#275344=CARTESIAN_POINT('Ctrl Pts',(-8.81886000300005,15.2,-5.49451190900001));
#275345=CARTESIAN_POINT('Ctrl Pts',(-8.81886000300005,11.6,-5.49451190900001));
#275346=CARTESIAN_POINT('Ctrl Pts',(-8.81792317400006,15.2,-5.49405261600001));
#275347=CARTESIAN_POINT('Ctrl Pts',(-8.81792317400006,11.6,-5.49405261600001));
#275348=CARTESIAN_POINT('Ctrl Pts',(-8.81699508900006,15.2,-5.49359646700001));
#275349=CARTESIAN_POINT('Ctrl Pts',(-8.81699508900006,11.6,-5.49359646700001));
#275350=CARTESIAN_POINT('Ctrl Pts',(-8.81607576700006,15.2,-5.49314348900001));
#275351=CARTESIAN_POINT('Ctrl Pts',(-8.81607576700006,11.6,-5.49314348900001));
#275352=CARTESIAN_POINT('Ctrl Pts',(-8.81516521900006,15.2,-5.49269371000001));
#275353=CARTESIAN_POINT('Ctrl Pts',(-8.81516521900006,11.6,-5.49269371000001));
#275354=CARTESIAN_POINT('Ctrl Pts',(-8.81426346300006,15.2,-5.49224715500001));
#275355=CARTESIAN_POINT('Ctrl Pts',(-8.81426346300006,11.6,-5.49224715500001));
#275356=CARTESIAN_POINT('Ctrl Pts',(-8.81337051400006,15.2,-5.49180385500001));
#275357=CARTESIAN_POINT('Ctrl Pts',(-8.81337051400006,11.6,-5.49180385500001));
#275358=CARTESIAN_POINT('Ctrl Pts',(-8.81248638700006,15.2,-5.49136383300001));
#275359=CARTESIAN_POINT('Ctrl Pts',(-8.81248638700006,11.6,-5.49136383300001));
#275360=CARTESIAN_POINT('Ctrl Pts',(-8.81161109900006,15.2,-5.49092711900002));
#275361=CARTESIAN_POINT('Ctrl Pts',(-8.81161109900006,11.6,-5.49092711900002));
#275362=CARTESIAN_POINT('Ctrl Pts',(-8.81074466500005,15.2,-5.49049374100001));
#275363=CARTESIAN_POINT('Ctrl Pts',(-8.81074466500005,11.6,-5.49049374100001));
#275364=CARTESIAN_POINT('Ctrl Pts',(-8.80988709900006,15.2,-5.49006372600001));
#275365=CARTESIAN_POINT('Ctrl Pts',(-8.80988709900006,11.6,-5.49006372600001));
#275366=CARTESIAN_POINT('Ctrl Pts',(-8.80903841900006,15.2,-5.48963710300002));
#275367=CARTESIAN_POINT('Ctrl Pts',(-8.80903841900006,11.6,-5.48963710300002));
#275368=CARTESIAN_POINT('Ctrl Pts',(-8.80819864000006,15.2,-5.48921389900002));
#275369=CARTESIAN_POINT('Ctrl Pts',(-8.80819864000006,11.6,-5.48921389900002));
#275370=CARTESIAN_POINT('Ctrl Pts',(-8.80736777900006,15.2,-5.48879414400002));
#275371=CARTESIAN_POINT('Ctrl Pts',(-8.80736777900006,11.6,-5.48879414400002));
#275372=CARTESIAN_POINT('Ctrl Pts',(-8.80655058300006,15.2,-5.48838026300002));
#275373=CARTESIAN_POINT('Ctrl Pts',(-8.80655058300006,11.6,-5.48838026300002));
#275374=CARTESIAN_POINT('Ctrl Pts',(-8.80590483100006,15.2,-5.48805240200001));
#275375=CARTESIAN_POINT('Ctrl Pts',(-8.80590483100006,11.6,-5.48805240200001));
#275376=CARTESIAN_POINT('Ctrl Pts',(-8.80542564400006,15.2,-5.48780866000001));
#275377=CARTESIAN_POINT('Ctrl Pts',(-8.80542564400006,11.6,-5.48780866000001));
#275378=CARTESIAN_POINT('Ctrl Pts',(-8.80510947800006,15.2,-5.48764764400001));
#275379=CARTESIAN_POINT('Ctrl Pts',(-8.80510947800006,11.6,-5.48764764400001));
#275380=CARTESIAN_POINT('Ctrl Pts',(-8.80495412800006,15.2,-5.48756848000002));
#275381=CARTESIAN_POINT('Ctrl Pts',(-8.80495412800006,11.6,-5.48756848000002));
#275382=CARTESIAN_POINT('',(-8.80495412746579,12.2,-5.48756847941587));
#275383=CARTESIAN_POINT('',(-8.80495412746579,15.2,-5.48756847941587));
#275384=CARTESIAN_POINT('',(-8.80495412700006,12.2,-5.48756847900002));
#275385=CARTESIAN_POINT('Ctrl Pts',(-9.95917514600006,12.2,-5.75020264100001));
#275386=CARTESIAN_POINT('Ctrl Pts',(-9.95409037794778,12.2,-5.74984643423629));
#275387=CARTESIAN_POINT('Ctrl Pts',(-9.94901787496109,12.2,-5.74948339722987));
#275388=CARTESIAN_POINT('Ctrl Pts',(-9.94395764896434,12.2,-5.74911352693123));
#275389=CARTESIAN_POINT('Ctrl Pts',(-9.9401624798115,12.2,-5.74883612423245));
#275390=CARTESIAN_POINT('Ctrl Pts',(-9.93637421526921,12.2,-5.74855488063251));
#275391=CARTESIAN_POINT('Ctrl Pts',(-9.93259287576015,12.2,-5.74826981171152));
#275392=CARTESIAN_POINT('Ctrl Pts',(-9.92881153625109,12.2,-5.74798474279053));
#275393=CARTESIAN_POINT('Ctrl Pts',(-9.92503712276863,12.2,-5.7476958515911));
#275394=CARTESIAN_POINT('Ctrl Pts',(-9.92126966961447,12.2,-5.74740316876808));
#275395=CARTESIAN_POINT('Ctrl Pts',(-9.91750221646032,12.2,-5.74711048594505));
#275396=CARTESIAN_POINT('Ctrl Pts',(-9.91374172529696,12.2,-5.74681401298914));
#275397=CARTESIAN_POINT('Ctrl Pts',(-9.909988229975,12.2,-5.74651378250004));
#275398=CARTESIAN_POINT('Ctrl Pts',(-9.90623473465304,12.2,-5.74621355201095));
#275399=CARTESIAN_POINT('Ctrl Pts',(-9.90248823458913,12.2,-5.74590956273868));
#275400=CARTESIAN_POINT('Ctrl Pts',(-9.89874875768272,12.2,-5.74560183979185));
#275401=CARTESIAN_POINT('Ctrl Pts',(-9.89500928077632,12.2,-5.74529411684502));
#275402=CARTESIAN_POINT('Ctrl Pts',(-9.89127682625575,12.2,-5.74498266149818));
#275403=CARTESIAN_POINT('Ctrl Pts',(-9.88755142274585,12.2,-5.74466749807765));
#275404=CARTESIAN_POINT('Ctrl Pts',(-9.88382601923595,12.2,-5.74435233465712));
#275405=CARTESIAN_POINT('Ctrl Pts',(-9.88010766652519,12.2,-5.74403346444147));
#275406=CARTESIAN_POINT('Ctrl Pts',(-9.87639639528407,12.2,-5.74371091607869));
#275407=CARTESIAN_POINT('Ctrl Pts',(-9.87268512336873,12.2,-5.74338836765731));
#275408=CARTESIAN_POINT('Ctrl Pts',(-9.86898093399704,12.2,-5.7430621426099));
#275409=CARTESIAN_POINT('Ctrl Pts',(-9.86528385746071,12.2,-5.74273226768646));
#275410=CARTESIAN_POINT('Ctrl Pts',(-9.86158678159601,12.2,-5.74240239282295));
#275411=CARTESIAN_POINT('Ctrl Pts',(-9.85789681776428,12.2,-5.74206886966797));
#275412=CARTESIAN_POINT('Ctrl Pts',(-9.85421399685703,12.2,-5.7417317256799));
#275413=CARTESIAN_POINT('Ctrl Pts',(-9.85053117594978,12.2,-5.74139458169183));
#275414=CARTESIAN_POINT('Ctrl Pts',(-9.84685549666336,12.2,-5.74105381605546));
#275415=CARTESIAN_POINT('Ctrl Pts',(-9.84318698982168,12.2,-5.74070945948306));
#275416=CARTESIAN_POINT('Ctrl Pts',(-9.83829564758826,12.2,-5.74025031740737));
#275417=CARTESIAN_POINT('Ctrl Pts',(-9.83341705508244,12.2,-5.73978478939629));
#275418=CARTESIAN_POINT('Ctrl Pts',(-9.82855128681223,12.2,-5.73931294360218));
#275419=CARTESIAN_POINT('Ctrl Pts',(-9.82490195978086,12.2,-5.73895905917623));
#275420=CARTESIAN_POINT('Ctrl Pts',(-9.82125984466824,12.2,-5.73860162195762));
#275421=CARTESIAN_POINT('Ctrl Pts',(-9.81762497368261,12.2,-5.73824066144635));
#275422=CARTESIAN_POINT('Ctrl Pts',(-9.81399010335732,12.2,-5.73787970100065));
#275423=CARTESIAN_POINT('Ctrl Pts',(-9.81036247660667,12.2,-5.73751521608014));
#275424=CARTESIAN_POINT('Ctrl Pts',(-9.80674212286384,12.2,-5.73714723713487));
#275425=CARTESIAN_POINT('Ctrl Pts',(-9.80312176912101,12.2,-5.73677925818961));
#275426=CARTESIAN_POINT('Ctrl Pts',(-9.79950868946539,12.2,-5.73640778523779));
#275427=CARTESIAN_POINT('Ctrl Pts',(-9.79590291370507,12.2,-5.73603284729136));
#275428=CARTESIAN_POINT('Ctrl Pts',(-9.79229713794475,12.2,-5.73565790934494));
#275429=CARTESIAN_POINT('Ctrl Pts',(-9.7886986668058,12.2,-5.7352795069549));
#275430=CARTESIAN_POINT('Ctrl Pts',(-9.78510753050327,12.2,-5.73489767050872));
#275431=CARTESIAN_POINT('Ctrl Pts',(-9.78151639420074,12.2,-5.73451583406254));
#275432=CARTESIAN_POINT('Ctrl Pts',(-9.77793259291067,12.2,-5.7341305624446));
#275433=CARTESIAN_POINT('Ctrl Pts',(-9.77435615712329,12.2,-5.73374188700068));
#275434=CARTESIAN_POINT('Ctrl Pts',(-9.76958757564029,12.2,-5.73322365302838));
#275435=CARTESIAN_POINT('Ctrl Pts',(-9.76483208952837,12.2,-5.73269936735814));
#275436=CARTESIAN_POINT('Ctrl Pts',(-9.76008977010411,12.2,-5.73216910143996));
#275437=CARTESIAN_POINT('Ctrl Pts',(-9.75653303085899,12.2,-5.73177140203746));
#275438=CARTESIAN_POINT('Ctrl Pts',(-9.75298369860466,12.2,-5.73137033946868));
#275439=CARTESIAN_POINT('Ctrl Pts',(-9.74944180473333,12.2,-5.73096594406671));
#275440=CARTESIAN_POINT('Ctrl Pts',(-9.745899910862,12.2,-5.73056154866473));
#275441=CARTESIAN_POINT('Ctrl Pts',(-9.74236545397374,12.2,-5.73015382064624));
#275442=CARTESIAN_POINT('Ctrl Pts',(-9.73883846614291,12.2,-5.72974279078645));
#275443=CARTESIAN_POINT('Ctrl Pts',(-9.73531147831207,12.2,-5.72933176092667));
#275444=CARTESIAN_POINT('Ctrl Pts',(-9.73179195946162,12.2,-5.72891742980278));
#275445=CARTESIAN_POINT('Ctrl Pts',(-9.72827994045456,12.2,-5.72849982783914));
#275446=CARTESIAN_POINT('Ctrl Pts',(-9.72476792144751,12.2,-5.72808222587549));
#275447=CARTESIAN_POINT('Ctrl Pts',(-9.72126340215299,12.2,-5.72766135264331));
#275448=CARTESIAN_POINT('Ctrl Pts',(-9.71776641477902,12.2,-5.72723724211749));
#275449=CARTESIAN_POINT('Ctrl Pts',(-9.71426942676977,12.2,-5.72681313151463));
#275450=CARTESIAN_POINT('Ctrl Pts',(-9.71077996901264,12.2,-5.72638578120253));
#275451=CARTESIAN_POINT('Ctrl Pts',(-9.70729807450762,12.2,-5.72595522418117));
#275452=CARTESIAN_POINT('Ctrl Pts',(-9.70381618063515,12.2,-5.72552466723804));
#275453=CARTESIAN_POINT('Ctrl Pts',(-9.70034184847897,12.2,-5.72509090265343));
#275454=CARTESIAN_POINT('Ctrl Pts',(-9.69687511114725,12.2,-5.72465396371069));
#275455=CARTESIAN_POINT('Ctrl Pts',(-9.69340837381553,12.2,-5.72421702476795));
#275456=CARTESIAN_POINT('Ctrl Pts',(-9.68994923005378,12.2,-5.72377691043556));
#275457=CARTESIAN_POINT('Ctrl Pts',(-9.68649771220521,12.2,-5.72333365403297));
#275458=CARTESIAN_POINT('Ctrl Pts',(-9.68304619435663,12.2,-5.72289039763038));
#275459=CARTESIAN_POINT('Ctrl Pts',(-9.67960230117726,12.2,-5.72244399855281));
#275460=CARTESIAN_POINT('Ctrl Pts',(-9.67616606624479,12.2,-5.72199448873378));
#275461=CARTESIAN_POINT('Ctrl Pts',(-9.67272983131232,12.2,-5.72154497891475));
#275462=CARTESIAN_POINT('Ctrl Pts',(-9.66930125221604,12.2,-5.7210923596995));
#275463=CARTESIAN_POINT('Ctrl Pts',(-9.66588036288134,12.2,-5.72063666284132));
#275464=CARTESIAN_POINT('Ctrl Pts',(-9.66245947354664,12.2,-5.72018096598314));
#275465=CARTESIAN_POINT('Ctrl Pts',(-9.65904627296974,12.2,-5.71972219145018));
#275466=CARTESIAN_POINT('Ctrl Pts',(-9.6556407927174,12.2,-5.71926037305071));
#275467=CARTESIAN_POINT('Ctrl Pts',(-9.65223531184641,12.2,-5.71879855456734));
#275468=CARTESIAN_POINT('Ctrl Pts',(-9.64883755221928,12.2,-5.71833369164978));
#275469=CARTESIAN_POINT('Ctrl Pts',(-9.64544754526932,12.2,-5.71786581770637));
#275470=CARTESIAN_POINT('Ctrl Pts',(-9.64205753893523,12.2,-5.71739794384796));
#275471=CARTESIAN_POINT('Ctrl Pts',(-9.63867528399229,12.2,-5.71692705929846));
#275472=CARTESIAN_POINT('Ctrl Pts',(-9.63530081407221,12.2,-5.71645319787499));
#275473=CARTESIAN_POINT('Ctrl Pts',(-9.63192634415214,12.2,-5.71597933645153));
#275474=CARTESIAN_POINT('Ctrl Pts',(-9.62855965989462,12.2,-5.71550249684718));
#275475=CARTESIAN_POINT('Ctrl Pts',(-9.62520079160068,12.2,-5.71502271444769));
#275476=CARTESIAN_POINT('Ctrl Pts',(-9.62184192330675,12.2,-5.7145429320482));
#275477=CARTESIAN_POINT('Ctrl Pts',(-9.61849087136186,12.2,-5.71406020668239));
#275478=CARTESIAN_POINT('Ctrl Pts',(-9.615147669025,12.2,-5.71357457178337));
#275479=CARTESIAN_POINT('Ctrl Pts',(-9.61180446668813,12.2,-5.71308893688435));
#275480=CARTESIAN_POINT('Ctrl Pts',(-9.60846911280929,12.2,-5.71260039226878));
#275481=CARTESIAN_POINT('Ctrl Pts',(-9.60514164009616,12.2,-5.71210897337022));
#275482=CARTESIAN_POINT('Ctrl Pts',(-9.60181416738304,12.2,-5.71161755447166));
#275483=CARTESIAN_POINT('Ctrl Pts',(-9.59849457728684,12.2,-5.71112326023597));
#275484=CARTESIAN_POINT('Ctrl Pts',(-9.59518289940747,12.2,-5.71062612639619));
#275485=CARTESIAN_POINT('Ctrl Pts',(-9.5918712215281,12.2,-5.71012899255641));
#275486=CARTESIAN_POINT('Ctrl Pts',(-9.5885674572665,12.2,-5.70962901887432));
#275487=CARTESIAN_POINT('Ctrl Pts',(-9.58527164042683,12.2,-5.70912623960131));
#275488=CARTESIAN_POINT('Ctrl Pts',(-9.58087721757477,12.2,-5.70845586717639));
#275489=CARTESIAN_POINT('Ctrl Pts',(-9.57649691992405,12.2,-5.70778050829822));
#275490=CARTESIAN_POINT('Ctrl Pts',(-9.57213082774167,12.2,-5.70710024648337));
#275491=CARTESIAN_POINT('Ctrl Pts',(-9.56776473555929,12.2,-5.70641998466852));
#275492=CARTESIAN_POINT('Ctrl Pts',(-9.56341284680075,12.2,-5.70573481985865));
#275493=CARTESIAN_POINT('Ctrl Pts',(-9.55907524006581,12.2,-5.70504483615388));
#275494=CARTESIAN_POINT('Ctrl Pts',(-9.55256883055439,12.2,-5.70400986069076));
#275495=CARTESIAN_POINT('Ctrl Pts',(-9.54609455572192,12.2,-5.70296404560449));
#275496=CARTESIAN_POINT('Ctrl Pts',(-9.53965267920738,12.2,-5.70190767697575));
#275497=CARTESIAN_POINT('Ctrl Pts',(-9.5353580950594,12.2,-5.70120343125523));
#275498=CARTESIAN_POINT('Ctrl Pts',(-9.53107790966964,12.2,-5.70049449661066));
#275499=CARTESIAN_POINT('Ctrl Pts',(-9.52681220340578,12.2,-5.69978095839169));
#275500=CARTESIAN_POINT('Ctrl Pts',(-9.52254649656072,12.2,-5.6990674200755));
#275501=CARTESIAN_POINT('Ctrl Pts',(-9.51829526704999,12.2,-5.69834928007278));
#275502=CARTESIAN_POINT('Ctrl Pts',(-9.51405859552212,12.2,-5.69762662497454));
#275503=CARTESIAN_POINT('Ctrl Pts',(-9.5098219245715,12.2,-5.69690396997476));
#275504=CARTESIAN_POINT('Ctrl Pts',(-9.50559980981213,12.2,-5.69617680117049));
#275505=CARTESIAN_POINT('Ctrl Pts',(-9.50139233115459,12.2,-5.69544520611965));
#275506=CARTESIAN_POINT('Ctrl Pts',(-9.4971848519238,12.2,-5.69471361096912));
#275507=CARTESIAN_POINT('Ctrl Pts',(-9.49299201074995,12.2,-5.69397758987372));
#275508=CARTESIAN_POINT('Ctrl Pts',(-9.48881388596666,12.2,-5.69323723350003));
#275509=CARTESIAN_POINT('Ctrl Pts',(-9.48463576118336,12.2,-5.69249687712634));
#275510=CARTESIAN_POINT('Ctrl Pts',(-9.48047235300741,12.2,-5.69175218570216));
#275511=CARTESIAN_POINT('Ctrl Pts',(-9.47632374033838,12.2,-5.69100324866091));
#275512=CARTESIAN_POINT('Ctrl Pts',(-9.47217512823461,12.2,-5.6902543117217));
#275513=CARTESIAN_POINT('Ctrl Pts',(-9.46804131249317,12.2,-5.68950113035317));
#275514=CARTESIAN_POINT('Ctrl Pts',(-9.46392237497781,12.2,-5.68874379730055));
#275515=CARTESIAN_POINT('Ctrl Pts',(-9.45980343690124,12.2,-5.68798646414473));
#275516=CARTESIAN_POINT('Ctrl Pts',(-9.45569937597219,12.2,-5.68722497653366));
#275517=CARTESIAN_POINT('Ctrl Pts',(-9.45161027380643,12.2,-5.6864594301582));
#275518=CARTESIAN_POINT('Ctrl Pts',(-9.44752117219781,12.2,-5.68569388388704));
#275519=CARTESIAN_POINT('Ctrl Pts',(-9.44344702710667,12.2,-5.68492427853029));
#275520=CARTESIAN_POINT('Ctrl Pts',(-9.43938792354864,12.2,-5.68415070753823));
#275521=CARTESIAN_POINT('Ctrl Pts',(-9.43329926793507,12.2,-5.68299035099745));
#275522=CARTESIAN_POINT('Ctrl Pts',(-9.42724444977319,12.2,-5.68182107141003));
#275523=CARTESIAN_POINT('Ctrl Pts',(-9.42122374915626,12.2,-5.68064319187008));
#275524=CARTESIAN_POINT('Ctrl Pts',(-9.41720994838038,12.2,-5.67985793877212));
#275525=CARTESIAN_POINT('Ctrl Pts',(-9.41321130928653,12.2,-5.67906886372935));
#275526=CARTESIAN_POINT('Ctrl Pts',(-9.40922791645832,12.2,-5.6782760627417));
#275527=CARTESIAN_POINT('Ctrl Pts',(-9.40524452363011,12.2,-5.67748326175405));
#275528=CARTESIAN_POINT('Ctrl Pts',(-9.4012763745148,12.2,-5.67668673501318));
#275529=CARTESIAN_POINT('Ctrl Pts',(-9.39732355457872,12.2,-5.67588658130254));
#275530=CARTESIAN_POINT('Ctrl Pts',(-9.39337073518123,12.2,-5.67508642770091));
#275531=CARTESIAN_POINT('Ctrl Pts',(-9.38943324447615,12.2,-5.67428264574698));
#275532=CARTESIAN_POINT('Ctrl Pts',(-9.38551116429577,12.2,-5.67347533675766));
#275533=CARTESIAN_POINT('Ctrl Pts',(-9.38158908358101,12.2,-5.67266802765834));
#275534=CARTESIAN_POINT('Ctrl Pts',(-9.37768241456836,12.2,-5.67185718898666));
#275535=CARTESIAN_POINT('Ctrl Pts',(-9.37379124038544,12.2,-5.67104292262352));
#275536=CARTESIAN_POINT('Ctrl Pts',(-9.36892727292189,12.2,-5.67002508972507));
#275537=CARTESIAN_POINT('Ctrl Pts',(-9.36408751697371,12.2,-5.66900190092705));
#275538=CARTESIAN_POINT('Ctrl Pts',(-9.35927213787848,12.2,-5.66797355314885));
#275539=CARTESIAN_POINT('Ctrl Pts',(-9.35541983491722,12.2,-5.66715087499355));
#275540=CARTESIAN_POINT('Ctrl Pts',(-9.35158313178172,12.2,-5.66632489584701));
#275541=CARTESIAN_POINT('Ctrl Pts',(-9.34776211437084,12.2,-5.66549571885945));
#275542=CARTESIAN_POINT('Ctrl Pts',(-9.34394109643936,12.2,-5.66466654175891));
#275543=CARTESIAN_POINT('Ctrl Pts',(-9.34013576407524,12.2,-5.66383416589132));
#275544=CARTESIAN_POINT('Ctrl Pts',(-9.33634620195853,12.2,-5.66299869563711));
#275545=CARTESIAN_POINT('Ctrl Pts',(-9.33255664035815,12.2,-5.66216322549674));
#275546=CARTESIAN_POINT('Ctrl Pts',(-9.32878285161785,12.2,-5.66132466031647));
#275547=CARTESIAN_POINT('Ctrl Pts',(-9.32502491759068,12.2,-5.66048310805213));
#275548=CARTESIAN_POINT('Ctrl Pts',(-9.3212669830515,12.2,-5.65964155567312));
#275549=CARTESIAN_POINT('Ctrl Pts',(-9.31752490530313,12.2,-5.65879701334654));
#275550=CARTESIAN_POINT('Ctrl Pts',(-9.3137987712122,12.2,-5.65794958968906));
#275551=CARTESIAN_POINT('Ctrl Pts',(-9.31007263762896,12.2,-5.65710216614704));
#275552=CARTESIAN_POINT('Ctrl Pts',(-9.30636244611732,12.2,-5.65625185991588));
#275553=CARTESIAN_POINT('Ctrl Pts',(-9.30266828451113,12.2,-5.65539878033213));
#275554=CARTESIAN_POINT('Ctrl Pts',(-9.29897412240161,12.2,-5.65454570063215));
#275555=CARTESIAN_POINT('Ctrl Pts',(-9.2952959901743,12.2,-5.65368984571845));
#275556=CARTESIAN_POINT('Ctrl Pts',(-9.29163397547577,12.2,-5.65283132617148));
#275557=CARTESIAN_POINT('Ctrl Pts',(-9.2879719612762,12.2,-5.65197280674148));
#275558=CARTESIAN_POINT('Ctrl Pts',(-9.28432606282339,12.2,-5.65111162334815));
#275559=CARTESIAN_POINT('Ctrl Pts',(-9.28069637061846,12.2,-5.65024788464124));
#275560=CARTESIAN_POINT('Ctrl Pts',(-9.27706667791898,12.2,-5.64938414581665));
#275561=CARTESIAN_POINT('Ctrl Pts',(-9.273453189371,12.2,-5.64851785205074));
#275562=CARTESIAN_POINT('Ctrl Pts',(-9.26985599471421,12.2,-5.64764911699943));
#275563=CARTESIAN_POINT('Ctrl Pts',(-9.26625880054753,12.2,-5.64678038206649));
#275564=CARTESIAN_POINT('Ctrl Pts',(-9.26267789834029,12.2,-5.64590920418508));
#275565=CARTESIAN_POINT('Ctrl Pts',(-9.25911337957447,12.2,-5.64503569686784));
#275566=CARTESIAN_POINT('Ctrl Pts',(-9.25554886032297,12.2,-5.64416218943158));
#275567=CARTESIAN_POINT('Ctrl Pts',(-9.25200072389246,12.2,-5.64328635198677));
#275568=CARTESIAN_POINT('Ctrl Pts',(-9.24846905803332,12.2,-5.64240830105002));
#275569=CARTESIAN_POINT('Ctrl Pts',(-9.24493739217417,12.2,-5.64153025011328));
#275570=CARTESIAN_POINT('Ctrl Pts',(-9.24142219814474,12.2,-5.64064998448184));
#275571=CARTESIAN_POINT('Ctrl Pts',(-9.23792356617797,12.2,-5.63976762032242));
#275572=CARTESIAN_POINT('Ctrl Pts',(-9.23442493468789,12.2,-5.63888525628323));
#275573=CARTESIAN_POINT('Ctrl Pts',(-9.23094286375706,12.2,-5.6380007941294));
#275574=CARTESIAN_POINT('Ctrl Pts',(-9.22747744680235,12.2,-5.63711435080896));
#275575=CARTESIAN_POINT('Ctrl Pts',(-9.22401202937549,12.2,-5.63622790736773));
#275576=CARTESIAN_POINT('Ctrl Pts',(-9.22056326270751,12.2,-5.63533948328094));
#275577=CARTESIAN_POINT('Ctrl Pts',(-9.21713124018886,12.2,-5.63444919712112));
#275578=CARTESIAN_POINT('Ctrl Pts',(-9.21369921813782,12.2,-5.63355891108261));
#275579=CARTESIAN_POINT('Ctrl Pts',(-9.2102839409179,12.2,-5.63266676329989));
#275580=CARTESIAN_POINT('Ctrl Pts',(-9.20688549752797,12.2,-5.63177287403975));
#275581=CARTESIAN_POINT('Ctrl Pts',(-9.20348705367501,12.2,-5.63087898465782));
#275582=CARTESIAN_POINT('Ctrl Pts',(-9.20010544519518,12.2,-5.62998335421368));
#275583=CARTESIAN_POINT('Ctrl Pts',(-9.19674076451184,12.2,-5.62908610411981));
#275584=CARTESIAN_POINT('Ctrl Pts',(-9.19337608428694,12.2,-5.6281888541482));
#275585=CARTESIAN_POINT('Ctrl Pts',(-9.19002833246516,12.2,-5.62728998641658));
#275586=CARTESIAN_POINT('Ctrl Pts',(-9.1866976010141,12.2,-5.62638962182361));
#275587=CARTESIAN_POINT('Ctrl Pts',(-9.18336686910923,12.2,-5.62548925710797));
#275588=CARTESIAN_POINT('Ctrl Pts',(-9.18005315646755,12.2,-5.62458739670882));
#275589=CARTESIAN_POINT('Ctrl Pts',(-9.17675656045565,12.2,-5.6236841666595));
#275590=CARTESIAN_POINT('Ctrl Pts',(-9.17345996489292,12.2,-5.62278093673325));
#275591=CARTESIAN_POINT('Ctrl Pts',(-9.17018048252125,12.2,-5.62187633587755));
#275592=CARTESIAN_POINT('Ctrl Pts',(-9.16691820895679,12.2,-5.62097049240645));
#275593=CARTESIAN_POINT('Ctrl Pts',(-9.16365593494787,12.2,-5.62006464881194));
#275594=CARTESIAN_POINT('Ctrl Pts',(-9.16041086977495,12.2,-5.61915756073922));
#275595=CARTESIAN_POINT('Ctrl Pts',(-9.15718310854462,12.2,-5.6182493586341));
#275596=CARTESIAN_POINT('Ctrl Pts',(-9.15395534775407,12.2,-5.61734115665272));
#275597=CARTESIAN_POINT('Ctrl Pts',(-9.15074489128502,12.2,-5.61643183876044));
#275598=CARTESIAN_POINT('Ctrl Pts',(-9.14755183332206,12.2,-5.61552153689052));
#275599=CARTESIAN_POINT('Ctrl Pts',(-9.14356051054207,12.2,-5.61438365946009));
#275600=CARTESIAN_POINT('Ctrl Pts',(-9.13959637408344,12.2,-5.61324424281155));
#275601=CARTESIAN_POINT('Ctrl Pts',(-9.13565961339875,12.2,-5.61210354615743));
#275602=CARTESIAN_POINT('Ctrl Pts',(-9.13172285271406,12.2,-5.6109628495033));
#275603=CARTESIAN_POINT('Ctrl Pts',(-9.12781346627214,12.2,-5.6098208716136));
#275604=CARTESIAN_POINT('Ctrl Pts',(-9.12393164502069,12.2,-5.60867787584976));
#275605=CARTESIAN_POINT('Ctrl Pts',(-9.12004982376924,12.2,-5.60753488008593));
#275606=CARTESIAN_POINT('Ctrl Pts',(-9.11619556795187,12.2,-5.60639086647484));
#275607=CARTESIAN_POINT('Ctrl Pts',(-9.11236906774208,12.2,-5.60524610084988));
#275608=CARTESIAN_POINT('Ctrl Pts',(-9.1085425675323,12.2,-5.60410133522491));
#275609=CARTESIAN_POINT('Ctrl Pts',(-9.10474382473154,12.2,-5.60295581854716));
#275610=CARTESIAN_POINT('Ctrl Pts',(-9.10097303348009,12.2,-5.60180982132496));
#275611=CARTESIAN_POINT('Ctrl Pts',(-9.09720224222865,12.2,-5.60066382410277));
#275612=CARTESIAN_POINT('Ctrl Pts',(-9.09345939989119,12.2,-5.59951734792806));
#275613=CARTESIAN_POINT('Ctrl Pts',(-9.08974470452701,12.2,-5.59837066653397));
#275614=CARTESIAN_POINT('Ctrl Pts',(-9.08603000916283,12.2,-5.59722398513988));
#275615=CARTESIAN_POINT('Ctrl Pts',(-9.08234346030553,12.2,-5.59607709923335));
#275616=CARTESIAN_POINT('Ctrl Pts',(-9.07868525495831,12.2,-5.59493029173335));
#275617=CARTESIAN_POINT('Ctrl Pts',(-9.07502704961108,12.2,-5.59378348423334));
#275618=CARTESIAN_POINT('Ctrl Pts',(-9.07139718858651,12.2,-5.59263675178237));
#275619=CARTESIAN_POINT('Ctrl Pts',(-9.06779587072302,12.2,-5.59149038274939));
#275620=CARTESIAN_POINT('Ctrl Pts',(-9.06419455285953,12.2,-5.59034401371641));
#275621=CARTESIAN_POINT('Ctrl Pts',(-9.06062177702242,12.2,-5.58919800558618));
#275622=CARTESIAN_POINT('Ctrl Pts',(-9.05707774751005,12.2,-5.58805265239178));
#275623=CARTESIAN_POINT('Ctrl Pts',(-9.05353371799768,12.2,-5.58690729919738));
#275624=CARTESIAN_POINT('Ctrl Pts',(-9.05001843272618,12.2,-5.58576259785294));
#275625=CARTESIAN_POINT('Ctrl Pts',(-9.04653209654715,12.2,-5.58461884570022));
#275626=CARTESIAN_POINT('Ctrl Pts',(-9.04304576036813,12.2,-5.5834750935475));
#275627=CARTESIAN_POINT('Ctrl Pts',(-9.03958837427692,12.2,-5.58233229076888));
#275628=CARTESIAN_POINT('Ctrl Pts',(-9.03616014063545,12.2,-5.58119073710083));
#275629=CARTESIAN_POINT('Ctrl Pts',(-9.03273190699398,12.2,-5.58004918343277));
#275630=CARTESIAN_POINT('Ctrl Pts',(-9.02933282980129,12.2,-5.57890888160094));
#275631=CARTESIAN_POINT('Ctrl Pts',(-9.0259631145259,12.2,-5.57777013535106));
#275632=CARTESIAN_POINT('Ctrl Pts',(-9.02259339925052,12.2,-5.57663138910119));
#275633=CARTESIAN_POINT('Ctrl Pts',(-9.01925304713674,12.2,-5.57549420050135));
#275634=CARTESIAN_POINT('Ctrl Pts',(-9.0159422678336,12.2,-5.57435888008484));
#275635=CARTESIAN_POINT('Ctrl Pts',(-9.01263148889134,12.2,-5.57322355979209));
#275636=CARTESIAN_POINT('Ctrl Pts',(-9.00935028375105,12.2,-5.57209010840261));
#275637=CARTESIAN_POINT('Ctrl Pts',(-9.0060988646586,12.2,-5.57095884262298));
#275638=CARTESIAN_POINT('Ctrl Pts',(-9.00284744521174,12.2,-5.56982757672003));
#275639=CARTESIAN_POINT('Ctrl Pts',(-8.99962581084212,12.2,-5.5686984999809));
#275640=CARTESIAN_POINT('Ctrl Pts',(-8.99643417965913,12.2,-5.56757193289736));
#275641=CARTESIAN_POINT('Ctrl Pts',(-8.99324254847613,12.2,-5.56644536581384));
#275642=CARTESIAN_POINT('Ctrl Pts',(-8.99008091774436,12.2,-5.56532130925861));
#275643=CARTESIAN_POINT('Ctrl Pts',(-8.9869495066136,12.2,-5.56420009385517));
#275644=CARTESIAN_POINT('Ctrl Pts',(-8.98319181305189,12.2,-5.56285463529771));
#275645=CARTESIAN_POINT('Ctrl Pts',(-8.97947763719697,12.2,-5.56151326617684));
#275646=CARTESIAN_POINT('Ctrl Pts',(-8.97580735783326,12.2,-5.56017657160431));
#275647=CARTESIAN_POINT('Ctrl Pts',(-8.97213707880293,12.2,-5.55883987715319));
#275648=CARTESIAN_POINT('Ctrl Pts',(-8.9685106971594,12.2,-5.55750785349889));
#275649=CARTESIAN_POINT('Ctrl Pts',(-8.96492860102335,12.2,-5.55618109929107));
#275650=CARTESIAN_POINT('Ctrl Pts',(-8.96134650488731,12.2,-5.55485434508325));
#275651=CARTESIAN_POINT('Ctrl Pts',(-8.95780869174889,12.2,-5.55353285835752));
#275652=CARTESIAN_POINT('Ctrl Pts',(-8.95431555770721,12.2,-5.55221725107173));
#275653=CARTESIAN_POINT('Ctrl Pts',(-8.95082242334824,12.2,-5.55090164366644));
#275654=CARTESIAN_POINT('Ctrl Pts',(-8.94737396721143,12.2,-5.54959191300355));
#275655=CARTESIAN_POINT('Ctrl Pts',(-8.94397058786236,12.2,-5.54828868584962));
#275656=CARTESIAN_POINT('Ctrl Pts',(-8.94056720882241,12.2,-5.54698545881408));
#275657=CARTESIAN_POINT('Ctrl Pts',(-8.93720890657228,12.2,-5.54568873347425));
#275658=CARTESIAN_POINT('Ctrl Pts',(-8.93389608761129,12.2,-5.54439915043808));
#275659=CARTESIAN_POINT('Ctrl Pts',(-8.9305832686503,12.2,-5.54310956740191));
#275660=CARTESIAN_POINT('Ctrl Pts',(-8.92731593080235,12.2,-5.54182712500687));
#275661=CARTESIAN_POINT('Ctrl Pts',(-8.92409449066741,12.2,-5.54055248005283));
#275662=CARTESIAN_POINT('Ctrl Pts',(-8.92087305053247,12.2,-5.53927783509881));
#275663=CARTESIAN_POINT('Ctrl Pts',(-8.9176975042139,12.2,-5.5380109859087));
#275664=CARTESIAN_POINT('Ctrl Pts',(-8.91456827232441,12.2,-5.5367526051205));
#275665=CARTESIAN_POINT('Ctrl Pts',(-8.91143904015069,12.2,-5.53549422421799));
#275666=CARTESIAN_POINT('Ctrl Pts',(-8.90835612418982,12.2,-5.53424431125798));
#275667=CARTESIAN_POINT('Ctrl Pts',(-8.90531994710969,12.2,-5.53300355444075));
#275668=CARTESIAN_POINT('Ctrl Pts',(-8.90228377030535,12.2,-5.53176279773622));
#275669=CARTESIAN_POINT('Ctrl Pts',(-8.89929433564735,12.2,-5.53053119599766));
#275670=CARTESIAN_POINT('Ctrl Pts',(-8.89635207566886,12.2,-5.52930945629162));
#275671=CARTESIAN_POINT('Ctrl Pts',(-8.89340981569037,12.2,-5.52808771658559));
#275672=CARTESIAN_POINT('Ctrl Pts',(-8.89051473087686,12.2,-5.52687583798803));
#275673=CARTESIAN_POINT('Ctrl Pts',(-8.88766726131037,12.2,-5.52567454636428));
#275674=CARTESIAN_POINT('Ctrl Pts',(-8.88481979148523,12.2,-5.5244732546314));
#275675=CARTESIAN_POINT('Ctrl Pts',(-8.88201994158144,12.2,-5.52328254665789));
#275676=CARTESIAN_POINT('Ctrl Pts',(-8.87926815660021,12.2,-5.52210316717744));
#275677=CARTESIAN_POINT('Ctrl Pts',(-8.87651637186895,12.2,-5.52092378780412));
#275678=CARTESIAN_POINT('Ctrl Pts',(-8.87381265496687,12.2,-5.51975573906379));
#275679=CARTESIAN_POINT('Ctrl Pts',(-8.87115746421785,12.2,-5.51859977976719));
#275680=CARTESIAN_POINT('Ctrl Pts',(-8.86850227346883,12.2,-5.51744382047058));
#275681=CARTESIAN_POINT('Ctrl Pts',(-8.86589560838085,12.2,-5.51629995355806));
#275682=CARTESIAN_POINT('Ctrl Pts',(-8.86333793755377,12.2,-5.51516896118161));
#275683=CARTESIAN_POINT('Ctrl Pts',(-8.86078026649437,12.2,-5.51403796870243));
#275684=CARTESIAN_POINT('Ctrl Pts',(-8.8582715898829,12.2,-5.51291984943276));
#275685=CARTESIAN_POINT('Ctrl Pts',(-8.85581238379553,12.2,-5.51181541290152));
#275686=CARTESIAN_POINT('Ctrl Pts',(-8.85335317793155,12.2,-5.51071097647061));
#275687=CARTESIAN_POINT('Ctrl Pts',(-8.85094344409755,12.2,-5.50962021750255));
#275688=CARTESIAN_POINT('Ctrl Pts',(-8.84858366851663,12.2,-5.50854396829165));
#275689=CARTESIAN_POINT('Ctrl Pts',(-8.8462238929357,12.2,-5.50746771908076));
#275690=CARTESIAN_POINT('Ctrl Pts',(-8.84391407709403,12.2,-5.50640597620805));
#275691=CARTESIAN_POINT('Ctrl Pts',(-8.84165471647699,12.2,-5.50535959410958));
#275692=CARTESIAN_POINT('Ctrl Pts',(-8.83939535565472,12.2,-5.50431321191606));
#275693=CARTESIAN_POINT('Ctrl Pts',(-8.83718645120391,12.2,-5.50328218836858));
#275694=CARTESIAN_POINT('Ctrl Pts',(-8.83502851250643,12.2,-5.50226740039771));
#275695=CARTESIAN_POINT('Ctrl Pts',(-8.83287057400498,12.2,-5.50125261251901));
#275696=CARTESIAN_POINT('Ctrl Pts',(-8.83076360063357,12.2,-5.50025405960163));
#275697=CARTESIAN_POINT('Ctrl Pts',(-8.82870811303237,12.2,-5.49927264479954));
#275698=CARTESIAN_POINT('Ctrl Pts',(-8.82665262543117,12.2,-5.49829122999746));
#275699=CARTESIAN_POINT('Ctrl Pts',(-8.82464862187126,12.2,-5.49732695060138));
#275700=CARTESIAN_POINT('Ctrl Pts',(-8.82269663660656,12.2,-5.49638073980162));
#275701=CARTESIAN_POINT('Ctrl Pts',(-8.82074465116457,12.2,-5.49543452891593));
#275702=CARTESIAN_POINT('Ctrl Pts',(-8.81884468407904,12.2,-5.49450638212414));
#275703=CARTESIAN_POINT('Ctrl Pts',(-8.81699727948194,12.2,-5.49359725965922));
#275704=CARTESIAN_POINT('Ctrl Pts',(-8.81514987505265,12.2,-5.49268813727688));
#275705=CARTESIAN_POINT('Ctrl Pts',(-8.81335503191469,12.2,-5.4917980403285));
#275706=CARTESIAN_POINT('Ctrl Pts',(-8.81161331239693,12.2,-5.49092795294431));
#275707=CARTESIAN_POINT('Ctrl Pts',(-8.80929937863631,12.2,-5.48977201219011));
#275708=CARTESIAN_POINT('Ctrl Pts',(-8.80707920106142,12.2,-5.48865138494897));
#275709=CARTESIAN_POINT('Ctrl Pts',(-8.80495412800006,12.2,-5.48756848000002));
#275710=CARTESIAN_POINT('Ctrl Pts',(-8.80495412800006,15.2,-5.48756848000002));
#275711=CARTESIAN_POINT('Ctrl Pts',(-8.80654601357685,15.2,-5.48837968070677));
#275712=CARTESIAN_POINT('Ctrl Pts',(-8.80819126582659,15.2,-5.48921205180374));
#275713=CARTESIAN_POINT('Ctrl Pts',(-8.809889320289,15.2,-5.49006457388994));
#275714=CARTESIAN_POINT('Ctrl Pts',(-8.81159556362836,15.2,-5.49092120726858));
#275715=CARTESIAN_POINT('Ctrl Pts',(-8.81335511570803,15.2,-5.49179818670865));
#275716=CARTESIAN_POINT('Ctrl Pts',(-8.81516741715041,15.2,-5.49269451613673));
#275717=CARTESIAN_POINT('Ctrl Pts',(-8.81697971842817,15.2,-5.49359084548341));
#275718=CARTESIAN_POINT('Ctrl Pts',(-8.81884476611964,15.2,-5.49450652398393));
#275719=CARTESIAN_POINT('Ctrl Pts',(-8.82076201154996,15.2,-5.49544058544998));
#275720=CARTESIAN_POINT('Ctrl Pts',(-8.82267925698027,15.2,-5.49637464691604));
#275721=CARTESIAN_POINT('Ctrl Pts',(-8.824648700705,15.2,-5.49732708982732));
#275722=CARTESIAN_POINT('Ctrl Pts',(-8.82666980631291,15.2,-5.49829697667287));
#275723=CARTESIAN_POINT('Ctrl Pts',(-8.8286909121044,15.2,-5.49926686360652));
#275724=CARTESIAN_POINT('Ctrl Pts',(-8.8307636790539,15.2,-5.50025419422024));
#275725=CARTESIAN_POINT('Ctrl Pts',(-8.83288758275648,15.2,-5.50125805810941));
#275726=CARTESIAN_POINT('Ctrl Pts',(-8.83501148626615,15.2,-5.5022619219074));
#275727=CARTESIAN_POINT('Ctrl Pts',(-8.83718652676331,15.2,-5.5032823192667));
#275728=CARTESIAN_POINT('Ctrl Pts',(-8.83941219327598,15.2,-5.50431836423379));
#275729=CARTESIAN_POINT('Ctrl Pts',(-8.84163785978865,15.2,-5.50535440920089));
#275730=CARTESIAN_POINT('Ctrl Pts',(-8.84391415062677,15.2,-5.50640610420631));
#275731=CARTESIAN_POINT('Ctrl Pts',(-8.84624056437339,15.2,-5.50747258641693));
#275732=CARTESIAN_POINT('Ctrl Pts',(-8.84856697833133,15.2,-5.50853906872442));
#275733=CARTESIAN_POINT('Ctrl Pts',(-8.85094351562051,15.2,-5.50962034055873));
#275734=CARTESIAN_POINT('Ctrl Pts',(-8.85336968650611,15.2,-5.51071556661937));
#275735=CARTESIAN_POINT('Ctrl Pts',(-8.85579585717132,15.2,-5.51181079258052));
#275736=CARTESIAN_POINT('Ctrl Pts',(-8.85827166062738,15.2,-5.51291996937641));
#275737=CARTESIAN_POINT('Ctrl Pts',(-8.86079661537112,15.2,-5.51404228958621));
#275738=CARTESIAN_POINT('Ctrl Pts',(-8.86332157011486,15.2,-5.51516460979602));
#275739=CARTESIAN_POINT('Ctrl Pts',(-8.86589567860466,15.2,-5.51630007113808));
#275740=CARTESIAN_POINT('Ctrl Pts',(-8.86851846634056,15.2,-5.51744788067916));
#275741=CARTESIAN_POINT('Ctrl Pts',(-8.87114125407647,15.2,-5.51859569022025));
#275742=CARTESIAN_POINT('Ctrl Pts',(-8.87381272327231,15.2,-5.51975585284065));
#275743=CARTESIAN_POINT('Ctrl Pts',(-8.87653241117021,15.2,-5.52092759338061));
#275744=CARTESIAN_POINT('Ctrl Pts',(-8.87925209931515,15.2,-5.52209933402701));
#275745=CARTESIAN_POINT('Ctrl Pts',(-8.88202000817308,15.2,-5.52328265684124));
#275746=CARTESIAN_POINT('Ctrl Pts',(-8.88483568141196,15.2,-5.52447681032346));
#275747=CARTESIAN_POINT('Ctrl Pts',(-8.88765135439507,15.2,-5.5256709636972));
#275748=CARTESIAN_POINT('Ctrl Pts',(-8.89051479414961,15.2,-5.52687594635476));
#275749=CARTESIAN_POINT('Ctrl Pts',(-8.89342555597366,15.2,-5.52809103098278));
#275750=CARTESIAN_POINT('Ctrl Pts',(-8.8963363177977,15.2,-5.52930611561081));
#275751=CARTESIAN_POINT('Ctrl Pts',(-8.89929439944313,15.2,-5.53053130127758));
#275752=CARTESIAN_POINT('Ctrl Pts',(-8.90229936641411,15.2,-5.53176587589877));
#275753=CARTESIAN_POINT('Ctrl Pts',(-8.90530433365805,15.2,-5.53300045063209));
#275754=CARTESIAN_POINT('Ctrl Pts',(-8.90835618651481,15.2,-5.53424441469965));
#275755=CARTESIAN_POINT('Ctrl Pts',(-8.9114544946857,15.2,-5.53549707276831));
#275756=CARTESIAN_POINT('Ctrl Pts',(-8.91455280257515,15.2,-5.53674973072317));
#275757=CARTESIAN_POINT('Ctrl Pts',(-8.91769756619174,15.2,-5.53801108558147));
#275758=CARTESIAN_POINT('Ctrl Pts',(-8.92088836400686,15.2,-5.53928045845776));
#275759=CARTESIAN_POINT('Ctrl Pts',(-8.92407916182198,15.2,-5.54054983133406));
#275760=CARTESIAN_POINT('Ctrl Pts',(-8.92731599336455,15.2,-5.54182722173214));
#275761=CARTESIAN_POINT('Ctrl Pts',(-8.93059844440887,15.2,-5.54311197160163));
#275762=CARTESIAN_POINT('Ctrl Pts',(-8.93388089575133,15.2,-5.54439672158783));
#275763=CARTESIAN_POINT('Ctrl Pts',(-8.93720896609641,15.2,-5.54568882888127));
#275764=CARTESIAN_POINT('Ctrl Pts',(-8.94058224953474,15.2,-5.54698765010066));
#275765=CARTESIAN_POINT('Ctrl Pts',(-8.94395553266667,15.2,-5.54828647120208));
#275766=CARTESIAN_POINT('Ctrl Pts',(-8.94737402688413,15.2,-5.54959200568932));
#275767=CARTESIAN_POINT('Ctrl Pts',(-8.95083733100831,15.2,-5.550903625725));
#275768=CARTESIAN_POINT('Ctrl Pts',(-8.95430063513249,15.2,-5.55221524576068));
#275769=CARTESIAN_POINT('Ctrl Pts',(-8.95780874996059,15.2,-5.55353294947097));
#275770=CARTESIAN_POINT('Ctrl Pts',(-8.96136128017309,15.2,-5.55485612365535));
#275771=CARTESIAN_POINT('Ctrl Pts',(-8.96491381070828,15.2,-5.55617929795992));
#275772=CARTESIAN_POINT('Ctrl Pts',(-8.96851075529544,15.2,-5.55750794212235));
#275773=CARTESIAN_POINT('Ctrl Pts',(-8.97215172666352,15.2,-5.55884145636203));
#275774=CARTESIAN_POINT('Ctrl Pts',(-8.97579269770089,15.2,-5.56017497048057));
#275775=CARTESIAN_POINT('Ctrl Pts',(-8.9794776951951,15.2,-5.56151335337662));
#275776=CARTESIAN_POINT('Ctrl Pts',(-8.98320633349334,15.2,-5.56285602050061));
#275777=CARTESIAN_POINT('Ctrl Pts',(-8.98693497179157,15.2,-5.56419868762461));
#275778=CARTESIAN_POINT('Ctrl Pts',(-8.99070725611604,15.2,-5.56554563715898));
#275779=CARTESIAN_POINT('Ctrl Pts',(-8.99452280230889,15.2,-5.56689629644308));
#275780=CARTESIAN_POINT('Ctrl Pts',(-8.99770242425178,15.2,-5.5680218458874));
#275781=CARTESIAN_POINT('Ctrl Pts',(-9.00091209151763,15.2,-5.56914997208176));
#275782=CARTESIAN_POINT('Ctrl Pts',(-9.00415158832164,15.2,-5.5702803484011));
#275783=CARTESIAN_POINT('Ctrl Pts',(-9.00739108512563,15.2,-5.57141072472042));
#275784=CARTESIAN_POINT('Ctrl Pts',(-9.01066041008883,15.2,-5.57254335434425));
#275785=CARTESIAN_POINT('Ctrl Pts',(-9.01395935121486,15.2,-5.57367791476606));
#275786=CARTESIAN_POINT('Ctrl Pts',(-9.01725829234089,15.2,-5.57481247518789));
#275787=CARTESIAN_POINT('Ctrl Pts',(-9.02058684908886,15.2,-5.57594896675556));
#275788=CARTESIAN_POINT('Ctrl Pts',(-9.02394481103331,15.2,-5.57708707724167));
#275789=CARTESIAN_POINT('Ctrl Pts',(-9.02730277297776,15.2,-5.57822518772779));
#275790=CARTESIAN_POINT('Ctrl Pts',(-9.03069013840847,15.2,-5.57936491817877));
#275791=CARTESIAN_POINT('Ctrl Pts',(-9.03410670120185,15.2,-5.58050595797563));
#275792=CARTESIAN_POINT('Ctrl Pts',(-9.03752326399521,15.2,-5.58164699777248));
#275793=CARTESIAN_POINT('Ctrl Pts',(-9.0409690221759,15.2,-5.58278935031363));
#275794=CARTESIAN_POINT('Ctrl Pts',(-9.04444377071907,15.2,-5.58393271079979));
#275795=CARTESIAN_POINT('Ctrl Pts',(-9.04791851926226,15.2,-5.58507607128596));
#275796=CARTESIAN_POINT('Ctrl Pts',(-9.05142225763523,15.2,-5.58622044081932));
#275797=CARTESIAN_POINT('Ctrl Pts',(-9.05495478124785,15.2,-5.58736552137491));
#275798=CARTESIAN_POINT('Ctrl Pts',(-9.05848730486047,15.2,-5.5885106019305));
#275799=CARTESIAN_POINT('Ctrl Pts',(-9.06204861416326,15.2,-5.58965639411467));
#275800=CARTESIAN_POINT('Ctrl Pts',(-9.06563850719182,15.2,-5.59080260715807));
#275801=CARTESIAN_POINT('Ctrl Pts',(-9.06922840022036,15.2,-5.59194882020148));
#275802=CARTESIAN_POINT('Ctrl Pts',(-9.07284687567467,15.2,-5.5930954523889));
#275803=CARTESIAN_POINT('Ctrl Pts',(-9.07649373526034,15.2,-5.59424221870834));
#275804=CARTESIAN_POINT('Ctrl Pts',(-9.080140594846,15.2,-5.5953889850278));
#275805=CARTESIAN_POINT('Ctrl Pts',(-9.08381583734878,15.2,-5.59653588415004));
#275806=CARTESIAN_POINT('Ctrl Pts',(-9.08751926672607,15.2,-5.59768263560834));
#275807=CARTESIAN_POINT('Ctrl Pts',(-9.0912226956997,15.2,-5.59882938694166));
#275808=CARTESIAN_POINT('Ctrl Pts',(-9.09495431111479,15.2,-5.59997599026944));
#275809=CARTESIAN_POINT('Ctrl Pts',(-9.09871391375824,15.2,-5.60112216757509));
#275810=CARTESIAN_POINT('Ctrl Pts',(-9.10247351681149,15.2,-5.60226834500568));
#275811=CARTESIAN_POINT('Ctrl Pts',(-9.10626111065876,15.2,-5.60341409837796));
#275812=CARTESIAN_POINT('Ctrl Pts',(-9.11007649947594,15.2,-5.60455915330858));
#275813=CARTESIAN_POINT('Ctrl Pts',(-9.11389188829312,15.2,-5.60570420823918));
#275814=CARTESIAN_POINT('Ctrl Pts',(-9.11773507289039,15.2,-5.6068485657226));
#275815=CARTESIAN_POINT('Ctrl Pts',(-9.12160586073537,15.2,-5.6079919580838));
#275816=CARTESIAN_POINT('Ctrl Pts',(-9.12547664858033,15.2,-5.60913535044498));
#275817=CARTESIAN_POINT('Ctrl Pts',(-9.12937503967234,15.2,-5.61027777802153));
#275818=CARTESIAN_POINT('Ctrl Pts',(-9.13330084285269,15.2,-5.61141897634254));
#275819=CARTESIAN_POINT('Ctrl Pts',(-9.13722664603305,15.2,-5.61256017466353));
#275820=CARTESIAN_POINT('Ctrl Pts',(-9.14117986225791,15.2,-5.61370014517547));
#275821=CARTESIAN_POINT('Ctrl Pts',(-9.14516030267316,15.2,-5.61483862767555));
#275822=CARTESIAN_POINT('Ctrl Pts',(-9.14914074308841,15.2,-5.61597711017563));
#275823=CARTESIAN_POINT('Ctrl Pts',(-9.15314840722661,15.2,-5.61711410606457));
#275824=CARTESIAN_POINT('Ctrl Pts',(-9.15718310854461,15.2,-5.6182493586341));
#275825=CARTESIAN_POINT('Ctrl Pts',(-9.1612178098626,15.2,-5.61938461120361));
#275826=CARTESIAN_POINT('Ctrl Pts',(-9.16527954857928,15.2,-5.62051812167203));
#275827=CARTESIAN_POINT('Ctrl Pts',(-9.16936813901443,15.2,-5.62164963994107));
#275828=CARTESIAN_POINT('Ctrl Pts',(-9.17345672944959,15.2,-5.6227811582101));
#275829=CARTESIAN_POINT('Ctrl Pts',(-9.17757216966108,15.2,-5.62391068283891));
#275830=CARTESIAN_POINT('Ctrl Pts',(-9.18171428000832,15.2,-5.62503796874169));
#275831=CARTESIAN_POINT('Ctrl Pts',(-9.18502796846671,15.2,-5.62593979751306));
#275832=CARTESIAN_POINT('Ctrl Pts',(-9.18835872356594,15.2,-5.62684019365371));
#275833=CARTESIAN_POINT('Ctrl Pts',(-9.19170645280569,15.2,-5.62773903114698));
#275834=CARTESIAN_POINT('Ctrl Pts',(-9.1950541815893,15.2,-5.62863786851779));
#275835=CARTESIAN_POINT('Ctrl Pts',(-9.19841888494494,15.2,-5.62953514950466));
#275836=CARTESIAN_POINT('Ctrl Pts',(-9.20180046973936,15.2,-5.63043074949108));
#275837=CARTESIAN_POINT('Ctrl Pts',(-9.2051820549945,15.2,-5.63132634959952));
#275838=CARTESIAN_POINT('Ctrl Pts',(-9.20858052225944,15.2,-5.63222026905579));
#275839=CARTESIAN_POINT('Ctrl Pts',(-9.21199577755839,15.2,-5.63311238660422));
#275840=CARTESIAN_POINT('Ctrl Pts',(-9.21541103239202,15.2,-5.6340045040311));
#275841=CARTESIAN_POINT('Ctrl Pts',(-9.21884307743735,15.2,-5.63489482060821));
#275842=CARTESIAN_POINT('Ctrl Pts',(-9.22229182020988,15.2,-5.63578321470237));
#275843=CARTESIAN_POINT('Ctrl Pts',(-9.2257405634523,15.2,-5.63667160891759));
#275844=CARTESIAN_POINT('Ctrl Pts',(-9.22920600346796,15.2,-5.63755808168615));
#275845=CARTESIAN_POINT('Ctrl Pts',(-9.23268805205535,15.2,-5.63844251511168));
#275846=CARTESIAN_POINT('Ctrl Pts',(-9.23617010016832,15.2,-5.63932694841672));
#275847=CARTESIAN_POINT('Ctrl Pts',(-9.23966875394013,15.2,-5.64020934176098));
#275848=CARTESIAN_POINT('Ctrl Pts',(-9.24318392476279,15.2,-5.64108957791138));
#275849=CARTESIAN_POINT('Ctrl Pts',(-9.24669909606439,15.2,-5.64196981418171));
#275850=CARTESIAN_POINT('Ctrl Pts',(-9.25023078448187,15.2,-5.64284789414069));
#275851=CARTESIAN_POINT('Ctrl Pts',(-9.25377889906521,15.2,-5.64372370285493));
#275852=CARTESIAN_POINT('Ctrl Pts',(-9.2573270131651,15.2,-5.64459951144985));
#275853=CARTESIAN_POINT('Ctrl Pts',(-9.2608915536624,15.2,-5.64547304632609));
#275854=CARTESIAN_POINT('Ctrl Pts',(-9.26447243321381,15.2,-5.6463441957986));
#275855=CARTESIAN_POINT('Ctrl Pts',(-9.26805331325311,15.2,-5.64721534538981));
#275856=CARTESIAN_POINT('Ctrl Pts',(-9.2716505298031,15.2,-5.64808410911266));
#275857=CARTESIAN_POINT('Ctrl Pts',(-9.27526399577888,15.2,-5.64895037460415));
#275858=CARTESIAN_POINT('Ctrl Pts',(-9.27887746126233,15.2,-5.64981663997761));
#275859=CARTESIAN_POINT('Ctrl Pts',(-9.28250717538693,15.2,-5.65068040619046));
#275860=CARTESIAN_POINT('Ctrl Pts',(-9.28615305142057,15.2,-5.65154156234256));
#275861=CARTESIAN_POINT('Ctrl Pts',(-9.28979892795095,15.2,-5.65240271861198));
#275862=CARTESIAN_POINT('Ctrl Pts',(-9.29346096421862,15.2,-5.65326126572231));
#275863=CARTESIAN_POINT('Ctrl Pts',(-9.29713907476917,15.2,-5.65411709321728));
#275864=CARTESIAN_POINT('Ctrl Pts',(-9.30081718481857,15.2,-5.65497292059564));
#275865=CARTESIAN_POINT('Ctrl Pts',(-9.30451136788721,15.2,-5.65582602702467));
#275866=CARTESIAN_POINT('Ctrl Pts',(-9.30822153736005,15.2,-5.65667630584434));
#275867=CARTESIAN_POINT('Ctrl Pts',(-9.3119317073384,15.2,-5.65752658477986));
#275868=CARTESIAN_POINT('Ctrl Pts',(-9.31565786331827,15.2,-5.65837403525957));
#275869=CARTESIAN_POINT('Ctrl Pts',(-9.31939991929999,15.2,-5.65921855075003));
#275870=CARTESIAN_POINT('Ctrl Pts',(-9.3231419752817,15.2,-5.6600630662405));
#275871=CARTESIAN_POINT('Ctrl Pts',(-9.32689993141806,15.2,-5.66090464463618));
#275872=CARTESIAN_POINT('Ctrl Pts',(-9.33067370012535,15.2,-5.66174318290379));
#275873=CARTESIAN_POINT('Ctrl Pts',(-9.33444746831846,15.2,-5.66258172105715));
#275874=CARTESIAN_POINT('Ctrl Pts',(-9.33823705201902,15.2,-5.66341721691093));
#275875=CARTESIAN_POINT('Ctrl Pts',(-9.34204236228074,15.2,-5.66424956645779));
#275876=CARTESIAN_POINT('Ctrl Pts',(-9.34584767306092,15.2,-5.66508191611807));
#275877=CARTESIAN_POINT('Ctrl Pts',(-9.34966871181662,15.2,-5.66591111958483));
#275878=CARTESIAN_POINT('Ctrl Pts',(-9.35350539436063,15.2,-5.66673707318507));
#275879=CARTESIAN_POINT('Ctrl Pts',(-9.3573420763819,15.2,-5.66756302667276));
#275880=CARTESIAN_POINT('Ctrl Pts',(-9.36119440090951,15.2,-5.66838573019423));
#275881=CARTESIAN_POINT('Ctrl Pts',(-9.36506228375894,15.2,-5.66920508168302));
#275882=CARTESIAN_POINT('Ctrl Pts',(-9.36893016713539,15.2,-5.67002443328345));
#275883=CARTESIAN_POINT('Ctrl Pts',(-9.37281360963223,15.2,-5.6708404320139));
#275884=CARTESIAN_POINT('Ctrl Pts',(-9.37671252587417,15.2,-5.67165297837625));
#275885=CARTESIAN_POINT('Ctrl Pts',(-9.3806114415849,15.2,-5.67246552462789));
#275886=CARTESIAN_POINT('Ctrl Pts',(-9.38452583170395,15.2,-5.67327461622755));
#275887=CARTESIAN_POINT('Ctrl Pts',(-9.38845561243721,15.2,-5.67408015571747));
#275888=CARTESIAN_POINT('Ctrl Pts',(-9.3923853937059,15.2,-5.67488569531716));
#275889=CARTESIAN_POINT('Ctrl Pts',(-9.3963305643515,15.2,-5.67568768109977));
#275890=CARTESIAN_POINT('Ctrl Pts',(-9.40029104312391,15.2,-5.67648601536526));
#275891=CARTESIAN_POINT('Ctrl Pts',(-9.4042515213567,15.2,-5.67728434952198));
#275892=CARTESIAN_POINT('Ctrl Pts',(-9.4082273074975,15.2,-5.67807903148776));
#275893=CARTESIAN_POINT('Ctrl Pts',(-9.41221831761414,15.2,-5.67886996314571));
#275894=CARTESIAN_POINT('Ctrl Pts',(-9.41620932827454,15.2,-5.67966089491143));
#275895=CARTESIAN_POINT('Ctrl Pts',(-9.42021556338748,15.2,-5.68044807716821));
#275896=CARTESIAN_POINT('Ctrl Pts',(-9.42423694073607,15.2,-5.68123141349223));
#275897=CARTESIAN_POINT('Ctrl Pts',(-9.42825831753676,15.2,-5.68201474970952));
#275898=CARTESIAN_POINT('Ctrl Pts',(-9.43229483704532,15.2,-5.682794239489));
#275899=CARTESIAN_POINT('Ctrl Pts',(-9.43634641587924,15.2,-5.68356978714823));
#275900=CARTESIAN_POINT('Ctrl Pts',(-9.44039799526518,15.2,-5.68434533491312));
#275901=CARTESIAN_POINT('Ctrl Pts',(-9.4444646351331,15.2,-5.68511694119431));
#275902=CARTESIAN_POINT('Ctrl Pts',(-9.44854625379999,15.2,-5.68588451095837));
#275903=CARTESIAN_POINT('Ctrl Pts',(-9.45364827685554,15.2,-5.68684397311115));
#275904=CARTESIAN_POINT('Ctrl Pts',(-9.4587737026627,15.2,-5.68779713090737));
#275905=CARTESIAN_POINT('Ctrl Pts',(-9.46392237497781,15.2,-5.68874379730055));
#275906=CARTESIAN_POINT('Ctrl Pts',(-9.46804131249317,15.2,-5.68950113035317));
#275907=CARTESIAN_POINT('Ctrl Pts',(-9.47217512823459,15.2,-5.6902543117217));
#275908=CARTESIAN_POINT('Ctrl Pts',(-9.47632374033837,15.2,-5.69100324866091));
#275909=CARTESIAN_POINT('Ctrl Pts',(-9.48047235300741,15.2,-5.69175218570217));
#275910=CARTESIAN_POINT('Ctrl Pts',(-9.48463576118337,15.2,-5.69249687712635));
#275911=CARTESIAN_POINT('Ctrl Pts',(-9.48881388596666,15.2,-5.69323723350004));
#275912=CARTESIAN_POINT('Ctrl Pts',(-9.49299201074995,15.2,-5.69397758987372));
#275913=CARTESIAN_POINT('Ctrl Pts',(-9.49718485192381,15.2,-5.69471361096912));
#275914=CARTESIAN_POINT('Ctrl Pts',(-9.50139233115459,15.2,-5.69544520611965));
#275915=CARTESIAN_POINT('Ctrl Pts',(-9.50559980981211,15.2,-5.69617680117049));
#275916=CARTESIAN_POINT('Ctrl Pts',(-9.50982192457151,15.2,-5.69690396997477));
#275917=CARTESIAN_POINT('Ctrl Pts',(-9.51405859552212,15.2,-5.69762662497454));
#275918=CARTESIAN_POINT('Ctrl Pts',(-9.51829526704998,15.2,-5.69834928007278));
#275919=CARTESIAN_POINT('Ctrl Pts',(-9.52254649656072,15.2,-5.6990674200755));
#275920=CARTESIAN_POINT('Ctrl Pts',(-9.52681220340578,15.2,-5.69978095839169));
#275921=CARTESIAN_POINT('Ctrl Pts',(-9.53107790966964,15.2,-5.70049449661066));
#275922=CARTESIAN_POINT('Ctrl Pts',(-9.53535809505942,15.2,-5.70120343125524));
#275923=CARTESIAN_POINT('Ctrl Pts',(-9.53965267920739,15.2,-5.70190767697575));
#275924=CARTESIAN_POINT('Ctrl Pts',(-9.54394726394048,15.2,-5.70261192279221));
#275925=CARTESIAN_POINT('Ctrl Pts',(-9.5482562481357,15.2,-5.70331147900367));
#275926=CARTESIAN_POINT('Ctrl Pts',(-9.55257955314409,15.2,-5.70400625890916));
#275927=CARTESIAN_POINT('Ctrl Pts',(-9.55690285756343,15.2,-5.70470103871999));
#275928=CARTESIAN_POINT('Ctrl Pts',(-9.56124048313994,15.2,-5.70539104347189));
#275929=CARTESIAN_POINT('Ctrl Pts',(-9.56559235189437,15.2,-5.70607618719398));
#275930=CARTESIAN_POINT('Ctrl Pts',(-9.57103218828209,15.2,-5.7069326169166));
#275931=CARTESIAN_POINT('Ctrl Pts',(-9.57649427917041,15.2,-5.70778145088903));
#275932=CARTESIAN_POINT('Ctrl Pts',(-9.58197847243313,15.2,-5.70862252644498));
#275933=CARTESIAN_POINT('Ctrl Pts',(-9.58636582728242,15.2,-5.70929538692643));
#275934=CARTESIAN_POINT('Ctrl Pts',(-9.59076732850055,15.2,-5.70996328121627));
#275935=CARTESIAN_POINT('Ctrl Pts',(-9.59518289940747,15.2,-5.71062612639619));
#275936=CARTESIAN_POINT('Ctrl Pts',(-9.59849457728686,15.2,-5.71112326023597));
#275937=CARTESIAN_POINT('Ctrl Pts',(-9.60181416738305,15.2,-5.71161755447166));
#275938=CARTESIAN_POINT('Ctrl Pts',(-9.60514164009616,15.2,-5.71210897337022));
#275939=CARTESIAN_POINT('Ctrl Pts',(-9.60846911280928,15.2,-5.71260039226878));
#275940=CARTESIAN_POINT('Ctrl Pts',(-9.61180446668815,15.2,-5.71308893688435));
#275941=CARTESIAN_POINT('Ctrl Pts',(-9.615147669025,15.2,-5.71357457178337));
#275942=CARTESIAN_POINT('Ctrl Pts',(-9.61849087136186,15.2,-5.71406020668239));
#275943=CARTESIAN_POINT('Ctrl Pts',(-9.62184192330674,15.2,-5.7145429320482));
#275944=CARTESIAN_POINT('Ctrl Pts',(-9.62520079160068,15.2,-5.71502271444769));
#275945=CARTESIAN_POINT('Ctrl Pts',(-9.62855965989462,15.2,-5.71550249684718));
#275946=CARTESIAN_POINT('Ctrl Pts',(-9.63192634415213,15.2,-5.71597933645152));
#275947=CARTESIAN_POINT('Ctrl Pts',(-9.63530081407221,15.2,-5.71645319787499));
#275948=CARTESIAN_POINT('Ctrl Pts',(-9.63867528399228,15.2,-5.71692705929846));
#275949=CARTESIAN_POINT('Ctrl Pts',(-9.64205753893522,15.2,-5.71739794384796));
#275950=CARTESIAN_POINT('Ctrl Pts',(-9.64544754526932,15.2,-5.71786581770637));
#275951=CARTESIAN_POINT('Ctrl Pts',(-9.64883755221928,15.2,-5.71833369164978));
#275952=CARTESIAN_POINT('Ctrl Pts',(-9.65223531184643,15.2,-5.71879855456734));
#275953=CARTESIAN_POINT('Ctrl Pts',(-9.65564079271741,15.2,-5.71926037305071));
#275954=CARTESIAN_POINT('Ctrl Pts',(-9.65904627296972,15.2,-5.71972219145018));
#275955=CARTESIAN_POINT('Ctrl Pts',(-9.66245947354663,15.2,-5.72018096598314));
#275956=CARTESIAN_POINT('Ctrl Pts',(-9.66588036288134,15.2,-5.72063666284132));
#275957=CARTESIAN_POINT('Ctrl Pts',(-9.66930125221606,15.2,-5.7210923596995));
#275958=CARTESIAN_POINT('Ctrl Pts',(-9.67272983131233,15.2,-5.72154497891475));
#275959=CARTESIAN_POINT('Ctrl Pts',(-9.67616606624479,15.2,-5.72199448873378));
#275960=CARTESIAN_POINT('Ctrl Pts',(-9.67960230117725,15.2,-5.72244399855281));
#275961=CARTESIAN_POINT('Ctrl Pts',(-9.68304619435662,15.2,-5.72289039763038));
#275962=CARTESIAN_POINT('Ctrl Pts',(-9.68649771220521,15.2,-5.72333365403297));
#275963=CARTESIAN_POINT('Ctrl Pts',(-9.68994923005379,15.2,-5.72377691043556));
#275964=CARTESIAN_POINT('Ctrl Pts',(-9.69340837381555,15.2,-5.72421702476796));
#275965=CARTESIAN_POINT('Ctrl Pts',(-9.69687511114726,15.2,-5.72465396371069));
#275966=CARTESIAN_POINT('Ctrl Pts',(-9.70034184847896,15.2,-5.72509090265342));
#275967=CARTESIAN_POINT('Ctrl Pts',(-9.70381618063514,15.2,-5.72552466723804));
#275968=CARTESIAN_POINT('Ctrl Pts',(-9.70729807450762,15.2,-5.72595522418117));
#275969=CARTESIAN_POINT('Ctrl Pts',(-9.71077996901264,15.2,-5.72638578120253));
#275970=CARTESIAN_POINT('Ctrl Pts',(-9.71426942676977,15.2,-5.72681313151463));
#275971=CARTESIAN_POINT('Ctrl Pts',(-9.71776641477902,15.2,-5.72723724211749));
#275972=CARTESIAN_POINT('Ctrl Pts',(-9.72242906439922,15.2,-5.7278027227929));
#275973=CARTESIAN_POINT('Ctrl Pts',(-9.72710510388947,15.2,-5.72836244767296));
#275974=CARTESIAN_POINT('Ctrl Pts',(-9.73179445747181,15.2,-5.72891633824133));
#275975=CARTESIAN_POINT('Ctrl Pts',(-9.73531147281829,15.2,-5.72933175618647));
#275976=CARTESIAN_POINT('Ctrl Pts',(-9.73883597809413,15.2,-5.72974389375332));
#275977=CARTESIAN_POINT('Ctrl Pts',(-9.74236794184014,15.2,-5.73015271873875));
#275978=CARTESIAN_POINT('Ctrl Pts',(-9.74589990558615,15.2,-5.73056154372418));
#275979=CARTESIAN_POINT('Ctrl Pts',(-9.74943932694002,15.2,-5.73096705712652));
#275980=CARTESIAN_POINT('Ctrl Pts',(-9.7529861762268,15.2,-5.73136922711236));
#275981=CARTESIAN_POINT('Ctrl Pts',(-9.75653302615793,15.2,-5.73177139717127));
#275982=CARTESIAN_POINT('Ctrl Pts',(-9.76008730432449,15.2,-5.73217022509589));
#275983=CARTESIAN_POINT('Ctrl Pts',(-9.76364897830146,15.2,-5.73256567861124));
#275984=CARTESIAN_POINT('Ctrl Pts',(-9.76839787585902,15.2,-5.7330929498453));
#275985=CARTESIAN_POINT('Ctrl Pts',(-9.77315992287876,15.2,-5.73361422294126));
#275986=CARTESIAN_POINT('Ctrl Pts',(-9.77793504637643,15.2,-5.73412942673287));
#275987=CARTESIAN_POINT('Ctrl Pts',(-9.78151638916232,15.2,-5.73451582959412));
#275988=CARTESIAN_POINT('Ctrl Pts',(-9.78510508708951,15.2,-5.734898817421));
#275989=CARTESIAN_POINT('Ctrl Pts',(-9.78870111005434,15.2,-5.73527836092658));
#275990=CARTESIAN_POINT('Ctrl Pts',(-9.79229713301916,15.2,-5.73565790443214));
#275991=CARTESIAN_POINT('Ctrl Pts',(-9.7959004807284,15.2,-5.7360340042152));
#275992=CARTESIAN_POINT('Ctrl Pts',(-9.79951112251289,15.2,-5.73640662911881));
#275993=CARTESIAN_POINT('Ctrl Pts',(-9.80432531199617,15.2,-5.73690346236873));
#275994=CARTESIAN_POINT('Ctrl Pts',(-9.8091524688362,15.2,-5.73739411877364));
#275995=CARTESIAN_POINT('Ctrl Pts',(-9.81399251976667,15.2,-5.73787852746671));
#275996=CARTESIAN_POINT('Ctrl Pts',(-9.81762255763479,15.2,-5.73824183395351));
#275997=CARTESIAN_POINT('Ctrl Pts',(-9.82125984956925,15.2,-5.73860162582378));
#275998=CARTESIAN_POINT('Ctrl Pts',(-9.82490436435288,15.2,-5.73895787568615));
#275999=CARTESIAN_POINT('Ctrl Pts',(-9.8285488791365,15.2,-5.73931412554851));
#276000=CARTESIAN_POINT('Ctrl Pts',(-9.83220061632649,15.2,-5.73966683146062));
#276001=CARTESIAN_POINT('Ctrl Pts',(-9.83585954683383,15.2,-5.74001596488246));
#276002=CARTESIAN_POINT('Ctrl Pts',(-9.83951847734118,15.2,-5.7403650983043));
#276003=CARTESIAN_POINT('Ctrl Pts',(-9.84318460051701,15.2,-5.74071065853743));
#276004=CARTESIAN_POINT('Ctrl Pts',(-9.84685788538257,15.2,-5.74105261790049));
#276005=CARTESIAN_POINT('Ctrl Pts',(-9.85053117091544,15.2,-5.74139457732568));
#276006=CARTESIAN_POINT('Ctrl Pts',(-9.85421161878367,15.2,-5.74173293480819));
#276007=CARTESIAN_POINT('Ctrl Pts',(-9.8578991987789,15.2,-5.74206766185634));
#276008=CARTESIAN_POINT('Ctrl Pts',(-9.86281597098936,15.2,-5.74251396448586));
#276009=CARTESIAN_POINT('Ctrl Pts',(-9.86774542312871,15.2,-5.74295381429955));
#276010=CARTESIAN_POINT('Ctrl Pts',(-9.87268748461278,15.2,-5.74338714293122));
#276011=CARTESIAN_POINT('Ctrl Pts',(-9.87639403089416,15.2,-5.74371213941973));
#276012=CARTESIAN_POINT('Ctrl Pts',(-9.88010766974699,15.2,-5.74403346845046));
#276013=CARTESIAN_POINT('Ctrl Pts',(-9.88382836925522,15.2,-5.74435109991355));
#276014=CARTESIAN_POINT('Ctrl Pts',(-9.88754906876343,15.2,-5.74466873137664));
#276015=CARTESIAN_POINT('Ctrl Pts',(-9.89127682890582,15.2,-5.74498266487651));
#276016=CARTESIAN_POINT('Ctrl Pts',(-9.89501162118583,15.2,-5.74529287340741));
#276017=CARTESIAN_POINT('Ctrl Pts',(-9.89874641414433,15.2,-5.74560308199467));
#276018=CARTESIAN_POINT('Ctrl Pts',(-9.90248823858813,15.2,-5.74590956647255));
#276019=CARTESIAN_POINT('Ctrl Pts',(-9.90623706809226,15.2,-5.7462123000577));
#276020=CARTESIAN_POINT('Ctrl Pts',(-9.90998589691535,15.2,-5.74651503358786));
#276021=CARTESIAN_POINT('Ctrl Pts',(-9.91374173067972,15.2,-5.74681401720988));
#276022=CARTESIAN_POINT('Ctrl Pts',(-9.91750453887694,15.2,-5.74710922349049));
#276023=CARTESIAN_POINT('Ctrl Pts',(-9.92126734707416,15.2,-5.7474044297711));
#276024=CARTESIAN_POINT('Ctrl Pts',(-9.92503712877347,15.2,-5.74769585587613));
#276025=CARTESIAN_POINT('Ctrl Pts',(-9.92881384702844,15.2,-5.74798346974197));
#276026=CARTESIAN_POINT('Ctrl Pts',(-9.9325905652834,15.2,-5.74827108360781));
#276027=CARTESIAN_POINT('Ctrl Pts',(-9.93637421943378,15.2,-5.74855488345867));
#276028=CARTESIAN_POINT('Ctrl Pts',(-9.9401647829799,15.2,-5.74883484474145));
#276029=CARTESIAN_POINT('Ctrl Pts',(-9.94648238911965,15.2,-5.74930144689638));
#276030=CARTESIAN_POINT('Ctrl Pts',(-9.95281918628111,15.2,-5.74975738256963));
#276031=CARTESIAN_POINT('Ctrl Pts',(-9.95917514600006,15.2,-5.75020264100001));
#276032=CARTESIAN_POINT('Origin',(-5.66257110645729E-14,15.2,-1.77635683940025E-14));
#276033=CARTESIAN_POINT('',(-8.56667970938041,15.2,-5.85257411403214));
#276034=CARTESIAN_POINT('',(-8.56667970938041,12.2,-5.85257411403214));
#276035=CARTESIAN_POINT('',(-8.56667970900006,15.2,-5.85257411400002));
#276036=CARTESIAN_POINT('Origin',(-5.66257110645729E-14,12.2,-1.77635683940025E-14));
#276037=CARTESIAN_POINT('Origin',(-5.66257110645729E-14,15.2,-1.77635683940025E-14));
#276038=CARTESIAN_POINT('Origin',(-5.66257110645729E-14,15.2,-1.77635683940025E-14));
#276039=CARTESIAN_POINT('',(-9.27155330300005,15.2,-6.80355049700001));
#276040=CARTESIAN_POINT('',(-9.03946594400006,15.2,-7.10901226900001));
#276041=CARTESIAN_POINT('Origin',(-5.66257110645729E-14,15.2,-1.77635683940025E-14));
#276042=CARTESIAN_POINT('',(-9.03946594400006,12.2,-7.10901226900001));
#276043=CARTESIAN_POINT('',(-9.03946594400006,15.2,-7.10901226900001));
#276044=CARTESIAN_POINT('',(-9.27155330300005,12.2,-6.80355049700001));
#276045=CARTESIAN_POINT('Origin',(-5.66257110645729E-14,12.2,-1.77635683940025E-14));
#276046=CARTESIAN_POINT('',(-9.27155330200006,15.2,-6.80355049700001));
#276047=CARTESIAN_POINT('Ctrl Pts',(-9.03946594400006,15.2,-7.10901226900001));
#276048=CARTESIAN_POINT('Ctrl Pts',(-9.03946594400006,11.6,-7.10901226900001));
#276049=CARTESIAN_POINT('Ctrl Pts',(-9.03871859600006,15.2,-7.10885083600001));
#276050=CARTESIAN_POINT('Ctrl Pts',(-9.03871859600006,11.6,-7.10885083600001));
#276051=CARTESIAN_POINT('Ctrl Pts',(-9.03722439200006,15.2,-7.10852778400002));
#276052=CARTESIAN_POINT('Ctrl Pts',(-9.03722439200006,11.6,-7.10852778400002));
#276053=CARTESIAN_POINT('Ctrl Pts',(-9.03498456200006,15.2,-7.10804263900001));
#276054=CARTESIAN_POINT('Ctrl Pts',(-9.03498456200006,11.6,-7.10804263900001));
#276055=CARTESIAN_POINT('Ctrl Pts',(-9.03200107200006,15.2,-7.10739465100002));
#276056=CARTESIAN_POINT('Ctrl Pts',(-9.03200107200006,11.6,-7.10739465100002));
#276057=CARTESIAN_POINT('Ctrl Pts',(-9.02827662900006,15.2,-7.10658278400001));
#276058=CARTESIAN_POINT('Ctrl Pts',(-9.02827662900006,11.6,-7.10658278400001));
#276059=CARTESIAN_POINT('Ctrl Pts',(-9.02455710700006,15.2,-7.10576903500002));
#276060=CARTESIAN_POINT('Ctrl Pts',(-9.02455710700006,11.6,-7.10576903500002));
#276061=CARTESIAN_POINT('Ctrl Pts',(-9.02084250600005,15.2,-7.10495340800002));
#276062=CARTESIAN_POINT('Ctrl Pts',(-9.02084250600005,11.6,-7.10495340800002));
#276063=CARTESIAN_POINT('Ctrl Pts',(-9.01713282900005,15.2,-7.10413590400002));
#276064=CARTESIAN_POINT('Ctrl Pts',(-9.01713282900005,11.6,-7.10413590400002));
#276065=CARTESIAN_POINT('Ctrl Pts',(-9.01342808000006,15.2,-7.10331652800001));
#276066=CARTESIAN_POINT('Ctrl Pts',(-9.01342808000006,11.6,-7.10331652800001));
#276067=CARTESIAN_POINT('Ctrl Pts',(-9.00972826500006,15.2,-7.10249528800002));
#276068=CARTESIAN_POINT('Ctrl Pts',(-9.00972826500006,11.6,-7.10249528800002));
#276069=CARTESIAN_POINT('Ctrl Pts',(-9.00603338900006,15.2,-7.10167218900001));
#276070=CARTESIAN_POINT('Ctrl Pts',(-9.00603338900006,11.6,-7.10167218900001));
#276071=CARTESIAN_POINT('Ctrl Pts',(-9.00234345900006,15.2,-7.10084724000002));
#276072=CARTESIAN_POINT('Ctrl Pts',(-9.00234345900006,11.6,-7.10084724000002));
#276073=CARTESIAN_POINT('Ctrl Pts',(-8.99865848200006,15.2,-7.10002045100002));
#276074=CARTESIAN_POINT('Ctrl Pts',(-8.99865848200006,11.6,-7.10002045100002));
#276075=CARTESIAN_POINT('Ctrl Pts',(-8.99497846500006,15.2,-7.09919182900002));
#276076=CARTESIAN_POINT('Ctrl Pts',(-8.99497846500006,11.6,-7.09919182900002));
#276077=CARTESIAN_POINT('Ctrl Pts',(-8.99130341600006,15.2,-7.09836138400001));
#276078=CARTESIAN_POINT('Ctrl Pts',(-8.99130341600006,11.6,-7.09836138400001));
#276079=CARTESIAN_POINT('Ctrl Pts',(-8.98763333900006,15.2,-7.09752912300001));
#276080=CARTESIAN_POINT('Ctrl Pts',(-8.98763333900006,11.6,-7.09752912300001));
#276081=CARTESIAN_POINT('Ctrl Pts',(-8.98396824000006,15.2,-7.09669505000001));
#276082=CARTESIAN_POINT('Ctrl Pts',(-8.98396824000006,11.6,-7.09669505000001));
#276083=CARTESIAN_POINT('Ctrl Pts',(-8.98030812400006,15.2,-7.09585917500001));
#276084=CARTESIAN_POINT('Ctrl Pts',(-8.98030812400006,11.6,-7.09585917500001));
#276085=CARTESIAN_POINT('Ctrl Pts',(-8.97665299700006,15.2,-7.09502150300001));
#276086=CARTESIAN_POINT('Ctrl Pts',(-8.97665299700006,11.6,-7.09502150300001));
#276087=CARTESIAN_POINT('Ctrl Pts',(-8.97300286400006,15.2,-7.09418203900002));
#276088=CARTESIAN_POINT('Ctrl Pts',(-8.97300286400006,11.6,-7.09418203900002));
#276089=CARTESIAN_POINT('Ctrl Pts',(-8.96935772900006,15.2,-7.09334079100002));
#276090=CARTESIAN_POINT('Ctrl Pts',(-8.96935772900006,11.6,-7.09334079100002));
#276091=CARTESIAN_POINT('Ctrl Pts',(-8.96571759800005,15.2,-7.09249776700001));
#276092=CARTESIAN_POINT('Ctrl Pts',(-8.96571759800005,11.6,-7.09249776700001));
#276093=CARTESIAN_POINT('Ctrl Pts',(-8.96208247800006,15.2,-7.09165297200002));
#276094=CARTESIAN_POINT('Ctrl Pts',(-8.96208247800006,11.6,-7.09165297200002));
#276095=CARTESIAN_POINT('Ctrl Pts',(-8.95845237400006,15.2,-7.09080641500002));
#276096=CARTESIAN_POINT('Ctrl Pts',(-8.95845237400006,11.6,-7.09080641500002));
#276097=CARTESIAN_POINT('Ctrl Pts',(-8.95482729200006,15.2,-7.08995810200002));
#276098=CARTESIAN_POINT('Ctrl Pts',(-8.95482729200006,11.6,-7.08995810200002));
#276099=CARTESIAN_POINT('Ctrl Pts',(-8.95120723800006,15.2,-7.08910804300002));
#276100=CARTESIAN_POINT('Ctrl Pts',(-8.95120723800006,11.6,-7.08910804300002));
#276101=CARTESIAN_POINT('Ctrl Pts',(-8.94759221900006,15.2,-7.08825624300002));
#276102=CARTESIAN_POINT('Ctrl Pts',(-8.94759221900006,11.6,-7.08825624300002));
#276103=CARTESIAN_POINT('Ctrl Pts',(-8.94398223900006,15.2,-7.08740271100002));
#276104=CARTESIAN_POINT('Ctrl Pts',(-8.94398223900006,11.6,-7.08740271100002));
#276105=CARTESIAN_POINT('Ctrl Pts',(-8.94037730400006,15.2,-7.08654745200001));
#276106=CARTESIAN_POINT('Ctrl Pts',(-8.94037730400006,11.6,-7.08654745200001));
#276107=CARTESIAN_POINT('Ctrl Pts',(-8.93677742100006,15.2,-7.08569047400001));
#276108=CARTESIAN_POINT('Ctrl Pts',(-8.93677742100006,11.6,-7.08569047400001));
#276109=CARTESIAN_POINT('Ctrl Pts',(-8.93318259400005,15.2,-7.08483178600002));
#276110=CARTESIAN_POINT('Ctrl Pts',(-8.93318259400005,11.6,-7.08483178600002));
#276111=CARTESIAN_POINT('Ctrl Pts',(-8.92959282900006,15.2,-7.08397139300001));
#276112=CARTESIAN_POINT('Ctrl Pts',(-8.92959282900006,11.6,-7.08397139300001));
#276113=CARTESIAN_POINT('Ctrl Pts',(-8.92600813200006,15.2,-7.08310930200001));
#276114=CARTESIAN_POINT('Ctrl Pts',(-8.92600813200006,11.6,-7.08310930200001));
#276115=CARTESIAN_POINT('Ctrl Pts',(-8.92242850800006,15.2,-7.08224552100001));
#276116=CARTESIAN_POINT('Ctrl Pts',(-8.92242850800006,11.6,-7.08224552100001));
#276117=CARTESIAN_POINT('Ctrl Pts',(-8.91885396500006,15.2,-7.08138005800001));
#276118=CARTESIAN_POINT('Ctrl Pts',(-8.91885396500006,11.6,-7.08138005800001));
#276119=CARTESIAN_POINT('Ctrl Pts',(-8.91528450600006,15.2,-7.08051292100001));
#276120=CARTESIAN_POINT('Ctrl Pts',(-8.91528450600006,11.6,-7.08051292100001));
#276121=CARTESIAN_POINT('Ctrl Pts',(-8.91172013800006,15.2,-7.07964411500001));
#276122=CARTESIAN_POINT('Ctrl Pts',(-8.91172013800006,11.6,-7.07964411500001));
#276123=CARTESIAN_POINT('Ctrl Pts',(-8.90816086700006,15.2,-7.07877364900002));
#276124=CARTESIAN_POINT('Ctrl Pts',(-8.90816086700006,11.6,-7.07877364900002));
#276125=CARTESIAN_POINT('Ctrl Pts',(-8.90460669800006,15.2,-7.07790152900002));
#276126=CARTESIAN_POINT('Ctrl Pts',(-8.90460669800006,11.6,-7.07790152900002));
#276127=CARTESIAN_POINT('Ctrl Pts',(-8.90105763800005,15.2,-7.07702776600001));
#276128=CARTESIAN_POINT('Ctrl Pts',(-8.90105763800005,11.6,-7.07702776600001));
#276129=CARTESIAN_POINT('Ctrl Pts',(-8.89751369200006,15.2,-7.07615236300001));
#276130=CARTESIAN_POINT('Ctrl Pts',(-8.89751369200006,11.6,-7.07615236300001));
#276131=CARTESIAN_POINT('Ctrl Pts',(-8.89397486600006,15.2,-7.07527533000002));
#276132=CARTESIAN_POINT('Ctrl Pts',(-8.89397486600006,11.6,-7.07527533000002));
#276133=CARTESIAN_POINT('Ctrl Pts',(-8.89044116400006,15.2,-7.07439667400001));
#276134=CARTESIAN_POINT('Ctrl Pts',(-8.89044116400006,11.6,-7.07439667400001));
#276135=CARTESIAN_POINT('Ctrl Pts',(-8.88691259400006,15.2,-7.07351640200002));
#276136=CARTESIAN_POINT('Ctrl Pts',(-8.88691259400006,11.6,-7.07351640200002));
#276137=CARTESIAN_POINT('Ctrl Pts',(-8.88338916200006,15.2,-7.07263452100002));
#276138=CARTESIAN_POINT('Ctrl Pts',(-8.88338916200006,11.6,-7.07263452100002));
#276139=CARTESIAN_POINT('Ctrl Pts',(-8.87987087300005,15.2,-7.07175104100001));
#276140=CARTESIAN_POINT('Ctrl Pts',(-8.87987087300005,11.6,-7.07175104100001));
#276141=CARTESIAN_POINT('Ctrl Pts',(-8.87635773200006,15.2,-7.07086596600002));
#276142=CARTESIAN_POINT('Ctrl Pts',(-8.87635773200006,11.6,-7.07086596600002));
#276143=CARTESIAN_POINT('Ctrl Pts',(-8.87284974500006,15.2,-7.06997930700001));
#276144=CARTESIAN_POINT('Ctrl Pts',(-8.87284974500006,11.6,-7.06997930700001));
#276145=CARTESIAN_POINT('Ctrl Pts',(-8.86934691800005,15.2,-7.06909107000002));
#276146=CARTESIAN_POINT('Ctrl Pts',(-8.86934691800005,11.6,-7.06909107000002));
#276147=CARTESIAN_POINT('Ctrl Pts',(-8.86584925900006,15.2,-7.06820126200002));
#276148=CARTESIAN_POINT('Ctrl Pts',(-8.86584925900006,11.6,-7.06820126200002));
#276149=CARTESIAN_POINT('Ctrl Pts',(-8.86235677000006,15.2,-7.06730989100001));
#276150=CARTESIAN_POINT('Ctrl Pts',(-8.86235677000006,11.6,-7.06730989100001));
#276151=CARTESIAN_POINT('Ctrl Pts',(-8.85886945900005,15.2,-7.06641696400002));
#276152=CARTESIAN_POINT('Ctrl Pts',(-8.85886945900005,11.6,-7.06641696400002));
#276153=CARTESIAN_POINT('Ctrl Pts',(-8.85538733200006,15.2,-7.06552249100002));
#276154=CARTESIAN_POINT('Ctrl Pts',(-8.85538733200006,11.6,-7.06552249100002));
#276155=CARTESIAN_POINT('Ctrl Pts',(-8.85191039400006,15.2,-7.06462647700001));
#276156=CARTESIAN_POINT('Ctrl Pts',(-8.85191039400006,11.6,-7.06462647700001));
#276157=CARTESIAN_POINT('Ctrl Pts',(-8.84843865100006,15.2,-7.06372893100002));
#276158=CARTESIAN_POINT('Ctrl Pts',(-8.84843865100006,11.6,-7.06372893100002));
#276159=CARTESIAN_POINT('Ctrl Pts',(-8.84497210900006,15.2,-7.06282986200002));
#276160=CARTESIAN_POINT('Ctrl Pts',(-8.84497210900006,11.6,-7.06282986200002));
#276161=CARTESIAN_POINT('Ctrl Pts',(-8.84151077400006,15.2,-7.06192927400001));
#276162=CARTESIAN_POINT('Ctrl Pts',(-8.84151077400006,11.6,-7.06192927400001));
#276163=CARTESIAN_POINT('Ctrl Pts',(-8.83805465100006,15.2,-7.06102717900002));
#276164=CARTESIAN_POINT('Ctrl Pts',(-8.83805465100006,11.6,-7.06102717900002));
#276165=CARTESIAN_POINT('Ctrl Pts',(-8.83460374700006,15.2,-7.06012358200002));
#276166=CARTESIAN_POINT('Ctrl Pts',(-8.83460374700006,11.6,-7.06012358200002));
#276167=CARTESIAN_POINT('Ctrl Pts',(-8.83115806700006,15.2,-7.05921849000001));
#276168=CARTESIAN_POINT('Ctrl Pts',(-8.83115806700006,11.6,-7.05921849000001));
#276169=CARTESIAN_POINT('Ctrl Pts',(-8.82771761700005,15.2,-7.05831191300001));
#276170=CARTESIAN_POINT('Ctrl Pts',(-8.82771761700005,11.6,-7.05831191300001));
#276171=CARTESIAN_POINT('Ctrl Pts',(-8.82428240300005,15.2,-7.05740385900001));
#276172=CARTESIAN_POINT('Ctrl Pts',(-8.82428240300005,11.6,-7.05740385900001));
#276173=CARTESIAN_POINT('Ctrl Pts',(-8.82085243100006,15.2,-7.05649433500002));
#276174=CARTESIAN_POINT('Ctrl Pts',(-8.82085243100006,11.6,-7.05649433500002));
#276175=CARTESIAN_POINT('Ctrl Pts',(-8.81742770700006,15.2,-7.05558334800001));
#276176=CARTESIAN_POINT('Ctrl Pts',(-8.81742770700006,11.6,-7.05558334800001));
#276177=CARTESIAN_POINT('Ctrl Pts',(-8.81400823600006,15.2,-7.05467090600001));
#276178=CARTESIAN_POINT('Ctrl Pts',(-8.81400823600006,11.6,-7.05467090600001));
#276179=CARTESIAN_POINT('Ctrl Pts',(-8.81059402400006,15.2,-7.05375701900002));
#276180=CARTESIAN_POINT('Ctrl Pts',(-8.81059402400006,11.6,-7.05375701900002));
#276181=CARTESIAN_POINT('Ctrl Pts',(-8.80718507800006,15.2,-7.05284169300001));
#276182=CARTESIAN_POINT('Ctrl Pts',(-8.80718507800006,11.6,-7.05284169300001));
#276183=CARTESIAN_POINT('Ctrl Pts',(-8.80378140200006,15.2,-7.05192493600002));
#276184=CARTESIAN_POINT('Ctrl Pts',(-8.80378140200006,11.6,-7.05192493600002));
#276185=CARTESIAN_POINT('Ctrl Pts',(-8.80038300400006,15.2,-7.05100675600002));
#276186=CARTESIAN_POINT('Ctrl Pts',(-8.80038300400006,11.6,-7.05100675600002));
#276187=CARTESIAN_POINT('Ctrl Pts',(-8.79698988900006,15.2,-7.05008716200001));
#276188=CARTESIAN_POINT('Ctrl Pts',(-8.79698988900006,11.6,-7.05008716200001));
#276189=CARTESIAN_POINT('Ctrl Pts',(-8.79360206200005,15.2,-7.04916616100002));
#276190=CARTESIAN_POINT('Ctrl Pts',(-8.79360206200005,11.6,-7.04916616100002));
#276191=CARTESIAN_POINT('Ctrl Pts',(-8.79021953000005,15.2,-7.04824376100002));
#276192=CARTESIAN_POINT('Ctrl Pts',(-8.79021953000005,11.6,-7.04824376100002));
#276193=CARTESIAN_POINT('Ctrl Pts',(-8.78684229800006,15.2,-7.04731997100002));
#276194=CARTESIAN_POINT('Ctrl Pts',(-8.78684229800006,11.6,-7.04731997100002));
#276195=CARTESIAN_POINT('Ctrl Pts',(-8.78347037400006,15.2,-7.04639479800001));
#276196=CARTESIAN_POINT('Ctrl Pts',(-8.78347037400006,11.6,-7.04639479800001));
#276197=CARTESIAN_POINT('Ctrl Pts',(-8.78010376100006,15.2,-7.04546825000002));
#276198=CARTESIAN_POINT('Ctrl Pts',(-8.78010376100006,11.6,-7.04546825000002));
#276199=CARTESIAN_POINT('Ctrl Pts',(-8.77674246700006,15.2,-7.04454033500002));
#276200=CARTESIAN_POINT('Ctrl Pts',(-8.77674246700006,11.6,-7.04454033500002));
#276201=CARTESIAN_POINT('Ctrl Pts',(-8.77338649600006,15.2,-7.04361106300002));
#276202=CARTESIAN_POINT('Ctrl Pts',(-8.77338649600006,11.6,-7.04361106300002));
#276203=CARTESIAN_POINT('Ctrl Pts',(-8.77003585700006,15.2,-7.04268044000001));
#276204=CARTESIAN_POINT('Ctrl Pts',(-8.77003585700006,11.6,-7.04268044000001));
#276205=CARTESIAN_POINT('Ctrl Pts',(-8.76669055200006,15.2,-7.04174847400001));
#276206=CARTESIAN_POINT('Ctrl Pts',(-8.76669055200006,11.6,-7.04174847400001));
#276207=CARTESIAN_POINT('Ctrl Pts',(-8.76335059000006,15.2,-7.04081517500001));
#276208=CARTESIAN_POINT('Ctrl Pts',(-8.76335059000006,11.6,-7.04081517500001));
#276209=CARTESIAN_POINT('Ctrl Pts',(-8.76001597600006,15.2,-7.03988055000002));
#276210=CARTESIAN_POINT('Ctrl Pts',(-8.76001597600006,11.6,-7.03988055000002));
#276211=CARTESIAN_POINT('Ctrl Pts',(-8.75668671600006,15.2,-7.03894460800001));
#276212=CARTESIAN_POINT('Ctrl Pts',(-8.75668671600006,11.6,-7.03894460800001));
#276213=CARTESIAN_POINT('Ctrl Pts',(-8.75336281400006,15.2,-7.03800735500002));
#276214=CARTESIAN_POINT('Ctrl Pts',(-8.75336281400006,11.6,-7.03800735500002));
#276215=CARTESIAN_POINT('Ctrl Pts',(-8.75004427900006,15.2,-7.03706880200002));
#276216=CARTESIAN_POINT('Ctrl Pts',(-8.75004427900006,11.6,-7.03706880200002));
#276217=CARTESIAN_POINT('Ctrl Pts',(-8.74673111600006,15.2,-7.03612895700001));
#276218=CARTESIAN_POINT('Ctrl Pts',(-8.74673111600006,11.6,-7.03612895700001));
#276219=CARTESIAN_POINT('Ctrl Pts',(-8.74342333000006,15.2,-7.03518782500002));
#276220=CARTESIAN_POINT('Ctrl Pts',(-8.74342333000006,11.6,-7.03518782500002));
#276221=CARTESIAN_POINT('Ctrl Pts',(-8.74012092800006,15.2,-7.03424541800001));
#276222=CARTESIAN_POINT('Ctrl Pts',(-8.74012092800006,11.6,-7.03424541800001));
#276223=CARTESIAN_POINT('Ctrl Pts',(-8.73682391500006,15.2,-7.03330174300002));
#276224=CARTESIAN_POINT('Ctrl Pts',(-8.73682391500006,11.6,-7.03330174300002));
#276225=CARTESIAN_POINT('Ctrl Pts',(-8.73353229800006,15.2,-7.03235680900002));
#276226=CARTESIAN_POINT('Ctrl Pts',(-8.73353229800006,11.6,-7.03235680900002));
#276227=CARTESIAN_POINT('Ctrl Pts',(-8.73024608200006,15.2,-7.03141062300002));
#276228=CARTESIAN_POINT('Ctrl Pts',(-8.73024608200006,11.6,-7.03141062300002));
#276229=CARTESIAN_POINT('Ctrl Pts',(-8.72696527300005,15.2,-7.03046319400002));
#276230=CARTESIAN_POINT('Ctrl Pts',(-8.72696527300005,11.6,-7.03046319400002));
#276231=CARTESIAN_POINT('Ctrl Pts',(-8.72368987800006,15.2,-7.02951453100002));
#276232=CARTESIAN_POINT('Ctrl Pts',(-8.72368987800006,11.6,-7.02951453100002));
#276233=CARTESIAN_POINT('Ctrl Pts',(-8.72041990300006,15.2,-7.02856464100002));
#276234=CARTESIAN_POINT('Ctrl Pts',(-8.72041990300006,11.6,-7.02856464100002));
#276235=CARTESIAN_POINT('Ctrl Pts',(-8.71715535200006,15.2,-7.02761353400001));
#276236=CARTESIAN_POINT('Ctrl Pts',(-8.71715535200006,11.6,-7.02761353400001));
#276237=CARTESIAN_POINT('Ctrl Pts',(-8.71389623400006,15.2,-7.02666121800001));
#276238=CARTESIAN_POINT('Ctrl Pts',(-8.71389623400006,11.6,-7.02666121800001));
#276239=CARTESIAN_POINT('Ctrl Pts',(-8.71064255200006,15.2,-7.02570770100002));
#276240=CARTESIAN_POINT('Ctrl Pts',(-8.71064255200006,11.6,-7.02570770100002));
#276241=CARTESIAN_POINT('Ctrl Pts',(-8.70739431400006,15.2,-7.02475299200002));
#276242=CARTESIAN_POINT('Ctrl Pts',(-8.70739431400006,11.6,-7.02475299200002));
#276243=CARTESIAN_POINT('Ctrl Pts',(-8.70415152500006,15.2,-7.02379710000002));
#276244=CARTESIAN_POINT('Ctrl Pts',(-8.70415152500006,11.6,-7.02379710000002));
#276245=CARTESIAN_POINT('Ctrl Pts',(-8.70091419100006,15.2,-7.02284003200001));
#276246=CARTESIAN_POINT('Ctrl Pts',(-8.70091419100006,11.6,-7.02284003200001));
#276247=CARTESIAN_POINT('Ctrl Pts',(-8.69768231900006,15.2,-7.02188179800002));
#276248=CARTESIAN_POINT('Ctrl Pts',(-8.69768231900006,11.6,-7.02188179800002));
#276249=CARTESIAN_POINT('Ctrl Pts',(-8.69445591400006,15.2,-7.02092240600001));
#276250=CARTESIAN_POINT('Ctrl Pts',(-8.69445591400006,11.6,-7.02092240600001));
#276251=CARTESIAN_POINT('Ctrl Pts',(-8.69123498300005,15.2,-7.01996186500002));
#276252=CARTESIAN_POINT('Ctrl Pts',(-8.69123498300005,11.6,-7.01996186500002));
#276253=CARTESIAN_POINT('Ctrl Pts',(-8.68801953200006,15.2,-7.01900018400002));
#276254=CARTESIAN_POINT('Ctrl Pts',(-8.68801953200006,11.6,-7.01900018400002));
#276255=CARTESIAN_POINT('Ctrl Pts',(-8.68480956600006,15.2,-7.01803737000001));
#276256=CARTESIAN_POINT('Ctrl Pts',(-8.68480956600006,11.6,-7.01803737000001));
#276257=CARTESIAN_POINT('Ctrl Pts',(-8.68160509100005,15.2,-7.01707343300002));
#276258=CARTESIAN_POINT('Ctrl Pts',(-8.68160509100005,11.6,-7.01707343300002));
#276259=CARTESIAN_POINT('Ctrl Pts',(-8.67840611400006,15.2,-7.01610838100001));
#276260=CARTESIAN_POINT('Ctrl Pts',(-8.67840611400006,11.6,-7.01610838100001));
#276261=CARTESIAN_POINT('Ctrl Pts',(-8.67521264100005,15.2,-7.01514222400001));
#276262=CARTESIAN_POINT('Ctrl Pts',(-8.67521264100005,11.6,-7.01514222400001));
#276263=CARTESIAN_POINT('Ctrl Pts',(-8.67202467700006,15.2,-7.01417496900002));
#276264=CARTESIAN_POINT('Ctrl Pts',(-8.67202467700006,11.6,-7.01417496900002));
#276265=CARTESIAN_POINT('Ctrl Pts',(-8.66884222900006,15.2,-7.01320662700001));
#276266=CARTESIAN_POINT('Ctrl Pts',(-8.66884222900006,11.6,-7.01320662700001));
#276267=CARTESIAN_POINT('Ctrl Pts',(-8.66566530400006,15.2,-7.01223720400002));
#276268=CARTESIAN_POINT('Ctrl Pts',(-8.66566530400006,11.6,-7.01223720400002));
#276269=CARTESIAN_POINT('Ctrl Pts',(-8.66249390600006,15.2,-7.01126671100001));
#276270=CARTESIAN_POINT('Ctrl Pts',(-8.66249390600006,11.6,-7.01126671100001));
#276271=CARTESIAN_POINT('Ctrl Pts',(-8.65932804200006,15.2,-7.01029515700001));
#276272=CARTESIAN_POINT('Ctrl Pts',(-8.65932804200006,11.6,-7.01029515700001));
#276273=CARTESIAN_POINT('Ctrl Pts',(-8.65616771800006,15.2,-7.00932254900002));
#276274=CARTESIAN_POINT('Ctrl Pts',(-8.65616771800006,11.6,-7.00932254900002));
#276275=CARTESIAN_POINT('Ctrl Pts',(-8.65301294000006,15.2,-7.00834889700002));
#276276=CARTESIAN_POINT('Ctrl Pts',(-8.65301294000006,11.6,-7.00834889700002));
#276277=CARTESIAN_POINT('Ctrl Pts',(-8.64986371500006,15.2,-7.00737421000002));
#276278=CARTESIAN_POINT('Ctrl Pts',(-8.64986371500006,11.6,-7.00737421000002));
#276279=CARTESIAN_POINT('Ctrl Pts',(-8.64672004800006,15.2,-7.00639849700002));
#276280=CARTESIAN_POINT('Ctrl Pts',(-8.64672004800006,11.6,-7.00639849700002));
#276281=CARTESIAN_POINT('Ctrl Pts',(-8.64358194600005,15.2,-7.00542176600001));
#276282=CARTESIAN_POINT('Ctrl Pts',(-8.64358194600005,11.6,-7.00542176600001));
#276283=CARTESIAN_POINT('Ctrl Pts',(-8.64044941400006,15.2,-7.00444402600001));
#276284=CARTESIAN_POINT('Ctrl Pts',(-8.64044941400006,11.6,-7.00444402600001));
#276285=CARTESIAN_POINT('Ctrl Pts',(-8.63732245800006,15.2,-7.00346528800001));
#276286=CARTESIAN_POINT('Ctrl Pts',(-8.63732245800006,11.6,-7.00346528800001));
#276287=CARTESIAN_POINT('Ctrl Pts',(-8.63420108600006,15.2,-7.00248556000002));
#276288=CARTESIAN_POINT('Ctrl Pts',(-8.63420108600006,11.6,-7.00248556000002));
#276289=CARTESIAN_POINT('Ctrl Pts',(-8.63108530200006,15.2,-7.00150485000002));
#276290=CARTESIAN_POINT('Ctrl Pts',(-8.63108530200006,11.6,-7.00150485000002));
#276291=CARTESIAN_POINT('Ctrl Pts',(-8.62797511400006,15.2,-7.00052316700001));
#276292=CARTESIAN_POINT('Ctrl Pts',(-8.62797511400006,11.6,-7.00052316700001));
#276293=CARTESIAN_POINT('Ctrl Pts',(-8.62487052700006,15.2,-6.99954052200002));
#276294=CARTESIAN_POINT('Ctrl Pts',(-8.62487052700006,11.6,-6.99954052200002));
#276295=CARTESIAN_POINT('Ctrl Pts',(-8.62177154800005,15.2,-6.99855692200002));
#276296=CARTESIAN_POINT('Ctrl Pts',(-8.62177154800005,11.6,-6.99855692200002));
#276297=CARTESIAN_POINT('Ctrl Pts',(-8.61867818200006,15.2,-6.99757237900001));
#276298=CARTESIAN_POINT('Ctrl Pts',(-8.61867818200006,11.6,-6.99757237900001));
#276299=CARTESIAN_POINT('Ctrl Pts',(-8.61559043500005,15.2,-6.99658689800001));
#276300=CARTESIAN_POINT('Ctrl Pts',(-8.61559043500005,11.6,-6.99658689800001));
#276301=CARTESIAN_POINT('Ctrl Pts',(-8.61250831400006,15.2,-6.99560049200001));
#276302=CARTESIAN_POINT('Ctrl Pts',(-8.61250831400006,11.6,-6.99560049200001));
#276303=CARTESIAN_POINT('Ctrl Pts',(-8.60943182500005,15.2,-6.99461316800001));
#276304=CARTESIAN_POINT('Ctrl Pts',(-8.60943182500005,11.6,-6.99461316800001));
#276305=CARTESIAN_POINT('Ctrl Pts',(-8.60636097400005,15.2,-6.99362493600002));
#276306=CARTESIAN_POINT('Ctrl Pts',(-8.60636097400005,11.6,-6.99362493600002));
#276307=CARTESIAN_POINT('Ctrl Pts',(-8.60329576800006,15.2,-6.99263580600002));
#276308=CARTESIAN_POINT('Ctrl Pts',(-8.60329576800006,11.6,-6.99263580600002));
#276309=CARTESIAN_POINT('Ctrl Pts',(-8.60023621200006,15.2,-6.99164578600002));
#276310=CARTESIAN_POINT('Ctrl Pts',(-8.60023621200006,11.6,-6.99164578600002));
#276311=CARTESIAN_POINT('Ctrl Pts',(-8.59718231200005,15.2,-6.99065488500001));
#276312=CARTESIAN_POINT('Ctrl Pts',(-8.59718231200005,11.6,-6.99065488500001));
#276313=CARTESIAN_POINT('Ctrl Pts',(-8.59413407600006,15.2,-6.98966311400002));
#276314=CARTESIAN_POINT('Ctrl Pts',(-8.59413407600006,11.6,-6.98966311400002));
#276315=CARTESIAN_POINT('Ctrl Pts',(-8.59109150900006,15.2,-6.98867048200002));
#276316=CARTESIAN_POINT('Ctrl Pts',(-8.59109150900006,11.6,-6.98867048200002));
#276317=CARTESIAN_POINT('Ctrl Pts',(-8.58805461700006,15.2,-6.98767699600002));
#276318=CARTESIAN_POINT('Ctrl Pts',(-8.58805461700006,11.6,-6.98767699600002));
#276319=CARTESIAN_POINT('Ctrl Pts',(-8.58502340600005,15.2,-6.98668266800002));
#276320=CARTESIAN_POINT('Ctrl Pts',(-8.58502340600005,11.6,-6.98668266800002));
#276321=CARTESIAN_POINT('Ctrl Pts',(-8.58199788300006,15.2,-6.98568750700002));
#276322=CARTESIAN_POINT('Ctrl Pts',(-8.58199788300006,11.6,-6.98568750700002));
#276323=CARTESIAN_POINT('Ctrl Pts',(-8.57897805400006,15.2,-6.98469152300002));
#276324=CARTESIAN_POINT('Ctrl Pts',(-8.57897805400006,11.6,-6.98469152300002));
#276325=CARTESIAN_POINT('Ctrl Pts',(-8.57596392500006,15.2,-6.98369472200002));
#276326=CARTESIAN_POINT('Ctrl Pts',(-8.57596392500006,11.6,-6.98369472200002));
#276327=CARTESIAN_POINT('Ctrl Pts',(-8.57295550200006,15.2,-6.98269711800001));
#276328=CARTESIAN_POINT('Ctrl Pts',(-8.57295550200006,11.6,-6.98269711800001));
#276329=CARTESIAN_POINT('Ctrl Pts',(-8.56995279100006,15.2,-6.98169871900002));
#276330=CARTESIAN_POINT('Ctrl Pts',(-8.56995279100006,11.6,-6.98169871900002));
#276331=CARTESIAN_POINT('Ctrl Pts',(-8.56695580000006,15.2,-6.98069953300001));
#276332=CARTESIAN_POINT('Ctrl Pts',(-8.56695580000006,11.6,-6.98069953300001));
#276333=CARTESIAN_POINT('Ctrl Pts',(-8.56396453400006,15.2,-6.97969957100002));
#276334=CARTESIAN_POINT('Ctrl Pts',(-8.56396453400006,11.6,-6.97969957100002));
#276335=CARTESIAN_POINT('Ctrl Pts',(-8.56097900000006,15.2,-6.97869884300002));
#276336=CARTESIAN_POINT('Ctrl Pts',(-8.56097900000006,11.6,-6.97869884300002));
#276337=CARTESIAN_POINT('Ctrl Pts',(-8.55799920200005,15.2,-6.97769735700002));
#276338=CARTESIAN_POINT('Ctrl Pts',(-8.55799920200005,11.6,-6.97769735700002));
#276339=CARTESIAN_POINT('Ctrl Pts',(-8.55502514900006,15.2,-6.97669512400001));
#276340=CARTESIAN_POINT('Ctrl Pts',(-8.55502514900006,11.6,-6.97669512400001));
#276341=CARTESIAN_POINT('Ctrl Pts',(-8.55205684500006,15.2,-6.97569215300001));
#276342=CARTESIAN_POINT('Ctrl Pts',(-8.55205684500006,11.6,-6.97569215300001));
#276343=CARTESIAN_POINT('Ctrl Pts',(-8.54909429800006,15.2,-6.97468845400002));
#276344=CARTESIAN_POINT('Ctrl Pts',(-8.54909429800006,11.6,-6.97468845400002));
#276345=CARTESIAN_POINT('Ctrl Pts',(-8.54613751300005,15.2,-6.97368403700001));
#276346=CARTESIAN_POINT('Ctrl Pts',(-8.54613751300005,11.6,-6.97368403700001));
#276347=CARTESIAN_POINT('Ctrl Pts',(-8.54318649800006,15.2,-6.97267891200001));
#276348=CARTESIAN_POINT('Ctrl Pts',(-8.54318649800006,11.6,-6.97267891200001));
#276349=CARTESIAN_POINT('Ctrl Pts',(-8.54024125700005,15.2,-6.97167308800001));
#276350=CARTESIAN_POINT('Ctrl Pts',(-8.54024125700005,11.6,-6.97167308800001));
#276351=CARTESIAN_POINT('Ctrl Pts',(-8.53730179800005,15.2,-6.97066657500002));
#276352=CARTESIAN_POINT('Ctrl Pts',(-8.53730179800005,11.6,-6.97066657500002));
#276353=CARTESIAN_POINT('Ctrl Pts',(-8.53436812700006,15.2,-6.96965938200002));
#276354=CARTESIAN_POINT('Ctrl Pts',(-8.53436812700006,11.6,-6.96965938200002));
#276355=CARTESIAN_POINT('Ctrl Pts',(-8.53144025100006,15.2,-6.96865152100001));
#276356=CARTESIAN_POINT('Ctrl Pts',(-8.53144025100006,11.6,-6.96865152100001));
#276357=CARTESIAN_POINT('Ctrl Pts',(-8.52851817400006,15.2,-6.96764300000002));
#276358=CARTESIAN_POINT('Ctrl Pts',(-8.52851817400006,11.6,-6.96764300000002));
#276359=CARTESIAN_POINT('Ctrl Pts',(-8.52560190400006,15.2,-6.96663382900002));
#276360=CARTESIAN_POINT('Ctrl Pts',(-8.52560190400006,11.6,-6.96663382900002));
#276361=CARTESIAN_POINT('Ctrl Pts',(-8.52269144900006,15.2,-6.96562402000002));
#276362=CARTESIAN_POINT('Ctrl Pts',(-8.52269144900006,11.6,-6.96562402000002));
#276363=CARTESIAN_POINT('Ctrl Pts',(-8.51978681100006,15.2,-6.96461358000001));
#276364=CARTESIAN_POINT('Ctrl Pts',(-8.51978681100006,11.6,-6.96461358000001));
#276365=CARTESIAN_POINT('Ctrl Pts',(-8.51688800000005,15.2,-6.96360252200002));
#276366=CARTESIAN_POINT('Ctrl Pts',(-8.51688800000005,11.6,-6.96360252200002));
#276367=CARTESIAN_POINT('Ctrl Pts',(-8.51399502100006,15.2,-6.96259085300002));
#276368=CARTESIAN_POINT('Ctrl Pts',(-8.51399502100006,11.6,-6.96259085300002));
#276369=CARTESIAN_POINT('Ctrl Pts',(-8.51110788000006,15.2,-6.96157858500002));
#276370=CARTESIAN_POINT('Ctrl Pts',(-8.51110788000006,11.6,-6.96157858500002));
#276371=CARTESIAN_POINT('Ctrl Pts',(-8.50822658400006,15.2,-6.96056572800002));
#276372=CARTESIAN_POINT('Ctrl Pts',(-8.50822658400006,11.6,-6.96056572800002));
#276373=CARTESIAN_POINT('Ctrl Pts',(-8.50535113900006,15.2,-6.95955229100001));
#276374=CARTESIAN_POINT('Ctrl Pts',(-8.50535113900006,11.6,-6.95955229100001));
#276375=CARTESIAN_POINT('Ctrl Pts',(-8.50248155100006,15.2,-6.95853828600002));
#276376=CARTESIAN_POINT('Ctrl Pts',(-8.50248155100006,11.6,-6.95853828600002));
#276377=CARTESIAN_POINT('Ctrl Pts',(-8.49961782900006,15.2,-6.95752372000002));
#276378=CARTESIAN_POINT('Ctrl Pts',(-8.49961782900006,11.6,-6.95752372000002));
#276379=CARTESIAN_POINT('Ctrl Pts',(-8.49675997600006,15.2,-6.95650860700002));
#276380=CARTESIAN_POINT('Ctrl Pts',(-8.49675997600006,11.6,-6.95650860700002));
#276381=CARTESIAN_POINT('Ctrl Pts',(-8.49390800000006,15.2,-6.95549295400002));
#276382=CARTESIAN_POINT('Ctrl Pts',(-8.49390800000006,11.6,-6.95549295400002));
#276383=CARTESIAN_POINT('Ctrl Pts',(-8.49106190600006,15.2,-6.95447677400002));
#276384=CARTESIAN_POINT('Ctrl Pts',(-8.49106190600006,11.6,-6.95447677400002));
#276385=CARTESIAN_POINT('Ctrl Pts',(-8.48822170400006,15.2,-6.95346007500002));
#276386=CARTESIAN_POINT('Ctrl Pts',(-8.48822170400006,11.6,-6.95346007500002));
#276387=CARTESIAN_POINT('Ctrl Pts',(-8.48538739600006,15.2,-6.95244286800002));
#276388=CARTESIAN_POINT('Ctrl Pts',(-8.48538739600006,11.6,-6.95244286800002));
#276389=CARTESIAN_POINT('Ctrl Pts',(-8.48255899100005,15.2,-6.95142516400002));
#276390=CARTESIAN_POINT('Ctrl Pts',(-8.48255899100005,11.6,-6.95142516400002));
#276391=CARTESIAN_POINT('Ctrl Pts',(-8.47973649400006,15.2,-6.95040697300002));
#276392=CARTESIAN_POINT('Ctrl Pts',(-8.47973649400006,11.6,-6.95040697300002));
#276393=CARTESIAN_POINT('Ctrl Pts',(-8.47691991300006,15.2,-6.94938830400002));
#276394=CARTESIAN_POINT('Ctrl Pts',(-8.47691991300006,11.6,-6.94938830400002));
#276395=CARTESIAN_POINT('Ctrl Pts',(-8.47410925300006,15.2,-6.94836916900002));
#276396=CARTESIAN_POINT('Ctrl Pts',(-8.47410925300006,11.6,-6.94836916900002));
#276397=CARTESIAN_POINT('Ctrl Pts',(-8.47130452200006,15.2,-6.94734957900002));
#276398=CARTESIAN_POINT('Ctrl Pts',(-8.47130452200006,11.6,-6.94734957900002));
#276399=CARTESIAN_POINT('Ctrl Pts',(-8.46850572600006,15.2,-6.94632954200002));
#276400=CARTESIAN_POINT('Ctrl Pts',(-8.46850572600006,11.6,-6.94632954200002));
#276401=CARTESIAN_POINT('Ctrl Pts',(-8.46571286900006,15.2,-6.94530907100001));
#276402=CARTESIAN_POINT('Ctrl Pts',(-8.46571286900006,11.6,-6.94530907100001));
#276403=CARTESIAN_POINT('Ctrl Pts',(-8.46292596100006,15.2,-6.94428817600001));
#276404=CARTESIAN_POINT('Ctrl Pts',(-8.46292596100006,11.6,-6.94428817600001));
#276405=CARTESIAN_POINT('Ctrl Pts',(-8.46014500600005,15.2,-6.94326686700002));
#276406=CARTESIAN_POINT('Ctrl Pts',(-8.46014500600005,11.6,-6.94326686700002));
#276407=CARTESIAN_POINT('Ctrl Pts',(-8.45737001200006,15.2,-6.94224515400002));
#276408=CARTESIAN_POINT('Ctrl Pts',(-8.45737001200006,11.6,-6.94224515400002));
#276409=CARTESIAN_POINT('Ctrl Pts',(-8.45460098500006,15.2,-6.94122304900001));
#276410=CARTESIAN_POINT('Ctrl Pts',(-8.45460098500006,11.6,-6.94122304900001));
#276411=CARTESIAN_POINT('Ctrl Pts',(-8.45183793100006,15.2,-6.94020056100002));
#276412=CARTESIAN_POINT('Ctrl Pts',(-8.45183793100006,11.6,-6.94020056100002));
#276413=CARTESIAN_POINT('Ctrl Pts',(-8.44908085600006,15.2,-6.93917770200001));
#276414=CARTESIAN_POINT('Ctrl Pts',(-8.44908085600006,11.6,-6.93917770200001));
#276415=CARTESIAN_POINT('Ctrl Pts',(-8.44632976900006,15.2,-6.93815448200001));
#276416=CARTESIAN_POINT('Ctrl Pts',(-8.44632976900006,11.6,-6.93815448200001));
#276417=CARTESIAN_POINT('Ctrl Pts',(-8.44358467400006,15.2,-6.93713091300002));
#276418=CARTESIAN_POINT('Ctrl Pts',(-8.44358467400006,11.6,-6.93713091300002));
#276419=CARTESIAN_POINT('Ctrl Pts',(-8.44084557900005,15.2,-6.93610700400002));
#276420=CARTESIAN_POINT('Ctrl Pts',(-8.44084557900005,11.6,-6.93610700400002));
#276421=CARTESIAN_POINT('Ctrl Pts',(-8.43811248900005,15.2,-6.93508276600002));
#276422=CARTESIAN_POINT('Ctrl Pts',(-8.43811248900005,11.6,-6.93508276600002));
#276423=CARTESIAN_POINT('Ctrl Pts',(-8.43538541200006,15.2,-6.93405821000002));
#276424=CARTESIAN_POINT('Ctrl Pts',(-8.43538541200006,11.6,-6.93405821000002));
#276425=CARTESIAN_POINT('Ctrl Pts',(-8.43266435300006,15.2,-6.93303334900002));
#276426=CARTESIAN_POINT('Ctrl Pts',(-8.43266435300006,11.6,-6.93303334900002));
#276427=CARTESIAN_POINT('Ctrl Pts',(-8.42994932200006,15.2,-6.93200819000002));
#276428=CARTESIAN_POINT('Ctrl Pts',(-8.42994932200006,11.6,-6.93200819000002));
#276429=CARTESIAN_POINT('Ctrl Pts',(-8.42724032100006,15.2,-6.93098274800001));
#276430=CARTESIAN_POINT('Ctrl Pts',(-8.42724032100006,11.6,-6.93098274800001));
#276431=CARTESIAN_POINT('Ctrl Pts',(-8.42453736000006,15.2,-6.92995703000002));
#276432=CARTESIAN_POINT('Ctrl Pts',(-8.42453736000006,11.6,-6.92995703000002));
#276433=CARTESIAN_POINT('Ctrl Pts',(-8.42184044300006,15.2,-6.92893105000002));
#276434=CARTESIAN_POINT('Ctrl Pts',(-8.42184044300006,11.6,-6.92893105000002));
#276435=CARTESIAN_POINT('Ctrl Pts',(-8.41914957900006,15.2,-6.92790481800002));
#276436=CARTESIAN_POINT('Ctrl Pts',(-8.41914957900006,11.6,-6.92790481800002));
#276437=CARTESIAN_POINT('Ctrl Pts',(-8.41646477200005,15.2,-6.92687834500001));
#276438=CARTESIAN_POINT('Ctrl Pts',(-8.41646477200005,11.6,-6.92687834500001));
#276439=CARTESIAN_POINT('Ctrl Pts',(-8.41378603100006,15.2,-6.92585164200001));
#276440=CARTESIAN_POINT('Ctrl Pts',(-8.41378603100006,11.6,-6.92585164200001));
#276441=CARTESIAN_POINT('Ctrl Pts',(-8.41111336100006,15.2,-6.92482472000002));
#276442=CARTESIAN_POINT('Ctrl Pts',(-8.41111336100006,11.6,-6.92482472000002));
#276443=CARTESIAN_POINT('Ctrl Pts',(-8.40844676900005,15.2,-6.92379758900002));
#276444=CARTESIAN_POINT('Ctrl Pts',(-8.40844676900005,11.6,-6.92379758900002));
#276445=CARTESIAN_POINT('Ctrl Pts',(-8.40578626200006,15.2,-6.92277026300002));
#276446=CARTESIAN_POINT('Ctrl Pts',(-8.40578626200006,11.6,-6.92277026300002));
#276447=CARTESIAN_POINT('Ctrl Pts',(-8.40313184700006,15.2,-6.92174275100002));
#276448=CARTESIAN_POINT('Ctrl Pts',(-8.40313184700006,11.6,-6.92174275100002));
#276449=CARTESIAN_POINT('Ctrl Pts',(-8.40048352900006,15.2,-6.92071506500002));
#276450=CARTESIAN_POINT('Ctrl Pts',(-8.40048352900006,11.6,-6.92071506500002));
#276451=CARTESIAN_POINT('Ctrl Pts',(-8.39784131700006,15.2,-6.91968721500002));
#276452=CARTESIAN_POINT('Ctrl Pts',(-8.39784131700006,11.6,-6.91968721500002));
#276453=CARTESIAN_POINT('Ctrl Pts',(-8.39520521500006,15.2,-6.91865921400002));
#276454=CARTESIAN_POINT('Ctrl Pts',(-8.39520521500006,11.6,-6.91865921400002));
#276455=CARTESIAN_POINT('Ctrl Pts',(-8.39257523200006,15.2,-6.91763107400002));
#276456=CARTESIAN_POINT('Ctrl Pts',(-8.39257523200006,11.6,-6.91763107400002));
#276457=CARTESIAN_POINT('Ctrl Pts',(-8.38995137300006,15.2,-6.91660280300002));
#276458=CARTESIAN_POINT('Ctrl Pts',(-8.38995137300006,11.6,-6.91660280300002));
#276459=CARTESIAN_POINT('Ctrl Pts',(-8.38733364500006,15.2,-6.91557441500001));
#276460=CARTESIAN_POINT('Ctrl Pts',(-8.38733364500006,11.6,-6.91557441500001));
#276461=CARTESIAN_POINT('Ctrl Pts',(-8.38472205600005,15.2,-6.91454592100002));
#276462=CARTESIAN_POINT('Ctrl Pts',(-8.38472205600005,11.6,-6.91454592100002));
#276463=CARTESIAN_POINT('Ctrl Pts',(-8.38211661100006,15.2,-6.91351733200002));
#276464=CARTESIAN_POINT('Ctrl Pts',(-8.38211661100006,11.6,-6.91351733200002));
#276465=CARTESIAN_POINT('Ctrl Pts',(-8.37951731800005,15.2,-6.91248865900001));
#276466=CARTESIAN_POINT('Ctrl Pts',(-8.37951731800005,11.6,-6.91248865900001));
#276467=CARTESIAN_POINT('Ctrl Pts',(-8.37692418100006,15.2,-6.91145991600001));
#276468=CARTESIAN_POINT('Ctrl Pts',(-8.37692418100006,11.6,-6.91145991600001));
#276469=CARTESIAN_POINT('Ctrl Pts',(-8.37433721100006,15.2,-6.91043111100001));
#276470=CARTESIAN_POINT('Ctrl Pts',(-8.37433721100006,11.6,-6.91043111100001));
#276471=CARTESIAN_POINT('Ctrl Pts',(-8.37175641100006,15.2,-6.90940225800002));
#276472=CARTESIAN_POINT('Ctrl Pts',(-8.37175641100006,11.6,-6.90940225800002));
#276473=CARTESIAN_POINT('Ctrl Pts',(-8.36918179000006,15.2,-6.90837336800002));
#276474=CARTESIAN_POINT('Ctrl Pts',(-8.36918179000006,11.6,-6.90837336800002));
#276475=CARTESIAN_POINT('Ctrl Pts',(-8.36661335300006,15.2,-6.90734445300001));
#276476=CARTESIAN_POINT('Ctrl Pts',(-8.36661335300006,11.6,-6.90734445300001));
#276477=CARTESIAN_POINT('Ctrl Pts',(-8.36405110900006,15.2,-6.90631552400002));
#276478=CARTESIAN_POINT('Ctrl Pts',(-8.36405110900006,11.6,-6.90631552400002));
#276479=CARTESIAN_POINT('Ctrl Pts',(-8.36149506200006,15.2,-6.90528659300002));
#276480=CARTESIAN_POINT('Ctrl Pts',(-8.36149506200006,11.6,-6.90528659300002));
#276481=CARTESIAN_POINT('Ctrl Pts',(-8.35894522100006,15.2,-6.90425767200002));
#276482=CARTESIAN_POINT('Ctrl Pts',(-8.35894522100006,11.6,-6.90425767200002));
#276483=CARTESIAN_POINT('Ctrl Pts',(-8.35640159200006,15.2,-6.90322877200002));
#276484=CARTESIAN_POINT('Ctrl Pts',(-8.35640159200006,11.6,-6.90322877200002));
#276485=CARTESIAN_POINT('Ctrl Pts',(-8.35386418000006,15.2,-6.90219990600001));
#276486=CARTESIAN_POINT('Ctrl Pts',(-8.35386418000006,11.6,-6.90219990600001));
#276487=CARTESIAN_POINT('Ctrl Pts',(-8.35133299600006,15.2,-6.90117108400001));
#276488=CARTESIAN_POINT('Ctrl Pts',(-8.35133299600006,11.6,-6.90117108400001));
#276489=CARTESIAN_POINT('Ctrl Pts',(-8.34880804200005,15.2,-6.90014232000002));
#276490=CARTESIAN_POINT('Ctrl Pts',(-8.34880804200005,11.6,-6.90014232000002));
#276491=CARTESIAN_POINT('Ctrl Pts',(-8.34628932800005,15.2,-6.89911362500002));
#276492=CARTESIAN_POINT('Ctrl Pts',(-8.34628932800005,11.6,-6.89911362500002));
#276493=CARTESIAN_POINT('Ctrl Pts',(-8.34377685900006,15.2,-6.89808501100002));
#276494=CARTESIAN_POINT('Ctrl Pts',(-8.34377685900006,11.6,-6.89808501100002));
#276495=CARTESIAN_POINT('Ctrl Pts',(-8.34127064400005,15.2,-6.89705649000001));
#276496=CARTESIAN_POINT('Ctrl Pts',(-8.34127064400005,11.6,-6.89705649000001));
#276497=CARTESIAN_POINT('Ctrl Pts',(-8.33877068700006,15.2,-6.89602807400002));
#276498=CARTESIAN_POINT('Ctrl Pts',(-8.33877068700006,11.6,-6.89602807400002));
#276499=CARTESIAN_POINT('Ctrl Pts',(-8.33627699700006,15.2,-6.89499977500001));
#276500=CARTESIAN_POINT('Ctrl Pts',(-8.33627699700006,11.6,-6.89499977500001));
#276501=CARTESIAN_POINT('Ctrl Pts',(-8.33378957900005,15.2,-6.89397160500001));
#276502=CARTESIAN_POINT('Ctrl Pts',(-8.33378957900005,11.6,-6.89397160500001));
#276503=CARTESIAN_POINT('Ctrl Pts',(-8.33130844300005,15.2,-6.89294357600001));
#276504=CARTESIAN_POINT('Ctrl Pts',(-8.33130844300005,11.6,-6.89294357600001));
#276505=CARTESIAN_POINT('Ctrl Pts',(-8.32883359200006,15.2,-6.89191570100002));
#276506=CARTESIAN_POINT('Ctrl Pts',(-8.32883359200006,11.6,-6.89191570100002));
#276507=CARTESIAN_POINT('Ctrl Pts',(-8.32636503500006,15.2,-6.89088799200002));
#276508=CARTESIAN_POINT('Ctrl Pts',(-8.32636503500006,11.6,-6.89088799200002));
#276509=CARTESIAN_POINT('Ctrl Pts',(-8.32390277900006,15.2,-6.88986046100001));
#276510=CARTESIAN_POINT('Ctrl Pts',(-8.32390277900006,11.6,-6.88986046100001));
#276511=CARTESIAN_POINT('Ctrl Pts',(-8.32144683000006,15.2,-6.88883311900002));
#276512=CARTESIAN_POINT('Ctrl Pts',(-8.32144683000006,11.6,-6.88883311900002));
#276513=CARTESIAN_POINT('Ctrl Pts',(-8.31899719600005,15.2,-6.88780598100001));
#276514=CARTESIAN_POINT('Ctrl Pts',(-8.31899719600005,11.6,-6.88780598100001));
#276515=CARTESIAN_POINT('Ctrl Pts',(-8.31655388200006,15.2,-6.88677905700001));
#276516=CARTESIAN_POINT('Ctrl Pts',(-8.31655388200006,11.6,-6.88677905700001));
#276517=CARTESIAN_POINT('Ctrl Pts',(-8.31411689600005,15.2,-6.88575236100001));
#276518=CARTESIAN_POINT('Ctrl Pts',(-8.31411689600005,11.6,-6.88575236100001));
#276519=CARTESIAN_POINT('Ctrl Pts',(-8.31168624600006,15.2,-6.88472590400002));
#276520=CARTESIAN_POINT('Ctrl Pts',(-8.31168624600006,11.6,-6.88472590400002));
#276521=CARTESIAN_POINT('Ctrl Pts',(-8.30926193800006,15.2,-6.88369969900001));
#276522=CARTESIAN_POINT('Ctrl Pts',(-8.30926193800006,11.6,-6.88369969900001));
#276523=CARTESIAN_POINT('Ctrl Pts',(-8.30684397800006,15.2,-6.88267375900002));
#276524=CARTESIAN_POINT('Ctrl Pts',(-8.30684397800006,11.6,-6.88267375900002));
#276525=CARTESIAN_POINT('Ctrl Pts',(-8.30443237500005,15.2,-6.88164809600002));
#276526=CARTESIAN_POINT('Ctrl Pts',(-8.30443237500005,11.6,-6.88164809600002));
#276527=CARTESIAN_POINT('Ctrl Pts',(-8.30202713400006,15.2,-6.88062272300002));
#276528=CARTESIAN_POINT('Ctrl Pts',(-8.30202713400006,11.6,-6.88062272300002));
#276529=CARTESIAN_POINT('Ctrl Pts',(-8.29962826300006,15.2,-6.87959765300001));
#276530=CARTESIAN_POINT('Ctrl Pts',(-8.29962826300006,11.6,-6.87959765300001));
#276531=CARTESIAN_POINT('Ctrl Pts',(-8.29723576800006,15.2,-6.87857289700001));
#276532=CARTESIAN_POINT('Ctrl Pts',(-8.29723576800006,11.6,-6.87857289700001));
#276533=CARTESIAN_POINT('Ctrl Pts',(-8.29484965700006,15.2,-6.87754847000001));
#276534=CARTESIAN_POINT('Ctrl Pts',(-8.29484965700006,11.6,-6.87754847000001));
#276535=CARTESIAN_POINT('Ctrl Pts',(-8.29246993600006,15.2,-6.87652438300002));
#276536=CARTESIAN_POINT('Ctrl Pts',(-8.29246993600006,11.6,-6.87652438300002));
#276537=CARTESIAN_POINT('Ctrl Pts',(-8.29009661400006,15.2,-6.87550064900002));
#276538=CARTESIAN_POINT('Ctrl Pts',(-8.29009661400006,11.6,-6.87550064900002));
#276539=CARTESIAN_POINT('Ctrl Pts',(-8.28772969600006,15.2,-6.87447728100001));
#276540=CARTESIAN_POINT('Ctrl Pts',(-8.28772969600006,11.6,-6.87447728100001));
#276541=CARTESIAN_POINT('Ctrl Pts',(-8.28536918900006,15.2,-6.87345429300001));
#276542=CARTESIAN_POINT('Ctrl Pts',(-8.28536918900006,11.6,-6.87345429300001));
#276543=CARTESIAN_POINT('Ctrl Pts',(-8.28301510100006,15.2,-6.87243169500002));
#276544=CARTESIAN_POINT('Ctrl Pts',(-8.28301510100006,11.6,-6.87243169500002));
#276545=CARTESIAN_POINT('Ctrl Pts',(-8.28066743900006,15.2,-6.87140950400002));
#276546=CARTESIAN_POINT('Ctrl Pts',(-8.28066743900006,11.6,-6.87140950400002));
#276547=CARTESIAN_POINT('Ctrl Pts',(-8.27832621000006,15.2,-6.87038772900002));
#276548=CARTESIAN_POINT('Ctrl Pts',(-8.27832621000006,11.6,-6.87038772900002));
#276549=CARTESIAN_POINT('Ctrl Pts',(-8.27599142100006,15.2,-6.86936638500002));
#276550=CARTESIAN_POINT('Ctrl Pts',(-8.27599142100006,11.6,-6.86936638500002));
#276551=CARTESIAN_POINT('Ctrl Pts',(-8.27366307900006,15.2,-6.86834548500002));
#276552=CARTESIAN_POINT('Ctrl Pts',(-8.27366307900006,11.6,-6.86834548500002));
#276553=CARTESIAN_POINT('Ctrl Pts',(-8.27134119000006,15.2,-6.86732504200001));
#276554=CARTESIAN_POINT('Ctrl Pts',(-8.27134119000006,11.6,-6.86732504200001));
#276555=CARTESIAN_POINT('Ctrl Pts',(-8.26902576200006,15.2,-6.86630507000002));
#276556=CARTESIAN_POINT('Ctrl Pts',(-8.26902576200006,11.6,-6.86630507000002));
#276557=CARTESIAN_POINT('Ctrl Pts',(-8.26671680300005,15.2,-6.86528558000001));
#276558=CARTESIAN_POINT('Ctrl Pts',(-8.26671680300005,11.6,-6.86528558000001));
#276559=CARTESIAN_POINT('Ctrl Pts',(-8.26441431900006,15.2,-6.86426658600002));
#276560=CARTESIAN_POINT('Ctrl Pts',(-8.26441431900006,11.6,-6.86426658600002));
#276561=CARTESIAN_POINT('Ctrl Pts',(-8.26211831700006,15.2,-6.86324810400002));
#276562=CARTESIAN_POINT('Ctrl Pts',(-8.26211831700006,11.6,-6.86324810400002));
#276563=CARTESIAN_POINT('Ctrl Pts',(-8.25982880500005,15.2,-6.86223014300002));
#276564=CARTESIAN_POINT('Ctrl Pts',(-8.25982880500005,11.6,-6.86223014300002));
#276565=CARTESIAN_POINT('Ctrl Pts',(-8.25754578900005,15.2,-6.86121271800002));
#276566=CARTESIAN_POINT('Ctrl Pts',(-8.25754578900005,11.6,-6.86121271800002));
#276567=CARTESIAN_POINT('Ctrl Pts',(-8.25526927700006,15.2,-6.86019584300002));
#276568=CARTESIAN_POINT('Ctrl Pts',(-8.25526927700006,11.6,-6.86019584300002));
#276569=CARTESIAN_POINT('Ctrl Pts',(-8.25299927600006,15.2,-6.85917953200001));
#276570=CARTESIAN_POINT('Ctrl Pts',(-8.25299927600006,11.6,-6.85917953200001));
#276571=CARTESIAN_POINT('Ctrl Pts',(-8.25073579400006,15.2,-6.85816379700002));
#276572=CARTESIAN_POINT('Ctrl Pts',(-8.25073579400006,11.6,-6.85816379700002));
#276573=CARTESIAN_POINT('Ctrl Pts',(-8.24847883600006,15.2,-6.85714865200002));
#276574=CARTESIAN_POINT('Ctrl Pts',(-8.24847883600006,11.6,-6.85714865200002));
#276575=CARTESIAN_POINT('Ctrl Pts',(-8.24622841100006,15.2,-6.85613411000002));
#276576=CARTESIAN_POINT('Ctrl Pts',(-8.24622841100006,11.6,-6.85613411000002));
#276577=CARTESIAN_POINT('Ctrl Pts',(-8.24398452500006,15.2,-6.85512018700001));
#276578=CARTESIAN_POINT('Ctrl Pts',(-8.24398452500006,11.6,-6.85512018700001));
#276579=CARTESIAN_POINT('Ctrl Pts',(-8.24174718700006,15.2,-6.85410689300002));
#276580=CARTESIAN_POINT('Ctrl Pts',(-8.24174718700006,11.6,-6.85410689300002));
#276581=CARTESIAN_POINT('Ctrl Pts',(-8.23951640200006,15.2,-6.85309424500002));
#276582=CARTESIAN_POINT('Ctrl Pts',(-8.23951640200006,11.6,-6.85309424500002));
#276583=CARTESIAN_POINT('Ctrl Pts',(-8.23729218000006,15.2,-6.85208225400002));
#276584=CARTESIAN_POINT('Ctrl Pts',(-8.23729218000006,11.6,-6.85208225400002));
#276585=CARTESIAN_POINT('Ctrl Pts',(-8.23507452500005,15.2,-6.85107093700001));
#276586=CARTESIAN_POINT('Ctrl Pts',(-8.23507452500005,11.6,-6.85107093700001));
#276587=CARTESIAN_POINT('Ctrl Pts',(-8.23286344500006,15.2,-6.85006030300002));
#276588=CARTESIAN_POINT('Ctrl Pts',(-8.23286344500006,11.6,-6.85006030300002));
#276589=CARTESIAN_POINT('Ctrl Pts',(-8.23065894900006,15.2,-6.84905037100001));
#276590=CARTESIAN_POINT('Ctrl Pts',(-8.23065894900006,11.6,-6.84905037100001));
#276591=CARTESIAN_POINT('Ctrl Pts',(-8.22846104400006,15.2,-6.84804115200001));
#276592=CARTESIAN_POINT('Ctrl Pts',(-8.22846104400006,11.6,-6.84804115200001));
#276593=CARTESIAN_POINT('Ctrl Pts',(-8.22626973600006,15.2,-6.84703266000002));
#276594=CARTESIAN_POINT('Ctrl Pts',(-8.22626973600006,11.6,-6.84703266000002));
#276595=CARTESIAN_POINT('Ctrl Pts',(-8.22408503300006,15.2,-6.84602491000001));
#276596=CARTESIAN_POINT('Ctrl Pts',(-8.22408503300006,11.6,-6.84602491000001));
#276597=CARTESIAN_POINT('Ctrl Pts',(-8.22190694200006,15.2,-6.84501791600002));
#276598=CARTESIAN_POINT('Ctrl Pts',(-8.22190694200006,11.6,-6.84501791600002));
#276599=CARTESIAN_POINT('Ctrl Pts',(-8.21973547100006,15.2,-6.84401169100001));
#276600=CARTESIAN_POINT('Ctrl Pts',(-8.21973547100006,11.6,-6.84401169100001));
#276601=CARTESIAN_POINT('Ctrl Pts',(-8.21757062600006,15.2,-6.84300624900001));
#276602=CARTESIAN_POINT('Ctrl Pts',(-8.21757062600006,11.6,-6.84300624900001));
#276603=CARTESIAN_POINT('Ctrl Pts',(-8.21541241600006,15.2,-6.84200160600002));
#276604=CARTESIAN_POINT('Ctrl Pts',(-8.21541241600006,11.6,-6.84200160600002));
#276605=CARTESIAN_POINT('Ctrl Pts',(-8.21326084700006,15.2,-6.84099777500002));
#276606=CARTESIAN_POINT('Ctrl Pts',(-8.21326084700006,11.6,-6.84099777500002));
#276607=CARTESIAN_POINT('Ctrl Pts',(-8.21111592700005,15.2,-6.83999477000001));
#276608=CARTESIAN_POINT('Ctrl Pts',(-8.21111592700005,11.6,-6.83999477000001));
#276609=CARTESIAN_POINT('Ctrl Pts',(-8.20897766400006,15.2,-6.83899260600001));
#276610=CARTESIAN_POINT('Ctrl Pts',(-8.20897766400006,11.6,-6.83899260600001));
#276611=CARTESIAN_POINT('Ctrl Pts',(-8.20684606400006,15.2,-6.83799129700001));
#276612=CARTESIAN_POINT('Ctrl Pts',(-8.20684606400006,11.6,-6.83799129700001));
#276613=CARTESIAN_POINT('Ctrl Pts',(-8.20472113500006,15.2,-6.83699085700002));
#276614=CARTESIAN_POINT('Ctrl Pts',(-8.20472113500006,11.6,-6.83699085700002));
#276615=CARTESIAN_POINT('Ctrl Pts',(-8.20260288500006,15.2,-6.83599130200002));
#276616=CARTESIAN_POINT('Ctrl Pts',(-8.20260288500006,11.6,-6.83599130200002));
#276617=CARTESIAN_POINT('Ctrl Pts',(-8.20049132100005,15.2,-6.83499264500002));
#276618=CARTESIAN_POINT('Ctrl Pts',(-8.20049132100005,11.6,-6.83499264500002));
#276619=CARTESIAN_POINT('Ctrl Pts',(-8.19838644900006,15.2,-6.83399490000002));
#276620=CARTESIAN_POINT('Ctrl Pts',(-8.19838644900006,11.6,-6.83399490000002));
#276621=CARTESIAN_POINT('Ctrl Pts',(-8.19628827900006,15.2,-6.83299808400001));
#276622=CARTESIAN_POINT('Ctrl Pts',(-8.19628827900006,11.6,-6.83299808400001));
#276623=CARTESIAN_POINT('Ctrl Pts',(-8.19419681700005,15.2,-6.83200220900002));
#276624=CARTESIAN_POINT('Ctrl Pts',(-8.19419681700005,11.6,-6.83200220900002));
#276625=CARTESIAN_POINT('Ctrl Pts',(-8.19211207000006,15.2,-6.83100729200002));
#276626=CARTESIAN_POINT('Ctrl Pts',(-8.19211207000006,11.6,-6.83100729200002));
#276627=CARTESIAN_POINT('Ctrl Pts',(-8.19003404800006,15.2,-6.83001334600001));
#276628=CARTESIAN_POINT('Ctrl Pts',(-8.19003404800006,11.6,-6.83001334600001));
#276629=CARTESIAN_POINT('Ctrl Pts',(-8.18796275500006,15.2,-6.82902038700002));
#276630=CARTESIAN_POINT('Ctrl Pts',(-8.18796275500006,11.6,-6.82902038700002));
#276631=CARTESIAN_POINT('Ctrl Pts',(-8.18589820000006,15.2,-6.82802842800001));
#276632=CARTESIAN_POINT('Ctrl Pts',(-8.18589820000006,11.6,-6.82802842800001));
#276633=CARTESIAN_POINT('Ctrl Pts',(-8.18384039200006,15.2,-6.82703748600002));
#276634=CARTESIAN_POINT('Ctrl Pts',(-8.18384039200006,11.6,-6.82703748600002));
#276635=CARTESIAN_POINT('Ctrl Pts',(-8.18178933600005,15.2,-6.82604757600001));
#276636=CARTESIAN_POINT('Ctrl Pts',(-8.18178933600005,11.6,-6.82604757600001));
#276637=CARTESIAN_POINT('Ctrl Pts',(-8.17974504200006,15.2,-6.82505871000001));
#276638=CARTESIAN_POINT('Ctrl Pts',(-8.17974504200006,11.6,-6.82505871000001));
#276639=CARTESIAN_POINT('Ctrl Pts',(-8.17770751500005,15.2,-6.82407090600002));
#276640=CARTESIAN_POINT('Ctrl Pts',(-8.17770751500005,11.6,-6.82407090600002));
#276641=CARTESIAN_POINT('Ctrl Pts',(-8.17567676400006,15.2,-6.82308417800002));
#276642=CARTESIAN_POINT('Ctrl Pts',(-8.17567676400006,11.6,-6.82308417800002));
#276643=CARTESIAN_POINT('Ctrl Pts',(-8.17365279800006,15.2,-6.82209854300002));
#276644=CARTESIAN_POINT('Ctrl Pts',(-8.17365279800006,11.6,-6.82209854300002));
#276645=CARTESIAN_POINT('Ctrl Pts',(-8.17163562200006,15.2,-6.82111401300002));
#276646=CARTESIAN_POINT('Ctrl Pts',(-8.17163562200006,11.6,-6.82111401300002));
#276647=CARTESIAN_POINT('Ctrl Pts',(-8.16962524500006,15.2,-6.82013060400001));
#276648=CARTESIAN_POINT('Ctrl Pts',(-8.16962524500006,11.6,-6.82013060400001));
#276649=CARTESIAN_POINT('Ctrl Pts',(-8.16762167300006,15.2,-6.81914833300001));
#276650=CARTESIAN_POINT('Ctrl Pts',(-8.16762167300006,11.6,-6.81914833300001));
#276651=CARTESIAN_POINT('Ctrl Pts',(-8.16562491600006,15.2,-6.81816721500001));
#276652=CARTESIAN_POINT('Ctrl Pts',(-8.16562491600006,11.6,-6.81816721500001));
#276653=CARTESIAN_POINT('Ctrl Pts',(-8.16363498100005,15.2,-6.81718726300002));
#276654=CARTESIAN_POINT('Ctrl Pts',(-8.16363498100005,11.6,-6.81718726300002));
#276655=CARTESIAN_POINT('Ctrl Pts',(-8.16165187500006,15.2,-6.81620849600002));
#276656=CARTESIAN_POINT('Ctrl Pts',(-8.16165187500006,11.6,-6.81620849600002));
#276657=CARTESIAN_POINT('Ctrl Pts',(-8.15967560600006,15.2,-6.81523092700001));
#276658=CARTESIAN_POINT('Ctrl Pts',(-8.15967560600006,11.6,-6.81523092700001));
#276659=CARTESIAN_POINT('Ctrl Pts',(-8.15770618100006,15.2,-6.81425457200002));
#276660=CARTESIAN_POINT('Ctrl Pts',(-8.15770618100006,11.6,-6.81425457200002));
#276661=CARTESIAN_POINT('Ctrl Pts',(-8.15574360800005,15.2,-6.81327944800002));
#276662=CARTESIAN_POINT('Ctrl Pts',(-8.15574360800005,11.6,-6.81327944800002));
#276663=CARTESIAN_POINT('Ctrl Pts',(-8.15378789600006,15.2,-6.81230556900001));
#276664=CARTESIAN_POINT('Ctrl Pts',(-8.15378789600006,11.6,-6.81230556900001));
#276665=CARTESIAN_POINT('Ctrl Pts',(-8.15183905100006,15.2,-6.81133295000001));
#276666=CARTESIAN_POINT('Ctrl Pts',(-8.15183905100006,11.6,-6.81133295000001));
#276667=CARTESIAN_POINT('Ctrl Pts',(-8.14989708100006,15.2,-6.81036160900002));
#276668=CARTESIAN_POINT('Ctrl Pts',(-8.14989708100006,11.6,-6.81036160900002));
#276669=CARTESIAN_POINT('Ctrl Pts',(-8.14796199500006,15.2,-6.80939156100001));
#276670=CARTESIAN_POINT('Ctrl Pts',(-8.14796199500006,11.6,-6.80939156100001));
#276671=CARTESIAN_POINT('Ctrl Pts',(-8.14603380000005,15.2,-6.80842282100001));
#276672=CARTESIAN_POINT('Ctrl Pts',(-8.14603380000005,11.6,-6.80842282100001));
#276673=CARTESIAN_POINT('Ctrl Pts',(-8.14411250400006,15.2,-6.80745540700002));
#276674=CARTESIAN_POINT('Ctrl Pts',(-8.14411250400006,11.6,-6.80745540700002));
#276675=CARTESIAN_POINT('Ctrl Pts',(-8.14219811500006,15.2,-6.80648933300001));
#276676=CARTESIAN_POINT('Ctrl Pts',(-8.14219811500006,11.6,-6.80648933300001));
#276677=CARTESIAN_POINT('Ctrl Pts',(-8.14029063900006,15.2,-6.80552461600002));
#276678=CARTESIAN_POINT('Ctrl Pts',(-8.14029063900006,11.6,-6.80552461600002));
#276679=CARTESIAN_POINT('Ctrl Pts',(-8.13839008600005,15.2,-6.80456127100002));
#276680=CARTESIAN_POINT('Ctrl Pts',(-8.13839008600005,11.6,-6.80456127100002));
#276681=CARTESIAN_POINT('Ctrl Pts',(-8.13649646400006,15.2,-6.80359931600002));
#276682=CARTESIAN_POINT('Ctrl Pts',(-8.13649646400006,11.6,-6.80359931600002));
#276683=CARTESIAN_POINT('Ctrl Pts',(-8.13460977800006,15.2,-6.80263876500002));
#276684=CARTESIAN_POINT('Ctrl Pts',(-8.13460977800006,11.6,-6.80263876500002));
#276685=CARTESIAN_POINT('Ctrl Pts',(-8.13273003800006,15.2,-6.80167963700002));
#276686=CARTESIAN_POINT('Ctrl Pts',(-8.13273003800006,11.6,-6.80167963700002));
#276687=CARTESIAN_POINT('Ctrl Pts',(-8.13085725300006,15.2,-6.80072194600001));
#276688=CARTESIAN_POINT('Ctrl Pts',(-8.13085725300006,11.6,-6.80072194600001));
#276689=CARTESIAN_POINT('Ctrl Pts',(-8.12899142800006,15.2,-6.79976570900001));
#276690=CARTESIAN_POINT('Ctrl Pts',(-8.12899142800006,11.6,-6.79976570900001));
#276691=CARTESIAN_POINT('Ctrl Pts',(-8.12713257400006,15.2,-6.79881094300002));
#276692=CARTESIAN_POINT('Ctrl Pts',(-8.12713257400006,11.6,-6.79881094300002));
#276693=CARTESIAN_POINT('Ctrl Pts',(-8.12528069700006,15.2,-6.79785766400002));
#276694=CARTESIAN_POINT('Ctrl Pts',(-8.12528069700006,11.6,-6.79785766400002));
#276695=CARTESIAN_POINT('Ctrl Pts',(-8.12343580400006,15.2,-6.79690588900002));
#276696=CARTESIAN_POINT('Ctrl Pts',(-8.12343580400006,11.6,-6.79690588900002));
#276697=CARTESIAN_POINT('Ctrl Pts',(-8.12159790600005,15.2,-6.79595563300002));
#276698=CARTESIAN_POINT('Ctrl Pts',(-8.12159790600005,11.6,-6.79595563300002));
#276699=CARTESIAN_POINT('Ctrl Pts',(-8.11976700800006,15.2,-6.79500691500002));
#276700=CARTESIAN_POINT('Ctrl Pts',(-8.11976700800006,11.6,-6.79500691500002));
#276701=CARTESIAN_POINT('Ctrl Pts',(-8.11794312000006,15.2,-6.79405975100002));
#276702=CARTESIAN_POINT('Ctrl Pts',(-8.11794312000006,11.6,-6.79405975100002));
#276703=CARTESIAN_POINT('Ctrl Pts',(-8.11612624900006,15.2,-6.79311415700001));
#276704=CARTESIAN_POINT('Ctrl Pts',(-8.11612624900006,11.6,-6.79311415700001));
#276705=CARTESIAN_POINT('Ctrl Pts',(-8.11431640400006,15.2,-6.79217015000001));
#276706=CARTESIAN_POINT('Ctrl Pts',(-8.11431640400006,11.6,-6.79217015000001));
#276707=CARTESIAN_POINT('Ctrl Pts',(-8.11251359200006,15.2,-6.79122774800001));
#276708=CARTESIAN_POINT('Ctrl Pts',(-8.11251359200006,11.6,-6.79122774800001));
#276709=CARTESIAN_POINT('Ctrl Pts',(-8.11071782100005,15.2,-6.79028696700002));
#276710=CARTESIAN_POINT('Ctrl Pts',(-8.11071782100005,11.6,-6.79028696700002));
#276711=CARTESIAN_POINT('Ctrl Pts',(-8.10892909900006,15.2,-6.78934782500002));
#276712=CARTESIAN_POINT('Ctrl Pts',(-8.10892909900006,11.6,-6.78934782500002));
#276713=CARTESIAN_POINT('Ctrl Pts',(-8.10714743500006,15.2,-6.78841033800002));
#276714=CARTESIAN_POINT('Ctrl Pts',(-8.10714743500006,11.6,-6.78841033800002));
#276715=CARTESIAN_POINT('Ctrl Pts',(-8.10537283700006,15.2,-6.78747452400002));
#276716=CARTESIAN_POINT('Ctrl Pts',(-8.10537283700006,11.6,-6.78747452400002));
#276717=CARTESIAN_POINT('Ctrl Pts',(-8.10360531200006,15.2,-6.78654039900002));
#276718=CARTESIAN_POINT('Ctrl Pts',(-8.10360531200006,11.6,-6.78654039900002));
#276719=CARTESIAN_POINT('Ctrl Pts',(-8.10184486900006,15.2,-6.78560798200002));
#276720=CARTESIAN_POINT('Ctrl Pts',(-8.10184486900006,11.6,-6.78560798200002));
#276721=CARTESIAN_POINT('Ctrl Pts',(-8.10009151600006,15.2,-6.78467728800002));
#276722=CARTESIAN_POINT('Ctrl Pts',(-8.10009151600006,11.6,-6.78467728800002));
#276723=CARTESIAN_POINT('Ctrl Pts',(-8.09834526200006,15.2,-6.78374833700002));
#276724=CARTESIAN_POINT('Ctrl Pts',(-8.09834526200006,11.6,-6.78374833700002));
#276725=CARTESIAN_POINT('Ctrl Pts',(-8.09660611400006,15.2,-6.78282114600002));
#276726=CARTESIAN_POINT('Ctrl Pts',(-8.09660611400006,11.6,-6.78282114600002));
#276727=CARTESIAN_POINT('Ctrl Pts',(-8.09487408000006,15.2,-6.78189573100001));
#276728=CARTESIAN_POINT('Ctrl Pts',(-8.09487408000006,11.6,-6.78189573100001));
#276729=CARTESIAN_POINT('Ctrl Pts',(-8.09314916900006,15.2,-6.78097211100001));
#276730=CARTESIAN_POINT('Ctrl Pts',(-8.09314916900006,11.6,-6.78097211100001));
#276731=CARTESIAN_POINT('Ctrl Pts',(-8.09143138900006,15.2,-6.78005030300002));
#276732=CARTESIAN_POINT('Ctrl Pts',(-8.09143138900006,11.6,-6.78005030300002));
#276733=CARTESIAN_POINT('Ctrl Pts',(-8.08972074900005,15.2,-6.77913032500002));
#276734=CARTESIAN_POINT('Ctrl Pts',(-8.08972074900005,11.6,-6.77913032500002));
#276735=CARTESIAN_POINT('Ctrl Pts',(-8.08801725500006,15.2,-6.77821219500002));
#276736=CARTESIAN_POINT('Ctrl Pts',(-8.08801725500006,11.6,-6.77821219500002));
#276737=CARTESIAN_POINT('Ctrl Pts',(-8.08632091900006,15.2,-6.77729593100001));
#276738=CARTESIAN_POINT('Ctrl Pts',(-8.08632091900006,11.6,-6.77729593100001));
#276739=CARTESIAN_POINT('Ctrl Pts',(-8.08463174500006,15.2,-6.77638154900002));
#276740=CARTESIAN_POINT('Ctrl Pts',(-8.08463174500006,11.6,-6.77638154900002));
#276741=CARTESIAN_POINT('Ctrl Pts',(-8.08294974400006,15.2,-6.77546907100002));
#276742=CARTESIAN_POINT('Ctrl Pts',(-8.08294974400006,11.6,-6.77546907100002));
#276743=CARTESIAN_POINT('Ctrl Pts',(-8.08127492400006,15.2,-6.77455851200002));
#276744=CARTESIAN_POINT('Ctrl Pts',(-8.08127492400006,11.6,-6.77455851200002));
#276745=CARTESIAN_POINT('Ctrl Pts',(-8.07960729300006,15.2,-6.77364988900001));
#276746=CARTESIAN_POINT('Ctrl Pts',(-8.07960729300006,11.6,-6.77364988900001));
#276747=CARTESIAN_POINT('Ctrl Pts',(-8.07794685900006,15.2,-6.77274322400002));
#276748=CARTESIAN_POINT('Ctrl Pts',(-8.07794685900006,11.6,-6.77274322400002));
#276749=CARTESIAN_POINT('Ctrl Pts',(-8.07629363200006,15.2,-6.77183853400001));
#276750=CARTESIAN_POINT('Ctrl Pts',(-8.07629363200006,11.6,-6.77183853400001));
#276751=CARTESIAN_POINT('Ctrl Pts',(-8.07464761900006,15.2,-6.77093583600002));
#276752=CARTESIAN_POINT('Ctrl Pts',(-8.07464761900006,11.6,-6.77093583600002));
#276753=CARTESIAN_POINT('Ctrl Pts',(-8.07300882800006,15.2,-6.77003514800001));
#276754=CARTESIAN_POINT('Ctrl Pts',(-8.07300882800006,11.6,-6.77003514800001));
#276755=CARTESIAN_POINT('Ctrl Pts',(-8.07137726900006,15.2,-6.76913649000002));
#276756=CARTESIAN_POINT('Ctrl Pts',(-8.07137726900006,11.6,-6.76913649000002));
#276757=CARTESIAN_POINT('Ctrl Pts',(-8.06975294900005,15.2,-6.76823988100002));
#276758=CARTESIAN_POINT('Ctrl Pts',(-8.06975294900005,11.6,-6.76823988100002));
#276759=CARTESIAN_POINT('Ctrl Pts',(-8.06813587700006,15.2,-6.76734533800002));
#276760=CARTESIAN_POINT('Ctrl Pts',(-8.06813587700006,11.6,-6.76734533800002));
#276761=CARTESIAN_POINT('Ctrl Pts',(-8.06652606200006,15.2,-6.76645288100002));
#276762=CARTESIAN_POINT('Ctrl Pts',(-8.06652606200006,11.6,-6.76645288100002));
#276763=CARTESIAN_POINT('Ctrl Pts',(-8.06492351200006,15.2,-6.76556252900002));
#276764=CARTESIAN_POINT('Ctrl Pts',(-8.06492351200006,11.6,-6.76556252900002));
#276765=CARTESIAN_POINT('Ctrl Pts',(-8.06332823500006,15.2,-6.76467429900002));
#276766=CARTESIAN_POINT('Ctrl Pts',(-8.06332823500006,11.6,-6.76467429900002));
#276767=CARTESIAN_POINT('Ctrl Pts',(-8.06174024100006,15.2,-6.76378821200001));
#276768=CARTESIAN_POINT('Ctrl Pts',(-8.06174024100006,11.6,-6.76378821200001));
#276769=CARTESIAN_POINT('Ctrl Pts',(-8.06015953800006,15.2,-6.76290428500002));
#276770=CARTESIAN_POINT('Ctrl Pts',(-8.06015953800006,11.6,-6.76290428500002));
#276771=CARTESIAN_POINT('Ctrl Pts',(-8.05858613400006,15.2,-6.76202254000002));
#276772=CARTESIAN_POINT('Ctrl Pts',(-8.05858613400006,11.6,-6.76202254000002));
#276773=CARTESIAN_POINT('Ctrl Pts',(-8.05702003900005,15.2,-6.76114299200002));
#276774=CARTESIAN_POINT('Ctrl Pts',(-8.05702003900005,11.6,-6.76114299200002));
#276775=CARTESIAN_POINT('Ctrl Pts',(-8.05546126000005,15.2,-6.76026566400001));
#276776=CARTESIAN_POINT('Ctrl Pts',(-8.05546126000005,11.6,-6.76026566400001));
#276777=CARTESIAN_POINT('Ctrl Pts',(-8.05390980500006,15.2,-6.75939057400001));
#276778=CARTESIAN_POINT('Ctrl Pts',(-8.05390980500006,11.6,-6.75939057400001));
#276779=CARTESIAN_POINT('Ctrl Pts',(-8.05236568500005,15.2,-6.75851774000002));
#276780=CARTESIAN_POINT('Ctrl Pts',(-8.05236568500005,11.6,-6.75851774000002));
#276781=CARTESIAN_POINT('Ctrl Pts',(-8.05082890800006,15.2,-6.75764718400002));
#276782=CARTESIAN_POINT('Ctrl Pts',(-8.05082890800006,11.6,-6.75764718400002));
#276783=CARTESIAN_POINT('Ctrl Pts',(-8.04929948200006,15.2,-6.75677892300002));
#276784=CARTESIAN_POINT('Ctrl Pts',(-8.04929948200006,11.6,-6.75677892300002));
#276785=CARTESIAN_POINT('Ctrl Pts',(-8.04777741600006,15.2,-6.75591297900001));
#276786=CARTESIAN_POINT('Ctrl Pts',(-8.04777741600006,11.6,-6.75591297900001));
#276787=CARTESIAN_POINT('Ctrl Pts',(-8.04626271900006,15.2,-6.75504936900002));
#276788=CARTESIAN_POINT('Ctrl Pts',(-8.04626271900006,11.6,-6.75504936900002));
#276789=CARTESIAN_POINT('Ctrl Pts',(-8.04475540000006,15.2,-6.75418811400001));
#276790=CARTESIAN_POINT('Ctrl Pts',(-8.04475540000006,11.6,-6.75418811400001));
#276791=CARTESIAN_POINT('Ctrl Pts',(-8.04325546700005,15.2,-6.75332923500001));
#276792=CARTESIAN_POINT('Ctrl Pts',(-8.04325546700005,11.6,-6.75332923500001));
#276793=CARTESIAN_POINT('Ctrl Pts',(-8.04176292900006,15.2,-6.75247275100002));
#276794=CARTESIAN_POINT('Ctrl Pts',(-8.04176292900006,11.6,-6.75247275100002));
#276795=CARTESIAN_POINT('Ctrl Pts',(-8.04027779600006,15.2,-6.75161868200002));
#276796=CARTESIAN_POINT('Ctrl Pts',(-8.04027779600006,11.6,-6.75161868200002));
#276797=CARTESIAN_POINT('Ctrl Pts',(-8.03880007500006,15.2,-6.75076704800002));
#276798=CARTESIAN_POINT('Ctrl Pts',(-8.03880007500006,11.6,-6.75076704800002));
#276799=CARTESIAN_POINT('Ctrl Pts',(-8.03732977700006,15.2,-6.74991786800001));
#276800=CARTESIAN_POINT('Ctrl Pts',(-8.03732977700006,11.6,-6.74991786800001));
#276801=CARTESIAN_POINT('Ctrl Pts',(-8.03586690900006,15.2,-6.74907116500002));
#276802=CARTESIAN_POINT('Ctrl Pts',(-8.03586690900006,11.6,-6.74907116500002));
#276803=CARTESIAN_POINT('Ctrl Pts',(-8.03441148100006,15.2,-6.74822695700002));
#276804=CARTESIAN_POINT('Ctrl Pts',(-8.03441148100006,11.6,-6.74822695700002));
#276805=CARTESIAN_POINT('Ctrl Pts',(-8.03296350200006,15.2,-6.74738526600001));
#276806=CARTESIAN_POINT('Ctrl Pts',(-8.03296350200006,11.6,-6.74738526600001));
#276807=CARTESIAN_POINT('Ctrl Pts',(-8.03152298000006,15.2,-6.74654611000002));
#276808=CARTESIAN_POINT('Ctrl Pts',(-8.03152298000006,11.6,-6.74654611000002));
#276809=CARTESIAN_POINT('Ctrl Pts',(-8.03008992500006,15.2,-6.74570951200002));
#276810=CARTESIAN_POINT('Ctrl Pts',(-8.03008992500006,11.6,-6.74570951200002));
#276811=CARTESIAN_POINT('Ctrl Pts',(-8.02866434500006,15.2,-6.74487549200002));
#276812=CARTESIAN_POINT('Ctrl Pts',(-8.02866434500006,11.6,-6.74487549200002));
#276813=CARTESIAN_POINT('Ctrl Pts',(-8.02724625000005,15.2,-6.74404407000001));
#276814=CARTESIAN_POINT('Ctrl Pts',(-8.02724625000005,11.6,-6.74404407000001));
#276815=CARTESIAN_POINT('Ctrl Pts',(-8.02583565000005,15.2,-6.74321526700002));
#276816=CARTESIAN_POINT('Ctrl Pts',(-8.02583565000005,11.6,-6.74321526700002));
#276817=CARTESIAN_POINT('Ctrl Pts',(-8.02443255200006,15.2,-6.74238910500002));
#276818=CARTESIAN_POINT('Ctrl Pts',(-8.02443255200006,11.6,-6.74238910500002));
#276819=CARTESIAN_POINT('Ctrl Pts',(-8.02303696600006,15.2,-6.74156560400001));
#276820=CARTESIAN_POINT('Ctrl Pts',(-8.02303696600006,11.6,-6.74156560400001));
#276821=CARTESIAN_POINT('Ctrl Pts',(-8.02164890100006,15.2,-6.74074478500001));
#276822=CARTESIAN_POINT('Ctrl Pts',(-8.02164890100006,11.6,-6.74074478500001));
#276823=CARTESIAN_POINT('Ctrl Pts',(-8.02026836500006,15.2,-6.73992667000002));
#276824=CARTESIAN_POINT('Ctrl Pts',(-8.02026836500006,11.6,-6.73992667000002));
#276825=CARTESIAN_POINT('Ctrl Pts',(-8.01889537100006,15.2,-6.73911127900002));
#276826=CARTESIAN_POINT('Ctrl Pts',(-8.01889537100006,11.6,-6.73911127900002));
#276827=CARTESIAN_POINT('Ctrl Pts',(-8.01752992300005,15.2,-6.73829863500002));
#276828=CARTESIAN_POINT('Ctrl Pts',(-8.01752992300005,11.6,-6.73829863500002));
#276829=CARTESIAN_POINT('Ctrl Pts',(-8.01617203400006,15.2,-6.73748875800002));
#276830=CARTESIAN_POINT('Ctrl Pts',(-8.01617203400006,11.6,-6.73748875800002));
#276831=CARTESIAN_POINT('Ctrl Pts',(-8.01482171200006,15.2,-6.73668166900002));
#276832=CARTESIAN_POINT('Ctrl Pts',(-8.01482171200006,11.6,-6.73668166900002));
#276833=CARTESIAN_POINT('Ctrl Pts',(-8.01347896700005,15.2,-6.73587739300002));
#276834=CARTESIAN_POINT('Ctrl Pts',(-8.01347896700005,11.6,-6.73587739300002));
#276835=CARTESIAN_POINT('Ctrl Pts',(-8.01214380700005,15.2,-6.73507594700002));
#276836=CARTESIAN_POINT('Ctrl Pts',(-8.01214380700005,11.6,-6.73507594700002));
#276837=CARTESIAN_POINT('Ctrl Pts',(-8.01081624200006,15.2,-6.73427735600002));
#276838=CARTESIAN_POINT('Ctrl Pts',(-8.01081624200006,11.6,-6.73427735600002));
#276839=CARTESIAN_POINT('Ctrl Pts',(-8.00949628200006,15.2,-6.73348164200001));
#276840=CARTESIAN_POINT('Ctrl Pts',(-8.00949628200006,11.6,-6.73348164200001));
#276841=CARTESIAN_POINT('Ctrl Pts',(-8.00818393600006,15.2,-6.73268882500001));
#276842=CARTESIAN_POINT('Ctrl Pts',(-8.00818393600006,11.6,-6.73268882500001));
#276843=CARTESIAN_POINT('Ctrl Pts',(-8.00687921200005,15.2,-6.73189892800002));
#276844=CARTESIAN_POINT('Ctrl Pts',(-8.00687921200005,11.6,-6.73189892800002));
#276845=CARTESIAN_POINT('Ctrl Pts',(-8.00558212100006,15.2,-6.73111197200001));
#276846=CARTESIAN_POINT('Ctrl Pts',(-8.00558212100006,11.6,-6.73111197200001));
#276847=CARTESIAN_POINT('Ctrl Pts',(-8.00429267200006,15.2,-6.73032798200002));
#276848=CARTESIAN_POINT('Ctrl Pts',(-8.00429267200006,11.6,-6.73032798200002));
#276849=CARTESIAN_POINT('Ctrl Pts',(-8.00301087500005,15.2,-6.72954697800002));
#276850=CARTESIAN_POINT('Ctrl Pts',(-8.00301087500005,11.6,-6.72954697800002));
#276851=CARTESIAN_POINT('Ctrl Pts',(-8.00173673800006,15.2,-6.72876898400002));
#276852=CARTESIAN_POINT('Ctrl Pts',(-8.00173673800006,11.6,-6.72876898400002));
#276853=CARTESIAN_POINT('Ctrl Pts',(-8.00047027300005,15.2,-6.72799402200001));
#276854=CARTESIAN_POINT('Ctrl Pts',(-8.00047027300005,11.6,-6.72799402200001));
#276855=CARTESIAN_POINT('Ctrl Pts',(-7.99921148700006,15.2,-6.72722211400002));
#276856=CARTESIAN_POINT('Ctrl Pts',(-7.99921148700006,11.6,-6.72722211400002));
#276857=CARTESIAN_POINT('Ctrl Pts',(-7.99796039100006,15.2,-6.72645328300002));
#276858=CARTESIAN_POINT('Ctrl Pts',(-7.99796039100006,11.6,-6.72645328300002));
#276859=CARTESIAN_POINT('Ctrl Pts',(-7.99671699500006,15.2,-6.72568755200002));
#276860=CARTESIAN_POINT('Ctrl Pts',(-7.99671699500006,11.6,-6.72568755200002));
#276861=CARTESIAN_POINT('Ctrl Pts',(-7.99548130800006,15.2,-6.72492494400001));
#276862=CARTESIAN_POINT('Ctrl Pts',(-7.99548130800006,11.6,-6.72492494400001));
#276863=CARTESIAN_POINT('Ctrl Pts',(-7.99425333800006,15.2,-6.72416548300002));
#276864=CARTESIAN_POINT('Ctrl Pts',(-7.99425333800006,11.6,-6.72416548300002));
#276865=CARTESIAN_POINT('Ctrl Pts',(-7.99303309800005,15.2,-6.72340919000002));
#276866=CARTESIAN_POINT('Ctrl Pts',(-7.99303309800005,11.6,-6.72340919000002));
#276867=CARTESIAN_POINT('Ctrl Pts',(-7.99182059500006,15.2,-6.72265608900001));
#276868=CARTESIAN_POINT('Ctrl Pts',(-7.99182059500006,11.6,-6.72265608900001));
#276869=CARTESIAN_POINT('Ctrl Pts',(-7.99061584100006,15.2,-6.72190620500002));
#276870=CARTESIAN_POINT('Ctrl Pts',(-7.99061584100006,11.6,-6.72190620500002));
#276871=CARTESIAN_POINT('Ctrl Pts',(-7.98941884300006,15.2,-6.72115955900002));
#276872=CARTESIAN_POINT('Ctrl Pts',(-7.98941884300006,11.6,-6.72115955900002));
#276873=CARTESIAN_POINT('Ctrl Pts',(-7.98822961400005,15.2,-6.72041617700001));
#276874=CARTESIAN_POINT('Ctrl Pts',(-7.98822961400005,11.6,-6.72041617700001));
#276875=CARTESIAN_POINT('Ctrl Pts',(-7.98704816100006,15.2,-6.71967608000001));
#276876=CARTESIAN_POINT('Ctrl Pts',(-7.98704816100006,11.6,-6.71967608000001));
#276877=CARTESIAN_POINT('Ctrl Pts',(-7.98587449600006,15.2,-6.71893929400002));
#276878=CARTESIAN_POINT('Ctrl Pts',(-7.98587449600006,11.6,-6.71893929400002));
#276879=CARTESIAN_POINT('Ctrl Pts',(-7.98470862800006,15.2,-6.71820584100002));
#276880=CARTESIAN_POINT('Ctrl Pts',(-7.98470862800006,11.6,-6.71820584100002));
#276881=CARTESIAN_POINT('Ctrl Pts',(-7.98355056700006,15.2,-6.71747574700002));
#276882=CARTESIAN_POINT('Ctrl Pts',(-7.98355056700006,11.6,-6.71747574700002));
#276883=CARTESIAN_POINT('Ctrl Pts',(-7.98240032200006,15.2,-6.71674903500002));
#276884=CARTESIAN_POINT('Ctrl Pts',(-7.98240032200006,11.6,-6.71674903500002));
#276885=CARTESIAN_POINT('Ctrl Pts',(-7.98125790500006,15.2,-6.71602572900002));
#276886=CARTESIAN_POINT('Ctrl Pts',(-7.98125790500006,11.6,-6.71602572900002));
#276887=CARTESIAN_POINT('Ctrl Pts',(-7.98012332400006,15.2,-6.71530585300002));
#276888=CARTESIAN_POINT('Ctrl Pts',(-7.98012332400006,11.6,-6.71530585300002));
#276889=CARTESIAN_POINT('Ctrl Pts',(-7.97899659000005,15.2,-6.71458943300002));
#276890=CARTESIAN_POINT('Ctrl Pts',(-7.97899659000005,11.6,-6.71458943300002));
#276891=CARTESIAN_POINT('Ctrl Pts',(-7.97787771400006,15.2,-6.71387649200001));
#276892=CARTESIAN_POINT('Ctrl Pts',(-7.97787771400006,11.6,-6.71387649200001));
#276893=CARTESIAN_POINT('Ctrl Pts',(-7.97676670400006,15.2,-6.71316705500002));
#276894=CARTESIAN_POINT('Ctrl Pts',(-7.97676670400006,11.6,-6.71316705500002));
#276895=CARTESIAN_POINT('Ctrl Pts',(-7.97566357200005,15.2,-6.71246114600001));
#276896=CARTESIAN_POINT('Ctrl Pts',(-7.97566357200005,11.6,-6.71246114600001));
#276897=CARTESIAN_POINT('Ctrl Pts',(-7.97456832700006,15.2,-6.71175879200002));
#276898=CARTESIAN_POINT('Ctrl Pts',(-7.97456832700006,11.6,-6.71175879200002));
#276899=CARTESIAN_POINT('Ctrl Pts',(-7.97348098000005,15.2,-6.71106001600001));
#276900=CARTESIAN_POINT('Ctrl Pts',(-7.97348098000005,11.6,-6.71106001600001));
#276901=CARTESIAN_POINT('Ctrl Pts',(-7.97240154100006,15.2,-6.71036484500001));
#276902=CARTESIAN_POINT('Ctrl Pts',(-7.97240154100006,11.6,-6.71036484500001));
#276903=CARTESIAN_POINT('Ctrl Pts',(-7.97133002000006,15.2,-6.70967330200002));
#276904=CARTESIAN_POINT('Ctrl Pts',(-7.97133002000006,11.6,-6.70967330200002));
#276905=CARTESIAN_POINT('Ctrl Pts',(-7.97026642700006,15.2,-6.70898541300001));
#276906=CARTESIAN_POINT('Ctrl Pts',(-7.97026642700006,11.6,-6.70898541300001));
#276907=CARTESIAN_POINT('Ctrl Pts',(-7.96921077400006,15.2,-6.70830120300002));
#276908=CARTESIAN_POINT('Ctrl Pts',(-7.96921077400006,11.6,-6.70830120300002));
#276909=CARTESIAN_POINT('Ctrl Pts',(-7.96816307000006,15.2,-6.70762070000002));
#276910=CARTESIAN_POINT('Ctrl Pts',(-7.96816307000006,11.6,-6.70762070000002));
#276911=CARTESIAN_POINT('Ctrl Pts',(-7.96712332500006,15.2,-6.70694392700002));
#276912=CARTESIAN_POINT('Ctrl Pts',(-7.96712332500006,11.6,-6.70694392700002));
#276913=CARTESIAN_POINT('Ctrl Pts',(-7.96609155000005,15.2,-6.70627091100001));
#276914=CARTESIAN_POINT('Ctrl Pts',(-7.96609155000005,11.6,-6.70627091100001));
#276915=CARTESIAN_POINT('Ctrl Pts',(-7.96506775600006,15.2,-6.70560167700001));
#276916=CARTESIAN_POINT('Ctrl Pts',(-7.96506775600006,11.6,-6.70560167700001));
#276917=CARTESIAN_POINT('Ctrl Pts',(-7.96405195200006,15.2,-6.70493625300002));
#276918=CARTESIAN_POINT('Ctrl Pts',(-7.96405195200006,11.6,-6.70493625300002));
#276919=CARTESIAN_POINT('Ctrl Pts',(-7.96304415000006,15.2,-6.70427466300002));
#276920=CARTESIAN_POINT('Ctrl Pts',(-7.96304415000006,11.6,-6.70427466300002));
#276921=CARTESIAN_POINT('Ctrl Pts',(-7.96204436100006,15.2,-6.70361693500002));
#276922=CARTESIAN_POINT('Ctrl Pts',(-7.96204436100006,11.6,-6.70361693500002));
#276923=CARTESIAN_POINT('Ctrl Pts',(-7.96105259400005,15.2,-6.70296309300002));
#276924=CARTESIAN_POINT('Ctrl Pts',(-7.96105259400005,11.6,-6.70296309300002));
#276925=CARTESIAN_POINT('Ctrl Pts',(-7.96006886100006,15.2,-6.70231316600002));
#276926=CARTESIAN_POINT('Ctrl Pts',(-7.96006886100006,11.6,-6.70231316600002));
#276927=CARTESIAN_POINT('Ctrl Pts',(-7.95909317200006,15.2,-6.70166718000001));
#276928=CARTESIAN_POINT('Ctrl Pts',(-7.95909317200006,11.6,-6.70166718000001));
#276929=CARTESIAN_POINT('Ctrl Pts',(-7.95812553700006,15.2,-6.70102516100001));
#276930=CARTESIAN_POINT('Ctrl Pts',(-7.95812553700006,11.6,-6.70102516100001));
#276931=CARTESIAN_POINT('Ctrl Pts',(-7.95716596800006,15.2,-6.70038713600002));
#276932=CARTESIAN_POINT('Ctrl Pts',(-7.95716596800006,11.6,-6.70038713600002));
#276933=CARTESIAN_POINT('Ctrl Pts',(-7.95621447600006,15.2,-6.69975313400001));
#276934=CARTESIAN_POINT('Ctrl Pts',(-7.95621447600006,11.6,-6.69975313400001));
#276935=CARTESIAN_POINT('Ctrl Pts',(-7.95527107000006,15.2,-6.69912317900001));
#276936=CARTESIAN_POINT('Ctrl Pts',(-7.95527107000006,11.6,-6.69912317900001));
#276937=CARTESIAN_POINT('Ctrl Pts',(-7.95433576200006,15.2,-6.69849730100001));
#276938=CARTESIAN_POINT('Ctrl Pts',(-7.95433576200006,11.6,-6.69849730100001));
#276939=CARTESIAN_POINT('Ctrl Pts',(-7.95340856400006,15.2,-6.69787552700001));
#276940=CARTESIAN_POINT('Ctrl Pts',(-7.95340856400006,11.6,-6.69787552700001));
#276941=CARTESIAN_POINT('Ctrl Pts',(-7.95248948500006,15.2,-6.69725788300001));
#276942=CARTESIAN_POINT('Ctrl Pts',(-7.95248948500006,11.6,-6.69725788300001));
#276943=CARTESIAN_POINT('Ctrl Pts',(-7.95157853800006,15.2,-6.69664439800002));
#276944=CARTESIAN_POINT('Ctrl Pts',(-7.95157853800006,11.6,-6.69664439800002));
#276945=CARTESIAN_POINT('Ctrl Pts',(-7.95067573200006,15.2,-6.69603510000002));
#276946=CARTESIAN_POINT('Ctrl Pts',(-7.95067573200006,11.6,-6.69603510000002));
#276947=CARTESIAN_POINT('Ctrl Pts',(-7.94978107900006,15.2,-6.69543001700001));
#276948=CARTESIAN_POINT('Ctrl Pts',(-7.94978107900006,11.6,-6.69543001700001));
#276949=CARTESIAN_POINT('Ctrl Pts',(-7.94889459000006,15.2,-6.69482917500002));
#276950=CARTESIAN_POINT('Ctrl Pts',(-7.94889459000006,11.6,-6.69482917500002));
#276951=CARTESIAN_POINT('Ctrl Pts',(-7.94801627800006,15.2,-6.69423260500002));
#276952=CARTESIAN_POINT('Ctrl Pts',(-7.94801627800006,11.6,-6.69423260500002));
#276953=CARTESIAN_POINT('Ctrl Pts',(-7.94714615000006,15.2,-6.69364033500001));
#276954=CARTESIAN_POINT('Ctrl Pts',(-7.94714615000006,11.6,-6.69364033500001));
#276955=CARTESIAN_POINT('Ctrl Pts',(-7.94628422000006,15.2,-6.69305239200002));
#276956=CARTESIAN_POINT('Ctrl Pts',(-7.94628422000006,11.6,-6.69305239200002));
#276957=CARTESIAN_POINT('Ctrl Pts',(-7.94543050000006,15.2,-6.69246880700002));
#276958=CARTESIAN_POINT('Ctrl Pts',(-7.94543050000006,11.6,-6.69246880700002));
#276959=CARTESIAN_POINT('Ctrl Pts',(-7.94458499900006,15.2,-6.69188960600002));
#276960=CARTESIAN_POINT('Ctrl Pts',(-7.94458499900006,11.6,-6.69188960600002));
#276961=CARTESIAN_POINT('Ctrl Pts',(-7.94374773100006,15.2,-6.69131482000001));
#276962=CARTESIAN_POINT('Ctrl Pts',(-7.94374773100006,11.6,-6.69131482000001));
#276963=CARTESIAN_POINT('Ctrl Pts',(-7.94291870400006,15.2,-6.69074447800002));
#276964=CARTESIAN_POINT('Ctrl Pts',(-7.94291870400006,11.6,-6.69074447800002));
#276965=CARTESIAN_POINT('Ctrl Pts',(-7.94209793300006,15.2,-6.69017860900002));
#276966=CARTESIAN_POINT('Ctrl Pts',(-7.94209793300006,11.6,-6.69017860900002));
#276967=CARTESIAN_POINT('Ctrl Pts',(-7.94128542700006,15.2,-6.68961724100001));
#276968=CARTESIAN_POINT('Ctrl Pts',(-7.94128542700006,11.6,-6.68961724100001));
#276969=CARTESIAN_POINT('Ctrl Pts',(-7.94048119900006,15.2,-6.68906040700002));
#276970=CARTESIAN_POINT('Ctrl Pts',(-7.94048119900006,11.6,-6.68906040700002));
#276971=CARTESIAN_POINT('Ctrl Pts',(-7.93968525900006,15.2,-6.68850813300002));
#276972=CARTESIAN_POINT('Ctrl Pts',(-7.93968525900006,11.6,-6.68850813300002));
#276973=CARTESIAN_POINT('Ctrl Pts',(-7.93889762000005,15.2,-6.68796045200001));
#276974=CARTESIAN_POINT('Ctrl Pts',(-7.93889762000005,11.6,-6.68796045200001));
#276975=CARTESIAN_POINT('Ctrl Pts',(-7.93811829300005,15.2,-6.68741739000002));
#276976=CARTESIAN_POINT('Ctrl Pts',(-7.93811829300005,11.6,-6.68741739000002));
#276977=CARTESIAN_POINT('Ctrl Pts',(-7.93734729000006,15.2,-6.68687898200002));
#276978=CARTESIAN_POINT('Ctrl Pts',(-7.93734729000006,11.6,-6.68687898200002));
#276979=CARTESIAN_POINT('Ctrl Pts',(-7.93658462200005,15.2,-6.68634525500002));
#276980=CARTESIAN_POINT('Ctrl Pts',(-7.93658462200005,11.6,-6.68634525500002));
#276981=CARTESIAN_POINT('Ctrl Pts',(-7.93583464600006,15.2,-6.68581928800001));
#276982=CARTESIAN_POINT('Ctrl Pts',(-7.93583464600006,11.6,-6.68581928800001));
#276983=CARTESIAN_POINT('Ctrl Pts',(-7.93524212700006,15.2,-6.68540286400002));
#276984=CARTESIAN_POINT('Ctrl Pts',(-7.93524212700006,11.6,-6.68540286400002));
#276985=CARTESIAN_POINT('Ctrl Pts',(-7.93480250500006,15.2,-6.68509340800002));
#276986=CARTESIAN_POINT('Ctrl Pts',(-7.93480250500006,11.6,-6.68509340800002));
#276987=CARTESIAN_POINT('Ctrl Pts',(-7.93451247300006,15.2,-6.68488903500001));
#276988=CARTESIAN_POINT('Ctrl Pts',(-7.93451247300006,11.6,-6.68488903500001));
#276989=CARTESIAN_POINT('Ctrl Pts',(-7.93436997000006,15.2,-6.68478856700002));
#276990=CARTESIAN_POINT('Ctrl Pts',(-7.93436997000006,11.6,-6.68478856700002));
#276991=CARTESIAN_POINT('',(-7.93436997000006,12.2,-6.68478856700002));
#276992=CARTESIAN_POINT('',(-7.93436997000006,15.2,-6.68478856700002));
#276993=CARTESIAN_POINT('',(-7.93436997000006,12.2,-6.68478856700002));
#276994=CARTESIAN_POINT('Ctrl Pts',(-9.03946594400006,12.2,-7.10901226900001));
#276995=CARTESIAN_POINT('Ctrl Pts',(-9.03871859600006,12.2,-7.10885083600001));
#276996=CARTESIAN_POINT('Ctrl Pts',(-9.03722439200006,12.2,-7.10852778400002));
#276997=CARTESIAN_POINT('Ctrl Pts',(-9.03498456200006,12.2,-7.10804263900001));
#276998=CARTESIAN_POINT('Ctrl Pts',(-9.03200107200006,12.2,-7.10739465100002));
#276999=CARTESIAN_POINT('Ctrl Pts',(-9.02827662900006,12.2,-7.10658278400001));
#277000=CARTESIAN_POINT('Ctrl Pts',(-9.02455710700006,12.2,-7.10576903500002));
#277001=CARTESIAN_POINT('Ctrl Pts',(-9.02084250600005,12.2,-7.10495340800002));
#277002=CARTESIAN_POINT('Ctrl Pts',(-9.01713282900005,12.2,-7.10413590400002));
#277003=CARTESIAN_POINT('Ctrl Pts',(-9.01342808000006,12.2,-7.10331652800001));
#277004=CARTESIAN_POINT('Ctrl Pts',(-9.00972826500006,12.2,-7.10249528800002));
#277005=CARTESIAN_POINT('Ctrl Pts',(-9.00603338900006,12.2,-7.10167218900001));
#277006=CARTESIAN_POINT('Ctrl Pts',(-9.00234345900006,12.2,-7.10084724000002));
#277007=CARTESIAN_POINT('Ctrl Pts',(-8.99865848200006,12.2,-7.10002045100002));
#277008=CARTESIAN_POINT('Ctrl Pts',(-8.99497846500006,12.2,-7.09919182900002));
#277009=CARTESIAN_POINT('Ctrl Pts',(-8.99130341600006,12.2,-7.09836138400001));
#277010=CARTESIAN_POINT('Ctrl Pts',(-8.98763333900006,12.2,-7.09752912300001));
#277011=CARTESIAN_POINT('Ctrl Pts',(-8.98396824000006,12.2,-7.09669505000001));
#277012=CARTESIAN_POINT('Ctrl Pts',(-8.98030812400006,12.2,-7.09585917500001));
#277013=CARTESIAN_POINT('Ctrl Pts',(-8.97665299700006,12.2,-7.09502150300001));
#277014=CARTESIAN_POINT('Ctrl Pts',(-8.97300286400006,12.2,-7.09418203900002));
#277015=CARTESIAN_POINT('Ctrl Pts',(-8.96935772900006,12.2,-7.09334079100002));
#277016=CARTESIAN_POINT('Ctrl Pts',(-8.96571759800005,12.2,-7.09249776700001));
#277017=CARTESIAN_POINT('Ctrl Pts',(-8.96208247800006,12.2,-7.09165297200002));
#277018=CARTESIAN_POINT('Ctrl Pts',(-8.95845237400006,12.2,-7.09080641500002));
#277019=CARTESIAN_POINT('Ctrl Pts',(-8.95482729200006,12.2,-7.08995810200002));
#277020=CARTESIAN_POINT('Ctrl Pts',(-8.95120723800006,12.2,-7.08910804300002));
#277021=CARTESIAN_POINT('Ctrl Pts',(-8.94759221900006,12.2,-7.08825624300002));
#277022=CARTESIAN_POINT('Ctrl Pts',(-8.94398223900006,12.2,-7.08740271100002));
#277023=CARTESIAN_POINT('Ctrl Pts',(-8.94037730400006,12.2,-7.08654745200001));
#277024=CARTESIAN_POINT('Ctrl Pts',(-8.93677742100006,12.2,-7.08569047400001));
#277025=CARTESIAN_POINT('Ctrl Pts',(-8.93318259400005,12.2,-7.08483178600002));
#277026=CARTESIAN_POINT('Ctrl Pts',(-8.92959282900006,12.2,-7.08397139300001));
#277027=CARTESIAN_POINT('Ctrl Pts',(-8.92600813200006,12.2,-7.08310930200001));
#277028=CARTESIAN_POINT('Ctrl Pts',(-8.92242850800006,12.2,-7.08224552100001));
#277029=CARTESIAN_POINT('Ctrl Pts',(-8.91885396500006,12.2,-7.08138005800001));
#277030=CARTESIAN_POINT('Ctrl Pts',(-8.91528450600006,12.2,-7.08051292100001));
#277031=CARTESIAN_POINT('Ctrl Pts',(-8.91172013800006,12.2,-7.07964411500001));
#277032=CARTESIAN_POINT('Ctrl Pts',(-8.90816086700006,12.2,-7.07877364900002));
#277033=CARTESIAN_POINT('Ctrl Pts',(-8.90460669800006,12.2,-7.07790152900002));
#277034=CARTESIAN_POINT('Ctrl Pts',(-8.90105763800005,12.2,-7.07702776600001));
#277035=CARTESIAN_POINT('Ctrl Pts',(-8.89751369200006,12.2,-7.07615236300001));
#277036=CARTESIAN_POINT('Ctrl Pts',(-8.89397486600006,12.2,-7.07527533000002));
#277037=CARTESIAN_POINT('Ctrl Pts',(-8.89044116400006,12.2,-7.07439667400001));
#277038=CARTESIAN_POINT('Ctrl Pts',(-8.88691259400006,12.2,-7.07351640200002));
#277039=CARTESIAN_POINT('Ctrl Pts',(-8.88338916200006,12.2,-7.07263452100002));
#277040=CARTESIAN_POINT('Ctrl Pts',(-8.87987087300005,12.2,-7.07175104100001));
#277041=CARTESIAN_POINT('Ctrl Pts',(-8.87635773200006,12.2,-7.07086596600002));
#277042=CARTESIAN_POINT('Ctrl Pts',(-8.87284974500006,12.2,-7.06997930700001));
#277043=CARTESIAN_POINT('Ctrl Pts',(-8.86934691800005,12.2,-7.06909107000002));
#277044=CARTESIAN_POINT('Ctrl Pts',(-8.86584925900006,12.2,-7.06820126200002));
#277045=CARTESIAN_POINT('Ctrl Pts',(-8.86235677000006,12.2,-7.06730989100001));
#277046=CARTESIAN_POINT('Ctrl Pts',(-8.85886945900005,12.2,-7.06641696400002));
#277047=CARTESIAN_POINT('Ctrl Pts',(-8.85538733200006,12.2,-7.06552249100002));
#277048=CARTESIAN_POINT('Ctrl Pts',(-8.85191039400006,12.2,-7.06462647700001));
#277049=CARTESIAN_POINT('Ctrl Pts',(-8.84843865100006,12.2,-7.06372893100002));
#277050=CARTESIAN_POINT('Ctrl Pts',(-8.84497210900006,12.2,-7.06282986200002));
#277051=CARTESIAN_POINT('Ctrl Pts',(-8.84151077400006,12.2,-7.06192927400001));
#277052=CARTESIAN_POINT('Ctrl Pts',(-8.83805465100006,12.2,-7.06102717900002));
#277053=CARTESIAN_POINT('Ctrl Pts',(-8.83391356635052,12.2,-7.05994286263941));
#277054=CARTESIAN_POINT('Ctrl Pts',(-8.82978031732483,12.2,-7.05885630368031));
#277055=CARTESIAN_POINT('Ctrl Pts',(-8.82565491667528,12.2,-7.05776752231972));
#277056=CARTESIAN_POINT('Ctrl Pts',(-8.82153737602361,12.2,-7.05667653245971));
#277057=CARTESIAN_POINT('Ctrl Pts',(-8.81742770700006,12.2,-7.05558334800001));
#277058=CARTESIAN_POINT('Ctrl Pts',(-8.81400823600006,12.2,-7.05467090600001));
#277059=CARTESIAN_POINT('Ctrl Pts',(-8.81059402400006,12.2,-7.05375701900002));
#277060=CARTESIAN_POINT('Ctrl Pts',(-8.80718507800006,12.2,-7.05284169300001));
#277061=CARTESIAN_POINT('Ctrl Pts',(-8.80378140200006,12.2,-7.05192493600002));
#277062=CARTESIAN_POINT('Ctrl Pts',(-8.80038300400006,12.2,-7.05100675600002));
#277063=CARTESIAN_POINT('Ctrl Pts',(-8.79698988900006,12.2,-7.05008716200001));
#277064=CARTESIAN_POINT('Ctrl Pts',(-8.79360206200005,12.2,-7.04916616100002));
#277065=CARTESIAN_POINT('Ctrl Pts',(-8.79021953000005,12.2,-7.04824376100002));
#277066=CARTESIAN_POINT('Ctrl Pts',(-8.78684229800006,12.2,-7.04731997100002));
#277067=CARTESIAN_POINT('Ctrl Pts',(-8.78347037400006,12.2,-7.04639479800001));
#277068=CARTESIAN_POINT('Ctrl Pts',(-8.78010376100006,12.2,-7.04546825000002));
#277069=CARTESIAN_POINT('Ctrl Pts',(-8.77674246700006,12.2,-7.04454033500002));
#277070=CARTESIAN_POINT('Ctrl Pts',(-8.77338649600006,12.2,-7.04361106300002));
#277071=CARTESIAN_POINT('Ctrl Pts',(-8.77003585700006,12.2,-7.04268044000001));
#277072=CARTESIAN_POINT('Ctrl Pts',(-8.76669055200006,12.2,-7.04174847400001));
#277073=CARTESIAN_POINT('Ctrl Pts',(-8.76335059000006,12.2,-7.04081517500001));
#277074=CARTESIAN_POINT('Ctrl Pts',(-8.76001597600006,12.2,-7.03988055000002));
#277075=CARTESIAN_POINT('Ctrl Pts',(-8.75668671600006,12.2,-7.03894460800001));
#277076=CARTESIAN_POINT('Ctrl Pts',(-8.75336281400006,12.2,-7.03800735500002));
#277077=CARTESIAN_POINT('Ctrl Pts',(-8.75004427900006,12.2,-7.03706880200002));
#277078=CARTESIAN_POINT('Ctrl Pts',(-8.74673111600006,12.2,-7.03612895700001));
#277079=CARTESIAN_POINT('Ctrl Pts',(-8.74342333000006,12.2,-7.03518782500002));
#277080=CARTESIAN_POINT('Ctrl Pts',(-8.74012092800006,12.2,-7.03424541800001));
#277081=CARTESIAN_POINT('Ctrl Pts',(-8.73682391500006,12.2,-7.03330174300002));
#277082=CARTESIAN_POINT('Ctrl Pts',(-8.73353229800006,12.2,-7.03235680900002));
#277083=CARTESIAN_POINT('Ctrl Pts',(-8.73024608200006,12.2,-7.03141062300002));
#277084=CARTESIAN_POINT('Ctrl Pts',(-8.72696527300005,12.2,-7.03046319400002));
#277085=CARTESIAN_POINT('Ctrl Pts',(-8.72368987800006,12.2,-7.02951453100002));
#277086=CARTESIAN_POINT('Ctrl Pts',(-8.72041990300006,12.2,-7.02856464100002));
#277087=CARTESIAN_POINT('Ctrl Pts',(-8.71715535200006,12.2,-7.02761353400001));
#277088=CARTESIAN_POINT('Ctrl Pts',(-8.71389623400006,12.2,-7.02666121800001));
#277089=CARTESIAN_POINT('Ctrl Pts',(-8.71064255200006,12.2,-7.02570770100002));
#277090=CARTESIAN_POINT('Ctrl Pts',(-8.70739431400006,12.2,-7.02475299200002));
#277091=CARTESIAN_POINT('Ctrl Pts',(-8.70415152500006,12.2,-7.02379710000002));
#277092=CARTESIAN_POINT('Ctrl Pts',(-8.70091419100006,12.2,-7.02284003200001));
#277093=CARTESIAN_POINT('Ctrl Pts',(-8.69768231900006,12.2,-7.02188179800002));
#277094=CARTESIAN_POINT('Ctrl Pts',(-8.69445591400006,12.2,-7.02092240600001));
#277095=CARTESIAN_POINT('Ctrl Pts',(-8.69123498300005,12.2,-7.01996186500002));
#277096=CARTESIAN_POINT('Ctrl Pts',(-8.68801953200006,12.2,-7.01900018400002));
#277097=CARTESIAN_POINT('Ctrl Pts',(-8.68480956600006,12.2,-7.01803737000001));
#277098=CARTESIAN_POINT('Ctrl Pts',(-8.68160509100005,12.2,-7.01707343300002));
#277099=CARTESIAN_POINT('Ctrl Pts',(-8.67840611400006,12.2,-7.01610838100001));
#277100=CARTESIAN_POINT('Ctrl Pts',(-8.67521264100005,12.2,-7.01514222400001));
#277101=CARTESIAN_POINT('Ctrl Pts',(-8.67202467700006,12.2,-7.01417496900002));
#277102=CARTESIAN_POINT('Ctrl Pts',(-8.66884222900006,12.2,-7.01320662700001));
#277103=CARTESIAN_POINT('Ctrl Pts',(-8.66566530400006,12.2,-7.01223720400002));
#277104=CARTESIAN_POINT('Ctrl Pts',(-8.66249390600006,12.2,-7.01126671100001));
#277105=CARTESIAN_POINT('Ctrl Pts',(-8.65932804200006,12.2,-7.01029515700001));
#277106=CARTESIAN_POINT('Ctrl Pts',(-8.65616771800006,12.2,-7.00932254900002));
#277107=CARTESIAN_POINT('Ctrl Pts',(-8.65301294000006,12.2,-7.00834889700002));
#277108=CARTESIAN_POINT('Ctrl Pts',(-8.64986371500006,12.2,-7.00737421000002));
#277109=CARTESIAN_POINT('Ctrl Pts',(-8.64672004800006,12.2,-7.00639849700002));
#277110=CARTESIAN_POINT('Ctrl Pts',(-8.64358194600005,12.2,-7.00542176600001));
#277111=CARTESIAN_POINT('Ctrl Pts',(-8.64044941400006,12.2,-7.00444402600001));
#277112=CARTESIAN_POINT('Ctrl Pts',(-8.63732245800006,12.2,-7.00346528800001));
#277113=CARTESIAN_POINT('Ctrl Pts',(-8.63420108600006,12.2,-7.00248556000002));
#277114=CARTESIAN_POINT('Ctrl Pts',(-8.63108530200006,12.2,-7.00150485000002));
#277115=CARTESIAN_POINT('Ctrl Pts',(-8.62797511400006,12.2,-7.00052316700001));
#277116=CARTESIAN_POINT('Ctrl Pts',(-8.62487052700006,12.2,-6.99954052200002));
#277117=CARTESIAN_POINT('Ctrl Pts',(-8.62177154800005,12.2,-6.99855692200002));
#277118=CARTESIAN_POINT('Ctrl Pts',(-8.61867818200006,12.2,-6.99757237900001));
#277119=CARTESIAN_POINT('Ctrl Pts',(-8.61559043500005,12.2,-6.99658689800001));
#277120=CARTESIAN_POINT('Ctrl Pts',(-8.61250831400006,12.2,-6.99560049200001));
#277121=CARTESIAN_POINT('Ctrl Pts',(-8.60943182500005,12.2,-6.99461316800001));
#277122=CARTESIAN_POINT('Ctrl Pts',(-8.60636097400005,12.2,-6.99362493600002));
#277123=CARTESIAN_POINT('Ctrl Pts',(-8.60329576800006,12.2,-6.99263580600002));
#277124=CARTESIAN_POINT('Ctrl Pts',(-8.60023621200006,12.2,-6.99164578600002));
#277125=CARTESIAN_POINT('Ctrl Pts',(-8.59718231200005,12.2,-6.99065488500001));
#277126=CARTESIAN_POINT('Ctrl Pts',(-8.59413407600006,12.2,-6.98966311400002));
#277127=CARTESIAN_POINT('Ctrl Pts',(-8.59109150900006,12.2,-6.98867048200002));
#277128=CARTESIAN_POINT('Ctrl Pts',(-8.58805461700006,12.2,-6.98767699600002));
#277129=CARTESIAN_POINT('Ctrl Pts',(-8.58502340600005,12.2,-6.98668266800002));
#277130=CARTESIAN_POINT('Ctrl Pts',(-8.58199788300006,12.2,-6.98568750700002));
#277131=CARTESIAN_POINT('Ctrl Pts',(-8.57897805400006,12.2,-6.98469152300002));
#277132=CARTESIAN_POINT('Ctrl Pts',(-8.57596392500006,12.2,-6.98369472200002));
#277133=CARTESIAN_POINT('Ctrl Pts',(-8.57295550200006,12.2,-6.98269711800001));
#277134=CARTESIAN_POINT('Ctrl Pts',(-8.56995279100006,12.2,-6.98169871900002));
#277135=CARTESIAN_POINT('Ctrl Pts',(-8.56695580000006,12.2,-6.98069953300001));
#277136=CARTESIAN_POINT('Ctrl Pts',(-8.56396453400006,12.2,-6.97969957100002));
#277137=CARTESIAN_POINT('Ctrl Pts',(-8.56097900000006,12.2,-6.97869884300002));
#277138=CARTESIAN_POINT('Ctrl Pts',(-8.55799920200005,12.2,-6.97769735700002));
#277139=CARTESIAN_POINT('Ctrl Pts',(-8.55502514900006,12.2,-6.97669512400001));
#277140=CARTESIAN_POINT('Ctrl Pts',(-8.55205684500006,12.2,-6.97569215300001));
#277141=CARTESIAN_POINT('Ctrl Pts',(-8.54909429800006,12.2,-6.97468845400002));
#277142=CARTESIAN_POINT('Ctrl Pts',(-8.54613751300005,12.2,-6.97368403700001));
#277143=CARTESIAN_POINT('Ctrl Pts',(-8.54318649800006,12.2,-6.97267891200001));
#277144=CARTESIAN_POINT('Ctrl Pts',(-8.54024125700005,12.2,-6.97167308800001));
#277145=CARTESIAN_POINT('Ctrl Pts',(-8.53730179800005,12.2,-6.97066657500002));
#277146=CARTESIAN_POINT('Ctrl Pts',(-8.53436812700006,12.2,-6.96965938200002));
#277147=CARTESIAN_POINT('Ctrl Pts',(-8.53144025100006,12.2,-6.96865152100001));
#277148=CARTESIAN_POINT('Ctrl Pts',(-8.52851817400006,12.2,-6.96764300000002));
#277149=CARTESIAN_POINT('Ctrl Pts',(-8.52560190400006,12.2,-6.96663382900002));
#277150=CARTESIAN_POINT('Ctrl Pts',(-8.52269144900006,12.2,-6.96562402000002));
#277151=CARTESIAN_POINT('Ctrl Pts',(-8.51978681100006,12.2,-6.96461358000001));
#277152=CARTESIAN_POINT('Ctrl Pts',(-8.51688800000005,12.2,-6.96360252200002));
#277153=CARTESIAN_POINT('Ctrl Pts',(-8.51399502100006,12.2,-6.96259085300002));
#277154=CARTESIAN_POINT('Ctrl Pts',(-8.51110788000006,12.2,-6.96157858500002));
#277155=CARTESIAN_POINT('Ctrl Pts',(-8.50822658400006,12.2,-6.96056572800002));
#277156=CARTESIAN_POINT('Ctrl Pts',(-8.50535113900006,12.2,-6.95955229100001));
#277157=CARTESIAN_POINT('Ctrl Pts',(-8.50248155100006,12.2,-6.95853828600002));
#277158=CARTESIAN_POINT('Ctrl Pts',(-8.49961782900006,12.2,-6.95752372000002));
#277159=CARTESIAN_POINT('Ctrl Pts',(-8.49675997600006,12.2,-6.95650860700002));
#277160=CARTESIAN_POINT('Ctrl Pts',(-8.49390800000006,12.2,-6.95549295400002));
#277161=CARTESIAN_POINT('Ctrl Pts',(-8.49106190600006,12.2,-6.95447677400002));
#277162=CARTESIAN_POINT('Ctrl Pts',(-8.48822170400006,12.2,-6.95346007500002));
#277163=CARTESIAN_POINT('Ctrl Pts',(-8.48538739600006,12.2,-6.95244286800002));
#277164=CARTESIAN_POINT('Ctrl Pts',(-8.48255899100005,12.2,-6.95142516400002));
#277165=CARTESIAN_POINT('Ctrl Pts',(-8.47973649400006,12.2,-6.95040697300002));
#277166=CARTESIAN_POINT('Ctrl Pts',(-8.47691991300006,12.2,-6.94938830400002));
#277167=CARTESIAN_POINT('Ctrl Pts',(-8.47410925300006,12.2,-6.94836916900002));
#277168=CARTESIAN_POINT('Ctrl Pts',(-8.47130452200006,12.2,-6.94734957900002));
#277169=CARTESIAN_POINT('Ctrl Pts',(-8.46850572600006,12.2,-6.94632954200002));
#277170=CARTESIAN_POINT('Ctrl Pts',(-8.46571286900006,12.2,-6.94530907100001));
#277171=CARTESIAN_POINT('Ctrl Pts',(-8.46292596100006,12.2,-6.94428817600001));
#277172=CARTESIAN_POINT('Ctrl Pts',(-8.46014500600005,12.2,-6.94326686700002));
#277173=CARTESIAN_POINT('Ctrl Pts',(-8.45737001200006,12.2,-6.94224515400002));
#277174=CARTESIAN_POINT('Ctrl Pts',(-8.45460098500006,12.2,-6.94122304900001));
#277175=CARTESIAN_POINT('Ctrl Pts',(-8.45183793100006,12.2,-6.94020056100002));
#277176=CARTESIAN_POINT('Ctrl Pts',(-8.44908085600006,12.2,-6.93917770200001));
#277177=CARTESIAN_POINT('Ctrl Pts',(-8.44632976900006,12.2,-6.93815448200001));
#277178=CARTESIAN_POINT('Ctrl Pts',(-8.44358467400006,12.2,-6.93713091300002));
#277179=CARTESIAN_POINT('Ctrl Pts',(-8.44084557900005,12.2,-6.93610700400002));
#277180=CARTESIAN_POINT('Ctrl Pts',(-8.43811248900005,12.2,-6.93508276600002));
#277181=CARTESIAN_POINT('Ctrl Pts',(-8.43538541200006,12.2,-6.93405821000002));
#277182=CARTESIAN_POINT('Ctrl Pts',(-8.43266435300006,12.2,-6.93303334900002));
#277183=CARTESIAN_POINT('Ctrl Pts',(-8.42994932200006,12.2,-6.93200819000002));
#277184=CARTESIAN_POINT('Ctrl Pts',(-8.42724032100006,12.2,-6.93098274800001));
#277185=CARTESIAN_POINT('Ctrl Pts',(-8.42453736000006,12.2,-6.92995703000002));
#277186=CARTESIAN_POINT('Ctrl Pts',(-8.42184044300006,12.2,-6.92893105000002));
#277187=CARTESIAN_POINT('Ctrl Pts',(-8.41914957900006,12.2,-6.92790481800002));
#277188=CARTESIAN_POINT('Ctrl Pts',(-8.41646477200005,12.2,-6.92687834500001));
#277189=CARTESIAN_POINT('Ctrl Pts',(-8.41378603100006,12.2,-6.92585164200001));
#277190=CARTESIAN_POINT('Ctrl Pts',(-8.41111336100006,12.2,-6.92482472000002));
#277191=CARTESIAN_POINT('Ctrl Pts',(-8.40844676900005,12.2,-6.92379758900002));
#277192=CARTESIAN_POINT('Ctrl Pts',(-8.40578626200006,12.2,-6.92277026300002));
#277193=CARTESIAN_POINT('Ctrl Pts',(-8.40313184700006,12.2,-6.92174275100002));
#277194=CARTESIAN_POINT('Ctrl Pts',(-8.40048352900006,12.2,-6.92071506500002));
#277195=CARTESIAN_POINT('Ctrl Pts',(-8.39784131700006,12.2,-6.91968721500002));
#277196=CARTESIAN_POINT('Ctrl Pts',(-8.39520521500006,12.2,-6.91865921400002));
#277197=CARTESIAN_POINT('Ctrl Pts',(-8.39257523200006,12.2,-6.91763107400002));
#277198=CARTESIAN_POINT('Ctrl Pts',(-8.38995137300006,12.2,-6.91660280300002));
#277199=CARTESIAN_POINT('Ctrl Pts',(-8.38733364500006,12.2,-6.91557441500001));
#277200=CARTESIAN_POINT('Ctrl Pts',(-8.38472205600005,12.2,-6.91454592100002));
#277201=CARTESIAN_POINT('Ctrl Pts',(-8.38211661100006,12.2,-6.91351733200002));
#277202=CARTESIAN_POINT('Ctrl Pts',(-8.37951731800005,12.2,-6.91248865900001));
#277203=CARTESIAN_POINT('Ctrl Pts',(-8.37692418100006,12.2,-6.91145991600001));
#277204=CARTESIAN_POINT('Ctrl Pts',(-8.37433721100006,12.2,-6.91043111100001));
#277205=CARTESIAN_POINT('Ctrl Pts',(-8.37175641100006,12.2,-6.90940225800002));
#277206=CARTESIAN_POINT('Ctrl Pts',(-8.36918179000006,12.2,-6.90837336800002));
#277207=CARTESIAN_POINT('Ctrl Pts',(-8.36661335300006,12.2,-6.90734445300001));
#277208=CARTESIAN_POINT('Ctrl Pts',(-8.36405110900006,12.2,-6.90631552400002));
#277209=CARTESIAN_POINT('Ctrl Pts',(-8.36149506200006,12.2,-6.90528659300002));
#277210=CARTESIAN_POINT('Ctrl Pts',(-8.35894522100006,12.2,-6.90425767200002));
#277211=CARTESIAN_POINT('Ctrl Pts',(-8.35640159200006,12.2,-6.90322877200002));
#277212=CARTESIAN_POINT('Ctrl Pts',(-8.35386418000006,12.2,-6.90219990600001));
#277213=CARTESIAN_POINT('Ctrl Pts',(-8.35133299600006,12.2,-6.90117108400001));
#277214=CARTESIAN_POINT('Ctrl Pts',(-8.34880804200005,12.2,-6.90014232000002));
#277215=CARTESIAN_POINT('Ctrl Pts',(-8.34628932800005,12.2,-6.89911362500002));
#277216=CARTESIAN_POINT('Ctrl Pts',(-8.34377685900006,12.2,-6.89808501100002));
#277217=CARTESIAN_POINT('Ctrl Pts',(-8.34127064400005,12.2,-6.89705649000001));
#277218=CARTESIAN_POINT('Ctrl Pts',(-8.33877068700006,12.2,-6.89602807400002));
#277219=CARTESIAN_POINT('Ctrl Pts',(-8.33627699700006,12.2,-6.89499977500001));
#277220=CARTESIAN_POINT('Ctrl Pts',(-8.33378957900005,12.2,-6.89397160500001));
#277221=CARTESIAN_POINT('Ctrl Pts',(-8.33130844300005,12.2,-6.89294357600001));
#277222=CARTESIAN_POINT('Ctrl Pts',(-8.32883359200006,12.2,-6.89191570100002));
#277223=CARTESIAN_POINT('Ctrl Pts',(-8.32636503500006,12.2,-6.89088799200002));
#277224=CARTESIAN_POINT('Ctrl Pts',(-8.32390277900006,12.2,-6.88986046100001));
#277225=CARTESIAN_POINT('Ctrl Pts',(-8.32144683000006,12.2,-6.88883311900002));
#277226=CARTESIAN_POINT('Ctrl Pts',(-8.31899719600005,12.2,-6.88780598100001));
#277227=CARTESIAN_POINT('Ctrl Pts',(-8.31655388200006,12.2,-6.88677905700001));
#277228=CARTESIAN_POINT('Ctrl Pts',(-8.31411689600005,12.2,-6.88575236100001));
#277229=CARTESIAN_POINT('Ctrl Pts',(-8.31168624600006,12.2,-6.88472590400002));
#277230=CARTESIAN_POINT('Ctrl Pts',(-8.30926193800006,12.2,-6.88369969900001));
#277231=CARTESIAN_POINT('Ctrl Pts',(-8.30684397800006,12.2,-6.88267375900002));
#277232=CARTESIAN_POINT('Ctrl Pts',(-8.30443237500005,12.2,-6.88164809600002));
#277233=CARTESIAN_POINT('Ctrl Pts',(-8.30202713400006,12.2,-6.88062272300002));
#277234=CARTESIAN_POINT('Ctrl Pts',(-8.29962826300006,12.2,-6.87959765300001));
#277235=CARTESIAN_POINT('Ctrl Pts',(-8.29723576800006,12.2,-6.87857289700001));
#277236=CARTESIAN_POINT('Ctrl Pts',(-8.29484965700006,12.2,-6.87754847000001));
#277237=CARTESIAN_POINT('Ctrl Pts',(-8.29246993600006,12.2,-6.87652438300002));
#277238=CARTESIAN_POINT('Ctrl Pts',(-8.29009661400006,12.2,-6.87550064900002));
#277239=CARTESIAN_POINT('Ctrl Pts',(-8.28772969600006,12.2,-6.87447728100001));
#277240=CARTESIAN_POINT('Ctrl Pts',(-8.28536918900006,12.2,-6.87345429300001));
#277241=CARTESIAN_POINT('Ctrl Pts',(-8.28301510100006,12.2,-6.87243169500002));
#277242=CARTESIAN_POINT('Ctrl Pts',(-8.28066743900006,12.2,-6.87140950400002));
#277243=CARTESIAN_POINT('Ctrl Pts',(-8.27832621000006,12.2,-6.87038772900002));
#277244=CARTESIAN_POINT('Ctrl Pts',(-8.27599142100006,12.2,-6.86936638500002));
#277245=CARTESIAN_POINT('Ctrl Pts',(-8.27366307900006,12.2,-6.86834548500002));
#277246=CARTESIAN_POINT('Ctrl Pts',(-8.27134119000006,12.2,-6.86732504200001));
#277247=CARTESIAN_POINT('Ctrl Pts',(-8.26902576200006,12.2,-6.86630507000002));
#277248=CARTESIAN_POINT('Ctrl Pts',(-8.26671680300005,12.2,-6.86528558000001));
#277249=CARTESIAN_POINT('Ctrl Pts',(-8.26441431900006,12.2,-6.86426658600002));
#277250=CARTESIAN_POINT('Ctrl Pts',(-8.26211831700006,12.2,-6.86324810400002));
#277251=CARTESIAN_POINT('Ctrl Pts',(-8.25982880500005,12.2,-6.86223014300002));
#277252=CARTESIAN_POINT('Ctrl Pts',(-8.25754578900005,12.2,-6.86121271800002));
#277253=CARTESIAN_POINT('Ctrl Pts',(-8.25526927700006,12.2,-6.86019584300002));
#277254=CARTESIAN_POINT('Ctrl Pts',(-8.25299927600006,12.2,-6.85917953200001));
#277255=CARTESIAN_POINT('Ctrl Pts',(-8.25073579400006,12.2,-6.85816379700002));
#277256=CARTESIAN_POINT('Ctrl Pts',(-8.24847883600006,12.2,-6.85714865200002));
#277257=CARTESIAN_POINT('Ctrl Pts',(-8.24622841100006,12.2,-6.85613411000002));
#277258=CARTESIAN_POINT('Ctrl Pts',(-8.24398452500006,12.2,-6.85512018700001));
#277259=CARTESIAN_POINT('Ctrl Pts',(-8.24174718700006,12.2,-6.85410689300002));
#277260=CARTESIAN_POINT('Ctrl Pts',(-8.23951640200006,12.2,-6.85309424500002));
#277261=CARTESIAN_POINT('Ctrl Pts',(-8.23729218000006,12.2,-6.85208225400002));
#277262=CARTESIAN_POINT('Ctrl Pts',(-8.23507452500005,12.2,-6.85107093700001));
#277263=CARTESIAN_POINT('Ctrl Pts',(-8.23286344500006,12.2,-6.85006030300002));
#277264=CARTESIAN_POINT('Ctrl Pts',(-8.23065894900006,12.2,-6.84905037100001));
#277265=CARTESIAN_POINT('Ctrl Pts',(-8.22846104400006,12.2,-6.84804115200001));
#277266=CARTESIAN_POINT('Ctrl Pts',(-8.22626973600006,12.2,-6.84703266000002));
#277267=CARTESIAN_POINT('Ctrl Pts',(-8.22408503300006,12.2,-6.84602491000001));
#277268=CARTESIAN_POINT('Ctrl Pts',(-8.22190694200006,12.2,-6.84501791600002));
#277269=CARTESIAN_POINT('Ctrl Pts',(-8.21973547100006,12.2,-6.84401169100001));
#277270=CARTESIAN_POINT('Ctrl Pts',(-8.21757062600006,12.2,-6.84300624900001));
#277271=CARTESIAN_POINT('Ctrl Pts',(-8.21541241600006,12.2,-6.84200160600002));
#277272=CARTESIAN_POINT('Ctrl Pts',(-8.21326084700006,12.2,-6.84099777500002));
#277273=CARTESIAN_POINT('Ctrl Pts',(-8.21111592700005,12.2,-6.83999477000001));
#277274=CARTESIAN_POINT('Ctrl Pts',(-8.20897766400006,12.2,-6.83899260600001));
#277275=CARTESIAN_POINT('Ctrl Pts',(-8.20684606400006,12.2,-6.83799129700001));
#277276=CARTESIAN_POINT('Ctrl Pts',(-8.20472113500006,12.2,-6.83699085700002));
#277277=CARTESIAN_POINT('Ctrl Pts',(-8.20260288500006,12.2,-6.83599130200002));
#277278=CARTESIAN_POINT('Ctrl Pts',(-8.20049132100005,12.2,-6.83499264500002));
#277279=CARTESIAN_POINT('Ctrl Pts',(-8.19838644900006,12.2,-6.83399490000002));
#277280=CARTESIAN_POINT('Ctrl Pts',(-8.19628827900006,12.2,-6.83299808400001));
#277281=CARTESIAN_POINT('Ctrl Pts',(-8.19419681700005,12.2,-6.83200220900002));
#277282=CARTESIAN_POINT('Ctrl Pts',(-8.19211207000006,12.2,-6.83100729200002));
#277283=CARTESIAN_POINT('Ctrl Pts',(-8.19003404800006,12.2,-6.83001334600001));
#277284=CARTESIAN_POINT('Ctrl Pts',(-8.18796275500006,12.2,-6.82902038700002));
#277285=CARTESIAN_POINT('Ctrl Pts',(-8.18589820000006,12.2,-6.82802842800001));
#277286=CARTESIAN_POINT('Ctrl Pts',(-8.18384039200006,12.2,-6.82703748600002));
#277287=CARTESIAN_POINT('Ctrl Pts',(-8.18178933600005,12.2,-6.82604757600001));
#277288=CARTESIAN_POINT('Ctrl Pts',(-8.17974504200006,12.2,-6.82505871000001));
#277289=CARTESIAN_POINT('Ctrl Pts',(-8.17770751500005,12.2,-6.82407090600002));
#277290=CARTESIAN_POINT('Ctrl Pts',(-8.17567676400006,12.2,-6.82308417800002));
#277291=CARTESIAN_POINT('Ctrl Pts',(-8.17365279800006,12.2,-6.82209854300002));
#277292=CARTESIAN_POINT('Ctrl Pts',(-8.17163562200006,12.2,-6.82111401300002));
#277293=CARTESIAN_POINT('Ctrl Pts',(-8.16962524500006,12.2,-6.82013060400001));
#277294=CARTESIAN_POINT('Ctrl Pts',(-8.16762167300006,12.2,-6.81914833300001));
#277295=CARTESIAN_POINT('Ctrl Pts',(-8.16562491600006,12.2,-6.81816721500001));
#277296=CARTESIAN_POINT('Ctrl Pts',(-8.16363498100005,12.2,-6.81718726300002));
#277297=CARTESIAN_POINT('Ctrl Pts',(-8.16165187500006,12.2,-6.81620849600002));
#277298=CARTESIAN_POINT('Ctrl Pts',(-8.15967560600006,12.2,-6.81523092700001));
#277299=CARTESIAN_POINT('Ctrl Pts',(-8.15770618100006,12.2,-6.81425457200002));
#277300=CARTESIAN_POINT('Ctrl Pts',(-8.15574360800005,12.2,-6.81327944800002));
#277301=CARTESIAN_POINT('Ctrl Pts',(-8.15378789600006,12.2,-6.81230556900001));
#277302=CARTESIAN_POINT('Ctrl Pts',(-8.15183905100006,12.2,-6.81133295000001));
#277303=CARTESIAN_POINT('Ctrl Pts',(-8.14989708100006,12.2,-6.81036160900002));
#277304=CARTESIAN_POINT('Ctrl Pts',(-8.14796199500006,12.2,-6.80939156100001));
#277305=CARTESIAN_POINT('Ctrl Pts',(-8.14603380000005,12.2,-6.80842282100001));
#277306=CARTESIAN_POINT('Ctrl Pts',(-8.14411250400006,12.2,-6.80745540700002));
#277307=CARTESIAN_POINT('Ctrl Pts',(-8.14219811500006,12.2,-6.80648933300001));
#277308=CARTESIAN_POINT('Ctrl Pts',(-8.14029063900006,12.2,-6.80552461600002));
#277309=CARTESIAN_POINT('Ctrl Pts',(-8.13839008600005,12.2,-6.80456127100002));
#277310=CARTESIAN_POINT('Ctrl Pts',(-8.13649646400006,12.2,-6.80359931600002));
#277311=CARTESIAN_POINT('Ctrl Pts',(-8.13460977800006,12.2,-6.80263876500002));
#277312=CARTESIAN_POINT('Ctrl Pts',(-8.13273003800006,12.2,-6.80167963700002));
#277313=CARTESIAN_POINT('Ctrl Pts',(-8.13085725300006,12.2,-6.80072194600001));
#277314=CARTESIAN_POINT('Ctrl Pts',(-8.12899142800006,12.2,-6.79976570900001));
#277315=CARTESIAN_POINT('Ctrl Pts',(-8.12713257400006,12.2,-6.79881094300002));
#277316=CARTESIAN_POINT('Ctrl Pts',(-8.12528069700006,12.2,-6.79785766400002));
#277317=CARTESIAN_POINT('Ctrl Pts',(-8.12343580400006,12.2,-6.79690588900002));
#277318=CARTESIAN_POINT('Ctrl Pts',(-8.12159790600005,12.2,-6.79595563300002));
#277319=CARTESIAN_POINT('Ctrl Pts',(-8.11976700800006,12.2,-6.79500691500002));
#277320=CARTESIAN_POINT('Ctrl Pts',(-8.11794312000006,12.2,-6.79405975100002));
#277321=CARTESIAN_POINT('Ctrl Pts',(-8.11612624900006,12.2,-6.79311415700001));
#277322=CARTESIAN_POINT('Ctrl Pts',(-8.11431640400006,12.2,-6.79217015000001));
#277323=CARTESIAN_POINT('Ctrl Pts',(-8.11251359200006,12.2,-6.79122774800001));
#277324=CARTESIAN_POINT('Ctrl Pts',(-8.11071782100005,12.2,-6.79028696700002));
#277325=CARTESIAN_POINT('Ctrl Pts',(-8.10892909900006,12.2,-6.78934782500002));
#277326=CARTESIAN_POINT('Ctrl Pts',(-8.10714743500006,12.2,-6.78841033800002));
#277327=CARTESIAN_POINT('Ctrl Pts',(-8.10537283700006,12.2,-6.78747452400002));
#277328=CARTESIAN_POINT('Ctrl Pts',(-8.10360531200006,12.2,-6.78654039900002));
#277329=CARTESIAN_POINT('Ctrl Pts',(-8.10184486900006,12.2,-6.78560798200002));
#277330=CARTESIAN_POINT('Ctrl Pts',(-8.10009151600006,12.2,-6.78467728800002));
#277331=CARTESIAN_POINT('Ctrl Pts',(-8.09834526200006,12.2,-6.78374833700002));
#277332=CARTESIAN_POINT('Ctrl Pts',(-8.09660611400006,12.2,-6.78282114600002));
#277333=CARTESIAN_POINT('Ctrl Pts',(-8.09487408000006,12.2,-6.78189573100001));
#277334=CARTESIAN_POINT('Ctrl Pts',(-8.09314916900006,12.2,-6.78097211100001));
#277335=CARTESIAN_POINT('Ctrl Pts',(-8.09143138900006,12.2,-6.78005030300002));
#277336=CARTESIAN_POINT('Ctrl Pts',(-8.08972074900005,12.2,-6.77913032500002));
#277337=CARTESIAN_POINT('Ctrl Pts',(-8.08801725500006,12.2,-6.77821219500002));
#277338=CARTESIAN_POINT('Ctrl Pts',(-8.08632091900006,12.2,-6.77729593100001));
#277339=CARTESIAN_POINT('Ctrl Pts',(-8.08463174500006,12.2,-6.77638154900002));
#277340=CARTESIAN_POINT('Ctrl Pts',(-8.08294974400006,12.2,-6.77546907100002));
#277341=CARTESIAN_POINT('Ctrl Pts',(-8.08127492400006,12.2,-6.77455851200002));
#277342=CARTESIAN_POINT('Ctrl Pts',(-8.07960729300006,12.2,-6.77364988900001));
#277343=CARTESIAN_POINT('Ctrl Pts',(-8.07794685900006,12.2,-6.77274322400002));
#277344=CARTESIAN_POINT('Ctrl Pts',(-8.07629363200006,12.2,-6.77183853400001));
#277345=CARTESIAN_POINT('Ctrl Pts',(-8.07464761900006,12.2,-6.77093583600002));
#277346=CARTESIAN_POINT('Ctrl Pts',(-8.07300882800006,12.2,-6.77003514800001));
#277347=CARTESIAN_POINT('Ctrl Pts',(-8.07137726900006,12.2,-6.76913649000002));
#277348=CARTESIAN_POINT('Ctrl Pts',(-8.06975294900005,12.2,-6.76823988100002));
#277349=CARTESIAN_POINT('Ctrl Pts',(-8.06813587700006,12.2,-6.76734533800002));
#277350=CARTESIAN_POINT('Ctrl Pts',(-8.06652606200006,12.2,-6.76645288100002));
#277351=CARTESIAN_POINT('Ctrl Pts',(-8.06492351200006,12.2,-6.76556252900002));
#277352=CARTESIAN_POINT('Ctrl Pts',(-8.06332823500006,12.2,-6.76467429900002));
#277353=CARTESIAN_POINT('Ctrl Pts',(-8.06174024100006,12.2,-6.76378821200001));
#277354=CARTESIAN_POINT('Ctrl Pts',(-8.06015953800006,12.2,-6.76290428500002));
#277355=CARTESIAN_POINT('Ctrl Pts',(-8.05858613400006,12.2,-6.76202254000002));
#277356=CARTESIAN_POINT('Ctrl Pts',(-8.05702003900005,12.2,-6.76114299200002));
#277357=CARTESIAN_POINT('Ctrl Pts',(-8.05546126000005,12.2,-6.76026566400001));
#277358=CARTESIAN_POINT('Ctrl Pts',(-8.05390980500006,12.2,-6.75939057400001));
#277359=CARTESIAN_POINT('Ctrl Pts',(-8.05236568500005,12.2,-6.75851774000002));
#277360=CARTESIAN_POINT('Ctrl Pts',(-8.05082890800006,12.2,-6.75764718400002));
#277361=CARTESIAN_POINT('Ctrl Pts',(-8.04929948200006,12.2,-6.75677892300002));
#277362=CARTESIAN_POINT('Ctrl Pts',(-8.04777741600006,12.2,-6.75591297900001));
#277363=CARTESIAN_POINT('Ctrl Pts',(-8.04626271900006,12.2,-6.75504936900002));
#277364=CARTESIAN_POINT('Ctrl Pts',(-8.04475540000006,12.2,-6.75418811400001));
#277365=CARTESIAN_POINT('Ctrl Pts',(-8.04325546700005,12.2,-6.75332923500001));
#277366=CARTESIAN_POINT('Ctrl Pts',(-8.04176292900006,12.2,-6.75247275100002));
#277367=CARTESIAN_POINT('Ctrl Pts',(-8.04027779600006,12.2,-6.75161868200002));
#277368=CARTESIAN_POINT('Ctrl Pts',(-8.03880007500006,12.2,-6.75076704800002));
#277369=CARTESIAN_POINT('Ctrl Pts',(-8.03732977700006,12.2,-6.74991786800001));
#277370=CARTESIAN_POINT('Ctrl Pts',(-8.03586690900006,12.2,-6.74907116500002));
#277371=CARTESIAN_POINT('Ctrl Pts',(-8.03441148100006,12.2,-6.74822695700002));
#277372=CARTESIAN_POINT('Ctrl Pts',(-8.03296350200006,12.2,-6.74738526600001));
#277373=CARTESIAN_POINT('Ctrl Pts',(-8.03152298000006,12.2,-6.74654611000002));
#277374=CARTESIAN_POINT('Ctrl Pts',(-8.03008992500006,12.2,-6.74570951200002));
#277375=CARTESIAN_POINT('Ctrl Pts',(-8.02866434500006,12.2,-6.74487549200002));
#277376=CARTESIAN_POINT('Ctrl Pts',(-8.02724625000005,12.2,-6.74404407000001));
#277377=CARTESIAN_POINT('Ctrl Pts',(-8.02583565000005,12.2,-6.74321526700002));
#277378=CARTESIAN_POINT('Ctrl Pts',(-8.02443255200006,12.2,-6.74238910500002));
#277379=CARTESIAN_POINT('Ctrl Pts',(-8.02303696600006,12.2,-6.74156560400001));
#277380=CARTESIAN_POINT('Ctrl Pts',(-8.02164890100006,12.2,-6.74074478500001));
#277381=CARTESIAN_POINT('Ctrl Pts',(-8.02026836500006,12.2,-6.73992667000002));
#277382=CARTESIAN_POINT('Ctrl Pts',(-8.01889537100006,12.2,-6.73911127900002));
#277383=CARTESIAN_POINT('Ctrl Pts',(-8.01752992300005,12.2,-6.73829863500002));
#277384=CARTESIAN_POINT('Ctrl Pts',(-8.01617203400006,12.2,-6.73748875800002));
#277385=CARTESIAN_POINT('Ctrl Pts',(-8.01482171200006,12.2,-6.73668166900002));
#277386=CARTESIAN_POINT('Ctrl Pts',(-8.01347896700005,12.2,-6.73587739300002));
#277387=CARTESIAN_POINT('Ctrl Pts',(-8.01214380700005,12.2,-6.73507594700002));
#277388=CARTESIAN_POINT('Ctrl Pts',(-8.01081624200006,12.2,-6.73427735600002));
#277389=CARTESIAN_POINT('Ctrl Pts',(-8.00949628200006,12.2,-6.73348164200001));
#277390=CARTESIAN_POINT('Ctrl Pts',(-8.00818393600006,12.2,-6.73268882500001));
#277391=CARTESIAN_POINT('Ctrl Pts',(-8.00687921200005,12.2,-6.73189892800002));
#277392=CARTESIAN_POINT('Ctrl Pts',(-8.00558212100006,12.2,-6.73111197200001));
#277393=CARTESIAN_POINT('Ctrl Pts',(-8.00429267200006,12.2,-6.73032798200002));
#277394=CARTESIAN_POINT('Ctrl Pts',(-8.00301087500005,12.2,-6.72954697800002));
#277395=CARTESIAN_POINT('Ctrl Pts',(-8.00173673800006,12.2,-6.72876898400002));
#277396=CARTESIAN_POINT('Ctrl Pts',(-8.00047027300005,12.2,-6.72799402200001));
#277397=CARTESIAN_POINT('Ctrl Pts',(-7.99921148700006,12.2,-6.72722211400002));
#277398=CARTESIAN_POINT('Ctrl Pts',(-7.99796039100006,12.2,-6.72645328300002));
#277399=CARTESIAN_POINT('Ctrl Pts',(-7.99671699500006,12.2,-6.72568755200002));
#277400=CARTESIAN_POINT('Ctrl Pts',(-7.99548130800006,12.2,-6.72492494400001));
#277401=CARTESIAN_POINT('Ctrl Pts',(-7.99425333800006,12.2,-6.72416548300002));
#277402=CARTESIAN_POINT('Ctrl Pts',(-7.99303309800005,12.2,-6.72340919000002));
#277403=CARTESIAN_POINT('Ctrl Pts',(-7.99182059500006,12.2,-6.72265608900001));
#277404=CARTESIAN_POINT('Ctrl Pts',(-7.99061584100006,12.2,-6.72190620500002));
#277405=CARTESIAN_POINT('Ctrl Pts',(-7.98941884300006,12.2,-6.72115955900002));
#277406=CARTESIAN_POINT('Ctrl Pts',(-7.98822961400005,12.2,-6.72041617700001));
#277407=CARTESIAN_POINT('Ctrl Pts',(-7.98704816100006,12.2,-6.71967608000001));
#277408=CARTESIAN_POINT('Ctrl Pts',(-7.98587449600006,12.2,-6.71893929400002));
#277409=CARTESIAN_POINT('Ctrl Pts',(-7.98470862800006,12.2,-6.71820584100002));
#277410=CARTESIAN_POINT('Ctrl Pts',(-7.98355056700006,12.2,-6.71747574700002));
#277411=CARTESIAN_POINT('Ctrl Pts',(-7.98240032200006,12.2,-6.71674903500002));
#277412=CARTESIAN_POINT('Ctrl Pts',(-7.98125790500006,12.2,-6.71602572900002));
#277413=CARTESIAN_POINT('Ctrl Pts',(-7.98012332400006,12.2,-6.71530585300002));
#277414=CARTESIAN_POINT('Ctrl Pts',(-7.97899659000005,12.2,-6.71458943300002));
#277415=CARTESIAN_POINT('Ctrl Pts',(-7.97787771400006,12.2,-6.71387649200001));
#277416=CARTESIAN_POINT('Ctrl Pts',(-7.97676670400006,12.2,-6.71316705500002));
#277417=CARTESIAN_POINT('Ctrl Pts',(-7.97566357200005,12.2,-6.71246114600001));
#277418=CARTESIAN_POINT('Ctrl Pts',(-7.97456832700006,12.2,-6.71175879200002));
#277419=CARTESIAN_POINT('Ctrl Pts',(-7.97348098000005,12.2,-6.71106001600001));
#277420=CARTESIAN_POINT('Ctrl Pts',(-7.97240154100006,12.2,-6.71036484500001));
#277421=CARTESIAN_POINT('Ctrl Pts',(-7.97133002000006,12.2,-6.70967330200002));
#277422=CARTESIAN_POINT('Ctrl Pts',(-7.97026642700006,12.2,-6.70898541300001));
#277423=CARTESIAN_POINT('Ctrl Pts',(-7.96921077400006,12.2,-6.70830120300002));
#277424=CARTESIAN_POINT('Ctrl Pts',(-7.96816307000006,12.2,-6.70762070000002));
#277425=CARTESIAN_POINT('Ctrl Pts',(-7.96712332500006,12.2,-6.70694392700002));
#277426=CARTESIAN_POINT('Ctrl Pts',(-7.96609155000005,12.2,-6.70627091100001));
#277427=CARTESIAN_POINT('Ctrl Pts',(-7.96506775600006,12.2,-6.70560167700001));
#277428=CARTESIAN_POINT('Ctrl Pts',(-7.96405195200006,12.2,-6.70493625300002));
#277429=CARTESIAN_POINT('Ctrl Pts',(-7.96304415000006,12.2,-6.70427466300002));
#277430=CARTESIAN_POINT('Ctrl Pts',(-7.96204436100006,12.2,-6.70361693500002));
#277431=CARTESIAN_POINT('Ctrl Pts',(-7.96105259400005,12.2,-6.70296309300002));
#277432=CARTESIAN_POINT('Ctrl Pts',(-7.96006886100006,12.2,-6.70231316600002));
#277433=CARTESIAN_POINT('Ctrl Pts',(-7.95909317200006,12.2,-6.70166718000001));
#277434=CARTESIAN_POINT('Ctrl Pts',(-7.95812553700006,12.2,-6.70102516100001));
#277435=CARTESIAN_POINT('Ctrl Pts',(-7.95716596800006,12.2,-6.70038713600002));
#277436=CARTESIAN_POINT('Ctrl Pts',(-7.95621447600006,12.2,-6.69975313400001));
#277437=CARTESIAN_POINT('Ctrl Pts',(-7.95527107000006,12.2,-6.69912317900001));
#277438=CARTESIAN_POINT('Ctrl Pts',(-7.95433576200006,12.2,-6.69849730100001));
#277439=CARTESIAN_POINT('Ctrl Pts',(-7.95340856400006,12.2,-6.69787552700001));
#277440=CARTESIAN_POINT('Ctrl Pts',(-7.95248948500006,12.2,-6.69725788300001));
#277441=CARTESIAN_POINT('Ctrl Pts',(-7.95157853800006,12.2,-6.69664439800002));
#277442=CARTESIAN_POINT('Ctrl Pts',(-7.95067573200006,12.2,-6.69603510000002));
#277443=CARTESIAN_POINT('Ctrl Pts',(-7.94978107900006,12.2,-6.69543001700001));
#277444=CARTESIAN_POINT('Ctrl Pts',(-7.94889459000006,12.2,-6.69482917500002));
#277445=CARTESIAN_POINT('Ctrl Pts',(-7.94801627800006,12.2,-6.69423260500002));
#277446=CARTESIAN_POINT('Ctrl Pts',(-7.94714615000006,12.2,-6.69364033500001));
#277447=CARTESIAN_POINT('Ctrl Pts',(-7.94628422000006,12.2,-6.69305239200002));
#277448=CARTESIAN_POINT('Ctrl Pts',(-7.94543050000006,12.2,-6.69246880700002));
#277449=CARTESIAN_POINT('Ctrl Pts',(-7.94458499900006,12.2,-6.69188960600002));
#277450=CARTESIAN_POINT('Ctrl Pts',(-7.94374773100006,12.2,-6.69131482000001));
#277451=CARTESIAN_POINT('Ctrl Pts',(-7.94291870400006,12.2,-6.69074447800002));
#277452=CARTESIAN_POINT('Ctrl Pts',(-7.94209793300006,12.2,-6.69017860900002));
#277453=CARTESIAN_POINT('Ctrl Pts',(-7.94128542700006,12.2,-6.68961724100001));
#277454=CARTESIAN_POINT('Ctrl Pts',(-7.94048119900006,12.2,-6.68906040700002));
#277455=CARTESIAN_POINT('Ctrl Pts',(-7.93968525900006,12.2,-6.68850813300002));
#277456=CARTESIAN_POINT('Ctrl Pts',(-7.93889762000005,12.2,-6.68796045200001));
#277457=CARTESIAN_POINT('Ctrl Pts',(-7.93811829300005,12.2,-6.68741739000002));
#277458=CARTESIAN_POINT('Ctrl Pts',(-7.93734729000006,12.2,-6.68687898200002));
#277459=CARTESIAN_POINT('Ctrl Pts',(-7.93658462200005,12.2,-6.68634525500002));
#277460=CARTESIAN_POINT('Ctrl Pts',(-7.93583464600006,12.2,-6.68581928800001));
#277461=CARTESIAN_POINT('Ctrl Pts',(-7.93524212700006,12.2,-6.68540286400002));
#277462=CARTESIAN_POINT('Ctrl Pts',(-7.93480250600006,12.2,-6.68509340700002));
#277463=CARTESIAN_POINT('Ctrl Pts',(-7.93451247200006,12.2,-6.68488903400001));
#277464=CARTESIAN_POINT('Ctrl Pts',(-7.93436997000006,12.2,-6.68478856700002));
#277465=CARTESIAN_POINT('Ctrl Pts',(-7.93436997000006,15.2,-6.68478856700002));
#277466=CARTESIAN_POINT('Ctrl Pts',(-7.93451247200006,15.2,-6.68488903400001));
#277467=CARTESIAN_POINT('Ctrl Pts',(-7.93480250600006,15.2,-6.68509340700002));
#277468=CARTESIAN_POINT('Ctrl Pts',(-7.93524212700006,15.2,-6.68540286400002));
#277469=CARTESIAN_POINT('Ctrl Pts',(-7.93583464600006,15.2,-6.68581928800001));
#277470=CARTESIAN_POINT('Ctrl Pts',(-7.93658462200005,15.2,-6.68634525500002));
#277471=CARTESIAN_POINT('Ctrl Pts',(-7.93734729000006,15.2,-6.68687898200002));
#277472=CARTESIAN_POINT('Ctrl Pts',(-7.93811829300005,15.2,-6.68741739000002));
#277473=CARTESIAN_POINT('Ctrl Pts',(-7.93889762000005,15.2,-6.68796045200001));
#277474=CARTESIAN_POINT('Ctrl Pts',(-7.93968525900006,15.2,-6.68850813300002));
#277475=CARTESIAN_POINT('Ctrl Pts',(-7.94048119900006,15.2,-6.68906040700002));
#277476=CARTESIAN_POINT('Ctrl Pts',(-7.94128542700006,15.2,-6.68961724100001));
#277477=CARTESIAN_POINT('Ctrl Pts',(-7.94209793300006,15.2,-6.69017860900002));
#277478=CARTESIAN_POINT('Ctrl Pts',(-7.94291870400006,15.2,-6.69074447800002));
#277479=CARTESIAN_POINT('Ctrl Pts',(-7.94374773100006,15.2,-6.69131482000001));
#277480=CARTESIAN_POINT('Ctrl Pts',(-7.94458499900006,15.2,-6.69188960600002));
#277481=CARTESIAN_POINT('Ctrl Pts',(-7.94543050000006,15.2,-6.69246880700002));
#277482=CARTESIAN_POINT('Ctrl Pts',(-7.94628422000006,15.2,-6.69305239200002));
#277483=CARTESIAN_POINT('Ctrl Pts',(-7.94714615000006,15.2,-6.69364033500001));
#277484=CARTESIAN_POINT('Ctrl Pts',(-7.94801627800006,15.2,-6.69423260500002));
#277485=CARTESIAN_POINT('Ctrl Pts',(-7.94889459000006,15.2,-6.69482917500002));
#277486=CARTESIAN_POINT('Ctrl Pts',(-7.94978107900006,15.2,-6.69543001700001));
#277487=CARTESIAN_POINT('Ctrl Pts',(-7.95067573200006,15.2,-6.69603510000002));
#277488=CARTESIAN_POINT('Ctrl Pts',(-7.95157853800006,15.2,-6.69664439800002));
#277489=CARTESIAN_POINT('Ctrl Pts',(-7.95248948500006,15.2,-6.69725788300001));
#277490=CARTESIAN_POINT('Ctrl Pts',(-7.95340856400006,15.2,-6.69787552700001));
#277491=CARTESIAN_POINT('Ctrl Pts',(-7.95433576200006,15.2,-6.69849730100001));
#277492=CARTESIAN_POINT('Ctrl Pts',(-7.95527107000006,15.2,-6.69912317900001));
#277493=CARTESIAN_POINT('Ctrl Pts',(-7.95621447600006,15.2,-6.69975313400001));
#277494=CARTESIAN_POINT('Ctrl Pts',(-7.95716596800006,15.2,-6.70038713600002));
#277495=CARTESIAN_POINT('Ctrl Pts',(-7.95812553700006,15.2,-6.70102516100001));
#277496=CARTESIAN_POINT('Ctrl Pts',(-7.95909317200006,15.2,-6.70166718000001));
#277497=CARTESIAN_POINT('Ctrl Pts',(-7.96006886100006,15.2,-6.70231316600002));
#277498=CARTESIAN_POINT('Ctrl Pts',(-7.96105259400005,15.2,-6.70296309300002));
#277499=CARTESIAN_POINT('Ctrl Pts',(-7.96204436100006,15.2,-6.70361693500002));
#277500=CARTESIAN_POINT('Ctrl Pts',(-7.96304415000006,15.2,-6.70427466300002));
#277501=CARTESIAN_POINT('Ctrl Pts',(-7.96405195200006,15.2,-6.70493625300002));
#277502=CARTESIAN_POINT('Ctrl Pts',(-7.96506775600006,15.2,-6.70560167700001));
#277503=CARTESIAN_POINT('Ctrl Pts',(-7.96609155000005,15.2,-6.70627091100001));
#277504=CARTESIAN_POINT('Ctrl Pts',(-7.96712332500006,15.2,-6.70694392700002));
#277505=CARTESIAN_POINT('Ctrl Pts',(-7.96816307000006,15.2,-6.70762070000002));
#277506=CARTESIAN_POINT('Ctrl Pts',(-7.96921077400006,15.2,-6.70830120300002));
#277507=CARTESIAN_POINT('Ctrl Pts',(-7.97026642700006,15.2,-6.70898541300001));
#277508=CARTESIAN_POINT('Ctrl Pts',(-7.97133002000006,15.2,-6.70967330200002));
#277509=CARTESIAN_POINT('Ctrl Pts',(-7.97240154100006,15.2,-6.71036484500001));
#277510=CARTESIAN_POINT('Ctrl Pts',(-7.97348098000005,15.2,-6.71106001600001));
#277511=CARTESIAN_POINT('Ctrl Pts',(-7.97456832700006,15.2,-6.71175879200002));
#277512=CARTESIAN_POINT('Ctrl Pts',(-7.97566357200005,15.2,-6.71246114600001));
#277513=CARTESIAN_POINT('Ctrl Pts',(-7.97676670400006,15.2,-6.71316705500002));
#277514=CARTESIAN_POINT('Ctrl Pts',(-7.97787771400006,15.2,-6.71387649200001));
#277515=CARTESIAN_POINT('Ctrl Pts',(-7.97899659000005,15.2,-6.71458943300002));
#277516=CARTESIAN_POINT('Ctrl Pts',(-7.98012332400006,15.2,-6.71530585300002));
#277517=CARTESIAN_POINT('Ctrl Pts',(-7.98125790500006,15.2,-6.71602572900002));
#277518=CARTESIAN_POINT('Ctrl Pts',(-7.98240032200006,15.2,-6.71674903500002));
#277519=CARTESIAN_POINT('Ctrl Pts',(-7.98355056700006,15.2,-6.71747574700002));
#277520=CARTESIAN_POINT('Ctrl Pts',(-7.98470862800006,15.2,-6.71820584100002));
#277521=CARTESIAN_POINT('Ctrl Pts',(-7.98587449600006,15.2,-6.71893929400002));
#277522=CARTESIAN_POINT('Ctrl Pts',(-7.98704816100006,15.2,-6.71967608000001));
#277523=CARTESIAN_POINT('Ctrl Pts',(-7.98822961400005,15.2,-6.72041617700001));
#277524=CARTESIAN_POINT('Ctrl Pts',(-7.98941884300006,15.2,-6.72115955900002));
#277525=CARTESIAN_POINT('Ctrl Pts',(-7.99061584100006,15.2,-6.72190620500002));
#277526=CARTESIAN_POINT('Ctrl Pts',(-7.99182059500006,15.2,-6.72265608900001));
#277527=CARTESIAN_POINT('Ctrl Pts',(-7.99303309800005,15.2,-6.72340919000002));
#277528=CARTESIAN_POINT('Ctrl Pts',(-7.99425333800006,15.2,-6.72416548300002));
#277529=CARTESIAN_POINT('Ctrl Pts',(-7.99548130800006,15.2,-6.72492494400001));
#277530=CARTESIAN_POINT('Ctrl Pts',(-7.99671699500006,15.2,-6.72568755200002));
#277531=CARTESIAN_POINT('Ctrl Pts',(-7.99796039100006,15.2,-6.72645328300002));
#277532=CARTESIAN_POINT('Ctrl Pts',(-7.99921148700006,15.2,-6.72722211400002));
#277533=CARTESIAN_POINT('Ctrl Pts',(-8.00047027300005,15.2,-6.72799402200001));
#277534=CARTESIAN_POINT('Ctrl Pts',(-8.00173673800006,15.2,-6.72876898400002));
#277535=CARTESIAN_POINT('Ctrl Pts',(-8.00301087500005,15.2,-6.72954697800002));
#277536=CARTESIAN_POINT('Ctrl Pts',(-8.00429267200006,15.2,-6.73032798200002));
#277537=CARTESIAN_POINT('Ctrl Pts',(-8.00558212100006,15.2,-6.73111197200001));
#277538=CARTESIAN_POINT('Ctrl Pts',(-8.00687921200005,15.2,-6.73189892800002));
#277539=CARTESIAN_POINT('Ctrl Pts',(-8.00818393600006,15.2,-6.73268882500001));
#277540=CARTESIAN_POINT('Ctrl Pts',(-8.00949628200006,15.2,-6.73348164200001));
#277541=CARTESIAN_POINT('Ctrl Pts',(-8.01081624200006,15.2,-6.73427735600002));
#277542=CARTESIAN_POINT('Ctrl Pts',(-8.01214380700005,15.2,-6.73507594700002));
#277543=CARTESIAN_POINT('Ctrl Pts',(-8.01347896700005,15.2,-6.73587739300002));
#277544=CARTESIAN_POINT('Ctrl Pts',(-8.01482171200006,15.2,-6.73668166900002));
#277545=CARTESIAN_POINT('Ctrl Pts',(-8.01617203400006,15.2,-6.73748875800002));
#277546=CARTESIAN_POINT('Ctrl Pts',(-8.01752992300005,15.2,-6.73829863500002));
#277547=CARTESIAN_POINT('Ctrl Pts',(-8.01889537100006,15.2,-6.73911127900002));
#277548=CARTESIAN_POINT('Ctrl Pts',(-8.02026836500006,15.2,-6.73992667000002));
#277549=CARTESIAN_POINT('Ctrl Pts',(-8.02164890100006,15.2,-6.74074478500001));
#277550=CARTESIAN_POINT('Ctrl Pts',(-8.02303696600006,15.2,-6.74156560400001));
#277551=CARTESIAN_POINT('Ctrl Pts',(-8.02443255200006,15.2,-6.74238910500002));
#277552=CARTESIAN_POINT('Ctrl Pts',(-8.02583565000005,15.2,-6.74321526700002));
#277553=CARTESIAN_POINT('Ctrl Pts',(-8.02724625000005,15.2,-6.74404407000001));
#277554=CARTESIAN_POINT('Ctrl Pts',(-8.02866434500006,15.2,-6.74487549200002));
#277555=CARTESIAN_POINT('Ctrl Pts',(-8.03008992500006,15.2,-6.74570951200002));
#277556=CARTESIAN_POINT('Ctrl Pts',(-8.03152298000006,15.2,-6.74654611000002));
#277557=CARTESIAN_POINT('Ctrl Pts',(-8.03296350200006,15.2,-6.74738526600001));
#277558=CARTESIAN_POINT('Ctrl Pts',(-8.03441148100006,15.2,-6.74822695700002));
#277559=CARTESIAN_POINT('Ctrl Pts',(-8.03586690900006,15.2,-6.74907116500002));
#277560=CARTESIAN_POINT('Ctrl Pts',(-8.03732977700006,15.2,-6.74991786800001));
#277561=CARTESIAN_POINT('Ctrl Pts',(-8.03880007500006,15.2,-6.75076704800002));
#277562=CARTESIAN_POINT('Ctrl Pts',(-8.04027779600006,15.2,-6.75161868200002));
#277563=CARTESIAN_POINT('Ctrl Pts',(-8.04176292900006,15.2,-6.75247275100002));
#277564=CARTESIAN_POINT('Ctrl Pts',(-8.04325546700005,15.2,-6.75332923500001));
#277565=CARTESIAN_POINT('Ctrl Pts',(-8.04475540000006,15.2,-6.75418811400001));
#277566=CARTESIAN_POINT('Ctrl Pts',(-8.04626271900006,15.2,-6.75504936900002));
#277567=CARTESIAN_POINT('Ctrl Pts',(-8.04777741600006,15.2,-6.75591297900001));
#277568=CARTESIAN_POINT('Ctrl Pts',(-8.04929948200006,15.2,-6.75677892300002));
#277569=CARTESIAN_POINT('Ctrl Pts',(-8.05082890800006,15.2,-6.75764718400002));
#277570=CARTESIAN_POINT('Ctrl Pts',(-8.05236568500005,15.2,-6.75851774000002));
#277571=CARTESIAN_POINT('Ctrl Pts',(-8.05390980500006,15.2,-6.75939057400001));
#277572=CARTESIAN_POINT('Ctrl Pts',(-8.05546126000005,15.2,-6.76026566400001));
#277573=CARTESIAN_POINT('Ctrl Pts',(-8.05702003900005,15.2,-6.76114299200002));
#277574=CARTESIAN_POINT('Ctrl Pts',(-8.05858613400006,15.2,-6.76202254000002));
#277575=CARTESIAN_POINT('Ctrl Pts',(-8.06015953800006,15.2,-6.76290428500002));
#277576=CARTESIAN_POINT('Ctrl Pts',(-8.06174024100006,15.2,-6.76378821200001));
#277577=CARTESIAN_POINT('Ctrl Pts',(-8.06332823500006,15.2,-6.76467429900002));
#277578=CARTESIAN_POINT('Ctrl Pts',(-8.06492351200006,15.2,-6.76556252900002));
#277579=CARTESIAN_POINT('Ctrl Pts',(-8.06652606200006,15.2,-6.76645288100002));
#277580=CARTESIAN_POINT('Ctrl Pts',(-8.06813587700006,15.2,-6.76734533800002));
#277581=CARTESIAN_POINT('Ctrl Pts',(-8.06975294900005,15.2,-6.76823988100002));
#277582=CARTESIAN_POINT('Ctrl Pts',(-8.07137726900006,15.2,-6.76913649000002));
#277583=CARTESIAN_POINT('Ctrl Pts',(-8.07300882800006,15.2,-6.77003514800001));
#277584=CARTESIAN_POINT('Ctrl Pts',(-8.07464761900006,15.2,-6.77093583600002));
#277585=CARTESIAN_POINT('Ctrl Pts',(-8.07629363200006,15.2,-6.77183853400001));
#277586=CARTESIAN_POINT('Ctrl Pts',(-8.07794685900006,15.2,-6.77274322400002));
#277587=CARTESIAN_POINT('Ctrl Pts',(-8.07960729300006,15.2,-6.77364988900001));
#277588=CARTESIAN_POINT('Ctrl Pts',(-8.08127492400006,15.2,-6.77455851200002));
#277589=CARTESIAN_POINT('Ctrl Pts',(-8.08294974400006,15.2,-6.77546907100002));
#277590=CARTESIAN_POINT('Ctrl Pts',(-8.08463174500006,15.2,-6.77638154900002));
#277591=CARTESIAN_POINT('Ctrl Pts',(-8.08632091900006,15.2,-6.77729593100001));
#277592=CARTESIAN_POINT('Ctrl Pts',(-8.08801725500006,15.2,-6.77821219500002));
#277593=CARTESIAN_POINT('Ctrl Pts',(-8.08972074900005,15.2,-6.77913032500002));
#277594=CARTESIAN_POINT('Ctrl Pts',(-8.09143138900006,15.2,-6.78005030300002));
#277595=CARTESIAN_POINT('Ctrl Pts',(-8.09314916900006,15.2,-6.78097211100001));
#277596=CARTESIAN_POINT('Ctrl Pts',(-8.09487408000006,15.2,-6.78189573100001));
#277597=CARTESIAN_POINT('Ctrl Pts',(-8.09660611400006,15.2,-6.78282114600002));
#277598=CARTESIAN_POINT('Ctrl Pts',(-8.09834526200006,15.2,-6.78374833700002));
#277599=CARTESIAN_POINT('Ctrl Pts',(-8.10009151600006,15.2,-6.78467728800002));
#277600=CARTESIAN_POINT('Ctrl Pts',(-8.10184486900006,15.2,-6.78560798200002));
#277601=CARTESIAN_POINT('Ctrl Pts',(-8.10360531200006,15.2,-6.78654039900002));
#277602=CARTESIAN_POINT('Ctrl Pts',(-8.10537283700006,15.2,-6.78747452400002));
#277603=CARTESIAN_POINT('Ctrl Pts',(-8.10714743500006,15.2,-6.78841033800002));
#277604=CARTESIAN_POINT('Ctrl Pts',(-8.10892909900006,15.2,-6.78934782500002));
#277605=CARTESIAN_POINT('Ctrl Pts',(-8.11071782100005,15.2,-6.79028696700002));
#277606=CARTESIAN_POINT('Ctrl Pts',(-8.11251359200006,15.2,-6.79122774800001));
#277607=CARTESIAN_POINT('Ctrl Pts',(-8.11431640400006,15.2,-6.79217015000001));
#277608=CARTESIAN_POINT('Ctrl Pts',(-8.11612624900006,15.2,-6.79311415700001));
#277609=CARTESIAN_POINT('Ctrl Pts',(-8.11794312000006,15.2,-6.79405975100002));
#277610=CARTESIAN_POINT('Ctrl Pts',(-8.11976700800006,15.2,-6.79500691500002));
#277611=CARTESIAN_POINT('Ctrl Pts',(-8.12159790600005,15.2,-6.79595563300002));
#277612=CARTESIAN_POINT('Ctrl Pts',(-8.12343580400006,15.2,-6.79690588900002));
#277613=CARTESIAN_POINT('Ctrl Pts',(-8.12528069700006,15.2,-6.79785766400002));
#277614=CARTESIAN_POINT('Ctrl Pts',(-8.12713257400006,15.2,-6.79881094300002));
#277615=CARTESIAN_POINT('Ctrl Pts',(-8.12899142800006,15.2,-6.79976570900001));
#277616=CARTESIAN_POINT('Ctrl Pts',(-8.13085725300006,15.2,-6.80072194600001));
#277617=CARTESIAN_POINT('Ctrl Pts',(-8.13273003800006,15.2,-6.80167963700002));
#277618=CARTESIAN_POINT('Ctrl Pts',(-8.13460977800006,15.2,-6.80263876500002));
#277619=CARTESIAN_POINT('Ctrl Pts',(-8.13649646400006,15.2,-6.80359931600002));
#277620=CARTESIAN_POINT('Ctrl Pts',(-8.13839008600005,15.2,-6.80456127100002));
#277621=CARTESIAN_POINT('Ctrl Pts',(-8.14029063900006,15.2,-6.80552461600002));
#277622=CARTESIAN_POINT('Ctrl Pts',(-8.14219811500006,15.2,-6.80648933300001));
#277623=CARTESIAN_POINT('Ctrl Pts',(-8.14411250400006,15.2,-6.80745540700002));
#277624=CARTESIAN_POINT('Ctrl Pts',(-8.14603380000005,15.2,-6.80842282100001));
#277625=CARTESIAN_POINT('Ctrl Pts',(-8.14796199500006,15.2,-6.80939156100001));
#277626=CARTESIAN_POINT('Ctrl Pts',(-8.14989708100006,15.2,-6.81036160900002));
#277627=CARTESIAN_POINT('Ctrl Pts',(-8.15183905100006,15.2,-6.81133295000001));
#277628=CARTESIAN_POINT('Ctrl Pts',(-8.15378789600006,15.2,-6.81230556900001));
#277629=CARTESIAN_POINT('Ctrl Pts',(-8.15574360800005,15.2,-6.81327944800002));
#277630=CARTESIAN_POINT('Ctrl Pts',(-8.15770618100006,15.2,-6.81425457200002));
#277631=CARTESIAN_POINT('Ctrl Pts',(-8.15967560600006,15.2,-6.81523092700001));
#277632=CARTESIAN_POINT('Ctrl Pts',(-8.16165187500006,15.2,-6.81620849600002));
#277633=CARTESIAN_POINT('Ctrl Pts',(-8.16363498100005,15.2,-6.81718726300002));
#277634=CARTESIAN_POINT('Ctrl Pts',(-8.16562491600006,15.2,-6.81816721500001));
#277635=CARTESIAN_POINT('Ctrl Pts',(-8.16762167300006,15.2,-6.81914833300001));
#277636=CARTESIAN_POINT('Ctrl Pts',(-8.16962524500006,15.2,-6.82013060400001));
#277637=CARTESIAN_POINT('Ctrl Pts',(-8.17163562200006,15.2,-6.82111401300002));
#277638=CARTESIAN_POINT('Ctrl Pts',(-8.17365279800006,15.2,-6.82209854300002));
#277639=CARTESIAN_POINT('Ctrl Pts',(-8.17567676400006,15.2,-6.82308417800002));
#277640=CARTESIAN_POINT('Ctrl Pts',(-8.17770751500005,15.2,-6.82407090600002));
#277641=CARTESIAN_POINT('Ctrl Pts',(-8.17974504200006,15.2,-6.82505871000001));
#277642=CARTESIAN_POINT('Ctrl Pts',(-8.18178933600005,15.2,-6.82604757600001));
#277643=CARTESIAN_POINT('Ctrl Pts',(-8.18384039200006,15.2,-6.82703748600002));
#277644=CARTESIAN_POINT('Ctrl Pts',(-8.18589820000006,15.2,-6.82802842800001));
#277645=CARTESIAN_POINT('Ctrl Pts',(-8.18796275500006,15.2,-6.82902038700002));
#277646=CARTESIAN_POINT('Ctrl Pts',(-8.19003404800006,15.2,-6.83001334600001));
#277647=CARTESIAN_POINT('Ctrl Pts',(-8.19211207000006,15.2,-6.83100729200002));
#277648=CARTESIAN_POINT('Ctrl Pts',(-8.19419681700005,15.2,-6.83200220900002));
#277649=CARTESIAN_POINT('Ctrl Pts',(-8.19628827900006,15.2,-6.83299808400001));
#277650=CARTESIAN_POINT('Ctrl Pts',(-8.19838644900006,15.2,-6.83399490000002));
#277651=CARTESIAN_POINT('Ctrl Pts',(-8.20049132100005,15.2,-6.83499264500002));
#277652=CARTESIAN_POINT('Ctrl Pts',(-8.20260288500006,15.2,-6.83599130200002));
#277653=CARTESIAN_POINT('Ctrl Pts',(-8.20472113500006,15.2,-6.83699085700002));
#277654=CARTESIAN_POINT('Ctrl Pts',(-8.20684606400006,15.2,-6.83799129700001));
#277655=CARTESIAN_POINT('Ctrl Pts',(-8.20897766400006,15.2,-6.83899260600001));
#277656=CARTESIAN_POINT('Ctrl Pts',(-8.21111592700005,15.2,-6.83999477000001));
#277657=CARTESIAN_POINT('Ctrl Pts',(-8.21326084700006,15.2,-6.84099777500002));
#277658=CARTESIAN_POINT('Ctrl Pts',(-8.21541241600006,15.2,-6.84200160600002));
#277659=CARTESIAN_POINT('Ctrl Pts',(-8.21757062600006,15.2,-6.84300624900001));
#277660=CARTESIAN_POINT('Ctrl Pts',(-8.21973547100006,15.2,-6.84401169100001));
#277661=CARTESIAN_POINT('Ctrl Pts',(-8.22190694200006,15.2,-6.84501791600002));
#277662=CARTESIAN_POINT('Ctrl Pts',(-8.22408503300006,15.2,-6.84602491000001));
#277663=CARTESIAN_POINT('Ctrl Pts',(-8.22626973600006,15.2,-6.84703266000002));
#277664=CARTESIAN_POINT('Ctrl Pts',(-8.22846104400006,15.2,-6.84804115200001));
#277665=CARTESIAN_POINT('Ctrl Pts',(-8.23065894900006,15.2,-6.84905037100001));
#277666=CARTESIAN_POINT('Ctrl Pts',(-8.23286344500006,15.2,-6.85006030300002));
#277667=CARTESIAN_POINT('Ctrl Pts',(-8.23507452500005,15.2,-6.85107093700001));
#277668=CARTESIAN_POINT('Ctrl Pts',(-8.23729218000006,15.2,-6.85208225400002));
#277669=CARTESIAN_POINT('Ctrl Pts',(-8.23951640200006,15.2,-6.85309424500002));
#277670=CARTESIAN_POINT('Ctrl Pts',(-8.24174718700006,15.2,-6.85410689300002));
#277671=CARTESIAN_POINT('Ctrl Pts',(-8.24398452500006,15.2,-6.85512018700001));
#277672=CARTESIAN_POINT('Ctrl Pts',(-8.24622841100006,15.2,-6.85613411000002));
#277673=CARTESIAN_POINT('Ctrl Pts',(-8.24847883600006,15.2,-6.85714865200002));
#277674=CARTESIAN_POINT('Ctrl Pts',(-8.25073579400006,15.2,-6.85816379700002));
#277675=CARTESIAN_POINT('Ctrl Pts',(-8.25299927600006,15.2,-6.85917953200001));
#277676=CARTESIAN_POINT('Ctrl Pts',(-8.25526927700006,15.2,-6.86019584300002));
#277677=CARTESIAN_POINT('Ctrl Pts',(-8.25754578900005,15.2,-6.86121271800002));
#277678=CARTESIAN_POINT('Ctrl Pts',(-8.25982880500005,15.2,-6.86223014300002));
#277679=CARTESIAN_POINT('Ctrl Pts',(-8.26211831700006,15.2,-6.86324810400002));
#277680=CARTESIAN_POINT('Ctrl Pts',(-8.26441431900006,15.2,-6.86426658600002));
#277681=CARTESIAN_POINT('Ctrl Pts',(-8.26671680300005,15.2,-6.86528558000001));
#277682=CARTESIAN_POINT('Ctrl Pts',(-8.26902576200006,15.2,-6.86630507000002));
#277683=CARTESIAN_POINT('Ctrl Pts',(-8.27134119000006,15.2,-6.86732504200001));
#277684=CARTESIAN_POINT('Ctrl Pts',(-8.27366307900006,15.2,-6.86834548500002));
#277685=CARTESIAN_POINT('Ctrl Pts',(-8.27599142100006,15.2,-6.86936638500002));
#277686=CARTESIAN_POINT('Ctrl Pts',(-8.27832621000006,15.2,-6.87038772900002));
#277687=CARTESIAN_POINT('Ctrl Pts',(-8.28066743900006,15.2,-6.87140950400002));
#277688=CARTESIAN_POINT('Ctrl Pts',(-8.28301510100006,15.2,-6.87243169500002));
#277689=CARTESIAN_POINT('Ctrl Pts',(-8.28536918900006,15.2,-6.87345429300001));
#277690=CARTESIAN_POINT('Ctrl Pts',(-8.28772969600006,15.2,-6.87447728100001));
#277691=CARTESIAN_POINT('Ctrl Pts',(-8.29009661400006,15.2,-6.87550064900002));
#277692=CARTESIAN_POINT('Ctrl Pts',(-8.29246993600006,15.2,-6.87652438300002));
#277693=CARTESIAN_POINT('Ctrl Pts',(-8.29484965700006,15.2,-6.87754847000001));
#277694=CARTESIAN_POINT('Ctrl Pts',(-8.29723576800006,15.2,-6.87857289700001));
#277695=CARTESIAN_POINT('Ctrl Pts',(-8.29962826300006,15.2,-6.87959765300001));
#277696=CARTESIAN_POINT('Ctrl Pts',(-8.30202713400006,15.2,-6.88062272300002));
#277697=CARTESIAN_POINT('Ctrl Pts',(-8.30443237500005,15.2,-6.88164809600002));
#277698=CARTESIAN_POINT('Ctrl Pts',(-8.30684397800006,15.2,-6.88267375900002));
#277699=CARTESIAN_POINT('Ctrl Pts',(-8.30926193800006,15.2,-6.88369969900001));
#277700=CARTESIAN_POINT('Ctrl Pts',(-8.31168624600006,15.2,-6.88472590400002));
#277701=CARTESIAN_POINT('Ctrl Pts',(-8.31411689600005,15.2,-6.88575236100001));
#277702=CARTESIAN_POINT('Ctrl Pts',(-8.31655388200006,15.2,-6.88677905700001));
#277703=CARTESIAN_POINT('Ctrl Pts',(-8.31899719600005,15.2,-6.88780598100001));
#277704=CARTESIAN_POINT('Ctrl Pts',(-8.32144683000006,15.2,-6.88883311900002));
#277705=CARTESIAN_POINT('Ctrl Pts',(-8.32390277900006,15.2,-6.88986046100001));
#277706=CARTESIAN_POINT('Ctrl Pts',(-8.32636503500006,15.2,-6.89088799200002));
#277707=CARTESIAN_POINT('Ctrl Pts',(-8.32883359200006,15.2,-6.89191570100002));
#277708=CARTESIAN_POINT('Ctrl Pts',(-8.33130844300005,15.2,-6.89294357600001));
#277709=CARTESIAN_POINT('Ctrl Pts',(-8.33378957900005,15.2,-6.89397160500001));
#277710=CARTESIAN_POINT('Ctrl Pts',(-8.33627699700006,15.2,-6.89499977500001));
#277711=CARTESIAN_POINT('Ctrl Pts',(-8.33877068700006,15.2,-6.89602807400002));
#277712=CARTESIAN_POINT('Ctrl Pts',(-8.34127064400005,15.2,-6.89705649000001));
#277713=CARTESIAN_POINT('Ctrl Pts',(-8.34377685900006,15.2,-6.89808501100002));
#277714=CARTESIAN_POINT('Ctrl Pts',(-8.34628932800005,15.2,-6.89911362500002));
#277715=CARTESIAN_POINT('Ctrl Pts',(-8.34880804200005,15.2,-6.90014232000002));
#277716=CARTESIAN_POINT('Ctrl Pts',(-8.35133299600006,15.2,-6.90117108400001));
#277717=CARTESIAN_POINT('Ctrl Pts',(-8.35386418000006,15.2,-6.90219990600001));
#277718=CARTESIAN_POINT('Ctrl Pts',(-8.35640159200006,15.2,-6.90322877200002));
#277719=CARTESIAN_POINT('Ctrl Pts',(-8.35894522100006,15.2,-6.90425767200002));
#277720=CARTESIAN_POINT('Ctrl Pts',(-8.36149506200006,15.2,-6.90528659300002));
#277721=CARTESIAN_POINT('Ctrl Pts',(-8.36405110900006,15.2,-6.90631552400002));
#277722=CARTESIAN_POINT('Ctrl Pts',(-8.36661335300006,15.2,-6.90734445300001));
#277723=CARTESIAN_POINT('Ctrl Pts',(-8.36918179000006,15.2,-6.90837336800002));
#277724=CARTESIAN_POINT('Ctrl Pts',(-8.37175641100006,15.2,-6.90940225800002));
#277725=CARTESIAN_POINT('Ctrl Pts',(-8.37433721100006,15.2,-6.91043111100001));
#277726=CARTESIAN_POINT('Ctrl Pts',(-8.37692418100006,15.2,-6.91145991600001));
#277727=CARTESIAN_POINT('Ctrl Pts',(-8.37951731800005,15.2,-6.91248865900001));
#277728=CARTESIAN_POINT('Ctrl Pts',(-8.38211661100006,15.2,-6.91351733200002));
#277729=CARTESIAN_POINT('Ctrl Pts',(-8.38472205600005,15.2,-6.91454592100002));
#277730=CARTESIAN_POINT('Ctrl Pts',(-8.38733364500006,15.2,-6.91557441500001));
#277731=CARTESIAN_POINT('Ctrl Pts',(-8.38995137300006,15.2,-6.91660280300002));
#277732=CARTESIAN_POINT('Ctrl Pts',(-8.39257523200006,15.2,-6.91763107400002));
#277733=CARTESIAN_POINT('Ctrl Pts',(-8.39520521500006,15.2,-6.91865921400002));
#277734=CARTESIAN_POINT('Ctrl Pts',(-8.39784131700006,15.2,-6.91968721500002));
#277735=CARTESIAN_POINT('Ctrl Pts',(-8.40048352900006,15.2,-6.92071506500002));
#277736=CARTESIAN_POINT('Ctrl Pts',(-8.40313184700006,15.2,-6.92174275100002));
#277737=CARTESIAN_POINT('Ctrl Pts',(-8.40578626200006,15.2,-6.92277026300002));
#277738=CARTESIAN_POINT('Ctrl Pts',(-8.40844676900005,15.2,-6.92379758900002));
#277739=CARTESIAN_POINT('Ctrl Pts',(-8.41111336100006,15.2,-6.92482472000002));
#277740=CARTESIAN_POINT('Ctrl Pts',(-8.41378603100006,15.2,-6.92585164200001));
#277741=CARTESIAN_POINT('Ctrl Pts',(-8.41646477200005,15.2,-6.92687834500001));
#277742=CARTESIAN_POINT('Ctrl Pts',(-8.41914957900006,15.2,-6.92790481800002));
#277743=CARTESIAN_POINT('Ctrl Pts',(-8.42184044300006,15.2,-6.92893105000002));
#277744=CARTESIAN_POINT('Ctrl Pts',(-8.42453736000006,15.2,-6.92995703000002));
#277745=CARTESIAN_POINT('Ctrl Pts',(-8.42724032100006,15.2,-6.93098274800001));
#277746=CARTESIAN_POINT('Ctrl Pts',(-8.42994932200006,15.2,-6.93200819000002));
#277747=CARTESIAN_POINT('Ctrl Pts',(-8.43266435300006,15.2,-6.93303334900002));
#277748=CARTESIAN_POINT('Ctrl Pts',(-8.43538541200006,15.2,-6.93405821000002));
#277749=CARTESIAN_POINT('Ctrl Pts',(-8.43811248900005,15.2,-6.93508276600002));
#277750=CARTESIAN_POINT('Ctrl Pts',(-8.44084557900005,15.2,-6.93610700400002));
#277751=CARTESIAN_POINT('Ctrl Pts',(-8.44358467400006,15.2,-6.93713091300002));
#277752=CARTESIAN_POINT('Ctrl Pts',(-8.44632976900006,15.2,-6.93815448200001));
#277753=CARTESIAN_POINT('Ctrl Pts',(-8.44908085600006,15.2,-6.93917770200001));
#277754=CARTESIAN_POINT('Ctrl Pts',(-8.45183793100006,15.2,-6.94020056100002));
#277755=CARTESIAN_POINT('Ctrl Pts',(-8.45460098500006,15.2,-6.94122304900001));
#277756=CARTESIAN_POINT('Ctrl Pts',(-8.45737001200006,15.2,-6.94224515400002));
#277757=CARTESIAN_POINT('Ctrl Pts',(-8.46014500600005,15.2,-6.94326686700002));
#277758=CARTESIAN_POINT('Ctrl Pts',(-8.46292596100006,15.2,-6.94428817600001));
#277759=CARTESIAN_POINT('Ctrl Pts',(-8.46571286900006,15.2,-6.94530907100001));
#277760=CARTESIAN_POINT('Ctrl Pts',(-8.46850572600006,15.2,-6.94632954200002));
#277761=CARTESIAN_POINT('Ctrl Pts',(-8.47130452200006,15.2,-6.94734957900002));
#277762=CARTESIAN_POINT('Ctrl Pts',(-8.47410925300006,15.2,-6.94836916900002));
#277763=CARTESIAN_POINT('Ctrl Pts',(-8.47691991300006,15.2,-6.94938830400002));
#277764=CARTESIAN_POINT('Ctrl Pts',(-8.47973649400006,15.2,-6.95040697300002));
#277765=CARTESIAN_POINT('Ctrl Pts',(-8.48255899100005,15.2,-6.95142516400002));
#277766=CARTESIAN_POINT('Ctrl Pts',(-8.48538739600006,15.2,-6.95244286800002));
#277767=CARTESIAN_POINT('Ctrl Pts',(-8.48822170400006,15.2,-6.95346007500002));
#277768=CARTESIAN_POINT('Ctrl Pts',(-8.49106190600006,15.2,-6.95447677400002));
#277769=CARTESIAN_POINT('Ctrl Pts',(-8.49390800000006,15.2,-6.95549295400002));
#277770=CARTESIAN_POINT('Ctrl Pts',(-8.49675997600006,15.2,-6.95650860700002));
#277771=CARTESIAN_POINT('Ctrl Pts',(-8.49961782900006,15.2,-6.95752372000002));
#277772=CARTESIAN_POINT('Ctrl Pts',(-8.50248155100006,15.2,-6.95853828600002));
#277773=CARTESIAN_POINT('Ctrl Pts',(-8.50535113900006,15.2,-6.95955229100001));
#277774=CARTESIAN_POINT('Ctrl Pts',(-8.50822658400006,15.2,-6.96056572800002));
#277775=CARTESIAN_POINT('Ctrl Pts',(-8.51110788000006,15.2,-6.96157858500002));
#277776=CARTESIAN_POINT('Ctrl Pts',(-8.51399502100006,15.2,-6.96259085300002));
#277777=CARTESIAN_POINT('Ctrl Pts',(-8.51688800000005,15.2,-6.96360252200002));
#277778=CARTESIAN_POINT('Ctrl Pts',(-8.51978681100006,15.2,-6.96461358000001));
#277779=CARTESIAN_POINT('Ctrl Pts',(-8.52269144900006,15.2,-6.96562402000002));
#277780=CARTESIAN_POINT('Ctrl Pts',(-8.52560190400006,15.2,-6.96663382900002));
#277781=CARTESIAN_POINT('Ctrl Pts',(-8.52851817400006,15.2,-6.96764300000002));
#277782=CARTESIAN_POINT('Ctrl Pts',(-8.53144025100006,15.2,-6.96865152100001));
#277783=CARTESIAN_POINT('Ctrl Pts',(-8.53436812700006,15.2,-6.96965938200002));
#277784=CARTESIAN_POINT('Ctrl Pts',(-8.53730179800005,15.2,-6.97066657500002));
#277785=CARTESIAN_POINT('Ctrl Pts',(-8.54024125700005,15.2,-6.97167308800001));
#277786=CARTESIAN_POINT('Ctrl Pts',(-8.54318649800006,15.2,-6.97267891200001));
#277787=CARTESIAN_POINT('Ctrl Pts',(-8.54613751300005,15.2,-6.97368403700001));
#277788=CARTESIAN_POINT('Ctrl Pts',(-8.54909429800006,15.2,-6.97468845400002));
#277789=CARTESIAN_POINT('Ctrl Pts',(-8.55205684500006,15.2,-6.97569215300001));
#277790=CARTESIAN_POINT('Ctrl Pts',(-8.55502514900006,15.2,-6.97669512400001));
#277791=CARTESIAN_POINT('Ctrl Pts',(-8.55799920200005,15.2,-6.97769735700002));
#277792=CARTESIAN_POINT('Ctrl Pts',(-8.56097900000006,15.2,-6.97869884300002));
#277793=CARTESIAN_POINT('Ctrl Pts',(-8.56396453400006,15.2,-6.97969957100002));
#277794=CARTESIAN_POINT('Ctrl Pts',(-8.56695580000006,15.2,-6.98069953300001));
#277795=CARTESIAN_POINT('Ctrl Pts',(-8.56995279100006,15.2,-6.98169871900002));
#277796=CARTESIAN_POINT('Ctrl Pts',(-8.57295550200006,15.2,-6.98269711800001));
#277797=CARTESIAN_POINT('Ctrl Pts',(-8.57596392500006,15.2,-6.98369472200002));
#277798=CARTESIAN_POINT('Ctrl Pts',(-8.57897805400006,15.2,-6.98469152300002));
#277799=CARTESIAN_POINT('Ctrl Pts',(-8.58199788300006,15.2,-6.98568750700002));
#277800=CARTESIAN_POINT('Ctrl Pts',(-8.58502340600005,15.2,-6.98668266800002));
#277801=CARTESIAN_POINT('Ctrl Pts',(-8.58805461700006,15.2,-6.98767699600002));
#277802=CARTESIAN_POINT('Ctrl Pts',(-8.59109150900006,15.2,-6.98867048200002));
#277803=CARTESIAN_POINT('Ctrl Pts',(-8.59413407600006,15.2,-6.98966311400002));
#277804=CARTESIAN_POINT('Ctrl Pts',(-8.59718231200005,15.2,-6.99065488500001));
#277805=CARTESIAN_POINT('Ctrl Pts',(-8.60023621200006,15.2,-6.99164578600002));
#277806=CARTESIAN_POINT('Ctrl Pts',(-8.60329576800006,15.2,-6.99263580600002));
#277807=CARTESIAN_POINT('Ctrl Pts',(-8.60636097400005,15.2,-6.99362493600002));
#277808=CARTESIAN_POINT('Ctrl Pts',(-8.60943182500005,15.2,-6.99461316800001));
#277809=CARTESIAN_POINT('Ctrl Pts',(-8.61250831400006,15.2,-6.99560049200001));
#277810=CARTESIAN_POINT('Ctrl Pts',(-8.61559043500005,15.2,-6.99658689800001));
#277811=CARTESIAN_POINT('Ctrl Pts',(-8.61867818200006,15.2,-6.99757237900001));
#277812=CARTESIAN_POINT('Ctrl Pts',(-8.62177154800005,15.2,-6.99855692200002));
#277813=CARTESIAN_POINT('Ctrl Pts',(-8.62487052700006,15.2,-6.99954052200002));
#277814=CARTESIAN_POINT('Ctrl Pts',(-8.62797511400006,15.2,-7.00052316700001));
#277815=CARTESIAN_POINT('Ctrl Pts',(-8.63108530200006,15.2,-7.00150485000002));
#277816=CARTESIAN_POINT('Ctrl Pts',(-8.63420108600006,15.2,-7.00248556000002));
#277817=CARTESIAN_POINT('Ctrl Pts',(-8.63732245800006,15.2,-7.00346528800001));
#277818=CARTESIAN_POINT('Ctrl Pts',(-8.64044941400006,15.2,-7.00444402600001));
#277819=CARTESIAN_POINT('Ctrl Pts',(-8.64358194600005,15.2,-7.00542176600001));
#277820=CARTESIAN_POINT('Ctrl Pts',(-8.64672004800006,15.2,-7.00639849700002));
#277821=CARTESIAN_POINT('Ctrl Pts',(-8.64986371500006,15.2,-7.00737421000002));
#277822=CARTESIAN_POINT('Ctrl Pts',(-8.65301294000006,15.2,-7.00834889700002));
#277823=CARTESIAN_POINT('Ctrl Pts',(-8.65616771800006,15.2,-7.00932254900002));
#277824=CARTESIAN_POINT('Ctrl Pts',(-8.65932804200006,15.2,-7.01029515700001));
#277825=CARTESIAN_POINT('Ctrl Pts',(-8.66249390600006,15.2,-7.01126671100001));
#277826=CARTESIAN_POINT('Ctrl Pts',(-8.66566530400006,15.2,-7.01223720400002));
#277827=CARTESIAN_POINT('Ctrl Pts',(-8.66884222900006,15.2,-7.01320662700001));
#277828=CARTESIAN_POINT('Ctrl Pts',(-8.67202467700006,15.2,-7.01417496900002));
#277829=CARTESIAN_POINT('Ctrl Pts',(-8.67521264100005,15.2,-7.01514222400001));
#277830=CARTESIAN_POINT('Ctrl Pts',(-8.67840611400006,15.2,-7.01610838100001));
#277831=CARTESIAN_POINT('Ctrl Pts',(-8.68160509100005,15.2,-7.01707343300002));
#277832=CARTESIAN_POINT('Ctrl Pts',(-8.68480956600006,15.2,-7.01803737000001));
#277833=CARTESIAN_POINT('Ctrl Pts',(-8.68801953200006,15.2,-7.01900018400002));
#277834=CARTESIAN_POINT('Ctrl Pts',(-8.69123498300005,15.2,-7.01996186500002));
#277835=CARTESIAN_POINT('Ctrl Pts',(-8.69445591400006,15.2,-7.02092240600001));
#277836=CARTESIAN_POINT('Ctrl Pts',(-8.69768231900006,15.2,-7.02188179800002));
#277837=CARTESIAN_POINT('Ctrl Pts',(-8.70091419100006,15.2,-7.02284003200001));
#277838=CARTESIAN_POINT('Ctrl Pts',(-8.70415152500006,15.2,-7.02379710000002));
#277839=CARTESIAN_POINT('Ctrl Pts',(-8.70739431400006,15.2,-7.02475299200002));
#277840=CARTESIAN_POINT('Ctrl Pts',(-8.71064255200006,15.2,-7.02570770100002));
#277841=CARTESIAN_POINT('Ctrl Pts',(-8.71389623400006,15.2,-7.02666121800001));
#277842=CARTESIAN_POINT('Ctrl Pts',(-8.71715535200006,15.2,-7.02761353400001));
#277843=CARTESIAN_POINT('Ctrl Pts',(-8.72041990300006,15.2,-7.02856464100002));
#277844=CARTESIAN_POINT('Ctrl Pts',(-8.72368987800006,15.2,-7.02951453100002));
#277845=CARTESIAN_POINT('Ctrl Pts',(-8.72696527300005,15.2,-7.03046319400002));
#277846=CARTESIAN_POINT('Ctrl Pts',(-8.73024608200006,15.2,-7.03141062300002));
#277847=CARTESIAN_POINT('Ctrl Pts',(-8.73353229800006,15.2,-7.03235680900002));
#277848=CARTESIAN_POINT('Ctrl Pts',(-8.73682391500006,15.2,-7.03330174300002));
#277849=CARTESIAN_POINT('Ctrl Pts',(-8.74012092800006,15.2,-7.03424541800001));
#277850=CARTESIAN_POINT('Ctrl Pts',(-8.74342333000006,15.2,-7.03518782500002));
#277851=CARTESIAN_POINT('Ctrl Pts',(-8.74673111600006,15.2,-7.03612895700001));
#277852=CARTESIAN_POINT('Ctrl Pts',(-8.75004427900006,15.2,-7.03706880200002));
#277853=CARTESIAN_POINT('Ctrl Pts',(-8.75336281400006,15.2,-7.03800735500002));
#277854=CARTESIAN_POINT('Ctrl Pts',(-8.75668671600006,15.2,-7.03894460800001));
#277855=CARTESIAN_POINT('Ctrl Pts',(-8.76001597600006,15.2,-7.03988055000002));
#277856=CARTESIAN_POINT('Ctrl Pts',(-8.76335059000006,15.2,-7.04081517500001));
#277857=CARTESIAN_POINT('Ctrl Pts',(-8.76669055200006,15.2,-7.04174847400001));
#277858=CARTESIAN_POINT('Ctrl Pts',(-8.77003585700006,15.2,-7.04268044000001));
#277859=CARTESIAN_POINT('Ctrl Pts',(-8.77338649600006,15.2,-7.04361106300002));
#277860=CARTESIAN_POINT('Ctrl Pts',(-8.77674246700006,15.2,-7.04454033500002));
#277861=CARTESIAN_POINT('Ctrl Pts',(-8.78010376100006,15.2,-7.04546825000002));
#277862=CARTESIAN_POINT('Ctrl Pts',(-8.78347037400006,15.2,-7.04639479800001));
#277863=CARTESIAN_POINT('Ctrl Pts',(-8.78684229800006,15.2,-7.04731997100002));
#277864=CARTESIAN_POINT('Ctrl Pts',(-8.79021953000005,15.2,-7.04824376100002));
#277865=CARTESIAN_POINT('Ctrl Pts',(-8.79360206200005,15.2,-7.04916616100002));
#277866=CARTESIAN_POINT('Ctrl Pts',(-8.79698988900006,15.2,-7.05008716200001));
#277867=CARTESIAN_POINT('Ctrl Pts',(-8.80038300400006,15.2,-7.05100675600002));
#277868=CARTESIAN_POINT('Ctrl Pts',(-8.80378140200006,15.2,-7.05192493600002));
#277869=CARTESIAN_POINT('Ctrl Pts',(-8.80718507800006,15.2,-7.05284169300001));
#277870=CARTESIAN_POINT('Ctrl Pts',(-8.81059402400006,15.2,-7.05375701900002));
#277871=CARTESIAN_POINT('Ctrl Pts',(-8.81400823600006,15.2,-7.05467090600001));
#277872=CARTESIAN_POINT('Ctrl Pts',(-8.81742770700006,15.2,-7.05558334800001));
#277873=CARTESIAN_POINT('Ctrl Pts',(-8.82153737602403,15.2,-7.0566765324596));
#277874=CARTESIAN_POINT('Ctrl Pts',(-8.82565491667507,15.2,-7.05776752231977));
#277875=CARTESIAN_POINT('Ctrl Pts',(-8.82978031732504,15.2,-7.05885630368026));
#277876=CARTESIAN_POINT('Ctrl Pts',(-8.8339135663501,15.2,-7.05994286263952));
#277877=CARTESIAN_POINT('Ctrl Pts',(-8.83805465100006,15.2,-7.06102717900002));
#277878=CARTESIAN_POINT('Ctrl Pts',(-8.84151077400006,15.2,-7.06192927400001));
#277879=CARTESIAN_POINT('Ctrl Pts',(-8.84497210900006,15.2,-7.06282986200002));
#277880=CARTESIAN_POINT('Ctrl Pts',(-8.84843865100006,15.2,-7.06372893100002));
#277881=CARTESIAN_POINT('Ctrl Pts',(-8.85191039400006,15.2,-7.06462647700001));
#277882=CARTESIAN_POINT('Ctrl Pts',(-8.85538733200006,15.2,-7.06552249100002));
#277883=CARTESIAN_POINT('Ctrl Pts',(-8.85886945900005,15.2,-7.06641696400002));
#277884=CARTESIAN_POINT('Ctrl Pts',(-8.86235677000006,15.2,-7.06730989100001));
#277885=CARTESIAN_POINT('Ctrl Pts',(-8.86584925900006,15.2,-7.06820126200002));
#277886=CARTESIAN_POINT('Ctrl Pts',(-8.86934691800005,15.2,-7.06909107000002));
#277887=CARTESIAN_POINT('Ctrl Pts',(-8.87284974500006,15.2,-7.06997930700001));
#277888=CARTESIAN_POINT('Ctrl Pts',(-8.87635773200006,15.2,-7.07086596600002));
#277889=CARTESIAN_POINT('Ctrl Pts',(-8.87987087300005,15.2,-7.07175104100001));
#277890=CARTESIAN_POINT('Ctrl Pts',(-8.88338916200006,15.2,-7.07263452100002));
#277891=CARTESIAN_POINT('Ctrl Pts',(-8.88691259400006,15.2,-7.07351640200002));
#277892=CARTESIAN_POINT('Ctrl Pts',(-8.89044116400006,15.2,-7.07439667400001));
#277893=CARTESIAN_POINT('Ctrl Pts',(-8.89397486600006,15.2,-7.07527533000002));
#277894=CARTESIAN_POINT('Ctrl Pts',(-8.89751369200006,15.2,-7.07615236300001));
#277895=CARTESIAN_POINT('Ctrl Pts',(-8.90105763800005,15.2,-7.07702776600001));
#277896=CARTESIAN_POINT('Ctrl Pts',(-8.90460669800006,15.2,-7.07790152900002));
#277897=CARTESIAN_POINT('Ctrl Pts',(-8.90816086700006,15.2,-7.07877364900002));
#277898=CARTESIAN_POINT('Ctrl Pts',(-8.91172013800006,15.2,-7.07964411500001));
#277899=CARTESIAN_POINT('Ctrl Pts',(-8.91528450600006,15.2,-7.08051292100001));
#277900=CARTESIAN_POINT('Ctrl Pts',(-8.91885396500006,15.2,-7.08138005800001));
#277901=CARTESIAN_POINT('Ctrl Pts',(-8.92242850800006,15.2,-7.08224552100001));
#277902=CARTESIAN_POINT('Ctrl Pts',(-8.92600813200006,15.2,-7.08310930200001));
#277903=CARTESIAN_POINT('Ctrl Pts',(-8.92959282900006,15.2,-7.08397139300001));
#277904=CARTESIAN_POINT('Ctrl Pts',(-8.93318259400005,15.2,-7.08483178600002));
#277905=CARTESIAN_POINT('Ctrl Pts',(-8.93677742100006,15.2,-7.08569047400001));
#277906=CARTESIAN_POINT('Ctrl Pts',(-8.94037730400006,15.2,-7.08654745200001));
#277907=CARTESIAN_POINT('Ctrl Pts',(-8.94398223900006,15.2,-7.08740271100002));
#277908=CARTESIAN_POINT('Ctrl Pts',(-8.94759221900006,15.2,-7.08825624300002));
#277909=CARTESIAN_POINT('Ctrl Pts',(-8.95120723800006,15.2,-7.08910804300002));
#277910=CARTESIAN_POINT('Ctrl Pts',(-8.95482729200006,15.2,-7.08995810200002));
#277911=CARTESIAN_POINT('Ctrl Pts',(-8.95845237400006,15.2,-7.09080641500002));
#277912=CARTESIAN_POINT('Ctrl Pts',(-8.96208247800006,15.2,-7.09165297200002));
#277913=CARTESIAN_POINT('Ctrl Pts',(-8.96571759800005,15.2,-7.09249776700001));
#277914=CARTESIAN_POINT('Ctrl Pts',(-8.96935772900006,15.2,-7.09334079100002));
#277915=CARTESIAN_POINT('Ctrl Pts',(-8.97300286400006,15.2,-7.09418203900002));
#277916=CARTESIAN_POINT('Ctrl Pts',(-8.97665299700006,15.2,-7.09502150300001));
#277917=CARTESIAN_POINT('Ctrl Pts',(-8.98030812400006,15.2,-7.09585917500001));
#277918=CARTESIAN_POINT('Ctrl Pts',(-8.98396824000006,15.2,-7.09669505000001));
#277919=CARTESIAN_POINT('Ctrl Pts',(-8.98763333900006,15.2,-7.09752912300001));
#277920=CARTESIAN_POINT('Ctrl Pts',(-8.99130341600006,15.2,-7.09836138400001));
#277921=CARTESIAN_POINT('Ctrl Pts',(-8.99497846500006,15.2,-7.09919182900002));
#277922=CARTESIAN_POINT('Ctrl Pts',(-8.99865848200006,15.2,-7.10002045100002));
#277923=CARTESIAN_POINT('Ctrl Pts',(-9.00234345900006,15.2,-7.10084724000002));
#277924=CARTESIAN_POINT('Ctrl Pts',(-9.00603338900006,15.2,-7.10167218900001));
#277925=CARTESIAN_POINT('Ctrl Pts',(-9.00972826500006,15.2,-7.10249528800002));
#277926=CARTESIAN_POINT('Ctrl Pts',(-9.01342808000006,15.2,-7.10331652800001));
#277927=CARTESIAN_POINT('Ctrl Pts',(-9.01713282900005,15.2,-7.10413590400002));
#277928=CARTESIAN_POINT('Ctrl Pts',(-9.02084250600005,15.2,-7.10495340800002));
#277929=CARTESIAN_POINT('Ctrl Pts',(-9.02455710700006,15.2,-7.10576903500002));
#277930=CARTESIAN_POINT('Ctrl Pts',(-9.02827662900006,15.2,-7.10658278400001));
#277931=CARTESIAN_POINT('Ctrl Pts',(-9.03200107200006,15.2,-7.10739465100002));
#277932=CARTESIAN_POINT('Ctrl Pts',(-9.03498456200006,15.2,-7.10804263900001));
#277933=CARTESIAN_POINT('Ctrl Pts',(-9.03722439200006,15.2,-7.10852778400002));
#277934=CARTESIAN_POINT('Ctrl Pts',(-9.03871859600006,15.2,-7.10885083600001));
#277935=CARTESIAN_POINT('Ctrl Pts',(-9.03946594400006,15.2,-7.10901226900001));
#277936=CARTESIAN_POINT('Ctrl Pts',(-8.56667971000006,15.2,-5.85257411400002));
#277937=CARTESIAN_POINT('Ctrl Pts',(-8.56667971000006,11.6,-5.85257411400002));
#277938=CARTESIAN_POINT('Ctrl Pts',(-8.56681469200005,15.2,-5.85268447900001));
#277939=CARTESIAN_POINT('Ctrl Pts',(-8.56681469200005,11.6,-5.85268447900001));
#277940=CARTESIAN_POINT('Ctrl Pts',(-8.56708931800006,15.2,-5.85290912800002));
#277941=CARTESIAN_POINT('Ctrl Pts',(-8.56708931800006,11.6,-5.85290912800002));
#277942=CARTESIAN_POINT('Ctrl Pts',(-8.56750527400006,15.2,-5.85324973300001));
#277943=CARTESIAN_POINT('Ctrl Pts',(-8.56750527400006,11.6,-5.85324973300001));
#277944=CARTESIAN_POINT('Ctrl Pts',(-8.56806526200005,15.2,-5.85370897400002));
#277945=CARTESIAN_POINT('Ctrl Pts',(-8.56806526200005,11.6,-5.85370897400002));
#277946=CARTESIAN_POINT('Ctrl Pts',(-8.56877298400006,15.2,-5.85429055400001));
#277947=CARTESIAN_POINT('Ctrl Pts',(-8.56877298400006,11.6,-5.85429055400001));
#277948=CARTESIAN_POINT('Ctrl Pts',(-8.56949158200005,15.2,-5.85488228200001));
#277949=CARTESIAN_POINT('Ctrl Pts',(-8.56949158200005,11.6,-5.85488228200001));
#277950=CARTESIAN_POINT('Ctrl Pts',(-8.57021692700006,15.2,-5.85548078500001));
#277951=CARTESIAN_POINT('Ctrl Pts',(-8.57021692700006,11.6,-5.85548078500001));
#277952=CARTESIAN_POINT('Ctrl Pts',(-8.57094898300006,15.2,-5.85608606100001));
#277953=CARTESIAN_POINT('Ctrl Pts',(-8.57094898300006,11.6,-5.85608606100001));
#277954=CARTESIAN_POINT('Ctrl Pts',(-8.57168771900006,15.2,-5.85669810600002));
#277955=CARTESIAN_POINT('Ctrl Pts',(-8.57168771900006,11.6,-5.85669810600002));
#277956=CARTESIAN_POINT('Ctrl Pts',(-8.57243310300005,15.2,-5.85731691800002));
#277957=CARTESIAN_POINT('Ctrl Pts',(-8.57243310300005,11.6,-5.85731691800002));
#277958=CARTESIAN_POINT('Ctrl Pts',(-8.57318510400006,15.2,-5.85794249300001));
#277959=CARTESIAN_POINT('Ctrl Pts',(-8.57318510400006,11.6,-5.85794249300001));
#277960=CARTESIAN_POINT('Ctrl Pts',(-8.57394368900006,15.2,-5.85857482800002));
#277961=CARTESIAN_POINT('Ctrl Pts',(-8.57394368900006,11.6,-5.85857482800002));
#277962=CARTESIAN_POINT('Ctrl Pts',(-8.57470882600006,15.2,-5.85921392000002));
#277963=CARTESIAN_POINT('Ctrl Pts',(-8.57470882600006,11.6,-5.85921392000002));
#277964=CARTESIAN_POINT('Ctrl Pts',(-8.57548048600006,15.2,-5.85985976500002));
#277965=CARTESIAN_POINT('Ctrl Pts',(-8.57548048600006,11.6,-5.85985976500002));
#277966=CARTESIAN_POINT('Ctrl Pts',(-8.57625863500006,15.2,-5.86051236100002));
#277967=CARTESIAN_POINT('Ctrl Pts',(-8.57625863500006,11.6,-5.86051236100002));
#277968=CARTESIAN_POINT('Ctrl Pts',(-8.57704324400006,15.2,-5.86117170400002));
#277969=CARTESIAN_POINT('Ctrl Pts',(-8.57704324400006,11.6,-5.86117170400002));
#277970=CARTESIAN_POINT('Ctrl Pts',(-8.57783428100005,15.2,-5.86183779100002));
#277971=CARTESIAN_POINT('Ctrl Pts',(-8.57783428100005,11.6,-5.86183779100002));
#277972=CARTESIAN_POINT('Ctrl Pts',(-8.57863171500006,15.2,-5.86251061900001));
#277973=CARTESIAN_POINT('Ctrl Pts',(-8.57863171500006,11.6,-5.86251061900001));
#277974=CARTESIAN_POINT('Ctrl Pts',(-8.57943551500006,15.2,-5.86319018600002));
#277975=CARTESIAN_POINT('Ctrl Pts',(-8.57943551500006,11.6,-5.86319018600002));
#277976=CARTESIAN_POINT('Ctrl Pts',(-8.58024565200006,15.2,-5.86387648600001));
#277977=CARTESIAN_POINT('Ctrl Pts',(-8.58024565200006,11.6,-5.86387648600001));
#277978=CARTESIAN_POINT('Ctrl Pts',(-8.58106209400006,15.2,-5.86456951900002));
#277979=CARTESIAN_POINT('Ctrl Pts',(-8.58106209400006,11.6,-5.86456951900002));
#277980=CARTESIAN_POINT('Ctrl Pts',(-8.58188481200006,15.2,-5.86526928000002));
#277981=CARTESIAN_POINT('Ctrl Pts',(-8.58188481200006,11.6,-5.86526928000002));
#277982=CARTESIAN_POINT('Ctrl Pts',(-8.58271377600006,15.2,-5.86597576500001));
#277983=CARTESIAN_POINT('Ctrl Pts',(-8.58271377600006,11.6,-5.86597576500001));
#277984=CARTESIAN_POINT('Ctrl Pts',(-8.58354895500005,15.2,-5.86668897300001));
#277985=CARTESIAN_POINT('Ctrl Pts',(-8.58354895500005,11.6,-5.86668897300001));
#277986=CARTESIAN_POINT('Ctrl Pts',(-8.58439032000006,15.2,-5.86740890000002));
#277987=CARTESIAN_POINT('Ctrl Pts',(-8.58439032000006,11.6,-5.86740890000002));
#277988=CARTESIAN_POINT('Ctrl Pts',(-8.58523784000005,15.2,-5.86813554200001));
#277989=CARTESIAN_POINT('Ctrl Pts',(-8.58523784000005,11.6,-5.86813554200001));
#277990=CARTESIAN_POINT('Ctrl Pts',(-8.58609148800005,15.2,-5.86886889800001));
#277991=CARTESIAN_POINT('Ctrl Pts',(-8.58609148800005,11.6,-5.86886889800001));
#277992=CARTESIAN_POINT('Ctrl Pts',(-8.58695123200006,15.2,-5.86960896200001));
#277993=CARTESIAN_POINT('Ctrl Pts',(-8.58695123200006,11.6,-5.86960896200001));
#277994=CARTESIAN_POINT('Ctrl Pts',(-8.58781704400006,15.2,-5.87035573200002));
#277995=CARTESIAN_POINT('Ctrl Pts',(-8.58781704400006,11.6,-5.87035573200002));
#277996=CARTESIAN_POINT('Ctrl Pts',(-8.58868889600006,15.2,-5.87110920600002));
#277997=CARTESIAN_POINT('Ctrl Pts',(-8.58868889600006,11.6,-5.87110920600002));
#277998=CARTESIAN_POINT('Ctrl Pts',(-8.58956675800006,15.2,-5.87186938100002));
#277999=CARTESIAN_POINT('Ctrl Pts',(-8.58956675800006,11.6,-5.87186938100002));
#278000=CARTESIAN_POINT('Ctrl Pts',(-8.59045060000006,15.2,-5.87263625100002));
#278001=CARTESIAN_POINT('Ctrl Pts',(-8.59045060000006,11.6,-5.87263625100002));
#278002=CARTESIAN_POINT('Ctrl Pts',(-8.59134039400006,15.2,-5.87340981600001));
#278003=CARTESIAN_POINT('Ctrl Pts',(-8.59134039400006,11.6,-5.87340981600001));
#278004=CARTESIAN_POINT('Ctrl Pts',(-8.59223611300006,15.2,-5.87419007000002));
#278005=CARTESIAN_POINT('Ctrl Pts',(-8.59223611300006,11.6,-5.87419007000002));
#278006=CARTESIAN_POINT('Ctrl Pts',(-8.59313772800006,15.2,-5.87497701200002));
#278007=CARTESIAN_POINT('Ctrl Pts',(-8.59313772800006,11.6,-5.87497701200002));
#278008=CARTESIAN_POINT('Ctrl Pts',(-8.59404520800006,15.2,-5.87577063900002));
#278009=CARTESIAN_POINT('Ctrl Pts',(-8.59404520800006,11.6,-5.87577063900002));
#278010=CARTESIAN_POINT('Ctrl Pts',(-8.59495852900006,15.2,-5.87657094700001));
#278011=CARTESIAN_POINT('Ctrl Pts',(-8.59495852900006,11.6,-5.87657094700001));
#278012=CARTESIAN_POINT('Ctrl Pts',(-8.59587766000006,15.2,-5.87737793200001));
#278013=CARTESIAN_POINT('Ctrl Pts',(-8.59587766000006,11.6,-5.87737793200001));
#278014=CARTESIAN_POINT('Ctrl Pts',(-8.59680257500005,15.2,-5.87819159300001));
#278015=CARTESIAN_POINT('Ctrl Pts',(-8.59680257500005,11.6,-5.87819159300001));
#278016=CARTESIAN_POINT('Ctrl Pts',(-8.59773324400006,15.2,-5.87901192500001));
#278017=CARTESIAN_POINT('Ctrl Pts',(-8.59773324400006,11.6,-5.87901192500001));
#278018=CARTESIAN_POINT('Ctrl Pts',(-8.59866964200006,15.2,-5.87983892500001));
#278019=CARTESIAN_POINT('Ctrl Pts',(-8.59866964200006,11.6,-5.87983892500001));
#278020=CARTESIAN_POINT('Ctrl Pts',(-8.59961174000006,15.2,-5.88067259100002));
#278021=CARTESIAN_POINT('Ctrl Pts',(-8.59961174000006,11.6,-5.88067259100002));
#278022=CARTESIAN_POINT('Ctrl Pts',(-8.60055950900006,15.2,-5.88151292000001));
#278023=CARTESIAN_POINT('Ctrl Pts',(-8.60055950900006,11.6,-5.88151292000001));
#278024=CARTESIAN_POINT('Ctrl Pts',(-8.60151292500005,15.2,-5.88235990700002));
#278025=CARTESIAN_POINT('Ctrl Pts',(-8.60151292500005,11.6,-5.88235990700002));
#278026=CARTESIAN_POINT('Ctrl Pts',(-8.60247195900006,15.2,-5.88321355000001));
#278027=CARTESIAN_POINT('Ctrl Pts',(-8.60247195900006,11.6,-5.88321355000001));
#278028=CARTESIAN_POINT('Ctrl Pts',(-8.60343658500006,15.2,-5.88407384600002));
#278029=CARTESIAN_POINT('Ctrl Pts',(-8.60343658500006,11.6,-5.88407384600002));
#278030=CARTESIAN_POINT('Ctrl Pts',(-8.60440677400006,15.2,-5.88494079200002));
#278031=CARTESIAN_POINT('Ctrl Pts',(-8.60440677400006,11.6,-5.88494079200002));
#278032=CARTESIAN_POINT('Ctrl Pts',(-8.60538250200005,15.2,-5.88581438400002));
#278033=CARTESIAN_POINT('Ctrl Pts',(-8.60538250200005,11.6,-5.88581438400002));
#278034=CARTESIAN_POINT('Ctrl Pts',(-8.60636373900006,15.2,-5.88669461900002));
#278035=CARTESIAN_POINT('Ctrl Pts',(-8.60636373900006,11.6,-5.88669461900002));
#278036=CARTESIAN_POINT('Ctrl Pts',(-8.60735046200006,15.2,-5.88758149500002));
#278037=CARTESIAN_POINT('Ctrl Pts',(-8.60735046200006,11.6,-5.88758149500002));
#278038=CARTESIAN_POINT('Ctrl Pts',(-8.60834264200006,15.2,-5.88847500800001));
#278039=CARTESIAN_POINT('Ctrl Pts',(-8.60834264200006,11.6,-5.88847500800001));
#278040=CARTESIAN_POINT('Ctrl Pts',(-8.60934025400006,15.2,-5.88937515500002));
#278041=CARTESIAN_POINT('Ctrl Pts',(-8.60934025400006,11.6,-5.88937515500002));
#278042=CARTESIAN_POINT('Ctrl Pts',(-8.61034327100005,15.2,-5.89028193300001));
#278043=CARTESIAN_POINT('Ctrl Pts',(-8.61034327100005,11.6,-5.89028193300001));
#278044=CARTESIAN_POINT('Ctrl Pts',(-8.61135166800005,15.2,-5.89119533800002));
#278045=CARTESIAN_POINT('Ctrl Pts',(-8.61135166800005,11.6,-5.89119533800002));
#278046=CARTESIAN_POINT('Ctrl Pts',(-8.61236541700006,15.2,-5.89211536900001));
#278047=CARTESIAN_POINT('Ctrl Pts',(-8.61236541700006,11.6,-5.89211536900001));
#278048=CARTESIAN_POINT('Ctrl Pts',(-8.61338449500006,15.2,-5.89304202000001));
#278049=CARTESIAN_POINT('Ctrl Pts',(-8.61338449500006,11.6,-5.89304202000001));
#278050=CARTESIAN_POINT('Ctrl Pts',(-8.61440887300006,15.2,-5.89397529000002));
#278051=CARTESIAN_POINT('Ctrl Pts',(-8.61440887300006,11.6,-5.89397529000002));
#278052=CARTESIAN_POINT('Ctrl Pts',(-8.61543852900006,15.2,-5.89491517500001));
#278053=CARTESIAN_POINT('Ctrl Pts',(-8.61543852900006,11.6,-5.89491517500001));
#278054=CARTESIAN_POINT('Ctrl Pts',(-8.61647343400006,15.2,-5.89586167100002));
#278055=CARTESIAN_POINT('Ctrl Pts',(-8.61647343400006,11.6,-5.89586167100002));
#278056=CARTESIAN_POINT('Ctrl Pts',(-8.61751356400006,15.2,-5.89681477700001));
#278057=CARTESIAN_POINT('Ctrl Pts',(-8.61751356400006,11.6,-5.89681477700001));
#278058=CARTESIAN_POINT('Ctrl Pts',(-8.61855889400006,15.2,-5.89777448800002));
#278059=CARTESIAN_POINT('Ctrl Pts',(-8.61855889400006,11.6,-5.89777448800002));
#278060=CARTESIAN_POINT('Ctrl Pts',(-8.61960939900005,15.2,-5.89874080200002));
#278061=CARTESIAN_POINT('Ctrl Pts',(-8.61960939900005,11.6,-5.89874080200002));
#278062=CARTESIAN_POINT('Ctrl Pts',(-8.62066505300006,15.2,-5.89971371600001));
#278063=CARTESIAN_POINT('Ctrl Pts',(-8.62066505300006,11.6,-5.89971371600001));
#278064=CARTESIAN_POINT('Ctrl Pts',(-8.62172583200006,15.2,-5.90069322500002));
#278065=CARTESIAN_POINT('Ctrl Pts',(-8.62172583200006,11.6,-5.90069322500002));
#278066=CARTESIAN_POINT('Ctrl Pts',(-8.62279170900005,15.2,-5.90167932800002));
#278067=CARTESIAN_POINT('Ctrl Pts',(-8.62279170900005,11.6,-5.90167932800002));
#278068=CARTESIAN_POINT('Ctrl Pts',(-8.62386266200006,15.2,-5.90267202100001));
#278069=CARTESIAN_POINT('Ctrl Pts',(-8.62386266200006,11.6,-5.90267202100001));
#278070=CARTESIAN_POINT('Ctrl Pts',(-8.62493866400006,15.2,-5.90367130100002));
#278071=CARTESIAN_POINT('Ctrl Pts',(-8.62493866400006,11.6,-5.90367130100002));
#278072=CARTESIAN_POINT('Ctrl Pts',(-8.62601969300006,15.2,-5.90467716400001));
#278073=CARTESIAN_POINT('Ctrl Pts',(-8.62601969300006,11.6,-5.90467716400001));
#278074=CARTESIAN_POINT('Ctrl Pts',(-8.62710572200006,15.2,-5.90568960800002));
#278075=CARTESIAN_POINT('Ctrl Pts',(-8.62710572200006,11.6,-5.90568960800002));
#278076=CARTESIAN_POINT('Ctrl Pts',(-8.62819672800006,15.2,-5.90670862900001));
#278077=CARTESIAN_POINT('Ctrl Pts',(-8.62819672800006,11.6,-5.90670862900001));
#278078=CARTESIAN_POINT('Ctrl Pts',(-8.62929268600006,15.2,-5.90773422500002));
#278079=CARTESIAN_POINT('Ctrl Pts',(-8.62929268600006,11.6,-5.90773422500002));
#278080=CARTESIAN_POINT('Ctrl Pts',(-8.63039357300006,15.2,-5.90876639200002));
#278081=CARTESIAN_POINT('Ctrl Pts',(-8.63039357300006,11.6,-5.90876639200002));
#278082=CARTESIAN_POINT('Ctrl Pts',(-8.63149936300006,15.2,-5.90980512700002));
#278083=CARTESIAN_POINT('Ctrl Pts',(-8.63149936300006,11.6,-5.90980512700002));
#278084=CARTESIAN_POINT('Ctrl Pts',(-8.63261003400006,15.2,-5.91085042600002));
#278085=CARTESIAN_POINT('Ctrl Pts',(-8.63261003400006,11.6,-5.91085042600002));
#278086=CARTESIAN_POINT('Ctrl Pts',(-8.63372556100006,15.2,-5.91190228700002));
#278087=CARTESIAN_POINT('Ctrl Pts',(-8.63372556100006,11.6,-5.91190228700002));
#278088=CARTESIAN_POINT('Ctrl Pts',(-8.63484592000006,15.2,-5.91296070700002));
#278089=CARTESIAN_POINT('Ctrl Pts',(-8.63484592000006,11.6,-5.91296070700002));
#278090=CARTESIAN_POINT('Ctrl Pts',(-8.63597108800005,15.2,-5.91402568300002));
#278091=CARTESIAN_POINT('Ctrl Pts',(-8.63597108800005,11.6,-5.91402568300002));
#278092=CARTESIAN_POINT('Ctrl Pts',(-8.63710104100005,15.2,-5.91509721000002));
#278093=CARTESIAN_POINT('Ctrl Pts',(-8.63710104100005,11.6,-5.91509721000002));
#278094=CARTESIAN_POINT('Ctrl Pts',(-8.63823575600006,15.2,-5.91617528700001));
#278095=CARTESIAN_POINT('Ctrl Pts',(-8.63823575600006,11.6,-5.91617528700001));
#278096=CARTESIAN_POINT('Ctrl Pts',(-8.63937520800006,15.2,-5.91725991000001));
#278097=CARTESIAN_POINT('Ctrl Pts',(-8.63937520800006,11.6,-5.91725991000001));
#278098=CARTESIAN_POINT('Ctrl Pts',(-8.64051937700006,15.2,-5.91835107600001));
#278099=CARTESIAN_POINT('Ctrl Pts',(-8.64051937700006,11.6,-5.91835107600001));
#278100=CARTESIAN_POINT('Ctrl Pts',(-8.64166823700005,15.2,-5.91944878100002));
#278101=CARTESIAN_POINT('Ctrl Pts',(-8.64166823700005,11.6,-5.91944878100002));
#278102=CARTESIAN_POINT('Ctrl Pts',(-8.64282176500006,15.2,-5.92055302300002));
#278103=CARTESIAN_POINT('Ctrl Pts',(-8.64282176500006,11.6,-5.92055302300002));
#278104=CARTESIAN_POINT('Ctrl Pts',(-8.64397994000005,15.2,-5.92166379800001));
#278105=CARTESIAN_POINT('Ctrl Pts',(-8.64397994000005,11.6,-5.92166379800001));
#278106=CARTESIAN_POINT('Ctrl Pts',(-8.64514273700006,15.2,-5.92278110300001));
#278107=CARTESIAN_POINT('Ctrl Pts',(-8.64514273700006,11.6,-5.92278110300001));
#278108=CARTESIAN_POINT('Ctrl Pts',(-8.64631013400006,15.2,-5.92390493600002));
#278109=CARTESIAN_POINT('Ctrl Pts',(-8.64631013400006,11.6,-5.92390493600002));
#278110=CARTESIAN_POINT('Ctrl Pts',(-8.64748210800006,15.2,-5.92503529300001));
#278111=CARTESIAN_POINT('Ctrl Pts',(-8.64748210800006,11.6,-5.92503529300001));
#278112=CARTESIAN_POINT('Ctrl Pts',(-8.64865863600006,15.2,-5.92617216900001));
#278113=CARTESIAN_POINT('Ctrl Pts',(-8.64865863600006,11.6,-5.92617216900001));
#278114=CARTESIAN_POINT('Ctrl Pts',(-8.64983969600006,15.2,-5.92731556500001));
#278115=CARTESIAN_POINT('Ctrl Pts',(-8.64983969600006,11.6,-5.92731556500001));
#278116=CARTESIAN_POINT('Ctrl Pts',(-8.65102526500005,15.2,-5.92846547300002));
#278117=CARTESIAN_POINT('Ctrl Pts',(-8.65102526500005,11.6,-5.92846547300002));
#278118=CARTESIAN_POINT('Ctrl Pts',(-8.65221532200006,15.2,-5.92962189400002));
#278119=CARTESIAN_POINT('Ctrl Pts',(-8.65221532200006,11.6,-5.92962189400002));
#278120=CARTESIAN_POINT('Ctrl Pts',(-8.65340984400006,15.2,-5.93078482300001));
#278121=CARTESIAN_POINT('Ctrl Pts',(-8.65340984400006,11.6,-5.93078482300001));
#278122=CARTESIAN_POINT('Ctrl Pts',(-8.65460880700006,15.2,-5.93195425700002));
#278123=CARTESIAN_POINT('Ctrl Pts',(-8.65460880700006,11.6,-5.93195425700002));
#278124=CARTESIAN_POINT('Ctrl Pts',(-8.65581219200006,15.2,-5.93313019200002));
#278125=CARTESIAN_POINT('Ctrl Pts',(-8.65581219200006,11.6,-5.93313019200002));
#278126=CARTESIAN_POINT('Ctrl Pts',(-8.65701997300006,15.2,-5.93431262700002));
#278127=CARTESIAN_POINT('Ctrl Pts',(-8.65701997300006,11.6,-5.93431262700002));
#278128=CARTESIAN_POINT('Ctrl Pts',(-8.65823213200006,15.2,-5.93550155700001));
#278129=CARTESIAN_POINT('Ctrl Pts',(-8.65823213200006,11.6,-5.93550155700001));
#278130=CARTESIAN_POINT('Ctrl Pts',(-8.65944864600005,15.2,-5.93669697900002));
#278131=CARTESIAN_POINT('Ctrl Pts',(-8.65944864600005,11.6,-5.93669697900002));
#278132=CARTESIAN_POINT('Ctrl Pts',(-8.66066949100006,15.2,-5.93789889000002));
#278133=CARTESIAN_POINT('Ctrl Pts',(-8.66066949100006,11.6,-5.93789889000002));
#278134=CARTESIAN_POINT('Ctrl Pts',(-8.66189464700006,15.2,-5.93910728900001));
#278135=CARTESIAN_POINT('Ctrl Pts',(-8.66189464700006,11.6,-5.93910728900001));
#278136=CARTESIAN_POINT('Ctrl Pts',(-8.66312409300006,15.2,-5.94032216900001));
#278137=CARTESIAN_POINT('Ctrl Pts',(-8.66312409300006,11.6,-5.94032216900001));
#278138=CARTESIAN_POINT('Ctrl Pts',(-8.66435780700006,15.2,-5.94154352900001));
#278139=CARTESIAN_POINT('Ctrl Pts',(-8.66435780700006,11.6,-5.94154352900001));
#278140=CARTESIAN_POINT('Ctrl Pts',(-8.66559576700006,15.2,-5.94277136600001));
#278141=CARTESIAN_POINT('Ctrl Pts',(-8.66559576700006,11.6,-5.94277136600001));
#278142=CARTESIAN_POINT('Ctrl Pts',(-8.66683795200006,15.2,-5.94400567600001));
#278143=CARTESIAN_POINT('Ctrl Pts',(-8.66683795200006,11.6,-5.94400567600001));
#278144=CARTESIAN_POINT('Ctrl Pts',(-8.66808434000006,15.2,-5.94524645700002));
#278145=CARTESIAN_POINT('Ctrl Pts',(-8.66808434000006,11.6,-5.94524645700002));
#278146=CARTESIAN_POINT('Ctrl Pts',(-8.66933491100006,15.2,-5.94649370400001));
#278147=CARTESIAN_POINT('Ctrl Pts',(-8.66933491100006,11.6,-5.94649370400001));
#278148=CARTESIAN_POINT('Ctrl Pts',(-8.67058964300006,15.2,-5.94774741600002));
#278149=CARTESIAN_POINT('Ctrl Pts',(-8.67058964300006,11.6,-5.94774741600002));
#278150=CARTESIAN_POINT('Ctrl Pts',(-8.67184851500006,15.2,-5.94900758800001));
#278151=CARTESIAN_POINT('Ctrl Pts',(-8.67184851500006,11.6,-5.94900758800001));
#278152=CARTESIAN_POINT('Ctrl Pts',(-8.67311150600005,15.2,-5.95027421800002));
#278153=CARTESIAN_POINT('Ctrl Pts',(-8.67311150600005,11.6,-5.95027421800002));
#278154=CARTESIAN_POINT('Ctrl Pts',(-8.67437859500006,15.2,-5.95154730200001));
#278155=CARTESIAN_POINT('Ctrl Pts',(-8.67437859500006,11.6,-5.95154730200001));
#278156=CARTESIAN_POINT('Ctrl Pts',(-8.67564976200006,15.2,-5.95282683700002));
#278157=CARTESIAN_POINT('Ctrl Pts',(-8.67564976200006,11.6,-5.95282683700002));
#278158=CARTESIAN_POINT('Ctrl Pts',(-8.67692498600006,15.2,-5.95411282200002));
#278159=CARTESIAN_POINT('Ctrl Pts',(-8.67692498600006,11.6,-5.95411282200002));
#278160=CARTESIAN_POINT('Ctrl Pts',(-8.67820424500006,15.2,-5.95540525000001));
#278161=CARTESIAN_POINT('Ctrl Pts',(-8.67820424500006,11.6,-5.95540525000001));
#278162=CARTESIAN_POINT('Ctrl Pts',(-8.67948752100006,15.2,-5.95670412000001));
#278163=CARTESIAN_POINT('Ctrl Pts',(-8.67948752100006,11.6,-5.95670412000001));
#278164=CARTESIAN_POINT('Ctrl Pts',(-8.68077479100006,15.2,-5.95800942900001));
#278165=CARTESIAN_POINT('Ctrl Pts',(-8.68077479100006,11.6,-5.95800942900001));
#278166=CARTESIAN_POINT('Ctrl Pts',(-8.68206603400006,15.2,-5.95932117300002));
#278167=CARTESIAN_POINT('Ctrl Pts',(-8.68206603400006,11.6,-5.95932117300002));
#278168=CARTESIAN_POINT('Ctrl Pts',(-8.68336123200006,15.2,-5.96063934900001));
#278169=CARTESIAN_POINT('Ctrl Pts',(-8.68336123200006,11.6,-5.96063934900001));
#278170=CARTESIAN_POINT('Ctrl Pts',(-8.68466036500006,15.2,-5.96196395400002));
#278171=CARTESIAN_POINT('Ctrl Pts',(-8.68466036500006,11.6,-5.96196395400002));
#278172=CARTESIAN_POINT('Ctrl Pts',(-8.68596340900006,15.2,-5.96329498600002));
#278173=CARTESIAN_POINT('Ctrl Pts',(-8.68596340900006,11.6,-5.96329498600002));
#278174=CARTESIAN_POINT('Ctrl Pts',(-8.68727034800006,15.2,-5.96463244000002));
#278175=CARTESIAN_POINT('Ctrl Pts',(-8.68727034800006,11.6,-5.96463244000002));
#278176=CARTESIAN_POINT('Ctrl Pts',(-8.68858116100006,15.2,-5.96597631400002));
#278177=CARTESIAN_POINT('Ctrl Pts',(-8.68858116100006,11.6,-5.96597631400002));
#278178=CARTESIAN_POINT('Ctrl Pts',(-8.68989582600006,15.2,-5.96732660300002));
#278179=CARTESIAN_POINT('Ctrl Pts',(-8.68989582600006,11.6,-5.96732660300002));
#278180=CARTESIAN_POINT('Ctrl Pts',(-8.69121432400006,15.2,-5.96868330600002));
#278181=CARTESIAN_POINT('Ctrl Pts',(-8.69121432400006,11.6,-5.96868330600002));
#278182=CARTESIAN_POINT('Ctrl Pts',(-8.69253663700006,15.2,-5.97004641800002));
#278183=CARTESIAN_POINT('Ctrl Pts',(-8.69253663700006,11.6,-5.97004641800002));
#278184=CARTESIAN_POINT('Ctrl Pts',(-8.69386274300006,15.2,-5.97141593800002));
#278185=CARTESIAN_POINT('Ctrl Pts',(-8.69386274300006,11.6,-5.97141593800002));
#278186=CARTESIAN_POINT('Ctrl Pts',(-8.69519262200006,15.2,-5.97279186100002));
#278187=CARTESIAN_POINT('Ctrl Pts',(-8.69519262200006,11.6,-5.97279186100002));
#278188=CARTESIAN_POINT('Ctrl Pts',(-8.69652625700006,15.2,-5.97417418400001));
#278189=CARTESIAN_POINT('Ctrl Pts',(-8.69652625700006,11.6,-5.97417418400001));
#278190=CARTESIAN_POINT('Ctrl Pts',(-8.69786362600006,15.2,-5.97556290600001));
#278191=CARTESIAN_POINT('Ctrl Pts',(-8.69786362600006,11.6,-5.97556290600001));
#278192=CARTESIAN_POINT('Ctrl Pts',(-8.69920471000006,15.2,-5.97695802000001));
#278193=CARTESIAN_POINT('Ctrl Pts',(-8.69920471000006,11.6,-5.97695802000001));
#278194=CARTESIAN_POINT('Ctrl Pts',(-8.70054949000006,15.2,-5.97835952600001));
#278195=CARTESIAN_POINT('Ctrl Pts',(-8.70054949000006,11.6,-5.97835952600001));
#278196=CARTESIAN_POINT('Ctrl Pts',(-8.70189794500006,15.2,-5.97976741900001));
#278197=CARTESIAN_POINT('Ctrl Pts',(-8.70189794500006,11.6,-5.97976741900001));
#278198=CARTESIAN_POINT('Ctrl Pts',(-8.70325005900006,15.2,-5.98118169700002));
#278199=CARTESIAN_POINT('Ctrl Pts',(-8.70325005900006,11.6,-5.98118169700002));
#278200=CARTESIAN_POINT('Ctrl Pts',(-8.70460581000006,15.2,-5.98260235600002));
#278201=CARTESIAN_POINT('Ctrl Pts',(-8.70460581000006,11.6,-5.98260235600002));
#278202=CARTESIAN_POINT('Ctrl Pts',(-8.70596518000006,15.2,-5.98402939300002));
#278203=CARTESIAN_POINT('Ctrl Pts',(-8.70596518000006,11.6,-5.98402939300002));
#278204=CARTESIAN_POINT('Ctrl Pts',(-8.70732814900006,15.2,-5.98546280500001));
#278205=CARTESIAN_POINT('Ctrl Pts',(-8.70732814900006,11.6,-5.98546280500001));
#278206=CARTESIAN_POINT('Ctrl Pts',(-8.70869469900006,15.2,-5.98690258900002));
#278207=CARTESIAN_POINT('Ctrl Pts',(-8.70869469900006,11.6,-5.98690258900002));
#278208=CARTESIAN_POINT('Ctrl Pts',(-8.71006481000006,15.2,-5.98834874100002));
#278209=CARTESIAN_POINT('Ctrl Pts',(-8.71006481000006,11.6,-5.98834874100002));
#278210=CARTESIAN_POINT('Ctrl Pts',(-8.71143846400006,15.2,-5.98980125800002));
#278211=CARTESIAN_POINT('Ctrl Pts',(-8.71143846400006,11.6,-5.98980125800002));
#278212=CARTESIAN_POINT('Ctrl Pts',(-8.71281564200006,15.2,-5.99126013700002));
#278213=CARTESIAN_POINT('Ctrl Pts',(-8.71281564200006,11.6,-5.99126013700002));
#278214=CARTESIAN_POINT('Ctrl Pts',(-8.71419632600006,15.2,-5.99272537600001));
#278215=CARTESIAN_POINT('Ctrl Pts',(-8.71419632600006,11.6,-5.99272537600001));
#278216=CARTESIAN_POINT('Ctrl Pts',(-8.71558049500005,15.2,-5.99419696900001));
#278217=CARTESIAN_POINT('Ctrl Pts',(-8.71558049500005,11.6,-5.99419696900001));
#278218=CARTESIAN_POINT('Ctrl Pts',(-8.71696813200005,15.2,-5.99567491600002));
#278219=CARTESIAN_POINT('Ctrl Pts',(-8.71696813200005,11.6,-5.99567491600002));
#278220=CARTESIAN_POINT('Ctrl Pts',(-8.71835921700006,15.2,-5.99715921100002));
#278221=CARTESIAN_POINT('Ctrl Pts',(-8.71835921700006,11.6,-5.99715921100002));
#278222=CARTESIAN_POINT('Ctrl Pts',(-8.71975373500005,15.2,-5.99864985300002));
#278223=CARTESIAN_POINT('Ctrl Pts',(-8.71975373500005,11.6,-5.99864985300002));
#278224=CARTESIAN_POINT('Ctrl Pts',(-8.72115166300006,15.2,-6.00014683800002));
#278225=CARTESIAN_POINT('Ctrl Pts',(-8.72115166300006,11.6,-6.00014683800002));
#278226=CARTESIAN_POINT('Ctrl Pts',(-8.72255298500006,15.2,-6.00165016200001));
#278227=CARTESIAN_POINT('Ctrl Pts',(-8.72255298500006,11.6,-6.00165016200001));
#278228=CARTESIAN_POINT('Ctrl Pts',(-8.72395768300006,15.2,-6.00315982300001));
#278229=CARTESIAN_POINT('Ctrl Pts',(-8.72395768300006,11.6,-6.00315982300001));
#278230=CARTESIAN_POINT('Ctrl Pts',(-8.72536573800006,15.2,-6.00467581600002));
#278231=CARTESIAN_POINT('Ctrl Pts',(-8.72536573800006,11.6,-6.00467581600002));
#278232=CARTESIAN_POINT('Ctrl Pts',(-8.72677713200006,15.2,-6.00619814100002));
#278233=CARTESIAN_POINT('Ctrl Pts',(-8.72677713200006,11.6,-6.00619814100002));
#278234=CARTESIAN_POINT('Ctrl Pts',(-8.72819184600005,15.2,-6.00772679200002));
#278235=CARTESIAN_POINT('Ctrl Pts',(-8.72819184600005,11.6,-6.00772679200002));
#278236=CARTESIAN_POINT('Ctrl Pts',(-8.72960986400006,15.2,-6.00926176600002));
#278237=CARTESIAN_POINT('Ctrl Pts',(-8.72960986400006,11.6,-6.00926176600002));
#278238=CARTESIAN_POINT('Ctrl Pts',(-8.73103116600005,15.2,-6.01080306100001));
#278239=CARTESIAN_POINT('Ctrl Pts',(-8.73103116600005,11.6,-6.01080306100001));
#278240=CARTESIAN_POINT('Ctrl Pts',(-8.73245573500006,15.2,-6.01235067300002));
#278241=CARTESIAN_POINT('Ctrl Pts',(-8.73245573500006,11.6,-6.01235067300002));
#278242=CARTESIAN_POINT('Ctrl Pts',(-8.73388355200006,15.2,-6.01390459800001));
#278243=CARTESIAN_POINT('Ctrl Pts',(-8.73388355200006,11.6,-6.01390459800001));
#278244=CARTESIAN_POINT('Ctrl Pts',(-8.73531460000006,15.2,-6.01546483500002));
#278245=CARTESIAN_POINT('Ctrl Pts',(-8.73531460000006,11.6,-6.01546483500002));
#278246=CARTESIAN_POINT('Ctrl Pts',(-8.73674886200006,15.2,-6.01703137900002));
#278247=CARTESIAN_POINT('Ctrl Pts',(-8.73674886200006,11.6,-6.01703137900002));
#278248=CARTESIAN_POINT('Ctrl Pts',(-8.73818631900006,15.2,-6.01860422700002));
#278249=CARTESIAN_POINT('Ctrl Pts',(-8.73818631900006,11.6,-6.01860422700002));
#278250=CARTESIAN_POINT('Ctrl Pts',(-8.73962695400006,15.2,-6.02018337700001));
#278251=CARTESIAN_POINT('Ctrl Pts',(-8.73962695400006,11.6,-6.02018337700001));
#278252=CARTESIAN_POINT('Ctrl Pts',(-8.74107074900006,15.2,-6.02176882400002));
#278253=CARTESIAN_POINT('Ctrl Pts',(-8.74107074900006,11.6,-6.02176882400002));
#278254=CARTESIAN_POINT('Ctrl Pts',(-8.74251768700006,15.2,-6.02336056500001));
#278255=CARTESIAN_POINT('Ctrl Pts',(-8.74251768700006,11.6,-6.02336056500001));
#278256=CARTESIAN_POINT('Ctrl Pts',(-8.74396774900006,15.2,-6.02495859900002));
#278257=CARTESIAN_POINT('Ctrl Pts',(-8.74396774900006,11.6,-6.02495859900002));
#278258=CARTESIAN_POINT('Ctrl Pts',(-8.74542091900006,15.2,-6.02656292000002));
#278259=CARTESIAN_POINT('Ctrl Pts',(-8.74542091900006,11.6,-6.02656292000002));
#278260=CARTESIAN_POINT('Ctrl Pts',(-8.74687718000006,15.2,-6.02817352700002));
#278261=CARTESIAN_POINT('Ctrl Pts',(-8.74687718000006,11.6,-6.02817352700002));
#278262=CARTESIAN_POINT('Ctrl Pts',(-8.74833651400006,15.2,-6.02979041500002));
#278263=CARTESIAN_POINT('Ctrl Pts',(-8.74833651400006,11.6,-6.02979041500002));
#278264=CARTESIAN_POINT('Ctrl Pts',(-8.74979890300006,15.2,-6.03141358100002));
#278265=CARTESIAN_POINT('Ctrl Pts',(-8.74979890300006,11.6,-6.03141358100002));
#278266=CARTESIAN_POINT('Ctrl Pts',(-8.75126433000006,15.2,-6.03304302300002));
#278267=CARTESIAN_POINT('Ctrl Pts',(-8.75126433000006,11.6,-6.03304302300002));
#278268=CARTESIAN_POINT('Ctrl Pts',(-8.75273277900006,15.2,-6.03467873700002));
#278269=CARTESIAN_POINT('Ctrl Pts',(-8.75273277900006,11.6,-6.03467873700002));
#278270=CARTESIAN_POINT('Ctrl Pts',(-8.75420423300006,15.2,-6.03632072000002));
#278271=CARTESIAN_POINT('Ctrl Pts',(-8.75420423300006,11.6,-6.03632072000002));
#278272=CARTESIAN_POINT('Ctrl Pts',(-8.75567867300006,15.2,-6.03796896800001));
#278273=CARTESIAN_POINT('Ctrl Pts',(-8.75567867300006,11.6,-6.03796896800001));
#278274=CARTESIAN_POINT('Ctrl Pts',(-8.75715608400006,15.2,-6.03962347800002));
#278275=CARTESIAN_POINT('Ctrl Pts',(-8.75715608400006,11.6,-6.03962347800002));
#278276=CARTESIAN_POINT('Ctrl Pts',(-8.75863644800006,15.2,-6.04128424800002));
#278277=CARTESIAN_POINT('Ctrl Pts',(-8.75863644800006,11.6,-6.04128424800002));
#278278=CARTESIAN_POINT('Ctrl Pts',(-8.76011974800005,15.2,-6.04295127200002));
#278279=CARTESIAN_POINT('Ctrl Pts',(-8.76011974800005,11.6,-6.04295127200002));
#278280=CARTESIAN_POINT('Ctrl Pts',(-8.76160596900006,15.2,-6.04462455100002));
#278281=CARTESIAN_POINT('Ctrl Pts',(-8.76160596900006,11.6,-6.04462455100002));
#278282=CARTESIAN_POINT('Ctrl Pts',(-8.76309509200006,15.2,-6.04630407800002));
#278283=CARTESIAN_POINT('Ctrl Pts',(-8.76309509200006,11.6,-6.04630407800002));
#278284=CARTESIAN_POINT('Ctrl Pts',(-8.76458710000006,15.2,-6.04798985100001));
#278285=CARTESIAN_POINT('Ctrl Pts',(-8.76458710000006,11.6,-6.04798985100001));
#278286=CARTESIAN_POINT('Ctrl Pts',(-8.76608197800006,15.2,-6.04968186700001));
#278287=CARTESIAN_POINT('Ctrl Pts',(-8.76608197800006,11.6,-6.04968186700001));
#278288=CARTESIAN_POINT('Ctrl Pts',(-8.76757970900006,15.2,-6.05138012300002));
#278289=CARTESIAN_POINT('Ctrl Pts',(-8.76757970900006,11.6,-6.05138012300002));
#278290=CARTESIAN_POINT('Ctrl Pts',(-8.76908027600006,15.2,-6.05308461500002));
#278291=CARTESIAN_POINT('Ctrl Pts',(-8.76908027600006,11.6,-6.05308461500002));
#278292=CARTESIAN_POINT('Ctrl Pts',(-8.77058366300006,15.2,-6.05479534100001));
#278293=CARTESIAN_POINT('Ctrl Pts',(-8.77058366300006,11.6,-6.05479534100001));
#278294=CARTESIAN_POINT('Ctrl Pts',(-8.77208985300006,15.2,-6.05651229500002));
#278295=CARTESIAN_POINT('Ctrl Pts',(-8.77208985300006,11.6,-6.05651229500002));
#278296=CARTESIAN_POINT('Ctrl Pts',(-8.77359883000006,15.2,-6.05823547700002));
#278297=CARTESIAN_POINT('Ctrl Pts',(-8.77359883000006,11.6,-6.05823547700002));
#278298=CARTESIAN_POINT('Ctrl Pts',(-8.77511057700006,15.2,-6.05996488200002));
#278299=CARTESIAN_POINT('Ctrl Pts',(-8.77511057700006,11.6,-6.05996488200002));
#278300=CARTESIAN_POINT('Ctrl Pts',(-8.77662507900006,15.2,-6.06170050700002));
#278301=CARTESIAN_POINT('Ctrl Pts',(-8.77662507900006,11.6,-6.06170050700002));
#278302=CARTESIAN_POINT('Ctrl Pts',(-8.77814231800006,15.2,-6.06344234800002));
#278303=CARTESIAN_POINT('Ctrl Pts',(-8.77814231800006,11.6,-6.06344234800002));
#278304=CARTESIAN_POINT('Ctrl Pts',(-8.77966227900006,15.2,-6.06519040400002));
#278305=CARTESIAN_POINT('Ctrl Pts',(-8.77966227900006,11.6,-6.06519040400002));
#278306=CARTESIAN_POINT('Ctrl Pts',(-8.78118494600006,15.2,-6.06694467000001));
#278307=CARTESIAN_POINT('Ctrl Pts',(-8.78118494600006,11.6,-6.06694467000001));
#278308=CARTESIAN_POINT('Ctrl Pts',(-8.78271030200005,15.2,-6.06870514200001));
#278309=CARTESIAN_POINT('Ctrl Pts',(-8.78271030200005,11.6,-6.06870514200001));
#278310=CARTESIAN_POINT('Ctrl Pts',(-8.78423833200005,15.2,-6.07047181900001));
#278311=CARTESIAN_POINT('Ctrl Pts',(-8.78423833200005,11.6,-6.07047181900001));
#278312=CARTESIAN_POINT('Ctrl Pts',(-8.78576901900006,15.2,-6.07224469600002));
#278313=CARTESIAN_POINT('Ctrl Pts',(-8.78576901900006,11.6,-6.07224469600002));
#278314=CARTESIAN_POINT('Ctrl Pts',(-8.78730234600006,15.2,-6.07402377000002));
#278315=CARTESIAN_POINT('Ctrl Pts',(-8.78730234600006,11.6,-6.07402377000002));
#278316=CARTESIAN_POINT('Ctrl Pts',(-8.78883830100006,15.2,-6.07580903900002));
#278317=CARTESIAN_POINT('Ctrl Pts',(-8.78883830100006,11.6,-6.07580903900002));
#278318=CARTESIAN_POINT('Ctrl Pts',(-8.79037686400006,15.2,-6.07760049900002));
#278319=CARTESIAN_POINT('Ctrl Pts',(-8.79037686400006,11.6,-6.07760049900002));
#278320=CARTESIAN_POINT('Ctrl Pts',(-8.79191802100006,15.2,-6.07939814500002));
#278321=CARTESIAN_POINT('Ctrl Pts',(-8.79191802100006,11.6,-6.07939814500002));
#278322=CARTESIAN_POINT('Ctrl Pts',(-8.79346175700006,15.2,-6.08120197500002));
#278323=CARTESIAN_POINT('Ctrl Pts',(-8.79346175700006,11.6,-6.08120197500002));
#278324=CARTESIAN_POINT('Ctrl Pts',(-8.79500805500006,15.2,-6.08301198800002));
#278325=CARTESIAN_POINT('Ctrl Pts',(-8.79500805500006,11.6,-6.08301198800002));
#278326=CARTESIAN_POINT('Ctrl Pts',(-8.79655690000006,15.2,-6.08482817600001));
#278327=CARTESIAN_POINT('Ctrl Pts',(-8.79655690000006,11.6,-6.08482817600001));
#278328=CARTESIAN_POINT('Ctrl Pts',(-8.79810827500006,15.2,-6.08665054000002));
#278329=CARTESIAN_POINT('Ctrl Pts',(-8.79810827500006,11.6,-6.08665054000002));
#278330=CARTESIAN_POINT('Ctrl Pts',(-8.79966216600006,15.2,-6.08847907500002));
#278331=CARTESIAN_POINT('Ctrl Pts',(-8.79966216600006,11.6,-6.08847907500002));
#278332=CARTESIAN_POINT('Ctrl Pts',(-8.80121855800006,15.2,-6.09031377800001));
#278333=CARTESIAN_POINT('Ctrl Pts',(-8.80121855800006,11.6,-6.09031377800001));
#278334=CARTESIAN_POINT('Ctrl Pts',(-8.80277743400006,15.2,-6.09215464600001));
#278335=CARTESIAN_POINT('Ctrl Pts',(-8.80277743400006,11.6,-6.09215464600001));
#278336=CARTESIAN_POINT('Ctrl Pts',(-8.80433877800006,15.2,-6.09400167400001));
#278337=CARTESIAN_POINT('Ctrl Pts',(-8.80433877800006,11.6,-6.09400167400001));
#278338=CARTESIAN_POINT('Ctrl Pts',(-8.80590257700005,15.2,-6.09585486100002));
#278339=CARTESIAN_POINT('Ctrl Pts',(-8.80590257700005,11.6,-6.09585486100002));
#278340=CARTESIAN_POINT('Ctrl Pts',(-8.80746881400006,15.2,-6.09771420100002));
#278341=CARTESIAN_POINT('Ctrl Pts',(-8.80746881400006,11.6,-6.09771420100002));
#278342=CARTESIAN_POINT('Ctrl Pts',(-8.80903747400006,15.2,-6.09957969500002));
#278343=CARTESIAN_POINT('Ctrl Pts',(-8.80903747400006,11.6,-6.09957969500002));
#278344=CARTESIAN_POINT('Ctrl Pts',(-8.81060854200006,15.2,-6.10145133500002));
#278345=CARTESIAN_POINT('Ctrl Pts',(-8.81060854200006,11.6,-6.10145133500002));
#278346=CARTESIAN_POINT('Ctrl Pts',(-8.81218200200006,15.2,-6.10332912100001));
#278347=CARTESIAN_POINT('Ctrl Pts',(-8.81218200200006,11.6,-6.10332912100001));
#278348=CARTESIAN_POINT('Ctrl Pts',(-8.81375784100005,15.2,-6.10521304800002));
#278349=CARTESIAN_POINT('Ctrl Pts',(-8.81375784100005,11.6,-6.10521304800002));
#278350=CARTESIAN_POINT('Ctrl Pts',(-8.81533604000006,15.2,-6.10710311400001));
#278351=CARTESIAN_POINT('Ctrl Pts',(-8.81533604000006,11.6,-6.10710311400001));
#278352=CARTESIAN_POINT('Ctrl Pts',(-8.81691658800005,15.2,-6.10899931400001));
#278353=CARTESIAN_POINT('Ctrl Pts',(-8.81691658800005,11.6,-6.10899931400001));
#278354=CARTESIAN_POINT('Ctrl Pts',(-8.81849946900006,15.2,-6.11090164700002));
#278355=CARTESIAN_POINT('Ctrl Pts',(-8.81849946900006,11.6,-6.11090164700002));
#278356=CARTESIAN_POINT('Ctrl Pts',(-8.82008466600006,15.2,-6.11281010700001));
#278357=CARTESIAN_POINT('Ctrl Pts',(-8.82008466600006,11.6,-6.11281010700001));
#278358=CARTESIAN_POINT('Ctrl Pts',(-8.82167216500006,15.2,-6.11472469300002));
#278359=CARTESIAN_POINT('Ctrl Pts',(-8.82167216500006,11.6,-6.11472469300002));
#278360=CARTESIAN_POINT('Ctrl Pts',(-8.82326195200006,15.2,-6.11664540100002));
#278361=CARTESIAN_POINT('Ctrl Pts',(-8.82326195200006,11.6,-6.11664540100002));
#278362=CARTESIAN_POINT('Ctrl Pts',(-8.82485401100006,15.2,-6.11857222700002));
#278363=CARTESIAN_POINT('Ctrl Pts',(-8.82485401100006,11.6,-6.11857222700002));
#278364=CARTESIAN_POINT('Ctrl Pts',(-8.82644832900005,15.2,-6.12050516800001));
#278365=CARTESIAN_POINT('Ctrl Pts',(-8.82644832900005,11.6,-6.12050516800001));
#278366=CARTESIAN_POINT('Ctrl Pts',(-8.82804488900006,15.2,-6.12244422100002));
#278367=CARTESIAN_POINT('Ctrl Pts',(-8.82804488900006,11.6,-6.12244422100002));
#278368=CARTESIAN_POINT('Ctrl Pts',(-8.82964367800006,15.2,-6.12438938300001));
#278369=CARTESIAN_POINT('Ctrl Pts',(-8.82964367800006,11.6,-6.12438938300001));
#278370=CARTESIAN_POINT('Ctrl Pts',(-8.83124468100006,15.2,-6.12634065100002));
#278371=CARTESIAN_POINT('Ctrl Pts',(-8.83124468100006,11.6,-6.12634065100002));
#278372=CARTESIAN_POINT('Ctrl Pts',(-8.83284788200006,15.2,-6.12829802000002));
#278373=CARTESIAN_POINT('Ctrl Pts',(-8.83284788200006,11.6,-6.12829802000002));
#278374=CARTESIAN_POINT('Ctrl Pts',(-8.83445326800006,15.2,-6.13026148800002));
#278375=CARTESIAN_POINT('Ctrl Pts',(-8.83445326800006,11.6,-6.13026148800002));
#278376=CARTESIAN_POINT('Ctrl Pts',(-8.83606082300006,15.2,-6.13223105100002));
#278377=CARTESIAN_POINT('Ctrl Pts',(-8.83606082300006,11.6,-6.13223105100002));
#278378=CARTESIAN_POINT('Ctrl Pts',(-8.83767053400006,15.2,-6.13420670600001));
#278379=CARTESIAN_POINT('Ctrl Pts',(-8.83767053400006,11.6,-6.13420670600001));
#278380=CARTESIAN_POINT('Ctrl Pts',(-8.83928238600006,15.2,-6.13618845100002));
#278381=CARTESIAN_POINT('Ctrl Pts',(-8.83928238600006,11.6,-6.13618845100002));
#278382=CARTESIAN_POINT('Ctrl Pts',(-8.84089636400006,15.2,-6.13817628100002));
#278383=CARTESIAN_POINT('Ctrl Pts',(-8.84089636400006,11.6,-6.13817628100002));
#278384=CARTESIAN_POINT('Ctrl Pts',(-8.84251245500005,15.2,-6.14017019300002));
#278385=CARTESIAN_POINT('Ctrl Pts',(-8.84251245500005,11.6,-6.14017019300002));
#278386=CARTESIAN_POINT('Ctrl Pts',(-8.84413064300006,15.2,-6.14217018300002));
#278387=CARTESIAN_POINT('Ctrl Pts',(-8.84413064300006,11.6,-6.14217018300002));
#278388=CARTESIAN_POINT('Ctrl Pts',(-8.84575091500006,15.2,-6.14417625000002));
#278389=CARTESIAN_POINT('Ctrl Pts',(-8.84575091500006,11.6,-6.14417625000002));
#278390=CARTESIAN_POINT('Ctrl Pts',(-8.84737325600006,15.2,-6.14618838800002));
#278391=CARTESIAN_POINT('Ctrl Pts',(-8.84737325600006,11.6,-6.14618838800002));
#278392=CARTESIAN_POINT('Ctrl Pts',(-8.84899765200006,15.2,-6.14820659600002));
#278393=CARTESIAN_POINT('Ctrl Pts',(-8.84899765200006,11.6,-6.14820659600002));
#278394=CARTESIAN_POINT('Ctrl Pts',(-8.85062408800006,15.2,-6.15023087000001));
#278395=CARTESIAN_POINT('Ctrl Pts',(-8.85062408800006,11.6,-6.15023087000001));
#278396=CARTESIAN_POINT('Ctrl Pts',(-8.85225255100006,15.2,-6.15226120500001));
#278397=CARTESIAN_POINT('Ctrl Pts',(-8.85225255100006,11.6,-6.15226120500001));
#278398=CARTESIAN_POINT('Ctrl Pts',(-8.85388302600006,15.2,-6.15429759900002));
#278399=CARTESIAN_POINT('Ctrl Pts',(-8.85388302600006,11.6,-6.15429759900002));
#278400=CARTESIAN_POINT('Ctrl Pts',(-8.85551550100006,15.2,-6.15634004900001));
#278401=CARTESIAN_POINT('Ctrl Pts',(-8.85551550100006,11.6,-6.15634004900001));
#278402=CARTESIAN_POINT('Ctrl Pts',(-8.85714995900006,15.2,-6.15838855200002));
#278403=CARTESIAN_POINT('Ctrl Pts',(-8.85714995900006,11.6,-6.15838855200002));
#278404=CARTESIAN_POINT('Ctrl Pts',(-8.85878638800006,15.2,-6.16044310300002));
#278405=CARTESIAN_POINT('Ctrl Pts',(-8.85878638800006,11.6,-6.16044310300002));
#278406=CARTESIAN_POINT('Ctrl Pts',(-8.86042477400006,15.2,-6.16250370000002));
#278407=CARTESIAN_POINT('Ctrl Pts',(-8.86042477400006,11.6,-6.16250370000002));
#278408=CARTESIAN_POINT('Ctrl Pts',(-8.86206510200006,15.2,-6.16457033900002));
#278409=CARTESIAN_POINT('Ctrl Pts',(-8.86206510200006,11.6,-6.16457033900002));
#278410=CARTESIAN_POINT('Ctrl Pts',(-8.86370735900006,15.2,-6.16664301800002));
#278411=CARTESIAN_POINT('Ctrl Pts',(-8.86370735900006,11.6,-6.16664301800002));
#278412=CARTESIAN_POINT('Ctrl Pts',(-8.86535153100006,15.2,-6.16872173200001));
#278413=CARTESIAN_POINT('Ctrl Pts',(-8.86535153100006,11.6,-6.16872173200001));
#278414=CARTESIAN_POINT('Ctrl Pts',(-8.86699760400005,15.2,-6.17080647800002));
#278415=CARTESIAN_POINT('Ctrl Pts',(-8.86699760400005,11.6,-6.17080647800002));
#278416=CARTESIAN_POINT('Ctrl Pts',(-8.86864556400005,15.2,-6.17289725400001));
#278417=CARTESIAN_POINT('Ctrl Pts',(-8.86864556400005,11.6,-6.17289725400001));
#278418=CARTESIAN_POINT('Ctrl Pts',(-8.87029539800006,15.2,-6.17499405500002));
#278419=CARTESIAN_POINT('Ctrl Pts',(-8.87029539800006,11.6,-6.17499405500002));
#278420=CARTESIAN_POINT('Ctrl Pts',(-8.87194709200006,15.2,-6.17709687800001));
#278421=CARTESIAN_POINT('Ctrl Pts',(-8.87194709200006,11.6,-6.17709687800001));
#278422=CARTESIAN_POINT('Ctrl Pts',(-8.87360063200006,15.2,-6.17920572000001));
#278423=CARTESIAN_POINT('Ctrl Pts',(-8.87360063200006,11.6,-6.17920572000001));
#278424=CARTESIAN_POINT('Ctrl Pts',(-8.87525600500006,15.2,-6.18132057900001));
#278425=CARTESIAN_POINT('Ctrl Pts',(-8.87525600500006,11.6,-6.18132057900001));
#278426=CARTESIAN_POINT('Ctrl Pts',(-8.87691319700006,15.2,-6.18344144900002));
#278427=CARTESIAN_POINT('Ctrl Pts',(-8.87691319700006,11.6,-6.18344144900002));
#278428=CARTESIAN_POINT('Ctrl Pts',(-8.87857219500006,15.2,-6.18556832800002));
#278429=CARTESIAN_POINT('Ctrl Pts',(-8.87857219500006,11.6,-6.18556832800002));
#278430=CARTESIAN_POINT('Ctrl Pts',(-8.88023298500006,15.2,-6.18770121300001));
#278431=CARTESIAN_POINT('Ctrl Pts',(-8.88023298500006,11.6,-6.18770121300001));
#278432=CARTESIAN_POINT('Ctrl Pts',(-8.88189555400006,15.2,-6.18984010100001));
#278433=CARTESIAN_POINT('Ctrl Pts',(-8.88189555400006,11.6,-6.18984010100001));
#278434=CARTESIAN_POINT('Ctrl Pts',(-8.88355988700006,15.2,-6.19198498700002));
#278435=CARTESIAN_POINT('Ctrl Pts',(-8.88355988700006,11.6,-6.19198498700002));
#278436=CARTESIAN_POINT('Ctrl Pts',(-8.88522597300006,15.2,-6.19413586900002));
#278437=CARTESIAN_POINT('Ctrl Pts',(-8.88522597300006,11.6,-6.19413586900002));
#278438=CARTESIAN_POINT('Ctrl Pts',(-8.88689379800006,15.2,-6.19629274300002));
#278439=CARTESIAN_POINT('Ctrl Pts',(-8.88689379800006,11.6,-6.19629274300002));
#278440=CARTESIAN_POINT('Ctrl Pts',(-8.88856334800005,15.2,-6.19845560600002));
#278441=CARTESIAN_POINT('Ctrl Pts',(-8.88856334800005,11.6,-6.19845560600002));
#278442=CARTESIAN_POINT('Ctrl Pts',(-8.89023460900006,15.2,-6.20062445500002));
#278443=CARTESIAN_POINT('Ctrl Pts',(-8.89023460900006,11.6,-6.20062445500002));
#278444=CARTESIAN_POINT('Ctrl Pts',(-8.89190757000006,15.2,-6.20279928600001));
#278445=CARTESIAN_POINT('Ctrl Pts',(-8.89190757000006,11.6,-6.20279928600001));
#278446=CARTESIAN_POINT('Ctrl Pts',(-8.89358221600006,15.2,-6.20498009500002));
#278447=CARTESIAN_POINT('Ctrl Pts',(-8.89358221600006,11.6,-6.20498009500002));
#278448=CARTESIAN_POINT('Ctrl Pts',(-8.89525853400006,15.2,-6.20716688000002));
#278449=CARTESIAN_POINT('Ctrl Pts',(-8.89525853400006,11.6,-6.20716688000002));
#278450=CARTESIAN_POINT('Ctrl Pts',(-8.89693651200006,15.2,-6.20935963800001));
#278451=CARTESIAN_POINT('Ctrl Pts',(-8.89693651200006,11.6,-6.20935963800001));
#278452=CARTESIAN_POINT('Ctrl Pts',(-8.89861613600005,15.2,-6.21155836400002));
#278453=CARTESIAN_POINT('Ctrl Pts',(-8.89861613600005,11.6,-6.21155836400002));
#278454=CARTESIAN_POINT('Ctrl Pts',(-8.90029739200006,15.2,-6.21376305500001));
#278455=CARTESIAN_POINT('Ctrl Pts',(-8.90029739200006,11.6,-6.21376305500001));
#278456=CARTESIAN_POINT('Ctrl Pts',(-8.90198026900006,15.2,-6.21597370900002));
#278457=CARTESIAN_POINT('Ctrl Pts',(-8.90198026900006,11.6,-6.21597370900002));
#278458=CARTESIAN_POINT('Ctrl Pts',(-8.90366475400005,15.2,-6.21819032100002));
#278459=CARTESIAN_POINT('Ctrl Pts',(-8.90366475400005,11.6,-6.21819032100002));
#278460=CARTESIAN_POINT('Ctrl Pts',(-8.90535083200006,15.2,-6.22041288900002));
#278461=CARTESIAN_POINT('Ctrl Pts',(-8.90535083200006,11.6,-6.22041288900002));
#278462=CARTESIAN_POINT('Ctrl Pts',(-8.90703849000005,15.2,-6.22264140900001));
#278463=CARTESIAN_POINT('Ctrl Pts',(-8.90703849000005,11.6,-6.22264140900001));
#278464=CARTESIAN_POINT('Ctrl Pts',(-8.90872771800005,15.2,-6.22487587700002));
#278465=CARTESIAN_POINT('Ctrl Pts',(-8.90872771800005,11.6,-6.22487587700002));
#278466=CARTESIAN_POINT('Ctrl Pts',(-8.91041850200006,15.2,-6.22711629000002));
#278467=CARTESIAN_POINT('Ctrl Pts',(-8.91041850200006,11.6,-6.22711629000002));
#278468=CARTESIAN_POINT('Ctrl Pts',(-8.91211082800006,15.2,-6.22936264500002));
#278469=CARTESIAN_POINT('Ctrl Pts',(-8.91211082800006,11.6,-6.22936264500002));
#278470=CARTESIAN_POINT('Ctrl Pts',(-8.91380468400006,15.2,-6.23161493900002));
#278471=CARTESIAN_POINT('Ctrl Pts',(-8.91380468400006,11.6,-6.23161493900002));
#278472=CARTESIAN_POINT('Ctrl Pts',(-8.91550005600006,15.2,-6.23387316900001));
#278473=CARTESIAN_POINT('Ctrl Pts',(-8.91550005600006,11.6,-6.23387316900001));
#278474=CARTESIAN_POINT('Ctrl Pts',(-8.91719693400006,15.2,-6.23613733000001));
#278475=CARTESIAN_POINT('Ctrl Pts',(-8.91719693400006,11.6,-6.23613733000001));
#278476=CARTESIAN_POINT('Ctrl Pts',(-8.91889530300006,15.2,-6.23840741900001));
#278477=CARTESIAN_POINT('Ctrl Pts',(-8.91889530300006,11.6,-6.23840741900001));
#278478=CARTESIAN_POINT('Ctrl Pts',(-8.92059515000006,15.2,-6.24068343300002));
#278479=CARTESIAN_POINT('Ctrl Pts',(-8.92059515000006,11.6,-6.24068343300002));
#278480=CARTESIAN_POINT('Ctrl Pts',(-8.92229646500006,15.2,-6.24296536900002));
#278481=CARTESIAN_POINT('Ctrl Pts',(-8.92229646500006,11.6,-6.24296536900002));
#278482=CARTESIAN_POINT('Ctrl Pts',(-8.92399923400006,15.2,-6.24525322300002));
#278483=CARTESIAN_POINT('Ctrl Pts',(-8.92399923400006,11.6,-6.24525322300002));
#278484=CARTESIAN_POINT('Ctrl Pts',(-8.92570344300006,15.2,-6.24754699200002));
#278485=CARTESIAN_POINT('Ctrl Pts',(-8.92570344300006,11.6,-6.24754699200002));
#278486=CARTESIAN_POINT('Ctrl Pts',(-8.92740908100006,15.2,-6.24984667200001));
#278487=CARTESIAN_POINT('Ctrl Pts',(-8.92740908100006,11.6,-6.24984667200001));
#278488=CARTESIAN_POINT('Ctrl Pts',(-8.92911613500005,15.2,-6.25215226100002));
#278489=CARTESIAN_POINT('Ctrl Pts',(-8.92911613500005,11.6,-6.25215226100002));
#278490=CARTESIAN_POINT('Ctrl Pts',(-8.93082459500006,15.2,-6.25446375500001));
#278491=CARTESIAN_POINT('Ctrl Pts',(-8.93082459500006,11.6,-6.25446375500001));
#278492=CARTESIAN_POINT('Ctrl Pts',(-8.93253444400005,15.2,-6.25678115000002));
#278493=CARTESIAN_POINT('Ctrl Pts',(-8.93253444400005,11.6,-6.25678115000002));
#278494=CARTESIAN_POINT('Ctrl Pts',(-8.93424567300006,15.2,-6.25910444200001));
#278495=CARTESIAN_POINT('Ctrl Pts',(-8.93424567300006,11.6,-6.25910444200001));
#278496=CARTESIAN_POINT('Ctrl Pts',(-8.93595826900006,15.2,-6.26143363000002));
#278497=CARTESIAN_POINT('Ctrl Pts',(-8.93595826900006,11.6,-6.26143363000002));
#278498=CARTESIAN_POINT('Ctrl Pts',(-8.93767221800006,15.2,-6.26376870800001));
#278499=CARTESIAN_POINT('Ctrl Pts',(-8.93767221800006,11.6,-6.26376870800001));
#278500=CARTESIAN_POINT('Ctrl Pts',(-8.93938751100006,15.2,-6.26610967500002));
#278501=CARTESIAN_POINT('Ctrl Pts',(-8.93938751100006,11.6,-6.26610967500002));
#278502=CARTESIAN_POINT('Ctrl Pts',(-8.94110413200006,15.2,-6.26845652500001));
#278503=CARTESIAN_POINT('Ctrl Pts',(-8.94110413200006,11.6,-6.26845652500001));
#278504=CARTESIAN_POINT('Ctrl Pts',(-8.94282207100006,15.2,-6.27080925700002));
#278505=CARTESIAN_POINT('Ctrl Pts',(-8.94282207100006,11.6,-6.27080925700002));
#278506=CARTESIAN_POINT('Ctrl Pts',(-8.94454131600006,15.2,-6.27316786700002));
#278507=CARTESIAN_POINT('Ctrl Pts',(-8.94454131600006,11.6,-6.27316786700002));
#278508=CARTESIAN_POINT('Ctrl Pts',(-8.94626185300006,15.2,-6.27553235000001));
#278509=CARTESIAN_POINT('Ctrl Pts',(-8.94626185300006,11.6,-6.27553235000001));
#278510=CARTESIAN_POINT('Ctrl Pts',(-8.94798367300006,15.2,-6.27790270500002));
#278511=CARTESIAN_POINT('Ctrl Pts',(-8.94798367300006,11.6,-6.27790270500002));
#278512=CARTESIAN_POINT('Ctrl Pts',(-8.94970676000005,15.2,-6.28027892700001));
#278513=CARTESIAN_POINT('Ctrl Pts',(-8.94970676000005,11.6,-6.28027892700001));
#278514=CARTESIAN_POINT('Ctrl Pts',(-8.95143110500005,15.2,-6.28266101300002));
#278515=CARTESIAN_POINT('Ctrl Pts',(-8.95143110500005,11.6,-6.28266101300002));
#278516=CARTESIAN_POINT('Ctrl Pts',(-8.95315669400006,15.2,-6.28504896000001));
#278517=CARTESIAN_POINT('Ctrl Pts',(-8.95315669400006,11.6,-6.28504896000001));
#278518=CARTESIAN_POINT('Ctrl Pts',(-8.95488351600006,15.2,-6.28744276400001));
#278519=CARTESIAN_POINT('Ctrl Pts',(-8.95488351600006,11.6,-6.28744276400001));
#278520=CARTESIAN_POINT('Ctrl Pts',(-8.95661155800006,15.2,-6.28984242200002));
#278521=CARTESIAN_POINT('Ctrl Pts',(-8.95661155800006,11.6,-6.28984242200002));
#278522=CARTESIAN_POINT('Ctrl Pts',(-8.95834081000006,15.2,-6.29224793100001));
#278523=CARTESIAN_POINT('Ctrl Pts',(-8.95834081000006,11.6,-6.29224793100001));
#278524=CARTESIAN_POINT('Ctrl Pts',(-8.96007125900006,15.2,-6.29465928600002));
#278525=CARTESIAN_POINT('Ctrl Pts',(-8.96007125900006,11.6,-6.29465928600002));
#278526=CARTESIAN_POINT('Ctrl Pts',(-8.96180289200006,15.2,-6.29707648500001));
#278527=CARTESIAN_POINT('Ctrl Pts',(-8.96180289200006,11.6,-6.29707648500001));
#278528=CARTESIAN_POINT('Ctrl Pts',(-8.96353569900005,15.2,-6.29949952400001));
#278529=CARTESIAN_POINT('Ctrl Pts',(-8.96353569900005,11.6,-6.29949952400001));
#278530=CARTESIAN_POINT('Ctrl Pts',(-8.96526966700005,15.2,-6.30192840000002));
#278531=CARTESIAN_POINT('Ctrl Pts',(-8.96526966700005,11.6,-6.30192840000002));
#278532=CARTESIAN_POINT('Ctrl Pts',(-8.96700478400006,15.2,-6.30436311000001));
#278533=CARTESIAN_POINT('Ctrl Pts',(-8.96700478400006,11.6,-6.30436311000001));
#278534=CARTESIAN_POINT('Ctrl Pts',(-8.96874103900006,15.2,-6.30680364900002));
#278535=CARTESIAN_POINT('Ctrl Pts',(-8.96874103900006,11.6,-6.30680364900002));
#278536=CARTESIAN_POINT('Ctrl Pts',(-8.97047842000006,15.2,-6.30925001600002));
#278537=CARTESIAN_POINT('Ctrl Pts',(-8.97047842000006,11.6,-6.30925001600002));
#278538=CARTESIAN_POINT('Ctrl Pts',(-8.97221691500006,15.2,-6.31170220500002));
#278539=CARTESIAN_POINT('Ctrl Pts',(-8.97221691500006,11.6,-6.31170220500002));
#278540=CARTESIAN_POINT('Ctrl Pts',(-8.97395651200006,15.2,-6.31416021300002));
#278541=CARTESIAN_POINT('Ctrl Pts',(-8.97395651200006,11.6,-6.31416021300002));
#278542=CARTESIAN_POINT('Ctrl Pts',(-8.97569720200006,15.2,-6.31662403900001));
#278543=CARTESIAN_POINT('Ctrl Pts',(-8.97569720200006,11.6,-6.31662403900001));
#278544=CARTESIAN_POINT('Ctrl Pts',(-8.97743896900005,15.2,-6.31909367700001));
#278545=CARTESIAN_POINT('Ctrl Pts',(-8.97743896900005,11.6,-6.31909367700001));
#278546=CARTESIAN_POINT('Ctrl Pts',(-8.97918180500006,15.2,-6.32156912600002));
#278547=CARTESIAN_POINT('Ctrl Pts',(-8.97918180500006,11.6,-6.32156912600002));
#278548=CARTESIAN_POINT('Ctrl Pts',(-8.98092569500006,15.2,-6.32405038000002));
#278549=CARTESIAN_POINT('Ctrl Pts',(-8.98092569500006,11.6,-6.32405038000002));
#278550=CARTESIAN_POINT('Ctrl Pts',(-8.98267063200005,15.2,-6.32653743600001));
#278551=CARTESIAN_POINT('Ctrl Pts',(-8.98267063200005,11.6,-6.32653743600001));
#278552=CARTESIAN_POINT('Ctrl Pts',(-8.98441660000006,15.2,-6.32903029200002));
#278553=CARTESIAN_POINT('Ctrl Pts',(-8.98441660000006,11.6,-6.32903029200002));
#278554=CARTESIAN_POINT('Ctrl Pts',(-8.98616359200006,15.2,-6.33152894400002));
#278555=CARTESIAN_POINT('Ctrl Pts',(-8.98616359200006,11.6,-6.33152894400002));
#278556=CARTESIAN_POINT('Ctrl Pts',(-8.98791159200006,15.2,-6.33403338800001));
#278557=CARTESIAN_POINT('Ctrl Pts',(-8.98791159200006,11.6,-6.33403338800001));
#278558=CARTESIAN_POINT('Ctrl Pts',(-8.98966059100006,15.2,-6.33654362100001));
#278559=CARTESIAN_POINT('Ctrl Pts',(-8.98966059100006,11.6,-6.33654362100001));
#278560=CARTESIAN_POINT('Ctrl Pts',(-8.99141057700006,15.2,-6.33905964000002));
#278561=CARTESIAN_POINT('Ctrl Pts',(-8.99141057700006,11.6,-6.33905964000002));
#278562=CARTESIAN_POINT('Ctrl Pts',(-8.99316153900006,15.2,-6.34158144100001));
#278563=CARTESIAN_POINT('Ctrl Pts',(-8.99316153900006,11.6,-6.34158144100001));
#278564=CARTESIAN_POINT('Ctrl Pts',(-8.99491346500006,15.2,-6.34410902000001));
#278565=CARTESIAN_POINT('Ctrl Pts',(-8.99491346500006,11.6,-6.34410902000001));
#278566=CARTESIAN_POINT('Ctrl Pts',(-8.99666634400005,15.2,-6.34664237500001));
#278567=CARTESIAN_POINT('Ctrl Pts',(-8.99666634400005,11.6,-6.34664237500001));
#278568=CARTESIAN_POINT('Ctrl Pts',(-8.99842016600006,15.2,-6.34918150200001));
#278569=CARTESIAN_POINT('Ctrl Pts',(-8.99842016600006,11.6,-6.34918150200001));
#278570=CARTESIAN_POINT('Ctrl Pts',(-9.00017491800006,15.2,-6.35172639700002));
#278571=CARTESIAN_POINT('Ctrl Pts',(-9.00017491800006,11.6,-6.35172639700002));
#278572=CARTESIAN_POINT('Ctrl Pts',(-9.00193058900006,15.2,-6.35427705700002));
#278573=CARTESIAN_POINT('Ctrl Pts',(-9.00193058900006,11.6,-6.35427705700002));
#278574=CARTESIAN_POINT('Ctrl Pts',(-9.00368716800006,15.2,-6.35683347800001));
#278575=CARTESIAN_POINT('Ctrl Pts',(-9.00368716800006,11.6,-6.35683347800001));
#278576=CARTESIAN_POINT('Ctrl Pts',(-9.00544464500006,15.2,-6.35939565800002));
#278577=CARTESIAN_POINT('Ctrl Pts',(-9.00544464500006,11.6,-6.35939565800002));
#278578=CARTESIAN_POINT('Ctrl Pts',(-9.00720300700005,15.2,-6.36196359300002));
#278579=CARTESIAN_POINT('Ctrl Pts',(-9.00720300700005,11.6,-6.36196359300002));
#278580=CARTESIAN_POINT('Ctrl Pts',(-9.00896224300006,15.2,-6.36453727700002));
#278581=CARTESIAN_POINT('Ctrl Pts',(-9.00896224300006,11.6,-6.36453727700002));
#278582=CARTESIAN_POINT('Ctrl Pts',(-9.01072234200005,15.2,-6.36711671100001));
#278583=CARTESIAN_POINT('Ctrl Pts',(-9.01072234200005,11.6,-6.36711671100001));
#278584=CARTESIAN_POINT('Ctrl Pts',(-9.01248329500006,15.2,-6.36970188800002));
#278585=CARTESIAN_POINT('Ctrl Pts',(-9.01248329500006,11.6,-6.36970188800002));
#278586=CARTESIAN_POINT('Ctrl Pts',(-9.01424508900006,15.2,-6.37229280700002));
#278587=CARTESIAN_POINT('Ctrl Pts',(-9.01424508900006,11.6,-6.37229280700002));
#278588=CARTESIAN_POINT('Ctrl Pts',(-9.01600771300006,15.2,-6.37488946300002));
#278589=CARTESIAN_POINT('Ctrl Pts',(-9.01600771300006,11.6,-6.37488946300002));
#278590=CARTESIAN_POINT('Ctrl Pts',(-9.01777115600006,15.2,-6.37749185300001));
#278591=CARTESIAN_POINT('Ctrl Pts',(-9.01777115600006,11.6,-6.37749185300001));
#278592=CARTESIAN_POINT('Ctrl Pts',(-9.01953540800006,15.2,-6.38009997300002));
#278593=CARTESIAN_POINT('Ctrl Pts',(-9.01953540800006,11.6,-6.38009997300002));
#278594=CARTESIAN_POINT('Ctrl Pts',(-9.02130045700006,15.2,-6.38271382100001));
#278595=CARTESIAN_POINT('Ctrl Pts',(-9.02130045700006,11.6,-6.38271382100001));
#278596=CARTESIAN_POINT('Ctrl Pts',(-9.02306629300006,15.2,-6.38533339200002));
#278597=CARTESIAN_POINT('Ctrl Pts',(-9.02306629300006,11.6,-6.38533339200002));
#278598=CARTESIAN_POINT('Ctrl Pts',(-9.02483290400006,15.2,-6.38795868400001));
#278599=CARTESIAN_POINT('Ctrl Pts',(-9.02483290400006,11.6,-6.38795868400001));
#278600=CARTESIAN_POINT('Ctrl Pts',(-9.02660028000006,15.2,-6.39058969200001));
#278601=CARTESIAN_POINT('Ctrl Pts',(-9.02660028000006,11.6,-6.39058969200001));
#278602=CARTESIAN_POINT('Ctrl Pts',(-9.02836840900006,15.2,-6.39322641400002));
#278603=CARTESIAN_POINT('Ctrl Pts',(-9.02836840900006,11.6,-6.39322641400002));
#278604=CARTESIAN_POINT('Ctrl Pts',(-9.03013728200006,15.2,-6.39586884500002));
#278605=CARTESIAN_POINT('Ctrl Pts',(-9.03013728200006,11.6,-6.39586884500002));
#278606=CARTESIAN_POINT('Ctrl Pts',(-9.03190688600005,15.2,-6.39851698200002));
#278607=CARTESIAN_POINT('Ctrl Pts',(-9.03190688600005,11.6,-6.39851698200002));
#278608=CARTESIAN_POINT('Ctrl Pts',(-9.03367721300006,15.2,-6.40117082400002));
#278609=CARTESIAN_POINT('Ctrl Pts',(-9.03367721300006,11.6,-6.40117082400002));
#278610=CARTESIAN_POINT('Ctrl Pts',(-9.03544825000006,15.2,-6.40383036400002));
#278611=CARTESIAN_POINT('Ctrl Pts',(-9.03544825000006,11.6,-6.40383036400002));
#278612=CARTESIAN_POINT('Ctrl Pts',(-9.03721998600006,15.2,-6.40649560000002));
#278613=CARTESIAN_POINT('Ctrl Pts',(-9.03721998600006,11.6,-6.40649560000002));
#278614=CARTESIAN_POINT('Ctrl Pts',(-9.03899241400006,15.2,-6.40916652900002));
#278615=CARTESIAN_POINT('Ctrl Pts',(-9.03899241400006,11.6,-6.40916652900002));
#278616=CARTESIAN_POINT('Ctrl Pts',(-9.04076551800006,15.2,-6.41184314700002));
#278617=CARTESIAN_POINT('Ctrl Pts',(-9.04076551800006,11.6,-6.41184314700002));
#278618=CARTESIAN_POINT('Ctrl Pts',(-9.04253929100006,15.2,-6.41452545100002));
#278619=CARTESIAN_POINT('Ctrl Pts',(-9.04253929100006,11.6,-6.41452545100002));
#278620=CARTESIAN_POINT('Ctrl Pts',(-9.04431372100006,15.2,-6.41721343600001));
#278621=CARTESIAN_POINT('Ctrl Pts',(-9.04431372100006,11.6,-6.41721343600001));
#278622=CARTESIAN_POINT('Ctrl Pts',(-9.04608879800006,15.2,-6.41990710100002));
#278623=CARTESIAN_POINT('Ctrl Pts',(-9.04608879800006,11.6,-6.41990710100002));
#278624=CARTESIAN_POINT('Ctrl Pts',(-9.04786451100006,15.2,-6.42260644100002));
#278625=CARTESIAN_POINT('Ctrl Pts',(-9.04786451100006,11.6,-6.42260644100002));
#278626=CARTESIAN_POINT('Ctrl Pts',(-9.04964085000006,15.2,-6.42531145100002));
#278627=CARTESIAN_POINT('Ctrl Pts',(-9.04964085000006,11.6,-6.42531145100002));
#278628=CARTESIAN_POINT('Ctrl Pts',(-9.05141780400006,15.2,-6.42802213200002));
#278629=CARTESIAN_POINT('Ctrl Pts',(-9.05141780400006,11.6,-6.42802213200002));
#278630=CARTESIAN_POINT('Ctrl Pts',(-9.05319536300006,15.2,-6.43073847600002));
#278631=CARTESIAN_POINT('Ctrl Pts',(-9.05319536300006,11.6,-6.43073847600002));
#278632=CARTESIAN_POINT('Ctrl Pts',(-9.05497351500006,15.2,-6.43346048200002));
#278633=CARTESIAN_POINT('Ctrl Pts',(-9.05497351500006,11.6,-6.43346048200002));
#278634=CARTESIAN_POINT('Ctrl Pts',(-9.05675225100006,15.2,-6.43618814600002));
#278635=CARTESIAN_POINT('Ctrl Pts',(-9.05675225100006,11.6,-6.43618814600002));
#278636=CARTESIAN_POINT('Ctrl Pts',(-9.05853156100006,15.2,-6.43892146500002));
#278637=CARTESIAN_POINT('Ctrl Pts',(-9.05853156100006,11.6,-6.43892146500002));
#278638=CARTESIAN_POINT('Ctrl Pts',(-9.06031143300006,15.2,-6.44166043400002));
#278639=CARTESIAN_POINT('Ctrl Pts',(-9.06031143300006,11.6,-6.44166043400002));
#278640=CARTESIAN_POINT('Ctrl Pts',(-9.06209185800006,15.2,-6.44440505100001));
#278641=CARTESIAN_POINT('Ctrl Pts',(-9.06209185800006,11.6,-6.44440505100001));
#278642=CARTESIAN_POINT('Ctrl Pts',(-9.06387282500006,15.2,-6.44715531100001));
#278643=CARTESIAN_POINT('Ctrl Pts',(-9.06387282500006,11.6,-6.44715531100001));
#278644=CARTESIAN_POINT('Ctrl Pts',(-9.06565432400006,15.2,-6.44991121200002));
#278645=CARTESIAN_POINT('Ctrl Pts',(-9.06565432400006,11.6,-6.44991121200002));
#278646=CARTESIAN_POINT('Ctrl Pts',(-9.06743634400006,15.2,-6.45267275100001));
#278647=CARTESIAN_POINT('Ctrl Pts',(-9.06743634400006,11.6,-6.45267275100001));
#278648=CARTESIAN_POINT('Ctrl Pts',(-9.06921887500006,15.2,-6.45543992300002));
#278649=CARTESIAN_POINT('Ctrl Pts',(-9.06921887500006,11.6,-6.45543992300002));
#278650=CARTESIAN_POINT('Ctrl Pts',(-9.07100190700006,15.2,-6.45821272500001));
#278651=CARTESIAN_POINT('Ctrl Pts',(-9.07100190700006,11.6,-6.45821272500001));
#278652=CARTESIAN_POINT('Ctrl Pts',(-9.07278543000006,15.2,-6.46099115300002));
#278653=CARTESIAN_POINT('Ctrl Pts',(-9.07278543000006,11.6,-6.46099115300002));
#278654=CARTESIAN_POINT('Ctrl Pts',(-9.07456943400006,15.2,-6.46377520400002));
#278655=CARTESIAN_POINT('Ctrl Pts',(-9.07456943400006,11.6,-6.46377520400002));
#278656=CARTESIAN_POINT('Ctrl Pts',(-9.07635390800005,15.2,-6.46656487600002));
#278657=CARTESIAN_POINT('Ctrl Pts',(-9.07635390800005,11.6,-6.46656487600002));
#278658=CARTESIAN_POINT('Ctrl Pts',(-9.07813884200005,15.2,-6.46936016400002));
#278659=CARTESIAN_POINT('Ctrl Pts',(-9.07813884200005,11.6,-6.46936016400002));
#278660=CARTESIAN_POINT('Ctrl Pts',(-9.07992422600006,15.2,-6.47216106300001));
#278661=CARTESIAN_POINT('Ctrl Pts',(-9.07992422600006,11.6,-6.47216106300001));
#278662=CARTESIAN_POINT('Ctrl Pts',(-9.08171005000005,15.2,-6.47496757300001));
#278663=CARTESIAN_POINT('Ctrl Pts',(-9.08171005000005,11.6,-6.47496757300001));
#278664=CARTESIAN_POINT('Ctrl Pts',(-9.08349630400006,15.2,-6.47777968800002));
#278665=CARTESIAN_POINT('Ctrl Pts',(-9.08349630400006,11.6,-6.47777968800002));
#278666=CARTESIAN_POINT('Ctrl Pts',(-9.08528297600006,15.2,-6.48059740600001));
#278667=CARTESIAN_POINT('Ctrl Pts',(-9.08528297600006,11.6,-6.48059740600001));
#278668=CARTESIAN_POINT('Ctrl Pts',(-9.08707006000006,15.2,-6.48342072200002));
#278669=CARTESIAN_POINT('Ctrl Pts',(-9.08707006000006,11.6,-6.48342072200002));
#278670=CARTESIAN_POINT('Ctrl Pts',(-9.08885754100006,15.2,-6.48624963300002));
#278671=CARTESIAN_POINT('Ctrl Pts',(-9.08885754100006,11.6,-6.48624963300002));
#278672=CARTESIAN_POINT('Ctrl Pts',(-9.09064541400006,15.2,-6.48908413600001));
#278673=CARTESIAN_POINT('Ctrl Pts',(-9.09064541400006,11.6,-6.48908413600001));
#278674=CARTESIAN_POINT('Ctrl Pts',(-9.09243366600006,15.2,-6.49192422600001));
#278675=CARTESIAN_POINT('Ctrl Pts',(-9.09243366600006,11.6,-6.49192422600001));
#278676=CARTESIAN_POINT('Ctrl Pts',(-9.09422228600006,15.2,-6.49476990200001));
#278677=CARTESIAN_POINT('Ctrl Pts',(-9.09422228600006,11.6,-6.49476990200001));
#278678=CARTESIAN_POINT('Ctrl Pts',(-9.09601126800006,15.2,-6.49762115900002));
#278679=CARTESIAN_POINT('Ctrl Pts',(-9.09601126800006,11.6,-6.49762115900002));
#278680=CARTESIAN_POINT('Ctrl Pts',(-9.09780059900006,15.2,-6.50047799400002));
#278681=CARTESIAN_POINT('Ctrl Pts',(-9.09780059900006,11.6,-6.50047799400002));
#278682=CARTESIAN_POINT('Ctrl Pts',(-9.09959026900006,15.2,-6.50334040300002));
#278683=CARTESIAN_POINT('Ctrl Pts',(-9.09959026900006,11.6,-6.50334040300002));
#278684=CARTESIAN_POINT('Ctrl Pts',(-9.10138027000006,15.2,-6.50620838300001));
#278685=CARTESIAN_POINT('Ctrl Pts',(-9.10138027000006,11.6,-6.50620838300001));
#278686=CARTESIAN_POINT('Ctrl Pts',(-9.10317059000005,15.2,-6.50908193000002));
#278687=CARTESIAN_POINT('Ctrl Pts',(-9.10317059000005,11.6,-6.50908193000002));
#278688=CARTESIAN_POINT('Ctrl Pts',(-9.10496122200006,15.2,-6.51196104000002));
#278689=CARTESIAN_POINT('Ctrl Pts',(-9.10496122200006,11.6,-6.51196104000002));
#278690=CARTESIAN_POINT('Ctrl Pts',(-9.10675215200006,15.2,-6.51484571200001));
#278691=CARTESIAN_POINT('Ctrl Pts',(-9.10675215200006,11.6,-6.51484571200001));
#278692=CARTESIAN_POINT('Ctrl Pts',(-9.10854337500006,15.2,-6.51773593900002));
#278693=CARTESIAN_POINT('Ctrl Pts',(-9.10854337500006,11.6,-6.51773593900002));
#278694=CARTESIAN_POINT('Ctrl Pts',(-9.11033487900006,15.2,-6.52063172000001));
#278695=CARTESIAN_POINT('Ctrl Pts',(-9.11033487900006,11.6,-6.52063172000001));
#278696=CARTESIAN_POINT('Ctrl Pts',(-9.11212665300006,15.2,-6.52353305100001));
#278697=CARTESIAN_POINT('Ctrl Pts',(-9.11212665300006,11.6,-6.52353305100001));
#278698=CARTESIAN_POINT('Ctrl Pts',(-9.11391868900006,15.2,-6.52643992700002));
#278699=CARTESIAN_POINT('Ctrl Pts',(-9.11391868900006,11.6,-6.52643992700002));
#278700=CARTESIAN_POINT('Ctrl Pts',(-9.11571097600006,15.2,-6.52935234700001));
#278701=CARTESIAN_POINT('Ctrl Pts',(-9.11571097600006,11.6,-6.52935234700001));
#278702=CARTESIAN_POINT('Ctrl Pts',(-9.11750350600006,15.2,-6.53227030600001));
#278703=CARTESIAN_POINT('Ctrl Pts',(-9.11750350600006,11.6,-6.53227030600001));
#278704=CARTESIAN_POINT('Ctrl Pts',(-9.11929626800006,15.2,-6.53519380000001));
#278705=CARTESIAN_POINT('Ctrl Pts',(-9.11929626800006,11.6,-6.53519380000001));
#278706=CARTESIAN_POINT('Ctrl Pts',(-9.12108925300006,15.2,-6.53812282700001));
#278707=CARTESIAN_POINT('Ctrl Pts',(-9.12108925300006,11.6,-6.53812282700001));
#278708=CARTESIAN_POINT('Ctrl Pts',(-9.12288245100006,15.2,-6.54105738200002));
#278709=CARTESIAN_POINT('Ctrl Pts',(-9.12288245100006,11.6,-6.54105738200002));
#278710=CARTESIAN_POINT('Ctrl Pts',(-9.12467585400006,15.2,-6.54399746200002));
#278711=CARTESIAN_POINT('Ctrl Pts',(-9.12467585400006,11.6,-6.54399746200002));
#278712=CARTESIAN_POINT('Ctrl Pts',(-9.12646945000006,15.2,-6.54694306500001));
#278713=CARTESIAN_POINT('Ctrl Pts',(-9.12646945000006,11.6,-6.54694306500001));
#278714=CARTESIAN_POINT('Ctrl Pts',(-9.12826322900005,15.2,-6.54989418500002));
#278715=CARTESIAN_POINT('Ctrl Pts',(-9.12826322900005,11.6,-6.54989418500002));
#278716=CARTESIAN_POINT('Ctrl Pts',(-9.13005718400006,15.2,-6.55285082000002));
#278717=CARTESIAN_POINT('Ctrl Pts',(-9.13005718400006,11.6,-6.55285082000002));
#278718=CARTESIAN_POINT('Ctrl Pts',(-9.13185130600005,15.2,-6.55581296500002));
#278719=CARTESIAN_POINT('Ctrl Pts',(-9.13185130600005,11.6,-6.55581296500002));
#278720=CARTESIAN_POINT('Ctrl Pts',(-9.13364558200006,15.2,-6.55878061800002));
#278721=CARTESIAN_POINT('Ctrl Pts',(-9.13364558200006,11.6,-6.55878061800002));
#278722=CARTESIAN_POINT('Ctrl Pts',(-9.13544000500006,15.2,-6.56175377700002));
#278723=CARTESIAN_POINT('Ctrl Pts',(-9.13544000500006,11.6,-6.56175377700002));
#278724=CARTESIAN_POINT('Ctrl Pts',(-9.13723456500006,15.2,-6.56473243400002));
#278725=CARTESIAN_POINT('Ctrl Pts',(-9.13723456500006,11.6,-6.56473243400002));
#278726=CARTESIAN_POINT('Ctrl Pts',(-9.13902925300006,15.2,-6.56771658900002));
#278727=CARTESIAN_POINT('Ctrl Pts',(-9.13902925300006,11.6,-6.56771658900002));
#278728=CARTESIAN_POINT('Ctrl Pts',(-9.14082405800006,15.2,-6.57070623800001));
#278729=CARTESIAN_POINT('Ctrl Pts',(-9.14082405800006,11.6,-6.57070623800001));
#278730=CARTESIAN_POINT('Ctrl Pts',(-9.14261897300005,15.2,-6.57370137600001));
#278731=CARTESIAN_POINT('Ctrl Pts',(-9.14261897300005,11.6,-6.57370137600001));
#278732=CARTESIAN_POINT('Ctrl Pts',(-9.14441398600006,15.2,-6.57670200000001));
#278733=CARTESIAN_POINT('Ctrl Pts',(-9.14441398600006,11.6,-6.57670200000001));
#278734=CARTESIAN_POINT('Ctrl Pts',(-9.14620909000006,15.2,-6.57970810800002));
#278735=CARTESIAN_POINT('Ctrl Pts',(-9.14620909000006,11.6,-6.57970810800002));
#278736=CARTESIAN_POINT('Ctrl Pts',(-9.14800427400005,15.2,-6.58271969500002));
#278737=CARTESIAN_POINT('Ctrl Pts',(-9.14800427400005,11.6,-6.58271969500002));
#278738=CARTESIAN_POINT('Ctrl Pts',(-9.14979953000006,15.2,-6.58573675700002));
#278739=CARTESIAN_POINT('Ctrl Pts',(-9.14979953000006,11.6,-6.58573675700002));
#278740=CARTESIAN_POINT('Ctrl Pts',(-9.15159484800006,15.2,-6.58875929200001));
#278741=CARTESIAN_POINT('Ctrl Pts',(-9.15159484800006,11.6,-6.58875929200001));
#278742=CARTESIAN_POINT('Ctrl Pts',(-9.15339022000006,15.2,-6.59178729700002));
#278743=CARTESIAN_POINT('Ctrl Pts',(-9.15339022000006,11.6,-6.59178729700002));
#278744=CARTESIAN_POINT('Ctrl Pts',(-9.15518563400006,15.2,-6.59482076600002));
#278745=CARTESIAN_POINT('Ctrl Pts',(-9.15518563400006,11.6,-6.59482076600002));
#278746=CARTESIAN_POINT('Ctrl Pts',(-9.15698108400005,15.2,-6.59785969700001));
#278747=CARTESIAN_POINT('Ctrl Pts',(-9.15698108400005,11.6,-6.59785969700001));
#278748=CARTESIAN_POINT('Ctrl Pts',(-9.15877655800006,15.2,-6.60090408500002));
#278749=CARTESIAN_POINT('Ctrl Pts',(-9.15877655800006,11.6,-6.60090408500002));
#278750=CARTESIAN_POINT('Ctrl Pts',(-9.16057204800006,15.2,-6.60395392900002));
#278751=CARTESIAN_POINT('Ctrl Pts',(-9.16057204800006,11.6,-6.60395392900002));
#278752=CARTESIAN_POINT('Ctrl Pts',(-9.16236754400006,15.2,-6.60700922400002));
#278753=CARTESIAN_POINT('Ctrl Pts',(-9.16236754400006,11.6,-6.60700922400002));
#278754=CARTESIAN_POINT('Ctrl Pts',(-9.16416303800006,15.2,-6.61006996600002));
#278755=CARTESIAN_POINT('Ctrl Pts',(-9.16416303800006,11.6,-6.61006996600002));
#278756=CARTESIAN_POINT('Ctrl Pts',(-9.16595852200006,15.2,-6.61313615300001));
#278757=CARTESIAN_POINT('Ctrl Pts',(-9.16595852200006,11.6,-6.61313615300001));
#278758=CARTESIAN_POINT('Ctrl Pts',(-9.16775398400006,15.2,-6.61620778000002));
#278759=CARTESIAN_POINT('Ctrl Pts',(-9.16775398400006,11.6,-6.61620778000002));
#278760=CARTESIAN_POINT('Ctrl Pts',(-9.16954941700006,15.2,-6.61928484400002));
#278761=CARTESIAN_POINT('Ctrl Pts',(-9.16954941700006,11.6,-6.61928484400002));
#278762=CARTESIAN_POINT('Ctrl Pts',(-9.17134481000006,15.2,-6.62236734100001));
#278763=CARTESIAN_POINT('Ctrl Pts',(-9.17134481000006,11.6,-6.62236734100001));
#278764=CARTESIAN_POINT('Ctrl Pts',(-9.17314015700006,15.2,-6.62545526700002));
#278765=CARTESIAN_POINT('Ctrl Pts',(-9.17314015700006,11.6,-6.62545526700002));
#278766=CARTESIAN_POINT('Ctrl Pts',(-9.17493544600006,15.2,-6.62854862000002));
#278767=CARTESIAN_POINT('Ctrl Pts',(-9.17493544600006,11.6,-6.62854862000002));
#278768=CARTESIAN_POINT('Ctrl Pts',(-9.17673066900005,15.2,-6.63164739700001));
#278769=CARTESIAN_POINT('Ctrl Pts',(-9.17673066900005,11.6,-6.63164739700001));
#278770=CARTESIAN_POINT('Ctrl Pts',(-9.17852581900006,15.2,-6.63475159300001));
#278771=CARTESIAN_POINT('Ctrl Pts',(-9.17852581900006,11.6,-6.63475159300001));
#278772=CARTESIAN_POINT('Ctrl Pts',(-9.18032088300006,15.2,-6.63786120300002));
#278773=CARTESIAN_POINT('Ctrl Pts',(-9.18032088300006,11.6,-6.63786120300002));
#278774=CARTESIAN_POINT('Ctrl Pts',(-9.18211585500006,15.2,-6.64097622700002));
#278775=CARTESIAN_POINT('Ctrl Pts',(-9.18211585500006,11.6,-6.64097622700002));
#278776=CARTESIAN_POINT('Ctrl Pts',(-9.18391072400006,15.2,-6.64409665900001));
#278777=CARTESIAN_POINT('Ctrl Pts',(-9.18391072400006,11.6,-6.64409665900001));
#278778=CARTESIAN_POINT('Ctrl Pts',(-9.18570548500006,15.2,-6.64722249500001));
#278779=CARTESIAN_POINT('Ctrl Pts',(-9.18570548500006,11.6,-6.64722249500001));
#278780=CARTESIAN_POINT('Ctrl Pts',(-9.18750012400006,15.2,-6.65035373300002));
#278781=CARTESIAN_POINT('Ctrl Pts',(-9.18750012400006,11.6,-6.65035373300002));
#278782=CARTESIAN_POINT('Ctrl Pts',(-9.18929463600006,15.2,-6.65349037000002));
#278783=CARTESIAN_POINT('Ctrl Pts',(-9.18929463600006,11.6,-6.65349037000002));
#278784=CARTESIAN_POINT('Ctrl Pts',(-9.19108901000006,15.2,-6.65663240000002));
#278785=CARTESIAN_POINT('Ctrl Pts',(-9.19108901000006,11.6,-6.65663240000002));
#278786=CARTESIAN_POINT('Ctrl Pts',(-9.19288323700006,15.2,-6.65977982200002));
#278787=CARTESIAN_POINT('Ctrl Pts',(-9.19288323700006,11.6,-6.65977982200002));
#278788=CARTESIAN_POINT('Ctrl Pts',(-9.19467731000006,15.2,-6.66293263100001));
#278789=CARTESIAN_POINT('Ctrl Pts',(-9.19467731000006,11.6,-6.66293263100001));
#278790=CARTESIAN_POINT('Ctrl Pts',(-9.19647122000006,15.2,-6.66609082300001));
#278791=CARTESIAN_POINT('Ctrl Pts',(-9.19647122000006,11.6,-6.66609082300001));
#278792=CARTESIAN_POINT('Ctrl Pts',(-9.19826495500006,15.2,-6.66925439600002));
#278793=CARTESIAN_POINT('Ctrl Pts',(-9.19826495500006,11.6,-6.66925439600002));
#278794=CARTESIAN_POINT('Ctrl Pts',(-9.20005851100006,15.2,-6.67242334500001));
#278795=CARTESIAN_POINT('Ctrl Pts',(-9.20005851100006,11.6,-6.67242334500001));
#278796=CARTESIAN_POINT('Ctrl Pts',(-9.20185187600006,15.2,-6.67559766700002));
#278797=CARTESIAN_POINT('Ctrl Pts',(-9.20185187600006,11.6,-6.67559766700002));
#278798=CARTESIAN_POINT('Ctrl Pts',(-9.20364504200006,15.2,-6.67877735900002));
#278799=CARTESIAN_POINT('Ctrl Pts',(-9.20364504200006,11.6,-6.67877735900002));
#278800=CARTESIAN_POINT('Ctrl Pts',(-9.20543800000006,15.2,-6.68196241700001));
#278801=CARTESIAN_POINT('Ctrl Pts',(-9.20543800000006,11.6,-6.68196241700001));
#278802=CARTESIAN_POINT('Ctrl Pts',(-9.20723074300006,15.2,-6.68515283700001));
#278803=CARTESIAN_POINT('Ctrl Pts',(-9.20723074300006,11.6,-6.68515283700001));
#278804=CARTESIAN_POINT('Ctrl Pts',(-9.20902326000006,15.2,-6.68834861600001));
#278805=CARTESIAN_POINT('Ctrl Pts',(-9.20902326000006,11.6,-6.68834861600001));
#278806=CARTESIAN_POINT('Ctrl Pts',(-9.21081554300006,15.2,-6.69154975000002));
#278807=CARTESIAN_POINT('Ctrl Pts',(-9.21081554300006,11.6,-6.69154975000002));
#278808=CARTESIAN_POINT('Ctrl Pts',(-9.21260758500006,15.2,-6.69475623600002));
#278809=CARTESIAN_POINT('Ctrl Pts',(-9.21260758500006,11.6,-6.69475623600002));
#278810=CARTESIAN_POINT('Ctrl Pts',(-9.21439937500006,15.2,-6.69796807000001));
#278811=CARTESIAN_POINT('Ctrl Pts',(-9.21439937500006,11.6,-6.69796807000001));
#278812=CARTESIAN_POINT('Ctrl Pts',(-9.21619090600006,15.2,-6.70118524900002));
#278813=CARTESIAN_POINT('Ctrl Pts',(-9.21619090600006,11.6,-6.70118524900002));
#278814=CARTESIAN_POINT('Ctrl Pts',(-9.21798216800006,15.2,-6.70440776900002));
#278815=CARTESIAN_POINT('Ctrl Pts',(-9.21798216800006,11.6,-6.70440776900002));
#278816=CARTESIAN_POINT('Ctrl Pts',(-9.21977315400006,15.2,-6.70763562500002));
#278817=CARTESIAN_POINT('Ctrl Pts',(-9.21977315400006,11.6,-6.70763562500002));
#278818=CARTESIAN_POINT('Ctrl Pts',(-9.22156385400006,15.2,-6.71086881600001));
#278819=CARTESIAN_POINT('Ctrl Pts',(-9.22156385400006,11.6,-6.71086881600001));
#278820=CARTESIAN_POINT('Ctrl Pts',(-9.22335426000006,15.2,-6.71410733700001));
#278821=CARTESIAN_POINT('Ctrl Pts',(-9.22335426000006,11.6,-6.71410733700001));
#278822=CARTESIAN_POINT('Ctrl Pts',(-9.22514436500006,15.2,-6.71735118500001));
#278823=CARTESIAN_POINT('Ctrl Pts',(-9.22514436500006,11.6,-6.71735118500001));
#278824=CARTESIAN_POINT('Ctrl Pts',(-9.22693415700006,15.2,-6.72060035600002));
#278825=CARTESIAN_POINT('Ctrl Pts',(-9.22693415700006,11.6,-6.72060035600002));
#278826=CARTESIAN_POINT('Ctrl Pts',(-9.22872363300005,15.2,-6.72385484600002));
#278827=CARTESIAN_POINT('Ctrl Pts',(-9.22872363300005,11.6,-6.72385484600002));
#278828=CARTESIAN_POINT('Ctrl Pts',(-9.23051278000005,15.2,-6.72711465300001));
#278829=CARTESIAN_POINT('Ctrl Pts',(-9.23051278000005,11.6,-6.72711465300001));
#278830=CARTESIAN_POINT('Ctrl Pts',(-9.23230159100006,15.2,-6.73037977300002));
#278831=CARTESIAN_POINT('Ctrl Pts',(-9.23230159100006,11.6,-6.73037977300002));
#278832=CARTESIAN_POINT('Ctrl Pts',(-9.23409005700006,15.2,-6.73365020100002));
#278833=CARTESIAN_POINT('Ctrl Pts',(-9.23409005700006,11.6,-6.73365020100002));
#278834=CARTESIAN_POINT('Ctrl Pts',(-9.23587817000006,15.2,-6.73692593400002));
#278835=CARTESIAN_POINT('Ctrl Pts',(-9.23587817000006,11.6,-6.73692593400002));
#278836=CARTESIAN_POINT('Ctrl Pts',(-9.23766592000005,15.2,-6.74020696900002));
#278837=CARTESIAN_POINT('Ctrl Pts',(-9.23766592000005,11.6,-6.74020696900002));
#278838=CARTESIAN_POINT('Ctrl Pts',(-9.23945330000006,15.2,-6.74349330100001));
#278839=CARTESIAN_POINT('Ctrl Pts',(-9.23945330000006,11.6,-6.74349330100001));
#278840=CARTESIAN_POINT('Ctrl Pts',(-9.24124030000005,15.2,-6.74678492800002));
#278841=CARTESIAN_POINT('Ctrl Pts',(-9.24124030000005,11.6,-6.74678492800002));
#278842=CARTESIAN_POINT('Ctrl Pts',(-9.24302691300005,15.2,-6.75008184600002));
#278843=CARTESIAN_POINT('Ctrl Pts',(-9.24302691300005,11.6,-6.75008184600002));
#278844=CARTESIAN_POINT('Ctrl Pts',(-9.24481313200006,15.2,-6.75338405000002));
#278845=CARTESIAN_POINT('Ctrl Pts',(-9.24481313200006,11.6,-6.75338405000002));
#278846=CARTESIAN_POINT('Ctrl Pts',(-9.24659894900006,15.2,-6.75669153900002));
#278847=CARTESIAN_POINT('Ctrl Pts',(-9.24659894900006,11.6,-6.75669153900002));
#278848=CARTESIAN_POINT('Ctrl Pts',(-9.24838435600006,15.2,-6.76000431000002));
#278849=CARTESIAN_POINT('Ctrl Pts',(-9.24838435600006,11.6,-6.76000431000002));
#278850=CARTESIAN_POINT('Ctrl Pts',(-9.25016934500006,15.2,-6.76332235800002));
#278851=CARTESIAN_POINT('Ctrl Pts',(-9.25016934500006,11.6,-6.76332235800002));
#278852=CARTESIAN_POINT('Ctrl Pts',(-9.25195390900006,15.2,-6.76664567900002));
#278853=CARTESIAN_POINT('Ctrl Pts',(-9.25195390900006,11.6,-6.76664567900002));
#278854=CARTESIAN_POINT('Ctrl Pts',(-9.25373803600005,15.2,-6.76997427200002));
#278855=CARTESIAN_POINT('Ctrl Pts',(-9.25373803600005,11.6,-6.76997427200002));
#278856=CARTESIAN_POINT('Ctrl Pts',(-9.25552171800006,15.2,-6.77330812800002));
#278857=CARTESIAN_POINT('Ctrl Pts',(-9.25552171800006,11.6,-6.77330812800002));
#278858=CARTESIAN_POINT('Ctrl Pts',(-9.25730494300005,15.2,-6.77664724600002));
#278859=CARTESIAN_POINT('Ctrl Pts',(-9.25730494300005,11.6,-6.77664724600002));
#278860=CARTESIAN_POINT('Ctrl Pts',(-9.25908770300006,15.2,-6.77999162000001));
#278861=CARTESIAN_POINT('Ctrl Pts',(-9.25908770300006,11.6,-6.77999162000001));
#278862=CARTESIAN_POINT('Ctrl Pts',(-9.26086998700006,15.2,-6.78334124800001));
#278863=CARTESIAN_POINT('Ctrl Pts',(-9.26086998700006,11.6,-6.78334124800001));
#278864=CARTESIAN_POINT('Ctrl Pts',(-9.26265178900006,15.2,-6.78669612500002));
#278865=CARTESIAN_POINT('Ctrl Pts',(-9.26265178900006,11.6,-6.78669612500002));
#278866=CARTESIAN_POINT('Ctrl Pts',(-9.26443310200005,15.2,-6.79005624800002));
#278867=CARTESIAN_POINT('Ctrl Pts',(-9.26443310200005,11.6,-6.79005624800002));
#278868=CARTESIAN_POINT('Ctrl Pts',(-9.26621392500006,15.2,-6.79342161700002));
#278869=CARTESIAN_POINT('Ctrl Pts',(-9.26621392500006,11.6,-6.79342161700002));
#278870=CARTESIAN_POINT('Ctrl Pts',(-9.26799425300005,15.2,-6.79679223000001));
#278871=CARTESIAN_POINT('Ctrl Pts',(-9.26799425300005,11.6,-6.79679223000001));
#278872=CARTESIAN_POINT('Ctrl Pts',(-9.26941812100005,15.2,-6.79949291400002));
#278873=CARTESIAN_POINT('Ctrl Pts',(-9.26941812100005,11.6,-6.79949291400002));
#278874=CARTESIAN_POINT('Ctrl Pts',(-9.27048579800006,15.2,-6.80152078800001));
#278875=CARTESIAN_POINT('Ctrl Pts',(-9.27048579800006,11.6,-6.80152078800001));
#278876=CARTESIAN_POINT('Ctrl Pts',(-9.27119748500006,15.2,-6.80287375200002));
#278877=CARTESIAN_POINT('Ctrl Pts',(-9.27119748500006,11.6,-6.80287375200002));
#278878=CARTESIAN_POINT('Ctrl Pts',(-9.27155330300005,15.2,-6.80355049700001));
#278879=CARTESIAN_POINT('Ctrl Pts',(-9.27155330300005,11.6,-6.80355049700001));
#278880=CARTESIAN_POINT('Ctrl Pts',(-8.56667971000006,15.2,-5.85257411400002));
#278881=CARTESIAN_POINT('Ctrl Pts',(-8.56806288384934,15.2,-5.85370503502559));
#278882=CARTESIAN_POINT('Ctrl Pts',(-8.56948692484017,15.2,-5.85487627493062));
#278883=CARTESIAN_POINT('Ctrl Pts',(-8.57095065283135,15.2,-5.85608775313393));
#278884=CARTESIAN_POINT('Ctrl Pts',(-8.57242143965877,15.2,-5.85730507369751));
#278885=CARTESIAN_POINT('Ctrl Pts',(-8.57393230452754,15.2,-5.85856301222101));
#278886=CARTESIAN_POINT('Ctrl Pts',(-8.57548210844168,15.2,-5.85986145285899));
#278887=CARTESIAN_POINT('Ctrl Pts',(-8.57703191221504,15.2,-5.86115989337901));
#278888=CARTESIAN_POINT('Ctrl Pts',(-8.57862065441741,15.2,-5.86249883667505));
#278889=CARTESIAN_POINT('Ctrl Pts',(-8.58024722827499,15.2,-5.86387816920827));
#278890=CARTESIAN_POINT('Ctrl Pts',(-8.58187380213257,15.2,-5.8652575017415));
#278891=CARTESIAN_POINT('Ctrl Pts',(-8.58353820868947,15.1999999999999,
-5.86667722288291));
#278892=CARTESIAN_POINT('Ctrl Pts',(-8.58523937179385,15.2,-5.86813722031714));
#278893=CARTESIAN_POINT('Ctrl Pts',(-8.58694053505276,15.2,-5.86959721788399));
#278894=CARTESIAN_POINT('Ctrl Pts',(-8.58867845668591,15.2,-5.87109749028118));
#278895=CARTESIAN_POINT('Ctrl Pts',(-8.59045208820166,15.2,-5.87263792486786));
#278896=CARTESIAN_POINT('Ctrl Pts',(-8.59222571955631,15.2,-5.87417835931461));
#278897=CARTESIAN_POINT('Ctrl Pts',(-8.59403506469271,15.2,-5.87575895551878));
#278898=CARTESIAN_POINT('Ctrl Pts',(-8.5958791059675,15.2,-5.87737960096735));
#278899=CARTESIAN_POINT('Ctrl Pts',(-8.59772314724229,15.2,-5.87900024641592));
#278900=CARTESIAN_POINT('Ctrl Pts',(-8.59960188407517,15.2,-5.88066094137928));
#278901=CARTESIAN_POINT('Ctrl Pts',(-8.60151432942091,15.2,-5.8823615708991));
#278902=CARTESIAN_POINT('Ctrl Pts',(-8.60342677494035,15.2,-5.88406220057339));
#278903=CARTESIAN_POINT('Ctrl Pts',(-8.60537292788893,15.2,-5.88580276593591));
#278904=CARTESIAN_POINT('Ctrl Pts',(-8.60735182649905,15.2,-5.88758315445236));
#278905=CARTESIAN_POINT('Ctrl Pts',(-8.6093307249294,15.2,-5.88936354280707));
#278906=CARTESIAN_POINT('Ctrl Pts',(-8.61134236849269,15.2,-5.89118375430898));
#278907=CARTESIAN_POINT('Ctrl Pts',(-8.61338582016984,15.2,-5.89304367482648));
#278908=CARTESIAN_POINT('Ctrl Pts',(-8.615429271847,15.2,-5.89490359534398));
#278909=CARTESIAN_POINT('Ctrl Pts',(-8.61750453139654,15.2,-5.89680322461661));
#278910=CARTESIAN_POINT('Ctrl Pts',(-8.61961068615201,15.2,-5.89874245187776));
#278911=CARTESIAN_POINT('Ctrl Pts',(-8.62171684090748,15.2,-5.90068167913891));
#278912=CARTESIAN_POINT('Ctrl Pts',(-8.62385388904458,15.2,-5.90266050258931));
#278913=CARTESIAN_POINT('Ctrl Pts',(-8.62602094279714,15.2,-5.9046788090133));
#278914=CARTESIAN_POINT('Ctrl Pts',(-8.62818799674654,15.2,-5.90669711562061));
#278915=CARTESIAN_POINT('Ctrl Pts',(-8.63038505409052,15.2,-5.90875490690673));
#278916=CARTESIAN_POINT('Ctrl Pts',(-8.63261124812979,15.2,-5.91085206660608));
#278917=CARTESIAN_POINT('Ctrl Pts',(-8.63483744196683,15.2,-5.91294922611493));
#278918=CARTESIAN_POINT('Ctrl Pts',(-8.63709277010499,15.2,-5.91508575739324));
#278919=CARTESIAN_POINT('Ctrl Pts',(-8.63937638719897,15.2,-5.91726154574063));
#278920=CARTESIAN_POINT('Ctrl Pts',(-8.64166000429297,15.2,-5.91943733408802));
#278921=CARTESIAN_POINT('Ctrl Pts',(-8.64397191091524,15.2,-5.9216523775805));
#278922=CARTESIAN_POINT('Ctrl Pts',(-8.64631127799502,15.2,-5.92390656674592));
#278923=CARTESIAN_POINT('Ctrl Pts',(-8.6486506452873,15.2,-5.92616075611608));
#278924=CARTESIAN_POINT('Ctrl Pts',(-8.65101747287396,15.2,-5.92845408682341));
#278925=CARTESIAN_POINT('Ctrl Pts',(-8.65341095442223,15.2,-5.93078644936889));
#278926=CARTESIAN_POINT('Ctrl Pts',(-8.6558044357531,15.2,-5.93311881170251));
#278927=CARTESIAN_POINT('Ctrl Pts',(-8.65822457123507,15.2,-5.93549020269225));
#278928=CARTESIAN_POINT('Ctrl Pts',(-8.66067056874057,15.2,-5.93790051194886));
#278929=CARTESIAN_POINT('Ctrl Pts',(-8.66311656624608,15.2,-5.94031082120545));
#278930=CARTESIAN_POINT('Ctrl Pts',(-8.66558843005363,15.2,-5.94276004585515));
#278931=CARTESIAN_POINT('Ctrl Pts',(-8.66808538546118,15.2,-5.94524807326209));
#278932=CARTESIAN_POINT('Ctrl Pts',(-8.67058234109555,15.2,-5.94773610089503));
#278933=CARTESIAN_POINT('Ctrl Pts',(-8.67310438880402,15.2,-5.95026293009468));
#278934=CARTESIAN_POINT('Ctrl Pts',(-8.67565077648807,15.2,-5.95282844969823));
#278935=CARTESIAN_POINT('Ctrl Pts',(-8.67819716394084,15.2,-5.95539396906875));
#278936=CARTESIAN_POINT('Ctrl Pts',(-8.68076788847761,15.2,-5.95799817577096));
#278937=CARTESIAN_POINT('Ctrl Pts',(-8.68336221571668,15.2,-5.96064095625828));
#278938=CARTESIAN_POINT('Ctrl Pts',(-8.68595654295576,15.2,-5.96328373674558));
#278939=CARTESIAN_POINT('Ctrl Pts',(-8.68857446975996,15.2,-5.96596509348544));
#278940=CARTESIAN_POINT('Ctrl Pts',(-8.69121527746127,15.2,-5.96868490802027));
#278941=CARTESIAN_POINT('Ctrl Pts',(-8.69385608540248,15.2,-5.97140472280214));
#278942=CARTESIAN_POINT('Ctrl Pts',(-8.69651977346154,15.2,-5.97416299852474));
#278943=CARTESIAN_POINT('Ctrl Pts',(-8.69920563427612,15.2,-5.97695961826312));
#278944=CARTESIAN_POINT('Ctrl Pts',(-8.70189149484673,15.2,-5.97975623774748));
#278945=CARTESIAN_POINT('Ctrl Pts',(-8.70459952848798,15.2,-5.98259120266751));
#278946=CARTESIAN_POINT('Ctrl Pts',(-8.70732904423459,15.2,-5.98546439799293));
#278947=CARTESIAN_POINT('Ctrl Pts',(-8.71005855998121,15.2,-5.98833759331834));
#278948=CARTESIAN_POINT('Ctrl Pts',(-8.712809559009,15.2,-5.99124901789818));
#278949=CARTESIAN_POINT('Ctrl Pts',(-8.71558136182404,15.2,-5.99419855728936));
#278950=CARTESIAN_POINT('Ctrl Pts',(-8.71789119758718,15.2,-5.99665650687132));
#278951=CARTESIAN_POINT('Ctrl Pts',(-8.72021548140903,15.2,-5.99914092571506));
#278952=CARTESIAN_POINT('Ctrl Pts',(-8.72255382883885,15.2,-6.0016517460609));
#278953=CARTESIAN_POINT('Ctrl Pts',(-8.72489217626867,15.2,-6.00416256640674));
#278954=CARTESIAN_POINT('Ctrl Pts',(-8.72724458758246,15.2,-6.00669978913697));
#278955=CARTESIAN_POINT('Ctrl Pts',(-8.72961068502373,15.2,-6.00926334623189));
#278956=CARTESIAN_POINT('Ctrl Pts',(-8.731976782465,15.2,-6.0118269033268));
#278957=CARTESIAN_POINT('Ctrl Pts',(-8.73435656410001,15.2,-6.0144167953555));
#278958=CARTESIAN_POINT('Ctrl Pts',(-8.73674966076669,15.2,-6.01703295500828));
#278959=CARTESIAN_POINT('Ctrl Pts',(-8.73914275743336,15.2,-6.01964911466105));
#278960=CARTESIAN_POINT('Ctrl Pts',(-8.74154916827364,15.2,-6.02229154210031));
#278961=CARTESIAN_POINT('Ctrl Pts',(-8.74396852599302,15.2,-6.02496017079308));
#278962=CARTESIAN_POINT('Ctrl Pts',(-8.74638788371239,15.2,-6.02762879948585));
#278963=CARTESIAN_POINT('Ctrl Pts',(-8.74882019127601,15.2,-6.0303236283378));
#278964=CARTESIAN_POINT('Ctrl Pts',(-8.75126508565167,15.2,-6.0330445911864));
#278965=CARTESIAN_POINT('Ctrl Pts',(-8.75370998002734,15.2,-6.03576555403501));
#278966=CARTESIAN_POINT('Ctrl Pts',(-8.75616746439987,15.2,-6.038512650419));
#278967=CARTESIAN_POINT('Ctrl Pts',(-8.75863718217829,15.2,-6.04128581173981));
#278968=CARTESIAN_POINT('Ctrl Pts',(-8.7611068999567,15.2,-6.0440589730606));
#278969=CARTESIAN_POINT('Ctrl Pts',(-8.76358885294193,15.2,-6.04685820099616));
#278970=CARTESIAN_POINT('Ctrl Pts',(-8.76608269153957,15.2,-6.04968342731967));
#278971=CARTESIAN_POINT('Ctrl Pts',(-8.7685765301372,15.2,-6.05250865364318));
#278972=CARTESIAN_POINT('Ctrl Pts',(-8.77108225506726,15.2,-6.05535987786309));
#278973=CARTESIAN_POINT('Ctrl Pts',(-8.77359952284596,15.2,-6.05823703314296));
#278974=CARTESIAN_POINT('Ctrl Pts',(-8.77611679062466,15.2,-6.06111418842282));
#278975=CARTESIAN_POINT('Ctrl Pts',(-8.77864560165358,15.2,-6.06401727391984));
#278976=CARTESIAN_POINT('Ctrl Pts',(-8.78118561859893,15.2,-6.06694622190807));
#278977=CARTESIAN_POINT('Ctrl Pts',(-8.78372563526744,15.2,-6.06987516957704));
#278978=CARTESIAN_POINT('Ctrl Pts',(-8.78627685702285,15.2,-6.07282997980375));
#278979=CARTESIAN_POINT('Ctrl Pts',(-8.78883895271491,15.2,-6.07581058635177));
#278980=CARTESIAN_POINT('Ctrl Pts',(-8.79140104868625,15.2,-6.07879119322466));
#278981=CARTESIAN_POINT('Ctrl Pts',(-8.79397401767406,15.2,-6.08179759316655));
#278982=CARTESIAN_POINT('Ctrl Pts',(-8.79655753218712,15.2,-6.08482971955336));
#278983=CARTESIAN_POINT('Ctrl Pts',(-8.79914104670016,15.2,-6.08786184594017));
#278984=CARTESIAN_POINT('Ctrl Pts',(-8.80173510762689,15.2,-6.09091970129317));
#278985=CARTESIAN_POINT('Ctrl Pts',(-8.80433939137606,15.2,-6.09400321330497));
#278986=CARTESIAN_POINT('Ctrl Pts',(-8.80694367512524,15.2,-6.09708672531678));
#278987=CARTESIAN_POINT('Ctrl Pts',(-8.80955818265387,15.2,-6.1001958954091));
#278988=CARTESIAN_POINT('Ctrl Pts',(-8.81218259639541,15.2,-6.10333065591114));
#278989=CARTESIAN_POINT('Ctrl Pts',(-8.81480701013694,15.2,-6.10646541641319));
#278990=CARTESIAN_POINT('Ctrl Pts',(-8.81744132993878,15.2,-6.10962576694863));
#278991=CARTESIAN_POINT('Ctrl Pts',(-8.82008524132718,15.2,-6.11281163826675));
#278992=CARTESIAN_POINT('Ctrl Pts',(-8.82272915271557,15.2,-6.11599750958487));
#278993=CARTESIAN_POINT('Ctrl Pts',(-8.82538265717086,15.2,-6.11920890262307));
#278994=CARTESIAN_POINT('Ctrl Pts',(-8.82804544605928,15.2,-6.12244574803842));
#278995=CARTESIAN_POINT('Ctrl Pts',(-8.8301756772861,15.2,-6.12503522451181));
#278996=CARTESIAN_POINT('Ctrl Pts',(-8.83231185130607,15.2,-6.12764099158576));
#278997=CARTESIAN_POINT('Ctrl Pts',(-8.83445381058588,15.2,-6.13026301213885));
#278998=CARTESIAN_POINT('Ctrl Pts',(-8.83659576957385,15.2,-6.13288503233469));
#278999=CARTESIAN_POINT('Ctrl Pts',(-8.83874351450323,15.2,-6.13552330721506));
#279000=CARTESIAN_POINT('Ctrl Pts',(-8.84089689204905,15.2,-6.13817780127477));
#279001=CARTESIAN_POINT('Ctrl Pts',(-8.84305026988826,15.2,-6.14083229569616));
#279002=CARTESIAN_POINT('Ctrl Pts',(-8.84520928007816,15.2,-6.14350300849172));
#279003=CARTESIAN_POINT('Ctrl Pts',(-8.8473737699187,15.2,-6.14618990569476));
#279004=CARTESIAN_POINT('Ctrl Pts',(-8.84953825946433,15.2,-6.14887680253172));
#279005=CARTESIAN_POINT('Ctrl Pts',(-8.85170822732348,15.2,-6.15157988369332));
#279006=CARTESIAN_POINT('Ctrl Pts',(-8.85388352564275,15.2,-6.15429911260547));
#279007=CARTESIAN_POINT('Ctrl Pts',(-8.8560588242584,15.2,-6.15701834188811));
#279008=CARTESIAN_POINT('Ctrl Pts',(-8.85823945179819,15.2,-6.15975372025736));
#279009=CARTESIAN_POINT('Ctrl Pts',(-8.86042525969545,15.2,-6.16250521074171));
#279010=CARTESIAN_POINT('Ctrl Pts',(-8.86261106729488,15.2,-6.16525670085117));
#279011=CARTESIAN_POINT('Ctrl Pts',(-8.86480205507935,15.2,-6.16802430430459));
#279012=CARTESIAN_POINT('Ctrl Pts',(-8.86699807539933,15.2,-6.17080798501983));
#279013=CARTESIAN_POINT('Ctrl Pts',(-8.86919409601849,15.2,-6.17359166611435));
#279014=CARTESIAN_POINT('Ctrl Pts',(-8.87139514961294,15.2,-6.17639142383001));
#279015=CARTESIAN_POINT('Ctrl Pts',(-8.87360109024321,15.2,-6.17920722421854));
#279016=CARTESIAN_POINT('Ctrl Pts',(-8.87580703057293,15.2,-6.18202302422343));
#279017=CARTESIAN_POINT('Ctrl Pts',(-8.87801785844163,15.2,-6.1848548652799));
#279018=CARTESIAN_POINT('Ctrl Pts',(-8.88023342937113,15.2,-6.18770271326767));
#279019=CARTESIAN_POINT('Ctrl Pts',(-8.8824490006025,15.2,-6.19055056164345));
#279020=CARTESIAN_POINT('Ctrl Pts',(-8.88466931401767,15.2,-6.19341441575966));
#279021=CARTESIAN_POINT('Ctrl Pts',(-8.88689422925004,15.2,-6.19629424024995));
#279022=CARTESIAN_POINT('Ctrl Pts',(-8.88911914448241,15.2,-6.19917406474024));
#279023=CARTESIAN_POINT('Ctrl Pts',(-8.89134865964033,15.2,-6.20206986025183));
#279024=CARTESIAN_POINT('Ctrl Pts',(-8.89358263437363,15.2,-6.20498158946769));
#279025=CARTESIAN_POINT('Ctrl Pts',(-8.89581660880255,15.2,-6.20789331828683));
#279026=CARTESIAN_POINT('Ctrl Pts',(-8.898055043405,15.2,-6.21082098300581));
#279027=CARTESIAN_POINT('Ctrl Pts',(-8.90029779723184,15.2,-6.21376454572295));
#279028=CARTESIAN_POINT('Ctrl Pts',(-8.90254055136426,15.2,-6.21670810884115));
#279029=CARTESIAN_POINT('Ctrl Pts',(-8.90478762671167,15.2,-6.21966757138653));
#279030=CARTESIAN_POINT('Ctrl Pts',(-8.90703888283479,15.2,-6.22264289649476));
#279031=CARTESIAN_POINT('Ctrl Pts',(-8.90985295283532,15.2,-6.22636205267735));
#279032=CARTESIAN_POINT('Ctrl Pts',(-8.91267355956372,15.2,-6.23010599364642));
#279033=CARTESIAN_POINT('Ctrl Pts',(-8.91550043282813,15.2,-6.23387465225957));
#279034=CARTESIAN_POINT('Ctrl Pts',(-8.91776193125479,15.2,-6.23688957890362));
#279035=CARTESIAN_POINT('Ctrl Pts',(-8.92002744089597,15.2,-6.23992032246372));
#279036=CARTESIAN_POINT('Ctrl Pts',(-8.9222968284985,15.2,-6.24296684850622));
#279037=CARTESIAN_POINT('Ctrl Pts',(-8.92456621641023,15.2,-6.24601337496379));
#279038=CARTESIAN_POINT('Ctrl Pts',(-8.92683947885619,15.2,-6.24907568269497));
#279039=CARTESIAN_POINT('Ctrl Pts',(-8.929116486814,15.2,-6.25215373775323));
#279040=CARTESIAN_POINT('Ctrl Pts',(-8.93196274660615,15.2,-6.25600130636636));
#279041=CARTESIAN_POINT('Ctrl Pts',(-8.9348148543845,15.2,-6.25987347703545));
#279042=CARTESIAN_POINT('Ctrl Pts',(-8.93767255431549,15.2,-6.26377018071798));
#279043=CARTESIAN_POINT('Ctrl Pts',(-8.93995871407339,15.2,-6.26688754340916));
#279044=CARTESIAN_POINT('Ctrl Pts',(-8.94224845249498,15.2,-6.27002060719097));
#279045=CARTESIAN_POINT('Ctrl Pts',(-8.94454163904014,15.2,-6.27316933528114));
#279046=CARTESIAN_POINT('Ctrl Pts',(-8.94683482589775,15.2,-6.27631806380033));
#279047=CARTESIAN_POINT('Ctrl Pts',(-8.94913146166429,15.2,-6.27948245697554));
#279048=CARTESIAN_POINT('Ctrl Pts',(-8.95143141640109,15.2,-6.28266247876156));
#279049=CARTESIAN_POINT('Ctrl Pts',(-8.95373137082452,15.2,-6.28584250011431));
#279050=CARTESIAN_POINT('Ctrl Pts',(-8.9560346433614,15.2,-6.28903815024836));
#279051=CARTESIAN_POINT('Ctrl Pts',(-8.95834110906152,15.2,-6.29224939226258));
#279052=CARTESIAN_POINT('Ctrl Pts',(-8.96064757507589,15.2,-6.29546063471434));
#279053=CARTESIAN_POINT('Ctrl Pts',(-8.96295723229657,15.2,-6.29868746839159));
#279054=CARTESIAN_POINT('Ctrl Pts',(-8.96526995459398,15.2,-6.30192985895386));
#279055=CARTESIAN_POINT('Ctrl Pts',(-8.96758267657627,15.2,-6.30517224907435));
#279056=CARTESIAN_POINT('Ctrl Pts',(-8.96989846369191,15.2,-6.30843019532333));
#279057=CARTESIAN_POINT('Ctrl Pts',(-8.97221719033552,15.2,-6.31170365949917));
#279058=CARTESIAN_POINT('Ctrl Pts',(-8.97453591729504,15.2,-6.31497712412101));
#279059=CARTESIAN_POINT('Ctrl Pts',(-8.97685758585211,15.2,-6.31826610919745));
#279060=CARTESIAN_POINT('Ctrl Pts',(-8.97918206875676,15.2,-6.32157057754524));
#279061=CARTESIAN_POINT('Ctrl Pts',(-8.98208767222923,15.2,-6.32570116275486));
#279062=CARTESIAN_POINT('Ctrl Pts',(-8.98499767754044,15.2,-6.3298559384388));
#279063=CARTESIAN_POINT('Ctrl Pts',(-8.98791184191566,15.2,-6.3340348355234));
#279064=CARTESIAN_POINT('Ctrl Pts',(-8.99024317322525,15.2,-6.33737795291779));
#279065=CARTESIAN_POINT('Ctrl Pts',(-8.99257716749385,15.2,-6.34073650793572));
#279066=CARTESIAN_POINT('Ctrl Pts',(-8.99491370291935,15.2,-6.34411046349379));
#279067=CARTESIAN_POINT('Ctrl Pts',(-8.9972502386632,15.2,-6.34748441951156));
#279068=CARTESIAN_POINT('Ctrl Pts',(-8.99958931723872,15.2,-6.35087377702523));
#279069=CARTESIAN_POINT('Ctrl Pts',(-9.00193081619982,15.2,-6.3542784975451));
#279070=CARTESIAN_POINT('Ctrl Pts',(-9.00427231484188,15.2,-6.35768321760108));
#279071=CARTESIAN_POINT('Ctrl Pts',(-9.0066162363529,15.2,-6.36110330248731));
#279072=CARTESIAN_POINT('Ctrl Pts',(-9.00896245838311,15.2,-6.3645387138716));
#279073=CARTESIAN_POINT('Ctrl Pts',(-9.01130868073298,15.2,-6.36797412572396));
#279074=CARTESIAN_POINT('Ctrl Pts',(-9.01365720745451,15.2,-6.3714248660115));
#279075=CARTESIAN_POINT('Ctrl Pts',(-9.01600791775998,15.2,-6.37489089649399));
#279076=CARTESIAN_POINT('Ctrl Pts',(-9.01894630548169,15.2,-6.37922343436098));
#279077=CARTESIAN_POINT('Ctrl Pts',(-9.02188810778695,15.2,-6.38357986379644));
#279078=CARTESIAN_POINT('Ctrl Pts',(-9.024833095426,15.2,-6.38796011331156));
#279079=CARTESIAN_POINT('Ctrl Pts',(-9.02718908534464,15.2,-6.3914643126372));
#279080=CARTESIAN_POINT('Ctrl Pts',(-9.02954711368232,15.2,-6.39498375569034));
#279081=CARTESIAN_POINT('Ctrl Pts',(-9.03190706632253,15.2,-6.39851840762205));
#279082=CARTESIAN_POINT('Ctrl Pts',(-9.03426701928429,15.2,-6.40205306003535));
#279083=CARTESIAN_POINT('Ctrl Pts',(-9.03662889621487,15.2,-6.40560292010574));
#279084=CARTESIAN_POINT('Ctrl Pts',(-9.03899258307666,15.2,-6.40916795126072));
#279085=CARTESIAN_POINT('Ctrl Pts',(-9.0413562696164,15.2,-6.41273298192997));
#279086=CARTESIAN_POINT('Ctrl Pts',(-9.04372176464837,15.2,-6.41631318334646));
#279087=CARTESIAN_POINT('Ctrl Pts',(-9.04608895662135,15.2,-6.41990851916213));
#279088=CARTESIAN_POINT('Ctrl Pts',(-9.04845614891687,15.2,-6.42350385546766));
#279089=CARTESIAN_POINT('Ctrl Pts',(-9.05082503831251,15.2,-6.42711432488845));
#279090=CARTESIAN_POINT('Ctrl Pts',(-9.05319551127505,15.2,-6.43073989147495));
#279091=CARTESIAN_POINT('Ctrl Pts',(-9.05556598423759,15.2,-6.43436545806145));
#279092=CARTESIAN_POINT('Ctrl Pts',(-9.05793804126972,15.2,-6.43800612276077));
#279093=CARTESIAN_POINT('Ctrl Pts',(-9.06031157162145,15.2,-6.44166184657267));
#279094=CARTESIAN_POINT('Ctrl Pts',(-9.0626851016498,15.2,-6.44531756988648));
#279095=CARTESIAN_POINT('Ctrl Pts',(-9.06506010570969,15.2,-6.44898835265985));
#279096=CARTESIAN_POINT('Ctrl Pts',(-9.06743647174844,15.2,-6.45267415926412));
#279097=CARTESIAN_POINT('Ctrl Pts',(-9.06981283811096,15.2,-6.45635996637058));
#279098=CARTESIAN_POINT('Ctrl Pts',(-9.0721905676009,15.2,-6.46006079468401));
#279099=CARTESIAN_POINT('Ctrl Pts',(-9.07456955189735,15.2,-6.4637766098325));
#279100=CARTESIAN_POINT('Ctrl Pts',(-9.07694853586966,15.2,-6.46749242447471));
#279101=CARTESIAN_POINT('Ctrl Pts',(-9.07932877337237,15.2,-6.47122322472885));
#279102=CARTESIAN_POINT('Ctrl Pts',(-9.08171015728871,15.2,-6.47496897397721));
#279103=CARTESIAN_POINT('Ctrl Pts',(-9.0834961953071,15.2,-6.47777828604108));
#279104=CARTESIAN_POINT('Ctrl Pts',(-9.08528287729666,15.2,-6.48059600691573));
#279105=CARTESIAN_POINT('Ctrl Pts',(-9.0870701589876,15.2,-6.48342212020326));
#279106=CARTESIAN_POINT('Ctrl Pts',(-9.08885744067855,15.2,-6.4862482334908));
#279107=CARTESIAN_POINT('Ctrl Pts',(-9.09064532242522,15.2,-6.4890827392013));
#279108=CARTESIAN_POINT('Ctrl Pts',(-9.09243375765184,15.2,-6.49192562184689));
#279109=CARTESIAN_POINT('Ctrl Pts',(-9.09422219320335,15.2,-6.49476850500892));
#279110=CARTESIAN_POINT('Ctrl Pts',(-9.09601118414669,15.2,-6.49761976600662));
#279111=CARTESIAN_POINT('Ctrl Pts',(-9.09780068415683,15.2,-6.50047938813169));
#279112=CARTESIAN_POINT('Ctrl Pts',(-9.09959018384188,15.2,-6.50333900973727));
#279113=CARTESIAN_POINT('Ctrl Pts',(-9.1013801930769,15.2,-6.50620699290073));
#279114=CARTESIAN_POINT('Ctrl Pts',(-9.10317066813689,15.2,-6.50908332108862));
#279115=CARTESIAN_POINT('Ctrl Pts',(-9.10496114319688,15.2,-6.51195964927651));
#279116=CARTESIAN_POINT('Ctrl Pts',(-9.1067520827753,15.2,-6.51484432377786));
#279117=CARTESIAN_POINT('Ctrl Pts',(-9.10854344526001,15.2,-6.51773732747758));
#279118=CARTESIAN_POINT('Ctrl Pts',(-9.11093192846448,15.2,-6.52159466556869));
#279119=CARTESIAN_POINT('Ctrl Pts',(-9.11332115958528,15.2,-6.5254668126087));
#279120=CARTESIAN_POINT('Ctrl Pts',(-9.11571103633431,15.2,-6.52935373112279));
#279121=CARTESIAN_POINT('Ctrl Pts',(-9.11750344430311,15.2,-6.53226892067035));
#279122=CARTESIAN_POINT('Ctrl Pts',(-9.11929621564698,15.2,-6.53519241856187));
#279123=CARTESIAN_POINT('Ctrl Pts',(-9.12108930665761,15.2,-6.53812420965575));
#279124=CARTESIAN_POINT('Ctrl Pts',(-9.12288239734251,15.2,-6.54105600021703));
#279125=CARTESIAN_POINT('Ctrl Pts',(-9.12467580924405,15.2,-6.54399608354453));
#279126=CARTESIAN_POINT('Ctrl Pts',(-9.12646949597057,15.2,-6.5469444446048));
#279127=CARTESIAN_POINT('Ctrl Pts',(-9.12826318269709,15.2,-6.54989280566507));
#279128=CARTESIAN_POINT('Ctrl Pts',(-9.13005714644206,15.2,-6.55284944326355));
#279129=CARTESIAN_POINT('Ctrl Pts',(-9.13185134455168,15.2,-6.55581434200265));
#279130=CARTESIAN_POINT('Ctrl Pts',(-9.13364554266131,15.2,-6.55877924074175));
#279131=CARTESIAN_POINT('Ctrl Pts',(-9.13543997387214,15.2,-6.5617524027254));
#279132=CARTESIAN_POINT('Ctrl Pts',(-9.13723459698176,15.2,-6.56473380846392));
#279133=CARTESIAN_POINT('Ctrl Pts',(-9.13902922009137,15.2,-6.56771521420243));
#279134=CARTESIAN_POINT('Ctrl Pts',(-9.14082403420296,15.2,-6.57070486649963));
#279135=CARTESIAN_POINT('Ctrl Pts',(-9.14261899734608,15.2,-6.57370274718166));
#279136=CARTESIAN_POINT('Ctrl Pts',(-9.14441396048919,15.2,-6.5767006278637));
#279137=CARTESIAN_POINT('Ctrl Pts',(-9.14620907240727,15.2,-6.57970673897014));
#279138=CARTESIAN_POINT('Ctrl Pts',(-9.14800429159204,15.2,-6.58272106310952));
#279139=CARTESIAN_POINT('Ctrl Pts',(-9.14979951110294,15.2,-6.5857353877965));
#279140=CARTESIAN_POINT('Ctrl Pts',(-9.15159483843051,15.2,-6.58875792658575));
#279141=CARTESIAN_POINT('Ctrl Pts',(-9.15339023094145,15.2,-6.591788663694));
#279142=CARTESIAN_POINT('Ctrl Pts',(-9.15518562312623,15.2,-6.59481940025167));
#279143=CARTESIAN_POINT('Ctrl Pts',(-9.1569810810563,15.2,-6.59785833376379));
#279144=CARTESIAN_POINT('Ctrl Pts',(-9.15877656233077,15.2,-6.60090544955625));
#279145=CARTESIAN_POINT('Ctrl Pts',(-9.16057204360524,15.2,-6.60395256534871));
#279146=CARTESIAN_POINT('Ctrl Pts',(-9.16236754756099,15.2,-6.60700786346127));
#279147=CARTESIAN_POINT('Ctrl Pts',(-9.16416303566243,15.2,-6.61007132755902));
#279148=CARTESIAN_POINT('Ctrl Pts',(-9.16595852376386,15.2,-6.61313479165675));
#279149=CARTESIAN_POINT('Ctrl Pts',(-9.16775399481528,15.2,-6.61620642219517));
#279150=CARTESIAN_POINT('Ctrl Pts',(-9.16954940704173,15.2,-6.61928620224996));
#279151=CARTESIAN_POINT('Ctrl Pts',(-9.17194329022776,15.2,-6.62339257602934));
#279152=CARTESIAN_POINT('Ctrl Pts',(-9.1743370700721,15.2,-6.62751343742149));
#279153=CARTESIAN_POINT('Ctrl Pts',(-9.1767306510914,15.2,-6.63164875242608));
#279154=CARTESIAN_POINT('Ctrl Pts',(-9.17852583669283,15.2,-6.63475023839782));
#279155=CARTESIAN_POINT('Ctrl Pts',(-9.18032090972761,15.2,-6.63785985188584));
#279156=CARTESIAN_POINT('Ctrl Pts',(-9.1821158294957,15.2,-6.64097757935659));
#279157=CARTESIAN_POINT('Ctrl Pts',(-9.1839107492638,15.2,-6.64409530682733));
#279158=CARTESIAN_POINT('Ctrl Pts',(-9.18570551742541,15.2,-6.6472211457024));
#279159=CARTESIAN_POINT('Ctrl Pts',(-9.18750009220169,15.2,-6.65035508272781));
#279160=CARTESIAN_POINT('Ctrl Pts',(-9.18929466697797,15.2,-6.65348901975321));
#279161=CARTESIAN_POINT('Ctrl Pts',(-9.19108904920546,15.2,-6.65663105373061));
#279162=CARTESIAN_POINT('Ctrl Pts',(-9.19288319848176,15.2,-6.65978116875544));
#279163=CARTESIAN_POINT('Ctrl Pts',(-9.19587344738425,15.2,-6.66503136065424));
#279164=CARTESIAN_POINT('Ctrl Pts',(-9.19886305158896,15.2,-6.67030399831107));
#279165=CARTESIAN_POINT('Ctrl Pts',(-9.20185182624172,15.2,-6.67559900949162));
#279166=CARTESIAN_POINT('Ctrl Pts',(-9.20424284609425,15.2,-6.67983501866692));
#279167=CARTESIAN_POINT('Ctrl Pts',(-9.20663333593562,15.2,-6.6840853469439));
#279168=CARTESIAN_POINT('Ctrl Pts',(-9.20902320189913,15.2,-6.68834995545556));
#279169=CARTESIAN_POINT('Ctrl Pts',(-9.21081560120895,15.2,-6.69154841154878));
#279170=CARTESIAN_POINT('Ctrl Pts',(-9.21260765075567,15.2,-6.69475490061058));
#279171=CARTESIAN_POINT('Ctrl Pts',(-9.2143993105717,15.2,-6.69796940686363));
#279172=CARTESIAN_POINT('Ctrl Pts',(-9.21619097038772,15.2,-6.70118391311667));
#279173=CARTESIAN_POINT('Ctrl Pts',(-9.21798224052702,15.2,-6.70440643593556));
#279174=CARTESIAN_POINT('Ctrl Pts',(-9.21977308271192,15.2,-6.70763695906889));
#279175=CARTESIAN_POINT('Ctrl Pts',(-9.22156392489683,15.2,-6.71086748220223));
#279176=CARTESIAN_POINT('Ctrl Pts',(-9.22335433901509,15.2,-6.71410600670124));
#279177=CARTESIAN_POINT('Ctrl Pts',(-9.22514428682506,15.2,-6.71735251574996));
#279178=CARTESIAN_POINT('Ctrl Pts',(-9.22753088412179,15.2,-6.72168119487477));
#279179=CARTESIAN_POINT('Ctrl Pts',(-9.22991665462957,15.2,-6.72602406893459));
#279180=CARTESIAN_POINT('Ctrl Pts',(-9.23230150514831,15.2,-6.730381100729));
#279181=CARTESIAN_POINT('Ctrl Pts',(-9.23468635534212,15.2,-6.73473813192977));
#279182=CARTESIAN_POINT('Ctrl Pts',(-9.23707028615185,15.2,-6.73910931940226));
#279183=CARTESIAN_POINT('Ctrl Pts',(-9.23945320502344,15.2,-6.74349462473031));
#279184=CARTESIAN_POINT('Ctrl Pts',(-9.24124039425829,15.2,-6.74678360387572));
#279185=CARTESIAN_POINT('Ctrl Pts',(-9.24302701403688,15.2,-6.75008052466064));
#279186=CARTESIAN_POINT('Ctrl Pts',(-9.24481303130537,15.2,-6.7533853708732));
#279187=CARTESIAN_POINT('Ctrl Pts',(-9.24659904857387,15.2,-6.75669021708576));
#279188=CARTESIAN_POINT('Ctrl Pts',(-9.24838446267574,15.2,-6.76000299138112));
#279189=CARTESIAN_POINT('Ctrl Pts',(-9.25016923831931,15.2,-6.76332367555106));
#279190=CARTESIAN_POINT('Ctrl Pts',(-9.25195401428712,15.2,-6.76664436032426));
#279191=CARTESIAN_POINT('Ctrl Pts',(-9.25373815124641,15.2,-6.76997295699134));
#279192=CARTESIAN_POINT('Ctrl Pts',(-9.25552160417219,15.2,-6.77330944418565));
#279193=CARTESIAN_POINT('Ctrl Pts',(-9.25730505677395,15.2,-6.77664593077383));
#279194=CARTESIAN_POINT('Ctrl Pts',(-9.25908782435398,15.2,-6.77999030870202));
#279195=CARTESIAN_POINT('Ctrl Pts',(-9.2608698668365,15.2,-6.78334256091528));
#279196=CARTESIAN_POINT('Ctrl Pts',(-9.26265190931903,15.2,-6.78669481312853));
#279197=CARTESIAN_POINT('Ctrl Pts',(-9.26443322619546,15.2,-6.7900549376617));
#279198=CARTESIAN_POINT('Ctrl Pts',(-9.26621380150165,15.2,-6.79342292836566));
#279199=CARTESIAN_POINT('Ctrl Pts',(-9.26799437680784,15.2,-6.79679091906962));
#279200=CARTESIAN_POINT('Ctrl Pts',(-9.26977421267685,15.2,-6.80016677138531));
#279201=CARTESIAN_POINT('Ctrl Pts',(-9.27155330300005,15.2,-6.80355049700001));
#279202=CARTESIAN_POINT('Ctrl Pts',(-8.56667971000006,12.2,-5.85257411400002));
#279203=CARTESIAN_POINT('Ctrl Pts',(-8.56806288384934,12.2,-5.85370503502559));
#279204=CARTESIAN_POINT('Ctrl Pts',(-8.56948692484017,12.2,-5.85487627493062));
#279205=CARTESIAN_POINT('Ctrl Pts',(-8.57095065283135,12.2,-5.85608775313393));
#279206=CARTESIAN_POINT('Ctrl Pts',(-8.57242143965877,12.2,-5.85730507369751));
#279207=CARTESIAN_POINT('Ctrl Pts',(-8.57393230452754,12.2,-5.85856301222101));
#279208=CARTESIAN_POINT('Ctrl Pts',(-8.57548210844168,12.2,-5.85986145285899));
#279209=CARTESIAN_POINT('Ctrl Pts',(-8.57703191221504,12.2,-5.86115989337901));
#279210=CARTESIAN_POINT('Ctrl Pts',(-8.57862065441741,12.2,-5.86249883667505));
#279211=CARTESIAN_POINT('Ctrl Pts',(-8.58024722827499,12.2,-5.86387816920827));
#279212=CARTESIAN_POINT('Ctrl Pts',(-8.58187380213257,12.2,-5.8652575017415));
#279213=CARTESIAN_POINT('Ctrl Pts',(-8.58353820868947,12.2,-5.86667722288291));
#279214=CARTESIAN_POINT('Ctrl Pts',(-8.58523937179385,12.2,-5.86813722031714));
#279215=CARTESIAN_POINT('Ctrl Pts',(-8.58694053505276,12.2,-5.86959721788399));
#279216=CARTESIAN_POINT('Ctrl Pts',(-8.58867845668591,12.2,-5.87109749028118));
#279217=CARTESIAN_POINT('Ctrl Pts',(-8.59045208820166,12.2,-5.87263792486786));
#279218=CARTESIAN_POINT('Ctrl Pts',(-8.59222571955631,12.2,-5.87417835931461));
#279219=CARTESIAN_POINT('Ctrl Pts',(-8.59403506469271,12.2,-5.87575895551878));
#279220=CARTESIAN_POINT('Ctrl Pts',(-8.5958791059675,12.2,-5.87737960096735));
#279221=CARTESIAN_POINT('Ctrl Pts',(-8.59772314724229,12.2,-5.87900024641592));
#279222=CARTESIAN_POINT('Ctrl Pts',(-8.59960188407517,12.2,-5.88066094137928));
#279223=CARTESIAN_POINT('Ctrl Pts',(-8.60151432942091,12.2,-5.8823615708991));
#279224=CARTESIAN_POINT('Ctrl Pts',(-8.60342677494035,12.2,-5.88406220057339));
#279225=CARTESIAN_POINT('Ctrl Pts',(-8.60537292788893,12.2,-5.88580276593591));
#279226=CARTESIAN_POINT('Ctrl Pts',(-8.60735182649905,12.2,-5.88758315445236));
#279227=CARTESIAN_POINT('Ctrl Pts',(-8.6093307249294,12.2,-5.88936354280707));
#279228=CARTESIAN_POINT('Ctrl Pts',(-8.61134236849269,12.2,-5.89118375430898));
#279229=CARTESIAN_POINT('Ctrl Pts',(-8.61338582016984,12.2,-5.89304367482648));
#279230=CARTESIAN_POINT('Ctrl Pts',(-8.615429271847,12.2,-5.89490359534398));
#279231=CARTESIAN_POINT('Ctrl Pts',(-8.61750453139654,12.2,-5.89680322461661));
#279232=CARTESIAN_POINT('Ctrl Pts',(-8.61961068615201,12.2,-5.89874245187776));
#279233=CARTESIAN_POINT('Ctrl Pts',(-8.62171684090748,12.2,-5.90068167913891));
#279234=CARTESIAN_POINT('Ctrl Pts',(-8.62385388904457,12.2,-5.90266050258931));
#279235=CARTESIAN_POINT('Ctrl Pts',(-8.62602094279714,12.2,-5.9046788090133));
#279236=CARTESIAN_POINT('Ctrl Pts',(-8.62818799674654,12.2,-5.90669711562061));
#279237=CARTESIAN_POINT('Ctrl Pts',(-8.63038505409052,12.2,-5.90875490690673));
#279238=CARTESIAN_POINT('Ctrl Pts',(-8.63261124812979,12.2,-5.91085206660607));
#279239=CARTESIAN_POINT('Ctrl Pts',(-8.63483744196683,12.2,-5.91294922611493));
#279240=CARTESIAN_POINT('Ctrl Pts',(-8.63709277010497,12.2,-5.91508575739323));
#279241=CARTESIAN_POINT('Ctrl Pts',(-8.63937638719896,12.2,-5.91726154574061));
#279242=CARTESIAN_POINT('Ctrl Pts',(-8.64166000429295,12.2,-5.919437334088));
#279243=CARTESIAN_POINT('Ctrl Pts',(-8.64397191091524,12.2,-5.9216523775805));
#279244=CARTESIAN_POINT('Ctrl Pts',(-8.64631127799502,12.2,-5.92390656674592));
#279245=CARTESIAN_POINT('Ctrl Pts',(-8.6486506452873,12.2,-5.92616075611608));
#279246=CARTESIAN_POINT('Ctrl Pts',(-8.65101747287396,12.2,-5.92845408682341));
#279247=CARTESIAN_POINT('Ctrl Pts',(-8.65341095442223,12.2,-5.93078644936889));
#279248=CARTESIAN_POINT('Ctrl Pts',(-8.6558044357531,12.2,-5.93311881170251));
#279249=CARTESIAN_POINT('Ctrl Pts',(-8.65822457123506,12.2,-5.93549020269223));
#279250=CARTESIAN_POINT('Ctrl Pts',(-8.66067056874055,12.2,-5.93790051194884));
#279251=CARTESIAN_POINT('Ctrl Pts',(-8.66311656624606,12.2,-5.94031082120544));
#279252=CARTESIAN_POINT('Ctrl Pts',(-8.66558843005363,12.2,-5.94276004585516));
#279253=CARTESIAN_POINT('Ctrl Pts',(-8.66808538546118,12.2,-5.94524807326209));
#279254=CARTESIAN_POINT('Ctrl Pts',(-8.67058234109555,12.2,-5.94773610089504));
#279255=CARTESIAN_POINT('Ctrl Pts',(-8.67310438880401,12.2,-5.95026293009466));
#279256=CARTESIAN_POINT('Ctrl Pts',(-8.67565077648806,12.2,-5.95282844969821));
#279257=CARTESIAN_POINT('Ctrl Pts',(-8.67819716394083,12.2,-5.95539396906874));
#279258=CARTESIAN_POINT('Ctrl Pts',(-8.68076788847761,12.2,-5.95799817577096));
#279259=CARTESIAN_POINT('Ctrl Pts',(-8.68336221571668,12.2,-5.96064095625827));
#279260=CARTESIAN_POINT('Ctrl Pts',(-8.68595654295576,12.2,-5.96328373674558));
#279261=CARTESIAN_POINT('Ctrl Pts',(-8.68857446975996,12.2,-5.96596509348544));
#279262=CARTESIAN_POINT('Ctrl Pts',(-8.69121527746127,12.2,-5.96868490802027));
#279263=CARTESIAN_POINT('Ctrl Pts',(-8.69385608540248,12.2,-5.97140472280214));
#279264=CARTESIAN_POINT('Ctrl Pts',(-8.69651977346155,12.2,-5.97416299852475));
#279265=CARTESIAN_POINT('Ctrl Pts',(-8.69920563427613,12.2,-5.97695961826314));
#279266=CARTESIAN_POINT('Ctrl Pts',(-8.70189149484674,12.2,-5.9797562377475));
#279267=CARTESIAN_POINT('Ctrl Pts',(-8.70459952848798,12.2,-5.98259120266751));
#279268=CARTESIAN_POINT('Ctrl Pts',(-8.70732904423459,12.2,-5.98546439799293));
#279269=CARTESIAN_POINT('Ctrl Pts',(-8.71005855998121,12.2,-5.98833759331834));
#279270=CARTESIAN_POINT('Ctrl Pts',(-8.712809559009,12.2,-5.99124901789818));
#279271=CARTESIAN_POINT('Ctrl Pts',(-8.71558136182404,12.2,-5.99419855728936));
#279272=CARTESIAN_POINT('Ctrl Pts',(-8.71789119758718,12.2,-5.99665650687131));
#279273=CARTESIAN_POINT('Ctrl Pts',(-8.72021548140903,12.2,-5.99914092571506));
#279274=CARTESIAN_POINT('Ctrl Pts',(-8.72255382883885,12.2,-6.0016517460609));
#279275=CARTESIAN_POINT('Ctrl Pts',(-8.72489217626867,12.2,-6.00416256640674));
#279276=CARTESIAN_POINT('Ctrl Pts',(-8.72724458758245,12.2,-6.00669978913697));
#279277=CARTESIAN_POINT('Ctrl Pts',(-8.72961068502373,12.2,-6.00926334623188));
#279278=CARTESIAN_POINT('Ctrl Pts',(-8.731976782465,12.2,-6.0118269033268));
#279279=CARTESIAN_POINT('Ctrl Pts',(-8.73435656410001,12.2,-6.0144167953555));
#279280=CARTESIAN_POINT('Ctrl Pts',(-8.73674966076669,12.2,-6.01703295500828));
#279281=CARTESIAN_POINT('Ctrl Pts',(-8.73914275743336,12.2,-6.01964911466105));
#279282=CARTESIAN_POINT('Ctrl Pts',(-8.74154916827364,12.2,-6.02229154210031));
#279283=CARTESIAN_POINT('Ctrl Pts',(-8.74396852599302,12.2,-6.02496017079308));
#279284=CARTESIAN_POINT('Ctrl Pts',(-8.74638788371239,12.2,-6.02762879948585));
#279285=CARTESIAN_POINT('Ctrl Pts',(-8.74882019127601,12.2,-6.0303236283378));
#279286=CARTESIAN_POINT('Ctrl Pts',(-8.75126508565167,12.2,-6.0330445911864));
#279287=CARTESIAN_POINT('Ctrl Pts',(-8.75370998002734,12.2,-6.03576555403501));
#279288=CARTESIAN_POINT('Ctrl Pts',(-8.75616746439987,12.2,-6.038512650419));
#279289=CARTESIAN_POINT('Ctrl Pts',(-8.75863718217829,12.2,-6.04128581173981));
#279290=CARTESIAN_POINT('Ctrl Pts',(-8.7611068999567,12.2,-6.0440589730606));
#279291=CARTESIAN_POINT('Ctrl Pts',(-8.76358885294193,12.2,-6.04685820099616));
#279292=CARTESIAN_POINT('Ctrl Pts',(-8.76608269153956,12.2,-6.04968342731967));
#279293=CARTESIAN_POINT('Ctrl Pts',(-8.76857653013719,12.2,-6.05250865364318));
#279294=CARTESIAN_POINT('Ctrl Pts',(-8.77108225506726,12.2,-6.05535987786309));
#279295=CARTESIAN_POINT('Ctrl Pts',(-8.77359952284596,12.2,-6.05823703314296));
#279296=CARTESIAN_POINT('Ctrl Pts',(-8.77611679062466,12.2,-6.06111418842282));
#279297=CARTESIAN_POINT('Ctrl Pts',(-8.77864560165358,12.2,-6.06401727391984));
#279298=CARTESIAN_POINT('Ctrl Pts',(-8.78118561859893,12.2,-6.06694622190807));
#279299=CARTESIAN_POINT('Ctrl Pts',(-8.78372563526744,12.2,-6.06987516957704));
#279300=CARTESIAN_POINT('Ctrl Pts',(-8.78627685702285,12.2,-6.07282997980376));
#279301=CARTESIAN_POINT('Ctrl Pts',(-8.78883895271491,12.2,-6.07581058635177));
#279302=CARTESIAN_POINT('Ctrl Pts',(-8.79140104868625,12.2,-6.07879119322467));
#279303=CARTESIAN_POINT('Ctrl Pts',(-8.79397401767406,12.2,-6.08179759316655));
#279304=CARTESIAN_POINT('Ctrl Pts',(-8.79655753218712,12.2,-6.08482971955336));
#279305=CARTESIAN_POINT('Ctrl Pts',(-8.79914104670016,12.2,-6.08786184594017));
#279306=CARTESIAN_POINT('Ctrl Pts',(-8.80173510762689,12.2,-6.09091970129317));
#279307=CARTESIAN_POINT('Ctrl Pts',(-8.80433939137607,12.2,-6.09400321330498));
#279308=CARTESIAN_POINT('Ctrl Pts',(-8.80694367512525,12.2,-6.09708672531679));
#279309=CARTESIAN_POINT('Ctrl Pts',(-8.80955818265387,12.2,-6.1001958954091));
#279310=CARTESIAN_POINT('Ctrl Pts',(-8.81218259639541,12.2,-6.10333065591114));
#279311=CARTESIAN_POINT('Ctrl Pts',(-8.81480701013694,12.2,-6.10646541641319));
#279312=CARTESIAN_POINT('Ctrl Pts',(-8.81744132993878,12.2,-6.10962576694863));
#279313=CARTESIAN_POINT('Ctrl Pts',(-8.82008524132718,12.2,-6.11281163826675));
#279314=CARTESIAN_POINT('Ctrl Pts',(-8.82272915271557,12.2,-6.11599750958487));
#279315=CARTESIAN_POINT('Ctrl Pts',(-8.82538265717086,12.2,-6.11920890262307));
#279316=CARTESIAN_POINT('Ctrl Pts',(-8.82804544605928,12.2,-6.12244574803842));
#279317=CARTESIAN_POINT('Ctrl Pts',(-8.8301756772861,12.2,-6.12503522451181));
#279318=CARTESIAN_POINT('Ctrl Pts',(-8.83231185130607,12.2,-6.12764099158576));
#279319=CARTESIAN_POINT('Ctrl Pts',(-8.83445381058588,12.2,-6.13026301213885));
#279320=CARTESIAN_POINT('Ctrl Pts',(-8.83659576957385,12.2,-6.13288503233469));
#279321=CARTESIAN_POINT('Ctrl Pts',(-8.83874351450323,12.2,-6.13552330721506));
#279322=CARTESIAN_POINT('Ctrl Pts',(-8.84089689204905,12.2,-6.13817780127477));
#279323=CARTESIAN_POINT('Ctrl Pts',(-8.84305026988826,12.2,-6.14083229569616));
#279324=CARTESIAN_POINT('Ctrl Pts',(-8.84520928007816,12.2,-6.14350300849172));
#279325=CARTESIAN_POINT('Ctrl Pts',(-8.8473737699187,12.2,-6.14618990569475));
#279326=CARTESIAN_POINT('Ctrl Pts',(-8.84953825946433,12.2,-6.14887680253171));
#279327=CARTESIAN_POINT('Ctrl Pts',(-8.85170822732348,12.2,-6.15157988369332));
#279328=CARTESIAN_POINT('Ctrl Pts',(-8.85388352564275,12.2,-6.15429911260547));
#279329=CARTESIAN_POINT('Ctrl Pts',(-8.8560588242584,12.2,-6.15701834188811));
#279330=CARTESIAN_POINT('Ctrl Pts',(-8.85823945179819,12.2,-6.15975372025736));
#279331=CARTESIAN_POINT('Ctrl Pts',(-8.86042525969545,12.2,-6.16250521074171));
#279332=CARTESIAN_POINT('Ctrl Pts',(-8.8631575194181,12.2,-6.1659445736597));
#279333=CARTESIAN_POINT('Ctrl Pts',(-8.8658978728794,12.2,-6.16940911354923));
#279334=CARTESIAN_POINT('Ctrl Pts',(-8.86864603267148,12.2,-6.172898760495));
#279335=CARTESIAN_POINT('Ctrl Pts',(-8.87084456032542,12.2,-6.17569047782338));
#279336=CARTESIAN_POINT('Ctrl Pts',(-8.87304808434192,12.2,-6.17849826257591));
#279337=CARTESIAN_POINT('Ctrl Pts',(-8.87525645943795,12.2,-6.18132208137362));
#279338=CARTESIAN_POINT('Ctrl Pts',(-8.87746483483486,12.2,-6.18414590055607));
#279339=CARTESIAN_POINT('Ctrl Pts',(-8.87967806187132,12.2,-6.18698575165742));
#279340=CARTESIAN_POINT('Ctrl Pts',(-8.88189599521473,12.2,-6.18984160075857));
#279341=CARTESIAN_POINT('Ctrl Pts',(-8.88411392825596,12.2,-6.19269744947061));
#279342=CARTESIAN_POINT('Ctrl Pts',(-8.88633656964897,12.2,-6.19556929464607));
#279343=CARTESIAN_POINT('Ctrl Pts',(-8.8885637754109,12.2,-6.19845710201947));
#279344=CARTESIAN_POINT('Ctrl Pts',(-8.89079098147626,12.2,-6.20134490978636));
#279345=CARTESIAN_POINT('Ctrl Pts',(-8.89302275296397,12.2,-6.20424867817396));
#279346=CARTESIAN_POINT('Ctrl Pts',(-8.8952589489849,12.2,-6.20716837323528));
#279347=CARTESIAN_POINT('Ctrl Pts',(-8.89749514470114,12.2,-6.21008806789879));
#279348=CARTESIAN_POINT('Ctrl Pts',(-8.89973576435583,12.2,-6.21302368800751));
#279349=CARTESIAN_POINT('Ctrl Pts',(-8.90198067061634,12.2,-6.2159751980424));
#279350=CARTESIAN_POINT('Ctrl Pts',(-8.9042255771827,12.2,-6.21892670847943));
#279351=CARTESIAN_POINT('Ctrl Pts',(-8.90647476709946,12.2,-6.22189410942071));
#279352=CARTESIAN_POINT('Ctrl Pts',(-8.90872810700003,12.2,-6.22487736324994));
#279353=CARTESIAN_POINT('Ctrl Pts',(-8.91098144690061,12.2,-6.22786061707918));
#279354=CARTESIAN_POINT('Ctrl Pts',(-8.91323893409335,12.2,-6.23085972520474));
#279355=CARTESIAN_POINT('Ctrl Pts',(-8.91550043282813,12.2,-6.23387465225957));
#279356=CARTESIAN_POINT('Ctrl Pts',(-8.91776193125479,12.2,-6.23688957890362));
#279357=CARTESIAN_POINT('Ctrl Pts',(-8.92002744089597,12.2,-6.23992032246372));
#279358=CARTESIAN_POINT('Ctrl Pts',(-8.9222968284985,12.2,-6.24296684850622));
#279359=CARTESIAN_POINT('Ctrl Pts',(-8.92456621641023,12.2,-6.2460133749638));
#279360=CARTESIAN_POINT('Ctrl Pts',(-8.92683947885618,12.2,-6.24907568269497));
#279361=CARTESIAN_POINT('Ctrl Pts',(-8.929116486814,12.2,-6.25215373775322));
#279362=CARTESIAN_POINT('Ctrl Pts',(-8.93139349446158,12.2,-6.2552317923921));
#279363=CARTESIAN_POINT('Ctrl Pts',(-8.93367424523641,12.2,-6.258325592265));
#279364=CARTESIAN_POINT('Ctrl Pts',(-8.935958607105,12.2,-6.26143510228757));
#279365=CARTESIAN_POINT('Ctrl Pts',(-8.93938515006349,12.2,-6.26609936753325));
#279366=CARTESIAN_POINT('Ctrl Pts',(-8.9428198185254,12.2,-6.27079898012494));
#279367=CARTESIAN_POINT('Ctrl Pts',(-8.94626217331649,12.2,-6.27553381745053));
#279368=CARTESIAN_POINT('Ctrl Pts',(-8.94855707671901,12.2,-6.27869037595431));
#279369=CARTESIAN_POINT('Ctrl Pts',(-8.95085539610796,12.2,-6.28186259047346));
#279370=CARTESIAN_POINT('Ctrl Pts',(-8.95315700223339,12.2,-6.28505042425829));
#279371=CARTESIAN_POINT('Ctrl Pts',(-8.95545860835881,12.2,-6.28823825804313));
#279372=CARTESIAN_POINT('Ctrl Pts',(-8.95776350188742,12.2,-6.29144171166591));
#279373=CARTESIAN_POINT('Ctrl Pts',(-8.96007155540241,12.2,-6.2946607475096));
#279374=CARTESIAN_POINT('Ctrl Pts',(-8.96237960860292,12.2,-6.2978797829147));
#279375=CARTESIAN_POINT('Ctrl Pts',(-8.9646908219466,12.2,-6.3011144018654));
#279376=CARTESIAN_POINT('Ctrl Pts',(-8.96700506849013,12.2,-6.30436456728108));
#279377=CARTESIAN_POINT('Ctrl Pts',(-8.96931931534898,12.2,-6.30761473313958));
#279378=CARTESIAN_POINT('Ctrl Pts',(-8.97163659549987,12.2,-6.31088044553658));
#279379=CARTESIAN_POINT('Ctrl Pts',(-8.97395678557107,12.2,-6.31416166799478));
#279380=CARTESIAN_POINT('Ctrl Pts',(-8.97627697532613,12.2,-6.3174428900059));
#279381=CARTESIAN_POINT('Ctrl Pts',(-8.97860007328637,12.2,-6.32073962412056));
#279382=CARTESIAN_POINT('Ctrl Pts',(-8.98092595648493,12.2,-6.32405183023766));
#279383=CARTESIAN_POINT('Ctrl Pts',(-8.98325184000039,12.2,-6.32736403680605));
#279384=CARTESIAN_POINT('Ctrl Pts',(-8.98558051028843,12.2,-6.33069171767352));
#279385=CARTESIAN_POINT('Ctrl Pts',(-8.98791184191566,12.2,-6.3340348355234));
#279386=CARTESIAN_POINT('Ctrl Pts',(-8.99024317322525,12.2,-6.33737795291779));
#279387=CARTESIAN_POINT('Ctrl Pts',(-8.99257716749385,12.2,-6.34073650793572));
#279388=CARTESIAN_POINT('Ctrl Pts',(-8.99491370291935,12.2,-6.34411046349379));
#279389=CARTESIAN_POINT('Ctrl Pts',(-8.9972502386632,12.2,-6.34748441951156));
#279390=CARTESIAN_POINT('Ctrl Pts',(-8.99958931723872,12.2,-6.35087377702523));
#279391=CARTESIAN_POINT('Ctrl Pts',(-9.00193081619982,12.2,-6.3542784975451));
#279392=CARTESIAN_POINT('Ctrl Pts',(-9.00427231484188,12.2,-6.35768321760108));
#279393=CARTESIAN_POINT('Ctrl Pts',(-9.0066162363529,12.2,-6.36110330248731));
#279394=CARTESIAN_POINT('Ctrl Pts',(-9.00896245838311,12.2,-6.3645387138716));
#279395=CARTESIAN_POINT('Ctrl Pts',(-9.01130868073298,12.2,-6.36797412572396));
#279396=CARTESIAN_POINT('Ctrl Pts',(-9.01365720745451,12.2,-6.3714248660115));
#279397=CARTESIAN_POINT('Ctrl Pts',(-9.01600791775998,12.2,-6.37489089649399));
#279398=CARTESIAN_POINT('Ctrl Pts',(-9.01835862774518,12.2,-6.37835692650424));
#279399=CARTESIAN_POINT('Ctrl Pts',(-9.02071152312996,12.2,-6.38183824699623));
#279400=CARTESIAN_POINT('Ctrl Pts',(-9.02306648638168,12.2,-6.38533482165327));
#279401=CARTESIAN_POINT('Ctrl Pts',(-9.02542144995427,12.2,-6.38883139678672));
#279402=CARTESIAN_POINT('Ctrl Pts',(-9.02777848116317,12.2,-6.3923432262133));
#279403=CARTESIAN_POINT('Ctrl Pts',(-9.03013746479171,12.2,-6.39587027151661));
#279404=CARTESIAN_POINT('Ctrl Pts',(-9.03249644842025,12.2,-6.39939731681992));
#279405=CARTESIAN_POINT('Ctrl Pts',(-9.03485738446018,12.2,-6.40293958068339));
#279406=CARTESIAN_POINT('Ctrl Pts',(-9.03722015931136,12.2,-6.40649702382327));
#279407=CARTESIAN_POINT('Ctrl Pts',(-9.03958293384062,12.2,-6.41005446647846));
#279408=CARTESIAN_POINT('Ctrl Pts',(-9.04194754608948,12.2,-6.41362708990791));
#279409=CARTESIAN_POINT('Ctrl Pts',(-9.0443138827401,12.2,-6.41721485596418));
#279410=CARTESIAN_POINT('Ctrl Pts',(-9.04668021971314,12.2,-6.42080262250928));
#279411=CARTESIAN_POINT('Ctrl Pts',(-9.0490482813804,12.2,-6.42440553203445));
#279412=CARTESIAN_POINT('Ctrl Pts',(-9.05141795562083,12.2,-6.42802354839985));
#279413=CARTESIAN_POINT('Ctrl Pts',(-9.05378762953839,12.2,-6.43164156427229));
#279414=CARTESIAN_POINT('Ctrl Pts',(-9.05615891469182,12.2,-6.43527468591496));
#279415=CARTESIAN_POINT('Ctrl Pts',(-9.05853170133109,12.2,-6.43892287722686));
#279416=CARTESIAN_POINT('Ctrl Pts',(-9.06090448829365,12.2,-6.44257106903582));
#279417=CARTESIAN_POINT('Ctrl Pts',(-9.06327877618818,12.2,-6.4462343287427));
#279418=CARTESIAN_POINT('Ctrl Pts',(-9.06565445460312,12.2,-6.44991262201711));
#279419=CARTESIAN_POINT('Ctrl Pts',(-9.06803013269437,12.2,-6.45359091479036));
#279420=CARTESIAN_POINT('Ctrl Pts',(-9.07040720007513,12.2,-6.45728423970382));
#279421=CARTESIAN_POINT('Ctrl Pts',(-9.07278555004731,12.2,-6.46099255845528));
#279422=CARTESIAN_POINT('Ctrl Pts',(-9.07516390034354,12.2,-6.46470087771199));
#279423=CARTESIAN_POINT('Ctrl Pts',(-9.07754353184263,12.2,-6.46842419346764));
#279424=CARTESIAN_POINT('Ctrl Pts',(-9.07992433619469,12.2,-6.4721624660057));
#279425=CARTESIAN_POINT('Ctrl Pts',(-9.08230514022236,12.2,-6.47590073803442));
#279426=CARTESIAN_POINT('Ctrl Pts',(-9.08468711684124,12.2,-6.47965396932436));
#279427=CARTESIAN_POINT('Ctrl Pts',(-9.0870701589876,12.2,-6.48342212020326));
#279428=CARTESIAN_POINT('Ctrl Pts',(-9.08885744067855,12.2,-6.48624823349079));
#279429=CARTESIAN_POINT('Ctrl Pts',(-9.09064532242522,12.2,-6.4890827392013));
#279430=CARTESIAN_POINT('Ctrl Pts',(-9.09243375765184,12.2,-6.49192562184688));
#279431=CARTESIAN_POINT('Ctrl Pts',(-9.09422219320335,12.2,-6.49476850500892));
#279432=CARTESIAN_POINT('Ctrl Pts',(-9.09601118414669,12.2,-6.49761976600661));
#279433=CARTESIAN_POINT('Ctrl Pts',(-9.09780068415682,12.2,-6.50047938813169));
#279434=CARTESIAN_POINT('Ctrl Pts',(-9.09959018384188,12.2,-6.50333900973726));
#279435=CARTESIAN_POINT('Ctrl Pts',(-9.1013801930769,12.2,-6.50620699290073));
#279436=CARTESIAN_POINT('Ctrl Pts',(-9.10317066813689,12.2,-6.50908332108862));
#279437=CARTESIAN_POINT('Ctrl Pts',(-9.10496114319688,12.2,-6.51195964927651));
#279438=CARTESIAN_POINT('Ctrl Pts',(-9.1067520827753,12.2,-6.51484432377786));
#279439=CARTESIAN_POINT('Ctrl Pts',(-9.10854344526001,12.2,-6.51773732747758));
#279440=CARTESIAN_POINT('Ctrl Pts',(-9.11033480774472,12.2,-6.5206303311773));
#279441=CARTESIAN_POINT('Ctrl Pts',(-9.11212659112207,12.2,-6.52353166530653));
#279442=CARTESIAN_POINT('Ctrl Pts',(-9.11391875177342,12.2,-6.52644131296398));
#279443=CARTESIAN_POINT('Ctrl Pts',(-9.11571091242477,12.2,-6.52935096062143));
#279444=CARTESIAN_POINT('Ctrl Pts',(-9.11750345090314,12.2,-6.53226892280484));
#279445=CARTESIAN_POINT('Ctrl Pts',(-9.1192963235463,12.2,-6.53519518290613));
#279446=CARTESIAN_POINT('Ctrl Pts',(-9.12108919618947,12.2,-6.53812144300742));
#279447=CARTESIAN_POINT('Ctrl Pts',(-9.12288240335759,12.2,-6.54105600101645));
#279448=CARTESIAN_POINT('Ctrl Pts',(-9.12467590187574,12.2,-6.54399884207509));
#279449=CARTESIAN_POINT('Ctrl Pts',(-9.1264694007197,12.2,-6.54694168366835));
#279450=CARTESIAN_POINT('Ctrl Pts',(-9.12826318826373,12.2,-6.54989280803055));
#279451=CARTESIAN_POINT('Ctrl Pts',(-9.13005722610782,12.2,-6.55285219817011));
#279452=CARTESIAN_POINT('Ctrl Pts',(-9.131851263626,12.2,-6.55581158777205));
#279453=CARTESIAN_POINT('Ctrl Pts',(-9.13364554887279,12.2,-6.55877924443433));
#279454=CARTESIAN_POINT('Ctrl Pts',(-9.13544003960558,12.2,-6.56175515214246));
#279455=CARTESIAN_POINT('Ctrl Pts',(-9.13723453033836,12.2,-6.5647310598506));
#279456=CARTESIAN_POINT('Ctrl Pts',(-9.13902922651089,12.2,-6.56771521753427));
#279457=CARTESIAN_POINT('Ctrl Pts',(-9.14082408565403,12.2,-6.57070761059293));
#279458=CARTESIAN_POINT('Ctrl Pts',(-9.14261894479717,12.2,-6.5737000036516));
#279459=CARTESIAN_POINT('Ctrl Pts',(-9.14441396688194,12.2,-6.5767006307426));
#279460=CARTESIAN_POINT('Ctrl Pts',(-9.14620911002505,12.2,-6.57970947775828));
#279461=CARTESIAN_POINT('Ctrl Pts',(-9.14800425316816,12.2,-6.58271832477397));
#279462=CARTESIAN_POINT('Ctrl Pts',(-9.14979951716959,12.2,-6.58573538963095));
#279463=CARTESIAN_POINT('Ctrl Pts',(-9.15159486127103,12.2,-6.58876065914535));
#279464=CARTESIAN_POINT('Ctrl Pts',(-9.15339020537247,12.2,-6.59178592865973));
#279465=CARTESIAN_POINT('Ctrl Pts',(-9.15518562849488,12.2,-6.5948194014044));
#279466=CARTESIAN_POINT('Ctrl Pts',(-9.15698108968601,12.2,-6.59786106069489));
#279467=CARTESIAN_POINT('Ctrl Pts',(-9.15937503815829,12.2,-6.60191660678392));
#279468=CARTESIAN_POINT('Ctrl Pts',(-9.16176905130973,12.2,-6.605986708391));
#279469=CARTESIAN_POINT('Ctrl Pts',(-9.16416303566243,12.2,-6.61007132755901));
#279470=CARTESIAN_POINT('Ctrl Pts',(-9.16595852376386,12.2,-6.61313479165675));
#279471=CARTESIAN_POINT('Ctrl Pts',(-9.16775399481528,12.2,-6.61620642219517));
#279472=CARTESIAN_POINT('Ctrl Pts',(-9.16954940704172,12.2,-6.61928620224996));
#279473=CARTESIAN_POINT('Ctrl Pts',(-9.17194329022776,12.2,-6.62339257602934));
#279474=CARTESIAN_POINT('Ctrl Pts',(-9.1743370700721,12.2,-6.62751343742149));
#279475=CARTESIAN_POINT('Ctrl Pts',(-9.1767306510914,12.2,-6.63164875242609));
#279476=CARTESIAN_POINT('Ctrl Pts',(-9.17852583669283,12.2,-6.63475023839782));
#279477=CARTESIAN_POINT('Ctrl Pts',(-9.18032090972761,12.2,-6.63785985188584));
#279478=CARTESIAN_POINT('Ctrl Pts',(-9.1821158294957,12.2,-6.64097757935659));
#279479=CARTESIAN_POINT('Ctrl Pts',(-9.1839107492638,12.2,-6.64409530682733));
#279480=CARTESIAN_POINT('Ctrl Pts',(-9.18570551742541,12.2,-6.6472211457024));
#279481=CARTESIAN_POINT('Ctrl Pts',(-9.18750009220169,12.2,-6.65035508272781));
#279482=CARTESIAN_POINT('Ctrl Pts',(-9.18929466697797,12.2,-6.65348901975322));
#279483=CARTESIAN_POINT('Ctrl Pts',(-9.19108904920546,12.2,-6.65663105373061));
#279484=CARTESIAN_POINT('Ctrl Pts',(-9.19288319848176,12.2,-6.65978116875544));
#279485=CARTESIAN_POINT('Ctrl Pts',(-9.19467734775807,12.2,-6.66293128378026));
#279486=CARTESIAN_POINT('Ctrl Pts',(-9.19647126521969,12.2,-6.66608947912071));
#279487=CARTESIAN_POINT('Ctrl Pts',(-9.19826490998788,12.2,-6.66925573967164));
#279488=CARTESIAN_POINT('Ctrl Pts',(-9.20005855475607,12.2,-6.67242200022257));
#279489=CARTESIAN_POINT('Ctrl Pts',(-9.2018519283576,12.2,-6.67559632525625));
#279490=CARTESIAN_POINT('Ctrl Pts',(-9.20364498962584,12.2,-6.67877869980621));
#279491=CARTESIAN_POINT('Ctrl Pts',(-9.20543805121982,12.2,-6.6819610749343));
#279492=CARTESIAN_POINT('Ctrl Pts',(-9.20723080226369,12.2,-6.68515149878128));
#279493=CARTESIAN_POINT('Ctrl Pts',(-9.20902320189913,12.2,-6.68834995545555));
#279494=CARTESIAN_POINT('Ctrl Pts',(-9.21081560120895,12.2,-6.69154841154877));
#279495=CARTESIAN_POINT('Ctrl Pts',(-9.21260765075567,12.2,-6.69475490061058));
#279496=CARTESIAN_POINT('Ctrl Pts',(-9.21439931057169,12.2,-6.69796940686362));
#279497=CARTESIAN_POINT('Ctrl Pts',(-9.21619097038772,12.2,-6.70118391311667));
#279498=CARTESIAN_POINT('Ctrl Pts',(-9.21798224052702,12.2,-6.70440643593556));
#279499=CARTESIAN_POINT('Ctrl Pts',(-9.21977308271192,12.2,-6.70763695906889));
#279500=CARTESIAN_POINT('Ctrl Pts',(-9.22156392489683,12.2,-6.71086748220222));
#279501=CARTESIAN_POINT('Ctrl Pts',(-9.22335433901509,12.2,-6.71410600670123));
#279502=CARTESIAN_POINT('Ctrl Pts',(-9.22514428682506,12.2,-6.71735251574995));
#279503=CARTESIAN_POINT('Ctrl Pts',(-9.22693423463502,12.2,-6.72059902479868));
#279504=CARTESIAN_POINT('Ctrl Pts',(-9.22872371752001,12.2,-6.72385351788039));
#279505=CARTESIAN_POINT('Ctrl Pts',(-9.23051269578838,12.2,-6.72711598088615));
#279506=CARTESIAN_POINT('Ctrl Pts',(-9.233494326344,12.2,-6.73255341942663));
#279507=CARTESIAN_POINT('Ctrl Pts',(-9.23647455619045,12.2,-6.73801299262213));
#279508=CARTESIAN_POINT('Ctrl Pts',(-9.23945320502344,12.2,-6.74349462473031));
#279509=CARTESIAN_POINT('Ctrl Pts',(-9.2412403942583,12.2,-6.74678360387573));
#279510=CARTESIAN_POINT('Ctrl Pts',(-9.24302701403688,12.2,-6.75008052466064));
#279511=CARTESIAN_POINT('Ctrl Pts',(-9.24481303130537,12.2,-6.7533853708732));
#279512=CARTESIAN_POINT('Ctrl Pts',(-9.24659904857387,12.2,-6.75669021708576));
#279513=CARTESIAN_POINT('Ctrl Pts',(-9.24838446267574,12.2,-6.76000299138112));
#279514=CARTESIAN_POINT('Ctrl Pts',(-9.25016923831931,12.2,-6.76332367555106));
#279515=CARTESIAN_POINT('Ctrl Pts',(-9.25195401428712,12.2,-6.76664436032426));
#279516=CARTESIAN_POINT('Ctrl Pts',(-9.25373815124641,12.2,-6.76997295699134));
#279517=CARTESIAN_POINT('Ctrl Pts',(-9.25552160417219,12.2,-6.77330944418565));
#279518=CARTESIAN_POINT('Ctrl Pts',(-9.25730505677395,12.2,-6.77664593077383));
#279519=CARTESIAN_POINT('Ctrl Pts',(-9.25908782435398,12.2,-6.77999030870202));
#279520=CARTESIAN_POINT('Ctrl Pts',(-9.2608698668365,12.2,-6.78334256091528));
#279521=CARTESIAN_POINT('Ctrl Pts',(-9.26265190931903,12.2,-6.78669481312853));
#279522=CARTESIAN_POINT('Ctrl Pts',(-9.26443322619546,12.2,-6.7900549376617));
#279523=CARTESIAN_POINT('Ctrl Pts',(-9.26621380150165,12.2,-6.79342292836566));
#279524=CARTESIAN_POINT('Ctrl Pts',(-9.26799437680784,12.2,-6.79679091906963));
#279525=CARTESIAN_POINT('Ctrl Pts',(-9.26977421267685,12.2,-6.80016677138531));
#279526=CARTESIAN_POINT('Ctrl Pts',(-9.27155330300005,12.2,-6.80355049700001));
#279527=CARTESIAN_POINT('Origin',(-5.66257110645729E-14,15.2,-1.77635683940025E-14));
#279528=CARTESIAN_POINT('',(-7.64657512344065,15.2,-7.01216898588537));
#279529=CARTESIAN_POINT('',(-7.64657512344065,12.2,-7.01216898588537));
#279530=CARTESIAN_POINT('',(-7.64657512300006,15.2,-7.01216898500002));
#279531=CARTESIAN_POINT('Origin',(-5.66257110645729E-14,12.2,-1.77635683940025E-14));
#279532=CARTESIAN_POINT('Origin',(-5.66257110645729E-14,15.2,-1.77635683940025E-14));
#279533=CARTESIAN_POINT('Origin',(-5.66257110645729E-14,15.2,-1.77635683940025E-14));
#279534=CARTESIAN_POINT('',(-8.20893607000006,15.2,-8.05377977100001));
#279535=CARTESIAN_POINT('',(-7.93573928331785,15.2,-8.32310290898372));
#279536=CARTESIAN_POINT('Origin',(-5.66257110645729E-14,15.2,-1.77635683940025E-14));
#279537=CARTESIAN_POINT('',(-7.93573928331785,12.2,-8.32310290898372));
#279538=CARTESIAN_POINT('',(-7.93573928300006,15.2,-8.32310290900002));
#279539=CARTESIAN_POINT('',(-8.20893607000006,12.2,-8.05377977100001));
#279540=CARTESIAN_POINT('Origin',(-5.66257110645729E-14,12.2,-1.77635683940025E-14));
#279541=CARTESIAN_POINT('',(-8.20893607000006,15.2,-8.05377977100001));
#279542=CARTESIAN_POINT('Ctrl Pts',(-7.64657512400006,15.2,-7.01216898700002));
#279543=CARTESIAN_POINT('Ctrl Pts',(-7.64657512400006,11.6,-7.01216898700002));
#279544=CARTESIAN_POINT('Ctrl Pts',(-7.64669302700005,15.2,-7.01229743700001));
#279545=CARTESIAN_POINT('Ctrl Pts',(-7.64669302700005,11.6,-7.01229743700001));
#279546=CARTESIAN_POINT('Ctrl Pts',(-7.64693288600006,15.2,-7.01255888400001));
#279547=CARTESIAN_POINT('Ctrl Pts',(-7.64693288600006,11.6,-7.01255888400001));
#279548=CARTESIAN_POINT('Ctrl Pts',(-7.64729613400006,15.2,-7.01295521700001));
#279549=CARTESIAN_POINT('Ctrl Pts',(-7.64729613400006,11.6,-7.01295521700001));
#279550=CARTESIAN_POINT('Ctrl Pts',(-7.64778506600006,15.2,-7.01348948000001));
#279551=CARTESIAN_POINT('Ctrl Pts',(-7.64778506600006,11.6,-7.01348948000001));
#279552=CARTESIAN_POINT('Ctrl Pts',(-7.64840281700006,15.2,-7.01416585800001));
#279553=CARTESIAN_POINT('Ctrl Pts',(-7.64840281700006,11.6,-7.01416585800001));
#279554=CARTESIAN_POINT('Ctrl Pts',(-7.64902989000006,15.2,-7.01485383100002));
#279555=CARTESIAN_POINT('Ctrl Pts',(-7.64902989000006,11.6,-7.01485383100002));
#279556=CARTESIAN_POINT('Ctrl Pts',(-7.64966267500006,15.2,-7.01554946900002));
#279557=CARTESIAN_POINT('Ctrl Pts',(-7.64966267500006,11.6,-7.01554946900002));
#279558=CARTESIAN_POINT('Ctrl Pts',(-7.65030113900006,15.2,-7.01625276700002));
#279559=CARTESIAN_POINT('Ctrl Pts',(-7.65030113900006,11.6,-7.01625276700002));
#279560=CARTESIAN_POINT('Ctrl Pts',(-7.65094525300006,15.2,-7.01696371500002));
#279561=CARTESIAN_POINT('Ctrl Pts',(-7.65094525300006,11.6,-7.01696371500002));
#279562=CARTESIAN_POINT('Ctrl Pts',(-7.65159498500006,15.2,-7.01768230800001));
#279563=CARTESIAN_POINT('Ctrl Pts',(-7.65159498500006,11.6,-7.01768230800001));
#279564=CARTESIAN_POINT('Ctrl Pts',(-7.65225030200006,15.2,-7.01840853700002));
#279565=CARTESIAN_POINT('Ctrl Pts',(-7.65225030200006,11.6,-7.01840853700002));
#279566=CARTESIAN_POINT('Ctrl Pts',(-7.65291117500006,15.2,-7.01914239300002));
#279567=CARTESIAN_POINT('Ctrl Pts',(-7.65291117500006,11.6,-7.01914239300002));
#279568=CARTESIAN_POINT('Ctrl Pts',(-7.65357757300006,15.2,-7.01988387000001));
#279569=CARTESIAN_POINT('Ctrl Pts',(-7.65357757300006,11.6,-7.01988387000001));
#279570=CARTESIAN_POINT('Ctrl Pts',(-7.65424946500006,15.2,-7.02063296100001));
#279571=CARTESIAN_POINT('Ctrl Pts',(-7.65424946500006,11.6,-7.02063296100001));
#279572=CARTESIAN_POINT('Ctrl Pts',(-7.65492682000006,15.2,-7.02138965600002));
#279573=CARTESIAN_POINT('Ctrl Pts',(-7.65492682000006,11.6,-7.02138965600002));
#279574=CARTESIAN_POINT('Ctrl Pts',(-7.65560960800006,15.2,-7.02215394900002));
#279575=CARTESIAN_POINT('Ctrl Pts',(-7.65560960800006,11.6,-7.02215394900002));
#279576=CARTESIAN_POINT('Ctrl Pts',(-7.65629779900006,15.2,-7.02292583300002));
#279577=CARTESIAN_POINT('Ctrl Pts',(-7.65629779900006,11.6,-7.02292583300002));
#279578=CARTESIAN_POINT('Ctrl Pts',(-7.65699136200006,15.2,-7.02370530000002));
#279579=CARTESIAN_POINT('Ctrl Pts',(-7.65699136200006,11.6,-7.02370530000002));
#279580=CARTESIAN_POINT('Ctrl Pts',(-7.65769027000006,15.2,-7.02449234200002));
#279581=CARTESIAN_POINT('Ctrl Pts',(-7.65769027000006,11.6,-7.02449234200002));
#279582=CARTESIAN_POINT('Ctrl Pts',(-7.65839449000006,15.2,-7.02528695200002));
#279583=CARTESIAN_POINT('Ctrl Pts',(-7.65839449000006,11.6,-7.02528695200002));
#279584=CARTESIAN_POINT('Ctrl Pts',(-7.65910399300005,15.2,-7.02608912100001));
#279585=CARTESIAN_POINT('Ctrl Pts',(-7.65910399300005,11.6,-7.02608912100001));
#279586=CARTESIAN_POINT('Ctrl Pts',(-7.65981875000006,15.2,-7.02689884500002));
#279587=CARTESIAN_POINT('Ctrl Pts',(-7.65981875000006,11.6,-7.02689884500002));
#279588=CARTESIAN_POINT('Ctrl Pts',(-7.66053873200006,15.2,-7.02771611300002));
#279589=CARTESIAN_POINT('Ctrl Pts',(-7.66053873200006,11.6,-7.02771611300002));
#279590=CARTESIAN_POINT('Ctrl Pts',(-7.66126391000006,15.2,-7.02854092000001));
#279591=CARTESIAN_POINT('Ctrl Pts',(-7.66126391000006,11.6,-7.02854092000001));
#279592=CARTESIAN_POINT('Ctrl Pts',(-7.66199425500006,15.2,-7.02937325800002));
#279593=CARTESIAN_POINT('Ctrl Pts',(-7.66199425500006,11.6,-7.02937325800002));
#279594=CARTESIAN_POINT('Ctrl Pts',(-7.66272973800006,15.2,-7.03021311800001));
#279595=CARTESIAN_POINT('Ctrl Pts',(-7.66272973800006,11.6,-7.03021311800001));
#279596=CARTESIAN_POINT('Ctrl Pts',(-7.66347032900006,15.2,-7.03106049500001));
#279597=CARTESIAN_POINT('Ctrl Pts',(-7.66347032900006,11.6,-7.03106049500001));
#279598=CARTESIAN_POINT('Ctrl Pts',(-7.66421600000006,15.2,-7.03191538200001));
#279599=CARTESIAN_POINT('Ctrl Pts',(-7.66421600000006,11.6,-7.03191538200001));
#279600=CARTESIAN_POINT('Ctrl Pts',(-7.66496672300006,15.2,-7.03277777000002));
#279601=CARTESIAN_POINT('Ctrl Pts',(-7.66496672300006,11.6,-7.03277777000002));
#279602=CARTESIAN_POINT('Ctrl Pts',(-7.66572246900005,15.2,-7.03364765100002));
#279603=CARTESIAN_POINT('Ctrl Pts',(-7.66572246900005,11.6,-7.03364765100002));
#279604=CARTESIAN_POINT('Ctrl Pts',(-7.66648321200006,15.2,-7.03452502000002));
#279605=CARTESIAN_POINT('Ctrl Pts',(-7.66648321200006,11.6,-7.03452502000002));
#279606=CARTESIAN_POINT('Ctrl Pts',(-7.66724892000005,15.2,-7.03540986900002));
#279607=CARTESIAN_POINT('Ctrl Pts',(-7.66724892000005,11.6,-7.03540986900002));
#279608=CARTESIAN_POINT('Ctrl Pts',(-7.66801956900006,15.2,-7.03630219100001));
#279609=CARTESIAN_POINT('Ctrl Pts',(-7.66801956900006,11.6,-7.03630219100001));
#279610=CARTESIAN_POINT('Ctrl Pts',(-7.66879512900006,15.2,-7.03720197800001));
#279611=CARTESIAN_POINT('Ctrl Pts',(-7.66879512900006,11.6,-7.03720197800001));
#279612=CARTESIAN_POINT('Ctrl Pts',(-7.66957557200006,15.2,-7.03810922400002));
#279613=CARTESIAN_POINT('Ctrl Pts',(-7.66957557200006,11.6,-7.03810922400002));
#279614=CARTESIAN_POINT('Ctrl Pts',(-7.67036087200006,15.2,-7.03902392000002));
#279615=CARTESIAN_POINT('Ctrl Pts',(-7.67036087200006,11.6,-7.03902392000002));
#279616=CARTESIAN_POINT('Ctrl Pts',(-7.67115100100006,15.2,-7.03994606100002));
#279617=CARTESIAN_POINT('Ctrl Pts',(-7.67115100100006,11.6,-7.03994606100002));
#279618=CARTESIAN_POINT('Ctrl Pts',(-7.67194593100006,15.2,-7.04087563800002));
#279619=CARTESIAN_POINT('Ctrl Pts',(-7.67194593100006,11.6,-7.04087563800002));
#279620=CARTESIAN_POINT('Ctrl Pts',(-7.67274563400005,15.2,-7.04181264600001));
#279621=CARTESIAN_POINT('Ctrl Pts',(-7.67274563400005,11.6,-7.04181264600001));
#279622=CARTESIAN_POINT('Ctrl Pts',(-7.67355008500005,15.2,-7.04275707600001));
#279623=CARTESIAN_POINT('Ctrl Pts',(-7.67355008500005,11.6,-7.04275707600001));
#279624=CARTESIAN_POINT('Ctrl Pts',(-7.67435925800006,15.2,-7.04370892300001));
#279625=CARTESIAN_POINT('Ctrl Pts',(-7.67435925800006,11.6,-7.04370892300001));
#279626=CARTESIAN_POINT('Ctrl Pts',(-7.67517312200006,15.2,-7.04466817700002));
#279627=CARTESIAN_POINT('Ctrl Pts',(-7.67517312200006,11.6,-7.04466817700002));
#279628=CARTESIAN_POINT('Ctrl Pts',(-7.67599165500006,15.2,-7.04563483400002));
#279629=CARTESIAN_POINT('Ctrl Pts',(-7.67599165500006,11.6,-7.04563483400002));
#279630=CARTESIAN_POINT('Ctrl Pts',(-7.67681482700005,15.2,-7.04660888500002));
#279631=CARTESIAN_POINT('Ctrl Pts',(-7.67681482700005,11.6,-7.04660888500002));
#279632=CARTESIAN_POINT('Ctrl Pts',(-7.67764261400006,15.2,-7.04759032400001));
#279633=CARTESIAN_POINT('Ctrl Pts',(-7.67764261400006,11.6,-7.04759032400001));
#279634=CARTESIAN_POINT('Ctrl Pts',(-7.67847498800006,15.2,-7.04857914500002));
#279635=CARTESIAN_POINT('Ctrl Pts',(-7.67847498800006,11.6,-7.04857914500002));
#279636=CARTESIAN_POINT('Ctrl Pts',(-7.67931192300006,15.2,-7.04957533800001));
#279637=CARTESIAN_POINT('Ctrl Pts',(-7.67931192300006,11.6,-7.04957533800001));
#279638=CARTESIAN_POINT('Ctrl Pts',(-7.68015339400005,15.2,-7.05057889900001));
#279639=CARTESIAN_POINT('Ctrl Pts',(-7.68015339400005,11.6,-7.05057889900001));
#279640=CARTESIAN_POINT('Ctrl Pts',(-7.68099937300006,15.2,-7.05158981900002));
#279641=CARTESIAN_POINT('Ctrl Pts',(-7.68099937300006,11.6,-7.05158981900002));
#279642=CARTESIAN_POINT('Ctrl Pts',(-7.68184983600006,15.2,-7.05260809300002));
#279643=CARTESIAN_POINT('Ctrl Pts',(-7.68184983600006,11.6,-7.05260809300002));
#279644=CARTESIAN_POINT('Ctrl Pts',(-7.68270475700006,15.2,-7.05363371400002));
#279645=CARTESIAN_POINT('Ctrl Pts',(-7.68270475700006,11.6,-7.05363371400002));
#279646=CARTESIAN_POINT('Ctrl Pts',(-7.68356411100005,15.2,-7.05466667300002));
#279647=CARTESIAN_POINT('Ctrl Pts',(-7.68356411100005,11.6,-7.05466667300002));
#279648=CARTESIAN_POINT('Ctrl Pts',(-7.68442787100006,15.2,-7.05570696600001));
#279649=CARTESIAN_POINT('Ctrl Pts',(-7.68442787100006,11.6,-7.05570696600001));
#279650=CARTESIAN_POINT('Ctrl Pts',(-7.68529601300005,15.2,-7.05675458400002));
#279651=CARTESIAN_POINT('Ctrl Pts',(-7.68529601300005,11.6,-7.05675458400002));
#279652=CARTESIAN_POINT('Ctrl Pts',(-7.68616851000005,15.2,-7.05780952100002));
#279653=CARTESIAN_POINT('Ctrl Pts',(-7.68616851000005,11.6,-7.05780952100002));
#279654=CARTESIAN_POINT('Ctrl Pts',(-7.68704533800006,15.2,-7.05887177000001));
#279655=CARTESIAN_POINT('Ctrl Pts',(-7.68704533800006,11.6,-7.05887177000001));
#279656=CARTESIAN_POINT('Ctrl Pts',(-7.68792647200006,15.2,-7.05994132500001));
#279657=CARTESIAN_POINT('Ctrl Pts',(-7.68792647200006,11.6,-7.05994132500001));
#279658=CARTESIAN_POINT('Ctrl Pts',(-7.68881188700006,15.2,-7.06101817800001));
#279659=CARTESIAN_POINT('Ctrl Pts',(-7.68881188700006,11.6,-7.06101817800001));
#279660=CARTESIAN_POINT('Ctrl Pts',(-7.68970155800006,15.2,-7.06210232300001));
#279661=CARTESIAN_POINT('Ctrl Pts',(-7.68970155800006,11.6,-7.06210232300001));
#279662=CARTESIAN_POINT('Ctrl Pts',(-7.69059546000006,15.2,-7.06319375400002));
#279663=CARTESIAN_POINT('Ctrl Pts',(-7.69059546000006,11.6,-7.06319375400002));
#279664=CARTESIAN_POINT('Ctrl Pts',(-7.69149356900006,15.2,-7.06429246300001));
#279665=CARTESIAN_POINT('Ctrl Pts',(-7.69149356900006,11.6,-7.06429246300001));
#279666=CARTESIAN_POINT('Ctrl Pts',(-7.69239586000006,15.2,-7.06539844300002));
#279667=CARTESIAN_POINT('Ctrl Pts',(-7.69239586000006,11.6,-7.06539844300002));
#279668=CARTESIAN_POINT('Ctrl Pts',(-7.69330230900006,15.2,-7.06651168900001));
#279669=CARTESIAN_POINT('Ctrl Pts',(-7.69330230900006,11.6,-7.06651168900001));
#279670=CARTESIAN_POINT('Ctrl Pts',(-7.69421289200006,15.2,-7.06763219300001));
#279671=CARTESIAN_POINT('Ctrl Pts',(-7.69421289200006,11.6,-7.06763219300001));
#279672=CARTESIAN_POINT('Ctrl Pts',(-7.69512758300006,15.2,-7.06875994900001));
#279673=CARTESIAN_POINT('Ctrl Pts',(-7.69512758300006,11.6,-7.06875994900001));
#279674=CARTESIAN_POINT('Ctrl Pts',(-7.69604636100006,15.2,-7.06989495100002));
#279675=CARTESIAN_POINT('Ctrl Pts',(-7.69604636100006,11.6,-7.06989495100002));
#279676=CARTESIAN_POINT('Ctrl Pts',(-7.69696919900006,15.2,-7.07103719000001));
#279677=CARTESIAN_POINT('Ctrl Pts',(-7.69696919900006,11.6,-7.07103719000001));
#279678=CARTESIAN_POINT('Ctrl Pts',(-7.69789607400006,15.2,-7.07218666200002));
#279679=CARTESIAN_POINT('Ctrl Pts',(-7.69789607400006,11.6,-7.07218666200002));
#279680=CARTESIAN_POINT('Ctrl Pts',(-7.69882696400006,15.2,-7.07334335800001));
#279681=CARTESIAN_POINT('Ctrl Pts',(-7.69882696400006,11.6,-7.07334335800001));
#279682=CARTESIAN_POINT('Ctrl Pts',(-7.69976184300005,15.2,-7.07450727300002));
#279683=CARTESIAN_POINT('Ctrl Pts',(-7.69976184300005,11.6,-7.07450727300002));
#279684=CARTESIAN_POINT('Ctrl Pts',(-7.70070068900005,15.2,-7.07567840100002));
#279685=CARTESIAN_POINT('Ctrl Pts',(-7.70070068900005,11.6,-7.07567840100002));
#279686=CARTESIAN_POINT('Ctrl Pts',(-7.70164347700005,15.2,-7.07685673500002));
#279687=CARTESIAN_POINT('Ctrl Pts',(-7.70164347700005,11.6,-7.07685673500002));
#279688=CARTESIAN_POINT('Ctrl Pts',(-7.70259018400005,15.2,-7.07804226800001));
#279689=CARTESIAN_POINT('Ctrl Pts',(-7.70259018400005,11.6,-7.07804226800001));
#279690=CARTESIAN_POINT('Ctrl Pts',(-7.70354078800005,15.2,-7.07923499200002));
#279691=CARTESIAN_POINT('Ctrl Pts',(-7.70354078800005,11.6,-7.07923499200002));
#279692=CARTESIAN_POINT('Ctrl Pts',(-7.70449526500006,15.2,-7.08043490300001));
#279693=CARTESIAN_POINT('Ctrl Pts',(-7.70449526500006,11.6,-7.08043490300001));
#279694=CARTESIAN_POINT('Ctrl Pts',(-7.70545359200005,15.2,-7.08164199400001));
#279695=CARTESIAN_POINT('Ctrl Pts',(-7.70545359200005,11.6,-7.08164199400001));
#279696=CARTESIAN_POINT('Ctrl Pts',(-7.70641574500005,15.2,-7.08285625800002));
#279697=CARTESIAN_POINT('Ctrl Pts',(-7.70641574500005,11.6,-7.08285625800002));
#279698=CARTESIAN_POINT('Ctrl Pts',(-7.70738170300006,15.2,-7.08407768800001));
#279699=CARTESIAN_POINT('Ctrl Pts',(-7.70738170300006,11.6,-7.08407768800001));
#279700=CARTESIAN_POINT('Ctrl Pts',(-7.70835144200006,15.2,-7.08530627800001));
#279701=CARTESIAN_POINT('Ctrl Pts',(-7.70835144200006,11.6,-7.08530627800001));
#279702=CARTESIAN_POINT('Ctrl Pts',(-7.70932493900006,15.2,-7.08654202100002));
#279703=CARTESIAN_POINT('Ctrl Pts',(-7.70932493900006,11.6,-7.08654202100002));
#279704=CARTESIAN_POINT('Ctrl Pts',(-7.71030217200006,15.2,-7.08778491300002));
#279705=CARTESIAN_POINT('Ctrl Pts',(-7.71030217200006,11.6,-7.08778491300002));
#279706=CARTESIAN_POINT('Ctrl Pts',(-7.71128311900006,15.2,-7.08903494500002));
#279707=CARTESIAN_POINT('Ctrl Pts',(-7.71128311900006,11.6,-7.08903494500002));
#279708=CARTESIAN_POINT('Ctrl Pts',(-7.71226775600006,15.2,-7.09029211100002));
#279709=CARTESIAN_POINT('Ctrl Pts',(-7.71226775600006,11.6,-7.09029211100002));
#279710=CARTESIAN_POINT('Ctrl Pts',(-7.71325606200006,15.2,-7.09155640600001));
#279711=CARTESIAN_POINT('Ctrl Pts',(-7.71325606200006,11.6,-7.09155640600001));
#279712=CARTESIAN_POINT('Ctrl Pts',(-7.71424801400006,15.2,-7.09282782200002));
#279713=CARTESIAN_POINT('Ctrl Pts',(-7.71424801400006,11.6,-7.09282782200002));
#279714=CARTESIAN_POINT('Ctrl Pts',(-7.71524359000006,15.2,-7.09410635300002));
#279715=CARTESIAN_POINT('Ctrl Pts',(-7.71524359000006,11.6,-7.09410635300002));
#279716=CARTESIAN_POINT('Ctrl Pts',(-7.71624276900006,15.2,-7.09539199400002));
#279717=CARTESIAN_POINT('Ctrl Pts',(-7.71624276900006,11.6,-7.09539199400002));
#279718=CARTESIAN_POINT('Ctrl Pts',(-7.71724552800006,15.2,-7.09668473700001));
#279719=CARTESIAN_POINT('Ctrl Pts',(-7.71724552800006,11.6,-7.09668473700001));
#279720=CARTESIAN_POINT('Ctrl Pts',(-7.71825184400006,15.2,-7.09798457600002));
#279721=CARTESIAN_POINT('Ctrl Pts',(-7.71825184400006,11.6,-7.09798457600002));
#279722=CARTESIAN_POINT('Ctrl Pts',(-7.71926169800006,15.2,-7.09929150500002));
#279723=CARTESIAN_POINT('Ctrl Pts',(-7.71926169800006,11.6,-7.09929150500002));
#279724=CARTESIAN_POINT('Ctrl Pts',(-7.72027506500006,15.2,-7.10060551700002));
#279725=CARTESIAN_POINT('Ctrl Pts',(-7.72027506500006,11.6,-7.10060551700002));
#279726=CARTESIAN_POINT('Ctrl Pts',(-7.72129192600006,15.2,-7.10192660800002));
#279727=CARTESIAN_POINT('Ctrl Pts',(-7.72129192600006,11.6,-7.10192660800002));
#279728=CARTESIAN_POINT('Ctrl Pts',(-7.72231225800006,15.2,-7.10325476900002));
#279729=CARTESIAN_POINT('Ctrl Pts',(-7.72231225800006,11.6,-7.10325476900002));
#279730=CARTESIAN_POINT('Ctrl Pts',(-7.72333604000006,15.2,-7.10458999400001));
#279731=CARTESIAN_POINT('Ctrl Pts',(-7.72333604000006,11.6,-7.10458999400001));
#279732=CARTESIAN_POINT('Ctrl Pts',(-7.72436325100006,15.2,-7.10593227900001));
#279733=CARTESIAN_POINT('Ctrl Pts',(-7.72436325100006,11.6,-7.10593227900001));
#279734=CARTESIAN_POINT('Ctrl Pts',(-7.72539386900006,15.2,-7.10728161400001));
#279735=CARTESIAN_POINT('Ctrl Pts',(-7.72539386900006,11.6,-7.10728161400001));
#279736=CARTESIAN_POINT('Ctrl Pts',(-7.72642787400006,15.2,-7.10863799800002));
#279737=CARTESIAN_POINT('Ctrl Pts',(-7.72642787400006,11.6,-7.10863799800002));
#279738=CARTESIAN_POINT('Ctrl Pts',(-7.72746524300005,15.2,-7.11000141900002));
#279739=CARTESIAN_POINT('Ctrl Pts',(-7.72746524300005,11.6,-7.11000141900002));
#279740=CARTESIAN_POINT('Ctrl Pts',(-7.72850595600006,15.2,-7.11137187600002));
#279741=CARTESIAN_POINT('Ctrl Pts',(-7.72850595600006,11.6,-7.11137187600002));
#279742=CARTESIAN_POINT('Ctrl Pts',(-7.72954999300006,15.2,-7.11274935900001));
#279743=CARTESIAN_POINT('Ctrl Pts',(-7.72954999300006,11.6,-7.11274935900001));
#279744=CARTESIAN_POINT('Ctrl Pts',(-7.73059733100006,15.2,-7.11413386300002));
#279745=CARTESIAN_POINT('Ctrl Pts',(-7.73059733100006,11.6,-7.11413386300002));
#279746=CARTESIAN_POINT('Ctrl Pts',(-7.73164795100006,15.2,-7.11552538200002));
#279747=CARTESIAN_POINT('Ctrl Pts',(-7.73164795100006,11.6,-7.11552538200002));
#279748=CARTESIAN_POINT('Ctrl Pts',(-7.73270183200006,15.2,-7.11692391000001));
#279749=CARTESIAN_POINT('Ctrl Pts',(-7.73270183200006,11.6,-7.11692391000001));
#279750=CARTESIAN_POINT('Ctrl Pts',(-7.73375895200005,15.2,-7.11832944100002));
#279751=CARTESIAN_POINT('Ctrl Pts',(-7.73375895200005,11.6,-7.11832944100002));
#279752=CARTESIAN_POINT('Ctrl Pts',(-7.73481929200006,15.2,-7.11974196800002));
#279753=CARTESIAN_POINT('Ctrl Pts',(-7.73481929200006,11.6,-7.11974196800002));
#279754=CARTESIAN_POINT('Ctrl Pts',(-7.73588283000005,15.2,-7.12116148600002));
#279755=CARTESIAN_POINT('Ctrl Pts',(-7.73588283000005,11.6,-7.12116148600002));
#279756=CARTESIAN_POINT('Ctrl Pts',(-7.73694954800006,15.2,-7.12258798800002));
#279757=CARTESIAN_POINT('Ctrl Pts',(-7.73694954800006,11.6,-7.12258798800002));
#279758=CARTESIAN_POINT('Ctrl Pts',(-7.73801942400006,15.2,-7.12402146700001));
#279759=CARTESIAN_POINT('Ctrl Pts',(-7.73801942400006,11.6,-7.12402146700001));
#279760=CARTESIAN_POINT('Ctrl Pts',(-7.73909243700006,15.2,-7.12546191900002));
#279761=CARTESIAN_POINT('Ctrl Pts',(-7.73909243700006,11.6,-7.12546191900002));
#279762=CARTESIAN_POINT('Ctrl Pts',(-7.74016856800006,15.2,-7.12690933700002));
#279763=CARTESIAN_POINT('Ctrl Pts',(-7.74016856800006,11.6,-7.12690933700002));
#279764=CARTESIAN_POINT('Ctrl Pts',(-7.74124779800006,15.2,-7.12836371300002));
#279765=CARTESIAN_POINT('Ctrl Pts',(-7.74124779800006,11.6,-7.12836371300002));
#279766=CARTESIAN_POINT('Ctrl Pts',(-7.74233010400006,15.2,-7.12982504500002));
#279767=CARTESIAN_POINT('Ctrl Pts',(-7.74233010400006,11.6,-7.12982504500002));
#279768=CARTESIAN_POINT('Ctrl Pts',(-7.74341546800006,15.2,-7.13129332400002));
#279769=CARTESIAN_POINT('Ctrl Pts',(-7.74341546800006,11.6,-7.13129332400002));
#279770=CARTESIAN_POINT('Ctrl Pts',(-7.74450387100006,15.2,-7.13276854400001));
#279771=CARTESIAN_POINT('Ctrl Pts',(-7.74450387100006,11.6,-7.13276854400001));
#279772=CARTESIAN_POINT('Ctrl Pts',(-7.74559529200006,15.2,-7.13425070000002));
#279773=CARTESIAN_POINT('Ctrl Pts',(-7.74559529200006,11.6,-7.13425070000002));
#279774=CARTESIAN_POINT('Ctrl Pts',(-7.74668971000006,15.2,-7.13573978500002));
#279775=CARTESIAN_POINT('Ctrl Pts',(-7.74668971000006,11.6,-7.13573978500002));
#279776=CARTESIAN_POINT('Ctrl Pts',(-7.74778710800006,15.2,-7.13723579300002));
#279777=CARTESIAN_POINT('Ctrl Pts',(-7.74778710800006,11.6,-7.13723579300002));
#279778=CARTESIAN_POINT('Ctrl Pts',(-7.74888746500006,15.2,-7.13873871900002));
#279779=CARTESIAN_POINT('Ctrl Pts',(-7.74888746500006,11.6,-7.13873871900002));
#279780=CARTESIAN_POINT('Ctrl Pts',(-7.74999076100006,15.2,-7.14024855600002));
#279781=CARTESIAN_POINT('Ctrl Pts',(-7.74999076100006,11.6,-7.14024855600002));
#279782=CARTESIAN_POINT('Ctrl Pts',(-7.75109697900006,15.2,-7.14176529900002));
#279783=CARTESIAN_POINT('Ctrl Pts',(-7.75109697900006,11.6,-7.14176529900002));
#279784=CARTESIAN_POINT('Ctrl Pts',(-7.75220609600006,15.2,-7.14328894200002));
#279785=CARTESIAN_POINT('Ctrl Pts',(-7.75220609600006,11.6,-7.14328894200002));
#279786=CARTESIAN_POINT('Ctrl Pts',(-7.75331809500006,15.2,-7.14481947600002));
#279787=CARTESIAN_POINT('Ctrl Pts',(-7.75331809500006,11.6,-7.14481947600002));
#279788=CARTESIAN_POINT('Ctrl Pts',(-7.75443295700006,15.2,-7.14635689900001));
#279789=CARTESIAN_POINT('Ctrl Pts',(-7.75443295700006,11.6,-7.14635689900001));
#279790=CARTESIAN_POINT('Ctrl Pts',(-7.75555066300005,15.2,-7.14790120400002));
#279791=CARTESIAN_POINT('Ctrl Pts',(-7.75555066300005,11.6,-7.14790120400002));
#279792=CARTESIAN_POINT('Ctrl Pts',(-7.75667119100006,15.2,-7.14945238400002));
#279793=CARTESIAN_POINT('Ctrl Pts',(-7.75667119100006,11.6,-7.14945238400002));
#279794=CARTESIAN_POINT('Ctrl Pts',(-7.75779452600006,15.2,-7.15101043300002));
#279795=CARTESIAN_POINT('Ctrl Pts',(-7.75779452600006,11.6,-7.15101043300002));
#279796=CARTESIAN_POINT('Ctrl Pts',(-7.75892064700006,15.2,-7.15257534600001));
#279797=CARTESIAN_POINT('Ctrl Pts',(-7.75892064700006,11.6,-7.15257534600001));
#279798=CARTESIAN_POINT('Ctrl Pts',(-7.76004953500006,15.2,-7.15414711700002));
#279799=CARTESIAN_POINT('Ctrl Pts',(-7.76004953500006,11.6,-7.15414711700002));
#279800=CARTESIAN_POINT('Ctrl Pts',(-7.76118117200006,15.2,-7.15572573900002));
#279801=CARTESIAN_POINT('Ctrl Pts',(-7.76118117200006,11.6,-7.15572573900002));
#279802=CARTESIAN_POINT('Ctrl Pts',(-7.76231553900006,15.2,-7.15731120800001));
#279803=CARTESIAN_POINT('Ctrl Pts',(-7.76231553900006,11.6,-7.15731120800001));
#279804=CARTESIAN_POINT('Ctrl Pts',(-7.76345261600006,15.2,-7.15890351600001));
#279805=CARTESIAN_POINT('Ctrl Pts',(-7.76345261600006,11.6,-7.15890351600001));
#279806=CARTESIAN_POINT('Ctrl Pts',(-7.76459238700006,15.2,-7.16050265800002));
#279807=CARTESIAN_POINT('Ctrl Pts',(-7.76459238700006,11.6,-7.16050265800002));
#279808=CARTESIAN_POINT('Ctrl Pts',(-7.76573483200006,15.2,-7.16210862900001));
#279809=CARTESIAN_POINT('Ctrl Pts',(-7.76573483200006,11.6,-7.16210862900001));
#279810=CARTESIAN_POINT('Ctrl Pts',(-7.76687993200006,15.2,-7.16372142100001));
#279811=CARTESIAN_POINT('Ctrl Pts',(-7.76687993200006,11.6,-7.16372142100001));
#279812=CARTESIAN_POINT('Ctrl Pts',(-7.76802767000006,15.2,-7.16534103000001));
#279813=CARTESIAN_POINT('Ctrl Pts',(-7.76802767000006,11.6,-7.16534103000001));
#279814=CARTESIAN_POINT('Ctrl Pts',(-7.76917802700006,15.2,-7.16696745000001));
#279815=CARTESIAN_POINT('Ctrl Pts',(-7.76917802700006,11.6,-7.16696745000001));
#279816=CARTESIAN_POINT('Ctrl Pts',(-7.77033098400005,15.2,-7.16860067400001));
#279817=CARTESIAN_POINT('Ctrl Pts',(-7.77033098400005,11.6,-7.16860067400001));
#279818=CARTESIAN_POINT('Ctrl Pts',(-7.77148652400006,15.2,-7.17024069600001));
#279819=CARTESIAN_POINT('Ctrl Pts',(-7.77148652400006,11.6,-7.17024069600001));
#279820=CARTESIAN_POINT('Ctrl Pts',(-7.77264462900006,15.2,-7.17188751300001));
#279821=CARTESIAN_POINT('Ctrl Pts',(-7.77264462900006,11.6,-7.17188751300001));
#279822=CARTESIAN_POINT('Ctrl Pts',(-7.77380527900006,15.2,-7.17354111600002));
#279823=CARTESIAN_POINT('Ctrl Pts',(-7.77380527900006,11.6,-7.17354111600002));
#279824=CARTESIAN_POINT('Ctrl Pts',(-7.77496845900006,15.2,-7.17520150000002));
#279825=CARTESIAN_POINT('Ctrl Pts',(-7.77496845900006,11.6,-7.17520150000002));
#279826=CARTESIAN_POINT('Ctrl Pts',(-7.77613414800006,15.2,-7.17686866000002));
#279827=CARTESIAN_POINT('Ctrl Pts',(-7.77613414800006,11.6,-7.17686866000002));
#279828=CARTESIAN_POINT('Ctrl Pts',(-7.77730233100005,15.2,-7.17854259000001));
#279829=CARTESIAN_POINT('Ctrl Pts',(-7.77730233100005,11.6,-7.17854259000001));
#279830=CARTESIAN_POINT('Ctrl Pts',(-7.77847298700006,15.2,-7.18022328300002));
#279831=CARTESIAN_POINT('Ctrl Pts',(-7.77847298700006,11.6,-7.18022328300002));
#279832=CARTESIAN_POINT('Ctrl Pts',(-7.77964610100006,15.2,-7.18191073400002));
#279833=CARTESIAN_POINT('Ctrl Pts',(-7.77964610100006,11.6,-7.18191073400002));
#279834=CARTESIAN_POINT('Ctrl Pts',(-7.78082165300006,15.2,-7.18360493900001));
#279835=CARTESIAN_POINT('Ctrl Pts',(-7.78082165300006,11.6,-7.18360493900001));
#279836=CARTESIAN_POINT('Ctrl Pts',(-7.78199962800005,15.2,-7.18530588900002));
#279837=CARTESIAN_POINT('Ctrl Pts',(-7.78199962800005,11.6,-7.18530588900002));
#279838=CARTESIAN_POINT('Ctrl Pts',(-7.78318000600006,15.2,-7.18701358000001));
#279839=CARTESIAN_POINT('Ctrl Pts',(-7.78318000600006,11.6,-7.18701358000001));
#279840=CARTESIAN_POINT('Ctrl Pts',(-7.78436277200005,15.2,-7.18872800600002));
#279841=CARTESIAN_POINT('Ctrl Pts',(-7.78436277200005,11.6,-7.18872800600002));
#279842=CARTESIAN_POINT('Ctrl Pts',(-7.78554790600006,15.2,-7.19044916200002));
#279843=CARTESIAN_POINT('Ctrl Pts',(-7.78554790600006,11.6,-7.19044916200002));
#279844=CARTESIAN_POINT('Ctrl Pts',(-7.78673539200006,15.2,-7.19217704100001));
#279845=CARTESIAN_POINT('Ctrl Pts',(-7.78673539200006,11.6,-7.19217704100001));
#279846=CARTESIAN_POINT('Ctrl Pts',(-7.78792521300005,15.2,-7.19391163700001));
#279847=CARTESIAN_POINT('Ctrl Pts',(-7.78792521300005,11.6,-7.19391163700001));
#279848=CARTESIAN_POINT('Ctrl Pts',(-7.78911735000006,15.2,-7.19565294600002));
#279849=CARTESIAN_POINT('Ctrl Pts',(-7.78911735000006,11.6,-7.19565294600002));
#279850=CARTESIAN_POINT('Ctrl Pts',(-7.79031178800006,15.2,-7.19740096100002));
#279851=CARTESIAN_POINT('Ctrl Pts',(-7.79031178800006,11.6,-7.19740096100002));
#279852=CARTESIAN_POINT('Ctrl Pts',(-7.79150850800006,15.2,-7.19915567700002));
#279853=CARTESIAN_POINT('Ctrl Pts',(-7.79150850800006,11.6,-7.19915567700002));
#279854=CARTESIAN_POINT('Ctrl Pts',(-7.79270749500006,15.2,-7.20091708700001));
#279855=CARTESIAN_POINT('Ctrl Pts',(-7.79270749500006,11.6,-7.20091708700001));
#279856=CARTESIAN_POINT('Ctrl Pts',(-7.79390872900006,15.2,-7.20268518700002));
#279857=CARTESIAN_POINT('Ctrl Pts',(-7.79390872900006,11.6,-7.20268518700002));
#279858=CARTESIAN_POINT('Ctrl Pts',(-7.79511219600005,15.2,-7.20445996900001));
#279859=CARTESIAN_POINT('Ctrl Pts',(-7.79511219600005,11.6,-7.20445996900001));
#279860=CARTESIAN_POINT('Ctrl Pts',(-7.79631787700006,15.2,-7.20624143100002));
#279861=CARTESIAN_POINT('Ctrl Pts',(-7.79631787700006,11.6,-7.20624143100002));
#279862=CARTESIAN_POINT('Ctrl Pts',(-7.79752575600006,15.2,-7.20802956400002));
#279863=CARTESIAN_POINT('Ctrl Pts',(-7.79752575600006,11.6,-7.20802956400002));
#279864=CARTESIAN_POINT('Ctrl Pts',(-7.79873581700006,15.2,-7.20982436300002));
#279865=CARTESIAN_POINT('Ctrl Pts',(-7.79873581700006,11.6,-7.20982436300002));
#279866=CARTESIAN_POINT('Ctrl Pts',(-7.79994804200006,15.2,-7.21162582400002));
#279867=CARTESIAN_POINT('Ctrl Pts',(-7.79994804200006,11.6,-7.21162582400002));
#279868=CARTESIAN_POINT('Ctrl Pts',(-7.80116241500006,15.2,-7.21343393900002));
#279869=CARTESIAN_POINT('Ctrl Pts',(-7.80116241500006,11.6,-7.21343393900002));
#279870=CARTESIAN_POINT('Ctrl Pts',(-7.80237891700006,15.2,-7.21524870400001));
#279871=CARTESIAN_POINT('Ctrl Pts',(-7.80237891700006,11.6,-7.21524870400001));
#279872=CARTESIAN_POINT('Ctrl Pts',(-7.80359753600005,15.2,-7.21707011200002));
#279873=CARTESIAN_POINT('Ctrl Pts',(-7.80359753600005,11.6,-7.21707011200002));
#279874=CARTESIAN_POINT('Ctrl Pts',(-7.80481825200006,15.2,-7.21889815900001));
#279875=CARTESIAN_POINT('Ctrl Pts',(-7.80481825200006,11.6,-7.21889815900001));
#279876=CARTESIAN_POINT('Ctrl Pts',(-7.80604105000006,15.2,-7.22073283800002));
#279877=CARTESIAN_POINT('Ctrl Pts',(-7.80604105000006,11.6,-7.22073283800002));
#279878=CARTESIAN_POINT('Ctrl Pts',(-7.80726591200006,15.2,-7.22257414400002));
#279879=CARTESIAN_POINT('Ctrl Pts',(-7.80726591200006,11.6,-7.22257414400002));
#279880=CARTESIAN_POINT('Ctrl Pts',(-7.80849282300006,15.2,-7.22442207200002));
#279881=CARTESIAN_POINT('Ctrl Pts',(-7.80849282300006,11.6,-7.22442207200002));
#279882=CARTESIAN_POINT('Ctrl Pts',(-7.80972176800006,15.2,-7.22627661400002));
#279883=CARTESIAN_POINT('Ctrl Pts',(-7.80972176800006,11.6,-7.22627661400002));
#279884=CARTESIAN_POINT('Ctrl Pts',(-7.81095272700006,15.2,-7.22813776700002));
#279885=CARTESIAN_POINT('Ctrl Pts',(-7.81095272700006,11.6,-7.22813776700002));
#279886=CARTESIAN_POINT('Ctrl Pts',(-7.81218568800006,15.2,-7.23000552500002));
#279887=CARTESIAN_POINT('Ctrl Pts',(-7.81218568800006,11.6,-7.23000552500002));
#279888=CARTESIAN_POINT('Ctrl Pts',(-7.81342063200006,15.2,-7.23187988100002));
#279889=CARTESIAN_POINT('Ctrl Pts',(-7.81342063200006,11.6,-7.23187988100002));
#279890=CARTESIAN_POINT('Ctrl Pts',(-7.81465754300006,15.2,-7.23376083000002));
#279891=CARTESIAN_POINT('Ctrl Pts',(-7.81465754300006,11.6,-7.23376083000002));
#279892=CARTESIAN_POINT('Ctrl Pts',(-7.81589640700006,15.2,-7.23564836800002));
#279893=CARTESIAN_POINT('Ctrl Pts',(-7.81589640700006,11.6,-7.23564836800002));
#279894=CARTESIAN_POINT('Ctrl Pts',(-7.81713720600005,15.2,-7.23754248800001));
#279895=CARTESIAN_POINT('Ctrl Pts',(-7.81713720600005,11.6,-7.23754248800001));
#279896=CARTESIAN_POINT('Ctrl Pts',(-7.81837992500006,15.2,-7.23944318200001));
#279897=CARTESIAN_POINT('Ctrl Pts',(-7.81837992500006,11.6,-7.23944318200001));
#279898=CARTESIAN_POINT('Ctrl Pts',(-7.81962454700006,15.2,-7.24135045000001));
#279899=CARTESIAN_POINT('Ctrl Pts',(-7.81962454700006,11.6,-7.24135045000001));
#279900=CARTESIAN_POINT('Ctrl Pts',(-7.82087105900005,15.2,-7.24326428200002));
#279901=CARTESIAN_POINT('Ctrl Pts',(-7.82087105900005,11.6,-7.24326428200002));
#279902=CARTESIAN_POINT('Ctrl Pts',(-7.82211944200006,15.2,-7.24518467400002));
#279903=CARTESIAN_POINT('Ctrl Pts',(-7.82211944200006,11.6,-7.24518467400002));
#279904=CARTESIAN_POINT('Ctrl Pts',(-7.82336968300006,15.2,-7.24711161900002));
#279905=CARTESIAN_POINT('Ctrl Pts',(-7.82336968300006,11.6,-7.24711161900002));
#279906=CARTESIAN_POINT('Ctrl Pts',(-7.82462176300006,15.2,-7.24904511400001));
#279907=CARTESIAN_POINT('Ctrl Pts',(-7.82462176300006,11.6,-7.24904511400001));
#279908=CARTESIAN_POINT('Ctrl Pts',(-7.82587566900006,15.2,-7.25098515300001));
#279909=CARTESIAN_POINT('Ctrl Pts',(-7.82587566900006,11.6,-7.25098515300001));
#279910=CARTESIAN_POINT('Ctrl Pts',(-7.82713138500006,15.2,-7.25293172800002));
#279911=CARTESIAN_POINT('Ctrl Pts',(-7.82713138500006,11.6,-7.25293172800002));
#279912=CARTESIAN_POINT('Ctrl Pts',(-7.82838889500006,15.2,-7.25488483600002));
#279913=CARTESIAN_POINT('Ctrl Pts',(-7.82838889500006,11.6,-7.25488483600002));
#279914=CARTESIAN_POINT('Ctrl Pts',(-7.82964818300006,15.2,-7.25684447100001));
#279915=CARTESIAN_POINT('Ctrl Pts',(-7.82964818300006,11.6,-7.25684447100001));
#279916=CARTESIAN_POINT('Ctrl Pts',(-7.83090923600006,15.2,-7.25881062600001));
#279917=CARTESIAN_POINT('Ctrl Pts',(-7.83090923600006,11.6,-7.25881062600001));
#279918=CARTESIAN_POINT('Ctrl Pts',(-7.83217203600006,15.2,-7.26078329800002));
#279919=CARTESIAN_POINT('Ctrl Pts',(-7.83217203600006,11.6,-7.26078329800002));
#279920=CARTESIAN_POINT('Ctrl Pts',(-7.83343656900006,15.2,-7.26276247900002));
#279921=CARTESIAN_POINT('Ctrl Pts',(-7.83343656900006,11.6,-7.26276247900002));
#279922=CARTESIAN_POINT('Ctrl Pts',(-7.83470281800006,15.2,-7.26474816500001));
#279923=CARTESIAN_POINT('Ctrl Pts',(-7.83470281800006,11.6,-7.26474816500001));
#279924=CARTESIAN_POINT('Ctrl Pts',(-7.83597077100006,15.2,-7.26674035100002));
#279925=CARTESIAN_POINT('Ctrl Pts',(-7.83597077100006,11.6,-7.26674035100002));
#279926=CARTESIAN_POINT('Ctrl Pts',(-7.83724040900006,15.2,-7.26873902900002));
#279927=CARTESIAN_POINT('Ctrl Pts',(-7.83724040900006,11.6,-7.26873902900002));
#279928=CARTESIAN_POINT('Ctrl Pts',(-7.83851172000006,15.2,-7.27074419600001));
#279929=CARTESIAN_POINT('Ctrl Pts',(-7.83851172000006,11.6,-7.27074419600001));
#279930=CARTESIAN_POINT('Ctrl Pts',(-7.83978468700005,15.2,-7.27275584500001));
#279931=CARTESIAN_POINT('Ctrl Pts',(-7.83978468700005,11.6,-7.27275584500001));
#279932=CARTESIAN_POINT('Ctrl Pts',(-7.84105929600006,15.2,-7.27477397100002));
#279933=CARTESIAN_POINT('Ctrl Pts',(-7.84105929600006,11.6,-7.27477397100002));
#279934=CARTESIAN_POINT('Ctrl Pts',(-7.84233553200006,15.2,-7.27679857100001));
#279935=CARTESIAN_POINT('Ctrl Pts',(-7.84233553200006,11.6,-7.27679857100001));
#279936=CARTESIAN_POINT('Ctrl Pts',(-7.84361337800006,15.2,-7.27882963500001));
#279937=CARTESIAN_POINT('Ctrl Pts',(-7.84361337800006,11.6,-7.27882963500001));
#279938=CARTESIAN_POINT('Ctrl Pts',(-7.84489282200005,15.2,-7.28086716100002));
#279939=CARTESIAN_POINT('Ctrl Pts',(-7.84489282200005,11.6,-7.28086716100002));
#279940=CARTESIAN_POINT('Ctrl Pts',(-7.84617384900006,15.2,-7.28291114200001));
#279941=CARTESIAN_POINT('Ctrl Pts',(-7.84617384900006,11.6,-7.28291114200001));
#279942=CARTESIAN_POINT('Ctrl Pts',(-7.84745644200005,15.2,-7.28496157300001));
#279943=CARTESIAN_POINT('Ctrl Pts',(-7.84745644200005,11.6,-7.28496157300001));
#279944=CARTESIAN_POINT('Ctrl Pts',(-7.84874058700006,15.2,-7.28701844800002));
#279945=CARTESIAN_POINT('Ctrl Pts',(-7.84874058700006,11.6,-7.28701844800002));
#279946=CARTESIAN_POINT('Ctrl Pts',(-7.85002627100006,15.2,-7.28908176300001));
#279947=CARTESIAN_POINT('Ctrl Pts',(-7.85002627100006,11.6,-7.28908176300001));
#279948=CARTESIAN_POINT('Ctrl Pts',(-7.85131347600006,15.2,-7.29115151100002));
#279949=CARTESIAN_POINT('Ctrl Pts',(-7.85131347600006,11.6,-7.29115151100002));
#279950=CARTESIAN_POINT('Ctrl Pts',(-7.85260219100006,15.2,-7.29322768800002));
#279951=CARTESIAN_POINT('Ctrl Pts',(-7.85260219100006,11.6,-7.29322768800002));
#279952=CARTESIAN_POINT('Ctrl Pts',(-7.85389239900006,15.2,-7.29531028800002));
#279953=CARTESIAN_POINT('Ctrl Pts',(-7.85389239900006,11.6,-7.29531028800002));
#279954=CARTESIAN_POINT('Ctrl Pts',(-7.85518408700005,15.2,-7.29739930400001));
#279955=CARTESIAN_POINT('Ctrl Pts',(-7.85518408700005,11.6,-7.29739930400001));
#279956=CARTESIAN_POINT('Ctrl Pts',(-7.85647723900006,15.2,-7.29949473300002));
#279957=CARTESIAN_POINT('Ctrl Pts',(-7.85647723900006,11.6,-7.29949473300002));
#279958=CARTESIAN_POINT('Ctrl Pts',(-7.85777184100005,15.2,-7.30159656800001));
#279959=CARTESIAN_POINT('Ctrl Pts',(-7.85777184100005,11.6,-7.30159656800001));
#279960=CARTESIAN_POINT('Ctrl Pts',(-7.85906787900006,15.2,-7.30370480400002));
#279961=CARTESIAN_POINT('Ctrl Pts',(-7.85906787900006,11.6,-7.30370480400002));
#279962=CARTESIAN_POINT('Ctrl Pts',(-7.86036533900005,15.2,-7.30581943700002));
#279963=CARTESIAN_POINT('Ctrl Pts',(-7.86036533900005,11.6,-7.30581943700002));
#279964=CARTESIAN_POINT('Ctrl Pts',(-7.86166420600006,15.2,-7.30794046000002));
#279965=CARTESIAN_POINT('Ctrl Pts',(-7.86166420600006,11.6,-7.30794046000002));
#279966=CARTESIAN_POINT('Ctrl Pts',(-7.86296446600005,15.2,-7.31006786700001));
#279967=CARTESIAN_POINT('Ctrl Pts',(-7.86296446600005,11.6,-7.31006786700001));
#279968=CARTESIAN_POINT('Ctrl Pts',(-7.86426610500006,15.2,-7.31220165500002));
#279969=CARTESIAN_POINT('Ctrl Pts',(-7.86426610500006,11.6,-7.31220165500002));
#279970=CARTESIAN_POINT('Ctrl Pts',(-7.86556910800006,15.2,-7.31434181700001));
#279971=CARTESIAN_POINT('Ctrl Pts',(-7.86556910800006,11.6,-7.31434181700001));
#279972=CARTESIAN_POINT('Ctrl Pts',(-7.86687346200006,15.2,-7.31648834800002));
#279973=CARTESIAN_POINT('Ctrl Pts',(-7.86687346200006,11.6,-7.31648834800002));
#279974=CARTESIAN_POINT('Ctrl Pts',(-7.86817915300006,15.2,-7.31864124200002));
#279975=CARTESIAN_POINT('Ctrl Pts',(-7.86817915300006,11.6,-7.31864124200002));
#279976=CARTESIAN_POINT('Ctrl Pts',(-7.86948616400006,15.2,-7.32080049500002));
#279977=CARTESIAN_POINT('Ctrl Pts',(-7.86948616400006,11.6,-7.32080049500002));
#279978=CARTESIAN_POINT('Ctrl Pts',(-7.87079448500006,15.2,-7.32296610000001));
#279979=CARTESIAN_POINT('Ctrl Pts',(-7.87079448500006,11.6,-7.32296610000001));
#279980=CARTESIAN_POINT('Ctrl Pts',(-7.87210409900006,15.2,-7.32513805300002));
#279981=CARTESIAN_POINT('Ctrl Pts',(-7.87210409900006,11.6,-7.32513805300002));
#279982=CARTESIAN_POINT('Ctrl Pts',(-7.87341499400006,15.2,-7.32731634800002));
#279983=CARTESIAN_POINT('Ctrl Pts',(-7.87341499400006,11.6,-7.32731634800002));
#279984=CARTESIAN_POINT('Ctrl Pts',(-7.87472715600006,15.2,-7.32950098000002));
#279985=CARTESIAN_POINT('Ctrl Pts',(-7.87472715600006,11.6,-7.32950098000002));
#279986=CARTESIAN_POINT('Ctrl Pts',(-7.87604057000006,15.2,-7.33169194300002));
#279987=CARTESIAN_POINT('Ctrl Pts',(-7.87604057000006,11.6,-7.33169194300002));
#279988=CARTESIAN_POINT('Ctrl Pts',(-7.87735522200006,15.2,-7.33388923300001));
#279989=CARTESIAN_POINT('Ctrl Pts',(-7.87735522200006,11.6,-7.33388923300001));
#279990=CARTESIAN_POINT('Ctrl Pts',(-7.87867110000006,15.2,-7.33609284300002));
#279991=CARTESIAN_POINT('Ctrl Pts',(-7.87867110000006,11.6,-7.33609284300002));
#279992=CARTESIAN_POINT('Ctrl Pts',(-7.87998818900006,15.2,-7.33830276900001));
#279993=CARTESIAN_POINT('Ctrl Pts',(-7.87998818900006,11.6,-7.33830276900001));
#279994=CARTESIAN_POINT('Ctrl Pts',(-7.88130647600005,15.2,-7.34051900600001));
#279995=CARTESIAN_POINT('Ctrl Pts',(-7.88130647600005,11.6,-7.34051900600001));
#279996=CARTESIAN_POINT('Ctrl Pts',(-7.88262594600005,15.2,-7.34274154700002));
#279997=CARTESIAN_POINT('Ctrl Pts',(-7.88262594600005,11.6,-7.34274154700002));
#279998=CARTESIAN_POINT('Ctrl Pts',(-7.88394658700006,15.2,-7.34497038800002));
#279999=CARTESIAN_POINT('Ctrl Pts',(-7.88394658700006,11.6,-7.34497038800002));
#280000=CARTESIAN_POINT('Ctrl Pts',(-7.88526838500006,15.2,-7.34720552200002));
#280001=CARTESIAN_POINT('Ctrl Pts',(-7.88526838500006,11.6,-7.34720552200002));
#280002=CARTESIAN_POINT('Ctrl Pts',(-7.88659132600006,15.2,-7.34944694700002));
#280003=CARTESIAN_POINT('Ctrl Pts',(-7.88659132600006,11.6,-7.34944694700002));
#280004=CARTESIAN_POINT('Ctrl Pts',(-7.88791539700006,15.2,-7.35169465400002));
#280005=CARTESIAN_POINT('Ctrl Pts',(-7.88791539700006,11.6,-7.35169465400002));
#280006=CARTESIAN_POINT('Ctrl Pts',(-7.88924058300006,15.2,-7.35394864100002));
#280007=CARTESIAN_POINT('Ctrl Pts',(-7.88924058300006,11.6,-7.35394864100002));
#280008=CARTESIAN_POINT('Ctrl Pts',(-7.89056687300006,15.2,-7.35620890000002));
#280009=CARTESIAN_POINT('Ctrl Pts',(-7.89056687300006,11.6,-7.35620890000002));
#280010=CARTESIAN_POINT('Ctrl Pts',(-7.89189425200006,15.2,-7.35847542700002));
#280011=CARTESIAN_POINT('Ctrl Pts',(-7.89189425200006,11.6,-7.35847542700002));
#280012=CARTESIAN_POINT('Ctrl Pts',(-7.89322270800006,15.2,-7.36074821600001));
#280013=CARTESIAN_POINT('Ctrl Pts',(-7.89322270800006,11.6,-7.36074821600001));
#280014=CARTESIAN_POINT('Ctrl Pts',(-7.89455222700005,15.2,-7.36302726400002));
#280015=CARTESIAN_POINT('Ctrl Pts',(-7.89455222700005,11.6,-7.36302726400002));
#280016=CARTESIAN_POINT('Ctrl Pts',(-7.89588279500006,15.2,-7.36531256200001));
#280017=CARTESIAN_POINT('Ctrl Pts',(-7.89588279500006,11.6,-7.36531256200001));
#280018=CARTESIAN_POINT('Ctrl Pts',(-7.89721440000006,15.2,-7.36760410800001));
#280019=CARTESIAN_POINT('Ctrl Pts',(-7.89721440000006,11.6,-7.36760410800001));
#280020=CARTESIAN_POINT('Ctrl Pts',(-7.89854702700006,15.2,-7.36990189500002));
#280021=CARTESIAN_POINT('Ctrl Pts',(-7.89854702700006,11.6,-7.36990189500002));
#280022=CARTESIAN_POINT('Ctrl Pts',(-7.89988066500006,15.2,-7.37220591900002));
#280023=CARTESIAN_POINT('Ctrl Pts',(-7.89988066500006,11.6,-7.37220591900002));
#280024=CARTESIAN_POINT('Ctrl Pts',(-7.90121530100006,15.2,-7.37451617400002));
#280025=CARTESIAN_POINT('Ctrl Pts',(-7.90121530100006,11.6,-7.37451617400002));
#280026=CARTESIAN_POINT('Ctrl Pts',(-7.90255092000006,15.2,-7.37683265400002));
#280027=CARTESIAN_POINT('Ctrl Pts',(-7.90255092000006,11.6,-7.37683265400002));
#280028=CARTESIAN_POINT('Ctrl Pts',(-7.90388750900006,15.2,-7.37915535500001));
#280029=CARTESIAN_POINT('Ctrl Pts',(-7.90388750900006,11.6,-7.37915535500001));
#280030=CARTESIAN_POINT('Ctrl Pts',(-7.90522505700006,15.2,-7.38148427100001));
#280031=CARTESIAN_POINT('Ctrl Pts',(-7.90522505700006,11.6,-7.38148427100001));
#280032=CARTESIAN_POINT('Ctrl Pts',(-7.90656355000006,15.2,-7.38381939700002));
#280033=CARTESIAN_POINT('Ctrl Pts',(-7.90656355000006,11.6,-7.38381939700002));
#280034=CARTESIAN_POINT('Ctrl Pts',(-7.90790297600005,15.2,-7.38616072800002));
#280035=CARTESIAN_POINT('Ctrl Pts',(-7.90790297600005,11.6,-7.38616072800002));
#280036=CARTESIAN_POINT('Ctrl Pts',(-7.90924332000006,15.2,-7.38850825800001));
#280037=CARTESIAN_POINT('Ctrl Pts',(-7.90924332000006,11.6,-7.38850825800001));
#280038=CARTESIAN_POINT('Ctrl Pts',(-7.91058457100006,15.2,-7.39086198300001));
#280039=CARTESIAN_POINT('Ctrl Pts',(-7.91058457100006,11.6,-7.39086198300001));
#280040=CARTESIAN_POINT('Ctrl Pts',(-7.91192671500006,15.2,-7.39322189600002));
#280041=CARTESIAN_POINT('Ctrl Pts',(-7.91192671500006,11.6,-7.39322189600002));
#280042=CARTESIAN_POINT('Ctrl Pts',(-7.91326974000006,15.2,-7.39558799400001));
#280043=CARTESIAN_POINT('Ctrl Pts',(-7.91326974000006,11.6,-7.39558799400001));
#280044=CARTESIAN_POINT('Ctrl Pts',(-7.91461363300006,15.2,-7.39796027100001));
#280045=CARTESIAN_POINT('Ctrl Pts',(-7.91461363300006,11.6,-7.39796027100001));
#280046=CARTESIAN_POINT('Ctrl Pts',(-7.91595838200006,15.2,-7.40033872100001));
#280047=CARTESIAN_POINT('Ctrl Pts',(-7.91595838200006,11.6,-7.40033872100001));
#280048=CARTESIAN_POINT('Ctrl Pts',(-7.91730397300006,15.2,-7.40272333900001));
#280049=CARTESIAN_POINT('Ctrl Pts',(-7.91730397300006,11.6,-7.40272333900001));
#280050=CARTESIAN_POINT('Ctrl Pts',(-7.91865039500006,15.2,-7.40511412000001));
#280051=CARTESIAN_POINT('Ctrl Pts',(-7.91865039500006,11.6,-7.40511412000001));
#280052=CARTESIAN_POINT('Ctrl Pts',(-7.91999763300005,15.2,-7.40751106000002));
#280053=CARTESIAN_POINT('Ctrl Pts',(-7.91999763300005,11.6,-7.40751106000002));
#280054=CARTESIAN_POINT('Ctrl Pts',(-7.92134567800005,15.2,-7.40991415100002));
#280055=CARTESIAN_POINT('Ctrl Pts',(-7.92134567800005,11.6,-7.40991415100002));
#280056=CARTESIAN_POINT('Ctrl Pts',(-7.92269451400006,15.2,-7.41232339000002));
#280057=CARTESIAN_POINT('Ctrl Pts',(-7.92269451400006,11.6,-7.41232339000002));
#280058=CARTESIAN_POINT('Ctrl Pts',(-7.92404413000006,15.2,-7.41473877200002));
#280059=CARTESIAN_POINT('Ctrl Pts',(-7.92404413000006,11.6,-7.41473877200002));
#280060=CARTESIAN_POINT('Ctrl Pts',(-7.92539451300006,15.2,-7.41716029100001));
#280061=CARTESIAN_POINT('Ctrl Pts',(-7.92539451300006,11.6,-7.41716029100001));
#280062=CARTESIAN_POINT('Ctrl Pts',(-7.92674565300005,15.2,-7.41958794100002));
#280063=CARTESIAN_POINT('Ctrl Pts',(-7.92674565300005,11.6,-7.41958794100002));
#280064=CARTESIAN_POINT('Ctrl Pts',(-7.92809753400006,15.2,-7.42202171900002));
#280065=CARTESIAN_POINT('Ctrl Pts',(-7.92809753400006,11.6,-7.42202171900002));
#280066=CARTESIAN_POINT('Ctrl Pts',(-7.92945014600006,15.2,-7.42446161800002));
#280067=CARTESIAN_POINT('Ctrl Pts',(-7.92945014600006,11.6,-7.42446161800002));
#280068=CARTESIAN_POINT('Ctrl Pts',(-7.93080347700006,15.2,-7.42690763300001));
#280069=CARTESIAN_POINT('Ctrl Pts',(-7.93080347700006,11.6,-7.42690763300001));
#280070=CARTESIAN_POINT('Ctrl Pts',(-7.93215751200006,15.2,-7.42935976000001));
#280071=CARTESIAN_POINT('Ctrl Pts',(-7.93215751200006,11.6,-7.42935976000001));
#280072=CARTESIAN_POINT('Ctrl Pts',(-7.93351224100006,15.2,-7.43181799300002));
#280073=CARTESIAN_POINT('Ctrl Pts',(-7.93351224100006,11.6,-7.43181799300002));
#280074=CARTESIAN_POINT('Ctrl Pts',(-7.93486765300005,15.2,-7.43428232700002));
#280075=CARTESIAN_POINT('Ctrl Pts',(-7.93486765300005,11.6,-7.43428232700002));
#280076=CARTESIAN_POINT('Ctrl Pts',(-7.93622373300006,15.2,-7.43675275700002));
#280077=CARTESIAN_POINT('Ctrl Pts',(-7.93622373300006,11.6,-7.43675275700002));
#280078=CARTESIAN_POINT('Ctrl Pts',(-7.93758046900006,15.2,-7.43922927700002));
#280079=CARTESIAN_POINT('Ctrl Pts',(-7.93758046900006,11.6,-7.43922927700002));
#280080=CARTESIAN_POINT('Ctrl Pts',(-7.93893785100006,15.2,-7.44171188300002));
#280081=CARTESIAN_POINT('Ctrl Pts',(-7.93893785100006,11.6,-7.44171188300002));
#280082=CARTESIAN_POINT('Ctrl Pts',(-7.94029586500006,15.2,-7.44420056900001));
#280083=CARTESIAN_POINT('Ctrl Pts',(-7.94029586500006,11.6,-7.44420056900001));
#280084=CARTESIAN_POINT('Ctrl Pts',(-7.94165450000006,15.2,-7.44669533000001));
#280085=CARTESIAN_POINT('Ctrl Pts',(-7.94165450000006,11.6,-7.44669533000001));
#280086=CARTESIAN_POINT('Ctrl Pts',(-7.94301374500006,15.2,-7.44919616200002));
#280087=CARTESIAN_POINT('Ctrl Pts',(-7.94301374500006,11.6,-7.44919616200002));
#280088=CARTESIAN_POINT('Ctrl Pts',(-7.94437358600005,15.2,-7.45170305800002));
#280089=CARTESIAN_POINT('Ctrl Pts',(-7.94437358600005,11.6,-7.45170305800002));
#280090=CARTESIAN_POINT('Ctrl Pts',(-7.94573401200006,15.2,-7.45421601400002));
#280091=CARTESIAN_POINT('Ctrl Pts',(-7.94573401200006,11.6,-7.45421601400002));
#280092=CARTESIAN_POINT('Ctrl Pts',(-7.94709501100006,15.2,-7.45673502500001));
#280093=CARTESIAN_POINT('Ctrl Pts',(-7.94709501100006,11.6,-7.45673502500001));
#280094=CARTESIAN_POINT('Ctrl Pts',(-7.94845657000005,15.2,-7.45926008500001));
#280095=CARTESIAN_POINT('Ctrl Pts',(-7.94845657000005,11.6,-7.45926008500001));
#280096=CARTESIAN_POINT('Ctrl Pts',(-7.94981868000006,15.2,-7.46179119000002));
#280097=CARTESIAN_POINT('Ctrl Pts',(-7.94981868000006,11.6,-7.46179119000002));
#280098=CARTESIAN_POINT('Ctrl Pts',(-7.95118132600006,15.2,-7.46432833400001));
#280099=CARTESIAN_POINT('Ctrl Pts',(-7.95118132600006,11.6,-7.46432833400001));
#280100=CARTESIAN_POINT('Ctrl Pts',(-7.95254449800006,15.2,-7.46687151200002));
#280101=CARTESIAN_POINT('Ctrl Pts',(-7.95254449800006,11.6,-7.46687151200002));
#280102=CARTESIAN_POINT('Ctrl Pts',(-7.95390818400006,15.2,-7.46942072000002));
#280103=CARTESIAN_POINT('Ctrl Pts',(-7.95390818400006,11.6,-7.46942072000002));
#280104=CARTESIAN_POINT('Ctrl Pts',(-7.95527237200006,15.2,-7.47197595100002));
#280105=CARTESIAN_POINT('Ctrl Pts',(-7.95527237200006,11.6,-7.47197595100002));
#280106=CARTESIAN_POINT('Ctrl Pts',(-7.95663705000005,15.2,-7.47453720100002));
#280107=CARTESIAN_POINT('Ctrl Pts',(-7.95663705000005,11.6,-7.47453720100002));
#280108=CARTESIAN_POINT('Ctrl Pts',(-7.95800220700006,15.2,-7.47710446400002));
#280109=CARTESIAN_POINT('Ctrl Pts',(-7.95800220700006,11.6,-7.47710446400002));
#280110=CARTESIAN_POINT('Ctrl Pts',(-7.95936783200006,15.2,-7.47967773800001));
#280111=CARTESIAN_POINT('Ctrl Pts',(-7.95936783200006,11.6,-7.47967773800001));
#280112=CARTESIAN_POINT('Ctrl Pts',(-7.96073391200006,15.2,-7.48225701400001));
#280113=CARTESIAN_POINT('Ctrl Pts',(-7.96073391200006,11.6,-7.48225701400001));
#280114=CARTESIAN_POINT('Ctrl Pts',(-7.96210043600006,15.2,-7.48484228900002));
#280115=CARTESIAN_POINT('Ctrl Pts',(-7.96210043600006,11.6,-7.48484228900002));
#280116=CARTESIAN_POINT('Ctrl Pts',(-7.96346739300006,15.2,-7.48743355600002));
#280117=CARTESIAN_POINT('Ctrl Pts',(-7.96346739300006,11.6,-7.48743355600002));
#280118=CARTESIAN_POINT('Ctrl Pts',(-7.96483477000006,15.2,-7.49003081400001));
#280119=CARTESIAN_POINT('Ctrl Pts',(-7.96483477000006,11.6,-7.49003081400001));
#280120=CARTESIAN_POINT('Ctrl Pts',(-7.96620255700006,15.2,-7.49263405300002));
#280121=CARTESIAN_POINT('Ctrl Pts',(-7.96620255700006,11.6,-7.49263405300002));
#280122=CARTESIAN_POINT('Ctrl Pts',(-7.96757074100006,15.2,-7.49524327100002));
#280123=CARTESIAN_POINT('Ctrl Pts',(-7.96757074100006,11.6,-7.49524327100002));
#280124=CARTESIAN_POINT('Ctrl Pts',(-7.96893931300006,15.2,-7.49785846200002));
#280125=CARTESIAN_POINT('Ctrl Pts',(-7.96893931300006,11.6,-7.49785846200002));
#280126=CARTESIAN_POINT('Ctrl Pts',(-7.97030826000006,15.2,-7.50047962100002));
#280127=CARTESIAN_POINT('Ctrl Pts',(-7.97030826000006,11.6,-7.50047962100002));
#280128=CARTESIAN_POINT('Ctrl Pts',(-7.97167757100006,15.2,-7.50310674200002));
#280129=CARTESIAN_POINT('Ctrl Pts',(-7.97167757100006,11.6,-7.50310674200002));
#280130=CARTESIAN_POINT('Ctrl Pts',(-7.97304723400006,15.2,-7.50573982200001));
#280131=CARTESIAN_POINT('Ctrl Pts',(-7.97304723400006,11.6,-7.50573982200001));
#280132=CARTESIAN_POINT('Ctrl Pts',(-7.97441723900005,15.2,-7.50837885600002));
#280133=CARTESIAN_POINT('Ctrl Pts',(-7.97441723900005,11.6,-7.50837885600002));
#280134=CARTESIAN_POINT('Ctrl Pts',(-7.97578757400006,15.2,-7.51102383600001));
#280135=CARTESIAN_POINT('Ctrl Pts',(-7.97578757400006,11.6,-7.51102383600001));
#280136=CARTESIAN_POINT('Ctrl Pts',(-7.97715822700006,15.2,-7.51367475900001));
#280137=CARTESIAN_POINT('Ctrl Pts',(-7.97715822700006,11.6,-7.51367475900001));
#280138=CARTESIAN_POINT('Ctrl Pts',(-7.97852918800006,15.2,-7.51633161900001));
#280139=CARTESIAN_POINT('Ctrl Pts',(-7.97852918800006,11.6,-7.51633161900001));
#280140=CARTESIAN_POINT('Ctrl Pts',(-7.97990044600006,15.2,-7.51899441200001));
#280141=CARTESIAN_POINT('Ctrl Pts',(-7.97990044600006,11.6,-7.51899441200001));
#280142=CARTESIAN_POINT('Ctrl Pts',(-7.98127198900006,15.2,-7.52166313300001));
#280143=CARTESIAN_POINT('Ctrl Pts',(-7.98127198900006,11.6,-7.52166313300001));
#280144=CARTESIAN_POINT('Ctrl Pts',(-7.98264380500005,15.2,-7.52433777700002));
#280145=CARTESIAN_POINT('Ctrl Pts',(-7.98264380500005,11.6,-7.52433777700002));
#280146=CARTESIAN_POINT('Ctrl Pts',(-7.98401588500005,15.2,-7.52701833700002));
#280147=CARTESIAN_POINT('Ctrl Pts',(-7.98401588500005,11.6,-7.52701833700002));
#280148=CARTESIAN_POINT('Ctrl Pts',(-7.98538821700006,15.2,-7.52970480900002));
#280149=CARTESIAN_POINT('Ctrl Pts',(-7.98538821700006,11.6,-7.52970480900002));
#280150=CARTESIAN_POINT('Ctrl Pts',(-7.98676079000006,15.2,-7.53239719000002));
#280151=CARTESIAN_POINT('Ctrl Pts',(-7.98676079000006,11.6,-7.53239719000002));
#280152=CARTESIAN_POINT('Ctrl Pts',(-7.98813359300006,15.2,-7.53509547300002));
#280153=CARTESIAN_POINT('Ctrl Pts',(-7.98813359300006,11.6,-7.53509547300002));
#280154=CARTESIAN_POINT('Ctrl Pts',(-7.98950661400006,15.2,-7.53779965300001));
#280155=CARTESIAN_POINT('Ctrl Pts',(-7.98950661400006,11.6,-7.53779965300001));
#280156=CARTESIAN_POINT('Ctrl Pts',(-7.99087984500006,15.2,-7.54050972600002));
#280157=CARTESIAN_POINT('Ctrl Pts',(-7.99087984500006,11.6,-7.54050972600002));
#280158=CARTESIAN_POINT('Ctrl Pts',(-7.99225327200006,15.2,-7.54322568500001));
#280159=CARTESIAN_POINT('Ctrl Pts',(-7.99225327200006,11.6,-7.54322568500001));
#280160=CARTESIAN_POINT('Ctrl Pts',(-7.99362688500005,15.2,-7.54594752700001));
#280161=CARTESIAN_POINT('Ctrl Pts',(-7.99362688500005,11.6,-7.54594752700001));
#280162=CARTESIAN_POINT('Ctrl Pts',(-7.99500067400006,15.2,-7.54867524600002));
#280163=CARTESIAN_POINT('Ctrl Pts',(-7.99500067400006,11.6,-7.54867524600002));
#280164=CARTESIAN_POINT('Ctrl Pts',(-7.99637462700005,15.2,-7.55140883700002));
#280165=CARTESIAN_POINT('Ctrl Pts',(-7.99637462700005,11.6,-7.55140883700002));
#280166=CARTESIAN_POINT('Ctrl Pts',(-7.99774873400006,15.2,-7.55414829500002));
#280167=CARTESIAN_POINT('Ctrl Pts',(-7.99774873400006,11.6,-7.55414829500002));
#280168=CARTESIAN_POINT('Ctrl Pts',(-7.99912298400006,15.2,-7.55689361500002));
#280169=CARTESIAN_POINT('Ctrl Pts',(-7.99912298400006,11.6,-7.55689361500002));
#280170=CARTESIAN_POINT('Ctrl Pts',(-8.00049736600006,15.2,-7.55964479300002));
#280171=CARTESIAN_POINT('Ctrl Pts',(-8.00049736600006,11.6,-7.55964479300002));
#280172=CARTESIAN_POINT('Ctrl Pts',(-8.00187187000006,15.2,-7.56240182300001));
#280173=CARTESIAN_POINT('Ctrl Pts',(-8.00187187000006,11.6,-7.56240182300001));
#280174=CARTESIAN_POINT('Ctrl Pts',(-8.00324648500006,15.2,-7.56516470000002));
#280175=CARTESIAN_POINT('Ctrl Pts',(-8.00324648500006,11.6,-7.56516470000002));
#280176=CARTESIAN_POINT('Ctrl Pts',(-8.00462120000006,15.2,-7.56793341800002));
#280177=CARTESIAN_POINT('Ctrl Pts',(-8.00462120000006,11.6,-7.56793341800002));
#280178=CARTESIAN_POINT('Ctrl Pts',(-8.00599600400006,15.2,-7.57070797400001));
#280179=CARTESIAN_POINT('Ctrl Pts',(-8.00599600400006,11.6,-7.57070797400001));
#280180=CARTESIAN_POINT('Ctrl Pts',(-8.00737088600006,15.2,-7.57348836200002));
#280181=CARTESIAN_POINT('Ctrl Pts',(-8.00737088600006,11.6,-7.57348836200002));
#280182=CARTESIAN_POINT('Ctrl Pts',(-8.00874583800006,15.2,-7.57627457800002));
#280183=CARTESIAN_POINT('Ctrl Pts',(-8.00874583800006,11.6,-7.57627457800002));
#280184=CARTESIAN_POINT('Ctrl Pts',(-8.01012084800006,15.2,-7.57906661500002));
#280185=CARTESIAN_POINT('Ctrl Pts',(-8.01012084800006,11.6,-7.57906661500002));
#280186=CARTESIAN_POINT('Ctrl Pts',(-8.01149590400006,15.2,-7.58186447000002));
#280187=CARTESIAN_POINT('Ctrl Pts',(-8.01149590400006,11.6,-7.58186447000002));
#280188=CARTESIAN_POINT('Ctrl Pts',(-8.01287099700006,15.2,-7.58466813700001));
#280189=CARTESIAN_POINT('Ctrl Pts',(-8.01287099700006,11.6,-7.58466813700001));
#280190=CARTESIAN_POINT('Ctrl Pts',(-8.01424611600006,15.2,-7.58747761000001));
#280191=CARTESIAN_POINT('Ctrl Pts',(-8.01424611600006,11.6,-7.58747761000001));
#280192=CARTESIAN_POINT('Ctrl Pts',(-8.01562125100006,15.2,-7.59029288600002));
#280193=CARTESIAN_POINT('Ctrl Pts',(-8.01562125100006,11.6,-7.59029288600002));
#280194=CARTESIAN_POINT('Ctrl Pts',(-8.01699639200006,15.2,-7.59311396000002));
#280195=CARTESIAN_POINT('Ctrl Pts',(-8.01699639200006,11.6,-7.59311396000002));
#280196=CARTESIAN_POINT('Ctrl Pts',(-8.01837152700006,15.2,-7.59594082500002));
#280197=CARTESIAN_POINT('Ctrl Pts',(-8.01837152700006,11.6,-7.59594082500002));
#280198=CARTESIAN_POINT('Ctrl Pts',(-8.01974664600005,15.2,-7.59877347800002));
#280199=CARTESIAN_POINT('Ctrl Pts',(-8.01974664600005,11.6,-7.59877347800002));
#280200=CARTESIAN_POINT('Ctrl Pts',(-8.02112174100006,15.2,-7.60161191300002));
#280201=CARTESIAN_POINT('Ctrl Pts',(-8.02112174100006,11.6,-7.60161191300002));
#280202=CARTESIAN_POINT('Ctrl Pts',(-8.02249679900006,15.2,-7.60445612600002));
#280203=CARTESIAN_POINT('Ctrl Pts',(-8.02249679900006,11.6,-7.60445612600002));
#280204=CARTESIAN_POINT('Ctrl Pts',(-8.02387181100006,15.2,-7.60730611100002));
#280205=CARTESIAN_POINT('Ctrl Pts',(-8.02387181100006,11.6,-7.60730611100002));
#280206=CARTESIAN_POINT('Ctrl Pts',(-8.02524676500006,15.2,-7.61016186300001));
#280207=CARTESIAN_POINT('Ctrl Pts',(-8.02524676500006,11.6,-7.61016186300001));
#280208=CARTESIAN_POINT('Ctrl Pts',(-8.02662165400006,15.2,-7.61302337700001));
#280209=CARTESIAN_POINT('Ctrl Pts',(-8.02662165400006,11.6,-7.61302337700001));
#280210=CARTESIAN_POINT('Ctrl Pts',(-8.02799646500005,15.2,-7.61589064900001));
#280211=CARTESIAN_POINT('Ctrl Pts',(-8.02799646500005,11.6,-7.61589064900001));
#280212=CARTESIAN_POINT('Ctrl Pts',(-8.02937118700006,15.2,-7.61876367400002));
#280213=CARTESIAN_POINT('Ctrl Pts',(-8.02937118700006,11.6,-7.61876367400002));
#280214=CARTESIAN_POINT('Ctrl Pts',(-8.03074581300006,15.2,-7.62164244600001));
#280215=CARTESIAN_POINT('Ctrl Pts',(-8.03074581300006,11.6,-7.62164244600001));
#280216=CARTESIAN_POINT('Ctrl Pts',(-8.03212033200005,15.2,-7.62452696000001));
#280217=CARTESIAN_POINT('Ctrl Pts',(-8.03212033200005,11.6,-7.62452696000001));
#280218=CARTESIAN_POINT('Ctrl Pts',(-8.03349473300005,15.2,-7.62741721300002));
#280219=CARTESIAN_POINT('Ctrl Pts',(-8.03349473300005,11.6,-7.62741721300002));
#280220=CARTESIAN_POINT('Ctrl Pts',(-8.03486900600006,15.2,-7.63031319800002));
#280221=CARTESIAN_POINT('Ctrl Pts',(-8.03486900600006,11.6,-7.63031319800002));
#280222=CARTESIAN_POINT('Ctrl Pts',(-8.03624314100006,15.2,-7.63321491200001));
#280223=CARTESIAN_POINT('Ctrl Pts',(-8.03624314100006,11.6,-7.63321491200001));
#280224=CARTESIAN_POINT('Ctrl Pts',(-8.03761712700006,15.2,-7.63612234800001));
#280225=CARTESIAN_POINT('Ctrl Pts',(-8.03761712700006,11.6,-7.63612234800001));
#280226=CARTESIAN_POINT('Ctrl Pts',(-8.03899095600006,15.2,-7.63903550000002));
#280227=CARTESIAN_POINT('Ctrl Pts',(-8.03899095600006,11.6,-7.63903550000002));
#280228=CARTESIAN_POINT('Ctrl Pts',(-8.04036461700005,15.2,-7.64195436700002));
#280229=CARTESIAN_POINT('Ctrl Pts',(-8.04036461700005,11.6,-7.64195436700002));
#280230=CARTESIAN_POINT('Ctrl Pts',(-8.04173810000006,15.2,-7.64487894200002));
#280231=CARTESIAN_POINT('Ctrl Pts',(-8.04173810000006,11.6,-7.64487894200002));
#280232=CARTESIAN_POINT('Ctrl Pts',(-8.04311139500006,15.2,-7.64780921900002));
#280233=CARTESIAN_POINT('Ctrl Pts',(-8.04311139500006,11.6,-7.64780921900002));
#280234=CARTESIAN_POINT('Ctrl Pts',(-8.04448449200006,15.2,-7.65074519500001));
#280235=CARTESIAN_POINT('Ctrl Pts',(-8.04448449200006,11.6,-7.65074519500001));
#280236=CARTESIAN_POINT('Ctrl Pts',(-8.04585738100006,15.2,-7.65368686400001));
#280237=CARTESIAN_POINT('Ctrl Pts',(-8.04585738100006,11.6,-7.65368686400001));
#280238=CARTESIAN_POINT('Ctrl Pts',(-8.04723005200006,15.2,-7.65663422200002));
#280239=CARTESIAN_POINT('Ctrl Pts',(-8.04723005200006,11.6,-7.65663422200002));
#280240=CARTESIAN_POINT('Ctrl Pts',(-8.04860249700006,15.2,-7.65958726300001));
#280241=CARTESIAN_POINT('Ctrl Pts',(-8.04860249700006,11.6,-7.65958726300001));
#280242=CARTESIAN_POINT('Ctrl Pts',(-8.04997470400006,15.2,-7.66254598200002));
#280243=CARTESIAN_POINT('Ctrl Pts',(-8.04997470400006,11.6,-7.66254598200002));
#280244=CARTESIAN_POINT('Ctrl Pts',(-8.05134666400006,15.2,-7.66551037400002));
#280245=CARTESIAN_POINT('Ctrl Pts',(-8.05134666400006,11.6,-7.66551037400002));
#280246=CARTESIAN_POINT('Ctrl Pts',(-8.05271836600006,15.2,-7.66848043600002));
#280247=CARTESIAN_POINT('Ctrl Pts',(-8.05271836600006,11.6,-7.66848043600002));
#280248=CARTESIAN_POINT('Ctrl Pts',(-8.05408980300006,15.2,-7.67145616100001));
#280249=CARTESIAN_POINT('Ctrl Pts',(-8.05408980300006,11.6,-7.67145616100001));
#280250=CARTESIAN_POINT('Ctrl Pts',(-8.05546096300005,15.2,-7.67443754500002));
#280251=CARTESIAN_POINT('Ctrl Pts',(-8.05546096300005,11.6,-7.67443754500002));
#280252=CARTESIAN_POINT('Ctrl Pts',(-8.05683183700006,15.2,-7.67742458300001));
#280253=CARTESIAN_POINT('Ctrl Pts',(-8.05683183700006,11.6,-7.67742458300001));
#280254=CARTESIAN_POINT('Ctrl Pts',(-8.05820241600006,15.2,-7.68041726900002));
#280255=CARTESIAN_POINT('Ctrl Pts',(-8.05820241600006,11.6,-7.68041726900002));
#280256=CARTESIAN_POINT('Ctrl Pts',(-8.05957268800006,15.2,-7.68341560100002));
#280257=CARTESIAN_POINT('Ctrl Pts',(-8.05957268800006,11.6,-7.68341560100002));
#280258=CARTESIAN_POINT('Ctrl Pts',(-8.06094264600006,15.2,-7.68641957000002));
#280259=CARTESIAN_POINT('Ctrl Pts',(-8.06094264600006,11.6,-7.68641957000002));
#280260=CARTESIAN_POINT('Ctrl Pts',(-8.06231227900006,15.2,-7.68942917500001));
#280261=CARTESIAN_POINT('Ctrl Pts',(-8.06231227900006,11.6,-7.68942917500001));
#280262=CARTESIAN_POINT('Ctrl Pts',(-8.06368157800006,15.2,-7.69244440900002));
#280263=CARTESIAN_POINT('Ctrl Pts',(-8.06368157800006,11.6,-7.69244440900002));
#280264=CARTESIAN_POINT('Ctrl Pts',(-8.06505053200006,15.2,-7.69546526700001));
#280265=CARTESIAN_POINT('Ctrl Pts',(-8.06505053200006,11.6,-7.69546526700001));
#280266=CARTESIAN_POINT('Ctrl Pts',(-8.06641913400006,15.2,-7.69849174400001));
#280267=CARTESIAN_POINT('Ctrl Pts',(-8.06641913400006,11.6,-7.69849174400001));
#280268=CARTESIAN_POINT('Ctrl Pts',(-8.06778737300006,15.2,-7.70152383700001));
#280269=CARTESIAN_POINT('Ctrl Pts',(-8.06778737300006,11.6,-7.70152383700001));
#280270=CARTESIAN_POINT('Ctrl Pts',(-8.06915523900006,15.2,-7.70456153800002));
#280271=CARTESIAN_POINT('Ctrl Pts',(-8.06915523900006,11.6,-7.70456153800002));
#280272=CARTESIAN_POINT('Ctrl Pts',(-8.07052272400006,15.2,-7.70760484600002));
#280273=CARTESIAN_POINT('Ctrl Pts',(-8.07052272400006,11.6,-7.70760484600002));
#280274=CARTESIAN_POINT('Ctrl Pts',(-8.07188981800006,15.2,-7.71065375300001));
#280275=CARTESIAN_POINT('Ctrl Pts',(-8.07188981800006,11.6,-7.71065375300001));
#280276=CARTESIAN_POINT('Ctrl Pts',(-8.07325651000006,15.2,-7.71370825500002));
#280277=CARTESIAN_POINT('Ctrl Pts',(-8.07325651000006,11.6,-7.71370825500002));
#280278=CARTESIAN_POINT('Ctrl Pts',(-8.07462279200006,15.2,-7.71676834700001));
#280279=CARTESIAN_POINT('Ctrl Pts',(-8.07462279200006,11.6,-7.71676834700001));
#280280=CARTESIAN_POINT('Ctrl Pts',(-8.07598865500006,15.2,-7.71983402500001));
#280281=CARTESIAN_POINT('Ctrl Pts',(-8.07598865500006,11.6,-7.71983402500001));
#280282=CARTESIAN_POINT('Ctrl Pts',(-8.07735408800006,15.2,-7.72290528300001));
#280283=CARTESIAN_POINT('Ctrl Pts',(-8.07735408800006,11.6,-7.72290528300001));
#280284=CARTESIAN_POINT('Ctrl Pts',(-8.07871908400006,15.2,-7.72598211700001));
#280285=CARTESIAN_POINT('Ctrl Pts',(-8.07871908400006,11.6,-7.72598211700001));
#280286=CARTESIAN_POINT('Ctrl Pts',(-8.08008363200006,15.2,-7.72906452200001));
#280287=CARTESIAN_POINT('Ctrl Pts',(-8.08008363200006,11.6,-7.72906452200001));
#280288=CARTESIAN_POINT('Ctrl Pts',(-8.08144772300006,15.2,-7.73215249200002));
#280289=CARTESIAN_POINT('Ctrl Pts',(-8.08144772300006,11.6,-7.73215249200002));
#280290=CARTESIAN_POINT('Ctrl Pts',(-8.08281134800006,15.2,-7.73524602300002));
#280291=CARTESIAN_POINT('Ctrl Pts',(-8.08281134800006,11.6,-7.73524602300002));
#280292=CARTESIAN_POINT('Ctrl Pts',(-8.08417449700006,15.2,-7.73834511200001));
#280293=CARTESIAN_POINT('Ctrl Pts',(-8.08417449700006,11.6,-7.73834511200001));
#280294=CARTESIAN_POINT('Ctrl Pts',(-8.08553716200005,15.2,-7.74144975000001));
#280295=CARTESIAN_POINT('Ctrl Pts',(-8.08553716200005,11.6,-7.74144975000001));
#280296=CARTESIAN_POINT('Ctrl Pts',(-8.08689933300006,15.2,-7.74455993500001));
#280297=CARTESIAN_POINT('Ctrl Pts',(-8.08689933300006,11.6,-7.74455993500001));
#280298=CARTESIAN_POINT('Ctrl Pts',(-8.08826100100006,15.2,-7.74767566300002));
#280299=CARTESIAN_POINT('Ctrl Pts',(-8.08826100100006,11.6,-7.74767566300002));
#280300=CARTESIAN_POINT('Ctrl Pts',(-8.08962215600006,15.2,-7.75079692600002));
#280301=CARTESIAN_POINT('Ctrl Pts',(-8.08962215600006,11.6,-7.75079692600002));
#280302=CARTESIAN_POINT('Ctrl Pts',(-8.09098279100006,15.2,-7.75392372200002));
#280303=CARTESIAN_POINT('Ctrl Pts',(-8.09098279100006,11.6,-7.75392372200002));
#280304=CARTESIAN_POINT('Ctrl Pts',(-8.09234289500005,15.2,-7.75705604400001));
#280305=CARTESIAN_POINT('Ctrl Pts',(-8.09234289500005,11.6,-7.75705604400001));
#280306=CARTESIAN_POINT('Ctrl Pts',(-8.09370246000006,15.2,-7.76019388800002));
#280307=CARTESIAN_POINT('Ctrl Pts',(-8.09370246000006,11.6,-7.76019388800002));
#280308=CARTESIAN_POINT('Ctrl Pts',(-8.09506147400005,15.2,-7.76333725000002));
#280309=CARTESIAN_POINT('Ctrl Pts',(-8.09506147400005,11.6,-7.76333725000002));
#280310=CARTESIAN_POINT('Ctrl Pts',(-8.09641993300006,15.2,-7.76648612400002));
#280311=CARTESIAN_POINT('Ctrl Pts',(-8.09641993300006,11.6,-7.76648612400002));
#280312=CARTESIAN_POINT('Ctrl Pts',(-8.09777782400005,15.2,-7.76964050600002));
#280313=CARTESIAN_POINT('Ctrl Pts',(-8.09777782400005,11.6,-7.76964050600002));
#280314=CARTESIAN_POINT('Ctrl Pts',(-8.09913513900005,15.2,-7.77280039000001));
#280315=CARTESIAN_POINT('Ctrl Pts',(-8.09913513900005,11.6,-7.77280039000001));
#280316=CARTESIAN_POINT('Ctrl Pts',(-8.10049186900006,15.2,-7.77596577200002));
#280317=CARTESIAN_POINT('Ctrl Pts',(-8.10049186900006,11.6,-7.77596577200002));
#280318=CARTESIAN_POINT('Ctrl Pts',(-8.10184800600006,15.2,-7.77913664800002));
#280319=CARTESIAN_POINT('Ctrl Pts',(-8.10184800600006,11.6,-7.77913664800002));
#280320=CARTESIAN_POINT('Ctrl Pts',(-8.10320354000006,15.2,-7.78231301200002));
#280321=CARTESIAN_POINT('Ctrl Pts',(-8.10320354000006,11.6,-7.78231301200002));
#280322=CARTESIAN_POINT('Ctrl Pts',(-8.10455846200006,15.2,-7.78549485800001));
#280323=CARTESIAN_POINT('Ctrl Pts',(-8.10455846200006,11.6,-7.78549485800001));
#280324=CARTESIAN_POINT('Ctrl Pts',(-8.10591276400006,15.2,-7.78868218400002));
#280325=CARTESIAN_POINT('Ctrl Pts',(-8.10591276400006,11.6,-7.78868218400002));
#280326=CARTESIAN_POINT('Ctrl Pts',(-8.10726643600006,15.2,-7.79187498200002));
#280327=CARTESIAN_POINT('Ctrl Pts',(-8.10726643600006,11.6,-7.79187498200002));
#280328=CARTESIAN_POINT('Ctrl Pts',(-8.10861947000006,15.2,-7.79507325000001));
#280329=CARTESIAN_POINT('Ctrl Pts',(-8.10861947000006,11.6,-7.79507325000001));
#280330=CARTESIAN_POINT('Ctrl Pts',(-8.10997185700005,15.2,-7.79827698300001));
#280331=CARTESIAN_POINT('Ctrl Pts',(-8.10997185700005,11.6,-7.79827698300001));
#280332=CARTESIAN_POINT('Ctrl Pts',(-8.11132358700006,15.2,-7.80148617400001));
#280333=CARTESIAN_POINT('Ctrl Pts',(-8.11132358700006,11.6,-7.80148617400001));
#280334=CARTESIAN_POINT('Ctrl Pts',(-8.11267465400006,15.2,-7.80470081900001));
#280335=CARTESIAN_POINT('Ctrl Pts',(-8.11267465400006,11.6,-7.80470081900001));
#280336=CARTESIAN_POINT('Ctrl Pts',(-8.11402504600006,15.2,-7.80792091400001));
#280337=CARTESIAN_POINT('Ctrl Pts',(-8.11402504600006,11.6,-7.80792091400001));
#280338=CARTESIAN_POINT('Ctrl Pts',(-8.11537475500005,15.2,-7.81114645400002));
#280339=CARTESIAN_POINT('Ctrl Pts',(-8.11537475500005,11.6,-7.81114645400002));
#280340=CARTESIAN_POINT('Ctrl Pts',(-8.11672377400006,15.2,-7.81437743400001));
#280341=CARTESIAN_POINT('Ctrl Pts',(-8.11672377400006,11.6,-7.81437743400001));
#280342=CARTESIAN_POINT('Ctrl Pts',(-8.11807209300006,15.2,-7.81761384900002));
#280343=CARTESIAN_POINT('Ctrl Pts',(-8.11807209300006,11.6,-7.81761384900002));
#280344=CARTESIAN_POINT('Ctrl Pts',(-8.11941970300006,15.2,-7.82085569400002));
#280345=CARTESIAN_POINT('Ctrl Pts',(-8.11941970300006,11.6,-7.82085569400002));
#280346=CARTESIAN_POINT('Ctrl Pts',(-8.12076659600006,15.2,-7.82410296400001));
#280347=CARTESIAN_POINT('Ctrl Pts',(-8.12076659600006,11.6,-7.82410296400001));
#280348=CARTESIAN_POINT('Ctrl Pts',(-8.12211276200006,15.2,-7.82735565500002));
#280349=CARTESIAN_POINT('Ctrl Pts',(-8.12211276200006,11.6,-7.82735565500002));
#280350=CARTESIAN_POINT('Ctrl Pts',(-8.12345819500005,15.2,-7.83061376200001));
#280351=CARTESIAN_POINT('Ctrl Pts',(-8.12345819500005,11.6,-7.83061376200001));
#280352=CARTESIAN_POINT('Ctrl Pts',(-8.12480288300006,15.2,-7.83387728000001));
#280353=CARTESIAN_POINT('Ctrl Pts',(-8.12480288300006,11.6,-7.83387728000001));
#280354=CARTESIAN_POINT('Ctrl Pts',(-8.12614682100006,15.2,-7.83714620400002));
#280355=CARTESIAN_POINT('Ctrl Pts',(-8.12614682100006,11.6,-7.83714620400002));
#280356=CARTESIAN_POINT('Ctrl Pts',(-8.12748999700006,15.2,-7.84042052900002));
#280357=CARTESIAN_POINT('Ctrl Pts',(-8.12748999700006,11.6,-7.84042052900002));
#280358=CARTESIAN_POINT('Ctrl Pts',(-8.12883240400006,15.2,-7.84370025200002));
#280359=CARTESIAN_POINT('Ctrl Pts',(-8.12883240400006,11.6,-7.84370025200002));
#280360=CARTESIAN_POINT('Ctrl Pts',(-8.13017403400006,15.2,-7.84698536500001));
#280361=CARTESIAN_POINT('Ctrl Pts',(-8.13017403400006,11.6,-7.84698536500001));
#280362=CARTESIAN_POINT('Ctrl Pts',(-8.13151487800006,15.2,-7.85027586600001));
#280363=CARTESIAN_POINT('Ctrl Pts',(-8.13151487800006,11.6,-7.85027586600001));
#280364=CARTESIAN_POINT('Ctrl Pts',(-8.13285492800006,15.2,-7.85357174900001));
#280365=CARTESIAN_POINT('Ctrl Pts',(-8.13285492800006,11.6,-7.85357174900001));
#280366=CARTESIAN_POINT('Ctrl Pts',(-8.13419417400005,15.2,-7.85687301000002));
#280367=CARTESIAN_POINT('Ctrl Pts',(-8.13419417400005,11.6,-7.85687301000002));
#280368=CARTESIAN_POINT('Ctrl Pts',(-8.13553260800006,15.2,-7.86017964300001));
#280369=CARTESIAN_POINT('Ctrl Pts',(-8.13553260800006,11.6,-7.86017964300001));
#280370=CARTESIAN_POINT('Ctrl Pts',(-8.13687022200006,15.2,-7.86349164400002));
#280371=CARTESIAN_POINT('Ctrl Pts',(-8.13687022200006,11.6,-7.86349164400002));
#280372=CARTESIAN_POINT('Ctrl Pts',(-8.13820700800006,15.2,-7.86680900800001));
#280373=CARTESIAN_POINT('Ctrl Pts',(-8.13820700800006,11.6,-7.86680900800001));
#280374=CARTESIAN_POINT('Ctrl Pts',(-8.13954295700006,15.2,-7.87013173000001));
#280375=CARTESIAN_POINT('Ctrl Pts',(-8.13954295700006,11.6,-7.87013173000001));
#280376=CARTESIAN_POINT('Ctrl Pts',(-8.14087806000006,15.2,-7.87345980500002));
#280377=CARTESIAN_POINT('Ctrl Pts',(-8.14087806000006,11.6,-7.87345980500002));
#280378=CARTESIAN_POINT('Ctrl Pts',(-8.14221230900005,15.2,-7.87679322900001));
#280379=CARTESIAN_POINT('Ctrl Pts',(-8.14221230900005,11.6,-7.87679322900001));
#280380=CARTESIAN_POINT('Ctrl Pts',(-8.14354569800006,15.2,-7.88013199700002));
#280381=CARTESIAN_POINT('Ctrl Pts',(-8.14354569800006,11.6,-7.88013199700002));
#280382=CARTESIAN_POINT('Ctrl Pts',(-8.14487821400006,15.2,-7.88347610400002));
#280383=CARTESIAN_POINT('Ctrl Pts',(-8.14487821400006,11.6,-7.88347610400002));
#280384=CARTESIAN_POINT('Ctrl Pts',(-8.14620985300006,15.2,-7.88682554500002));
#280385=CARTESIAN_POINT('Ctrl Pts',(-8.14620985300006,11.6,-7.88682554500002));
#280386=CARTESIAN_POINT('Ctrl Pts',(-8.14754060400006,15.2,-7.89018031600002));
#280387=CARTESIAN_POINT('Ctrl Pts',(-8.14754060400006,11.6,-7.89018031600002));
#280388=CARTESIAN_POINT('Ctrl Pts',(-8.14887046000005,15.2,-7.89354041100002));
#280389=CARTESIAN_POINT('Ctrl Pts',(-8.14887046000005,11.6,-7.89354041100002));
#280390=CARTESIAN_POINT('Ctrl Pts',(-8.15019941300006,15.2,-7.89690582600001));
#280391=CARTESIAN_POINT('Ctrl Pts',(-8.15019941300006,11.6,-7.89690582600001));
#280392=CARTESIAN_POINT('Ctrl Pts',(-8.15152745300006,15.2,-7.90027655700002));
#280393=CARTESIAN_POINT('Ctrl Pts',(-8.15152745300006,11.6,-7.90027655700002));
#280394=CARTESIAN_POINT('Ctrl Pts',(-8.15285457300006,15.2,-7.90365259800001));
#280395=CARTESIAN_POINT('Ctrl Pts',(-8.15285457300006,11.6,-7.90365259800001));
#280396=CARTESIAN_POINT('Ctrl Pts',(-8.15418076600006,15.2,-7.90703394400002));
#280397=CARTESIAN_POINT('Ctrl Pts',(-8.15418076600006,11.6,-7.90703394400002));
#280398=CARTESIAN_POINT('Ctrl Pts',(-8.15550602100006,15.2,-7.91042059200001));
#280399=CARTESIAN_POINT('Ctrl Pts',(-8.15550602100006,11.6,-7.91042059200001));
#280400=CARTESIAN_POINT('Ctrl Pts',(-8.15683033200006,15.2,-7.91381253500001));
#280401=CARTESIAN_POINT('Ctrl Pts',(-8.15683033200006,11.6,-7.91381253500001));
#280402=CARTESIAN_POINT('Ctrl Pts',(-8.15815368900006,15.2,-7.91720976900002));
#280403=CARTESIAN_POINT('Ctrl Pts',(-8.15815368900006,11.6,-7.91720976900002));
#280404=CARTESIAN_POINT('Ctrl Pts',(-8.15947608700006,15.2,-7.92061229100002));
#280405=CARTESIAN_POINT('Ctrl Pts',(-8.15947608700006,11.6,-7.92061229100002));
#280406=CARTESIAN_POINT('Ctrl Pts',(-8.16079751400006,15.2,-7.92402009500002));
#280407=CARTESIAN_POINT('Ctrl Pts',(-8.16079751400006,11.6,-7.92402009500002));
#280408=CARTESIAN_POINT('Ctrl Pts',(-8.16211796400006,15.2,-7.92743317400002));
#280409=CARTESIAN_POINT('Ctrl Pts',(-8.16211796400006,11.6,-7.92743317400002));
#280410=CARTESIAN_POINT('Ctrl Pts',(-8.16343743000006,15.2,-7.93085152700002));
#280411=CARTESIAN_POINT('Ctrl Pts',(-8.16343743000006,11.6,-7.93085152700002));
#280412=CARTESIAN_POINT('Ctrl Pts',(-8.16475590200006,15.2,-7.93427514600002));
#280413=CARTESIAN_POINT('Ctrl Pts',(-8.16475590200006,11.6,-7.93427514600002));
#280414=CARTESIAN_POINT('Ctrl Pts',(-8.16607337200006,15.2,-7.93770403000002));
#280415=CARTESIAN_POINT('Ctrl Pts',(-8.16607337200006,11.6,-7.93770403000002));
#280416=CARTESIAN_POINT('Ctrl Pts',(-8.16738983300005,15.2,-7.94113817000002));
#280417=CARTESIAN_POINT('Ctrl Pts',(-8.16738983300005,11.6,-7.94113817000002));
#280418=CARTESIAN_POINT('Ctrl Pts',(-8.16870527600006,15.2,-7.94457756400002));
#280419=CARTESIAN_POINT('Ctrl Pts',(-8.16870527600006,11.6,-7.94457756400002));
#280420=CARTESIAN_POINT('Ctrl Pts',(-8.17001969400006,15.2,-7.94802220500002));
#280421=CARTESIAN_POINT('Ctrl Pts',(-8.17001969400006,11.6,-7.94802220500002));
#280422=CARTESIAN_POINT('Ctrl Pts',(-8.17133307700006,15.2,-7.95147209200002));
#280423=CARTESIAN_POINT('Ctrl Pts',(-8.17133307700006,11.6,-7.95147209200002));
#280424=CARTESIAN_POINT('Ctrl Pts',(-8.17264542000006,15.2,-7.95492721600001));
#280425=CARTESIAN_POINT('Ctrl Pts',(-8.17264542000006,11.6,-7.95492721600001));
#280426=CARTESIAN_POINT('Ctrl Pts',(-8.17395671300006,15.2,-7.95838757500002));
#280427=CARTESIAN_POINT('Ctrl Pts',(-8.17395671300006,11.6,-7.95838757500002));
#280428=CARTESIAN_POINT('Ctrl Pts',(-8.17526694900006,15.2,-7.96185316300001));
#280429=CARTESIAN_POINT('Ctrl Pts',(-8.17526694900006,11.6,-7.96185316300001));
#280430=CARTESIAN_POINT('Ctrl Pts',(-8.17657612000006,15.2,-7.96532397700001));
#280431=CARTESIAN_POINT('Ctrl Pts',(-8.17657612000006,11.6,-7.96532397700001));
#280432=CARTESIAN_POINT('Ctrl Pts',(-8.17788421700006,15.2,-7.96880001000002));
#280433=CARTESIAN_POINT('Ctrl Pts',(-8.17788421700006,11.6,-7.96880001000002));
#280434=CARTESIAN_POINT('Ctrl Pts',(-8.17919123500005,15.2,-7.97228125900002));
#280435=CARTESIAN_POINT('Ctrl Pts',(-8.17919123500005,11.6,-7.97228125900002));
#280436=CARTESIAN_POINT('Ctrl Pts',(-8.18049716300006,15.2,-7.97576771900002));
#280437=CARTESIAN_POINT('Ctrl Pts',(-8.18049716300006,11.6,-7.97576771900002));
#280438=CARTESIAN_POINT('Ctrl Pts',(-8.18180199500006,15.2,-7.97925938400001));
#280439=CARTESIAN_POINT('Ctrl Pts',(-8.18180199500006,11.6,-7.97925938400001));
#280440=CARTESIAN_POINT('Ctrl Pts',(-8.18310572200006,15.2,-7.98275625000001));
#280441=CARTESIAN_POINT('Ctrl Pts',(-8.18310572200006,11.6,-7.98275625000001));
#280442=CARTESIAN_POINT('Ctrl Pts',(-8.18440833700006,15.2,-7.98625831200001));
#280443=CARTESIAN_POINT('Ctrl Pts',(-8.18440833700006,11.6,-7.98625831200001));
#280444=CARTESIAN_POINT('Ctrl Pts',(-8.18570982900006,15.2,-7.98976556500002));
#280445=CARTESIAN_POINT('Ctrl Pts',(-8.18570982900006,11.6,-7.98976556500002));
#280446=CARTESIAN_POINT('Ctrl Pts',(-8.18701019300006,15.2,-7.99327800400001));
#280447=CARTESIAN_POINT('Ctrl Pts',(-8.18701019300006,11.6,-7.99327800400001));
#280448=CARTESIAN_POINT('Ctrl Pts',(-8.18830942000006,15.2,-7.99679562500001));
#280449=CARTESIAN_POINT('Ctrl Pts',(-8.18830942000006,11.6,-7.99679562500001));
#280450=CARTESIAN_POINT('Ctrl Pts',(-8.18960750500005,15.2,-8.00031842400001));
#280451=CARTESIAN_POINT('Ctrl Pts',(-8.18960750500005,11.6,-8.00031842400001));
#280452=CARTESIAN_POINT('Ctrl Pts',(-8.19090444000006,15.2,-8.00384639600002));
#280453=CARTESIAN_POINT('Ctrl Pts',(-8.19090444000006,11.6,-8.00384639600002));
#280454=CARTESIAN_POINT('Ctrl Pts',(-8.19220021800006,15.2,-8.00737953800001));
#280455=CARTESIAN_POINT('Ctrl Pts',(-8.19220021800006,11.6,-8.00737953800001));
#280456=CARTESIAN_POINT('Ctrl Pts',(-8.19349483100006,15.2,-8.01091784200001));
#280457=CARTESIAN_POINT('Ctrl Pts',(-8.19349483100006,11.6,-8.01091784200001));
#280458=CARTESIAN_POINT('Ctrl Pts',(-8.19478827300006,15.2,-8.01446130700001));
#280459=CARTESIAN_POINT('Ctrl Pts',(-8.19478827300006,11.6,-8.01446130700001));
#280460=CARTESIAN_POINT('Ctrl Pts',(-8.19608053200006,15.2,-8.01800992700001));
#280461=CARTESIAN_POINT('Ctrl Pts',(-8.19608053200006,11.6,-8.01800992700001));
#280462=CARTESIAN_POINT('Ctrl Pts',(-8.19737160100006,15.2,-8.02156369400001));
#280463=CARTESIAN_POINT('Ctrl Pts',(-8.19737160100006,11.6,-8.02156369400001));
#280464=CARTESIAN_POINT('Ctrl Pts',(-8.19866147000005,15.2,-8.02512260400002));
#280465=CARTESIAN_POINT('Ctrl Pts',(-8.19866147000005,11.6,-8.02512260400002));
#280466=CARTESIAN_POINT('Ctrl Pts',(-8.19995012900005,15.2,-8.02868665000002));
#280467=CARTESIAN_POINT('Ctrl Pts',(-8.19995012900005,11.6,-8.02868665000002));
#280468=CARTESIAN_POINT('Ctrl Pts',(-8.20123757100006,15.2,-8.03225582900001));
#280469=CARTESIAN_POINT('Ctrl Pts',(-8.20123757100006,11.6,-8.03225582900001));
#280470=CARTESIAN_POINT('Ctrl Pts',(-8.20252378800006,15.2,-8.03583013400001));
#280471=CARTESIAN_POINT('Ctrl Pts',(-8.20252378800006,11.6,-8.03583013400001));
#280472=CARTESIAN_POINT('Ctrl Pts',(-8.20380877600006,15.2,-8.03940956400002));
#280473=CARTESIAN_POINT('Ctrl Pts',(-8.20380877600006,11.6,-8.03940956400002));
#280474=CARTESIAN_POINT('Ctrl Pts',(-8.20509253000006,15.2,-8.04299411600002));
#280475=CARTESIAN_POINT('Ctrl Pts',(-8.20509253000006,11.6,-8.04299411600002));
#280476=CARTESIAN_POINT('Ctrl Pts',(-8.20637504900006,15.2,-8.04658378800001));
#280477=CARTESIAN_POINT('Ctrl Pts',(-8.20637504900006,11.6,-8.04658378800001));
#280478=CARTESIAN_POINT('Ctrl Pts',(-8.20740007500006,15.2,-8.04945962200001));
#280479=CARTESIAN_POINT('Ctrl Pts',(-8.20740007500006,11.6,-8.04945962200001));
#280480=CARTESIAN_POINT('Ctrl Pts',(-8.20816828900006,15.2,-8.05161880000002));
#280481=CARTESIAN_POINT('Ctrl Pts',(-8.20816828900006,11.6,-8.05161880000002));
#280482=CARTESIAN_POINT('Ctrl Pts',(-8.20868018400006,15.2,-8.05305927700001));
#280483=CARTESIAN_POINT('Ctrl Pts',(-8.20868018400006,11.6,-8.05305927700001));
#280484=CARTESIAN_POINT('Ctrl Pts',(-8.20893607000006,15.2,-8.05377977100001));
#280485=CARTESIAN_POINT('Ctrl Pts',(-8.20893607000006,11.6,-8.05377977100001));
#280486=CARTESIAN_POINT('Ctrl Pts',(-7.64657512400006,15.2,-7.01216898700002));
#280487=CARTESIAN_POINT('Ctrl Pts',(-7.64778328679899,15.2,-7.01348522587027));
#280488=CARTESIAN_POINT('Ctrl Pts',(-7.64902613388113,15.2,-7.01484722203433));
#280489=CARTESIAN_POINT('Ctrl Pts',(-7.65030255133521,15.2,-7.01625467938746));
#280490=CARTESIAN_POINT('Ctrl Pts',(-7.65158512431943,15.2,-7.01766892421138));
#280491=CARTESIAN_POINT('Ctrl Pts',(-7.65290158882944,15.2,-7.01912907735244));
#280492=CARTESIAN_POINT('Ctrl Pts',(-7.65425083088893,15.2,-7.02063486217904));
#280493=CARTESIAN_POINT('Ctrl Pts',(-7.65560007282589,15.2,-7.02214064686888));
#280494=CARTESIAN_POINT('Ctrl Pts',(-7.6569820926347,15.2,-7.02369206393294));
#280495=CARTESIAN_POINT('Ctrl Pts',(-7.65839581074999,15.2,-7.02528884179159));
#280496=CARTESIAN_POINT('Ctrl Pts',(-7.65980952886529,15.2,-7.02688561965024));
#280497=CARTESIAN_POINT('Ctrl Pts',(-7.66125494568895,15.1999999999999,
-7.02852776104979));
#280498=CARTESIAN_POINT('Ctrl Pts',(-7.66273101487395,15.2,-7.03021499707016));
#280499=CARTESIAN_POINT('Ctrl Pts',(-7.66420708419303,15.2,-7.03190223324379));
#280500=CARTESIAN_POINT('Ctrl Pts',(-7.66571380278172,15.2,-7.03363456758543));
#280501=CARTESIAN_POINT('Ctrl Pts',(-7.66725015536747,15.2,-7.03541173743532));
#280502=CARTESIAN_POINT('Ctrl Pts',(-7.66878650781365,15.2,-7.03718890712378));
#280503=CARTESIAN_POINT('Ctrl Pts',(-7.67035249574304,15.2,-7.03901091194339));
#280504=CARTESIAN_POINT('Ctrl Pts',(-7.67194712427573,15.2,-7.04087749571745));
#280505=CARTESIAN_POINT('Ctrl Pts',(-7.67354175280843,15.2,-7.04274407949153));
#280506=CARTESIAN_POINT('Ctrl Pts',(-7.67516502602135,15.2,-7.04465524296655));
#280507=CARTESIAN_POINT('Ctrl Pts',(-7.67681598062681,15.2,-7.04661073189355));
#280508=CARTESIAN_POINT('Ctrl Pts',(-7.67846693538224,15.2,-7.04856622099817));
#280509=CARTESIAN_POINT('Ctrl Pts',(-7.68014557084944,15.2,-7.05056603617498));
#280510=CARTESIAN_POINT('Ctrl Pts',(-7.68185095069424,15.2,-7.05260992995607));
#280511=CARTESIAN_POINT('Ctrl Pts',(-7.68355633038413,15.2,-7.05465382355151));
#280512=CARTESIAN_POINT('Ctrl Pts',(-7.68528845682534,15.2,-7.05674179384187));
#280513=CARTESIAN_POINT('Ctrl Pts',(-7.68704641459593,15.2,-7.05887359659964));
#280514=CARTESIAN_POINT('Ctrl Pts',(-7.68880437236652,15.2,-7.06100539935743));
#280515=CARTESIAN_POINT('Ctrl Pts',(-7.69058816346834,15.2,-7.06318103452004));
#280516=CARTESIAN_POINT('Ctrl Pts',(-7.69239689940154,15.2,-7.06540025935418));
#280517=CARTESIAN_POINT('Ctrl Pts',(-7.69420563533474,15.2,-7.06761948418832));
#280518=CARTESIAN_POINT('Ctrl Pts',(-7.69603931658333,15.2,-7.06988230103532));
#280519=CARTESIAN_POINT('Ctrl Pts',(-7.69789707751419,15.2,-7.07218846778191));
#280520=CARTESIAN_POINT('Ctrl Pts',(-7.6997548386138,15.2,-7.07449463473798));
#280521=CARTESIAN_POINT('Ctrl Pts',(-7.7016366791741,15.2,-7.07684415463993));
#280522=CARTESIAN_POINT('Ctrl Pts',(-7.70354175636227,15.2,-7.07923678885552));
#280523=CARTESIAN_POINT('Ctrl Pts',(-7.70544683337737,15.2,-7.08162942285377));
#280524=CARTESIAN_POINT('Ctrl Pts',(-7.70737514672789,15.2,-7.08406517436941));
#280525=CARTESIAN_POINT('Ctrl Pts',(-7.70932587299913,15.2,-7.08654380820715));
#280526=CARTESIAN_POINT('Ctrl Pts',(-7.71127659927036,15.2,-7.08902244204489));
#280527=CARTESIAN_POINT('Ctrl Pts',(-7.71324973925656,15.2,-7.09154395937487));
#280528=CARTESIAN_POINT('Ctrl Pts',(-7.71524449051593,15.2,-7.09410813019545));
#280529=CARTESIAN_POINT('Ctrl Pts',(-7.71723924195649,15.2,-7.09667230124895));
#280530=CARTESIAN_POINT('Ctrl Pts',(-7.71925560443252,15.2,-7.09927912477326));
#280531=CARTESIAN_POINT('Ctrl Pts',(-7.7212927938778,15.2,-7.10192837566951));
#280532=CARTESIAN_POINT('Ctrl Pts',(-7.72332998313804,15.2,-7.10457762632511));
#280533=CARTESIAN_POINT('Ctrl Pts',(-7.72538800039852,15.2,-7.10726930092739));
#280534=CARTESIAN_POINT('Ctrl Pts',(-7.72746607899908,15.2,-7.1100031779237));
#280535=CARTESIAN_POINT('Ctrl Pts',(-7.72954415759964,15.2,-7.11273705492003));
#280536=CARTESIAN_POINT('Ctrl Pts',(-7.73164230023916,15.2,-7.11551313281472));
#280537=CARTESIAN_POINT('Ctrl Pts',(-7.73375975674422,15.2,-7.11833118970945));
#280538=CARTESIAN_POINT('Ctrl Pts',(-7.73587721344161,15.2,-7.12114924686015));
#280539=CARTESIAN_POINT('Ctrl Pts',(-7.73801398519903,15.2,-7.12400928335858));
#280540=CARTESIAN_POINT('Ctrl Pts',(-7.74016934292524,15.2,-7.12691107683075));
#280541=CARTESIAN_POINT('Ctrl Pts',(-7.74232470045566,15.2,-7.12981287003936));
#280542=CARTESIAN_POINT('Ctrl Pts',(-7.74449864221298,15.2,-7.13275642378339));
#280543=CARTESIAN_POINT('Ctrl Pts',(-7.74669045496669,15.2,-7.13574151575828));
#280544=CARTESIAN_POINT('Ctrl Pts',(-7.74888226772041,15.2,-7.13872660773317));
#280545=CARTESIAN_POINT('Ctrl Pts',(-7.751091952672,15.2,-7.14175324162221));
#280546=CARTESIAN_POINT('Ctrl Pts',(-7.75331881053465,15.2,-7.14482119791159));
#280547=CARTESIAN_POINT('Ctrl Pts',(-7.75554566859958,15.2,-7.14788915447964));
#280548=CARTESIAN_POINT('Ctrl Pts',(-7.75778970044714,15.2,-7.15099843786054));
#280549=CARTESIAN_POINT('Ctrl Pts',(-7.76005022248809,15.2,-7.15414883011834));
#280550=CARTESIAN_POINT('Ctrl Pts',(-7.76231074432373,15.2,-7.15729922208999));
#280551=CARTESIAN_POINT('Ctrl Pts',(-7.76458775655725,15.2,-7.16049072517074));
#280552=CARTESIAN_POINT('Ctrl Pts',(-7.76688059148441,15.2,-7.16372312523475));
#280553=CARTESIAN_POINT('Ctrl Pts',(-7.76917342641157,15.2,-7.16695552529877));
#280554=CARTESIAN_POINT('Ctrl Pts',(-7.77148208440855,15.2,-7.17022882502503));
#280555=CARTESIAN_POINT('Ctrl Pts',(-7.77380591132344,15.2,-7.1735428110695));
#280556=CARTESIAN_POINT('Ctrl Pts',(-7.77574243382289,15.2,-7.1763044662069));
#280557=CARTESIAN_POINT('Ctrl Pts',(-7.77768949117817,15.2,-7.17909437651173));
#280558=CARTESIAN_POINT('Ctrl Pts',(-7.77964671041376,15.2,-7.18191242227416));
#280559=CARTESIAN_POINT('Ctrl Pts',(-7.78160392964934,15.2,-7.18473046803657));
#280560=CARTESIAN_POINT('Ctrl Pts',(-7.78357131294,15.2,-7.18757664781318));
#280561=CARTESIAN_POINT('Ctrl Pts',(-7.78554849399062,15.2,-7.19045084275672));
#280562=CARTESIAN_POINT('Ctrl Pts',(-7.78752567504124,15.2,-7.19332503770024));
#280563=CARTESIAN_POINT('Ctrl Pts',(-7.78951265463893,15.2,-7.19622724628885));
#280564=CARTESIAN_POINT('Ctrl Pts',(-7.79150907470837,15.2,-7.19915735052494));
#280565=CARTESIAN_POINT('Ctrl Pts',(-7.79350549477779,15.2,-7.20208745476103));
#280566=CARTESIAN_POINT('Ctrl Pts',(-7.79551135383639,15.2,-7.2050454544546));
#280567=CARTESIAN_POINT('Ctrl Pts',(-7.79752630148447,15.2,-7.20803123050991));
#280568=CARTESIAN_POINT('Ctrl Pts',(-7.79954124913253,15.2,-7.21101700656521));
#280569=CARTESIAN_POINT('Ctrl Pts',(-7.80156528368813,15.2,-7.21403056018646));
#280570=CARTESIAN_POINT('Ctrl Pts',(-7.80359806042469,15.2,-7.21707177192401));
#280571=CARTESIAN_POINT('Ctrl Pts',(-7.80563083716125,15.2,-7.22011298366154));
#280572=CARTESIAN_POINT('Ctrl Pts',(-7.80767235392262,15.2,-7.2231818550512));
#280573=CARTESIAN_POINT('Ctrl Pts',(-7.80972227170081,15.2,-7.22627826692762));
#280574=CARTESIAN_POINT('Ctrl Pts',(-7.81177218947903,15.2,-7.22937467880403));
#280575=CARTESIAN_POINT('Ctrl Pts',(-7.81383050736948,15.2,-7.23249863307319));
#280576=CARTESIAN_POINT('Ctrl Pts',(-7.81589689101494,15.2,-7.23565001385754));
#280577=CARTESIAN_POINT('Ctrl Pts',(-7.81796327466039,15.2,-7.23880139464188));
#280578=CARTESIAN_POINT('Ctrl Pts',(-7.8200377222773,15.2,-7.24198019922819));
#280579=CARTESIAN_POINT('Ctrl Pts',(-7.82211990672239,15.2,-7.24518631270265));
#280580=CARTESIAN_POINT('Ctrl Pts',(-7.82420209116748,15.2,-7.24839242617711));
#280581=CARTESIAN_POINT('Ctrl Pts',(-7.826292010146,15.2,-7.251625849902));
#280582=CARTESIAN_POINT('Ctrl Pts',(-7.82838933979937,15.2,-7.25488646816811));
#280583=CARTESIAN_POINT('Ctrl Pts',(-7.83048666922415,15.2,-7.25814708607882));
#280584=CARTESIAN_POINT('Ctrl Pts',(-7.83259141104903,15.2,-7.26143489747436));
#280585=CARTESIAN_POINT('Ctrl Pts',(-7.83470324366548,15.2,-7.26474978954136));
#280586=CARTESIAN_POINT('Ctrl Pts',(-7.8368150765121,15.2,-7.26806468196968));
#280587=CARTESIAN_POINT('Ctrl Pts',(-7.83893400051145,15.2,-7.27140665157262));
#280588=CARTESIAN_POINT('Ctrl Pts',(-7.84105970245533,15.2,-7.27477558900096));
#280589=CARTESIAN_POINT('Ctrl Pts',(-7.84318540439921,15.2,-7.2781445264293));
#280590=CARTESIAN_POINT('Ctrl Pts',(-7.84531788327079,15.2,-7.28154042926555));
#280591=CARTESIAN_POINT('Ctrl Pts',(-7.8474568297286,15.2,-7.28496318356893));
#280592=CARTESIAN_POINT('Ctrl Pts',(-7.84959577618641,15.2,-7.2883859378723));
#280593=CARTESIAN_POINT('Ctrl Pts',(-7.85174119063211,15.2,-7.29183554548579));
#280594=CARTESIAN_POINT('Ctrl Pts',(-7.8538927687253,15.2,-7.29531189162982));
#280595=CARTESIAN_POINT('Ctrl Pts',(-7.85647466257781,15.2,-7.29948350723001));
#280596=CARTESIAN_POINT('Ctrl Pts',(-7.85906542972445,15.2,-7.30369362700386));
#280597=CARTESIAN_POINT('Ctrl Pts',(-7.86166455453335,15.2,-7.30794205648804));
#280598=CARTESIAN_POINT('Ctrl Pts',(-7.86339730416987,15.2,-7.31077434242493));
#280599=CARTESIAN_POINT('Ctrl Pts',(-7.86513376794754,15.2,-7.31362365599012));
#280600=CARTESIAN_POINT('Ctrl Pts',(-7.86687379608283,15.2,-7.31648993853246));
#280601=CARTESIAN_POINT('Ctrl Pts',(-7.8686138244552,15.2,-7.31935622146532));
#280602=CARTESIAN_POINT('Ctrl Pts',(-7.87035741474857,15.2,-7.32223947390259));
#280603=CARTESIAN_POINT('Ctrl Pts',(-7.8721044194869,15.2,-7.32513963892921));
#280604=CARTESIAN_POINT('Ctrl Pts',(-7.8742881752908,15.2,-7.32876484501491));
#280605=CARTESIAN_POINT('Ctrl Pts',(-7.87647726583108,15.2,-7.33241647642887));
#280606=CARTESIAN_POINT('Ctrl Pts',(-7.8786714030537,15.2,-7.3360944224727));
#280607=CARTESIAN_POINT('Ctrl Pts',(-7.88042671268832,15.2,-7.33903677906723));
#280608=CARTESIAN_POINT('Ctrl Pts',(-7.88218525180583,15.2,-7.34199597845954));
#280609=CARTESIAN_POINT('Ctrl Pts',(-7.88394687610606,15.2,-7.34497196104849));
#280610=CARTESIAN_POINT('Ctrl Pts',(-7.88570850064631,15.2,-7.34794794404292));
#280611=CARTESIAN_POINT('Ctrl Pts',(-7.88747320981608,15.2,-7.35094071248756));
#280612=CARTESIAN_POINT('Ctrl Pts',(-7.88924085922323,15.2,-7.35395020947007));
#280613=CARTESIAN_POINT('Ctrl Pts',(-7.89100850838952,15.2,-7.35695970604254));
#280614=CARTESIAN_POINT('Ctrl Pts',(-7.89277909937803,15.2,-7.3599859298373));
#280615=CARTESIAN_POINT('Ctrl Pts',(-7.89455248912176,15.2,-7.36302882630968));
#280616=CARTESIAN_POINT('Ctrl Pts',(-7.89632587910712,15.2,-7.36607172319666));
#280617=CARTESIAN_POINT('Ctrl Pts',(-7.89810206675392,15.2,-7.36913129149951));
#280618=CARTESIAN_POINT('Ctrl Pts',(-7.89988091462883,15.2,-7.37220747700159));
#280619=CARTESIAN_POINT('Ctrl Pts',(-7.90165976226136,15.2,-7.37528366208454));
#280620=CARTESIAN_POINT('Ctrl Pts',(-7.9034412671759,15.2,-7.37837646237136));
#280621=CARTESIAN_POINT('Ctrl Pts',(-7.90522529300786,15.2,-7.38148582304886));
#280622=CARTESIAN_POINT('Ctrl Pts',(-7.90700931908289,15.2,-7.38459518415));
#280623=CARTESIAN_POINT('Ctrl Pts',(-7.90879586575977,15.2,-7.38772110534022));
#280624=CARTESIAN_POINT('Ctrl Pts',(-7.91058479441298,15.2,-7.39086353029033));
#280625=CARTESIAN_POINT('Ctrl Pts',(-7.91237372282244,15.2,-7.39400595481229));
#280626=CARTESIAN_POINT('Ctrl Pts',(-7.91416503376754,15.2,-7.39716488463093));
#280627=CARTESIAN_POINT('Ctrl Pts',(-7.9159585922318,15.2,-7.40034026248078));
#280628=CARTESIAN_POINT('Ctrl Pts',(-7.91820054049541,15.2,-7.40430948511758));
#280629=CARTESIAN_POINT('Ctrl Pts',(-7.92044600027689,15.2,-7.40830440833977));
#280630=CARTESIAN_POINT('Ctrl Pts',(-7.92269470872235,15.2,-7.41232492527499));
#280631=CARTESIAN_POINT('Ctrl Pts',(-7.92449367557676,15.2,-7.41554133899845));
#280632=CARTESIAN_POINT('Ctrl Pts',(-7.92629472267131,15.2,-7.41877413202094));
#280633=CARTESIAN_POINT('Ctrl Pts',(-7.92809771688079,15.2,-7.42202324953238));
#280634=CARTESIAN_POINT('Ctrl Pts',(-7.92990071084462,15.2,-7.42527236660113));
#280635=CARTESIAN_POINT('Ctrl Pts',(-7.93170565234697,15.2,-7.42853780720556));
#280636=CARTESIAN_POINT('Ctrl Pts',(-7.93351241142132,15.2,-7.43181951771341));
#280637=CARTESIAN_POINT('Ctrl Pts',(-7.93531917074182,15.2,-7.43510122866839));
#280638=CARTESIAN_POINT('Ctrl Pts',(-7.93712774630829,15.2,-7.43839920875926));
#280639=CARTESIAN_POINT('Ctrl Pts',(-7.93893800902628,15.2,-7.44171340301054));
#280640=CARTESIAN_POINT('Ctrl Pts',(-7.94074827149763,15.2,-7.44502759681028));
#280641=CARTESIAN_POINT('Ctrl Pts',(-7.94256022203805,15.2,-7.44835800521968));
#280642=CARTESIAN_POINT('Ctrl Pts',(-7.94437373194521,15.2,-7.45170457244446));
#280643=CARTESIAN_POINT('Ctrl Pts',(-7.94618724209945,15.2,-7.45505114012521));
#280644=CARTESIAN_POINT('Ctrl Pts',(-7.9480023113316,15.2,-7.45841386751856));
#280645=CARTESIAN_POINT('Ctrl Pts',(-7.94981881404171,15.2,-7.46179269975828));
#280646=CARTESIAN_POINT('Ctrl Pts',(-7.95163531675183,15.2,-7.46517153199799));
#280647=CARTESIAN_POINT('Ctrl Pts',(-7.95345325198433,15.2,-7.46856646932567));
#280648=CARTESIAN_POINT('Ctrl Pts',(-7.95527249480583,15.2,-7.47197745629099));
#280649=CARTESIAN_POINT('Ctrl Pts',(-7.95709173737946,15.2,-7.47538844279156));
#280650=CARTESIAN_POINT('Ctrl Pts',(-7.95891228836167,15.2,-7.4788154805357));
#280651=CARTESIAN_POINT('Ctrl Pts',(-7.96073402299881,15.2,-7.48225851371428));
#280652=CARTESIAN_POINT('Ctrl Pts',(-7.96301119148139,15.2,-7.48656230553934));
#280653=CARTESIAN_POINT('Ctrl Pts',(-7.96529020949449,15.2,-7.49089109085549));
#280654=CARTESIAN_POINT('Ctrl Pts',(-7.96757083796672,15.2,-7.49524476425828));
#280655=CARTESIAN_POINT('Ctrl Pts',(-7.96939534084394,15.2,-7.49872770317033));
#280656=CARTESIAN_POINT('Ctrl Pts',(-7.97122087557127,15.2,-7.50222656891201));
#280657=CARTESIAN_POINT('Ctrl Pts',(-7.97304731978201,15.2,-7.50574131104962));
#280658=CARTESIAN_POINT('Ctrl Pts',(-7.97487376374389,15.2,-7.50925605270834));
#280659=CARTESIAN_POINT('Ctrl Pts',(-7.97670111765941,15.2,-7.51278666767974));
#280660=CARTESIAN_POINT('Ctrl Pts',(-7.97852926224048,15.2,-7.51633310223921));
#280661=CARTESIAN_POINT('Ctrl Pts',(-7.98035740707063,15.2,-7.51987953728188));
#280662=CARTESIAN_POINT('Ctrl Pts',(-7.98218634148551,15.2,-7.52344179445225));
#280663=CARTESIAN_POINT('Ctrl Pts',(-7.98401594830752,15.2,-7.5270198155933));
#280664=CARTESIAN_POINT('Ctrl Pts',(-7.98584555488024,15.2,-7.53059783624684));
#280665=CARTESIAN_POINT('Ctrl Pts',(-7.98767583300565,15.2,-7.53419162483724));
#280666=CARTESIAN_POINT('Ctrl Pts',(-7.98950666630039,15.2,-7.53780112593003));
#280667=CARTESIAN_POINT('Ctrl Pts',(-7.99133749984458,15.2,-7.54141062751461));
#280668=CARTESIAN_POINT('Ctrl Pts',(-7.99316888828883,15.2,-7.54503584132052));
#280669=CARTESIAN_POINT('Ctrl Pts',(-7.99500071516648,15.2,-7.54867671429774));
#280670=CARTESIAN_POINT('Ctrl Pts',(-7.99683254179453,15.2,-7.5523175867789));
#280671=CARTESIAN_POINT('Ctrl Pts',(-7.99866480678408,15.2,-7.55597411753806));
#280672=CARTESIAN_POINT('Ctrl Pts',(-8.00049739622581,15.2,-7.55964625547553));
#280673=CARTESIAN_POINT('Ctrl Pts',(-8.00232998591722,15.2,-7.56331839391334));
#280674=CARTESIAN_POINT('Ctrl Pts',(-8.00416290063055,15.2,-7.56700613667224));
#280675=CARTESIAN_POINT('Ctrl Pts',(-8.00599602367491,15.2,-7.57070943231951));
#280676=CARTESIAN_POINT('Ctrl Pts',(-8.00782914646951,15.2,-7.57441272746221));
#280677=CARTESIAN_POINT('Ctrl Pts',(-8.00966248152796,15.2,-7.57813157536295));
#280678=CARTESIAN_POINT('Ctrl Pts',(-8.01149591293363,15.2,-7.5818659223894));
#280679=CARTESIAN_POINT('Ctrl Pts',(-8.01332934458909,15.2,-7.58560026992465));
#280680=CARTESIAN_POINT('Ctrl Pts',(-8.01516287429861,15.2,-7.58935011545238));
#280681=CARTESIAN_POINT('Ctrl Pts',(-8.01699639051797,15.2,-7.59311540778586));
#280682=CARTESIAN_POINT('Ctrl Pts',(-8.01882990648751,15.2,-7.59688069960631));
#280683=CARTESIAN_POINT('Ctrl Pts',(-8.02066340849183,15.2,-7.60066143731065));
#280684=CARTESIAN_POINT('Ctrl Pts',(-8.0224967871753,15.2,-7.60445756838763));
#280685=CARTESIAN_POINT('Ctrl Pts',(-8.02433016610857,15.2,-7.60825369998183));
#280686=CARTESIAN_POINT('Ctrl Pts',(-8.02616342168349,15.2,-7.6120652229775));
#280687=CARTESIAN_POINT('Ctrl Pts',(-8.02799644278339,15.2,-7.61589208724161));
#280688=CARTESIAN_POINT('Ctrl Pts',(-8.02982946388329,15.2,-7.61971895150572));
#280689=CARTESIAN_POINT('Ctrl Pts',(-8.0316622529776,15.2,-7.62356115500774));
#280690=CARTESIAN_POINT('Ctrl Pts',(-8.03349470129966,15.2,-7.627418646664));
#280691=CARTESIAN_POINT('Ctrl Pts',(-8.03532714937206,15.2,-7.63127613779468));
#280692=CARTESIAN_POINT('Ctrl Pts',(-8.03715925531522,15.2,-7.63514891677531));
#280693=CARTESIAN_POINT('Ctrl Pts',(-8.03899091400714,15.2,-7.6390369286973));
#280694=CARTESIAN_POINT('Ctrl Pts',(-8.04082257294861,15.2,-7.64292494114903));
#280695=CARTESIAN_POINT('Ctrl Pts',(-8.04265378397744,15.2,-7.64682818924774));
#280696=CARTESIAN_POINT('Ctrl Pts',(-8.04448444029937,15.2,-7.65074661890729));
#280697=CARTESIAN_POINT('Ctrl Pts',(-8.04631509637188,15.2,-7.65466504803296));
#280698=CARTESIAN_POINT('Ctrl Pts',(-8.04814519867778,15.2,-7.65859866004553));
#280699=CARTESIAN_POINT('Ctrl Pts',(-8.04997464208383,15.2,-7.66254739994396));
#280700=CARTESIAN_POINT('Ctrl Pts',(-8.05180408573913,15.2,-7.6664961403804));
#280701=CARTESIAN_POINT('Ctrl Pts',(-8.05363286990777,15.2,-7.67046001126325));
#280702=CARTESIAN_POINT('Ctrl Pts',(-8.05546089176531,15.2,-7.67443895906907));
#280703=CARTESIAN_POINT('Ctrl Pts',(-8.0577459189627,15.2,-7.67941264355528));
#280704=CARTESIAN_POINT('Ctrl Pts',(-8.06002975383759,15.2,-7.68440988458806));
#280705=CARTESIAN_POINT('Ctrl Pts',(-8.06231219578194,15.2,-7.68943058292334));
#280706=CARTESIAN_POINT('Ctrl Pts',(-8.06459463772628,15.2,-7.69445128125862));
#280707=CARTESIAN_POINT('Ctrl Pts',(-8.06687568611503,15.2,-7.69949543347758));
#280708=CARTESIAN_POINT('Ctrl Pts',(-8.06915514403155,15.2,-7.70456294035446));
#280709=CARTESIAN_POINT('Ctrl Pts',(-8.07052281873177,15.2,-7.70760344437012));
#280710=CARTESIAN_POINT('Ctrl Pts',(-8.07188992144589,15.2,-7.71065235643226));
#280711=CARTESIAN_POINT('Ctrl Pts',(-8.0732564077561,15.2,-7.71370965309988));
#280712=CARTESIAN_POINT('Ctrl Pts',(-8.07462289406632,15.2,-7.71676694976752));
#280713=CARTESIAN_POINT('Ctrl Pts',(-8.07598876516518,15.2,-7.71983263181279));
#280714=CARTESIAN_POINT('Ctrl Pts',(-8.07735397886553,15.2,-7.72290667732684));
#280715=CARTESIAN_POINT('Ctrl Pts',(-8.07871919256587,15.2,-7.72598072284089));
#280716=CARTESIAN_POINT('Ctrl Pts',(-8.08008374933296,15.2,-7.72906313216229));
#280717=CARTESIAN_POINT('Ctrl Pts',(-8.08144760649173,15.2,-7.73215388225828));
#280718=CARTESIAN_POINT('Ctrl Pts',(-8.08281146365049,15.2,-7.73524463235428));
#280719=CARTESIAN_POINT('Ctrl Pts',(-8.08417462120098,15.2,-7.73834372525835));
#280720=CARTESIAN_POINT('Ctrl Pts',(-8.08553703835988,15.2,-7.74145113639472));
#280721=CARTESIAN_POINT('Ctrl Pts',(-8.08689945551878,15.2,-7.7445585475311));
#280722=CARTESIAN_POINT('Ctrl Pts',(-8.08826113143478,15.2,-7.74767427943733));
#280723=CARTESIAN_POINT('Ctrl Pts',(-8.08962202570342,15.2,-7.75079830860395));
#280724=CARTESIAN_POINT('Ctrl Pts',(-8.09098291997206,15.2,-7.75392233777057));
#280725=CARTESIAN_POINT('Ctrl Pts',(-8.09234303323634,15.2,-7.75705466433054));
#280726=CARTESIAN_POINT('Ctrl Pts',(-8.09370232202041,15.2,-7.76019526679865));
#280727=CARTESIAN_POINT('Ctrl Pts',(-8.09506161105141,15.2,-7.76333586983731));
#280728=CARTESIAN_POINT('Ctrl Pts',(-8.09642007779883,15.2,-7.7664847491616));
#280729=CARTESIAN_POINT('Ctrl Pts',(-8.09777768028768,15.2,-7.76964188220488));
#280730=CARTESIAN_POINT('Ctrl Pts',(-8.09913528252989,15.2,-7.77279901467461));
#280731=CARTESIAN_POINT('Ctrl Pts',(-8.10049202074717,15.2,-7.77596440096061));
#280732=CARTESIAN_POINT('Ctrl Pts',(-8.10184785540617,15.2,-7.77913802034602));
#280733=CARTESIAN_POINT('Ctrl Pts',(-8.10320369006516,15.2,-7.78231163973143));
#280734=CARTESIAN_POINT('Ctrl Pts',(-8.10455862031101,15.2,-7.7854934905709));
#280735=CARTESIAN_POINT('Ctrl Pts',(-8.10591260651796,15.2,-7.78868355205287));
#280736=CARTESIAN_POINT('Ctrl Pts',(-8.10726659272491,15.2,-7.79187361353483));
#280737=CARTESIAN_POINT('Ctrl Pts',(-8.10861963499181,15.2,-7.79507188608236));
#280738=CARTESIAN_POINT('Ctrl Pts',(-8.10997169278217,15.2,-7.79827834752205));
#280739=CARTESIAN_POINT('Ctrl Pts',(-8.11132375057252,15.2,-7.80148480896174));
#280740=CARTESIAN_POINT('Ctrl Pts',(-8.11267482528518,15.2,-7.80469945793326));
#280741=CARTESIAN_POINT('Ctrl Pts',(-8.11402487511122,15.2,-7.80792227489881));
#280742=CARTESIAN_POINT('Ctrl Pts',(-8.11537492493727,15.2,-7.81114509186436));
#280743=CARTESIAN_POINT('Ctrl Pts',(-8.1167239517217,15.2,-7.81437607632928));
#280744=CARTESIAN_POINT('Ctrl Pts',(-8.11807191546454,15.2,-7.81761520579384));
#280745=CARTESIAN_POINT('Ctrl Pts',(-8.11941987945226,15.2,-7.82085433584683));
#280746=CARTESIAN_POINT('Ctrl Pts',(-8.12076678004801,15.2,-7.82410161065208));
#280747=CARTESIAN_POINT('Ctrl Pts',(-8.12211257899344,15.2,-7.82735700970964));
#280748=CARTESIAN_POINT('Ctrl Pts',(-8.12345837769439,15.2,-7.8306124081758));
#280749=CARTESIAN_POINT('Ctrl Pts',(-8.12480307457515,15.2,-7.8338759306875));
#280750=CARTESIAN_POINT('Ctrl Pts',(-8.12614663080166,15.2,-7.83714755489968));
#280751=CARTESIAN_POINT('Ctrl Pts',(-8.12749018702817,15.2,-7.84041917911187));
#280752=CARTESIAN_POINT('Ctrl Pts',(-8.12883260141174,15.2,-7.84369890577722));
#280753=CARTESIAN_POINT('Ctrl Pts',(-8.13017383765457,15.2,-7.84698671232513));
#280754=CARTESIAN_POINT('Ctrl Pts',(-8.1315150738974,15.2,-7.85027451887304));
#280755=CARTESIAN_POINT('Ctrl Pts',(-8.13285513171538,15.2,-7.85357040655335));
#280756=CARTESIAN_POINT('Ctrl Pts',(-8.13419397100006,15.2,-7.85687435301662));
#280757=CARTESIAN_POINT('Ctrl Pts',(-8.13597909020845,15.2,-7.8612796153678));
#280758=CARTESIAN_POINT('Ctrl Pts',(-8.13776204531384,15.2,-7.86569920457347));
#280759=CARTESIAN_POINT('Ctrl Pts',(-8.13954274579954,15.2,-7.87013306898324));
#280760=CARTESIAN_POINT('Ctrl Pts',(-8.1408782710425,15.2,-7.8734584669885));
#280761=CARTESIAN_POINT('Ctrl Pts',(-8.14221252822721,15.2,-7.87679189515169));
#280762=CARTESIAN_POINT('Ctrl Pts',(-8.14354547997034,15.2,-7.88013333211432));
#280763=CARTESIAN_POINT('Ctrl Pts',(-8.14487843171346,15.2,-7.88347476907694));
#280764=CARTESIAN_POINT('Ctrl Pts',(-8.14621007741024,15.2,-7.88682421454305));
#280765=CARTESIAN_POINT('Ctrl Pts',(-8.14754038024294,15.2,-7.89018164701968));
#280766=CARTESIAN_POINT('Ctrl Pts',(-8.14887068307564,15.2,-7.8935390794963));
#280767=CARTESIAN_POINT('Ctrl Pts',(-8.15019964362439,15.2,-7.89690449907083));
#280768=CARTESIAN_POINT('Ctrl Pts',(-8.15152722299886,15.2,-7.90027788450523));
#280769=CARTESIAN_POINT('Ctrl Pts',(-8.15285480237333,15.2,-7.90365126993963));
#280770=CARTESIAN_POINT('Ctrl Pts',(-8.15418100253699,15.2,-7.90703262048783));
#280771=CARTESIAN_POINT('Ctrl Pts',(-8.15550578482231,15.2,-7.91042191540566));
#280772=CARTESIAN_POINT('Ctrl Pts',(-8.15683056710763,15.2,-7.91381121032349));
#280773=CARTESIAN_POINT('Ctrl Pts',(-8.15815393230972,15.2,-7.91720844841578));
#280774=CARTESIAN_POINT('Ctrl Pts',(-8.15947584401189,15.2,-7.92061361074931));
#280775=CARTESIAN_POINT('Ctrl Pts',(-8.1607977559542,15.2,-7.92401877370144));
#280776=CARTESIAN_POINT('Ctrl Pts',(-8.16211821336277,15.2,-7.9274318581808));
#280777=CARTESIAN_POINT('Ctrl Pts',(-8.16343718180427,15.2,-7.93085284430408));
#280778=CARTESIAN_POINT('Ctrl Pts',(-8.16475615000615,15.2,-7.93427382980588));
#280779=CARTESIAN_POINT('Ctrl Pts',(-8.16607362742023,15.2,-7.93770271745056));
#280780=CARTESIAN_POINT('Ctrl Pts',(-8.16738957877132,15.2,-7.9411394841233));
#280781=CARTESIAN_POINT('Ctrl Pts',(-8.1687055301224,15.2,-7.94457625079604));
#280782=CARTESIAN_POINT('Ctrl Pts',(-8.17001995477432,15.2,-7.94802089676783));
#280783=CARTESIAN_POINT('Ctrl Pts',(-8.17133281710148,15.2,-7.95147340168475));
#280784=CARTESIAN_POINT('Ctrl Pts',(-8.17264567942864,15.2,-7.95492590660167));
#280785=CARTESIAN_POINT('Ctrl Pts',(-8.17395697999766,15.2,-7.95838626900931));
#280786=CARTESIAN_POINT('Ctrl Pts',(-8.17526668274173,15.2,-7.96185446946661));
#280787=CARTESIAN_POINT('Ctrl Pts',(-8.17701295322578,15.2,-7.96647873716306));
#280788=CARTESIAN_POINT('Ctrl Pts',(-8.17875638333175,15.2,-7.97111693799453));
#280789=CARTESIAN_POINT('Ctrl Pts',(-8.18049688925963,15.2,-7.97576902102724));
#280790=CARTESIAN_POINT('Ctrl Pts',(-8.18180226858697,15.2,-7.97925808298485));
#280791=CARTESIAN_POINT('Ctrl Pts',(-8.18310600370109,15.2,-7.98275495329611));
#280792=CARTESIAN_POINT('Ctrl Pts',(-8.18440805655197,15.2,-7.9862596104281));
#280793=CARTESIAN_POINT('Ctrl Pts',(-8.18571010940285,15.2,-7.98976426756009));
#280794=CARTESIAN_POINT('Ctrl Pts',(-8.1870104792056,15.2,-7.9932767103777));
#280795=CARTESIAN_POINT('Ctrl Pts',(-8.18830913461659,15.2,-7.99679691987545));
#280796=CARTESIAN_POINT('Ctrl Pts',(-8.18960779002758,15.2,-8.00031712937321));
#280797=CARTESIAN_POINT('Ctrl Pts',(-8.19090473189713,15.2,-8.00384510606176));
#280798=CARTESIAN_POINT('Ctrl Pts',(-8.19219992676674,15.2,-8.00738082855829));
#280799=CARTESIAN_POINT('Ctrl Pts',(-8.19349512163635,15.2,-8.01091655105482));
#280800=CARTESIAN_POINT('Ctrl Pts',(-8.19478857108935,15.2,-8.01446002052605));
#280801=CARTESIAN_POINT('Ctrl Pts',(-8.19608023433425,15.2,-8.01801121339634));
#280802=CARTESIAN_POINT('Ctrl Pts',(-8.19737189757914,15.2,-8.02156240626663));
#280803=CARTESIAN_POINT('Ctrl Pts',(-8.19866177459974,15.2,-8.02512132039559));
#280804=CARTESIAN_POINT('Ctrl Pts',(-8.19994982449251,15.2,-8.02868793252666));
#280805=CARTESIAN_POINT('Ctrl Pts',(-8.20123787438529,15.2,-8.03225454465772));
#280806=CARTESIAN_POINT('Ctrl Pts',(-8.20252409654982,15.2,-8.03582885306697));
#280807=CARTESIAN_POINT('Ctrl Pts',(-8.20380846725341,15.2,-8.03941084372744));
#280808=CARTESIAN_POINT('Ctrl Pts',(-8.2055209616804,15.2,-8.04418683170854));
#280809=CARTESIAN_POINT('Ctrl Pts',(-8.20723016286852,15.2,-8.04897647635779));
#280810=CARTESIAN_POINT('Ctrl Pts',(-8.20893607000006,15.2,-8.05377977100001));
#280811=CARTESIAN_POINT('Ctrl Pts',(-7.64657512400006,12.2,-7.01216898700002));
#280812=CARTESIAN_POINT('Ctrl Pts',(-7.64778328679899,12.2,-7.01348522587027));
#280813=CARTESIAN_POINT('Ctrl Pts',(-7.64902613388113,12.2,-7.01484722203433));
#280814=CARTESIAN_POINT('Ctrl Pts',(-7.65030255133521,12.2,-7.01625467938746));
#280815=CARTESIAN_POINT('Ctrl Pts',(-7.65158512431943,12.2,-7.01766892421138));
#280816=CARTESIAN_POINT('Ctrl Pts',(-7.65290158882944,12.2,-7.01912907735244));
#280817=CARTESIAN_POINT('Ctrl Pts',(-7.65425083088893,12.2,-7.02063486217904));
#280818=CARTESIAN_POINT('Ctrl Pts',(-7.65560007282589,12.2,-7.02214064686888));
#280819=CARTESIAN_POINT('Ctrl Pts',(-7.6569820926347,12.2,-7.02369206393294));
#280820=CARTESIAN_POINT('Ctrl Pts',(-7.65839581074999,12.2,-7.02528884179159));
#280821=CARTESIAN_POINT('Ctrl Pts',(-7.65980952886529,12.2,-7.02688561965024));
#280822=CARTESIAN_POINT('Ctrl Pts',(-7.66125494568895,12.2,-7.02852776104979));
#280823=CARTESIAN_POINT('Ctrl Pts',(-7.66273101487395,12.2,-7.03021499707016));
#280824=CARTESIAN_POINT('Ctrl Pts',(-7.66420708419303,12.2,-7.03190223324379));
#280825=CARTESIAN_POINT('Ctrl Pts',(-7.66571380278172,12.2,-7.03363456758543));
#280826=CARTESIAN_POINT('Ctrl Pts',(-7.66725015536747,12.2,-7.03541173743532));
#280827=CARTESIAN_POINT('Ctrl Pts',(-7.66878650781365,12.2,-7.03718890712378));
#280828=CARTESIAN_POINT('Ctrl Pts',(-7.67035249574304,12.2,-7.03901091194339));
#280829=CARTESIAN_POINT('Ctrl Pts',(-7.67194712427573,12.2,-7.04087749571745));
#280830=CARTESIAN_POINT('Ctrl Pts',(-7.67354175280843,12.2,-7.04274407949153));
#280831=CARTESIAN_POINT('Ctrl Pts',(-7.67516502602135,12.2,-7.04465524296655));
#280832=CARTESIAN_POINT('Ctrl Pts',(-7.67681598062681,12.2,-7.04661073189355));
#280833=CARTESIAN_POINT('Ctrl Pts',(-7.67846693538224,12.2,-7.04856622099817));
#280834=CARTESIAN_POINT('Ctrl Pts',(-7.68014557084944,12.2,-7.05056603617498));
#280835=CARTESIAN_POINT('Ctrl Pts',(-7.68185095069424,12.2,-7.05260992995607));
#280836=CARTESIAN_POINT('Ctrl Pts',(-7.68355633038413,12.2,-7.05465382355151));
#280837=CARTESIAN_POINT('Ctrl Pts',(-7.68528845682534,12.2,-7.05674179384187));
#280838=CARTESIAN_POINT('Ctrl Pts',(-7.68704641459593,12.2,-7.05887359659964));
#280839=CARTESIAN_POINT('Ctrl Pts',(-7.68880437236652,12.2,-7.06100539935743));
#280840=CARTESIAN_POINT('Ctrl Pts',(-7.69058816346834,12.2,-7.06318103452004));
#280841=CARTESIAN_POINT('Ctrl Pts',(-7.69239689940154,12.2,-7.06540025935418));
#280842=CARTESIAN_POINT('Ctrl Pts',(-7.69420563533474,12.2,-7.06761948418832));
#280843=CARTESIAN_POINT('Ctrl Pts',(-7.69603931658333,12.2,-7.06988230103532));
#280844=CARTESIAN_POINT('Ctrl Pts',(-7.69789707751419,12.2,-7.07218846778191));
#280845=CARTESIAN_POINT('Ctrl Pts',(-7.6997548386138,12.2,-7.07449463473798));
#280846=CARTESIAN_POINT('Ctrl Pts',(-7.7016366791741,12.2,-7.07684415463993));
#280847=CARTESIAN_POINT('Ctrl Pts',(-7.70354175636227,12.2,-7.07923678885552));
#280848=CARTESIAN_POINT('Ctrl Pts',(-7.70544683337737,12.2,-7.08162942285377));
#280849=CARTESIAN_POINT('Ctrl Pts',(-7.70737514672789,12.2,-7.08406517436941));
#280850=CARTESIAN_POINT('Ctrl Pts',(-7.70932587299913,12.2,-7.08654380820715));
#280851=CARTESIAN_POINT('Ctrl Pts',(-7.71127659927036,12.2,-7.08902244204489));
#280852=CARTESIAN_POINT('Ctrl Pts',(-7.71324973925656,12.2,-7.09154395937487));
#280853=CARTESIAN_POINT('Ctrl Pts',(-7.71524449051593,12.2,-7.09410813019545));
#280854=CARTESIAN_POINT('Ctrl Pts',(-7.71723924195649,12.2,-7.09667230124895));
#280855=CARTESIAN_POINT('Ctrl Pts',(-7.71925560443252,12.2,-7.09927912477326));
#280856=CARTESIAN_POINT('Ctrl Pts',(-7.7212927938778,12.2,-7.10192837566951));
#280857=CARTESIAN_POINT('Ctrl Pts',(-7.72332998313804,12.2,-7.10457762632511));
#280858=CARTESIAN_POINT('Ctrl Pts',(-7.72538800039851,12.2,-7.10726930092738));
#280859=CARTESIAN_POINT('Ctrl Pts',(-7.72746607899907,12.2,-7.11000317792369));
#280860=CARTESIAN_POINT('Ctrl Pts',(-7.72954415759963,12.2,-7.11273705492002));
#280861=CARTESIAN_POINT('Ctrl Pts',(-7.73164230023916,12.2,-7.11551313281472));
#280862=CARTESIAN_POINT('Ctrl Pts',(-7.73375975674422,12.2,-7.11833118970945));
#280863=CARTESIAN_POINT('Ctrl Pts',(-7.73587721344161,12.2,-7.12114924686015));
#280864=CARTESIAN_POINT('Ctrl Pts',(-7.73801398519903,12.2,-7.12400928335858));
#280865=CARTESIAN_POINT('Ctrl Pts',(-7.74016934292524,12.2,-7.12691107683076));
#280866=CARTESIAN_POINT('Ctrl Pts',(-7.74232470045566,12.2,-7.12981287003937));
#280867=CARTESIAN_POINT('Ctrl Pts',(-7.74449864221298,12.2,-7.13275642378339));
#280868=CARTESIAN_POINT('Ctrl Pts',(-7.74669045496669,12.2,-7.13574151575828));
#280869=CARTESIAN_POINT('Ctrl Pts',(-7.74888226772041,12.2,-7.13872660773317));
#280870=CARTESIAN_POINT('Ctrl Pts',(-7.751091952672,12.2,-7.14175324162222));
#280871=CARTESIAN_POINT('Ctrl Pts',(-7.75331881053465,12.2,-7.14482119791159));
#280872=CARTESIAN_POINT('Ctrl Pts',(-7.75554566859958,12.2,-7.14788915447965));
#280873=CARTESIAN_POINT('Ctrl Pts',(-7.75778970044715,12.2,-7.15099843786056));
#280874=CARTESIAN_POINT('Ctrl Pts',(-7.7600502224881,12.2,-7.15414883011836));
#280875=CARTESIAN_POINT('Ctrl Pts',(-7.76231074432374,12.2,-7.15729922209));
#280876=CARTESIAN_POINT('Ctrl Pts',(-7.76458775655725,12.2,-7.16049072517075));
#280877=CARTESIAN_POINT('Ctrl Pts',(-7.76688059148441,12.2,-7.16372312523475));
#280878=CARTESIAN_POINT('Ctrl Pts',(-7.76917342641157,12.2,-7.16695552529877));
#280879=CARTESIAN_POINT('Ctrl Pts',(-7.77148208440854,12.2,-7.17022882502502));
#280880=CARTESIAN_POINT('Ctrl Pts',(-7.77380591132343,12.2,-7.17354281106948));
#280881=CARTESIAN_POINT('Ctrl Pts',(-7.77574243382287,12.2,-7.17630446620688));
#280882=CARTESIAN_POINT('Ctrl Pts',(-7.77768949117817,12.2,-7.17909437651173));
#280883=CARTESIAN_POINT('Ctrl Pts',(-7.77964671041376,12.2,-7.18191242227415));
#280884=CARTESIAN_POINT('Ctrl Pts',(-7.78160392964934,12.2,-7.18473046803657));
#280885=CARTESIAN_POINT('Ctrl Pts',(-7.78357131294001,12.2,-7.18757664781319));
#280886=CARTESIAN_POINT('Ctrl Pts',(-7.78554849399063,12.2,-7.19045084275673));
#280887=CARTESIAN_POINT('Ctrl Pts',(-7.78752567504125,12.2,-7.19332503770025));
#280888=CARTESIAN_POINT('Ctrl Pts',(-7.78951265463893,12.2,-7.19622724628885));
#280889=CARTESIAN_POINT('Ctrl Pts',(-7.79150907470837,12.2,-7.19915735052494));
#280890=CARTESIAN_POINT('Ctrl Pts',(-7.79350549477779,12.2,-7.20208745476104));
#280891=CARTESIAN_POINT('Ctrl Pts',(-7.79551135383639,12.2,-7.2050454544546));
#280892=CARTESIAN_POINT('Ctrl Pts',(-7.79752630148447,12.2,-7.20803123050992));
#280893=CARTESIAN_POINT('Ctrl Pts',(-7.79954124913254,12.2,-7.21101700656522));
#280894=CARTESIAN_POINT('Ctrl Pts',(-7.80156528368812,12.2,-7.21403056018645));
#280895=CARTESIAN_POINT('Ctrl Pts',(-7.80359806042469,12.2,-7.217071771924));
#280896=CARTESIAN_POINT('Ctrl Pts',(-7.80563083716125,12.2,-7.22011298366153));
#280897=CARTESIAN_POINT('Ctrl Pts',(-7.80767235392262,12.2,-7.2231818550512));
#280898=CARTESIAN_POINT('Ctrl Pts',(-7.80972227170081,12.2,-7.22627826692761));
#280899=CARTESIAN_POINT('Ctrl Pts',(-7.81177218947903,12.2,-7.22937467880403));
#280900=CARTESIAN_POINT('Ctrl Pts',(-7.81383050736948,12.2,-7.2324986330732));
#280901=CARTESIAN_POINT('Ctrl Pts',(-7.81589689101494,12.2,-7.23565001385754));
#280902=CARTESIAN_POINT('Ctrl Pts',(-7.81796327466039,12.2,-7.23880139464188));
#280903=CARTESIAN_POINT('Ctrl Pts',(-7.82003772227731,12.2,-7.24198019922819));
#280904=CARTESIAN_POINT('Ctrl Pts',(-7.8221199067224,12.2,-7.24518631270266));
#280905=CARTESIAN_POINT('Ctrl Pts',(-7.82420209116748,12.2,-7.24839242617712));
#280906=CARTESIAN_POINT('Ctrl Pts',(-7.826292010146,12.2,-7.251625849902));
#280907=CARTESIAN_POINT('Ctrl Pts',(-7.82838933979937,12.2,-7.25488646816811));
#280908=CARTESIAN_POINT('Ctrl Pts',(-7.83048666922415,12.2,-7.25814708607882));
#280909=CARTESIAN_POINT('Ctrl Pts',(-7.83259141104903,12.2,-7.26143489747436));
#280910=CARTESIAN_POINT('Ctrl Pts',(-7.83470324366548,12.2,-7.26474978954136));
#280911=CARTESIAN_POINT('Ctrl Pts',(-7.8368150765121,12.2,-7.26806468196968));
#280912=CARTESIAN_POINT('Ctrl Pts',(-7.83893400051145,12.2,-7.27140665157263));
#280913=CARTESIAN_POINT('Ctrl Pts',(-7.84105970245533,12.2,-7.27477558900097));
#280914=CARTESIAN_POINT('Ctrl Pts',(-7.84318540439921,12.2,-7.2781445264293));
#280915=CARTESIAN_POINT('Ctrl Pts',(-7.8453178832708,12.2,-7.28154042926556));
#280916=CARTESIAN_POINT('Ctrl Pts',(-7.84745682972861,12.2,-7.28496318356893));
#280917=CARTESIAN_POINT('Ctrl Pts',(-7.84959577618641,12.2,-7.2883859378723));
#280918=CARTESIAN_POINT('Ctrl Pts',(-7.85174119063212,12.2,-7.2918355454858));
#280919=CARTESIAN_POINT('Ctrl Pts',(-7.8538927687253,12.2,-7.29531189162983));
#280920=CARTESIAN_POINT('Ctrl Pts',(-7.85604434681847,12.2,-7.29878823777386));
#280921=CARTESIAN_POINT('Ctrl Pts',(-7.85820208679777,12.2,-7.30229132184845));
#280922=CARTESIAN_POINT('Ctrl Pts',(-7.86036569061691,12.2,-7.3058210342776));
#280923=CARTESIAN_POINT('Ctrl Pts',(-7.86252929443604,12.2,-7.30935074670676));
#280924=CARTESIAN_POINT('Ctrl Pts',(-7.86469876073591,12.2,-7.31290708506164));
#280925=CARTESIAN_POINT('Ctrl Pts',(-7.86687379608283,12.2,-7.31648993853245));
#280926=CARTESIAN_POINT('Ctrl Pts',(-7.86904883142975,12.2,-7.32007279200327));
#280927=CARTESIAN_POINT('Ctrl Pts',(-7.87122943191116,12.2,-7.32368216048709));
#280928=CARTESIAN_POINT('Ctrl Pts',(-7.87341531074052,12.2,-7.32731793223964));
#280929=CARTESIAN_POINT('Ctrl Pts',(-7.87516401389931,12.2,-7.3302265498002));
#280930=CARTESIAN_POINT('Ctrl Pts',(-7.87691609317994,12.2,-7.33315206547728));
#280931=CARTESIAN_POINT('Ctrl Pts',(-7.8786714030537,12.2,-7.3360944224727));
#280932=CARTESIAN_POINT('Ctrl Pts',(-7.88042671268832,12.2,-7.33903677906723));
#280933=CARTESIAN_POINT('Ctrl Pts',(-7.88218525180583,12.2,-7.34199597845954));
#280934=CARTESIAN_POINT('Ctrl Pts',(-7.88394687610606,12.2,-7.34497196104849));
#280935=CARTESIAN_POINT('Ctrl Pts',(-7.88570850064631,12.2,-7.34794794404292));
#280936=CARTESIAN_POINT('Ctrl Pts',(-7.88747320981609,12.2,-7.35094071248757));
#280937=CARTESIAN_POINT('Ctrl Pts',(-7.88924085922323,12.2,-7.35395020947008));
#280938=CARTESIAN_POINT('Ctrl Pts',(-7.89100850838953,12.2,-7.35695970604255));
#280939=CARTESIAN_POINT('Ctrl Pts',(-7.89277909937803,12.2,-7.3599859298373));
#280940=CARTESIAN_POINT('Ctrl Pts',(-7.89455248912176,12.2,-7.36302882630968));
#280941=CARTESIAN_POINT('Ctrl Pts',(-7.89632587910712,12.2,-7.36607172319666));
#280942=CARTESIAN_POINT('Ctrl Pts',(-7.89810206675392,12.2,-7.36913129149951));
#280943=CARTESIAN_POINT('Ctrl Pts',(-7.89988091462883,12.2,-7.37220747700159));
#280944=CARTESIAN_POINT('Ctrl Pts',(-7.90165976226136,12.2,-7.37528366208455));
#280945=CARTESIAN_POINT('Ctrl Pts',(-7.9034412671759,12.2,-7.37837646237136));
#280946=CARTESIAN_POINT('Ctrl Pts',(-7.90522529300786,12.2,-7.38148582304886));
#280947=CARTESIAN_POINT('Ctrl Pts',(-7.90700931908289,12.2,-7.38459518415));
#280948=CARTESIAN_POINT('Ctrl Pts',(-7.90879586575977,12.2,-7.38772110534021));
#280949=CARTESIAN_POINT('Ctrl Pts',(-7.91058479441298,12.2,-7.39086353029033));
#280950=CARTESIAN_POINT('Ctrl Pts',(-7.91237372282244,12.2,-7.39400595481229));
#280951=CARTESIAN_POINT('Ctrl Pts',(-7.91416503376754,12.2,-7.39716488463093));
#280952=CARTESIAN_POINT('Ctrl Pts',(-7.9159585922318,12.2,-7.40034026248078));
#280953=CARTESIAN_POINT('Ctrl Pts',(-7.91775215094043,12.2,-7.40351564076328));
#280954=CARTESIAN_POINT('Ctrl Pts',(-7.91954795652011,12.2,-7.40670746824044));
#280955=CARTESIAN_POINT('Ctrl Pts',(-7.92134587579294,12.2,-7.40991568798548));
#280956=CARTESIAN_POINT('Ctrl Pts',(-7.9231437948208,12.2,-7.41312390729339));
#280957=CARTESIAN_POINT('Ctrl Pts',(-7.92494382559738,12.2,-7.41634852125891));
#280958=CARTESIAN_POINT('Ctrl Pts',(-7.92674583800542,12.2,-7.41958947243673));
#280959=CARTESIAN_POINT('Ctrl Pts',(-7.92854785065898,12.2,-7.42283042405612));
#280960=CARTESIAN_POINT('Ctrl Pts',(-7.93035184389329,12.2,-7.42608771360763));
#280961=CARTESIAN_POINT('Ctrl Pts',(-7.93215768549172,12.2,-7.42936128650828));
#280962=CARTESIAN_POINT('Ctrl Pts',(-7.93396352709014,12.2,-7.43263485940892));
#280963=CARTESIAN_POINT('Ctrl Pts',(-7.9357712199971,12.2,-7.43592471539755));
#280964=CARTESIAN_POINT('Ctrl Pts',(-7.93758063076256,12.2,-7.43923079902384));
#280965=CARTESIAN_POINT('Ctrl Pts',(-7.93939004128148,12.2,-7.44253688219967));
#280966=CARTESIAN_POINT('Ctrl Pts',(-7.94120117155267,12.2,-7.44585919355828));
#280967=CARTESIAN_POINT('Ctrl Pts',(-7.94301389402381,12.2,-7.44919767802268));
#280968=CARTESIAN_POINT('Ctrl Pts',(-7.94482661674193,12.2,-7.45253616294194));
#280969=CARTESIAN_POINT('Ctrl Pts',(-7.94664092989783,12.2,-7.45589082048797));
#280970=CARTESIAN_POINT('Ctrl Pts',(-7.94845670799693,12.2,-7.45926159678441));
#280971=CARTESIAN_POINT('Ctrl Pts',(-7.95027248584863,12.2,-7.46263237262158));
#280972=CARTESIAN_POINT('Ctrl Pts',(-7.95208972816681,12.2,-7.46601926705391));
#280973=CARTESIAN_POINT('Ctrl Pts',(-7.9539083093514,12.2,-7.46942222549692));
#280974=CARTESIAN_POINT('Ctrl Pts',(-7.95572689078377,12.2,-7.47282518440357));
#280975=CARTESIAN_POINT('Ctrl Pts',(-7.95754681050731,12.2,-7.47624420602161));
#280976=CARTESIAN_POINT('Ctrl Pts',(-7.95936794603098,12.2,-7.47967923904849));
#280977=CARTESIAN_POINT('Ctrl Pts',(-7.96118908130653,12.2,-7.48311427160735));
#280978=CARTESIAN_POINT('Ctrl Pts',(-7.96301143108625,12.2,-7.48656531198448));
#280979=CARTESIAN_POINT('Ctrl Pts',(-7.964834872326,12.2,-7.49003230903334));
#280980=CARTESIAN_POINT('Ctrl Pts',(-7.96711417406201,12.2,-7.4943660556987));
#280981=CARTESIAN_POINT('Ctrl Pts',(-7.96939518206196,12.2,-7.49872473117026));
#280982=CARTESIAN_POINT('Ctrl Pts',(-7.97167765886746,12.2,-7.50310823144676));
#280983=CARTESIAN_POINT('Ctrl Pts',(-7.97350364041137,12.2,-7.50661503185908));
#280984=CARTESIAN_POINT('Ctrl Pts',(-7.97533056256594,12.2,-7.51013772196472));
#280985=CARTESIAN_POINT('Ctrl Pts',(-7.97715830425694,12.2,-7.51367624378017));
#280986=CARTESIAN_POINT('Ctrl Pts',(-7.9789860456989,12.2,-7.51721476511349));
#280987=CARTESIAN_POINT('Ctrl Pts',(-7.98081460814177,12.2,-7.52076912063723));
#280988=CARTESIAN_POINT('Ctrl Pts',(-7.98264387082552,12.2,-7.52433925573324));
#280989=CARTESIAN_POINT('Ctrl Pts',(-7.9844731337585,12.2,-7.52790939131568));
#280990=CARTESIAN_POINT('Ctrl Pts',(-7.98630309936101,12.2,-7.53149530585554));
#280991=CARTESIAN_POINT('Ctrl Pts',(-7.98813364768304,12.2,-7.53509694755286));
#280992=CARTESIAN_POINT('Ctrl Pts',(-7.98996419575566,12.2,-7.53869858875946));
#280993=CARTESIAN_POINT('Ctrl Pts',(-7.9917953287226,12.2,-7.54231595590735));
#280994=CARTESIAN_POINT('Ctrl Pts',(-7.99362692868392,12.2,-7.5459489956643));
#280995=CARTESIAN_POINT('Ctrl Pts',(-7.9954585288948,12.2,-7.54958203591625));
#280996=CARTESIAN_POINT('Ctrl Pts',(-7.99729059673478,12.2,-7.55323074782494));
#280997=CARTESIAN_POINT('Ctrl Pts',(-7.99912301700964,12.2,-7.55689507948579));
#280998=CARTESIAN_POINT('Ctrl Pts',(-8.00095543703482,12.2,-7.56055941064737));
#280999=CARTESIAN_POINT('Ctrl Pts',(-8.00278821065578,12.2,-7.56423936167444));
#281000=CARTESIAN_POINT('Ctrl Pts',(-8.00462122195036,12.2,-7.56793487687075));
#281001=CARTESIAN_POINT('Ctrl Pts',(-8.00645423349468,12.2,-7.57163039257056));
#281002=CARTESIAN_POINT('Ctrl Pts',(-8.00828748325846,12.2,-7.57534147510517));
#281003=CARTESIAN_POINT('Ctrl Pts',(-8.01012085952506,12.2,-7.57906806947495));
#281004=CARTESIAN_POINT('Ctrl Pts',(-8.01195423579165,12.2,-7.58279466384472));
#281005=CARTESIAN_POINT('Ctrl Pts',(-8.01378773657214,12.2,-7.58653676989129));
#281006=CARTESIAN_POINT('Ctrl Pts',(-8.01562125278317,12.2,-7.59029433609766));
#281007=CARTESIAN_POINT('Ctrl Pts',(-8.01745476874439,12.2,-7.59405190179206));
#281008=CARTESIAN_POINT('Ctrl Pts',(-8.01928829781258,12.2,-7.59782492632881));
#281009=CARTESIAN_POINT('Ctrl Pts',(-8.02112173178214,12.2,-7.6016133574807));
#281010=CARTESIAN_POINT('Ctrl Pts',(-8.0229551660015,12.2,-7.60540178914877));
#281011=CARTESIAN_POINT('Ctrl Pts',(-8.02478850271655,12.2,-7.60920562673968));
#281012=CARTESIAN_POINT('Ctrl Pts',(-8.02662163481644,12.2,-7.61302481711606));
#281013=CARTESIAN_POINT('Ctrl Pts',(-8.02845476666656,12.2,-7.61684400697208));
#281014=CARTESIAN_POINT('Ctrl Pts',(-8.0302876903417,12.2,-7.62067855060665));
#281015=CARTESIAN_POINT('Ctrl Pts',(-8.03212030235857,12.2,-7.62452839440204));
#281016=CARTESIAN_POINT('Ctrl Pts',(-8.03395291462513,12.2,-7.62837823872196));
#281017=CARTESIAN_POINT('Ctrl Pts',(-8.03578521218844,12.2,-7.632243385587));
#281018=CARTESIAN_POINT('Ctrl Pts',(-8.03761708799087,12.2,-7.63612377760477));
#281019=CARTESIAN_POINT('Ctrl Pts',(-8.03944896354372,12.2,-7.64000416909386));
#281020=CARTESIAN_POINT('Ctrl Pts',(-8.04128041861114,12.2,-7.64389980889278));
#281021=CARTESIAN_POINT('Ctrl Pts',(-8.04311134535038,12.2,-7.64781064340539));
#281022=CARTESIAN_POINT('Ctrl Pts',(-8.04494227233908,12.2,-7.65172147845086));
#281023=CARTESIAN_POINT('Ctrl Pts',(-8.04677267074162,12.2,-7.65564750982872));
#281024=CARTESIAN_POINT('Ctrl Pts',(-8.04860243767464,12.2,-7.65958868282229));
#281025=CARTESIAN_POINT('Ctrl Pts',(-8.05043220435835,12.2,-7.66352985527887));
#281026=CARTESIAN_POINT('Ctrl Pts',(-8.05226133673446,12.2,-7.66748616979299));
#281027=CARTESIAN_POINT('Ctrl Pts',(-8.05408973350974,12.2,-7.67145757516543));
#281028=CARTESIAN_POINT('Ctrl Pts',(-8.05591813053414,12.2,-7.67542898107897));
#281029=CARTESIAN_POINT('Ctrl Pts',(-8.05774579051655,12.2,-7.67941547698038));
#281030=CARTESIAN_POINT('Ctrl Pts',(-8.05957260961606,12.2,-7.68341701064389));
#281031=CARTESIAN_POINT('Ctrl Pts',(-8.061856133366,12.2,-7.68841892745067));
#281032=CARTESIAN_POINT('Ctrl Pts',(-8.06413834403262,12.2,-7.69344434071793));
#281033=CARTESIAN_POINT('Ctrl Pts',(-8.06641904340754,12.2,-7.69849314828861));
#281034=CARTESIAN_POINT('Ctrl Pts',(-8.06824360275832,12.2,-7.70253219401496));
#281035=CARTESIAN_POINT('Ctrl Pts',(-8.070067194374,12.2,-7.70658621244861));
#281036=CARTESIAN_POINT('Ctrl Pts',(-8.0718897172606,12.2,-7.71065515115128));
#281037=CARTESIAN_POINT('Ctrl Pts',(-8.0737122403955,12.2,-7.71472409040834));
#281038=CARTESIAN_POINT('Ctrl Pts',(-8.07553369376639,12.2,-7.71880794960248));
#281039=CARTESIAN_POINT('Ctrl Pts',(-8.07735397886553,12.2,-7.72290667732684));
#281040=CARTESIAN_POINT('Ctrl Pts',(-8.07871919256587,12.2,-7.72598072284089));
#281041=CARTESIAN_POINT('Ctrl Pts',(-8.08008374933296,12.2,-7.72906313216229));
#281042=CARTESIAN_POINT('Ctrl Pts',(-8.08144760649173,12.2,-7.73215388225828));
#281043=CARTESIAN_POINT('Ctrl Pts',(-8.08281146365049,12.2,-7.73524463235428));
#281044=CARTESIAN_POINT('Ctrl Pts',(-8.08417462120097,12.2,-7.73834372525835));
#281045=CARTESIAN_POINT('Ctrl Pts',(-8.08553703835988,12.2,-7.74145113639472));
#281046=CARTESIAN_POINT('Ctrl Pts',(-8.08689945551878,12.2,-7.7445585475311));
#281047=CARTESIAN_POINT('Ctrl Pts',(-8.08826113143478,12.2,-7.74767427943733));
#281048=CARTESIAN_POINT('Ctrl Pts',(-8.08962202570342,12.2,-7.75079830860395));
#281049=CARTESIAN_POINT('Ctrl Pts',(-8.09098291997206,12.2,-7.75392233777057));
#281050=CARTESIAN_POINT('Ctrl Pts',(-8.09234303323634,12.2,-7.75705466433054));
#281051=CARTESIAN_POINT('Ctrl Pts',(-8.09370232202041,12.2,-7.76019526679865));
#281052=CARTESIAN_POINT('Ctrl Pts',(-8.09506161105141,12.2,-7.76333586983731));
#281053=CARTESIAN_POINT('Ctrl Pts',(-8.09642007779883,12.2,-7.7664847491616));
#281054=CARTESIAN_POINT('Ctrl Pts',(-8.09777768028768,12.2,-7.76964188220488));
#281055=CARTESIAN_POINT('Ctrl Pts',(-8.09913528252989,12.2,-7.77279901467461));
#281056=CARTESIAN_POINT('Ctrl Pts',(-8.10049202074717,12.2,-7.77596440096061));
#281057=CARTESIAN_POINT('Ctrl Pts',(-8.10184785540617,12.2,-7.77913802034602));
#281058=CARTESIAN_POINT('Ctrl Pts',(-8.10320369006516,12.2,-7.78231163973142));
#281059=CARTESIAN_POINT('Ctrl Pts',(-8.10455862031101,12.2,-7.7854934905709));
#281060=CARTESIAN_POINT('Ctrl Pts',(-8.10591260651796,12.2,-7.78868355205286));
#281061=CARTESIAN_POINT('Ctrl Pts',(-8.10726659272491,12.2,-7.79187361353483));
#281062=CARTESIAN_POINT('Ctrl Pts',(-8.10861963499181,12.2,-7.79507188608236));
#281063=CARTESIAN_POINT('Ctrl Pts',(-8.10997169278217,12.2,-7.79827834752205));
#281064=CARTESIAN_POINT('Ctrl Pts',(-8.11132375057252,12.2,-7.80148480896174));
#281065=CARTESIAN_POINT('Ctrl Pts',(-8.11267482528518,12.2,-7.80469945793325));
#281066=CARTESIAN_POINT('Ctrl Pts',(-8.11402487511122,12.2,-7.80792227489881));
#281067=CARTESIAN_POINT('Ctrl Pts',(-8.11537492493727,12.2,-7.81114509186436));
#281068=CARTESIAN_POINT('Ctrl Pts',(-8.1167239517217,12.2,-7.81437607632928));
#281069=CARTESIAN_POINT('Ctrl Pts',(-8.11807191546454,12.2,-7.81761520579384));
#281070=CARTESIAN_POINT('Ctrl Pts',(-8.11941987945226,12.2,-7.82085433584683));
#281071=CARTESIAN_POINT('Ctrl Pts',(-8.12076678004801,12.2,-7.82410161065208));
#281072=CARTESIAN_POINT('Ctrl Pts',(-8.12211257899344,12.2,-7.82735700970964));
#281073=CARTESIAN_POINT('Ctrl Pts',(-8.12390697717988,12.2,-7.83169754080072));
#281074=CARTESIAN_POINT('Ctrl Pts',(-8.12569941704539,12.2,-7.83605251407049));
#281075=CARTESIAN_POINT('Ctrl Pts',(-8.12748980474051,12.2,-7.84042187845532));
#281076=CARTESIAN_POINT('Ctrl Pts',(-8.12883259557284,12.2,-7.84369890189279));
#281077=CARTESIAN_POINT('Ctrl Pts',(-8.13017423313587,12.2,-7.84698401969482));
#281078=CARTESIAN_POINT('Ctrl Pts',(-8.13151467933727,12.2,-7.85027721115781));
#281079=CARTESIAN_POINT('Ctrl Pts',(-8.13330194110149,12.2,-7.85466813350729));
#281080=CARTESIAN_POINT('Ctrl Pts',(-8.13508708265155,12.2,-7.8590734087585));
#281081=CARTESIAN_POINT('Ctrl Pts',(-8.13687001513746,12.2,-7.86349298511139));
#281082=CARTESIAN_POINT('Ctrl Pts',(-8.13820721438043,12.2,-7.86680766707499));
#281083=CARTESIAN_POINT('Ctrl Pts',(-8.13954317114856,12.2,-7.87013039323764));
#281084=CARTESIAN_POINT('Ctrl Pts',(-8.14087784651673,12.2,-7.87346114224161));
#281085=CARTESIAN_POINT('Ctrl Pts',(-8.1422125218849,12.2,-7.87679189124559));
#281086=CARTESIAN_POINT('Ctrl Pts',(-8.14354591771979,12.2,-7.88013066364091));
#281087=CARTESIAN_POINT('Ctrl Pts',(-8.14487799454652,12.2,-7.88347743714363));
#281088=CARTESIAN_POINT('Ctrl Pts',(-8.14621007137323,12.2,-7.88682421064635));
#281089=CARTESIAN_POINT('Ctrl Pts',(-8.1475408302079,12.2,-7.89017898563784));
#281090=CARTESIAN_POINT('Ctrl Pts',(-8.14887023397618,12.2,-7.89354174034943));
#281091=CARTESIAN_POINT('Ctrl Pts',(-8.15019963774445,12.2,-7.89690449506101));
#281092=CARTESIAN_POINT('Ctrl Pts',(-8.15152768522553,12.2,-7.90027523048724));
#281093=CARTESIAN_POINT('Ctrl Pts',(-8.15285434092753,12.2,-7.9036539235301));
#281094=CARTESIAN_POINT('Ctrl Pts',(-8.15418099687053,12.2,-7.90703261718674));
#281095=CARTESIAN_POINT('Ctrl Pts',(-8.15550626026313,12.2,-7.91041926979558));
#281096=CARTESIAN_POINT('Ctrl Pts',(-8.15683009383033,12.2,-7.91381385849832));
#281097=CARTESIAN_POINT('Ctrl Pts',(-8.15815392715703,12.2,-7.91720844658438));
#281098=CARTESIAN_POINT('Ctrl Pts',(-8.15947633197548,12.2,-7.92061097312839));
#281099=CARTESIAN_POINT('Ctrl Pts',(-8.16079726988569,12.2,-7.92402141417183));
#281100=CARTESIAN_POINT('Ctrl Pts',(-8.16211820779591,12.2,-7.92743185521529));
#281101=CARTESIAN_POINT('Ctrl Pts',(-8.1634376811765,12.2,-7.93085021121197));
#281102=CARTESIAN_POINT('Ctrl Pts',(-8.1647556515096,12.2,-7.93427646218641));
#281103=CARTESIAN_POINT('Ctrl Pts',(-8.1660736218427,12.2,-7.93770271316086));
#281104=CARTESIAN_POINT('Ctrl Pts',(-8.16739008997401,12.2,-7.94113685873964));
#281105=CARTESIAN_POINT('Ctrl Pts',(-8.16870501972387,12.2,-7.94457887579683));
#281106=CARTESIAN_POINT('Ctrl Pts',(-8.17001994947374,12.2,-7.94802089285403));
#281107=CARTESIAN_POINT('Ctrl Pts',(-8.1713333401379,12.2,-7.95147078329948));
#281108=CARTESIAN_POINT('Ctrl Pts',(-8.17264515738206,12.2,-7.95492852433987));
#281109=CARTESIAN_POINT('Ctrl Pts',(-8.17395697462621,12.2,-7.95838626538026));
#281110=CARTESIAN_POINT('Ctrl Pts',(-8.17526721787878,12.2,-7.96185185807003));
#281111=CARTESIAN_POINT('Ctrl Pts',(-8.17657585124812,12.2,-7.9653252810261));
#281112=CARTESIAN_POINT('Ctrl Pts',(-8.17788448485519,12.2,-7.96879870461317));
#281113=CARTESIAN_POINT('Ctrl Pts',(-8.17919150969515,12.2,-7.97227995843579));
#281114=CARTESIAN_POINT('Ctrl Pts',(-8.18049688925964,12.2,-7.97576902102725));
#281115=CARTESIAN_POINT('Ctrl Pts',(-8.18180226858697,12.2,-7.97925808298485));
#281116=CARTESIAN_POINT('Ctrl Pts',(-8.18310600370109,12.2,-7.98275495329611));
#281117=CARTESIAN_POINT('Ctrl Pts',(-8.18440805655197,12.2,-7.9862596104281));
#281118=CARTESIAN_POINT('Ctrl Pts',(-8.18614412694096,12.2,-7.99093248639187));
#281119=CARTESIAN_POINT('Ctrl Pts',(-8.18787720500818,12.2,-7.99561920371212));
#281120=CARTESIAN_POINT('Ctrl Pts',(-8.18960721736694,12.2,-8.00031971688249));
#281121=CARTESIAN_POINT('Ctrl Pts',(-8.19133722996142,12.2,-8.0050202306933));
#281122=CARTESIAN_POINT('Ctrl Pts',(-8.19306417772778,12.2,-8.00973453997248));
#281123=CARTESIAN_POINT('Ctrl Pts',(-8.19478797743263,12.2,-8.01446259611994));
#281124=CARTESIAN_POINT('Ctrl Pts',(-8.19608082709383,12.2,-8.01800863790843));
#281125=CARTESIAN_POINT('Ctrl Pts',(-8.19737190427557,12.2,-8.0215624105664));
#281126=CARTESIAN_POINT('Ctrl Pts',(-8.19866116752624,12.2,-8.02512388803653));
#281127=CARTESIAN_POINT('Ctrl Pts',(-8.19995043077691,12.2,-8.02868536550668));
#281128=CARTESIAN_POINT('Ctrl Pts',(-8.20123787865643,12.2,-8.03225454801044));
#281129=CARTESIAN_POINT('Ctrl Pts',(-8.20252348074057,12.2,-8.03583141523005));
#281130=CARTESIAN_POINT('Ctrl Pts',(-8.20466615095866,12.2,-8.04179286081266));
#281131=CARTESIAN_POINT('Ctrl Pts',(-8.20680368620185,12.2,-8.04777565302446));
#281132=CARTESIAN_POINT('Ctrl Pts',(-8.20893607000006,12.2,-8.05377977100001));
#281133=CARTESIAN_POINT('Ctrl Pts',(-7.93573928400006,15.2,-8.32310290900002));
#281134=CARTESIAN_POINT('Ctrl Pts',(-7.93573928400006,11.6,-8.32310290900002));
#281135=CARTESIAN_POINT('Ctrl Pts',(-7.93502251600006,15.2,-8.32283676100002));
#281136=CARTESIAN_POINT('Ctrl Pts',(-7.93502251600006,11.6,-8.32283676100002));
#281137=CARTESIAN_POINT('Ctrl Pts',(-7.93358949600006,15.2,-8.32230434800002));
#281138=CARTESIAN_POINT('Ctrl Pts',(-7.93358949600006,11.6,-8.32230434800002));
#281139=CARTESIAN_POINT('Ctrl Pts',(-7.93144150800006,15.2,-8.32150538100001));
#281140=CARTESIAN_POINT('Ctrl Pts',(-7.93144150800006,11.6,-8.32150538100001));
#281141=CARTESIAN_POINT('Ctrl Pts',(-7.92858060400006,15.2,-8.32043939400002));
#281142=CARTESIAN_POINT('Ctrl Pts',(-7.92858060400006,11.6,-8.32043939400002));
#281143=CARTESIAN_POINT('Ctrl Pts',(-7.92500961100006,15.2,-8.31910574700002));
#281144=CARTESIAN_POINT('Ctrl Pts',(-7.92500961100006,11.6,-8.31910574700002));
#281145=CARTESIAN_POINT('Ctrl Pts',(-7.92144375600006,15.2,-8.31777093800002));
#281146=CARTESIAN_POINT('Ctrl Pts',(-7.92144375600006,11.6,-8.31777093800002));
#281147=CARTESIAN_POINT('Ctrl Pts',(-7.91788304100006,15.2,-8.31643496900002));
#281148=CARTESIAN_POINT('Ctrl Pts',(-7.91788304100006,11.6,-8.31643496900002));
#281149=CARTESIAN_POINT('Ctrl Pts',(-7.91432746600006,15.2,-8.31509784400002));
#281150=CARTESIAN_POINT('Ctrl Pts',(-7.91432746600006,11.6,-8.31509784400002));
#281151=CARTESIAN_POINT('Ctrl Pts',(-7.91077703600005,15.2,-8.31375956800001));
#281152=CARTESIAN_POINT('Ctrl Pts',(-7.91077703600005,11.6,-8.31375956800001));
#281153=CARTESIAN_POINT('Ctrl Pts',(-7.90723175400006,15.2,-8.31242014700001));
#281154=CARTESIAN_POINT('Ctrl Pts',(-7.90723175400006,11.6,-8.31242014700001));
#281155=CARTESIAN_POINT('Ctrl Pts',(-7.90369162500006,15.2,-8.31107959100001));
#281156=CARTESIAN_POINT('Ctrl Pts',(-7.90369162500006,11.6,-8.31107959100001));
#281157=CARTESIAN_POINT('Ctrl Pts',(-7.90015665700006,15.2,-8.30973790700002));
#281158=CARTESIAN_POINT('Ctrl Pts',(-7.90015665700006,11.6,-8.30973790700002));
#281159=CARTESIAN_POINT('Ctrl Pts',(-7.89662685200006,15.2,-8.30839510700002));
#281160=CARTESIAN_POINT('Ctrl Pts',(-7.89662685200006,11.6,-8.30839510700002));
#281161=CARTESIAN_POINT('Ctrl Pts',(-7.89310221700006,15.2,-8.30705119800001));
#281162=CARTESIAN_POINT('Ctrl Pts',(-7.89310221700006,11.6,-8.30705119800001));
#281163=CARTESIAN_POINT('Ctrl Pts',(-7.88958275900006,15.2,-8.30570619200002));
#281164=CARTESIAN_POINT('Ctrl Pts',(-7.88958275900006,11.6,-8.30570619200002));
#281165=CARTESIAN_POINT('Ctrl Pts',(-7.88606848200006,15.2,-8.30436009400002));
#281166=CARTESIAN_POINT('Ctrl Pts',(-7.88606848200006,11.6,-8.30436009400002));
#281167=CARTESIAN_POINT('Ctrl Pts',(-7.88255938900006,15.2,-8.30301291500002));
#281168=CARTESIAN_POINT('Ctrl Pts',(-7.88255938900006,11.6,-8.30301291500002));
#281169=CARTESIAN_POINT('Ctrl Pts',(-7.87905548600006,15.2,-8.30166465900002));
#281170=CARTESIAN_POINT('Ctrl Pts',(-7.87905548600006,11.6,-8.30166465900002));
#281171=CARTESIAN_POINT('Ctrl Pts',(-7.87555677500006,15.2,-8.30031533300001));
#281172=CARTESIAN_POINT('Ctrl Pts',(-7.87555677500006,11.6,-8.30031533300001));
#281173=CARTESIAN_POINT('Ctrl Pts',(-7.87206326300005,15.2,-8.29896494600002));
#281174=CARTESIAN_POINT('Ctrl Pts',(-7.87206326300005,11.6,-8.29896494600002));
#281175=CARTESIAN_POINT('Ctrl Pts',(-7.86857495100006,15.2,-8.29761350400002));
#281176=CARTESIAN_POINT('Ctrl Pts',(-7.86857495100006,11.6,-8.29761350400002));
#281177=CARTESIAN_POINT('Ctrl Pts',(-7.86509184800006,15.2,-8.29626101600001));
#281178=CARTESIAN_POINT('Ctrl Pts',(-7.86509184800006,11.6,-8.29626101600001));
#281179=CARTESIAN_POINT('Ctrl Pts',(-7.86161395500006,15.2,-8.29490748900002));
#281180=CARTESIAN_POINT('Ctrl Pts',(-7.86161395500006,11.6,-8.29490748900002));
#281181=CARTESIAN_POINT('Ctrl Pts',(-7.85814127800006,15.2,-8.29355293000001));
#281182=CARTESIAN_POINT('Ctrl Pts',(-7.85814127800006,11.6,-8.29355293000001));
#281183=CARTESIAN_POINT('Ctrl Pts',(-7.85467382200006,15.2,-8.29219735000001));
#281184=CARTESIAN_POINT('Ctrl Pts',(-7.85467382200006,11.6,-8.29219735000001));
#281185=CARTESIAN_POINT('Ctrl Pts',(-7.85121159100005,15.2,-8.29084075600001));
#281186=CARTESIAN_POINT('Ctrl Pts',(-7.85121159100005,11.6,-8.29084075600001));
#281187=CARTESIAN_POINT('Ctrl Pts',(-7.84775459100005,15.2,-8.28948315400002));
#281188=CARTESIAN_POINT('Ctrl Pts',(-7.84775459100005,11.6,-8.28948315400002));
#281189=CARTESIAN_POINT('Ctrl Pts',(-7.84430282600006,15.2,-8.28812455600002));
#281190=CARTESIAN_POINT('Ctrl Pts',(-7.84430282600006,11.6,-8.28812455600002));
#281191=CARTESIAN_POINT('Ctrl Pts',(-7.84085629900006,15.2,-8.28676496700002));
#281192=CARTESIAN_POINT('Ctrl Pts',(-7.84085629900006,11.6,-8.28676496700002));
#281193=CARTESIAN_POINT('Ctrl Pts',(-7.83741501900005,15.2,-8.28540439500001));
#281194=CARTESIAN_POINT('Ctrl Pts',(-7.83741501900005,11.6,-8.28540439500001));
#281195=CARTESIAN_POINT('Ctrl Pts',(-7.83397898600006,15.2,-8.28404285000002));
#281196=CARTESIAN_POINT('Ctrl Pts',(-7.83397898600006,11.6,-8.28404285000002));
#281197=CARTESIAN_POINT('Ctrl Pts',(-7.83054820600006,15.2,-8.28268033700001));
#281198=CARTESIAN_POINT('Ctrl Pts',(-7.83054820600006,11.6,-8.28268033700001));
#281199=CARTESIAN_POINT('Ctrl Pts',(-7.82712268500006,15.2,-8.28131686600001));
#281200=CARTESIAN_POINT('Ctrl Pts',(-7.82712268500006,11.6,-8.28131686600001));
#281201=CARTESIAN_POINT('Ctrl Pts',(-7.82370242500006,15.2,-8.27995244400002));
#281202=CARTESIAN_POINT('Ctrl Pts',(-7.82370242500006,11.6,-8.27995244400002));
#281203=CARTESIAN_POINT('Ctrl Pts',(-7.82028743300006,15.2,-8.27858708000001));
#281204=CARTESIAN_POINT('Ctrl Pts',(-7.82028743300006,11.6,-8.27858708000001));
#281205=CARTESIAN_POINT('Ctrl Pts',(-7.81687771300006,15.2,-8.27722078100001));
#281206=CARTESIAN_POINT('Ctrl Pts',(-7.81687771300006,11.6,-8.27722078100001));
#281207=CARTESIAN_POINT('Ctrl Pts',(-7.81347326900006,15.2,-8.27585355600002));
#281208=CARTESIAN_POINT('Ctrl Pts',(-7.81347326900006,11.6,-8.27585355600002));
#281209=CARTESIAN_POINT('Ctrl Pts',(-7.81007410700005,15.2,-8.27448541300001));
#281210=CARTESIAN_POINT('Ctrl Pts',(-7.81007410700005,11.6,-8.27448541300001));
#281211=CARTESIAN_POINT('Ctrl Pts',(-7.80668023000005,15.2,-8.27311636000001));
#281212=CARTESIAN_POINT('Ctrl Pts',(-7.80668023000005,11.6,-8.27311636000001));
#281213=CARTESIAN_POINT('Ctrl Pts',(-7.80329164300006,15.2,-8.27174640500001));
#281214=CARTESIAN_POINT('Ctrl Pts',(-7.80329164300006,11.6,-8.27174640500001));
#281215=CARTESIAN_POINT('Ctrl Pts',(-7.79990835200006,15.2,-8.27037555700001));
#281216=CARTESIAN_POINT('Ctrl Pts',(-7.79990835200006,11.6,-8.27037555700001));
#281217=CARTESIAN_POINT('Ctrl Pts',(-7.79653036100005,15.2,-8.26900382300002));
#281218=CARTESIAN_POINT('Ctrl Pts',(-7.79653036100005,11.6,-8.26900382300002));
#281219=CARTESIAN_POINT('Ctrl Pts',(-7.79315767400006,15.2,-8.26763121300001));
#281220=CARTESIAN_POINT('Ctrl Pts',(-7.79315767400006,11.6,-8.26763121300001));
#281221=CARTESIAN_POINT('Ctrl Pts',(-7.78979029600006,15.2,-8.26625773300002));
#281222=CARTESIAN_POINT('Ctrl Pts',(-7.78979029600006,11.6,-8.26625773300002));
#281223=CARTESIAN_POINT('Ctrl Pts',(-7.78642823100006,15.2,-8.26488339200001));
#281224=CARTESIAN_POINT('Ctrl Pts',(-7.78642823100006,11.6,-8.26488339200001));
#281225=CARTESIAN_POINT('Ctrl Pts',(-7.78307148500006,15.2,-8.26350819900001));
#281226=CARTESIAN_POINT('Ctrl Pts',(-7.78307148500006,11.6,-8.26350819900001));
#281227=CARTESIAN_POINT('Ctrl Pts',(-7.77972006200006,15.2,-8.26213216200001));
#281228=CARTESIAN_POINT('Ctrl Pts',(-7.77972006200006,11.6,-8.26213216200001));
#281229=CARTESIAN_POINT('Ctrl Pts',(-7.77637396600006,15.2,-8.26075528800001));
#281230=CARTESIAN_POINT('Ctrl Pts',(-7.77637396600006,11.6,-8.26075528800001));
#281231=CARTESIAN_POINT('Ctrl Pts',(-7.77303320300006,15.2,-8.25937758700002));
#281232=CARTESIAN_POINT('Ctrl Pts',(-7.77303320300006,11.6,-8.25937758700002));
#281233=CARTESIAN_POINT('Ctrl Pts',(-7.76969777700005,15.2,-8.25799906700002));
#281234=CARTESIAN_POINT('Ctrl Pts',(-7.76969777700005,11.6,-8.25799906700002));
#281235=CARTESIAN_POINT('Ctrl Pts',(-7.76636769300006,15.2,-8.25661973600001));
#281236=CARTESIAN_POINT('Ctrl Pts',(-7.76636769300006,11.6,-8.25661973600001));
#281237=CARTESIAN_POINT('Ctrl Pts',(-7.76304295400006,15.2,-8.25523960300002));
#281238=CARTESIAN_POINT('Ctrl Pts',(-7.76304295400006,11.6,-8.25523960300002));
#281239=CARTESIAN_POINT('Ctrl Pts',(-7.75972356700006,15.2,-8.25385867500002));
#281240=CARTESIAN_POINT('Ctrl Pts',(-7.75972356700006,11.6,-8.25385867500002));
#281241=CARTESIAN_POINT('Ctrl Pts',(-7.75640953500006,15.2,-8.25247696200002));
#281242=CARTESIAN_POINT('Ctrl Pts',(-7.75640953500006,11.6,-8.25247696200002));
#281243=CARTESIAN_POINT('Ctrl Pts',(-7.75310086300006,15.2,-8.25109447100001));
#281244=CARTESIAN_POINT('Ctrl Pts',(-7.75310086300006,11.6,-8.25109447100001));
#281245=CARTESIAN_POINT('Ctrl Pts',(-7.74979755700006,15.2,-8.24971121200001));
#281246=CARTESIAN_POINT('Ctrl Pts',(-7.74979755700006,11.6,-8.24971121200001));
#281247=CARTESIAN_POINT('Ctrl Pts',(-7.74649962000005,15.2,-8.24832719300002));
#281248=CARTESIAN_POINT('Ctrl Pts',(-7.74649962000005,11.6,-8.24832719300002));
#281249=CARTESIAN_POINT('Ctrl Pts',(-7.74320705800006,15.2,-8.24694242100002));
#281250=CARTESIAN_POINT('Ctrl Pts',(-7.74320705800006,11.6,-8.24694242100002));
#281251=CARTESIAN_POINT('Ctrl Pts',(-7.73991987400005,15.2,-8.24555690600001));
#281252=CARTESIAN_POINT('Ctrl Pts',(-7.73991987400005,11.6,-8.24555690600001));
#281253=CARTESIAN_POINT('Ctrl Pts',(-7.73663807400006,15.2,-8.24417065600001));
#281254=CARTESIAN_POINT('Ctrl Pts',(-7.73663807400006,11.6,-8.24417065600001));
#281255=CARTESIAN_POINT('Ctrl Pts',(-7.73336166200006,15.2,-8.24278368100002));
#281256=CARTESIAN_POINT('Ctrl Pts',(-7.73336166200006,11.6,-8.24278368100002));
#281257=CARTESIAN_POINT('Ctrl Pts',(-7.73009064300006,15.2,-8.24139598700001));
#281258=CARTESIAN_POINT('Ctrl Pts',(-7.73009064300006,11.6,-8.24139598700001));
#281259=CARTESIAN_POINT('Ctrl Pts',(-7.72682502200006,15.2,-8.24000758400001));
#281260=CARTESIAN_POINT('Ctrl Pts',(-7.72682502200006,11.6,-8.24000758400001));
#281261=CARTESIAN_POINT('Ctrl Pts',(-7.72356480300005,15.2,-8.23861848000002));
#281262=CARTESIAN_POINT('Ctrl Pts',(-7.72356480300005,11.6,-8.23861848000002));
#281263=CARTESIAN_POINT('Ctrl Pts',(-7.72030999100006,15.2,-8.23722868500001));
#281264=CARTESIAN_POINT('Ctrl Pts',(-7.72030999100006,11.6,-8.23722868500001));
#281265=CARTESIAN_POINT('Ctrl Pts',(-7.71706059200006,15.2,-8.23583820700001));
#281266=CARTESIAN_POINT('Ctrl Pts',(-7.71706059200006,11.6,-8.23583820700001));
#281267=CARTESIAN_POINT('Ctrl Pts',(-7.71381660800006,15.2,-8.23444705300002));
#281268=CARTESIAN_POINT('Ctrl Pts',(-7.71381660800006,11.6,-8.23444705300002));
#281269=CARTESIAN_POINT('Ctrl Pts',(-7.71057804500006,15.2,-8.23305523500002));
#281270=CARTESIAN_POINT('Ctrl Pts',(-7.71057804500006,11.6,-8.23305523500002));
#281271=CARTESIAN_POINT('Ctrl Pts',(-7.70734490800006,15.2,-8.23166275800002));
#281272=CARTESIAN_POINT('Ctrl Pts',(-7.70734490800006,11.6,-8.23166275800002));
#281273=CARTESIAN_POINT('Ctrl Pts',(-7.70411720100006,15.2,-8.23026963400002));
#281274=CARTESIAN_POINT('Ctrl Pts',(-7.70411720100006,11.6,-8.23026963400002));
#281275=CARTESIAN_POINT('Ctrl Pts',(-7.70089493000006,15.2,-8.22887586900002));
#281276=CARTESIAN_POINT('Ctrl Pts',(-7.70089493000006,11.6,-8.22887586900002));
#281277=CARTESIAN_POINT('Ctrl Pts',(-7.69767809900006,15.2,-8.22748147300001));
#281278=CARTESIAN_POINT('Ctrl Pts',(-7.69767809900006,11.6,-8.22748147300001));
#281279=CARTESIAN_POINT('Ctrl Pts',(-7.69446671100006,15.2,-8.22608645500001));
#281280=CARTESIAN_POINT('Ctrl Pts',(-7.69446671100006,11.6,-8.22608645500001));
#281281=CARTESIAN_POINT('Ctrl Pts',(-7.69126077400006,15.2,-8.22469082400002));
#281282=CARTESIAN_POINT('Ctrl Pts',(-7.69126077400006,11.6,-8.22469082400002));
#281283=CARTESIAN_POINT('Ctrl Pts',(-7.68806028900006,15.2,-8.22329458900001));
#281284=CARTESIAN_POINT('Ctrl Pts',(-7.68806028900006,11.6,-8.22329458900001));
#281285=CARTESIAN_POINT('Ctrl Pts',(-7.68486526500006,15.2,-8.22189775700001));
#281286=CARTESIAN_POINT('Ctrl Pts',(-7.68486526500006,11.6,-8.22189775700001));
#281287=CARTESIAN_POINT('Ctrl Pts',(-7.68167570300006,15.2,-8.22050033900002));
#281288=CARTESIAN_POINT('Ctrl Pts',(-7.68167570300006,11.6,-8.22050033900002));
#281289=CARTESIAN_POINT('Ctrl Pts',(-7.67849160900005,15.2,-8.21910234200002));
#281290=CARTESIAN_POINT('Ctrl Pts',(-7.67849160900005,11.6,-8.21910234200002));
#281291=CARTESIAN_POINT('Ctrl Pts',(-7.67531298800006,15.2,-8.21770377700001));
#281292=CARTESIAN_POINT('Ctrl Pts',(-7.67531298800006,11.6,-8.21770377700001));
#281293=CARTESIAN_POINT('Ctrl Pts',(-7.67213984400006,15.2,-8.21630465100002));
#281294=CARTESIAN_POINT('Ctrl Pts',(-7.67213984400006,11.6,-8.21630465100002));
#281295=CARTESIAN_POINT('Ctrl Pts',(-7.66897218200006,15.2,-8.21490497400001));
#281296=CARTESIAN_POINT('Ctrl Pts',(-7.66897218200006,11.6,-8.21490497400001));
#281297=CARTESIAN_POINT('Ctrl Pts',(-7.66581000700005,15.2,-8.21350475500001));
#281298=CARTESIAN_POINT('Ctrl Pts',(-7.66581000700005,11.6,-8.21350475500001));
#281299=CARTESIAN_POINT('Ctrl Pts',(-7.66265332400006,15.2,-8.21210400200002));
#281300=CARTESIAN_POINT('Ctrl Pts',(-7.66265332400006,11.6,-8.21210400200002));
#281301=CARTESIAN_POINT('Ctrl Pts',(-7.65950213700006,15.2,-8.21070272500002));
#281302=CARTESIAN_POINT('Ctrl Pts',(-7.65950213700006,11.6,-8.21070272500002));
#281303=CARTESIAN_POINT('Ctrl Pts',(-7.65635645000006,15.2,-8.20930093200002));
#281304=CARTESIAN_POINT('Ctrl Pts',(-7.65635645000006,11.6,-8.20930093200002));
#281305=CARTESIAN_POINT('Ctrl Pts',(-7.65321627000005,15.2,-8.20789863500002));
#281306=CARTESIAN_POINT('Ctrl Pts',(-7.65321627000005,11.6,-8.20789863500002));
#281307=CARTESIAN_POINT('Ctrl Pts',(-7.65008160000006,15.2,-8.20649583800002));
#281308=CARTESIAN_POINT('Ctrl Pts',(-7.65008160000006,11.6,-8.20649583800002));
#281309=CARTESIAN_POINT('Ctrl Pts',(-7.64695244500006,15.2,-8.20509255500001));
#281310=CARTESIAN_POINT('Ctrl Pts',(-7.64695244500006,11.6,-8.20509255500001));
#281311=CARTESIAN_POINT('Ctrl Pts',(-7.64382881000006,15.2,-8.20368879300002));
#281312=CARTESIAN_POINT('Ctrl Pts',(-7.64382881000006,11.6,-8.20368879300002));
#281313=CARTESIAN_POINT('Ctrl Pts',(-7.64071069900006,15.2,-8.20228456000001));
#281314=CARTESIAN_POINT('Ctrl Pts',(-7.64071069900006,11.6,-8.20228456000001));
#281315=CARTESIAN_POINT('Ctrl Pts',(-7.63759811700006,15.2,-8.20087986700001));
#281316=CARTESIAN_POINT('Ctrl Pts',(-7.63759811700006,11.6,-8.20087986700001));
#281317=CARTESIAN_POINT('Ctrl Pts',(-7.63449107100006,15.2,-8.19947472200001));
#281318=CARTESIAN_POINT('Ctrl Pts',(-7.63449107100006,11.6,-8.19947472200001));
#281319=CARTESIAN_POINT('Ctrl Pts',(-7.63138956200006,15.2,-8.19806913500001));
#281320=CARTESIAN_POINT('Ctrl Pts',(-7.63138956200006,11.6,-8.19806913500001));
#281321=CARTESIAN_POINT('Ctrl Pts',(-7.62829359600006,15.2,-8.19666311500002));
#281322=CARTESIAN_POINT('Ctrl Pts',(-7.62829359600006,11.6,-8.19666311500002));
#281323=CARTESIAN_POINT('Ctrl Pts',(-7.62520317900006,15.2,-8.19525667200002));
#281324=CARTESIAN_POINT('Ctrl Pts',(-7.62520317900006,11.6,-8.19525667200002));
#281325=CARTESIAN_POINT('Ctrl Pts',(-7.62211831500006,15.2,-8.19384981300002));
#281326=CARTESIAN_POINT('Ctrl Pts',(-7.62211831500006,11.6,-8.19384981300002));
#281327=CARTESIAN_POINT('Ctrl Pts',(-7.61903900800006,15.2,-8.19244254900001));
#281328=CARTESIAN_POINT('Ctrl Pts',(-7.61903900800006,11.6,-8.19244254900001));
#281329=CARTESIAN_POINT('Ctrl Pts',(-7.61596526500006,15.2,-8.19103488900002));
#281330=CARTESIAN_POINT('Ctrl Pts',(-7.61596526500006,11.6,-8.19103488900002));
#281331=CARTESIAN_POINT('Ctrl Pts',(-7.61289708700006,15.2,-8.18962684300002));
#281332=CARTESIAN_POINT('Ctrl Pts',(-7.61289708700006,11.6,-8.18962684300002));
#281333=CARTESIAN_POINT('Ctrl Pts',(-7.60983448200006,15.2,-8.18821841900002));
#281334=CARTESIAN_POINT('Ctrl Pts',(-7.60983448200006,11.6,-8.18821841900002));
#281335=CARTESIAN_POINT('Ctrl Pts',(-7.60677745300006,15.2,-8.18680962700002));
#281336=CARTESIAN_POINT('Ctrl Pts',(-7.60677745300006,11.6,-8.18680962700002));
#281337=CARTESIAN_POINT('Ctrl Pts',(-7.60372600600006,15.2,-8.18540047600001));
#281338=CARTESIAN_POINT('Ctrl Pts',(-7.60372600600006,11.6,-8.18540047600001));
#281339=CARTESIAN_POINT('Ctrl Pts',(-7.60068014400006,15.2,-8.18399097600001));
#281340=CARTESIAN_POINT('Ctrl Pts',(-7.60068014400006,11.6,-8.18399097600001));
#281341=CARTESIAN_POINT('Ctrl Pts',(-7.59763987400006,15.2,-8.18258113800002));
#281342=CARTESIAN_POINT('Ctrl Pts',(-7.59763987400006,11.6,-8.18258113800002));
#281343=CARTESIAN_POINT('Ctrl Pts',(-7.59460519800006,15.2,-8.18117096700002));
#281344=CARTESIAN_POINT('Ctrl Pts',(-7.59460519800006,11.6,-8.18117096700002));
#281345=CARTESIAN_POINT('Ctrl Pts',(-7.59157612400006,15.2,-8.17976047600002));
#281346=CARTESIAN_POINT('Ctrl Pts',(-7.59157612400006,11.6,-8.17976047600002));
#281347=CARTESIAN_POINT('Ctrl Pts',(-7.58855265400006,15.2,-8.17834967500002));
#281348=CARTESIAN_POINT('Ctrl Pts',(-7.58855265400006,11.6,-8.17834967500002));
#281349=CARTESIAN_POINT('Ctrl Pts',(-7.58553479300006,15.2,-8.17693857100002));
#281350=CARTESIAN_POINT('Ctrl Pts',(-7.58553479300006,11.6,-8.17693857100002));
#281351=CARTESIAN_POINT('Ctrl Pts',(-7.58252254900006,15.2,-8.17552717500002));
#281352=CARTESIAN_POINT('Ctrl Pts',(-7.58252254900006,11.6,-8.17552717500002));
#281353=CARTESIAN_POINT('Ctrl Pts',(-7.57951592200006,15.2,-8.17411549700001));
#281354=CARTESIAN_POINT('Ctrl Pts',(-7.57951592200006,11.6,-8.17411549700001));
#281355=CARTESIAN_POINT('Ctrl Pts',(-7.57651492000005,15.2,-8.17270354500002));
#281356=CARTESIAN_POINT('Ctrl Pts',(-7.57651492000005,11.6,-8.17270354500002));
#281357=CARTESIAN_POINT('Ctrl Pts',(-7.57351954700006,15.2,-8.17129132900002));
#281358=CARTESIAN_POINT('Ctrl Pts',(-7.57351954700006,11.6,-8.17129132900002));
#281359=CARTESIAN_POINT('Ctrl Pts',(-7.57052980700006,15.2,-8.16987886100002));
#281360=CARTESIAN_POINT('Ctrl Pts',(-7.57052980700006,11.6,-8.16987886100002));
#281361=CARTESIAN_POINT('Ctrl Pts',(-7.56754570500006,15.2,-8.16846614700001));
#281362=CARTESIAN_POINT('Ctrl Pts',(-7.56754570500006,11.6,-8.16846614700001));
#281363=CARTESIAN_POINT('Ctrl Pts',(-7.56456724700006,15.2,-8.16705320000001));
#281364=CARTESIAN_POINT('Ctrl Pts',(-7.56456724700006,11.6,-8.16705320000001));
#281365=CARTESIAN_POINT('Ctrl Pts',(-7.56159443700006,15.2,-8.16564002700002));
#281366=CARTESIAN_POINT('Ctrl Pts',(-7.56159443700006,11.6,-8.16564002700002));
#281367=CARTESIAN_POINT('Ctrl Pts',(-7.55862727900006,15.2,-8.16422664000001));
#281368=CARTESIAN_POINT('Ctrl Pts',(-7.55862727900006,11.6,-8.16422664000001));
#281369=CARTESIAN_POINT('Ctrl Pts',(-7.55566577800005,15.2,-8.16281304700002));
#281370=CARTESIAN_POINT('Ctrl Pts',(-7.55566577800005,11.6,-8.16281304700002));
#281371=CARTESIAN_POINT('Ctrl Pts',(-7.55270994000006,15.2,-8.16139925900002));
#281372=CARTESIAN_POINT('Ctrl Pts',(-7.55270994000006,11.6,-8.16139925900002));
#281373=CARTESIAN_POINT('Ctrl Pts',(-7.54975976900005,15.2,-8.15998528500002));
#281374=CARTESIAN_POINT('Ctrl Pts',(-7.54975976900005,11.6,-8.15998528500002));
#281375=CARTESIAN_POINT('Ctrl Pts',(-7.54681526900006,15.2,-8.15857113500002));
#281376=CARTESIAN_POINT('Ctrl Pts',(-7.54681526900006,11.6,-8.15857113500002));
#281377=CARTESIAN_POINT('Ctrl Pts',(-7.54387644600006,15.2,-8.15715681800001));
#281378=CARTESIAN_POINT('Ctrl Pts',(-7.54387644600006,11.6,-8.15715681800001));
#281379=CARTESIAN_POINT('Ctrl Pts',(-7.54094330500005,15.2,-8.15574234600002));
#281380=CARTESIAN_POINT('Ctrl Pts',(-7.54094330500005,11.6,-8.15574234600002));
#281381=CARTESIAN_POINT('Ctrl Pts',(-7.53801584800006,15.2,-8.15432772800002));
#281382=CARTESIAN_POINT('Ctrl Pts',(-7.53801584800006,11.6,-8.15432772800002));
#281383=CARTESIAN_POINT('Ctrl Pts',(-7.53509408300006,15.2,-8.15291297300002));
#281384=CARTESIAN_POINT('Ctrl Pts',(-7.53509408300006,11.6,-8.15291297300002));
#281385=CARTESIAN_POINT('Ctrl Pts',(-7.53217801300006,15.2,-8.15149809200001));
#281386=CARTESIAN_POINT('Ctrl Pts',(-7.53217801300006,11.6,-8.15149809200001));
#281387=CARTESIAN_POINT('Ctrl Pts',(-7.52926764400006,15.2,-8.15008309300002));
#281388=CARTESIAN_POINT('Ctrl Pts',(-7.52926764400006,11.6,-8.15008309300002));
#281389=CARTESIAN_POINT('Ctrl Pts',(-7.52636298100006,15.2,-8.14866798900002));
#281390=CARTESIAN_POINT('Ctrl Pts',(-7.52636298100006,11.6,-8.14866798900002));
#281391=CARTESIAN_POINT('Ctrl Pts',(-7.52346402700006,15.2,-8.14725278900001));
#281392=CARTESIAN_POINT('Ctrl Pts',(-7.52346402700006,11.6,-8.14725278900001));
#281393=CARTESIAN_POINT('Ctrl Pts',(-7.52057078800006,15.2,-8.14583750100002));
#281394=CARTESIAN_POINT('Ctrl Pts',(-7.52057078800006,11.6,-8.14583750100002));
#281395=CARTESIAN_POINT('Ctrl Pts',(-7.51768326900006,15.2,-8.14442213800002));
#281396=CARTESIAN_POINT('Ctrl Pts',(-7.51768326900006,11.6,-8.14442213800002));
#281397=CARTESIAN_POINT('Ctrl Pts',(-7.51480147300006,15.2,-8.14300670900002));
#281398=CARTESIAN_POINT('Ctrl Pts',(-7.51480147300006,11.6,-8.14300670900002));
#281399=CARTESIAN_POINT('Ctrl Pts',(-7.51192540700006,15.2,-8.14159122300002));
#281400=CARTESIAN_POINT('Ctrl Pts',(-7.51192540700006,11.6,-8.14159122300002));
#281401=CARTESIAN_POINT('Ctrl Pts',(-7.50905507600006,15.2,-8.14017569100002));
#281402=CARTESIAN_POINT('Ctrl Pts',(-7.50905507600006,11.6,-8.14017569100002));
#281403=CARTESIAN_POINT('Ctrl Pts',(-7.50619048200006,15.2,-8.13876012300002));
#281404=CARTESIAN_POINT('Ctrl Pts',(-7.50619048200006,11.6,-8.13876012300002));
#281405=CARTESIAN_POINT('Ctrl Pts',(-7.50333163300006,15.2,-8.13734453000002));
#281406=CARTESIAN_POINT('Ctrl Pts',(-7.50333163300006,11.6,-8.13734453000002));
#281407=CARTESIAN_POINT('Ctrl Pts',(-7.50047853100006,15.2,-8.13592892200001));
#281408=CARTESIAN_POINT('Ctrl Pts',(-7.50047853100006,11.6,-8.13592892200001));
#281409=CARTESIAN_POINT('Ctrl Pts',(-7.49763118300006,15.2,-8.13451330800002));
#281410=CARTESIAN_POINT('Ctrl Pts',(-7.49763118300006,11.6,-8.13451330800002));
#281411=CARTESIAN_POINT('Ctrl Pts',(-7.49478959200006,15.2,-8.13309769900001));
#281412=CARTESIAN_POINT('Ctrl Pts',(-7.49478959200006,11.6,-8.13309769900001));
#281413=CARTESIAN_POINT('Ctrl Pts',(-7.49195376600006,15.2,-8.13168210600002));
#281414=CARTESIAN_POINT('Ctrl Pts',(-7.49195376600006,11.6,-8.13168210600002));
#281415=CARTESIAN_POINT('Ctrl Pts',(-7.48912370600006,15.2,-8.13026653800001));
#281416=CARTESIAN_POINT('Ctrl Pts',(-7.48912370600006,11.6,-8.13026653800001));
#281417=CARTESIAN_POINT('Ctrl Pts',(-7.48629941800006,15.2,-8.12885100600001));
#281418=CARTESIAN_POINT('Ctrl Pts',(-7.48629941800006,11.6,-8.12885100600001));
#281419=CARTESIAN_POINT('Ctrl Pts',(-7.48348090800006,15.2,-8.12743552100001));
#281420=CARTESIAN_POINT('Ctrl Pts',(-7.48348090800006,11.6,-8.12743552100001));
#281421=CARTESIAN_POINT('Ctrl Pts',(-7.48066818000006,15.2,-8.12602009200001));
#281422=CARTESIAN_POINT('Ctrl Pts',(-7.48066818000006,11.6,-8.12602009200001));
#281423=CARTESIAN_POINT('Ctrl Pts',(-7.47786123900006,15.2,-8.12460473100002));
#281424=CARTESIAN_POINT('Ctrl Pts',(-7.47786123900006,11.6,-8.12460473100002));
#281425=CARTESIAN_POINT('Ctrl Pts',(-7.47506009000006,15.2,-8.12318944700002));
#281426=CARTESIAN_POINT('Ctrl Pts',(-7.47506009000006,11.6,-8.12318944700002));
#281427=CARTESIAN_POINT('Ctrl Pts',(-7.47226473700006,15.2,-8.12177425100002));
#281428=CARTESIAN_POINT('Ctrl Pts',(-7.47226473700006,11.6,-8.12177425100002));
#281429=CARTESIAN_POINT('Ctrl Pts',(-7.46947518600006,15.2,-8.12035915500001));
#281430=CARTESIAN_POINT('Ctrl Pts',(-7.46947518600006,11.6,-8.12035915500001));
#281431=CARTESIAN_POINT('Ctrl Pts',(-7.46669144100006,15.2,-8.11894416700002));
#281432=CARTESIAN_POINT('Ctrl Pts',(-7.46669144100006,11.6,-8.11894416700002));
#281433=CARTESIAN_POINT('Ctrl Pts',(-7.46391350600006,15.2,-8.11752929900001));
#281434=CARTESIAN_POINT('Ctrl Pts',(-7.46391350600006,11.6,-8.11752929900001));
#281435=CARTESIAN_POINT('Ctrl Pts',(-7.46114138800006,15.2,-8.11611456100002));
#281436=CARTESIAN_POINT('Ctrl Pts',(-7.46114138800006,11.6,-8.11611456100002));
#281437=CARTESIAN_POINT('Ctrl Pts',(-7.45837509000006,15.2,-8.11469996500002));
#281438=CARTESIAN_POINT('Ctrl Pts',(-7.45837509000006,11.6,-8.11469996500002));
#281439=CARTESIAN_POINT('Ctrl Pts',(-7.45561461800006,15.2,-8.11328551900001));
#281440=CARTESIAN_POINT('Ctrl Pts',(-7.45561461800006,11.6,-8.11328551900001));
#281441=CARTESIAN_POINT('Ctrl Pts',(-7.45285997600006,15.2,-8.11187123600002));
#281442=CARTESIAN_POINT('Ctrl Pts',(-7.45285997600006,11.6,-8.11187123600002));
#281443=CARTESIAN_POINT('Ctrl Pts',(-7.45011117000006,15.2,-8.11045712500002));
#281444=CARTESIAN_POINT('Ctrl Pts',(-7.45011117000006,11.6,-8.11045712500002));
#281445=CARTESIAN_POINT('Ctrl Pts',(-7.44736820400006,15.2,-8.10904319800001));
#281446=CARTESIAN_POINT('Ctrl Pts',(-7.44736820400006,11.6,-8.10904319800001));
#281447=CARTESIAN_POINT('Ctrl Pts',(-7.44463108200006,15.2,-8.10762946600001));
#281448=CARTESIAN_POINT('Ctrl Pts',(-7.44463108200006,11.6,-8.10762946600001));
#281449=CARTESIAN_POINT('Ctrl Pts',(-7.44189981100006,15.2,-8.10621593800001));
#281450=CARTESIAN_POINT('Ctrl Pts',(-7.44189981100006,11.6,-8.10621593800001));
#281451=CARTESIAN_POINT('Ctrl Pts',(-7.43917439300006,15.2,-8.10480262600001));
#281452=CARTESIAN_POINT('Ctrl Pts',(-7.43917439300006,11.6,-8.10480262600001));
#281453=CARTESIAN_POINT('Ctrl Pts',(-7.43645483600006,15.2,-8.10338954200001));
#281454=CARTESIAN_POINT('Ctrl Pts',(-7.43645483600006,11.6,-8.10338954200001));
#281455=CARTESIAN_POINT('Ctrl Pts',(-7.43374114300006,15.2,-8.10197669500001));
#281456=CARTESIAN_POINT('Ctrl Pts',(-7.43374114300006,11.6,-8.10197669500001));
#281457=CARTESIAN_POINT('Ctrl Pts',(-7.43103332000006,15.2,-8.10056409500002));
#281458=CARTESIAN_POINT('Ctrl Pts',(-7.43103332000006,11.6,-8.10056409500002));
#281459=CARTESIAN_POINT('Ctrl Pts',(-7.42833137000006,15.2,-8.09915175500001));
#281460=CARTESIAN_POINT('Ctrl Pts',(-7.42833137000006,11.6,-8.09915175500001));
#281461=CARTESIAN_POINT('Ctrl Pts',(-7.42563529900006,15.2,-8.09773968600001));
#281462=CARTESIAN_POINT('Ctrl Pts',(-7.42563529900006,11.6,-8.09773968600001));
#281463=CARTESIAN_POINT('Ctrl Pts',(-7.42294511200006,15.2,-8.09632789700002));
#281464=CARTESIAN_POINT('Ctrl Pts',(-7.42294511200006,11.6,-8.09632789700002));
#281465=CARTESIAN_POINT('Ctrl Pts',(-7.42026081300006,15.2,-8.09491640100001));
#281466=CARTESIAN_POINT('Ctrl Pts',(-7.42026081300006,11.6,-8.09491640100001));
#281467=CARTESIAN_POINT('Ctrl Pts',(-7.41758240900006,15.2,-8.09350520800002));
#281468=CARTESIAN_POINT('Ctrl Pts',(-7.41758240900006,11.6,-8.09350520800002));
#281469=CARTESIAN_POINT('Ctrl Pts',(-7.41490990300006,15.2,-8.09209433000002));
#281470=CARTESIAN_POINT('Ctrl Pts',(-7.41490990300006,11.6,-8.09209433000002));
#281471=CARTESIAN_POINT('Ctrl Pts',(-7.41224330000006,15.2,-8.09068377600001));
#281472=CARTESIAN_POINT('Ctrl Pts',(-7.41224330000006,11.6,-8.09068377600001));
#281473=CARTESIAN_POINT('Ctrl Pts',(-7.40958260500006,15.2,-8.08927355900002));
#281474=CARTESIAN_POINT('Ctrl Pts',(-7.40958260500006,11.6,-8.08927355900002));
#281475=CARTESIAN_POINT('Ctrl Pts',(-7.40692782300005,15.2,-8.08786369000002));
#281476=CARTESIAN_POINT('Ctrl Pts',(-7.40692782300005,11.6,-8.08786369000002));
#281477=CARTESIAN_POINT('Ctrl Pts',(-7.40427895900006,15.2,-8.08645417900001));
#281478=CARTESIAN_POINT('Ctrl Pts',(-7.40427895900006,11.6,-8.08645417900001));
#281479=CARTESIAN_POINT('Ctrl Pts',(-7.40163601900006,15.2,-8.08504503800001));
#281480=CARTESIAN_POINT('Ctrl Pts',(-7.40163601900006,11.6,-8.08504503800001));
#281481=CARTESIAN_POINT('Ctrl Pts',(-7.39899900500006,15.2,-8.08363627800002));
#281482=CARTESIAN_POINT('Ctrl Pts',(-7.39899900500006,11.6,-8.08363627800002));
#281483=CARTESIAN_POINT('Ctrl Pts',(-7.39636792500006,15.2,-8.08222791100001));
#281484=CARTESIAN_POINT('Ctrl Pts',(-7.39636792500006,11.6,-8.08222791100001));
#281485=CARTESIAN_POINT('Ctrl Pts',(-7.39374278200006,15.2,-8.08081994600002));
#281486=CARTESIAN_POINT('Ctrl Pts',(-7.39374278200006,11.6,-8.08081994600002));
#281487=CARTESIAN_POINT('Ctrl Pts',(-7.39112358200006,15.2,-8.07941239800002));
#281488=CARTESIAN_POINT('Ctrl Pts',(-7.39112358200006,11.6,-8.07941239800002));
#281489=CARTESIAN_POINT('Ctrl Pts',(-7.38851032900006,15.2,-8.07800527400002));
#281490=CARTESIAN_POINT('Ctrl Pts',(-7.38851032900006,11.6,-8.07800527400002));
#281491=CARTESIAN_POINT('Ctrl Pts',(-7.38590302800006,15.2,-8.07659859000001));
#281492=CARTESIAN_POINT('Ctrl Pts',(-7.38590302800006,11.6,-8.07659859000001));
#281493=CARTESIAN_POINT('Ctrl Pts',(-7.38330168300006,15.2,-8.07519235400001));
#281494=CARTESIAN_POINT('Ctrl Pts',(-7.38330168300006,11.6,-8.07519235400001));
#281495=CARTESIAN_POINT('Ctrl Pts',(-7.38070630100006,15.2,-8.07378657700001));
#281496=CARTESIAN_POINT('Ctrl Pts',(-7.38070630100006,11.6,-8.07378657700001));
#281497=CARTESIAN_POINT('Ctrl Pts',(-7.37811688700006,15.2,-8.07238127400002));
#281498=CARTESIAN_POINT('Ctrl Pts',(-7.37811688700006,11.6,-8.07238127400002));
#281499=CARTESIAN_POINT('Ctrl Pts',(-7.37553344400006,15.2,-8.07097645400002));
#281500=CARTESIAN_POINT('Ctrl Pts',(-7.37553344400006,11.6,-8.07097645400002));
#281501=CARTESIAN_POINT('Ctrl Pts',(-7.37295597700006,15.2,-8.06957212800001));
#281502=CARTESIAN_POINT('Ctrl Pts',(-7.37295597700006,11.6,-8.06957212800001));
#281503=CARTESIAN_POINT('Ctrl Pts',(-7.37038449300006,15.2,-8.06816830900001));
#281504=CARTESIAN_POINT('Ctrl Pts',(-7.37038449300006,11.6,-8.06816830900001));
#281505=CARTESIAN_POINT('Ctrl Pts',(-7.36781899500006,15.2,-8.06676500900002));
#281506=CARTESIAN_POINT('Ctrl Pts',(-7.36781899500006,11.6,-8.06676500900002));
#281507=CARTESIAN_POINT('Ctrl Pts',(-7.36525948900006,15.2,-8.06536223600002));
#281508=CARTESIAN_POINT('Ctrl Pts',(-7.36525948900006,11.6,-8.06536223600002));
#281509=CARTESIAN_POINT('Ctrl Pts',(-7.36270597800006,15.2,-8.06396000700002));
#281510=CARTESIAN_POINT('Ctrl Pts',(-7.36270597800006,11.6,-8.06396000700002));
#281511=CARTESIAN_POINT('Ctrl Pts',(-7.36015847000006,15.2,-8.06255832900002));
#281512=CARTESIAN_POINT('Ctrl Pts',(-7.36015847000006,11.6,-8.06255832900002));
#281513=CARTESIAN_POINT('Ctrl Pts',(-7.35761696800005,15.2,-8.06115721700002));
#281514=CARTESIAN_POINT('Ctrl Pts',(-7.35761696800005,11.6,-8.06115721700002));
#281515=CARTESIAN_POINT('Ctrl Pts',(-7.35508147700005,15.2,-8.05975668000002));
#281516=CARTESIAN_POINT('Ctrl Pts',(-7.35508147700005,11.6,-8.05975668000002));
#281517=CARTESIAN_POINT('Ctrl Pts',(-7.35255200200006,15.2,-8.05835673200002));
#281518=CARTESIAN_POINT('Ctrl Pts',(-7.35255200200006,11.6,-8.05835673200002));
#281519=CARTESIAN_POINT('Ctrl Pts',(-7.35002854900006,15.2,-8.05695738400001));
#281520=CARTESIAN_POINT('Ctrl Pts',(-7.35002854900006,11.6,-8.05695738400001));
#281521=CARTESIAN_POINT('Ctrl Pts',(-7.34751112100006,15.2,-8.05555864700001));
#281522=CARTESIAN_POINT('Ctrl Pts',(-7.34751112100006,11.6,-8.05555864700001));
#281523=CARTESIAN_POINT('Ctrl Pts',(-7.34499972500006,15.2,-8.05416053400002));
#281524=CARTESIAN_POINT('Ctrl Pts',(-7.34499972500006,11.6,-8.05416053400002));
#281525=CARTESIAN_POINT('Ctrl Pts',(-7.34249436400006,15.2,-8.05276305700002));
#281526=CARTESIAN_POINT('Ctrl Pts',(-7.34249436400006,11.6,-8.05276305700002));
#281527=CARTESIAN_POINT('Ctrl Pts',(-7.33999504500006,15.2,-8.05136622600001));
#281528=CARTESIAN_POINT('Ctrl Pts',(-7.33999504500006,11.6,-8.05136622600001));
#281529=CARTESIAN_POINT('Ctrl Pts',(-7.33750177100006,15.2,-8.04997005600002));
#281530=CARTESIAN_POINT('Ctrl Pts',(-7.33750177100006,11.6,-8.04997005600002));
#281531=CARTESIAN_POINT('Ctrl Pts',(-7.33501454800006,15.2,-8.04857455600001));
#281532=CARTESIAN_POINT('Ctrl Pts',(-7.33501454800006,11.6,-8.04857455600001));
#281533=CARTESIAN_POINT('Ctrl Pts',(-7.33253338100006,15.2,-8.04717974000001));
#281534=CARTESIAN_POINT('Ctrl Pts',(-7.33253338100006,11.6,-8.04717974000001));
#281535=CARTESIAN_POINT('Ctrl Pts',(-7.33005827500006,15.2,-8.04578561900002));
#281536=CARTESIAN_POINT('Ctrl Pts',(-7.33005827500006,11.6,-8.04578561900002));
#281537=CARTESIAN_POINT('Ctrl Pts',(-7.32758923400006,15.2,-8.04439220600001));
#281538=CARTESIAN_POINT('Ctrl Pts',(-7.32758923400006,11.6,-8.04439220600001));
#281539=CARTESIAN_POINT('Ctrl Pts',(-7.32512626500006,15.2,-8.04299951200001));
#281540=CARTESIAN_POINT('Ctrl Pts',(-7.32512626500006,11.6,-8.04299951200001));
#281541=CARTESIAN_POINT('Ctrl Pts',(-7.32266937000006,15.2,-8.04160755000002));
#281542=CARTESIAN_POINT('Ctrl Pts',(-7.32266937000006,11.6,-8.04160755000002));
#281543=CARTESIAN_POINT('Ctrl Pts',(-7.32021855600006,15.2,-8.04021633200002));
#281544=CARTESIAN_POINT('Ctrl Pts',(-7.32021855600006,11.6,-8.04021633200002));
#281545=CARTESIAN_POINT('Ctrl Pts',(-7.31777382800006,15.2,-8.03882587000002));
#281546=CARTESIAN_POINT('Ctrl Pts',(-7.31777382800006,11.6,-8.03882587000002));
#281547=CARTESIAN_POINT('Ctrl Pts',(-7.31533519000005,15.2,-8.03743617600002));
#281548=CARTESIAN_POINT('Ctrl Pts',(-7.31533519000005,11.6,-8.03743617600002));
#281549=CARTESIAN_POINT('Ctrl Pts',(-7.31290264900006,15.2,-8.03604726400001));
#281550=CARTESIAN_POINT('Ctrl Pts',(-7.31290264900006,11.6,-8.03604726400001));
#281551=CARTESIAN_POINT('Ctrl Pts',(-7.31047620800005,15.2,-8.03465914400002));
#281552=CARTESIAN_POINT('Ctrl Pts',(-7.31047620800005,11.6,-8.03465914400002));
#281553=CARTESIAN_POINT('Ctrl Pts',(-7.30805587300006,15.2,-8.03327182900002));
#281554=CARTESIAN_POINT('Ctrl Pts',(-7.30805587300006,11.6,-8.03327182900002));
#281555=CARTESIAN_POINT('Ctrl Pts',(-7.30564164700006,15.2,-8.03188533200002));
#281556=CARTESIAN_POINT('Ctrl Pts',(-7.30564164700006,11.6,-8.03188533200002));
#281557=CARTESIAN_POINT('Ctrl Pts',(-7.30323353700006,15.2,-8.03049966500001));
#281558=CARTESIAN_POINT('Ctrl Pts',(-7.30323353700006,11.6,-8.03049966500001));
#281559=CARTESIAN_POINT('Ctrl Pts',(-7.30083154800006,15.2,-8.02911484100001));
#281560=CARTESIAN_POINT('Ctrl Pts',(-7.30083154800006,11.6,-8.02911484100001));
#281561=CARTESIAN_POINT('Ctrl Pts',(-7.29843568500006,15.2,-8.02773087300002));
#281562=CARTESIAN_POINT('Ctrl Pts',(-7.29843568500006,11.6,-8.02773087300002));
#281563=CARTESIAN_POINT('Ctrl Pts',(-7.29604595200006,15.2,-8.02634777100002));
#281564=CARTESIAN_POINT('Ctrl Pts',(-7.29604595200006,11.6,-8.02634777100002));
#281565=CARTESIAN_POINT('Ctrl Pts',(-7.29366235400006,15.2,-8.02496555000002));
#281566=CARTESIAN_POINT('Ctrl Pts',(-7.29366235400006,11.6,-8.02496555000002));
#281567=CARTESIAN_POINT('Ctrl Pts',(-7.29128489700006,15.2,-8.02358422100001));
#281568=CARTESIAN_POINT('Ctrl Pts',(-7.29128489700006,11.6,-8.02358422100001));
#281569=CARTESIAN_POINT('Ctrl Pts',(-7.28891358600006,15.2,-8.02220379800002));
#281570=CARTESIAN_POINT('Ctrl Pts',(-7.28891358600006,11.6,-8.02220379800002));
#281571=CARTESIAN_POINT('Ctrl Pts',(-7.28654842500006,15.2,-8.02082429200001));
#281572=CARTESIAN_POINT('Ctrl Pts',(-7.28654842500006,11.6,-8.02082429200001));
#281573=CARTESIAN_POINT('Ctrl Pts',(-7.28418942000006,15.2,-8.01944571800002));
#281574=CARTESIAN_POINT('Ctrl Pts',(-7.28418942000006,11.6,-8.01944571800002));
#281575=CARTESIAN_POINT('Ctrl Pts',(-7.28183657600006,15.2,-8.01806808600002));
#281576=CARTESIAN_POINT('Ctrl Pts',(-7.28183657600006,11.6,-8.01806808600002));
#281577=CARTESIAN_POINT('Ctrl Pts',(-7.27948989700006,15.2,-8.01669141200002));
#281578=CARTESIAN_POINT('Ctrl Pts',(-7.27948989700006,11.6,-8.01669141200002));
#281579=CARTESIAN_POINT('Ctrl Pts',(-7.27714938800006,15.2,-8.01531570600002));
#281580=CARTESIAN_POINT('Ctrl Pts',(-7.27714938800006,11.6,-8.01531570600002));
#281581=CARTESIAN_POINT('Ctrl Pts',(-7.27481505600006,15.2,-8.01394098200002));
#281582=CARTESIAN_POINT('Ctrl Pts',(-7.27481505600006,11.6,-8.01394098200002));
#281583=CARTESIAN_POINT('Ctrl Pts',(-7.27248690400006,15.2,-8.01256725300002));
#281584=CARTESIAN_POINT('Ctrl Pts',(-7.27248690400006,11.6,-8.01256725300002));
#281585=CARTESIAN_POINT('Ctrl Pts',(-7.27016493900006,15.2,-8.01119453200002));
#281586=CARTESIAN_POINT('Ctrl Pts',(-7.27016493900006,11.6,-8.01119453200002));
#281587=CARTESIAN_POINT('Ctrl Pts',(-7.26784916400006,15.2,-8.00982283100002));
#281588=CARTESIAN_POINT('Ctrl Pts',(-7.26784916400006,11.6,-8.00982283100002));
#281589=CARTESIAN_POINT('Ctrl Pts',(-7.26553958500006,15.2,-8.00845216300001));
#281590=CARTESIAN_POINT('Ctrl Pts',(-7.26553958500006,11.6,-8.00845216300001));
#281591=CARTESIAN_POINT('Ctrl Pts',(-7.26323620700006,15.2,-8.00708254200002));
#281592=CARTESIAN_POINT('Ctrl Pts',(-7.26323620700006,11.6,-8.00708254200002));
#281593=CARTESIAN_POINT('Ctrl Pts',(-7.26093903400006,15.2,-8.00571398200002));
#281594=CARTESIAN_POINT('Ctrl Pts',(-7.26093903400006,11.6,-8.00571398200002));
#281595=CARTESIAN_POINT('Ctrl Pts',(-7.25864807300006,15.2,-8.00434649300002));
#281596=CARTESIAN_POINT('Ctrl Pts',(-7.25864807300006,11.6,-8.00434649300002));
#281597=CARTESIAN_POINT('Ctrl Pts',(-7.25636332800006,15.2,-8.00298009100001));
#281598=CARTESIAN_POINT('Ctrl Pts',(-7.25636332800006,11.6,-8.00298009100001));
#281599=CARTESIAN_POINT('Ctrl Pts',(-7.25408480500006,15.2,-8.00161478700002));
#281600=CARTESIAN_POINT('Ctrl Pts',(-7.25408480500006,11.6,-8.00161478700002));
#281601=CARTESIAN_POINT('Ctrl Pts',(-7.25181250700006,15.2,-8.00025059700002));
#281602=CARTESIAN_POINT('Ctrl Pts',(-7.25181250700006,11.6,-8.00025059700002));
#281603=CARTESIAN_POINT('Ctrl Pts',(-7.24954644200006,15.2,-7.99888753100002));
#281604=CARTESIAN_POINT('Ctrl Pts',(-7.24954644200006,11.6,-7.99888753100002));
#281605=CARTESIAN_POINT('Ctrl Pts',(-7.24728661100006,15.2,-7.99752560500002));
#281606=CARTESIAN_POINT('Ctrl Pts',(-7.24728661100006,11.6,-7.99752560500002));
#281607=CARTESIAN_POINT('Ctrl Pts',(-7.24503302300006,15.2,-7.99616483000002));
#281608=CARTESIAN_POINT('Ctrl Pts',(-7.24503302300006,11.6,-7.99616483000002));
#281609=CARTESIAN_POINT('Ctrl Pts',(-7.24278568100006,15.2,-7.99480522100002));
#281610=CARTESIAN_POINT('Ctrl Pts',(-7.24278568100006,11.6,-7.99480522100002));
#281611=CARTESIAN_POINT('Ctrl Pts',(-7.24054459100006,15.2,-7.99344679100002));
#281612=CARTESIAN_POINT('Ctrl Pts',(-7.24054459100006,11.6,-7.99344679100002));
#281613=CARTESIAN_POINT('Ctrl Pts',(-7.23830975800006,15.2,-7.99208955400001));
#281614=CARTESIAN_POINT('Ctrl Pts',(-7.23830975800006,11.6,-7.99208955400001));
#281615=CARTESIAN_POINT('Ctrl Pts',(-7.23608118600006,15.2,-7.99073352300002));
#281616=CARTESIAN_POINT('Ctrl Pts',(-7.23608118600006,11.6,-7.99073352300002));
#281617=CARTESIAN_POINT('Ctrl Pts',(-7.23385888100006,15.2,-7.98937871000001));
#281618=CARTESIAN_POINT('Ctrl Pts',(-7.23385888100006,11.6,-7.98937871000001));
#281619=CARTESIAN_POINT('Ctrl Pts',(-7.23164285000006,15.2,-7.98802513000001));
#281620=CARTESIAN_POINT('Ctrl Pts',(-7.23164285000006,11.6,-7.98802513000001));
#281621=CARTESIAN_POINT('Ctrl Pts',(-7.22943309400006,15.2,-7.98667279800001));
#281622=CARTESIAN_POINT('Ctrl Pts',(-7.22943309400006,11.6,-7.98667279800001));
#281623=CARTESIAN_POINT('Ctrl Pts',(-7.22722962100006,15.2,-7.98532172500002));
#281624=CARTESIAN_POINT('Ctrl Pts',(-7.22722962100006,11.6,-7.98532172500002));
#281625=CARTESIAN_POINT('Ctrl Pts',(-7.22503243500006,15.2,-7.98397192600002));
#281626=CARTESIAN_POINT('Ctrl Pts',(-7.22503243500006,11.6,-7.98397192600002));
#281627=CARTESIAN_POINT('Ctrl Pts',(-7.22284154100006,15.2,-7.98262341500001));
#281628=CARTESIAN_POINT('Ctrl Pts',(-7.22284154100006,11.6,-7.98262341500001));
#281629=CARTESIAN_POINT('Ctrl Pts',(-7.22065694500006,15.2,-7.98127620500001));
#281630=CARTESIAN_POINT('Ctrl Pts',(-7.22065694500006,11.6,-7.98127620500001));
#281631=CARTESIAN_POINT('Ctrl Pts',(-7.21847865200006,15.2,-7.97993031000002));
#281632=CARTESIAN_POINT('Ctrl Pts',(-7.21847865200006,11.6,-7.97993031000002));
#281633=CARTESIAN_POINT('Ctrl Pts',(-7.21630666700006,15.2,-7.97858574400002));
#281634=CARTESIAN_POINT('Ctrl Pts',(-7.21630666700006,11.6,-7.97858574400002));
#281635=CARTESIAN_POINT('Ctrl Pts',(-7.21414099500006,15.2,-7.97724252200001));
#281636=CARTESIAN_POINT('Ctrl Pts',(-7.21414099500006,11.6,-7.97724252200001));
#281637=CARTESIAN_POINT('Ctrl Pts',(-7.21198164100006,15.2,-7.97590065400002));
#281638=CARTESIAN_POINT('Ctrl Pts',(-7.21198164100006,11.6,-7.97590065400002));
#281639=CARTESIAN_POINT('Ctrl Pts',(-7.20982861000006,15.2,-7.97456016000002));
#281640=CARTESIAN_POINT('Ctrl Pts',(-7.20982861000006,11.6,-7.97456016000002));
#281641=CARTESIAN_POINT('Ctrl Pts',(-7.20768190700006,15.2,-7.97322104900001));
#281642=CARTESIAN_POINT('Ctrl Pts',(-7.20768190700006,11.6,-7.97322104900001));
#281643=CARTESIAN_POINT('Ctrl Pts',(-7.20554153900006,15.2,-7.97188333700002));
#281644=CARTESIAN_POINT('Ctrl Pts',(-7.20554153900006,11.6,-7.97188333700002));
#281645=CARTESIAN_POINT('Ctrl Pts',(-7.20340750800006,15.2,-7.97054703800002));
#281646=CARTESIAN_POINT('Ctrl Pts',(-7.20340750800006,11.6,-7.97054703800002));
#281647=CARTESIAN_POINT('Ctrl Pts',(-7.20127982200006,15.2,-7.96921216600002));
#281648=CARTESIAN_POINT('Ctrl Pts',(-7.20127982200006,11.6,-7.96921216600002));
#281649=CARTESIAN_POINT('Ctrl Pts',(-7.19915848500006,15.2,-7.96787873500002));
#281650=CARTESIAN_POINT('Ctrl Pts',(-7.19915848500006,11.6,-7.96787873500002));
#281651=CARTESIAN_POINT('Ctrl Pts',(-7.19704350100006,15.2,-7.96654675900001));
#281652=CARTESIAN_POINT('Ctrl Pts',(-7.19704350100006,11.6,-7.96654675900001));
#281653=CARTESIAN_POINT('Ctrl Pts',(-7.19493487700006,15.2,-7.96521625400001));
#281654=CARTESIAN_POINT('Ctrl Pts',(-7.19493487700006,11.6,-7.96521625400001));
#281655=CARTESIAN_POINT('Ctrl Pts',(-7.19283261800006,15.2,-7.96388723200002));
#281656=CARTESIAN_POINT('Ctrl Pts',(-7.19283261800006,11.6,-7.96388723200002));
#281657=CARTESIAN_POINT('Ctrl Pts',(-7.19073672800006,15.2,-7.96255970800001));
#281658=CARTESIAN_POINT('Ctrl Pts',(-7.19073672800006,11.6,-7.96255970800001));
#281659=CARTESIAN_POINT('Ctrl Pts',(-7.18864721300006,15.2,-7.96123369700001));
#281660=CARTESIAN_POINT('Ctrl Pts',(-7.18864721300006,11.6,-7.96123369700001));
#281661=CARTESIAN_POINT('Ctrl Pts',(-7.18656407900006,15.2,-7.95990921400002));
#281662=CARTESIAN_POINT('Ctrl Pts',(-7.18656407900006,11.6,-7.95990921400002));
#281663=CARTESIAN_POINT('Ctrl Pts',(-7.18448732900006,15.2,-7.95858627200002));
#281664=CARTESIAN_POINT('Ctrl Pts',(-7.18448732900006,11.6,-7.95858627200002));
#281665=CARTESIAN_POINT('Ctrl Pts',(-7.18241697000006,15.2,-7.95726488600002));
#281666=CARTESIAN_POINT('Ctrl Pts',(-7.18241697000006,11.6,-7.95726488600002));
#281667=CARTESIAN_POINT('Ctrl Pts',(-7.18035300600006,15.2,-7.95594507100001));
#281668=CARTESIAN_POINT('Ctrl Pts',(-7.18035300600006,11.6,-7.95594507100001));
#281669=CARTESIAN_POINT('Ctrl Pts',(-7.17829544400006,15.2,-7.95462684200002));
#281670=CARTESIAN_POINT('Ctrl Pts',(-7.17829544400006,11.6,-7.95462684200002));
#281671=CARTESIAN_POINT('Ctrl Pts',(-7.17624428700006,15.2,-7.95331021100001));
#281672=CARTESIAN_POINT('Ctrl Pts',(-7.17624428700006,11.6,-7.95331021100001));
#281673=CARTESIAN_POINT('Ctrl Pts',(-7.17419954100006,15.2,-7.95199519700001));
#281674=CARTESIAN_POINT('Ctrl Pts',(-7.17419954100006,11.6,-7.95199519700001));
#281675=CARTESIAN_POINT('Ctrl Pts',(-7.17216121300006,15.2,-7.95068181000002));
#281676=CARTESIAN_POINT('Ctrl Pts',(-7.17216121300006,11.6,-7.95068181000002));
#281677=CARTESIAN_POINT('Ctrl Pts',(-7.17012930600006,15.2,-7.94937007000001));
#281678=CARTESIAN_POINT('Ctrl Pts',(-7.17012930600006,11.6,-7.94937007000001));
#281679=CARTESIAN_POINT('Ctrl Pts',(-7.16810382600006,15.2,-7.94805998700002));
#281680=CARTESIAN_POINT('Ctrl Pts',(-7.16810382600006,11.6,-7.94805998700002));
#281681=CARTESIAN_POINT('Ctrl Pts',(-7.16608477700006,15.2,-7.94675157900001));
#281682=CARTESIAN_POINT('Ctrl Pts',(-7.16608477700006,11.6,-7.94675157900001));
#281683=CARTESIAN_POINT('Ctrl Pts',(-7.16407216700006,15.2,-7.94544485900002));
#281684=CARTESIAN_POINT('Ctrl Pts',(-7.16407216700006,11.6,-7.94544485900002));
#281685=CARTESIAN_POINT('Ctrl Pts',(-7.16206599800006,15.2,-7.94413984400002));
#281686=CARTESIAN_POINT('Ctrl Pts',(-7.16206599800006,11.6,-7.94413984400002));
#281687=CARTESIAN_POINT('Ctrl Pts',(-7.16006627800006,15.2,-7.94283654700001));
#281688=CARTESIAN_POINT('Ctrl Pts',(-7.16006627800006,11.6,-7.94283654700001));
#281689=CARTESIAN_POINT('Ctrl Pts',(-7.15807301100006,15.2,-7.94153498400001));
#281690=CARTESIAN_POINT('Ctrl Pts',(-7.15807301100006,11.6,-7.94153498400001));
#281691=CARTESIAN_POINT('Ctrl Pts',(-7.15608620200006,15.2,-7.94023517100002));
#281692=CARTESIAN_POINT('Ctrl Pts',(-7.15608620200006,11.6,-7.94023517100002));
#281693=CARTESIAN_POINT('Ctrl Pts',(-7.15410585700006,15.2,-7.93893712100001));
#281694=CARTESIAN_POINT('Ctrl Pts',(-7.15410585700006,11.6,-7.93893712100001));
#281695=CARTESIAN_POINT('Ctrl Pts',(-7.15213198100006,15.2,-7.93764085100002));
#281696=CARTESIAN_POINT('Ctrl Pts',(-7.15213198100006,11.6,-7.93764085100002));
#281697=CARTESIAN_POINT('Ctrl Pts',(-7.15016457900005,15.2,-7.93634637500002));
#281698=CARTESIAN_POINT('Ctrl Pts',(-7.15016457900005,11.6,-7.93634637500002));
#281699=CARTESIAN_POINT('Ctrl Pts',(-7.14820365700006,15.2,-7.93505371000002));
#281700=CARTESIAN_POINT('Ctrl Pts',(-7.14820365700006,11.6,-7.93505371000002));
#281701=CARTESIAN_POINT('Ctrl Pts',(-7.14624921900006,15.2,-7.93376287100001));
#281702=CARTESIAN_POINT('Ctrl Pts',(-7.14624921900006,11.6,-7.93376287100001));
#281703=CARTESIAN_POINT('Ctrl Pts',(-7.14430127000006,15.2,-7.93247387100001));
#281704=CARTESIAN_POINT('Ctrl Pts',(-7.14430127000006,11.6,-7.93247387100001));
#281705=CARTESIAN_POINT('Ctrl Pts',(-7.14235981800006,15.2,-7.93118672800002));
#281706=CARTESIAN_POINT('Ctrl Pts',(-7.14235981800006,11.6,-7.93118672800002));
#281707=CARTESIAN_POINT('Ctrl Pts',(-7.14042486500006,15.2,-7.92990145700001));
#281708=CARTESIAN_POINT('Ctrl Pts',(-7.14042486500006,11.6,-7.92990145700001));
#281709=CARTESIAN_POINT('Ctrl Pts',(-7.13849641900006,15.2,-7.92861807300002));
#281710=CARTESIAN_POINT('Ctrl Pts',(-7.13849641900006,11.6,-7.92861807300002));
#281711=CARTESIAN_POINT('Ctrl Pts',(-7.13657448400006,15.2,-7.92733659100002));
#281712=CARTESIAN_POINT('Ctrl Pts',(-7.13657448400006,11.6,-7.92733659100002));
#281713=CARTESIAN_POINT('Ctrl Pts',(-7.13465906500006,15.2,-7.92605702900002));
#281714=CARTESIAN_POINT('Ctrl Pts',(-7.13465906500006,11.6,-7.92605702900002));
#281715=CARTESIAN_POINT('Ctrl Pts',(-7.13275016800006,15.2,-7.92477940100002));
#281716=CARTESIAN_POINT('Ctrl Pts',(-7.13275016800006,11.6,-7.92477940100002));
#281717=CARTESIAN_POINT('Ctrl Pts',(-7.13084779900006,15.2,-7.92350372200002));
#281718=CARTESIAN_POINT('Ctrl Pts',(-7.13084779900006,11.6,-7.92350372200002));
#281719=CARTESIAN_POINT('Ctrl Pts',(-7.12895196100006,15.2,-7.92223001000002));
#281720=CARTESIAN_POINT('Ctrl Pts',(-7.12895196100006,11.6,-7.92223001000002));
#281721=CARTESIAN_POINT('Ctrl Pts',(-7.12706266200006,15.2,-7.92095827900001));
#281722=CARTESIAN_POINT('Ctrl Pts',(-7.12706266200006,11.6,-7.92095827900001));
#281723=CARTESIAN_POINT('Ctrl Pts',(-7.12517990500006,15.2,-7.91968854600002));
#281724=CARTESIAN_POINT('Ctrl Pts',(-7.12517990500006,11.6,-7.91968854600002));
#281725=CARTESIAN_POINT('Ctrl Pts',(-7.12330369600005,15.2,-7.91842082600001));
#281726=CARTESIAN_POINT('Ctrl Pts',(-7.12330369600005,11.6,-7.91842082600001));
#281727=CARTESIAN_POINT('Ctrl Pts',(-7.12143404200006,15.2,-7.91715513600002));
#281728=CARTESIAN_POINT('Ctrl Pts',(-7.12143404200006,11.6,-7.91715513600002));
#281729=CARTESIAN_POINT('Ctrl Pts',(-7.11957094800006,15.2,-7.91589149100002));
#281730=CARTESIAN_POINT('Ctrl Pts',(-7.11957094800006,11.6,-7.91589149100002));
#281731=CARTESIAN_POINT('Ctrl Pts',(-7.11771441600006,15.2,-7.91462990800002));
#281732=CARTESIAN_POINT('Ctrl Pts',(-7.11771441600006,11.6,-7.91462990800002));
#281733=CARTESIAN_POINT('Ctrl Pts',(-7.11586445500005,15.2,-7.91337040400002));
#281734=CARTESIAN_POINT('Ctrl Pts',(-7.11586445500005,11.6,-7.91337040400002));
#281735=CARTESIAN_POINT('Ctrl Pts',(-7.11402107000006,15.2,-7.91211299300001));
#281736=CARTESIAN_POINT('Ctrl Pts',(-7.11402107000006,11.6,-7.91211299300001));
#281737=CARTESIAN_POINT('Ctrl Pts',(-7.11218426500006,15.2,-7.91085769300001));
#281738=CARTESIAN_POINT('Ctrl Pts',(-7.11218426500006,11.6,-7.91085769300001));
#281739=CARTESIAN_POINT('Ctrl Pts',(-7.11035404400006,15.2,-7.90960451900002));
#281740=CARTESIAN_POINT('Ctrl Pts',(-7.11035404400006,11.6,-7.90960451900002));
#281741=CARTESIAN_POINT('Ctrl Pts',(-7.10853041700005,15.2,-7.90835348800002));
#281742=CARTESIAN_POINT('Ctrl Pts',(-7.10853041700005,11.6,-7.90835348800002));
#281743=CARTESIAN_POINT('Ctrl Pts',(-7.10671338600006,15.2,-7.90710461700002));
#281744=CARTESIAN_POINT('Ctrl Pts',(-7.10671338600006,11.6,-7.90710461700002));
#281745=CARTESIAN_POINT('Ctrl Pts',(-7.10490295600006,15.2,-7.90585792200002));
#281746=CARTESIAN_POINT('Ctrl Pts',(-7.10490295600006,11.6,-7.90585792200002));
#281747=CARTESIAN_POINT('Ctrl Pts',(-7.10309913500006,15.2,-7.90461341900001));
#281748=CARTESIAN_POINT('Ctrl Pts',(-7.10309913500006,11.6,-7.90461341900001));
#281749=CARTESIAN_POINT('Ctrl Pts',(-7.10130192600006,15.2,-7.90337112600002));
#281750=CARTESIAN_POINT('Ctrl Pts',(-7.10130192600006,11.6,-7.90337112600002));
#281751=CARTESIAN_POINT('Ctrl Pts',(-7.09951133700006,15.2,-7.90213105800002));
#281752=CARTESIAN_POINT('Ctrl Pts',(-7.09951133700006,11.6,-7.90213105800002));
#281753=CARTESIAN_POINT('Ctrl Pts',(-7.09772736900006,15.2,-7.90089323300001));
#281754=CARTESIAN_POINT('Ctrl Pts',(-7.09772736900006,11.6,-7.90089323300001));
#281755=CARTESIAN_POINT('Ctrl Pts',(-7.09595003200006,15.2,-7.89965766700002));
#281756=CARTESIAN_POINT('Ctrl Pts',(-7.09595003200006,11.6,-7.89965766700002));
#281757=CARTESIAN_POINT('Ctrl Pts',(-7.09417932900006,15.2,-7.89842437800001));
#281758=CARTESIAN_POINT('Ctrl Pts',(-7.09417932900006,11.6,-7.89842437800001));
#281759=CARTESIAN_POINT('Ctrl Pts',(-7.09241526600006,15.2,-7.89719338000002));
#281760=CARTESIAN_POINT('Ctrl Pts',(-7.09241526600006,11.6,-7.89719338000002));
#281761=CARTESIAN_POINT('Ctrl Pts',(-7.09065785000006,15.2,-7.89596469400001));
#281762=CARTESIAN_POINT('Ctrl Pts',(-7.09065785000006,11.6,-7.89596469400001));
#281763=CARTESIAN_POINT('Ctrl Pts',(-7.08890708300006,15.2,-7.89473833400002));
#281764=CARTESIAN_POINT('Ctrl Pts',(-7.08890708300006,11.6,-7.89473833400002));
#281765=CARTESIAN_POINT('Ctrl Pts',(-7.08716297200006,15.2,-7.89351431800001));
#281766=CARTESIAN_POINT('Ctrl Pts',(-7.08716297200006,11.6,-7.89351431800001));
#281767=CARTESIAN_POINT('Ctrl Pts',(-7.08542552400006,15.2,-7.89229266300002));
#281768=CARTESIAN_POINT('Ctrl Pts',(-7.08542552400006,11.6,-7.89229266300002));
#281769=CARTESIAN_POINT('Ctrl Pts',(-7.08369474300006,15.2,-7.89107338700001));
#281770=CARTESIAN_POINT('Ctrl Pts',(-7.08369474300006,11.6,-7.89107338700001));
#281771=CARTESIAN_POINT('Ctrl Pts',(-7.08197063600006,15.2,-7.88985650600001));
#281772=CARTESIAN_POINT('Ctrl Pts',(-7.08197063600006,11.6,-7.88985650600001));
#281773=CARTESIAN_POINT('Ctrl Pts',(-7.08025320600006,15.2,-7.88864203800002));
#281774=CARTESIAN_POINT('Ctrl Pts',(-7.08025320600006,11.6,-7.88864203800002));
#281775=CARTESIAN_POINT('Ctrl Pts',(-7.07854246000006,15.2,-7.88742999900002));
#281776=CARTESIAN_POINT('Ctrl Pts',(-7.07854246000006,11.6,-7.88742999900002));
#281777=CARTESIAN_POINT('Ctrl Pts',(-7.07683840300006,15.2,-7.88622040800002));
#281778=CARTESIAN_POINT('Ctrl Pts',(-7.07683840300006,11.6,-7.88622040800002));
#281779=CARTESIAN_POINT('Ctrl Pts',(-7.07514104100006,15.2,-7.88501328300002));
#281780=CARTESIAN_POINT('Ctrl Pts',(-7.07514104100006,11.6,-7.88501328300002));
#281781=CARTESIAN_POINT('Ctrl Pts',(-7.07345037900006,15.2,-7.88380863900001));
#281782=CARTESIAN_POINT('Ctrl Pts',(-7.07345037900006,11.6,-7.88380863900001));
#281783=CARTESIAN_POINT('Ctrl Pts',(-7.07176642300006,15.2,-7.88260649600002));
#281784=CARTESIAN_POINT('Ctrl Pts',(-7.07176642300006,11.6,-7.88260649600002));
#281785=CARTESIAN_POINT('Ctrl Pts',(-7.07008917700006,15.2,-7.88140687100002));
#281786=CARTESIAN_POINT('Ctrl Pts',(-7.07008917700006,11.6,-7.88140687100002));
#281787=CARTESIAN_POINT('Ctrl Pts',(-7.06841864900006,15.2,-7.88020978100001));
#281788=CARTESIAN_POINT('Ctrl Pts',(-7.06841864900006,11.6,-7.88020978100001));
#281789=CARTESIAN_POINT('Ctrl Pts',(-7.06675484400006,15.2,-7.87901524400001));
#281790=CARTESIAN_POINT('Ctrl Pts',(-7.06675484400006,11.6,-7.87901524400001));
#281791=CARTESIAN_POINT('Ctrl Pts',(-7.06509776700006,15.2,-7.87782327800001));
#281792=CARTESIAN_POINT('Ctrl Pts',(-7.06509776700006,11.6,-7.87782327800001));
#281793=CARTESIAN_POINT('Ctrl Pts',(-7.06344742100006,15.2,-7.87663390200001));
#281794=CARTESIAN_POINT('Ctrl Pts',(-7.06344742100006,11.6,-7.87663390200001));
#281795=CARTESIAN_POINT('Ctrl Pts',(-7.06180381600006,15.2,-7.87544713100001));
#281796=CARTESIAN_POINT('Ctrl Pts',(-7.06180381600006,11.6,-7.87544713100001));
#281797=CARTESIAN_POINT('Ctrl Pts',(-7.06016695600006,15.2,-7.87426298700002));
#281798=CARTESIAN_POINT('Ctrl Pts',(-7.06016695600006,11.6,-7.87426298700002));
#281799=CARTESIAN_POINT('Ctrl Pts',(-7.05853684500005,15.2,-7.87308148400002));
#281800=CARTESIAN_POINT('Ctrl Pts',(-7.05853684500005,11.6,-7.87308148400002));
#281801=CARTESIAN_POINT('Ctrl Pts',(-7.05691349000006,15.2,-7.87190264400002));
#281802=CARTESIAN_POINT('Ctrl Pts',(-7.05691349000006,11.6,-7.87190264400002));
#281803=CARTESIAN_POINT('Ctrl Pts',(-7.05529689500006,15.2,-7.87072648200001));
#281804=CARTESIAN_POINT('Ctrl Pts',(-7.05529689500006,11.6,-7.87072648200001));
#281805=CARTESIAN_POINT('Ctrl Pts',(-7.05368706800006,15.2,-7.86955301900001));
#281806=CARTESIAN_POINT('Ctrl Pts',(-7.05368706800006,11.6,-7.86955301900001));
#281807=CARTESIAN_POINT('Ctrl Pts',(-7.05208401300006,15.2,-7.86838227100001));
#281808=CARTESIAN_POINT('Ctrl Pts',(-7.05208401300006,11.6,-7.86838227100001));
#281809=CARTESIAN_POINT('Ctrl Pts',(-7.05048773700006,15.2,-7.86721425700001));
#281810=CARTESIAN_POINT('Ctrl Pts',(-7.05048773700006,11.6,-7.86721425700001));
#281811=CARTESIAN_POINT('Ctrl Pts',(-7.04889824400006,15.2,-7.86604899600002));
#281812=CARTESIAN_POINT('Ctrl Pts',(-7.04889824400006,11.6,-7.86604899600002));
#281813=CARTESIAN_POINT('Ctrl Pts',(-7.04731554000006,15.2,-7.86488650600001));
#281814=CARTESIAN_POINT('Ctrl Pts',(-7.04731554000006,11.6,-7.86488650600001));
#281815=CARTESIAN_POINT('Ctrl Pts',(-7.04573963100006,15.2,-7.86372680800002));
#281816=CARTESIAN_POINT('Ctrl Pts',(-7.04573963100006,11.6,-7.86372680800002));
#281817=CARTESIAN_POINT('Ctrl Pts',(-7.04417052200006,15.2,-7.86256991700002));
#281818=CARTESIAN_POINT('Ctrl Pts',(-7.04417052200006,11.6,-7.86256991700002));
#281819=CARTESIAN_POINT('Ctrl Pts',(-7.04260822000006,15.2,-7.86141585300002));
#281820=CARTESIAN_POINT('Ctrl Pts',(-7.04260822000006,11.6,-7.86141585300002));
#281821=CARTESIAN_POINT('Ctrl Pts',(-7.04105273000006,15.2,-7.86026463600002));
#281822=CARTESIAN_POINT('Ctrl Pts',(-7.04105273000006,11.6,-7.86026463600002));
#281823=CARTESIAN_POINT('Ctrl Pts',(-7.03950405700006,15.2,-7.85911628400001));
#281824=CARTESIAN_POINT('Ctrl Pts',(-7.03950405700006,11.6,-7.85911628400001));
#281825=CARTESIAN_POINT('Ctrl Pts',(-7.03796220600006,15.2,-7.85797081600002));
#281826=CARTESIAN_POINT('Ctrl Pts',(-7.03796220600006,11.6,-7.85797081600002));
#281827=CARTESIAN_POINT('Ctrl Pts',(-7.03642718500006,15.2,-7.85682825100002));
#281828=CARTESIAN_POINT('Ctrl Pts',(-7.03642718500006,11.6,-7.85682825100002));
#281829=CARTESIAN_POINT('Ctrl Pts',(-7.03489899900006,15.2,-7.85568860800002));
#281830=CARTESIAN_POINT('Ctrl Pts',(-7.03489899900006,11.6,-7.85568860800002));
#281831=CARTESIAN_POINT('Ctrl Pts',(-7.03337765200006,15.2,-7.85455190700001));
#281832=CARTESIAN_POINT('Ctrl Pts',(-7.03337765200006,11.6,-7.85455190700001));
#281833=CARTESIAN_POINT('Ctrl Pts',(-7.03186315100006,15.2,-7.85341816500001));
#281834=CARTESIAN_POINT('Ctrl Pts',(-7.03186315100006,11.6,-7.85341816500001));
#281835=CARTESIAN_POINT('Ctrl Pts',(-7.03035550200005,15.2,-7.85228740300001));
#281836=CARTESIAN_POINT('Ctrl Pts',(-7.03035550200005,11.6,-7.85228740300001));
#281837=CARTESIAN_POINT('Ctrl Pts',(-7.02885471100006,15.2,-7.85115964100001));
#281838=CARTESIAN_POINT('Ctrl Pts',(-7.02885471100006,11.6,-7.85115964100001));
#281839=CARTESIAN_POINT('Ctrl Pts',(-7.02736078200005,15.2,-7.85003489800002));
#281840=CARTESIAN_POINT('Ctrl Pts',(-7.02736078200005,11.6,-7.85003489800002));
#281841=CARTESIAN_POINT('Ctrl Pts',(-7.02587372100006,15.2,-7.84891319200002));
#281842=CARTESIAN_POINT('Ctrl Pts',(-7.02587372100006,11.6,-7.84891319200002));
#281843=CARTESIAN_POINT('Ctrl Pts',(-7.02439353500006,15.2,-7.84779454400002));
#281844=CARTESIAN_POINT('Ctrl Pts',(-7.02439353500006,11.6,-7.84779454400002));
#281845=CARTESIAN_POINT('Ctrl Pts',(-7.02292023000005,15.2,-7.84667897200002));
#281846=CARTESIAN_POINT('Ctrl Pts',(-7.02292023000005,11.6,-7.84667897200002));
#281847=CARTESIAN_POINT('Ctrl Pts',(-7.02145381000006,15.2,-7.84556649900002));
#281848=CARTESIAN_POINT('Ctrl Pts',(-7.02145381000006,11.6,-7.84556649900002));
#281849=CARTESIAN_POINT('Ctrl Pts',(-7.01999428200006,15.2,-7.84445714300002));
#281850=CARTESIAN_POINT('Ctrl Pts',(-7.01999428200006,11.6,-7.84445714300002));
#281851=CARTESIAN_POINT('Ctrl Pts',(-7.01854165200006,15.2,-7.84335092300001));
#281852=CARTESIAN_POINT('Ctrl Pts',(-7.01854165200006,11.6,-7.84335092300001));
#281853=CARTESIAN_POINT('Ctrl Pts',(-7.01709592400006,15.2,-7.84224785900002));
#281854=CARTESIAN_POINT('Ctrl Pts',(-7.01709592400006,11.6,-7.84224785900002));
#281855=CARTESIAN_POINT('Ctrl Pts',(-7.01565710600006,15.2,-7.84114797200001));
#281856=CARTESIAN_POINT('Ctrl Pts',(-7.01565710600006,11.6,-7.84114797200001));
#281857=CARTESIAN_POINT('Ctrl Pts',(-7.01422520300006,15.2,-7.84005128300001));
#281858=CARTESIAN_POINT('Ctrl Pts',(-7.01422520300006,11.6,-7.84005128300001));
#281859=CARTESIAN_POINT('Ctrl Pts',(-7.01280022000006,15.2,-7.83895780900002));
#281860=CARTESIAN_POINT('Ctrl Pts',(-7.01280022000006,11.6,-7.83895780900002));
#281861=CARTESIAN_POINT('Ctrl Pts',(-7.01138216400006,15.2,-7.83786757300001));
#281862=CARTESIAN_POINT('Ctrl Pts',(-7.01138216400006,11.6,-7.83786757300001));
#281863=CARTESIAN_POINT('Ctrl Pts',(-7.00997103900006,15.2,-7.83678059500001));
#281864=CARTESIAN_POINT('Ctrl Pts',(-7.00997103900006,11.6,-7.83678059500001));
#281865=CARTESIAN_POINT('Ctrl Pts',(-7.00856685400006,15.2,-7.83569689500001));
#281866=CARTESIAN_POINT('Ctrl Pts',(-7.00856685400006,11.6,-7.83569689500001));
#281867=CARTESIAN_POINT('Ctrl Pts',(-7.00716961100006,15.2,-7.83461649300002));
#281868=CARTESIAN_POINT('Ctrl Pts',(-7.00716961100006,11.6,-7.83461649300002));
#281869=CARTESIAN_POINT('Ctrl Pts',(-7.00577931900006,15.2,-7.83353941000002));
#281870=CARTESIAN_POINT('Ctrl Pts',(-7.00577931900006,11.6,-7.83353941000002));
#281871=CARTESIAN_POINT('Ctrl Pts',(-7.00439598300005,15.2,-7.83246566700001));
#281872=CARTESIAN_POINT('Ctrl Pts',(-7.00439598300005,11.6,-7.83246566700001));
#281873=CARTESIAN_POINT('Ctrl Pts',(-7.00301960800005,15.2,-7.83139528400002));
#281874=CARTESIAN_POINT('Ctrl Pts',(-7.00301960800005,11.6,-7.83139528400002));
#281875=CARTESIAN_POINT('Ctrl Pts',(-7.00165020000005,15.2,-7.83032828300002));
#281876=CARTESIAN_POINT('Ctrl Pts',(-7.00165020000005,11.6,-7.83032828300002));
#281877=CARTESIAN_POINT('Ctrl Pts',(-7.00028776600006,15.2,-7.82926468300002));
#281878=CARTESIAN_POINT('Ctrl Pts',(-7.00028776600006,11.6,-7.82926468300002));
#281879=CARTESIAN_POINT('Ctrl Pts',(-6.99893231000006,15.2,-7.82820450600001));
#281880=CARTESIAN_POINT('Ctrl Pts',(-6.99893231000006,11.6,-7.82820450600001));
#281881=CARTESIAN_POINT('Ctrl Pts',(-6.99758384000006,15.2,-7.82714777300002));
#281882=CARTESIAN_POINT('Ctrl Pts',(-6.99758384000006,11.6,-7.82714777300002));
#281883=CARTESIAN_POINT('Ctrl Pts',(-6.99624236100005,15.2,-7.82609450600001));
#281884=CARTESIAN_POINT('Ctrl Pts',(-6.99624236100005,11.6,-7.82609450600001));
#281885=CARTESIAN_POINT('Ctrl Pts',(-6.99490787900006,15.2,-7.82504472400002));
#281886=CARTESIAN_POINT('Ctrl Pts',(-6.99490787900006,11.6,-7.82504472400002));
#281887=CARTESIAN_POINT('Ctrl Pts',(-6.99358039900006,15.2,-7.82399845200001));
#281888=CARTESIAN_POINT('Ctrl Pts',(-6.99358039900006,11.6,-7.82399845200001));
#281889=CARTESIAN_POINT('Ctrl Pts',(-6.99225992900006,15.2,-7.82295570700001));
#281890=CARTESIAN_POINT('Ctrl Pts',(-6.99225992900006,11.6,-7.82295570700001));
#281891=CARTESIAN_POINT('Ctrl Pts',(-6.99094647300006,15.2,-7.82191651400002));
#281892=CARTESIAN_POINT('Ctrl Pts',(-6.99094647300006,11.6,-7.82191651400002));
#281893=CARTESIAN_POINT('Ctrl Pts',(-6.98964003800006,15.2,-7.82088089200002));
#281894=CARTESIAN_POINT('Ctrl Pts',(-6.98964003800006,11.6,-7.82088089200002));
#281895=CARTESIAN_POINT('Ctrl Pts',(-6.98834063000006,15.2,-7.81984886400001));
#281896=CARTESIAN_POINT('Ctrl Pts',(-6.98834063000006,11.6,-7.81984886400001));
#281897=CARTESIAN_POINT('Ctrl Pts',(-6.98704825400006,15.2,-7.81882045200001));
#281898=CARTESIAN_POINT('Ctrl Pts',(-6.98704825400006,11.6,-7.81882045200001));
#281899=CARTESIAN_POINT('Ctrl Pts',(-6.98576291700006,15.2,-7.81779567700001));
#281900=CARTESIAN_POINT('Ctrl Pts',(-6.98576291700006,11.6,-7.81779567700001));
#281901=CARTESIAN_POINT('Ctrl Pts',(-6.98448462500005,15.2,-7.81677456100001));
#281902=CARTESIAN_POINT('Ctrl Pts',(-6.98448462500005,11.6,-7.81677456100001));
#281903=CARTESIAN_POINT('Ctrl Pts',(-6.98321338300006,15.2,-7.81575712600001));
#281904=CARTESIAN_POINT('Ctrl Pts',(-6.98321338300006,11.6,-7.81575712600001));
#281905=CARTESIAN_POINT('Ctrl Pts',(-6.98194919900006,15.2,-7.81474339500001));
#281906=CARTESIAN_POINT('Ctrl Pts',(-6.98194919900006,11.6,-7.81474339500001));
#281907=CARTESIAN_POINT('Ctrl Pts',(-6.98069207700006,15.2,-7.81373338900002));
#281908=CARTESIAN_POINT('Ctrl Pts',(-6.98069207700006,11.6,-7.81373338900002));
#281909=CARTESIAN_POINT('Ctrl Pts',(-6.97944202300006,15.2,-7.81272712900002));
#281910=CARTESIAN_POINT('Ctrl Pts',(-6.97944202300006,11.6,-7.81272712900002));
#281911=CARTESIAN_POINT('Ctrl Pts',(-6.97819904600006,15.2,-7.81172464200001));
#281912=CARTESIAN_POINT('Ctrl Pts',(-6.97819904600006,11.6,-7.81172464200001));
#281913=CARTESIAN_POINT('Ctrl Pts',(-6.97696314800006,15.2,-7.81072594500002));
#281914=CARTESIAN_POINT('Ctrl Pts',(-6.97696314800006,11.6,-7.81072594500002));
#281915=CARTESIAN_POINT('Ctrl Pts',(-6.97573433800006,15.2,-7.80973106400002));
#281916=CARTESIAN_POINT('Ctrl Pts',(-6.97573433800006,11.6,-7.80973106400002));
#281917=CARTESIAN_POINT('Ctrl Pts',(-6.97451262200006,15.2,-7.80874002000001));
#281918=CARTESIAN_POINT('Ctrl Pts',(-6.97451262200006,11.6,-7.80874002000001));
#281919=CARTESIAN_POINT('Ctrl Pts',(-6.97329800400006,15.2,-7.80775283600001));
#281920=CARTESIAN_POINT('Ctrl Pts',(-6.97329800400006,11.6,-7.80775283600001));
#281921=CARTESIAN_POINT('Ctrl Pts',(-6.97209049200006,15.2,-7.80676953600001));
#281922=CARTESIAN_POINT('Ctrl Pts',(-6.97209049200006,11.6,-7.80676953600001));
#281923=CARTESIAN_POINT('Ctrl Pts',(-6.97089009100006,15.2,-7.80579014100002));
#281924=CARTESIAN_POINT('Ctrl Pts',(-6.97089009100006,11.6,-7.80579014100002));
#281925=CARTESIAN_POINT('Ctrl Pts',(-6.96969680800006,15.2,-7.80481467500002));
#281926=CARTESIAN_POINT('Ctrl Pts',(-6.96969680800006,11.6,-7.80481467500002));
#281927=CARTESIAN_POINT('Ctrl Pts',(-6.96851064900006,15.2,-7.80384316100001));
#281928=CARTESIAN_POINT('Ctrl Pts',(-6.96851064900006,11.6,-7.80384316100001));
#281929=CARTESIAN_POINT('Ctrl Pts',(-6.96733161900006,15.2,-7.80287562300002));
#281930=CARTESIAN_POINT('Ctrl Pts',(-6.96733161900006,11.6,-7.80287562300002));
#281931=CARTESIAN_POINT('Ctrl Pts',(-6.96615972600005,15.2,-7.80191208300002));
#281932=CARTESIAN_POINT('Ctrl Pts',(-6.96615972600005,11.6,-7.80191208300002));
#281933=CARTESIAN_POINT('Ctrl Pts',(-6.96499497600006,15.2,-7.80095256500001));
#281934=CARTESIAN_POINT('Ctrl Pts',(-6.96499497600006,11.6,-7.80095256500001));
#281935=CARTESIAN_POINT('Ctrl Pts',(-6.96383737400006,15.2,-7.79999709300002));
#281936=CARTESIAN_POINT('Ctrl Pts',(-6.96383737400006,11.6,-7.79999709300002));
#281937=CARTESIAN_POINT('Ctrl Pts',(-6.96268692700006,15.2,-7.79904568800001));
#281938=CARTESIAN_POINT('Ctrl Pts',(-6.96268692700006,11.6,-7.79904568800001));
#281939=CARTESIAN_POINT('Ctrl Pts',(-6.96154364000006,15.2,-7.79809837700002));
#281940=CARTESIAN_POINT('Ctrl Pts',(-6.96154364000006,11.6,-7.79809837700002));
#281941=CARTESIAN_POINT('Ctrl Pts',(-6.96040752100005,15.2,-7.79715518200002));
#281942=CARTESIAN_POINT('Ctrl Pts',(-6.96040752100005,11.6,-7.79715518200002));
#281943=CARTESIAN_POINT('Ctrl Pts',(-6.95927857600006,15.2,-7.79621612700002));
#281944=CARTESIAN_POINT('Ctrl Pts',(-6.95927857600006,11.6,-7.79621612700002));
#281945=CARTESIAN_POINT('Ctrl Pts',(-6.95815681000005,15.2,-7.79528123600001));
#281946=CARTESIAN_POINT('Ctrl Pts',(-6.95815681000005,11.6,-7.79528123600001));
#281947=CARTESIAN_POINT('Ctrl Pts',(-6.95704223000006,15.2,-7.79435053500002));
#281948=CARTESIAN_POINT('Ctrl Pts',(-6.95704223000006,11.6,-7.79435053500002));
#281949=CARTESIAN_POINT('Ctrl Pts',(-6.95593484300006,15.2,-7.79342404500002));
#281950=CARTESIAN_POINT('Ctrl Pts',(-6.95593484300006,11.6,-7.79342404500002));
#281951=CARTESIAN_POINT('Ctrl Pts',(-6.95483465400006,15.2,-7.79250179100002));
#281952=CARTESIAN_POINT('Ctrl Pts',(-6.95483465400006,11.6,-7.79250179100002));
#281953=CARTESIAN_POINT('Ctrl Pts',(-6.95374167100006,15.2,-7.79158379900001));
#281954=CARTESIAN_POINT('Ctrl Pts',(-6.95374167100006,11.6,-7.79158379900001));
#281955=CARTESIAN_POINT('Ctrl Pts',(-6.95265589800006,15.2,-7.79067009300002));
#281956=CARTESIAN_POINT('Ctrl Pts',(-6.95265589800006,11.6,-7.79067009300002));
#281957=CARTESIAN_POINT('Ctrl Pts',(-6.95157734400006,15.2,-7.78976069600001));
#281958=CARTESIAN_POINT('Ctrl Pts',(-6.95157734400006,11.6,-7.78976069600001));
#281959=CARTESIAN_POINT('Ctrl Pts',(-6.95050601300006,15.2,-7.78885563600002));
#281960=CARTESIAN_POINT('Ctrl Pts',(-6.95050601300006,11.6,-7.78885563600002));
#281961=CARTESIAN_POINT('Ctrl Pts',(-6.94944191300006,15.2,-7.78795493400001));
#281962=CARTESIAN_POINT('Ctrl Pts',(-6.94944191300006,11.6,-7.78795493400001));
#281963=CARTESIAN_POINT('Ctrl Pts',(-6.94838505000006,15.2,-7.78705861700002));
#281964=CARTESIAN_POINT('Ctrl Pts',(-6.94838505000006,11.6,-7.78705861700002));
#281965=CARTESIAN_POINT('Ctrl Pts',(-6.94733542900006,15.2,-7.78616671000002));
#281966=CARTESIAN_POINT('Ctrl Pts',(-6.94733542900006,11.6,-7.78616671000002));
#281967=CARTESIAN_POINT('Ctrl Pts',(-6.94629305800006,15.2,-7.78527923700001));
#281968=CARTESIAN_POINT('Ctrl Pts',(-6.94629305800006,11.6,-7.78527923700001));
#281969=CARTESIAN_POINT('Ctrl Pts',(-6.94525794400006,15.2,-7.78439622500001));
#281970=CARTESIAN_POINT('Ctrl Pts',(-6.94525794400006,11.6,-7.78439622500001));
#281971=CARTESIAN_POINT('Ctrl Pts',(-6.94423009200006,15.2,-7.78351769800001));
#281972=CARTESIAN_POINT('Ctrl Pts',(-6.94423009200006,11.6,-7.78351769800001));
#281973=CARTESIAN_POINT('Ctrl Pts',(-6.94320950800006,15.2,-7.78264368200002));
#281974=CARTESIAN_POINT('Ctrl Pts',(-6.94320950800006,11.6,-7.78264368200002));
#281975=CARTESIAN_POINT('Ctrl Pts',(-6.94219620100006,15.2,-7.78177420300001));
#281976=CARTESIAN_POINT('Ctrl Pts',(-6.94219620100006,11.6,-7.78177420300001));
#281977=CARTESIAN_POINT('Ctrl Pts',(-6.94119017500006,15.2,-7.78090928600002));
#281978=CARTESIAN_POINT('Ctrl Pts',(-6.94119017500006,11.6,-7.78090928600002));
#281979=CARTESIAN_POINT('Ctrl Pts',(-6.94019143600006,15.2,-7.78004895700001));
#281980=CARTESIAN_POINT('Ctrl Pts',(-6.94019143600006,11.6,-7.78004895700001));
#281981=CARTESIAN_POINT('Ctrl Pts',(-6.93919999400006,15.2,-7.77919324200001));
#281982=CARTESIAN_POINT('Ctrl Pts',(-6.93919999400006,11.6,-7.77919324200001));
#281983=CARTESIAN_POINT('Ctrl Pts',(-6.93821585300006,15.2,-7.77834216700001));
#281984=CARTESIAN_POINT('Ctrl Pts',(-6.93821585300006,11.6,-7.77834216700001));
#281985=CARTESIAN_POINT('Ctrl Pts',(-6.93723901900006,15.2,-7.77749575800001));
#281986=CARTESIAN_POINT('Ctrl Pts',(-6.93723901900006,11.6,-7.77749575800001));
#281987=CARTESIAN_POINT('Ctrl Pts',(-6.93626950100006,15.2,-7.77665404200001));
#281988=CARTESIAN_POINT('Ctrl Pts',(-6.93626950100006,11.6,-7.77665404200001));
#281989=CARTESIAN_POINT('Ctrl Pts',(-6.93530730300006,15.2,-7.77581704500002));
#281990=CARTESIAN_POINT('Ctrl Pts',(-6.93530730300006,11.6,-7.77581704500002));
#281991=CARTESIAN_POINT('Ctrl Pts',(-6.93435243400006,15.2,-7.77498479200001));
#281992=CARTESIAN_POINT('Ctrl Pts',(-6.93435243400006,11.6,-7.77498479200001));
#281993=CARTESIAN_POINT('Ctrl Pts',(-6.93340489800006,15.2,-7.77415731300002));
#281994=CARTESIAN_POINT('Ctrl Pts',(-6.93340489800006,11.6,-7.77415731300002));
#281995=CARTESIAN_POINT('Ctrl Pts',(-6.93246470300006,15.2,-7.77333463100002));
#281996=CARTESIAN_POINT('Ctrl Pts',(-6.93246470300006,11.6,-7.77333463100002));
#281997=CARTESIAN_POINT('Ctrl Pts',(-6.93153185600006,15.2,-7.77251677600002));
#281998=CARTESIAN_POINT('Ctrl Pts',(-6.93153185600006,11.6,-7.77251677600002));
#281999=CARTESIAN_POINT('Ctrl Pts',(-6.93060636400006,15.2,-7.77170377300001));
#282000=CARTESIAN_POINT('Ctrl Pts',(-6.93060636400006,11.6,-7.77170377300001));
#282001=CARTESIAN_POINT('Ctrl Pts',(-6.92968823200006,15.2,-7.77089565100002));
#282002=CARTESIAN_POINT('Ctrl Pts',(-6.92968823200006,11.6,-7.77089565100002));
#282003=CARTESIAN_POINT('Ctrl Pts',(-6.92877746800006,15.2,-7.77009243500002));
#282004=CARTESIAN_POINT('Ctrl Pts',(-6.92877746800006,11.6,-7.77009243500002));
#282005=CARTESIAN_POINT('Ctrl Pts',(-6.92787407800005,15.2,-7.76929415300001));
#282006=CARTESIAN_POINT('Ctrl Pts',(-6.92787407800005,11.6,-7.76929415300001));
#282007=CARTESIAN_POINT('Ctrl Pts',(-6.92697807000005,15.2,-7.76850083500002));
#282008=CARTESIAN_POINT('Ctrl Pts',(-6.92697807000005,11.6,-7.76850083500002));
#282009=CARTESIAN_POINT('Ctrl Pts',(-6.92608944900006,15.2,-7.76771250600002));
#282010=CARTESIAN_POINT('Ctrl Pts',(-6.92608944900006,11.6,-7.76771250600002));
#282011=CARTESIAN_POINT('Ctrl Pts',(-6.92520822300006,15.2,-7.76692919400002));
#282012=CARTESIAN_POINT('Ctrl Pts',(-6.92520822300006,11.6,-7.76692919400002));
#282013=CARTESIAN_POINT('Ctrl Pts',(-6.92433439800006,15.2,-7.76615092800002));
#282014=CARTESIAN_POINT('Ctrl Pts',(-6.92433439800006,11.6,-7.76615092800002));
#282015=CARTESIAN_POINT('Ctrl Pts',(-6.92346798200006,15.2,-7.76537773600002));
#282016=CARTESIAN_POINT('Ctrl Pts',(-6.92346798200006,11.6,-7.76537773600002));
#282017=CARTESIAN_POINT('Ctrl Pts',(-6.92260898000006,15.2,-7.76460964400002));
#282018=CARTESIAN_POINT('Ctrl Pts',(-6.92260898000006,11.6,-7.76460964400002));
#282019=CARTESIAN_POINT('Ctrl Pts',(-6.92175740000006,15.2,-7.76384668300001));
#282020=CARTESIAN_POINT('Ctrl Pts',(-6.92175740000006,11.6,-7.76384668300001));
#282021=CARTESIAN_POINT('Ctrl Pts',(-6.92091324900006,15.2,-7.76308888100001));
#282022=CARTESIAN_POINT('Ctrl Pts',(-6.92091324900006,11.6,-7.76308888100001));
#282023=CARTESIAN_POINT('Ctrl Pts',(-6.92007653400006,15.2,-7.76233626500002));
#282024=CARTESIAN_POINT('Ctrl Pts',(-6.92007653400006,11.6,-7.76233626500002));
#282025=CARTESIAN_POINT('Ctrl Pts',(-6.91924726000006,15.2,-7.76158886500002));
#282026=CARTESIAN_POINT('Ctrl Pts',(-6.91924726000006,11.6,-7.76158886500002));
#282027=CARTESIAN_POINT('Ctrl Pts',(-6.91842543700006,15.2,-7.76084670900002));
#282028=CARTESIAN_POINT('Ctrl Pts',(-6.91842543700006,11.6,-7.76084670900002));
#282029=CARTESIAN_POINT('Ctrl Pts',(-6.91761106900006,15.2,-7.76010982800001));
#282030=CARTESIAN_POINT('Ctrl Pts',(-6.91761106900006,11.6,-7.76010982800001));
#282031=CARTESIAN_POINT('Ctrl Pts',(-6.91680416500006,15.2,-7.75937824900002));
#282032=CARTESIAN_POINT('Ctrl Pts',(-6.91680416500006,11.6,-7.75937824900002));
#282033=CARTESIAN_POINT('Ctrl Pts',(-6.91600473100006,15.2,-7.75865200100001));
#282034=CARTESIAN_POINT('Ctrl Pts',(-6.91600473100006,11.6,-7.75865200100001));
#282035=CARTESIAN_POINT('Ctrl Pts',(-6.91521277400006,15.2,-7.75793111500001));
#282036=CARTESIAN_POINT('Ctrl Pts',(-6.91521277400006,11.6,-7.75793111500001));
#282037=CARTESIAN_POINT('Ctrl Pts',(-6.91442830100006,15.2,-7.75721562100002));
#282038=CARTESIAN_POINT('Ctrl Pts',(-6.91442830100006,11.6,-7.75721562100002));
#282039=CARTESIAN_POINT('Ctrl Pts',(-6.91365131900006,15.2,-7.75650554700002));
#282040=CARTESIAN_POINT('Ctrl Pts',(-6.91365131900006,11.6,-7.75650554700002));
#282041=CARTESIAN_POINT('Ctrl Pts',(-6.91288183600006,15.2,-7.75580092300002));
#282042=CARTESIAN_POINT('Ctrl Pts',(-6.91288183600006,11.6,-7.75580092300002));
#282043=CARTESIAN_POINT('Ctrl Pts',(-6.91211985800006,15.2,-7.75510178100002));
#282044=CARTESIAN_POINT('Ctrl Pts',(-6.91211985800006,11.6,-7.75510178100002));
#282045=CARTESIAN_POINT('Ctrl Pts',(-6.91136539200006,15.2,-7.75440814800002));
#282046=CARTESIAN_POINT('Ctrl Pts',(-6.91136539200006,11.6,-7.75440814800002));
#282047=CARTESIAN_POINT('Ctrl Pts',(-6.91061844600006,15.2,-7.75372005700002));
#282048=CARTESIAN_POINT('Ctrl Pts',(-6.91061844600006,11.6,-7.75372005700002));
#282049=CARTESIAN_POINT('Ctrl Pts',(-6.90987902600006,15.2,-7.75303753700002));
#282050=CARTESIAN_POINT('Ctrl Pts',(-6.90987902600006,11.6,-7.75303753700002));
#282051=CARTESIAN_POINT('Ctrl Pts',(-6.90914714100006,15.2,-7.75236061900002));
#282052=CARTESIAN_POINT('Ctrl Pts',(-6.90914714100006,11.6,-7.75236061900002));
#282053=CARTESIAN_POINT('Ctrl Pts',(-6.90842279600006,15.2,-7.75168933500002));
#282054=CARTESIAN_POINT('Ctrl Pts',(-6.90842279600006,11.6,-7.75168933500002));
#282055=CARTESIAN_POINT('Ctrl Pts',(-6.90770600000006,15.2,-7.75102371400001));
#282056=CARTESIAN_POINT('Ctrl Pts',(-6.90770600000006,11.6,-7.75102371400001));
#282057=CARTESIAN_POINT('Ctrl Pts',(-6.90699675800006,15.2,-7.75036378800002));
#282058=CARTESIAN_POINT('Ctrl Pts',(-6.90699675800006,11.6,-7.75036378800002));
#282059=CARTESIAN_POINT('Ctrl Pts',(-6.90629508000006,15.2,-7.74970958700001));
#282060=CARTESIAN_POINT('Ctrl Pts',(-6.90629508000006,11.6,-7.74970958700001));
#282061=CARTESIAN_POINT('Ctrl Pts',(-6.90560097000006,15.2,-7.74906114500002));
#282062=CARTESIAN_POINT('Ctrl Pts',(-6.90560097000006,11.6,-7.74906114500002));
#282063=CARTESIAN_POINT('Ctrl Pts',(-6.90491443800005,15.2,-7.74841849200002));
#282064=CARTESIAN_POINT('Ctrl Pts',(-6.90491443800005,11.6,-7.74841849200002));
#282065=CARTESIAN_POINT('Ctrl Pts',(-6.90423549100006,15.2,-7.74778165800001));
#282066=CARTESIAN_POINT('Ctrl Pts',(-6.90423549100006,11.6,-7.74778165800001));
#282067=CARTESIAN_POINT('Ctrl Pts',(-6.90356800200006,15.2,-7.74715431200002));
#282068=CARTESIAN_POINT('Ctrl Pts',(-6.90356800200006,11.6,-7.74715431200002));
#282069=CARTESIAN_POINT('Ctrl Pts',(-6.90304077600006,15.2,-7.74665780200002));
#282070=CARTESIAN_POINT('Ctrl Pts',(-6.90304077600006,11.6,-7.74665780200002));
#282071=CARTESIAN_POINT('Ctrl Pts',(-6.90264967000005,15.2,-7.74628893100001));
#282072=CARTESIAN_POINT('Ctrl Pts',(-6.90264967000005,11.6,-7.74628893100001));
#282073=CARTESIAN_POINT('Ctrl Pts',(-6.90239167400006,15.2,-7.74604536200002));
#282074=CARTESIAN_POINT('Ctrl Pts',(-6.90239167400006,11.6,-7.74604536200002));
#282075=CARTESIAN_POINT('Ctrl Pts',(-6.90226492000006,15.2,-7.74592563800002));
#282076=CARTESIAN_POINT('Ctrl Pts',(-6.90226492000006,11.6,-7.74592563800002));
#282077=CARTESIAN_POINT('',(-6.90226492000223,12.2,-7.74592563733579));
#282078=CARTESIAN_POINT('',(-6.90226492000223,15.2,-7.74592563733579));
#282079=CARTESIAN_POINT('',(-6.90226492000006,12.2,-7.74592563700002));
#282080=CARTESIAN_POINT('Ctrl Pts',(-7.93573928312123,12.2,-8.32310290867369));
#282081=CARTESIAN_POINT('Ctrl Pts',(-7.93215544686481,12.2,-8.32177217006299));
#282082=CARTESIAN_POINT('Ctrl Pts',(-7.9285793196337,12.2,-8.320439684464));
#282083=CARTESIAN_POINT('Ctrl Pts',(-7.9250108958958,12.2,-8.31910545665107));
#282084=CARTESIAN_POINT('Ctrl Pts',(-7.92144247215791,12.2,-8.31777122883814));
#282085=CARTESIAN_POINT('Ctrl Pts',(-7.9178817551368,12.2,-8.31643525657686));
#282086=CARTESIAN_POINT('Ctrl Pts',(-7.91432875292083,12.2,-8.31509755651716));
#282087=CARTESIAN_POINT('Ctrl Pts',(-7.91077575070486,12.2,-8.31375985645747));
#282088=CARTESIAN_POINT('Ctrl Pts',(-7.90723046392704,12.2,-8.31242042849342));
#282089=CARTESIAN_POINT('Ctrl Pts',(-7.9036929159712,12.2,-8.31107930933406));
#282090=CARTESIAN_POINT('Ctrl Pts',(-7.9001553673727,12.2,-8.30973818993105));
#282091=CARTESIAN_POINT('Ctrl Pts',(-7.89662555700969,12.2,-8.30839538038589));
#282092=CARTESIAN_POINT('Ctrl Pts',(-7.89310351045721,12.2,-8.3070509233986));
#282093=CARTESIAN_POINT('Ctrl Pts',(-7.88958146454457,12.2,-8.30570646665556));
#282094=CARTESIAN_POINT('Ctrl Pts',(-7.88606718362318,12.2,-8.30436036262094));
#282095=CARTESIAN_POINT('Ctrl Pts',(-7.88256068608459,12.2,-8.3030126456281));
#282096=CARTESIAN_POINT('Ctrl Pts',(-7.87905418854601,12.2,-8.30166492863525));
#282097=CARTESIAN_POINT('Ctrl Pts',(-7.87555547453582,12.2,-8.30031559610586));
#282098=CARTESIAN_POINT('Ctrl Pts',(-7.8720645630635,12.2,-8.2989646822738));
#282099=CARTESIAN_POINT('Ctrl Pts',(-7.86741001464514,12.2,-8.29716346391286));
#282100=CARTESIAN_POINT('Ctrl Pts',(-7.86276933845468,12.2,-8.29535943319745));
#282101=CARTESIAN_POINT('Ctrl Pts',(-7.85814258399815,12.2,-8.29355267501209));
#282102=CARTESIAN_POINT('Ctrl Pts',(-7.85467251736775,12.2,-8.29219760606535));
#282103=CARTESIAN_POINT('Ctrl Pts',(-7.85121028169792,12.2,-8.29084100413487));
#282104=CARTESIAN_POINT('Ctrl Pts',(-7.84775589898862,12.2,-8.28948290464563));
#282105=CARTESIAN_POINT('Ctrl Pts',(-7.84430151690686,12.2,-8.28812480540311));
#282106=CARTESIAN_POINT('Ctrl Pts',(-7.8408549865497,12.2,-8.28676520938565));
#282107=CARTESIAN_POINT('Ctrl Pts',(-7.83741633042532,12.2,-8.28540415155998));
#282108=CARTESIAN_POINT('Ctrl Pts',(-7.83397767430094,12.2,-8.28404309373431));
#282109=CARTESIAN_POINT('Ctrl Pts',(-7.83054689030472,12.2,-8.28268057405543));
#282110=CARTESIAN_POINT('Ctrl Pts',(-7.82712400028857,12.2,-8.28131662826545));
#282111=CARTESIAN_POINT('Ctrl Pts',(-7.82370111027241,12.2,-8.27995268247547));
#282112=CARTESIAN_POINT('Ctrl Pts',(-7.82028611349482,12.2,-8.27858731074114));
#282113=CARTESIAN_POINT('Ctrl Pts',(-7.81687903201977,12.2,-8.27722054949293));
#282114=CARTESIAN_POINT('Ctrl Pts',(-7.81347195054471,12.2,-8.27585378824472));
#282115=CARTESIAN_POINT('Ctrl Pts',(-7.81007278429725,12.2,-8.27448563789939));
#282116=CARTESIAN_POINT('Ctrl Pts',(-7.80668155287811,12.2,-8.27311613465761));
#282117=CARTESIAN_POINT('Ctrl Pts',(-7.80329032145898,12.2,-8.27174663141583));
#282118=CARTESIAN_POINT('Ctrl Pts',(-7.79990702624761,12.2,-8.27037577554912));
#282119=CARTESIAN_POINT('Ctrl Pts',(-7.79653168774416,12.2,-8.26900360426582));
#282120=CARTESIAN_POINT('Ctrl Pts',(-7.79315634862753,12.2,-8.26763143273325));
#282121=CARTESIAN_POINT('Ctrl Pts',(-7.78978896557149,12.2,-8.26625794518364));
#282122=CARTESIAN_POINT('Ctrl Pts',(-7.78642956000099,12.2,-8.26488317869199));
#282123=CARTESIAN_POINT('Ctrl Pts',(-7.78307015504078,12.2,-8.26350841245009));
#282124=CARTESIAN_POINT('Ctrl Pts',(-7.77971872771451,12.2,-8.26213236773578));
#282125=CARTESIAN_POINT('Ctrl Pts',(-7.77637529858655,12.2,-8.26075508096688));
#282126=CARTESIAN_POINT('Ctrl Pts',(-7.77303186945859,12.2,-8.25937779419796));
#282127=CARTESIAN_POINT('Ctrl Pts',(-7.76969643988251,12.2,-8.25799926661625));
#282128=CARTESIAN_POINT('Ctrl Pts',(-7.76636902892078,12.2,-8.25661953533294));
#282129=CARTESIAN_POINT('Ctrl Pts',(-7.76304161795905,12.2,-8.25523980404964));
#282130=CARTESIAN_POINT('Ctrl Pts',(-7.75972222642969,12.2,-8.25385886876648));
#282131=CARTESIAN_POINT('Ctrl Pts',(-7.75641087500833,12.2,-8.25247676752503));
#282132=CARTESIAN_POINT('Ctrl Pts',(-7.75309952358697,12.2,-8.25109466628356));
#282133=CARTESIAN_POINT('Ctrl Pts',(-7.7497962130903,12.2,-8.24971139966717));
#282134=CARTESIAN_POINT('Ctrl Pts',(-7.74650096408431,12.2,-8.2483270049259));
#282135=CARTESIAN_POINT('Ctrl Pts',(-7.74320571507833,12.2,-8.24694261018463));
#282136=CARTESIAN_POINT('Ctrl Pts',(-7.73991852723015,12.2,-8.24555708680177));
#282137=CARTESIAN_POINT('Ctrl Pts',(-7.73663942172319,12.2,-8.24417047501897));
#282138=CARTESIAN_POINT('Ctrl Pts',(-7.73336031562052,12.2,-8.24278386298426));
#282139=CARTESIAN_POINT('Ctrl Pts',(-7.73008929189515,12.2,-8.24139616141592));
#282140=CARTESIAN_POINT('Ctrl Pts',(-7.72682637179704,12.2,-8.24000740846395));
#282141=CARTESIAN_POINT('Ctrl Pts',(-7.7235634522917,12.2,-8.23861865576426));
#282142=CARTESIAN_POINT('Ctrl Pts',(-7.72030863636521,12.2,-8.23722885299999));
#282143=CARTESIAN_POINT('Ctrl Pts',(-7.71706194515526,12.2,-8.23583803777259));
#282144=CARTESIAN_POINT('Ctrl Pts',(-7.7138152539453,12.2,-8.23444722254519));
#282145=CARTESIAN_POINT('Ctrl Pts',(-7.71057668662994,12.2,-8.23305539574767));
#282146=CARTESIAN_POINT('Ctrl Pts',(-7.70734626516469,12.2,-8.23166259604819));
#282147=CARTESIAN_POINT('Ctrl Pts',(-7.70411584369943,12.2,-8.23026979634871));
#282148=CARTESIAN_POINT('Ctrl Pts',(-7.70089356871654,12.2,-8.22887602369935));
#282149=CARTESIAN_POINT('Ctrl Pts',(-7.69767945979166,12.2,-8.22748131750002));
#282150=CARTESIAN_POINT('Ctrl Pts',(-7.69446535086678,12.2,-8.2260866113007));
#282151=CARTESIAN_POINT('Ctrl Pts',(-7.69125940849989,12.2,-8.22469097263474));
#282152=CARTESIAN_POINT('Ctrl Pts',(-7.68806165453202,12.2,-8.22329443993556));
#282153=CARTESIAN_POINT('Ctrl Pts',(-7.68486390056416,12.2,-8.22189790723637));
#282154=CARTESIAN_POINT('Ctrl Pts',(-7.68167433502656,12.2,-8.22050048050616));
#282155=CARTESIAN_POINT('Ctrl Pts',(-7.67849297785725,12.2,-8.21910220023721));
#282156=CARTESIAN_POINT('Ctrl Pts',(-7.67531162068794,12.2,-8.21770391996824));
#282157=CARTESIAN_POINT('Ctrl Pts',(-7.67213847240943,12.2,-8.21630478603757));
#282158=CARTESIAN_POINT('Ctrl Pts',(-7.66897355443996,12.2,-8.21490483879688));
#282159=CARTESIAN_POINT('Ctrl Pts',(-7.66580863589553,12.2,-8.21350489130186));
#282160=CARTESIAN_POINT('Ctrl Pts',(-7.66265194833678,12.2,-8.21210413009828));
#282161=CARTESIAN_POINT('Ctrl Pts',(-7.65950351133866,12.2,-8.21070259572783));
#282162=CARTESIAN_POINT('Ctrl Pts',(-7.65635507491252,12.2,-8.20930106161198));
#282163=CARTESIAN_POINT('Ctrl Pts',(-7.65321489037758,12.2,-8.20789875536284));
#282164=CARTESIAN_POINT('Ctrl Pts',(-7.65008297840876,12.2,-8.20649571628874));
#282165=CARTESIAN_POINT('Ctrl Pts',(-7.64695106643993,12.2,-8.20509267721465));
#282166=CARTESIAN_POINT('Ctrl Pts',(-7.64382742716476,12.2,-8.20368890713743));
#282167=CARTESIAN_POINT('Ctrl Pts',(-7.64071208126384,12.2,-8.20228444497374));
#282168=CARTESIAN_POINT('Ctrl Pts',(-7.63759673536292,12.2,-8.20087998281006));
#282169=CARTESIAN_POINT('Ctrl Pts',(-7.63448968465434,12.2,-8.19947482942327));
#282170=CARTESIAN_POINT('Ctrl Pts',(-7.63139094775282,12.2,-8.19806902675963));
#282171=CARTESIAN_POINT('Ctrl Pts',(-7.62829221085129,12.2,-8.19666322409599));
#282172=CARTESIAN_POINT('Ctrl Pts',(-7.6252017895415,12.2,-8.1952567725022));
#282173=CARTESIAN_POINT('Ctrl Pts',(-7.62211970461109,12.2,-8.19384971188671));
#282174=CARTESIAN_POINT('Ctrl Pts',(-7.61903761968067,12.2,-8.19244265127122));
#282175=CARTESIAN_POINT('Ctrl Pts',(-7.61596387180803,12.2,-8.19103498302244));
#282176=CARTESIAN_POINT('Ctrl Pts',(-7.6128984808766,12.2,-8.18962674882368));
#282177=CARTESIAN_POINT('Ctrl Pts',(-7.60983308938827,12.2,-8.18821851436909));
#282178=CARTESIAN_POINT('Ctrl Pts',(-7.60677605614401,12.2,-8.18680971328102));
#282179=CARTESIAN_POINT('Ctrl Pts',(-7.60372740161874,12.2,-8.18540038845112));
#282180=CARTESIAN_POINT('Ctrl Pts',(-7.60067874764731,12.2,-8.18399106387725));
#282181=CARTESIAN_POINT('Ctrl Pts',(-7.59763847248716,12.2,-8.18258121676309));
#282182=CARTESIAN_POINT('Ctrl Pts',(-7.59460659786349,12.2,-8.18117088670215));
#282183=CARTESIAN_POINT('Ctrl Pts',(-7.59157472323982,12.2,-8.17976055664121));
#282184=CARTESIAN_POINT('Ctrl Pts',(-7.58855124891122,12.2,-8.17834974691161));
#282185=CARTESIAN_POINT('Ctrl Pts',(-7.58553619685484,12.2,-8.17693849783785));
#282186=CARTESIAN_POINT('Ctrl Pts',(-7.58151612762892,12.2,-8.17505683249163));
#282187=CARTESIAN_POINT('Ctrl Pts',(-7.57751103041939,12.2,-8.17317438777057));
#282188=CARTESIAN_POINT('Ctrl Pts',(-7.57352095591071,12.2,-8.17129126625791));
#282189=CARTESIAN_POINT('Ctrl Pts',(-7.56953088085838,12.2,-8.16940814448868));
#282190=CARTESIAN_POINT('Ctrl Pts',(-7.56555582840605,12.2,-8.16752434579888));
#282191=CARTESIAN_POINT('Ctrl Pts',(-7.56159585000564,12.2,-8.1656399734654));
#282192=CARTESIAN_POINT('Ctrl Pts',(-7.55763587214477,12.2,-8.16375560138867));
#282193=CARTESIAN_POINT('Ctrl Pts',(-7.55369096720059,12.2,-8.16187065609021));
#282194=CARTESIAN_POINT('Ctrl Pts',(-7.54976118740919,12.2,-8.15998524129995));
#282195=CARTESIAN_POINT('Ctrl Pts',(-7.54583140708236,12.2,-8.1580998262528));
#282196=CARTESIAN_POINT('Ctrl Pts',(-7.54191675189306,12.2,-8.15621394142504));
#282197=CARTESIAN_POINT('Ctrl Pts',(-7.53801727095833,12.2,-8.15432769376669));
#282198=CARTESIAN_POINT('Ctrl Pts',(-7.53411779002358,12.2,-8.15244144610833));
#282199=CARTESIAN_POINT('Ctrl Pts',(-7.53023348535174,12.2,-8.15055483317495));
#282200=CARTESIAN_POINT('Ctrl Pts',(-7.5263644076424,12.2,-8.14866796468318));
#282201=CARTESIAN_POINT('Ctrl Pts',(-7.52249533046023,12.2,-8.1467810964485));
#282202=CARTESIAN_POINT('Ctrl Pts',(-7.51864147918963,12.2,-8.14489397017781));
#282203=CARTESIAN_POINT('Ctrl Pts',(-7.51480290548595,12.2,-8.14300669476797));
#282204=CARTESIAN_POINT('Ctrl Pts',(-7.51096433125928,12.2,-8.141119419101));
#282205=CARTESIAN_POINT('Ctrl Pts',(-7.50714103620837,12.2,-8.13923199231373));
#282206=CARTESIAN_POINT('Ctrl Pts',(-7.50333306916907,12.2,-8.13734452593308));
#282207=CARTESIAN_POINT('Ctrl Pts',(-7.4995251026486,12.2,-8.1354570598096));
#282208=CARTESIAN_POINT('Ctrl Pts',(-7.49573246448723,12.2,-8.13356955182223));
#282209=CARTESIAN_POINT('Ctrl Pts',(-7.4919552078506,12.2,-8.13168211242098));
#282210=CARTESIAN_POINT('Ctrl Pts',(-7.48817795069932,12.2,-8.12979467276257));
#282211=CARTESIAN_POINT('Ctrl Pts',(-7.48441607204093,12.2,-8.12790730106497));
#282212=CARTESIAN_POINT('Ctrl Pts',(-7.48066962620645,12.2,-8.12602010870117));
#282213=CARTESIAN_POINT('Ctrl Pts',(-7.47692318088242,12.2,-8.1241329165945));
#282214=CARTESIAN_POINT('Ctrl Pts',(-7.4731921677234,12.2,-8.12224590358893));
#282215=CARTESIAN_POINT('Ctrl Pts',(-7.46947663780388,12.2,-8.12035918218759));
#282216=CARTESIAN_POINT('Ctrl Pts',(-7.46576110737813,12.2,-8.11847246052918));
#282217=CARTESIAN_POINT('Ctrl Pts',(-7.46206105915984,12.2,-8.1165860293236));
#282218=CARTESIAN_POINT('Ctrl Pts',(-7.45837654618227,12.2,-8.1147000023875));
#282219=CARTESIAN_POINT('Ctrl Pts',(-7.45469203370671,12.2,-8.11281397570838));
#282220=CARTESIAN_POINT('Ctrl Pts',(-7.4510230568293,12.2,-8.11092835183589));
#282221=CARTESIAN_POINT('Ctrl Pts',(-7.4473696655552,12.2,-8.10904324700689));
#282222=CARTESIAN_POINT('Ctrl Pts',(-7.44371627378333,12.2,-8.10715814192103));
#282223=CARTESIAN_POINT('Ctrl Pts',(-7.44007846809209,12.2,-8.10527355415142));
#282224=CARTESIAN_POINT('Ctrl Pts',(-7.43645630172902,12.2,-8.10338960110433));
#282225=CARTESIAN_POINT('Ctrl Pts',(-7.43283413585948,12.2,-8.10150564831394));
#282226=CARTESIAN_POINT('Ctrl Pts',(-7.42922760845351,12.2,-8.0996223269651));
#282227=CARTESIAN_POINT('Ctrl Pts',(-7.42563677057877,12.2,-8.09773975634114));
#282228=CARTESIAN_POINT('Ctrl Pts',(-7.42204593221477,12.2,-8.09585718546067));
#282229=CARTESIAN_POINT('Ctrl Pts',(-7.41847078438843,12.2,-8.0939753645803));
#282230=CARTESIAN_POINT('Ctrl Pts',(-7.41491137874999,12.2,-8.09209441103335));
#282231=CARTESIAN_POINT('Ctrl Pts',(-7.41135197311155,12.2,-8.09021345748639));
#282232=CARTESIAN_POINT('Ctrl Pts',(-7.4078083084694,12.2,-8.08833337134231));
#282233=CARTESIAN_POINT('Ctrl Pts',(-7.40428043938986,12.2,-8.08645427118445));
#282234=CARTESIAN_POINT('Ctrl Pts',(-7.40075257079099,12.2,-8.08457517128261));
#282235=CARTESIAN_POINT('Ctrl Pts',(-7.39724049557693,12.2,-8.08269705748415));
#282236=CARTESIAN_POINT('Ctrl Pts',(-7.39374426773571,12.2,-8.08082005018462));
#282237=CARTESIAN_POINT('Ctrl Pts',(-7.39024803941813,12.2,-8.07894304262935));
#282238=CARTESIAN_POINT('Ctrl Pts',(-7.38676765735409,12.2,-8.07706714246778));
#282239=CARTESIAN_POINT('Ctrl Pts',(-7.38330317316689,12.2,-8.07519246847683));
#282240=CARTESIAN_POINT('Ctrl Pts',(-7.37983868945174,12.2,-8.07331779474132));
#282241=CARTESIAN_POINT('Ctrl Pts',(-7.3763901061623,12.2,-8.07144435001955));
#282242=CARTESIAN_POINT('Ctrl Pts',(-7.37295747299743,12.2,-8.06957225489473));
#282243=CARTESIAN_POINT('Ctrl Pts',(-7.36952483936486,12.2,-8.06770015951484));
#282244=CARTESIAN_POINT('Ctrl Pts',(-7.36610815729102,12.2,-8.06582941485169));
#282245=CARTESIAN_POINT('Ctrl Pts',(-7.36270747821495,12.2,-8.06396014454544));
#282246=CARTESIAN_POINT('Ctrl Pts',(-7.35930679960223,12.2,-8.06209087449389));
#282247=CARTESIAN_POINT('Ctrl Pts',(-7.35592212564285,12.2,-8.06022307811124));
#282248=CARTESIAN_POINT('Ctrl Pts',(-7.35255350775053,12.2,-8.05835688215259));
#282249=CARTESIAN_POINT('Ctrl Pts',(-7.34918488939922,12.2,-8.05649068593966));
#282250=CARTESIAN_POINT('Ctrl Pts',(-7.34583232715261,12.2,-8.05462608910192));
#282251=CARTESIAN_POINT('Ctrl Pts',(-7.34249587419406,12.2,-8.0527632183894));
#282252=CARTESIAN_POINT('Ctrl Pts',(-7.33915942169009,12.2,-8.0509003479307));
#282253=CARTESIAN_POINT('Ctrl Pts',(-7.33583907811755,12.2,-8.04903920397751));
#282254=CARTESIAN_POINT('Ctrl Pts',(-7.33253489672121,12.2,-8.04717991403648));
#282255=CARTESIAN_POINT('Ctrl Pts',(-7.32923071487467,12.2,-8.04532062384212));
#282256=CARTESIAN_POINT('Ctrl Pts',(-7.32594269547659,12.2,-8.04346318794932));
#282257=CARTESIAN_POINT('Ctrl Pts',(-7.32267088996601,12.2,-8.04160773584834));
#282258=CARTESIAN_POINT('Ctrl Pts',(-7.31939908490122,12.2,-8.03975228400016));
#282259=CARTESIAN_POINT('Ctrl Pts',(-7.3161434951248,12.2,-8.03789881556546));
#282260=CARTESIAN_POINT('Ctrl Pts',(-7.31290417455464,12.2,-8.03604746232771));
#282261=CARTESIAN_POINT('Ctrl Pts',(-7.3096648535431,12.2,-8.03419610883771));
#282262=CARTESIAN_POINT('Ctrl Pts',(-7.3064417995482,12.2,-8.03234686841334));
#282263=CARTESIAN_POINT('Ctrl Pts',(-7.30323506724781,12.2,-8.03049987574875));
#282264=CARTESIAN_POINT('Ctrl Pts',(-7.30002833538435,12.2,-8.02865288333581));
#282265=CARTESIAN_POINT('Ctrl Pts',(-7.29683792555837,12.2,-8.02680813845364));
#282266=CARTESIAN_POINT('Ctrl Pts',(-7.29366388976062,12.2,-8.02496577332624));
#282267=CARTESIAN_POINT('Ctrl Pts',(-7.29048985353041,12.2,-8.0231234079478));
#282268=CARTESIAN_POINT('Ctrl Pts',(-7.28733219257952,12.2,-8.02128342287237));
#282269=CARTESIAN_POINT('Ctrl Pts',(-7.28419096024165,12.2,-8.01944595355));
#282270=CARTESIAN_POINT('Ctrl Pts',(-7.28104972790377,12.2,-8.01760848422763));
#282271=CARTESIAN_POINT('Ctrl Pts',(-7.27792492280393,12.2,-8.01577353110556));
#282272=CARTESIAN_POINT('Ctrl Pts',(-7.27481660052511,12.2,-8.01394123045042));
#282273=CARTESIAN_POINT('Ctrl Pts',(-7.2717082786698,12.2,-8.01210893004493));
#282274=CARTESIAN_POINT('Ctrl Pts',(-7.26861643917305,12.2,-8.01027928238799));
#282275=CARTESIAN_POINT('Ctrl Pts',(-7.26554113524376,12.2,-8.00845242475125));
#282276=CARTESIAN_POINT('Ctrl Pts',(-7.26246583089545,12.2,-8.00662556686559));
#282277=CARTESIAN_POINT('Ctrl Pts',(-7.2594070613084,12.2,-8.00480150117622));
#282278=CARTESIAN_POINT('Ctrl Pts',(-7.25636488297762,12.2,-8.00298036524392));
#282279=CARTESIAN_POINT('Ctrl Pts',(-7.25332270506134,12.2,-8.00115922955977));
#282280=CARTESIAN_POINT('Ctrl Pts',(-7.25029711703457,12.2,-7.99934102533912));
#282281=CARTESIAN_POINT('Ctrl Pts',(-7.24728817194613,12.2,-7.99752589293175));
#282282=CARTESIAN_POINT('Ctrl Pts',(-7.24277475410848,12.2,-7.99480319419703));
#282283=CARTESIAN_POINT('Ctrl Pts',(-7.23829878510839,12.2,-7.99208740894731));
#282284=CARTESIAN_POINT('Ctrl Pts',(-7.23386044993378,12.2,-7.98937901854522));
#282285=CARTESIAN_POINT('Ctrl Pts',(-7.23090155954861,12.2,-7.98757342477982));
#282286=CARTESIAN_POINT('Ctrl Pts',(-7.22795939422332,12.2,-7.98577111992305));
#282287=CARTESIAN_POINT('Ctrl Pts',(-7.22503400800832,12.2,-7.98397224799167));
#282288=CARTESIAN_POINT('Ctrl Pts',(-7.22210862179332,12.2,-7.98217337606029));
#282289=CARTESIAN_POINT('Ctrl Pts',(-7.21920001571086,12.2,-7.98037793704044));
#282290=CARTESIAN_POINT('Ctrl Pts',(-7.21630824477718,12.2,-7.97858607966536));
#282291=CARTESIAN_POINT('Ctrl Pts',(-7.21341647423752,12.2,-7.97679422253443));
#282292=CARTESIAN_POINT('Ctrl Pts',(-7.210541537323,12.2,-7.97500594559678));
#282293=CARTESIAN_POINT('Ctrl Pts',(-7.20768349071027,12.2,-7.97322139873455));
#282294=CARTESIAN_POINT('Ctrl Pts',(-7.20482544370815,12.2,-7.97143685162918));
#282295=CARTESIAN_POINT('Ctrl Pts',(-7.20198428635432,12.2,-7.96965603490592));
#282296=CARTESIAN_POINT('Ctrl Pts',(-7.19916007281324,12.2,-7.96787909847614));
#282297=CARTESIAN_POINT('Ctrl Pts',(-7.19562980607929,12.2,-7.96565792805996));
#282298=CARTESIAN_POINT('Ctrl Pts',(-7.192126014643,12.2,-7.96344282174945));
#282299=CARTESIAN_POINT('Ctrl Pts',(-7.18864880777018,12.2,-7.96123407869443));
#282300=CARTESIAN_POINT('Ctrl Pts',(-7.18517160127638,12.2,-7.95902533588016));
#282301=CARTESIAN_POINT('Ctrl Pts',(-7.1817209772268,12.2,-7.95682295612061));
#282302=CARTESIAN_POINT('Ctrl Pts',(-7.17829704572285,12.2,-7.95462724184554));
#282303=CARTESIAN_POINT('Ctrl Pts',(-7.1748731138457,12.2,-7.95243152733112));
#282304=CARTESIAN_POINT('Ctrl Pts',(-7.17147587422639,12.2,-7.95024247967488));
#282305=CARTESIAN_POINT('Ctrl Pts',(-7.16810543422419,12.2,-7.94806040599375));
#282306=CARTESIAN_POINT('Ctrl Pts',(-7.16473499422198,12.2,-7.94587833231261));
#282307=CARTESIAN_POINT('Ctrl Pts',(-7.16139135518046,12.2,-7.94370323307859));
#282308=CARTESIAN_POINT('Ctrl Pts',(-7.15807462594216,12.2,-7.94153542175855));
#282309=CARTESIAN_POINT('Ctrl Pts',(-7.15475789670386,12.2,-7.93936761043851));
#282310=CARTESIAN_POINT('Ctrl Pts',(-7.15146807792705,12.2,-7.93720708489693));
#282311=CARTESIAN_POINT('Ctrl Pts',(-7.14820527838718,12.2,-7.93505416673328));
#282312=CARTESIAN_POINT('Ctrl Pts',(-7.1449424788473,12.2,-7.93290124856964));
#282313=CARTESIAN_POINT('Ctrl Pts',(-7.14170669717808,12.2,-7.93075593470691));
#282314=CARTESIAN_POINT('Ctrl Pts',(-7.13849804696834,12.2,-7.92861854866483));
#282315=CARTESIAN_POINT('Ctrl Pts',(-7.1352893967586,12.2,-7.92648116262276));
#282316=CARTESIAN_POINT('Ctrl Pts',(-7.13210787598566,12.2,-7.92435170576144));
#282317=CARTESIAN_POINT('Ctrl Pts',(-7.12895359591477,12.2,-7.92223050541377));
#282318=CARTESIAN_POINT('Ctrl Pts',(-7.12579931584389,12.2,-7.9201093050661));
#282319=CARTESIAN_POINT('Ctrl Pts',(-7.12267227614361,12.2,-7.91799636081627));
#282320=CARTESIAN_POINT('Ctrl Pts',(-7.11957258856001,12.2,-7.91589200650114));
#282321=CARTESIAN_POINT('Ctrl Pts',(-7.11647290097642,12.2,-7.91378765218601));
#282322=CARTESIAN_POINT('Ctrl Pts',(-7.11340056493333,12.2,-7.91169188988889));
#282323=CARTESIAN_POINT('Ctrl Pts',(-7.11035569243332,12.2,-7.90960505474999));
#282324=CARTESIAN_POINT('Ctrl Pts',(-7.1073108199333,12.2,-7.9075182196111));
#282325=CARTESIAN_POINT('Ctrl Pts',(-7.1042934119952,12.2,-7.90544031415824));
#282326=CARTESIAN_POINT('Ctrl Pts',(-7.10130358094003,12.2,-7.90337168227387));
#282327=CARTESIAN_POINT('Ctrl Pts',(-7.09831374988486,12.2,-7.9013030503895));
#282328=CARTESIAN_POINT('Ctrl Pts',(-7.09535149272347,12.2,-7.89924369204327));
#282329=CARTESIAN_POINT('Ctrl Pts',(-7.09241692751658,12.2,-7.89719395780768));
#282330=CARTESIAN_POINT('Ctrl Pts',(-7.08948236230969,12.2,-7.89514422357207));
#282331=CARTESIAN_POINT('Ctrl Pts',(-7.08657548391596,12.2,-7.89310411410564));
#282332=CARTESIAN_POINT('Ctrl Pts',(-7.08369641127853,12.2,-7.89107398563395));
#282333=CARTESIAN_POINT('Ctrl Pts',(-7.08081733864111,12.2,-7.88904385716226));
#282334=CARTESIAN_POINT('Ctrl Pts',(-7.07796606838923,12.2,-7.88702370822752));
#282335=CARTESIAN_POINT('Ctrl Pts',(-7.07514271568067,12.2,-7.88501390305838));
#282336=CARTESIAN_POINT('Ctrl Pts',(-7.07231936297211,12.2,-7.88300409788925));
#282337=CARTESIAN_POINT('Ctrl Pts',(-7.06952392673015,12.2,-7.88100463642787));
#282338=CARTESIAN_POINT('Ctrl Pts',(-7.06675652562136,12.2,-7.8790158864982));
#282339=CARTESIAN_POINT('Ctrl Pts',(-7.06398912451256,12.2,-7.87702713656852));
#282340=CARTESIAN_POINT('Ctrl Pts',(-7.06124975452084,12.2,-7.87504909936403));
#282341=CARTESIAN_POINT('Ctrl Pts',(-7.05853853362037,12.2,-7.87308214943438));
#282342=CARTESIAN_POINT('Ctrl Pts',(-7.05528506865801,12.2,-7.87072180960457));
#282343=CARTESIAN_POINT('Ctrl Pts',(-7.05207213696025,12.2,-7.8683774363129));
#282344=CARTESIAN_POINT('Ctrl Pts',(-7.04889994107727,12.2,-7.86604968864819));
#282345=CARTESIAN_POINT('Ctrl Pts',(-7.0457277451943,12.2,-7.86372194098349));
#282346=CARTESIAN_POINT('Ctrl Pts',(-7.04259628549976,12.2,-7.86141082187582));
#282347=CARTESIAN_POINT('Ctrl Pts',(-7.03950576269359,12.2,-7.85911700512507));
#282348=CARTESIAN_POINT('Ctrl Pts',(-7.03641523988741,12.2,-7.85682318837432));
#282349=CARTESIAN_POINT('Ctrl Pts',(-7.03336565587143,12.2,-7.854546673907));
#282350=CARTESIAN_POINT('Ctrl Pts',(-7.03035721681124,12.2,-7.85228815323783));
#282351=CARTESIAN_POINT('Ctrl Pts',(-7.02734877747779,12.2,-7.8500296323635));
#282352=CARTESIAN_POINT('Ctrl Pts',(-7.02438147990668,12.2,-7.84778910417424));
#282353=CARTESIAN_POINT('Ctrl Pts',(-7.02145553283236,12.2,-7.84556727813731));
#282354=CARTESIAN_POINT('Ctrl Pts',(-7.01852958602383,12.2,-7.84334545230219));
#282355=CARTESIAN_POINT('Ctrl Pts',(-7.0156449897193,12.2,-7.84114232482326));
#282356=CARTESIAN_POINT('Ctrl Pts',(-7.01280195172628,12.2,-7.83895861847598));
#282357=CARTESIAN_POINT('Ctrl Pts',(-7.00995891373326,12.2,-7.83677491212871));
#282358=CARTESIAN_POINT('Ctrl Pts',(-7.00715743354507,12.2,-7.83461062967385));
#282359=CARTESIAN_POINT('Ctrl Pts',(-7.00439772355913,12.2,-7.83246650725036));
#282360=CARTESIAN_POINT('Ctrl Pts',(-7.00163801332253,12.2,-7.83032238463211));
#282361=CARTESIAN_POINT('Ctrl Pts',(-6.99892007034333,12.2,-7.82819842264841));
#282362=CARTESIAN_POINT('Ctrl Pts',(-6.99624410998289,12.2,-7.82609537709659));
#282363=CARTESIAN_POINT('Ctrl Pts',(-6.99356814986552,12.2,-7.82399233173581));
#282364=CARTESIAN_POINT('Ctrl Pts',(-6.99093417092248,12.2,-7.82191020433345));
#282365=CARTESIAN_POINT('Ctrl Pts',(-6.98834238801665,12.2,-7.81984976799165));
#282366=CARTESIAN_POINT('Ctrl Pts',(-6.98575060511082,12.2,-7.81778933164984));
#282367=CARTESIAN_POINT('Ctrl Pts',(-6.98320101896006,12.2,-7.81575058769804));
#282368=CARTESIAN_POINT('Ctrl Pts',(-6.98069384429828,12.2,-7.81373432576976));
#282369=CARTESIAN_POINT('Ctrl Pts',(-6.97818666940873,12.2,-7.81171806365833));
#282370=CARTESIAN_POINT('Ctrl Pts',(-6.97572190940799,12.2,-7.80972428723889));
#282371=CARTESIAN_POINT('Ctrl Pts',(-6.97329978024078,12.2,-7.80775380678441));
#282372=CARTESIAN_POINT('Ctrl Pts',(-6.97087765129358,12.2,-7.80578332650892));
#282373=CARTESIAN_POINT('Ctrl Pts',(-6.96849815374008,12.2,-7.80383614243011));
#282374=CARTESIAN_POINT('Ctrl Pts',(-6.96616151174164,12.2,-7.80191308849997));
#282375=CARTESIAN_POINT('Ctrl Pts',(-6.96382486974319,12.2,-7.79999003456982));
#282376=CARTESIAN_POINT('Ctrl Pts',(-6.96153108101764,12.2,-7.79809111005829));
#282377=CARTESIAN_POINT('Ctrl Pts',(-6.95928037098448,12.2,-7.79621716819798));
#282378=CARTESIAN_POINT('Ctrl Pts',(-6.95702966074689,12.2,-7.79434322616746));
#282379=CARTESIAN_POINT('Ctrl Pts',(-6.95482202850409,12.2,-7.79249426894052));
#282380=CARTESIAN_POINT('Ctrl Pts',(-6.95265770247241,12.2,-7.79067117009293));
#282381=CARTESIAN_POINT('Ctrl Pts',(-6.95049337663734,12.2,-7.78884807141093));
#282382=CARTESIAN_POINT('Ctrl Pts',(-6.94837235616622,12.2,-7.78705083291782));
#282383=CARTESIAN_POINT('Ctrl Pts',(-6.94629487223237,12.2,-7.78528035222416));
#282384=CARTESIAN_POINT('Ctrl Pts',(-6.94421738829851,12.2,-7.7835098715305));
#282385=CARTESIAN_POINT('Ctrl Pts',(-6.94218344007158,12.2,-7.78176615019914));
#282386=CARTESIAN_POINT('Ctrl Pts',(-6.94019326030863,12.2,-7.7800501105936));
#282387=CARTESIAN_POINT('Ctrl Pts',(-6.93820308036491,12.2,-7.7783340708322));
#282388=CARTESIAN_POINT('Ctrl Pts',(-6.93625667117666,12.2,-7.77664571293258));
#282389=CARTESIAN_POINT('Ctrl Pts',(-6.93435426707596,12.2,-7.77498598526073));
#282390=CARTESIAN_POINT('Ctrl Pts',(-6.93245186314808,12.2,-7.77332625773965));
#282391=CARTESIAN_POINT('Ctrl Pts',(-6.93059346418344,12.2,-7.77169516153665));
#282392=CARTESIAN_POINT('Ctrl Pts',(-6.92877931141796,12.2,-7.77009366842948));
#282393=CARTESIAN_POINT('Ctrl Pts',(-6.92696515865248,12.2,-7.7684921753223));
#282394=CARTESIAN_POINT('Ctrl Pts',(-6.92519525247513,12.2,-7.76692029032111));
#282395=CARTESIAN_POINT('Ctrl Pts',(-6.9234698356192,12.2,-7.76537901112575));
#282396=CARTESIAN_POINT('Ctrl Pts',(-6.92174441876326,12.2,-7.76383773193041));
#282397=CARTESIAN_POINT('Ctrl Pts',(-6.92006349083027,12.2,-7.76232705999294));
#282398=CARTESIAN_POINT('Ctrl Pts',(-6.91842730097,12.2,-7.76084802787785));
#282399=CARTESIAN_POINT('Ctrl Pts',(-6.91679111096111,12.2,-7.7593689956284));
#282400=CARTESIAN_POINT('Ctrl Pts',(-6.91519965756486,12.2,-7.75792160234866));
#282401=CARTESIAN_POINT('Ctrl Pts',(-6.91365319364922,12.2,-7.75650690943966));
#282402=CARTESIAN_POINT('Ctrl Pts',(-6.91210672987404,12.2,-7.75509221665915));
#282403=CARTESIAN_POINT('Ctrl Pts',(-6.91060525482109,12.2,-7.75371022434943));
#282404=CARTESIAN_POINT('Ctrl Pts',(-6.90914902603396,12.2,-7.75236202747556));
#282405=CARTESIAN_POINT('Ctrl Pts',(-6.90672896680257,12.2,-7.75012150296511));
#282406=CARTESIAN_POINT('Ctrl Pts',(-6.90443386327613,12.2,-7.74797428786345));
#282407=CARTESIAN_POINT('Ctrl Pts',(-6.90226492000006,12.2,-7.74592563800002));
#282408=CARTESIAN_POINT('Ctrl Pts',(-6.90226492000006,15.2,-7.74592563800002));
#282409=CARTESIAN_POINT('Ctrl Pts',(-6.90356378046103,15.2,-7.7471524613731));
#282410=CARTESIAN_POINT('Ctrl Pts',(-6.90490788387611,15.2,-7.74841464066746));
#282411=CARTESIAN_POINT('Ctrl Pts',(-6.90629697189785,15.2,-7.74971102657464));
#282412=CARTESIAN_POINT('Ctrl Pts',(-6.90769275880418,15.2,-7.75101366430997));
#282413=CARTESIAN_POINT('Ctrl Pts',(-6.90913396276099,15.2,-7.75235084375419));
#282414=CARTESIAN_POINT('Ctrl Pts',(-6.91062032766887,15.2,-7.75372144989929));
#282415=CARTESIAN_POINT('Ctrl Pts',(-6.91210669244173,15.2,-7.7550920559199));
#282416=CARTESIAN_POINT('Ctrl Pts',(-6.9136382162239,15.2,-7.75649608786879));
#282417=CARTESIAN_POINT('Ctrl Pts',(-6.91521464499997,15.2,-7.75793246298329));
#282418=CARTESIAN_POINT('Ctrl Pts',(-6.91679107377605,15.2,-7.75936883809779));
#282419=CARTESIAN_POINT('Ctrl Pts',(-6.91841240636048,15.2,-7.76083755765297));
#282420=CARTESIAN_POINT('Ctrl Pts',(-6.9200783941306,15.2,-7.76233756883827));
#282421=CARTESIAN_POINT('Ctrl Pts',(-6.92174438205206,15.2,-7.76383758015982));
#282422=CARTESIAN_POINT('Ctrl Pts',(-6.92345502352597,15.2,-7.76536888232471));
#282423=CARTESIAN_POINT('Ctrl Pts',(-6.92521007345795,15.2,-7.76693045566184));
#282424=CARTESIAN_POINT('Ctrl Pts',(-6.92696512323052,15.2,-7.76849202885716));
#282425=CARTESIAN_POINT('Ctrl Pts',(-6.92876458116769,15.2,-7.77008387276886));
#282426=CARTESIAN_POINT('Ctrl Pts',(-6.93060820402582,15.2,-7.77170499321737));
#282427=CARTESIAN_POINT('Ctrl Pts',(-6.93245182688396,15.2,-7.77332611366589));
#282428=CARTESIAN_POINT('Ctrl Pts',(-6.93433961609195,15.2,-7.77497651296247));
#282429=CARTESIAN_POINT('Ctrl Pts',(-6.93627133093655,15.2,-7.77665522165026));
#282430=CARTESIAN_POINT('Ctrl Pts',(-6.9382030459566,15.2,-7.77833393049054));
#282431=CARTESIAN_POINT('Ctrl Pts',(-6.94017868920707,15.2,-7.78004095185096));
#282432=CARTESIAN_POINT('Ctrl Pts',(-6.94219802148676,15.2,-7.78177534369736));
#282433=CARTESIAN_POINT('Ctrl Pts',(-6.94421735358306,15.2,-7.78350973538623));
#282434=CARTESIAN_POINT('Ctrl Pts',(-6.94628037779796,15.2,-7.78527149973637));
#282435=CARTESIAN_POINT('Ctrl Pts',(-6.94838686063996,15.2,-7.7870597195892));
#282436=CARTESIAN_POINT('Ctrl Pts',(-6.95049334348198,15.2,-7.78884793944203));
#282437=CARTESIAN_POINT('Ctrl Pts',(-6.95264328442885,15.2,-7.79066261461775));
#282438=CARTESIAN_POINT('Ctrl Pts',(-6.9548364553473,15.2,-7.79250285638312));
#282439=CARTESIAN_POINT('Ctrl Pts',(-6.95702962626574,15.2,-7.79434309814849));
#282440=CARTESIAN_POINT('Ctrl Pts',(-6.9592660269873,15.2,-7.79620890371429));
#282441=CARTESIAN_POINT('Ctrl Pts',(-6.96154543173487,15.2,-7.79809940581058));
#282442=CARTESIAN_POINT('Ctrl Pts',(-6.96382483668951,15.2,-7.7999899080786));
#282443=CARTESIAN_POINT('Ctrl Pts',(-6.96614724335662,15.2,-7.80190510681569));
#282444=CARTESIAN_POINT('Ctrl Pts',(-6.96851243140407,15.2,-7.80384415508909));
#282445=CARTESIAN_POINT('Ctrl Pts',(-6.97087761923667,15.2,-7.80578320318635));
#282446=CARTESIAN_POINT('Ctrl Pts',(-6.97328558639354,15.2,-7.8077461019956));
#282447=CARTESIAN_POINT('Ctrl Pts',(-6.97573611148221,15.2,-7.80973202326574));
#282448=CARTESIAN_POINT('Ctrl Pts',(-6.97818663657087,15.2,-7.81171794453589));
#282449=CARTESIAN_POINT('Ctrl Pts',(-6.98067972228528,15.2,-7.81372688950389));
#282450=CARTESIAN_POINT('Ctrl Pts',(-6.9832151471903,15.2,-7.81575805176192));
#282451=CARTESIAN_POINT('Ctrl Pts',(-6.98575057232562,15.2,-7.81778921420446));
#282452=CARTESIAN_POINT('Ctrl Pts',(-6.98832833832333,15.2,-7.81984259528247));
#282453=CARTESIAN_POINT('Ctrl Pts',(-6.99094822838461,15.2,-7.82191740689648));
#282454=CARTESIAN_POINT('Ctrl Pts',(-6.99356811820792,15.2,-7.82399221832202));
#282455=CARTESIAN_POINT('Ctrl Pts',(-6.99623013164313,15.2,-7.82608846065803));
#282456=CARTESIAN_POINT('Ctrl Pts',(-6.99893405647376,15.2,-7.82820536700736));
#282457=CARTESIAN_POINT('Ctrl Pts',(-7.00163798130439,15.2,-7.83032227335668));
#282458=CARTESIAN_POINT('Ctrl Pts',(-7.00438381468365,15.2,-7.83245984109461));
#282459=CARTESIAN_POINT('Ctrl Pts',(-7.00717134841282,15.2,-7.83461732251482));
#282460=CARTESIAN_POINT('Ctrl Pts',(-7.00995888239519,15.2,-7.83677480413101));
#282461=CARTESIAN_POINT('Ctrl Pts',(-7.01278811455884,15.2,-7.83895219861528));
#282462=CARTESIAN_POINT('Ctrl Pts',(-7.01565883502779,15.2,-7.84114877167919));
#282463=CARTESIAN_POINT('Ctrl Pts',(-7.018529555236,15.2,-7.84334534454358));
#282464=CARTESIAN_POINT('Ctrl Pts',(-7.02144176517394,15.2,-7.84556109653948));
#282465=CARTESIAN_POINT('Ctrl Pts',(-7.02439525523331,15.2,-7.84779531304165));
#282466=CARTESIAN_POINT('Ctrl Pts',(-7.0273487452927,15.2,-7.85002952954382));
#282467=CARTESIAN_POINT('Ctrl Pts',(-7.03034351624243,15.2,-7.85228220670049));
#282468=CARTESIAN_POINT('Ctrl Pts',(-7.03337936319807,15.2,-7.85455264656372));
#282469=CARTESIAN_POINT('Ctrl Pts',(-7.03641521042948,15.2,-7.85682308663319));
#282470=CARTESIAN_POINT('Ctrl Pts',(-7.03949213200048,15.2,-7.85911128702447));
#282471=CARTESIAN_POINT('Ctrl Pts',(-7.04260992333984,15.2,-7.8614165649846));
#282472=CARTESIAN_POINT('Ctrl Pts',(-7.045727714396,15.2,-7.86372184273533));
#282473=CARTESIAN_POINT('Ctrl Pts',(-7.04888637774473,15.2,-7.86604419574202));
#282474=CARTESIAN_POINT('Ctrl Pts',(-7.05208570772644,15.2,-7.86838295450105));
#282475=CARTESIAN_POINT('Ctrl Pts',(-7.05528503770815,15.2,-7.87072171326007));
#282476=CARTESIAN_POINT('Ctrl Pts',(-7.05852503785898,15.2,-7.87307687564098));
#282477=CARTESIAN_POINT('Ctrl Pts',(-7.06180550207137,15.2,-7.87544778755417));
#282478=CARTESIAN_POINT('Ctrl Pts',(-7.06453922234769,15.2,-7.8774235475536));
#282479=CARTESIAN_POINT('Ctrl Pts',(-7.06730104553029,15.2,-7.87941024455887));
#282480=CARTESIAN_POINT('Ctrl Pts',(-7.0700908562927,15.2,-7.88140750462777));
#282481=CARTESIAN_POINT('Ctrl Pts',(-7.07288066705511,15.2,-7.88340476469665));
#282482=CARTESIAN_POINT('Ctrl Pts',(-7.07569846384115,15.2,-7.88541258855086));
#282483=CARTESIAN_POINT('Ctrl Pts',(-7.07854413225677,15.2,-7.88743061099056));
#282484=CARTESIAN_POINT('Ctrl Pts',(-7.0813898006724,15.2,-7.88944863343025));
#282485=CARTESIAN_POINT('Ctrl Pts',(-7.08426333932221,15.2,-7.89147685152221));
#282486=CARTESIAN_POINT('Ctrl Pts',(-7.08716463772498,15.2,-7.89351490825832));
#282487=CARTESIAN_POINT('Ctrl Pts',(-7.09006593612776,15.2,-7.89555296499443));
#282488=CARTESIAN_POINT('Ctrl Pts',(-7.0929949911381,15.2,-7.89760085926397));
#282489=CARTESIAN_POINT('Ctrl Pts',(-7.0959516905266,15.2,-7.89965823621778));
#282490=CARTESIAN_POINT('Ctrl Pts',(-7.0989083899151,15.2,-7.9017156131716));
#282491=CARTESIAN_POINT('Ctrl Pts',(-7.10189273333459,15.2,-7.90378247417979));
#282492=CARTESIAN_POINT('Ctrl Pts',(-7.10490460840547,15.2,-7.90585847015249));
#282493=CARTESIAN_POINT('Ctrl Pts',(-7.10791648347634,15.2,-7.90793446612519));
#282494=CARTESIAN_POINT('Ctrl Pts',(-7.11095589075484,15.2,-7.91001959731986));
#282495=CARTESIAN_POINT('Ctrl Pts',(-7.11402271520072,15.2,-7.91211352086199));
#282496=CARTESIAN_POINT('Ctrl Pts',(-7.1170895396466,15.2,-7.91420744440412));
#282497=CARTESIAN_POINT('Ctrl Pts',(-7.12018378327127,15.2,-7.9163101608446));
#282498=CARTESIAN_POINT('Ctrl Pts',(-7.12330533509578,15.2,-7.91842133372843));
#282499=CARTESIAN_POINT('Ctrl Pts',(-7.1264268869203,15.2,-7.92053250661227));
#282500=CARTESIAN_POINT('Ctrl Pts',(-7.12957574601321,15.2,-7.92265213501098));
#282501=CARTESIAN_POINT('Ctrl Pts',(-7.13275180039043,15.2,-7.92477988855331));
#282502=CARTESIAN_POINT('Ctrl Pts',(-7.13592785476766,15.2,-7.92690764209564));
#282503=CARTESIAN_POINT('Ctrl Pts',(-7.13913110641476,15.2,-7.92904352002977));
#282504=CARTESIAN_POINT('Ctrl Pts',(-7.14236144322252,15.2,-7.93118719628039));
#282505=CARTESIAN_POINT('Ctrl Pts',(-7.14559177967818,15.2,-7.93333087229737));
#282506=CARTESIAN_POINT('Ctrl Pts',(-7.14884920186948,15.2,-7.93548234663131));
#282507=CARTESIAN_POINT('Ctrl Pts',(-7.15213359907873,15.2,-7.93764129924261));
#282508=CARTESIAN_POINT('Ctrl Pts',(-7.15541799664599,15.2,-7.93980025208922));
#282509=CARTESIAN_POINT('Ctrl Pts',(-7.15872936978221,15.2,-7.94196668192182));
#282510=CARTESIAN_POINT('Ctrl Pts',(-7.16206760978002,15.2,-7.94414027324069));
#282511=CARTESIAN_POINT('Ctrl Pts',(-7.16540584977783,15.2,-7.94631386455955));
#282512=CARTESIAN_POINT('Ctrl Pts',(-7.1687709559585,15.2,-7.94849461763107));
#282513=CARTESIAN_POINT('Ctrl Pts',(-7.17216281783134,15.2,-7.95068222138053));
#282514=CARTESIAN_POINT('Ctrl Pts',(-7.17555467970418,15.2,-7.95286982512998));
#282515=CARTESIAN_POINT('Ctrl Pts',(-7.1789732998021,15.2,-7.95506427963502));
#282516=CARTESIAN_POINT('Ctrl Pts',(-7.18241856837514,15.2,-7.95726527849452));
#282517=CARTESIAN_POINT('Ctrl Pts',(-7.18586383694817,15.2,-7.95946627735403));
#282518=CARTESIAN_POINT('Ctrl Pts',(-7.18933575323386,15.2,-7.96167382010558));
#282519=CARTESIAN_POINT('Ctrl Pts',(-7.19283421003802,15.2,-7.96388760635526));
#282520=CARTESIAN_POINT('Ctrl Pts',(-7.19633266684219,15.2,-7.96610139260493));
#282521=CARTESIAN_POINT('Ctrl Pts',(-7.19985766398591,15.2,-7.96832142071588));
#282522=CARTESIAN_POINT('Ctrl Pts',(-7.20340909398455,15.2,-7.97054739460446));
#282523=CARTESIAN_POINT('Ctrl Pts',(-7.20625023813829,15.2,-7.97232817381238));
#282524=CARTESIAN_POINT('Ctrl Pts',(-7.20910829908769,15.2,-7.9741127577585));
#282525=CARTESIAN_POINT('Ctrl Pts',(-7.21198322216725,15.2,-7.97590099766784));
#282526=CARTESIAN_POINT('Ctrl Pts',(-7.2148581448551,15.2,-7.97768923733353));
#282527=CARTESIAN_POINT('Ctrl Pts',(-7.21774992864015,15.2,-7.97948113197249));
#282528=CARTESIAN_POINT('Ctrl Pts',(-7.22065852051237,15.2,-7.98127653360326));
#282529=CARTESIAN_POINT('Ctrl Pts',(-7.22356711278089,15.2,-7.98307193547865));
#282530=CARTESIAN_POINT('Ctrl Pts',(-7.22649251279589,15.2,-7.9848708442767));
#282531=CARTESIAN_POINT('Ctrl Pts',(-7.22943466495734,15.2,-7.9866731129307));
#282532=CARTESIAN_POINT('Ctrl Pts',(-7.23237681671792,15.2,-7.98847538133914));
#282533=CARTESIAN_POINT('Ctrl Pts',(-7.23533572015325,15.2,-7.99028101134255));
#282534=CARTESIAN_POINT('Ctrl Pts',(-7.23831132283497,15.2,-7.99208985522921));
#282535=CARTESIAN_POINT('Ctrl Pts',(-7.24203082649119,15.2,-7.99435091027237));
#282536=CARTESIAN_POINT('Ctrl Pts',(-7.24577642101596,15.2,-7.99661699101844));
#282537=CARTESIAN_POINT('Ctrl Pts',(-7.24954800032015,15.2,-7.99888781580985));
#282538=CARTESIAN_POINT('Ctrl Pts',(-7.25256526392795,15.2,-8.000704475742));
#282539=CARTESIAN_POINT('Ctrl Pts',(-7.25559915698775,15.2,-8.00252417225784));
#282540=CARTESIAN_POINT('Ctrl Pts',(-7.25864962726619,15.2,-8.00434676485736));
#282541=CARTESIAN_POINT('Ctrl Pts',(-7.26170009712902,15.2,-8.00616935720856));
#282542=CARTESIAN_POINT('Ctrl Pts',(-7.26476714392154,15.2,-8.00799484455141));
#282543=CARTESIAN_POINT('Ctrl Pts',(-7.26785071254431,15.2,-8.00982308899306));
#282544=CARTESIAN_POINT('Ctrl Pts',(-7.27093428158721,15.2,-8.01165133368381));
#282545=CARTESIAN_POINT('Ctrl Pts',(-7.27403437218955,15.2,-8.01348233304148));
#282546=CARTESIAN_POINT('Ctrl Pts',(-7.27715093247159,15.2,-8.0153159516416));
#282547=CARTESIAN_POINT('Ctrl Pts',(-7.28026749232901,15.2,-8.01714956999188));
#282548=CARTESIAN_POINT('Ctrl Pts',(-7.283400520347,15.2,-8.01898580619718));
#282549=CARTESIAN_POINT('Ctrl Pts',(-7.28654996347673,15.2,-8.02082452465771));
#282550=CARTESIAN_POINT('Ctrl Pts',(-7.28969940703557,15.2,-8.02266324336877));
#282551=CARTESIAN_POINT('Ctrl Pts',(-7.292865265517,15.2,-8.02450444388685));
#282552=CARTESIAN_POINT('Ctrl Pts',(-7.29604748576049,15.2,-8.02634799121793));
#282553=CARTESIAN_POINT('Ctrl Pts',(-7.29922970557041,15.2,-8.02819153829781));
#282554=CARTESIAN_POINT('Ctrl Pts',(-7.30242828572217,15.2,-8.03003743141303));
#282555=CARTESIAN_POINT('Ctrl Pts',(-7.3056431754577,15.2,-8.03188553920617));
#282556=CARTESIAN_POINT('Ctrl Pts',(-7.30885806563126,15.2,-8.03373364725113));
#282557=CARTESIAN_POINT('Ctrl Pts',(-7.31208926192854,15.2,-8.03558396869904));
#282558=CARTESIAN_POINT('Ctrl Pts',(-7.31533671421666,15.2,-8.03743637146668));
#282559=CARTESIAN_POINT('Ctrl Pts',(-7.31858416650477,15.2,-8.03928877423431));
#282560=CARTESIAN_POINT('Ctrl Pts',(-7.3218478750642,15.2,-8.04114325924939));
#282561=CARTESIAN_POINT('Ctrl Pts',(-7.32512778407793,15.2,-8.0429996952952));
#282562=CARTESIAN_POINT('Ctrl Pts',(-7.32840769264477,15.2,-8.04485613108806));
#282563=CARTESIAN_POINT('Ctrl Pts',(-7.33170380280908,15.2,-8.04671451783959));
#282564=CARTESIAN_POINT('Ctrl Pts',(-7.33501606199774,15.2,-8.04857472697374));
#282565=CARTESIAN_POINT('Ctrl Pts',(-7.3383283216377,15.2,-8.05043493636135));
#282566=CARTESIAN_POINT('Ctrl Pts',(-7.34165673003512,15.2,-8.05229696774187));
#282567=CARTESIAN_POINT('Ctrl Pts',(-7.34500123433016,15.2,-8.05416069328806));
#282568=CARTESIAN_POINT('Ctrl Pts',(-7.34834573816952,15.2,-8.05602441858032));
#282569=CARTESIAN_POINT('Ctrl Pts',(-7.35170633762062,15.2,-8.05788983861401));
#282570=CARTESIAN_POINT('Ctrl Pts',(-7.35508298073244,15.2,-8.0597568270724));
#282571=CARTESIAN_POINT('Ctrl Pts',(-7.35845962430432,15.2,-8.06162381578516));
#282572=CARTESIAN_POINT('Ctrl Pts',(-7.36185231054002,15.2,-8.06349237199257));
#282573=CARTESIAN_POINT('Ctrl Pts',(-7.36526098828637,15.2,-8.06536237218803));
#282574=CARTESIAN_POINT('Ctrl Pts',(-7.36866966556828,15.2,-8.06723237212871));
#282575=CARTESIAN_POINT('Ctrl Pts',(-7.37209433201785,15.2,-8.06910381485011));
#282576=CARTESIAN_POINT('Ctrl Pts',(-7.37553493773554,15.2,-8.07097657736359));
#282577=CARTESIAN_POINT('Ctrl Pts',(-7.37897554392202,15.2,-8.07284934013224));
#282578=CARTESIAN_POINT('Ctrl Pts',(-7.38243208706319,15.2,-8.07472342313161));
#282579=CARTESIAN_POINT('Ctrl Pts',(-7.38590451730901,15.2,-8.07659870217832));
#282580=CARTESIAN_POINT('Ctrl Pts',(-7.38937694708172,15.2,-8.07847398096954));
#282581=CARTESIAN_POINT('Ctrl Pts',(-7.39286526071272,15.2,-8.08035045800401));
#282582=CARTESIAN_POINT('Ctrl Pts',(-7.39636940876661,15.2,-8.08222801127757));
#282583=CARTESIAN_POINT('Ctrl Pts',(-7.39987355729795,15.2,-8.08410556480694));
#282584=CARTESIAN_POINT('Ctrl Pts',(-7.4033935392149,15.2,-8.0859841941234));
#282585=CARTESIAN_POINT('Ctrl Pts',(-7.40692930279752,15.2,-8.08786377967034));
#282586=CARTESIAN_POINT('Ctrl Pts',(-7.41046506589838,15.2,-8.08974336496119));
#282587=CARTESIAN_POINT('Ctrl Pts',(-7.41401661033778,15.2,-8.0916239070713));
#282588=CARTESIAN_POINT('Ctrl Pts',(-7.41758388293342,15.2,-8.09350528641741));
#282589=CARTESIAN_POINT('Ctrl Pts',(-7.42115115601511,15.2,-8.09538666601985));
#282590=CARTESIAN_POINT('Ctrl Pts',(-7.42473415948997,15.2,-8.09726888440849));
#282591=CARTESIAN_POINT('Ctrl Pts',(-7.42833283974166,15.2,-8.09915182273335));
#282592=CARTESIAN_POINT('Ctrl Pts',(-7.43193151999336,15.2,-8.1010347610582));
#282593=CARTESIAN_POINT('Ctrl Pts',(-7.4355458758802,15.2,-8.10291842034701));
#282594=CARTESIAN_POINT('Ctrl Pts',(-7.43917585880184,15.2,-8.10480268328309));
#282595=CARTESIAN_POINT('Ctrl Pts',(-7.4428058412289,15.2,-8.10668694596244));
#282596=CARTESIAN_POINT('Ctrl Pts',(-7.44645144939133,15.2,-8.10857181374707));
#282597=CARTESIAN_POINT('Ctrl Pts',(-7.45011262999751,15.2,-8.1104571709904));
#282598=CARTESIAN_POINT('Ctrl Pts',(-7.45377381110251,15.2,-8.1123425284906));
#282599=CARTESIAN_POINT('Ctrl Pts',(-7.45745056659253,15.2,-8.11422837511668));
#282600=CARTESIAN_POINT('Ctrl Pts',(-7.46114284362869,15.2,-8.11611459677508));
#282601=CARTESIAN_POINT('Ctrl Pts',(-7.46483512016178,15.2,-8.11800081817648));
#282602=CARTESIAN_POINT('Ctrl Pts',(-7.46854291870671,15.2,-8.11988741574448));
#282603=CARTESIAN_POINT('Ctrl Pts',(-7.4722661871791,15.2,-8.12177427581243));
#282604=CARTESIAN_POINT('Ctrl Pts',(-7.4759894561588,15.2,-8.12366113613748));
#282605=CARTESIAN_POINT('Ctrl Pts',(-7.47972819549303,15.2,-8.1255482602684));
#282606=CARTESIAN_POINT('Ctrl Pts',(-7.48348235405317,15.2,-8.12743553529887));
#282607=CARTESIAN_POINT('Ctrl Pts',(-7.48723651210181,15.2,-8.12932281007221));
#282608=CARTESIAN_POINT('Ctrl Pts',(-7.49100608902614,15.2,-8.13121023609446));
#282609=CARTESIAN_POINT('Ctrl Pts',(-7.49479103288239,15.2,-8.13309770282905));
#282610=CARTESIAN_POINT('Ctrl Pts',(-7.49857597725434,15.2,-8.1349851698208));
#282611=CARTESIAN_POINT('Ctrl Pts',(-7.50237629019201,15.2,-8.13687267729312));
#282612=CARTESIAN_POINT('Ctrl Pts',(-7.50619191851206,15.2,-8.13876011689598));
#282613=CARTESIAN_POINT('Ctrl Pts',(-7.51000754631224,15.2,-8.14064755624167));
#282614=CARTESIAN_POINT('Ctrl Pts',(-7.51383848990446,15.2,-8.14253492761949));
#282615=CARTESIAN_POINT('Ctrl Pts',(-7.5176846992253,15.2,-8.14442212122617));
#282616=CARTESIAN_POINT('Ctrl Pts',(-7.52153090907019,15.2,-8.14630931508999));
#282617=CARTESIAN_POINT('Ctrl Pts',(-7.52539238303256,15.2,-8.148196332657));
#282618=CARTESIAN_POINT('Ctrl Pts',(-7.5292690708004,15.2,-8.15008306687093));
#282619=CARTESIAN_POINT('Ctrl Pts',(-7.53314575804004,15.2,-8.15196980082778));
#282620=CARTESIAN_POINT('Ctrl Pts',(-7.53703766095438,15.2,-8.15385625034579));
#282621=CARTESIAN_POINT('Ctrl Pts',(-7.5409447254112,15.2,-8.15574230919165));
#282622=CARTESIAN_POINT('Ctrl Pts',(-7.54485179040036,15.2,-8.15762836829447));
#282623=CARTESIAN_POINT('Ctrl Pts',(-7.54877401763127,15.2,-8.15951403878722));
#282624=CARTESIAN_POINT('Ctrl Pts',(-7.55271135675268,15.2,-8.16139921250964));
#282625=CARTESIAN_POINT('Ctrl Pts',(-7.55664869533762,15.2,-8.16328438597519));
#282626=CARTESIAN_POINT('Ctrl Pts',(-7.56060114712165,15.2,-8.16516906444316));
#282627=CARTESIAN_POINT('Ctrl Pts',(-7.56456865835132,15.2,-8.16705314323364));
#282628=CARTESIAN_POINT('Ctrl Pts',(-7.56853617012155,15.2,-8.16893722228082));
#282629=CARTESIAN_POINT('Ctrl Pts',(-7.57251874414324,15.2,-8.17082070146963));
#282630=CARTESIAN_POINT('Ctrl Pts',(-7.57651632724999,15.2,-8.17270347901669));
#282631=CARTESIAN_POINT('Ctrl Pts',(-7.5815133058611,15.2,-8.17505695082224));
#282632=CARTESIAN_POINT('Ctrl Pts',(-7.58653373882422,15.2,-8.17740932297951));
#282633=CARTESIAN_POINT('Ctrl Pts',(-7.59157752502775,15.2,-8.1797603984763));
#282634=CARTESIAN_POINT('Ctrl Pts',(-7.59460379663991,15.2,-8.18117104372312));
#282635=CARTESIAN_POINT('Ctrl Pts',(-7.59763847642735,15.2,-8.18258122316021));
#282636=CARTESIAN_POINT('Ctrl Pts',(-7.60068154195557,15.2,-8.18399089144874));
#282637=CARTESIAN_POINT('Ctrl Pts',(-7.60372460748379,15.2,-8.18540055973726));
#282638=CARTESIAN_POINT('Ctrl Pts',(-7.60677605917854,15.2,-8.18680971968094));
#282639=CARTESIAN_POINT('Ctrl Pts',(-7.60983587569162,15.2,-8.18821832683814));
#282640=CARTESIAN_POINT('Ctrl Pts',(-7.6128956922047,15.2,-8.18962693399533));
#282641=CARTESIAN_POINT('Ctrl Pts',(-7.61596387372557,15.2,-8.19103498854425));
#282642=CARTESIAN_POINT('Ctrl Pts',(-7.61904039827933,15.2,-8.19244244970152));
#282643=CARTESIAN_POINT('Ctrl Pts',(-7.62211692339197,15.2,-8.19384991111449));
#282644=CARTESIAN_POINT('Ctrl Pts',(-7.62520179237365,15.2,-8.19525677853563));
#282645=CARTESIAN_POINT('Ctrl Pts',(-7.62829498390766,15.2,-8.19666300953158));
#282646=CARTESIAN_POINT('Ctrl Pts',(-7.63138817487973,15.2,-8.19806924027206));
#282647=CARTESIAN_POINT('Ctrl Pts',(-7.63448968784177,15.2,-8.19947483601944));
#282648=CARTESIAN_POINT('Ctrl Pts',(-7.63759950155175,15.2,-8.2008797542885));
#282649=CARTESIAN_POINT('Ctrl Pts',(-7.64070931526173,15.2,-8.20228467255755));
#282650=CARTESIAN_POINT('Ctrl Pts',(-7.64382743082045,15.2,-8.20368891358738));
#282651=CARTESIAN_POINT('Ctrl Pts',(-7.64695382533258,15.2,-8.20509243541132));
#282652=CARTESIAN_POINT('Ctrl Pts',(-7.65008021984471,15.2,-8.20649595723526));
#282653=CARTESIAN_POINT('Ctrl Pts',(-7.65321489374752,15.2,-8.20789876165096));
#282654=CARTESIAN_POINT('Ctrl Pts',(-7.65635782671666,15.2,-8.20930080593335));
#282655=CARTESIAN_POINT('Ctrl Pts',(-7.6595007596858,15.2,-8.21070285021575));
#282656=CARTESIAN_POINT('Ctrl Pts',(-7.66265195113792,15.2,-8.21210413616483));
#282657=CARTESIAN_POINT('Ctrl Pts',(-7.66581137964743,15.2,-8.21350462136402));
#282658=CARTESIAN_POINT('Ctrl Pts',(-7.66897080815692,15.2,-8.21490510656321));
#282659=CARTESIAN_POINT('Ctrl Pts',(-7.67213847447665,15.2,-8.21630479169355));
#282660=CARTESIAN_POINT('Ctrl Pts',(-7.67531435664396,15.2,-8.21770363650437));
#282661=CARTESIAN_POINT('Ctrl Pts',(-7.67849023881125,15.2,-8.21910248131519));
#282662=CARTESIAN_POINT('Ctrl Pts',(-7.68167433725452,15.2,-8.22050048596276));
#282663=CARTESIAN_POINT('Ctrl Pts',(-7.68486662984576,15.2,-8.22189761016211));
#282664=CARTESIAN_POINT('Ctrl Pts',(-7.68805892301693,15.2,-8.22329473461529));
#282665=CARTESIAN_POINT('Ctrl Pts',(-7.69125941179872,15.2,-8.22469097810154));
#282666=CARTESIAN_POINT('Ctrl Pts',(-7.69446807439117,15.2,-8.2260863020542));
#282667=CARTESIAN_POINT('Ctrl Pts',(-7.69767673640071,15.2,-8.22748162575338));
#282668=CARTESIAN_POINT('Ctrl Pts',(-7.70089357186813,15.2,-8.2288760301526));
#282669=CARTESIAN_POINT('Ctrl Pts',(-7.70411856033499,15.2,-8.23026947393523));
#282670=CARTESIAN_POINT('Ctrl Pts',(-7.70734354880185,15.2,-8.23166291771784));
#282671=CARTESIAN_POINT('Ctrl Pts',(-7.71057669030596,15.2,-8.23305540169553));
#282672=CARTESIAN_POINT('Ctrl Pts',(-7.71381796324461,15.2,-8.23444688694295));
#282673=CARTESIAN_POINT('Ctrl Pts',(-7.71705923618327,15.2,-8.23583837219038));
#282674=CARTESIAN_POINT('Ctrl Pts',(-7.7203086398173,15.2,-8.23722885852626));
#282675=CARTESIAN_POINT('Ctrl Pts',(-7.72356615475538,15.2,-8.23861830723209));
#282676=CARTESIAN_POINT('Ctrl Pts',(-7.72682366969345,15.2,-8.24000775593793));
#282677=CARTESIAN_POINT('Ctrl Pts',(-7.73008929492962,15.2,-8.2413961673491));
#282678=CARTESIAN_POINT('Ctrl Pts',(-7.7333630098933,15.2,-8.24278350113212));
#282679=CARTESIAN_POINT('Ctrl Pts',(-7.73663672485699,15.2,-8.24417083491514));
#282680=CARTESIAN_POINT('Ctrl Pts',(-7.73991852930344,15.2,-8.24555709223157));
#282681=CARTESIAN_POINT('Ctrl Pts',(-7.74320840180781,15.2,-8.2469422349314));
#282682=CARTESIAN_POINT('Ctrl Pts',(-7.74649827490985,15.2,-8.24832737788286));
#282683=CARTESIAN_POINT('Ctrl Pts',(-7.74979621608915,15.2,-8.249711404834));
#282684=CARTESIAN_POINT('Ctrl Pts',(-7.75310220519572,15.2,-8.25109427928482));
#282685=CARTESIAN_POINT('Ctrl Pts',(-7.7564081937017,15.2,-8.25247715348442));
#282686=CARTESIAN_POINT('Ctrl Pts',(-7.75972222986558,15.2,-8.25385887468408));
#282687=CARTESIAN_POINT('Ctrl Pts',(-7.76304429232891,15.2,-8.25523940442548));
#282688=CARTESIAN_POINT('Ctrl Pts',(-7.76636635479223,15.2,-8.25661993416688));
#282689=CARTESIAN_POINT('Ctrl Pts',(-7.76969644324246,15.2,-8.25799927246176));
#282690=CARTESIAN_POINT('Ctrl Pts',(-7.77303453726137,15.2,-8.25937738225128));
#282691=CARTESIAN_POINT('Ctrl Pts',(-7.77637263128028,15.2,-8.26075549204079));
#282692=CARTESIAN_POINT('Ctrl Pts',(-7.77971873168696,15.2,-8.26213237365917));
#282693=CARTESIAN_POINT('Ctrl Pts',(-7.78307281574696,15.2,-8.26350798799044));
#282694=CARTESIAN_POINT('Ctrl Pts',(-7.78642689980696,15.2,-8.26488360232171));
#282695=CARTESIAN_POINT('Ctrl Pts',(-7.7897889688726,15.2,-8.26625795105011));
#282696=CARTESIAN_POINT('Ctrl Pts',(-7.79315900087447,15.2,-8.26763099537534));
#282697=CARTESIAN_POINT('Ctrl Pts',(-7.79652903287633,15.2,-8.26900403970057));
#282698=CARTESIAN_POINT('Ctrl Pts',(-7.79990702778598,15.2,-8.27037578065088));
#282699=CARTESIAN_POINT('Ctrl Pts',(-7.80329296624521,15.2,-8.27174618143461));
#282700=CARTESIAN_POINT('Ctrl Pts',(-7.80667890531956,15.2,-8.2731165824673));
#282701=CARTESIAN_POINT('Ctrl Pts',(-7.81007278709614,15.2,-8.27448564326627));
#282702=CARTESIAN_POINT('Ctrl Pts',(-7.8134745902166,15.2,-8.27585332679818));
#282703=CARTESIAN_POINT('Ctrl Pts',(-7.81687639271907,15.2,-8.27722101008163));
#282704=CARTESIAN_POINT('Ctrl Pts',(-7.82028611704716,15.2,-8.27858731639565));
#282705=CARTESIAN_POINT('Ctrl Pts',(-7.82370374263631,15.2,-8.27995220874742));
#282706=CARTESIAN_POINT('Ctrl Pts',(-7.82712136822545,15.2,-8.28131710109918));
#282707=CARTESIAN_POINT('Ctrl Pts',(-7.83054689374844,15.2,-8.28268057986474));
#282708=CARTESIAN_POINT('Ctrl Pts',(-7.83398029962438,15.2,-8.28404260819013));
#282709=CARTESIAN_POINT('Ctrl Pts',(-7.83741370550031,15.2,-8.28540463651551));
#282710=CARTESIAN_POINT('Ctrl Pts',(-7.8408549901753,15.2,-8.28676521536607));
#282711=CARTESIAN_POINT('Ctrl Pts',(-7.84430413555,15.2,-8.28812430827503));
#282712=CARTESIAN_POINT('Ctrl Pts',(-7.8477532809247,15.2,-8.28948340118399));
#282713=CARTESIAN_POINT('Ctrl Pts',(-7.85121028493238,15.2,-8.29084100993467));
#282714=CARTESIAN_POINT('Ctrl Pts',(-7.85467512788913,15.2,-8.29219709634385));
#282715=CARTESIAN_POINT('Ctrl Pts',(-7.85813997084589,15.2,-8.29355318275304));
#282716=CARTESIAN_POINT('Ctrl Pts',(-7.8616126521135,15.2,-8.29490774905296));
#282717=CARTESIAN_POINT('Ctrl Pts',(-7.86509314986836,15.2,-8.29626075598824));
#282718=CARTESIAN_POINT('Ctrl Pts',(-7.86857364762321,15.2,-8.29761376292352));
#282719=CARTESIAN_POINT('Ctrl Pts',(-7.87206196289928,15.2,-8.29896521160459));
#282720=CARTESIAN_POINT('Ctrl Pts',(-7.87555807393786,15.2,-8.30031506743076));
#282721=CARTESIAN_POINT('Ctrl Pts',(-7.87905418561156,15.2,-8.30166492350216));
#282722=CARTESIAN_POINT('Ctrl Pts',(-7.88255809365415,15.2,-8.30301318591478));
#282723=CARTESIAN_POINT('Ctrl Pts',(-7.88606977879056,15.2,-8.30435982398526));
#282724=CARTESIAN_POINT('Ctrl Pts',(-7.88958146328901,15.2,-8.30570646181111));
#282725=CARTESIAN_POINT('Ctrl Pts',(-7.89310092559542,15.2,-8.30705147627872));
#282726=CARTESIAN_POINT('Ctrl Pts',(-7.8966281448846,15.2,-8.30839482993809));
#282727=CARTESIAN_POINT('Ctrl Pts',(-7.90015536417378,15.2,-8.30973818359747));
#282728=CARTESIAN_POINT('Ctrl Pts',(-7.90369033743249,15.2,-8.31107987547719));
#282729=CARTESIAN_POINT('Ctrl Pts',(-7.90723304227822,15.2,-8.31241986322624));
#282730=CARTESIAN_POINT('Ctrl Pts',(-7.91077574712395,15.2,-8.31375985097529));
#282731=CARTESIAN_POINT('Ctrl Pts',(-7.91432618135994,15.2,-8.31509813342464));
#282732=CARTESIAN_POINT('Ctrl Pts',(-7.91788432603843,15.2,-8.31643468000715));
#282733=CARTESIAN_POINT('Ctrl Pts',(-7.92381456738474,15.2,-8.31866225772561));
#282734=CARTESIAN_POINT('Ctrl Pts',(-7.92976622247684,15.2,-8.32088501090861));
#282735=CARTESIAN_POINT('Ctrl Pts',(-7.93573928312123,15.2,-8.32310290867369));
#282736=CARTESIAN_POINT('Origin',(-5.66257110645729E-14,15.2,-1.77635683940025E-14));
#282737=CARTESIAN_POINT('',(-6.57080831900006,15.2,-8.02901631800001));
#282738=CARTESIAN_POINT('',(-6.57080831900006,12.2,-8.02901631800001));
#282739=CARTESIAN_POINT('',(-6.57080831900006,15.2,-8.02901631800001));
#282740=CARTESIAN_POINT('Origin',(-5.66257110645729E-14,12.2,-1.77635683940025E-14));
#282741=CARTESIAN_POINT('Origin',(-5.66257110645729E-14,15.2,-1.77635683940025E-14));
#282742=CARTESIAN_POINT('Origin',(-5.66257110645729E-14,15.2,-1.77635683940025E-14));
#282743=CARTESIAN_POINT('',(-6.97920857100006,15.2,-9.14005731500002));
#282744=CARTESIAN_POINT('',(-6.67046385600006,15.2,-9.36775917400002));
#282745=CARTESIAN_POINT('Origin',(-5.66257110645729E-14,15.2,-1.77635683940025E-14));
#282746=CARTESIAN_POINT('',(-6.67046385600006,12.2,-9.36775917400002));
#282747=CARTESIAN_POINT('',(-6.67046385600006,15.2,-9.36775917400002));
#282748=CARTESIAN_POINT('',(-6.97920857100006,12.2,-9.14005731500002));
#282749=CARTESIAN_POINT('Origin',(-5.66257110645729E-14,12.2,-1.77635683940025E-14));
#282750=CARTESIAN_POINT('',(-6.97920857100006,15.2,-9.14005731500002));
#282751=CARTESIAN_POINT('Ctrl Pts',(-6.67046385600006,15.2,-9.36775917400002));
#282752=CARTESIAN_POINT('Ctrl Pts',(-6.67046385600006,11.6,-9.36775917400002));
#282753=CARTESIAN_POINT('Ctrl Pts',(-6.66979226100006,15.2,-9.36739373000002));
#282754=CARTESIAN_POINT('Ctrl Pts',(-6.66979226100006,11.6,-9.36739373000002));
#282755=CARTESIAN_POINT('Ctrl Pts',(-6.66844959800006,15.2,-9.36666279600002));
#282756=CARTESIAN_POINT('Ctrl Pts',(-6.66844959800006,11.6,-9.36666279600002));
#282757=CARTESIAN_POINT('Ctrl Pts',(-6.66643717700006,15.2,-9.36556627000002));
#282758=CARTESIAN_POINT('Ctrl Pts',(-6.66643717700006,11.6,-9.36556627000002));
#282759=CARTESIAN_POINT('Ctrl Pts',(-6.66375709900006,15.2,-9.36410398400002));
#282760=CARTESIAN_POINT('Ctrl Pts',(-6.66375709900006,11.6,-9.36410398400002));
#282761=CARTESIAN_POINT('Ctrl Pts',(-6.66041225200006,15.2,-9.36227570600002));
#282762=CARTESIAN_POINT('Ctrl Pts',(-6.66041225200006,11.6,-9.36227570600002));
#282763=CARTESIAN_POINT('Ctrl Pts',(-6.65707265500005,15.2,-9.36044701000002));
#282764=CARTESIAN_POINT('Ctrl Pts',(-6.65707265500005,11.6,-9.36044701000002));
#282765=CARTESIAN_POINT('Ctrl Pts',(-6.65373831000006,15.2,-9.35861789600001));
#282766=CARTESIAN_POINT('Ctrl Pts',(-6.65373831000006,11.6,-9.35861789600001));
#282767=CARTESIAN_POINT('Ctrl Pts',(-6.65040921900006,15.2,-9.35678837000001));
#282768=CARTESIAN_POINT('Ctrl Pts',(-6.65040921900006,11.6,-9.35678837000001));
#282769=CARTESIAN_POINT('Ctrl Pts',(-6.64708538300006,15.2,-9.35495843700001));
#282770=CARTESIAN_POINT('Ctrl Pts',(-6.64708538300006,11.6,-9.35495843700001));
#282771=CARTESIAN_POINT('Ctrl Pts',(-6.64376680700006,15.2,-9.35312810300001));
#282772=CARTESIAN_POINT('Ctrl Pts',(-6.64376680700006,11.6,-9.35312810300001));
#282773=CARTESIAN_POINT('Ctrl Pts',(-6.64045349300006,15.2,-9.35129737900001));
#282774=CARTESIAN_POINT('Ctrl Pts',(-6.64045349300006,11.6,-9.35129737900001));
#282775=CARTESIAN_POINT('Ctrl Pts',(-6.63714544700006,15.2,-9.34946627300001));
#282776=CARTESIAN_POINT('Ctrl Pts',(-6.63714544700006,11.6,-9.34946627300001));
#282777=CARTESIAN_POINT('Ctrl Pts',(-6.63384267100006,15.2,-9.34763479700001));
#282778=CARTESIAN_POINT('Ctrl Pts',(-6.63384267100006,11.6,-9.34763479700001));
#282779=CARTESIAN_POINT('Ctrl Pts',(-6.63054517000006,15.2,-9.34580296000001));
#282780=CARTESIAN_POINT('Ctrl Pts',(-6.63054517000006,11.6,-9.34580296000001));
#282781=CARTESIAN_POINT('Ctrl Pts',(-6.62725294900006,15.2,-9.34397077300002));
#282782=CARTESIAN_POINT('Ctrl Pts',(-6.62725294900006,11.6,-9.34397077300002));
#282783=CARTESIAN_POINT('Ctrl Pts',(-6.62396601100006,15.2,-9.34213824300001));
#282784=CARTESIAN_POINT('Ctrl Pts',(-6.62396601100006,11.6,-9.34213824300001));
#282785=CARTESIAN_POINT('Ctrl Pts',(-6.62068436000006,15.2,-9.34030538000002));
#282786=CARTESIAN_POINT('Ctrl Pts',(-6.62068436000006,11.6,-9.34030538000002));
#282787=CARTESIAN_POINT('Ctrl Pts',(-6.61740799800006,15.2,-9.33847218900001));
#282788=CARTESIAN_POINT('Ctrl Pts',(-6.61740799800006,11.6,-9.33847218900001));
#282789=CARTESIAN_POINT('Ctrl Pts',(-6.61413692800005,15.2,-9.33663868000002));
#282790=CARTESIAN_POINT('Ctrl Pts',(-6.61413692800005,11.6,-9.33663868000002));
#282791=CARTESIAN_POINT('Ctrl Pts',(-6.61087115500006,15.2,-9.33480485900001));
#282792=CARTESIAN_POINT('Ctrl Pts',(-6.61087115500006,11.6,-9.33480485900001));
#282793=CARTESIAN_POINT('Ctrl Pts',(-6.60761068100006,15.2,-9.33297073500002));
#282794=CARTESIAN_POINT('Ctrl Pts',(-6.60761068100006,11.6,-9.33297073500002));
#282795=CARTESIAN_POINT('Ctrl Pts',(-6.60435550800006,15.2,-9.33113631500002));
#282796=CARTESIAN_POINT('Ctrl Pts',(-6.60435550800006,11.6,-9.33113631500002));
#282797=CARTESIAN_POINT('Ctrl Pts',(-6.60110564300005,15.2,-9.32930161000002));
#282798=CARTESIAN_POINT('Ctrl Pts',(-6.60110564300005,11.6,-9.32930161000002));
#282799=CARTESIAN_POINT('Ctrl Pts',(-6.59786108600006,15.2,-9.32746662500002));
#282800=CARTESIAN_POINT('Ctrl Pts',(-6.59786108600006,11.6,-9.32746662500002));
#282801=CARTESIAN_POINT('Ctrl Pts',(-6.59462184300006,15.2,-9.32563137200002));
#282802=CARTESIAN_POINT('Ctrl Pts',(-6.59462184300006,11.6,-9.32563137200002));
#282803=CARTESIAN_POINT('Ctrl Pts',(-6.59138791700006,15.2,-9.32379585900001));
#282804=CARTESIAN_POINT('Ctrl Pts',(-6.59138791700006,11.6,-9.32379585900001));
#282805=CARTESIAN_POINT('Ctrl Pts',(-6.58815931000006,15.2,-9.32196009500002));
#282806=CARTESIAN_POINT('Ctrl Pts',(-6.58815931000006,11.6,-9.32196009500002));
#282807=CARTESIAN_POINT('Ctrl Pts',(-6.58493602700006,15.2,-9.32012408600002));
#282808=CARTESIAN_POINT('Ctrl Pts',(-6.58493602700006,11.6,-9.32012408600002));
#282809=CARTESIAN_POINT('Ctrl Pts',(-6.58171807300006,15.2,-9.31828784500001));
#282810=CARTESIAN_POINT('Ctrl Pts',(-6.58171807300006,11.6,-9.31828784500001));
#282811=CARTESIAN_POINT('Ctrl Pts',(-6.57850544800006,15.2,-9.31645137700002));
#282812=CARTESIAN_POINT('Ctrl Pts',(-6.57850544800006,11.6,-9.31645137700002));
#282813=CARTESIAN_POINT('Ctrl Pts',(-6.57529815700006,15.2,-9.31461469100002));
#282814=CARTESIAN_POINT('Ctrl Pts',(-6.57529815700006,11.6,-9.31461469100002));
#282815=CARTESIAN_POINT('Ctrl Pts',(-6.57209620400006,15.2,-9.31277779500002));
#282816=CARTESIAN_POINT('Ctrl Pts',(-6.57209620400006,11.6,-9.31277779500002));
#282817=CARTESIAN_POINT('Ctrl Pts',(-6.56889959100006,15.2,-9.31094070000002));
#282818=CARTESIAN_POINT('Ctrl Pts',(-6.56889959100006,11.6,-9.31094070000002));
#282819=CARTESIAN_POINT('Ctrl Pts',(-6.56570832300006,15.2,-9.30910341200001));
#282820=CARTESIAN_POINT('Ctrl Pts',(-6.56570832300006,11.6,-9.30910341200001));
#282821=CARTESIAN_POINT('Ctrl Pts',(-6.56252240200006,15.2,-9.30726594200002));
#282822=CARTESIAN_POINT('Ctrl Pts',(-6.56252240200006,11.6,-9.30726594200002));
#282823=CARTESIAN_POINT('Ctrl Pts',(-6.55934183200006,15.2,-9.30542829500002));
#282824=CARTESIAN_POINT('Ctrl Pts',(-6.55934183200006,11.6,-9.30542829500002));
#282825=CARTESIAN_POINT('Ctrl Pts',(-6.55616661700006,15.2,-9.30359048400001));
#282826=CARTESIAN_POINT('Ctrl Pts',(-6.55616661700006,11.6,-9.30359048400001));
#282827=CARTESIAN_POINT('Ctrl Pts',(-6.55299676000006,15.2,-9.30175251500001));
#282828=CARTESIAN_POINT('Ctrl Pts',(-6.55299676000006,11.6,-9.30175251500001));
#282829=CARTESIAN_POINT('Ctrl Pts',(-6.54983226500006,15.2,-9.29991439900002));
#282830=CARTESIAN_POINT('Ctrl Pts',(-6.54983226500006,11.6,-9.29991439900002));
#282831=CARTESIAN_POINT('Ctrl Pts',(-6.54667313400005,15.2,-9.29807614200002));
#282832=CARTESIAN_POINT('Ctrl Pts',(-6.54667313400005,11.6,-9.29807614200002));
#282833=CARTESIAN_POINT('Ctrl Pts',(-6.54351937200006,15.2,-9.29623775500002));
#282834=CARTESIAN_POINT('Ctrl Pts',(-6.54351937200006,11.6,-9.29623775500002));
#282835=CARTESIAN_POINT('Ctrl Pts',(-6.54037098100006,15.2,-9.29439924500001));
#282836=CARTESIAN_POINT('Ctrl Pts',(-6.54037098100006,11.6,-9.29439924500001));
#282837=CARTESIAN_POINT('Ctrl Pts',(-6.53722796600006,15.2,-9.29256062200002));
#282838=CARTESIAN_POINT('Ctrl Pts',(-6.53722796600006,11.6,-9.29256062200002));
#282839=CARTESIAN_POINT('Ctrl Pts',(-6.53409033000006,15.2,-9.29072189400001));
#282840=CARTESIAN_POINT('Ctrl Pts',(-6.53409033000006,11.6,-9.29072189400001));
#282841=CARTESIAN_POINT('Ctrl Pts',(-6.53095807500006,15.2,-9.28888307000001));
#282842=CARTESIAN_POINT('Ctrl Pts',(-6.53095807500006,11.6,-9.28888307000001));
#282843=CARTESIAN_POINT('Ctrl Pts',(-6.52783120600006,15.2,-9.28704416000001));
#282844=CARTESIAN_POINT('Ctrl Pts',(-6.52783120600006,11.6,-9.28704416000001));
#282845=CARTESIAN_POINT('Ctrl Pts',(-6.52470972700006,15.2,-9.28520517200001));
#282846=CARTESIAN_POINT('Ctrl Pts',(-6.52470972700006,11.6,-9.28520517200001));
#282847=CARTESIAN_POINT('Ctrl Pts',(-6.52159363900005,15.2,-9.28336611300002));
#282848=CARTESIAN_POINT('Ctrl Pts',(-6.52159363900005,11.6,-9.28336611300002));
#282849=CARTESIAN_POINT('Ctrl Pts',(-6.51848294800006,15.2,-9.28152699600002));
#282850=CARTESIAN_POINT('Ctrl Pts',(-6.51848294800006,11.6,-9.28152699600002));
#282851=CARTESIAN_POINT('Ctrl Pts',(-6.51537765500006,15.2,-9.27968782700002));
#282852=CARTESIAN_POINT('Ctrl Pts',(-6.51537765500006,11.6,-9.27968782700002));
#282853=CARTESIAN_POINT('Ctrl Pts',(-6.51227776500006,15.2,-9.27784861500001));
#282854=CARTESIAN_POINT('Ctrl Pts',(-6.51227776500006,11.6,-9.27784861500001));
#282855=CARTESIAN_POINT('Ctrl Pts',(-6.50918328200006,15.2,-9.27600936900001));
#282856=CARTESIAN_POINT('Ctrl Pts',(-6.50918328200006,11.6,-9.27600936900001));
#282857=CARTESIAN_POINT('Ctrl Pts',(-6.50609420700006,15.2,-9.27417010000001));
#282858=CARTESIAN_POINT('Ctrl Pts',(-6.50609420700006,11.6,-9.27417010000001));
#282859=CARTESIAN_POINT('Ctrl Pts',(-6.50301054600006,15.2,-9.27233081400002));
#282860=CARTESIAN_POINT('Ctrl Pts',(-6.50301054600006,11.6,-9.27233081400002));
#282861=CARTESIAN_POINT('Ctrl Pts',(-6.49993230100006,15.2,-9.27049152200001));
#282862=CARTESIAN_POINT('Ctrl Pts',(-6.49993230100006,11.6,-9.27049152200001));
#282863=CARTESIAN_POINT('Ctrl Pts',(-6.49685947500006,15.2,-9.26865223300002));
#282864=CARTESIAN_POINT('Ctrl Pts',(-6.49685947500006,11.6,-9.26865223300002));
#282865=CARTESIAN_POINT('Ctrl Pts',(-6.49379207300006,15.2,-9.26681295500002));
#282866=CARTESIAN_POINT('Ctrl Pts',(-6.49379207300006,11.6,-9.26681295500002));
#282867=CARTESIAN_POINT('Ctrl Pts',(-6.49073009700006,15.2,-9.26497369800002));
#282868=CARTESIAN_POINT('Ctrl Pts',(-6.49073009700006,11.6,-9.26497369800002));
#282869=CARTESIAN_POINT('Ctrl Pts',(-6.48767355200006,15.2,-9.26313447100001));
#282870=CARTESIAN_POINT('Ctrl Pts',(-6.48767355200006,11.6,-9.26313447100001));
#282871=CARTESIAN_POINT('Ctrl Pts',(-6.48462244000005,15.2,-9.26129528200001));
#282872=CARTESIAN_POINT('Ctrl Pts',(-6.48462244000005,11.6,-9.26129528200001));
#282873=CARTESIAN_POINT('Ctrl Pts',(-6.48157676400006,15.2,-9.25945614200002));
#282874=CARTESIAN_POINT('Ctrl Pts',(-6.48157676400006,11.6,-9.25945614200002));
#282875=CARTESIAN_POINT('Ctrl Pts',(-6.47853652900006,15.2,-9.25761705800002));
#282876=CARTESIAN_POINT('Ctrl Pts',(-6.47853652900006,11.6,-9.25761705800002));
#282877=CARTESIAN_POINT('Ctrl Pts',(-6.47550173800005,15.2,-9.25577804100002));
#282878=CARTESIAN_POINT('Ctrl Pts',(-6.47550173800005,11.6,-9.25577804100002));
#282879=CARTESIAN_POINT('Ctrl Pts',(-6.47247239300006,15.2,-9.25393910000002));
#282880=CARTESIAN_POINT('Ctrl Pts',(-6.47247239300006,11.6,-9.25393910000002));
#282881=CARTESIAN_POINT('Ctrl Pts',(-6.46944849900006,15.2,-9.25210024200002));
#282882=CARTESIAN_POINT('Ctrl Pts',(-6.46944849900006,11.6,-9.25210024200002));
#282883=CARTESIAN_POINT('Ctrl Pts',(-6.46643005900006,15.2,-9.25026147900001));
#282884=CARTESIAN_POINT('Ctrl Pts',(-6.46643005900006,11.6,-9.25026147900001));
#282885=CARTESIAN_POINT('Ctrl Pts',(-6.46341707600006,15.2,-9.24842281800002));
#282886=CARTESIAN_POINT('Ctrl Pts',(-6.46341707600006,11.6,-9.24842281800002));
#282887=CARTESIAN_POINT('Ctrl Pts',(-6.46040955400006,15.2,-9.24658427100002));
#282888=CARTESIAN_POINT('Ctrl Pts',(-6.46040955400006,11.6,-9.24658427100002));
#282889=CARTESIAN_POINT('Ctrl Pts',(-6.45740749600006,15.2,-9.24474584400001));
#282890=CARTESIAN_POINT('Ctrl Pts',(-6.45740749600006,11.6,-9.24474584400001));
#282891=CARTESIAN_POINT('Ctrl Pts',(-6.45441090500006,15.2,-9.24290754900002));
#282892=CARTESIAN_POINT('Ctrl Pts',(-6.45441090500006,11.6,-9.24290754900002));
#282893=CARTESIAN_POINT('Ctrl Pts',(-6.45141978500006,15.2,-9.24106939400002));
#282894=CARTESIAN_POINT('Ctrl Pts',(-6.45141978500006,11.6,-9.24106939400002));
#282895=CARTESIAN_POINT('Ctrl Pts',(-6.44843413900006,15.2,-9.23923138800001));
#282896=CARTESIAN_POINT('Ctrl Pts',(-6.44843413900006,11.6,-9.23923138800001));
#282897=CARTESIAN_POINT('Ctrl Pts',(-6.44545397200006,15.2,-9.23739354200002));
#282898=CARTESIAN_POINT('Ctrl Pts',(-6.44545397200006,11.6,-9.23739354200002));
#282899=CARTESIAN_POINT('Ctrl Pts',(-6.44247928500006,15.2,-9.23555586400001));
#282900=CARTESIAN_POINT('Ctrl Pts',(-6.44247928500006,11.6,-9.23555586400001));
#282901=CARTESIAN_POINT('Ctrl Pts',(-6.43951008200006,15.2,-9.23371836400002));
#282902=CARTESIAN_POINT('Ctrl Pts',(-6.43951008200006,11.6,-9.23371836400002));
#282903=CARTESIAN_POINT('Ctrl Pts',(-6.43654636800005,15.2,-9.23188105000002));
#282904=CARTESIAN_POINT('Ctrl Pts',(-6.43654636800005,11.6,-9.23188105000002));
#282905=CARTESIAN_POINT('Ctrl Pts',(-6.43358814400006,15.2,-9.23004393300002));
#282906=CARTESIAN_POINT('Ctrl Pts',(-6.43358814400006,11.6,-9.23004393300002));
#282907=CARTESIAN_POINT('Ctrl Pts',(-6.43063541500006,15.2,-9.22820702200001));
#282908=CARTESIAN_POINT('Ctrl Pts',(-6.43063541500006,11.6,-9.22820702200001));
#282909=CARTESIAN_POINT('Ctrl Pts',(-6.42768818400006,15.2,-9.22637032800001));
#282910=CARTESIAN_POINT('Ctrl Pts',(-6.42768818400006,11.6,-9.22637032800001));
#282911=CARTESIAN_POINT('Ctrl Pts',(-6.42474645500006,15.2,-9.22453385700001));
#282912=CARTESIAN_POINT('Ctrl Pts',(-6.42474645500006,11.6,-9.22453385700001));
#282913=CARTESIAN_POINT('Ctrl Pts',(-6.42181023000005,15.2,-9.22269762200001));
#282914=CARTESIAN_POINT('Ctrl Pts',(-6.42181023000005,11.6,-9.22269762200001));
#282915=CARTESIAN_POINT('Ctrl Pts',(-6.41887951300006,15.2,-9.22086163100002));
#282916=CARTESIAN_POINT('Ctrl Pts',(-6.41887951300006,11.6,-9.22086163100002));
#282917=CARTESIAN_POINT('Ctrl Pts',(-6.41595430900006,15.2,-9.21902589200002));
#282918=CARTESIAN_POINT('Ctrl Pts',(-6.41595430900006,11.6,-9.21902589200002));
#282919=CARTESIAN_POINT('Ctrl Pts',(-6.41303461900006,15.2,-9.21719041800002));
#282920=CARTESIAN_POINT('Ctrl Pts',(-6.41303461900006,11.6,-9.21719041800002));
#282921=CARTESIAN_POINT('Ctrl Pts',(-6.41012044700005,15.2,-9.21535521600001));
#282922=CARTESIAN_POINT('Ctrl Pts',(-6.41012044700005,11.6,-9.21535521600001));
#282923=CARTESIAN_POINT('Ctrl Pts',(-6.40721179700006,15.2,-9.21352029700002));
#282924=CARTESIAN_POINT('Ctrl Pts',(-6.40721179700006,11.6,-9.21352029700002));
#282925=CARTESIAN_POINT('Ctrl Pts',(-6.40430867200006,15.2,-9.21168566900001));
#282926=CARTESIAN_POINT('Ctrl Pts',(-6.40430867200006,11.6,-9.21168566900001));
#282927=CARTESIAN_POINT('Ctrl Pts',(-6.40141107500006,15.2,-9.20985134500001));
#282928=CARTESIAN_POINT('Ctrl Pts',(-6.40141107500006,11.6,-9.20985134500001));
#282929=CARTESIAN_POINT('Ctrl Pts',(-6.39851901000006,15.2,-9.20801733000001));
#282930=CARTESIAN_POINT('Ctrl Pts',(-6.39851901000006,11.6,-9.20801733000001));
#282931=CARTESIAN_POINT('Ctrl Pts',(-6.39563248000006,15.2,-9.20618363800001));
#282932=CARTESIAN_POINT('Ctrl Pts',(-6.39563248000006,11.6,-9.20618363800001));
#282933=CARTESIAN_POINT('Ctrl Pts',(-6.39275149000006,15.2,-9.20435027600002));
#282934=CARTESIAN_POINT('Ctrl Pts',(-6.39275149000006,11.6,-9.20435027600002));
#282935=CARTESIAN_POINT('Ctrl Pts',(-6.38987604000006,15.2,-9.20251725400002));
#282936=CARTESIAN_POINT('Ctrl Pts',(-6.38987604000006,11.6,-9.20251725400002));
#282937=CARTESIAN_POINT('Ctrl Pts',(-6.38700613600006,15.2,-9.20068458400002));
#282938=CARTESIAN_POINT('Ctrl Pts',(-6.38700613600006,11.6,-9.20068458400002));
#282939=CARTESIAN_POINT('Ctrl Pts',(-6.38414178100006,15.2,-9.19885227300002));
#282940=CARTESIAN_POINT('Ctrl Pts',(-6.38414178100006,11.6,-9.19885227300002));
#282941=CARTESIAN_POINT('Ctrl Pts',(-6.38128297700006,15.2,-9.19702033200002));
#282942=CARTESIAN_POINT('Ctrl Pts',(-6.38128297700006,11.6,-9.19702033200002));
#282943=CARTESIAN_POINT('Ctrl Pts',(-6.37842973000006,15.2,-9.19518877200002));
#282944=CARTESIAN_POINT('Ctrl Pts',(-6.37842973000006,11.6,-9.19518877200002));
#282945=CARTESIAN_POINT('Ctrl Pts',(-6.37558204100006,15.2,-9.19335760100001));
#282946=CARTESIAN_POINT('Ctrl Pts',(-6.37558204100006,11.6,-9.19335760100001));
#282947=CARTESIAN_POINT('Ctrl Pts',(-6.37273991300006,15.2,-9.19152682900001));
#282948=CARTESIAN_POINT('Ctrl Pts',(-6.37273991300006,11.6,-9.19152682900001));
#282949=CARTESIAN_POINT('Ctrl Pts',(-6.36990335200006,15.2,-9.18969646800001));
#282950=CARTESIAN_POINT('Ctrl Pts',(-6.36990335200006,11.6,-9.18969646800001));
#282951=CARTESIAN_POINT('Ctrl Pts',(-6.36707236000006,15.2,-9.18786652500001));
#282952=CARTESIAN_POINT('Ctrl Pts',(-6.36707236000006,11.6,-9.18786652500001));
#282953=CARTESIAN_POINT('Ctrl Pts',(-6.36424693800006,15.2,-9.18603701200002));
#282954=CARTESIAN_POINT('Ctrl Pts',(-6.36424693800006,11.6,-9.18603701200002));
#282955=CARTESIAN_POINT('Ctrl Pts',(-6.36142709400006,15.2,-9.18420793900001));
#282956=CARTESIAN_POINT('Ctrl Pts',(-6.36142709400006,11.6,-9.18420793900001));
#282957=CARTESIAN_POINT('Ctrl Pts',(-6.35861282700006,15.2,-9.18237931400002));
#282958=CARTESIAN_POINT('Ctrl Pts',(-6.35861282700006,11.6,-9.18237931400002));
#282959=CARTESIAN_POINT('Ctrl Pts',(-6.35580414300006,15.2,-9.18055114900002));
#282960=CARTESIAN_POINT('Ctrl Pts',(-6.35580414300006,11.6,-9.18055114900002));
#282961=CARTESIAN_POINT('Ctrl Pts',(-6.35300104500006,15.2,-9.17872345400001));
#282962=CARTESIAN_POINT('Ctrl Pts',(-6.35300104500006,11.6,-9.17872345400001));
#282963=CARTESIAN_POINT('Ctrl Pts',(-6.35020353500006,15.2,-9.17689623700002));
#282964=CARTESIAN_POINT('Ctrl Pts',(-6.35020353500006,11.6,-9.17689623700002));
#282965=CARTESIAN_POINT('Ctrl Pts',(-6.34741161800005,15.2,-9.17506951100002));
#282966=CARTESIAN_POINT('Ctrl Pts',(-6.34741161800005,11.6,-9.17506951100002));
#282967=CARTESIAN_POINT('Ctrl Pts',(-6.34462529700006,15.2,-9.17324328400002));
#282968=CARTESIAN_POINT('Ctrl Pts',(-6.34462529700006,11.6,-9.17324328400002));
#282969=CARTESIAN_POINT('Ctrl Pts',(-6.34184457400006,15.2,-9.17141756700002));
#282970=CARTESIAN_POINT('Ctrl Pts',(-6.34184457400006,11.6,-9.17141756700002));
#282971=CARTESIAN_POINT('Ctrl Pts',(-6.33906945400006,15.2,-9.16959237000002));
#282972=CARTESIAN_POINT('Ctrl Pts',(-6.33906945400006,11.6,-9.16959237000002));
#282973=CARTESIAN_POINT('Ctrl Pts',(-6.33629993900006,15.2,-9.16776770200002));
#282974=CARTESIAN_POINT('Ctrl Pts',(-6.33629993900006,11.6,-9.16776770200002));
#282975=CARTESIAN_POINT('Ctrl Pts',(-6.33353603400006,15.2,-9.16594357600001));
#282976=CARTESIAN_POINT('Ctrl Pts',(-6.33353603400006,11.6,-9.16594357600001));
#282977=CARTESIAN_POINT('Ctrl Pts',(-6.33077774100006,15.2,-9.16411999900001));
#282978=CARTESIAN_POINT('Ctrl Pts',(-6.33077774100006,11.6,-9.16411999900001));
#282979=CARTESIAN_POINT('Ctrl Pts',(-6.32802506300005,15.2,-9.16229698300001));
#282980=CARTESIAN_POINT('Ctrl Pts',(-6.32802506300005,11.6,-9.16229698300001));
#282981=CARTESIAN_POINT('Ctrl Pts',(-6.32527800500006,15.2,-9.16047453800001));
#282982=CARTESIAN_POINT('Ctrl Pts',(-6.32527800500006,11.6,-9.16047453800001));
#282983=CARTESIAN_POINT('Ctrl Pts',(-6.32253656800006,15.2,-9.15865267500001));
#282984=CARTESIAN_POINT('Ctrl Pts',(-6.32253656800006,11.6,-9.15865267500001));
#282985=CARTESIAN_POINT('Ctrl Pts',(-6.31980075800006,15.2,-9.15683140300001));
#282986=CARTESIAN_POINT('Ctrl Pts',(-6.31980075800006,11.6,-9.15683140300001));
#282987=CARTESIAN_POINT('Ctrl Pts',(-6.31707057700006,15.2,-9.15501073400002));
#282988=CARTESIAN_POINT('Ctrl Pts',(-6.31707057700006,11.6,-9.15501073400002));
#282989=CARTESIAN_POINT('Ctrl Pts',(-6.31434602800006,15.2,-9.15319067500001));
#282990=CARTESIAN_POINT('Ctrl Pts',(-6.31434602800006,11.6,-9.15319067500001));
#282991=CARTESIAN_POINT('Ctrl Pts',(-6.31162711400005,15.2,-9.15137124000001));
#282992=CARTESIAN_POINT('Ctrl Pts',(-6.31162711400005,11.6,-9.15137124000001));
#282993=CARTESIAN_POINT('Ctrl Pts',(-6.30891384000006,15.2,-9.14955243900001));
#282994=CARTESIAN_POINT('Ctrl Pts',(-6.30891384000006,11.6,-9.14955243900001));
#282995=CARTESIAN_POINT('Ctrl Pts',(-6.30620620800006,15.2,-9.14773428000002));
#282996=CARTESIAN_POINT('Ctrl Pts',(-6.30620620800006,11.6,-9.14773428000002));
#282997=CARTESIAN_POINT('Ctrl Pts',(-6.30350422100006,15.2,-9.14591677500002));
#282998=CARTESIAN_POINT('Ctrl Pts',(-6.30350422100006,11.6,-9.14591677500002));
#282999=CARTESIAN_POINT('Ctrl Pts',(-6.30080788400006,15.2,-9.14409993500002));
#283000=CARTESIAN_POINT('Ctrl Pts',(-6.30080788400006,11.6,-9.14409993500002));
#283001=CARTESIAN_POINT('Ctrl Pts',(-6.29811719900006,15.2,-9.14228377000001));
#283002=CARTESIAN_POINT('Ctrl Pts',(-6.29811719900006,11.6,-9.14228377000001));
#283003=CARTESIAN_POINT('Ctrl Pts',(-6.29543217000006,15.2,-9.14046829000002));
#283004=CARTESIAN_POINT('Ctrl Pts',(-6.29543217000006,11.6,-9.14046829000002));
#283005=CARTESIAN_POINT('Ctrl Pts',(-6.29275279900006,15.2,-9.13865350600001));
#283006=CARTESIAN_POINT('Ctrl Pts',(-6.29275279900006,11.6,-9.13865350600001));
#283007=CARTESIAN_POINT('Ctrl Pts',(-6.29007909100006,15.2,-9.13683942900001));
#283008=CARTESIAN_POINT('Ctrl Pts',(-6.29007909100006,11.6,-9.13683942900001));
#283009=CARTESIAN_POINT('Ctrl Pts',(-6.28741104800006,15.2,-9.13502606900002));
#283010=CARTESIAN_POINT('Ctrl Pts',(-6.28741104800006,11.6,-9.13502606900002));
#283011=CARTESIAN_POINT('Ctrl Pts',(-6.28474867400006,15.2,-9.13321343700002));
#283012=CARTESIAN_POINT('Ctrl Pts',(-6.28474867400006,11.6,-9.13321343700002));
#283013=CARTESIAN_POINT('Ctrl Pts',(-6.28209197200006,15.2,-9.13140154300002));
#283014=CARTESIAN_POINT('Ctrl Pts',(-6.28209197200006,11.6,-9.13140154300002));
#283015=CARTESIAN_POINT('Ctrl Pts',(-6.27944094700006,15.2,-9.12959039800001));
#283016=CARTESIAN_POINT('Ctrl Pts',(-6.27944094700006,11.6,-9.12959039800001));
#283017=CARTESIAN_POINT('Ctrl Pts',(-6.27679559900006,15.2,-9.12778001300002));
#283018=CARTESIAN_POINT('Ctrl Pts',(-6.27679559900006,11.6,-9.12778001300002));
#283019=CARTESIAN_POINT('Ctrl Pts',(-6.27415593500006,15.2,-9.12597039800002));
#283020=CARTESIAN_POINT('Ctrl Pts',(-6.27415593500006,11.6,-9.12597039800002));
#283021=CARTESIAN_POINT('Ctrl Pts',(-6.27152195600006,15.2,-9.12416156500001));
#283022=CARTESIAN_POINT('Ctrl Pts',(-6.27152195600006,11.6,-9.12416156500001));
#283023=CARTESIAN_POINT('Ctrl Pts',(-6.26889366400006,15.2,-9.12235352300002));
#283024=CARTESIAN_POINT('Ctrl Pts',(-6.26889366400006,11.6,-9.12235352300002));
#283025=CARTESIAN_POINT('Ctrl Pts',(-6.26627106600006,15.2,-9.12054628500002));
#283026=CARTESIAN_POINT('Ctrl Pts',(-6.26627106600006,11.6,-9.12054628500002));
#283027=CARTESIAN_POINT('Ctrl Pts',(-6.26365416200006,15.2,-9.11873986000002));
#283028=CARTESIAN_POINT('Ctrl Pts',(-6.26365416200006,11.6,-9.11873986000002));
#283029=CARTESIAN_POINT('Ctrl Pts',(-6.26104295800006,15.2,-9.11693426000001));
#283030=CARTESIAN_POINT('Ctrl Pts',(-6.26104295800006,11.6,-9.11693426000001));
#283031=CARTESIAN_POINT('Ctrl Pts',(-6.25843745500006,15.2,-9.11512949500001));
#283032=CARTESIAN_POINT('Ctrl Pts',(-6.25843745500006,11.6,-9.11512949500001));
#283033=CARTESIAN_POINT('Ctrl Pts',(-6.25583765700005,15.2,-9.11332557600002));
#283034=CARTESIAN_POINT('Ctrl Pts',(-6.25583765700005,11.6,-9.11332557600002));
#283035=CARTESIAN_POINT('Ctrl Pts',(-6.25324356800006,15.2,-9.11152251400001));
#283036=CARTESIAN_POINT('Ctrl Pts',(-6.25324356800006,11.6,-9.11152251400001));
#283037=CARTESIAN_POINT('Ctrl Pts',(-6.25065519100006,15.2,-9.10972032100002));
#283038=CARTESIAN_POINT('Ctrl Pts',(-6.25065519100006,11.6,-9.10972032100002));
#283039=CARTESIAN_POINT('Ctrl Pts',(-6.24807252900006,15.2,-9.10791900700002));
#283040=CARTESIAN_POINT('Ctrl Pts',(-6.24807252900006,11.6,-9.10791900700002));
#283041=CARTESIAN_POINT('Ctrl Pts',(-6.24549558500005,15.2,-9.10611858200001));
#283042=CARTESIAN_POINT('Ctrl Pts',(-6.24549558500005,11.6,-9.10611858200001));
#283043=CARTESIAN_POINT('Ctrl Pts',(-6.24292436400006,15.2,-9.10431905900002));
#283044=CARTESIAN_POINT('Ctrl Pts',(-6.24292436400006,11.6,-9.10431905900002));
#283045=CARTESIAN_POINT('Ctrl Pts',(-6.24035886600006,15.2,-9.10252044800002));
#283046=CARTESIAN_POINT('Ctrl Pts',(-6.24035886600006,11.6,-9.10252044800002));
#283047=CARTESIAN_POINT('Ctrl Pts',(-6.23779909800006,15.2,-9.10072276100001));
#283048=CARTESIAN_POINT('Ctrl Pts',(-6.23779909800006,11.6,-9.10072276100001));
#283049=CARTESIAN_POINT('Ctrl Pts',(-6.23524506100006,15.2,-9.09892600700001));
#283050=CARTESIAN_POINT('Ctrl Pts',(-6.23524506100006,11.6,-9.09892600700001));
#283051=CARTESIAN_POINT('Ctrl Pts',(-6.23269675900006,15.2,-9.09713019900002));
#283052=CARTESIAN_POINT('Ctrl Pts',(-6.23269675900006,11.6,-9.09713019900002));
#283053=CARTESIAN_POINT('Ctrl Pts',(-6.23015419600006,15.2,-9.09533534700002));
#283054=CARTESIAN_POINT('Ctrl Pts',(-6.23015419600006,11.6,-9.09533534700002));
#283055=CARTESIAN_POINT('Ctrl Pts',(-6.22761737300006,15.2,-9.09354146400002));
#283056=CARTESIAN_POINT('Ctrl Pts',(-6.22761737300006,11.6,-9.09354146400002));
#283057=CARTESIAN_POINT('Ctrl Pts',(-6.22508629500006,15.2,-9.09174855900002));
#283058=CARTESIAN_POINT('Ctrl Pts',(-6.22508629500006,11.6,-9.09174855900002));
#283059=CARTESIAN_POINT('Ctrl Pts',(-6.22256096500006,15.2,-9.08995664500001));
#283060=CARTESIAN_POINT('Ctrl Pts',(-6.22256096500006,11.6,-9.08995664500001));
#283061=CARTESIAN_POINT('Ctrl Pts',(-6.22004138600006,15.2,-9.08816573200001));
#283062=CARTESIAN_POINT('Ctrl Pts',(-6.22004138600006,11.6,-9.08816573200001));
#283063=CARTESIAN_POINT('Ctrl Pts',(-6.21752756200006,15.2,-9.08637583200001));
#283064=CARTESIAN_POINT('Ctrl Pts',(-6.21752756200006,11.6,-9.08637583200001));
#283065=CARTESIAN_POINT('Ctrl Pts',(-6.21501949600006,15.2,-9.08458695700002));
#283066=CARTESIAN_POINT('Ctrl Pts',(-6.21501949600006,11.6,-9.08458695700002));
#283067=CARTESIAN_POINT('Ctrl Pts',(-6.21251719100006,15.2,-9.08279911600001));
#283068=CARTESIAN_POINT('Ctrl Pts',(-6.21251719100006,11.6,-9.08279911600001));
#283069=CARTESIAN_POINT('Ctrl Pts',(-6.21002065000006,15.2,-9.08101232300002));
#283070=CARTESIAN_POINT('Ctrl Pts',(-6.21002065000006,11.6,-9.08101232300002));
#283071=CARTESIAN_POINT('Ctrl Pts',(-6.20752987700006,15.2,-9.07922658700001));
#283072=CARTESIAN_POINT('Ctrl Pts',(-6.20752987700006,11.6,-9.07922658700001));
#283073=CARTESIAN_POINT('Ctrl Pts',(-6.20504487400006,15.2,-9.07744192200001));
#283074=CARTESIAN_POINT('Ctrl Pts',(-6.20504487400006,11.6,-9.07744192200001));
#283075=CARTESIAN_POINT('Ctrl Pts',(-6.20256564600006,15.2,-9.07565833800002));
#283076=CARTESIAN_POINT('Ctrl Pts',(-6.20256564600006,11.6,-9.07565833800002));
#283077=CARTESIAN_POINT('Ctrl Pts',(-6.20009219500006,15.2,-9.07387584600002));
#283078=CARTESIAN_POINT('Ctrl Pts',(-6.20009219500006,11.6,-9.07387584600002));
#283079=CARTESIAN_POINT('Ctrl Pts',(-6.19762452500006,15.2,-9.07209445800002));
#283080=CARTESIAN_POINT('Ctrl Pts',(-6.19762452500006,11.6,-9.07209445800002));
#283081=CARTESIAN_POINT('Ctrl Pts',(-6.19516263900006,15.2,-9.07031418600001));
#283082=CARTESIAN_POINT('Ctrl Pts',(-6.19516263900006,11.6,-9.07031418600001));
#283083=CARTESIAN_POINT('Ctrl Pts',(-6.19270653900006,15.2,-9.06853504200001));
#283084=CARTESIAN_POINT('Ctrl Pts',(-6.19270653900006,11.6,-9.06853504200001));
#283085=CARTESIAN_POINT('Ctrl Pts',(-6.19025623000006,15.2,-9.06675703600002));
#283086=CARTESIAN_POINT('Ctrl Pts',(-6.19025623000006,11.6,-9.06675703600002));
#283087=CARTESIAN_POINT('Ctrl Pts',(-6.18781171500006,15.2,-9.06498018100002));
#283088=CARTESIAN_POINT('Ctrl Pts',(-6.18781171500006,11.6,-9.06498018100002));
#283089=CARTESIAN_POINT('Ctrl Pts',(-6.18537299700006,15.2,-9.06320448700002));
#283090=CARTESIAN_POINT('Ctrl Pts',(-6.18537299700006,11.6,-9.06320448700002));
#283091=CARTESIAN_POINT('Ctrl Pts',(-6.18294008000006,15.2,-9.06142996800002));
#283092=CARTESIAN_POINT('Ctrl Pts',(-6.18294008000006,11.6,-9.06142996800002));
#283093=CARTESIAN_POINT('Ctrl Pts',(-6.18051296500005,15.2,-9.05965663400002));
#283094=CARTESIAN_POINT('Ctrl Pts',(-6.18051296500005,11.6,-9.05965663400002));
#283095=CARTESIAN_POINT('Ctrl Pts',(-6.17809165700006,15.2,-9.05788449800001));
#283096=CARTESIAN_POINT('Ctrl Pts',(-6.17809165700006,11.6,-9.05788449800001));
#283097=CARTESIAN_POINT('Ctrl Pts',(-6.17567615900006,15.2,-9.05611357000002));
#283098=CARTESIAN_POINT('Ctrl Pts',(-6.17567615900006,11.6,-9.05611357000002));
#283099=CARTESIAN_POINT('Ctrl Pts',(-6.17326647500006,15.2,-9.05434386300002));
#283100=CARTESIAN_POINT('Ctrl Pts',(-6.17326647500006,11.6,-9.05434386300002));
#283101=CARTESIAN_POINT('Ctrl Pts',(-6.17086260700006,15.2,-9.05257538800001));
#283102=CARTESIAN_POINT('Ctrl Pts',(-6.17086260700006,11.6,-9.05257538800001));
#283103=CARTESIAN_POINT('Ctrl Pts',(-6.16846455700006,15.2,-9.05080815900002));
#283104=CARTESIAN_POINT('Ctrl Pts',(-6.16846455700006,11.6,-9.05080815900002));
#283105=CARTESIAN_POINT('Ctrl Pts',(-6.16607233200006,15.2,-9.04904218600001));
#283106=CARTESIAN_POINT('Ctrl Pts',(-6.16607233200006,11.6,-9.04904218600001));
#283107=CARTESIAN_POINT('Ctrl Pts',(-6.16368593200006,15.2,-9.04727748100001));
#283108=CARTESIAN_POINT('Ctrl Pts',(-6.16368593200006,11.6,-9.04727748100001));
#283109=CARTESIAN_POINT('Ctrl Pts',(-6.16130536200005,15.2,-9.04551405600002));
#283110=CARTESIAN_POINT('Ctrl Pts',(-6.16130536200005,11.6,-9.04551405600002));
#283111=CARTESIAN_POINT('Ctrl Pts',(-6.15893062400006,15.2,-9.04375192400002));
#283112=CARTESIAN_POINT('Ctrl Pts',(-6.15893062400006,11.6,-9.04375192400002));
#283113=CARTESIAN_POINT('Ctrl Pts',(-6.15656172200006,15.2,-9.04199109600002));
#283114=CARTESIAN_POINT('Ctrl Pts',(-6.15656172200006,11.6,-9.04199109600002));
#283115=CARTESIAN_POINT('Ctrl Pts',(-6.15419866000006,15.2,-9.04023158300001));
#283116=CARTESIAN_POINT('Ctrl Pts',(-6.15419866000006,11.6,-9.04023158300001));
#283117=CARTESIAN_POINT('Ctrl Pts',(-6.15184143900006,15.2,-9.03847340000001));
#283118=CARTESIAN_POINT('Ctrl Pts',(-6.15184143900006,11.6,-9.03847340000001));
#283119=CARTESIAN_POINT('Ctrl Pts',(-6.14949006400006,15.2,-9.03671655700002));
#283120=CARTESIAN_POINT('Ctrl Pts',(-6.14949006400006,11.6,-9.03671655700002));
#283121=CARTESIAN_POINT('Ctrl Pts',(-6.14714453800006,15.2,-9.03496106700001));
#283122=CARTESIAN_POINT('Ctrl Pts',(-6.14714453800006,11.6,-9.03496106700001));
#283123=CARTESIAN_POINT('Ctrl Pts',(-6.14480486400006,15.2,-9.03320694000002));
#283124=CARTESIAN_POINT('Ctrl Pts',(-6.14480486400006,11.6,-9.03320694000002));
#283125=CARTESIAN_POINT('Ctrl Pts',(-6.14247104500006,15.2,-9.03145419100002));
#283126=CARTESIAN_POINT('Ctrl Pts',(-6.14247104500006,11.6,-9.03145419100002));
#283127=CARTESIAN_POINT('Ctrl Pts',(-6.14014308400006,15.2,-9.02970283200002));
#283128=CARTESIAN_POINT('Ctrl Pts',(-6.14014308400006,11.6,-9.02970283200002));
#283129=CARTESIAN_POINT('Ctrl Pts',(-6.13782098400006,15.2,-9.02795287300002));
#283130=CARTESIAN_POINT('Ctrl Pts',(-6.13782098400006,11.6,-9.02795287300002));
#283131=CARTESIAN_POINT('Ctrl Pts',(-6.13550475100006,15.2,-9.02620432800001));
#283132=CARTESIAN_POINT('Ctrl Pts',(-6.13550475100006,11.6,-9.02620432800001));
#283133=CARTESIAN_POINT('Ctrl Pts',(-6.13319438500006,15.2,-9.02445720900002));
#283134=CARTESIAN_POINT('Ctrl Pts',(-6.13319438500006,11.6,-9.02445720900002));
#283135=CARTESIAN_POINT('Ctrl Pts',(-6.13088988900006,15.2,-9.02271152900001));
#283136=CARTESIAN_POINT('Ctrl Pts',(-6.13088988900006,11.6,-9.02271152900001));
#283137=CARTESIAN_POINT('Ctrl Pts',(-6.12859126900006,15.2,-9.02096729900002));
#283138=CARTESIAN_POINT('Ctrl Pts',(-6.12859126900006,11.6,-9.02096729900002));
#283139=CARTESIAN_POINT('Ctrl Pts',(-6.12629852600006,15.2,-9.01922453300001));
#283140=CARTESIAN_POINT('Ctrl Pts',(-6.12629852600006,11.6,-9.01922453300001));
#283141=CARTESIAN_POINT('Ctrl Pts',(-6.12401166400006,15.2,-9.01748324100001));
#283142=CARTESIAN_POINT('Ctrl Pts',(-6.12401166400006,11.6,-9.01748324100001));
#283143=CARTESIAN_POINT('Ctrl Pts',(-6.12173068600006,15.2,-9.01574343800002));
#283144=CARTESIAN_POINT('Ctrl Pts',(-6.12173068600006,11.6,-9.01574343800002));
#283145=CARTESIAN_POINT('Ctrl Pts',(-6.11945559600006,15.2,-9.01400513500001));
#283146=CARTESIAN_POINT('Ctrl Pts',(-6.11945559600006,11.6,-9.01400513500001));
#283147=CARTESIAN_POINT('Ctrl Pts',(-6.11718639600006,15.2,-9.01226834500001));
#283148=CARTESIAN_POINT('Ctrl Pts',(-6.11718639600006,11.6,-9.01226834500001));
#283149=CARTESIAN_POINT('Ctrl Pts',(-6.11492309000006,15.2,-9.01053308200002));
#283150=CARTESIAN_POINT('Ctrl Pts',(-6.11492309000006,11.6,-9.01053308200002));
#283151=CARTESIAN_POINT('Ctrl Pts',(-6.11266568000006,15.2,-9.00879935600001));
#283152=CARTESIAN_POINT('Ctrl Pts',(-6.11266568000006,11.6,-9.00879935600001));
#283153=CARTESIAN_POINT('Ctrl Pts',(-6.11041417200005,15.2,-9.00706718000002));
#283154=CARTESIAN_POINT('Ctrl Pts',(-6.11041417200005,11.6,-9.00706718000002));
#283155=CARTESIAN_POINT('Ctrl Pts',(-6.10816856500006,15.2,-9.00533656900001));
#283156=CARTESIAN_POINT('Ctrl Pts',(-6.10816856500006,11.6,-9.00533656900001));
#283157=CARTESIAN_POINT('Ctrl Pts',(-6.10592886600006,15.2,-9.00360753300001));
#283158=CARTESIAN_POINT('Ctrl Pts',(-6.10592886600006,11.6,-9.00360753300001));
#283159=CARTESIAN_POINT('Ctrl Pts',(-6.10369507600006,15.2,-9.00188008700002));
#283160=CARTESIAN_POINT('Ctrl Pts',(-6.10369507600006,11.6,-9.00188008700002));
#283161=CARTESIAN_POINT('Ctrl Pts',(-6.10146719900006,15.2,-9.00015424200001));
#283162=CARTESIAN_POINT('Ctrl Pts',(-6.10146719900006,11.6,-9.00015424200001));
#283163=CARTESIAN_POINT('Ctrl Pts',(-6.09924523800006,15.2,-8.99843001200002));
#283164=CARTESIAN_POINT('Ctrl Pts',(-6.09924523800006,11.6,-8.99843001200002));
#283165=CARTESIAN_POINT('Ctrl Pts',(-6.09702919700006,15.2,-8.99670741000002));
#283166=CARTESIAN_POINT('Ctrl Pts',(-6.09702919700006,11.6,-8.99670741000002));
#283167=CARTESIAN_POINT('Ctrl Pts',(-6.09481907700006,15.2,-8.99498644800002));
#283168=CARTESIAN_POINT('Ctrl Pts',(-6.09481907700006,11.6,-8.99498644800002));
#283169=CARTESIAN_POINT('Ctrl Pts',(-6.09261488400006,15.2,-8.99326713800002));
#283170=CARTESIAN_POINT('Ctrl Pts',(-6.09261488400006,11.6,-8.99326713800002));
#283171=CARTESIAN_POINT('Ctrl Pts',(-6.09041662000006,15.2,-8.99154949500002));
#283172=CARTESIAN_POINT('Ctrl Pts',(-6.09041662000006,11.6,-8.99154949500002));
#283173=CARTESIAN_POINT('Ctrl Pts',(-6.08822428600006,15.2,-8.98983353000002));
#283174=CARTESIAN_POINT('Ctrl Pts',(-6.08822428600006,11.6,-8.98983353000002));
#283175=CARTESIAN_POINT('Ctrl Pts',(-6.08603788900006,15.2,-8.98811925800001));
#283176=CARTESIAN_POINT('Ctrl Pts',(-6.08603788900006,11.6,-8.98811925800001));
#283177=CARTESIAN_POINT('Ctrl Pts',(-6.08385743000006,15.2,-8.98640669100002));
#283178=CARTESIAN_POINT('Ctrl Pts',(-6.08385743000006,11.6,-8.98640669100002));
#283179=CARTESIAN_POINT('Ctrl Pts',(-6.08168291200006,15.2,-8.98469584100001));
#283180=CARTESIAN_POINT('Ctrl Pts',(-6.08168291200006,11.6,-8.98469584100001));
#283181=CARTESIAN_POINT('Ctrl Pts',(-6.07951433900006,15.2,-8.98298672300001));
#283182=CARTESIAN_POINT('Ctrl Pts',(-6.07951433900006,11.6,-8.98298672300001));
#283183=CARTESIAN_POINT('Ctrl Pts',(-6.07735171400006,15.2,-8.98127934900002));
#283184=CARTESIAN_POINT('Ctrl Pts',(-6.07735171400006,11.6,-8.98127934900002));
#283185=CARTESIAN_POINT('Ctrl Pts',(-6.07519504000006,15.2,-8.97957373400001));
#283186=CARTESIAN_POINT('Ctrl Pts',(-6.07519504000006,11.6,-8.97957373400001));
#283187=CARTESIAN_POINT('Ctrl Pts',(-6.07304431900006,15.2,-8.97786988800001));
#283188=CARTESIAN_POINT('Ctrl Pts',(-6.07304431900006,11.6,-8.97786988800001));
#283189=CARTESIAN_POINT('Ctrl Pts',(-6.07089955600006,15.2,-8.97616782700002));
#283190=CARTESIAN_POINT('Ctrl Pts',(-6.07089955600006,11.6,-8.97616782700002));
#283191=CARTESIAN_POINT('Ctrl Pts',(-6.06876075400006,15.2,-8.97446756300001));
#283192=CARTESIAN_POINT('Ctrl Pts',(-6.06876075400006,11.6,-8.97446756300001));
#283193=CARTESIAN_POINT('Ctrl Pts',(-6.06662791600006,15.2,-8.97276910900001));
#283194=CARTESIAN_POINT('Ctrl Pts',(-6.06662791600006,11.6,-8.97276910900001));
#283195=CARTESIAN_POINT('Ctrl Pts',(-6.06450104400006,15.2,-8.97107248000001));
#283196=CARTESIAN_POINT('Ctrl Pts',(-6.06450104400006,11.6,-8.97107248000001));
#283197=CARTESIAN_POINT('Ctrl Pts',(-6.06238014200006,15.2,-8.96937768800001));
#283198=CARTESIAN_POINT('Ctrl Pts',(-6.06238014200006,11.6,-8.96937768800001));
#283199=CARTESIAN_POINT('Ctrl Pts',(-6.06026521300006,15.2,-8.96768474600002));
#283200=CARTESIAN_POINT('Ctrl Pts',(-6.06026521300006,11.6,-8.96768474600002));
#283201=CARTESIAN_POINT('Ctrl Pts',(-6.05815626100005,15.2,-8.96599367000002));
#283202=CARTESIAN_POINT('Ctrl Pts',(-6.05815626100005,11.6,-8.96599367000002));
#283203=CARTESIAN_POINT('Ctrl Pts',(-6.05605328900006,15.2,-8.96430447000002));
#283204=CARTESIAN_POINT('Ctrl Pts',(-6.05605328900006,11.6,-8.96430447000002));
#283205=CARTESIAN_POINT('Ctrl Pts',(-6.05395629800006,15.2,-8.96261716200002));
#283206=CARTESIAN_POINT('Ctrl Pts',(-6.05395629800006,11.6,-8.96261716200002));
#283207=CARTESIAN_POINT('Ctrl Pts',(-6.05186529400005,15.2,-8.96093175800001));
#283208=CARTESIAN_POINT('Ctrl Pts',(-6.05186529400005,11.6,-8.96093175800001));
#283209=CARTESIAN_POINT('Ctrl Pts',(-6.04978027800006,15.2,-8.95924827300002));
#283210=CARTESIAN_POINT('Ctrl Pts',(-6.04978027800006,11.6,-8.95924827300002));
#283211=CARTESIAN_POINT('Ctrl Pts',(-6.04770125400006,15.2,-8.95756672100001));
#283212=CARTESIAN_POINT('Ctrl Pts',(-6.04770125400006,11.6,-8.95756672100001));
#283213=CARTESIAN_POINT('Ctrl Pts',(-6.04562822600006,15.2,-8.95588711400002));
#283214=CARTESIAN_POINT('Ctrl Pts',(-6.04562822600006,11.6,-8.95588711400002));
#283215=CARTESIAN_POINT('Ctrl Pts',(-6.04356119600006,15.2,-8.95420946700002));
#283216=CARTESIAN_POINT('Ctrl Pts',(-6.04356119600006,11.6,-8.95420946700002));
#283217=CARTESIAN_POINT('Ctrl Pts',(-6.04150016700006,15.2,-8.95253379300001));
#283218=CARTESIAN_POINT('Ctrl Pts',(-6.04150016700006,11.6,-8.95253379300001));
#283219=CARTESIAN_POINT('Ctrl Pts',(-6.03944514200006,15.2,-8.95086010500002));
#283220=CARTESIAN_POINT('Ctrl Pts',(-6.03944514200006,11.6,-8.95086010500002));
#283221=CARTESIAN_POINT('Ctrl Pts',(-6.03739612600006,15.2,-8.94918841900001));
#283222=CARTESIAN_POINT('Ctrl Pts',(-6.03739612600006,11.6,-8.94918841900001));
#283223=CARTESIAN_POINT('Ctrl Pts',(-6.03535312000006,15.2,-8.94751874800002));
#283224=CARTESIAN_POINT('Ctrl Pts',(-6.03535312000006,11.6,-8.94751874800002));
#283225=CARTESIAN_POINT('Ctrl Pts',(-6.03331612900006,15.2,-8.94585110500002));
#283226=CARTESIAN_POINT('Ctrl Pts',(-6.03331612900006,11.6,-8.94585110500002));
#283227=CARTESIAN_POINT('Ctrl Pts',(-6.03128515400006,15.2,-8.94418550400001));
#283228=CARTESIAN_POINT('Ctrl Pts',(-6.03128515400006,11.6,-8.94418550400001));
#283229=CARTESIAN_POINT('Ctrl Pts',(-6.02926019900006,15.2,-8.94252196100001));
#283230=CARTESIAN_POINT('Ctrl Pts',(-6.02926019900006,11.6,-8.94252196100001));
#283231=CARTESIAN_POINT('Ctrl Pts',(-6.02724126900006,15.2,-8.94086048800002));
#283232=CARTESIAN_POINT('Ctrl Pts',(-6.02724126900006,11.6,-8.94086048800002));
#283233=CARTESIAN_POINT('Ctrl Pts',(-6.02522836400006,15.2,-8.93920110000002));
#283234=CARTESIAN_POINT('Ctrl Pts',(-6.02522836400006,11.6,-8.93920110000002));
#283235=CARTESIAN_POINT('Ctrl Pts',(-6.02322148900006,15.2,-8.93754381100001));
#283236=CARTESIAN_POINT('Ctrl Pts',(-6.02322148900006,11.6,-8.93754381100001));
#283237=CARTESIAN_POINT('Ctrl Pts',(-6.02122064700006,15.2,-8.93588863500002));
#283238=CARTESIAN_POINT('Ctrl Pts',(-6.02122064700006,11.6,-8.93588863500002));
#283239=CARTESIAN_POINT('Ctrl Pts',(-6.01922584100006,15.2,-8.93423558600002));
#283240=CARTESIAN_POINT('Ctrl Pts',(-6.01922584100006,11.6,-8.93423558600002));
#283241=CARTESIAN_POINT('Ctrl Pts',(-6.01723707400006,15.2,-8.93258467900001));
#283242=CARTESIAN_POINT('Ctrl Pts',(-6.01723707400006,11.6,-8.93258467900001));
#283243=CARTESIAN_POINT('Ctrl Pts',(-6.01525434800006,15.2,-8.93093592700002));
#283244=CARTESIAN_POINT('Ctrl Pts',(-6.01525434800006,11.6,-8.93093592700002));
#283245=CARTESIAN_POINT('Ctrl Pts',(-6.01327766800006,15.2,-8.92928934400001));
#283246=CARTESIAN_POINT('Ctrl Pts',(-6.01327766800006,11.6,-8.92928934400001));
#283247=CARTESIAN_POINT('Ctrl Pts',(-6.01130703700006,15.2,-8.92764494600002));
#283248=CARTESIAN_POINT('Ctrl Pts',(-6.01130703700006,11.6,-8.92764494600002));
#283249=CARTESIAN_POINT('Ctrl Pts',(-6.00934245600006,15.2,-8.92600274700002));
#283250=CARTESIAN_POINT('Ctrl Pts',(-6.00934245600006,11.6,-8.92600274700002));
#283251=CARTESIAN_POINT('Ctrl Pts',(-6.00738393100006,15.2,-8.92436276200002));
#283252=CARTESIAN_POINT('Ctrl Pts',(-6.00738393100006,11.6,-8.92436276200002));
#283253=CARTESIAN_POINT('Ctrl Pts',(-6.00543146200006,15.2,-8.92272500300002));
#283254=CARTESIAN_POINT('Ctrl Pts',(-6.00543146200006,11.6,-8.92272500300002));
#283255=CARTESIAN_POINT('Ctrl Pts',(-6.00348505500006,15.2,-8.92108948700002));
#283256=CARTESIAN_POINT('Ctrl Pts',(-6.00348505500006,11.6,-8.92108948700002));
#283257=CARTESIAN_POINT('Ctrl Pts',(-6.00154471100006,15.2,-8.91945622800002));
#283258=CARTESIAN_POINT('Ctrl Pts',(-6.00154471100006,11.6,-8.91945622800002));
#283259=CARTESIAN_POINT('Ctrl Pts',(-5.99961043400006,15.2,-8.91782524000002));
#283260=CARTESIAN_POINT('Ctrl Pts',(-5.99961043400006,11.6,-8.91782524000002));
#283261=CARTESIAN_POINT('Ctrl Pts',(-5.99768222800006,15.2,-8.91619653700002));
#283262=CARTESIAN_POINT('Ctrl Pts',(-5.99768222800006,11.6,-8.91619653700002));
#283263=CARTESIAN_POINT('Ctrl Pts',(-5.99576009400006,15.2,-8.91457013600002));
#283264=CARTESIAN_POINT('Ctrl Pts',(-5.99576009400006,11.6,-8.91457013600002));
#283265=CARTESIAN_POINT('Ctrl Pts',(-5.99384403600006,15.2,-8.91294604900001));
#283266=CARTESIAN_POINT('Ctrl Pts',(-5.99384403600006,11.6,-8.91294604900001));
#283267=CARTESIAN_POINT('Ctrl Pts',(-5.99193405800006,15.2,-8.91132429300002));
#283268=CARTESIAN_POINT('Ctrl Pts',(-5.99193405800006,11.6,-8.91132429300002));
#283269=CARTESIAN_POINT('Ctrl Pts',(-5.99003016200006,15.2,-8.90970488200002));
#283270=CARTESIAN_POINT('Ctrl Pts',(-5.99003016200006,11.6,-8.90970488200002));
#283271=CARTESIAN_POINT('Ctrl Pts',(-5.98813235200006,15.2,-8.90808783100002));
#283272=CARTESIAN_POINT('Ctrl Pts',(-5.98813235200006,11.6,-8.90808783100002));
#283273=CARTESIAN_POINT('Ctrl Pts',(-5.98624062900006,15.2,-8.90647315300001));
#283274=CARTESIAN_POINT('Ctrl Pts',(-5.98624062900006,11.6,-8.90647315300001));
#283275=CARTESIAN_POINT('Ctrl Pts',(-5.98435500000006,15.2,-8.90486086600001));
#283276=CARTESIAN_POINT('Ctrl Pts',(-5.98435500000006,11.6,-8.90486086600001));
#283277=CARTESIAN_POINT('Ctrl Pts',(-5.98247546400006,15.2,-8.90325098400002));
#283278=CARTESIAN_POINT('Ctrl Pts',(-5.98247546400006,11.6,-8.90325098400002));
#283279=CARTESIAN_POINT('Ctrl Pts',(-5.98060202600006,15.2,-8.90164352000001));
#283280=CARTESIAN_POINT('Ctrl Pts',(-5.98060202600006,11.6,-8.90164352000001));
#283281=CARTESIAN_POINT('Ctrl Pts',(-5.97873468900006,15.2,-8.90003849100001));
#283282=CARTESIAN_POINT('Ctrl Pts',(-5.97873468900006,11.6,-8.90003849100001));
#283283=CARTESIAN_POINT('Ctrl Pts',(-5.97687345600006,15.2,-8.89843591300002));
#283284=CARTESIAN_POINT('Ctrl Pts',(-5.97687345600006,11.6,-8.89843591300002));
#283285=CARTESIAN_POINT('Ctrl Pts',(-5.97501833000006,15.2,-8.89683579900002));
#283286=CARTESIAN_POINT('Ctrl Pts',(-5.97501833000006,11.6,-8.89683579900002));
#283287=CARTESIAN_POINT('Ctrl Pts',(-5.97316931400006,15.2,-8.89523816500001));
#283288=CARTESIAN_POINT('Ctrl Pts',(-5.97316931400006,11.6,-8.89523816500001));
#283289=CARTESIAN_POINT('Ctrl Pts',(-5.97132641200006,15.2,-8.89364302600002));
#283290=CARTESIAN_POINT('Ctrl Pts',(-5.97132641200006,11.6,-8.89364302600002));
#283291=CARTESIAN_POINT('Ctrl Pts',(-5.96948962500006,15.2,-8.89205039900002));
#283292=CARTESIAN_POINT('Ctrl Pts',(-5.96948962500006,11.6,-8.89205039900002));
#283293=CARTESIAN_POINT('Ctrl Pts',(-5.96765895700006,15.2,-8.89046029700001));
#283294=CARTESIAN_POINT('Ctrl Pts',(-5.96765895700006,11.6,-8.89046029700001));
#283295=CARTESIAN_POINT('Ctrl Pts',(-5.96583441200006,15.2,-8.88887273700002));
#283296=CARTESIAN_POINT('Ctrl Pts',(-5.96583441200006,11.6,-8.88887273700002));
#283297=CARTESIAN_POINT('Ctrl Pts',(-5.96401599300005,15.2,-8.88728773400001));
#283298=CARTESIAN_POINT('Ctrl Pts',(-5.96401599300005,11.6,-8.88728773400001));
#283299=CARTESIAN_POINT('Ctrl Pts',(-5.96220370200006,15.2,-8.88570530200001));
#283300=CARTESIAN_POINT('Ctrl Pts',(-5.96220370200006,11.6,-8.88570530200001));
#283301=CARTESIAN_POINT('Ctrl Pts',(-5.96039754200006,15.2,-8.88412545900002));
#283302=CARTESIAN_POINT('Ctrl Pts',(-5.96039754200006,11.6,-8.88412545900002));
#283303=CARTESIAN_POINT('Ctrl Pts',(-5.95859751600006,15.2,-8.88254821900002));
#283304=CARTESIAN_POINT('Ctrl Pts',(-5.95859751600006,11.6,-8.88254821900002));
#283305=CARTESIAN_POINT('Ctrl Pts',(-5.95680362900006,15.2,-8.88097359800001));
#283306=CARTESIAN_POINT('Ctrl Pts',(-5.95680362900006,11.6,-8.88097359800001));
#283307=CARTESIAN_POINT('Ctrl Pts',(-5.95501588200006,15.2,-8.87940161100002));
#283308=CARTESIAN_POINT('Ctrl Pts',(-5.95501588200006,11.6,-8.87940161100002));
#283309=CARTESIAN_POINT('Ctrl Pts',(-5.95323427900006,15.2,-8.87783227600002));
#283310=CARTESIAN_POINT('Ctrl Pts',(-5.95323427900006,11.6,-8.87783227600002));
#283311=CARTESIAN_POINT('Ctrl Pts',(-5.95145882200006,15.2,-8.87626560600001));
#283312=CARTESIAN_POINT('Ctrl Pts',(-5.95145882200006,11.6,-8.87626560600001));
#283313=CARTESIAN_POINT('Ctrl Pts',(-5.94968951600006,15.2,-8.87470161900002));
#283314=CARTESIAN_POINT('Ctrl Pts',(-5.94968951600006,11.6,-8.87470161900002));
#283315=CARTESIAN_POINT('Ctrl Pts',(-5.94792636200006,15.2,-8.87314032800001));
#283316=CARTESIAN_POINT('Ctrl Pts',(-5.94792636200006,11.6,-8.87314032800001));
#283317=CARTESIAN_POINT('Ctrl Pts',(-5.94616936500006,15.2,-8.87158175200002));
#283318=CARTESIAN_POINT('Ctrl Pts',(-5.94616936500006,11.6,-8.87158175200002));
#283319=CARTESIAN_POINT('Ctrl Pts',(-5.94441852600006,15.2,-8.87002590600002));
#283320=CARTESIAN_POINT('Ctrl Pts',(-5.94441852600006,11.6,-8.87002590600002));
#283321=CARTESIAN_POINT('Ctrl Pts',(-5.94267384900006,15.2,-8.86847280400002));
#283322=CARTESIAN_POINT('Ctrl Pts',(-5.94267384900006,11.6,-8.86847280400002));
#283323=CARTESIAN_POINT('Ctrl Pts',(-5.94093533700006,15.2,-8.86692246600001));
#283324=CARTESIAN_POINT('Ctrl Pts',(-5.94093533700006,11.6,-8.86692246600001));
#283325=CARTESIAN_POINT('Ctrl Pts',(-5.93920299300006,15.2,-8.86537490400002));
#283326=CARTESIAN_POINT('Ctrl Pts',(-5.93920299300006,11.6,-8.86537490400002));
#283327=CARTESIAN_POINT('Ctrl Pts',(-5.93747681900005,15.2,-8.86383013700001));
#283328=CARTESIAN_POINT('Ctrl Pts',(-5.93747681900005,11.6,-8.86383013700001));
#283329=CARTESIAN_POINT('Ctrl Pts',(-5.93575682000006,15.2,-8.86228817900001));
#283330=CARTESIAN_POINT('Ctrl Pts',(-5.93575682000006,11.6,-8.86228817900001));
#283331=CARTESIAN_POINT('Ctrl Pts',(-5.93404299900006,15.2,-8.86074904800001));
#283332=CARTESIAN_POINT('Ctrl Pts',(-5.93404299900006,11.6,-8.86074904800001));
#283333=CARTESIAN_POINT('Ctrl Pts',(-5.93233535700006,15.2,-8.85921276000002));
#283334=CARTESIAN_POINT('Ctrl Pts',(-5.93233535700006,11.6,-8.85921276000002));
#283335=CARTESIAN_POINT('Ctrl Pts',(-5.93063389800006,15.2,-8.85767933100002));
#283336=CARTESIAN_POINT('Ctrl Pts',(-5.93063389800006,11.6,-8.85767933100002));
#283337=CARTESIAN_POINT('Ctrl Pts',(-5.92893862600006,15.2,-8.85614877700002));
#283338=CARTESIAN_POINT('Ctrl Pts',(-5.92893862600006,11.6,-8.85614877700002));
#283339=CARTESIAN_POINT('Ctrl Pts',(-5.92724954300006,15.2,-8.85462111500001));
#283340=CARTESIAN_POINT('Ctrl Pts',(-5.92724954300006,11.6,-8.85462111500001));
#283341=CARTESIAN_POINT('Ctrl Pts',(-5.92556665300005,15.2,-8.85309636200001));
#283342=CARTESIAN_POINT('Ctrl Pts',(-5.92556665300005,11.6,-8.85309636200001));
#283343=CARTESIAN_POINT('Ctrl Pts',(-5.92388995600006,15.2,-8.85157453400002));
#283344=CARTESIAN_POINT('Ctrl Pts',(-5.92388995600006,11.6,-8.85157453400002));
#283345=CARTESIAN_POINT('Ctrl Pts',(-5.92221945900006,15.2,-8.85005564700002));
#283346=CARTESIAN_POINT('Ctrl Pts',(-5.92221945900006,11.6,-8.85005564700002));
#283347=CARTESIAN_POINT('Ctrl Pts',(-5.92055516300006,15.2,-8.84853971800002));
#283348=CARTESIAN_POINT('Ctrl Pts',(-5.92055516300006,11.6,-8.84853971800002));
#283349=CARTESIAN_POINT('Ctrl Pts',(-5.91889707100006,15.2,-8.84702676400002));
#283350=CARTESIAN_POINT('Ctrl Pts',(-5.91889707100006,11.6,-8.84702676400002));
#283351=CARTESIAN_POINT('Ctrl Pts',(-5.91724518600006,15.2,-8.84551680200002));
#283352=CARTESIAN_POINT('Ctrl Pts',(-5.91724518600006,11.6,-8.84551680200002));
#283353=CARTESIAN_POINT('Ctrl Pts',(-5.91559951200006,15.2,-8.84400984900001));
#283354=CARTESIAN_POINT('Ctrl Pts',(-5.91559951200006,11.6,-8.84400984900001));
#283355=CARTESIAN_POINT('Ctrl Pts',(-5.91396005000006,15.2,-8.84250592100001));
#283356=CARTESIAN_POINT('Ctrl Pts',(-5.91396005000006,11.6,-8.84250592100001));
#283357=CARTESIAN_POINT('Ctrl Pts',(-5.91232680500006,15.2,-8.84100503500001));
#283358=CARTESIAN_POINT('Ctrl Pts',(-5.91232680500006,11.6,-8.84100503500001));
#283359=CARTESIAN_POINT('Ctrl Pts',(-5.91069977900006,15.2,-8.83950721000001));
#283360=CARTESIAN_POINT('Ctrl Pts',(-5.91069977900006,11.6,-8.83950721000001));
#283361=CARTESIAN_POINT('Ctrl Pts',(-5.90907897600006,15.2,-8.83801246000001));
#283362=CARTESIAN_POINT('Ctrl Pts',(-5.90907897600006,11.6,-8.83801246000001));
#283363=CARTESIAN_POINT('Ctrl Pts',(-5.90746439700006,15.2,-8.83652080200001));
#283364=CARTESIAN_POINT('Ctrl Pts',(-5.90746439700006,11.6,-8.83652080200001));
#283365=CARTESIAN_POINT('Ctrl Pts',(-5.90585604700006,15.2,-8.83503225700002));
#283366=CARTESIAN_POINT('Ctrl Pts',(-5.90585604700006,11.6,-8.83503225700002));
#283367=CARTESIAN_POINT('Ctrl Pts',(-5.90425392900006,15.2,-8.83354683900002));
#283368=CARTESIAN_POINT('Ctrl Pts',(-5.90425392900006,11.6,-8.83354683900002));
#283369=CARTESIAN_POINT('Ctrl Pts',(-5.90265804300006,15.2,-8.83206456600002));
#283370=CARTESIAN_POINT('Ctrl Pts',(-5.90265804300006,11.6,-8.83206456600002));
#283371=CARTESIAN_POINT('Ctrl Pts',(-5.90106839700006,15.2,-8.83058545500001));
#283372=CARTESIAN_POINT('Ctrl Pts',(-5.90106839700006,11.6,-8.83058545500001));
#283373=CARTESIAN_POINT('Ctrl Pts',(-5.89948498900006,15.2,-8.82910952300002));
#283374=CARTESIAN_POINT('Ctrl Pts',(-5.89948498900006,11.6,-8.82910952300002));
#283375=CARTESIAN_POINT('Ctrl Pts',(-5.89790782500006,15.2,-8.82763679000002));
#283376=CARTESIAN_POINT('Ctrl Pts',(-5.89790782500006,11.6,-8.82763679000002));
#283377=CARTESIAN_POINT('Ctrl Pts',(-5.89633690700006,15.2,-8.82616727000002));
#283378=CARTESIAN_POINT('Ctrl Pts',(-5.89633690700006,11.6,-8.82616727000002));
#283379=CARTESIAN_POINT('Ctrl Pts',(-5.89477223700006,15.2,-8.82470098400002));
#283380=CARTESIAN_POINT('Ctrl Pts',(-5.89477223700006,11.6,-8.82470098400002));
#283381=CARTESIAN_POINT('Ctrl Pts',(-5.89321382100006,15.2,-8.82323794600002));
#283382=CARTESIAN_POINT('Ctrl Pts',(-5.89321382100006,11.6,-8.82323794600002));
#283383=CARTESIAN_POINT('Ctrl Pts',(-5.89166165900005,15.2,-8.82177817600001));
#283384=CARTESIAN_POINT('Ctrl Pts',(-5.89166165900005,11.6,-8.82177817600001));
#283385=CARTESIAN_POINT('Ctrl Pts',(-5.89011575500006,15.2,-8.82032169100002));
#283386=CARTESIAN_POINT('Ctrl Pts',(-5.89011575500006,11.6,-8.82032169100002));
#283387=CARTESIAN_POINT('Ctrl Pts',(-5.88857611200006,15.2,-8.81886851000001));
#283388=CARTESIAN_POINT('Ctrl Pts',(-5.88857611200006,11.6,-8.81886851000001));
#283389=CARTESIAN_POINT('Ctrl Pts',(-5.88704273400006,15.2,-8.81741864800002));
#283390=CARTESIAN_POINT('Ctrl Pts',(-5.88704273400006,11.6,-8.81741864800002));
#283391=CARTESIAN_POINT('Ctrl Pts',(-5.88551562100006,15.2,-8.81597212600001));
#283392=CARTESIAN_POINT('Ctrl Pts',(-5.88551562100006,11.6,-8.81597212600001));
#283393=CARTESIAN_POINT('Ctrl Pts',(-5.88399477900006,15.2,-8.81452896000001));
#283394=CARTESIAN_POINT('Ctrl Pts',(-5.88399477900006,11.6,-8.81452896000001));
#283395=CARTESIAN_POINT('Ctrl Pts',(-5.88248021000005,15.2,-8.81308916900002));
#283396=CARTESIAN_POINT('Ctrl Pts',(-5.88248021000005,11.6,-8.81308916900002));
#283397=CARTESIAN_POINT('Ctrl Pts',(-5.88097191600006,15.2,-8.81165276900001));
#283398=CARTESIAN_POINT('Ctrl Pts',(-5.88097191600006,11.6,-8.81165276900001));
#283399=CARTESIAN_POINT('Ctrl Pts',(-5.87946990200006,15.2,-8.81021978100001));
#283400=CARTESIAN_POINT('Ctrl Pts',(-5.87946990200006,11.6,-8.81021978100001));
#283401=CARTESIAN_POINT('Ctrl Pts',(-5.87797416900006,15.2,-8.80879022300002));
#283402=CARTESIAN_POINT('Ctrl Pts',(-5.87797416900006,11.6,-8.80879022300002));
#283403=CARTESIAN_POINT('Ctrl Pts',(-5.87648472000006,15.2,-8.80736411100001));
#283404=CARTESIAN_POINT('Ctrl Pts',(-5.87648472000006,11.6,-8.80736411100001));
#283405=CARTESIAN_POINT('Ctrl Pts',(-5.87500155900006,15.2,-8.80594146500002));
#283406=CARTESIAN_POINT('Ctrl Pts',(-5.87500155900006,11.6,-8.80594146500002));
#283407=CARTESIAN_POINT('Ctrl Pts',(-5.87352468900006,15.2,-8.80452230300002));
#283408=CARTESIAN_POINT('Ctrl Pts',(-5.87352468900006,11.6,-8.80452230300002));
#283409=CARTESIAN_POINT('Ctrl Pts',(-5.87205411200006,15.2,-8.80310664200002));
#283410=CARTESIAN_POINT('Ctrl Pts',(-5.87205411200006,11.6,-8.80310664200002));
#283411=CARTESIAN_POINT('Ctrl Pts',(-5.87058983200006,15.2,-8.80169450300002));
#283412=CARTESIAN_POINT('Ctrl Pts',(-5.87058983200006,11.6,-8.80169450300002));
#283413=CARTESIAN_POINT('Ctrl Pts',(-5.86913185000006,15.2,-8.80028590300002));
#283414=CARTESIAN_POINT('Ctrl Pts',(-5.86913185000006,11.6,-8.80028590300002));
#283415=CARTESIAN_POINT('Ctrl Pts',(-5.86768017200006,15.2,-8.79888086200001));
#283416=CARTESIAN_POINT('Ctrl Pts',(-5.86768017200006,11.6,-8.79888086200001));
#283417=CARTESIAN_POINT('Ctrl Pts',(-5.86623479900005,15.2,-8.79747939600002));
#283418=CARTESIAN_POINT('Ctrl Pts',(-5.86623479900005,11.6,-8.79747939600002));
#283419=CARTESIAN_POINT('Ctrl Pts',(-5.86479573400006,15.2,-8.79608152700002));
#283420=CARTESIAN_POINT('Ctrl Pts',(-5.86479573400006,11.6,-8.79608152700002));
#283421=CARTESIAN_POINT('Ctrl Pts',(-5.86336298000006,15.2,-8.79468727200001));
#283422=CARTESIAN_POINT('Ctrl Pts',(-5.86336298000006,11.6,-8.79468727200001));
#283423=CARTESIAN_POINT('Ctrl Pts',(-5.86193653900006,15.2,-8.79329665000002));
#283424=CARTESIAN_POINT('Ctrl Pts',(-5.86193653900006,11.6,-8.79329665000002));
#283425=CARTESIAN_POINT('Ctrl Pts',(-5.86051641600006,15.2,-8.79190968000002));
#283426=CARTESIAN_POINT('Ctrl Pts',(-5.86051641600006,11.6,-8.79190968000002));
#283427=CARTESIAN_POINT('Ctrl Pts',(-5.85910261300006,15.2,-8.79052638100001));
#283428=CARTESIAN_POINT('Ctrl Pts',(-5.85910261300006,11.6,-8.79052638100001));
#283429=CARTESIAN_POINT('Ctrl Pts',(-5.85769513200006,15.2,-8.78914677200001));
#283430=CARTESIAN_POINT('Ctrl Pts',(-5.85769513200006,11.6,-8.78914677200001));
#283431=CARTESIAN_POINT('Ctrl Pts',(-5.85629397700006,15.2,-8.78777087300002));
#283432=CARTESIAN_POINT('Ctrl Pts',(-5.85629397700006,11.6,-8.78777087300002));
#283433=CARTESIAN_POINT('Ctrl Pts',(-5.85489915200006,15.2,-8.78639870300002));
#283434=CARTESIAN_POINT('Ctrl Pts',(-5.85489915200006,11.6,-8.78639870300002));
#283435=CARTESIAN_POINT('Ctrl Pts',(-5.85351065700006,15.2,-8.78503028000001));
#283436=CARTESIAN_POINT('Ctrl Pts',(-5.85351065700006,11.6,-8.78503028000001));
#283437=CARTESIAN_POINT('Ctrl Pts',(-5.85212849700006,15.2,-8.78366562400002));
#283438=CARTESIAN_POINT('Ctrl Pts',(-5.85212849700006,11.6,-8.78366562400002));
#283439=CARTESIAN_POINT('Ctrl Pts',(-5.85075267500006,15.2,-8.78230475600001));
#283440=CARTESIAN_POINT('Ctrl Pts',(-5.85075267500006,11.6,-8.78230475600001));
#283441=CARTESIAN_POINT('Ctrl Pts',(-5.84938319300006,15.2,-8.78094769400001));
#283442=CARTESIAN_POINT('Ctrl Pts',(-5.84938319300006,11.6,-8.78094769400001));
#283443=CARTESIAN_POINT('Ctrl Pts',(-5.84802005400006,15.2,-8.77959445700002));
#283444=CARTESIAN_POINT('Ctrl Pts',(-5.84802005400006,11.6,-8.77959445700002));
#283445=CARTESIAN_POINT('Ctrl Pts',(-5.84666326000006,15.2,-8.77824506500002));
#283446=CARTESIAN_POINT('Ctrl Pts',(-5.84666326000006,11.6,-8.77824506500002));
#283447=CARTESIAN_POINT('Ctrl Pts',(-5.84531281700006,15.2,-8.77689953800001));
#283448=CARTESIAN_POINT('Ctrl Pts',(-5.84531281700006,11.6,-8.77689953800001));
#283449=CARTESIAN_POINT('Ctrl Pts',(-5.84396872500006,15.2,-8.77555789600001));
#283450=CARTESIAN_POINT('Ctrl Pts',(-5.84396872500006,11.6,-8.77555789600001));
#283451=CARTESIAN_POINT('Ctrl Pts',(-5.84263098700006,15.2,-8.77422015900001));
#283452=CARTESIAN_POINT('Ctrl Pts',(-5.84263098700006,11.6,-8.77422015900001));
#283453=CARTESIAN_POINT('Ctrl Pts',(-5.84129960800006,15.2,-8.77288634600001));
#283454=CARTESIAN_POINT('Ctrl Pts',(-5.84129960800006,11.6,-8.77288634600001));
#283455=CARTESIAN_POINT('Ctrl Pts',(-5.83997459000006,15.2,-8.77155647700001));
#283456=CARTESIAN_POINT('Ctrl Pts',(-5.83997459000006,11.6,-8.77155647700001));
#283457=CARTESIAN_POINT('Ctrl Pts',(-5.83865593500006,15.2,-8.77023057400002));
#283458=CARTESIAN_POINT('Ctrl Pts',(-5.83865593500006,11.6,-8.77023057400002));
#283459=CARTESIAN_POINT('Ctrl Pts',(-5.83734364600006,15.2,-8.76890865500001));
#283460=CARTESIAN_POINT('Ctrl Pts',(-5.83734364600006,11.6,-8.76890865500001));
#283461=CARTESIAN_POINT('Ctrl Pts',(-5.83603772700005,15.2,-8.76759074100002));
#283462=CARTESIAN_POINT('Ctrl Pts',(-5.83603772700005,11.6,-8.76759074100002));
#283463=CARTESIAN_POINT('Ctrl Pts',(-5.83473817900006,15.2,-8.76627685200001));
#283464=CARTESIAN_POINT('Ctrl Pts',(-5.83473817900006,11.6,-8.76627685200001));
#283465=CARTESIAN_POINT('Ctrl Pts',(-5.83344500700006,15.2,-8.76496700800002));
#283466=CARTESIAN_POINT('Ctrl Pts',(-5.83344500700006,11.6,-8.76496700800002));
#283467=CARTESIAN_POINT('Ctrl Pts',(-5.83215821300006,15.2,-8.76366123100001));
#283468=CARTESIAN_POINT('Ctrl Pts',(-5.83215821300006,11.6,-8.76366123100001));
#283469=CARTESIAN_POINT('Ctrl Pts',(-5.83087780000006,15.2,-8.76235953900002));
#283470=CARTESIAN_POINT('Ctrl Pts',(-5.83087780000006,11.6,-8.76235953900002));
#283471=CARTESIAN_POINT('Ctrl Pts',(-5.82960377000005,15.2,-8.76106195500002));
#283472=CARTESIAN_POINT('Ctrl Pts',(-5.82960377000005,11.6,-8.76106195500002));
#283473=CARTESIAN_POINT('Ctrl Pts',(-5.82833612700006,15.2,-8.75976849900002));
#283474=CARTESIAN_POINT('Ctrl Pts',(-5.82833612700006,11.6,-8.75976849900002));
#283475=CARTESIAN_POINT('Ctrl Pts',(-5.82707487300006,15.2,-8.75847919000002));
#283476=CARTESIAN_POINT('Ctrl Pts',(-5.82707487300006,11.6,-8.75847919000002));
#283477=CARTESIAN_POINT('Ctrl Pts',(-5.82582001200006,15.2,-8.75719405100002));
#283478=CARTESIAN_POINT('Ctrl Pts',(-5.82582001200006,11.6,-8.75719405100002));
#283479=CARTESIAN_POINT('Ctrl Pts',(-5.82457154700006,15.2,-8.75591310200001));
#283480=CARTESIAN_POINT('Ctrl Pts',(-5.82457154700006,11.6,-8.75591310200001));
#283481=CARTESIAN_POINT('Ctrl Pts',(-5.82332948000006,15.2,-8.75463636300001));
#283482=CARTESIAN_POINT('Ctrl Pts',(-5.82332948000006,11.6,-8.75463636300001));
#283483=CARTESIAN_POINT('Ctrl Pts',(-5.82209381200006,15.2,-8.75336385700002));
#283484=CARTESIAN_POINT('Ctrl Pts',(-5.82209381200006,11.6,-8.75336385700002));
#283485=CARTESIAN_POINT('Ctrl Pts',(-5.82086454900006,15.2,-8.75209560300001));
#283486=CARTESIAN_POINT('Ctrl Pts',(-5.82086454900006,11.6,-8.75209560300001));
#283487=CARTESIAN_POINT('Ctrl Pts',(-5.81964169300006,15.2,-8.75083162500001));
#283488=CARTESIAN_POINT('Ctrl Pts',(-5.81964169300006,11.6,-8.75083162500001));
#283489=CARTESIAN_POINT('Ctrl Pts',(-5.81842524600006,15.2,-8.74957194100002));
#283490=CARTESIAN_POINT('Ctrl Pts',(-5.81842524600006,11.6,-8.74957194100002));
#283491=CARTESIAN_POINT('Ctrl Pts',(-5.81721521200006,15.2,-8.74831657400001));
#283492=CARTESIAN_POINT('Ctrl Pts',(-5.81721521200006,11.6,-8.74831657400001));
#283493=CARTESIAN_POINT('Ctrl Pts',(-5.81601159400006,15.2,-8.74706554600002));
#283494=CARTESIAN_POINT('Ctrl Pts',(-5.81601159400006,11.6,-8.74706554600002));
#283495=CARTESIAN_POINT('Ctrl Pts',(-5.81481439300005,15.2,-8.74581887800002));
#283496=CARTESIAN_POINT('Ctrl Pts',(-5.81481439300005,11.6,-8.74581887800002));
#283497=CARTESIAN_POINT('Ctrl Pts',(-5.81362361300005,15.2,-8.74457659100001));
#283498=CARTESIAN_POINT('Ctrl Pts',(-5.81362361300005,11.6,-8.74457659100001));
#283499=CARTESIAN_POINT('Ctrl Pts',(-5.81243925700006,15.2,-8.74333870700001));
#283500=CARTESIAN_POINT('Ctrl Pts',(-5.81243925700006,11.6,-8.74333870700001));
#283501=CARTESIAN_POINT('Ctrl Pts',(-5.81126132800006,15.2,-8.74210524800001));
#283502=CARTESIAN_POINT('Ctrl Pts',(-5.81126132800006,11.6,-8.74210524800001));
#283503=CARTESIAN_POINT('Ctrl Pts',(-5.81008982800006,15.2,-8.74087623600002));
#283504=CARTESIAN_POINT('Ctrl Pts',(-5.81008982800006,11.6,-8.74087623600002));
#283505=CARTESIAN_POINT('Ctrl Pts',(-5.80892476100006,15.2,-8.73965169300002));
#283506=CARTESIAN_POINT('Ctrl Pts',(-5.80892476100006,11.6,-8.73965169300002));
#283507=CARTESIAN_POINT('Ctrl Pts',(-5.80776612900006,15.2,-8.73843163900002));
#283508=CARTESIAN_POINT('Ctrl Pts',(-5.80776612900006,11.6,-8.73843163900002));
#283509=CARTESIAN_POINT('Ctrl Pts',(-5.80661393400006,15.2,-8.73721609800001));
#283510=CARTESIAN_POINT('Ctrl Pts',(-5.80661393400006,11.6,-8.73721609800001));
#283511=CARTESIAN_POINT('Ctrl Pts',(-5.80546818100006,15.2,-8.73600509300001));
#283512=CARTESIAN_POINT('Ctrl Pts',(-5.80546818100006,11.6,-8.73600509300001));
#283513=CARTESIAN_POINT('Ctrl Pts',(-5.80432887200006,15.2,-8.73479864500002));
#283514=CARTESIAN_POINT('Ctrl Pts',(-5.80432887200006,11.6,-8.73479864500002));
#283515=CARTESIAN_POINT('Ctrl Pts',(-5.80319600900006,15.2,-8.73359677600002));
#283516=CARTESIAN_POINT('Ctrl Pts',(-5.80319600900006,11.6,-8.73359677600002));
#283517=CARTESIAN_POINT('Ctrl Pts',(-5.80206959600006,15.2,-8.73239950900001));
#283518=CARTESIAN_POINT('Ctrl Pts',(-5.80206959600006,11.6,-8.73239950900001));
#283519=CARTESIAN_POINT('Ctrl Pts',(-5.80094963500006,15.2,-8.73120686600002));
#283520=CARTESIAN_POINT('Ctrl Pts',(-5.80094963500006,11.6,-8.73120686600002));
#283521=CARTESIAN_POINT('Ctrl Pts',(-5.79983612800006,15.2,-8.73001887100001));
#283522=CARTESIAN_POINT('Ctrl Pts',(-5.79983612800006,11.6,-8.73001887100001));
#283523=CARTESIAN_POINT('Ctrl Pts',(-5.79872908000006,15.2,-8.72883554600002));
#283524=CARTESIAN_POINT('Ctrl Pts',(-5.79872908000006,11.6,-8.72883554600002));
#283525=CARTESIAN_POINT('Ctrl Pts',(-5.79762849300006,15.2,-8.72765691300001));
#283526=CARTESIAN_POINT('Ctrl Pts',(-5.79762849300006,11.6,-8.72765691300001));
#283527=CARTESIAN_POINT('Ctrl Pts',(-5.79653437000006,15.2,-8.72648299600002));
#283528=CARTESIAN_POINT('Ctrl Pts',(-5.79653437000006,11.6,-8.72648299600002));
#283529=CARTESIAN_POINT('Ctrl Pts',(-5.79544671200006,15.2,-8.72531381700002));
#283530=CARTESIAN_POINT('Ctrl Pts',(-5.79544671200006,11.6,-8.72531381700002));
#283531=CARTESIAN_POINT('Ctrl Pts',(-5.79436552400006,15.2,-8.72414939900001));
#283532=CARTESIAN_POINT('Ctrl Pts',(-5.79436552400006,11.6,-8.72414939900001));
#283533=CARTESIAN_POINT('Ctrl Pts',(-5.79329080800006,15.2,-8.72298976600002));
#283534=CARTESIAN_POINT('Ctrl Pts',(-5.79329080800006,11.6,-8.72298976600002));
#283535=CARTESIAN_POINT('Ctrl Pts',(-5.79222256600006,15.2,-8.72183494100002));
#283536=CARTESIAN_POINT('Ctrl Pts',(-5.79222256600006,11.6,-8.72183494100002));
#283537=CARTESIAN_POINT('Ctrl Pts',(-5.79116080300006,15.2,-8.72068494800001));
#283538=CARTESIAN_POINT('Ctrl Pts',(-5.79116080300006,11.6,-8.72068494800001));
#283539=CARTESIAN_POINT('Ctrl Pts',(-5.79010551900006,15.2,-8.71953980900001));
#283540=CARTESIAN_POINT('Ctrl Pts',(-5.79010551900006,11.6,-8.71953980900001));
#283541=CARTESIAN_POINT('Ctrl Pts',(-5.78905671900006,15.2,-8.71839954800001));
#283542=CARTESIAN_POINT('Ctrl Pts',(-5.78905671900006,11.6,-8.71839954800001));
#283543=CARTESIAN_POINT('Ctrl Pts',(-5.78801440500006,15.2,-8.71726418900002));
#283544=CARTESIAN_POINT('Ctrl Pts',(-5.78801440500006,11.6,-8.71726418900002));
#283545=CARTESIAN_POINT('Ctrl Pts',(-5.78697858000006,15.2,-8.71613375700001));
#283546=CARTESIAN_POINT('Ctrl Pts',(-5.78697858000006,11.6,-8.71613375700001));
#283547=CARTESIAN_POINT('Ctrl Pts',(-5.78594924700006,15.2,-8.71500827300002));
#283548=CARTESIAN_POINT('Ctrl Pts',(-5.78594924700006,11.6,-8.71500827300002));
#283549=CARTESIAN_POINT('Ctrl Pts',(-5.78492640800006,15.2,-8.71388776300002));
#283550=CARTESIAN_POINT('Ctrl Pts',(-5.78492640800006,11.6,-8.71388776300002));
#283551=CARTESIAN_POINT('Ctrl Pts',(-5.78391006700006,15.2,-8.71277225000001));
#283552=CARTESIAN_POINT('Ctrl Pts',(-5.78391006700006,11.6,-8.71277225000001));
#283553=CARTESIAN_POINT('Ctrl Pts',(-5.78290022600005,15.2,-8.71166175800001));
#283554=CARTESIAN_POINT('Ctrl Pts',(-5.78290022600005,11.6,-8.71166175800001));
#283555=CARTESIAN_POINT('Ctrl Pts',(-5.78189688700006,15.2,-8.71055631200001));
#283556=CARTESIAN_POINT('Ctrl Pts',(-5.78189688700006,11.6,-8.71055631200001));
#283557=CARTESIAN_POINT('Ctrl Pts',(-5.78090005400006,15.2,-8.70945593700002));
#283558=CARTESIAN_POINT('Ctrl Pts',(-5.78090005400006,11.6,-8.70945593700002));
#283559=CARTESIAN_POINT('Ctrl Pts',(-5.77990973100006,15.2,-8.70836065500002));
#283560=CARTESIAN_POINT('Ctrl Pts',(-5.77990973100006,11.6,-8.70836065500002));
#283561=CARTESIAN_POINT('Ctrl Pts',(-5.77892591700006,15.2,-8.70727049300001));
#283562=CARTESIAN_POINT('Ctrl Pts',(-5.77892591700006,11.6,-8.70727049300001));
#283563=CARTESIAN_POINT('Ctrl Pts',(-5.77794861800006,15.2,-8.70618547500002));
#283564=CARTESIAN_POINT('Ctrl Pts',(-5.77794861800006,11.6,-8.70618547500002));
#283565=CARTESIAN_POINT('Ctrl Pts',(-5.77697783600006,15.2,-8.70510562400002));
#283566=CARTESIAN_POINT('Ctrl Pts',(-5.77697783600006,11.6,-8.70510562400002));
#283567=CARTESIAN_POINT('Ctrl Pts',(-5.77601357300006,15.2,-8.70403096700001));
#283568=CARTESIAN_POINT('Ctrl Pts',(-5.77601357300006,11.6,-8.70403096700001));
#283569=CARTESIAN_POINT('Ctrl Pts',(-5.77505583400006,15.2,-8.70296152800002));
#283570=CARTESIAN_POINT('Ctrl Pts',(-5.77505583400006,11.6,-8.70296152800002));
#283571=CARTESIAN_POINT('Ctrl Pts',(-5.77410461900006,15.2,-8.70189733200002));
#283572=CARTESIAN_POINT('Ctrl Pts',(-5.77410461900006,11.6,-8.70189733200002));
#283573=CARTESIAN_POINT('Ctrl Pts',(-5.77315993200005,15.2,-8.70083840400002));
#283574=CARTESIAN_POINT('Ctrl Pts',(-5.77315993200005,11.6,-8.70083840400002));
#283575=CARTESIAN_POINT('Ctrl Pts',(-5.77222177600006,15.2,-8.69978477000002));
#283576=CARTESIAN_POINT('Ctrl Pts',(-5.77222177600006,11.6,-8.69978477000002));
#283577=CARTESIAN_POINT('Ctrl Pts',(-5.77129015400006,15.2,-8.69873645500002));
#283578=CARTESIAN_POINT('Ctrl Pts',(-5.77129015400006,11.6,-8.69873645500002));
#283579=CARTESIAN_POINT('Ctrl Pts',(-5.77036506700006,15.2,-8.69769348400002));
#283580=CARTESIAN_POINT('Ctrl Pts',(-5.77036506700006,11.6,-8.69769348400002));
#283581=CARTESIAN_POINT('Ctrl Pts',(-5.76944652100006,15.2,-8.69665588300002));
#283582=CARTESIAN_POINT('Ctrl Pts',(-5.76944652100006,11.6,-8.69665588300002));
#283583=CARTESIAN_POINT('Ctrl Pts',(-5.76853451500006,15.2,-8.69562367700001));
#283584=CARTESIAN_POINT('Ctrl Pts',(-5.76853451500006,11.6,-8.69562367700001));
#283585=CARTESIAN_POINT('Ctrl Pts',(-5.76762905500006,15.2,-8.69459689400001));
#283586=CARTESIAN_POINT('Ctrl Pts',(-5.76762905500006,11.6,-8.69459689400001));
#283587=CARTESIAN_POINT('Ctrl Pts',(-5.76673014200006,15.2,-8.69357555700002));
#283588=CARTESIAN_POINT('Ctrl Pts',(-5.76673014200006,11.6,-8.69357555700002));
#283589=CARTESIAN_POINT('Ctrl Pts',(-5.76583777900006,15.2,-8.69255969400001));
#283590=CARTESIAN_POINT('Ctrl Pts',(-5.76583777900006,11.6,-8.69255969400001));
#283591=CARTESIAN_POINT('Ctrl Pts',(-5.76495197000006,15.2,-8.69154933000001));
#283592=CARTESIAN_POINT('Ctrl Pts',(-5.76495197000006,11.6,-8.69154933000001));
#283593=CARTESIAN_POINT('Ctrl Pts',(-5.76407271500006,15.2,-8.69054449200001));
#283594=CARTESIAN_POINT('Ctrl Pts',(-5.76407271500006,11.6,-8.69054449200001));
#283595=CARTESIAN_POINT('Ctrl Pts',(-5.76320002000006,15.2,-8.68954520600001));
#283596=CARTESIAN_POINT('Ctrl Pts',(-5.76320002000006,11.6,-8.68954520600001));
#283597=CARTESIAN_POINT('Ctrl Pts',(-5.76233388600006,15.2,-8.68855149800002));
#283598=CARTESIAN_POINT('Ctrl Pts',(-5.76233388600006,11.6,-8.68855149800002));
#283599=CARTESIAN_POINT('Ctrl Pts',(-5.76147431600006,15.2,-8.68756339600001));
#283600=CARTESIAN_POINT('Ctrl Pts',(-5.76147431600006,11.6,-8.68756339600001));
#283601=CARTESIAN_POINT('Ctrl Pts',(-5.76062131200006,15.2,-8.68658092600001));
#283602=CARTESIAN_POINT('Ctrl Pts',(-5.76062131200006,11.6,-8.68658092600001));
#283603=CARTESIAN_POINT('Ctrl Pts',(-5.75977487800006,15.2,-8.68560411500002));
#283604=CARTESIAN_POINT('Ctrl Pts',(-5.75977487800006,11.6,-8.68560411500002));
#283605=CARTESIAN_POINT('Ctrl Pts',(-5.75893501600006,15.2,-8.68463298900001));
#283606=CARTESIAN_POINT('Ctrl Pts',(-5.75893501600006,11.6,-8.68463298900001));
#283607=CARTESIAN_POINT('Ctrl Pts',(-5.75810173000006,15.2,-8.68366757600001));
#283608=CARTESIAN_POINT('Ctrl Pts',(-5.75810173000006,11.6,-8.68366757600001));
#283609=CARTESIAN_POINT('Ctrl Pts',(-5.75727502100006,15.2,-8.68270790200001));
#283610=CARTESIAN_POINT('Ctrl Pts',(-5.75727502100006,11.6,-8.68270790200001));
#283611=CARTESIAN_POINT('Ctrl Pts',(-5.75645489300006,15.2,-8.68175399800002));
#283612=CARTESIAN_POINT('Ctrl Pts',(-5.75645489300006,11.6,-8.68175399800002));
#283613=CARTESIAN_POINT('Ctrl Pts',(-5.75564134700006,15.2,-8.68080588500002));
#283614=CARTESIAN_POINT('Ctrl Pts',(-5.75564134700006,11.6,-8.68080588500002));
#283615=CARTESIAN_POINT('Ctrl Pts',(-5.75483438800005,15.2,-8.67986359700001));
#283616=CARTESIAN_POINT('Ctrl Pts',(-5.75483438800005,11.6,-8.67986359700001));
#283617=CARTESIAN_POINT('Ctrl Pts',(-5.75403401900005,15.2,-8.67892715900001));
#283618=CARTESIAN_POINT('Ctrl Pts',(-5.75403401900005,11.6,-8.67892715900001));
#283619=CARTESIAN_POINT('Ctrl Pts',(-5.75324024000006,15.2,-8.67799659800001));
#283620=CARTESIAN_POINT('Ctrl Pts',(-5.75324024000006,11.6,-8.67799659800001));
#283621=CARTESIAN_POINT('Ctrl Pts',(-5.75245305600006,15.2,-8.67707194200002));
#283622=CARTESIAN_POINT('Ctrl Pts',(-5.75245305600006,11.6,-8.67707194200002));
#283623=CARTESIAN_POINT('Ctrl Pts',(-5.75167246900006,15.2,-8.67615322100002));
#283624=CARTESIAN_POINT('Ctrl Pts',(-5.75167246900006,11.6,-8.67615322100002));
#283625=CARTESIAN_POINT('Ctrl Pts',(-5.75089848100006,15.2,-8.67524046100002));
#283626=CARTESIAN_POINT('Ctrl Pts',(-5.75089848100006,11.6,-8.67524046100002));
#283627=CARTESIAN_POINT('Ctrl Pts',(-5.75013109600006,15.2,-8.67433369300001));
#283628=CARTESIAN_POINT('Ctrl Pts',(-5.75013109600006,11.6,-8.67433369300001));
#283629=CARTESIAN_POINT('Ctrl Pts',(-5.74937031600006,15.2,-8.67343294300002));
#283630=CARTESIAN_POINT('Ctrl Pts',(-5.74937031600006,11.6,-8.67343294300002));
#283631=CARTESIAN_POINT('Ctrl Pts',(-5.74861614500006,15.2,-8.67253824000001));
#283632=CARTESIAN_POINT('Ctrl Pts',(-5.74861614500006,11.6,-8.67253824000001));
#283633=CARTESIAN_POINT('Ctrl Pts',(-5.74786858400006,15.2,-8.67164961300002));
#283634=CARTESIAN_POINT('Ctrl Pts',(-5.74786858400006,11.6,-8.67164961300002));
#283635=CARTESIAN_POINT('Ctrl Pts',(-5.74712763600006,15.2,-8.67076709200001));
#283636=CARTESIAN_POINT('Ctrl Pts',(-5.74712763600006,11.6,-8.67076709200001));
#283637=CARTESIAN_POINT('Ctrl Pts',(-5.74639330500006,15.2,-8.66989070400002));
#283638=CARTESIAN_POINT('Ctrl Pts',(-5.74639330500006,11.6,-8.66989070400002));
#283639=CARTESIAN_POINT('Ctrl Pts',(-5.74566559300006,15.2,-8.66902047900002));
#283640=CARTESIAN_POINT('Ctrl Pts',(-5.74566559300006,11.6,-8.66902047900002));
#283641=CARTESIAN_POINT('Ctrl Pts',(-5.74494450300006,15.2,-8.66815644700001));
#283642=CARTESIAN_POINT('Ctrl Pts',(-5.74494450300006,11.6,-8.66815644700001));
#283643=CARTESIAN_POINT('Ctrl Pts',(-5.74423003600006,15.2,-8.66729863600002));
#283644=CARTESIAN_POINT('Ctrl Pts',(-5.74423003600006,11.6,-8.66729863600002));
#283645=CARTESIAN_POINT('Ctrl Pts',(-5.74352219700006,15.2,-8.66644707700001));
#283646=CARTESIAN_POINT('Ctrl Pts',(-5.74352219700006,11.6,-8.66644707700001));
#283647=CARTESIAN_POINT('Ctrl Pts',(-5.74282098800006,15.2,-8.66560180000001));
#283648=CARTESIAN_POINT('Ctrl Pts',(-5.74282098800006,11.6,-8.66560180000001));
#283649=CARTESIAN_POINT('Ctrl Pts',(-5.74212641100006,15.2,-8.66476283200001));
#283650=CARTESIAN_POINT('Ctrl Pts',(-5.74212641100006,11.6,-8.66476283200001));
#283651=CARTESIAN_POINT('Ctrl Pts',(-5.74143847000006,15.2,-8.66393020500002));
#283652=CARTESIAN_POINT('Ctrl Pts',(-5.74143847000006,11.6,-8.66393020500002));
#283653=CARTESIAN_POINT('Ctrl Pts',(-5.74075716700006,15.2,-8.66310395100001));
#283654=CARTESIAN_POINT('Ctrl Pts',(-5.74075716700006,11.6,-8.66310395100001));
#283655=CARTESIAN_POINT('Ctrl Pts',(-5.74008250400006,15.2,-8.66228409600001));
#283656=CARTESIAN_POINT('Ctrl Pts',(-5.74008250400006,11.6,-8.66228409600001));
#283657=CARTESIAN_POINT('Ctrl Pts',(-5.73941448500006,15.2,-8.66147067400002));
#283658=CARTESIAN_POINT('Ctrl Pts',(-5.73941448500006,11.6,-8.66147067400002));
#283659=CARTESIAN_POINT('Ctrl Pts',(-5.73875311300006,15.2,-8.66066371300001));
#283660=CARTESIAN_POINT('Ctrl Pts',(-5.73875311300006,11.6,-8.66066371300001));
#283661=CARTESIAN_POINT('Ctrl Pts',(-5.73809838900006,15.2,-8.65986324600001));
#283662=CARTESIAN_POINT('Ctrl Pts',(-5.73809838900006,11.6,-8.65986324600001));
#283663=CARTESIAN_POINT('Ctrl Pts',(-5.73745031600006,15.2,-8.65906930200002));
#283664=CARTESIAN_POINT('Ctrl Pts',(-5.73745031600006,11.6,-8.65906930200002));
#283665=CARTESIAN_POINT('Ctrl Pts',(-5.73680889900006,15.2,-8.65828191300002));
#283666=CARTESIAN_POINT('Ctrl Pts',(-5.73680889900006,11.6,-8.65828191300002));
#283667=CARTESIAN_POINT('Ctrl Pts',(-5.73617413900006,15.2,-8.65750111000001));
#283668=CARTESIAN_POINT('Ctrl Pts',(-5.73617413900006,11.6,-8.65750111000001));
#283669=CARTESIAN_POINT('Ctrl Pts',(-5.73554603700006,15.2,-8.65672692500001));
#283670=CARTESIAN_POINT('Ctrl Pts',(-5.73554603700006,11.6,-8.65672692500001));
#283671=CARTESIAN_POINT('Ctrl Pts',(-5.73492459900006,15.2,-8.65595938700002));
#283672=CARTESIAN_POINT('Ctrl Pts',(-5.73492459900006,11.6,-8.65595938700002));
#283673=CARTESIAN_POINT('Ctrl Pts',(-5.73430982600006,15.2,-8.65519853100002));
#283674=CARTESIAN_POINT('Ctrl Pts',(-5.73430982600006,11.6,-8.65519853100002));
#283675=CARTESIAN_POINT('Ctrl Pts',(-5.73370172100006,15.2,-8.65444438600001));
#283676=CARTESIAN_POINT('Ctrl Pts',(-5.73370172100006,11.6,-8.65444438600001));
#283677=CARTESIAN_POINT('Ctrl Pts',(-5.73310028700006,15.2,-8.65369698500002));
#283678=CARTESIAN_POINT('Ctrl Pts',(-5.73310028700006,11.6,-8.65369698500002));
#283679=CARTESIAN_POINT('Ctrl Pts',(-5.73250552600006,15.2,-8.65295636100001));
#283680=CARTESIAN_POINT('Ctrl Pts',(-5.73250552600006,11.6,-8.65295636100001));
#283681=CARTESIAN_POINT('Ctrl Pts',(-5.73191744100006,15.2,-8.65222254500001));
#283682=CARTESIAN_POINT('Ctrl Pts',(-5.73191744100006,11.6,-8.65222254500001));
#283683=CARTESIAN_POINT('Ctrl Pts',(-5.73133603500006,15.2,-8.65149557000001));
#283684=CARTESIAN_POINT('Ctrl Pts',(-5.73133603500006,11.6,-8.65149557000001));
#283685=CARTESIAN_POINT('Ctrl Pts',(-5.73076462000006,15.2,-8.65077961500001));
#283686=CARTESIAN_POINT('Ctrl Pts',(-5.73076462000006,11.6,-8.65077961500001));
#283687=CARTESIAN_POINT('Ctrl Pts',(-5.73031342200006,15.2,-8.65021312700001));
#283688=CARTESIAN_POINT('Ctrl Pts',(-5.73031342200006,11.6,-8.65021312700001));
#283689=CARTESIAN_POINT('Ctrl Pts',(-5.72997879300006,15.2,-8.64979235000002));
#283690=CARTESIAN_POINT('Ctrl Pts',(-5.72997879300006,11.6,-8.64979235000002));
#283691=CARTESIAN_POINT('Ctrl Pts',(-5.72975808700006,15.2,-8.64951454400002));
#283692=CARTESIAN_POINT('Ctrl Pts',(-5.72975808700006,11.6,-8.64951454400002));
#283693=CARTESIAN_POINT('Ctrl Pts',(-5.72964966100006,15.2,-8.64937799900002));
#283694=CARTESIAN_POINT('Ctrl Pts',(-5.72964966100006,11.6,-8.64937799900002));
#283695=CARTESIAN_POINT('',(-5.72964966108803,12.2,-8.64937799846615));
#283696=CARTESIAN_POINT('',(-5.72964966108803,15.2,-8.64937799846615));
#283697=CARTESIAN_POINT('',(-5.72964966100006,12.2,-8.64937799800002));
#283698=CARTESIAN_POINT('Ctrl Pts',(-6.67046385600006,12.2,-9.36775917400002));
#283699=CARTESIAN_POINT('Ctrl Pts',(-6.66979226100006,12.2,-9.36739373000002));
#283700=CARTESIAN_POINT('Ctrl Pts',(-6.66844959800006,12.2,-9.36666279600002));
#283701=CARTESIAN_POINT('Ctrl Pts',(-6.66643717700006,12.2,-9.36556627000002));
#283702=CARTESIAN_POINT('Ctrl Pts',(-6.66375709900006,12.2,-9.36410398400002));
#283703=CARTESIAN_POINT('Ctrl Pts',(-6.66041225200006,12.2,-9.36227570600002));
#283704=CARTESIAN_POINT('Ctrl Pts',(-6.65707265500005,12.2,-9.36044701000002));
#283705=CARTESIAN_POINT('Ctrl Pts',(-6.65373831000006,12.2,-9.35861789600001));
#283706=CARTESIAN_POINT('Ctrl Pts',(-6.65040921900006,12.2,-9.35678837000001));
#283707=CARTESIAN_POINT('Ctrl Pts',(-6.64708538300006,12.2,-9.35495843700001));
#283708=CARTESIAN_POINT('Ctrl Pts',(-6.64376680700006,12.2,-9.35312810300001));
#283709=CARTESIAN_POINT('Ctrl Pts',(-6.64045349300006,12.2,-9.35129737900001));
#283710=CARTESIAN_POINT('Ctrl Pts',(-6.63714544700006,12.2,-9.34946627300001));
#283711=CARTESIAN_POINT('Ctrl Pts',(-6.63384267100006,12.2,-9.34763479700001));
#283712=CARTESIAN_POINT('Ctrl Pts',(-6.63054517000006,12.2,-9.34580296000001));
#283713=CARTESIAN_POINT('Ctrl Pts',(-6.62725294900006,12.2,-9.34397077300002));
#283714=CARTESIAN_POINT('Ctrl Pts',(-6.62396601100006,12.2,-9.34213824300001));
#283715=CARTESIAN_POINT('Ctrl Pts',(-6.62068436000006,12.2,-9.34030538000002));
#283716=CARTESIAN_POINT('Ctrl Pts',(-6.61740799800006,12.2,-9.33847218900001));
#283717=CARTESIAN_POINT('Ctrl Pts',(-6.61413692800005,12.2,-9.33663868000002));
#283718=CARTESIAN_POINT('Ctrl Pts',(-6.61087115500006,12.2,-9.33480485900001));
#283719=CARTESIAN_POINT('Ctrl Pts',(-6.60761068100006,12.2,-9.33297073500002));
#283720=CARTESIAN_POINT('Ctrl Pts',(-6.60435550800006,12.2,-9.33113631500002));
#283721=CARTESIAN_POINT('Ctrl Pts',(-6.60110564300005,12.2,-9.32930161000002));
#283722=CARTESIAN_POINT('Ctrl Pts',(-6.59786108600006,12.2,-9.32746662500002));
#283723=CARTESIAN_POINT('Ctrl Pts',(-6.59462184300006,12.2,-9.32563137200002));
#283724=CARTESIAN_POINT('Ctrl Pts',(-6.59138791700006,12.2,-9.32379585900001));
#283725=CARTESIAN_POINT('Ctrl Pts',(-6.58815931000006,12.2,-9.32196009500002));
#283726=CARTESIAN_POINT('Ctrl Pts',(-6.58493602700006,12.2,-9.32012408600002));
#283727=CARTESIAN_POINT('Ctrl Pts',(-6.58171807300006,12.2,-9.31828784500001));
#283728=CARTESIAN_POINT('Ctrl Pts',(-6.57850544800006,12.2,-9.31645137700002));
#283729=CARTESIAN_POINT('Ctrl Pts',(-6.57529815700006,12.2,-9.31461469100002));
#283730=CARTESIAN_POINT('Ctrl Pts',(-6.57209620400006,12.2,-9.31277779500002));
#283731=CARTESIAN_POINT('Ctrl Pts',(-6.56889959100006,12.2,-9.31094070000002));
#283732=CARTESIAN_POINT('Ctrl Pts',(-6.56570832300006,12.2,-9.30910341200001));
#283733=CARTESIAN_POINT('Ctrl Pts',(-6.56252240200006,12.2,-9.30726594200002));
#283734=CARTESIAN_POINT('Ctrl Pts',(-6.55934183200006,12.2,-9.30542829500002));
#283735=CARTESIAN_POINT('Ctrl Pts',(-6.55616661700006,12.2,-9.30359048400001));
#283736=CARTESIAN_POINT('Ctrl Pts',(-6.55299676000006,12.2,-9.30175251500001));
#283737=CARTESIAN_POINT('Ctrl Pts',(-6.54983226500006,12.2,-9.29991439900002));
#283738=CARTESIAN_POINT('Ctrl Pts',(-6.54667313400005,12.2,-9.29807614200002));
#283739=CARTESIAN_POINT('Ctrl Pts',(-6.54351937200006,12.2,-9.29623775500002));
#283740=CARTESIAN_POINT('Ctrl Pts',(-6.54037098100006,12.2,-9.29439924500001));
#283741=CARTESIAN_POINT('Ctrl Pts',(-6.53722796600006,12.2,-9.29256062200002));
#283742=CARTESIAN_POINT('Ctrl Pts',(-6.53409033000006,12.2,-9.29072189400001));
#283743=CARTESIAN_POINT('Ctrl Pts',(-6.53095807500006,12.2,-9.28888307000001));
#283744=CARTESIAN_POINT('Ctrl Pts',(-6.52783120600006,12.2,-9.28704416000001));
#283745=CARTESIAN_POINT('Ctrl Pts',(-6.52470972700006,12.2,-9.28520517200001));
#283746=CARTESIAN_POINT('Ctrl Pts',(-6.52159363900005,12.2,-9.28336611300002));
#283747=CARTESIAN_POINT('Ctrl Pts',(-6.51848294800006,12.2,-9.28152699600002));
#283748=CARTESIAN_POINT('Ctrl Pts',(-6.51537765500006,12.2,-9.27968782700002));
#283749=CARTESIAN_POINT('Ctrl Pts',(-6.51227776500006,12.2,-9.27784861500001));
#283750=CARTESIAN_POINT('Ctrl Pts',(-6.50918328200006,12.2,-9.27600936900001));
#283751=CARTESIAN_POINT('Ctrl Pts',(-6.50609420700006,12.2,-9.27417010000001));
#283752=CARTESIAN_POINT('Ctrl Pts',(-6.50301054600006,12.2,-9.27233081400002));
#283753=CARTESIAN_POINT('Ctrl Pts',(-6.49993230100006,12.2,-9.27049152200001));
#283754=CARTESIAN_POINT('Ctrl Pts',(-6.49685947500006,12.2,-9.26865223300002));
#283755=CARTESIAN_POINT('Ctrl Pts',(-6.49379207300006,12.2,-9.26681295500002));
#283756=CARTESIAN_POINT('Ctrl Pts',(-6.49073009700006,12.2,-9.26497369800002));
#283757=CARTESIAN_POINT('Ctrl Pts',(-6.48767355200006,12.2,-9.26313447100001));
#283758=CARTESIAN_POINT('Ctrl Pts',(-6.48462244000005,12.2,-9.26129528200001));
#283759=CARTESIAN_POINT('Ctrl Pts',(-6.48157676400006,12.2,-9.25945614200002));
#283760=CARTESIAN_POINT('Ctrl Pts',(-6.47853652900006,12.2,-9.25761705800002));
#283761=CARTESIAN_POINT('Ctrl Pts',(-6.47550173800005,12.2,-9.25577804100002));
#283762=CARTESIAN_POINT('Ctrl Pts',(-6.47247239300006,12.2,-9.25393910000002));
#283763=CARTESIAN_POINT('Ctrl Pts',(-6.46944849900006,12.2,-9.25210024200002));
#283764=CARTESIAN_POINT('Ctrl Pts',(-6.46643005900006,12.2,-9.25026147900001));
#283765=CARTESIAN_POINT('Ctrl Pts',(-6.46341707600006,12.2,-9.24842281800002));
#283766=CARTESIAN_POINT('Ctrl Pts',(-6.46040955400006,12.2,-9.24658427100002));
#283767=CARTESIAN_POINT('Ctrl Pts',(-6.45740749600006,12.2,-9.24474584400001));
#283768=CARTESIAN_POINT('Ctrl Pts',(-6.45441090500006,12.2,-9.24290754900002));
#283769=CARTESIAN_POINT('Ctrl Pts',(-6.45141978500006,12.2,-9.24106939400002));
#283770=CARTESIAN_POINT('Ctrl Pts',(-6.44843413900006,12.2,-9.23923138800001));
#283771=CARTESIAN_POINT('Ctrl Pts',(-6.44545397200006,12.2,-9.23739354200002));
#283772=CARTESIAN_POINT('Ctrl Pts',(-6.44247928500006,12.2,-9.23555586400001));
#283773=CARTESIAN_POINT('Ctrl Pts',(-6.43951008200006,12.2,-9.23371836400002));
#283774=CARTESIAN_POINT('Ctrl Pts',(-6.43654636800005,12.2,-9.23188105000002));
#283775=CARTESIAN_POINT('Ctrl Pts',(-6.43358814400006,12.2,-9.23004393300002));
#283776=CARTESIAN_POINT('Ctrl Pts',(-6.43063541500006,12.2,-9.22820702200001));
#283777=CARTESIAN_POINT('Ctrl Pts',(-6.42768818400006,12.2,-9.22637032800001));
#283778=CARTESIAN_POINT('Ctrl Pts',(-6.42474645500006,12.2,-9.22453385700001));
#283779=CARTESIAN_POINT('Ctrl Pts',(-6.42181023000005,12.2,-9.22269762200001));
#283780=CARTESIAN_POINT('Ctrl Pts',(-6.41887951300006,12.2,-9.22086163100002));
#283781=CARTESIAN_POINT('Ctrl Pts',(-6.41595430900006,12.2,-9.21902589200002));
#283782=CARTESIAN_POINT('Ctrl Pts',(-6.41303461900006,12.2,-9.21719041800002));
#283783=CARTESIAN_POINT('Ctrl Pts',(-6.41012044700005,12.2,-9.21535521600001));
#283784=CARTESIAN_POINT('Ctrl Pts',(-6.40721179700006,12.2,-9.21352029700002));
#283785=CARTESIAN_POINT('Ctrl Pts',(-6.40430867200006,12.2,-9.21168566900001));
#283786=CARTESIAN_POINT('Ctrl Pts',(-6.40141107500006,12.2,-9.20985134500001));
#283787=CARTESIAN_POINT('Ctrl Pts',(-6.39851901000006,12.2,-9.20801733000001));
#283788=CARTESIAN_POINT('Ctrl Pts',(-6.39563248000006,12.2,-9.20618363800001));
#283789=CARTESIAN_POINT('Ctrl Pts',(-6.39275149000006,12.2,-9.20435027600002));
#283790=CARTESIAN_POINT('Ctrl Pts',(-6.38987604000006,12.2,-9.20251725400002));
#283791=CARTESIAN_POINT('Ctrl Pts',(-6.38700613600006,12.2,-9.20068458400002));
#283792=CARTESIAN_POINT('Ctrl Pts',(-6.38414178100006,12.2,-9.19885227300002));
#283793=CARTESIAN_POINT('Ctrl Pts',(-6.38128297700006,12.2,-9.19702033200002));
#283794=CARTESIAN_POINT('Ctrl Pts',(-6.37842973000006,12.2,-9.19518877200002));
#283795=CARTESIAN_POINT('Ctrl Pts',(-6.37558204100006,12.2,-9.19335760100001));
#283796=CARTESIAN_POINT('Ctrl Pts',(-6.37273991300006,12.2,-9.19152682900001));
#283797=CARTESIAN_POINT('Ctrl Pts',(-6.36990335200006,12.2,-9.18969646800001));
#283798=CARTESIAN_POINT('Ctrl Pts',(-6.36707236000006,12.2,-9.18786652500001));
#283799=CARTESIAN_POINT('Ctrl Pts',(-6.36424693800006,12.2,-9.18603701200002));
#283800=CARTESIAN_POINT('Ctrl Pts',(-6.36142709400006,12.2,-9.18420793900001));
#283801=CARTESIAN_POINT('Ctrl Pts',(-6.35861282700006,12.2,-9.18237931400002));
#283802=CARTESIAN_POINT('Ctrl Pts',(-6.35580414300006,12.2,-9.18055114900002));
#283803=CARTESIAN_POINT('Ctrl Pts',(-6.35300104500006,12.2,-9.17872345400001));
#283804=CARTESIAN_POINT('Ctrl Pts',(-6.35020353500006,12.2,-9.17689623700002));
#283805=CARTESIAN_POINT('Ctrl Pts',(-6.34741161800005,12.2,-9.17506951100002));
#283806=CARTESIAN_POINT('Ctrl Pts',(-6.34462529700006,12.2,-9.17324328400002));
#283807=CARTESIAN_POINT('Ctrl Pts',(-6.34184457400006,12.2,-9.17141756700002));
#283808=CARTESIAN_POINT('Ctrl Pts',(-6.33906945400006,12.2,-9.16959237000002));
#283809=CARTESIAN_POINT('Ctrl Pts',(-6.33629993900006,12.2,-9.16776770200002));
#283810=CARTESIAN_POINT('Ctrl Pts',(-6.33353603400006,12.2,-9.16594357600001));
#283811=CARTESIAN_POINT('Ctrl Pts',(-6.33077774100006,12.2,-9.16411999900001));
#283812=CARTESIAN_POINT('Ctrl Pts',(-6.32802506300005,12.2,-9.16229698300001));
#283813=CARTESIAN_POINT('Ctrl Pts',(-6.32527800500006,12.2,-9.16047453800001));
#283814=CARTESIAN_POINT('Ctrl Pts',(-6.32253656800006,12.2,-9.15865267500001));
#283815=CARTESIAN_POINT('Ctrl Pts',(-6.31980075800006,12.2,-9.15683140300001));
#283816=CARTESIAN_POINT('Ctrl Pts',(-6.31707057700006,12.2,-9.15501073400002));
#283817=CARTESIAN_POINT('Ctrl Pts',(-6.31434602800006,12.2,-9.15319067500001));
#283818=CARTESIAN_POINT('Ctrl Pts',(-6.31162711400005,12.2,-9.15137124000001));
#283819=CARTESIAN_POINT('Ctrl Pts',(-6.30891384000006,12.2,-9.14955243900001));
#283820=CARTESIAN_POINT('Ctrl Pts',(-6.30620620800006,12.2,-9.14773428000002));
#283821=CARTESIAN_POINT('Ctrl Pts',(-6.30350422100006,12.2,-9.14591677500002));
#283822=CARTESIAN_POINT('Ctrl Pts',(-6.30080788400006,12.2,-9.14409993500002));
#283823=CARTESIAN_POINT('Ctrl Pts',(-6.29811719900006,12.2,-9.14228377000001));
#283824=CARTESIAN_POINT('Ctrl Pts',(-6.29543217000006,12.2,-9.14046829000002));
#283825=CARTESIAN_POINT('Ctrl Pts',(-6.29275279900006,12.2,-9.13865350600001));
#283826=CARTESIAN_POINT('Ctrl Pts',(-6.29007909100006,12.2,-9.13683942900001));
#283827=CARTESIAN_POINT('Ctrl Pts',(-6.28741104800006,12.2,-9.13502606900002));
#283828=CARTESIAN_POINT('Ctrl Pts',(-6.28474867400006,12.2,-9.13321343700002));
#283829=CARTESIAN_POINT('Ctrl Pts',(-6.28209197200006,12.2,-9.13140154300002));
#283830=CARTESIAN_POINT('Ctrl Pts',(-6.27944094700006,12.2,-9.12959039800001));
#283831=CARTESIAN_POINT('Ctrl Pts',(-6.27679559900006,12.2,-9.12778001300002));
#283832=CARTESIAN_POINT('Ctrl Pts',(-6.27415593500006,12.2,-9.12597039800002));
#283833=CARTESIAN_POINT('Ctrl Pts',(-6.27152195600006,12.2,-9.12416156500001));
#283834=CARTESIAN_POINT('Ctrl Pts',(-6.26889366400006,12.2,-9.12235352300002));
#283835=CARTESIAN_POINT('Ctrl Pts',(-6.26627106600006,12.2,-9.12054628500002));
#283836=CARTESIAN_POINT('Ctrl Pts',(-6.26365416200006,12.2,-9.11873986000002));
#283837=CARTESIAN_POINT('Ctrl Pts',(-6.26104295800006,12.2,-9.11693426000001));
#283838=CARTESIAN_POINT('Ctrl Pts',(-6.25843745500006,12.2,-9.11512949500001));
#283839=CARTESIAN_POINT('Ctrl Pts',(-6.25583765700005,12.2,-9.11332557600002));
#283840=CARTESIAN_POINT('Ctrl Pts',(-6.25324356800006,12.2,-9.11152251400001));
#283841=CARTESIAN_POINT('Ctrl Pts',(-6.25065519100006,12.2,-9.10972032100002));
#283842=CARTESIAN_POINT('Ctrl Pts',(-6.24807252900006,12.2,-9.10791900700002));
#283843=CARTESIAN_POINT('Ctrl Pts',(-6.24549558500005,12.2,-9.10611858200001));
#283844=CARTESIAN_POINT('Ctrl Pts',(-6.24292436400006,12.2,-9.10431905900002));
#283845=CARTESIAN_POINT('Ctrl Pts',(-6.24035886600006,12.2,-9.10252044800002));
#283846=CARTESIAN_POINT('Ctrl Pts',(-6.23779909800006,12.2,-9.10072276100001));
#283847=CARTESIAN_POINT('Ctrl Pts',(-6.23524506100006,12.2,-9.09892600700001));
#283848=CARTESIAN_POINT('Ctrl Pts',(-6.23269675900006,12.2,-9.09713019900002));
#283849=CARTESIAN_POINT('Ctrl Pts',(-6.23015419600006,12.2,-9.09533534700002));
#283850=CARTESIAN_POINT('Ctrl Pts',(-6.22761737300006,12.2,-9.09354146400002));
#283851=CARTESIAN_POINT('Ctrl Pts',(-6.22508629500006,12.2,-9.09174855900002));
#283852=CARTESIAN_POINT('Ctrl Pts',(-6.22256096500006,12.2,-9.08995664500001));
#283853=CARTESIAN_POINT('Ctrl Pts',(-6.22004138600006,12.2,-9.08816573200001));
#283854=CARTESIAN_POINT('Ctrl Pts',(-6.21752756200006,12.2,-9.08637583200001));
#283855=CARTESIAN_POINT('Ctrl Pts',(-6.21501949600006,12.2,-9.08458695700002));
#283856=CARTESIAN_POINT('Ctrl Pts',(-6.21251719100006,12.2,-9.08279911600001));
#283857=CARTESIAN_POINT('Ctrl Pts',(-6.21002065000006,12.2,-9.08101232300002));
#283858=CARTESIAN_POINT('Ctrl Pts',(-6.20752987700006,12.2,-9.07922658700001));
#283859=CARTESIAN_POINT('Ctrl Pts',(-6.20504487400006,12.2,-9.07744192200001));
#283860=CARTESIAN_POINT('Ctrl Pts',(-6.20256564600006,12.2,-9.07565833800002));
#283861=CARTESIAN_POINT('Ctrl Pts',(-6.20009219500006,12.2,-9.07387584600002));
#283862=CARTESIAN_POINT('Ctrl Pts',(-6.19762452500006,12.2,-9.07209445800002));
#283863=CARTESIAN_POINT('Ctrl Pts',(-6.19516263900006,12.2,-9.07031418600001));
#283864=CARTESIAN_POINT('Ctrl Pts',(-6.19270653900006,12.2,-9.06853504200001));
#283865=CARTESIAN_POINT('Ctrl Pts',(-6.19025623000006,12.2,-9.06675703600002));
#283866=CARTESIAN_POINT('Ctrl Pts',(-6.18781171500006,12.2,-9.06498018100002));
#283867=CARTESIAN_POINT('Ctrl Pts',(-6.18537299700006,12.2,-9.06320448700002));
#283868=CARTESIAN_POINT('Ctrl Pts',(-6.18294008000006,12.2,-9.06142996800002));
#283869=CARTESIAN_POINT('Ctrl Pts',(-6.18051296500005,12.2,-9.05965663400002));
#283870=CARTESIAN_POINT('Ctrl Pts',(-6.17809165700006,12.2,-9.05788449800001));
#283871=CARTESIAN_POINT('Ctrl Pts',(-6.17567615900006,12.2,-9.05611357000002));
#283872=CARTESIAN_POINT('Ctrl Pts',(-6.17326647500006,12.2,-9.05434386300002));
#283873=CARTESIAN_POINT('Ctrl Pts',(-6.17086260700006,12.2,-9.05257538800001));
#283874=CARTESIAN_POINT('Ctrl Pts',(-6.16846455700006,12.2,-9.05080815900002));
#283875=CARTESIAN_POINT('Ctrl Pts',(-6.16607233200006,12.2,-9.04904218600001));
#283876=CARTESIAN_POINT('Ctrl Pts',(-6.16368593200006,12.2,-9.04727748100001));
#283877=CARTESIAN_POINT('Ctrl Pts',(-6.16130536200005,12.2,-9.04551405600002));
#283878=CARTESIAN_POINT('Ctrl Pts',(-6.15893062400006,12.2,-9.04375192400002));
#283879=CARTESIAN_POINT('Ctrl Pts',(-6.15656172200006,12.2,-9.04199109600002));
#283880=CARTESIAN_POINT('Ctrl Pts',(-6.15419866000006,12.2,-9.04023158300001));
#283881=CARTESIAN_POINT('Ctrl Pts',(-6.15184143900006,12.2,-9.03847340000001));
#283882=CARTESIAN_POINT('Ctrl Pts',(-6.14949006400006,12.2,-9.03671655700002));
#283883=CARTESIAN_POINT('Ctrl Pts',(-6.14714453800006,12.2,-9.03496106700001));
#283884=CARTESIAN_POINT('Ctrl Pts',(-6.14480486400006,12.2,-9.03320694000002));
#283885=CARTESIAN_POINT('Ctrl Pts',(-6.14247104500006,12.2,-9.03145419100002));
#283886=CARTESIAN_POINT('Ctrl Pts',(-6.14014308400006,12.2,-9.02970283200002));
#283887=CARTESIAN_POINT('Ctrl Pts',(-6.13782098400006,12.2,-9.02795287300002));
#283888=CARTESIAN_POINT('Ctrl Pts',(-6.13550475100006,12.2,-9.02620432800001));
#283889=CARTESIAN_POINT('Ctrl Pts',(-6.13319438500006,12.2,-9.02445720900002));
#283890=CARTESIAN_POINT('Ctrl Pts',(-6.13088988900006,12.2,-9.02271152900001));
#283891=CARTESIAN_POINT('Ctrl Pts',(-6.12859126900006,12.2,-9.02096729900002));
#283892=CARTESIAN_POINT('Ctrl Pts',(-6.12629852600006,12.2,-9.01922453300001));
#283893=CARTESIAN_POINT('Ctrl Pts',(-6.12401166400006,12.2,-9.01748324100001));
#283894=CARTESIAN_POINT('Ctrl Pts',(-6.12173068600006,12.2,-9.01574343800002));
#283895=CARTESIAN_POINT('Ctrl Pts',(-6.11945559600006,12.2,-9.01400513500001));
#283896=CARTESIAN_POINT('Ctrl Pts',(-6.11718639600006,12.2,-9.01226834500001));
#283897=CARTESIAN_POINT('Ctrl Pts',(-6.11492309000006,12.2,-9.01053308200002));
#283898=CARTESIAN_POINT('Ctrl Pts',(-6.11266568000006,12.2,-9.00879935600001));
#283899=CARTESIAN_POINT('Ctrl Pts',(-6.11041417200005,12.2,-9.00706718000002));
#283900=CARTESIAN_POINT('Ctrl Pts',(-6.10816856500006,12.2,-9.00533656900001));
#283901=CARTESIAN_POINT('Ctrl Pts',(-6.10592886600006,12.2,-9.00360753300001));
#283902=CARTESIAN_POINT('Ctrl Pts',(-6.10369507600006,12.2,-9.00188008700002));
#283903=CARTESIAN_POINT('Ctrl Pts',(-6.10146719900006,12.2,-9.00015424200001));
#283904=CARTESIAN_POINT('Ctrl Pts',(-6.09924523800006,12.2,-8.99843001200002));
#283905=CARTESIAN_POINT('Ctrl Pts',(-6.09702919700006,12.2,-8.99670741000002));
#283906=CARTESIAN_POINT('Ctrl Pts',(-6.09481907700006,12.2,-8.99498644800002));
#283907=CARTESIAN_POINT('Ctrl Pts',(-6.09261488400006,12.2,-8.99326713800002));
#283908=CARTESIAN_POINT('Ctrl Pts',(-6.09041662000006,12.2,-8.99154949500002));
#283909=CARTESIAN_POINT('Ctrl Pts',(-6.08822428600006,12.2,-8.98983353000002));
#283910=CARTESIAN_POINT('Ctrl Pts',(-6.08603788900006,12.2,-8.98811925800001));
#283911=CARTESIAN_POINT('Ctrl Pts',(-6.08385743000006,12.2,-8.98640669100002));
#283912=CARTESIAN_POINT('Ctrl Pts',(-6.08168291200006,12.2,-8.98469584100001));
#283913=CARTESIAN_POINT('Ctrl Pts',(-6.07951433900006,12.2,-8.98298672300001));
#283914=CARTESIAN_POINT('Ctrl Pts',(-6.07735171400006,12.2,-8.98127934900002));
#283915=CARTESIAN_POINT('Ctrl Pts',(-6.07519504000006,12.2,-8.97957373400001));
#283916=CARTESIAN_POINT('Ctrl Pts',(-6.07304431900006,12.2,-8.97786988800001));
#283917=CARTESIAN_POINT('Ctrl Pts',(-6.07089955600006,12.2,-8.97616782700002));
#283918=CARTESIAN_POINT('Ctrl Pts',(-6.06876075400006,12.2,-8.97446756300001));
#283919=CARTESIAN_POINT('Ctrl Pts',(-6.06662791600006,12.2,-8.97276910900001));
#283920=CARTESIAN_POINT('Ctrl Pts',(-6.06450104400006,12.2,-8.97107248000001));
#283921=CARTESIAN_POINT('Ctrl Pts',(-6.06238014200006,12.2,-8.96937768800001));
#283922=CARTESIAN_POINT('Ctrl Pts',(-6.06026521300006,12.2,-8.96768474600002));
#283923=CARTESIAN_POINT('Ctrl Pts',(-6.05815626100005,12.2,-8.96599367000002));
#283924=CARTESIAN_POINT('Ctrl Pts',(-6.05605328900006,12.2,-8.96430447000002));
#283925=CARTESIAN_POINT('Ctrl Pts',(-6.05395629800006,12.2,-8.96261716200002));
#283926=CARTESIAN_POINT('Ctrl Pts',(-6.05186529400005,12.2,-8.96093175800001));
#283927=CARTESIAN_POINT('Ctrl Pts',(-6.04978027800006,12.2,-8.95924827300002));
#283928=CARTESIAN_POINT('Ctrl Pts',(-6.04770125400006,12.2,-8.95756672100001));
#283929=CARTESIAN_POINT('Ctrl Pts',(-6.04562822600006,12.2,-8.95588711400002));
#283930=CARTESIAN_POINT('Ctrl Pts',(-6.04356119600006,12.2,-8.95420946700002));
#283931=CARTESIAN_POINT('Ctrl Pts',(-6.04150016700006,12.2,-8.95253379300001));
#283932=CARTESIAN_POINT('Ctrl Pts',(-6.03944514200006,12.2,-8.95086010500002));
#283933=CARTESIAN_POINT('Ctrl Pts',(-6.03739612600006,12.2,-8.94918841900001));
#283934=CARTESIAN_POINT('Ctrl Pts',(-6.03535312000006,12.2,-8.94751874800002));
#283935=CARTESIAN_POINT('Ctrl Pts',(-6.03331612900006,12.2,-8.94585110500002));
#283936=CARTESIAN_POINT('Ctrl Pts',(-6.03128515400006,12.2,-8.94418550400001));
#283937=CARTESIAN_POINT('Ctrl Pts',(-6.02926019900006,12.2,-8.94252196100001));
#283938=CARTESIAN_POINT('Ctrl Pts',(-6.02724126900006,12.2,-8.94086048800002));
#283939=CARTESIAN_POINT('Ctrl Pts',(-6.02522836400006,12.2,-8.93920110000002));
#283940=CARTESIAN_POINT('Ctrl Pts',(-6.02322148900006,12.2,-8.93754381100001));
#283941=CARTESIAN_POINT('Ctrl Pts',(-6.02122064700006,12.2,-8.93588863500002));
#283942=CARTESIAN_POINT('Ctrl Pts',(-6.01922584100006,12.2,-8.93423558600002));
#283943=CARTESIAN_POINT('Ctrl Pts',(-6.01723707400006,12.2,-8.93258467900001));
#283944=CARTESIAN_POINT('Ctrl Pts',(-6.01525434800006,12.2,-8.93093592700002));
#283945=CARTESIAN_POINT('Ctrl Pts',(-6.01327766800006,12.2,-8.92928934400001));
#283946=CARTESIAN_POINT('Ctrl Pts',(-6.01130703700006,12.2,-8.92764494600002));
#283947=CARTESIAN_POINT('Ctrl Pts',(-6.00934245600006,12.2,-8.92600274700002));
#283948=CARTESIAN_POINT('Ctrl Pts',(-6.00738393100006,12.2,-8.92436276200002));
#283949=CARTESIAN_POINT('Ctrl Pts',(-6.00543146200006,12.2,-8.92272500300002));
#283950=CARTESIAN_POINT('Ctrl Pts',(-6.00348505500006,12.2,-8.92108948700002));
#283951=CARTESIAN_POINT('Ctrl Pts',(-6.00154471100006,12.2,-8.91945622800002));
#283952=CARTESIAN_POINT('Ctrl Pts',(-5.99961043400006,12.2,-8.91782524000002));
#283953=CARTESIAN_POINT('Ctrl Pts',(-5.99768222800006,12.2,-8.91619653700002));
#283954=CARTESIAN_POINT('Ctrl Pts',(-5.99576009400006,12.2,-8.91457013600002));
#283955=CARTESIAN_POINT('Ctrl Pts',(-5.99384403600006,12.2,-8.91294604900001));
#283956=CARTESIAN_POINT('Ctrl Pts',(-5.99193405800006,12.2,-8.91132429300002));
#283957=CARTESIAN_POINT('Ctrl Pts',(-5.99003016200006,12.2,-8.90970488200002));
#283958=CARTESIAN_POINT('Ctrl Pts',(-5.98813235200006,12.2,-8.90808783100002));
#283959=CARTESIAN_POINT('Ctrl Pts',(-5.98624062900006,12.2,-8.90647315300001));
#283960=CARTESIAN_POINT('Ctrl Pts',(-5.98435500000006,12.2,-8.90486086600001));
#283961=CARTESIAN_POINT('Ctrl Pts',(-5.98247546400006,12.2,-8.90325098400002));
#283962=CARTESIAN_POINT('Ctrl Pts',(-5.98060202600006,12.2,-8.90164352000001));
#283963=CARTESIAN_POINT('Ctrl Pts',(-5.97873468900006,12.2,-8.90003849100001));
#283964=CARTESIAN_POINT('Ctrl Pts',(-5.97687345600006,12.2,-8.89843591300002));
#283965=CARTESIAN_POINT('Ctrl Pts',(-5.97501833000006,12.2,-8.89683579900002));
#283966=CARTESIAN_POINT('Ctrl Pts',(-5.97316931400006,12.2,-8.89523816500001));
#283967=CARTESIAN_POINT('Ctrl Pts',(-5.97132641200006,12.2,-8.89364302600002));
#283968=CARTESIAN_POINT('Ctrl Pts',(-5.96948962500006,12.2,-8.89205039900002));
#283969=CARTESIAN_POINT('Ctrl Pts',(-5.96765895700006,12.2,-8.89046029700001));
#283970=CARTESIAN_POINT('Ctrl Pts',(-5.96583441200006,12.2,-8.88887273700002));
#283971=CARTESIAN_POINT('Ctrl Pts',(-5.96401599300005,12.2,-8.88728773400001));
#283972=CARTESIAN_POINT('Ctrl Pts',(-5.96220370200006,12.2,-8.88570530200001));
#283973=CARTESIAN_POINT('Ctrl Pts',(-5.96039754200006,12.2,-8.88412545900002));
#283974=CARTESIAN_POINT('Ctrl Pts',(-5.95859751600006,12.2,-8.88254821900002));
#283975=CARTESIAN_POINT('Ctrl Pts',(-5.95680362900006,12.2,-8.88097359800001));
#283976=CARTESIAN_POINT('Ctrl Pts',(-5.95501588200006,12.2,-8.87940161100002));
#283977=CARTESIAN_POINT('Ctrl Pts',(-5.95323427900006,12.2,-8.87783227600002));
#283978=CARTESIAN_POINT('Ctrl Pts',(-5.95145882200006,12.2,-8.87626560600001));
#283979=CARTESIAN_POINT('Ctrl Pts',(-5.94968951600006,12.2,-8.87470161900002));
#283980=CARTESIAN_POINT('Ctrl Pts',(-5.94792636200006,12.2,-8.87314032800001));
#283981=CARTESIAN_POINT('Ctrl Pts',(-5.94616936500006,12.2,-8.87158175200002));
#283982=CARTESIAN_POINT('Ctrl Pts',(-5.94441852600006,12.2,-8.87002590600002));
#283983=CARTESIAN_POINT('Ctrl Pts',(-5.94267384900006,12.2,-8.86847280400002));
#283984=CARTESIAN_POINT('Ctrl Pts',(-5.94093533700006,12.2,-8.86692246600001));
#283985=CARTESIAN_POINT('Ctrl Pts',(-5.93920299300006,12.2,-8.86537490400002));
#283986=CARTESIAN_POINT('Ctrl Pts',(-5.93747681900005,12.2,-8.86383013700001));
#283987=CARTESIAN_POINT('Ctrl Pts',(-5.93575682000006,12.2,-8.86228817900001));
#283988=CARTESIAN_POINT('Ctrl Pts',(-5.93404299900006,12.2,-8.86074904800001));
#283989=CARTESIAN_POINT('Ctrl Pts',(-5.93233535700006,12.2,-8.85921276000002));
#283990=CARTESIAN_POINT('Ctrl Pts',(-5.93063389800006,12.2,-8.85767933100002));
#283991=CARTESIAN_POINT('Ctrl Pts',(-5.92893862600006,12.2,-8.85614877700002));
#283992=CARTESIAN_POINT('Ctrl Pts',(-5.92724954300006,12.2,-8.85462111500001));
#283993=CARTESIAN_POINT('Ctrl Pts',(-5.92556665300005,12.2,-8.85309636200001));
#283994=CARTESIAN_POINT('Ctrl Pts',(-5.92388995600006,12.2,-8.85157453400002));
#283995=CARTESIAN_POINT('Ctrl Pts',(-5.92221945900006,12.2,-8.85005564700002));
#283996=CARTESIAN_POINT('Ctrl Pts',(-5.92055516300006,12.2,-8.84853971800002));
#283997=CARTESIAN_POINT('Ctrl Pts',(-5.91889707100006,12.2,-8.84702676400002));
#283998=CARTESIAN_POINT('Ctrl Pts',(-5.91724518600006,12.2,-8.84551680200002));
#283999=CARTESIAN_POINT('Ctrl Pts',(-5.91559951200006,12.2,-8.84400984900001));
#284000=CARTESIAN_POINT('Ctrl Pts',(-5.91396005000006,12.2,-8.84250592100001));
#284001=CARTESIAN_POINT('Ctrl Pts',(-5.91232680500006,12.2,-8.84100503500001));
#284002=CARTESIAN_POINT('Ctrl Pts',(-5.91069977900006,12.2,-8.83950721000001));
#284003=CARTESIAN_POINT('Ctrl Pts',(-5.90907897600006,12.2,-8.83801246000001));
#284004=CARTESIAN_POINT('Ctrl Pts',(-5.90746439700006,12.2,-8.83652080200001));
#284005=CARTESIAN_POINT('Ctrl Pts',(-5.90585604700006,12.2,-8.83503225700002));
#284006=CARTESIAN_POINT('Ctrl Pts',(-5.90425392900006,12.2,-8.83354683900002));
#284007=CARTESIAN_POINT('Ctrl Pts',(-5.90265804300006,12.2,-8.83206456600002));
#284008=CARTESIAN_POINT('Ctrl Pts',(-5.90106839700006,12.2,-8.83058545500001));
#284009=CARTESIAN_POINT('Ctrl Pts',(-5.89948498900006,12.2,-8.82910952300002));
#284010=CARTESIAN_POINT('Ctrl Pts',(-5.89790782500006,12.2,-8.82763679000002));
#284011=CARTESIAN_POINT('Ctrl Pts',(-5.89633690700006,12.2,-8.82616727000002));
#284012=CARTESIAN_POINT('Ctrl Pts',(-5.89477223700006,12.2,-8.82470098400002));
#284013=CARTESIAN_POINT('Ctrl Pts',(-5.89321382100006,12.2,-8.82323794600002));
#284014=CARTESIAN_POINT('Ctrl Pts',(-5.89166165900005,12.2,-8.82177817600001));
#284015=CARTESIAN_POINT('Ctrl Pts',(-5.89011575500006,12.2,-8.82032169100002));
#284016=CARTESIAN_POINT('Ctrl Pts',(-5.88857611200006,12.2,-8.81886851000001));
#284017=CARTESIAN_POINT('Ctrl Pts',(-5.88704273400006,12.2,-8.81741864800002));
#284018=CARTESIAN_POINT('Ctrl Pts',(-5.88551562100006,12.2,-8.81597212600001));
#284019=CARTESIAN_POINT('Ctrl Pts',(-5.88399477900006,12.2,-8.81452896000001));
#284020=CARTESIAN_POINT('Ctrl Pts',(-5.88248021000005,12.2,-8.81308916900002));
#284021=CARTESIAN_POINT('Ctrl Pts',(-5.88097191600006,12.2,-8.81165276900001));
#284022=CARTESIAN_POINT('Ctrl Pts',(-5.87946990200006,12.2,-8.81021978100001));
#284023=CARTESIAN_POINT('Ctrl Pts',(-5.87797416900006,12.2,-8.80879022300002));
#284024=CARTESIAN_POINT('Ctrl Pts',(-5.87648472000006,12.2,-8.80736411100001));
#284025=CARTESIAN_POINT('Ctrl Pts',(-5.87500155900006,12.2,-8.80594146500002));
#284026=CARTESIAN_POINT('Ctrl Pts',(-5.87352468900006,12.2,-8.80452230300002));
#284027=CARTESIAN_POINT('Ctrl Pts',(-5.87205411200006,12.2,-8.80310664200002));
#284028=CARTESIAN_POINT('Ctrl Pts',(-5.87058983200006,12.2,-8.80169450300002));
#284029=CARTESIAN_POINT('Ctrl Pts',(-5.86913185000006,12.2,-8.80028590300002));
#284030=CARTESIAN_POINT('Ctrl Pts',(-5.86768017200006,12.2,-8.79888086200001));
#284031=CARTESIAN_POINT('Ctrl Pts',(-5.86623479900005,12.2,-8.79747939600002));
#284032=CARTESIAN_POINT('Ctrl Pts',(-5.86479573400006,12.2,-8.79608152700002));
#284033=CARTESIAN_POINT('Ctrl Pts',(-5.86336298000006,12.2,-8.79468727200001));
#284034=CARTESIAN_POINT('Ctrl Pts',(-5.86193653900006,12.2,-8.79329665000002));
#284035=CARTESIAN_POINT('Ctrl Pts',(-5.86051641600006,12.2,-8.79190968000002));
#284036=CARTESIAN_POINT('Ctrl Pts',(-5.85910261300006,12.2,-8.79052638100001));
#284037=CARTESIAN_POINT('Ctrl Pts',(-5.85769513200006,12.2,-8.78914677200001));
#284038=CARTESIAN_POINT('Ctrl Pts',(-5.85629397700006,12.2,-8.78777087300002));
#284039=CARTESIAN_POINT('Ctrl Pts',(-5.85489915200006,12.2,-8.78639870300002));
#284040=CARTESIAN_POINT('Ctrl Pts',(-5.85351065700006,12.2,-8.78503028000001));
#284041=CARTESIAN_POINT('Ctrl Pts',(-5.85212849700006,12.2,-8.78366562400002));
#284042=CARTESIAN_POINT('Ctrl Pts',(-5.85075267500006,12.2,-8.78230475600001));
#284043=CARTESIAN_POINT('Ctrl Pts',(-5.84938319300006,12.2,-8.78094769400001));
#284044=CARTESIAN_POINT('Ctrl Pts',(-5.84802005400006,12.2,-8.77959445700002));
#284045=CARTESIAN_POINT('Ctrl Pts',(-5.84666326000006,12.2,-8.77824506500002));
#284046=CARTESIAN_POINT('Ctrl Pts',(-5.84531281700006,12.2,-8.77689953800001));
#284047=CARTESIAN_POINT('Ctrl Pts',(-5.84396872500006,12.2,-8.77555789600001));
#284048=CARTESIAN_POINT('Ctrl Pts',(-5.84263098700006,12.2,-8.77422015900001));
#284049=CARTESIAN_POINT('Ctrl Pts',(-5.84129960800006,12.2,-8.77288634600001));
#284050=CARTESIAN_POINT('Ctrl Pts',(-5.83997459000006,12.2,-8.77155647700001));
#284051=CARTESIAN_POINT('Ctrl Pts',(-5.83865593500006,12.2,-8.77023057400002));
#284052=CARTESIAN_POINT('Ctrl Pts',(-5.83734364600006,12.2,-8.76890865500001));
#284053=CARTESIAN_POINT('Ctrl Pts',(-5.83603772700005,12.2,-8.76759074100002));
#284054=CARTESIAN_POINT('Ctrl Pts',(-5.83473817900006,12.2,-8.76627685200001));
#284055=CARTESIAN_POINT('Ctrl Pts',(-5.83344500700006,12.2,-8.76496700800002));
#284056=CARTESIAN_POINT('Ctrl Pts',(-5.83215821300006,12.2,-8.76366123100001));
#284057=CARTESIAN_POINT('Ctrl Pts',(-5.83087780000006,12.2,-8.76235953900002));
#284058=CARTESIAN_POINT('Ctrl Pts',(-5.82960377000005,12.2,-8.76106195500002));
#284059=CARTESIAN_POINT('Ctrl Pts',(-5.82833612700006,12.2,-8.75976849900002));
#284060=CARTESIAN_POINT('Ctrl Pts',(-5.82707487300006,12.2,-8.75847919000002));
#284061=CARTESIAN_POINT('Ctrl Pts',(-5.82582001200006,12.2,-8.75719405100002));
#284062=CARTESIAN_POINT('Ctrl Pts',(-5.82457154700006,12.2,-8.75591310200001));
#284063=CARTESIAN_POINT('Ctrl Pts',(-5.82332948000006,12.2,-8.75463636300001));
#284064=CARTESIAN_POINT('Ctrl Pts',(-5.82209381200006,12.2,-8.75336385700002));
#284065=CARTESIAN_POINT('Ctrl Pts',(-5.82086454900006,12.2,-8.75209560300001));
#284066=CARTESIAN_POINT('Ctrl Pts',(-5.81964169300006,12.2,-8.75083162500001));
#284067=CARTESIAN_POINT('Ctrl Pts',(-5.81842524600006,12.2,-8.74957194100002));
#284068=CARTESIAN_POINT('Ctrl Pts',(-5.81721521200006,12.2,-8.74831657400001));
#284069=CARTESIAN_POINT('Ctrl Pts',(-5.81601159400006,12.2,-8.74706554600002));
#284070=CARTESIAN_POINT('Ctrl Pts',(-5.81481439300005,12.2,-8.74581887800002));
#284071=CARTESIAN_POINT('Ctrl Pts',(-5.81362361300005,12.2,-8.74457659100001));
#284072=CARTESIAN_POINT('Ctrl Pts',(-5.81243925700006,12.2,-8.74333870700001));
#284073=CARTESIAN_POINT('Ctrl Pts',(-5.81126132800006,12.2,-8.74210524800001));
#284074=CARTESIAN_POINT('Ctrl Pts',(-5.81008982800006,12.2,-8.74087623600002));
#284075=CARTESIAN_POINT('Ctrl Pts',(-5.80892476100006,12.2,-8.73965169300002));
#284076=CARTESIAN_POINT('Ctrl Pts',(-5.80776612900006,12.2,-8.73843163900002));
#284077=CARTESIAN_POINT('Ctrl Pts',(-5.80661393400006,12.2,-8.73721609800001));
#284078=CARTESIAN_POINT('Ctrl Pts',(-5.80546818100006,12.2,-8.73600509300001));
#284079=CARTESIAN_POINT('Ctrl Pts',(-5.80432887200006,12.2,-8.73479864500002));
#284080=CARTESIAN_POINT('Ctrl Pts',(-5.80319600900006,12.2,-8.73359677600002));
#284081=CARTESIAN_POINT('Ctrl Pts',(-5.80206959600006,12.2,-8.73239950900001));
#284082=CARTESIAN_POINT('Ctrl Pts',(-5.80094963500006,12.2,-8.73120686600002));
#284083=CARTESIAN_POINT('Ctrl Pts',(-5.79983612800006,12.2,-8.73001887100001));
#284084=CARTESIAN_POINT('Ctrl Pts',(-5.79872908000006,12.2,-8.72883554600002));
#284085=CARTESIAN_POINT('Ctrl Pts',(-5.79762849300006,12.2,-8.72765691300001));
#284086=CARTESIAN_POINT('Ctrl Pts',(-5.79653437000006,12.2,-8.72648299600002));
#284087=CARTESIAN_POINT('Ctrl Pts',(-5.79544671200006,12.2,-8.72531381700002));
#284088=CARTESIAN_POINT('Ctrl Pts',(-5.79436552400006,12.2,-8.72414939900001));
#284089=CARTESIAN_POINT('Ctrl Pts',(-5.79329080800006,12.2,-8.72298976600002));
#284090=CARTESIAN_POINT('Ctrl Pts',(-5.79222256600006,12.2,-8.72183494100002));
#284091=CARTESIAN_POINT('Ctrl Pts',(-5.79116080300006,12.2,-8.72068494800001));
#284092=CARTESIAN_POINT('Ctrl Pts',(-5.79010551900006,12.2,-8.71953980900001));
#284093=CARTESIAN_POINT('Ctrl Pts',(-5.78905671900006,12.2,-8.71839954800001));
#284094=CARTESIAN_POINT('Ctrl Pts',(-5.78801440500006,12.2,-8.71726418900002));
#284095=CARTESIAN_POINT('Ctrl Pts',(-5.78697858000006,12.2,-8.71613375700001));
#284096=CARTESIAN_POINT('Ctrl Pts',(-5.78594924700006,12.2,-8.71500827300002));
#284097=CARTESIAN_POINT('Ctrl Pts',(-5.78492640800006,12.2,-8.71388776300002));
#284098=CARTESIAN_POINT('Ctrl Pts',(-5.78391006700006,12.2,-8.71277225000001));
#284099=CARTESIAN_POINT('Ctrl Pts',(-5.78290022600005,12.2,-8.71166175800001));
#284100=CARTESIAN_POINT('Ctrl Pts',(-5.78189688700006,12.2,-8.71055631200001));
#284101=CARTESIAN_POINT('Ctrl Pts',(-5.78090005400006,12.2,-8.70945593700002));
#284102=CARTESIAN_POINT('Ctrl Pts',(-5.77990973100006,12.2,-8.70836065500002));
#284103=CARTESIAN_POINT('Ctrl Pts',(-5.77892591700006,12.2,-8.70727049300001));
#284104=CARTESIAN_POINT('Ctrl Pts',(-5.77794861800006,12.2,-8.70618547500002));
#284105=CARTESIAN_POINT('Ctrl Pts',(-5.77697783600006,12.2,-8.70510562400002));
#284106=CARTESIAN_POINT('Ctrl Pts',(-5.77601357300006,12.2,-8.70403096700001));
#284107=CARTESIAN_POINT('Ctrl Pts',(-5.77505583400006,12.2,-8.70296152800002));
#284108=CARTESIAN_POINT('Ctrl Pts',(-5.77410461900006,12.2,-8.70189733200002));
#284109=CARTESIAN_POINT('Ctrl Pts',(-5.77315993200005,12.2,-8.70083840400002));
#284110=CARTESIAN_POINT('Ctrl Pts',(-5.77222177600006,12.2,-8.69978477000002));
#284111=CARTESIAN_POINT('Ctrl Pts',(-5.77129015400006,12.2,-8.69873645500002));
#284112=CARTESIAN_POINT('Ctrl Pts',(-5.77036506700006,12.2,-8.69769348400002));
#284113=CARTESIAN_POINT('Ctrl Pts',(-5.76944652100006,12.2,-8.69665588300002));
#284114=CARTESIAN_POINT('Ctrl Pts',(-5.76853451500006,12.2,-8.69562367700001));
#284115=CARTESIAN_POINT('Ctrl Pts',(-5.76762905500006,12.2,-8.69459689400001));
#284116=CARTESIAN_POINT('Ctrl Pts',(-5.76673014200006,12.2,-8.69357555700002));
#284117=CARTESIAN_POINT('Ctrl Pts',(-5.76583777900006,12.2,-8.69255969400001));
#284118=CARTESIAN_POINT('Ctrl Pts',(-5.76495197000006,12.2,-8.69154933000001));
#284119=CARTESIAN_POINT('Ctrl Pts',(-5.76407271500006,12.2,-8.69054449200001));
#284120=CARTESIAN_POINT('Ctrl Pts',(-5.76320002000006,12.2,-8.68954520600001));
#284121=CARTESIAN_POINT('Ctrl Pts',(-5.76233388600006,12.2,-8.68855149800002));
#284122=CARTESIAN_POINT('Ctrl Pts',(-5.76147431600006,12.2,-8.68756339600001));
#284123=CARTESIAN_POINT('Ctrl Pts',(-5.76062131200006,12.2,-8.68658092600001));
#284124=CARTESIAN_POINT('Ctrl Pts',(-5.75977487800006,12.2,-8.68560411500002));
#284125=CARTESIAN_POINT('Ctrl Pts',(-5.75893501600006,12.2,-8.68463298900001));
#284126=CARTESIAN_POINT('Ctrl Pts',(-5.75810173000006,12.2,-8.68366757600001));
#284127=CARTESIAN_POINT('Ctrl Pts',(-5.75727502100006,12.2,-8.68270790200001));
#284128=CARTESIAN_POINT('Ctrl Pts',(-5.75645489300006,12.2,-8.68175399800002));
#284129=CARTESIAN_POINT('Ctrl Pts',(-5.75564134700006,12.2,-8.68080588500002));
#284130=CARTESIAN_POINT('Ctrl Pts',(-5.75483438800005,12.2,-8.67986359700001));
#284131=CARTESIAN_POINT('Ctrl Pts',(-5.75403401900005,12.2,-8.67892715900001));
#284132=CARTESIAN_POINT('Ctrl Pts',(-5.75324024000006,12.2,-8.67799659800001));
#284133=CARTESIAN_POINT('Ctrl Pts',(-5.75245305600006,12.2,-8.67707194200002));
#284134=CARTESIAN_POINT('Ctrl Pts',(-5.75167246900006,12.2,-8.67615322100002));
#284135=CARTESIAN_POINT('Ctrl Pts',(-5.75089848100006,12.2,-8.67524046100002));
#284136=CARTESIAN_POINT('Ctrl Pts',(-5.75013109600006,12.2,-8.67433369300001));
#284137=CARTESIAN_POINT('Ctrl Pts',(-5.74937031600006,12.2,-8.67343294300002));
#284138=CARTESIAN_POINT('Ctrl Pts',(-5.74861614500006,12.2,-8.67253824000001));
#284139=CARTESIAN_POINT('Ctrl Pts',(-5.74786858400006,12.2,-8.67164961300002));
#284140=CARTESIAN_POINT('Ctrl Pts',(-5.74712763600006,12.2,-8.67076709200001));
#284141=CARTESIAN_POINT('Ctrl Pts',(-5.74639330500006,12.2,-8.66989070400002));
#284142=CARTESIAN_POINT('Ctrl Pts',(-5.74566559300006,12.2,-8.66902047900002));
#284143=CARTESIAN_POINT('Ctrl Pts',(-5.74494450300006,12.2,-8.66815644700001));
#284144=CARTESIAN_POINT('Ctrl Pts',(-5.74423003600006,12.2,-8.66729863600002));
#284145=CARTESIAN_POINT('Ctrl Pts',(-5.74352219700006,12.2,-8.66644707700001));
#284146=CARTESIAN_POINT('Ctrl Pts',(-5.74282098800006,12.2,-8.66560180000001));
#284147=CARTESIAN_POINT('Ctrl Pts',(-5.74212641100006,12.2,-8.66476283200001));
#284148=CARTESIAN_POINT('Ctrl Pts',(-5.74143847000006,12.2,-8.66393020500002));
#284149=CARTESIAN_POINT('Ctrl Pts',(-5.74075716700006,12.2,-8.66310395100001));
#284150=CARTESIAN_POINT('Ctrl Pts',(-5.74008250400006,12.2,-8.66228409600001));
#284151=CARTESIAN_POINT('Ctrl Pts',(-5.73941448500006,12.2,-8.66147067400002));
#284152=CARTESIAN_POINT('Ctrl Pts',(-5.73875311300006,12.2,-8.66066371300001));
#284153=CARTESIAN_POINT('Ctrl Pts',(-5.73809838900006,12.2,-8.65986324600001));
#284154=CARTESIAN_POINT('Ctrl Pts',(-5.73745031600006,12.2,-8.65906930200002));
#284155=CARTESIAN_POINT('Ctrl Pts',(-5.73680889900006,12.2,-8.65828191300002));
#284156=CARTESIAN_POINT('Ctrl Pts',(-5.73617413900006,12.2,-8.65750111000001));
#284157=CARTESIAN_POINT('Ctrl Pts',(-5.73554603700006,12.2,-8.65672692500001));
#284158=CARTESIAN_POINT('Ctrl Pts',(-5.73492459900006,12.2,-8.65595938700002));
#284159=CARTESIAN_POINT('Ctrl Pts',(-5.73430982600006,12.2,-8.65519853100002));
#284160=CARTESIAN_POINT('Ctrl Pts',(-5.73370172100006,12.2,-8.65444438600001));
#284161=CARTESIAN_POINT('Ctrl Pts',(-5.73310028700006,12.2,-8.65369698500002));
#284162=CARTESIAN_POINT('Ctrl Pts',(-5.73250552600006,12.2,-8.65295636100001));
#284163=CARTESIAN_POINT('Ctrl Pts',(-5.73191744100006,12.2,-8.65222254500001));
#284164=CARTESIAN_POINT('Ctrl Pts',(-5.73133603500006,12.2,-8.65149557000001));
#284165=CARTESIAN_POINT('Ctrl Pts',(-5.73076462000006,12.2,-8.65077961500001));
#284166=CARTESIAN_POINT('Ctrl Pts',(-5.73031342200006,12.2,-8.65021312700001));
#284167=CARTESIAN_POINT('Ctrl Pts',(-5.72997879300006,12.2,-8.64979235000002));
#284168=CARTESIAN_POINT('Ctrl Pts',(-5.72975808700006,12.2,-8.64951454400002));
#284169=CARTESIAN_POINT('Ctrl Pts',(-5.72964966100006,12.2,-8.64937799900002));
#284170=CARTESIAN_POINT('Ctrl Pts',(-5.72964966100006,15.2,-8.64937799900002));
#284171=CARTESIAN_POINT('Ctrl Pts',(-5.72975808700006,15.2,-8.64951454400002));
#284172=CARTESIAN_POINT('Ctrl Pts',(-5.72997879300006,15.2,-8.64979235000002));
#284173=CARTESIAN_POINT('Ctrl Pts',(-5.73031342200006,15.2,-8.65021312700001));
#284174=CARTESIAN_POINT('Ctrl Pts',(-5.73076462000006,15.2,-8.65077961500001));
#284175=CARTESIAN_POINT('Ctrl Pts',(-5.73133603500006,15.2,-8.65149557000001));
#284176=CARTESIAN_POINT('Ctrl Pts',(-5.73191744100006,15.2,-8.65222254500001));
#284177=CARTESIAN_POINT('Ctrl Pts',(-5.73250552600006,15.2,-8.65295636100001));
#284178=CARTESIAN_POINT('Ctrl Pts',(-5.73310028700006,15.2,-8.65369698500002));
#284179=CARTESIAN_POINT('Ctrl Pts',(-5.73370172100006,15.2,-8.65444438600001));
#284180=CARTESIAN_POINT('Ctrl Pts',(-5.73430982600006,15.2,-8.65519853100002));
#284181=CARTESIAN_POINT('Ctrl Pts',(-5.73492459900006,15.2,-8.65595938700002));
#284182=CARTESIAN_POINT('Ctrl Pts',(-5.73554603700006,15.2,-8.65672692500001));
#284183=CARTESIAN_POINT('Ctrl Pts',(-5.73617413900006,15.2,-8.65750111000001));
#284184=CARTESIAN_POINT('Ctrl Pts',(-5.73680889900006,15.2,-8.65828191300002));
#284185=CARTESIAN_POINT('Ctrl Pts',(-5.73745031600006,15.2,-8.65906930200002));
#284186=CARTESIAN_POINT('Ctrl Pts',(-5.73809838900006,15.2,-8.65986324600001));
#284187=CARTESIAN_POINT('Ctrl Pts',(-5.73875311300006,15.2,-8.66066371300001));
#284188=CARTESIAN_POINT('Ctrl Pts',(-5.73941448500006,15.2,-8.66147067400002));
#284189=CARTESIAN_POINT('Ctrl Pts',(-5.74008250400006,15.2,-8.66228409600001));
#284190=CARTESIAN_POINT('Ctrl Pts',(-5.74075716700006,15.2,-8.66310395100001));
#284191=CARTESIAN_POINT('Ctrl Pts',(-5.74143847000006,15.2,-8.66393020500002));
#284192=CARTESIAN_POINT('Ctrl Pts',(-5.74212641100006,15.2,-8.66476283200001));
#284193=CARTESIAN_POINT('Ctrl Pts',(-5.74282098800006,15.2,-8.66560180000001));
#284194=CARTESIAN_POINT('Ctrl Pts',(-5.74352219700006,15.2,-8.66644707700001));
#284195=CARTESIAN_POINT('Ctrl Pts',(-5.74423003600006,15.2,-8.66729863600002));
#284196=CARTESIAN_POINT('Ctrl Pts',(-5.74494450300006,15.2,-8.66815644700001));
#284197=CARTESIAN_POINT('Ctrl Pts',(-5.74566559300006,15.2,-8.66902047900002));
#284198=CARTESIAN_POINT('Ctrl Pts',(-5.74639330500006,15.2,-8.66989070400002));
#284199=CARTESIAN_POINT('Ctrl Pts',(-5.74712763600006,15.2,-8.67076709200001));
#284200=CARTESIAN_POINT('Ctrl Pts',(-5.74786858400006,15.2,-8.67164961300002));
#284201=CARTESIAN_POINT('Ctrl Pts',(-5.74861614500006,15.2,-8.67253824000001));
#284202=CARTESIAN_POINT('Ctrl Pts',(-5.74937031600006,15.2,-8.67343294300002));
#284203=CARTESIAN_POINT('Ctrl Pts',(-5.75013109600006,15.2,-8.67433369300001));
#284204=CARTESIAN_POINT('Ctrl Pts',(-5.75089848100006,15.2,-8.67524046100002));
#284205=CARTESIAN_POINT('Ctrl Pts',(-5.75167246900006,15.2,-8.67615322100002));
#284206=CARTESIAN_POINT('Ctrl Pts',(-5.75245305600006,15.2,-8.67707194200002));
#284207=CARTESIAN_POINT('Ctrl Pts',(-5.75324024000006,15.2,-8.67799659800001));
#284208=CARTESIAN_POINT('Ctrl Pts',(-5.75403401900005,15.2,-8.67892715900001));
#284209=CARTESIAN_POINT('Ctrl Pts',(-5.75483438800005,15.2,-8.67986359700001));
#284210=CARTESIAN_POINT('Ctrl Pts',(-5.75564134700006,15.2,-8.68080588500002));
#284211=CARTESIAN_POINT('Ctrl Pts',(-5.75645489300006,15.2,-8.68175399800002));
#284212=CARTESIAN_POINT('Ctrl Pts',(-5.75727502100006,15.2,-8.68270790200001));
#284213=CARTESIAN_POINT('Ctrl Pts',(-5.75810173000006,15.2,-8.68366757600001));
#284214=CARTESIAN_POINT('Ctrl Pts',(-5.75893501600006,15.2,-8.68463298900001));
#284215=CARTESIAN_POINT('Ctrl Pts',(-5.75977487800006,15.2,-8.68560411500002));
#284216=CARTESIAN_POINT('Ctrl Pts',(-5.76062131200006,15.2,-8.68658092600001));
#284217=CARTESIAN_POINT('Ctrl Pts',(-5.76147431600006,15.2,-8.68756339600001));
#284218=CARTESIAN_POINT('Ctrl Pts',(-5.76233388600006,15.2,-8.68855149800002));
#284219=CARTESIAN_POINT('Ctrl Pts',(-5.76320002000006,15.2,-8.68954520600001));
#284220=CARTESIAN_POINT('Ctrl Pts',(-5.76407271500006,15.2,-8.69054449200001));
#284221=CARTESIAN_POINT('Ctrl Pts',(-5.76495197000006,15.2,-8.69154933000001));
#284222=CARTESIAN_POINT('Ctrl Pts',(-5.76583777900006,15.2,-8.69255969400001));
#284223=CARTESIAN_POINT('Ctrl Pts',(-5.76673014200006,15.2,-8.69357555700002));
#284224=CARTESIAN_POINT('Ctrl Pts',(-5.76762905500006,15.2,-8.69459689400001));
#284225=CARTESIAN_POINT('Ctrl Pts',(-5.76853451500006,15.2,-8.69562367700001));
#284226=CARTESIAN_POINT('Ctrl Pts',(-5.76944652100006,15.2,-8.69665588300002));
#284227=CARTESIAN_POINT('Ctrl Pts',(-5.77036506700006,15.2,-8.69769348400002));
#284228=CARTESIAN_POINT('Ctrl Pts',(-5.77129015400006,15.2,-8.69873645500002));
#284229=CARTESIAN_POINT('Ctrl Pts',(-5.77222177600006,15.2,-8.69978477000002));
#284230=CARTESIAN_POINT('Ctrl Pts',(-5.77315993200005,15.2,-8.70083840400002));
#284231=CARTESIAN_POINT('Ctrl Pts',(-5.77410461900006,15.2,-8.70189733200002));
#284232=CARTESIAN_POINT('Ctrl Pts',(-5.77505583400006,15.2,-8.70296152800002));
#284233=CARTESIAN_POINT('Ctrl Pts',(-5.77601357300006,15.2,-8.70403096700001));
#284234=CARTESIAN_POINT('Ctrl Pts',(-5.77697783600006,15.2,-8.70510562400002));
#284235=CARTESIAN_POINT('Ctrl Pts',(-5.77794861800006,15.2,-8.70618547500002));
#284236=CARTESIAN_POINT('Ctrl Pts',(-5.77892591700006,15.2,-8.70727049300001));
#284237=CARTESIAN_POINT('Ctrl Pts',(-5.77990973100006,15.2,-8.70836065500002));
#284238=CARTESIAN_POINT('Ctrl Pts',(-5.78090005400006,15.2,-8.70945593700002));
#284239=CARTESIAN_POINT('Ctrl Pts',(-5.78189688700006,15.2,-8.71055631200001));
#284240=CARTESIAN_POINT('Ctrl Pts',(-5.78290022600005,15.2,-8.71166175800001));
#284241=CARTESIAN_POINT('Ctrl Pts',(-5.78391006700006,15.2,-8.71277225000001));
#284242=CARTESIAN_POINT('Ctrl Pts',(-5.78492640800006,15.2,-8.71388776300002));
#284243=CARTESIAN_POINT('Ctrl Pts',(-5.78594924700006,15.2,-8.71500827300002));
#284244=CARTESIAN_POINT('Ctrl Pts',(-5.78697858000006,15.2,-8.71613375700001));
#284245=CARTESIAN_POINT('Ctrl Pts',(-5.78801440500006,15.2,-8.71726418900002));
#284246=CARTESIAN_POINT('Ctrl Pts',(-5.78905671900006,15.2,-8.71839954800001));
#284247=CARTESIAN_POINT('Ctrl Pts',(-5.79010551900006,15.2,-8.71953980900001));
#284248=CARTESIAN_POINT('Ctrl Pts',(-5.79116080300006,15.2,-8.72068494800001));
#284249=CARTESIAN_POINT('Ctrl Pts',(-5.79222256600006,15.2,-8.72183494100002));
#284250=CARTESIAN_POINT('Ctrl Pts',(-5.79329080800006,15.2,-8.72298976600002));
#284251=CARTESIAN_POINT('Ctrl Pts',(-5.79436552400006,15.2,-8.72414939900001));
#284252=CARTESIAN_POINT('Ctrl Pts',(-5.79544671200006,15.2,-8.72531381700002));
#284253=CARTESIAN_POINT('Ctrl Pts',(-5.79653437000006,15.2,-8.72648299600002));
#284254=CARTESIAN_POINT('Ctrl Pts',(-5.79762849300006,15.2,-8.72765691300001));
#284255=CARTESIAN_POINT('Ctrl Pts',(-5.79872908000006,15.2,-8.72883554600002));
#284256=CARTESIAN_POINT('Ctrl Pts',(-5.79983612800006,15.2,-8.73001887100001));
#284257=CARTESIAN_POINT('Ctrl Pts',(-5.80094963500006,15.2,-8.73120686600002));
#284258=CARTESIAN_POINT('Ctrl Pts',(-5.80206959600006,15.2,-8.73239950900001));
#284259=CARTESIAN_POINT('Ctrl Pts',(-5.80319600900006,15.2,-8.73359677600002));
#284260=CARTESIAN_POINT('Ctrl Pts',(-5.80432887200006,15.2,-8.73479864500002));
#284261=CARTESIAN_POINT('Ctrl Pts',(-5.80546818100006,15.2,-8.73600509300001));
#284262=CARTESIAN_POINT('Ctrl Pts',(-5.80661393400006,15.2,-8.73721609800001));
#284263=CARTESIAN_POINT('Ctrl Pts',(-5.80776612900006,15.2,-8.73843163900002));
#284264=CARTESIAN_POINT('Ctrl Pts',(-5.80892476100006,15.2,-8.73965169300002));
#284265=CARTESIAN_POINT('Ctrl Pts',(-5.81008982800006,15.2,-8.74087623600002));
#284266=CARTESIAN_POINT('Ctrl Pts',(-5.81126132800006,15.2,-8.74210524800001));
#284267=CARTESIAN_POINT('Ctrl Pts',(-5.81243925700006,15.2,-8.74333870700001));
#284268=CARTESIAN_POINT('Ctrl Pts',(-5.81362361300005,15.2,-8.74457659100001));
#284269=CARTESIAN_POINT('Ctrl Pts',(-5.81481439300005,15.2,-8.74581887800002));
#284270=CARTESIAN_POINT('Ctrl Pts',(-5.81601159400006,15.2,-8.74706554600002));
#284271=CARTESIAN_POINT('Ctrl Pts',(-5.81721521200006,15.2,-8.74831657400001));
#284272=CARTESIAN_POINT('Ctrl Pts',(-5.81842524600006,15.2,-8.74957194100002));
#284273=CARTESIAN_POINT('Ctrl Pts',(-5.81964169300006,15.2,-8.75083162500001));
#284274=CARTESIAN_POINT('Ctrl Pts',(-5.82086454900006,15.2,-8.75209560300001));
#284275=CARTESIAN_POINT('Ctrl Pts',(-5.82209381200006,15.2,-8.75336385700002));
#284276=CARTESIAN_POINT('Ctrl Pts',(-5.82332948000006,15.2,-8.75463636300001));
#284277=CARTESIAN_POINT('Ctrl Pts',(-5.82457154700006,15.2,-8.75591310200001));
#284278=CARTESIAN_POINT('Ctrl Pts',(-5.82582001200006,15.2,-8.75719405100002));
#284279=CARTESIAN_POINT('Ctrl Pts',(-5.82707487300006,15.2,-8.75847919000002));
#284280=CARTESIAN_POINT('Ctrl Pts',(-5.82833612700006,15.2,-8.75976849900002));
#284281=CARTESIAN_POINT('Ctrl Pts',(-5.82960377000005,15.2,-8.76106195500002));
#284282=CARTESIAN_POINT('Ctrl Pts',(-5.83087780000006,15.2,-8.76235953900002));
#284283=CARTESIAN_POINT('Ctrl Pts',(-5.83215821300006,15.2,-8.76366123100001));
#284284=CARTESIAN_POINT('Ctrl Pts',(-5.83344500700006,15.2,-8.76496700800002));
#284285=CARTESIAN_POINT('Ctrl Pts',(-5.83473817900006,15.2,-8.76627685200001));
#284286=CARTESIAN_POINT('Ctrl Pts',(-5.83603772700005,15.2,-8.76759074100002));
#284287=CARTESIAN_POINT('Ctrl Pts',(-5.83734364600006,15.2,-8.76890865500001));
#284288=CARTESIAN_POINT('Ctrl Pts',(-5.83865593500006,15.2,-8.77023057400002));
#284289=CARTESIAN_POINT('Ctrl Pts',(-5.83997459000006,15.2,-8.77155647700001));
#284290=CARTESIAN_POINT('Ctrl Pts',(-5.84129960800006,15.2,-8.77288634600001));
#284291=CARTESIAN_POINT('Ctrl Pts',(-5.84263098700006,15.2,-8.77422015900001));
#284292=CARTESIAN_POINT('Ctrl Pts',(-5.84396872500006,15.2,-8.77555789600001));
#284293=CARTESIAN_POINT('Ctrl Pts',(-5.84531281700006,15.2,-8.77689953800001));
#284294=CARTESIAN_POINT('Ctrl Pts',(-5.84666326000006,15.2,-8.77824506500002));
#284295=CARTESIAN_POINT('Ctrl Pts',(-5.84802005400006,15.2,-8.77959445700002));
#284296=CARTESIAN_POINT('Ctrl Pts',(-5.84938319300006,15.2,-8.78094769400001));
#284297=CARTESIAN_POINT('Ctrl Pts',(-5.85075267500006,15.2,-8.78230475600001));
#284298=CARTESIAN_POINT('Ctrl Pts',(-5.85212849700006,15.2,-8.78366562400002));
#284299=CARTESIAN_POINT('Ctrl Pts',(-5.85351065700006,15.2,-8.78503028000001));
#284300=CARTESIAN_POINT('Ctrl Pts',(-5.85489915200006,15.2,-8.78639870300002));
#284301=CARTESIAN_POINT('Ctrl Pts',(-5.85629397700006,15.2,-8.78777087300002));
#284302=CARTESIAN_POINT('Ctrl Pts',(-5.85769513200006,15.2,-8.78914677200001));
#284303=CARTESIAN_POINT('Ctrl Pts',(-5.85910261300006,15.2,-8.79052638100001));
#284304=CARTESIAN_POINT('Ctrl Pts',(-5.86051641600006,15.2,-8.79190968000002));
#284305=CARTESIAN_POINT('Ctrl Pts',(-5.86193653900006,15.2,-8.79329665000002));
#284306=CARTESIAN_POINT('Ctrl Pts',(-5.86336298000006,15.2,-8.79468727200001));
#284307=CARTESIAN_POINT('Ctrl Pts',(-5.86479573400006,15.2,-8.79608152700002));
#284308=CARTESIAN_POINT('Ctrl Pts',(-5.86623479900005,15.2,-8.79747939600002));
#284309=CARTESIAN_POINT('Ctrl Pts',(-5.86768017200006,15.2,-8.79888086200001));
#284310=CARTESIAN_POINT('Ctrl Pts',(-5.86913185000006,15.2,-8.80028590300002));
#284311=CARTESIAN_POINT('Ctrl Pts',(-5.87058983200006,15.2,-8.80169450300002));
#284312=CARTESIAN_POINT('Ctrl Pts',(-5.87205411200006,15.2,-8.80310664200002));
#284313=CARTESIAN_POINT('Ctrl Pts',(-5.87352468900006,15.2,-8.80452230300002));
#284314=CARTESIAN_POINT('Ctrl Pts',(-5.87500155900006,15.2,-8.80594146500002));
#284315=CARTESIAN_POINT('Ctrl Pts',(-5.87648472000006,15.2,-8.80736411100001));
#284316=CARTESIAN_POINT('Ctrl Pts',(-5.87797416900006,15.2,-8.80879022300002));
#284317=CARTESIAN_POINT('Ctrl Pts',(-5.87946990200006,15.2,-8.81021978100001));
#284318=CARTESIAN_POINT('Ctrl Pts',(-5.88097191600006,15.2,-8.81165276900001));
#284319=CARTESIAN_POINT('Ctrl Pts',(-5.88248021000005,15.2,-8.81308916900002));
#284320=CARTESIAN_POINT('Ctrl Pts',(-5.88399477900006,15.2,-8.81452896000001));
#284321=CARTESIAN_POINT('Ctrl Pts',(-5.88551562100006,15.2,-8.81597212600001));
#284322=CARTESIAN_POINT('Ctrl Pts',(-5.88704273400006,15.2,-8.81741864800002));
#284323=CARTESIAN_POINT('Ctrl Pts',(-5.88857611200006,15.2,-8.81886851000001));
#284324=CARTESIAN_POINT('Ctrl Pts',(-5.89011575500006,15.2,-8.82032169100002));
#284325=CARTESIAN_POINT('Ctrl Pts',(-5.89166165900005,15.2,-8.82177817600001));
#284326=CARTESIAN_POINT('Ctrl Pts',(-5.89321382100006,15.2,-8.82323794600002));
#284327=CARTESIAN_POINT('Ctrl Pts',(-5.89477223700006,15.2,-8.82470098400002));
#284328=CARTESIAN_POINT('Ctrl Pts',(-5.89633690700006,15.2,-8.82616727000002));
#284329=CARTESIAN_POINT('Ctrl Pts',(-5.89790782500006,15.2,-8.82763679000002));
#284330=CARTESIAN_POINT('Ctrl Pts',(-5.89948498900006,15.2,-8.82910952300002));
#284331=CARTESIAN_POINT('Ctrl Pts',(-5.90106839700006,15.2,-8.83058545500001));
#284332=CARTESIAN_POINT('Ctrl Pts',(-5.90265804300006,15.2,-8.83206456600002));
#284333=CARTESIAN_POINT('Ctrl Pts',(-5.90425392900006,15.2,-8.83354683900002));
#284334=CARTESIAN_POINT('Ctrl Pts',(-5.90585604700006,15.2,-8.83503225700002));
#284335=CARTESIAN_POINT('Ctrl Pts',(-5.90746439700006,15.2,-8.83652080200001));
#284336=CARTESIAN_POINT('Ctrl Pts',(-5.90907897600006,15.2,-8.83801246000001));
#284337=CARTESIAN_POINT('Ctrl Pts',(-5.91069977900006,15.2,-8.83950721000001));
#284338=CARTESIAN_POINT('Ctrl Pts',(-5.91232680500006,15.2,-8.84100503500001));
#284339=CARTESIAN_POINT('Ctrl Pts',(-5.91396005000006,15.2,-8.84250592100001));
#284340=CARTESIAN_POINT('Ctrl Pts',(-5.91559951200006,15.2,-8.84400984900001));
#284341=CARTESIAN_POINT('Ctrl Pts',(-5.91724518600006,15.2,-8.84551680200002));
#284342=CARTESIAN_POINT('Ctrl Pts',(-5.91889707100006,15.2,-8.84702676400002));
#284343=CARTESIAN_POINT('Ctrl Pts',(-5.92055516300006,15.2,-8.84853971800002));
#284344=CARTESIAN_POINT('Ctrl Pts',(-5.92221945900006,15.2,-8.85005564700002));
#284345=CARTESIAN_POINT('Ctrl Pts',(-5.92388995600006,15.2,-8.85157453400002));
#284346=CARTESIAN_POINT('Ctrl Pts',(-5.92556665300005,15.2,-8.85309636200001));
#284347=CARTESIAN_POINT('Ctrl Pts',(-5.92724954300006,15.2,-8.85462111500001));
#284348=CARTESIAN_POINT('Ctrl Pts',(-5.92893862600006,15.2,-8.85614877700002));
#284349=CARTESIAN_POINT('Ctrl Pts',(-5.93063389800006,15.2,-8.85767933100002));
#284350=CARTESIAN_POINT('Ctrl Pts',(-5.93233535700006,15.2,-8.85921276000002));
#284351=CARTESIAN_POINT('Ctrl Pts',(-5.93404299900006,15.2,-8.86074904800001));
#284352=CARTESIAN_POINT('Ctrl Pts',(-5.93575682000006,15.2,-8.86228817900001));
#284353=CARTESIAN_POINT('Ctrl Pts',(-5.93747681900005,15.2,-8.86383013700001));
#284354=CARTESIAN_POINT('Ctrl Pts',(-5.93920299300006,15.2,-8.86537490400002));
#284355=CARTESIAN_POINT('Ctrl Pts',(-5.94093533700006,15.2,-8.86692246600001));
#284356=CARTESIAN_POINT('Ctrl Pts',(-5.94267384900006,15.2,-8.86847280400002));
#284357=CARTESIAN_POINT('Ctrl Pts',(-5.94441852600006,15.2,-8.87002590600002));
#284358=CARTESIAN_POINT('Ctrl Pts',(-5.94616936500006,15.2,-8.87158175200002));
#284359=CARTESIAN_POINT('Ctrl Pts',(-5.94792636200006,15.2,-8.87314032800001));
#284360=CARTESIAN_POINT('Ctrl Pts',(-5.94968951600006,15.2,-8.87470161900002));
#284361=CARTESIAN_POINT('Ctrl Pts',(-5.95145882200006,15.2,-8.87626560600001));
#284362=CARTESIAN_POINT('Ctrl Pts',(-5.95323427900006,15.2,-8.87783227600002));
#284363=CARTESIAN_POINT('Ctrl Pts',(-5.95501588200006,15.2,-8.87940161100002));
#284364=CARTESIAN_POINT('Ctrl Pts',(-5.95680362900006,15.2,-8.88097359800001));
#284365=CARTESIAN_POINT('Ctrl Pts',(-5.95859751600006,15.2,-8.88254821900002));
#284366=CARTESIAN_POINT('Ctrl Pts',(-5.96039754200006,15.2,-8.88412545900002));
#284367=CARTESIAN_POINT('Ctrl Pts',(-5.96220370200006,15.2,-8.88570530200001));
#284368=CARTESIAN_POINT('Ctrl Pts',(-5.96401599300005,15.2,-8.88728773400001));
#284369=CARTESIAN_POINT('Ctrl Pts',(-5.96583441200006,15.2,-8.88887273700002));
#284370=CARTESIAN_POINT('Ctrl Pts',(-5.96765895700006,15.2,-8.89046029700001));
#284371=CARTESIAN_POINT('Ctrl Pts',(-5.96948962500006,15.2,-8.89205039900002));
#284372=CARTESIAN_POINT('Ctrl Pts',(-5.97132641200006,15.2,-8.89364302600002));
#284373=CARTESIAN_POINT('Ctrl Pts',(-5.97316931400006,15.2,-8.89523816500001));
#284374=CARTESIAN_POINT('Ctrl Pts',(-5.97501833000006,15.2,-8.89683579900002));
#284375=CARTESIAN_POINT('Ctrl Pts',(-5.97687345600006,15.2,-8.89843591300002));
#284376=CARTESIAN_POINT('Ctrl Pts',(-5.97873468900006,15.2,-8.90003849100001));
#284377=CARTESIAN_POINT('Ctrl Pts',(-5.98060202600006,15.2,-8.90164352000001));
#284378=CARTESIAN_POINT('Ctrl Pts',(-5.98247546400006,15.2,-8.90325098400002));
#284379=CARTESIAN_POINT('Ctrl Pts',(-5.98435500000006,15.2,-8.90486086600001));
#284380=CARTESIAN_POINT('Ctrl Pts',(-5.98624062900006,15.2,-8.90647315300001));
#284381=CARTESIAN_POINT('Ctrl Pts',(-5.98813235200006,15.2,-8.90808783100002));
#284382=CARTESIAN_POINT('Ctrl Pts',(-5.99003016200006,15.2,-8.90970488200002));
#284383=CARTESIAN_POINT('Ctrl Pts',(-5.99193405800006,15.2,-8.91132429300002));
#284384=CARTESIAN_POINT('Ctrl Pts',(-5.99384403600006,15.2,-8.91294604900001));
#284385=CARTESIAN_POINT('Ctrl Pts',(-5.99576009400006,15.2,-8.91457013600002));
#284386=CARTESIAN_POINT('Ctrl Pts',(-5.99768222800006,15.2,-8.91619653700002));
#284387=CARTESIAN_POINT('Ctrl Pts',(-5.99961043400006,15.2,-8.91782524000002));
#284388=CARTESIAN_POINT('Ctrl Pts',(-6.00154471100006,15.2,-8.91945622800002));
#284389=CARTESIAN_POINT('Ctrl Pts',(-6.00348505500006,15.2,-8.92108948700002));
#284390=CARTESIAN_POINT('Ctrl Pts',(-6.00543146200006,15.2,-8.92272500300002));
#284391=CARTESIAN_POINT('Ctrl Pts',(-6.00738393100006,15.2,-8.92436276200002));
#284392=CARTESIAN_POINT('Ctrl Pts',(-6.00934245600006,15.2,-8.92600274700002));
#284393=CARTESIAN_POINT('Ctrl Pts',(-6.01130703700006,15.2,-8.92764494600002));
#284394=CARTESIAN_POINT('Ctrl Pts',(-6.01327766800006,15.2,-8.92928934400001));
#284395=CARTESIAN_POINT('Ctrl Pts',(-6.01525434800006,15.2,-8.93093592700002));
#284396=CARTESIAN_POINT('Ctrl Pts',(-6.01723707400006,15.2,-8.93258467900001));
#284397=CARTESIAN_POINT('Ctrl Pts',(-6.01922584100006,15.2,-8.93423558600002));
#284398=CARTESIAN_POINT('Ctrl Pts',(-6.02122064700006,15.2,-8.93588863500002));
#284399=CARTESIAN_POINT('Ctrl Pts',(-6.02322148900006,15.2,-8.93754381100001));
#284400=CARTESIAN_POINT('Ctrl Pts',(-6.02522836400006,15.2,-8.93920110000002));
#284401=CARTESIAN_POINT('Ctrl Pts',(-6.02724126900006,15.2,-8.94086048800002));
#284402=CARTESIAN_POINT('Ctrl Pts',(-6.02926019900006,15.2,-8.94252196100001));
#284403=CARTESIAN_POINT('Ctrl Pts',(-6.03128515400006,15.2,-8.94418550400001));
#284404=CARTESIAN_POINT('Ctrl Pts',(-6.03331612900006,15.2,-8.94585110500002));
#284405=CARTESIAN_POINT('Ctrl Pts',(-6.03535312000006,15.2,-8.94751874800002));
#284406=CARTESIAN_POINT('Ctrl Pts',(-6.03739612600006,15.2,-8.94918841900001));
#284407=CARTESIAN_POINT('Ctrl Pts',(-6.03944514200006,15.2,-8.95086010500002));
#284408=CARTESIAN_POINT('Ctrl Pts',(-6.04150016700006,15.2,-8.95253379300001));
#284409=CARTESIAN_POINT('Ctrl Pts',(-6.04356119600006,15.2,-8.95420946700002));
#284410=CARTESIAN_POINT('Ctrl Pts',(-6.04562822600006,15.2,-8.95588711400002));
#284411=CARTESIAN_POINT('Ctrl Pts',(-6.04770125400006,15.2,-8.95756672100001));
#284412=CARTESIAN_POINT('Ctrl Pts',(-6.04978027800006,15.2,-8.95924827300002));
#284413=CARTESIAN_POINT('Ctrl Pts',(-6.05186529400005,15.2,-8.96093175800001));
#284414=CARTESIAN_POINT('Ctrl Pts',(-6.05395629800006,15.2,-8.96261716200002));
#284415=CARTESIAN_POINT('Ctrl Pts',(-6.05605328900006,15.2,-8.96430447000002));
#284416=CARTESIAN_POINT('Ctrl Pts',(-6.05815626100005,15.2,-8.96599367000002));
#284417=CARTESIAN_POINT('Ctrl Pts',(-6.06026521300006,15.2,-8.96768474600002));
#284418=CARTESIAN_POINT('Ctrl Pts',(-6.06238014200006,15.2,-8.96937768800001));
#284419=CARTESIAN_POINT('Ctrl Pts',(-6.06450104400006,15.2,-8.97107248000001));
#284420=CARTESIAN_POINT('Ctrl Pts',(-6.06662791600006,15.2,-8.97276910900001));
#284421=CARTESIAN_POINT('Ctrl Pts',(-6.06876075400006,15.2,-8.97446756300001));
#284422=CARTESIAN_POINT('Ctrl Pts',(-6.07089955600006,15.2,-8.97616782700002));
#284423=CARTESIAN_POINT('Ctrl Pts',(-6.07304431900006,15.2,-8.97786988800001));
#284424=CARTESIAN_POINT('Ctrl Pts',(-6.07519504000006,15.2,-8.97957373400001));
#284425=CARTESIAN_POINT('Ctrl Pts',(-6.07735171400006,15.2,-8.98127934900002));
#284426=CARTESIAN_POINT('Ctrl Pts',(-6.07951433900006,15.2,-8.98298672300001));
#284427=CARTESIAN_POINT('Ctrl Pts',(-6.08168291200006,15.2,-8.98469584100001));
#284428=CARTESIAN_POINT('Ctrl Pts',(-6.08385743000006,15.2,-8.98640669100002));
#284429=CARTESIAN_POINT('Ctrl Pts',(-6.08603788900006,15.2,-8.98811925800001));
#284430=CARTESIAN_POINT('Ctrl Pts',(-6.08822428600006,15.2,-8.98983353000002));
#284431=CARTESIAN_POINT('Ctrl Pts',(-6.09041662000006,15.2,-8.99154949500002));
#284432=CARTESIAN_POINT('Ctrl Pts',(-6.09261488400006,15.2,-8.99326713800002));
#284433=CARTESIAN_POINT('Ctrl Pts',(-6.09481907700006,15.2,-8.99498644800002));
#284434=CARTESIAN_POINT('Ctrl Pts',(-6.09702919700006,15.2,-8.99670741000002));
#284435=CARTESIAN_POINT('Ctrl Pts',(-6.09924523800006,15.2,-8.99843001200002));
#284436=CARTESIAN_POINT('Ctrl Pts',(-6.10146719900006,15.2,-9.00015424200001));
#284437=CARTESIAN_POINT('Ctrl Pts',(-6.10369507600006,15.2,-9.00188008700002));
#284438=CARTESIAN_POINT('Ctrl Pts',(-6.10592886600006,15.2,-9.00360753300001));
#284439=CARTESIAN_POINT('Ctrl Pts',(-6.10816856500006,15.2,-9.00533656900001));
#284440=CARTESIAN_POINT('Ctrl Pts',(-6.11041417200005,15.2,-9.00706718000002));
#284441=CARTESIAN_POINT('Ctrl Pts',(-6.11266568000006,15.2,-9.00879935600001));
#284442=CARTESIAN_POINT('Ctrl Pts',(-6.11492309000006,15.2,-9.01053308200002));
#284443=CARTESIAN_POINT('Ctrl Pts',(-6.11718639600006,15.2,-9.01226834500001));
#284444=CARTESIAN_POINT('Ctrl Pts',(-6.11945559600006,15.2,-9.01400513500001));
#284445=CARTESIAN_POINT('Ctrl Pts',(-6.12173068600006,15.2,-9.01574343800002));
#284446=CARTESIAN_POINT('Ctrl Pts',(-6.12401166400006,15.2,-9.01748324100001));
#284447=CARTESIAN_POINT('Ctrl Pts',(-6.12629852600006,15.2,-9.01922453300001));
#284448=CARTESIAN_POINT('Ctrl Pts',(-6.12859126900006,15.2,-9.02096729900002));
#284449=CARTESIAN_POINT('Ctrl Pts',(-6.13088988900006,15.2,-9.02271152900001));
#284450=CARTESIAN_POINT('Ctrl Pts',(-6.13319438500006,15.2,-9.02445720900002));
#284451=CARTESIAN_POINT('Ctrl Pts',(-6.13550475100006,15.2,-9.02620432800001));
#284452=CARTESIAN_POINT('Ctrl Pts',(-6.13782098400006,15.2,-9.02795287300002));
#284453=CARTESIAN_POINT('Ctrl Pts',(-6.14014308400006,15.2,-9.02970283200002));
#284454=CARTESIAN_POINT('Ctrl Pts',(-6.14247104500006,15.2,-9.03145419100002));
#284455=CARTESIAN_POINT('Ctrl Pts',(-6.14480486400006,15.2,-9.03320694000002));
#284456=CARTESIAN_POINT('Ctrl Pts',(-6.14714453800006,15.2,-9.03496106700001));
#284457=CARTESIAN_POINT('Ctrl Pts',(-6.14949006400006,15.2,-9.03671655700002));
#284458=CARTESIAN_POINT('Ctrl Pts',(-6.15184143900006,15.2,-9.03847340000001));
#284459=CARTESIAN_POINT('Ctrl Pts',(-6.15419866000006,15.2,-9.04023158300001));
#284460=CARTESIAN_POINT('Ctrl Pts',(-6.15656172200006,15.2,-9.04199109600002));
#284461=CARTESIAN_POINT('Ctrl Pts',(-6.15893062400006,15.2,-9.04375192400002));
#284462=CARTESIAN_POINT('Ctrl Pts',(-6.16130536200005,15.2,-9.04551405600002));
#284463=CARTESIAN_POINT('Ctrl Pts',(-6.16368593200006,15.2,-9.04727748100001));
#284464=CARTESIAN_POINT('Ctrl Pts',(-6.16607233200006,15.2,-9.04904218600001));
#284465=CARTESIAN_POINT('Ctrl Pts',(-6.16846455700006,15.2,-9.05080815900002));
#284466=CARTESIAN_POINT('Ctrl Pts',(-6.17086260700006,15.2,-9.05257538800001));
#284467=CARTESIAN_POINT('Ctrl Pts',(-6.17326647500006,15.2,-9.05434386300002));
#284468=CARTESIAN_POINT('Ctrl Pts',(-6.17567615900006,15.2,-9.05611357000002));
#284469=CARTESIAN_POINT('Ctrl Pts',(-6.17809165700006,15.2,-9.05788449800001));
#284470=CARTESIAN_POINT('Ctrl Pts',(-6.18051296500005,15.2,-9.05965663400002));
#284471=CARTESIAN_POINT('Ctrl Pts',(-6.18294008000006,15.2,-9.06142996800002));
#284472=CARTESIAN_POINT('Ctrl Pts',(-6.18537299700006,15.2,-9.06320448700002));
#284473=CARTESIAN_POINT('Ctrl Pts',(-6.18781171500006,15.2,-9.06498018100002));
#284474=CARTESIAN_POINT('Ctrl Pts',(-6.19025623000006,15.2,-9.06675703600002));
#284475=CARTESIAN_POINT('Ctrl Pts',(-6.19270653900006,15.2,-9.06853504200001));
#284476=CARTESIAN_POINT('Ctrl Pts',(-6.19516263900006,15.2,-9.07031418600001));
#284477=CARTESIAN_POINT('Ctrl Pts',(-6.19762452500006,15.2,-9.07209445800002));
#284478=CARTESIAN_POINT('Ctrl Pts',(-6.20009219500006,15.2,-9.07387584600002));
#284479=CARTESIAN_POINT('Ctrl Pts',(-6.20256564600006,15.2,-9.07565833800002));
#284480=CARTESIAN_POINT('Ctrl Pts',(-6.20504487400006,15.2,-9.07744192200001));
#284481=CARTESIAN_POINT('Ctrl Pts',(-6.20752987700006,15.2,-9.07922658700001));
#284482=CARTESIAN_POINT('Ctrl Pts',(-6.21002065000006,15.2,-9.08101232300002));
#284483=CARTESIAN_POINT('Ctrl Pts',(-6.21251719100006,15.2,-9.08279911600001));
#284484=CARTESIAN_POINT('Ctrl Pts',(-6.21501949600006,15.2,-9.08458695700002));
#284485=CARTESIAN_POINT('Ctrl Pts',(-6.21752756200006,15.2,-9.08637583200001));
#284486=CARTESIAN_POINT('Ctrl Pts',(-6.22004138600006,15.2,-9.08816573200001));
#284487=CARTESIAN_POINT('Ctrl Pts',(-6.22256096500006,15.2,-9.08995664500001));
#284488=CARTESIAN_POINT('Ctrl Pts',(-6.22508629500006,15.2,-9.09174855900002));
#284489=CARTESIAN_POINT('Ctrl Pts',(-6.22761737300006,15.2,-9.09354146400002));
#284490=CARTESIAN_POINT('Ctrl Pts',(-6.23015419600006,15.2,-9.09533534700002));
#284491=CARTESIAN_POINT('Ctrl Pts',(-6.23269675900006,15.2,-9.09713019900002));
#284492=CARTESIAN_POINT('Ctrl Pts',(-6.23524506100006,15.2,-9.09892600700001));
#284493=CARTESIAN_POINT('Ctrl Pts',(-6.23779909800006,15.2,-9.10072276100001));
#284494=CARTESIAN_POINT('Ctrl Pts',(-6.24035886600006,15.2,-9.10252044800002));
#284495=CARTESIAN_POINT('Ctrl Pts',(-6.24292436400006,15.2,-9.10431905900002));
#284496=CARTESIAN_POINT('Ctrl Pts',(-6.24549558500005,15.2,-9.10611858200001));
#284497=CARTESIAN_POINT('Ctrl Pts',(-6.24807252900006,15.2,-9.10791900700002));
#284498=CARTESIAN_POINT('Ctrl Pts',(-6.25065519100006,15.2,-9.10972032100002));
#284499=CARTESIAN_POINT('Ctrl Pts',(-6.25324356800006,15.2,-9.11152251400001));
#284500=CARTESIAN_POINT('Ctrl Pts',(-6.25583765700005,15.2,-9.11332557600002));
#284501=CARTESIAN_POINT('Ctrl Pts',(-6.25843745500006,15.2,-9.11512949500001));
#284502=CARTESIAN_POINT('Ctrl Pts',(-6.26104295800006,15.2,-9.11693426000001));
#284503=CARTESIAN_POINT('Ctrl Pts',(-6.26365416200006,15.2,-9.11873986000002));
#284504=CARTESIAN_POINT('Ctrl Pts',(-6.26627106600006,15.2,-9.12054628500002));
#284505=CARTESIAN_POINT('Ctrl Pts',(-6.26889366400006,15.2,-9.12235352300002));
#284506=CARTESIAN_POINT('Ctrl Pts',(-6.27152195600006,15.2,-9.12416156500001));
#284507=CARTESIAN_POINT('Ctrl Pts',(-6.27415593500006,15.2,-9.12597039800002));
#284508=CARTESIAN_POINT('Ctrl Pts',(-6.27679559900006,15.2,-9.12778001300002));
#284509=CARTESIAN_POINT('Ctrl Pts',(-6.27944094700006,15.2,-9.12959039800001));
#284510=CARTESIAN_POINT('Ctrl Pts',(-6.28209197200006,15.2,-9.13140154300002));
#284511=CARTESIAN_POINT('Ctrl Pts',(-6.28474867400006,15.2,-9.13321343700002));
#284512=CARTESIAN_POINT('Ctrl Pts',(-6.28741104800006,15.2,-9.13502606900002));
#284513=CARTESIAN_POINT('Ctrl Pts',(-6.29007909100006,15.2,-9.13683942900001));
#284514=CARTESIAN_POINT('Ctrl Pts',(-6.29275279900006,15.2,-9.13865350600001));
#284515=CARTESIAN_POINT('Ctrl Pts',(-6.29543217000006,15.2,-9.14046829000002));
#284516=CARTESIAN_POINT('Ctrl Pts',(-6.29811719900006,15.2,-9.14228377000001));
#284517=CARTESIAN_POINT('Ctrl Pts',(-6.30080788400006,15.2,-9.14409993500002));
#284518=CARTESIAN_POINT('Ctrl Pts',(-6.30350422100006,15.2,-9.14591677500002));
#284519=CARTESIAN_POINT('Ctrl Pts',(-6.30620620800006,15.2,-9.14773428000002));
#284520=CARTESIAN_POINT('Ctrl Pts',(-6.30891384000006,15.2,-9.14955243900001));
#284521=CARTESIAN_POINT('Ctrl Pts',(-6.31162711400005,15.2,-9.15137124000001));
#284522=CARTESIAN_POINT('Ctrl Pts',(-6.31434602800006,15.2,-9.15319067500001));
#284523=CARTESIAN_POINT('Ctrl Pts',(-6.31707057700006,15.2,-9.15501073400002));
#284524=CARTESIAN_POINT('Ctrl Pts',(-6.31980075800006,15.2,-9.15683140300001));
#284525=CARTESIAN_POINT('Ctrl Pts',(-6.32253656800006,15.2,-9.15865267500001));
#284526=CARTESIAN_POINT('Ctrl Pts',(-6.32527800500006,15.2,-9.16047453800001));
#284527=CARTESIAN_POINT('Ctrl Pts',(-6.32802506300005,15.2,-9.16229698300001));
#284528=CARTESIAN_POINT('Ctrl Pts',(-6.33077774100006,15.2,-9.16411999900001));
#284529=CARTESIAN_POINT('Ctrl Pts',(-6.33353603400006,15.2,-9.16594357600001));
#284530=CARTESIAN_POINT('Ctrl Pts',(-6.33629993900006,15.2,-9.16776770200002));
#284531=CARTESIAN_POINT('Ctrl Pts',(-6.33906945400006,15.2,-9.16959237000002));
#284532=CARTESIAN_POINT('Ctrl Pts',(-6.34184457400006,15.2,-9.17141756700002));
#284533=CARTESIAN_POINT('Ctrl Pts',(-6.34462529700006,15.2,-9.17324328400002));
#284534=CARTESIAN_POINT('Ctrl Pts',(-6.34741161800005,15.2,-9.17506951100002));
#284535=CARTESIAN_POINT('Ctrl Pts',(-6.35020353500006,15.2,-9.17689623700002));
#284536=CARTESIAN_POINT('Ctrl Pts',(-6.35300104500006,15.2,-9.17872345400001));
#284537=CARTESIAN_POINT('Ctrl Pts',(-6.35580414300006,15.2,-9.18055114900002));
#284538=CARTESIAN_POINT('Ctrl Pts',(-6.35861282700006,15.2,-9.18237931400002));
#284539=CARTESIAN_POINT('Ctrl Pts',(-6.36142709400006,15.2,-9.18420793900001));
#284540=CARTESIAN_POINT('Ctrl Pts',(-6.36424693800006,15.2,-9.18603701200002));
#284541=CARTESIAN_POINT('Ctrl Pts',(-6.36707236000006,15.2,-9.18786652500001));
#284542=CARTESIAN_POINT('Ctrl Pts',(-6.36990335200006,15.2,-9.18969646800001));
#284543=CARTESIAN_POINT('Ctrl Pts',(-6.37273991300006,15.2,-9.19152682900001));
#284544=CARTESIAN_POINT('Ctrl Pts',(-6.37558204100006,15.2,-9.19335760100001));
#284545=CARTESIAN_POINT('Ctrl Pts',(-6.37842973000006,15.2,-9.19518877200002));
#284546=CARTESIAN_POINT('Ctrl Pts',(-6.38128297700006,15.2,-9.19702033200002));
#284547=CARTESIAN_POINT('Ctrl Pts',(-6.38414178100006,15.2,-9.19885227300002));
#284548=CARTESIAN_POINT('Ctrl Pts',(-6.38700613600006,15.2,-9.20068458400002));
#284549=CARTESIAN_POINT('Ctrl Pts',(-6.38987604000006,15.2,-9.20251725400002));
#284550=CARTESIAN_POINT('Ctrl Pts',(-6.39275149000006,15.2,-9.20435027600002));
#284551=CARTESIAN_POINT('Ctrl Pts',(-6.39563248000006,15.2,-9.20618363800001));
#284552=CARTESIAN_POINT('Ctrl Pts',(-6.39851901000006,15.2,-9.20801733000001));
#284553=CARTESIAN_POINT('Ctrl Pts',(-6.40141107500006,15.2,-9.20985134500001));
#284554=CARTESIAN_POINT('Ctrl Pts',(-6.40430867200006,15.2,-9.21168566900001));
#284555=CARTESIAN_POINT('Ctrl Pts',(-6.40721179700006,15.2,-9.21352029700002));
#284556=CARTESIAN_POINT('Ctrl Pts',(-6.41012044700005,15.2,-9.21535521600001));
#284557=CARTESIAN_POINT('Ctrl Pts',(-6.41303461900006,15.2,-9.21719041800002));
#284558=CARTESIAN_POINT('Ctrl Pts',(-6.41595430900006,15.2,-9.21902589200002));
#284559=CARTESIAN_POINT('Ctrl Pts',(-6.41887951300006,15.2,-9.22086163100002));
#284560=CARTESIAN_POINT('Ctrl Pts',(-6.42181023000005,15.2,-9.22269762200001));
#284561=CARTESIAN_POINT('Ctrl Pts',(-6.42474645500006,15.2,-9.22453385700001));
#284562=CARTESIAN_POINT('Ctrl Pts',(-6.42768818400006,15.2,-9.22637032800001));
#284563=CARTESIAN_POINT('Ctrl Pts',(-6.43063541500006,15.2,-9.22820702200001));
#284564=CARTESIAN_POINT('Ctrl Pts',(-6.43358814400006,15.2,-9.23004393300002));
#284565=CARTESIAN_POINT('Ctrl Pts',(-6.43654636800005,15.2,-9.23188105000002));
#284566=CARTESIAN_POINT('Ctrl Pts',(-6.43951008200006,15.2,-9.23371836400002));
#284567=CARTESIAN_POINT('Ctrl Pts',(-6.44247928500006,15.2,-9.23555586400001));
#284568=CARTESIAN_POINT('Ctrl Pts',(-6.44545397200006,15.2,-9.23739354200002));
#284569=CARTESIAN_POINT('Ctrl Pts',(-6.44843413900006,15.2,-9.23923138800001));
#284570=CARTESIAN_POINT('Ctrl Pts',(-6.45141978500006,15.2,-9.24106939400002));
#284571=CARTESIAN_POINT('Ctrl Pts',(-6.45441090500006,15.2,-9.24290754900002));
#284572=CARTESIAN_POINT('Ctrl Pts',(-6.45740749600006,15.2,-9.24474584400001));
#284573=CARTESIAN_POINT('Ctrl Pts',(-6.46040955400006,15.2,-9.24658427100002));
#284574=CARTESIAN_POINT('Ctrl Pts',(-6.46341707600006,15.2,-9.24842281800002));
#284575=CARTESIAN_POINT('Ctrl Pts',(-6.46643005900006,15.2,-9.25026147900001));
#284576=CARTESIAN_POINT('Ctrl Pts',(-6.46944849900006,15.2,-9.25210024200002));
#284577=CARTESIAN_POINT('Ctrl Pts',(-6.47247239300006,15.2,-9.25393910000002));
#284578=CARTESIAN_POINT('Ctrl Pts',(-6.47550173800005,15.2,-9.25577804100002));
#284579=CARTESIAN_POINT('Ctrl Pts',(-6.47853652900006,15.2,-9.25761705800002));
#284580=CARTESIAN_POINT('Ctrl Pts',(-6.48157676400006,15.2,-9.25945614200002));
#284581=CARTESIAN_POINT('Ctrl Pts',(-6.48462244000005,15.2,-9.26129528200001));
#284582=CARTESIAN_POINT('Ctrl Pts',(-6.48767355200006,15.2,-9.26313447100001));
#284583=CARTESIAN_POINT('Ctrl Pts',(-6.49073009700006,15.2,-9.26497369800002));
#284584=CARTESIAN_POINT('Ctrl Pts',(-6.49379207300006,15.2,-9.26681295500002));
#284585=CARTESIAN_POINT('Ctrl Pts',(-6.49685947500006,15.2,-9.26865223300002));
#284586=CARTESIAN_POINT('Ctrl Pts',(-6.49993230100006,15.2,-9.27049152200001));
#284587=CARTESIAN_POINT('Ctrl Pts',(-6.50301054600006,15.2,-9.27233081400002));
#284588=CARTESIAN_POINT('Ctrl Pts',(-6.50609420700006,15.2,-9.27417010000001));
#284589=CARTESIAN_POINT('Ctrl Pts',(-6.50918328200006,15.2,-9.27600936900001));
#284590=CARTESIAN_POINT('Ctrl Pts',(-6.51227776500006,15.2,-9.27784861500001));
#284591=CARTESIAN_POINT('Ctrl Pts',(-6.51537765500006,15.2,-9.27968782700002));
#284592=CARTESIAN_POINT('Ctrl Pts',(-6.51848294800006,15.2,-9.28152699600002));
#284593=CARTESIAN_POINT('Ctrl Pts',(-6.52159363900005,15.2,-9.28336611300002));
#284594=CARTESIAN_POINT('Ctrl Pts',(-6.52470972700006,15.2,-9.28520517200001));
#284595=CARTESIAN_POINT('Ctrl Pts',(-6.52783120600006,15.2,-9.28704416000001));
#284596=CARTESIAN_POINT('Ctrl Pts',(-6.53095807500006,15.2,-9.28888307000001));
#284597=CARTESIAN_POINT('Ctrl Pts',(-6.53409033000006,15.2,-9.29072189400001));
#284598=CARTESIAN_POINT('Ctrl Pts',(-6.53722796600006,15.2,-9.29256062200002));
#284599=CARTESIAN_POINT('Ctrl Pts',(-6.54037098100006,15.2,-9.29439924500001));
#284600=CARTESIAN_POINT('Ctrl Pts',(-6.54351937200006,15.2,-9.29623775500002));
#284601=CARTESIAN_POINT('Ctrl Pts',(-6.54667313400005,15.2,-9.29807614200002));
#284602=CARTESIAN_POINT('Ctrl Pts',(-6.54983226500006,15.2,-9.29991439900002));
#284603=CARTESIAN_POINT('Ctrl Pts',(-6.55299676000006,15.2,-9.30175251500001));
#284604=CARTESIAN_POINT('Ctrl Pts',(-6.55616661700006,15.2,-9.30359048400001));
#284605=CARTESIAN_POINT('Ctrl Pts',(-6.55934183200006,15.2,-9.30542829500002));
#284606=CARTESIAN_POINT('Ctrl Pts',(-6.56252240200006,15.2,-9.30726594200002));
#284607=CARTESIAN_POINT('Ctrl Pts',(-6.56570832300006,15.2,-9.30910341200001));
#284608=CARTESIAN_POINT('Ctrl Pts',(-6.56889959100006,15.2,-9.31094070000002));
#284609=CARTESIAN_POINT('Ctrl Pts',(-6.57209620400006,15.2,-9.31277779500002));
#284610=CARTESIAN_POINT('Ctrl Pts',(-6.57529815700006,15.2,-9.31461469100002));
#284611=CARTESIAN_POINT('Ctrl Pts',(-6.57850544800006,15.2,-9.31645137700002));
#284612=CARTESIAN_POINT('Ctrl Pts',(-6.58171807300006,15.2,-9.31828784500001));
#284613=CARTESIAN_POINT('Ctrl Pts',(-6.58493602700006,15.2,-9.32012408600002));
#284614=CARTESIAN_POINT('Ctrl Pts',(-6.58815931000006,15.2,-9.32196009500002));
#284615=CARTESIAN_POINT('Ctrl Pts',(-6.59138791700006,15.2,-9.32379585900001));
#284616=CARTESIAN_POINT('Ctrl Pts',(-6.59462184300006,15.2,-9.32563137200002));
#284617=CARTESIAN_POINT('Ctrl Pts',(-6.59786108600006,15.2,-9.32746662500002));
#284618=CARTESIAN_POINT('Ctrl Pts',(-6.60110564300005,15.2,-9.32930161000002));
#284619=CARTESIAN_POINT('Ctrl Pts',(-6.60435550800006,15.2,-9.33113631500002));
#284620=CARTESIAN_POINT('Ctrl Pts',(-6.60761068100006,15.2,-9.33297073500002));
#284621=CARTESIAN_POINT('Ctrl Pts',(-6.61087115500006,15.2,-9.33480485900001));
#284622=CARTESIAN_POINT('Ctrl Pts',(-6.61413692800005,15.2,-9.33663868000002));
#284623=CARTESIAN_POINT('Ctrl Pts',(-6.61740799800006,15.2,-9.33847218900001));
#284624=CARTESIAN_POINT('Ctrl Pts',(-6.62068436000006,15.2,-9.34030538000002));
#284625=CARTESIAN_POINT('Ctrl Pts',(-6.62396601100006,15.2,-9.34213824300001));
#284626=CARTESIAN_POINT('Ctrl Pts',(-6.62725294900006,15.2,-9.34397077300002));
#284627=CARTESIAN_POINT('Ctrl Pts',(-6.63054517000006,15.2,-9.34580296000001));
#284628=CARTESIAN_POINT('Ctrl Pts',(-6.63384267100006,15.2,-9.34763479700001));
#284629=CARTESIAN_POINT('Ctrl Pts',(-6.63714544700006,15.2,-9.34946627300001));
#284630=CARTESIAN_POINT('Ctrl Pts',(-6.64045349300006,15.2,-9.35129737900001));
#284631=CARTESIAN_POINT('Ctrl Pts',(-6.64376680700006,15.2,-9.35312810300001));
#284632=CARTESIAN_POINT('Ctrl Pts',(-6.64708538300006,15.2,-9.35495843700001));
#284633=CARTESIAN_POINT('Ctrl Pts',(-6.65040921900006,15.2,-9.35678837000001));
#284634=CARTESIAN_POINT('Ctrl Pts',(-6.65373831000006,15.2,-9.35861789600001));
#284635=CARTESIAN_POINT('Ctrl Pts',(-6.65707265500005,15.2,-9.36044701000002));
#284636=CARTESIAN_POINT('Ctrl Pts',(-6.66041225200006,15.2,-9.36227570600002));
#284637=CARTESIAN_POINT('Ctrl Pts',(-6.66375709900006,15.2,-9.36410398400002));
#284638=CARTESIAN_POINT('Ctrl Pts',(-6.66643717700006,15.2,-9.36556627000002));
#284639=CARTESIAN_POINT('Ctrl Pts',(-6.66844959800006,15.2,-9.36666279600002));
#284640=CARTESIAN_POINT('Ctrl Pts',(-6.66979226100006,15.2,-9.36739373000002));
#284641=CARTESIAN_POINT('Ctrl Pts',(-6.67046385600006,15.2,-9.36775917400002));
#284642=CARTESIAN_POINT('Ctrl Pts',(-6.57080831900006,15.2,-8.02901631800001));
#284643=CARTESIAN_POINT('Ctrl Pts',(-6.57080831900006,11.6,-8.02901631800001));
#284644=CARTESIAN_POINT('Ctrl Pts',(-6.57090674100006,15.2,-8.02916024100002));
#284645=CARTESIAN_POINT('Ctrl Pts',(-6.57090674100006,11.6,-8.02916024100002));
#284646=CARTESIAN_POINT('Ctrl Pts',(-6.57110695100006,15.2,-8.02945316300002));
#284647=CARTESIAN_POINT('Ctrl Pts',(-6.57110695100006,11.6,-8.02945316300002));
#284648=CARTESIAN_POINT('Ctrl Pts',(-6.57141009900006,15.2,-8.02989715700001));
#284649=CARTESIAN_POINT('Ctrl Pts',(-6.57141009900006,11.6,-8.02989715700001));
#284650=CARTESIAN_POINT('Ctrl Pts',(-6.57181802000006,15.2,-8.03049556400002));
#284651=CARTESIAN_POINT('Ctrl Pts',(-6.57181802000006,11.6,-8.03049556400002));
#284652=CARTESIAN_POINT('Ctrl Pts',(-6.57233322400006,15.2,-8.03125297300002));
#284653=CARTESIAN_POINT('Ctrl Pts',(-6.57233322400006,11.6,-8.03125297300002));
#284654=CARTESIAN_POINT('Ctrl Pts',(-6.57285600600006,15.2,-8.03202318500002));
#284655=CARTESIAN_POINT('Ctrl Pts',(-6.57285600600006,11.6,-8.03202318500002));
#284656=CARTESIAN_POINT('Ctrl Pts',(-6.57338335000006,15.2,-8.03280179700002));
#284657=CARTESIAN_POINT('Ctrl Pts',(-6.57338335000006,11.6,-8.03280179700002));
#284658=CARTESIAN_POINT('Ctrl Pts',(-6.57391522700006,15.2,-8.03358880000001));
#284659=CARTESIAN_POINT('Ctrl Pts',(-6.57391522700006,11.6,-8.03358880000001));
#284660=CARTESIAN_POINT('Ctrl Pts',(-6.57445160600005,15.2,-8.03438417800002));
#284661=CARTESIAN_POINT('Ctrl Pts',(-6.57445160600005,11.6,-8.03438417800002));
#284662=CARTESIAN_POINT('Ctrl Pts',(-6.57499245700006,15.2,-8.03518792300002));
#284663=CARTESIAN_POINT('Ctrl Pts',(-6.57499245700006,11.6,-8.03518792300002));
#284664=CARTESIAN_POINT('Ctrl Pts',(-6.57553775200006,15.2,-8.03600002100002));
#284665=CARTESIAN_POINT('Ctrl Pts',(-6.57553775200006,11.6,-8.03600002100002));
#284666=CARTESIAN_POINT('Ctrl Pts',(-6.57608746000006,15.2,-8.03682046000001));
#284667=CARTESIAN_POINT('Ctrl Pts',(-6.57608746000006,11.6,-8.03682046000001));
#284668=CARTESIAN_POINT('Ctrl Pts',(-6.57664155100006,15.2,-8.03764922800001));
#284669=CARTESIAN_POINT('Ctrl Pts',(-6.57664155100006,11.6,-8.03764922800001));
#284670=CARTESIAN_POINT('Ctrl Pts',(-6.57719999700006,15.2,-8.03848631500001));
#284671=CARTESIAN_POINT('Ctrl Pts',(-6.57719999700006,11.6,-8.03848631500001));
#284672=CARTESIAN_POINT('Ctrl Pts',(-6.57776276900006,15.2,-8.03933170500001));
#284673=CARTESIAN_POINT('Ctrl Pts',(-6.57776276900006,11.6,-8.03933170500001));
#284674=CARTESIAN_POINT('Ctrl Pts',(-6.57832983700006,15.2,-8.04018539000002));
#284675=CARTESIAN_POINT('Ctrl Pts',(-6.57832983700006,11.6,-8.04018539000002));
#284676=CARTESIAN_POINT('Ctrl Pts',(-6.57890117200005,15.2,-8.04104735800001));
#284677=CARTESIAN_POINT('Ctrl Pts',(-6.57890117200005,11.6,-8.04104735800001));
#284678=CARTESIAN_POINT('Ctrl Pts',(-6.57947674700006,15.2,-8.04191759500002));
#284679=CARTESIAN_POINT('Ctrl Pts',(-6.57947674700006,11.6,-8.04191759500002));
#284680=CARTESIAN_POINT('Ctrl Pts',(-6.58005653200005,15.2,-8.04279609000002));
#284681=CARTESIAN_POINT('Ctrl Pts',(-6.58005653200005,11.6,-8.04279609000002));
#284682=CARTESIAN_POINT('Ctrl Pts',(-6.58064050000006,15.2,-8.04368283300001));
#284683=CARTESIAN_POINT('Ctrl Pts',(-6.58064050000006,11.6,-8.04368283300001));
#284684=CARTESIAN_POINT('Ctrl Pts',(-6.58122862000006,15.2,-8.04457781100002));
#284685=CARTESIAN_POINT('Ctrl Pts',(-6.58122862000006,11.6,-8.04457781100002));
#284686=CARTESIAN_POINT('Ctrl Pts',(-6.58182086700006,15.2,-8.04548101200002));
#284687=CARTESIAN_POINT('Ctrl Pts',(-6.58182086700006,11.6,-8.04548101200002));
#284688=CARTESIAN_POINT('Ctrl Pts',(-6.58241721200006,15.2,-8.04639242700001));
#284689=CARTESIAN_POINT('Ctrl Pts',(-6.58241721200006,11.6,-8.04639242700001));
#284690=CARTESIAN_POINT('Ctrl Pts',(-6.58301762700006,15.2,-8.04731204200002));
#284691=CARTESIAN_POINT('Ctrl Pts',(-6.58301762700006,11.6,-8.04731204200002));
#284692=CARTESIAN_POINT('Ctrl Pts',(-6.58362208300006,15.2,-8.04823984600001));
#284693=CARTESIAN_POINT('Ctrl Pts',(-6.58362208300006,11.6,-8.04823984600001));
#284694=CARTESIAN_POINT('Ctrl Pts',(-6.58423055400006,15.2,-8.04917582900002));
#284695=CARTESIAN_POINT('Ctrl Pts',(-6.58423055400006,11.6,-8.04917582900002));
#284696=CARTESIAN_POINT('Ctrl Pts',(-6.58484301300006,15.2,-8.05011997800002));
#284697=CARTESIAN_POINT('Ctrl Pts',(-6.58484301300006,11.6,-8.05011997800002));
#284698=CARTESIAN_POINT('Ctrl Pts',(-6.58545943100005,15.2,-8.05107228200002));
#284699=CARTESIAN_POINT('Ctrl Pts',(-6.58545943100005,11.6,-8.05107228200002));
#284700=CARTESIAN_POINT('Ctrl Pts',(-6.58607978300005,15.2,-8.05203273100001));
#284701=CARTESIAN_POINT('Ctrl Pts',(-6.58607978300005,11.6,-8.05203273100001));
#284702=CARTESIAN_POINT('Ctrl Pts',(-6.58670404000006,15.2,-8.05300131300001));
#284703=CARTESIAN_POINT('Ctrl Pts',(-6.58670404000006,11.6,-8.05300131300001));
#284704=CARTESIAN_POINT('Ctrl Pts',(-6.58733217600005,15.2,-8.05397801700002));
#284705=CARTESIAN_POINT('Ctrl Pts',(-6.58733217600005,11.6,-8.05397801700002));
#284706=CARTESIAN_POINT('Ctrl Pts',(-6.58796416400006,15.2,-8.05496283100002));
#284707=CARTESIAN_POINT('Ctrl Pts',(-6.58796416400006,11.6,-8.05496283100002));
#284708=CARTESIAN_POINT('Ctrl Pts',(-6.58859997800006,15.2,-8.05595574500002));
#284709=CARTESIAN_POINT('Ctrl Pts',(-6.58859997800006,11.6,-8.05595574500002));
#284710=CARTESIAN_POINT('Ctrl Pts',(-6.58923959000006,15.2,-8.05695674700001));
#284711=CARTESIAN_POINT('Ctrl Pts',(-6.58923959000006,11.6,-8.05695674700001));
#284712=CARTESIAN_POINT('Ctrl Pts',(-6.58988297600006,15.2,-8.05796582700001));
#284713=CARTESIAN_POINT('Ctrl Pts',(-6.58988297600006,11.6,-8.05796582700001));
#284714=CARTESIAN_POINT('Ctrl Pts',(-6.59053010700006,15.2,-8.05898297300002));
#284715=CARTESIAN_POINT('Ctrl Pts',(-6.59053010700006,11.6,-8.05898297300002));
#284716=CARTESIAN_POINT('Ctrl Pts',(-6.59118095900006,15.2,-8.06000817400001));
#284717=CARTESIAN_POINT('Ctrl Pts',(-6.59118095900006,11.6,-8.06000817400001));
#284718=CARTESIAN_POINT('Ctrl Pts',(-6.59183550500006,15.2,-8.06104142000001));
#284719=CARTESIAN_POINT('Ctrl Pts',(-6.59183550500006,11.6,-8.06104142000001));
#284720=CARTESIAN_POINT('Ctrl Pts',(-6.59249371900006,15.2,-8.06208270100001));
#284721=CARTESIAN_POINT('Ctrl Pts',(-6.59249371900006,11.6,-8.06208270100001));
#284722=CARTESIAN_POINT('Ctrl Pts',(-6.59315557600006,15.2,-8.06313200300002));
#284723=CARTESIAN_POINT('Ctrl Pts',(-6.59315557600006,11.6,-8.06313200300002));
#284724=CARTESIAN_POINT('Ctrl Pts',(-6.59382104900006,15.2,-8.06418931800001));
#284725=CARTESIAN_POINT('Ctrl Pts',(-6.59382104900006,11.6,-8.06418931800001));
#284726=CARTESIAN_POINT('Ctrl Pts',(-6.59449011500006,15.2,-8.06525463500002));
#284727=CARTESIAN_POINT('Ctrl Pts',(-6.59449011500006,11.6,-8.06525463500002));
#284728=CARTESIAN_POINT('Ctrl Pts',(-6.59516274600006,15.2,-8.06632794100001));
#284729=CARTESIAN_POINT('Ctrl Pts',(-6.59516274600006,11.6,-8.06632794100001));
#284730=CARTESIAN_POINT('Ctrl Pts',(-6.59583891700006,15.2,-8.06740922800002));
#284731=CARTESIAN_POINT('Ctrl Pts',(-6.59583891700006,11.6,-8.06740922800002));
#284732=CARTESIAN_POINT('Ctrl Pts',(-6.59651860500006,15.2,-8.06849848300002));
#284733=CARTESIAN_POINT('Ctrl Pts',(-6.59651860500006,11.6,-8.06849848300002));
#284734=CARTESIAN_POINT('Ctrl Pts',(-6.59720178300006,15.2,-8.06959569800001));
#284735=CARTESIAN_POINT('Ctrl Pts',(-6.59720178300006,11.6,-8.06959569800001));
#284736=CARTESIAN_POINT('Ctrl Pts',(-6.59788842600006,15.2,-8.07070086000002));
#284737=CARTESIAN_POINT('Ctrl Pts',(-6.59788842600006,11.6,-8.07070086000002));
#284738=CARTESIAN_POINT('Ctrl Pts',(-6.59857851000006,15.2,-8.07181396000002));
#284739=CARTESIAN_POINT('Ctrl Pts',(-6.59857851000006,11.6,-8.07181396000002));
#284740=CARTESIAN_POINT('Ctrl Pts',(-6.59927200900006,15.2,-8.07293498700002));
#284741=CARTESIAN_POINT('Ctrl Pts',(-6.59927200900006,11.6,-8.07293498700002));
#284742=CARTESIAN_POINT('Ctrl Pts',(-6.59996890100006,15.2,-8.07406392900001));
#284743=CARTESIAN_POINT('Ctrl Pts',(-6.59996890100006,11.6,-8.07406392900001));
#284744=CARTESIAN_POINT('Ctrl Pts',(-6.60066916000006,15.2,-8.07520077800002));
#284745=CARTESIAN_POINT('Ctrl Pts',(-6.60066916000006,11.6,-8.07520077800002));
#284746=CARTESIAN_POINT('Ctrl Pts',(-6.60137276000006,15.2,-8.07634552200001));
#284747=CARTESIAN_POINT('Ctrl Pts',(-6.60137276000006,11.6,-8.07634552200001));
#284748=CARTESIAN_POINT('Ctrl Pts',(-6.60207968000006,15.2,-8.07749815200001));
#284749=CARTESIAN_POINT('Ctrl Pts',(-6.60207968000006,11.6,-8.07749815200001));
#284750=CARTESIAN_POINT('Ctrl Pts',(-6.60278989300005,15.2,-8.07865865600002));
#284751=CARTESIAN_POINT('Ctrl Pts',(-6.60278989300005,11.6,-8.07865865600002));
#284752=CARTESIAN_POINT('Ctrl Pts',(-6.60350337600006,15.2,-8.07982702500002));
#284753=CARTESIAN_POINT('Ctrl Pts',(-6.60350337600006,11.6,-8.07982702500002));
#284754=CARTESIAN_POINT('Ctrl Pts',(-6.60422010600006,15.2,-8.08100324800002));
#284755=CARTESIAN_POINT('Ctrl Pts',(-6.60422010600006,11.6,-8.08100324800002));
#284756=CARTESIAN_POINT('Ctrl Pts',(-6.60494005800006,15.2,-8.08218731500002));
#284757=CARTESIAN_POINT('Ctrl Pts',(-6.60494005800006,11.6,-8.08218731500002));
#284758=CARTESIAN_POINT('Ctrl Pts',(-6.60566320900006,15.2,-8.08337921500001));
#284759=CARTESIAN_POINT('Ctrl Pts',(-6.60566320900006,11.6,-8.08337921500001));
#284760=CARTESIAN_POINT('Ctrl Pts',(-6.60638953400006,15.2,-8.08457893900002));
#284761=CARTESIAN_POINT('Ctrl Pts',(-6.60638953400006,11.6,-8.08457893900002));
#284762=CARTESIAN_POINT('Ctrl Pts',(-6.60711901100006,15.2,-8.08578647500001));
#284763=CARTESIAN_POINT('Ctrl Pts',(-6.60711901100006,11.6,-8.08578647500001));
#284764=CARTESIAN_POINT('Ctrl Pts',(-6.60785161500006,15.2,-8.08700181500001));
#284765=CARTESIAN_POINT('Ctrl Pts',(-6.60785161500006,11.6,-8.08700181500001));
#284766=CARTESIAN_POINT('Ctrl Pts',(-6.60858732500006,15.2,-8.08822494800001));
#284767=CARTESIAN_POINT('Ctrl Pts',(-6.60858732500006,11.6,-8.08822494800001));
#284768=CARTESIAN_POINT('Ctrl Pts',(-6.60932611700006,15.2,-8.08945586400002));
#284769=CARTESIAN_POINT('Ctrl Pts',(-6.60932611700006,11.6,-8.08945586400002));
#284770=CARTESIAN_POINT('Ctrl Pts',(-6.61006796600006,15.2,-8.09069455200002));
#284771=CARTESIAN_POINT('Ctrl Pts',(-6.61006796600006,11.6,-8.09069455200002));
#284772=CARTESIAN_POINT('Ctrl Pts',(-6.61081285100006,15.2,-8.09194100300001));
#284773=CARTESIAN_POINT('Ctrl Pts',(-6.61081285100006,11.6,-8.09194100300001));
#284774=CARTESIAN_POINT('Ctrl Pts',(-6.61156074900005,15.2,-8.09319520700001));
#284775=CARTESIAN_POINT('Ctrl Pts',(-6.61156074900005,11.6,-8.09319520700001));
#284776=CARTESIAN_POINT('Ctrl Pts',(-6.61231163600006,15.2,-8.09445715400001));
#284777=CARTESIAN_POINT('Ctrl Pts',(-6.61231163600006,11.6,-8.09445715400001));
#284778=CARTESIAN_POINT('Ctrl Pts',(-6.61306549000006,15.2,-8.09572683400001));
#284779=CARTESIAN_POINT('Ctrl Pts',(-6.61306549000006,11.6,-8.09572683400001));
#284780=CARTESIAN_POINT('Ctrl Pts',(-6.61382229000006,15.2,-8.09700423600002));
#284781=CARTESIAN_POINT('Ctrl Pts',(-6.61382229000006,11.6,-8.09700423600002));
#284782=CARTESIAN_POINT('Ctrl Pts',(-6.61458201100006,15.2,-8.09828935200001));
#284783=CARTESIAN_POINT('Ctrl Pts',(-6.61458201100006,11.6,-8.09828935200001));
#284784=CARTESIAN_POINT('Ctrl Pts',(-6.61534463100006,15.2,-8.09958217100002));
#284785=CARTESIAN_POINT('Ctrl Pts',(-6.61534463100006,11.6,-8.09958217100002));
#284786=CARTESIAN_POINT('Ctrl Pts',(-6.61611012900006,15.2,-8.10088268300002));
#284787=CARTESIAN_POINT('Ctrl Pts',(-6.61611012900006,11.6,-8.10088268300002));
#284788=CARTESIAN_POINT('Ctrl Pts',(-6.61687848200006,15.2,-8.10219087900002));
#284789=CARTESIAN_POINT('Ctrl Pts',(-6.61687848200006,11.6,-8.10219087900002));
#284790=CARTESIAN_POINT('Ctrl Pts',(-6.61764966700006,15.2,-8.10350674900001));
#284791=CARTESIAN_POINT('Ctrl Pts',(-6.61764966700006,11.6,-8.10350674900001));
#284792=CARTESIAN_POINT('Ctrl Pts',(-6.61842366400006,15.2,-8.10483028300002));
#284793=CARTESIAN_POINT('Ctrl Pts',(-6.61842366400006,11.6,-8.10483028300002));
#284794=CARTESIAN_POINT('Ctrl Pts',(-6.61920045000006,15.2,-8.10616147100001));
#284795=CARTESIAN_POINT('Ctrl Pts',(-6.61920045000006,11.6,-8.10616147100001));
#284796=CARTESIAN_POINT('Ctrl Pts',(-6.61998000200006,15.2,-8.10750030400002));
#284797=CARTESIAN_POINT('Ctrl Pts',(-6.61998000200006,11.6,-8.10750030400002));
#284798=CARTESIAN_POINT('Ctrl Pts',(-6.62076230000006,15.2,-8.10884677100002));
#284799=CARTESIAN_POINT('Ctrl Pts',(-6.62076230000006,11.6,-8.10884677100002));
#284800=CARTESIAN_POINT('Ctrl Pts',(-6.62154732100006,15.2,-8.11020086400001));
#284801=CARTESIAN_POINT('Ctrl Pts',(-6.62154732100006,11.6,-8.11020086400001));
#284802=CARTESIAN_POINT('Ctrl Pts',(-6.62233504600006,15.2,-8.11156257400001));
#284803=CARTESIAN_POINT('Ctrl Pts',(-6.62233504600006,11.6,-8.11156257400001));
#284804=CARTESIAN_POINT('Ctrl Pts',(-6.62312545000006,15.2,-8.11293188900001));
#284805=CARTESIAN_POINT('Ctrl Pts',(-6.62312545000006,11.6,-8.11293188900001));
#284806=CARTESIAN_POINT('Ctrl Pts',(-6.62391851400006,15.2,-8.11430880100002));
#284807=CARTESIAN_POINT('Ctrl Pts',(-6.62391851400006,11.6,-8.11430880100002));
#284808=CARTESIAN_POINT('Ctrl Pts',(-6.62471421500006,15.2,-8.11569329900001));
#284809=CARTESIAN_POINT('Ctrl Pts',(-6.62471421500006,11.6,-8.11569329900001));
#284810=CARTESIAN_POINT('Ctrl Pts',(-6.62551253400006,15.2,-8.11708537600002));
#284811=CARTESIAN_POINT('Ctrl Pts',(-6.62551253400006,11.6,-8.11708537600002));
#284812=CARTESIAN_POINT('Ctrl Pts',(-6.62631344800006,15.2,-8.11848502000002));
#284813=CARTESIAN_POINT('Ctrl Pts',(-6.62631344800006,11.6,-8.11848502000002));
#284814=CARTESIAN_POINT('Ctrl Pts',(-6.62711693700006,15.2,-8.11989222400002));
#284815=CARTESIAN_POINT('Ctrl Pts',(-6.62711693700006,11.6,-8.11989222400002));
#284816=CARTESIAN_POINT('Ctrl Pts',(-6.62792298000006,15.2,-8.12130697600002));
#284817=CARTESIAN_POINT('Ctrl Pts',(-6.62792298000006,11.6,-8.12130697600002));
#284818=CARTESIAN_POINT('Ctrl Pts',(-6.62873155500006,15.2,-8.12272926700001));
#284819=CARTESIAN_POINT('Ctrl Pts',(-6.62873155500006,11.6,-8.12272926700001));
#284820=CARTESIAN_POINT('Ctrl Pts',(-6.62954264200006,15.2,-8.12415909000002));
#284821=CARTESIAN_POINT('Ctrl Pts',(-6.62954264200006,11.6,-8.12415909000002));
#284822=CARTESIAN_POINT('Ctrl Pts',(-6.63035622100006,15.2,-8.12559643400002));
#284823=CARTESIAN_POINT('Ctrl Pts',(-6.63035622100006,11.6,-8.12559643400002));
#284824=CARTESIAN_POINT('Ctrl Pts',(-6.63117227000006,15.2,-8.12704128900002));
#284825=CARTESIAN_POINT('Ctrl Pts',(-6.63117227000006,11.6,-8.12704128900002));
#284826=CARTESIAN_POINT('Ctrl Pts',(-6.63199077100006,15.2,-8.12849364600002));
#284827=CARTESIAN_POINT('Ctrl Pts',(-6.63199077100006,11.6,-8.12849364600002));
#284828=CARTESIAN_POINT('Ctrl Pts',(-6.63281170000006,15.2,-8.12995349700002));
#284829=CARTESIAN_POINT('Ctrl Pts',(-6.63281170000006,11.6,-8.12995349700002));
#284830=CARTESIAN_POINT('Ctrl Pts',(-6.63363504000006,15.2,-8.13142083100002));
#284831=CARTESIAN_POINT('Ctrl Pts',(-6.63363504000006,11.6,-8.13142083100002));
#284832=CARTESIAN_POINT('Ctrl Pts',(-6.63446076800006,15.2,-8.13289564100002));
#284833=CARTESIAN_POINT('Ctrl Pts',(-6.63446076800006,11.6,-8.13289564100002));
#284834=CARTESIAN_POINT('Ctrl Pts',(-6.63528886600006,15.2,-8.13437791500002));
#284835=CARTESIAN_POINT('Ctrl Pts',(-6.63528886600006,11.6,-8.13437791500002));
#284836=CARTESIAN_POINT('Ctrl Pts',(-6.63611931200006,15.2,-8.13586764600002));
#284837=CARTESIAN_POINT('Ctrl Pts',(-6.63611931200006,11.6,-8.13586764600002));
#284838=CARTESIAN_POINT('Ctrl Pts',(-6.63695208700006,15.2,-8.13736482400002));
#284839=CARTESIAN_POINT('Ctrl Pts',(-6.63695208700006,11.6,-8.13736482400002));
#284840=CARTESIAN_POINT('Ctrl Pts',(-6.63778717100006,15.2,-8.13886943900001));
#284841=CARTESIAN_POINT('Ctrl Pts',(-6.63778717100006,11.6,-8.13886943900001));
#284842=CARTESIAN_POINT('Ctrl Pts',(-6.63862454400006,15.2,-8.14038148300002));
#284843=CARTESIAN_POINT('Ctrl Pts',(-6.63862454400006,11.6,-8.14038148300002));
#284844=CARTESIAN_POINT('Ctrl Pts',(-6.63946418700006,15.2,-8.14190094700002));
#284845=CARTESIAN_POINT('Ctrl Pts',(-6.63946418700006,11.6,-8.14190094700002));
#284846=CARTESIAN_POINT('Ctrl Pts',(-6.64030607900005,15.2,-8.14342782100002));
#284847=CARTESIAN_POINT('Ctrl Pts',(-6.64030607900005,11.6,-8.14342782100002));
#284848=CARTESIAN_POINT('Ctrl Pts',(-6.64115020100006,15.2,-8.14496209700001));
#284849=CARTESIAN_POINT('Ctrl Pts',(-6.64115020100006,11.6,-8.14496209700001));
#284850=CARTESIAN_POINT('Ctrl Pts',(-6.64199653400006,15.2,-8.14650376600002));
#284851=CARTESIAN_POINT('Ctrl Pts',(-6.64199653400006,11.6,-8.14650376600002));
#284852=CARTESIAN_POINT('Ctrl Pts',(-6.64284505800006,15.2,-8.14805281700002));
#284853=CARTESIAN_POINT('Ctrl Pts',(-6.64284505800006,11.6,-8.14805281700002));
#284854=CARTESIAN_POINT('Ctrl Pts',(-6.64369575300006,15.2,-8.14960924300001));
#284855=CARTESIAN_POINT('Ctrl Pts',(-6.64369575300006,11.6,-8.14960924300001));
#284856=CARTESIAN_POINT('Ctrl Pts',(-6.64454859900006,15.2,-8.15117303500001));
#284857=CARTESIAN_POINT('Ctrl Pts',(-6.64454859900006,11.6,-8.15117303500001));
#284858=CARTESIAN_POINT('Ctrl Pts',(-6.64540358000006,15.2,-8.15274418300002));
#284859=CARTESIAN_POINT('Ctrl Pts',(-6.64540358000006,11.6,-8.15274418300002));
#284860=CARTESIAN_POINT('Ctrl Pts',(-6.64626067400006,15.2,-8.15432267900002));
#284861=CARTESIAN_POINT('Ctrl Pts',(-6.64626067400006,11.6,-8.15432267900002));
#284862=CARTESIAN_POINT('Ctrl Pts',(-6.64711986400006,15.2,-8.15590851400002));
#284863=CARTESIAN_POINT('Ctrl Pts',(-6.64711986400006,11.6,-8.15590851400002));
#284864=CARTESIAN_POINT('Ctrl Pts',(-6.64798112800006,15.2,-8.15750167800001));
#284865=CARTESIAN_POINT('Ctrl Pts',(-6.64798112800006,11.6,-8.15750167800001));
#284866=CARTESIAN_POINT('Ctrl Pts',(-6.64884444900006,15.2,-8.15910216300002));
#284867=CARTESIAN_POINT('Ctrl Pts',(-6.64884444900006,11.6,-8.15910216300002));
#284868=CARTESIAN_POINT('Ctrl Pts',(-6.64970980800006,15.2,-8.16070996000001));
#284869=CARTESIAN_POINT('Ctrl Pts',(-6.64970980800006,11.6,-8.16070996000001));
#284870=CARTESIAN_POINT('Ctrl Pts',(-6.65057718600006,15.2,-8.16232506100001));
#284871=CARTESIAN_POINT('Ctrl Pts',(-6.65057718600006,11.6,-8.16232506100001));
#284872=CARTESIAN_POINT('Ctrl Pts',(-6.65144656600006,15.2,-8.16394745500002));
#284873=CARTESIAN_POINT('Ctrl Pts',(-6.65144656600006,11.6,-8.16394745500002));
#284874=CARTESIAN_POINT('Ctrl Pts',(-6.65231792600006,15.2,-8.16557713600002));
#284875=CARTESIAN_POINT('Ctrl Pts',(-6.65231792600006,11.6,-8.16557713600002));
#284876=CARTESIAN_POINT('Ctrl Pts',(-6.65319124900006,15.2,-8.16721409300002));
#284877=CARTESIAN_POINT('Ctrl Pts',(-6.65319124900006,11.6,-8.16721409300002));
#284878=CARTESIAN_POINT('Ctrl Pts',(-6.65406651700006,15.2,-8.16885831900001));
#284879=CARTESIAN_POINT('Ctrl Pts',(-6.65406651700006,11.6,-8.16885831900001));
#284880=CARTESIAN_POINT('Ctrl Pts',(-6.65494371100006,15.2,-8.17050980400002));
#284881=CARTESIAN_POINT('Ctrl Pts',(-6.65494371100006,11.6,-8.17050980400002));
#284882=CARTESIAN_POINT('Ctrl Pts',(-6.65582281300006,15.2,-8.17216853900002));
#284883=CARTESIAN_POINT('Ctrl Pts',(-6.65582281300006,11.6,-8.17216853900002));
#284884=CARTESIAN_POINT('Ctrl Pts',(-6.65670380500006,15.2,-8.17383451600002));
#284885=CARTESIAN_POINT('Ctrl Pts',(-6.65670380500006,11.6,-8.17383451600002));
#284886=CARTESIAN_POINT('Ctrl Pts',(-6.65758666800006,15.2,-8.17550772700002));
#284887=CARTESIAN_POINT('Ctrl Pts',(-6.65758666800006,11.6,-8.17550772700002));
#284888=CARTESIAN_POINT('Ctrl Pts',(-6.65847138400006,15.2,-8.17718816300001));
#284889=CARTESIAN_POINT('Ctrl Pts',(-6.65847138400006,11.6,-8.17718816300001));
#284890=CARTESIAN_POINT('Ctrl Pts',(-6.65935793500006,15.2,-8.17887581400001));
#284891=CARTESIAN_POINT('Ctrl Pts',(-6.65935793500006,11.6,-8.17887581400001));
#284892=CARTESIAN_POINT('Ctrl Pts',(-6.66024630300006,15.2,-8.18057067400002));
#284893=CARTESIAN_POINT('Ctrl Pts',(-6.66024630300006,11.6,-8.18057067400002));
#284894=CARTESIAN_POINT('Ctrl Pts',(-6.66113647000006,15.2,-8.18227273100002));
#284895=CARTESIAN_POINT('Ctrl Pts',(-6.66113647000006,11.6,-8.18227273100002));
#284896=CARTESIAN_POINT('Ctrl Pts',(-6.66202841900006,15.2,-8.18398198000001));
#284897=CARTESIAN_POINT('Ctrl Pts',(-6.66202841900006,11.6,-8.18398198000001));
#284898=CARTESIAN_POINT('Ctrl Pts',(-6.66292212900006,15.2,-8.18569840900001));
#284899=CARTESIAN_POINT('Ctrl Pts',(-6.66292212900006,11.6,-8.18569840900001));
#284900=CARTESIAN_POINT('Ctrl Pts',(-6.66381758700005,15.2,-8.18742201300001));
#284901=CARTESIAN_POINT('Ctrl Pts',(-6.66381758700005,11.6,-8.18742201300001));
#284902=CARTESIAN_POINT('Ctrl Pts',(-6.66471477200006,15.2,-8.18915278000001));
#284903=CARTESIAN_POINT('Ctrl Pts',(-6.66471477200006,11.6,-8.18915278000001));
#284904=CARTESIAN_POINT('Ctrl Pts',(-6.66561366700006,15.2,-8.19089070400001));
#284905=CARTESIAN_POINT('Ctrl Pts',(-6.66561366700006,11.6,-8.19089070400001));
#284906=CARTESIAN_POINT('Ctrl Pts',(-6.66651425400006,15.2,-8.19263577600001));
#284907=CARTESIAN_POINT('Ctrl Pts',(-6.66651425400006,11.6,-8.19263577600001));
#284908=CARTESIAN_POINT('Ctrl Pts',(-6.66741651800006,15.2,-8.19438798600002));
#284909=CARTESIAN_POINT('Ctrl Pts',(-6.66741651800006,11.6,-8.19438798600002));
#284910=CARTESIAN_POINT('Ctrl Pts',(-6.66832043800006,15.2,-8.19614732700002));
#284911=CARTESIAN_POINT('Ctrl Pts',(-6.66832043800006,11.6,-8.19614732700002));
#284912=CARTESIAN_POINT('Ctrl Pts',(-6.66922600000006,15.2,-8.19791379200002));
#284913=CARTESIAN_POINT('Ctrl Pts',(-6.66922600000006,11.6,-8.19791379200002));
#284914=CARTESIAN_POINT('Ctrl Pts',(-6.67013318300006,15.2,-8.19968736900002));
#284915=CARTESIAN_POINT('Ctrl Pts',(-6.67013318300006,11.6,-8.19968736900002));
#284916=CARTESIAN_POINT('Ctrl Pts',(-6.67104197300006,15.2,-8.20146805200002));
#284917=CARTESIAN_POINT('Ctrl Pts',(-6.67104197300006,11.6,-8.20146805200002));
#284918=CARTESIAN_POINT('Ctrl Pts',(-6.67195235200006,15.2,-8.20325583300002));
#284919=CARTESIAN_POINT('Ctrl Pts',(-6.67195235200006,11.6,-8.20325583300002));
#284920=CARTESIAN_POINT('Ctrl Pts',(-6.67286430200006,15.2,-8.20505070200002));
#284921=CARTESIAN_POINT('Ctrl Pts',(-6.67286430200006,11.6,-8.20505070200002));
#284922=CARTESIAN_POINT('Ctrl Pts',(-6.67377780700006,15.2,-8.20685265200002));
#284923=CARTESIAN_POINT('Ctrl Pts',(-6.67377780700006,11.6,-8.20685265200002));
#284924=CARTESIAN_POINT('Ctrl Pts',(-6.67469285000006,15.2,-8.20866167300002));
#284925=CARTESIAN_POINT('Ctrl Pts',(-6.67469285000006,11.6,-8.20866167300002));
#284926=CARTESIAN_POINT('Ctrl Pts',(-6.67560941300006,15.2,-8.21047775800002));
#284927=CARTESIAN_POINT('Ctrl Pts',(-6.67560941300006,11.6,-8.21047775800002));
#284928=CARTESIAN_POINT('Ctrl Pts',(-6.67652747900005,15.2,-8.21230089900002));
#284929=CARTESIAN_POINT('Ctrl Pts',(-6.67652747900005,11.6,-8.21230089900002));
#284930=CARTESIAN_POINT('Ctrl Pts',(-6.67744703200006,15.2,-8.21413108800002));
#284931=CARTESIAN_POINT('Ctrl Pts',(-6.67744703200006,11.6,-8.21413108800002));
#284932=CARTESIAN_POINT('Ctrl Pts',(-6.67836805600006,15.2,-8.21596831500001));
#284933=CARTESIAN_POINT('Ctrl Pts',(-6.67836805600006,11.6,-8.21596831500001));
#284934=CARTESIAN_POINT('Ctrl Pts',(-6.67929053300006,15.2,-8.21781257300002));
#284935=CARTESIAN_POINT('Ctrl Pts',(-6.67929053300006,11.6,-8.21781257300002));
#284936=CARTESIAN_POINT('Ctrl Pts',(-6.68021444700006,15.2,-8.21966385300002));
#284937=CARTESIAN_POINT('Ctrl Pts',(-6.68021444700006,11.6,-8.21966385300002));
#284938=CARTESIAN_POINT('Ctrl Pts',(-6.68113978100005,15.2,-8.22152214800001));
#284939=CARTESIAN_POINT('Ctrl Pts',(-6.68113978100005,11.6,-8.22152214800001));
#284940=CARTESIAN_POINT('Ctrl Pts',(-6.68206651900006,15.2,-8.22338745000001));
#284941=CARTESIAN_POINT('Ctrl Pts',(-6.68206651900006,11.6,-8.22338745000001));
#284942=CARTESIAN_POINT('Ctrl Pts',(-6.68299464500006,15.2,-8.22525974700002));
#284943=CARTESIAN_POINT('Ctrl Pts',(-6.68299464500006,11.6,-8.22525974700002));
#284944=CARTESIAN_POINT('Ctrl Pts',(-6.68392414200006,15.2,-8.22713903600001));
#284945=CARTESIAN_POINT('Ctrl Pts',(-6.68392414200006,11.6,-8.22713903600001));
#284946=CARTESIAN_POINT('Ctrl Pts',(-6.68485499200006,15.2,-8.22902530700001));
#284947=CARTESIAN_POINT('Ctrl Pts',(-6.68485499200006,11.6,-8.22902530700001));
#284948=CARTESIAN_POINT('Ctrl Pts',(-6.68578718200005,15.2,-8.23091855000002));
#284949=CARTESIAN_POINT('Ctrl Pts',(-6.68578718200005,11.6,-8.23091855000002));
#284950=CARTESIAN_POINT('Ctrl Pts',(-6.68672069300006,15.2,-8.23281875900001));
#284951=CARTESIAN_POINT('Ctrl Pts',(-6.68672069300006,11.6,-8.23281875900001));
#284952=CARTESIAN_POINT('Ctrl Pts',(-6.68765551100006,15.2,-8.23472592600002));
#284953=CARTESIAN_POINT('Ctrl Pts',(-6.68765551100006,11.6,-8.23472592600002));
#284954=CARTESIAN_POINT('Ctrl Pts',(-6.68859161800006,15.2,-8.23664004100002));
#284955=CARTESIAN_POINT('Ctrl Pts',(-6.68859161800006,11.6,-8.23664004100002));
#284956=CARTESIAN_POINT('Ctrl Pts',(-6.68952899900006,15.2,-8.23856109700002));
#284957=CARTESIAN_POINT('Ctrl Pts',(-6.68952899900006,11.6,-8.23856109700002));
#284958=CARTESIAN_POINT('Ctrl Pts',(-6.69046763700006,15.2,-8.24048908700002));
#284959=CARTESIAN_POINT('Ctrl Pts',(-6.69046763700006,11.6,-8.24048908700002));
#284960=CARTESIAN_POINT('Ctrl Pts',(-6.69140751900006,15.2,-8.24242400100001));
#284961=CARTESIAN_POINT('Ctrl Pts',(-6.69140751900006,11.6,-8.24242400100001));
#284962=CARTESIAN_POINT('Ctrl Pts',(-6.69234862600006,15.2,-8.24436583300002));
#284963=CARTESIAN_POINT('Ctrl Pts',(-6.69234862600006,11.6,-8.24436583300002));
#284964=CARTESIAN_POINT('Ctrl Pts',(-6.69329094300006,15.2,-8.24631457300002));
#284965=CARTESIAN_POINT('Ctrl Pts',(-6.69329094300006,11.6,-8.24631457300002));
#284966=CARTESIAN_POINT('Ctrl Pts',(-6.69423445500006,15.2,-8.24827021500001));
#284967=CARTESIAN_POINT('Ctrl Pts',(-6.69423445500006,11.6,-8.24827021500001));
#284968=CARTESIAN_POINT('Ctrl Pts',(-6.69517914500006,15.2,-8.25023274900002));
#284969=CARTESIAN_POINT('Ctrl Pts',(-6.69517914500006,11.6,-8.25023274900002));
#284970=CARTESIAN_POINT('Ctrl Pts',(-6.69612499800006,15.2,-8.25220216900002));
#284971=CARTESIAN_POINT('Ctrl Pts',(-6.69612499800006,11.6,-8.25220216900002));
#284972=CARTESIAN_POINT('Ctrl Pts',(-6.69707199900006,15.2,-8.25417846500001));
#284973=CARTESIAN_POINT('Ctrl Pts',(-6.69707199900006,11.6,-8.25417846500001));
#284974=CARTESIAN_POINT('Ctrl Pts',(-6.69802013200006,15.2,-8.25616163100002));
#284975=CARTESIAN_POINT('Ctrl Pts',(-6.69802013200006,11.6,-8.25616163100002));
#284976=CARTESIAN_POINT('Ctrl Pts',(-6.69896938100006,15.2,-8.25815165900002));
#284977=CARTESIAN_POINT('Ctrl Pts',(-6.69896938100006,11.6,-8.25815165900002));
#284978=CARTESIAN_POINT('Ctrl Pts',(-6.69991973100006,15.2,-8.26014853800002));
#284979=CARTESIAN_POINT('Ctrl Pts',(-6.69991973100006,11.6,-8.26014853800002));
#284980=CARTESIAN_POINT('Ctrl Pts',(-6.70087116700006,15.2,-8.26215226500001));
#284981=CARTESIAN_POINT('Ctrl Pts',(-6.70087116700006,11.6,-8.26215226500001));
#284982=CARTESIAN_POINT('Ctrl Pts',(-6.70182367300006,15.2,-8.26416282800002));
#284983=CARTESIAN_POINT('Ctrl Pts',(-6.70182367300006,11.6,-8.26416282800002));
#284984=CARTESIAN_POINT('Ctrl Pts',(-6.70277723400006,15.2,-8.26618022100002));
#284985=CARTESIAN_POINT('Ctrl Pts',(-6.70277723400006,11.6,-8.26618022100002));
#284986=CARTESIAN_POINT('Ctrl Pts',(-6.70373183500006,15.2,-8.26820443600001));
#284987=CARTESIAN_POINT('Ctrl Pts',(-6.70373183500006,11.6,-8.26820443600001));
#284988=CARTESIAN_POINT('Ctrl Pts',(-6.70468746000005,15.2,-8.27023546500002));
#284989=CARTESIAN_POINT('Ctrl Pts',(-6.70468746000005,11.6,-8.27023546500002));
#284990=CARTESIAN_POINT('Ctrl Pts',(-6.70564409500006,15.2,-8.27227330000002));
#284991=CARTESIAN_POINT('Ctrl Pts',(-6.70564409500006,11.6,-8.27227330000002));
#284992=CARTESIAN_POINT('Ctrl Pts',(-6.70660172400006,15.2,-8.27431793400002));
#284993=CARTESIAN_POINT('Ctrl Pts',(-6.70660172400006,11.6,-8.27431793400002));
#284994=CARTESIAN_POINT('Ctrl Pts',(-6.70756033200006,15.2,-8.27636935700001));
#284995=CARTESIAN_POINT('Ctrl Pts',(-6.70756033200006,11.6,-8.27636935700001));
#284996=CARTESIAN_POINT('Ctrl Pts',(-6.70851990500006,15.2,-8.27842756400001));
#284997=CARTESIAN_POINT('Ctrl Pts',(-6.70851990500006,11.6,-8.27842756400001));
#284998=CARTESIAN_POINT('Ctrl Pts',(-6.70948042600005,15.2,-8.28049254600002));
#284999=CARTESIAN_POINT('Ctrl Pts',(-6.70948042600005,11.6,-8.28049254600002));
#285000=CARTESIAN_POINT('Ctrl Pts',(-6.71044188300006,15.2,-8.28256429500002));
#285001=CARTESIAN_POINT('Ctrl Pts',(-6.71044188300006,11.6,-8.28256429500002));
#285002=CARTESIAN_POINT('Ctrl Pts',(-6.71140426000005,15.2,-8.28464280400001));
#285003=CARTESIAN_POINT('Ctrl Pts',(-6.71140426000005,11.6,-8.28464280400001));
#285004=CARTESIAN_POINT('Ctrl Pts',(-6.71236754100006,15.2,-8.28672806400002));
#285005=CARTESIAN_POINT('Ctrl Pts',(-6.71236754100006,11.6,-8.28672806400002));
#285006=CARTESIAN_POINT('Ctrl Pts',(-6.71333171300006,15.2,-8.28882006800002));
#285007=CARTESIAN_POINT('Ctrl Pts',(-6.71333171300006,11.6,-8.28882006800002));
#285008=CARTESIAN_POINT('Ctrl Pts',(-6.71429675900006,15.2,-8.29091880900001));
#285009=CARTESIAN_POINT('Ctrl Pts',(-6.71429675900006,11.6,-8.29091880900001));
#285010=CARTESIAN_POINT('Ctrl Pts',(-6.71526266700006,15.2,-8.29302427800001));
#285011=CARTESIAN_POINT('Ctrl Pts',(-6.71526266700006,11.6,-8.29302427800001));
#285012=CARTESIAN_POINT('Ctrl Pts',(-6.71622942200006,15.2,-8.29513646900002));
#285013=CARTESIAN_POINT('Ctrl Pts',(-6.71622942200006,11.6,-8.29513646900002));
#285014=CARTESIAN_POINT('Ctrl Pts',(-6.71719700800006,15.2,-8.29725537200002));
#285015=CARTESIAN_POINT('Ctrl Pts',(-6.71719700800006,11.6,-8.29725537200002));
#285016=CARTESIAN_POINT('Ctrl Pts',(-6.71816541100006,15.2,-8.29938098200002));
#285017=CARTESIAN_POINT('Ctrl Pts',(-6.71816541100006,11.6,-8.29938098200002));
#285018=CARTESIAN_POINT('Ctrl Pts',(-6.71913461600006,15.2,-8.30151328900002));
#285019=CARTESIAN_POINT('Ctrl Pts',(-6.71913461600006,11.6,-8.30151328900002));
#285020=CARTESIAN_POINT('Ctrl Pts',(-6.72010461200006,15.2,-8.30365228700002));
#285021=CARTESIAN_POINT('Ctrl Pts',(-6.72010461200006,11.6,-8.30365228700002));
#285022=CARTESIAN_POINT('Ctrl Pts',(-6.72107538000006,15.2,-8.30579796800002));
#285023=CARTESIAN_POINT('Ctrl Pts',(-6.72107538000006,11.6,-8.30579796800002));
#285024=CARTESIAN_POINT('Ctrl Pts',(-6.72204690900006,15.2,-8.30795032300001));
#285025=CARTESIAN_POINT('Ctrl Pts',(-6.72204690900006,11.6,-8.30795032300001));
#285026=CARTESIAN_POINT('Ctrl Pts',(-6.72301918300006,15.2,-8.31010934800002));
#285027=CARTESIAN_POINT('Ctrl Pts',(-6.72301918300006,11.6,-8.31010934800002));
#285028=CARTESIAN_POINT('Ctrl Pts',(-6.72399218800006,15.2,-8.31227503100001));
#285029=CARTESIAN_POINT('Ctrl Pts',(-6.72399218800006,11.6,-8.31227503100001));
#285030=CARTESIAN_POINT('Ctrl Pts',(-6.72496591100006,15.2,-8.31444736700002));
#285031=CARTESIAN_POINT('Ctrl Pts',(-6.72496591100006,11.6,-8.31444736700002));
#285032=CARTESIAN_POINT('Ctrl Pts',(-6.72594033700006,15.2,-8.31662634800002));
#285033=CARTESIAN_POINT('Ctrl Pts',(-6.72594033700006,11.6,-8.31662634800002));
#285034=CARTESIAN_POINT('Ctrl Pts',(-6.72691545200006,15.2,-8.31881196600002));
#285035=CARTESIAN_POINT('Ctrl Pts',(-6.72691545200006,11.6,-8.31881196600002));
#285036=CARTESIAN_POINT('Ctrl Pts',(-6.72789124200006,15.2,-8.32100421400002));
#285037=CARTESIAN_POINT('Ctrl Pts',(-6.72789124200006,11.6,-8.32100421400002));
#285038=CARTESIAN_POINT('Ctrl Pts',(-6.72886769300006,15.2,-8.32320308500002));
#285039=CARTESIAN_POINT('Ctrl Pts',(-6.72886769300006,11.6,-8.32320308500002));
#285040=CARTESIAN_POINT('Ctrl Pts',(-6.72984479100006,15.2,-8.32540857000001));
#285041=CARTESIAN_POINT('Ctrl Pts',(-6.72984479100006,11.6,-8.32540857000001));
#285042=CARTESIAN_POINT('Ctrl Pts',(-6.73082252300006,15.2,-8.32762066300001));
#285043=CARTESIAN_POINT('Ctrl Pts',(-6.73082252300006,11.6,-8.32762066300001));
#285044=CARTESIAN_POINT('Ctrl Pts',(-6.73180087300006,15.2,-8.32983935500001));
#285045=CARTESIAN_POINT('Ctrl Pts',(-6.73180087300006,11.6,-8.32983935500001));
#285046=CARTESIAN_POINT('Ctrl Pts',(-6.73277982900006,15.2,-8.33206464000002));
#285047=CARTESIAN_POINT('Ctrl Pts',(-6.73277982900006,11.6,-8.33206464000002));
#285048=CARTESIAN_POINT('Ctrl Pts',(-6.73375937800006,15.2,-8.33429650900002));
#285049=CARTESIAN_POINT('Ctrl Pts',(-6.73375937800006,11.6,-8.33429650900002));
#285050=CARTESIAN_POINT('Ctrl Pts',(-6.73473950400005,15.2,-8.33653495700002));
#285051=CARTESIAN_POINT('Ctrl Pts',(-6.73473950400005,11.6,-8.33653495700002));
#285052=CARTESIAN_POINT('Ctrl Pts',(-6.73572019500006,15.2,-8.33877997400002));
#285053=CARTESIAN_POINT('Ctrl Pts',(-6.73572019500006,11.6,-8.33877997400002));
#285054=CARTESIAN_POINT('Ctrl Pts',(-6.73670143700006,15.2,-8.34103155300001));
#285055=CARTESIAN_POINT('Ctrl Pts',(-6.73670143700006,11.6,-8.34103155300001));
#285056=CARTESIAN_POINT('Ctrl Pts',(-6.73768321600006,15.2,-8.34328968900002));
#285057=CARTESIAN_POINT('Ctrl Pts',(-6.73768321600006,11.6,-8.34328968900002));
#285058=CARTESIAN_POINT('Ctrl Pts',(-6.73866551900006,15.2,-8.34555437100001));
#285059=CARTESIAN_POINT('Ctrl Pts',(-6.73866551900006,11.6,-8.34555437100001));
#285060=CARTESIAN_POINT('Ctrl Pts',(-6.73964833200006,15.2,-8.34782559500002));
#285061=CARTESIAN_POINT('Ctrl Pts',(-6.73964833200006,11.6,-8.34782559500002));
#285062=CARTESIAN_POINT('Ctrl Pts',(-6.74063164200006,15.2,-8.35010335100002));
#285063=CARTESIAN_POINT('Ctrl Pts',(-6.74063164200006,11.6,-8.35010335100002));
#285064=CARTESIAN_POINT('Ctrl Pts',(-6.74161543500006,15.2,-8.35238763300002));
#285065=CARTESIAN_POINT('Ctrl Pts',(-6.74161543500006,11.6,-8.35238763300002));
#285066=CARTESIAN_POINT('Ctrl Pts',(-6.74259969900006,15.2,-8.35467843300002));
#285067=CARTESIAN_POINT('Ctrl Pts',(-6.74259969900006,11.6,-8.35467843300002));
#285068=CARTESIAN_POINT('Ctrl Pts',(-6.74358442000006,15.2,-8.35697574500001));
#285069=CARTESIAN_POINT('Ctrl Pts',(-6.74358442000006,11.6,-8.35697574500001));
#285070=CARTESIAN_POINT('Ctrl Pts',(-6.74456958400006,15.2,-8.35927956000001));
#285071=CARTESIAN_POINT('Ctrl Pts',(-6.74456958400006,11.6,-8.35927956000001));
#285072=CARTESIAN_POINT('Ctrl Pts',(-6.74555517700006,15.2,-8.36158987000001));
#285073=CARTESIAN_POINT('Ctrl Pts',(-6.74555517700006,11.6,-8.36158987000001));
#285074=CARTESIAN_POINT('Ctrl Pts',(-6.74654118900006,15.2,-8.36390667000002));
#285075=CARTESIAN_POINT('Ctrl Pts',(-6.74654118900006,11.6,-8.36390667000002));
#285076=CARTESIAN_POINT('Ctrl Pts',(-6.74752760400006,15.2,-8.36622995200001));
#285077=CARTESIAN_POINT('Ctrl Pts',(-6.74752760400006,11.6,-8.36622995200001));
#285078=CARTESIAN_POINT('Ctrl Pts',(-6.74851441000006,15.2,-8.36855970800002));
#285079=CARTESIAN_POINT('Ctrl Pts',(-6.74851441000006,11.6,-8.36855970800002));
#285080=CARTESIAN_POINT('Ctrl Pts',(-6.74950159300006,15.2,-8.37089593100002));
#285081=CARTESIAN_POINT('Ctrl Pts',(-6.74950159300006,11.6,-8.37089593100002));
#285082=CARTESIAN_POINT('Ctrl Pts',(-6.75048914200006,15.2,-8.37323861500002));
#285083=CARTESIAN_POINT('Ctrl Pts',(-6.75048914200006,11.6,-8.37323861500002));
#285084=CARTESIAN_POINT('Ctrl Pts',(-6.75147704200006,15.2,-8.37558775000002));
#285085=CARTESIAN_POINT('Ctrl Pts',(-6.75147704200006,11.6,-8.37558775000002));
#285086=CARTESIAN_POINT('Ctrl Pts',(-6.75246528000006,15.2,-8.37794333100002));
#285087=CARTESIAN_POINT('Ctrl Pts',(-6.75246528000006,11.6,-8.37794333100002));
#285088=CARTESIAN_POINT('Ctrl Pts',(-6.75345384400006,15.2,-8.38030535000001));
#285089=CARTESIAN_POINT('Ctrl Pts',(-6.75345384400006,11.6,-8.38030535000001));
#285090=CARTESIAN_POINT('Ctrl Pts',(-6.75444272200005,15.2,-8.38267380000002));
#285091=CARTESIAN_POINT('Ctrl Pts',(-6.75444272200005,11.6,-8.38267380000002));
#285092=CARTESIAN_POINT('Ctrl Pts',(-6.75543189900006,15.2,-8.38504867300001));
#285093=CARTESIAN_POINT('Ctrl Pts',(-6.75543189900006,11.6,-8.38504867300001));
#285094=CARTESIAN_POINT('Ctrl Pts',(-6.75642136400006,15.2,-8.38742996300001));
#285095=CARTESIAN_POINT('Ctrl Pts',(-6.75642136400006,11.6,-8.38742996300001));
#285096=CARTESIAN_POINT('Ctrl Pts',(-6.75741110400006,15.2,-8.38981766200002));
#285097=CARTESIAN_POINT('Ctrl Pts',(-6.75741110400006,11.6,-8.38981766200002));
#285098=CARTESIAN_POINT('Ctrl Pts',(-6.75840110500006,15.2,-8.39221176300001));
#285099=CARTESIAN_POINT('Ctrl Pts',(-6.75840110500006,11.6,-8.39221176300001));
#285100=CARTESIAN_POINT('Ctrl Pts',(-6.75939135700006,15.2,-8.39461225900001));
#285101=CARTESIAN_POINT('Ctrl Pts',(-6.75939135700006,11.6,-8.39461225900001));
#285102=CARTESIAN_POINT('Ctrl Pts',(-6.76038184400006,15.2,-8.39701914200001));
#285103=CARTESIAN_POINT('Ctrl Pts',(-6.76038184400006,11.6,-8.39701914200001));
#285104=CARTESIAN_POINT('Ctrl Pts',(-6.76137255500006,15.2,-8.39943240700002));
#285105=CARTESIAN_POINT('Ctrl Pts',(-6.76137255500006,11.6,-8.39943240700002));
#285106=CARTESIAN_POINT('Ctrl Pts',(-6.76236347800006,15.2,-8.40185204500001));
#285107=CARTESIAN_POINT('Ctrl Pts',(-6.76236347800006,11.6,-8.40185204500001));
#285108=CARTESIAN_POINT('Ctrl Pts',(-6.76335460000006,15.2,-8.40427804800001));
#285109=CARTESIAN_POINT('Ctrl Pts',(-6.76335460000006,11.6,-8.40427804800001));
#285110=CARTESIAN_POINT('Ctrl Pts',(-6.76434590800006,15.2,-8.40671041100002));
#285111=CARTESIAN_POINT('Ctrl Pts',(-6.76434590800006,11.6,-8.40671041100002));
#285112=CARTESIAN_POINT('Ctrl Pts',(-6.76533739000006,15.2,-8.40914912700002));
#285113=CARTESIAN_POINT('Ctrl Pts',(-6.76533739000006,11.6,-8.40914912700002));
#285114=CARTESIAN_POINT('Ctrl Pts',(-6.76632903400006,15.2,-8.41159418600002));
#285115=CARTESIAN_POINT('Ctrl Pts',(-6.76632903400006,11.6,-8.41159418600002));
#285116=CARTESIAN_POINT('Ctrl Pts',(-6.76732082700005,15.2,-8.41404558300002));
#285117=CARTESIAN_POINT('Ctrl Pts',(-6.76732082700005,11.6,-8.41404558300002));
#285118=CARTESIAN_POINT('Ctrl Pts',(-6.76831275600006,15.2,-8.41650331100002));
#285119=CARTESIAN_POINT('Ctrl Pts',(-6.76831275600006,11.6,-8.41650331100002));
#285120=CARTESIAN_POINT('Ctrl Pts',(-6.76930481100006,15.2,-8.41896736400002));
#285121=CARTESIAN_POINT('Ctrl Pts',(-6.76930481100006,11.6,-8.41896736400002));
#285122=CARTESIAN_POINT('Ctrl Pts',(-6.77029697800006,15.2,-8.42143773200002));
#285123=CARTESIAN_POINT('Ctrl Pts',(-6.77029697800006,11.6,-8.42143773200002));
#285124=CARTESIAN_POINT('Ctrl Pts',(-6.77128924400006,15.2,-8.42391441000002));
#285125=CARTESIAN_POINT('Ctrl Pts',(-6.77128924400006,11.6,-8.42391441000002));
#285126=CARTESIAN_POINT('Ctrl Pts',(-6.77228160000006,15.2,-8.42639739000001));
#285127=CARTESIAN_POINT('Ctrl Pts',(-6.77228160000006,11.6,-8.42639739000001));
#285128=CARTESIAN_POINT('Ctrl Pts',(-6.77327403000006,15.2,-8.42888666600001));
#285129=CARTESIAN_POINT('Ctrl Pts',(-6.77327403000006,11.6,-8.42888666600001));
#285130=CARTESIAN_POINT('Ctrl Pts',(-6.77426652500006,15.2,-8.43138223000001));
#285131=CARTESIAN_POINT('Ctrl Pts',(-6.77426652500006,11.6,-8.43138223000001));
#285132=CARTESIAN_POINT('Ctrl Pts',(-6.77525907000006,15.2,-8.43388407500001));
#285133=CARTESIAN_POINT('Ctrl Pts',(-6.77525907000006,11.6,-8.43388407500001));
#285134=CARTESIAN_POINT('Ctrl Pts',(-6.77625165600006,15.2,-8.43639219400002));
#285135=CARTESIAN_POINT('Ctrl Pts',(-6.77625165600006,11.6,-8.43639219400002));
#285136=CARTESIAN_POINT('Ctrl Pts',(-6.77724426900006,15.2,-8.43890658100002));
#285137=CARTESIAN_POINT('Ctrl Pts',(-6.77724426900006,11.6,-8.43890658100002));
#285138=CARTESIAN_POINT('Ctrl Pts',(-6.77823689800006,15.2,-8.44142722800001));
#285139=CARTESIAN_POINT('Ctrl Pts',(-6.77823689800006,11.6,-8.44142722800001));
#285140=CARTESIAN_POINT('Ctrl Pts',(-6.77922953100006,15.2,-8.44395412900001));
#285141=CARTESIAN_POINT('Ctrl Pts',(-6.77922953100006,11.6,-8.44395412900001));
#285142=CARTESIAN_POINT('Ctrl Pts',(-6.78022215500006,15.2,-8.44648727600001));
#285143=CARTESIAN_POINT('Ctrl Pts',(-6.78022215500006,11.6,-8.44648727600001));
#285144=CARTESIAN_POINT('Ctrl Pts',(-6.78121475800006,15.2,-8.44902666100002));
#285145=CARTESIAN_POINT('Ctrl Pts',(-6.78121475800006,11.6,-8.44902666100002));
#285146=CARTESIAN_POINT('Ctrl Pts',(-6.78220733100006,15.2,-8.45157227900001));
#285147=CARTESIAN_POINT('Ctrl Pts',(-6.78220733100006,11.6,-8.45157227900001));
#285148=CARTESIAN_POINT('Ctrl Pts',(-6.78319986000006,15.2,-8.45412412300002));
#285149=CARTESIAN_POINT('Ctrl Pts',(-6.78319986000006,11.6,-8.45412412300002));
#285150=CARTESIAN_POINT('Ctrl Pts',(-6.78419233200006,15.2,-8.45668218600002));
#285151=CARTESIAN_POINT('Ctrl Pts',(-6.78419233200006,11.6,-8.45668218600002));
#285152=CARTESIAN_POINT('Ctrl Pts',(-6.78518473900006,15.2,-8.45924645900002));
#285153=CARTESIAN_POINT('Ctrl Pts',(-6.78518473900006,11.6,-8.45924645900002));
#285154=CARTESIAN_POINT('Ctrl Pts',(-6.78617706600006,15.2,-8.46181693800002));
#285155=CARTESIAN_POINT('Ctrl Pts',(-6.78617706600006,11.6,-8.46181693800002));
#285156=CARTESIAN_POINT('Ctrl Pts',(-6.78716930300006,15.2,-8.46439361500002));
#285157=CARTESIAN_POINT('Ctrl Pts',(-6.78716930300006,11.6,-8.46439361500002));
#285158=CARTESIAN_POINT('Ctrl Pts',(-6.78816143700006,15.2,-8.46697648200001));
#285159=CARTESIAN_POINT('Ctrl Pts',(-6.78816143700006,11.6,-8.46697648200001));
#285160=CARTESIAN_POINT('Ctrl Pts',(-6.78915345800006,15.2,-8.46956553300002));
#285161=CARTESIAN_POINT('Ctrl Pts',(-6.78915345800006,11.6,-8.46956553300002));
#285162=CARTESIAN_POINT('Ctrl Pts',(-6.79014535300006,15.2,-8.47216076000001));
#285163=CARTESIAN_POINT('Ctrl Pts',(-6.79014535300006,11.6,-8.47216076000001));
#285164=CARTESIAN_POINT('Ctrl Pts',(-6.79113711200006,15.2,-8.47476215800001));
#285165=CARTESIAN_POINT('Ctrl Pts',(-6.79113711200006,11.6,-8.47476215800001));
#285166=CARTESIAN_POINT('Ctrl Pts',(-6.79212872200006,15.2,-8.47736971900002));
#285167=CARTESIAN_POINT('Ctrl Pts',(-6.79212872200006,11.6,-8.47736971900002));
#285168=CARTESIAN_POINT('Ctrl Pts',(-6.79312017300005,15.2,-8.47998343700001));
#285169=CARTESIAN_POINT('Ctrl Pts',(-6.79312017300005,11.6,-8.47998343700001));
#285170=CARTESIAN_POINT('Ctrl Pts',(-6.79411145300006,15.2,-8.48260330400001));
#285171=CARTESIAN_POINT('Ctrl Pts',(-6.79411145300006,11.6,-8.48260330400001));
#285172=CARTESIAN_POINT('Ctrl Pts',(-6.79510255000006,15.2,-8.48522931400002));
#285173=CARTESIAN_POINT('Ctrl Pts',(-6.79510255000006,11.6,-8.48522931400002));
#285174=CARTESIAN_POINT('Ctrl Pts',(-6.79609345300006,15.2,-8.48786145900002));
#285175=CARTESIAN_POINT('Ctrl Pts',(-6.79609345300006,11.6,-8.48786145900002));
#285176=CARTESIAN_POINT('Ctrl Pts',(-6.79708415200006,15.2,-8.49049973300002));
#285177=CARTESIAN_POINT('Ctrl Pts',(-6.79708415200006,11.6,-8.49049973300002));
#285178=CARTESIAN_POINT('Ctrl Pts',(-6.79807463300006,15.2,-8.49314413000002));
#285179=CARTESIAN_POINT('Ctrl Pts',(-6.79807463300006,11.6,-8.49314413000002));
#285180=CARTESIAN_POINT('Ctrl Pts',(-6.79906488700006,15.2,-8.49579464200002));
#285181=CARTESIAN_POINT('Ctrl Pts',(-6.79906488700006,11.6,-8.49579464200002));
#285182=CARTESIAN_POINT('Ctrl Pts',(-6.80005490300006,15.2,-8.49845126300002));
#285183=CARTESIAN_POINT('Ctrl Pts',(-6.80005490300006,11.6,-8.49845126300002));
#285184=CARTESIAN_POINT('Ctrl Pts',(-6.80104466800006,15.2,-8.50111398400001));
#285185=CARTESIAN_POINT('Ctrl Pts',(-6.80104466800006,11.6,-8.50111398400001));
#285186=CARTESIAN_POINT('Ctrl Pts',(-6.80203417100006,15.2,-8.50378280200001));
#285187=CARTESIAN_POINT('Ctrl Pts',(-6.80203417100006,11.6,-8.50378280200001));
#285188=CARTESIAN_POINT('Ctrl Pts',(-6.80302340200006,15.2,-8.50645770700002));
#285189=CARTESIAN_POINT('Ctrl Pts',(-6.80302340200006,11.6,-8.50645770700002));
#285190=CARTESIAN_POINT('Ctrl Pts',(-6.80401234900006,15.2,-8.50913869300001));
#285191=CARTESIAN_POINT('Ctrl Pts',(-6.80401234900006,11.6,-8.50913869300001));
#285192=CARTESIAN_POINT('Ctrl Pts',(-6.80500100400006,15.2,-8.51182575500001));
#285193=CARTESIAN_POINT('Ctrl Pts',(-6.80500100400006,11.6,-8.51182575500001));
#285194=CARTESIAN_POINT('Ctrl Pts',(-6.80598935100006,15.2,-8.51451888400002));
#285195=CARTESIAN_POINT('Ctrl Pts',(-6.80598935100006,11.6,-8.51451888400002));
#285196=CARTESIAN_POINT('Ctrl Pts',(-6.80697738200006,15.2,-8.51721807500001));
#285197=CARTESIAN_POINT('Ctrl Pts',(-6.80697738200006,11.6,-8.51721807500001));
#285198=CARTESIAN_POINT('Ctrl Pts',(-6.80796508500006,15.2,-8.51992331800002));
#285199=CARTESIAN_POINT('Ctrl Pts',(-6.80796508500006,11.6,-8.51992331800002));
#285200=CARTESIAN_POINT('Ctrl Pts',(-6.80895244900006,15.2,-8.52263461100002));
#285201=CARTESIAN_POINT('Ctrl Pts',(-6.80895244900006,11.6,-8.52263461100002));
#285202=CARTESIAN_POINT('Ctrl Pts',(-6.80993946500006,15.2,-8.52535194300001));
#285203=CARTESIAN_POINT('Ctrl Pts',(-6.80993946500006,11.6,-8.52535194300001));
#285204=CARTESIAN_POINT('Ctrl Pts',(-6.81092612100006,15.2,-8.52807531000002));
#285205=CARTESIAN_POINT('Ctrl Pts',(-6.81092612100006,11.6,-8.52807531000002));
#285206=CARTESIAN_POINT('Ctrl Pts',(-6.81191240500006,15.2,-8.53080470500002));
#285207=CARTESIAN_POINT('Ctrl Pts',(-6.81191240500006,11.6,-8.53080470500002));
#285208=CARTESIAN_POINT('Ctrl Pts',(-6.81289830700006,15.2,-8.53354012000001));
#285209=CARTESIAN_POINT('Ctrl Pts',(-6.81289830700006,11.6,-8.53354012000001));
#285210=CARTESIAN_POINT('Ctrl Pts',(-6.81388381700006,15.2,-8.53628154900001));
#285211=CARTESIAN_POINT('Ctrl Pts',(-6.81388381700006,11.6,-8.53628154900001));
#285212=CARTESIAN_POINT('Ctrl Pts',(-6.81486892200006,15.2,-8.53902898500002));
#285213=CARTESIAN_POINT('Ctrl Pts',(-6.81486892200006,11.6,-8.53902898500002));
#285214=CARTESIAN_POINT('Ctrl Pts',(-6.81585361400006,15.2,-8.54178242200001));
#285215=CARTESIAN_POINT('Ctrl Pts',(-6.81585361400006,11.6,-8.54178242200001));
#285216=CARTESIAN_POINT('Ctrl Pts',(-6.81683788100006,15.2,-8.54454185300002));
#285217=CARTESIAN_POINT('Ctrl Pts',(-6.81683788100006,11.6,-8.54454185300002));
#285218=CARTESIAN_POINT('Ctrl Pts',(-6.81782171200005,15.2,-8.54730727200002));
#285219=CARTESIAN_POINT('Ctrl Pts',(-6.81782171200005,11.6,-8.54730727200002));
#285220=CARTESIAN_POINT('Ctrl Pts',(-6.81880509800005,15.2,-8.55007867000002));
#285221=CARTESIAN_POINT('Ctrl Pts',(-6.81880509800005,11.6,-8.55007867000002));
#285222=CARTESIAN_POINT('Ctrl Pts',(-6.81978802600006,15.2,-8.55285604300001));
#285223=CARTESIAN_POINT('Ctrl Pts',(-6.81978802600006,11.6,-8.55285604300001));
#285224=CARTESIAN_POINT('Ctrl Pts',(-6.82077048700005,15.2,-8.55563938300002));
#285225=CARTESIAN_POINT('Ctrl Pts',(-6.82077048700005,11.6,-8.55563938300002));
#285226=CARTESIAN_POINT('Ctrl Pts',(-6.82175247000006,15.2,-8.55842868400002));
#285227=CARTESIAN_POINT('Ctrl Pts',(-6.82175247000006,11.6,-8.55842868400002));
#285228=CARTESIAN_POINT('Ctrl Pts',(-6.82273396500006,15.2,-8.56122393900002));
#285229=CARTESIAN_POINT('Ctrl Pts',(-6.82273396500006,11.6,-8.56122393900002));
#285230=CARTESIAN_POINT('Ctrl Pts',(-6.82371496100005,15.2,-8.56402514100001));
#285231=CARTESIAN_POINT('Ctrl Pts',(-6.82371496100005,11.6,-8.56402514100001));
#285232=CARTESIAN_POINT('Ctrl Pts',(-6.82469544700006,15.2,-8.56683228400002));
#285233=CARTESIAN_POINT('Ctrl Pts',(-6.82469544700006,11.6,-8.56683228400002));
#285234=CARTESIAN_POINT('Ctrl Pts',(-6.82567541400006,15.2,-8.56964536100002));
#285235=CARTESIAN_POINT('Ctrl Pts',(-6.82567541400006,11.6,-8.56964536100002));
#285236=CARTESIAN_POINT('Ctrl Pts',(-6.82665485100006,15.2,-8.57246436600001));
#285237=CARTESIAN_POINT('Ctrl Pts',(-6.82665485100006,11.6,-8.57246436600001));
#285238=CARTESIAN_POINT('Ctrl Pts',(-6.82763374600006,15.2,-8.57528929200001));
#285239=CARTESIAN_POINT('Ctrl Pts',(-6.82763374600006,11.6,-8.57528929200001));
#285240=CARTESIAN_POINT('Ctrl Pts',(-6.82861209100006,15.2,-8.57812013100002));
#285241=CARTESIAN_POINT('Ctrl Pts',(-6.82861209100006,11.6,-8.57812013100002));
#285242=CARTESIAN_POINT('Ctrl Pts',(-6.82958987600006,15.2,-8.58095688000001));
#285243=CARTESIAN_POINT('Ctrl Pts',(-6.82958987600006,11.6,-8.58095688000001));
#285244=CARTESIAN_POINT('Ctrl Pts',(-6.83056708700006,15.2,-8.58379952900002));
#285245=CARTESIAN_POINT('Ctrl Pts',(-6.83056708700006,11.6,-8.58379952900002));
#285246=CARTESIAN_POINT('Ctrl Pts',(-6.83154371800006,15.2,-8.58664807300002));
#285247=CARTESIAN_POINT('Ctrl Pts',(-6.83154371800006,11.6,-8.58664807300002));
#285248=CARTESIAN_POINT('Ctrl Pts',(-6.83251975600006,15.2,-8.58950250500002));
#285249=CARTESIAN_POINT('Ctrl Pts',(-6.83251975600006,11.6,-8.58950250500002));
#285250=CARTESIAN_POINT('Ctrl Pts',(-6.83349519400006,15.2,-8.59236281800002));
#285251=CARTESIAN_POINT('Ctrl Pts',(-6.83349519400006,11.6,-8.59236281800002));
#285252=CARTESIAN_POINT('Ctrl Pts',(-6.83447001700006,15.2,-8.59522900700001));
#285253=CARTESIAN_POINT('Ctrl Pts',(-6.83447001700006,11.6,-8.59522900700001));
#285254=CARTESIAN_POINT('Ctrl Pts',(-6.83544421900006,15.2,-8.59810106300002));
#285255=CARTESIAN_POINT('Ctrl Pts',(-6.83544421900006,11.6,-8.59810106300002));
#285256=CARTESIAN_POINT('Ctrl Pts',(-6.83641778800006,15.2,-8.60097898100002));
#285257=CARTESIAN_POINT('Ctrl Pts',(-6.83641778800006,11.6,-8.60097898100002));
#285258=CARTESIAN_POINT('Ctrl Pts',(-6.83739071400006,15.2,-8.60386275500002));
#285259=CARTESIAN_POINT('Ctrl Pts',(-6.83739071400006,11.6,-8.60386275500002));
#285260=CARTESIAN_POINT('Ctrl Pts',(-6.83836298800006,15.2,-8.60675237800002));
#285261=CARTESIAN_POINT('Ctrl Pts',(-6.83836298800006,11.6,-8.60675237800002));
#285262=CARTESIAN_POINT('Ctrl Pts',(-6.83933459800006,15.2,-8.60964784300002));
#285263=CARTESIAN_POINT('Ctrl Pts',(-6.83933459800006,11.6,-8.60964784300002));
#285264=CARTESIAN_POINT('Ctrl Pts',(-6.84030553600006,15.2,-8.61254914500002));
#285265=CARTESIAN_POINT('Ctrl Pts',(-6.84030553600006,11.6,-8.61254914500002));
#285266=CARTESIAN_POINT('Ctrl Pts',(-6.84127579200006,15.2,-8.61545627500002));
#285267=CARTESIAN_POINT('Ctrl Pts',(-6.84127579200006,11.6,-8.61545627500002));
#285268=CARTESIAN_POINT('Ctrl Pts',(-6.84224535400006,15.2,-8.61836922800002));
#285269=CARTESIAN_POINT('Ctrl Pts',(-6.84224535400006,11.6,-8.61836922800002));
#285270=CARTESIAN_POINT('Ctrl Pts',(-6.84321421300006,15.2,-8.62128799800002));
#285271=CARTESIAN_POINT('Ctrl Pts',(-6.84321421300006,11.6,-8.62128799800002));
#285272=CARTESIAN_POINT('Ctrl Pts',(-6.84418236000006,15.2,-8.62421257800002));
#285273=CARTESIAN_POINT('Ctrl Pts',(-6.84418236000006,11.6,-8.62421257800002));
#285274=CARTESIAN_POINT('Ctrl Pts',(-6.84514978400006,15.2,-8.62714296000001));
#285275=CARTESIAN_POINT('Ctrl Pts',(-6.84514978400006,11.6,-8.62714296000001));
#285276=CARTESIAN_POINT('Ctrl Pts',(-6.84611647700006,15.2,-8.63007914000002));
#285277=CARTESIAN_POINT('Ctrl Pts',(-6.84611647700006,11.6,-8.63007914000002));
#285278=CARTESIAN_POINT('Ctrl Pts',(-6.84708242700006,15.2,-8.63302111000002));
#285279=CARTESIAN_POINT('Ctrl Pts',(-6.84708242700006,11.6,-8.63302111000002));
#285280=CARTESIAN_POINT('Ctrl Pts',(-6.84804762500006,15.2,-8.63596886400002));
#285281=CARTESIAN_POINT('Ctrl Pts',(-6.84804762500006,11.6,-8.63596886400002));
#285282=CARTESIAN_POINT('Ctrl Pts',(-6.84901206200006,15.2,-8.63892239500002));
#285283=CARTESIAN_POINT('Ctrl Pts',(-6.84901206200006,11.6,-8.63892239500002));
#285284=CARTESIAN_POINT('Ctrl Pts',(-6.84997572700006,15.2,-8.64188169800002));
#285285=CARTESIAN_POINT('Ctrl Pts',(-6.84997572700006,11.6,-8.64188169800002));
#285286=CARTESIAN_POINT('Ctrl Pts',(-6.85093861100006,15.2,-8.64484676500001));
#285287=CARTESIAN_POINT('Ctrl Pts',(-6.85093861100006,11.6,-8.64484676500001));
#285288=CARTESIAN_POINT('Ctrl Pts',(-6.85190070400005,15.2,-8.64781759100002));
#285289=CARTESIAN_POINT('Ctrl Pts',(-6.85190070400005,11.6,-8.64781759100002));
#285290=CARTESIAN_POINT('Ctrl Pts',(-6.85286199700006,15.2,-8.65079416800001));
#285291=CARTESIAN_POINT('Ctrl Pts',(-6.85286199700006,11.6,-8.65079416800001));
#285292=CARTESIAN_POINT('Ctrl Pts',(-6.85382248000006,15.2,-8.65377649100001));
#285293=CARTESIAN_POINT('Ctrl Pts',(-6.85382248000006,11.6,-8.65377649100001));
#285294=CARTESIAN_POINT('Ctrl Pts',(-6.85478214300006,15.2,-8.65676455300001));
#285295=CARTESIAN_POINT('Ctrl Pts',(-6.85478214300006,11.6,-8.65676455300001));
#285296=CARTESIAN_POINT('Ctrl Pts',(-6.85574097600006,15.2,-8.65975834700001));
#285297=CARTESIAN_POINT('Ctrl Pts',(-6.85574097600006,11.6,-8.65975834700001));
#285298=CARTESIAN_POINT('Ctrl Pts',(-6.85669897100006,15.2,-8.66275786700001));
#285299=CARTESIAN_POINT('Ctrl Pts',(-6.85669897100006,11.6,-8.66275786700001));
#285300=CARTESIAN_POINT('Ctrl Pts',(-6.85765611700006,15.2,-8.66576310700001));
#285301=CARTESIAN_POINT('Ctrl Pts',(-6.85765611700006,11.6,-8.66576310700001));
#285302=CARTESIAN_POINT('Ctrl Pts',(-6.85861240500006,15.2,-8.66877406100001));
#285303=CARTESIAN_POINT('Ctrl Pts',(-6.85861240500006,11.6,-8.66877406100001));
#285304=CARTESIAN_POINT('Ctrl Pts',(-6.85956782600006,15.2,-8.67179072200001));
#285305=CARTESIAN_POINT('Ctrl Pts',(-6.85956782600006,11.6,-8.67179072200001));
#285306=CARTESIAN_POINT('Ctrl Pts',(-6.86052237000006,15.2,-8.67481308300002));
#285307=CARTESIAN_POINT('Ctrl Pts',(-6.86052237000006,11.6,-8.67481308300002));
#285308=CARTESIAN_POINT('Ctrl Pts',(-6.86147602800006,15.2,-8.67784113800001));
#285309=CARTESIAN_POINT('Ctrl Pts',(-6.86147602800006,11.6,-8.67784113800001));
#285310=CARTESIAN_POINT('Ctrl Pts',(-6.86242879000006,15.2,-8.68087488200001));
#285311=CARTESIAN_POINT('Ctrl Pts',(-6.86242879000006,11.6,-8.68087488200001));
#285312=CARTESIAN_POINT('Ctrl Pts',(-6.86338064600006,15.2,-8.68391430700001));
#285313=CARTESIAN_POINT('Ctrl Pts',(-6.86338064600006,11.6,-8.68391430700001));
#285314=CARTESIAN_POINT('Ctrl Pts',(-6.86433158900006,15.2,-8.68695940700002));
#285315=CARTESIAN_POINT('Ctrl Pts',(-6.86433158900006,11.6,-8.68695940700002));
#285316=CARTESIAN_POINT('Ctrl Pts',(-6.86528160700006,15.2,-8.69001017600001));
#285317=CARTESIAN_POINT('Ctrl Pts',(-6.86528160700006,11.6,-8.69001017600001));
#285318=CARTESIAN_POINT('Ctrl Pts',(-6.86623069200006,15.2,-8.69306660700002));
#285319=CARTESIAN_POINT('Ctrl Pts',(-6.86623069200006,11.6,-8.69306660700002));
#285320=CARTESIAN_POINT('Ctrl Pts',(-6.86717883600005,15.2,-8.69612869500001));
#285321=CARTESIAN_POINT('Ctrl Pts',(-6.86717883600005,11.6,-8.69612869500001));
#285322=CARTESIAN_POINT('Ctrl Pts',(-6.86812602700006,15.2,-8.69919643300002));
#285323=CARTESIAN_POINT('Ctrl Pts',(-6.86812602700006,11.6,-8.69919643300002));
#285324=CARTESIAN_POINT('Ctrl Pts',(-6.86907225800006,15.2,-8.70226981300002));
#285325=CARTESIAN_POINT('Ctrl Pts',(-6.86907225800006,11.6,-8.70226981300002));
#285326=CARTESIAN_POINT('Ctrl Pts',(-6.87001751800006,15.2,-8.70534883200002));
#285327=CARTESIAN_POINT('Ctrl Pts',(-6.87001751800006,11.6,-8.70534883200002));
#285328=CARTESIAN_POINT('Ctrl Pts',(-6.87096179900006,15.2,-8.70843348100001));
#285329=CARTESIAN_POINT('Ctrl Pts',(-6.87096179900006,11.6,-8.70843348100001));
#285330=CARTESIAN_POINT('Ctrl Pts',(-6.87190509000006,15.2,-8.71152375400002));
#285331=CARTESIAN_POINT('Ctrl Pts',(-6.87190509000006,11.6,-8.71152375400002));
#285332=CARTESIAN_POINT('Ctrl Pts',(-6.87284738500006,15.2,-8.71461964600002));
#285333=CARTESIAN_POINT('Ctrl Pts',(-6.87284738500006,11.6,-8.71461964600002));
#285334=CARTESIAN_POINT('Ctrl Pts',(-6.87378867400006,15.2,-8.71772115000002));
#285335=CARTESIAN_POINT('Ctrl Pts',(-6.87378867400006,11.6,-8.71772115000002));
#285336=CARTESIAN_POINT('Ctrl Pts',(-6.87472894500006,15.2,-8.72082826000002));
#285337=CARTESIAN_POINT('Ctrl Pts',(-6.87472894500006,11.6,-8.72082826000002));
#285338=CARTESIAN_POINT('Ctrl Pts',(-6.87566819300006,15.2,-8.72394096800001));
#285339=CARTESIAN_POINT('Ctrl Pts',(-6.87566819300006,11.6,-8.72394096800001));
#285340=CARTESIAN_POINT('Ctrl Pts',(-6.87660640700006,15.2,-8.72705927100002));
#285341=CARTESIAN_POINT('Ctrl Pts',(-6.87660640700006,11.6,-8.72705927100002));
#285342=CARTESIAN_POINT('Ctrl Pts',(-6.87754357700006,15.2,-8.73018316100002));
#285343=CARTESIAN_POINT('Ctrl Pts',(-6.87754357700006,11.6,-8.73018316100002));
#285344=CARTESIAN_POINT('Ctrl Pts',(-6.87847969500006,15.2,-8.73331263000001));
#285345=CARTESIAN_POINT('Ctrl Pts',(-6.87847969500006,11.6,-8.73331263000001));
#285346=CARTESIAN_POINT('Ctrl Pts',(-6.87941475200006,15.2,-8.73644767400001));
#285347=CARTESIAN_POINT('Ctrl Pts',(-6.87941475200006,11.6,-8.73644767400001));
#285348=CARTESIAN_POINT('Ctrl Pts',(-6.88034873900006,15.2,-8.73958828600001));
#285349=CARTESIAN_POINT('Ctrl Pts',(-6.88034873900006,11.6,-8.73958828600001));
#285350=CARTESIAN_POINT('Ctrl Pts',(-6.88128164800006,15.2,-8.74273446000002));
#285351=CARTESIAN_POINT('Ctrl Pts',(-6.88128164800006,11.6,-8.74273446000002));
#285352=CARTESIAN_POINT('Ctrl Pts',(-6.88221346800006,15.2,-8.74588619000002));
#285353=CARTESIAN_POINT('Ctrl Pts',(-6.88221346800006,11.6,-8.74588619000002));
#285354=CARTESIAN_POINT('Ctrl Pts',(-6.88314419200006,15.2,-8.74904347000001));
#285355=CARTESIAN_POINT('Ctrl Pts',(-6.88314419200006,11.6,-8.74904347000001));
#285356=CARTESIAN_POINT('Ctrl Pts',(-6.88407381100006,15.2,-8.75220629200001));
#285357=CARTESIAN_POINT('Ctrl Pts',(-6.88407381100006,11.6,-8.75220629200001));
#285358=CARTESIAN_POINT('Ctrl Pts',(-6.88500231400006,15.2,-8.75537465100001));
#285359=CARTESIAN_POINT('Ctrl Pts',(-6.88500231400006,11.6,-8.75537465100001));
#285360=CARTESIAN_POINT('Ctrl Pts',(-6.88592969500006,15.2,-8.75854854100002));
#285361=CARTESIAN_POINT('Ctrl Pts',(-6.88592969500006,11.6,-8.75854854100002));
#285362=CARTESIAN_POINT('Ctrl Pts',(-6.88685594400006,15.2,-8.76172795500001));
#285363=CARTESIAN_POINT('Ctrl Pts',(-6.88685594400006,11.6,-8.76172795500001));
#285364=CARTESIAN_POINT('Ctrl Pts',(-6.88778105300006,15.2,-8.76491288800001));
#285365=CARTESIAN_POINT('Ctrl Pts',(-6.88778105300006,11.6,-8.76491288800001));
#285366=CARTESIAN_POINT('Ctrl Pts',(-6.88870501100006,15.2,-8.76810333200002));
#285367=CARTESIAN_POINT('Ctrl Pts',(-6.88870501100006,11.6,-8.76810333200002));
#285368=CARTESIAN_POINT('Ctrl Pts',(-6.88962781100006,15.2,-8.77129928300001));
#285369=CARTESIAN_POINT('Ctrl Pts',(-6.88962781100006,11.6,-8.77129928300001));
#285370=CARTESIAN_POINT('Ctrl Pts',(-6.89054944500006,15.2,-8.77450073400002));
#285371=CARTESIAN_POINT('Ctrl Pts',(-6.89054944500006,11.6,-8.77450073400002));
#285372=CARTESIAN_POINT('Ctrl Pts',(-6.89146990300006,15.2,-8.77770767800002));
#285373=CARTESIAN_POINT('Ctrl Pts',(-6.89146990300006,11.6,-8.77770767800002));
#285374=CARTESIAN_POINT('Ctrl Pts',(-6.89238917600006,15.2,-8.78092010900002));
#285375=CARTESIAN_POINT('Ctrl Pts',(-6.89238917600006,11.6,-8.78092010900002));
#285376=CARTESIAN_POINT('Ctrl Pts',(-6.89330725700006,15.2,-8.78413802100001));
#285377=CARTESIAN_POINT('Ctrl Pts',(-6.89330725700006,11.6,-8.78413802100001));
#285378=CARTESIAN_POINT('Ctrl Pts',(-6.89422413500006,15.2,-8.78736140900001));
#285379=CARTESIAN_POINT('Ctrl Pts',(-6.89422413500006,11.6,-8.78736140900001));
#285380=CARTESIAN_POINT('Ctrl Pts',(-6.89513980400006,15.2,-8.79059026500002));
#285381=CARTESIAN_POINT('Ctrl Pts',(-6.89513980400006,11.6,-8.79059026500002));
#285382=CARTESIAN_POINT('Ctrl Pts',(-6.89605425400006,15.2,-8.79382458400002));
#285383=CARTESIAN_POINT('Ctrl Pts',(-6.89605425400006,11.6,-8.79382458400002));
#285384=CARTESIAN_POINT('Ctrl Pts',(-6.89696747600006,15.2,-8.79706435900001));
#285385=CARTESIAN_POINT('Ctrl Pts',(-6.89696747600006,11.6,-8.79706435900001));
#285386=CARTESIAN_POINT('Ctrl Pts',(-6.89787946300005,15.2,-8.80030958500001));
#285387=CARTESIAN_POINT('Ctrl Pts',(-6.89787946300005,11.6,-8.80030958500001));
#285388=CARTESIAN_POINT('Ctrl Pts',(-6.89879020600006,15.2,-8.80356025400001));
#285389=CARTESIAN_POINT('Ctrl Pts',(-6.89879020600006,11.6,-8.80356025400001));
#285390=CARTESIAN_POINT('Ctrl Pts',(-6.89969969600006,15.2,-8.80681636200002));
#285391=CARTESIAN_POINT('Ctrl Pts',(-6.89969969600006,11.6,-8.80681636200002));
#285392=CARTESIAN_POINT('Ctrl Pts',(-6.90060792400006,15.2,-8.81007790200002));
#285393=CARTESIAN_POINT('Ctrl Pts',(-6.90060792400006,11.6,-8.81007790200002));
#285394=CARTESIAN_POINT('Ctrl Pts',(-6.90151488200006,15.2,-8.81334486800002));
#285395=CARTESIAN_POINT('Ctrl Pts',(-6.90151488200006,11.6,-8.81334486800002));
#285396=CARTESIAN_POINT('Ctrl Pts',(-6.90242056300006,15.2,-8.81661725300001));
#285397=CARTESIAN_POINT('Ctrl Pts',(-6.90242056300006,11.6,-8.81661725300001));
#285398=CARTESIAN_POINT('Ctrl Pts',(-6.90332495800006,15.2,-8.81989505100002));
#285399=CARTESIAN_POINT('Ctrl Pts',(-6.90332495800006,11.6,-8.81989505100002));
#285400=CARTESIAN_POINT('Ctrl Pts',(-6.90422805600006,15.2,-8.82317825800002));
#285401=CARTESIAN_POINT('Ctrl Pts',(-6.90422805600006,11.6,-8.82317825800002));
#285402=CARTESIAN_POINT('Ctrl Pts',(-6.90512985200006,15.2,-8.82646686600001));
#285403=CARTESIAN_POINT('Ctrl Pts',(-6.90512985200006,11.6,-8.82646686600001));
#285404=CARTESIAN_POINT('Ctrl Pts',(-6.90603033600006,15.2,-8.82976086800002));
#285405=CARTESIAN_POINT('Ctrl Pts',(-6.90603033600006,11.6,-8.82976086800002));
#285406=CARTESIAN_POINT('Ctrl Pts',(-6.90692950100006,15.2,-8.83306026000002));
#285407=CARTESIAN_POINT('Ctrl Pts',(-6.90692950100006,11.6,-8.83306026000002));
#285408=CARTESIAN_POINT('Ctrl Pts',(-6.90782733600006,15.2,-8.83636503500002));
#285409=CARTESIAN_POINT('Ctrl Pts',(-6.90782733600006,11.6,-8.83636503500002));
#285410=CARTESIAN_POINT('Ctrl Pts',(-6.90872383500006,15.2,-8.83967518700001));
#285411=CARTESIAN_POINT('Ctrl Pts',(-6.90872383500006,11.6,-8.83967518700001));
#285412=CARTESIAN_POINT('Ctrl Pts',(-6.90961899000006,15.2,-8.84299071000001));
#285413=CARTESIAN_POINT('Ctrl Pts',(-6.90961899000006,11.6,-8.84299071000001));
#285414=CARTESIAN_POINT('Ctrl Pts',(-6.91051279100006,15.2,-8.84631159700002));
#285415=CARTESIAN_POINT('Ctrl Pts',(-6.91051279100006,11.6,-8.84631159700002));
#285416=CARTESIAN_POINT('Ctrl Pts',(-6.91140523100006,15.2,-8.84963784300002));
#285417=CARTESIAN_POINT('Ctrl Pts',(-6.91140523100006,11.6,-8.84963784300002));
#285418=CARTESIAN_POINT('Ctrl Pts',(-6.91229630100006,15.2,-8.85296944200002));
#285419=CARTESIAN_POINT('Ctrl Pts',(-6.91229630100006,11.6,-8.85296944200002));
#285420=CARTESIAN_POINT('Ctrl Pts',(-6.91318599400006,15.2,-8.85630638800002));
#285421=CARTESIAN_POINT('Ctrl Pts',(-6.91318599400006,11.6,-8.85630638800002));
#285422=CARTESIAN_POINT('Ctrl Pts',(-6.91407430200006,15.2,-8.85964867300002));
#285423=CARTESIAN_POINT('Ctrl Pts',(-6.91407430200006,11.6,-8.85964867300002));
#285424=CARTESIAN_POINT('Ctrl Pts',(-6.91496121500006,15.2,-8.86299629400002));
#285425=CARTESIAN_POINT('Ctrl Pts',(-6.91496121500006,11.6,-8.86299629400002));
#285426=CARTESIAN_POINT('Ctrl Pts',(-6.91584672600006,15.2,-8.86634924200001));
#285427=CARTESIAN_POINT('Ctrl Pts',(-6.91584672600006,11.6,-8.86634924200001));
#285428=CARTESIAN_POINT('Ctrl Pts',(-6.91673082700006,15.2,-8.86970751300002));
#285429=CARTESIAN_POINT('Ctrl Pts',(-6.91673082700006,11.6,-8.86970751300002));
#285430=CARTESIAN_POINT('Ctrl Pts',(-6.91761351000006,15.2,-8.87307110000001));
#285431=CARTESIAN_POINT('Ctrl Pts',(-6.91761351000006,11.6,-8.87307110000001));
#285432=CARTESIAN_POINT('Ctrl Pts',(-6.91849476600006,15.2,-8.87643999800002));
#285433=CARTESIAN_POINT('Ctrl Pts',(-6.91849476600006,11.6,-8.87643999800002));
#285434=CARTESIAN_POINT('Ctrl Pts',(-6.91937458800005,15.2,-8.87981420000001));
#285435=CARTESIAN_POINT('Ctrl Pts',(-6.91937458800005,11.6,-8.87981420000001));
#285436=CARTESIAN_POINT('Ctrl Pts',(-6.92025296800006,15.2,-8.88319369900002));
#285437=CARTESIAN_POINT('Ctrl Pts',(-6.92025296800006,11.6,-8.88319369900002));
#285438=CARTESIAN_POINT('Ctrl Pts',(-6.92112989800005,15.2,-8.88657849200002));
#285439=CARTESIAN_POINT('Ctrl Pts',(-6.92112989800005,11.6,-8.88657849200002));
#285440=CARTESIAN_POINT('Ctrl Pts',(-6.92200536800006,15.2,-8.88996857000001));
#285441=CARTESIAN_POINT('Ctrl Pts',(-6.92200536800006,11.6,-8.88996857000001));
#285442=CARTESIAN_POINT('Ctrl Pts',(-6.92287937300006,15.2,-8.89336392900002));
#285443=CARTESIAN_POINT('Ctrl Pts',(-6.92287937300006,11.6,-8.89336392900002));
#285444=CARTESIAN_POINT('Ctrl Pts',(-6.92375190400006,15.2,-8.89676456100002));
#285445=CARTESIAN_POINT('Ctrl Pts',(-6.92375190400006,11.6,-8.89676456100002));
#285446=CARTESIAN_POINT('Ctrl Pts',(-6.92462295300006,15.2,-8.90017046300001));
#285447=CARTESIAN_POINT('Ctrl Pts',(-6.92462295300006,11.6,-8.90017046300001));
#285448=CARTESIAN_POINT('Ctrl Pts',(-6.92549251200006,15.2,-8.90358162500002));
#285449=CARTESIAN_POINT('Ctrl Pts',(-6.92549251200006,11.6,-8.90358162500002));
#285450=CARTESIAN_POINT('Ctrl Pts',(-6.92636057200006,15.2,-8.90699804400001));
#285451=CARTESIAN_POINT('Ctrl Pts',(-6.92636057200006,11.6,-8.90699804400001));
#285452=CARTESIAN_POINT('Ctrl Pts',(-6.92722712700006,15.2,-8.91041971300002));
#285453=CARTESIAN_POINT('Ctrl Pts',(-6.92722712700006,11.6,-8.91041971300002));
#285454=CARTESIAN_POINT('Ctrl Pts',(-6.92809216800006,15.2,-8.91384662700002));
#285455=CARTESIAN_POINT('Ctrl Pts',(-6.92809216800006,11.6,-8.91384662700002));
#285456=CARTESIAN_POINT('Ctrl Pts',(-6.92895568900005,15.2,-8.91727877800001));
#285457=CARTESIAN_POINT('Ctrl Pts',(-6.92895568900005,11.6,-8.91727877800001));
#285458=CARTESIAN_POINT('Ctrl Pts',(-6.92981767900006,15.2,-8.92071616200001));
#285459=CARTESIAN_POINT('Ctrl Pts',(-6.92981767900006,11.6,-8.92071616200001));
#285460=CARTESIAN_POINT('Ctrl Pts',(-6.93067813200006,15.2,-8.92415877200002));
#285461=CARTESIAN_POINT('Ctrl Pts',(-6.93067813200006,11.6,-8.92415877200002));
#285462=CARTESIAN_POINT('Ctrl Pts',(-6.93153704100006,15.2,-8.92760660300001));
#285463=CARTESIAN_POINT('Ctrl Pts',(-6.93153704100006,11.6,-8.92760660300001));
#285464=CARTESIAN_POINT('Ctrl Pts',(-6.93239439700006,15.2,-8.93105964700002));
#285465=CARTESIAN_POINT('Ctrl Pts',(-6.93239439700006,11.6,-8.93105964700002));
#285466=CARTESIAN_POINT('Ctrl Pts',(-6.93325019300006,15.2,-8.93451789900002));
#285467=CARTESIAN_POINT('Ctrl Pts',(-6.93325019300006,11.6,-8.93451789900002));
#285468=CARTESIAN_POINT('Ctrl Pts',(-6.93410442200006,15.2,-8.93798135500001));
#285469=CARTESIAN_POINT('Ctrl Pts',(-6.93410442200006,11.6,-8.93798135500001));
#285470=CARTESIAN_POINT('Ctrl Pts',(-6.93495707400006,15.2,-8.94145000600002));
#285471=CARTESIAN_POINT('Ctrl Pts',(-6.93495707400006,11.6,-8.94145000600002));
#285472=CARTESIAN_POINT('Ctrl Pts',(-6.93580814300006,15.2,-8.94492384900002));
#285473=CARTESIAN_POINT('Ctrl Pts',(-6.93580814300006,11.6,-8.94492384900002));
#285474=CARTESIAN_POINT('Ctrl Pts',(-6.93665762200006,15.2,-8.94840287600001));
#285475=CARTESIAN_POINT('Ctrl Pts',(-6.93665762200006,11.6,-8.94840287600001));
#285476=CARTESIAN_POINT('Ctrl Pts',(-6.93750550100006,15.2,-8.95188708100001));
#285477=CARTESIAN_POINT('Ctrl Pts',(-6.93750550100006,11.6,-8.95188708100001));
#285478=CARTESIAN_POINT('Ctrl Pts',(-6.93835177400006,15.2,-8.95537645900001));
#285479=CARTESIAN_POINT('Ctrl Pts',(-6.93835177400006,11.6,-8.95537645900001));
#285480=CARTESIAN_POINT('Ctrl Pts',(-6.93919643300006,15.2,-8.95887100400002));
#285481=CARTESIAN_POINT('Ctrl Pts',(-6.93919643300006,11.6,-8.95887100400002));
#285482=CARTESIAN_POINT('Ctrl Pts',(-6.94003947100006,15.2,-8.96237071000002));
#285483=CARTESIAN_POINT('Ctrl Pts',(-6.94003947100006,11.6,-8.96237071000002));
#285484=CARTESIAN_POINT('Ctrl Pts',(-6.94088088100006,15.2,-8.96587557000002));
#285485=CARTESIAN_POINT('Ctrl Pts',(-6.94088088100006,11.6,-8.96587557000002));
#285486=CARTESIAN_POINT('Ctrl Pts',(-6.94172065300006,15.2,-8.96938558000001));
#285487=CARTESIAN_POINT('Ctrl Pts',(-6.94172065300006,11.6,-8.96938558000001));
#285488=CARTESIAN_POINT('Ctrl Pts',(-6.94255878100006,15.2,-8.97290073300002));
#285489=CARTESIAN_POINT('Ctrl Pts',(-6.94255878100006,11.6,-8.97290073300002));
#285490=CARTESIAN_POINT('Ctrl Pts',(-6.94339525800006,15.2,-8.97642102300001));
#285491=CARTESIAN_POINT('Ctrl Pts',(-6.94339525800006,11.6,-8.97642102300001));
#285492=CARTESIAN_POINT('Ctrl Pts',(-6.94423007700006,15.2,-8.97994644400002));
#285493=CARTESIAN_POINT('Ctrl Pts',(-6.94423007700006,11.6,-8.97994644400002));
#285494=CARTESIAN_POINT('Ctrl Pts',(-6.94506322800006,15.2,-8.98347699100002));
#285495=CARTESIAN_POINT('Ctrl Pts',(-6.94506322800006,11.6,-8.98347699100002));
#285496=CARTESIAN_POINT('Ctrl Pts',(-6.94589470500006,15.2,-8.98701265600002));
#285497=CARTESIAN_POINT('Ctrl Pts',(-6.94589470500006,11.6,-8.98701265600002));
#285498=CARTESIAN_POINT('Ctrl Pts',(-6.94672450200006,15.2,-8.99055343700002));
#285499=CARTESIAN_POINT('Ctrl Pts',(-6.94672450200006,11.6,-8.99055343700002));
#285500=CARTESIAN_POINT('Ctrl Pts',(-6.94755260900005,15.2,-8.99409932400001));
#285501=CARTESIAN_POINT('Ctrl Pts',(-6.94755260900005,11.6,-8.99409932400001));
#285502=CARTESIAN_POINT('Ctrl Pts',(-6.94837902000006,15.2,-8.99765031300002));
#285503=CARTESIAN_POINT('Ctrl Pts',(-6.94837902000006,11.6,-8.99765031300002));
#285504=CARTESIAN_POINT('Ctrl Pts',(-6.94920372700006,15.2,-9.00120639800001));
#285505=CARTESIAN_POINT('Ctrl Pts',(-6.94920372700006,11.6,-9.00120639800001));
#285506=CARTESIAN_POINT('Ctrl Pts',(-6.95002672400006,15.2,-9.00476757400002));
#285507=CARTESIAN_POINT('Ctrl Pts',(-6.95002672400006,11.6,-9.00476757400002));
#285508=CARTESIAN_POINT('Ctrl Pts',(-6.95084800200005,15.2,-9.00833383300002));
#285509=CARTESIAN_POINT('Ctrl Pts',(-6.95084800200005,11.6,-9.00833383300002));
#285510=CARTESIAN_POINT('Ctrl Pts',(-6.95166755500006,15.2,-9.01190517100002));
#285511=CARTESIAN_POINT('Ctrl Pts',(-6.95166755500006,11.6,-9.01190517100002));
#285512=CARTESIAN_POINT('Ctrl Pts',(-6.95248537400006,15.2,-9.01548158100002));
#285513=CARTESIAN_POINT('Ctrl Pts',(-6.95248537400006,11.6,-9.01548158100002));
#285514=CARTESIAN_POINT('Ctrl Pts',(-6.95330145500006,15.2,-9.01906305900001));
#285515=CARTESIAN_POINT('Ctrl Pts',(-6.95330145500006,11.6,-9.01906305900001));
#285516=CARTESIAN_POINT('Ctrl Pts',(-6.95411578700006,15.2,-9.02264959600002));
#285517=CARTESIAN_POINT('Ctrl Pts',(-6.95411578700006,11.6,-9.02264959600002));
#285518=CARTESIAN_POINT('Ctrl Pts',(-6.95492836400006,15.2,-9.02624119000001));
#285519=CARTESIAN_POINT('Ctrl Pts',(-6.95492836400006,11.6,-9.02624119000001));
#285520=CARTESIAN_POINT('Ctrl Pts',(-6.95573917800006,15.2,-9.02983783100002));
#285521=CARTESIAN_POINT('Ctrl Pts',(-6.95573917800006,11.6,-9.02983783100002));
#285522=CARTESIAN_POINT('Ctrl Pts',(-6.95654822400006,15.2,-9.03343951600002));
#285523=CARTESIAN_POINT('Ctrl Pts',(-6.95654822400006,11.6,-9.03343951600002));
#285524=CARTESIAN_POINT('Ctrl Pts',(-6.95735549400006,15.2,-9.03704623800002));
#285525=CARTESIAN_POINT('Ctrl Pts',(-6.95735549400006,11.6,-9.03704623800002));
#285526=CARTESIAN_POINT('Ctrl Pts',(-6.95816097900006,15.2,-9.04065799200002));
#285527=CARTESIAN_POINT('Ctrl Pts',(-6.95816097900006,11.6,-9.04065799200002));
#285528=CARTESIAN_POINT('Ctrl Pts',(-6.95896467400006,15.2,-9.04427477200001));
#285529=CARTESIAN_POINT('Ctrl Pts',(-6.95896467400006,11.6,-9.04427477200001));
#285530=CARTESIAN_POINT('Ctrl Pts',(-6.95976657100006,15.2,-9.04789657100002));
#285531=CARTESIAN_POINT('Ctrl Pts',(-6.95976657100006,11.6,-9.04789657100002));
#285532=CARTESIAN_POINT('Ctrl Pts',(-6.96056666300006,15.2,-9.05152338500002));
#285533=CARTESIAN_POINT('Ctrl Pts',(-6.96056666300006,11.6,-9.05152338500002));
#285534=CARTESIAN_POINT('Ctrl Pts',(-6.96136494300006,15.2,-9.05515520900002));
#285535=CARTESIAN_POINT('Ctrl Pts',(-6.96136494300006,11.6,-9.05515520900002));
#285536=CARTESIAN_POINT('Ctrl Pts',(-6.96216140500006,15.2,-9.05879203500002));
#285537=CARTESIAN_POINT('Ctrl Pts',(-6.96216140500006,11.6,-9.05879203500002));
#285538=CARTESIAN_POINT('Ctrl Pts',(-6.96295604000006,15.2,-9.06243385600002));
#285539=CARTESIAN_POINT('Ctrl Pts',(-6.96295604000006,11.6,-9.06243385600002));
#285540=CARTESIAN_POINT('Ctrl Pts',(-6.96374884000006,15.2,-9.06608066900001));
#285541=CARTESIAN_POINT('Ctrl Pts',(-6.96374884000006,11.6,-9.06608066900001));
#285542=CARTESIAN_POINT('Ctrl Pts',(-6.96453980000006,15.2,-9.06973246600002));
#285543=CARTESIAN_POINT('Ctrl Pts',(-6.96453980000006,11.6,-9.06973246600002));
#285544=CARTESIAN_POINT('Ctrl Pts',(-6.96532891100006,15.2,-9.07338924200002));
#285545=CARTESIAN_POINT('Ctrl Pts',(-6.96532891100006,11.6,-9.07338924200002));
#285546=CARTESIAN_POINT('Ctrl Pts',(-6.96611616800006,15.2,-9.07705099100001));
#285547=CARTESIAN_POINT('Ctrl Pts',(-6.96611616800006,11.6,-9.07705099100001));
#285548=CARTESIAN_POINT('Ctrl Pts',(-6.96690156100006,15.2,-9.08071770700002));
#285549=CARTESIAN_POINT('Ctrl Pts',(-6.96690156100006,11.6,-9.08071770700002));
#285550=CARTESIAN_POINT('Ctrl Pts',(-6.96768508700006,15.2,-9.08438938500002));
#285551=CARTESIAN_POINT('Ctrl Pts',(-6.96768508700006,11.6,-9.08438938500002));
#285552=CARTESIAN_POINT('Ctrl Pts',(-6.96846673800006,15.2,-9.08806602100002));
#285553=CARTESIAN_POINT('Ctrl Pts',(-6.96846673800006,11.6,-9.08806602100002));
#285554=CARTESIAN_POINT('Ctrl Pts',(-6.96924650800006,15.2,-9.09174760800001));
#285555=CARTESIAN_POINT('Ctrl Pts',(-6.96924650800006,11.6,-9.09174760800001));
#285556=CARTESIAN_POINT('Ctrl Pts',(-6.97002439000006,15.2,-9.09543414100002));
#285557=CARTESIAN_POINT('Ctrl Pts',(-6.97002439000006,11.6,-9.09543414100002));
#285558=CARTESIAN_POINT('Ctrl Pts',(-6.97080037900006,15.2,-9.09912561500001));
#285559=CARTESIAN_POINT('Ctrl Pts',(-6.97080037900006,11.6,-9.09912561500001));
#285560=CARTESIAN_POINT('Ctrl Pts',(-6.97157446400006,15.2,-9.10282202200002));
#285561=CARTESIAN_POINT('Ctrl Pts',(-6.97157446400006,11.6,-9.10282202200002));
#285562=CARTESIAN_POINT('Ctrl Pts',(-6.97234663900006,15.2,-9.10652335600002));
#285563=CARTESIAN_POINT('Ctrl Pts',(-6.97234663900006,11.6,-9.10652335600002));
#285564=CARTESIAN_POINT('Ctrl Pts',(-6.97311689200006,15.2,-9.11022960800001));
#285565=CARTESIAN_POINT('Ctrl Pts',(-6.97311689200006,11.6,-9.11022960800001));
#285566=CARTESIAN_POINT('Ctrl Pts',(-6.97388521800006,15.2,-9.11394077400002));
#285567=CARTESIAN_POINT('Ctrl Pts',(-6.97388521800006,11.6,-9.11394077400002));
#285568=CARTESIAN_POINT('Ctrl Pts',(-6.97465160800006,15.2,-9.11765684500002));
#285569=CARTESIAN_POINT('Ctrl Pts',(-6.97465160800006,11.6,-9.11765684500002));
#285570=CARTESIAN_POINT('Ctrl Pts',(-6.97541605700006,15.2,-9.12137781700002));
#285571=CARTESIAN_POINT('Ctrl Pts',(-6.97541605700006,11.6,-9.12137781700002));
#285572=CARTESIAN_POINT('Ctrl Pts',(-6.97617855900006,15.2,-9.12510368500002));
#285573=CARTESIAN_POINT('Ctrl Pts',(-6.97617855900006,11.6,-9.12510368500002));
#285574=CARTESIAN_POINT('Ctrl Pts',(-6.97693911100006,15.2,-9.12883444900002));
#285575=CARTESIAN_POINT('Ctrl Pts',(-6.97693911100006,11.6,-9.12883444900002));
#285576=CARTESIAN_POINT('Ctrl Pts',(-6.97769771300006,15.2,-9.13257010500002));
#285577=CARTESIAN_POINT('Ctrl Pts',(-6.97769771300006,11.6,-9.13257010500002));
#285578=CARTESIAN_POINT('Ctrl Pts',(-6.97830303200006,15.2,-9.13556254300002));
#285579=CARTESIAN_POINT('Ctrl Pts',(-6.97830303200006,11.6,-9.13556254300002));
#285580=CARTESIAN_POINT('Ctrl Pts',(-6.97875614300006,15.2,-9.13780907300002));
#285581=CARTESIAN_POINT('Ctrl Pts',(-6.97875614300006,11.6,-9.13780907300002));
#285582=CARTESIAN_POINT('Ctrl Pts',(-6.97905782800006,15.2,-9.13930773800002));
#285583=CARTESIAN_POINT('Ctrl Pts',(-6.97905782800006,11.6,-9.13930773800002));
#285584=CARTESIAN_POINT('Ctrl Pts',(-6.97920857100006,15.2,-9.14005731500002));
#285585=CARTESIAN_POINT('Ctrl Pts',(-6.97920857100006,11.6,-9.14005731500002));
#285586=CARTESIAN_POINT('Ctrl Pts',(-6.57080831900006,15.2,-8.02901631800001));
#285587=CARTESIAN_POINT('Ctrl Pts',(-6.57090674100006,15.2,-8.02916024100002));
#285588=CARTESIAN_POINT('Ctrl Pts',(-6.57110695100006,15.2,-8.02945316300002));
#285589=CARTESIAN_POINT('Ctrl Pts',(-6.57141009900006,15.2,-8.02989715700001));
#285590=CARTESIAN_POINT('Ctrl Pts',(-6.57181802000006,15.2,-8.03049556400002));
#285591=CARTESIAN_POINT('Ctrl Pts',(-6.57233322400006,15.2,-8.03125297300002));
#285592=CARTESIAN_POINT('Ctrl Pts',(-6.57285600600006,15.2,-8.03202318500002));
#285593=CARTESIAN_POINT('Ctrl Pts',(-6.57338335000006,15.2,-8.03280179700002));
#285594=CARTESIAN_POINT('Ctrl Pts',(-6.57391522700006,15.2,-8.03358880000001));
#285595=CARTESIAN_POINT('Ctrl Pts',(-6.57445160600005,15.2,-8.03438417800002));
#285596=CARTESIAN_POINT('Ctrl Pts',(-6.57499245700006,15.2,-8.03518792300002));
#285597=CARTESIAN_POINT('Ctrl Pts',(-6.57553775200006,15.2,-8.03600002100002));
#285598=CARTESIAN_POINT('Ctrl Pts',(-6.57608746000006,15.2,-8.03682046000001));
#285599=CARTESIAN_POINT('Ctrl Pts',(-6.57664155100006,15.2,-8.03764922800001));
#285600=CARTESIAN_POINT('Ctrl Pts',(-6.57719999700006,15.2,-8.03848631500001));
#285601=CARTESIAN_POINT('Ctrl Pts',(-6.57776276900006,15.2,-8.03933170500001));
#285602=CARTESIAN_POINT('Ctrl Pts',(-6.57832983700006,15.2,-8.04018539000002));
#285603=CARTESIAN_POINT('Ctrl Pts',(-6.57890117200005,15.2,-8.04104735800001));
#285604=CARTESIAN_POINT('Ctrl Pts',(-6.57947674700006,15.2,-8.04191759500002));
#285605=CARTESIAN_POINT('Ctrl Pts',(-6.58005653200005,15.2,-8.04279609000002));
#285606=CARTESIAN_POINT('Ctrl Pts',(-6.58064050000006,15.2,-8.04368283300001));
#285607=CARTESIAN_POINT('Ctrl Pts',(-6.58122862000006,15.2,-8.04457781100002));
#285608=CARTESIAN_POINT('Ctrl Pts',(-6.58182086700006,15.2,-8.04548101200002));
#285609=CARTESIAN_POINT('Ctrl Pts',(-6.58241721200006,15.2,-8.04639242700001));
#285610=CARTESIAN_POINT('Ctrl Pts',(-6.58301762700006,15.2,-8.04731204200002));
#285611=CARTESIAN_POINT('Ctrl Pts',(-6.58362208300006,15.2,-8.04823984600001));
#285612=CARTESIAN_POINT('Ctrl Pts',(-6.58423055400006,15.2,-8.04917582900002));
#285613=CARTESIAN_POINT('Ctrl Pts',(-6.58484301300006,15.2,-8.05011997800002));
#285614=CARTESIAN_POINT('Ctrl Pts',(-6.58545943100005,15.2,-8.05107228200002));
#285615=CARTESIAN_POINT('Ctrl Pts',(-6.58607978300005,15.2,-8.05203273100001));
#285616=CARTESIAN_POINT('Ctrl Pts',(-6.58670404000006,15.2,-8.05300131300001));
#285617=CARTESIAN_POINT('Ctrl Pts',(-6.58733217600005,15.2,-8.05397801700002));
#285618=CARTESIAN_POINT('Ctrl Pts',(-6.58796416400006,15.2,-8.05496283100002));
#285619=CARTESIAN_POINT('Ctrl Pts',(-6.58859997800006,15.2,-8.05595574500002));
#285620=CARTESIAN_POINT('Ctrl Pts',(-6.58923959000006,15.2,-8.05695674700001));
#285621=CARTESIAN_POINT('Ctrl Pts',(-6.58988297600006,15.2,-8.05796582700001));
#285622=CARTESIAN_POINT('Ctrl Pts',(-6.59053010700006,15.2,-8.05898297300002));
#285623=CARTESIAN_POINT('Ctrl Pts',(-6.59118095900006,15.2,-8.06000817400001));
#285624=CARTESIAN_POINT('Ctrl Pts',(-6.59183550500006,15.2,-8.06104142000001));
#285625=CARTESIAN_POINT('Ctrl Pts',(-6.59249371900006,15.2,-8.06208270100001));
#285626=CARTESIAN_POINT('Ctrl Pts',(-6.59315557600006,15.2,-8.06313200300002));
#285627=CARTESIAN_POINT('Ctrl Pts',(-6.59382104900006,15.2,-8.06418931800001));
#285628=CARTESIAN_POINT('Ctrl Pts',(-6.59449011500006,15.2,-8.06525463500002));
#285629=CARTESIAN_POINT('Ctrl Pts',(-6.59516274600006,15.2,-8.06632794100001));
#285630=CARTESIAN_POINT('Ctrl Pts',(-6.59583891700006,15.2,-8.06740922800002));
#285631=CARTESIAN_POINT('Ctrl Pts',(-6.59651860500006,15.2,-8.06849848300002));
#285632=CARTESIAN_POINT('Ctrl Pts',(-6.59720178300006,15.2,-8.06959569800001));
#285633=CARTESIAN_POINT('Ctrl Pts',(-6.59788842600006,15.2,-8.07070086000002));
#285634=CARTESIAN_POINT('Ctrl Pts',(-6.59857851000006,15.2,-8.07181396000002));
#285635=CARTESIAN_POINT('Ctrl Pts',(-6.59927200900006,15.2,-8.07293498700002));
#285636=CARTESIAN_POINT('Ctrl Pts',(-6.59996890100006,15.2,-8.07406392900001));
#285637=CARTESIAN_POINT('Ctrl Pts',(-6.60066916000006,15.2,-8.07520077800002));
#285638=CARTESIAN_POINT('Ctrl Pts',(-6.60137276000006,15.2,-8.07634552200001));
#285639=CARTESIAN_POINT('Ctrl Pts',(-6.60207968000006,15.2,-8.07749815200001));
#285640=CARTESIAN_POINT('Ctrl Pts',(-6.60278989300005,15.2,-8.07865865600002));
#285641=CARTESIAN_POINT('Ctrl Pts',(-6.60350337600006,15.2,-8.07982702500002));
#285642=CARTESIAN_POINT('Ctrl Pts',(-6.60422010600006,15.2,-8.08100324800002));
#285643=CARTESIAN_POINT('Ctrl Pts',(-6.60494005800006,15.2,-8.08218731500002));
#285644=CARTESIAN_POINT('Ctrl Pts',(-6.60566320900006,15.2,-8.08337921500001));
#285645=CARTESIAN_POINT('Ctrl Pts',(-6.60638953400006,15.2,-8.08457893900002));
#285646=CARTESIAN_POINT('Ctrl Pts',(-6.60711901100006,15.2,-8.08578647500001));
#285647=CARTESIAN_POINT('Ctrl Pts',(-6.60785161500006,15.2,-8.08700181500001));
#285648=CARTESIAN_POINT('Ctrl Pts',(-6.60858732500006,15.2,-8.08822494800001));
#285649=CARTESIAN_POINT('Ctrl Pts',(-6.60932611700006,15.2,-8.08945586400002));
#285650=CARTESIAN_POINT('Ctrl Pts',(-6.61006796600006,15.2,-8.09069455200002));
#285651=CARTESIAN_POINT('Ctrl Pts',(-6.61081285100006,15.2,-8.09194100300001));
#285652=CARTESIAN_POINT('Ctrl Pts',(-6.61156074900005,15.2,-8.09319520700001));
#285653=CARTESIAN_POINT('Ctrl Pts',(-6.61231163600006,15.2,-8.09445715400001));
#285654=CARTESIAN_POINT('Ctrl Pts',(-6.61306549000006,15.2,-8.09572683400001));
#285655=CARTESIAN_POINT('Ctrl Pts',(-6.61382229000006,15.2,-8.09700423600002));
#285656=CARTESIAN_POINT('Ctrl Pts',(-6.61458201100006,15.2,-8.09828935200001));
#285657=CARTESIAN_POINT('Ctrl Pts',(-6.61534463100006,15.2,-8.09958217100002));
#285658=CARTESIAN_POINT('Ctrl Pts',(-6.61611012900006,15.2,-8.10088268300002));
#285659=CARTESIAN_POINT('Ctrl Pts',(-6.61687848200006,15.2,-8.10219087900002));
#285660=CARTESIAN_POINT('Ctrl Pts',(-6.61764966700006,15.2,-8.10350674900001));
#285661=CARTESIAN_POINT('Ctrl Pts',(-6.61842366400006,15.2,-8.10483028300002));
#285662=CARTESIAN_POINT('Ctrl Pts',(-6.61920045000006,15.2,-8.10616147100001));
#285663=CARTESIAN_POINT('Ctrl Pts',(-6.61998000200006,15.2,-8.10750030400002));
#285664=CARTESIAN_POINT('Ctrl Pts',(-6.62076230000006,15.2,-8.10884677100002));
#285665=CARTESIAN_POINT('Ctrl Pts',(-6.62154732100006,15.2,-8.11020086400001));
#285666=CARTESIAN_POINT('Ctrl Pts',(-6.62233504600006,15.2,-8.11156257400001));
#285667=CARTESIAN_POINT('Ctrl Pts',(-6.62312545000006,15.2,-8.11293188900001));
#285668=CARTESIAN_POINT('Ctrl Pts',(-6.62391851400006,15.2,-8.11430880100002));
#285669=CARTESIAN_POINT('Ctrl Pts',(-6.62471421500006,15.2,-8.11569329900001));
#285670=CARTESIAN_POINT('Ctrl Pts',(-6.62551253400006,15.2,-8.11708537600002));
#285671=CARTESIAN_POINT('Ctrl Pts',(-6.62631344800006,15.2,-8.11848502000002));
#285672=CARTESIAN_POINT('Ctrl Pts',(-6.62711693700006,15.2,-8.11989222400002));
#285673=CARTESIAN_POINT('Ctrl Pts',(-6.62792298000006,15.2,-8.12130697600002));
#285674=CARTESIAN_POINT('Ctrl Pts',(-6.62873155500006,15.2,-8.12272926700001));
#285675=CARTESIAN_POINT('Ctrl Pts',(-6.62954264200006,15.2,-8.12415909000002));
#285676=CARTESIAN_POINT('Ctrl Pts',(-6.63035622100006,15.2,-8.12559643400002));
#285677=CARTESIAN_POINT('Ctrl Pts',(-6.63117227000006,15.2,-8.12704128900002));
#285678=CARTESIAN_POINT('Ctrl Pts',(-6.63199077100006,15.2,-8.12849364600002));
#285679=CARTESIAN_POINT('Ctrl Pts',(-6.63281170000006,15.2,-8.12995349700002));
#285680=CARTESIAN_POINT('Ctrl Pts',(-6.63363504000006,15.2,-8.13142083100002));
#285681=CARTESIAN_POINT('Ctrl Pts',(-6.63446076800006,15.2,-8.13289564100002));
#285682=CARTESIAN_POINT('Ctrl Pts',(-6.63528886600006,15.2,-8.13437791500002));
#285683=CARTESIAN_POINT('Ctrl Pts',(-6.63611931200006,15.2,-8.13586764600002));
#285684=CARTESIAN_POINT('Ctrl Pts',(-6.63695208700006,15.2,-8.13736482400002));
#285685=CARTESIAN_POINT('Ctrl Pts',(-6.63778717100006,15.2,-8.13886943900001));
#285686=CARTESIAN_POINT('Ctrl Pts',(-6.63862454400006,15.2,-8.14038148300002));
#285687=CARTESIAN_POINT('Ctrl Pts',(-6.63946418700006,15.2,-8.14190094700002));
#285688=CARTESIAN_POINT('Ctrl Pts',(-6.64030607900005,15.2,-8.14342782100002));
#285689=CARTESIAN_POINT('Ctrl Pts',(-6.64115020100006,15.2,-8.14496209700001));
#285690=CARTESIAN_POINT('Ctrl Pts',(-6.64199653400006,15.2,-8.14650376600002));
#285691=CARTESIAN_POINT('Ctrl Pts',(-6.64284505800006,15.2,-8.14805281700002));
#285692=CARTESIAN_POINT('Ctrl Pts',(-6.64369575300006,15.2,-8.14960924300001));
#285693=CARTESIAN_POINT('Ctrl Pts',(-6.64454859900006,15.2,-8.15117303500001));
#285694=CARTESIAN_POINT('Ctrl Pts',(-6.64540358000006,15.2,-8.15274418300002));
#285695=CARTESIAN_POINT('Ctrl Pts',(-6.64626067400006,15.2,-8.15432267900002));
#285696=CARTESIAN_POINT('Ctrl Pts',(-6.64711986400006,15.2,-8.15590851400002));
#285697=CARTESIAN_POINT('Ctrl Pts',(-6.64798112800006,15.2,-8.15750167800001));
#285698=CARTESIAN_POINT('Ctrl Pts',(-6.64884444900006,15.2,-8.15910216300002));
#285699=CARTESIAN_POINT('Ctrl Pts',(-6.64970980800006,15.2,-8.16070996000001));
#285700=CARTESIAN_POINT('Ctrl Pts',(-6.65057718600006,15.2,-8.16232506100001));
#285701=CARTESIAN_POINT('Ctrl Pts',(-6.65144656600006,15.2,-8.16394745500002));
#285702=CARTESIAN_POINT('Ctrl Pts',(-6.65231792600006,15.2,-8.16557713600002));
#285703=CARTESIAN_POINT('Ctrl Pts',(-6.65319124900006,15.2,-8.16721409300002));
#285704=CARTESIAN_POINT('Ctrl Pts',(-6.65406651700006,15.2,-8.16885831900001));
#285705=CARTESIAN_POINT('Ctrl Pts',(-6.65494371100006,15.2,-8.17050980400002));
#285706=CARTESIAN_POINT('Ctrl Pts',(-6.65582281300006,15.2,-8.17216853900002));
#285707=CARTESIAN_POINT('Ctrl Pts',(-6.65670380500006,15.2,-8.17383451600002));
#285708=CARTESIAN_POINT('Ctrl Pts',(-6.65758666800006,15.2,-8.17550772700002));
#285709=CARTESIAN_POINT('Ctrl Pts',(-6.65847138400006,15.2,-8.17718816300001));
#285710=CARTESIAN_POINT('Ctrl Pts',(-6.65935793500006,15.2,-8.17887581400001));
#285711=CARTESIAN_POINT('Ctrl Pts',(-6.66024630300006,15.2,-8.18057067400002));
#285712=CARTESIAN_POINT('Ctrl Pts',(-6.66113647000006,15.2,-8.18227273100002));
#285713=CARTESIAN_POINT('Ctrl Pts',(-6.66202841900006,15.2,-8.18398198000001));
#285714=CARTESIAN_POINT('Ctrl Pts',(-6.66292212900006,15.2,-8.18569840900001));
#285715=CARTESIAN_POINT('Ctrl Pts',(-6.66381758700005,15.2,-8.18742201300001));
#285716=CARTESIAN_POINT('Ctrl Pts',(-6.66471477200006,15.2,-8.18915278000001));
#285717=CARTESIAN_POINT('Ctrl Pts',(-6.66561366700006,15.2,-8.19089070400001));
#285718=CARTESIAN_POINT('Ctrl Pts',(-6.66651425400006,15.2,-8.19263577600001));
#285719=CARTESIAN_POINT('Ctrl Pts',(-6.66741651800006,15.2,-8.19438798600002));
#285720=CARTESIAN_POINT('Ctrl Pts',(-6.66832043800006,15.2,-8.19614732700002));
#285721=CARTESIAN_POINT('Ctrl Pts',(-6.66922600000006,15.2,-8.19791379200002));
#285722=CARTESIAN_POINT('Ctrl Pts',(-6.67013318300006,15.2,-8.19968736900002));
#285723=CARTESIAN_POINT('Ctrl Pts',(-6.67104197300006,15.2,-8.20146805200002));
#285724=CARTESIAN_POINT('Ctrl Pts',(-6.67195235200006,15.2,-8.20325583300002));
#285725=CARTESIAN_POINT('Ctrl Pts',(-6.67286430200006,15.2,-8.20505070200002));
#285726=CARTESIAN_POINT('Ctrl Pts',(-6.67377780700006,15.2,-8.20685265200002));
#285727=CARTESIAN_POINT('Ctrl Pts',(-6.67469285000006,15.2,-8.20866167300002));
#285728=CARTESIAN_POINT('Ctrl Pts',(-6.67560941300006,15.2,-8.21047775800002));
#285729=CARTESIAN_POINT('Ctrl Pts',(-6.67652747900005,15.2,-8.21230089900002));
#285730=CARTESIAN_POINT('Ctrl Pts',(-6.67744703200006,15.2,-8.21413108800002));
#285731=CARTESIAN_POINT('Ctrl Pts',(-6.67836805600006,15.2,-8.21596831500001));
#285732=CARTESIAN_POINT('Ctrl Pts',(-6.67929053300006,15.2,-8.21781257300002));
#285733=CARTESIAN_POINT('Ctrl Pts',(-6.68021444700006,15.2,-8.21966385300002));
#285734=CARTESIAN_POINT('Ctrl Pts',(-6.68113978100005,15.2,-8.22152214800001));
#285735=CARTESIAN_POINT('Ctrl Pts',(-6.68206651900006,15.2,-8.22338745000001));
#285736=CARTESIAN_POINT('Ctrl Pts',(-6.68299464500006,15.2,-8.22525974700002));
#285737=CARTESIAN_POINT('Ctrl Pts',(-6.68392414200006,15.2,-8.22713903600001));
#285738=CARTESIAN_POINT('Ctrl Pts',(-6.68485499200006,15.2,-8.22902530700001));
#285739=CARTESIAN_POINT('Ctrl Pts',(-6.68578718200005,15.2,-8.23091855000002));
#285740=CARTESIAN_POINT('Ctrl Pts',(-6.68672069300006,15.2,-8.23281875900001));
#285741=CARTESIAN_POINT('Ctrl Pts',(-6.68765551100006,15.2,-8.23472592600002));
#285742=CARTESIAN_POINT('Ctrl Pts',(-6.68859161800006,15.2,-8.23664004100002));
#285743=CARTESIAN_POINT('Ctrl Pts',(-6.68952899900006,15.2,-8.23856109700002));
#285744=CARTESIAN_POINT('Ctrl Pts',(-6.69046763700006,15.2,-8.24048908700002));
#285745=CARTESIAN_POINT('Ctrl Pts',(-6.69140751900006,15.2,-8.24242400100001));
#285746=CARTESIAN_POINT('Ctrl Pts',(-6.69234862600006,15.2,-8.24436583300002));
#285747=CARTESIAN_POINT('Ctrl Pts',(-6.69329094300006,15.2,-8.24631457300002));
#285748=CARTESIAN_POINT('Ctrl Pts',(-6.69423445500006,15.2,-8.24827021500001));
#285749=CARTESIAN_POINT('Ctrl Pts',(-6.69517914500006,15.2,-8.25023274900002));
#285750=CARTESIAN_POINT('Ctrl Pts',(-6.69612499800006,15.2,-8.25220216900002));
#285751=CARTESIAN_POINT('Ctrl Pts',(-6.69707199900006,15.2,-8.25417846500001));
#285752=CARTESIAN_POINT('Ctrl Pts',(-6.69802013200006,15.2,-8.25616163100002));
#285753=CARTESIAN_POINT('Ctrl Pts',(-6.69896938100006,15.2,-8.25815165900002));
#285754=CARTESIAN_POINT('Ctrl Pts',(-6.69991973100006,15.2,-8.26014853800002));
#285755=CARTESIAN_POINT('Ctrl Pts',(-6.70087116700006,15.2,-8.26215226500001));
#285756=CARTESIAN_POINT('Ctrl Pts',(-6.70182367300006,15.2,-8.26416282800002));
#285757=CARTESIAN_POINT('Ctrl Pts',(-6.70277723400006,15.2,-8.26618022100002));
#285758=CARTESIAN_POINT('Ctrl Pts',(-6.70373183500006,15.2,-8.26820443600001));
#285759=CARTESIAN_POINT('Ctrl Pts',(-6.70468746000005,15.2,-8.27023546500002));
#285760=CARTESIAN_POINT('Ctrl Pts',(-6.70564409500006,15.2,-8.27227330000002));
#285761=CARTESIAN_POINT('Ctrl Pts',(-6.70660172400006,15.2,-8.27431793400002));
#285762=CARTESIAN_POINT('Ctrl Pts',(-6.70756033200006,15.2,-8.27636935700001));
#285763=CARTESIAN_POINT('Ctrl Pts',(-6.70851990500006,15.2,-8.27842756400001));
#285764=CARTESIAN_POINT('Ctrl Pts',(-6.70948042600005,15.2,-8.28049254600002));
#285765=CARTESIAN_POINT('Ctrl Pts',(-6.71044188300006,15.2,-8.28256429500002));
#285766=CARTESIAN_POINT('Ctrl Pts',(-6.71140426000005,15.2,-8.28464280400001));
#285767=CARTESIAN_POINT('Ctrl Pts',(-6.71236754100006,15.2,-8.28672806400002));
#285768=CARTESIAN_POINT('Ctrl Pts',(-6.71333171300006,15.2,-8.28882006800002));
#285769=CARTESIAN_POINT('Ctrl Pts',(-6.71429675900006,15.2,-8.29091880900001));
#285770=CARTESIAN_POINT('Ctrl Pts',(-6.71526266700006,15.2,-8.29302427800001));
#285771=CARTESIAN_POINT('Ctrl Pts',(-6.71622942200006,15.2,-8.29513646900002));
#285772=CARTESIAN_POINT('Ctrl Pts',(-6.71719700800006,15.2,-8.29725537200002));
#285773=CARTESIAN_POINT('Ctrl Pts',(-6.71816541100006,15.2,-8.29938098200002));
#285774=CARTESIAN_POINT('Ctrl Pts',(-6.71913461600006,15.2,-8.30151328900002));
#285775=CARTESIAN_POINT('Ctrl Pts',(-6.72010461200006,15.2,-8.30365228700002));
#285776=CARTESIAN_POINT('Ctrl Pts',(-6.72107538000006,15.2,-8.30579796800002));
#285777=CARTESIAN_POINT('Ctrl Pts',(-6.72204690900006,15.2,-8.30795032300001));
#285778=CARTESIAN_POINT('Ctrl Pts',(-6.72301918300006,15.2,-8.31010934800002));
#285779=CARTESIAN_POINT('Ctrl Pts',(-6.72399218800006,15.2,-8.31227503100001));
#285780=CARTESIAN_POINT('Ctrl Pts',(-6.72496591100006,15.2,-8.31444736700002));
#285781=CARTESIAN_POINT('Ctrl Pts',(-6.72594033700006,15.2,-8.31662634800002));
#285782=CARTESIAN_POINT('Ctrl Pts',(-6.72691545200006,15.2,-8.31881196600002));
#285783=CARTESIAN_POINT('Ctrl Pts',(-6.72789124200006,15.2,-8.32100421400002));
#285784=CARTESIAN_POINT('Ctrl Pts',(-6.72886769300006,15.2,-8.32320308500002));
#285785=CARTESIAN_POINT('Ctrl Pts',(-6.72984479100006,15.2,-8.32540857000001));
#285786=CARTESIAN_POINT('Ctrl Pts',(-6.73082252300006,15.2,-8.32762066300001));
#285787=CARTESIAN_POINT('Ctrl Pts',(-6.73180087300006,15.2,-8.32983935500001));
#285788=CARTESIAN_POINT('Ctrl Pts',(-6.73277982900006,15.2,-8.33206464000002));
#285789=CARTESIAN_POINT('Ctrl Pts',(-6.73375937800006,15.2,-8.33429650900002));
#285790=CARTESIAN_POINT('Ctrl Pts',(-6.73473950400005,15.2,-8.33653495700002));
#285791=CARTESIAN_POINT('Ctrl Pts',(-6.73572019500006,15.2,-8.33877997400002));
#285792=CARTESIAN_POINT('Ctrl Pts',(-6.73670143700006,15.2,-8.34103155300001));
#285793=CARTESIAN_POINT('Ctrl Pts',(-6.73768321600006,15.2,-8.34328968900002));
#285794=CARTESIAN_POINT('Ctrl Pts',(-6.73866551900006,15.2,-8.34555437100001));
#285795=CARTESIAN_POINT('Ctrl Pts',(-6.73964833200006,15.2,-8.34782559500002));
#285796=CARTESIAN_POINT('Ctrl Pts',(-6.74063164200006,15.2,-8.35010335100002));
#285797=CARTESIAN_POINT('Ctrl Pts',(-6.74161543500006,15.2,-8.35238763300002));
#285798=CARTESIAN_POINT('Ctrl Pts',(-6.74259969900006,15.2,-8.35467843300002));
#285799=CARTESIAN_POINT('Ctrl Pts',(-6.74358442000006,15.2,-8.35697574500001));
#285800=CARTESIAN_POINT('Ctrl Pts',(-6.74456958400006,15.2,-8.35927956000001));
#285801=CARTESIAN_POINT('Ctrl Pts',(-6.74555517700006,15.2,-8.36158987000001));
#285802=CARTESIAN_POINT('Ctrl Pts',(-6.74654118900006,15.2,-8.36390667000002));
#285803=CARTESIAN_POINT('Ctrl Pts',(-6.74752760400006,15.2,-8.36622995200001));
#285804=CARTESIAN_POINT('Ctrl Pts',(-6.74851441000006,15.2,-8.36855970800002));
#285805=CARTESIAN_POINT('Ctrl Pts',(-6.74950159300006,15.2,-8.37089593100002));
#285806=CARTESIAN_POINT('Ctrl Pts',(-6.75048914200006,15.2,-8.37323861500002));
#285807=CARTESIAN_POINT('Ctrl Pts',(-6.75147704200006,15.2,-8.37558775000002));
#285808=CARTESIAN_POINT('Ctrl Pts',(-6.75246528000006,15.2,-8.37794333100002));
#285809=CARTESIAN_POINT('Ctrl Pts',(-6.75345384400006,15.2,-8.38030535000001));
#285810=CARTESIAN_POINT('Ctrl Pts',(-6.75444272200005,15.2,-8.38267380000002));
#285811=CARTESIAN_POINT('Ctrl Pts',(-6.75543189900006,15.2,-8.38504867300001));
#285812=CARTESIAN_POINT('Ctrl Pts',(-6.75642136400006,15.2,-8.38742996300001));
#285813=CARTESIAN_POINT('Ctrl Pts',(-6.75741110400006,15.2,-8.38981766200002));
#285814=CARTESIAN_POINT('Ctrl Pts',(-6.75840110500006,15.2,-8.39221176300001));
#285815=CARTESIAN_POINT('Ctrl Pts',(-6.75939135700006,15.2,-8.39461225900001));
#285816=CARTESIAN_POINT('Ctrl Pts',(-6.76038184400006,15.2,-8.39701914200001));
#285817=CARTESIAN_POINT('Ctrl Pts',(-6.76137255500006,15.2,-8.39943240700002));
#285818=CARTESIAN_POINT('Ctrl Pts',(-6.76236347800006,15.2,-8.40185204500001));
#285819=CARTESIAN_POINT('Ctrl Pts',(-6.76335460000006,15.2,-8.40427804800001));
#285820=CARTESIAN_POINT('Ctrl Pts',(-6.76434590800006,15.2,-8.40671041100002));
#285821=CARTESIAN_POINT('Ctrl Pts',(-6.76533739000006,15.2,-8.40914912700002));
#285822=CARTESIAN_POINT('Ctrl Pts',(-6.76632903400006,15.2,-8.41159418600002));
#285823=CARTESIAN_POINT('Ctrl Pts',(-6.76732082700005,15.2,-8.41404558300002));
#285824=CARTESIAN_POINT('Ctrl Pts',(-6.76831275600006,15.2,-8.41650331100002));
#285825=CARTESIAN_POINT('Ctrl Pts',(-6.76930481100006,15.2,-8.41896736400002));
#285826=CARTESIAN_POINT('Ctrl Pts',(-6.77029697800006,15.2,-8.42143773200002));
#285827=CARTESIAN_POINT('Ctrl Pts',(-6.77128924400006,15.2,-8.42391441000002));
#285828=CARTESIAN_POINT('Ctrl Pts',(-6.77228160000006,15.2,-8.42639739000001));
#285829=CARTESIAN_POINT('Ctrl Pts',(-6.77327403000006,15.2,-8.42888666600001));
#285830=CARTESIAN_POINT('Ctrl Pts',(-6.77426652500006,15.2,-8.43138223000001));
#285831=CARTESIAN_POINT('Ctrl Pts',(-6.77525907000006,15.2,-8.43388407500001));
#285832=CARTESIAN_POINT('Ctrl Pts',(-6.77625165600006,15.2,-8.43639219400002));
#285833=CARTESIAN_POINT('Ctrl Pts',(-6.77724426900006,15.2,-8.43890658100002));
#285834=CARTESIAN_POINT('Ctrl Pts',(-6.77823689800006,15.2,-8.44142722800001));
#285835=CARTESIAN_POINT('Ctrl Pts',(-6.77922953100006,15.2,-8.44395412900001));
#285836=CARTESIAN_POINT('Ctrl Pts',(-6.78022215500006,15.2,-8.44648727600001));
#285837=CARTESIAN_POINT('Ctrl Pts',(-6.78121475800006,15.2,-8.44902666100002));
#285838=CARTESIAN_POINT('Ctrl Pts',(-6.78220733100006,15.2,-8.45157227900001));
#285839=CARTESIAN_POINT('Ctrl Pts',(-6.78319986000006,15.2,-8.45412412300002));
#285840=CARTESIAN_POINT('Ctrl Pts',(-6.78419233200006,15.2,-8.45668218600002));
#285841=CARTESIAN_POINT('Ctrl Pts',(-6.78518473900006,15.2,-8.45924645900002));
#285842=CARTESIAN_POINT('Ctrl Pts',(-6.78617706600006,15.2,-8.46181693800002));
#285843=CARTESIAN_POINT('Ctrl Pts',(-6.78716930300006,15.2,-8.46439361500002));
#285844=CARTESIAN_POINT('Ctrl Pts',(-6.78816143700006,15.2,-8.46697648200001));
#285845=CARTESIAN_POINT('Ctrl Pts',(-6.78915345800006,15.2,-8.46956553300002));
#285846=CARTESIAN_POINT('Ctrl Pts',(-6.79014535300006,15.2,-8.47216076000001));
#285847=CARTESIAN_POINT('Ctrl Pts',(-6.79113711200006,15.2,-8.47476215800001));
#285848=CARTESIAN_POINT('Ctrl Pts',(-6.79212872200006,15.2,-8.47736971900002));
#285849=CARTESIAN_POINT('Ctrl Pts',(-6.79312017300005,15.2,-8.47998343700001));
#285850=CARTESIAN_POINT('Ctrl Pts',(-6.79411145300006,15.2,-8.48260330400001));
#285851=CARTESIAN_POINT('Ctrl Pts',(-6.79510255000006,15.2,-8.48522931400002));
#285852=CARTESIAN_POINT('Ctrl Pts',(-6.79609345300006,15.2,-8.48786145900002));
#285853=CARTESIAN_POINT('Ctrl Pts',(-6.79708415200006,15.2,-8.49049973300002));
#285854=CARTESIAN_POINT('Ctrl Pts',(-6.79807463300006,15.2,-8.49314413000002));
#285855=CARTESIAN_POINT('Ctrl Pts',(-6.79906488700006,15.2,-8.49579464200002));
#285856=CARTESIAN_POINT('Ctrl Pts',(-6.80005490300006,15.2,-8.49845126300002));
#285857=CARTESIAN_POINT('Ctrl Pts',(-6.80104466800006,15.2,-8.50111398400001));
#285858=CARTESIAN_POINT('Ctrl Pts',(-6.80203417100006,15.2,-8.50378280200001));
#285859=CARTESIAN_POINT('Ctrl Pts',(-6.80302340200006,15.2,-8.50645770700002));
#285860=CARTESIAN_POINT('Ctrl Pts',(-6.80401234900006,15.2,-8.50913869300001));
#285861=CARTESIAN_POINT('Ctrl Pts',(-6.80500100400006,15.2,-8.51182575500001));
#285862=CARTESIAN_POINT('Ctrl Pts',(-6.80598935100006,15.2,-8.51451888400002));
#285863=CARTESIAN_POINT('Ctrl Pts',(-6.80697738200006,15.2,-8.51721807500001));
#285864=CARTESIAN_POINT('Ctrl Pts',(-6.80796508500006,15.2,-8.51992331800002));
#285865=CARTESIAN_POINT('Ctrl Pts',(-6.80895244900006,15.2,-8.52263461100002));
#285866=CARTESIAN_POINT('Ctrl Pts',(-6.80993946500006,15.2,-8.52535194300001));
#285867=CARTESIAN_POINT('Ctrl Pts',(-6.81092612100006,15.2,-8.52807531000002));
#285868=CARTESIAN_POINT('Ctrl Pts',(-6.81191240500006,15.2,-8.53080470500002));
#285869=CARTESIAN_POINT('Ctrl Pts',(-6.81289830700006,15.2,-8.53354012000001));
#285870=CARTESIAN_POINT('Ctrl Pts',(-6.81388381700006,15.2,-8.53628154900001));
#285871=CARTESIAN_POINT('Ctrl Pts',(-6.81486892200006,15.2,-8.53902898500002));
#285872=CARTESIAN_POINT('Ctrl Pts',(-6.81585361400006,15.2,-8.54178242200001));
#285873=CARTESIAN_POINT('Ctrl Pts',(-6.81683788100006,15.2,-8.54454185300002));
#285874=CARTESIAN_POINT('Ctrl Pts',(-6.81782171200005,15.2,-8.54730727200002));
#285875=CARTESIAN_POINT('Ctrl Pts',(-6.81880509800005,15.2,-8.55007867000002));
#285876=CARTESIAN_POINT('Ctrl Pts',(-6.81978802600006,15.2,-8.55285604300001));
#285877=CARTESIAN_POINT('Ctrl Pts',(-6.82077048700005,15.2,-8.55563938300002));
#285878=CARTESIAN_POINT('Ctrl Pts',(-6.82175247000006,15.2,-8.55842868400002));
#285879=CARTESIAN_POINT('Ctrl Pts',(-6.82273396500006,15.2,-8.56122393900002));
#285880=CARTESIAN_POINT('Ctrl Pts',(-6.82371496100005,15.2,-8.56402514100001));
#285881=CARTESIAN_POINT('Ctrl Pts',(-6.82469544700006,15.2,-8.56683228400002));
#285882=CARTESIAN_POINT('Ctrl Pts',(-6.82567541400006,15.2,-8.56964536100002));
#285883=CARTESIAN_POINT('Ctrl Pts',(-6.82665485100006,15.2,-8.57246436600001));
#285884=CARTESIAN_POINT('Ctrl Pts',(-6.82763374600006,15.2,-8.57528929200001));
#285885=CARTESIAN_POINT('Ctrl Pts',(-6.82861209100006,15.2,-8.57812013100002));
#285886=CARTESIAN_POINT('Ctrl Pts',(-6.82958987600006,15.2,-8.58095688000001));
#285887=CARTESIAN_POINT('Ctrl Pts',(-6.83056708700006,15.2,-8.58379952900002));
#285888=CARTESIAN_POINT('Ctrl Pts',(-6.83154371800006,15.2,-8.58664807300002));
#285889=CARTESIAN_POINT('Ctrl Pts',(-6.83251975600006,15.2,-8.58950250500002));
#285890=CARTESIAN_POINT('Ctrl Pts',(-6.83349519400006,15.2,-8.59236281800002));
#285891=CARTESIAN_POINT('Ctrl Pts',(-6.83447001700006,15.2,-8.59522900700001));
#285892=CARTESIAN_POINT('Ctrl Pts',(-6.83544421900006,15.2,-8.59810106300002));
#285893=CARTESIAN_POINT('Ctrl Pts',(-6.83641778800006,15.2,-8.60097898100002));
#285894=CARTESIAN_POINT('Ctrl Pts',(-6.83739071400006,15.2,-8.60386275500002));
#285895=CARTESIAN_POINT('Ctrl Pts',(-6.83836298800006,15.2,-8.60675237800002));
#285896=CARTESIAN_POINT('Ctrl Pts',(-6.83933459800006,15.2,-8.60964784300002));
#285897=CARTESIAN_POINT('Ctrl Pts',(-6.84030553600006,15.2,-8.61254914500002));
#285898=CARTESIAN_POINT('Ctrl Pts',(-6.84127579200006,15.2,-8.61545627500002));
#285899=CARTESIAN_POINT('Ctrl Pts',(-6.84224535400006,15.2,-8.61836922800002));
#285900=CARTESIAN_POINT('Ctrl Pts',(-6.84321421300006,15.2,-8.62128799800002));
#285901=CARTESIAN_POINT('Ctrl Pts',(-6.84418236000006,15.2,-8.62421257800002));
#285902=CARTESIAN_POINT('Ctrl Pts',(-6.84514978400006,15.2,-8.62714296000001));
#285903=CARTESIAN_POINT('Ctrl Pts',(-6.84611647700006,15.2,-8.63007914000002));
#285904=CARTESIAN_POINT('Ctrl Pts',(-6.84708242700006,15.2,-8.63302111000002));
#285905=CARTESIAN_POINT('Ctrl Pts',(-6.84804762500006,15.2,-8.63596886400002));
#285906=CARTESIAN_POINT('Ctrl Pts',(-6.84901206200006,15.2,-8.63892239500002));
#285907=CARTESIAN_POINT('Ctrl Pts',(-6.84997572700006,15.2,-8.64188169800002));
#285908=CARTESIAN_POINT('Ctrl Pts',(-6.85093861100006,15.2,-8.64484676500001));
#285909=CARTESIAN_POINT('Ctrl Pts',(-6.85190070400005,15.2,-8.64781759100002));
#285910=CARTESIAN_POINT('Ctrl Pts',(-6.85286199700006,15.2,-8.65079416800001));
#285911=CARTESIAN_POINT('Ctrl Pts',(-6.85382248000006,15.2,-8.65377649100001));
#285912=CARTESIAN_POINT('Ctrl Pts',(-6.85478214300006,15.2,-8.65676455300001));
#285913=CARTESIAN_POINT('Ctrl Pts',(-6.85574097600006,15.2,-8.65975834700001));
#285914=CARTESIAN_POINT('Ctrl Pts',(-6.85669897100006,15.2,-8.66275786700001));
#285915=CARTESIAN_POINT('Ctrl Pts',(-6.85765611700006,15.2,-8.66576310700001));
#285916=CARTESIAN_POINT('Ctrl Pts',(-6.85861240500006,15.2,-8.66877406100001));
#285917=CARTESIAN_POINT('Ctrl Pts',(-6.85956782600006,15.2,-8.67179072200001));
#285918=CARTESIAN_POINT('Ctrl Pts',(-6.86052237000006,15.2,-8.67481308300002));
#285919=CARTESIAN_POINT('Ctrl Pts',(-6.86147602800006,15.2,-8.67784113800001));
#285920=CARTESIAN_POINT('Ctrl Pts',(-6.86242879000006,15.2,-8.68087488200001));
#285921=CARTESIAN_POINT('Ctrl Pts',(-6.86338064600006,15.2,-8.68391430700001));
#285922=CARTESIAN_POINT('Ctrl Pts',(-6.86433158900006,15.2,-8.68695940700002));
#285923=CARTESIAN_POINT('Ctrl Pts',(-6.86528160700006,15.2,-8.69001017600001));
#285924=CARTESIAN_POINT('Ctrl Pts',(-6.86623069200006,15.2,-8.69306660700002));
#285925=CARTESIAN_POINT('Ctrl Pts',(-6.86717883600005,15.2,-8.69612869500001));
#285926=CARTESIAN_POINT('Ctrl Pts',(-6.86812602700006,15.2,-8.69919643300002));
#285927=CARTESIAN_POINT('Ctrl Pts',(-6.86907225800006,15.2,-8.70226981300002));
#285928=CARTESIAN_POINT('Ctrl Pts',(-6.87001751800006,15.2,-8.70534883200002));
#285929=CARTESIAN_POINT('Ctrl Pts',(-6.87096179900006,15.2,-8.70843348100001));
#285930=CARTESIAN_POINT('Ctrl Pts',(-6.87190509000006,15.2,-8.71152375400002));
#285931=CARTESIAN_POINT('Ctrl Pts',(-6.87284738500006,15.2,-8.71461964600002));
#285932=CARTESIAN_POINT('Ctrl Pts',(-6.87378867400006,15.2,-8.71772115000002));
#285933=CARTESIAN_POINT('Ctrl Pts',(-6.87472894500006,15.2,-8.72082826000002));
#285934=CARTESIAN_POINT('Ctrl Pts',(-6.87566819300006,15.2,-8.72394096800001));
#285935=CARTESIAN_POINT('Ctrl Pts',(-6.87660640700006,15.2,-8.72705927100002));
#285936=CARTESIAN_POINT('Ctrl Pts',(-6.87754357700006,15.2,-8.73018316100002));
#285937=CARTESIAN_POINT('Ctrl Pts',(-6.87847969500006,15.2,-8.73331263000001));
#285938=CARTESIAN_POINT('Ctrl Pts',(-6.87941475200006,15.2,-8.73644767400001));
#285939=CARTESIAN_POINT('Ctrl Pts',(-6.88034873900006,15.2,-8.73958828600001));
#285940=CARTESIAN_POINT('Ctrl Pts',(-6.88128164800006,15.2,-8.74273446000002));
#285941=CARTESIAN_POINT('Ctrl Pts',(-6.88221346800006,15.2,-8.74588619000002));
#285942=CARTESIAN_POINT('Ctrl Pts',(-6.88314419200006,15.2,-8.74904347000001));
#285943=CARTESIAN_POINT('Ctrl Pts',(-6.88407381100006,15.2,-8.75220629200001));
#285944=CARTESIAN_POINT('Ctrl Pts',(-6.88500231400006,15.2,-8.75537465100001));
#285945=CARTESIAN_POINT('Ctrl Pts',(-6.88592969500006,15.2,-8.75854854100002));
#285946=CARTESIAN_POINT('Ctrl Pts',(-6.88685594400006,15.2,-8.76172795500001));
#285947=CARTESIAN_POINT('Ctrl Pts',(-6.88778105300006,15.2,-8.76491288800001));
#285948=CARTESIAN_POINT('Ctrl Pts',(-6.88870501100006,15.2,-8.76810333200002));
#285949=CARTESIAN_POINT('Ctrl Pts',(-6.88962781100006,15.2,-8.77129928300001));
#285950=CARTESIAN_POINT('Ctrl Pts',(-6.89054944500006,15.2,-8.77450073400002));
#285951=CARTESIAN_POINT('Ctrl Pts',(-6.89146990300006,15.2,-8.77770767800002));
#285952=CARTESIAN_POINT('Ctrl Pts',(-6.89238917600006,15.2,-8.78092010900002));
#285953=CARTESIAN_POINT('Ctrl Pts',(-6.89330725700006,15.2,-8.78413802100001));
#285954=CARTESIAN_POINT('Ctrl Pts',(-6.89422413500006,15.2,-8.78736140900001));
#285955=CARTESIAN_POINT('Ctrl Pts',(-6.89513980400006,15.2,-8.79059026500002));
#285956=CARTESIAN_POINT('Ctrl Pts',(-6.89605425400006,15.2,-8.79382458400002));
#285957=CARTESIAN_POINT('Ctrl Pts',(-6.89696747600006,15.2,-8.79706435900001));
#285958=CARTESIAN_POINT('Ctrl Pts',(-6.89787946300005,15.2,-8.80030958500001));
#285959=CARTESIAN_POINT('Ctrl Pts',(-6.89879020600006,15.2,-8.80356025400001));
#285960=CARTESIAN_POINT('Ctrl Pts',(-6.89969969600006,15.2,-8.80681636200002));
#285961=CARTESIAN_POINT('Ctrl Pts',(-6.90060792400006,15.2,-8.81007790200002));
#285962=CARTESIAN_POINT('Ctrl Pts',(-6.90151488200006,15.2,-8.81334486800002));
#285963=CARTESIAN_POINT('Ctrl Pts',(-6.90242056300006,15.2,-8.81661725300001));
#285964=CARTESIAN_POINT('Ctrl Pts',(-6.90332495800006,15.2,-8.81989505100002));
#285965=CARTESIAN_POINT('Ctrl Pts',(-6.90422805600006,15.2,-8.82317825800002));
#285966=CARTESIAN_POINT('Ctrl Pts',(-6.90512985200006,15.2,-8.82646686600001));
#285967=CARTESIAN_POINT('Ctrl Pts',(-6.90603033600006,15.2,-8.82976086800002));
#285968=CARTESIAN_POINT('Ctrl Pts',(-6.90692950100006,15.2,-8.83306026000002));
#285969=CARTESIAN_POINT('Ctrl Pts',(-6.90782733600006,15.2,-8.83636503500002));
#285970=CARTESIAN_POINT('Ctrl Pts',(-6.90872383500006,15.2,-8.83967518700001));
#285971=CARTESIAN_POINT('Ctrl Pts',(-6.90961899000006,15.2,-8.84299071000001));
#285972=CARTESIAN_POINT('Ctrl Pts',(-6.91051279100006,15.2,-8.84631159700002));
#285973=CARTESIAN_POINT('Ctrl Pts',(-6.91140523100006,15.2,-8.84963784300002));
#285974=CARTESIAN_POINT('Ctrl Pts',(-6.91229630100006,15.2,-8.85296944200002));
#285975=CARTESIAN_POINT('Ctrl Pts',(-6.91318599400006,15.2,-8.85630638800002));
#285976=CARTESIAN_POINT('Ctrl Pts',(-6.91407430200006,15.2,-8.85964867300002));
#285977=CARTESIAN_POINT('Ctrl Pts',(-6.91496121500006,15.2,-8.86299629400002));
#285978=CARTESIAN_POINT('Ctrl Pts',(-6.91584672600006,15.2,-8.86634924200001));
#285979=CARTESIAN_POINT('Ctrl Pts',(-6.91673082700006,15.2,-8.86970751300002));
#285980=CARTESIAN_POINT('Ctrl Pts',(-6.91761351000006,15.2,-8.87307110000001));
#285981=CARTESIAN_POINT('Ctrl Pts',(-6.91849476600006,15.2,-8.87643999800002));
#285982=CARTESIAN_POINT('Ctrl Pts',(-6.91937458800005,15.2,-8.87981420000001));
#285983=CARTESIAN_POINT('Ctrl Pts',(-6.92025296800006,15.2,-8.88319369900002));
#285984=CARTESIAN_POINT('Ctrl Pts',(-6.92112989800005,15.2,-8.88657849200002));
#285985=CARTESIAN_POINT('Ctrl Pts',(-6.92200536800006,15.2,-8.88996857000001));
#285986=CARTESIAN_POINT('Ctrl Pts',(-6.92287937300006,15.2,-8.89336392900002));
#285987=CARTESIAN_POINT('Ctrl Pts',(-6.92375190400006,15.2,-8.89676456100002));
#285988=CARTESIAN_POINT('Ctrl Pts',(-6.92462295300006,15.2,-8.90017046300001));
#285989=CARTESIAN_POINT('Ctrl Pts',(-6.92549251200006,15.2,-8.90358162500002));
#285990=CARTESIAN_POINT('Ctrl Pts',(-6.92636057200006,15.2,-8.90699804400001));
#285991=CARTESIAN_POINT('Ctrl Pts',(-6.92722712700006,15.2,-8.91041971300002));
#285992=CARTESIAN_POINT('Ctrl Pts',(-6.92809216800006,15.2,-8.91384662700002));
#285993=CARTESIAN_POINT('Ctrl Pts',(-6.92895568900005,15.2,-8.91727877800001));
#285994=CARTESIAN_POINT('Ctrl Pts',(-6.92981767900006,15.2,-8.92071616200001));
#285995=CARTESIAN_POINT('Ctrl Pts',(-6.93067813200006,15.2,-8.92415877200002));
#285996=CARTESIAN_POINT('Ctrl Pts',(-6.93153704100006,15.2,-8.92760660300001));
#285997=CARTESIAN_POINT('Ctrl Pts',(-6.93239439700006,15.2,-8.93105964700002));
#285998=CARTESIAN_POINT('Ctrl Pts',(-6.93325019300006,15.2,-8.93451789900002));
#285999=CARTESIAN_POINT('Ctrl Pts',(-6.93410442200006,15.2,-8.93798135500001));
#286000=CARTESIAN_POINT('Ctrl Pts',(-6.93495707400006,15.2,-8.94145000600002));
#286001=CARTESIAN_POINT('Ctrl Pts',(-6.93580814300006,15.2,-8.94492384900002));
#286002=CARTESIAN_POINT('Ctrl Pts',(-6.93665762200006,15.2,-8.94840287600001));
#286003=CARTESIAN_POINT('Ctrl Pts',(-6.93750550100006,15.2,-8.95188708100001));
#286004=CARTESIAN_POINT('Ctrl Pts',(-6.93835177400006,15.2,-8.95537645900001));
#286005=CARTESIAN_POINT('Ctrl Pts',(-6.93919643300006,15.2,-8.95887100400002));
#286006=CARTESIAN_POINT('Ctrl Pts',(-6.94003947100006,15.2,-8.96237071000002));
#286007=CARTESIAN_POINT('Ctrl Pts',(-6.94088088100006,15.2,-8.96587557000002));
#286008=CARTESIAN_POINT('Ctrl Pts',(-6.94172065300006,15.2,-8.96938558000001));
#286009=CARTESIAN_POINT('Ctrl Pts',(-6.94255878100006,15.2,-8.97290073300002));
#286010=CARTESIAN_POINT('Ctrl Pts',(-6.94339525800006,15.2,-8.97642102300001));
#286011=CARTESIAN_POINT('Ctrl Pts',(-6.94423007700006,15.2,-8.97994644400002));
#286012=CARTESIAN_POINT('Ctrl Pts',(-6.94506322800006,15.2,-8.98347699100002));
#286013=CARTESIAN_POINT('Ctrl Pts',(-6.94589470500006,15.2,-8.98701265600002));
#286014=CARTESIAN_POINT('Ctrl Pts',(-6.94672450200006,15.2,-8.99055343700002));
#286015=CARTESIAN_POINT('Ctrl Pts',(-6.94755260900005,15.2,-8.99409932400001));
#286016=CARTESIAN_POINT('Ctrl Pts',(-6.94837902000006,15.2,-8.99765031300002));
#286017=CARTESIAN_POINT('Ctrl Pts',(-6.94920372700006,15.2,-9.00120639800001));
#286018=CARTESIAN_POINT('Ctrl Pts',(-6.95002672400006,15.2,-9.00476757400002));
#286019=CARTESIAN_POINT('Ctrl Pts',(-6.95084800200005,15.2,-9.00833383300002));
#286020=CARTESIAN_POINT('Ctrl Pts',(-6.95166755500006,15.2,-9.01190517100002));
#286021=CARTESIAN_POINT('Ctrl Pts',(-6.95248537400006,15.2,-9.01548158100002));
#286022=CARTESIAN_POINT('Ctrl Pts',(-6.95330145500006,15.2,-9.01906305900001));
#286023=CARTESIAN_POINT('Ctrl Pts',(-6.95411578700006,15.2,-9.02264959600002));
#286024=CARTESIAN_POINT('Ctrl Pts',(-6.95492836400006,15.2,-9.02624119000001));
#286025=CARTESIAN_POINT('Ctrl Pts',(-6.95573917800006,15.2,-9.02983783100002));
#286026=CARTESIAN_POINT('Ctrl Pts',(-6.95654822400006,15.2,-9.03343951600002));
#286027=CARTESIAN_POINT('Ctrl Pts',(-6.95735549400006,15.2,-9.03704623800002));
#286028=CARTESIAN_POINT('Ctrl Pts',(-6.95816097900006,15.2,-9.04065799200002));
#286029=CARTESIAN_POINT('Ctrl Pts',(-6.95896467400006,15.2,-9.04427477200001));
#286030=CARTESIAN_POINT('Ctrl Pts',(-6.95976657100006,15.2,-9.04789657100002));
#286031=CARTESIAN_POINT('Ctrl Pts',(-6.96056666300006,15.2,-9.05152338500002));
#286032=CARTESIAN_POINT('Ctrl Pts',(-6.96136494300006,15.2,-9.05515520900002));
#286033=CARTESIAN_POINT('Ctrl Pts',(-6.96216140500006,15.2,-9.05879203500002));
#286034=CARTESIAN_POINT('Ctrl Pts',(-6.96295604000006,15.2,-9.06243385600002));
#286035=CARTESIAN_POINT('Ctrl Pts',(-6.96374884000006,15.2,-9.06608066900001));
#286036=CARTESIAN_POINT('Ctrl Pts',(-6.96453980000006,15.2,-9.06973246600002));
#286037=CARTESIAN_POINT('Ctrl Pts',(-6.96532891100006,15.2,-9.07338924200002));
#286038=CARTESIAN_POINT('Ctrl Pts',(-6.96611616800006,15.2,-9.07705099100001));
#286039=CARTESIAN_POINT('Ctrl Pts',(-6.96690156100006,15.2,-9.08071770700002));
#286040=CARTESIAN_POINT('Ctrl Pts',(-6.96768508700006,15.2,-9.08438938500002));
#286041=CARTESIAN_POINT('Ctrl Pts',(-6.96846673800006,15.2,-9.08806602100002));
#286042=CARTESIAN_POINT('Ctrl Pts',(-6.96924650800006,15.2,-9.09174760800001));
#286043=CARTESIAN_POINT('Ctrl Pts',(-6.97002439000006,15.2,-9.09543414100002));
#286044=CARTESIAN_POINT('Ctrl Pts',(-6.97080037900006,15.2,-9.09912561500001));
#286045=CARTESIAN_POINT('Ctrl Pts',(-6.97157446400006,15.2,-9.10282202200002));
#286046=CARTESIAN_POINT('Ctrl Pts',(-6.97234663900006,15.2,-9.10652335600002));
#286047=CARTESIAN_POINT('Ctrl Pts',(-6.97311689200006,15.2,-9.11022960800001));
#286048=CARTESIAN_POINT('Ctrl Pts',(-6.97388521800006,15.2,-9.11394077400002));
#286049=CARTESIAN_POINT('Ctrl Pts',(-6.97465160800006,15.2,-9.11765684500002));
#286050=CARTESIAN_POINT('Ctrl Pts',(-6.97541605700006,15.2,-9.12137781700002));
#286051=CARTESIAN_POINT('Ctrl Pts',(-6.97617855900006,15.2,-9.12510368500002));
#286052=CARTESIAN_POINT('Ctrl Pts',(-6.97693911100006,15.2,-9.12883444900002));
#286053=CARTESIAN_POINT('Ctrl Pts',(-6.97769771300006,15.2,-9.13257010500002));
#286054=CARTESIAN_POINT('Ctrl Pts',(-6.97830303200006,15.2,-9.13556254300002));
#286055=CARTESIAN_POINT('Ctrl Pts',(-6.97875614300006,15.2,-9.13780907300002));
#286056=CARTESIAN_POINT('Ctrl Pts',(-6.97905782800006,15.2,-9.13930773800002));
#286057=CARTESIAN_POINT('Ctrl Pts',(-6.97920857100006,15.2,-9.14005731500002));
#286058=CARTESIAN_POINT('Ctrl Pts',(-6.57080831900006,12.2,-8.02901631800001));
#286059=CARTESIAN_POINT('Ctrl Pts',(-6.57090674100006,12.2,-8.02916024100002));
#286060=CARTESIAN_POINT('Ctrl Pts',(-6.57110695100006,12.2,-8.02945316300002));
#286061=CARTESIAN_POINT('Ctrl Pts',(-6.57141009900006,12.2,-8.02989715700001));
#286062=CARTESIAN_POINT('Ctrl Pts',(-6.57181802000006,12.2,-8.03049556400002));
#286063=CARTESIAN_POINT('Ctrl Pts',(-6.57233322400006,12.2,-8.03125297300002));
#286064=CARTESIAN_POINT('Ctrl Pts',(-6.57285600600006,12.2,-8.03202318500002));
#286065=CARTESIAN_POINT('Ctrl Pts',(-6.57338335000006,12.2,-8.03280179700002));
#286066=CARTESIAN_POINT('Ctrl Pts',(-6.57391522700006,12.2,-8.03358880000001));
#286067=CARTESIAN_POINT('Ctrl Pts',(-6.57445160600005,12.2,-8.03438417800002));
#286068=CARTESIAN_POINT('Ctrl Pts',(-6.57499245700006,12.2,-8.03518792300002));
#286069=CARTESIAN_POINT('Ctrl Pts',(-6.57553775200006,12.2,-8.03600002100002));
#286070=CARTESIAN_POINT('Ctrl Pts',(-6.57608746000006,12.2,-8.03682046000001));
#286071=CARTESIAN_POINT('Ctrl Pts',(-6.57664155100006,12.2,-8.03764922800001));
#286072=CARTESIAN_POINT('Ctrl Pts',(-6.57719999700006,12.2,-8.03848631500001));
#286073=CARTESIAN_POINT('Ctrl Pts',(-6.57776276900006,12.2,-8.03933170500001));
#286074=CARTESIAN_POINT('Ctrl Pts',(-6.57832983700006,12.2,-8.04018539000002));
#286075=CARTESIAN_POINT('Ctrl Pts',(-6.57890117200005,12.2,-8.04104735800001));
#286076=CARTESIAN_POINT('Ctrl Pts',(-6.57947674700006,12.2,-8.04191759500002));
#286077=CARTESIAN_POINT('Ctrl Pts',(-6.58005653200005,12.2,-8.04279609000002));
#286078=CARTESIAN_POINT('Ctrl Pts',(-6.58064050000006,12.2,-8.04368283300001));
#286079=CARTESIAN_POINT('Ctrl Pts',(-6.58122862000006,12.2,-8.04457781100002));
#286080=CARTESIAN_POINT('Ctrl Pts',(-6.58182086700006,12.2,-8.04548101200002));
#286081=CARTESIAN_POINT('Ctrl Pts',(-6.58241721200006,12.2,-8.04639242700001));
#286082=CARTESIAN_POINT('Ctrl Pts',(-6.58301762700006,12.2,-8.04731204200002));
#286083=CARTESIAN_POINT('Ctrl Pts',(-6.58362208300006,12.2,-8.04823984600001));
#286084=CARTESIAN_POINT('Ctrl Pts',(-6.58423055400006,12.2,-8.04917582900002));
#286085=CARTESIAN_POINT('Ctrl Pts',(-6.58484301300006,12.2,-8.05011997800002));
#286086=CARTESIAN_POINT('Ctrl Pts',(-6.58545943100005,12.2,-8.05107228200002));
#286087=CARTESIAN_POINT('Ctrl Pts',(-6.58607978300005,12.2,-8.05203273100001));
#286088=CARTESIAN_POINT('Ctrl Pts',(-6.58670404000006,12.2,-8.05300131300001));
#286089=CARTESIAN_POINT('Ctrl Pts',(-6.58733217600005,12.2,-8.05397801700002));
#286090=CARTESIAN_POINT('Ctrl Pts',(-6.58796416400006,12.2,-8.05496283100002));
#286091=CARTESIAN_POINT('Ctrl Pts',(-6.58859997800006,12.2,-8.05595574500002));
#286092=CARTESIAN_POINT('Ctrl Pts',(-6.58923959000006,12.2,-8.05695674700001));
#286093=CARTESIAN_POINT('Ctrl Pts',(-6.58988297600006,12.2,-8.05796582700001));
#286094=CARTESIAN_POINT('Ctrl Pts',(-6.59053010700006,12.2,-8.05898297300002));
#286095=CARTESIAN_POINT('Ctrl Pts',(-6.59118095900006,12.2,-8.06000817400001));
#286096=CARTESIAN_POINT('Ctrl Pts',(-6.59183550500006,12.2,-8.06104142000001));
#286097=CARTESIAN_POINT('Ctrl Pts',(-6.59249371900006,12.2,-8.06208270100001));
#286098=CARTESIAN_POINT('Ctrl Pts',(-6.59315557600006,12.2,-8.06313200300002));
#286099=CARTESIAN_POINT('Ctrl Pts',(-6.59382104900006,12.2,-8.06418931800001));
#286100=CARTESIAN_POINT('Ctrl Pts',(-6.59449011500006,12.2,-8.06525463500002));
#286101=CARTESIAN_POINT('Ctrl Pts',(-6.59516274600006,12.2,-8.06632794100001));
#286102=CARTESIAN_POINT('Ctrl Pts',(-6.59583891700006,12.2,-8.06740922800002));
#286103=CARTESIAN_POINT('Ctrl Pts',(-6.59651860500006,12.2,-8.06849848300002));
#286104=CARTESIAN_POINT('Ctrl Pts',(-6.59720178300006,12.2,-8.06959569800001));
#286105=CARTESIAN_POINT('Ctrl Pts',(-6.59788842600006,12.2,-8.07070086000002));
#286106=CARTESIAN_POINT('Ctrl Pts',(-6.59857851000006,12.2,-8.07181396000002));
#286107=CARTESIAN_POINT('Ctrl Pts',(-6.59927200900006,12.2,-8.07293498700002));
#286108=CARTESIAN_POINT('Ctrl Pts',(-6.59996890100006,12.2,-8.07406392900001));
#286109=CARTESIAN_POINT('Ctrl Pts',(-6.60066916000006,12.2,-8.07520077800002));
#286110=CARTESIAN_POINT('Ctrl Pts',(-6.60137276000006,12.2,-8.07634552200001));
#286111=CARTESIAN_POINT('Ctrl Pts',(-6.60207968000006,12.2,-8.07749815200001));
#286112=CARTESIAN_POINT('Ctrl Pts',(-6.60278989300005,12.2,-8.07865865600002));
#286113=CARTESIAN_POINT('Ctrl Pts',(-6.60350337600006,12.2,-8.07982702500002));
#286114=CARTESIAN_POINT('Ctrl Pts',(-6.60422010600006,12.2,-8.08100324800002));
#286115=CARTESIAN_POINT('Ctrl Pts',(-6.60494005800006,12.2,-8.08218731500002));
#286116=CARTESIAN_POINT('Ctrl Pts',(-6.60566320900006,12.2,-8.08337921500001));
#286117=CARTESIAN_POINT('Ctrl Pts',(-6.60638953400006,12.2,-8.08457893900002));
#286118=CARTESIAN_POINT('Ctrl Pts',(-6.60711901100006,12.2,-8.08578647500001));
#286119=CARTESIAN_POINT('Ctrl Pts',(-6.60785161500006,12.2,-8.08700181500001));
#286120=CARTESIAN_POINT('Ctrl Pts',(-6.60858732500006,12.2,-8.08822494800001));
#286121=CARTESIAN_POINT('Ctrl Pts',(-6.60932611700006,12.2,-8.08945586400002));
#286122=CARTESIAN_POINT('Ctrl Pts',(-6.61006796600006,12.2,-8.09069455200002));
#286123=CARTESIAN_POINT('Ctrl Pts',(-6.61081285100006,12.2,-8.09194100300001));
#286124=CARTESIAN_POINT('Ctrl Pts',(-6.61156074900005,12.2,-8.09319520700001));
#286125=CARTESIAN_POINT('Ctrl Pts',(-6.61231163600006,12.2,-8.09445715400001));
#286126=CARTESIAN_POINT('Ctrl Pts',(-6.61306549000006,12.2,-8.09572683400001));
#286127=CARTESIAN_POINT('Ctrl Pts',(-6.61382229000006,12.2,-8.09700423600002));
#286128=CARTESIAN_POINT('Ctrl Pts',(-6.61458201100006,12.2,-8.09828935200001));
#286129=CARTESIAN_POINT('Ctrl Pts',(-6.61534463100006,12.2,-8.09958217100002));
#286130=CARTESIAN_POINT('Ctrl Pts',(-6.61611012900006,12.2,-8.10088268300002));
#286131=CARTESIAN_POINT('Ctrl Pts',(-6.61687848200006,12.2,-8.10219087900002));
#286132=CARTESIAN_POINT('Ctrl Pts',(-6.61764966700006,12.2,-8.10350674900001));
#286133=CARTESIAN_POINT('Ctrl Pts',(-6.61842366400006,12.2,-8.10483028300002));
#286134=CARTESIAN_POINT('Ctrl Pts',(-6.61920045000006,12.2,-8.10616147100001));
#286135=CARTESIAN_POINT('Ctrl Pts',(-6.61998000200006,12.2,-8.10750030400002));
#286136=CARTESIAN_POINT('Ctrl Pts',(-6.62076230000006,12.2,-8.10884677100002));
#286137=CARTESIAN_POINT('Ctrl Pts',(-6.62154732100006,12.2,-8.11020086400001));
#286138=CARTESIAN_POINT('Ctrl Pts',(-6.62233504600006,12.2,-8.11156257400001));
#286139=CARTESIAN_POINT('Ctrl Pts',(-6.62312545000006,12.2,-8.11293188900001));
#286140=CARTESIAN_POINT('Ctrl Pts',(-6.62391851400006,12.2,-8.11430880100002));
#286141=CARTESIAN_POINT('Ctrl Pts',(-6.62471421500006,12.2,-8.11569329900001));
#286142=CARTESIAN_POINT('Ctrl Pts',(-6.62551253400006,12.2,-8.11708537600002));
#286143=CARTESIAN_POINT('Ctrl Pts',(-6.62631344800006,12.2,-8.11848502000002));
#286144=CARTESIAN_POINT('Ctrl Pts',(-6.62711693700006,12.2,-8.11989222400002));
#286145=CARTESIAN_POINT('Ctrl Pts',(-6.62792298000006,12.2,-8.12130697600002));
#286146=CARTESIAN_POINT('Ctrl Pts',(-6.62873155500006,12.2,-8.12272926700001));
#286147=CARTESIAN_POINT('Ctrl Pts',(-6.62954264200006,12.2,-8.12415909000002));
#286148=CARTESIAN_POINT('Ctrl Pts',(-6.63035622100006,12.2,-8.12559643400002));
#286149=CARTESIAN_POINT('Ctrl Pts',(-6.63117227000006,12.2,-8.12704128900002));
#286150=CARTESIAN_POINT('Ctrl Pts',(-6.63199077100006,12.2,-8.12849364600002));
#286151=CARTESIAN_POINT('Ctrl Pts',(-6.63281170000006,12.2,-8.12995349700002));
#286152=CARTESIAN_POINT('Ctrl Pts',(-6.63363504000006,12.2,-8.13142083100002));
#286153=CARTESIAN_POINT('Ctrl Pts',(-6.63446076800006,12.2,-8.13289564100002));
#286154=CARTESIAN_POINT('Ctrl Pts',(-6.63528886600006,12.2,-8.13437791500002));
#286155=CARTESIAN_POINT('Ctrl Pts',(-6.63611931200006,12.2,-8.13586764600002));
#286156=CARTESIAN_POINT('Ctrl Pts',(-6.63695208700006,12.2,-8.13736482400002));
#286157=CARTESIAN_POINT('Ctrl Pts',(-6.63778717100006,12.2,-8.13886943900001));
#286158=CARTESIAN_POINT('Ctrl Pts',(-6.63862454400006,12.2,-8.14038148300002));
#286159=CARTESIAN_POINT('Ctrl Pts',(-6.63946418700006,12.2,-8.14190094700002));
#286160=CARTESIAN_POINT('Ctrl Pts',(-6.64030607900005,12.2,-8.14342782100002));
#286161=CARTESIAN_POINT('Ctrl Pts',(-6.64115020100006,12.2,-8.14496209700001));
#286162=CARTESIAN_POINT('Ctrl Pts',(-6.64199653400006,12.2,-8.14650376600002));
#286163=CARTESIAN_POINT('Ctrl Pts',(-6.64284505800006,12.2,-8.14805281700002));
#286164=CARTESIAN_POINT('Ctrl Pts',(-6.64369575300006,12.2,-8.14960924300001));
#286165=CARTESIAN_POINT('Ctrl Pts',(-6.64454859900006,12.2,-8.15117303500001));
#286166=CARTESIAN_POINT('Ctrl Pts',(-6.64540358000006,12.2,-8.15274418300002));
#286167=CARTESIAN_POINT('Ctrl Pts',(-6.64626067400006,12.2,-8.15432267900002));
#286168=CARTESIAN_POINT('Ctrl Pts',(-6.64711986400006,12.2,-8.15590851400002));
#286169=CARTESIAN_POINT('Ctrl Pts',(-6.64798112800006,12.2,-8.15750167800001));
#286170=CARTESIAN_POINT('Ctrl Pts',(-6.64884444900006,12.2,-8.15910216300002));
#286171=CARTESIAN_POINT('Ctrl Pts',(-6.64970980800006,12.2,-8.16070996000001));
#286172=CARTESIAN_POINT('Ctrl Pts',(-6.65057718600006,12.2,-8.16232506100001));
#286173=CARTESIAN_POINT('Ctrl Pts',(-6.65144656600006,12.2,-8.16394745500002));
#286174=CARTESIAN_POINT('Ctrl Pts',(-6.65231792600006,12.2,-8.16557713600002));
#286175=CARTESIAN_POINT('Ctrl Pts',(-6.65319124900006,12.2,-8.16721409300002));
#286176=CARTESIAN_POINT('Ctrl Pts',(-6.65406651700006,12.2,-8.16885831900001));
#286177=CARTESIAN_POINT('Ctrl Pts',(-6.65494371100006,12.2,-8.17050980400002));
#286178=CARTESIAN_POINT('Ctrl Pts',(-6.65582281300006,12.2,-8.17216853900002));
#286179=CARTESIAN_POINT('Ctrl Pts',(-6.65670380500006,12.2,-8.17383451600002));
#286180=CARTESIAN_POINT('Ctrl Pts',(-6.65758666800006,12.2,-8.17550772700002));
#286181=CARTESIAN_POINT('Ctrl Pts',(-6.65847138400006,12.2,-8.17718816300001));
#286182=CARTESIAN_POINT('Ctrl Pts',(-6.65935793500006,12.2,-8.17887581400001));
#286183=CARTESIAN_POINT('Ctrl Pts',(-6.66024630300006,12.2,-8.18057067400002));
#286184=CARTESIAN_POINT('Ctrl Pts',(-6.66113647000006,12.2,-8.18227273100002));
#286185=CARTESIAN_POINT('Ctrl Pts',(-6.66202841900006,12.2,-8.18398198000001));
#286186=CARTESIAN_POINT('Ctrl Pts',(-6.66292212900006,12.2,-8.18569840900001));
#286187=CARTESIAN_POINT('Ctrl Pts',(-6.66381758700005,12.2,-8.18742201300001));
#286188=CARTESIAN_POINT('Ctrl Pts',(-6.66471477200006,12.2,-8.18915278000001));
#286189=CARTESIAN_POINT('Ctrl Pts',(-6.66561366700006,12.2,-8.19089070400001));
#286190=CARTESIAN_POINT('Ctrl Pts',(-6.66651425400006,12.2,-8.19263577600001));
#286191=CARTESIAN_POINT('Ctrl Pts',(-6.66741651800006,12.2,-8.19438798600002));
#286192=CARTESIAN_POINT('Ctrl Pts',(-6.66832043800006,12.2,-8.19614732700002));
#286193=CARTESIAN_POINT('Ctrl Pts',(-6.66922600000006,12.2,-8.19791379200002));
#286194=CARTESIAN_POINT('Ctrl Pts',(-6.67013318300006,12.2,-8.19968736900002));
#286195=CARTESIAN_POINT('Ctrl Pts',(-6.67104197300006,12.2,-8.20146805200002));
#286196=CARTESIAN_POINT('Ctrl Pts',(-6.67195235200006,12.2,-8.20325583300002));
#286197=CARTESIAN_POINT('Ctrl Pts',(-6.67286430200006,12.2,-8.20505070200002));
#286198=CARTESIAN_POINT('Ctrl Pts',(-6.67377780700006,12.2,-8.20685265200002));
#286199=CARTESIAN_POINT('Ctrl Pts',(-6.67469285000006,12.2,-8.20866167300002));
#286200=CARTESIAN_POINT('Ctrl Pts',(-6.67560941300006,12.2,-8.21047775800002));
#286201=CARTESIAN_POINT('Ctrl Pts',(-6.67652747900005,12.2,-8.21230089900002));
#286202=CARTESIAN_POINT('Ctrl Pts',(-6.67744703200006,12.2,-8.21413108800002));
#286203=CARTESIAN_POINT('Ctrl Pts',(-6.67836805600006,12.2,-8.21596831500001));
#286204=CARTESIAN_POINT('Ctrl Pts',(-6.67929053300006,12.2,-8.21781257300002));
#286205=CARTESIAN_POINT('Ctrl Pts',(-6.68021444700006,12.2,-8.21966385300002));
#286206=CARTESIAN_POINT('Ctrl Pts',(-6.68113978100005,12.2,-8.22152214800001));
#286207=CARTESIAN_POINT('Ctrl Pts',(-6.68206651900006,12.2,-8.22338745000001));
#286208=CARTESIAN_POINT('Ctrl Pts',(-6.68299464500006,12.2,-8.22525974700002));
#286209=CARTESIAN_POINT('Ctrl Pts',(-6.68392414200006,12.2,-8.22713903600001));
#286210=CARTESIAN_POINT('Ctrl Pts',(-6.68485499200006,12.2,-8.22902530700001));
#286211=CARTESIAN_POINT('Ctrl Pts',(-6.68578718200005,12.2,-8.23091855000002));
#286212=CARTESIAN_POINT('Ctrl Pts',(-6.68672069300006,12.2,-8.23281875900001));
#286213=CARTESIAN_POINT('Ctrl Pts',(-6.68765551100006,12.2,-8.23472592600002));
#286214=CARTESIAN_POINT('Ctrl Pts',(-6.68859161800006,12.2,-8.23664004100002));
#286215=CARTESIAN_POINT('Ctrl Pts',(-6.68952899900006,12.2,-8.23856109700002));
#286216=CARTESIAN_POINT('Ctrl Pts',(-6.69046763700006,12.2,-8.24048908700002));
#286217=CARTESIAN_POINT('Ctrl Pts',(-6.69140751900006,12.2,-8.24242400100001));
#286218=CARTESIAN_POINT('Ctrl Pts',(-6.69234862600006,12.2,-8.24436583300002));
#286219=CARTESIAN_POINT('Ctrl Pts',(-6.69329094300006,12.2,-8.24631457300002));
#286220=CARTESIAN_POINT('Ctrl Pts',(-6.69423445500006,12.2,-8.24827021500001));
#286221=CARTESIAN_POINT('Ctrl Pts',(-6.69517914500006,12.2,-8.25023274900002));
#286222=CARTESIAN_POINT('Ctrl Pts',(-6.69612499800006,12.2,-8.25220216900002));
#286223=CARTESIAN_POINT('Ctrl Pts',(-6.69707199900006,12.2,-8.25417846500001));
#286224=CARTESIAN_POINT('Ctrl Pts',(-6.69802013200006,12.2,-8.25616163100002));
#286225=CARTESIAN_POINT('Ctrl Pts',(-6.69896938100006,12.2,-8.25815165900002));
#286226=CARTESIAN_POINT('Ctrl Pts',(-6.69991973100006,12.2,-8.26014853800002));
#286227=CARTESIAN_POINT('Ctrl Pts',(-6.70087116700006,12.2,-8.26215226500001));
#286228=CARTESIAN_POINT('Ctrl Pts',(-6.70182367300006,12.2,-8.26416282800002));
#286229=CARTESIAN_POINT('Ctrl Pts',(-6.70277723400006,12.2,-8.26618022100002));
#286230=CARTESIAN_POINT('Ctrl Pts',(-6.70373183500006,12.2,-8.26820443600001));
#286231=CARTESIAN_POINT('Ctrl Pts',(-6.70468746000005,12.2,-8.27023546500002));
#286232=CARTESIAN_POINT('Ctrl Pts',(-6.70564409500006,12.2,-8.27227330000002));
#286233=CARTESIAN_POINT('Ctrl Pts',(-6.70660172400006,12.2,-8.27431793400002));
#286234=CARTESIAN_POINT('Ctrl Pts',(-6.70756033200006,12.2,-8.27636935700001));
#286235=CARTESIAN_POINT('Ctrl Pts',(-6.70851990500006,12.2,-8.27842756400001));
#286236=CARTESIAN_POINT('Ctrl Pts',(-6.70948042600005,12.2,-8.28049254600002));
#286237=CARTESIAN_POINT('Ctrl Pts',(-6.71044188300006,12.2,-8.28256429500002));
#286238=CARTESIAN_POINT('Ctrl Pts',(-6.71140426000005,12.2,-8.28464280400001));
#286239=CARTESIAN_POINT('Ctrl Pts',(-6.71236754100006,12.2,-8.28672806400002));
#286240=CARTESIAN_POINT('Ctrl Pts',(-6.71333171300006,12.2,-8.28882006800002));
#286241=CARTESIAN_POINT('Ctrl Pts',(-6.71429675900006,12.2,-8.29091880900001));
#286242=CARTESIAN_POINT('Ctrl Pts',(-6.71526266700006,12.2,-8.29302427800001));
#286243=CARTESIAN_POINT('Ctrl Pts',(-6.71622942200006,12.2,-8.29513646900002));
#286244=CARTESIAN_POINT('Ctrl Pts',(-6.71719700800006,12.2,-8.29725537200002));
#286245=CARTESIAN_POINT('Ctrl Pts',(-6.71816541100006,12.2,-8.29938098200002));
#286246=CARTESIAN_POINT('Ctrl Pts',(-6.71913461600006,12.2,-8.30151328900002));
#286247=CARTESIAN_POINT('Ctrl Pts',(-6.72010461200006,12.2,-8.30365228700002));
#286248=CARTESIAN_POINT('Ctrl Pts',(-6.72107538000006,12.2,-8.30579796800002));
#286249=CARTESIAN_POINT('Ctrl Pts',(-6.72204690900006,12.2,-8.30795032300001));
#286250=CARTESIAN_POINT('Ctrl Pts',(-6.72301918300006,12.2,-8.31010934800002));
#286251=CARTESIAN_POINT('Ctrl Pts',(-6.72399218800006,12.2,-8.31227503100001));
#286252=CARTESIAN_POINT('Ctrl Pts',(-6.72496591100006,12.2,-8.31444736700002));
#286253=CARTESIAN_POINT('Ctrl Pts',(-6.72594033700006,12.2,-8.31662634800002));
#286254=CARTESIAN_POINT('Ctrl Pts',(-6.72691545200006,12.2,-8.31881196600002));
#286255=CARTESIAN_POINT('Ctrl Pts',(-6.72789124200006,12.2,-8.32100421400002));
#286256=CARTESIAN_POINT('Ctrl Pts',(-6.72886769300006,12.2,-8.32320308500002));
#286257=CARTESIAN_POINT('Ctrl Pts',(-6.72984479100006,12.2,-8.32540857000001));
#286258=CARTESIAN_POINT('Ctrl Pts',(-6.73082252300006,12.2,-8.32762066300001));
#286259=CARTESIAN_POINT('Ctrl Pts',(-6.73180087300006,12.2,-8.32983935500001));
#286260=CARTESIAN_POINT('Ctrl Pts',(-6.73277982900006,12.2,-8.33206464000002));
#286261=CARTESIAN_POINT('Ctrl Pts',(-6.73375937800006,12.2,-8.33429650900002));
#286262=CARTESIAN_POINT('Ctrl Pts',(-6.73473950400005,12.2,-8.33653495700002));
#286263=CARTESIAN_POINT('Ctrl Pts',(-6.73572019500006,12.2,-8.33877997400002));
#286264=CARTESIAN_POINT('Ctrl Pts',(-6.73670143700006,12.2,-8.34103155300001));
#286265=CARTESIAN_POINT('Ctrl Pts',(-6.73768321600006,12.2,-8.34328968900002));
#286266=CARTESIAN_POINT('Ctrl Pts',(-6.73866551900006,12.2,-8.34555437100001));
#286267=CARTESIAN_POINT('Ctrl Pts',(-6.73964833200006,12.2,-8.34782559500002));
#286268=CARTESIAN_POINT('Ctrl Pts',(-6.74063164200006,12.2,-8.35010335100002));
#286269=CARTESIAN_POINT('Ctrl Pts',(-6.74161543500006,12.2,-8.35238763300002));
#286270=CARTESIAN_POINT('Ctrl Pts',(-6.74259969900006,12.2,-8.35467843300002));
#286271=CARTESIAN_POINT('Ctrl Pts',(-6.74358442000006,12.2,-8.35697574500001));
#286272=CARTESIAN_POINT('Ctrl Pts',(-6.74456958400006,12.2,-8.35927956000001));
#286273=CARTESIAN_POINT('Ctrl Pts',(-6.74555517700006,12.2,-8.36158987000001));
#286274=CARTESIAN_POINT('Ctrl Pts',(-6.74654118900006,12.2,-8.36390667000002));
#286275=CARTESIAN_POINT('Ctrl Pts',(-6.74752760400006,12.2,-8.36622995200001));
#286276=CARTESIAN_POINT('Ctrl Pts',(-6.74851441000006,12.2,-8.36855970800002));
#286277=CARTESIAN_POINT('Ctrl Pts',(-6.74950159300006,12.2,-8.37089593100002));
#286278=CARTESIAN_POINT('Ctrl Pts',(-6.75048914200006,12.2,-8.37323861500002));
#286279=CARTESIAN_POINT('Ctrl Pts',(-6.75147704200006,12.2,-8.37558775000002));
#286280=CARTESIAN_POINT('Ctrl Pts',(-6.75246528000006,12.2,-8.37794333100002));
#286281=CARTESIAN_POINT('Ctrl Pts',(-6.75345384400006,12.2,-8.38030535000001));
#286282=CARTESIAN_POINT('Ctrl Pts',(-6.75444272200005,12.2,-8.38267380000002));
#286283=CARTESIAN_POINT('Ctrl Pts',(-6.75543189900006,12.2,-8.38504867300001));
#286284=CARTESIAN_POINT('Ctrl Pts',(-6.75642136400006,12.2,-8.38742996300001));
#286285=CARTESIAN_POINT('Ctrl Pts',(-6.75741110400006,12.2,-8.38981766200002));
#286286=CARTESIAN_POINT('Ctrl Pts',(-6.75840110500006,12.2,-8.39221176300001));
#286287=CARTESIAN_POINT('Ctrl Pts',(-6.75939135700006,12.2,-8.39461225900001));
#286288=CARTESIAN_POINT('Ctrl Pts',(-6.76038184400006,12.2,-8.39701914200001));
#286289=CARTESIAN_POINT('Ctrl Pts',(-6.76137255500006,12.2,-8.39943240700002));
#286290=CARTESIAN_POINT('Ctrl Pts',(-6.76236347800006,12.2,-8.40185204500001));
#286291=CARTESIAN_POINT('Ctrl Pts',(-6.76335460000006,12.2,-8.40427804800001));
#286292=CARTESIAN_POINT('Ctrl Pts',(-6.76434590800006,12.2,-8.40671041100002));
#286293=CARTESIAN_POINT('Ctrl Pts',(-6.76533739000006,12.2,-8.40914912700002));
#286294=CARTESIAN_POINT('Ctrl Pts',(-6.76632903400006,12.2,-8.41159418600002));
#286295=CARTESIAN_POINT('Ctrl Pts',(-6.76732082700005,12.2,-8.41404558300002));
#286296=CARTESIAN_POINT('Ctrl Pts',(-6.76831275600006,12.2,-8.41650331100002));
#286297=CARTESIAN_POINT('Ctrl Pts',(-6.76930481100006,12.2,-8.41896736400002));
#286298=CARTESIAN_POINT('Ctrl Pts',(-6.77029697800006,12.2,-8.42143773200002));
#286299=CARTESIAN_POINT('Ctrl Pts',(-6.77128924400006,12.2,-8.42391441000002));
#286300=CARTESIAN_POINT('Ctrl Pts',(-6.77228160000006,12.2,-8.42639739000001));
#286301=CARTESIAN_POINT('Ctrl Pts',(-6.77327403000006,12.2,-8.42888666600001));
#286302=CARTESIAN_POINT('Ctrl Pts',(-6.77426652500006,12.2,-8.43138223000001));
#286303=CARTESIAN_POINT('Ctrl Pts',(-6.77525907000006,12.2,-8.43388407500001));
#286304=CARTESIAN_POINT('Ctrl Pts',(-6.77625165600006,12.2,-8.43639219400002));
#286305=CARTESIAN_POINT('Ctrl Pts',(-6.77724426900006,12.2,-8.43890658100002));
#286306=CARTESIAN_POINT('Ctrl Pts',(-6.77823689800006,12.2,-8.44142722800001));
#286307=CARTESIAN_POINT('Ctrl Pts',(-6.77922953100006,12.2,-8.44395412900001));
#286308=CARTESIAN_POINT('Ctrl Pts',(-6.78022215500006,12.2,-8.44648727600001));
#286309=CARTESIAN_POINT('Ctrl Pts',(-6.78121475800006,12.2,-8.44902666100002));
#286310=CARTESIAN_POINT('Ctrl Pts',(-6.78220733100006,12.2,-8.45157227900001));
#286311=CARTESIAN_POINT('Ctrl Pts',(-6.78319986000006,12.2,-8.45412412300002));
#286312=CARTESIAN_POINT('Ctrl Pts',(-6.78419233200006,12.2,-8.45668218600002));
#286313=CARTESIAN_POINT('Ctrl Pts',(-6.78518473900006,12.2,-8.45924645900002));
#286314=CARTESIAN_POINT('Ctrl Pts',(-6.78617706600006,12.2,-8.46181693800002));
#286315=CARTESIAN_POINT('Ctrl Pts',(-6.78716930300006,12.2,-8.46439361500002));
#286316=CARTESIAN_POINT('Ctrl Pts',(-6.78816143700006,12.2,-8.46697648200001));
#286317=CARTESIAN_POINT('Ctrl Pts',(-6.78915345800006,12.2,-8.46956553300002));
#286318=CARTESIAN_POINT('Ctrl Pts',(-6.79014535300006,12.2,-8.47216076000001));
#286319=CARTESIAN_POINT('Ctrl Pts',(-6.79113711200006,12.2,-8.47476215800001));
#286320=CARTESIAN_POINT('Ctrl Pts',(-6.79212872200006,12.2,-8.47736971900002));
#286321=CARTESIAN_POINT('Ctrl Pts',(-6.79312017300005,12.2,-8.47998343700001));
#286322=CARTESIAN_POINT('Ctrl Pts',(-6.79411145300006,12.2,-8.48260330400001));
#286323=CARTESIAN_POINT('Ctrl Pts',(-6.79510255000006,12.2,-8.48522931400002));
#286324=CARTESIAN_POINT('Ctrl Pts',(-6.79609345300006,12.2,-8.48786145900002));
#286325=CARTESIAN_POINT('Ctrl Pts',(-6.79708415200006,12.2,-8.49049973300002));
#286326=CARTESIAN_POINT('Ctrl Pts',(-6.79807463300006,12.2,-8.49314413000002));
#286327=CARTESIAN_POINT('Ctrl Pts',(-6.79906488700006,12.2,-8.49579464200002));
#286328=CARTESIAN_POINT('Ctrl Pts',(-6.80005490300006,12.2,-8.49845126300002));
#286329=CARTESIAN_POINT('Ctrl Pts',(-6.80104466800006,12.2,-8.50111398400001));
#286330=CARTESIAN_POINT('Ctrl Pts',(-6.80203417100006,12.2,-8.50378280200001));
#286331=CARTESIAN_POINT('Ctrl Pts',(-6.80302340200006,12.2,-8.50645770700002));
#286332=CARTESIAN_POINT('Ctrl Pts',(-6.80401234900006,12.2,-8.50913869300001));
#286333=CARTESIAN_POINT('Ctrl Pts',(-6.80500100400006,12.2,-8.51182575500001));
#286334=CARTESIAN_POINT('Ctrl Pts',(-6.80598935100006,12.2,-8.51451888400002));
#286335=CARTESIAN_POINT('Ctrl Pts',(-6.80697738200006,12.2,-8.51721807500001));
#286336=CARTESIAN_POINT('Ctrl Pts',(-6.80796508500006,12.2,-8.51992331800002));
#286337=CARTESIAN_POINT('Ctrl Pts',(-6.80895244900006,12.2,-8.52263461100002));
#286338=CARTESIAN_POINT('Ctrl Pts',(-6.80993946500006,12.2,-8.52535194300001));
#286339=CARTESIAN_POINT('Ctrl Pts',(-6.81092612100006,12.2,-8.52807531000002));
#286340=CARTESIAN_POINT('Ctrl Pts',(-6.81191240500006,12.2,-8.53080470500002));
#286341=CARTESIAN_POINT('Ctrl Pts',(-6.81289830700006,12.2,-8.53354012000001));
#286342=CARTESIAN_POINT('Ctrl Pts',(-6.81388381700006,12.2,-8.53628154900001));
#286343=CARTESIAN_POINT('Ctrl Pts',(-6.81486892200006,12.2,-8.53902898500002));
#286344=CARTESIAN_POINT('Ctrl Pts',(-6.81585361400006,12.2,-8.54178242200001));
#286345=CARTESIAN_POINT('Ctrl Pts',(-6.81683788100006,12.2,-8.54454185300002));
#286346=CARTESIAN_POINT('Ctrl Pts',(-6.81782171200005,12.2,-8.54730727200002));
#286347=CARTESIAN_POINT('Ctrl Pts',(-6.81880509800005,12.2,-8.55007867000002));
#286348=CARTESIAN_POINT('Ctrl Pts',(-6.81978802600006,12.2,-8.55285604300001));
#286349=CARTESIAN_POINT('Ctrl Pts',(-6.82077048700005,12.2,-8.55563938300002));
#286350=CARTESIAN_POINT('Ctrl Pts',(-6.82175247000006,12.2,-8.55842868400002));
#286351=CARTESIAN_POINT('Ctrl Pts',(-6.82273396500006,12.2,-8.56122393900002));
#286352=CARTESIAN_POINT('Ctrl Pts',(-6.82371496100005,12.2,-8.56402514100001));
#286353=CARTESIAN_POINT('Ctrl Pts',(-6.82469544700006,12.2,-8.56683228400002));
#286354=CARTESIAN_POINT('Ctrl Pts',(-6.82567541400006,12.2,-8.56964536100002));
#286355=CARTESIAN_POINT('Ctrl Pts',(-6.82665485100006,12.2,-8.57246436600001));
#286356=CARTESIAN_POINT('Ctrl Pts',(-6.82763374600006,12.2,-8.57528929200001));
#286357=CARTESIAN_POINT('Ctrl Pts',(-6.82861209100006,12.2,-8.57812013100002));
#286358=CARTESIAN_POINT('Ctrl Pts',(-6.82958987600006,12.2,-8.58095688000001));
#286359=CARTESIAN_POINT('Ctrl Pts',(-6.83056708700006,12.2,-8.58379952900002));
#286360=CARTESIAN_POINT('Ctrl Pts',(-6.83154371800006,12.2,-8.58664807300002));
#286361=CARTESIAN_POINT('Ctrl Pts',(-6.83251975600006,12.2,-8.58950250500002));
#286362=CARTESIAN_POINT('Ctrl Pts',(-6.83349519400006,12.2,-8.59236281800002));
#286363=CARTESIAN_POINT('Ctrl Pts',(-6.83447001700006,12.2,-8.59522900700001));
#286364=CARTESIAN_POINT('Ctrl Pts',(-6.83544421900006,12.2,-8.59810106300002));
#286365=CARTESIAN_POINT('Ctrl Pts',(-6.83641778800006,12.2,-8.60097898100002));
#286366=CARTESIAN_POINT('Ctrl Pts',(-6.83739071400006,12.2,-8.60386275500002));
#286367=CARTESIAN_POINT('Ctrl Pts',(-6.83836298800006,12.2,-8.60675237800002));
#286368=CARTESIAN_POINT('Ctrl Pts',(-6.83933459800006,12.2,-8.60964784300002));
#286369=CARTESIAN_POINT('Ctrl Pts',(-6.84030553600006,12.2,-8.61254914500002));
#286370=CARTESIAN_POINT('Ctrl Pts',(-6.84127579200006,12.2,-8.61545627500002));
#286371=CARTESIAN_POINT('Ctrl Pts',(-6.84224535400006,12.2,-8.61836922800002));
#286372=CARTESIAN_POINT('Ctrl Pts',(-6.84321421300006,12.2,-8.62128799800002));
#286373=CARTESIAN_POINT('Ctrl Pts',(-6.84418236000006,12.2,-8.62421257800002));
#286374=CARTESIAN_POINT('Ctrl Pts',(-6.84514978400006,12.2,-8.62714296000001));
#286375=CARTESIAN_POINT('Ctrl Pts',(-6.84611647700006,12.2,-8.63007914000002));
#286376=CARTESIAN_POINT('Ctrl Pts',(-6.84708242700006,12.2,-8.63302111000002));
#286377=CARTESIAN_POINT('Ctrl Pts',(-6.84804762500006,12.2,-8.63596886400002));
#286378=CARTESIAN_POINT('Ctrl Pts',(-6.84901206200006,12.2,-8.63892239500002));
#286379=CARTESIAN_POINT('Ctrl Pts',(-6.84997572700006,12.2,-8.64188169800002));
#286380=CARTESIAN_POINT('Ctrl Pts',(-6.85093861100006,12.2,-8.64484676500001));
#286381=CARTESIAN_POINT('Ctrl Pts',(-6.85190070400005,12.2,-8.64781759100002));
#286382=CARTESIAN_POINT('Ctrl Pts',(-6.85286199700006,12.2,-8.65079416800001));
#286383=CARTESIAN_POINT('Ctrl Pts',(-6.85382248000006,12.2,-8.65377649100001));
#286384=CARTESIAN_POINT('Ctrl Pts',(-6.85478214300006,12.2,-8.65676455300001));
#286385=CARTESIAN_POINT('Ctrl Pts',(-6.85574097600006,12.2,-8.65975834700001));
#286386=CARTESIAN_POINT('Ctrl Pts',(-6.85669897100006,12.2,-8.66275786700001));
#286387=CARTESIAN_POINT('Ctrl Pts',(-6.85765611700006,12.2,-8.66576310700001));
#286388=CARTESIAN_POINT('Ctrl Pts',(-6.85861240500006,12.2,-8.66877406100001));
#286389=CARTESIAN_POINT('Ctrl Pts',(-6.85956782600006,12.2,-8.67179072200001));
#286390=CARTESIAN_POINT('Ctrl Pts',(-6.86052237000006,12.2,-8.67481308300002));
#286391=CARTESIAN_POINT('Ctrl Pts',(-6.86147602800006,12.2,-8.67784113800001));
#286392=CARTESIAN_POINT('Ctrl Pts',(-6.86242879000006,12.2,-8.68087488200001));
#286393=CARTESIAN_POINT('Ctrl Pts',(-6.86338064600006,12.2,-8.68391430700001));
#286394=CARTESIAN_POINT('Ctrl Pts',(-6.86433158900006,12.2,-8.68695940700002));
#286395=CARTESIAN_POINT('Ctrl Pts',(-6.86528160700006,12.2,-8.69001017600001));
#286396=CARTESIAN_POINT('Ctrl Pts',(-6.86623069200006,12.2,-8.69306660700002));
#286397=CARTESIAN_POINT('Ctrl Pts',(-6.86717883600005,12.2,-8.69612869500001));
#286398=CARTESIAN_POINT('Ctrl Pts',(-6.86812602700006,12.2,-8.69919643300002));
#286399=CARTESIAN_POINT('Ctrl Pts',(-6.86907225800006,12.2,-8.70226981300002));
#286400=CARTESIAN_POINT('Ctrl Pts',(-6.87001751800006,12.2,-8.70534883200002));
#286401=CARTESIAN_POINT('Ctrl Pts',(-6.87096179900006,12.2,-8.70843348100001));
#286402=CARTESIAN_POINT('Ctrl Pts',(-6.87190509000006,12.2,-8.71152375400002));
#286403=CARTESIAN_POINT('Ctrl Pts',(-6.87284738500006,12.2,-8.71461964600002));
#286404=CARTESIAN_POINT('Ctrl Pts',(-6.87378867400006,12.2,-8.71772115000002));
#286405=CARTESIAN_POINT('Ctrl Pts',(-6.87472894500006,12.2,-8.72082826000002));
#286406=CARTESIAN_POINT('Ctrl Pts',(-6.87566819300006,12.2,-8.72394096800001));
#286407=CARTESIAN_POINT('Ctrl Pts',(-6.87660640700006,12.2,-8.72705927100002));
#286408=CARTESIAN_POINT('Ctrl Pts',(-6.87754357700006,12.2,-8.73018316100002));
#286409=CARTESIAN_POINT('Ctrl Pts',(-6.87847969500006,12.2,-8.73331263000001));
#286410=CARTESIAN_POINT('Ctrl Pts',(-6.87941475200006,12.2,-8.73644767400001));
#286411=CARTESIAN_POINT('Ctrl Pts',(-6.88034873900006,12.2,-8.73958828600001));
#286412=CARTESIAN_POINT('Ctrl Pts',(-6.88128164800006,12.2,-8.74273446000002));
#286413=CARTESIAN_POINT('Ctrl Pts',(-6.88221346800006,12.2,-8.74588619000002));
#286414=CARTESIAN_POINT('Ctrl Pts',(-6.88314419200006,12.2,-8.74904347000001));
#286415=CARTESIAN_POINT('Ctrl Pts',(-6.88407381100006,12.2,-8.75220629200001));
#286416=CARTESIAN_POINT('Ctrl Pts',(-6.88500231400006,12.2,-8.75537465100001));
#286417=CARTESIAN_POINT('Ctrl Pts',(-6.88592969500006,12.2,-8.75854854100002));
#286418=CARTESIAN_POINT('Ctrl Pts',(-6.88685594400006,12.2,-8.76172795500001));
#286419=CARTESIAN_POINT('Ctrl Pts',(-6.88778105300006,12.2,-8.76491288800001));
#286420=CARTESIAN_POINT('Ctrl Pts',(-6.88870501100006,12.2,-8.76810333200002));
#286421=CARTESIAN_POINT('Ctrl Pts',(-6.88962781100006,12.2,-8.77129928300001));
#286422=CARTESIAN_POINT('Ctrl Pts',(-6.89054944500006,12.2,-8.77450073400002));
#286423=CARTESIAN_POINT('Ctrl Pts',(-6.89146990300006,12.2,-8.77770767800002));
#286424=CARTESIAN_POINT('Ctrl Pts',(-6.89238917600006,12.2,-8.78092010900002));
#286425=CARTESIAN_POINT('Ctrl Pts',(-6.89330725700006,12.2,-8.78413802100001));
#286426=CARTESIAN_POINT('Ctrl Pts',(-6.89422413500006,12.2,-8.78736140900001));
#286427=CARTESIAN_POINT('Ctrl Pts',(-6.89513980400006,12.2,-8.79059026500002));
#286428=CARTESIAN_POINT('Ctrl Pts',(-6.89605425400006,12.2,-8.79382458400002));
#286429=CARTESIAN_POINT('Ctrl Pts',(-6.89696747600006,12.2,-8.79706435900001));
#286430=CARTESIAN_POINT('Ctrl Pts',(-6.89787946300005,12.2,-8.80030958500001));
#286431=CARTESIAN_POINT('Ctrl Pts',(-6.89879020600006,12.2,-8.80356025400001));
#286432=CARTESIAN_POINT('Ctrl Pts',(-6.89969969600006,12.2,-8.80681636200002));
#286433=CARTESIAN_POINT('Ctrl Pts',(-6.90060792400006,12.2,-8.81007790200002));
#286434=CARTESIAN_POINT('Ctrl Pts',(-6.90151488200006,12.2,-8.81334486800002));
#286435=CARTESIAN_POINT('Ctrl Pts',(-6.90242056300006,12.2,-8.81661725300001));
#286436=CARTESIAN_POINT('Ctrl Pts',(-6.90332495800006,12.2,-8.81989505100002));
#286437=CARTESIAN_POINT('Ctrl Pts',(-6.90422805600006,12.2,-8.82317825800002));
#286438=CARTESIAN_POINT('Ctrl Pts',(-6.90512985200006,12.2,-8.82646686600001));
#286439=CARTESIAN_POINT('Ctrl Pts',(-6.90603033600006,12.2,-8.82976086800002));
#286440=CARTESIAN_POINT('Ctrl Pts',(-6.90692950100006,12.2,-8.83306026000002));
#286441=CARTESIAN_POINT('Ctrl Pts',(-6.90782733600006,12.2,-8.83636503500002));
#286442=CARTESIAN_POINT('Ctrl Pts',(-6.90872383500006,12.2,-8.83967518700001));
#286443=CARTESIAN_POINT('Ctrl Pts',(-6.90961899000006,12.2,-8.84299071000001));
#286444=CARTESIAN_POINT('Ctrl Pts',(-6.91051279100006,12.2,-8.84631159700002));
#286445=CARTESIAN_POINT('Ctrl Pts',(-6.91140523100006,12.2,-8.84963784300002));
#286446=CARTESIAN_POINT('Ctrl Pts',(-6.91229630100006,12.2,-8.85296944200002));
#286447=CARTESIAN_POINT('Ctrl Pts',(-6.91318599400006,12.2,-8.85630638800002));
#286448=CARTESIAN_POINT('Ctrl Pts',(-6.91407430200006,12.2,-8.85964867300002));
#286449=CARTESIAN_POINT('Ctrl Pts',(-6.91496121500006,12.2,-8.86299629400002));
#286450=CARTESIAN_POINT('Ctrl Pts',(-6.91584672600006,12.2,-8.86634924200001));
#286451=CARTESIAN_POINT('Ctrl Pts',(-6.91673082700006,12.2,-8.86970751300002));
#286452=CARTESIAN_POINT('Ctrl Pts',(-6.91761351000006,12.2,-8.87307110000001));
#286453=CARTESIAN_POINT('Ctrl Pts',(-6.91849476600006,12.2,-8.87643999800002));
#286454=CARTESIAN_POINT('Ctrl Pts',(-6.91937458800005,12.2,-8.87981420000001));
#286455=CARTESIAN_POINT('Ctrl Pts',(-6.92025296800006,12.2,-8.88319369900002));
#286456=CARTESIAN_POINT('Ctrl Pts',(-6.92112989800005,12.2,-8.88657849200002));
#286457=CARTESIAN_POINT('Ctrl Pts',(-6.92200536800006,12.2,-8.88996857000001));
#286458=CARTESIAN_POINT('Ctrl Pts',(-6.92287937300006,12.2,-8.89336392900002));
#286459=CARTESIAN_POINT('Ctrl Pts',(-6.92375190400006,12.2,-8.89676456100002));
#286460=CARTESIAN_POINT('Ctrl Pts',(-6.92462295300006,12.2,-8.90017046300001));
#286461=CARTESIAN_POINT('Ctrl Pts',(-6.92549251200006,12.2,-8.90358162500002));
#286462=CARTESIAN_POINT('Ctrl Pts',(-6.92636057200006,12.2,-8.90699804400001));
#286463=CARTESIAN_POINT('Ctrl Pts',(-6.92722712700006,12.2,-8.91041971300002));
#286464=CARTESIAN_POINT('Ctrl Pts',(-6.92809216800006,12.2,-8.91384662700002));
#286465=CARTESIAN_POINT('Ctrl Pts',(-6.92895568900005,12.2,-8.91727877800001));
#286466=CARTESIAN_POINT('Ctrl Pts',(-6.92981767900006,12.2,-8.92071616200001));
#286467=CARTESIAN_POINT('Ctrl Pts',(-6.93067813200006,12.2,-8.92415877200002));
#286468=CARTESIAN_POINT('Ctrl Pts',(-6.93153704100006,12.2,-8.92760660300001));
#286469=CARTESIAN_POINT('Ctrl Pts',(-6.93239439700006,12.2,-8.93105964700002));
#286470=CARTESIAN_POINT('Ctrl Pts',(-6.93325019300006,12.2,-8.93451789900002));
#286471=CARTESIAN_POINT('Ctrl Pts',(-6.93410442200006,12.2,-8.93798135500001));
#286472=CARTESIAN_POINT('Ctrl Pts',(-6.93495707400006,12.2,-8.94145000600002));
#286473=CARTESIAN_POINT('Ctrl Pts',(-6.93580814300006,12.2,-8.94492384900002));
#286474=CARTESIAN_POINT('Ctrl Pts',(-6.93665762200006,12.2,-8.94840287600001));
#286475=CARTESIAN_POINT('Ctrl Pts',(-6.93750550100006,12.2,-8.95188708100001));
#286476=CARTESIAN_POINT('Ctrl Pts',(-6.93835177400006,12.2,-8.95537645900001));
#286477=CARTESIAN_POINT('Ctrl Pts',(-6.93919643300006,12.2,-8.95887100400002));
#286478=CARTESIAN_POINT('Ctrl Pts',(-6.94003947100006,12.2,-8.96237071000002));
#286479=CARTESIAN_POINT('Ctrl Pts',(-6.94088088100006,12.2,-8.96587557000002));
#286480=CARTESIAN_POINT('Ctrl Pts',(-6.94172065300006,12.2,-8.96938558000001));
#286481=CARTESIAN_POINT('Ctrl Pts',(-6.94255878100006,12.2,-8.97290073300002));
#286482=CARTESIAN_POINT('Ctrl Pts',(-6.94339525800006,12.2,-8.97642102300001));
#286483=CARTESIAN_POINT('Ctrl Pts',(-6.94423007700006,12.2,-8.97994644400002));
#286484=CARTESIAN_POINT('Ctrl Pts',(-6.94506322800006,12.2,-8.98347699100002));
#286485=CARTESIAN_POINT('Ctrl Pts',(-6.94589470500006,12.2,-8.98701265600002));
#286486=CARTESIAN_POINT('Ctrl Pts',(-6.94672450200006,12.2,-8.99055343700002));
#286487=CARTESIAN_POINT('Ctrl Pts',(-6.94755260900005,12.2,-8.99409932400001));
#286488=CARTESIAN_POINT('Ctrl Pts',(-6.94837902000006,12.2,-8.99765031300002));
#286489=CARTESIAN_POINT('Ctrl Pts',(-6.94920372700006,12.2,-9.00120639800001));
#286490=CARTESIAN_POINT('Ctrl Pts',(-6.95002672400006,12.2,-9.00476757400002));
#286491=CARTESIAN_POINT('Ctrl Pts',(-6.95084800200005,12.2,-9.00833383300002));
#286492=CARTESIAN_POINT('Ctrl Pts',(-6.95166755500006,12.2,-9.01190517100002));
#286493=CARTESIAN_POINT('Ctrl Pts',(-6.95248537400006,12.2,-9.01548158100002));
#286494=CARTESIAN_POINT('Ctrl Pts',(-6.95330145500006,12.2,-9.01906305900001));
#286495=CARTESIAN_POINT('Ctrl Pts',(-6.95411578700006,12.2,-9.02264959600002));
#286496=CARTESIAN_POINT('Ctrl Pts',(-6.95492836400006,12.2,-9.02624119000001));
#286497=CARTESIAN_POINT('Ctrl Pts',(-6.95573917800006,12.2,-9.02983783100002));
#286498=CARTESIAN_POINT('Ctrl Pts',(-6.95654822400006,12.2,-9.03343951600002));
#286499=CARTESIAN_POINT('Ctrl Pts',(-6.95735549400006,12.2,-9.03704623800002));
#286500=CARTESIAN_POINT('Ctrl Pts',(-6.95816097900006,12.2,-9.04065799200002));
#286501=CARTESIAN_POINT('Ctrl Pts',(-6.95896467400006,12.2,-9.04427477200001));
#286502=CARTESIAN_POINT('Ctrl Pts',(-6.95976657100006,12.2,-9.04789657100002));
#286503=CARTESIAN_POINT('Ctrl Pts',(-6.96056666300006,12.2,-9.05152338500002));
#286504=CARTESIAN_POINT('Ctrl Pts',(-6.96136494300006,12.2,-9.05515520900002));
#286505=CARTESIAN_POINT('Ctrl Pts',(-6.96216140500006,12.2,-9.05879203500002));
#286506=CARTESIAN_POINT('Ctrl Pts',(-6.96295604000006,12.2,-9.06243385600002));
#286507=CARTESIAN_POINT('Ctrl Pts',(-6.96374884000006,12.2,-9.06608066900001));
#286508=CARTESIAN_POINT('Ctrl Pts',(-6.96453980000006,12.2,-9.06973246600002));
#286509=CARTESIAN_POINT('Ctrl Pts',(-6.96532891100006,12.2,-9.07338924200002));
#286510=CARTESIAN_POINT('Ctrl Pts',(-6.96611616800006,12.2,-9.07705099100001));
#286511=CARTESIAN_POINT('Ctrl Pts',(-6.96690156100006,12.2,-9.08071770700002));
#286512=CARTESIAN_POINT('Ctrl Pts',(-6.96768508700006,12.2,-9.08438938500002));
#286513=CARTESIAN_POINT('Ctrl Pts',(-6.96846673800006,12.2,-9.08806602100002));
#286514=CARTESIAN_POINT('Ctrl Pts',(-6.96924650800006,12.2,-9.09174760800001));
#286515=CARTESIAN_POINT('Ctrl Pts',(-6.97002439000006,12.2,-9.09543414100002));
#286516=CARTESIAN_POINT('Ctrl Pts',(-6.97080037900006,12.2,-9.09912561500001));
#286517=CARTESIAN_POINT('Ctrl Pts',(-6.97157446400006,12.2,-9.10282202200002));
#286518=CARTESIAN_POINT('Ctrl Pts',(-6.97234663900006,12.2,-9.10652335600002));
#286519=CARTESIAN_POINT('Ctrl Pts',(-6.97311689200006,12.2,-9.11022960800001));
#286520=CARTESIAN_POINT('Ctrl Pts',(-6.97388521800006,12.2,-9.11394077400002));
#286521=CARTESIAN_POINT('Ctrl Pts',(-6.97465160800006,12.2,-9.11765684500002));
#286522=CARTESIAN_POINT('Ctrl Pts',(-6.97541605700006,12.2,-9.12137781700002));
#286523=CARTESIAN_POINT('Ctrl Pts',(-6.97617855900006,12.2,-9.12510368500002));
#286524=CARTESIAN_POINT('Ctrl Pts',(-6.97693911100006,12.2,-9.12883444900002));
#286525=CARTESIAN_POINT('Ctrl Pts',(-6.97769771300006,12.2,-9.13257010500002));
#286526=CARTESIAN_POINT('Ctrl Pts',(-6.97830303200006,12.2,-9.13556254300002));
#286527=CARTESIAN_POINT('Ctrl Pts',(-6.97875614300006,12.2,-9.13780907300002));
#286528=CARTESIAN_POINT('Ctrl Pts',(-6.97905782800006,12.2,-9.13930773800002));
#286529=CARTESIAN_POINT('Ctrl Pts',(-6.97920857100006,12.2,-9.14005731500002));
#286530=CARTESIAN_POINT('Origin',(-5.66257110645729E-14,15.2,-1.77635683940025E-14));
#286531=CARTESIAN_POINT('',(-5.36127880600006,15.2,-8.88241603200001));
#286532=CARTESIAN_POINT('',(-5.36127880600006,12.2,-8.88241603200001));
#286533=CARTESIAN_POINT('',(-5.36127880600006,15.2,-8.88241603200001));
#286534=CARTESIAN_POINT('Origin',(-5.66257110645729E-14,12.2,-1.77635683940025E-14));
#286535=CARTESIAN_POINT('Origin',(-5.66257110645729E-14,15.2,-1.77635683940025E-14));
#286536=CARTESIAN_POINT('Origin',(-5.66257110645729E-14,15.2,-1.77635683940025E-14));
#286537=CARTESIAN_POINT('',(-5.60740451300005,15.2,-10.040269649));
#286538=CARTESIAN_POINT('',(-5.26939701900006,15.2,-10.221714878));
#286539=CARTESIAN_POINT('Origin',(-5.66257110645729E-14,15.2,-1.77635683940025E-14));
#286540=CARTESIAN_POINT('',(-5.26939701900006,12.2,-10.221714878));
#286541=CARTESIAN_POINT('',(-5.26939701900006,15.2,-10.221714878));
#286542=CARTESIAN_POINT('',(-5.60740451300005,12.2,-10.040269649));
#286543=CARTESIAN_POINT('Origin',(-5.66257110645729E-14,12.2,-1.77635683940025E-14));
#286544=CARTESIAN_POINT('',(-5.60740451300005,15.2,-10.040269649));
#286545=CARTESIAN_POINT('Ctrl Pts',(-5.36127880600006,15.2,-8.88241603200001));
#286546=CARTESIAN_POINT('Ctrl Pts',(-5.36127880600006,11.6,-8.88241603200001));
#286547=CARTESIAN_POINT('Ctrl Pts',(-5.36135574300006,15.2,-8.88257249700001));
#286548=CARTESIAN_POINT('Ctrl Pts',(-5.36135574300006,11.6,-8.88257249700001));
#286549=CARTESIAN_POINT('Ctrl Pts',(-5.36151222900005,15.2,-8.88289093000001));
#286550=CARTESIAN_POINT('Ctrl Pts',(-5.36151222900005,11.6,-8.88289093000001));
#286551=CARTESIAN_POINT('Ctrl Pts',(-5.36174910500006,15.2,-8.88337354800001));
#286552=CARTESIAN_POINT('Ctrl Pts',(-5.36174910500006,11.6,-8.88337354800001));
#286553=CARTESIAN_POINT('Ctrl Pts',(-5.36206771100006,15.2,-8.88402391700001));
#286554=CARTESIAN_POINT('Ctrl Pts',(-5.36206771100006,11.6,-8.88402391700001));
#286555=CARTESIAN_POINT('Ctrl Pts',(-5.36246988000006,15.2,-8.88484693800002));
#286556=CARTESIAN_POINT('Ctrl Pts',(-5.36246988000006,11.6,-8.88484693800002));
#286557=CARTESIAN_POINT('Ctrl Pts',(-5.36287772900006,15.2,-8.88568371000002));
#286558=CARTESIAN_POINT('Ctrl Pts',(-5.36287772900006,11.6,-8.88568371000002));
#286559=CARTESIAN_POINT('Ctrl Pts',(-5.36328889700005,15.2,-8.88652944600001));
#286560=CARTESIAN_POINT('Ctrl Pts',(-5.36328889700005,11.6,-8.88652944600001));
#286561=CARTESIAN_POINT('Ctrl Pts',(-5.36370335800005,15.2,-8.88738413200001));
#286562=CARTESIAN_POINT('Ctrl Pts',(-5.36370335800005,11.6,-8.88738413200001));
#286563=CARTESIAN_POINT('Ctrl Pts',(-5.36412108300006,15.2,-8.88824775000002));
#286564=CARTESIAN_POINT('Ctrl Pts',(-5.36412108300006,11.6,-8.88824775000002));
#286565=CARTESIAN_POINT('Ctrl Pts',(-5.36454204500005,15.2,-8.88912028400001));
#286566=CARTESIAN_POINT('Ctrl Pts',(-5.36454204500005,11.6,-8.88912028400001));
#286567=CARTESIAN_POINT('Ctrl Pts',(-5.36496621600006,15.2,-8.89000172000001));
#286568=CARTESIAN_POINT('Ctrl Pts',(-5.36496621600006,11.6,-8.89000172000001));
#286569=CARTESIAN_POINT('Ctrl Pts',(-5.36539356700006,15.2,-8.89089203900001));
#286570=CARTESIAN_POINT('Ctrl Pts',(-5.36539356700006,11.6,-8.89089203900001));
#286571=CARTESIAN_POINT('Ctrl Pts',(-5.36582407300005,15.2,-8.89179122800002));
#286572=CARTESIAN_POINT('Ctrl Pts',(-5.36582407300005,11.6,-8.89179122800002));
#286573=CARTESIAN_POINT('Ctrl Pts',(-5.36625770500006,15.2,-8.89269926800001));
#286574=CARTESIAN_POINT('Ctrl Pts',(-5.36625770500006,11.6,-8.89269926800001));
#286575=CARTESIAN_POINT('Ctrl Pts',(-5.36669443700006,15.2,-8.89361614500002));
#286576=CARTESIAN_POINT('Ctrl Pts',(-5.36669443700006,11.6,-8.89361614500002));
#286577=CARTESIAN_POINT('Ctrl Pts',(-5.36713424100006,15.2,-8.89454184300002));
#286578=CARTESIAN_POINT('Ctrl Pts',(-5.36713424100006,11.6,-8.89454184300002));
#286579=CARTESIAN_POINT('Ctrl Pts',(-5.36757709000006,15.2,-8.89547634600002));
#286580=CARTESIAN_POINT('Ctrl Pts',(-5.36757709000006,11.6,-8.89547634600002));
#286581=CARTESIAN_POINT('Ctrl Pts',(-5.36802295900006,15.2,-8.89641963800001));
#286582=CARTESIAN_POINT('Ctrl Pts',(-5.36802295900006,11.6,-8.89641963800001));
#286583=CARTESIAN_POINT('Ctrl Pts',(-5.36847181900006,15.2,-8.89737170400002));
#286584=CARTESIAN_POINT('Ctrl Pts',(-5.36847181900006,11.6,-8.89737170400002));
#286585=CARTESIAN_POINT('Ctrl Pts',(-5.36892364700006,15.2,-8.89833252800001));
#286586=CARTESIAN_POINT('Ctrl Pts',(-5.36892364700006,11.6,-8.89833252800001));
#286587=CARTESIAN_POINT('Ctrl Pts',(-5.36937841200006,15.2,-8.89930209500001));
#286588=CARTESIAN_POINT('Ctrl Pts',(-5.36937841200006,11.6,-8.89930209500001));
#286589=CARTESIAN_POINT('Ctrl Pts',(-5.36983609200006,15.2,-8.90028038900001));
#286590=CARTESIAN_POINT('Ctrl Pts',(-5.36983609200006,11.6,-8.90028038900001));
#286591=CARTESIAN_POINT('Ctrl Pts',(-5.37029665900006,15.2,-8.90126739500002));
#286592=CARTESIAN_POINT('Ctrl Pts',(-5.37029665900006,11.6,-8.90126739500002));
#286593=CARTESIAN_POINT('Ctrl Pts',(-5.37076008700006,15.2,-8.90226309800001));
#286594=CARTESIAN_POINT('Ctrl Pts',(-5.37076008700006,11.6,-8.90226309800001));
#286595=CARTESIAN_POINT('Ctrl Pts',(-5.37122635100006,15.2,-8.90326748100001));
#286596=CARTESIAN_POINT('Ctrl Pts',(-5.37122635100006,11.6,-8.90326748100001));
#286597=CARTESIAN_POINT('Ctrl Pts',(-5.37169542500005,15.2,-8.90428053100001));
#286598=CARTESIAN_POINT('Ctrl Pts',(-5.37169542500005,11.6,-8.90428053100001));
#286599=CARTESIAN_POINT('Ctrl Pts',(-5.37216728300006,15.2,-8.90530223200001));
#286600=CARTESIAN_POINT('Ctrl Pts',(-5.37216728300006,11.6,-8.90530223200001));
#286601=CARTESIAN_POINT('Ctrl Pts',(-5.37264189900006,15.2,-8.90633257000001));
#286602=CARTESIAN_POINT('Ctrl Pts',(-5.37264189900006,11.6,-8.90633257000001));
#286603=CARTESIAN_POINT('Ctrl Pts',(-5.37311925100005,15.2,-8.90737152700002));
#286604=CARTESIAN_POINT('Ctrl Pts',(-5.37311925100005,11.6,-8.90737152700002));
#286605=CARTESIAN_POINT('Ctrl Pts',(-5.37359931100006,15.2,-8.90841909100001));
#286606=CARTESIAN_POINT('Ctrl Pts',(-5.37359931100006,11.6,-8.90841909100001));
#286607=CARTESIAN_POINT('Ctrl Pts',(-5.37408205300006,15.2,-8.90947524700002));
#286608=CARTESIAN_POINT('Ctrl Pts',(-5.37408205300006,11.6,-8.90947524700002));
#286609=CARTESIAN_POINT('Ctrl Pts',(-5.37456745500006,15.2,-8.91053997800002));
#286610=CARTESIAN_POINT('Ctrl Pts',(-5.37456745500006,11.6,-8.91053997800002));
#286611=CARTESIAN_POINT('Ctrl Pts',(-5.37505549100006,15.2,-8.91161327200001));
#286612=CARTESIAN_POINT('Ctrl Pts',(-5.37505549100006,11.6,-8.91161327200001));
#286613=CARTESIAN_POINT('Ctrl Pts',(-5.37554613600006,15.2,-8.91269511100001));
#286614=CARTESIAN_POINT('Ctrl Pts',(-5.37554613600006,11.6,-8.91269511100001));
#286615=CARTESIAN_POINT('Ctrl Pts',(-5.37603936500005,15.2,-8.91378548300001));
#286616=CARTESIAN_POINT('Ctrl Pts',(-5.37603936500005,11.6,-8.91378548300001));
#286617=CARTESIAN_POINT('Ctrl Pts',(-5.37653515500006,15.2,-8.91488437200002));
#286618=CARTESIAN_POINT('Ctrl Pts',(-5.37653515500006,11.6,-8.91488437200002));
#286619=CARTESIAN_POINT('Ctrl Pts',(-5.37703348100006,15.2,-8.91599176500002));
#286620=CARTESIAN_POINT('Ctrl Pts',(-5.37703348100006,11.6,-8.91599176500002));
#286621=CARTESIAN_POINT('Ctrl Pts',(-5.37753431800006,15.2,-8.91710764600001));
#286622=CARTESIAN_POINT('Ctrl Pts',(-5.37753431800006,11.6,-8.91710764600001));
#286623=CARTESIAN_POINT('Ctrl Pts',(-5.37803764200006,15.2,-8.91823200100001));
#286624=CARTESIAN_POINT('Ctrl Pts',(-5.37803764200006,11.6,-8.91823200100001));
#286625=CARTESIAN_POINT('Ctrl Pts',(-5.37854343200006,15.2,-8.91936481500002));
#286626=CARTESIAN_POINT('Ctrl Pts',(-5.37854343200006,11.6,-8.91936481500002));
#286627=CARTESIAN_POINT('Ctrl Pts',(-5.37905166000006,15.2,-8.92050607500002));
#286628=CARTESIAN_POINT('Ctrl Pts',(-5.37905166000006,11.6,-8.92050607500002));
#286629=CARTESIAN_POINT('Ctrl Pts',(-5.37956230500006,15.2,-8.92165576600001));
#286630=CARTESIAN_POINT('Ctrl Pts',(-5.37956230500006,11.6,-8.92165576600001));
#286631=CARTESIAN_POINT('Ctrl Pts',(-5.38007534200006,15.2,-8.92281387300002));
#286632=CARTESIAN_POINT('Ctrl Pts',(-5.38007534200006,11.6,-8.92281387300002));
#286633=CARTESIAN_POINT('Ctrl Pts',(-5.38059074800006,15.2,-8.92398038200002));
#286634=CARTESIAN_POINT('Ctrl Pts',(-5.38059074800006,11.6,-8.92398038200002));
#286635=CARTESIAN_POINT('Ctrl Pts',(-5.38110850100006,15.2,-8.92515528100001));
#286636=CARTESIAN_POINT('Ctrl Pts',(-5.38110850100006,11.6,-8.92515528100001));
#286637=CARTESIAN_POINT('Ctrl Pts',(-5.38162857400006,15.2,-8.92633855400002));
#286638=CARTESIAN_POINT('Ctrl Pts',(-5.38162857400006,11.6,-8.92633855400002));
#286639=CARTESIAN_POINT('Ctrl Pts',(-5.38215094700006,15.2,-8.92753018600001));
#286640=CARTESIAN_POINT('Ctrl Pts',(-5.38215094700006,11.6,-8.92753018600001));
#286641=CARTESIAN_POINT('Ctrl Pts',(-5.38267559700006,15.2,-8.92873016600002));
#286642=CARTESIAN_POINT('Ctrl Pts',(-5.38267559700006,11.6,-8.92873016600002));
#286643=CARTESIAN_POINT('Ctrl Pts',(-5.38320250000006,15.2,-8.92993847700001));
#286644=CARTESIAN_POINT('Ctrl Pts',(-5.38320250000006,11.6,-8.92993847700001));
#286645=CARTESIAN_POINT('Ctrl Pts',(-5.38373163200006,15.2,-8.93115510700002));
#286646=CARTESIAN_POINT('Ctrl Pts',(-5.38373163200006,11.6,-8.93115510700002));
#286647=CARTESIAN_POINT('Ctrl Pts',(-5.38426297200005,15.2,-8.93238004100001));
#286648=CARTESIAN_POINT('Ctrl Pts',(-5.38426297200005,11.6,-8.93238004100001));
#286649=CARTESIAN_POINT('Ctrl Pts',(-5.38479649700006,15.2,-8.93361326700001));
#286650=CARTESIAN_POINT('Ctrl Pts',(-5.38479649700006,11.6,-8.93361326700001));
#286651=CARTESIAN_POINT('Ctrl Pts',(-5.38533218400006,15.2,-8.93485477000001));
#286652=CARTESIAN_POINT('Ctrl Pts',(-5.38533218400006,11.6,-8.93485477000001));
#286653=CARTESIAN_POINT('Ctrl Pts',(-5.38587001200006,15.2,-8.93610453600001));
#286654=CARTESIAN_POINT('Ctrl Pts',(-5.38587001200006,11.6,-8.93610453600001));
#286655=CARTESIAN_POINT('Ctrl Pts',(-5.38640995700006,15.2,-8.93736255200002));
#286656=CARTESIAN_POINT('Ctrl Pts',(-5.38640995700006,11.6,-8.93736255200002));
#286657=CARTESIAN_POINT('Ctrl Pts',(-5.38695199800006,15.2,-8.93862880300002));
#286658=CARTESIAN_POINT('Ctrl Pts',(-5.38695199800006,11.6,-8.93862880300002));
#286659=CARTESIAN_POINT('Ctrl Pts',(-5.38749611100005,15.2,-8.93990327800001));
#286660=CARTESIAN_POINT('Ctrl Pts',(-5.38749611100005,11.6,-8.93990327800001));
#286661=CARTESIAN_POINT('Ctrl Pts',(-5.38804227600005,15.2,-8.94118596000002));
#286662=CARTESIAN_POINT('Ctrl Pts',(-5.38804227600005,11.6,-8.94118596000002));
#286663=CARTESIAN_POINT('Ctrl Pts',(-5.38859046900006,15.2,-8.94247684000002));
#286664=CARTESIAN_POINT('Ctrl Pts',(-5.38859046900006,11.6,-8.94247684000002));
#286665=CARTESIAN_POINT('Ctrl Pts',(-5.38914067100006,15.2,-8.94377590100002));
#286666=CARTESIAN_POINT('Ctrl Pts',(-5.38914067100006,11.6,-8.94377590100002));
#286667=CARTESIAN_POINT('Ctrl Pts',(-5.38969285900006,15.2,-8.94508313100001));
#286668=CARTESIAN_POINT('Ctrl Pts',(-5.38969285900006,11.6,-8.94508313100001));
#286669=CARTESIAN_POINT('Ctrl Pts',(-5.39024701000006,15.2,-8.94639851600001));
#286670=CARTESIAN_POINT('Ctrl Pts',(-5.39024701000006,11.6,-8.94639851600001));
#286671=CARTESIAN_POINT('Ctrl Pts',(-5.39080310300006,15.2,-8.94772204400001));
#286672=CARTESIAN_POINT('Ctrl Pts',(-5.39080310300006,11.6,-8.94772204400001));
#286673=CARTESIAN_POINT('Ctrl Pts',(-5.39136111800006,15.2,-8.94905370100001));
#286674=CARTESIAN_POINT('Ctrl Pts',(-5.39136111800006,11.6,-8.94905370100001));
#286675=CARTESIAN_POINT('Ctrl Pts',(-5.39192103300006,15.2,-8.95039347300001));
#286676=CARTESIAN_POINT('Ctrl Pts',(-5.39192103300006,11.6,-8.95039347300001));
#286677=CARTESIAN_POINT('Ctrl Pts',(-5.39248282700005,15.2,-8.95174134800002));
#286678=CARTESIAN_POINT('Ctrl Pts',(-5.39248282700005,11.6,-8.95174134800002));
#286679=CARTESIAN_POINT('Ctrl Pts',(-5.39304647700006,15.2,-8.95309731200001));
#286680=CARTESIAN_POINT('Ctrl Pts',(-5.39304647700006,11.6,-8.95309731200001));
#286681=CARTESIAN_POINT('Ctrl Pts',(-5.39361196500006,15.2,-8.95446135300002));
#286682=CARTESIAN_POINT('Ctrl Pts',(-5.39361196500006,11.6,-8.95446135300002));
#286683=CARTESIAN_POINT('Ctrl Pts',(-5.39417926700006,15.2,-8.95583345700001));
#286684=CARTESIAN_POINT('Ctrl Pts',(-5.39417926700006,11.6,-8.95583345700001));
#286685=CARTESIAN_POINT('Ctrl Pts',(-5.39474836400006,15.2,-8.95721361200001));
#286686=CARTESIAN_POINT('Ctrl Pts',(-5.39474836400006,11.6,-8.95721361200001));
#286687=CARTESIAN_POINT('Ctrl Pts',(-5.39531923500006,15.2,-8.95860180500001));
#286688=CARTESIAN_POINT('Ctrl Pts',(-5.39531923500006,11.6,-8.95860180500001));
#286689=CARTESIAN_POINT('Ctrl Pts',(-5.39589185800006,15.2,-8.95999802100001));
#286690=CARTESIAN_POINT('Ctrl Pts',(-5.39589185800006,11.6,-8.95999802100001));
#286691=CARTESIAN_POINT('Ctrl Pts',(-5.39646621500006,15.2,-8.96140225000002));
#286692=CARTESIAN_POINT('Ctrl Pts',(-5.39646621500006,11.6,-8.96140225000002));
#286693=CARTESIAN_POINT('Ctrl Pts',(-5.39704228400006,15.2,-8.96281447600002));
#286694=CARTESIAN_POINT('Ctrl Pts',(-5.39704228400006,11.6,-8.96281447600002));
#286695=CARTESIAN_POINT('Ctrl Pts',(-5.39762004300006,15.2,-8.96423469000002));
#286696=CARTESIAN_POINT('Ctrl Pts',(-5.39762004300006,11.6,-8.96423469000002));
#286697=CARTESIAN_POINT('Ctrl Pts',(-5.39819947500006,15.2,-8.96566287700002));
#286698=CARTESIAN_POINT('Ctrl Pts',(-5.39819947500006,11.6,-8.96566287700002));
#286699=CARTESIAN_POINT('Ctrl Pts',(-5.39878055600005,15.2,-8.96709902300002));
#286700=CARTESIAN_POINT('Ctrl Pts',(-5.39878055600005,11.6,-8.96709902300002));
#286701=CARTESIAN_POINT('Ctrl Pts',(-5.39936326900006,15.2,-8.96854312000002));
#286702=CARTESIAN_POINT('Ctrl Pts',(-5.39936326900006,11.6,-8.96854312000002));
#286703=CARTESIAN_POINT('Ctrl Pts',(-5.39994759300006,15.2,-8.96999515000001));
#286704=CARTESIAN_POINT('Ctrl Pts',(-5.39994759300006,11.6,-8.96999515000001));
#286705=CARTESIAN_POINT('Ctrl Pts',(-5.40053350800005,15.2,-8.97145510400001));
#286706=CARTESIAN_POINT('Ctrl Pts',(-5.40053350800005,11.6,-8.97145510400001));
#286707=CARTESIAN_POINT('Ctrl Pts',(-5.40112099300006,15.2,-8.97292296800002));
#286708=CARTESIAN_POINT('Ctrl Pts',(-5.40112099300006,11.6,-8.97292296800002));
#286709=CARTESIAN_POINT('Ctrl Pts',(-5.40171003000006,15.2,-8.97439872800001));
#286710=CARTESIAN_POINT('Ctrl Pts',(-5.40171003000006,11.6,-8.97439872800001));
#286711=CARTESIAN_POINT('Ctrl Pts',(-5.40230059700006,15.2,-8.97588237500001));
#286712=CARTESIAN_POINT('Ctrl Pts',(-5.40230059700006,11.6,-8.97588237500001));
#286713=CARTESIAN_POINT('Ctrl Pts',(-5.40289267700006,15.2,-8.97737389500002));
#286714=CARTESIAN_POINT('Ctrl Pts',(-5.40289267700006,11.6,-8.97737389500002));
#286715=CARTESIAN_POINT('Ctrl Pts',(-5.40348624900005,15.2,-8.97887327500002));
#286716=CARTESIAN_POINT('Ctrl Pts',(-5.40348624900005,11.6,-8.97887327500002));
#286717=CARTESIAN_POINT('Ctrl Pts',(-5.40408129300006,15.2,-8.98038050300002));
#286718=CARTESIAN_POINT('Ctrl Pts',(-5.40408129300006,11.6,-8.98038050300002));
#286719=CARTESIAN_POINT('Ctrl Pts',(-5.40467779100006,15.2,-8.98189556700002));
#286720=CARTESIAN_POINT('Ctrl Pts',(-5.40467779100006,11.6,-8.98189556700002));
#286721=CARTESIAN_POINT('Ctrl Pts',(-5.40527572300006,15.2,-8.98341845500001));
#286722=CARTESIAN_POINT('Ctrl Pts',(-5.40527572300006,11.6,-8.98341845500001));
#286723=CARTESIAN_POINT('Ctrl Pts',(-5.40587507000006,15.2,-8.98494915300001));
#286724=CARTESIAN_POINT('Ctrl Pts',(-5.40587507000006,11.6,-8.98494915300001));
#286725=CARTESIAN_POINT('Ctrl Pts',(-5.40647581300005,15.2,-8.98648765100001));
#286726=CARTESIAN_POINT('Ctrl Pts',(-5.40647581300005,11.6,-8.98648765100001));
#286727=CARTESIAN_POINT('Ctrl Pts',(-5.40707793100006,15.2,-8.98803393600001));
#286728=CARTESIAN_POINT('Ctrl Pts',(-5.40707793100006,11.6,-8.98803393600001));
#286729=CARTESIAN_POINT('Ctrl Pts',(-5.40768140800005,15.2,-8.98958799500001));
#286730=CARTESIAN_POINT('Ctrl Pts',(-5.40768140800005,11.6,-8.98958799500001));
#286731=CARTESIAN_POINT('Ctrl Pts',(-5.40828622400006,15.2,-8.99114981800002));
#286732=CARTESIAN_POINT('Ctrl Pts',(-5.40828622400006,11.6,-8.99114981800002));
#286733=CARTESIAN_POINT('Ctrl Pts',(-5.40889235900006,15.2,-8.99271939000002));
#286734=CARTESIAN_POINT('Ctrl Pts',(-5.40889235900006,11.6,-8.99271939000002));
#286735=CARTESIAN_POINT('Ctrl Pts',(-5.40949979600006,15.2,-8.99429670100002));
#286736=CARTESIAN_POINT('Ctrl Pts',(-5.40949979600006,11.6,-8.99429670100002));
#286737=CARTESIAN_POINT('Ctrl Pts',(-5.41010851400006,15.2,-8.99588173800002));
#286738=CARTESIAN_POINT('Ctrl Pts',(-5.41010851400006,11.6,-8.99588173800002));
#286739=CARTESIAN_POINT('Ctrl Pts',(-5.41071849700006,15.2,-8.99747449100002));
#286740=CARTESIAN_POINT('Ctrl Pts',(-5.41071849700006,11.6,-8.99747449100002));
#286741=CARTESIAN_POINT('Ctrl Pts',(-5.41132972500006,15.2,-8.99907494500002));
#286742=CARTESIAN_POINT('Ctrl Pts',(-5.41132972500006,11.6,-8.99907494500002));
#286743=CARTESIAN_POINT('Ctrl Pts',(-5.41194218100006,15.2,-9.00068309100002));
#286744=CARTESIAN_POINT('Ctrl Pts',(-5.41194218100006,11.6,-9.00068309100002));
#286745=CARTESIAN_POINT('Ctrl Pts',(-5.41255584400006,15.2,-9.00229891600001));
#286746=CARTESIAN_POINT('Ctrl Pts',(-5.41255584400006,11.6,-9.00229891600001));
#286747=CARTESIAN_POINT('Ctrl Pts',(-5.41317069800006,15.2,-9.00392240700001));
#286748=CARTESIAN_POINT('Ctrl Pts',(-5.41317069800006,11.6,-9.00392240700001));
#286749=CARTESIAN_POINT('Ctrl Pts',(-5.41378672400006,15.2,-9.00555355400002));
#286750=CARTESIAN_POINT('Ctrl Pts',(-5.41378672400006,11.6,-9.00555355400002));
#286751=CARTESIAN_POINT('Ctrl Pts',(-5.41440390400005,15.2,-9.00719234400002));
#286752=CARTESIAN_POINT('Ctrl Pts',(-5.41440390400005,11.6,-9.00719234400002));
#286753=CARTESIAN_POINT('Ctrl Pts',(-5.41502222100006,15.2,-9.00883876600002));
#286754=CARTESIAN_POINT('Ctrl Pts',(-5.41502222100006,11.6,-9.00883876600002));
#286755=CARTESIAN_POINT('Ctrl Pts',(-5.41564165400006,15.2,-9.01049280800001));
#286756=CARTESIAN_POINT('Ctrl Pts',(-5.41564165400006,11.6,-9.01049280800001));
#286757=CARTESIAN_POINT('Ctrl Pts',(-5.41626218800006,15.2,-9.01215445900002));
#286758=CARTESIAN_POINT('Ctrl Pts',(-5.41626218800006,11.6,-9.01215445900002));
#286759=CARTESIAN_POINT('Ctrl Pts',(-5.41688380400006,15.2,-9.01382370600002));
#286760=CARTESIAN_POINT('Ctrl Pts',(-5.41688380400006,11.6,-9.01382370600002));
#286761=CARTESIAN_POINT('Ctrl Pts',(-5.41750648400006,15.2,-9.01550053800002));
#286762=CARTESIAN_POINT('Ctrl Pts',(-5.41750648400006,11.6,-9.01550053800002));
#286763=CARTESIAN_POINT('Ctrl Pts',(-5.41813021000006,15.2,-9.01718494400002));
#286764=CARTESIAN_POINT('Ctrl Pts',(-5.41813021000006,11.6,-9.01718494400002));
#286765=CARTESIAN_POINT('Ctrl Pts',(-5.41875496600006,15.2,-9.01887691300002));
#286766=CARTESIAN_POINT('Ctrl Pts',(-5.41875496600006,11.6,-9.01887691300002));
#286767=CARTESIAN_POINT('Ctrl Pts',(-5.41938073300006,15.2,-9.02057643200001));
#286768=CARTESIAN_POINT('Ctrl Pts',(-5.41938073300006,11.6,-9.02057643200001));
#286769=CARTESIAN_POINT('Ctrl Pts',(-5.42000749500006,15.2,-9.02228349000002));
#286770=CARTESIAN_POINT('Ctrl Pts',(-5.42000749500006,11.6,-9.02228349000002));
#286771=CARTESIAN_POINT('Ctrl Pts',(-5.42063523200006,15.2,-9.02399807600002));
#286772=CARTESIAN_POINT('Ctrl Pts',(-5.42063523200006,11.6,-9.02399807600002));
#286773=CARTESIAN_POINT('Ctrl Pts',(-5.42126392900006,15.2,-9.02572017700002));
#286774=CARTESIAN_POINT('Ctrl Pts',(-5.42126392900006,11.6,-9.02572017700002));
#286775=CARTESIAN_POINT('Ctrl Pts',(-5.42189356700006,15.2,-9.02744978400002));
#286776=CARTESIAN_POINT('Ctrl Pts',(-5.42189356700006,11.6,-9.02744978400002));
#286777=CARTESIAN_POINT('Ctrl Pts',(-5.42252413200006,15.2,-9.02918688400002));
#286778=CARTESIAN_POINT('Ctrl Pts',(-5.42252413200006,11.6,-9.02918688400002));
#286779=CARTESIAN_POINT('Ctrl Pts',(-5.42315560300006,15.2,-9.03093146700002));
#286780=CARTESIAN_POINT('Ctrl Pts',(-5.42315560300006,11.6,-9.03093146700002));
#286781=CARTESIAN_POINT('Ctrl Pts',(-5.42378796400006,15.2,-9.03268352000002));
#286782=CARTESIAN_POINT('Ctrl Pts',(-5.42378796400006,11.6,-9.03268352000002));
#286783=CARTESIAN_POINT('Ctrl Pts',(-5.42442119900006,15.2,-9.03444303200001));
#286784=CARTESIAN_POINT('Ctrl Pts',(-5.42442119900006,11.6,-9.03444303200001));
#286785=CARTESIAN_POINT('Ctrl Pts',(-5.42505529100006,15.2,-9.03620999300001));
#286786=CARTESIAN_POINT('Ctrl Pts',(-5.42505529100006,11.6,-9.03620999300001));
#286787=CARTESIAN_POINT('Ctrl Pts',(-5.42569022200006,15.2,-9.03798439200001));
#286788=CARTESIAN_POINT('Ctrl Pts',(-5.42569022200006,11.6,-9.03798439200001));
#286789=CARTESIAN_POINT('Ctrl Pts',(-5.42632597500006,15.2,-9.03976621700001));
#286790=CARTESIAN_POINT('Ctrl Pts',(-5.42632597500006,11.6,-9.03976621700001));
#286791=CARTESIAN_POINT('Ctrl Pts',(-5.42696253600006,15.2,-9.04155545600002));
#286792=CARTESIAN_POINT('Ctrl Pts',(-5.42696253600006,11.6,-9.04155545600002));
#286793=CARTESIAN_POINT('Ctrl Pts',(-5.42759988400006,15.2,-9.04335209900001));
#286794=CARTESIAN_POINT('Ctrl Pts',(-5.42759988400006,11.6,-9.04335209900001));
#286795=CARTESIAN_POINT('Ctrl Pts',(-5.42823800600006,15.2,-9.04515613500001));
#286796=CARTESIAN_POINT('Ctrl Pts',(-5.42823800600006,11.6,-9.04515613500001));
#286797=CARTESIAN_POINT('Ctrl Pts',(-5.42887688500006,15.2,-9.04696755200002));
#286798=CARTESIAN_POINT('Ctrl Pts',(-5.42887688500006,11.6,-9.04696755200002));
#286799=CARTESIAN_POINT('Ctrl Pts',(-5.42951650300005,15.2,-9.04878634000001));
#286800=CARTESIAN_POINT('Ctrl Pts',(-5.42951650300005,11.6,-9.04878634000001));
#286801=CARTESIAN_POINT('Ctrl Pts',(-5.43015684400006,15.2,-9.05061248700001));
#286802=CARTESIAN_POINT('Ctrl Pts',(-5.43015684400006,11.6,-9.05061248700001));
#286803=CARTESIAN_POINT('Ctrl Pts',(-5.43079789200006,15.2,-9.05244598400002));
#286804=CARTESIAN_POINT('Ctrl Pts',(-5.43079789200006,11.6,-9.05244598400002));
#286805=CARTESIAN_POINT('Ctrl Pts',(-5.43143963200006,15.2,-9.05428681700002));
#286806=CARTESIAN_POINT('Ctrl Pts',(-5.43143963200006,11.6,-9.05428681700002));
#286807=CARTESIAN_POINT('Ctrl Pts',(-5.43208204500006,15.2,-9.05613497700001));
#286808=CARTESIAN_POINT('Ctrl Pts',(-5.43208204500006,11.6,-9.05613497700001));
#286809=CARTESIAN_POINT('Ctrl Pts',(-5.43272511700006,15.2,-9.05799045400002));
#286810=CARTESIAN_POINT('Ctrl Pts',(-5.43272511700006,11.6,-9.05799045400002));
#286811=CARTESIAN_POINT('Ctrl Pts',(-5.43336883000006,15.2,-9.05985323500002));
#286812=CARTESIAN_POINT('Ctrl Pts',(-5.43336883000006,11.6,-9.05985323500002));
#286813=CARTESIAN_POINT('Ctrl Pts',(-5.43401316900006,15.2,-9.06172331100001));
#286814=CARTESIAN_POINT('Ctrl Pts',(-5.43401316900006,11.6,-9.06172331100001));
#286815=CARTESIAN_POINT('Ctrl Pts',(-5.43465811900006,15.2,-9.06360066900002));
#286816=CARTESIAN_POINT('Ctrl Pts',(-5.43465811900006,11.6,-9.06360066900002));
#286817=CARTESIAN_POINT('Ctrl Pts',(-5.43530366400006,15.2,-9.06548530000002));
#286818=CARTESIAN_POINT('Ctrl Pts',(-5.43530366400006,11.6,-9.06548530000002));
#286819=CARTESIAN_POINT('Ctrl Pts',(-5.43594978500006,15.2,-9.06737719300001));
#286820=CARTESIAN_POINT('Ctrl Pts',(-5.43594978500006,11.6,-9.06737719300001));
#286821=CARTESIAN_POINT('Ctrl Pts',(-5.43659647000006,15.2,-9.06927633700001));
#286822=CARTESIAN_POINT('Ctrl Pts',(-5.43659647000006,11.6,-9.06927633700001));
#286823=CARTESIAN_POINT('Ctrl Pts',(-5.43724370200006,15.2,-9.07118272100002));
#286824=CARTESIAN_POINT('Ctrl Pts',(-5.43724370200006,11.6,-9.07118272100002));
#286825=CARTESIAN_POINT('Ctrl Pts',(-5.43789146400006,15.2,-9.07309633400001));
#286826=CARTESIAN_POINT('Ctrl Pts',(-5.43789146400006,11.6,-9.07309633400001));
#286827=CARTESIAN_POINT('Ctrl Pts',(-5.43853974200006,15.2,-9.07501716600001));
#286828=CARTESIAN_POINT('Ctrl Pts',(-5.43853974200006,11.6,-9.07501716600001));
#286829=CARTESIAN_POINT('Ctrl Pts',(-5.43918852000006,15.2,-9.07694520700002));
#286830=CARTESIAN_POINT('Ctrl Pts',(-5.43918852000006,11.6,-9.07694520700002));
#286831=CARTESIAN_POINT('Ctrl Pts',(-5.43983778200006,15.2,-9.07888044600002));
#286832=CARTESIAN_POINT('Ctrl Pts',(-5.43983778200006,11.6,-9.07888044600002));
#286833=CARTESIAN_POINT('Ctrl Pts',(-5.44048751200005,15.2,-9.08082287200001));
#286834=CARTESIAN_POINT('Ctrl Pts',(-5.44048751200005,11.6,-9.08082287200001));
#286835=CARTESIAN_POINT('Ctrl Pts',(-5.44113769600005,15.2,-9.08277247400001));
#286836=CARTESIAN_POINT('Ctrl Pts',(-5.44113769600005,11.6,-9.08277247400001));
#286837=CARTESIAN_POINT('Ctrl Pts',(-5.44178831900005,15.2,-9.08472924200002));
#286838=CARTESIAN_POINT('Ctrl Pts',(-5.44178831900005,11.6,-9.08472924200002));
#286839=CARTESIAN_POINT('Ctrl Pts',(-5.44243936400005,15.2,-9.08669316600001));
#286840=CARTESIAN_POINT('Ctrl Pts',(-5.44243936400005,11.6,-9.08669316600001));
#286841=CARTESIAN_POINT('Ctrl Pts',(-5.44309081700006,15.2,-9.08866423400001));
#286842=CARTESIAN_POINT('Ctrl Pts',(-5.44309081700006,11.6,-9.08866423400001));
#286843=CARTESIAN_POINT('Ctrl Pts',(-5.44374266300006,15.2,-9.09064243800002));
#286844=CARTESIAN_POINT('Ctrl Pts',(-5.44374266300006,11.6,-9.09064243800002));
#286845=CARTESIAN_POINT('Ctrl Pts',(-5.44439488400006,15.2,-9.09262776600002));
#286846=CARTESIAN_POINT('Ctrl Pts',(-5.44439488400006,11.6,-9.09262776600002));
#286847=CARTESIAN_POINT('Ctrl Pts',(-5.44504746900006,15.2,-9.09462020700002));
#286848=CARTESIAN_POINT('Ctrl Pts',(-5.44504746900006,11.6,-9.09462020700002));
#286849=CARTESIAN_POINT('Ctrl Pts',(-5.44570040100006,15.2,-9.09661975100001));
#286850=CARTESIAN_POINT('Ctrl Pts',(-5.44570040100006,11.6,-9.09661975100001));
#286851=CARTESIAN_POINT('Ctrl Pts',(-5.44635366500006,15.2,-9.09862638900002));
#286852=CARTESIAN_POINT('Ctrl Pts',(-5.44635366500006,11.6,-9.09862638900002));
#286853=CARTESIAN_POINT('Ctrl Pts',(-5.44700724700006,15.2,-9.10064010900001));
#286854=CARTESIAN_POINT('Ctrl Pts',(-5.44700724700006,11.6,-9.10064010900001));
#286855=CARTESIAN_POINT('Ctrl Pts',(-5.44766113200006,15.2,-9.10266090100002));
#286856=CARTESIAN_POINT('Ctrl Pts',(-5.44766113200006,11.6,-9.10266090100002));
#286857=CARTESIAN_POINT('Ctrl Pts',(-5.44831530400006,15.2,-9.10468875600002));
#286858=CARTESIAN_POINT('Ctrl Pts',(-5.44831530400006,11.6,-9.10468875600002));
#286859=CARTESIAN_POINT('Ctrl Pts',(-5.44896974900006,15.2,-9.10672366200002));
#286860=CARTESIAN_POINT('Ctrl Pts',(-5.44896974900006,11.6,-9.10672366200002));
#286861=CARTESIAN_POINT('Ctrl Pts',(-5.44962445200006,15.2,-9.10876561000002));
#286862=CARTESIAN_POINT('Ctrl Pts',(-5.44962445200006,11.6,-9.10876561000002));
#286863=CARTESIAN_POINT('Ctrl Pts',(-5.45027939900006,15.2,-9.11081458800002));
#286864=CARTESIAN_POINT('Ctrl Pts',(-5.45027939900006,11.6,-9.11081458800002));
#286865=CARTESIAN_POINT('Ctrl Pts',(-5.45093457600006,15.2,-9.11287058900001));
#286866=CARTESIAN_POINT('Ctrl Pts',(-5.45093457600006,11.6,-9.11287058900001));
#286867=CARTESIAN_POINT('Ctrl Pts',(-5.45158996700006,15.2,-9.11493360000001));
#286868=CARTESIAN_POINT('Ctrl Pts',(-5.45158996700006,11.6,-9.11493360000001));
#286869=CARTESIAN_POINT('Ctrl Pts',(-5.45224555800006,15.2,-9.11700361100002));
#286870=CARTESIAN_POINT('Ctrl Pts',(-5.45224555800006,11.6,-9.11700361100002));
#286871=CARTESIAN_POINT('Ctrl Pts',(-5.45290133500006,15.2,-9.11908061300002));
#286872=CARTESIAN_POINT('Ctrl Pts',(-5.45290133500006,11.6,-9.11908061300002));
#286873=CARTESIAN_POINT('Ctrl Pts',(-5.45355728400006,15.2,-9.12116459600002));
#286874=CARTESIAN_POINT('Ctrl Pts',(-5.45355728400006,11.6,-9.12116459600002));
#286875=CARTESIAN_POINT('Ctrl Pts',(-5.45421338900006,15.2,-9.12325554900002));
#286876=CARTESIAN_POINT('Ctrl Pts',(-5.45421338900006,11.6,-9.12325554900002));
#286877=CARTESIAN_POINT('Ctrl Pts',(-5.45486963700006,15.2,-9.12535346200002));
#286878=CARTESIAN_POINT('Ctrl Pts',(-5.45486963700006,11.6,-9.12535346200002));
#286879=CARTESIAN_POINT('Ctrl Pts',(-5.45552601400006,15.2,-9.12745832600002));
#286880=CARTESIAN_POINT('Ctrl Pts',(-5.45552601400006,11.6,-9.12745832600002));
#286881=CARTESIAN_POINT('Ctrl Pts',(-5.45618250500006,15.2,-9.12957013000002));
#286882=CARTESIAN_POINT('Ctrl Pts',(-5.45618250500006,11.6,-9.12957013000002));
#286883=CARTESIAN_POINT('Ctrl Pts',(-5.45683909700006,15.2,-9.13168886400002));
#286884=CARTESIAN_POINT('Ctrl Pts',(-5.45683909700006,11.6,-9.13168886400002));
#286885=CARTESIAN_POINT('Ctrl Pts',(-5.45749577500006,15.2,-9.13381451800002));
#286886=CARTESIAN_POINT('Ctrl Pts',(-5.45749577500006,11.6,-9.13381451800002));
#286887=CARTESIAN_POINT('Ctrl Pts',(-5.45815252500006,15.2,-9.13594708400002));
#286888=CARTESIAN_POINT('Ctrl Pts',(-5.45815252500006,11.6,-9.13594708400002));
#286889=CARTESIAN_POINT('Ctrl Pts',(-5.45880933300006,15.2,-9.13808654900001));
#286890=CARTESIAN_POINT('Ctrl Pts',(-5.45880933300006,11.6,-9.13808654900001));
#286891=CARTESIAN_POINT('Ctrl Pts',(-5.45946618600006,15.2,-9.14023290400002));
#286892=CARTESIAN_POINT('Ctrl Pts',(-5.45946618600006,11.6,-9.14023290400002));
#286893=CARTESIAN_POINT('Ctrl Pts',(-5.46012307000006,15.2,-9.14238614000002));
#286894=CARTESIAN_POINT('Ctrl Pts',(-5.46012307000006,11.6,-9.14238614000002));
#286895=CARTESIAN_POINT('Ctrl Pts',(-5.46077997000006,15.2,-9.14454624700002));
#286896=CARTESIAN_POINT('Ctrl Pts',(-5.46077997000006,11.6,-9.14454624700002));
#286897=CARTESIAN_POINT('Ctrl Pts',(-5.46143687300006,15.2,-9.14671321500002));
#286898=CARTESIAN_POINT('Ctrl Pts',(-5.46143687300006,11.6,-9.14671321500002));
#286899=CARTESIAN_POINT('Ctrl Pts',(-5.46209376500006,15.2,-9.14888703300001));
#286900=CARTESIAN_POINT('Ctrl Pts',(-5.46209376500006,11.6,-9.14888703300001));
#286901=CARTESIAN_POINT('Ctrl Pts',(-5.46275063300006,15.2,-9.15106769300002));
#286902=CARTESIAN_POINT('Ctrl Pts',(-5.46275063300006,11.6,-9.15106769300002));
#286903=CARTESIAN_POINT('Ctrl Pts',(-5.46340746300006,15.2,-9.15325518400002));
#286904=CARTESIAN_POINT('Ctrl Pts',(-5.46340746300006,11.6,-9.15325518400002));
#286905=CARTESIAN_POINT('Ctrl Pts',(-5.46406424000006,15.2,-9.15544949700001));
#286906=CARTESIAN_POINT('Ctrl Pts',(-5.46406424000006,11.6,-9.15544949700001));
#286907=CARTESIAN_POINT('Ctrl Pts',(-5.46472095400006,15.2,-9.15765062100002));
#286908=CARTESIAN_POINT('Ctrl Pts',(-5.46472095400006,11.6,-9.15765062100002));
#286909=CARTESIAN_POINT('Ctrl Pts',(-5.46537758800006,15.2,-9.15985854900002));
#286910=CARTESIAN_POINT('Ctrl Pts',(-5.46537758800006,11.6,-9.15985854900002));
#286911=CARTESIAN_POINT('Ctrl Pts',(-5.46603413000006,15.2,-9.16207326700002));
#286912=CARTESIAN_POINT('Ctrl Pts',(-5.46603413000006,11.6,-9.16207326700002));
#286913=CARTESIAN_POINT('Ctrl Pts',(-5.46669056700006,15.2,-9.16429476900002));
#286914=CARTESIAN_POINT('Ctrl Pts',(-5.46669056700006,11.6,-9.16429476900002));
#286915=CARTESIAN_POINT('Ctrl Pts',(-5.46734688500006,15.2,-9.16652304400002));
#286916=CARTESIAN_POINT('Ctrl Pts',(-5.46734688500006,11.6,-9.16652304400002));
#286917=CARTESIAN_POINT('Ctrl Pts',(-5.46800307000006,15.2,-9.16875808200002));
#286918=CARTESIAN_POINT('Ctrl Pts',(-5.46800307000006,11.6,-9.16875808200002));
#286919=CARTESIAN_POINT('Ctrl Pts',(-5.46865911200006,15.2,-9.17099987400002));
#286920=CARTESIAN_POINT('Ctrl Pts',(-5.46865911200006,11.6,-9.17099987400002));
#286921=CARTESIAN_POINT('Ctrl Pts',(-5.46931499300006,15.2,-9.17324841000001));
#286922=CARTESIAN_POINT('Ctrl Pts',(-5.46931499300006,11.6,-9.17324841000001));
#286923=CARTESIAN_POINT('Ctrl Pts',(-5.46997070400006,15.2,-9.17550368100001));
#286924=CARTESIAN_POINT('Ctrl Pts',(-5.46997070400006,11.6,-9.17550368100001));
#286925=CARTESIAN_POINT('Ctrl Pts',(-5.47062622900006,15.2,-9.17776567700002));
#286926=CARTESIAN_POINT('Ctrl Pts',(-5.47062622900006,11.6,-9.17776567700002));
#286927=CARTESIAN_POINT('Ctrl Pts',(-5.47128155700006,15.2,-9.18003438700002));
#286928=CARTESIAN_POINT('Ctrl Pts',(-5.47128155700006,11.6,-9.18003438700002));
#286929=CARTESIAN_POINT('Ctrl Pts',(-5.47193667400006,15.2,-9.18230980400002));
#286930=CARTESIAN_POINT('Ctrl Pts',(-5.47193667400006,11.6,-9.18230980400002));
#286931=CARTESIAN_POINT('Ctrl Pts',(-5.47259156600005,15.2,-9.18459191700002));
#286932=CARTESIAN_POINT('Ctrl Pts',(-5.47259156600005,11.6,-9.18459191700002));
#286933=CARTESIAN_POINT('Ctrl Pts',(-5.47324622200006,15.2,-9.18688071700002));
#286934=CARTESIAN_POINT('Ctrl Pts',(-5.47324622200006,11.6,-9.18688071700002));
#286935=CARTESIAN_POINT('Ctrl Pts',(-5.47390062900006,15.2,-9.18917619500002));
#286936=CARTESIAN_POINT('Ctrl Pts',(-5.47390062900006,11.6,-9.18917619500002));
#286937=CARTESIAN_POINT('Ctrl Pts',(-5.47455477300006,15.2,-9.19147833900002));
#286938=CARTESIAN_POINT('Ctrl Pts',(-5.47455477300006,11.6,-9.19147833900002));
#286939=CARTESIAN_POINT('Ctrl Pts',(-5.47520864000006,15.2,-9.19378714300001));
#286940=CARTESIAN_POINT('Ctrl Pts',(-5.47520864000006,11.6,-9.19378714300001));
#286941=CARTESIAN_POINT('Ctrl Pts',(-5.47586222100006,15.2,-9.19610259600002));
#286942=CARTESIAN_POINT('Ctrl Pts',(-5.47586222100006,11.6,-9.19610259600002));
#286943=CARTESIAN_POINT('Ctrl Pts',(-5.47651550000006,15.2,-9.19842468800002));
#286944=CARTESIAN_POINT('Ctrl Pts',(-5.47651550000006,11.6,-9.19842468800002));
#286945=CARTESIAN_POINT('Ctrl Pts',(-5.47716846700006,15.2,-9.20075341100001));
#286946=CARTESIAN_POINT('Ctrl Pts',(-5.47716846700006,11.6,-9.20075341100001));
#286947=CARTESIAN_POINT('Ctrl Pts',(-5.47782110600005,15.2,-9.20308875400002));
#286948=CARTESIAN_POINT('Ctrl Pts',(-5.47782110600005,11.6,-9.20308875400002));
#286949=CARTESIAN_POINT('Ctrl Pts',(-5.47847340700006,15.2,-9.20543070800001));
#286950=CARTESIAN_POINT('Ctrl Pts',(-5.47847340700006,11.6,-9.20543070800001));
#286951=CARTESIAN_POINT('Ctrl Pts',(-5.47912535700006,15.2,-9.20777926500002));
#286952=CARTESIAN_POINT('Ctrl Pts',(-5.47912535700006,11.6,-9.20777926500002));
#286953=CARTESIAN_POINT('Ctrl Pts',(-5.47977694300006,15.2,-9.21013441500002));
#286954=CARTESIAN_POINT('Ctrl Pts',(-5.47977694300006,11.6,-9.21013441500002));
#286955=CARTESIAN_POINT('Ctrl Pts',(-5.48042815200006,15.2,-9.21249614700002));
#286956=CARTESIAN_POINT('Ctrl Pts',(-5.48042815200006,11.6,-9.21249614700002));
#286957=CARTESIAN_POINT('Ctrl Pts',(-5.48107897400006,15.2,-9.21486445500001));
#286958=CARTESIAN_POINT('Ctrl Pts',(-5.48107897400006,11.6,-9.21486445500001));
#286959=CARTESIAN_POINT('Ctrl Pts',(-5.48172939300006,15.2,-9.21723932700001));
#286960=CARTESIAN_POINT('Ctrl Pts',(-5.48172939300006,11.6,-9.21723932700001));
#286961=CARTESIAN_POINT('Ctrl Pts',(-5.48237940000006,15.2,-9.21962075500002));
#286962=CARTESIAN_POINT('Ctrl Pts',(-5.48237940000006,11.6,-9.21962075500002));
#286963=CARTESIAN_POINT('Ctrl Pts',(-5.48302898100006,15.2,-9.22200872900002));
#286964=CARTESIAN_POINT('Ctrl Pts',(-5.48302898100006,11.6,-9.22200872900002));
#286965=CARTESIAN_POINT('Ctrl Pts',(-5.48367812400006,15.2,-9.22440324100002));
#286966=CARTESIAN_POINT('Ctrl Pts',(-5.48367812400006,11.6,-9.22440324100002));
#286967=CARTESIAN_POINT('Ctrl Pts',(-5.48432681600006,15.2,-9.22680428100002));
#286968=CARTESIAN_POINT('Ctrl Pts',(-5.48432681600006,11.6,-9.22680428100002));
#286969=CARTESIAN_POINT('Ctrl Pts',(-5.48497504600006,15.2,-9.22921183900002));
#286970=CARTESIAN_POINT('Ctrl Pts',(-5.48497504600006,11.6,-9.22921183900002));
#286971=CARTESIAN_POINT('Ctrl Pts',(-5.48562280200006,15.2,-9.23162590700001));
#286972=CARTESIAN_POINT('Ctrl Pts',(-5.48562280200006,11.6,-9.23162590700001));
#286973=CARTESIAN_POINT('Ctrl Pts',(-5.48627007100006,15.2,-9.23404647600002));
#286974=CARTESIAN_POINT('Ctrl Pts',(-5.48627007100006,11.6,-9.23404647600002));
#286975=CARTESIAN_POINT('Ctrl Pts',(-5.48691684200006,15.2,-9.23647353500002));
#286976=CARTESIAN_POINT('Ctrl Pts',(-5.48691684200006,11.6,-9.23647353500002));
#286977=CARTESIAN_POINT('Ctrl Pts',(-5.48756310200006,15.2,-9.23890707800001));
#286978=CARTESIAN_POINT('Ctrl Pts',(-5.48756310200006,11.6,-9.23890707800001));
#286979=CARTESIAN_POINT('Ctrl Pts',(-5.48820883900006,15.2,-9.24134709400001));
#286980=CARTESIAN_POINT('Ctrl Pts',(-5.48820883900006,11.6,-9.24134709400001));
#286981=CARTESIAN_POINT('Ctrl Pts',(-5.48885404200006,15.2,-9.24379357300002));
#286982=CARTESIAN_POINT('Ctrl Pts',(-5.48885404200006,11.6,-9.24379357300002));
#286983=CARTESIAN_POINT('Ctrl Pts',(-5.48949869800006,15.2,-9.24624650800002));
#286984=CARTESIAN_POINT('Ctrl Pts',(-5.48949869800006,11.6,-9.24624650800002));
#286985=CARTESIAN_POINT('Ctrl Pts',(-5.49014279600006,15.2,-9.24870588900001));
#286986=CARTESIAN_POINT('Ctrl Pts',(-5.49014279600006,11.6,-9.24870588900001));
#286987=CARTESIAN_POINT('Ctrl Pts',(-5.49078632300006,15.2,-9.25117170600002));
#286988=CARTESIAN_POINT('Ctrl Pts',(-5.49078632300006,11.6,-9.25117170600002));
#286989=CARTESIAN_POINT('Ctrl Pts',(-5.49142927000006,15.2,-9.25364395200001));
#286990=CARTESIAN_POINT('Ctrl Pts',(-5.49142927000006,11.6,-9.25364395200001));
#286991=CARTESIAN_POINT('Ctrl Pts',(-5.49207162100006,15.2,-9.25612261600002));
#286992=CARTESIAN_POINT('Ctrl Pts',(-5.49207162100006,11.6,-9.25612261600002));
#286993=CARTESIAN_POINT('Ctrl Pts',(-5.49271336800006,15.2,-9.25860769100002));
#286994=CARTESIAN_POINT('Ctrl Pts',(-5.49271336800006,11.6,-9.25860769100002));
#286995=CARTESIAN_POINT('Ctrl Pts',(-5.49335449800005,15.2,-9.26109916700002));
#286996=CARTESIAN_POINT('Ctrl Pts',(-5.49335449800005,11.6,-9.26109916700002));
#286997=CARTESIAN_POINT('Ctrl Pts',(-5.49399499900006,15.2,-9.26359703400001));
#286998=CARTESIAN_POINT('Ctrl Pts',(-5.49399499900006,11.6,-9.26359703400001));
#286999=CARTESIAN_POINT('Ctrl Pts',(-5.49463485900006,15.2,-9.26610128400002));
#287000=CARTESIAN_POINT('Ctrl Pts',(-5.49463485900006,11.6,-9.26610128400002));
#287001=CARTESIAN_POINT('Ctrl Pts',(-5.49527406800006,15.2,-9.26861190900001));
#287002=CARTESIAN_POINT('Ctrl Pts',(-5.49527406800006,11.6,-9.26861190900001));
#287003=CARTESIAN_POINT('Ctrl Pts',(-5.49591261300006,15.2,-9.27112889800001));
#287004=CARTESIAN_POINT('Ctrl Pts',(-5.49591261300006,11.6,-9.27112889800001));
#287005=CARTESIAN_POINT('Ctrl Pts',(-5.49655048300006,15.2,-9.27365224400001));
#287006=CARTESIAN_POINT('Ctrl Pts',(-5.49655048300006,11.6,-9.27365224400001));
#287007=CARTESIAN_POINT('Ctrl Pts',(-5.49718766700006,15.2,-9.27618193800001));
#287008=CARTESIAN_POINT('Ctrl Pts',(-5.49718766700006,11.6,-9.27618193800001));
#287009=CARTESIAN_POINT('Ctrl Pts',(-5.49782415300006,15.2,-9.27871797000002));
#287010=CARTESIAN_POINT('Ctrl Pts',(-5.49782415300006,11.6,-9.27871797000002));
#287011=CARTESIAN_POINT('Ctrl Pts',(-5.49845993000006,15.2,-9.28126033100002));
#287012=CARTESIAN_POINT('Ctrl Pts',(-5.49845993000006,11.6,-9.28126033100002));
#287013=CARTESIAN_POINT('Ctrl Pts',(-5.49909498700006,15.2,-9.28380901500002));
#287014=CARTESIAN_POINT('Ctrl Pts',(-5.49909498700006,11.6,-9.28380901500002));
#287015=CARTESIAN_POINT('Ctrl Pts',(-5.49972931200006,15.2,-9.28636401000002));
#287016=CARTESIAN_POINT('Ctrl Pts',(-5.49972931200006,11.6,-9.28636401000002));
#287017=CARTESIAN_POINT('Ctrl Pts',(-5.50036289400006,15.2,-9.28892530800002));
#287018=CARTESIAN_POINT('Ctrl Pts',(-5.50036289400006,11.6,-9.28892530800002));
#287019=CARTESIAN_POINT('Ctrl Pts',(-5.50099572200006,15.2,-9.29149290000002));
#287020=CARTESIAN_POINT('Ctrl Pts',(-5.50099572200006,11.6,-9.29149290000002));
#287021=CARTESIAN_POINT('Ctrl Pts',(-5.50162778400006,15.2,-9.29406678000002));
#287022=CARTESIAN_POINT('Ctrl Pts',(-5.50162778400006,11.6,-9.29406678000002));
#287023=CARTESIAN_POINT('Ctrl Pts',(-5.50225906900006,15.2,-9.29664693400002));
#287024=CARTESIAN_POINT('Ctrl Pts',(-5.50225906900006,11.6,-9.29664693400002));
#287025=CARTESIAN_POINT('Ctrl Pts',(-5.50288956700006,15.2,-9.29923335800002));
#287026=CARTESIAN_POINT('Ctrl Pts',(-5.50288956700006,11.6,-9.29923335800002));
#287027=CARTESIAN_POINT('Ctrl Pts',(-5.50351926700006,15.2,-9.30182604100001));
#287028=CARTESIAN_POINT('Ctrl Pts',(-5.50351926700006,11.6,-9.30182604100001));
#287029=CARTESIAN_POINT('Ctrl Pts',(-5.50414815600006,15.2,-9.30442497500002));
#287030=CARTESIAN_POINT('Ctrl Pts',(-5.50414815600006,11.6,-9.30442497500002));
#287031=CARTESIAN_POINT('Ctrl Pts',(-5.50477622400006,15.2,-9.30703015100002));
#287032=CARTESIAN_POINT('Ctrl Pts',(-5.50477622400006,11.6,-9.30703015100002));
#287033=CARTESIAN_POINT('Ctrl Pts',(-5.50540346100005,15.2,-9.30964156000002));
#287034=CARTESIAN_POINT('Ctrl Pts',(-5.50540346100005,11.6,-9.30964156000002));
#287035=CARTESIAN_POINT('Ctrl Pts',(-5.50602985400006,15.2,-9.31225919400001));
#287036=CARTESIAN_POINT('Ctrl Pts',(-5.50602985400006,11.6,-9.31225919400001));
#287037=CARTESIAN_POINT('Ctrl Pts',(-5.50665539400006,15.2,-9.31488304500002));
#287038=CARTESIAN_POINT('Ctrl Pts',(-5.50665539400006,11.6,-9.31488304500002));
#287039=CARTESIAN_POINT('Ctrl Pts',(-5.50728006900005,15.2,-9.31751310200001));
#287040=CARTESIAN_POINT('Ctrl Pts',(-5.50728006900005,11.6,-9.31751310200001));
#287041=CARTESIAN_POINT('Ctrl Pts',(-5.50790386900006,15.2,-9.32014935900002));
#287042=CARTESIAN_POINT('Ctrl Pts',(-5.50790386900006,11.6,-9.32014935900002));
#287043=CARTESIAN_POINT('Ctrl Pts',(-5.50852678200005,15.2,-9.32279180500002));
#287044=CARTESIAN_POINT('Ctrl Pts',(-5.50852678200005,11.6,-9.32279180500002));
#287045=CARTESIAN_POINT('Ctrl Pts',(-5.50914879900006,15.2,-9.32544043300001));
#287046=CARTESIAN_POINT('Ctrl Pts',(-5.50914879900006,11.6,-9.32544043300001));
#287047=CARTESIAN_POINT('Ctrl Pts',(-5.50976990800006,15.2,-9.32809523400002));
#287048=CARTESIAN_POINT('Ctrl Pts',(-5.50976990800006,11.6,-9.32809523400002));
#287049=CARTESIAN_POINT('Ctrl Pts',(-5.51039009700006,15.2,-9.33075620000002));
#287050=CARTESIAN_POINT('Ctrl Pts',(-5.51039009700006,11.6,-9.33075620000002));
#287051=CARTESIAN_POINT('Ctrl Pts',(-5.51100935800005,15.2,-9.33342332100001));
#287052=CARTESIAN_POINT('Ctrl Pts',(-5.51100935800005,11.6,-9.33342332100001));
#287053=CARTESIAN_POINT('Ctrl Pts',(-5.51162767900006,15.2,-9.33609659000001));
#287054=CARTESIAN_POINT('Ctrl Pts',(-5.51162767900006,11.6,-9.33609659000001));
#287055=CARTESIAN_POINT('Ctrl Pts',(-5.51224505000006,15.2,-9.33877599700002));
#287056=CARTESIAN_POINT('Ctrl Pts',(-5.51224505000006,11.6,-9.33877599700002));
#287057=CARTESIAN_POINT('Ctrl Pts',(-5.51286145900006,15.2,-9.34146153400001));
#287058=CARTESIAN_POINT('Ctrl Pts',(-5.51286145900006,11.6,-9.34146153400001));
#287059=CARTESIAN_POINT('Ctrl Pts',(-5.51347689600005,15.2,-9.34415319400001));
#287060=CARTESIAN_POINT('Ctrl Pts',(-5.51347689600005,11.6,-9.34415319400001));
#287061=CARTESIAN_POINT('Ctrl Pts',(-5.51409135300006,15.2,-9.34685096600001));
#287062=CARTESIAN_POINT('Ctrl Pts',(-5.51409135300006,11.6,-9.34685096600001));
#287063=CARTESIAN_POINT('Ctrl Pts',(-5.51470481600006,15.2,-9.34955484400002));
#287064=CARTESIAN_POINT('Ctrl Pts',(-5.51470481600006,11.6,-9.34955484400002));
#287065=CARTESIAN_POINT('Ctrl Pts',(-5.51531727600006,15.2,-9.35226481800001));
#287066=CARTESIAN_POINT('Ctrl Pts',(-5.51531727600006,11.6,-9.35226481800001));
#287067=CARTESIAN_POINT('Ctrl Pts',(-5.51592872200006,15.2,-9.35498087900001));
#287068=CARTESIAN_POINT('Ctrl Pts',(-5.51592872200006,11.6,-9.35498087900001));
#287069=CARTESIAN_POINT('Ctrl Pts',(-5.51653914500006,15.2,-9.35770301900002));
#287070=CARTESIAN_POINT('Ctrl Pts',(-5.51653914500006,11.6,-9.35770301900002));
#287071=CARTESIAN_POINT('Ctrl Pts',(-5.51714853300005,15.2,-9.36043123200001));
#287072=CARTESIAN_POINT('Ctrl Pts',(-5.51714853300005,11.6,-9.36043123200001));
#287073=CARTESIAN_POINT('Ctrl Pts',(-5.51775687700006,15.2,-9.36316550500001));
#287074=CARTESIAN_POINT('Ctrl Pts',(-5.51775687700006,11.6,-9.36316550500001));
#287075=CARTESIAN_POINT('Ctrl Pts',(-5.51836416700006,15.2,-9.36590583500001));
#287076=CARTESIAN_POINT('Ctrl Pts',(-5.51836416700006,11.6,-9.36590583500001));
#287077=CARTESIAN_POINT('Ctrl Pts',(-5.51897039000006,15.2,-9.36865220900001));
#287078=CARTESIAN_POINT('Ctrl Pts',(-5.51897039000006,11.6,-9.36865220900001));
#287079=CARTESIAN_POINT('Ctrl Pts',(-5.51957553900006,15.2,-9.37140462000002));
#287080=CARTESIAN_POINT('Ctrl Pts',(-5.51957553900006,11.6,-9.37140462000002));
#287081=CARTESIAN_POINT('Ctrl Pts',(-5.52017960200006,15.2,-9.37416306100002));
#287082=CARTESIAN_POINT('Ctrl Pts',(-5.52017960200006,11.6,-9.37416306100002));
#287083=CARTESIAN_POINT('Ctrl Pts',(-5.52078257000006,15.2,-9.37692752200002));
#287084=CARTESIAN_POINT('Ctrl Pts',(-5.52078257000006,11.6,-9.37692752200002));
#287085=CARTESIAN_POINT('Ctrl Pts',(-5.52138443200006,15.2,-9.37969799600002));
#287086=CARTESIAN_POINT('Ctrl Pts',(-5.52138443200006,11.6,-9.37969799600002));
#287087=CARTESIAN_POINT('Ctrl Pts',(-5.52198517700006,15.2,-9.38247447400002));
#287088=CARTESIAN_POINT('Ctrl Pts',(-5.52198517700006,11.6,-9.38247447400002));
#287089=CARTESIAN_POINT('Ctrl Pts',(-5.52258479700006,15.2,-9.38525694700001));
#287090=CARTESIAN_POINT('Ctrl Pts',(-5.52258479700006,11.6,-9.38525694700001));
#287091=CARTESIAN_POINT('Ctrl Pts',(-5.52318328100006,15.2,-9.38804540800002));
#287092=CARTESIAN_POINT('Ctrl Pts',(-5.52318328100006,11.6,-9.38804540800002));
#287093=CARTESIAN_POINT('Ctrl Pts',(-5.52378061800006,15.2,-9.39083984800002));
#287094=CARTESIAN_POINT('Ctrl Pts',(-5.52378061800006,11.6,-9.39083984800002));
#287095=CARTESIAN_POINT('Ctrl Pts',(-5.52437679900006,15.2,-9.39364025800002));
#287096=CARTESIAN_POINT('Ctrl Pts',(-5.52437679900006,11.6,-9.39364025800002));
#287097=CARTESIAN_POINT('Ctrl Pts',(-5.52497181400006,15.2,-9.39644663300001));
#287098=CARTESIAN_POINT('Ctrl Pts',(-5.52497181400006,11.6,-9.39644663300001));
#287099=CARTESIAN_POINT('Ctrl Pts',(-5.52556565400006,15.2,-9.39925896000002));
#287100=CARTESIAN_POINT('Ctrl Pts',(-5.52556565400006,11.6,-9.39925896000002));
#287101=CARTESIAN_POINT('Ctrl Pts',(-5.52615830800006,15.2,-9.40207723400002));
#287102=CARTESIAN_POINT('Ctrl Pts',(-5.52615830800006,11.6,-9.40207723400002));
#287103=CARTESIAN_POINT('Ctrl Pts',(-5.52674976600006,15.2,-9.40490144500002));
#287104=CARTESIAN_POINT('Ctrl Pts',(-5.52674976600006,11.6,-9.40490144500002));
#287105=CARTESIAN_POINT('Ctrl Pts',(-5.52734001800006,15.2,-9.40773158700001));
#287106=CARTESIAN_POINT('Ctrl Pts',(-5.52734001800006,11.6,-9.40773158700001));
#287107=CARTESIAN_POINT('Ctrl Pts',(-5.52792905500006,15.2,-9.41056764900001));
#287108=CARTESIAN_POINT('Ctrl Pts',(-5.52792905500006,11.6,-9.41056764900001));
#287109=CARTESIAN_POINT('Ctrl Pts',(-5.52851686600006,15.2,-9.41340962500002));
#287110=CARTESIAN_POINT('Ctrl Pts',(-5.52851686600006,11.6,-9.41340962500002));
#287111=CARTESIAN_POINT('Ctrl Pts',(-5.52910344300006,15.2,-9.41625750600002));
#287112=CARTESIAN_POINT('Ctrl Pts',(-5.52910344300006,11.6,-9.41625750600002));
#287113=CARTESIAN_POINT('Ctrl Pts',(-5.52968877600006,15.2,-9.41911128400001));
#287114=CARTESIAN_POINT('Ctrl Pts',(-5.52968877600006,11.6,-9.41911128400001));
#287115=CARTESIAN_POINT('Ctrl Pts',(-5.53027285400006,15.2,-9.42197095100001));
#287116=CARTESIAN_POINT('Ctrl Pts',(-5.53027285400006,11.6,-9.42197095100001));
#287117=CARTESIAN_POINT('Ctrl Pts',(-5.53085566800006,15.2,-9.42483649900002));
#287118=CARTESIAN_POINT('Ctrl Pts',(-5.53085566800006,11.6,-9.42483649900002));
#287119=CARTESIAN_POINT('Ctrl Pts',(-5.53143720800006,15.2,-9.42770791800001));
#287120=CARTESIAN_POINT('Ctrl Pts',(-5.53143720800006,11.6,-9.42770791800001));
#287121=CARTESIAN_POINT('Ctrl Pts',(-5.53201746600006,15.2,-9.43058520200001));
#287122=CARTESIAN_POINT('Ctrl Pts',(-5.53201746600006,11.6,-9.43058520200001));
#287123=CARTESIAN_POINT('Ctrl Pts',(-5.53259643100006,15.2,-9.43346834200002));
#287124=CARTESIAN_POINT('Ctrl Pts',(-5.53259643100006,11.6,-9.43346834200002));
#287125=CARTESIAN_POINT('Ctrl Pts',(-5.53317409300006,15.2,-9.43635733100002));
#287126=CARTESIAN_POINT('Ctrl Pts',(-5.53317409300006,11.6,-9.43635733100002));
#287127=CARTESIAN_POINT('Ctrl Pts',(-5.53375044300005,15.2,-9.43925216000002));
#287128=CARTESIAN_POINT('Ctrl Pts',(-5.53375044300005,11.6,-9.43925216000002));
#287129=CARTESIAN_POINT('Ctrl Pts',(-5.53432547200006,15.2,-9.44215282000001));
#287130=CARTESIAN_POINT('Ctrl Pts',(-5.53432547200006,11.6,-9.44215282000001));
#287131=CARTESIAN_POINT('Ctrl Pts',(-5.53489917000006,15.2,-9.44505930400002));
#287132=CARTESIAN_POINT('Ctrl Pts',(-5.53489917000006,11.6,-9.44505930400002));
#287133=CARTESIAN_POINT('Ctrl Pts',(-5.53547152800006,15.2,-9.44797160400002));
#287134=CARTESIAN_POINT('Ctrl Pts',(-5.53547152800006,11.6,-9.44797160400002));
#287135=CARTESIAN_POINT('Ctrl Pts',(-5.53604253700006,15.2,-9.45088971200001));
#287136=CARTESIAN_POINT('Ctrl Pts',(-5.53604253700006,11.6,-9.45088971200001));
#287137=CARTESIAN_POINT('Ctrl Pts',(-5.53661218600006,15.2,-9.45381362000001));
#287138=CARTESIAN_POINT('Ctrl Pts',(-5.53661218600006,11.6,-9.45381362000001));
#287139=CARTESIAN_POINT('Ctrl Pts',(-5.53718046800006,15.2,-9.45674332000002));
#287140=CARTESIAN_POINT('Ctrl Pts',(-5.53718046800006,11.6,-9.45674332000002));
#287141=CARTESIAN_POINT('Ctrl Pts',(-5.53774737000006,15.2,-9.45967880400002));
#287142=CARTESIAN_POINT('Ctrl Pts',(-5.53774737000006,11.6,-9.45967880400002));
#287143=CARTESIAN_POINT('Ctrl Pts',(-5.53831288800006,15.2,-9.46262006300002));
#287144=CARTESIAN_POINT('Ctrl Pts',(-5.53831288800006,11.6,-9.46262006300002));
#287145=CARTESIAN_POINT('Ctrl Pts',(-5.53887700700006,15.2,-9.46556709000001));
#287146=CARTESIAN_POINT('Ctrl Pts',(-5.53887700700006,11.6,-9.46556709000001));
#287147=CARTESIAN_POINT('Ctrl Pts',(-5.53943972200006,15.2,-9.46851987700001));
#287148=CARTESIAN_POINT('Ctrl Pts',(-5.53943972200006,11.6,-9.46851987700001));
#287149=CARTESIAN_POINT('Ctrl Pts',(-5.54000102100006,15.2,-9.47147841500002));
#287150=CARTESIAN_POINT('Ctrl Pts',(-5.54000102100006,11.6,-9.47147841500002));
#287151=CARTESIAN_POINT('Ctrl Pts',(-5.54056089800006,15.2,-9.47444269800001));
#287152=CARTESIAN_POINT('Ctrl Pts',(-5.54056089800006,11.6,-9.47444269800001));
#287153=CARTESIAN_POINT('Ctrl Pts',(-5.54111934100006,15.2,-9.47741271600002));
#287154=CARTESIAN_POINT('Ctrl Pts',(-5.54111934100006,11.6,-9.47741271600002));
#287155=CARTESIAN_POINT('Ctrl Pts',(-5.54167634100006,15.2,-9.48038846300001));
#287156=CARTESIAN_POINT('Ctrl Pts',(-5.54167634100006,11.6,-9.48038846300001));
#287157=CARTESIAN_POINT('Ctrl Pts',(-5.54223189100005,15.2,-9.48336993000002));
#287158=CARTESIAN_POINT('Ctrl Pts',(-5.54223189100005,11.6,-9.48336993000002));
#287159=CARTESIAN_POINT('Ctrl Pts',(-5.54278597900006,15.2,-9.48635710900002));
#287160=CARTESIAN_POINT('Ctrl Pts',(-5.54278597900006,11.6,-9.48635710900002));
#287161=CARTESIAN_POINT('Ctrl Pts',(-5.54333859900006,15.2,-9.48934999200001));
#287162=CARTESIAN_POINT('Ctrl Pts',(-5.54333859900006,11.6,-9.48934999200001));
#287163=CARTESIAN_POINT('Ctrl Pts',(-5.54388974000006,15.2,-9.49234857200001));
#287164=CARTESIAN_POINT('Ctrl Pts',(-5.54388974000006,11.6,-9.49234857200001));
#287165=CARTESIAN_POINT('Ctrl Pts',(-5.54443939300006,15.2,-9.49535284000002));
#287166=CARTESIAN_POINT('Ctrl Pts',(-5.54443939300006,11.6,-9.49535284000002));
#287167=CARTESIAN_POINT('Ctrl Pts',(-5.54498755000006,15.2,-9.49836278900002));
#287168=CARTESIAN_POINT('Ctrl Pts',(-5.54498755000006,11.6,-9.49836278900002));
#287169=CARTESIAN_POINT('Ctrl Pts',(-5.54553420100006,15.2,-9.50137841100002));
#287170=CARTESIAN_POINT('Ctrl Pts',(-5.54553420100006,11.6,-9.50137841100002));
#287171=CARTESIAN_POINT('Ctrl Pts',(-5.54607933800006,15.2,-9.50439969700002));
#287172=CARTESIAN_POINT('Ctrl Pts',(-5.54607933800006,11.6,-9.50439969700002));
#287173=CARTESIAN_POINT('Ctrl Pts',(-5.54662295300006,15.2,-9.50742664100002));
#287174=CARTESIAN_POINT('Ctrl Pts',(-5.54662295300006,11.6,-9.50742664100002));
#287175=CARTESIAN_POINT('Ctrl Pts',(-5.54716503400006,15.2,-9.51045923400001));
#287176=CARTESIAN_POINT('Ctrl Pts',(-5.54716503400006,11.6,-9.51045923400001));
#287177=CARTESIAN_POINT('Ctrl Pts',(-5.54770557400006,15.2,-9.51349746900001));
#287178=CARTESIAN_POINT('Ctrl Pts',(-5.54770557400006,11.6,-9.51349746900001));
#287179=CARTESIAN_POINT('Ctrl Pts',(-5.54824456500006,15.2,-9.51654133600002));
#287180=CARTESIAN_POINT('Ctrl Pts',(-5.54824456500006,11.6,-9.51654133600002));
#287181=CARTESIAN_POINT('Ctrl Pts',(-5.54878199800006,15.2,-9.51959083100002));
#287182=CARTESIAN_POINT('Ctrl Pts',(-5.54878199800006,11.6,-9.51959083100002));
#287183=CARTESIAN_POINT('Ctrl Pts',(-5.54931786200005,15.2,-9.52264594300001));
#287184=CARTESIAN_POINT('Ctrl Pts',(-5.54931786200005,11.6,-9.52264594300001));
#287185=CARTESIAN_POINT('Ctrl Pts',(-5.54985215100006,15.2,-9.52570666600002));
#287186=CARTESIAN_POINT('Ctrl Pts',(-5.54985215100006,11.6,-9.52570666600002));
#287187=CARTESIAN_POINT('Ctrl Pts',(-5.55038485500006,15.2,-9.52877299000002));
#287188=CARTESIAN_POINT('Ctrl Pts',(-5.55038485500006,11.6,-9.52877299000002));
#287189=CARTESIAN_POINT('Ctrl Pts',(-5.55091596500006,15.2,-9.53184491000002));
#287190=CARTESIAN_POINT('Ctrl Pts',(-5.55091596500006,11.6,-9.53184491000002));
#287191=CARTESIAN_POINT('Ctrl Pts',(-5.55144547200006,15.2,-9.53492241800001));
#287192=CARTESIAN_POINT('Ctrl Pts',(-5.55144547200006,11.6,-9.53492241800001));
#287193=CARTESIAN_POINT('Ctrl Pts',(-5.55197337000005,15.2,-9.53800550400001));
#287194=CARTESIAN_POINT('Ctrl Pts',(-5.55197337000005,11.6,-9.53800550400001));
#287195=CARTESIAN_POINT('Ctrl Pts',(-5.55249964700006,15.2,-9.54109416100002));
#287196=CARTESIAN_POINT('Ctrl Pts',(-5.55249964700006,11.6,-9.54109416100002));
#287197=CARTESIAN_POINT('Ctrl Pts',(-5.55302429700006,15.2,-9.54418838400001));
#287198=CARTESIAN_POINT('Ctrl Pts',(-5.55302429700006,11.6,-9.54418838400001));
#287199=CARTESIAN_POINT('Ctrl Pts',(-5.55354730900006,15.2,-9.54728816200002));
#287200=CARTESIAN_POINT('Ctrl Pts',(-5.55354730900006,11.6,-9.54728816200002));
#287201=CARTESIAN_POINT('Ctrl Pts',(-5.55406867700006,15.2,-9.55039348800002));
#287202=CARTESIAN_POINT('Ctrl Pts',(-5.55406867700006,11.6,-9.55039348800002));
#287203=CARTESIAN_POINT('Ctrl Pts',(-5.55458839100006,15.2,-9.55350435500002));
#287204=CARTESIAN_POINT('Ctrl Pts',(-5.55458839100006,11.6,-9.55350435500002));
#287205=CARTESIAN_POINT('Ctrl Pts',(-5.55510644200006,15.2,-9.55662075600002));
#287206=CARTESIAN_POINT('Ctrl Pts',(-5.55510644200006,11.6,-9.55662075600002));
#287207=CARTESIAN_POINT('Ctrl Pts',(-5.55562282200006,15.2,-9.55974268200002));
#287208=CARTESIAN_POINT('Ctrl Pts',(-5.55562282200006,11.6,-9.55974268200002));
#287209=CARTESIAN_POINT('Ctrl Pts',(-5.55613752400006,15.2,-9.56287012600002));
#287210=CARTESIAN_POINT('Ctrl Pts',(-5.55613752400006,11.6,-9.56287012600002));
#287211=CARTESIAN_POINT('Ctrl Pts',(-5.55665053700006,15.2,-9.56600308000001));
#287212=CARTESIAN_POINT('Ctrl Pts',(-5.55665053700006,11.6,-9.56600308000001));
#287213=CARTESIAN_POINT('Ctrl Pts',(-5.55716185500006,15.2,-9.56914153600002));
#287214=CARTESIAN_POINT('Ctrl Pts',(-5.55716185500006,11.6,-9.56914153600002));
#287215=CARTESIAN_POINT('Ctrl Pts',(-5.55767146700005,15.2,-9.57228548700002));
#287216=CARTESIAN_POINT('Ctrl Pts',(-5.55767146700005,11.6,-9.57228548700002));
#287217=CARTESIAN_POINT('Ctrl Pts',(-5.55817936700006,15.2,-9.57543492600001));
#287218=CARTESIAN_POINT('Ctrl Pts',(-5.55817936700006,11.6,-9.57543492600001));
#287219=CARTESIAN_POINT('Ctrl Pts',(-5.55868554700006,15.2,-9.57858984400002));
#287220=CARTESIAN_POINT('Ctrl Pts',(-5.55868554700006,11.6,-9.57858984400002));
#287221=CARTESIAN_POINT('Ctrl Pts',(-5.55918999600006,15.2,-9.58175023500001));
#287222=CARTESIAN_POINT('Ctrl Pts',(-5.55918999600006,11.6,-9.58175023500001));
#287223=CARTESIAN_POINT('Ctrl Pts',(-5.55969270800006,15.2,-9.58491608900001));
#287224=CARTESIAN_POINT('Ctrl Pts',(-5.55969270800006,11.6,-9.58491608900001));
#287225=CARTESIAN_POINT('Ctrl Pts',(-5.56019367400006,15.2,-9.58808740000002));
#287226=CARTESIAN_POINT('Ctrl Pts',(-5.56019367400006,11.6,-9.58808740000002));
#287227=CARTESIAN_POINT('Ctrl Pts',(-5.56069288500006,15.2,-9.59126416200002));
#287228=CARTESIAN_POINT('Ctrl Pts',(-5.56069288500006,11.6,-9.59126416200002));
#287229=CARTESIAN_POINT('Ctrl Pts',(-5.56119033400006,15.2,-9.59444636500002));
#287230=CARTESIAN_POINT('Ctrl Pts',(-5.56119033400006,11.6,-9.59444636500002));
#287231=CARTESIAN_POINT('Ctrl Pts',(-5.56168601200006,15.2,-9.59763400200002));
#287232=CARTESIAN_POINT('Ctrl Pts',(-5.56168601200006,11.6,-9.59763400200002));
#287233=CARTESIAN_POINT('Ctrl Pts',(-5.56217991100006,15.2,-9.60082706600002));
#287234=CARTESIAN_POINT('Ctrl Pts',(-5.56217991100006,11.6,-9.60082706600002));
#287235=CARTESIAN_POINT('Ctrl Pts',(-5.56267202400006,15.2,-9.60402554800002));
#287236=CARTESIAN_POINT('Ctrl Pts',(-5.56267202400006,11.6,-9.60402554800002));
#287237=CARTESIAN_POINT('Ctrl Pts',(-5.56316234000006,15.2,-9.60722944300001));
#287238=CARTESIAN_POINT('Ctrl Pts',(-5.56316234000006,11.6,-9.60722944300001));
#287239=CARTESIAN_POINT('Ctrl Pts',(-5.56365085400006,15.2,-9.61043874100002));
#287240=CARTESIAN_POINT('Ctrl Pts',(-5.56365085400006,11.6,-9.61043874100002));
#287241=CARTESIAN_POINT('Ctrl Pts',(-5.56413755700006,15.2,-9.61365343600002));
#287242=CARTESIAN_POINT('Ctrl Pts',(-5.56413755700006,11.6,-9.61365343600002));
#287243=CARTESIAN_POINT('Ctrl Pts',(-5.56462243900006,15.2,-9.61687352000002));
#287244=CARTESIAN_POINT('Ctrl Pts',(-5.56462243900006,11.6,-9.61687352000002));
#287245=CARTESIAN_POINT('Ctrl Pts',(-5.56510549500006,15.2,-9.62009898500002));
#287246=CARTESIAN_POINT('Ctrl Pts',(-5.56510549500006,11.6,-9.62009898500002));
#287247=CARTESIAN_POINT('Ctrl Pts',(-5.56558671400006,15.2,-9.62332982500002));
#287248=CARTESIAN_POINT('Ctrl Pts',(-5.56558671400006,11.6,-9.62332982500002));
#287249=CARTESIAN_POINT('Ctrl Pts',(-5.56606609100006,15.2,-9.62656603200001));
#287250=CARTESIAN_POINT('Ctrl Pts',(-5.56606609100006,11.6,-9.62656603200001));
#287251=CARTESIAN_POINT('Ctrl Pts',(-5.56654361600006,15.2,-9.62980759800002));
#287252=CARTESIAN_POINT('Ctrl Pts',(-5.56654361600006,11.6,-9.62980759800002));
#287253=CARTESIAN_POINT('Ctrl Pts',(-5.56701928100006,15.2,-9.63305451500002));
#287254=CARTESIAN_POINT('Ctrl Pts',(-5.56701928100006,11.6,-9.63305451500002));
#287255=CARTESIAN_POINT('Ctrl Pts',(-5.56749308000006,15.2,-9.63630677700002));
#287256=CARTESIAN_POINT('Ctrl Pts',(-5.56749308000006,11.6,-9.63630677700002));
#287257=CARTESIAN_POINT('Ctrl Pts',(-5.56796500300006,15.2,-9.63956437500002));
#287258=CARTESIAN_POINT('Ctrl Pts',(-5.56796500300006,11.6,-9.63956437500002));
#287259=CARTESIAN_POINT('Ctrl Pts',(-5.56843504200006,15.2,-9.64282730200001));
#287260=CARTESIAN_POINT('Ctrl Pts',(-5.56843504200006,11.6,-9.64282730200001));
#287261=CARTESIAN_POINT('Ctrl Pts',(-5.56890319100006,15.2,-9.64609555300001));
#287262=CARTESIAN_POINT('Ctrl Pts',(-5.56890319100006,11.6,-9.64609555300001));
#287263=CARTESIAN_POINT('Ctrl Pts',(-5.56936944100006,15.2,-9.64936911600002));
#287264=CARTESIAN_POINT('Ctrl Pts',(-5.56936944100006,11.6,-9.64936911600002));
#287265=CARTESIAN_POINT('Ctrl Pts',(-5.56983378400006,15.2,-9.65264798800001));
#287266=CARTESIAN_POINT('Ctrl Pts',(-5.56983378400006,11.6,-9.65264798800001));
#287267=CARTESIAN_POINT('Ctrl Pts',(-5.57029621300006,15.2,-9.65593215900001));
#287268=CARTESIAN_POINT('Ctrl Pts',(-5.57029621300006,11.6,-9.65593215900001));
#287269=CARTESIAN_POINT('Ctrl Pts',(-5.57075671900006,15.2,-9.65922162300001));
#287270=CARTESIAN_POINT('Ctrl Pts',(-5.57075671900006,11.6,-9.65922162300001));
#287271=CARTESIAN_POINT('Ctrl Pts',(-5.57121529500006,15.2,-9.66251637100001));
#287272=CARTESIAN_POINT('Ctrl Pts',(-5.57121529500006,11.6,-9.66251637100001));
#287273=CARTESIAN_POINT('Ctrl Pts',(-5.57167193400006,15.2,-9.66581639800001));
#287274=CARTESIAN_POINT('Ctrl Pts',(-5.57167193400006,11.6,-9.66581639800001));
#287275=CARTESIAN_POINT('Ctrl Pts',(-5.57212662700006,15.2,-9.66912169500001));
#287276=CARTESIAN_POINT('Ctrl Pts',(-5.57212662700006,11.6,-9.66912169500001));
#287277=CARTESIAN_POINT('Ctrl Pts',(-5.57257936700006,15.2,-9.67243225400001));
#287278=CARTESIAN_POINT('Ctrl Pts',(-5.57257936700006,11.6,-9.67243225400001));
#287279=CARTESIAN_POINT('Ctrl Pts',(-5.57303014600006,15.2,-9.67574807000001));
#287280=CARTESIAN_POINT('Ctrl Pts',(-5.57303014600006,11.6,-9.67574807000001));
#287281=CARTESIAN_POINT('Ctrl Pts',(-5.57347895600006,15.2,-9.67906913300001));
#287282=CARTESIAN_POINT('Ctrl Pts',(-5.57347895600006,11.6,-9.67906913300001));
#287283=CARTESIAN_POINT('Ctrl Pts',(-5.57392579000005,15.2,-9.68239543700001));
#287284=CARTESIAN_POINT('Ctrl Pts',(-5.57392579000005,11.6,-9.68239543700001));
#287285=CARTESIAN_POINT('Ctrl Pts',(-5.57437064100006,15.2,-9.68572697500001));
#287286=CARTESIAN_POINT('Ctrl Pts',(-5.57437064100006,11.6,-9.68572697500001));
#287287=CARTESIAN_POINT('Ctrl Pts',(-5.57481350100006,15.2,-9.68906373900001));
#287288=CARTESIAN_POINT('Ctrl Pts',(-5.57481350100006,11.6,-9.68906373900001));
#287289=CARTESIAN_POINT('Ctrl Pts',(-5.57525436100006,15.2,-9.69240572200001));
#287290=CARTESIAN_POINT('Ctrl Pts',(-5.57525436100006,11.6,-9.69240572200001));
#287291=CARTESIAN_POINT('Ctrl Pts',(-5.57569321500006,15.2,-9.69575291700002));
#287292=CARTESIAN_POINT('Ctrl Pts',(-5.57569321500006,11.6,-9.69575291700002));
#287293=CARTESIAN_POINT('Ctrl Pts',(-5.57613005500006,15.2,-9.69910531700001));
#287294=CARTESIAN_POINT('Ctrl Pts',(-5.57613005500006,11.6,-9.69910531700001));
#287295=CARTESIAN_POINT('Ctrl Pts',(-5.57656487300005,15.2,-9.70246291300001));
#287296=CARTESIAN_POINT('Ctrl Pts',(-5.57656487300005,11.6,-9.70246291300001));
#287297=CARTESIAN_POINT('Ctrl Pts',(-5.57699766300006,15.2,-9.70582570000001));
#287298=CARTESIAN_POINT('Ctrl Pts',(-5.57699766300006,11.6,-9.70582570000001));
#287299=CARTESIAN_POINT('Ctrl Pts',(-5.57742841600006,15.2,-9.70919366800001));
#287300=CARTESIAN_POINT('Ctrl Pts',(-5.57742841600006,11.6,-9.70919366800001));
#287301=CARTESIAN_POINT('Ctrl Pts',(-5.57785712500006,15.2,-9.71256681200001));
#287302=CARTESIAN_POINT('Ctrl Pts',(-5.57785712500006,11.6,-9.71256681200001));
#287303=CARTESIAN_POINT('Ctrl Pts',(-5.57828378300006,15.2,-9.71594512400001));
#287304=CARTESIAN_POINT('Ctrl Pts',(-5.57828378300006,11.6,-9.71594512400001));
#287305=CARTESIAN_POINT('Ctrl Pts',(-5.57870838200006,15.2,-9.71932859700001));
#287306=CARTESIAN_POINT('Ctrl Pts',(-5.57870838200006,11.6,-9.71932859700001));
#287307=CARTESIAN_POINT('Ctrl Pts',(-5.57913091500006,15.2,-9.72271722400001));
#287308=CARTESIAN_POINT('Ctrl Pts',(-5.57913091500006,11.6,-9.72271722400001));
#287309=CARTESIAN_POINT('Ctrl Pts',(-5.57955137400006,15.2,-9.72611099700002));
#287310=CARTESIAN_POINT('Ctrl Pts',(-5.57955137400006,11.6,-9.72611099700002));
#287311=CARTESIAN_POINT('Ctrl Pts',(-5.57996975300005,15.2,-9.72950991000001));
#287312=CARTESIAN_POINT('Ctrl Pts',(-5.57996975300005,11.6,-9.72950991000001));
#287313=CARTESIAN_POINT('Ctrl Pts',(-5.58038604400006,15.2,-9.73291395500001));
#287314=CARTESIAN_POINT('Ctrl Pts',(-5.58038604400006,11.6,-9.73291395500001));
#287315=CARTESIAN_POINT('Ctrl Pts',(-5.58080023800006,15.2,-9.73632312400001));
#287316=CARTESIAN_POINT('Ctrl Pts',(-5.58080023800006,11.6,-9.73632312400001));
#287317=CARTESIAN_POINT('Ctrl Pts',(-5.58121233100006,15.2,-9.73973741000002));
#287318=CARTESIAN_POINT('Ctrl Pts',(-5.58121233100006,11.6,-9.73973741000002));
#287319=CARTESIAN_POINT('Ctrl Pts',(-5.58162231200006,15.2,-9.74315680800001));
#287320=CARTESIAN_POINT('Ctrl Pts',(-5.58162231200006,11.6,-9.74315680800001));
#287321=CARTESIAN_POINT('Ctrl Pts',(-5.58203017800006,15.2,-9.74658130900002));
#287322=CARTESIAN_POINT('Ctrl Pts',(-5.58203017800006,11.6,-9.74658130900002));
#287323=CARTESIAN_POINT('Ctrl Pts',(-5.58243591800006,15.2,-9.75001090500001));
#287324=CARTESIAN_POINT('Ctrl Pts',(-5.58243591800006,11.6,-9.75001090500001));
#287325=CARTESIAN_POINT('Ctrl Pts',(-5.58283952600005,15.2,-9.75344559000001));
#287326=CARTESIAN_POINT('Ctrl Pts',(-5.58283952600005,11.6,-9.75344559000001));
#287327=CARTESIAN_POINT('Ctrl Pts',(-5.58324099600005,15.2,-9.75688535700001));
#287328=CARTESIAN_POINT('Ctrl Pts',(-5.58324099600005,11.6,-9.75688535700001));
#287329=CARTESIAN_POINT('Ctrl Pts',(-5.58364031900005,15.2,-9.76033019900001));
#287330=CARTESIAN_POINT('Ctrl Pts',(-5.58364031900005,11.6,-9.76033019900001));
#287331=CARTESIAN_POINT('Ctrl Pts',(-5.58403748900006,15.2,-9.76378010900001));
#287332=CARTESIAN_POINT('Ctrl Pts',(-5.58403748900006,11.6,-9.76378010900001));
#287333=CARTESIAN_POINT('Ctrl Pts',(-5.58443250000006,15.2,-9.76723507800001));
#287334=CARTESIAN_POINT('Ctrl Pts',(-5.58443250000006,11.6,-9.76723507800001));
#287335=CARTESIAN_POINT('Ctrl Pts',(-5.58482534200006,15.2,-9.77069510100001));
#287336=CARTESIAN_POINT('Ctrl Pts',(-5.58482534200006,11.6,-9.77069510100001));
#287337=CARTESIAN_POINT('Ctrl Pts',(-5.58521601000006,15.2,-9.77416017100001));
#287338=CARTESIAN_POINT('Ctrl Pts',(-5.58521601000006,11.6,-9.77416017100001));
#287339=CARTESIAN_POINT('Ctrl Pts',(-5.58560449700006,15.2,-9.77763027800002));
#287340=CARTESIAN_POINT('Ctrl Pts',(-5.58560449700006,11.6,-9.77763027800002));
#287341=CARTESIAN_POINT('Ctrl Pts',(-5.58599079400006,15.2,-9.78110541800001));
#287342=CARTESIAN_POINT('Ctrl Pts',(-5.58599079400006,11.6,-9.78110541800001));
#287343=CARTESIAN_POINT('Ctrl Pts',(-5.58637489600006,15.2,-9.78458558300001));
#287344=CARTESIAN_POINT('Ctrl Pts',(-5.58637489600006,11.6,-9.78458558300001));
#287345=CARTESIAN_POINT('Ctrl Pts',(-5.58675679500006,15.2,-9.78807076600001));
#287346=CARTESIAN_POINT('Ctrl Pts',(-5.58675679500006,11.6,-9.78807076600001));
#287347=CARTESIAN_POINT('Ctrl Pts',(-5.58713648300006,15.2,-9.79156095800001));
#287348=CARTESIAN_POINT('Ctrl Pts',(-5.58713648300006,11.6,-9.79156095800001));
#287349=CARTESIAN_POINT('Ctrl Pts',(-5.58751395600006,15.2,-9.79505615600001));
#287350=CARTESIAN_POINT('Ctrl Pts',(-5.58751395600006,11.6,-9.79505615600001));
#287351=CARTESIAN_POINT('Ctrl Pts',(-5.58788920500006,15.2,-9.79855634900001));
#287352=CARTESIAN_POINT('Ctrl Pts',(-5.58788920500006,11.6,-9.79855634900001));
#287353=CARTESIAN_POINT('Ctrl Pts',(-5.58826222200006,15.2,-9.80206153200001));
#287354=CARTESIAN_POINT('Ctrl Pts',(-5.58826222200006,11.6,-9.80206153200001));
#287355=CARTESIAN_POINT('Ctrl Pts',(-5.58863300300006,15.2,-9.80557169700001));
#287356=CARTESIAN_POINT('Ctrl Pts',(-5.58863300300006,11.6,-9.80557169700001));
#287357=CARTESIAN_POINT('Ctrl Pts',(-5.58900153800006,15.2,-9.80908683700001));
#287358=CARTESIAN_POINT('Ctrl Pts',(-5.58900153800006,11.6,-9.80908683700001));
#287359=CARTESIAN_POINT('Ctrl Pts',(-5.58936782300006,15.2,-9.81260694600001));
#287360=CARTESIAN_POINT('Ctrl Pts',(-5.58936782300006,11.6,-9.81260694600001));
#287361=CARTESIAN_POINT('Ctrl Pts',(-5.58973184900006,15.2,-9.81613201700001));
#287362=CARTESIAN_POINT('Ctrl Pts',(-5.58973184900006,11.6,-9.81613201700001));
#287363=CARTESIAN_POINT('Ctrl Pts',(-5.59009361000006,15.2,-9.81966204100001));
#287364=CARTESIAN_POINT('Ctrl Pts',(-5.59009361000006,11.6,-9.81966204100001));
#287365=CARTESIAN_POINT('Ctrl Pts',(-5.59045309900006,15.2,-9.82319701200001));
#287366=CARTESIAN_POINT('Ctrl Pts',(-5.59045309900006,11.6,-9.82319701200001));
#287367=CARTESIAN_POINT('Ctrl Pts',(-5.59081030900006,15.2,-9.82673692500001));
#287368=CARTESIAN_POINT('Ctrl Pts',(-5.59081030900006,11.6,-9.82673692500001));
#287369=CARTESIAN_POINT('Ctrl Pts',(-5.59116523300006,15.2,-9.83028176900001));
#287370=CARTESIAN_POINT('Ctrl Pts',(-5.59116523300006,11.6,-9.83028176900001));
#287371=CARTESIAN_POINT('Ctrl Pts',(-5.59151786600006,15.2,-9.83383154100001));
#287372=CARTESIAN_POINT('Ctrl Pts',(-5.59151786600006,11.6,-9.83383154100001));
#287373=CARTESIAN_POINT('Ctrl Pts',(-5.59186819900006,15.2,-9.83738623200001));
#287374=CARTESIAN_POINT('Ctrl Pts',(-5.59186819900006,11.6,-9.83738623200001));
#287375=CARTESIAN_POINT('Ctrl Pts',(-5.59221622500006,15.2,-9.84094583600001));
#287376=CARTESIAN_POINT('Ctrl Pts',(-5.59221622500006,11.6,-9.84094583600001));
#287377=CARTESIAN_POINT('Ctrl Pts',(-5.59256194100006,15.2,-9.84451034500001));
#287378=CARTESIAN_POINT('Ctrl Pts',(-5.59256194100006,11.6,-9.84451034500001));
#287379=CARTESIAN_POINT('Ctrl Pts',(-5.59290533600006,15.2,-9.84807975100001));
#287380=CARTESIAN_POINT('Ctrl Pts',(-5.59290533600006,11.6,-9.84807975100001));
#287381=CARTESIAN_POINT('Ctrl Pts',(-5.59324640500006,15.2,-9.85165405000001));
#287382=CARTESIAN_POINT('Ctrl Pts',(-5.59324640500006,11.6,-9.85165405000001));
#287383=CARTESIAN_POINT('Ctrl Pts',(-5.59358514100006,15.2,-9.85523323300001));
#287384=CARTESIAN_POINT('Ctrl Pts',(-5.59358514100006,11.6,-9.85523323300001));
#287385=CARTESIAN_POINT('Ctrl Pts',(-5.59392153800006,15.2,-9.85881729400001));
#287386=CARTESIAN_POINT('Ctrl Pts',(-5.59392153800006,11.6,-9.85881729400001));
#287387=CARTESIAN_POINT('Ctrl Pts',(-5.59425559000006,15.2,-9.86240622500001));
#287388=CARTESIAN_POINT('Ctrl Pts',(-5.59425559000006,11.6,-9.86240622500001));
#287389=CARTESIAN_POINT('Ctrl Pts',(-5.59458728700006,15.2,-9.86600002000001));
#287390=CARTESIAN_POINT('Ctrl Pts',(-5.59458728700006,11.6,-9.86600002000001));
#287391=CARTESIAN_POINT('Ctrl Pts',(-5.59491662700006,15.2,-9.86959867100001));
#287392=CARTESIAN_POINT('Ctrl Pts',(-5.59491662700006,11.6,-9.86959867100001));
#287393=CARTESIAN_POINT('Ctrl Pts',(-5.59524360000006,15.2,-9.87320217300001));
#287394=CARTESIAN_POINT('Ctrl Pts',(-5.59524360000006,11.6,-9.87320217300001));
#287395=CARTESIAN_POINT('Ctrl Pts',(-5.59556820200006,15.2,-9.87681051700001));
#287396=CARTESIAN_POINT('Ctrl Pts',(-5.59556820200006,11.6,-9.87681051700001));
#287397=CARTESIAN_POINT('Ctrl Pts',(-5.59589042400006,15.2,-9.88042369800001));
#287398=CARTESIAN_POINT('Ctrl Pts',(-5.59589042400006,11.6,-9.88042369800001));
#287399=CARTESIAN_POINT('Ctrl Pts',(-5.59621026000006,15.2,-9.88404170800001));
#287400=CARTESIAN_POINT('Ctrl Pts',(-5.59621026000006,11.6,-9.88404170800001));
#287401=CARTESIAN_POINT('Ctrl Pts',(-5.59652770400006,15.2,-9.88766454000001));
#287402=CARTESIAN_POINT('Ctrl Pts',(-5.59652770400006,11.6,-9.88766454000001));
#287403=CARTESIAN_POINT('Ctrl Pts',(-5.59684275000006,15.2,-9.89129218700001));
#287404=CARTESIAN_POINT('Ctrl Pts',(-5.59684275000006,11.6,-9.89129218700001));
#287405=CARTESIAN_POINT('Ctrl Pts',(-5.59715539100006,15.2,-9.89492464200001));
#287406=CARTESIAN_POINT('Ctrl Pts',(-5.59715539100006,11.6,-9.89492464200001));
#287407=CARTESIAN_POINT('Ctrl Pts',(-5.59746562000006,15.2,-9.89856190000001));
#287408=CARTESIAN_POINT('Ctrl Pts',(-5.59746562000006,11.6,-9.89856190000001));
#287409=CARTESIAN_POINT('Ctrl Pts',(-5.59777343200006,15.2,-9.90220395300001));
#287410=CARTESIAN_POINT('Ctrl Pts',(-5.59777343200006,11.6,-9.90220395300001));
#287411=CARTESIAN_POINT('Ctrl Pts',(-5.59807881900006,15.2,-9.90585079300001));
#287412=CARTESIAN_POINT('Ctrl Pts',(-5.59807881900006,11.6,-9.90585079300001));
#287413=CARTESIAN_POINT('Ctrl Pts',(-5.59838177600006,15.2,-9.90950241400001));
#287414=CARTESIAN_POINT('Ctrl Pts',(-5.59838177600006,11.6,-9.90950241400001));
#287415=CARTESIAN_POINT('Ctrl Pts',(-5.59868229500006,15.2,-9.91315881000001));
#287416=CARTESIAN_POINT('Ctrl Pts',(-5.59868229500006,11.6,-9.91315881000001));
#287417=CARTESIAN_POINT('Ctrl Pts',(-5.59898037100006,15.2,-9.91681997300001));
#287418=CARTESIAN_POINT('Ctrl Pts',(-5.59898037100006,11.6,-9.91681997300001));
#287419=CARTESIAN_POINT('Ctrl Pts',(-5.59927599700006,15.2,-9.92048589600001));
#287420=CARTESIAN_POINT('Ctrl Pts',(-5.59927599700006,11.6,-9.92048589600001));
#287421=CARTESIAN_POINT('Ctrl Pts',(-5.59956916600005,15.2,-9.92415657400001));
#287422=CARTESIAN_POINT('Ctrl Pts',(-5.59956916600005,11.6,-9.92415657400001));
#287423=CARTESIAN_POINT('Ctrl Pts',(-5.59985987300006,15.2,-9.92783199800001));
#287424=CARTESIAN_POINT('Ctrl Pts',(-5.59985987300006,11.6,-9.92783199800001));
#287425=CARTESIAN_POINT('Ctrl Pts',(-5.60014811000006,15.2,-9.93151216200001));
#287426=CARTESIAN_POINT('Ctrl Pts',(-5.60014811000006,11.6,-9.93151216200001));
#287427=CARTESIAN_POINT('Ctrl Pts',(-5.60043387200006,15.2,-9.93519706000001));
#287428=CARTESIAN_POINT('Ctrl Pts',(-5.60043387200006,11.6,-9.93519706000001));
#287429=CARTESIAN_POINT('Ctrl Pts',(-5.60071715300006,15.2,-9.93888668300001));
#287430=CARTESIAN_POINT('Ctrl Pts',(-5.60071715300006,11.6,-9.93888668300001));
#287431=CARTESIAN_POINT('Ctrl Pts',(-5.60099794600006,15.2,-9.94258102700002));
#287432=CARTESIAN_POINT('Ctrl Pts',(-5.60099794600006,11.6,-9.94258102700002));
#287433=CARTESIAN_POINT('Ctrl Pts',(-5.60127624500006,15.2,-9.94628008400001));
#287434=CARTESIAN_POINT('Ctrl Pts',(-5.60127624500006,11.6,-9.94628008400001));
#287435=CARTESIAN_POINT('Ctrl Pts',(-5.60155204400006,15.2,-9.94998384700001));
#287436=CARTESIAN_POINT('Ctrl Pts',(-5.60155204400006,11.6,-9.94998384700001));
#287437=CARTESIAN_POINT('Ctrl Pts',(-5.60182533700006,15.2,-9.95369231100001));
#287438=CARTESIAN_POINT('Ctrl Pts',(-5.60182533700006,11.6,-9.95369231100001));
#287439=CARTESIAN_POINT('Ctrl Pts',(-5.60209611700006,15.2,-9.95740546800001));
#287440=CARTESIAN_POINT('Ctrl Pts',(-5.60209611700006,11.6,-9.95740546800001));
#287441=CARTESIAN_POINT('Ctrl Pts',(-5.60236437800006,15.2,-9.96112330900001));
#287442=CARTESIAN_POINT('Ctrl Pts',(-5.60236437800006,11.6,-9.96112330900001));
#287443=CARTESIAN_POINT('Ctrl Pts',(-5.60263011400005,15.2,-9.96484583000001));
#287444=CARTESIAN_POINT('Ctrl Pts',(-5.60263011400005,11.6,-9.96484583000001));
#287445=CARTESIAN_POINT('Ctrl Pts',(-5.60289331800006,15.2,-9.96857302300001));
#287446=CARTESIAN_POINT('Ctrl Pts',(-5.60289331800006,11.6,-9.96857302300001));
#287447=CARTESIAN_POINT('Ctrl Pts',(-5.60315398400006,15.2,-9.97230488000001));
#287448=CARTESIAN_POINT('Ctrl Pts',(-5.60315398400006,11.6,-9.97230488000001));
#287449=CARTESIAN_POINT('Ctrl Pts',(-5.60341210500006,15.2,-9.97604139500002));
#287450=CARTESIAN_POINT('Ctrl Pts',(-5.60341210500006,11.6,-9.97604139500002));
#287451=CARTESIAN_POINT('Ctrl Pts',(-5.60366767700006,15.2,-9.97978256300001));
#287452=CARTESIAN_POINT('Ctrl Pts',(-5.60366767700006,11.6,-9.97978256300001));
#287453=CARTESIAN_POINT('Ctrl Pts',(-5.60392069300006,15.2,-9.98352837700001));
#287454=CARTESIAN_POINT('Ctrl Pts',(-5.60392069300006,11.6,-9.98352837700001));
#287455=CARTESIAN_POINT('Ctrl Pts',(-5.60417114800006,15.2,-9.98727882900001));
#287456=CARTESIAN_POINT('Ctrl Pts',(-5.60417114800006,11.6,-9.98727882900001));
#287457=CARTESIAN_POINT('Ctrl Pts',(-5.60441903700006,15.2,-9.99103391600001));
#287458=CARTESIAN_POINT('Ctrl Pts',(-5.60441903700006,11.6,-9.99103391600001));
#287459=CARTESIAN_POINT('Ctrl Pts',(-5.60466435400006,15.2,-9.99479363100001));
#287460=CARTESIAN_POINT('Ctrl Pts',(-5.60466435400006,11.6,-9.99479363100001));
#287461=CARTESIAN_POINT('Ctrl Pts',(-5.60490709200006,15.2,-9.99855796400001));
#287462=CARTESIAN_POINT('Ctrl Pts',(-5.60490709200006,11.6,-9.99855796400001));
#287463=CARTESIAN_POINT('Ctrl Pts',(-5.60514724500006,15.2,-10.002326912));
#287464=CARTESIAN_POINT('Ctrl Pts',(-5.60514724500006,11.6,-10.002326912));
#287465=CARTESIAN_POINT('Ctrl Pts',(-5.60538480400006,15.2,-10.006100463));
#287466=CARTESIAN_POINT('Ctrl Pts',(-5.60538480400006,11.6,-10.006100463));
#287467=CARTESIAN_POINT('Ctrl Pts',(-5.60561976300006,15.2,-10.00987861));
#287468=CARTESIAN_POINT('Ctrl Pts',(-5.60561976300006,11.6,-10.00987861));
#287469=CARTESIAN_POINT('Ctrl Pts',(-5.60585211500006,15.2,-10.013661344));
#287470=CARTESIAN_POINT('Ctrl Pts',(-5.60585211500006,11.6,-10.013661344));
#287471=CARTESIAN_POINT('Ctrl Pts',(-5.60608185300006,15.2,-10.01744866));
#287472=CARTESIAN_POINT('Ctrl Pts',(-5.60608185300006,11.6,-10.01744866));
#287473=CARTESIAN_POINT('Ctrl Pts',(-5.60630897000006,15.2,-10.02124055));
#287474=CARTESIAN_POINT('Ctrl Pts',(-5.60630897000006,11.6,-10.02124055));
#287475=CARTESIAN_POINT('Ctrl Pts',(-5.60653346400006,15.2,-10.025037011));
#287476=CARTESIAN_POINT('Ctrl Pts',(-5.60653346400006,11.6,-10.025037011));
#287477=CARTESIAN_POINT('Ctrl Pts',(-5.60675533300006,15.2,-10.028838039));
#287478=CARTESIAN_POINT('Ctrl Pts',(-5.60675533300006,11.6,-10.028838039));
#287479=CARTESIAN_POINT('Ctrl Pts',(-5.60697457300006,15.2,-10.032643631));
#287480=CARTESIAN_POINT('Ctrl Pts',(-5.60697457300006,11.6,-10.032643631));
#287481=CARTESIAN_POINT('Ctrl Pts',(-5.60714786300006,15.2,-10.035691757));
#287482=CARTESIAN_POINT('Ctrl Pts',(-5.60714786300006,11.6,-10.035691757));
#287483=CARTESIAN_POINT('Ctrl Pts',(-5.60727664800006,15.2,-10.037979904));
#287484=CARTESIAN_POINT('Ctrl Pts',(-5.60727664800006,11.6,-10.037979904));
#287485=CARTESIAN_POINT('Ctrl Pts',(-5.60736197900006,15.2,-10.039506249));
#287486=CARTESIAN_POINT('Ctrl Pts',(-5.60736197900006,11.6,-10.039506249));
#287487=CARTESIAN_POINT('Ctrl Pts',(-5.60740451300005,15.2,-10.040269649));
#287488=CARTESIAN_POINT('Ctrl Pts',(-5.60740451300005,11.6,-10.040269649));
#287489=CARTESIAN_POINT('Ctrl Pts',(-5.36127880600006,15.2,-8.88241603200001));
#287490=CARTESIAN_POINT('Ctrl Pts',(-5.36135574400006,15.2,-8.88257249600001));
#287491=CARTESIAN_POINT('Ctrl Pts',(-5.36151222900005,15.2,-8.88289092900001));
#287492=CARTESIAN_POINT('Ctrl Pts',(-5.36174910400006,15.2,-8.88337354800001));
#287493=CARTESIAN_POINT('Ctrl Pts',(-5.36206771100006,15.2,-8.88402391700001));
#287494=CARTESIAN_POINT('Ctrl Pts',(-5.36246988000006,15.2,-8.88484693800002));
#287495=CARTESIAN_POINT('Ctrl Pts',(-5.36287772900006,15.2,-8.88568371000002));
#287496=CARTESIAN_POINT('Ctrl Pts',(-5.36328889700005,15.2,-8.88652944600001));
#287497=CARTESIAN_POINT('Ctrl Pts',(-5.36370335800005,15.2,-8.88738413200001));
#287498=CARTESIAN_POINT('Ctrl Pts',(-5.36412108300006,15.2,-8.88824775000002));
#287499=CARTESIAN_POINT('Ctrl Pts',(-5.36454204500005,15.2,-8.88912028400001));
#287500=CARTESIAN_POINT('Ctrl Pts',(-5.36496621600006,15.2,-8.89000172000001));
#287501=CARTESIAN_POINT('Ctrl Pts',(-5.36539356700006,15.2,-8.89089203900001));
#287502=CARTESIAN_POINT('Ctrl Pts',(-5.36582407300005,15.2,-8.89179122800002));
#287503=CARTESIAN_POINT('Ctrl Pts',(-5.36625770500006,15.2,-8.89269926800001));
#287504=CARTESIAN_POINT('Ctrl Pts',(-5.36669443700006,15.2,-8.89361614500002));
#287505=CARTESIAN_POINT('Ctrl Pts',(-5.36713424100006,15.2,-8.89454184300002));
#287506=CARTESIAN_POINT('Ctrl Pts',(-5.36757709000006,15.2,-8.89547634600002));
#287507=CARTESIAN_POINT('Ctrl Pts',(-5.36802295900006,15.2,-8.89641963800001));
#287508=CARTESIAN_POINT('Ctrl Pts',(-5.36847181900006,15.2,-8.89737170400002));
#287509=CARTESIAN_POINT('Ctrl Pts',(-5.36892364700006,15.2,-8.89833252800001));
#287510=CARTESIAN_POINT('Ctrl Pts',(-5.36937841200006,15.2,-8.89930209500001));
#287511=CARTESIAN_POINT('Ctrl Pts',(-5.36983609200006,15.2,-8.90028038900001));
#287512=CARTESIAN_POINT('Ctrl Pts',(-5.37029665900006,15.2,-8.90126739500002));
#287513=CARTESIAN_POINT('Ctrl Pts',(-5.37076008700006,15.2,-8.90226309800001));
#287514=CARTESIAN_POINT('Ctrl Pts',(-5.37122635100006,15.2,-8.90326748100001));
#287515=CARTESIAN_POINT('Ctrl Pts',(-5.37169542500005,15.2,-8.90428053100001));
#287516=CARTESIAN_POINT('Ctrl Pts',(-5.37216728300006,15.2,-8.90530223200001));
#287517=CARTESIAN_POINT('Ctrl Pts',(-5.37264189900006,15.2,-8.90633257000001));
#287518=CARTESIAN_POINT('Ctrl Pts',(-5.37311925100005,15.2,-8.90737152700002));
#287519=CARTESIAN_POINT('Ctrl Pts',(-5.37359931100006,15.2,-8.90841909100001));
#287520=CARTESIAN_POINT('Ctrl Pts',(-5.37408205300006,15.2,-8.90947524700002));
#287521=CARTESIAN_POINT('Ctrl Pts',(-5.37456745500006,15.2,-8.91053997800002));
#287522=CARTESIAN_POINT('Ctrl Pts',(-5.37505549100006,15.2,-8.91161327200001));
#287523=CARTESIAN_POINT('Ctrl Pts',(-5.37554613600006,15.2,-8.91269511100001));
#287524=CARTESIAN_POINT('Ctrl Pts',(-5.37603936500005,15.2,-8.91378548300001));
#287525=CARTESIAN_POINT('Ctrl Pts',(-5.37653515500006,15.2,-8.91488437200002));
#287526=CARTESIAN_POINT('Ctrl Pts',(-5.37703348100006,15.2,-8.91599176500002));
#287527=CARTESIAN_POINT('Ctrl Pts',(-5.37753431800006,15.2,-8.91710764600001));
#287528=CARTESIAN_POINT('Ctrl Pts',(-5.37803764200006,15.2,-8.91823200100001));
#287529=CARTESIAN_POINT('Ctrl Pts',(-5.37854343200006,15.2,-8.91936481500002));
#287530=CARTESIAN_POINT('Ctrl Pts',(-5.37905166000006,15.2,-8.92050607500002));
#287531=CARTESIAN_POINT('Ctrl Pts',(-5.37956230500006,15.2,-8.92165576600001));
#287532=CARTESIAN_POINT('Ctrl Pts',(-5.38007534200006,15.2,-8.92281387300002));
#287533=CARTESIAN_POINT('Ctrl Pts',(-5.38059074800006,15.2,-8.92398038200002));
#287534=CARTESIAN_POINT('Ctrl Pts',(-5.38110850100006,15.2,-8.92515528100001));
#287535=CARTESIAN_POINT('Ctrl Pts',(-5.38162857400006,15.2,-8.92633855400002));
#287536=CARTESIAN_POINT('Ctrl Pts',(-5.38215094700006,15.2,-8.92753018600001));
#287537=CARTESIAN_POINT('Ctrl Pts',(-5.38267559700006,15.2,-8.92873016600002));
#287538=CARTESIAN_POINT('Ctrl Pts',(-5.38320250000006,15.2,-8.92993847700001));
#287539=CARTESIAN_POINT('Ctrl Pts',(-5.38373163200006,15.2,-8.93115510700002));
#287540=CARTESIAN_POINT('Ctrl Pts',(-5.38426297200005,15.2,-8.93238004100001));
#287541=CARTESIAN_POINT('Ctrl Pts',(-5.38479649700006,15.2,-8.93361326700001));
#287542=CARTESIAN_POINT('Ctrl Pts',(-5.38533218400006,15.2,-8.93485477000001));
#287543=CARTESIAN_POINT('Ctrl Pts',(-5.38587001200006,15.2,-8.93610453600001));
#287544=CARTESIAN_POINT('Ctrl Pts',(-5.38640995700006,15.2,-8.93736255200002));
#287545=CARTESIAN_POINT('Ctrl Pts',(-5.38695199800006,15.2,-8.93862880300002));
#287546=CARTESIAN_POINT('Ctrl Pts',(-5.38749611100005,15.2,-8.93990327800001));
#287547=CARTESIAN_POINT('Ctrl Pts',(-5.38804227600005,15.2,-8.94118596000002));
#287548=CARTESIAN_POINT('Ctrl Pts',(-5.38859046900006,15.2,-8.94247684000002));
#287549=CARTESIAN_POINT('Ctrl Pts',(-5.38914067100006,15.2,-8.94377590100002));
#287550=CARTESIAN_POINT('Ctrl Pts',(-5.38969285900006,15.2,-8.94508313100001));
#287551=CARTESIAN_POINT('Ctrl Pts',(-5.39024701000006,15.2,-8.94639851600001));
#287552=CARTESIAN_POINT('Ctrl Pts',(-5.39080310300006,15.2,-8.94772204400001));
#287553=CARTESIAN_POINT('Ctrl Pts',(-5.39136111800006,15.2,-8.94905370100001));
#287554=CARTESIAN_POINT('Ctrl Pts',(-5.39192103300006,15.2,-8.95039347300001));
#287555=CARTESIAN_POINT('Ctrl Pts',(-5.39248282700005,15.2,-8.95174134800002));
#287556=CARTESIAN_POINT('Ctrl Pts',(-5.39304647700006,15.2,-8.95309731200001));
#287557=CARTESIAN_POINT('Ctrl Pts',(-5.39361196500006,15.2,-8.95446135300002));
#287558=CARTESIAN_POINT('Ctrl Pts',(-5.39417926700006,15.2,-8.95583345700001));
#287559=CARTESIAN_POINT('Ctrl Pts',(-5.39474836400006,15.2,-8.95721361200001));
#287560=CARTESIAN_POINT('Ctrl Pts',(-5.39531923500006,15.2,-8.95860180500001));
#287561=CARTESIAN_POINT('Ctrl Pts',(-5.39589185800006,15.2,-8.95999802100001));
#287562=CARTESIAN_POINT('Ctrl Pts',(-5.39646621500006,15.2,-8.96140225000002));
#287563=CARTESIAN_POINT('Ctrl Pts',(-5.39704228400006,15.2,-8.96281447600002));
#287564=CARTESIAN_POINT('Ctrl Pts',(-5.39762004300006,15.2,-8.96423469000002));
#287565=CARTESIAN_POINT('Ctrl Pts',(-5.39819947500006,15.2,-8.96566287700002));
#287566=CARTESIAN_POINT('Ctrl Pts',(-5.39878055600005,15.2,-8.96709902300002));
#287567=CARTESIAN_POINT('Ctrl Pts',(-5.39936326900006,15.2,-8.96854312000002));
#287568=CARTESIAN_POINT('Ctrl Pts',(-5.39994759300006,15.2,-8.96999515000001));
#287569=CARTESIAN_POINT('Ctrl Pts',(-5.40053350800005,15.2,-8.97145510400001));
#287570=CARTESIAN_POINT('Ctrl Pts',(-5.40112099300006,15.2,-8.97292296800002));
#287571=CARTESIAN_POINT('Ctrl Pts',(-5.40171003000006,15.2,-8.97439872800001));
#287572=CARTESIAN_POINT('Ctrl Pts',(-5.40230059700006,15.2,-8.97588237500001));
#287573=CARTESIAN_POINT('Ctrl Pts',(-5.40289267700006,15.2,-8.97737389500002));
#287574=CARTESIAN_POINT('Ctrl Pts',(-5.40348624900005,15.2,-8.97887327500002));
#287575=CARTESIAN_POINT('Ctrl Pts',(-5.40408129300006,15.2,-8.98038050300002));
#287576=CARTESIAN_POINT('Ctrl Pts',(-5.40467779100006,15.2,-8.98189556700002));
#287577=CARTESIAN_POINT('Ctrl Pts',(-5.40527572300006,15.2,-8.98341845500001));
#287578=CARTESIAN_POINT('Ctrl Pts',(-5.40587507000006,15.2,-8.98494915300001));
#287579=CARTESIAN_POINT('Ctrl Pts',(-5.40647581300005,15.2,-8.98648765100001));
#287580=CARTESIAN_POINT('Ctrl Pts',(-5.40707793100006,15.2,-8.98803393600001));
#287581=CARTESIAN_POINT('Ctrl Pts',(-5.40768140800005,15.2,-8.98958799500001));
#287582=CARTESIAN_POINT('Ctrl Pts',(-5.40828622400006,15.2,-8.99114981800002));
#287583=CARTESIAN_POINT('Ctrl Pts',(-5.40889235900006,15.2,-8.99271939000002));
#287584=CARTESIAN_POINT('Ctrl Pts',(-5.40949979600006,15.2,-8.99429670100002));
#287585=CARTESIAN_POINT('Ctrl Pts',(-5.41010851400006,15.2,-8.99588173800002));
#287586=CARTESIAN_POINT('Ctrl Pts',(-5.41071849700006,15.2,-8.99747449100002));
#287587=CARTESIAN_POINT('Ctrl Pts',(-5.41132972500006,15.2,-8.99907494500002));
#287588=CARTESIAN_POINT('Ctrl Pts',(-5.41194218100006,15.2,-9.00068309100002));
#287589=CARTESIAN_POINT('Ctrl Pts',(-5.41255584400006,15.2,-9.00229891600001));
#287590=CARTESIAN_POINT('Ctrl Pts',(-5.41317069800006,15.2,-9.00392240700001));
#287591=CARTESIAN_POINT('Ctrl Pts',(-5.41378672400006,15.2,-9.00555355400002));
#287592=CARTESIAN_POINT('Ctrl Pts',(-5.41440390400005,15.2,-9.00719234400002));
#287593=CARTESIAN_POINT('Ctrl Pts',(-5.41502222100006,15.2,-9.00883876600002));
#287594=CARTESIAN_POINT('Ctrl Pts',(-5.41564165400006,15.2,-9.01049280800001));
#287595=CARTESIAN_POINT('Ctrl Pts',(-5.41626218800006,15.2,-9.01215445900002));
#287596=CARTESIAN_POINT('Ctrl Pts',(-5.41688380400006,15.2,-9.01382370600002));
#287597=CARTESIAN_POINT('Ctrl Pts',(-5.41750648400006,15.2,-9.01550053800002));
#287598=CARTESIAN_POINT('Ctrl Pts',(-5.41813021000006,15.2,-9.01718494400002));
#287599=CARTESIAN_POINT('Ctrl Pts',(-5.41875496600006,15.2,-9.01887691300002));
#287600=CARTESIAN_POINT('Ctrl Pts',(-5.41938073300006,15.2,-9.02057643200001));
#287601=CARTESIAN_POINT('Ctrl Pts',(-5.42000749500006,15.2,-9.02228349000002));
#287602=CARTESIAN_POINT('Ctrl Pts',(-5.42063523200006,15.2,-9.02399807600002));
#287603=CARTESIAN_POINT('Ctrl Pts',(-5.42126392900006,15.2,-9.02572017700002));
#287604=CARTESIAN_POINT('Ctrl Pts',(-5.42189356700006,15.2,-9.02744978400002));
#287605=CARTESIAN_POINT('Ctrl Pts',(-5.42252413200006,15.2,-9.02918688400002));
#287606=CARTESIAN_POINT('Ctrl Pts',(-5.42315560300006,15.2,-9.03093146700002));
#287607=CARTESIAN_POINT('Ctrl Pts',(-5.42378796400006,15.2,-9.03268352000002));
#287608=CARTESIAN_POINT('Ctrl Pts',(-5.42442119900006,15.2,-9.03444303200001));
#287609=CARTESIAN_POINT('Ctrl Pts',(-5.42505529100006,15.2,-9.03620999300001));
#287610=CARTESIAN_POINT('Ctrl Pts',(-5.42569022200006,15.2,-9.03798439200001));
#287611=CARTESIAN_POINT('Ctrl Pts',(-5.42632597500006,15.2,-9.03976621700001));
#287612=CARTESIAN_POINT('Ctrl Pts',(-5.42696253600006,15.2,-9.04155545600002));
#287613=CARTESIAN_POINT('Ctrl Pts',(-5.42759988400006,15.2,-9.04335209900001));
#287614=CARTESIAN_POINT('Ctrl Pts',(-5.42823800600006,15.2,-9.04515613500001));
#287615=CARTESIAN_POINT('Ctrl Pts',(-5.42887688500006,15.2,-9.04696755200002));
#287616=CARTESIAN_POINT('Ctrl Pts',(-5.42951650300005,15.2,-9.04878634000001));
#287617=CARTESIAN_POINT('Ctrl Pts',(-5.43015684400006,15.2,-9.05061248700001));
#287618=CARTESIAN_POINT('Ctrl Pts',(-5.43079789200006,15.2,-9.05244598400002));
#287619=CARTESIAN_POINT('Ctrl Pts',(-5.43143963200006,15.2,-9.05428681700002));
#287620=CARTESIAN_POINT('Ctrl Pts',(-5.43208204500006,15.2,-9.05613497700001));
#287621=CARTESIAN_POINT('Ctrl Pts',(-5.43272511700006,15.2,-9.05799045400002));
#287622=CARTESIAN_POINT('Ctrl Pts',(-5.43336883000006,15.2,-9.05985323500002));
#287623=CARTESIAN_POINT('Ctrl Pts',(-5.43401316900006,15.2,-9.06172331100001));
#287624=CARTESIAN_POINT('Ctrl Pts',(-5.43465811900006,15.2,-9.06360066900002));
#287625=CARTESIAN_POINT('Ctrl Pts',(-5.43530366400006,15.2,-9.06548530000002));
#287626=CARTESIAN_POINT('Ctrl Pts',(-5.43594978500006,15.2,-9.06737719300001));
#287627=CARTESIAN_POINT('Ctrl Pts',(-5.43659647000006,15.2,-9.06927633700001));
#287628=CARTESIAN_POINT('Ctrl Pts',(-5.43724370200006,15.2,-9.07118272100002));
#287629=CARTESIAN_POINT('Ctrl Pts',(-5.43789146400006,15.2,-9.07309633400001));
#287630=CARTESIAN_POINT('Ctrl Pts',(-5.43853974200006,15.2,-9.07501716600001));
#287631=CARTESIAN_POINT('Ctrl Pts',(-5.43918852000006,15.2,-9.07694520700002));
#287632=CARTESIAN_POINT('Ctrl Pts',(-5.43983778200006,15.2,-9.07888044600002));
#287633=CARTESIAN_POINT('Ctrl Pts',(-5.44048751200005,15.2,-9.08082287200001));
#287634=CARTESIAN_POINT('Ctrl Pts',(-5.44113769600005,15.2,-9.08277247400001));
#287635=CARTESIAN_POINT('Ctrl Pts',(-5.44178831900005,15.2,-9.08472924200002));
#287636=CARTESIAN_POINT('Ctrl Pts',(-5.44243936400005,15.2,-9.08669316600001));
#287637=CARTESIAN_POINT('Ctrl Pts',(-5.44309081700006,15.2,-9.08866423400001));
#287638=CARTESIAN_POINT('Ctrl Pts',(-5.44374266300006,15.2,-9.09064243800002));
#287639=CARTESIAN_POINT('Ctrl Pts',(-5.44439488400006,15.2,-9.09262776600002));
#287640=CARTESIAN_POINT('Ctrl Pts',(-5.44504746900006,15.2,-9.09462020700002));
#287641=CARTESIAN_POINT('Ctrl Pts',(-5.44570040100006,15.2,-9.09661975100001));
#287642=CARTESIAN_POINT('Ctrl Pts',(-5.44635366500006,15.2,-9.09862638900002));
#287643=CARTESIAN_POINT('Ctrl Pts',(-5.44700724700006,15.2,-9.10064010900001));
#287644=CARTESIAN_POINT('Ctrl Pts',(-5.44766113200006,15.2,-9.10266090100002));
#287645=CARTESIAN_POINT('Ctrl Pts',(-5.44831530400006,15.2,-9.10468875600002));
#287646=CARTESIAN_POINT('Ctrl Pts',(-5.44896974900006,15.2,-9.10672366200002));
#287647=CARTESIAN_POINT('Ctrl Pts',(-5.44962445200006,15.2,-9.10876561000002));
#287648=CARTESIAN_POINT('Ctrl Pts',(-5.45027939900006,15.2,-9.11081458800002));
#287649=CARTESIAN_POINT('Ctrl Pts',(-5.45093457600006,15.2,-9.11287058900001));
#287650=CARTESIAN_POINT('Ctrl Pts',(-5.45158996700006,15.2,-9.11493360000001));
#287651=CARTESIAN_POINT('Ctrl Pts',(-5.45224555800006,15.2,-9.11700361100002));
#287652=CARTESIAN_POINT('Ctrl Pts',(-5.45290133500006,15.2,-9.11908061300002));
#287653=CARTESIAN_POINT('Ctrl Pts',(-5.45355728400006,15.2,-9.12116459600002));
#287654=CARTESIAN_POINT('Ctrl Pts',(-5.45421338900006,15.2,-9.12325554900002));
#287655=CARTESIAN_POINT('Ctrl Pts',(-5.45486963700006,15.2,-9.12535346200002));
#287656=CARTESIAN_POINT('Ctrl Pts',(-5.45552601400006,15.2,-9.12745832600002));
#287657=CARTESIAN_POINT('Ctrl Pts',(-5.45618250500006,15.2,-9.12957013000002));
#287658=CARTESIAN_POINT('Ctrl Pts',(-5.45683909700006,15.2,-9.13168886400002));
#287659=CARTESIAN_POINT('Ctrl Pts',(-5.45749577500006,15.2,-9.13381451800002));
#287660=CARTESIAN_POINT('Ctrl Pts',(-5.45815252500006,15.2,-9.13594708400002));
#287661=CARTESIAN_POINT('Ctrl Pts',(-5.45880933300006,15.2,-9.13808654900001));
#287662=CARTESIAN_POINT('Ctrl Pts',(-5.45946618600006,15.2,-9.14023290400002));
#287663=CARTESIAN_POINT('Ctrl Pts',(-5.46012307000006,15.2,-9.14238614000002));
#287664=CARTESIAN_POINT('Ctrl Pts',(-5.46077997000006,15.2,-9.14454624700002));
#287665=CARTESIAN_POINT('Ctrl Pts',(-5.46143687300006,15.2,-9.14671321500002));
#287666=CARTESIAN_POINT('Ctrl Pts',(-5.46209376500006,15.2,-9.14888703300001));
#287667=CARTESIAN_POINT('Ctrl Pts',(-5.46275063300006,15.2,-9.15106769300002));
#287668=CARTESIAN_POINT('Ctrl Pts',(-5.46340746300006,15.2,-9.15325518400002));
#287669=CARTESIAN_POINT('Ctrl Pts',(-5.46406424000006,15.2,-9.15544949700001));
#287670=CARTESIAN_POINT('Ctrl Pts',(-5.46472095400006,15.2,-9.15765062100002));
#287671=CARTESIAN_POINT('Ctrl Pts',(-5.46537758800006,15.2,-9.15985854900002));
#287672=CARTESIAN_POINT('Ctrl Pts',(-5.46603413000006,15.2,-9.16207326700002));
#287673=CARTESIAN_POINT('Ctrl Pts',(-5.46669056700006,15.2,-9.16429476900002));
#287674=CARTESIAN_POINT('Ctrl Pts',(-5.46734688500006,15.2,-9.16652304400002));
#287675=CARTESIAN_POINT('Ctrl Pts',(-5.46800307000006,15.2,-9.16875808200002));
#287676=CARTESIAN_POINT('Ctrl Pts',(-5.46865911200006,15.2,-9.17099987400002));
#287677=CARTESIAN_POINT('Ctrl Pts',(-5.46931499300006,15.2,-9.17324841000001));
#287678=CARTESIAN_POINT('Ctrl Pts',(-5.46997070400006,15.2,-9.17550368100001));
#287679=CARTESIAN_POINT('Ctrl Pts',(-5.47062622900006,15.2,-9.17776567700002));
#287680=CARTESIAN_POINT('Ctrl Pts',(-5.47128155700006,15.2,-9.18003438700002));
#287681=CARTESIAN_POINT('Ctrl Pts',(-5.47193667400006,15.2,-9.18230980400002));
#287682=CARTESIAN_POINT('Ctrl Pts',(-5.47259156600005,15.2,-9.18459191700002));
#287683=CARTESIAN_POINT('Ctrl Pts',(-5.47324622200006,15.2,-9.18688071700002));
#287684=CARTESIAN_POINT('Ctrl Pts',(-5.47390062900006,15.2,-9.18917619500002));
#287685=CARTESIAN_POINT('Ctrl Pts',(-5.47455477300006,15.2,-9.19147833900002));
#287686=CARTESIAN_POINT('Ctrl Pts',(-5.47520864000006,15.2,-9.19378714300001));
#287687=CARTESIAN_POINT('Ctrl Pts',(-5.47586222100006,15.2,-9.19610259600002));
#287688=CARTESIAN_POINT('Ctrl Pts',(-5.47651550000006,15.2,-9.19842468800002));
#287689=CARTESIAN_POINT('Ctrl Pts',(-5.47716846700006,15.2,-9.20075341100001));
#287690=CARTESIAN_POINT('Ctrl Pts',(-5.47782110600005,15.2,-9.20308875400002));
#287691=CARTESIAN_POINT('Ctrl Pts',(-5.47847340700006,15.2,-9.20543070800001));
#287692=CARTESIAN_POINT('Ctrl Pts',(-5.47912535700006,15.2,-9.20777926500002));
#287693=CARTESIAN_POINT('Ctrl Pts',(-5.47977694300006,15.2,-9.21013441500002));
#287694=CARTESIAN_POINT('Ctrl Pts',(-5.48042815200006,15.2,-9.21249614700002));
#287695=CARTESIAN_POINT('Ctrl Pts',(-5.48107897400006,15.2,-9.21486445500001));
#287696=CARTESIAN_POINT('Ctrl Pts',(-5.48172939300006,15.2,-9.21723932700001));
#287697=CARTESIAN_POINT('Ctrl Pts',(-5.48237940000006,15.2,-9.21962075500002));
#287698=CARTESIAN_POINT('Ctrl Pts',(-5.48302898100006,15.2,-9.22200872900002));
#287699=CARTESIAN_POINT('Ctrl Pts',(-5.48367812400006,15.2,-9.22440324100002));
#287700=CARTESIAN_POINT('Ctrl Pts',(-5.48432681600006,15.2,-9.22680428100002));
#287701=CARTESIAN_POINT('Ctrl Pts',(-5.48497504600006,15.2,-9.22921183900002));
#287702=CARTESIAN_POINT('Ctrl Pts',(-5.48562280200006,15.2,-9.23162590700001));
#287703=CARTESIAN_POINT('Ctrl Pts',(-5.48627007100006,15.2,-9.23404647600002));
#287704=CARTESIAN_POINT('Ctrl Pts',(-5.48691684200006,15.2,-9.23647353500002));
#287705=CARTESIAN_POINT('Ctrl Pts',(-5.48756310200006,15.2,-9.23890707800001));
#287706=CARTESIAN_POINT('Ctrl Pts',(-5.48820883900006,15.2,-9.24134709400001));
#287707=CARTESIAN_POINT('Ctrl Pts',(-5.48885404200006,15.2,-9.24379357300002));
#287708=CARTESIAN_POINT('Ctrl Pts',(-5.48949869800006,15.2,-9.24624650800002));
#287709=CARTESIAN_POINT('Ctrl Pts',(-5.49014279600006,15.2,-9.24870588900001));
#287710=CARTESIAN_POINT('Ctrl Pts',(-5.49078632300006,15.2,-9.25117170600002));
#287711=CARTESIAN_POINT('Ctrl Pts',(-5.49142927000006,15.2,-9.25364395200001));
#287712=CARTESIAN_POINT('Ctrl Pts',(-5.49207162100006,15.2,-9.25612261600002));
#287713=CARTESIAN_POINT('Ctrl Pts',(-5.49271336800006,15.2,-9.25860769100002));
#287714=CARTESIAN_POINT('Ctrl Pts',(-5.49335449800005,15.2,-9.26109916700002));
#287715=CARTESIAN_POINT('Ctrl Pts',(-5.49399499900006,15.2,-9.26359703400001));
#287716=CARTESIAN_POINT('Ctrl Pts',(-5.49463485900006,15.2,-9.26610128400002));
#287717=CARTESIAN_POINT('Ctrl Pts',(-5.49527406800006,15.2,-9.26861190900001));
#287718=CARTESIAN_POINT('Ctrl Pts',(-5.49591261300006,15.2,-9.27112889800001));
#287719=CARTESIAN_POINT('Ctrl Pts',(-5.49655048300006,15.2,-9.27365224400001));
#287720=CARTESIAN_POINT('Ctrl Pts',(-5.49718766700006,15.2,-9.27618193800001));
#287721=CARTESIAN_POINT('Ctrl Pts',(-5.49782415300006,15.2,-9.27871797000002));
#287722=CARTESIAN_POINT('Ctrl Pts',(-5.49845993000006,15.2,-9.28126033100002));
#287723=CARTESIAN_POINT('Ctrl Pts',(-5.49909498700006,15.2,-9.28380901500002));
#287724=CARTESIAN_POINT('Ctrl Pts',(-5.49972931200006,15.2,-9.28636401000002));
#287725=CARTESIAN_POINT('Ctrl Pts',(-5.50036289400006,15.2,-9.28892530800002));
#287726=CARTESIAN_POINT('Ctrl Pts',(-5.50099572200006,15.2,-9.29149290000002));
#287727=CARTESIAN_POINT('Ctrl Pts',(-5.50162778400006,15.2,-9.29406678000002));
#287728=CARTESIAN_POINT('Ctrl Pts',(-5.50225906900006,15.2,-9.29664693400002));
#287729=CARTESIAN_POINT('Ctrl Pts',(-5.50288956700006,15.2,-9.29923335800002));
#287730=CARTESIAN_POINT('Ctrl Pts',(-5.50351926700006,15.2,-9.30182604100001));
#287731=CARTESIAN_POINT('Ctrl Pts',(-5.50414815600006,15.2,-9.30442497500002));
#287732=CARTESIAN_POINT('Ctrl Pts',(-5.50477622400006,15.2,-9.30703015100002));
#287733=CARTESIAN_POINT('Ctrl Pts',(-5.50540346100005,15.2,-9.30964156000002));
#287734=CARTESIAN_POINT('Ctrl Pts',(-5.50602985400006,15.2,-9.31225919400001));
#287735=CARTESIAN_POINT('Ctrl Pts',(-5.50665539400006,15.2,-9.31488304500002));
#287736=CARTESIAN_POINT('Ctrl Pts',(-5.50728006900005,15.2,-9.31751310200001));
#287737=CARTESIAN_POINT('Ctrl Pts',(-5.50790386900006,15.2,-9.32014935900002));
#287738=CARTESIAN_POINT('Ctrl Pts',(-5.50852678200005,15.2,-9.32279180500002));
#287739=CARTESIAN_POINT('Ctrl Pts',(-5.50914879900006,15.2,-9.32544043300001));
#287740=CARTESIAN_POINT('Ctrl Pts',(-5.50976990800006,15.2,-9.32809523400002));
#287741=CARTESIAN_POINT('Ctrl Pts',(-5.51039009700006,15.2,-9.33075620000002));
#287742=CARTESIAN_POINT('Ctrl Pts',(-5.51100935800005,15.2,-9.33342332100001));
#287743=CARTESIAN_POINT('Ctrl Pts',(-5.51162767900006,15.2,-9.33609659000001));
#287744=CARTESIAN_POINT('Ctrl Pts',(-5.51224505000006,15.2,-9.33877599700002));
#287745=CARTESIAN_POINT('Ctrl Pts',(-5.51286145900006,15.2,-9.34146153400001));
#287746=CARTESIAN_POINT('Ctrl Pts',(-5.51347689600005,15.2,-9.34415319400001));
#287747=CARTESIAN_POINT('Ctrl Pts',(-5.51409135300006,15.2,-9.34685096600001));
#287748=CARTESIAN_POINT('Ctrl Pts',(-5.51470481600006,15.2,-9.34955484400002));
#287749=CARTESIAN_POINT('Ctrl Pts',(-5.51531727600006,15.2,-9.35226481800001));
#287750=CARTESIAN_POINT('Ctrl Pts',(-5.51592872200006,15.2,-9.35498087900001));
#287751=CARTESIAN_POINT('Ctrl Pts',(-5.51653914500006,15.2,-9.35770301900002));
#287752=CARTESIAN_POINT('Ctrl Pts',(-5.51714853300005,15.2,-9.36043123200001));
#287753=CARTESIAN_POINT('Ctrl Pts',(-5.51775687700006,15.2,-9.36316550500001));
#287754=CARTESIAN_POINT('Ctrl Pts',(-5.51836416700006,15.2,-9.36590583500001));
#287755=CARTESIAN_POINT('Ctrl Pts',(-5.51897039000006,15.2,-9.36865220900001));
#287756=CARTESIAN_POINT('Ctrl Pts',(-5.51957553900006,15.2,-9.37140462000002));
#287757=CARTESIAN_POINT('Ctrl Pts',(-5.52017960200006,15.2,-9.37416306100002));
#287758=CARTESIAN_POINT('Ctrl Pts',(-5.52078257000006,15.2,-9.37692752200002));
#287759=CARTESIAN_POINT('Ctrl Pts',(-5.52138443200006,15.2,-9.37969799600002));
#287760=CARTESIAN_POINT('Ctrl Pts',(-5.52198517700006,15.2,-9.38247447400002));
#287761=CARTESIAN_POINT('Ctrl Pts',(-5.52258479700006,15.2,-9.38525694700001));
#287762=CARTESIAN_POINT('Ctrl Pts',(-5.52318328100006,15.2,-9.38804540800002));
#287763=CARTESIAN_POINT('Ctrl Pts',(-5.52378061800006,15.2,-9.39083984800002));
#287764=CARTESIAN_POINT('Ctrl Pts',(-5.52437679900006,15.2,-9.39364025800002));
#287765=CARTESIAN_POINT('Ctrl Pts',(-5.52497181400006,15.2,-9.39644663300001));
#287766=CARTESIAN_POINT('Ctrl Pts',(-5.52556565400006,15.2,-9.39925896000002));
#287767=CARTESIAN_POINT('Ctrl Pts',(-5.52615830800006,15.2,-9.40207723400002));
#287768=CARTESIAN_POINT('Ctrl Pts',(-5.52674976600006,15.2,-9.40490144500002));
#287769=CARTESIAN_POINT('Ctrl Pts',(-5.52734001800006,15.2,-9.40773158700001));
#287770=CARTESIAN_POINT('Ctrl Pts',(-5.52792905500006,15.2,-9.41056764900001));
#287771=CARTESIAN_POINT('Ctrl Pts',(-5.52851686600006,15.2,-9.41340962500002));
#287772=CARTESIAN_POINT('Ctrl Pts',(-5.52910344300006,15.2,-9.41625750600002));
#287773=CARTESIAN_POINT('Ctrl Pts',(-5.52968877600006,15.2,-9.41911128400001));
#287774=CARTESIAN_POINT('Ctrl Pts',(-5.53027285400006,15.2,-9.42197095100001));
#287775=CARTESIAN_POINT('Ctrl Pts',(-5.53085566800006,15.2,-9.42483649900002));
#287776=CARTESIAN_POINT('Ctrl Pts',(-5.53143720800006,15.2,-9.42770791800001));
#287777=CARTESIAN_POINT('Ctrl Pts',(-5.53213351757476,15.2,-9.43116065867457));
#287778=CARTESIAN_POINT('Ctrl Pts',(-5.53282788771271,15.2,-9.43462218366274));
#287779=CARTESIAN_POINT('Ctrl Pts',(-5.53352029828741,15.2,-9.43809247833729));
#287780=CARTESIAN_POINT('Ctrl Pts',(-5.53421073242535,15.2,-9.44157152332546));
#287781=CARTESIAN_POINT('Ctrl Pts',(-5.53489917000006,15.2,-9.44505930400002));
#287782=CARTESIAN_POINT('Ctrl Pts',(-5.53547152800006,15.2,-9.44797160400002));
#287783=CARTESIAN_POINT('Ctrl Pts',(-5.53604253700006,15.2,-9.45088971200001));
#287784=CARTESIAN_POINT('Ctrl Pts',(-5.53661218600006,15.2,-9.45381362000001));
#287785=CARTESIAN_POINT('Ctrl Pts',(-5.53718046800006,15.2,-9.45674332000002));
#287786=CARTESIAN_POINT('Ctrl Pts',(-5.53774737000006,15.2,-9.45967880400002));
#287787=CARTESIAN_POINT('Ctrl Pts',(-5.53831288800006,15.2,-9.46262006300002));
#287788=CARTESIAN_POINT('Ctrl Pts',(-5.53887700700006,15.2,-9.46556709000001));
#287789=CARTESIAN_POINT('Ctrl Pts',(-5.53943972200006,15.2,-9.46851987700001));
#287790=CARTESIAN_POINT('Ctrl Pts',(-5.54000102100006,15.2,-9.47147841500002));
#287791=CARTESIAN_POINT('Ctrl Pts',(-5.54056089800006,15.2,-9.47444269800001));
#287792=CARTESIAN_POINT('Ctrl Pts',(-5.54111934100006,15.2,-9.47741271600002));
#287793=CARTESIAN_POINT('Ctrl Pts',(-5.54167634100006,15.2,-9.48038846300001));
#287794=CARTESIAN_POINT('Ctrl Pts',(-5.54223189100005,15.2,-9.48336993000002));
#287795=CARTESIAN_POINT('Ctrl Pts',(-5.54278597900006,15.2,-9.48635710900002));
#287796=CARTESIAN_POINT('Ctrl Pts',(-5.54333859900006,15.2,-9.48934999200001));
#287797=CARTESIAN_POINT('Ctrl Pts',(-5.54388974000006,15.2,-9.49234857200001));
#287798=CARTESIAN_POINT('Ctrl Pts',(-5.54443939300006,15.2,-9.49535284000002));
#287799=CARTESIAN_POINT('Ctrl Pts',(-5.54498755000006,15.2,-9.49836278900002));
#287800=CARTESIAN_POINT('Ctrl Pts',(-5.54553420100006,15.2,-9.50137841100002));
#287801=CARTESIAN_POINT('Ctrl Pts',(-5.54607933800006,15.2,-9.50439969700002));
#287802=CARTESIAN_POINT('Ctrl Pts',(-5.54662295300006,15.2,-9.50742664100002));
#287803=CARTESIAN_POINT('Ctrl Pts',(-5.54716503400006,15.2,-9.51045923400001));
#287804=CARTESIAN_POINT('Ctrl Pts',(-5.54770557400006,15.2,-9.51349746900001));
#287805=CARTESIAN_POINT('Ctrl Pts',(-5.54824456500006,15.2,-9.51654133600002));
#287806=CARTESIAN_POINT('Ctrl Pts',(-5.54878199800006,15.2,-9.51959083100002));
#287807=CARTESIAN_POINT('Ctrl Pts',(-5.54931786200005,15.2,-9.52264594300001));
#287808=CARTESIAN_POINT('Ctrl Pts',(-5.54985215100006,15.2,-9.52570666600002));
#287809=CARTESIAN_POINT('Ctrl Pts',(-5.55038485500006,15.2,-9.52877299000002));
#287810=CARTESIAN_POINT('Ctrl Pts',(-5.55091596500006,15.2,-9.53184491000002));
#287811=CARTESIAN_POINT('Ctrl Pts',(-5.55144547200006,15.2,-9.53492241800001));
#287812=CARTESIAN_POINT('Ctrl Pts',(-5.55197337000005,15.2,-9.53800550400001));
#287813=CARTESIAN_POINT('Ctrl Pts',(-5.55249964700006,15.2,-9.54109416100002));
#287814=CARTESIAN_POINT('Ctrl Pts',(-5.55302429700006,15.2,-9.54418838400001));
#287815=CARTESIAN_POINT('Ctrl Pts',(-5.55354730900006,15.2,-9.54728816200002));
#287816=CARTESIAN_POINT('Ctrl Pts',(-5.55406867700006,15.2,-9.55039348800002));
#287817=CARTESIAN_POINT('Ctrl Pts',(-5.55458839100006,15.2,-9.55350435500002));
#287818=CARTESIAN_POINT('Ctrl Pts',(-5.55510644200006,15.2,-9.55662075600002));
#287819=CARTESIAN_POINT('Ctrl Pts',(-5.55562282200006,15.2,-9.55974268200002));
#287820=CARTESIAN_POINT('Ctrl Pts',(-5.55613752400006,15.2,-9.56287012600002));
#287821=CARTESIAN_POINT('Ctrl Pts',(-5.55665053700006,15.2,-9.56600308000001));
#287822=CARTESIAN_POINT('Ctrl Pts',(-5.55716185500006,15.2,-9.56914153600002));
#287823=CARTESIAN_POINT('Ctrl Pts',(-5.55767146700005,15.2,-9.57228548700002));
#287824=CARTESIAN_POINT('Ctrl Pts',(-5.55817936700006,15.2,-9.57543492600001));
#287825=CARTESIAN_POINT('Ctrl Pts',(-5.55868554700006,15.2,-9.57858984400002));
#287826=CARTESIAN_POINT('Ctrl Pts',(-5.55918999600006,15.2,-9.58175023500001));
#287827=CARTESIAN_POINT('Ctrl Pts',(-5.55969270800006,15.2,-9.58491608900001));
#287828=CARTESIAN_POINT('Ctrl Pts',(-5.56019367400006,15.2,-9.58808740000002));
#287829=CARTESIAN_POINT('Ctrl Pts',(-5.56069288500006,15.2,-9.59126416200002));
#287830=CARTESIAN_POINT('Ctrl Pts',(-5.56119033400006,15.2,-9.59444636500002));
#287831=CARTESIAN_POINT('Ctrl Pts',(-5.56168601200006,15.2,-9.59763400200002));
#287832=CARTESIAN_POINT('Ctrl Pts',(-5.56217991100006,15.2,-9.60082706600002));
#287833=CARTESIAN_POINT('Ctrl Pts',(-5.56267202400006,15.2,-9.60402554800002));
#287834=CARTESIAN_POINT('Ctrl Pts',(-5.56316234000006,15.2,-9.60722944300001));
#287835=CARTESIAN_POINT('Ctrl Pts',(-5.56365085400006,15.2,-9.61043874100002));
#287836=CARTESIAN_POINT('Ctrl Pts',(-5.56413755700006,15.2,-9.61365343600002));
#287837=CARTESIAN_POINT('Ctrl Pts',(-5.56462243900006,15.2,-9.61687352000002));
#287838=CARTESIAN_POINT('Ctrl Pts',(-5.56510549500006,15.2,-9.62009898500002));
#287839=CARTESIAN_POINT('Ctrl Pts',(-5.56558671400006,15.2,-9.62332982500002));
#287840=CARTESIAN_POINT('Ctrl Pts',(-5.56606609100006,15.2,-9.62656603200001));
#287841=CARTESIAN_POINT('Ctrl Pts',(-5.56654361600006,15.2,-9.62980759800002));
#287842=CARTESIAN_POINT('Ctrl Pts',(-5.56701928100006,15.2,-9.63305451500002));
#287843=CARTESIAN_POINT('Ctrl Pts',(-5.56749308000006,15.2,-9.63630677700002));
#287844=CARTESIAN_POINT('Ctrl Pts',(-5.56796500300006,15.2,-9.63956437500002));
#287845=CARTESIAN_POINT('Ctrl Pts',(-5.56843504200006,15.2,-9.64282730200001));
#287846=CARTESIAN_POINT('Ctrl Pts',(-5.56890319100006,15.2,-9.64609555300001));
#287847=CARTESIAN_POINT('Ctrl Pts',(-5.56936944100006,15.2,-9.64936911600002));
#287848=CARTESIAN_POINT('Ctrl Pts',(-5.56983378400006,15.2,-9.65264798800001));
#287849=CARTESIAN_POINT('Ctrl Pts',(-5.57029621300006,15.2,-9.65593215900001));
#287850=CARTESIAN_POINT('Ctrl Pts',(-5.57075671900006,15.2,-9.65922162300001));
#287851=CARTESIAN_POINT('Ctrl Pts',(-5.57121529500006,15.2,-9.66251637100001));
#287852=CARTESIAN_POINT('Ctrl Pts',(-5.57167193400006,15.2,-9.66581639800001));
#287853=CARTESIAN_POINT('Ctrl Pts',(-5.57212662700006,15.2,-9.66912169500001));
#287854=CARTESIAN_POINT('Ctrl Pts',(-5.57257936700006,15.2,-9.67243225400001));
#287855=CARTESIAN_POINT('Ctrl Pts',(-5.57303014600006,15.2,-9.67574807000001));
#287856=CARTESIAN_POINT('Ctrl Pts',(-5.57347895600006,15.2,-9.67906913300001));
#287857=CARTESIAN_POINT('Ctrl Pts',(-5.57392579000005,15.2,-9.68239543700001));
#287858=CARTESIAN_POINT('Ctrl Pts',(-5.57437064100006,15.2,-9.68572697500001));
#287859=CARTESIAN_POINT('Ctrl Pts',(-5.57481350100006,15.2,-9.68906373900001));
#287860=CARTESIAN_POINT('Ctrl Pts',(-5.57525436100006,15.2,-9.69240572200001));
#287861=CARTESIAN_POINT('Ctrl Pts',(-5.57569321500006,15.2,-9.69575291700002));
#287862=CARTESIAN_POINT('Ctrl Pts',(-5.57613005500006,15.2,-9.69910531700001));
#287863=CARTESIAN_POINT('Ctrl Pts',(-5.57656487300005,15.2,-9.70246291300001));
#287864=CARTESIAN_POINT('Ctrl Pts',(-5.57699766300006,15.2,-9.70582570000001));
#287865=CARTESIAN_POINT('Ctrl Pts',(-5.57742841600006,15.2,-9.70919366800001));
#287866=CARTESIAN_POINT('Ctrl Pts',(-5.57785712500006,15.2,-9.71256681200001));
#287867=CARTESIAN_POINT('Ctrl Pts',(-5.57828378300006,15.2,-9.71594512400001));
#287868=CARTESIAN_POINT('Ctrl Pts',(-5.57870838200006,15.2,-9.71932859700001));
#287869=CARTESIAN_POINT('Ctrl Pts',(-5.57913091500006,15.2,-9.72271722400001));
#287870=CARTESIAN_POINT('Ctrl Pts',(-5.57955137400006,15.2,-9.72611099700002));
#287871=CARTESIAN_POINT('Ctrl Pts',(-5.57996975300005,15.2,-9.72950991000001));
#287872=CARTESIAN_POINT('Ctrl Pts',(-5.58038604400006,15.2,-9.73291395500001));
#287873=CARTESIAN_POINT('Ctrl Pts',(-5.58080023800006,15.2,-9.73632312400001));
#287874=CARTESIAN_POINT('Ctrl Pts',(-5.58121233100006,15.2,-9.73973741000002));
#287875=CARTESIAN_POINT('Ctrl Pts',(-5.58162231200006,15.2,-9.74315680800001));
#287876=CARTESIAN_POINT('Ctrl Pts',(-5.58203017800006,15.2,-9.74658130900002));
#287877=CARTESIAN_POINT('Ctrl Pts',(-5.58243591800006,15.2,-9.75001090500001));
#287878=CARTESIAN_POINT('Ctrl Pts',(-5.58283952600005,15.2,-9.75344559000001));
#287879=CARTESIAN_POINT('Ctrl Pts',(-5.58324099600005,15.2,-9.75688535700001));
#287880=CARTESIAN_POINT('Ctrl Pts',(-5.58364031900005,15.2,-9.76033019900001));
#287881=CARTESIAN_POINT('Ctrl Pts',(-5.58403748900006,15.2,-9.76378010900001));
#287882=CARTESIAN_POINT('Ctrl Pts',(-5.58443250000006,15.2,-9.76723507800001));
#287883=CARTESIAN_POINT('Ctrl Pts',(-5.58482534200006,15.2,-9.77069510100001));
#287884=CARTESIAN_POINT('Ctrl Pts',(-5.58521601000006,15.2,-9.77416017100001));
#287885=CARTESIAN_POINT('Ctrl Pts',(-5.58560449700006,15.2,-9.77763027800002));
#287886=CARTESIAN_POINT('Ctrl Pts',(-5.58599079400006,15.2,-9.78110541800001));
#287887=CARTESIAN_POINT('Ctrl Pts',(-5.58637489600006,15.2,-9.78458558300001));
#287888=CARTESIAN_POINT('Ctrl Pts',(-5.58675679500006,15.2,-9.78807076600001));
#287889=CARTESIAN_POINT('Ctrl Pts',(-5.58713648300006,15.2,-9.79156095800001));
#287890=CARTESIAN_POINT('Ctrl Pts',(-5.58751395600006,15.2,-9.79505615600001));
#287891=CARTESIAN_POINT('Ctrl Pts',(-5.58788920500006,15.2,-9.79855634900001));
#287892=CARTESIAN_POINT('Ctrl Pts',(-5.58826222200006,15.2,-9.80206153200001));
#287893=CARTESIAN_POINT('Ctrl Pts',(-5.58863300300006,15.2,-9.80557169700001));
#287894=CARTESIAN_POINT('Ctrl Pts',(-5.58900153800006,15.2,-9.80908683700001));
#287895=CARTESIAN_POINT('Ctrl Pts',(-5.58936782300006,15.2,-9.81260694600001));
#287896=CARTESIAN_POINT('Ctrl Pts',(-5.58973184900006,15.2,-9.81613201700001));
#287897=CARTESIAN_POINT('Ctrl Pts',(-5.59009361000006,15.2,-9.81966204100001));
#287898=CARTESIAN_POINT('Ctrl Pts',(-5.59045309900006,15.2,-9.82319701200001));
#287899=CARTESIAN_POINT('Ctrl Pts',(-5.59081030900006,15.2,-9.82673692500001));
#287900=CARTESIAN_POINT('Ctrl Pts',(-5.59116523300006,15.2,-9.83028176900001));
#287901=CARTESIAN_POINT('Ctrl Pts',(-5.59151786600006,15.2,-9.83383154100001));
#287902=CARTESIAN_POINT('Ctrl Pts',(-5.59186819900006,15.2,-9.83738623200001));
#287903=CARTESIAN_POINT('Ctrl Pts',(-5.59221622500006,15.2,-9.84094583600001));
#287904=CARTESIAN_POINT('Ctrl Pts',(-5.59256194100006,15.2,-9.84451034500001));
#287905=CARTESIAN_POINT('Ctrl Pts',(-5.59290533600006,15.2,-9.84807975100001));
#287906=CARTESIAN_POINT('Ctrl Pts',(-5.59324640500006,15.2,-9.85165405000001));
#287907=CARTESIAN_POINT('Ctrl Pts',(-5.59358514100006,15.2,-9.85523323300001));
#287908=CARTESIAN_POINT('Ctrl Pts',(-5.59392153800006,15.2,-9.85881729400001));
#287909=CARTESIAN_POINT('Ctrl Pts',(-5.59425559000006,15.2,-9.86240622500001));
#287910=CARTESIAN_POINT('Ctrl Pts',(-5.59458728700006,15.2,-9.86600002000001));
#287911=CARTESIAN_POINT('Ctrl Pts',(-5.59491662700006,15.2,-9.86959867100001));
#287912=CARTESIAN_POINT('Ctrl Pts',(-5.59524360000006,15.2,-9.87320217300001));
#287913=CARTESIAN_POINT('Ctrl Pts',(-5.59556820200006,15.2,-9.87681051700001));
#287914=CARTESIAN_POINT('Ctrl Pts',(-5.59589042400006,15.2,-9.88042369800001));
#287915=CARTESIAN_POINT('Ctrl Pts',(-5.59621026000006,15.2,-9.88404170800001));
#287916=CARTESIAN_POINT('Ctrl Pts',(-5.59652770400006,15.2,-9.88766454000001));
#287917=CARTESIAN_POINT('Ctrl Pts',(-5.59684275000006,15.2,-9.89129218700001));
#287918=CARTESIAN_POINT('Ctrl Pts',(-5.59715539100006,15.2,-9.89492464200001));
#287919=CARTESIAN_POINT('Ctrl Pts',(-5.59746562000006,15.2,-9.89856190000001));
#287920=CARTESIAN_POINT('Ctrl Pts',(-5.59777343200006,15.2,-9.90220395300001));
#287921=CARTESIAN_POINT('Ctrl Pts',(-5.59807881900006,15.2,-9.90585079300001));
#287922=CARTESIAN_POINT('Ctrl Pts',(-5.59838177600006,15.2,-9.90950241400001));
#287923=CARTESIAN_POINT('Ctrl Pts',(-5.59868229500006,15.2,-9.91315881000001));
#287924=CARTESIAN_POINT('Ctrl Pts',(-5.59898037100006,15.2,-9.91681997300001));
#287925=CARTESIAN_POINT('Ctrl Pts',(-5.59927599700006,15.2,-9.92048589600001));
#287926=CARTESIAN_POINT('Ctrl Pts',(-5.59956916600005,15.2,-9.92415657400001));
#287927=CARTESIAN_POINT('Ctrl Pts',(-5.59985987300006,15.2,-9.92783199800001));
#287928=CARTESIAN_POINT('Ctrl Pts',(-5.60014811000006,15.2,-9.93151216200001));
#287929=CARTESIAN_POINT('Ctrl Pts',(-5.60043387200006,15.2,-9.93519706000001));
#287930=CARTESIAN_POINT('Ctrl Pts',(-5.60071715300006,15.2,-9.93888668300001));
#287931=CARTESIAN_POINT('Ctrl Pts',(-5.60099794600006,15.2,-9.94258102700002));
#287932=CARTESIAN_POINT('Ctrl Pts',(-5.60127624500006,15.2,-9.94628008400001));
#287933=CARTESIAN_POINT('Ctrl Pts',(-5.60155204400006,15.2,-9.94998384700001));
#287934=CARTESIAN_POINT('Ctrl Pts',(-5.60182533700006,15.2,-9.95369231100001));
#287935=CARTESIAN_POINT('Ctrl Pts',(-5.60209611700006,15.2,-9.95740546800001));
#287936=CARTESIAN_POINT('Ctrl Pts',(-5.60236437800006,15.2,-9.96112330900001));
#287937=CARTESIAN_POINT('Ctrl Pts',(-5.60263011400005,15.2,-9.96484583000001));
#287938=CARTESIAN_POINT('Ctrl Pts',(-5.60289331800006,15.2,-9.96857302300001));
#287939=CARTESIAN_POINT('Ctrl Pts',(-5.60315398400006,15.2,-9.97230488000001));
#287940=CARTESIAN_POINT('Ctrl Pts',(-5.60341210500006,15.2,-9.97604139500002));
#287941=CARTESIAN_POINT('Ctrl Pts',(-5.60366767700006,15.2,-9.97978256300001));
#287942=CARTESIAN_POINT('Ctrl Pts',(-5.60392069300006,15.2,-9.98352837700001));
#287943=CARTESIAN_POINT('Ctrl Pts',(-5.60417114800006,15.2,-9.98727882900001));
#287944=CARTESIAN_POINT('Ctrl Pts',(-5.60441903700006,15.2,-9.99103391600001));
#287945=CARTESIAN_POINT('Ctrl Pts',(-5.60466435400006,15.2,-9.99479363100001));
#287946=CARTESIAN_POINT('Ctrl Pts',(-5.60490709200006,15.2,-9.99855796400001));
#287947=CARTESIAN_POINT('Ctrl Pts',(-5.60514724500006,15.2,-10.002326912));
#287948=CARTESIAN_POINT('Ctrl Pts',(-5.60538480400006,15.2,-10.006100463));
#287949=CARTESIAN_POINT('Ctrl Pts',(-5.60561976300006,15.2,-10.00987861));
#287950=CARTESIAN_POINT('Ctrl Pts',(-5.60585211500006,15.2,-10.013661344));
#287951=CARTESIAN_POINT('Ctrl Pts',(-5.60608185300006,15.2,-10.01744866));
#287952=CARTESIAN_POINT('Ctrl Pts',(-5.60630897000006,15.2,-10.02124055));
#287953=CARTESIAN_POINT('Ctrl Pts',(-5.60653346400006,15.2,-10.025037011));
#287954=CARTESIAN_POINT('Ctrl Pts',(-5.60675533300006,15.2,-10.028838039));
#287955=CARTESIAN_POINT('Ctrl Pts',(-5.60697457300006,15.2,-10.032643631));
#287956=CARTESIAN_POINT('Ctrl Pts',(-5.60714786300006,15.2,-10.035691757));
#287957=CARTESIAN_POINT('Ctrl Pts',(-5.60727664800006,15.2,-10.037979904));
#287958=CARTESIAN_POINT('Ctrl Pts',(-5.60736197900006,15.2,-10.039506249));
#287959=CARTESIAN_POINT('Ctrl Pts',(-5.60740451300005,15.2,-10.040269649));
#287960=CARTESIAN_POINT('Ctrl Pts',(-5.36127880600006,12.2,-8.88241603200001));
#287961=CARTESIAN_POINT('Ctrl Pts',(-5.36135574400006,12.2,-8.88257249600001));
#287962=CARTESIAN_POINT('Ctrl Pts',(-5.36151222900005,12.2,-8.88289092900001));
#287963=CARTESIAN_POINT('Ctrl Pts',(-5.36174910400006,12.2,-8.88337354800001));
#287964=CARTESIAN_POINT('Ctrl Pts',(-5.36206771100006,12.2,-8.88402391700001));
#287965=CARTESIAN_POINT('Ctrl Pts',(-5.36246988000006,12.2,-8.88484693800002));
#287966=CARTESIAN_POINT('Ctrl Pts',(-5.36287772900006,12.2,-8.88568371000002));
#287967=CARTESIAN_POINT('Ctrl Pts',(-5.36328889700005,12.2,-8.88652944600001));
#287968=CARTESIAN_POINT('Ctrl Pts',(-5.36370335800005,12.2,-8.88738413200001));
#287969=CARTESIAN_POINT('Ctrl Pts',(-5.36412108300006,12.2,-8.88824775000002));
#287970=CARTESIAN_POINT('Ctrl Pts',(-5.36454204500005,12.2,-8.88912028400001));
#287971=CARTESIAN_POINT('Ctrl Pts',(-5.36496621600006,12.2,-8.89000172000001));
#287972=CARTESIAN_POINT('Ctrl Pts',(-5.36539356700006,12.2,-8.89089203900001));
#287973=CARTESIAN_POINT('Ctrl Pts',(-5.36582407300005,12.2,-8.89179122800002));
#287974=CARTESIAN_POINT('Ctrl Pts',(-5.36625770500006,12.2,-8.89269926800001));
#287975=CARTESIAN_POINT('Ctrl Pts',(-5.36669443700006,12.2,-8.89361614500002));
#287976=CARTESIAN_POINT('Ctrl Pts',(-5.36713424100006,12.2,-8.89454184300002));
#287977=CARTESIAN_POINT('Ctrl Pts',(-5.36757709000006,12.2,-8.89547634600002));
#287978=CARTESIAN_POINT('Ctrl Pts',(-5.36802295900006,12.2,-8.89641963800001));
#287979=CARTESIAN_POINT('Ctrl Pts',(-5.36847181900006,12.2,-8.89737170400002));
#287980=CARTESIAN_POINT('Ctrl Pts',(-5.36892364700006,12.2,-8.89833252800001));
#287981=CARTESIAN_POINT('Ctrl Pts',(-5.36937841200006,12.2,-8.89930209500001));
#287982=CARTESIAN_POINT('Ctrl Pts',(-5.36983609200006,12.2,-8.90028038900001));
#287983=CARTESIAN_POINT('Ctrl Pts',(-5.37029665900006,12.2,-8.90126739500002));
#287984=CARTESIAN_POINT('Ctrl Pts',(-5.37076008700006,12.2,-8.90226309800001));
#287985=CARTESIAN_POINT('Ctrl Pts',(-5.37122635100006,12.2,-8.90326748100001));
#287986=CARTESIAN_POINT('Ctrl Pts',(-5.37169542500005,12.2,-8.90428053100001));
#287987=CARTESIAN_POINT('Ctrl Pts',(-5.37216728300006,12.2,-8.90530223200001));
#287988=CARTESIAN_POINT('Ctrl Pts',(-5.37264189900006,12.2,-8.90633257000001));
#287989=CARTESIAN_POINT('Ctrl Pts',(-5.37311925100005,12.2,-8.90737152700002));
#287990=CARTESIAN_POINT('Ctrl Pts',(-5.37359931100006,12.2,-8.90841909100001));
#287991=CARTESIAN_POINT('Ctrl Pts',(-5.37408205300006,12.2,-8.90947524700002));
#287992=CARTESIAN_POINT('Ctrl Pts',(-5.37456745500006,12.2,-8.91053997800002));
#287993=CARTESIAN_POINT('Ctrl Pts',(-5.37505549100006,12.2,-8.91161327200001));
#287994=CARTESIAN_POINT('Ctrl Pts',(-5.37554613600006,12.2,-8.91269511100001));
#287995=CARTESIAN_POINT('Ctrl Pts',(-5.37603936500005,12.2,-8.91378548300001));
#287996=CARTESIAN_POINT('Ctrl Pts',(-5.37653515500006,12.2,-8.91488437200002));
#287997=CARTESIAN_POINT('Ctrl Pts',(-5.37703348100006,12.2,-8.91599176500002));
#287998=CARTESIAN_POINT('Ctrl Pts',(-5.37753431800006,12.2,-8.91710764600001));
#287999=CARTESIAN_POINT('Ctrl Pts',(-5.37803764200006,12.2,-8.91823200100001));
#288000=CARTESIAN_POINT('Ctrl Pts',(-5.37854343200006,12.2,-8.91936481500002));
#288001=CARTESIAN_POINT('Ctrl Pts',(-5.37905166000006,12.2,-8.92050607500002));
#288002=CARTESIAN_POINT('Ctrl Pts',(-5.37956230500006,12.2,-8.92165576600001));
#288003=CARTESIAN_POINT('Ctrl Pts',(-5.38007534200006,12.2,-8.92281387300002));
#288004=CARTESIAN_POINT('Ctrl Pts',(-5.38059074800006,12.2,-8.92398038200002));
#288005=CARTESIAN_POINT('Ctrl Pts',(-5.38110850100006,12.2,-8.92515528100001));
#288006=CARTESIAN_POINT('Ctrl Pts',(-5.38162857400006,12.2,-8.92633855400002));
#288007=CARTESIAN_POINT('Ctrl Pts',(-5.38215094700006,12.2,-8.92753018600001));
#288008=CARTESIAN_POINT('Ctrl Pts',(-5.38267559700006,12.2,-8.92873016600002));
#288009=CARTESIAN_POINT('Ctrl Pts',(-5.38320250000006,12.2,-8.92993847700001));
#288010=CARTESIAN_POINT('Ctrl Pts',(-5.38373163200006,12.2,-8.93115510700002));
#288011=CARTESIAN_POINT('Ctrl Pts',(-5.38426297200005,12.2,-8.93238004100001));
#288012=CARTESIAN_POINT('Ctrl Pts',(-5.38479649700006,12.2,-8.93361326700001));
#288013=CARTESIAN_POINT('Ctrl Pts',(-5.38533218400006,12.2,-8.93485477000001));
#288014=CARTESIAN_POINT('Ctrl Pts',(-5.38587001200006,12.2,-8.93610453600001));
#288015=CARTESIAN_POINT('Ctrl Pts',(-5.38640995700006,12.2,-8.93736255200002));
#288016=CARTESIAN_POINT('Ctrl Pts',(-5.38695199800006,12.2,-8.93862880300002));
#288017=CARTESIAN_POINT('Ctrl Pts',(-5.38749611100005,12.2,-8.93990327800001));
#288018=CARTESIAN_POINT('Ctrl Pts',(-5.38804227600005,12.2,-8.94118596000002));
#288019=CARTESIAN_POINT('Ctrl Pts',(-5.38859046900006,12.2,-8.94247684000002));
#288020=CARTESIAN_POINT('Ctrl Pts',(-5.38914067100006,12.2,-8.94377590100002));
#288021=CARTESIAN_POINT('Ctrl Pts',(-5.38969285900006,12.2,-8.94508313100001));
#288022=CARTESIAN_POINT('Ctrl Pts',(-5.39024701000006,12.2,-8.94639851600001));
#288023=CARTESIAN_POINT('Ctrl Pts',(-5.39080310300006,12.2,-8.94772204400001));
#288024=CARTESIAN_POINT('Ctrl Pts',(-5.39136111800006,12.2,-8.94905370100001));
#288025=CARTESIAN_POINT('Ctrl Pts',(-5.39192103300006,12.2,-8.95039347300001));
#288026=CARTESIAN_POINT('Ctrl Pts',(-5.39248282700005,12.2,-8.95174134800002));
#288027=CARTESIAN_POINT('Ctrl Pts',(-5.39304647700006,12.2,-8.95309731200001));
#288028=CARTESIAN_POINT('Ctrl Pts',(-5.39361196500006,12.2,-8.95446135300002));
#288029=CARTESIAN_POINT('Ctrl Pts',(-5.39417926700006,12.2,-8.95583345700001));
#288030=CARTESIAN_POINT('Ctrl Pts',(-5.39474836400006,12.2,-8.95721361200001));
#288031=CARTESIAN_POINT('Ctrl Pts',(-5.39531923500006,12.2,-8.95860180500001));
#288032=CARTESIAN_POINT('Ctrl Pts',(-5.39589185800006,12.2,-8.95999802100001));
#288033=CARTESIAN_POINT('Ctrl Pts',(-5.39646621500006,12.2,-8.96140225000002));
#288034=CARTESIAN_POINT('Ctrl Pts',(-5.39704228400006,12.2,-8.96281447600002));
#288035=CARTESIAN_POINT('Ctrl Pts',(-5.39762004300006,12.2,-8.96423469000002));
#288036=CARTESIAN_POINT('Ctrl Pts',(-5.39819947500006,12.2,-8.96566287700002));
#288037=CARTESIAN_POINT('Ctrl Pts',(-5.39878055600005,12.2,-8.96709902300002));
#288038=CARTESIAN_POINT('Ctrl Pts',(-5.39936326900006,12.2,-8.96854312000002));
#288039=CARTESIAN_POINT('Ctrl Pts',(-5.39994759300006,12.2,-8.96999515000001));
#288040=CARTESIAN_POINT('Ctrl Pts',(-5.40053350800005,12.2,-8.97145510400001));
#288041=CARTESIAN_POINT('Ctrl Pts',(-5.40112099300006,12.2,-8.97292296800002));
#288042=CARTESIAN_POINT('Ctrl Pts',(-5.40171003000006,12.2,-8.97439872800001));
#288043=CARTESIAN_POINT('Ctrl Pts',(-5.40230059700006,12.2,-8.97588237500001));
#288044=CARTESIAN_POINT('Ctrl Pts',(-5.40289267700006,12.2,-8.97737389500002));
#288045=CARTESIAN_POINT('Ctrl Pts',(-5.40348624900005,12.2,-8.97887327500002));
#288046=CARTESIAN_POINT('Ctrl Pts',(-5.40408129300006,12.2,-8.98038050300002));
#288047=CARTESIAN_POINT('Ctrl Pts',(-5.40467779100006,12.2,-8.98189556700002));
#288048=CARTESIAN_POINT('Ctrl Pts',(-5.40527572300006,12.2,-8.98341845500001));
#288049=CARTESIAN_POINT('Ctrl Pts',(-5.40587507000006,12.2,-8.98494915300001));
#288050=CARTESIAN_POINT('Ctrl Pts',(-5.40647581300005,12.2,-8.98648765100001));
#288051=CARTESIAN_POINT('Ctrl Pts',(-5.40707793100006,12.2,-8.98803393600001));
#288052=CARTESIAN_POINT('Ctrl Pts',(-5.40768140800005,12.2,-8.98958799500001));
#288053=CARTESIAN_POINT('Ctrl Pts',(-5.40828622400006,12.2,-8.99114981800002));
#288054=CARTESIAN_POINT('Ctrl Pts',(-5.40889235900006,12.2,-8.99271939000002));
#288055=CARTESIAN_POINT('Ctrl Pts',(-5.40949979600006,12.2,-8.99429670100002));
#288056=CARTESIAN_POINT('Ctrl Pts',(-5.41010851400006,12.2,-8.99588173800002));
#288057=CARTESIAN_POINT('Ctrl Pts',(-5.41071849700006,12.2,-8.99747449100002));
#288058=CARTESIAN_POINT('Ctrl Pts',(-5.41132972500006,12.2,-8.99907494500002));
#288059=CARTESIAN_POINT('Ctrl Pts',(-5.41194218100006,12.2,-9.00068309100002));
#288060=CARTESIAN_POINT('Ctrl Pts',(-5.41255584400006,12.2,-9.00229891600001));
#288061=CARTESIAN_POINT('Ctrl Pts',(-5.41317069800006,12.2,-9.00392240700001));
#288062=CARTESIAN_POINT('Ctrl Pts',(-5.41378672400006,12.2,-9.00555355400002));
#288063=CARTESIAN_POINT('Ctrl Pts',(-5.41440390400005,12.2,-9.00719234400002));
#288064=CARTESIAN_POINT('Ctrl Pts',(-5.41502222100006,12.2,-9.00883876600002));
#288065=CARTESIAN_POINT('Ctrl Pts',(-5.41564165400006,12.2,-9.01049280800001));
#288066=CARTESIAN_POINT('Ctrl Pts',(-5.41626218800006,12.2,-9.01215445900002));
#288067=CARTESIAN_POINT('Ctrl Pts',(-5.41688380400006,12.2,-9.01382370600002));
#288068=CARTESIAN_POINT('Ctrl Pts',(-5.41750648400006,12.2,-9.01550053800002));
#288069=CARTESIAN_POINT('Ctrl Pts',(-5.41813021000006,12.2,-9.01718494400002));
#288070=CARTESIAN_POINT('Ctrl Pts',(-5.41875496600006,12.2,-9.01887691300002));
#288071=CARTESIAN_POINT('Ctrl Pts',(-5.41938073300006,12.2,-9.02057643200001));
#288072=CARTESIAN_POINT('Ctrl Pts',(-5.42000749500006,12.2,-9.02228349000002));
#288073=CARTESIAN_POINT('Ctrl Pts',(-5.42063523200006,12.2,-9.02399807600002));
#288074=CARTESIAN_POINT('Ctrl Pts',(-5.42126392900006,12.2,-9.02572017700002));
#288075=CARTESIAN_POINT('Ctrl Pts',(-5.42189356700006,12.2,-9.02744978400002));
#288076=CARTESIAN_POINT('Ctrl Pts',(-5.42252413200006,12.2,-9.02918688400002));
#288077=CARTESIAN_POINT('Ctrl Pts',(-5.42315560300006,12.2,-9.03093146700002));
#288078=CARTESIAN_POINT('Ctrl Pts',(-5.42378796400006,12.2,-9.03268352000002));
#288079=CARTESIAN_POINT('Ctrl Pts',(-5.42442119900006,12.2,-9.03444303200001));
#288080=CARTESIAN_POINT('Ctrl Pts',(-5.42505529100006,12.2,-9.03620999300001));
#288081=CARTESIAN_POINT('Ctrl Pts',(-5.42569022200006,12.2,-9.03798439200001));
#288082=CARTESIAN_POINT('Ctrl Pts',(-5.42632597500006,12.2,-9.03976621700001));
#288083=CARTESIAN_POINT('Ctrl Pts',(-5.42696253600006,12.2,-9.04155545600002));
#288084=CARTESIAN_POINT('Ctrl Pts',(-5.42759988400006,12.2,-9.04335209900001));
#288085=CARTESIAN_POINT('Ctrl Pts',(-5.42823800600006,12.2,-9.04515613500001));
#288086=CARTESIAN_POINT('Ctrl Pts',(-5.42887688500006,12.2,-9.04696755200002));
#288087=CARTESIAN_POINT('Ctrl Pts',(-5.42951650300005,12.2,-9.04878634000001));
#288088=CARTESIAN_POINT('Ctrl Pts',(-5.43015684400006,12.2,-9.05061248700001));
#288089=CARTESIAN_POINT('Ctrl Pts',(-5.43079789200006,12.2,-9.05244598400002));
#288090=CARTESIAN_POINT('Ctrl Pts',(-5.43143963200006,12.2,-9.05428681700002));
#288091=CARTESIAN_POINT('Ctrl Pts',(-5.43208204500006,12.2,-9.05613497700001));
#288092=CARTESIAN_POINT('Ctrl Pts',(-5.43272511700006,12.2,-9.05799045400002));
#288093=CARTESIAN_POINT('Ctrl Pts',(-5.43336883000006,12.2,-9.05985323500002));
#288094=CARTESIAN_POINT('Ctrl Pts',(-5.43401316900006,12.2,-9.06172331100001));
#288095=CARTESIAN_POINT('Ctrl Pts',(-5.43465811900006,12.2,-9.06360066900002));
#288096=CARTESIAN_POINT('Ctrl Pts',(-5.43530366400006,12.2,-9.06548530000002));
#288097=CARTESIAN_POINT('Ctrl Pts',(-5.43594978500006,12.2,-9.06737719300001));
#288098=CARTESIAN_POINT('Ctrl Pts',(-5.43659647000006,12.2,-9.06927633700001));
#288099=CARTESIAN_POINT('Ctrl Pts',(-5.43724370200006,12.2,-9.07118272100002));
#288100=CARTESIAN_POINT('Ctrl Pts',(-5.43789146400006,12.2,-9.07309633400001));
#288101=CARTESIAN_POINT('Ctrl Pts',(-5.43853974200006,12.2,-9.07501716600001));
#288102=CARTESIAN_POINT('Ctrl Pts',(-5.43918852000006,12.2,-9.07694520700002));
#288103=CARTESIAN_POINT('Ctrl Pts',(-5.43983778200006,12.2,-9.07888044600002));
#288104=CARTESIAN_POINT('Ctrl Pts',(-5.44048751200005,12.2,-9.08082287200001));
#288105=CARTESIAN_POINT('Ctrl Pts',(-5.44113769600005,12.2,-9.08277247400001));
#288106=CARTESIAN_POINT('Ctrl Pts',(-5.44178831900005,12.2,-9.08472924200002));
#288107=CARTESIAN_POINT('Ctrl Pts',(-5.44243936400005,12.2,-9.08669316600001));
#288108=CARTESIAN_POINT('Ctrl Pts',(-5.44309081700006,12.2,-9.08866423400001));
#288109=CARTESIAN_POINT('Ctrl Pts',(-5.44374266300006,12.2,-9.09064243800002));
#288110=CARTESIAN_POINT('Ctrl Pts',(-5.44439488400006,12.2,-9.09262776600002));
#288111=CARTESIAN_POINT('Ctrl Pts',(-5.44504746900006,12.2,-9.09462020700002));
#288112=CARTESIAN_POINT('Ctrl Pts',(-5.44570040100006,12.2,-9.09661975100001));
#288113=CARTESIAN_POINT('Ctrl Pts',(-5.44635366500006,12.2,-9.09862638900002));
#288114=CARTESIAN_POINT('Ctrl Pts',(-5.44700724700006,12.2,-9.10064010900001));
#288115=CARTESIAN_POINT('Ctrl Pts',(-5.44766113200006,12.2,-9.10266090100002));
#288116=CARTESIAN_POINT('Ctrl Pts',(-5.44831530400006,12.2,-9.10468875600002));
#288117=CARTESIAN_POINT('Ctrl Pts',(-5.44896974900006,12.2,-9.10672366200002));
#288118=CARTESIAN_POINT('Ctrl Pts',(-5.44962445200006,12.2,-9.10876561000002));
#288119=CARTESIAN_POINT('Ctrl Pts',(-5.45027939900006,12.2,-9.11081458800002));
#288120=CARTESIAN_POINT('Ctrl Pts',(-5.45093457600006,12.2,-9.11287058900001));
#288121=CARTESIAN_POINT('Ctrl Pts',(-5.45158996700006,12.2,-9.11493360000001));
#288122=CARTESIAN_POINT('Ctrl Pts',(-5.45224555800006,12.2,-9.11700361100002));
#288123=CARTESIAN_POINT('Ctrl Pts',(-5.45290133500006,12.2,-9.11908061300002));
#288124=CARTESIAN_POINT('Ctrl Pts',(-5.45355728400006,12.2,-9.12116459600002));
#288125=CARTESIAN_POINT('Ctrl Pts',(-5.45421338900006,12.2,-9.12325554900002));
#288126=CARTESIAN_POINT('Ctrl Pts',(-5.45486963700006,12.2,-9.12535346200002));
#288127=CARTESIAN_POINT('Ctrl Pts',(-5.45552601400006,12.2,-9.12745832600002));
#288128=CARTESIAN_POINT('Ctrl Pts',(-5.45618250500006,12.2,-9.12957013000002));
#288129=CARTESIAN_POINT('Ctrl Pts',(-5.45683909700006,12.2,-9.13168886400002));
#288130=CARTESIAN_POINT('Ctrl Pts',(-5.45749577500006,12.2,-9.13381451800002));
#288131=CARTESIAN_POINT('Ctrl Pts',(-5.45815252500006,12.2,-9.13594708400002));
#288132=CARTESIAN_POINT('Ctrl Pts',(-5.45880933300006,12.2,-9.13808654900001));
#288133=CARTESIAN_POINT('Ctrl Pts',(-5.45946618600006,12.2,-9.14023290400002));
#288134=CARTESIAN_POINT('Ctrl Pts',(-5.46012307000006,12.2,-9.14238614000002));
#288135=CARTESIAN_POINT('Ctrl Pts',(-5.46077997000006,12.2,-9.14454624700002));
#288136=CARTESIAN_POINT('Ctrl Pts',(-5.46143687300006,12.2,-9.14671321500002));
#288137=CARTESIAN_POINT('Ctrl Pts',(-5.46209376500006,12.2,-9.14888703300001));
#288138=CARTESIAN_POINT('Ctrl Pts',(-5.46275063300006,12.2,-9.15106769300002));
#288139=CARTESIAN_POINT('Ctrl Pts',(-5.46340746300006,12.2,-9.15325518400002));
#288140=CARTESIAN_POINT('Ctrl Pts',(-5.46406424000006,12.2,-9.15544949700001));
#288141=CARTESIAN_POINT('Ctrl Pts',(-5.46472095400006,12.2,-9.15765062100002));
#288142=CARTESIAN_POINT('Ctrl Pts',(-5.46537758800006,12.2,-9.15985854900002));
#288143=CARTESIAN_POINT('Ctrl Pts',(-5.46603413000006,12.2,-9.16207326700002));
#288144=CARTESIAN_POINT('Ctrl Pts',(-5.46669056700006,12.2,-9.16429476900002));
#288145=CARTESIAN_POINT('Ctrl Pts',(-5.46734688500006,12.2,-9.16652304400002));
#288146=CARTESIAN_POINT('Ctrl Pts',(-5.46800307000006,12.2,-9.16875808200002));
#288147=CARTESIAN_POINT('Ctrl Pts',(-5.46865911200006,12.2,-9.17099987400002));
#288148=CARTESIAN_POINT('Ctrl Pts',(-5.46931499300006,12.2,-9.17324841000001));
#288149=CARTESIAN_POINT('Ctrl Pts',(-5.46997070400006,12.2,-9.17550368100001));
#288150=CARTESIAN_POINT('Ctrl Pts',(-5.47062622900006,12.2,-9.17776567700002));
#288151=CARTESIAN_POINT('Ctrl Pts',(-5.47128155700006,12.2,-9.18003438700002));
#288152=CARTESIAN_POINT('Ctrl Pts',(-5.47193667400006,12.2,-9.18230980400002));
#288153=CARTESIAN_POINT('Ctrl Pts',(-5.47259156600005,12.2,-9.18459191700002));
#288154=CARTESIAN_POINT('Ctrl Pts',(-5.47324622200006,12.2,-9.18688071700002));
#288155=CARTESIAN_POINT('Ctrl Pts',(-5.47390062900006,12.2,-9.18917619500002));
#288156=CARTESIAN_POINT('Ctrl Pts',(-5.47455477300006,12.2,-9.19147833900002));
#288157=CARTESIAN_POINT('Ctrl Pts',(-5.47520864000006,12.2,-9.19378714300001));
#288158=CARTESIAN_POINT('Ctrl Pts',(-5.47586222100006,12.2,-9.19610259600002));
#288159=CARTESIAN_POINT('Ctrl Pts',(-5.47651550000006,12.2,-9.19842468800002));
#288160=CARTESIAN_POINT('Ctrl Pts',(-5.47716846700006,12.2,-9.20075341100001));
#288161=CARTESIAN_POINT('Ctrl Pts',(-5.47782110600005,12.2,-9.20308875400002));
#288162=CARTESIAN_POINT('Ctrl Pts',(-5.47847340700006,12.2,-9.20543070800001));
#288163=CARTESIAN_POINT('Ctrl Pts',(-5.47912535700006,12.2,-9.20777926500002));
#288164=CARTESIAN_POINT('Ctrl Pts',(-5.47977694300006,12.2,-9.21013441500002));
#288165=CARTESIAN_POINT('Ctrl Pts',(-5.48042815200006,12.2,-9.21249614700002));
#288166=CARTESIAN_POINT('Ctrl Pts',(-5.48107897400006,12.2,-9.21486445500001));
#288167=CARTESIAN_POINT('Ctrl Pts',(-5.48172939300006,12.2,-9.21723932700001));
#288168=CARTESIAN_POINT('Ctrl Pts',(-5.48237940000006,12.2,-9.21962075500002));
#288169=CARTESIAN_POINT('Ctrl Pts',(-5.48302898100006,12.2,-9.22200872900002));
#288170=CARTESIAN_POINT('Ctrl Pts',(-5.48367812400006,12.2,-9.22440324100002));
#288171=CARTESIAN_POINT('Ctrl Pts',(-5.48432681600006,12.2,-9.22680428100002));
#288172=CARTESIAN_POINT('Ctrl Pts',(-5.48497504600006,12.2,-9.22921183900002));
#288173=CARTESIAN_POINT('Ctrl Pts',(-5.48562280200006,12.2,-9.23162590700001));
#288174=CARTESIAN_POINT('Ctrl Pts',(-5.48627007100006,12.2,-9.23404647600002));
#288175=CARTESIAN_POINT('Ctrl Pts',(-5.48691684200006,12.2,-9.23647353500002));
#288176=CARTESIAN_POINT('Ctrl Pts',(-5.48756310200006,12.2,-9.23890707800001));
#288177=CARTESIAN_POINT('Ctrl Pts',(-5.48820883900006,12.2,-9.24134709400001));
#288178=CARTESIAN_POINT('Ctrl Pts',(-5.48885404200006,12.2,-9.24379357300002));
#288179=CARTESIAN_POINT('Ctrl Pts',(-5.48949869800006,12.2,-9.24624650800002));
#288180=CARTESIAN_POINT('Ctrl Pts',(-5.49014279600006,12.2,-9.24870588900001));
#288181=CARTESIAN_POINT('Ctrl Pts',(-5.49078632300006,12.2,-9.25117170600002));
#288182=CARTESIAN_POINT('Ctrl Pts',(-5.49142927000006,12.2,-9.25364395200001));
#288183=CARTESIAN_POINT('Ctrl Pts',(-5.49207162100006,12.2,-9.25612261600002));
#288184=CARTESIAN_POINT('Ctrl Pts',(-5.49271336800006,12.2,-9.25860769100002));
#288185=CARTESIAN_POINT('Ctrl Pts',(-5.49335449800005,12.2,-9.26109916700002));
#288186=CARTESIAN_POINT('Ctrl Pts',(-5.49399499900006,12.2,-9.26359703400001));
#288187=CARTESIAN_POINT('Ctrl Pts',(-5.49463485900006,12.2,-9.26610128400002));
#288188=CARTESIAN_POINT('Ctrl Pts',(-5.49527406800006,12.2,-9.26861190900001));
#288189=CARTESIAN_POINT('Ctrl Pts',(-5.49591261300006,12.2,-9.27112889800001));
#288190=CARTESIAN_POINT('Ctrl Pts',(-5.49655048300006,12.2,-9.27365224400001));
#288191=CARTESIAN_POINT('Ctrl Pts',(-5.49718766700006,12.2,-9.27618193800001));
#288192=CARTESIAN_POINT('Ctrl Pts',(-5.49782415300006,12.2,-9.27871797000002));
#288193=CARTESIAN_POINT('Ctrl Pts',(-5.49845993000006,12.2,-9.28126033100002));
#288194=CARTESIAN_POINT('Ctrl Pts',(-5.49909498700006,12.2,-9.28380901500002));
#288195=CARTESIAN_POINT('Ctrl Pts',(-5.49972931200006,12.2,-9.28636401000002));
#288196=CARTESIAN_POINT('Ctrl Pts',(-5.50036289400006,12.2,-9.28892530800002));
#288197=CARTESIAN_POINT('Ctrl Pts',(-5.50099572200006,12.2,-9.29149290000002));
#288198=CARTESIAN_POINT('Ctrl Pts',(-5.50162778400006,12.2,-9.29406678000002));
#288199=CARTESIAN_POINT('Ctrl Pts',(-5.50225906900006,12.2,-9.29664693400002));
#288200=CARTESIAN_POINT('Ctrl Pts',(-5.50288956700006,12.2,-9.29923335800002));
#288201=CARTESIAN_POINT('Ctrl Pts',(-5.50351926700006,12.2,-9.30182604100001));
#288202=CARTESIAN_POINT('Ctrl Pts',(-5.50414815600006,12.2,-9.30442497500002));
#288203=CARTESIAN_POINT('Ctrl Pts',(-5.50477622400006,12.2,-9.30703015100002));
#288204=CARTESIAN_POINT('Ctrl Pts',(-5.50540346100005,12.2,-9.30964156000002));
#288205=CARTESIAN_POINT('Ctrl Pts',(-5.50602985400006,12.2,-9.31225919400001));
#288206=CARTESIAN_POINT('Ctrl Pts',(-5.50665539400006,12.2,-9.31488304500002));
#288207=CARTESIAN_POINT('Ctrl Pts',(-5.50728006900005,12.2,-9.31751310200001));
#288208=CARTESIAN_POINT('Ctrl Pts',(-5.50790386900006,12.2,-9.32014935900002));
#288209=CARTESIAN_POINT('Ctrl Pts',(-5.50852678200005,12.2,-9.32279180500002));
#288210=CARTESIAN_POINT('Ctrl Pts',(-5.50914879900006,12.2,-9.32544043300001));
#288211=CARTESIAN_POINT('Ctrl Pts',(-5.50976990800006,12.2,-9.32809523400002));
#288212=CARTESIAN_POINT('Ctrl Pts',(-5.51039009700006,12.2,-9.33075620000002));
#288213=CARTESIAN_POINT('Ctrl Pts',(-5.51100935800005,12.2,-9.33342332100001));
#288214=CARTESIAN_POINT('Ctrl Pts',(-5.51162767900006,12.2,-9.33609659000001));
#288215=CARTESIAN_POINT('Ctrl Pts',(-5.51224505000006,12.2,-9.33877599700002));
#288216=CARTESIAN_POINT('Ctrl Pts',(-5.51286145900006,12.2,-9.34146153400001));
#288217=CARTESIAN_POINT('Ctrl Pts',(-5.51347689600005,12.2,-9.34415319400001));
#288218=CARTESIAN_POINT('Ctrl Pts',(-5.51409135300006,12.2,-9.34685096600001));
#288219=CARTESIAN_POINT('Ctrl Pts',(-5.51470481600006,12.2,-9.34955484400002));
#288220=CARTESIAN_POINT('Ctrl Pts',(-5.51531727600006,12.2,-9.35226481800001));
#288221=CARTESIAN_POINT('Ctrl Pts',(-5.51592872200006,12.2,-9.35498087900001));
#288222=CARTESIAN_POINT('Ctrl Pts',(-5.51653914500006,12.2,-9.35770301900002));
#288223=CARTESIAN_POINT('Ctrl Pts',(-5.51714853300005,12.2,-9.36043123200001));
#288224=CARTESIAN_POINT('Ctrl Pts',(-5.51775687700006,12.2,-9.36316550500001));
#288225=CARTESIAN_POINT('Ctrl Pts',(-5.51836416700006,12.2,-9.36590583500001));
#288226=CARTESIAN_POINT('Ctrl Pts',(-5.51897039000006,12.2,-9.36865220900001));
#288227=CARTESIAN_POINT('Ctrl Pts',(-5.51957553900006,12.2,-9.37140462000002));
#288228=CARTESIAN_POINT('Ctrl Pts',(-5.52017960200006,12.2,-9.37416306100002));
#288229=CARTESIAN_POINT('Ctrl Pts',(-5.52078257000006,12.2,-9.37692752200002));
#288230=CARTESIAN_POINT('Ctrl Pts',(-5.52138443200006,12.2,-9.37969799600002));
#288231=CARTESIAN_POINT('Ctrl Pts',(-5.52198517700006,12.2,-9.38247447400002));
#288232=CARTESIAN_POINT('Ctrl Pts',(-5.52258479700006,12.2,-9.38525694700001));
#288233=CARTESIAN_POINT('Ctrl Pts',(-5.52318328100006,12.2,-9.38804540800002));
#288234=CARTESIAN_POINT('Ctrl Pts',(-5.52378061800006,12.2,-9.39083984800002));
#288235=CARTESIAN_POINT('Ctrl Pts',(-5.52437679900006,12.2,-9.39364025800002));
#288236=CARTESIAN_POINT('Ctrl Pts',(-5.52497181400006,12.2,-9.39644663300001));
#288237=CARTESIAN_POINT('Ctrl Pts',(-5.52556565400006,12.2,-9.39925896000002));
#288238=CARTESIAN_POINT('Ctrl Pts',(-5.52615830800006,12.2,-9.40207723400002));
#288239=CARTESIAN_POINT('Ctrl Pts',(-5.52674976600006,12.2,-9.40490144500002));
#288240=CARTESIAN_POINT('Ctrl Pts',(-5.52734001800006,12.2,-9.40773158700001));
#288241=CARTESIAN_POINT('Ctrl Pts',(-5.52792905500006,12.2,-9.41056764900001));
#288242=CARTESIAN_POINT('Ctrl Pts',(-5.52851686600006,12.2,-9.41340962500002));
#288243=CARTESIAN_POINT('Ctrl Pts',(-5.52910344300006,12.2,-9.41625750600002));
#288244=CARTESIAN_POINT('Ctrl Pts',(-5.52968877600006,12.2,-9.41911128400001));
#288245=CARTESIAN_POINT('Ctrl Pts',(-5.53027285400006,12.2,-9.42197095100001));
#288246=CARTESIAN_POINT('Ctrl Pts',(-5.53085566800006,12.2,-9.42483649900002));
#288247=CARTESIAN_POINT('Ctrl Pts',(-5.53143720800006,12.2,-9.42770791800001));
#288248=CARTESIAN_POINT('Ctrl Pts',(-5.53213351757476,12.2,-9.43116065867457));
#288249=CARTESIAN_POINT('Ctrl Pts',(-5.53282788771271,12.2,-9.43462218366274));
#288250=CARTESIAN_POINT('Ctrl Pts',(-5.53352029828741,12.2,-9.43809247833729));
#288251=CARTESIAN_POINT('Ctrl Pts',(-5.53421073242535,12.2,-9.44157152332546));
#288252=CARTESIAN_POINT('Ctrl Pts',(-5.53489917000006,12.2,-9.44505930400002));
#288253=CARTESIAN_POINT('Ctrl Pts',(-5.53547152800006,12.2,-9.44797160400002));
#288254=CARTESIAN_POINT('Ctrl Pts',(-5.53604253700006,12.2,-9.45088971200001));
#288255=CARTESIAN_POINT('Ctrl Pts',(-5.53661218600006,12.2,-9.45381362000001));
#288256=CARTESIAN_POINT('Ctrl Pts',(-5.53718046800006,12.2,-9.45674332000002));
#288257=CARTESIAN_POINT('Ctrl Pts',(-5.53774737000006,12.2,-9.45967880400002));
#288258=CARTESIAN_POINT('Ctrl Pts',(-5.53831288800006,12.2,-9.46262006300002));
#288259=CARTESIAN_POINT('Ctrl Pts',(-5.53887700700006,12.2,-9.46556709000001));
#288260=CARTESIAN_POINT('Ctrl Pts',(-5.53943972200006,12.2,-9.46851987700001));
#288261=CARTESIAN_POINT('Ctrl Pts',(-5.54000102100006,12.2,-9.47147841500002));
#288262=CARTESIAN_POINT('Ctrl Pts',(-5.54056089800006,12.2,-9.47444269800001));
#288263=CARTESIAN_POINT('Ctrl Pts',(-5.54111934100006,12.2,-9.47741271600002));
#288264=CARTESIAN_POINT('Ctrl Pts',(-5.54167634100006,12.2,-9.48038846300001));
#288265=CARTESIAN_POINT('Ctrl Pts',(-5.54223189100005,12.2,-9.48336993000002));
#288266=CARTESIAN_POINT('Ctrl Pts',(-5.54278597900006,12.2,-9.48635710900002));
#288267=CARTESIAN_POINT('Ctrl Pts',(-5.54333859900006,12.2,-9.48934999200001));
#288268=CARTESIAN_POINT('Ctrl Pts',(-5.54388974000006,12.2,-9.49234857200001));
#288269=CARTESIAN_POINT('Ctrl Pts',(-5.54443939300006,12.2,-9.49535284000002));
#288270=CARTESIAN_POINT('Ctrl Pts',(-5.54498755000006,12.2,-9.49836278900002));
#288271=CARTESIAN_POINT('Ctrl Pts',(-5.54553420100006,12.2,-9.50137841100002));
#288272=CARTESIAN_POINT('Ctrl Pts',(-5.54607933800006,12.2,-9.50439969700002));
#288273=CARTESIAN_POINT('Ctrl Pts',(-5.54662295300006,12.2,-9.50742664100002));
#288274=CARTESIAN_POINT('Ctrl Pts',(-5.54716503400006,12.2,-9.51045923400001));
#288275=CARTESIAN_POINT('Ctrl Pts',(-5.54770557400006,12.2,-9.51349746900001));
#288276=CARTESIAN_POINT('Ctrl Pts',(-5.54824456500006,12.2,-9.51654133600002));
#288277=CARTESIAN_POINT('Ctrl Pts',(-5.54878199800006,12.2,-9.51959083100002));
#288278=CARTESIAN_POINT('Ctrl Pts',(-5.54931786200005,12.2,-9.52264594300001));
#288279=CARTESIAN_POINT('Ctrl Pts',(-5.54985215100006,12.2,-9.52570666600002));
#288280=CARTESIAN_POINT('Ctrl Pts',(-5.55038485500006,12.2,-9.52877299000002));
#288281=CARTESIAN_POINT('Ctrl Pts',(-5.55091596500006,12.2,-9.53184491000002));
#288282=CARTESIAN_POINT('Ctrl Pts',(-5.55144547200006,12.2,-9.53492241800001));
#288283=CARTESIAN_POINT('Ctrl Pts',(-5.55197337000005,12.2,-9.53800550400001));
#288284=CARTESIAN_POINT('Ctrl Pts',(-5.55249964700006,12.2,-9.54109416100002));
#288285=CARTESIAN_POINT('Ctrl Pts',(-5.55302429700006,12.2,-9.54418838400001));
#288286=CARTESIAN_POINT('Ctrl Pts',(-5.55354730900006,12.2,-9.54728816200002));
#288287=CARTESIAN_POINT('Ctrl Pts',(-5.55406867700006,12.2,-9.55039348800002));
#288288=CARTESIAN_POINT('Ctrl Pts',(-5.55458839100006,12.2,-9.55350435500002));
#288289=CARTESIAN_POINT('Ctrl Pts',(-5.55510644200006,12.2,-9.55662075600002));
#288290=CARTESIAN_POINT('Ctrl Pts',(-5.55562282200006,12.2,-9.55974268200002));
#288291=CARTESIAN_POINT('Ctrl Pts',(-5.55613752400006,12.2,-9.56287012600002));
#288292=CARTESIAN_POINT('Ctrl Pts',(-5.55665053700006,12.2,-9.56600308000001));
#288293=CARTESIAN_POINT('Ctrl Pts',(-5.55716185500006,12.2,-9.56914153600002));
#288294=CARTESIAN_POINT('Ctrl Pts',(-5.55767146700005,12.2,-9.57228548700002));
#288295=CARTESIAN_POINT('Ctrl Pts',(-5.55817936700006,12.2,-9.57543492600001));
#288296=CARTESIAN_POINT('Ctrl Pts',(-5.55868554700006,12.2,-9.57858984400002));
#288297=CARTESIAN_POINT('Ctrl Pts',(-5.55918999600006,12.2,-9.58175023500001));
#288298=CARTESIAN_POINT('Ctrl Pts',(-5.55969270800006,12.2,-9.58491608900001));
#288299=CARTESIAN_POINT('Ctrl Pts',(-5.56019367400006,12.2,-9.58808740000002));
#288300=CARTESIAN_POINT('Ctrl Pts',(-5.56069288500006,12.2,-9.59126416200002));
#288301=CARTESIAN_POINT('Ctrl Pts',(-5.56119033400006,12.2,-9.59444636500002));
#288302=CARTESIAN_POINT('Ctrl Pts',(-5.56168601200006,12.2,-9.59763400200002));
#288303=CARTESIAN_POINT('Ctrl Pts',(-5.56217991100006,12.2,-9.60082706600002));
#288304=CARTESIAN_POINT('Ctrl Pts',(-5.56267202400006,12.2,-9.60402554800002));
#288305=CARTESIAN_POINT('Ctrl Pts',(-5.56316234000006,12.2,-9.60722944300001));
#288306=CARTESIAN_POINT('Ctrl Pts',(-5.56365085400006,12.2,-9.61043874100002));
#288307=CARTESIAN_POINT('Ctrl Pts',(-5.56413755700006,12.2,-9.61365343600002));
#288308=CARTESIAN_POINT('Ctrl Pts',(-5.56462243900006,12.2,-9.61687352000002));
#288309=CARTESIAN_POINT('Ctrl Pts',(-5.56510549500006,12.2,-9.62009898500002));
#288310=CARTESIAN_POINT('Ctrl Pts',(-5.56558671400006,12.2,-9.62332982500002));
#288311=CARTESIAN_POINT('Ctrl Pts',(-5.56606609100006,12.2,-9.62656603200001));
#288312=CARTESIAN_POINT('Ctrl Pts',(-5.56654361600006,12.2,-9.62980759800002));
#288313=CARTESIAN_POINT('Ctrl Pts',(-5.56701928100006,12.2,-9.63305451500002));
#288314=CARTESIAN_POINT('Ctrl Pts',(-5.56749308000006,12.2,-9.63630677700002));
#288315=CARTESIAN_POINT('Ctrl Pts',(-5.56796500300006,12.2,-9.63956437500002));
#288316=CARTESIAN_POINT('Ctrl Pts',(-5.56843504200006,12.2,-9.64282730200001));
#288317=CARTESIAN_POINT('Ctrl Pts',(-5.56890319100006,12.2,-9.64609555300001));
#288318=CARTESIAN_POINT('Ctrl Pts',(-5.56936944100006,12.2,-9.64936911600002));
#288319=CARTESIAN_POINT('Ctrl Pts',(-5.56983378400006,12.2,-9.65264798800001));
#288320=CARTESIAN_POINT('Ctrl Pts',(-5.57029621300006,12.2,-9.65593215900001));
#288321=CARTESIAN_POINT('Ctrl Pts',(-5.57075671900006,12.2,-9.65922162300001));
#288322=CARTESIAN_POINT('Ctrl Pts',(-5.57121529500006,12.2,-9.66251637100001));
#288323=CARTESIAN_POINT('Ctrl Pts',(-5.57167193400006,12.2,-9.66581639800001));
#288324=CARTESIAN_POINT('Ctrl Pts',(-5.57212662700006,12.2,-9.66912169500001));
#288325=CARTESIAN_POINT('Ctrl Pts',(-5.57257936700006,12.2,-9.67243225400001));
#288326=CARTESIAN_POINT('Ctrl Pts',(-5.57303014600006,12.2,-9.67574807000001));
#288327=CARTESIAN_POINT('Ctrl Pts',(-5.57347895600006,12.2,-9.67906913300001));
#288328=CARTESIAN_POINT('Ctrl Pts',(-5.57392579000005,12.2,-9.68239543700001));
#288329=CARTESIAN_POINT('Ctrl Pts',(-5.57437064100006,12.2,-9.68572697500001));
#288330=CARTESIAN_POINT('Ctrl Pts',(-5.57481350100006,12.2,-9.68906373900001));
#288331=CARTESIAN_POINT('Ctrl Pts',(-5.57525436100006,12.2,-9.69240572200001));
#288332=CARTESIAN_POINT('Ctrl Pts',(-5.57569321500006,12.2,-9.69575291700002));
#288333=CARTESIAN_POINT('Ctrl Pts',(-5.57613005500006,12.2,-9.69910531700001));
#288334=CARTESIAN_POINT('Ctrl Pts',(-5.57656487300005,12.2,-9.70246291300001));
#288335=CARTESIAN_POINT('Ctrl Pts',(-5.57699766300006,12.2,-9.70582570000001));
#288336=CARTESIAN_POINT('Ctrl Pts',(-5.57742841600006,12.2,-9.70919366800001));
#288337=CARTESIAN_POINT('Ctrl Pts',(-5.57785712500006,12.2,-9.71256681200001));
#288338=CARTESIAN_POINT('Ctrl Pts',(-5.57828378300006,12.2,-9.71594512400001));
#288339=CARTESIAN_POINT('Ctrl Pts',(-5.57870838200006,12.2,-9.71932859700001));
#288340=CARTESIAN_POINT('Ctrl Pts',(-5.57913091500006,12.2,-9.72271722400001));
#288341=CARTESIAN_POINT('Ctrl Pts',(-5.57955137400006,12.2,-9.72611099700002));
#288342=CARTESIAN_POINT('Ctrl Pts',(-5.57996975300005,12.2,-9.72950991000001));
#288343=CARTESIAN_POINT('Ctrl Pts',(-5.58038604400006,12.2,-9.73291395500001));
#288344=CARTESIAN_POINT('Ctrl Pts',(-5.58080023800006,12.2,-9.73632312400001));
#288345=CARTESIAN_POINT('Ctrl Pts',(-5.58121233100006,12.2,-9.73973741000002));
#288346=CARTESIAN_POINT('Ctrl Pts',(-5.58162231200006,12.2,-9.74315680800001));
#288347=CARTESIAN_POINT('Ctrl Pts',(-5.58203017800006,12.2,-9.74658130900002));
#288348=CARTESIAN_POINT('Ctrl Pts',(-5.58243591800006,12.2,-9.75001090500001));
#288349=CARTESIAN_POINT('Ctrl Pts',(-5.58283952600005,12.2,-9.75344559000001));
#288350=CARTESIAN_POINT('Ctrl Pts',(-5.58324099600005,12.2,-9.75688535700001));
#288351=CARTESIAN_POINT('Ctrl Pts',(-5.58364031900005,12.2,-9.76033019900001));
#288352=CARTESIAN_POINT('Ctrl Pts',(-5.58403748900006,12.2,-9.76378010900001));
#288353=CARTESIAN_POINT('Ctrl Pts',(-5.58443250000006,12.2,-9.76723507800001));
#288354=CARTESIAN_POINT('Ctrl Pts',(-5.58482534200006,12.2,-9.77069510100001));
#288355=CARTESIAN_POINT('Ctrl Pts',(-5.58521601000006,12.2,-9.77416017100001));
#288356=CARTESIAN_POINT('Ctrl Pts',(-5.58560449700006,12.2,-9.77763027800002));
#288357=CARTESIAN_POINT('Ctrl Pts',(-5.58599079400006,12.2,-9.78110541800001));
#288358=CARTESIAN_POINT('Ctrl Pts',(-5.58637489600006,12.2,-9.78458558300001));
#288359=CARTESIAN_POINT('Ctrl Pts',(-5.58675679500006,12.2,-9.78807076600001));
#288360=CARTESIAN_POINT('Ctrl Pts',(-5.58713648300006,12.2,-9.79156095800001));
#288361=CARTESIAN_POINT('Ctrl Pts',(-5.58751395600006,12.2,-9.79505615600001));
#288362=CARTESIAN_POINT('Ctrl Pts',(-5.58788920500006,12.2,-9.79855634900001));
#288363=CARTESIAN_POINT('Ctrl Pts',(-5.58826222200006,12.2,-9.80206153200001));
#288364=CARTESIAN_POINT('Ctrl Pts',(-5.58863300300006,12.2,-9.80557169700001));
#288365=CARTESIAN_POINT('Ctrl Pts',(-5.58900153800006,12.2,-9.80908683700001));
#288366=CARTESIAN_POINT('Ctrl Pts',(-5.58936782300006,12.2,-9.81260694600001));
#288367=CARTESIAN_POINT('Ctrl Pts',(-5.58973184900006,12.2,-9.81613201700001));
#288368=CARTESIAN_POINT('Ctrl Pts',(-5.59009361000006,12.2,-9.81966204100001));
#288369=CARTESIAN_POINT('Ctrl Pts',(-5.59045309900006,12.2,-9.82319701200001));
#288370=CARTESIAN_POINT('Ctrl Pts',(-5.59081030900006,12.2,-9.82673692500001));
#288371=CARTESIAN_POINT('Ctrl Pts',(-5.59116523300006,12.2,-9.83028176900001));
#288372=CARTESIAN_POINT('Ctrl Pts',(-5.59151786600006,12.2,-9.83383154100001));
#288373=CARTESIAN_POINT('Ctrl Pts',(-5.59186819900006,12.2,-9.83738623200001));
#288374=CARTESIAN_POINT('Ctrl Pts',(-5.59221622500006,12.2,-9.84094583600001));
#288375=CARTESIAN_POINT('Ctrl Pts',(-5.59256194100006,12.2,-9.84451034500001));
#288376=CARTESIAN_POINT('Ctrl Pts',(-5.59290533600006,12.2,-9.84807975100001));
#288377=CARTESIAN_POINT('Ctrl Pts',(-5.59324640500006,12.2,-9.85165405000001));
#288378=CARTESIAN_POINT('Ctrl Pts',(-5.59358514100006,12.2,-9.85523323300001));
#288379=CARTESIAN_POINT('Ctrl Pts',(-5.59392153800006,12.2,-9.85881729400001));
#288380=CARTESIAN_POINT('Ctrl Pts',(-5.59425559000006,12.2,-9.86240622500001));
#288381=CARTESIAN_POINT('Ctrl Pts',(-5.59458728700006,12.2,-9.86600002000001));
#288382=CARTESIAN_POINT('Ctrl Pts',(-5.59491662700006,12.2,-9.86959867100001));
#288383=CARTESIAN_POINT('Ctrl Pts',(-5.59524360000006,12.2,-9.87320217300001));
#288384=CARTESIAN_POINT('Ctrl Pts',(-5.59556820200006,12.2,-9.87681051700001));
#288385=CARTESIAN_POINT('Ctrl Pts',(-5.59589042400006,12.2,-9.88042369800001));
#288386=CARTESIAN_POINT('Ctrl Pts',(-5.59621026000006,12.2,-9.88404170800001));
#288387=CARTESIAN_POINT('Ctrl Pts',(-5.59652770400006,12.2,-9.88766454000001));
#288388=CARTESIAN_POINT('Ctrl Pts',(-5.59684275000006,12.2,-9.89129218700001));
#288389=CARTESIAN_POINT('Ctrl Pts',(-5.59715539100006,12.2,-9.89492464200001));
#288390=CARTESIAN_POINT('Ctrl Pts',(-5.59746562000006,12.2,-9.89856190000001));
#288391=CARTESIAN_POINT('Ctrl Pts',(-5.59777343200006,12.2,-9.90220395300001));
#288392=CARTESIAN_POINT('Ctrl Pts',(-5.59807881900006,12.2,-9.90585079300001));
#288393=CARTESIAN_POINT('Ctrl Pts',(-5.59838177600006,12.2,-9.90950241400001));
#288394=CARTESIAN_POINT('Ctrl Pts',(-5.59868229500006,12.2,-9.91315881000001));
#288395=CARTESIAN_POINT('Ctrl Pts',(-5.59898037100006,12.2,-9.91681997300001));
#288396=CARTESIAN_POINT('Ctrl Pts',(-5.59927599700006,12.2,-9.92048589600001));
#288397=CARTESIAN_POINT('Ctrl Pts',(-5.59956916600005,12.2,-9.92415657400001));
#288398=CARTESIAN_POINT('Ctrl Pts',(-5.59985987300006,12.2,-9.92783199800001));
#288399=CARTESIAN_POINT('Ctrl Pts',(-5.60014811000006,12.2,-9.93151216200001));
#288400=CARTESIAN_POINT('Ctrl Pts',(-5.60043387200006,12.2,-9.93519706000001));
#288401=CARTESIAN_POINT('Ctrl Pts',(-5.60071715300006,12.2,-9.93888668300001));
#288402=CARTESIAN_POINT('Ctrl Pts',(-5.60099794600006,12.2,-9.94258102700002));
#288403=CARTESIAN_POINT('Ctrl Pts',(-5.60127624500006,12.2,-9.94628008400001));
#288404=CARTESIAN_POINT('Ctrl Pts',(-5.60155204400006,12.2,-9.94998384700001));
#288405=CARTESIAN_POINT('Ctrl Pts',(-5.60182533700006,12.2,-9.95369231100001));
#288406=CARTESIAN_POINT('Ctrl Pts',(-5.60209611700006,12.2,-9.95740546800001));
#288407=CARTESIAN_POINT('Ctrl Pts',(-5.60236437800006,12.2,-9.96112330900001));
#288408=CARTESIAN_POINT('Ctrl Pts',(-5.60263011400005,12.2,-9.96484583000001));
#288409=CARTESIAN_POINT('Ctrl Pts',(-5.60289331800006,12.2,-9.96857302300001));
#288410=CARTESIAN_POINT('Ctrl Pts',(-5.60315398400006,12.2,-9.97230488000001));
#288411=CARTESIAN_POINT('Ctrl Pts',(-5.60341210500006,12.2,-9.97604139500002));
#288412=CARTESIAN_POINT('Ctrl Pts',(-5.60366767700006,12.2,-9.97978256300001));
#288413=CARTESIAN_POINT('Ctrl Pts',(-5.60392069300006,12.2,-9.98352837700001));
#288414=CARTESIAN_POINT('Ctrl Pts',(-5.60417114800006,12.2,-9.98727882900001));
#288415=CARTESIAN_POINT('Ctrl Pts',(-5.60441903700006,12.2,-9.99103391600001));
#288416=CARTESIAN_POINT('Ctrl Pts',(-5.60466435400006,12.2,-9.99479363100001));
#288417=CARTESIAN_POINT('Ctrl Pts',(-5.60490709200006,12.2,-9.99855796400001));
#288418=CARTESIAN_POINT('Ctrl Pts',(-5.60514724500006,12.2,-10.002326912));
#288419=CARTESIAN_POINT('Ctrl Pts',(-5.60538480400006,12.2,-10.006100463));
#288420=CARTESIAN_POINT('Ctrl Pts',(-5.60561976300006,12.2,-10.00987861));
#288421=CARTESIAN_POINT('Ctrl Pts',(-5.60585211500006,12.2,-10.013661344));
#288422=CARTESIAN_POINT('Ctrl Pts',(-5.60608185300006,12.2,-10.01744866));
#288423=CARTESIAN_POINT('Ctrl Pts',(-5.60630897000006,12.2,-10.02124055));
#288424=CARTESIAN_POINT('Ctrl Pts',(-5.60653346400006,12.2,-10.025037011));
#288425=CARTESIAN_POINT('Ctrl Pts',(-5.60675533300006,12.2,-10.028838039));
#288426=CARTESIAN_POINT('Ctrl Pts',(-5.60697457300006,12.2,-10.032643631));
#288427=CARTESIAN_POINT('Ctrl Pts',(-5.60714786300006,12.2,-10.035691757));
#288428=CARTESIAN_POINT('Ctrl Pts',(-5.60727664800006,12.2,-10.037979904));
#288429=CARTESIAN_POINT('Ctrl Pts',(-5.60736197900006,12.2,-10.039506249));
#288430=CARTESIAN_POINT('Ctrl Pts',(-5.60740451300005,12.2,-10.040269649));
#288431=CARTESIAN_POINT('Ctrl Pts',(-5.26939701900006,15.2,-10.221714879));
#288432=CARTESIAN_POINT('Ctrl Pts',(-5.26939701900006,11.6,-10.221714879));
#288433=CARTESIAN_POINT('Ctrl Pts',(-5.26878426900006,15.2,-10.221257574));
#288434=CARTESIAN_POINT('Ctrl Pts',(-5.26878426900006,11.6,-10.221257574));
#288435=CARTESIAN_POINT('Ctrl Pts',(-5.26755929400006,15.2,-10.220343));
#288436=CARTESIAN_POINT('Ctrl Pts',(-5.26755929400006,11.6,-10.220343));
#288437=CARTESIAN_POINT('Ctrl Pts',(-5.26572340900006,15.2,-10.218971238));
#288438=CARTESIAN_POINT('Ctrl Pts',(-5.26572340900006,11.6,-10.218971238));
#288439=CARTESIAN_POINT('Ctrl Pts',(-5.26327871600006,15.2,-10.217142421));
#288440=CARTESIAN_POINT('Ctrl Pts',(-5.26327871600006,11.6,-10.217142421));
#288441=CARTESIAN_POINT('Ctrl Pts',(-5.26022810600006,15.2,-10.214856731));
#288442=CARTESIAN_POINT('Ctrl Pts',(-5.26022810600006,11.6,-10.214856731));
#288443=CARTESIAN_POINT('Ctrl Pts',(-5.25718275200005,15.2,-10.212571373));
#288444=CARTESIAN_POINT('Ctrl Pts',(-5.25718275200005,11.6,-10.212571373));
#288445=CARTESIAN_POINT('Ctrl Pts',(-5.25414265600006,15.2,-10.210286352));
#288446=CARTESIAN_POINT('Ctrl Pts',(-5.25414265600006,11.6,-10.210286352));
#288447=CARTESIAN_POINT('Ctrl Pts',(-5.25110781900006,15.2,-10.208001669));
#288448=CARTESIAN_POINT('Ctrl Pts',(-5.25110781900006,11.6,-10.208001669));
#288449=CARTESIAN_POINT('Ctrl Pts',(-5.24807824200006,15.2,-10.20571733));
#288450=CARTESIAN_POINT('Ctrl Pts',(-5.24807824200006,11.6,-10.20571733));
#288451=CARTESIAN_POINT('Ctrl Pts',(-5.24505392700005,15.2,-10.203433345));
#288452=CARTESIAN_POINT('Ctrl Pts',(-5.24505392700005,11.6,-10.203433345));
#288453=CARTESIAN_POINT('Ctrl Pts',(-5.24203487700006,15.2,-10.20114972));
#288454=CARTESIAN_POINT('Ctrl Pts',(-5.24203487700006,11.6,-10.20114972));
#288455=CARTESIAN_POINT('Ctrl Pts',(-5.23902109500006,15.2,-10.198866468));
#288456=CARTESIAN_POINT('Ctrl Pts',(-5.23902109500006,11.6,-10.198866468));
#288457=CARTESIAN_POINT('Ctrl Pts',(-5.23601258300006,15.2,-10.1965836));
#288458=CARTESIAN_POINT('Ctrl Pts',(-5.23601258300006,11.6,-10.1965836));
#288459=CARTESIAN_POINT('Ctrl Pts',(-5.23300934400006,15.2,-10.194301125));
#288460=CARTESIAN_POINT('Ctrl Pts',(-5.23300934400006,11.6,-10.194301125));
#288461=CARTESIAN_POINT('Ctrl Pts',(-5.23001138100006,15.2,-10.192019055));
#288462=CARTESIAN_POINT('Ctrl Pts',(-5.23001138100006,11.6,-10.192019055));
#288463=CARTESIAN_POINT('Ctrl Pts',(-5.22701869500006,15.2,-10.189737398));
#288464=CARTESIAN_POINT('Ctrl Pts',(-5.22701869500006,11.6,-10.189737398));
#288465=CARTESIAN_POINT('Ctrl Pts',(-5.22403128900006,15.2,-10.187456162));
#288466=CARTESIAN_POINT('Ctrl Pts',(-5.22403128900006,11.6,-10.187456162));
#288467=CARTESIAN_POINT('Ctrl Pts',(-5.22104916700005,15.2,-10.185175356));
#288468=CARTESIAN_POINT('Ctrl Pts',(-5.22104916700005,11.6,-10.185175356));
#288469=CARTESIAN_POINT('Ctrl Pts',(-5.21807232800006,15.2,-10.182894987));
#288470=CARTESIAN_POINT('Ctrl Pts',(-5.21807232800006,11.6,-10.182894987));
#288471=CARTESIAN_POINT('Ctrl Pts',(-5.21510077500006,15.2,-10.180615064));
#288472=CARTESIAN_POINT('Ctrl Pts',(-5.21510077500006,11.6,-10.180615064));
#288473=CARTESIAN_POINT('Ctrl Pts',(-5.21213451000006,15.2,-10.178335595));
#288474=CARTESIAN_POINT('Ctrl Pts',(-5.21213451000006,11.6,-10.178335595));
#288475=CARTESIAN_POINT('Ctrl Pts',(-5.20917353600006,15.2,-10.176056588));
#288476=CARTESIAN_POINT('Ctrl Pts',(-5.20917353600006,11.6,-10.176056588));
#288477=CARTESIAN_POINT('Ctrl Pts',(-5.20621785500006,15.2,-10.173778052));
#288478=CARTESIAN_POINT('Ctrl Pts',(-5.20621785500006,11.6,-10.173778052));
#288479=CARTESIAN_POINT('Ctrl Pts',(-5.20326747000006,15.2,-10.171499997));
#288480=CARTESIAN_POINT('Ctrl Pts',(-5.20326747000006,11.6,-10.171499997));
#288481=CARTESIAN_POINT('Ctrl Pts',(-5.20032238000006,15.2,-10.169222432));
#288482=CARTESIAN_POINT('Ctrl Pts',(-5.20032238000006,11.6,-10.169222432));
#288483=CARTESIAN_POINT('Ctrl Pts',(-5.19738259200006,15.2,-10.166945366));
#288484=CARTESIAN_POINT('Ctrl Pts',(-5.19738259200006,11.6,-10.166945366));
#288485=CARTESIAN_POINT('Ctrl Pts',(-5.19444810400006,15.2,-10.164668808));
#288486=CARTESIAN_POINT('Ctrl Pts',(-5.19444810400006,11.6,-10.164668808));
#288487=CARTESIAN_POINT('Ctrl Pts',(-5.19151892100005,15.2,-10.162392768));
#288488=CARTESIAN_POINT('Ctrl Pts',(-5.19151892100005,11.6,-10.162392768));
#288489=CARTESIAN_POINT('Ctrl Pts',(-5.18859504500006,15.2,-10.160117253));
#288490=CARTESIAN_POINT('Ctrl Pts',(-5.18859504500006,11.6,-10.160117253));
#288491=CARTESIAN_POINT('Ctrl Pts',(-5.18567647700006,15.2,-10.157842273));
#288492=CARTESIAN_POINT('Ctrl Pts',(-5.18567647700006,11.6,-10.157842273));
#288493=CARTESIAN_POINT('Ctrl Pts',(-5.18276322000006,15.2,-10.155567837));
#288494=CARTESIAN_POINT('Ctrl Pts',(-5.18276322000006,11.6,-10.155567837));
#288495=CARTESIAN_POINT('Ctrl Pts',(-5.17985527400006,15.2,-10.153293954));
#288496=CARTESIAN_POINT('Ctrl Pts',(-5.17985527400006,11.6,-10.153293954));
#288497=CARTESIAN_POINT('Ctrl Pts',(-5.17695264500006,15.2,-10.151020632));
#288498=CARTESIAN_POINT('Ctrl Pts',(-5.17695264500006,11.6,-10.151020632));
#288499=CARTESIAN_POINT('Ctrl Pts',(-5.17405533300006,15.2,-10.14874788));
#288500=CARTESIAN_POINT('Ctrl Pts',(-5.17405533300006,11.6,-10.14874788));
#288501=CARTESIAN_POINT('Ctrl Pts',(-5.17116333900006,15.2,-10.146475708));
#288502=CARTESIAN_POINT('Ctrl Pts',(-5.17116333900006,11.6,-10.146475708));
#288503=CARTESIAN_POINT('Ctrl Pts',(-5.16827666700006,15.2,-10.144204125));
#288504=CARTESIAN_POINT('Ctrl Pts',(-5.16827666700006,11.6,-10.144204125));
#288505=CARTESIAN_POINT('Ctrl Pts',(-5.16539531900006,15.2,-10.14193314));
#288506=CARTESIAN_POINT('Ctrl Pts',(-5.16539531900006,11.6,-10.14193314));
#288507=CARTESIAN_POINT('Ctrl Pts',(-5.16251929700006,15.2,-10.139662761));
#288508=CARTESIAN_POINT('Ctrl Pts',(-5.16251929700006,11.6,-10.139662761));
#288509=CARTESIAN_POINT('Ctrl Pts',(-5.15964860300006,15.2,-10.137392999));
#288510=CARTESIAN_POINT('Ctrl Pts',(-5.15964860300006,11.6,-10.137392999));
#288511=CARTESIAN_POINT('Ctrl Pts',(-5.15678323800006,15.2,-10.135123862));
#288512=CARTESIAN_POINT('Ctrl Pts',(-5.15678323800006,11.6,-10.135123862));
#288513=CARTESIAN_POINT('Ctrl Pts',(-5.15392320700006,15.2,-10.132855359));
#288514=CARTESIAN_POINT('Ctrl Pts',(-5.15392320700006,11.6,-10.132855359));
#288515=CARTESIAN_POINT('Ctrl Pts',(-5.15106851000006,15.2,-10.130587501));
#288516=CARTESIAN_POINT('Ctrl Pts',(-5.15106851000006,11.6,-10.130587501));
#288517=CARTESIAN_POINT('Ctrl Pts',(-5.14821915000006,15.2,-10.128320294));
#288518=CARTESIAN_POINT('Ctrl Pts',(-5.14821915000006,11.6,-10.128320294));
#288519=CARTESIAN_POINT('Ctrl Pts',(-5.14537512800006,15.2,-10.12605375));
#288520=CARTESIAN_POINT('Ctrl Pts',(-5.14537512800006,11.6,-10.12605375));
#288521=CARTESIAN_POINT('Ctrl Pts',(-5.14253644700006,15.2,-10.123787877));
#288522=CARTESIAN_POINT('Ctrl Pts',(-5.14253644700006,11.6,-10.123787877));
#288523=CARTESIAN_POINT('Ctrl Pts',(-5.13970311000006,15.2,-10.121522683));
#288524=CARTESIAN_POINT('Ctrl Pts',(-5.13970311000006,11.6,-10.121522683));
#288525=CARTESIAN_POINT('Ctrl Pts',(-5.13687511700006,15.2,-10.119258181));
#288526=CARTESIAN_POINT('Ctrl Pts',(-5.13687511700006,11.6,-10.119258181));
#288527=CARTESIAN_POINT('Ctrl Pts',(-5.13405247200006,15.2,-10.116994376));
#288528=CARTESIAN_POINT('Ctrl Pts',(-5.13405247200006,11.6,-10.116994376));
#288529=CARTESIAN_POINT('Ctrl Pts',(-5.13123517700006,15.2,-10.11473128));
#288530=CARTESIAN_POINT('Ctrl Pts',(-5.13123517700006,11.6,-10.11473128));
#288531=CARTESIAN_POINT('Ctrl Pts',(-5.12842323300006,15.2,-10.112468901));
#288532=CARTESIAN_POINT('Ctrl Pts',(-5.12842323300006,11.6,-10.112468901));
#288533=CARTESIAN_POINT('Ctrl Pts',(-5.12561664200006,15.2,-10.11020725));
#288534=CARTESIAN_POINT('Ctrl Pts',(-5.12561664200006,11.6,-10.11020725));
#288535=CARTESIAN_POINT('Ctrl Pts',(-5.12281540700006,15.2,-10.107946335));
#288536=CARTESIAN_POINT('Ctrl Pts',(-5.12281540700006,11.6,-10.107946335));
#288537=CARTESIAN_POINT('Ctrl Pts',(-5.12001953100006,15.2,-10.105686165));
#288538=CARTESIAN_POINT('Ctrl Pts',(-5.12001953100006,11.6,-10.105686165));
#288539=CARTESIAN_POINT('Ctrl Pts',(-5.11722901500006,15.2,-10.10342675));
#288540=CARTESIAN_POINT('Ctrl Pts',(-5.11722901500006,11.6,-10.10342675));
#288541=CARTESIAN_POINT('Ctrl Pts',(-5.11444386000006,15.2,-10.1011681));
#288542=CARTESIAN_POINT('Ctrl Pts',(-5.11444386000006,11.6,-10.1011681));
#288543=CARTESIAN_POINT('Ctrl Pts',(-5.11166407000006,15.2,-10.098910223));
#288544=CARTESIAN_POINT('Ctrl Pts',(-5.11166407000006,11.6,-10.098910223));
#288545=CARTESIAN_POINT('Ctrl Pts',(-5.10888964600006,15.2,-10.09665313));
#288546=CARTESIAN_POINT('Ctrl Pts',(-5.10888964600006,11.6,-10.09665313));
#288547=CARTESIAN_POINT('Ctrl Pts',(-5.10612059000006,15.2,-10.094396829));
#288548=CARTESIAN_POINT('Ctrl Pts',(-5.10612059000006,11.6,-10.094396829));
#288549=CARTESIAN_POINT('Ctrl Pts',(-5.10335690600006,15.2,-10.092141331));
#288550=CARTESIAN_POINT('Ctrl Pts',(-5.10335690600006,11.6,-10.092141331));
#288551=CARTESIAN_POINT('Ctrl Pts',(-5.10059859200005,15.2,-10.089886644));
#288552=CARTESIAN_POINT('Ctrl Pts',(-5.10059859200005,11.6,-10.089886644));
#288553=CARTESIAN_POINT('Ctrl Pts',(-5.09784565500006,15.2,-10.087632779));
#288554=CARTESIAN_POINT('Ctrl Pts',(-5.09784565500006,11.6,-10.087632779));
#288555=CARTESIAN_POINT('Ctrl Pts',(-5.09509809400006,15.2,-10.085379743));
#288556=CARTESIAN_POINT('Ctrl Pts',(-5.09509809400006,11.6,-10.085379743));
#288557=CARTESIAN_POINT('Ctrl Pts',(-5.09235591200006,15.2,-10.083127549));
#288558=CARTESIAN_POINT('Ctrl Pts',(-5.09235591200006,11.6,-10.083127549));
#288559=CARTESIAN_POINT('Ctrl Pts',(-5.08961911100006,15.2,-10.080876204));
#288560=CARTESIAN_POINT('Ctrl Pts',(-5.08961911100006,11.6,-10.080876204));
#288561=CARTESIAN_POINT('Ctrl Pts',(-5.08688769200006,15.2,-10.078625719));
#288562=CARTESIAN_POINT('Ctrl Pts',(-5.08688769200006,11.6,-10.078625719));
#288563=CARTESIAN_POINT('Ctrl Pts',(-5.08416165800006,15.2,-10.076376102));
#288564=CARTESIAN_POINT('Ctrl Pts',(-5.08416165800006,11.6,-10.076376102));
#288565=CARTESIAN_POINT('Ctrl Pts',(-5.08144101200006,15.2,-10.074127365));
#288566=CARTESIAN_POINT('Ctrl Pts',(-5.08144101200006,11.6,-10.074127365));
#288567=CARTESIAN_POINT('Ctrl Pts',(-5.07872575400006,15.2,-10.071879516));
#288568=CARTESIAN_POINT('Ctrl Pts',(-5.07872575400006,11.6,-10.071879516));
#288569=CARTESIAN_POINT('Ctrl Pts',(-5.07601588800005,15.2,-10.069632565));
#288570=CARTESIAN_POINT('Ctrl Pts',(-5.07601588800005,11.6,-10.069632565));
#288571=CARTESIAN_POINT('Ctrl Pts',(-5.07331141500006,15.2,-10.067386522));
#288572=CARTESIAN_POINT('Ctrl Pts',(-5.07331141500006,11.6,-10.067386522));
#288573=CARTESIAN_POINT('Ctrl Pts',(-5.07061233700006,15.2,-10.065141396));
#288574=CARTESIAN_POINT('Ctrl Pts',(-5.07061233700006,11.6,-10.065141396));
#288575=CARTESIAN_POINT('Ctrl Pts',(-5.06791865700006,15.2,-10.062897196));
#288576=CARTESIAN_POINT('Ctrl Pts',(-5.06791865700006,11.6,-10.062897196));
#288577=CARTESIAN_POINT('Ctrl Pts',(-5.06523037500005,15.2,-10.060653935));
#288578=CARTESIAN_POINT('Ctrl Pts',(-5.06523037500005,11.6,-10.060653935));
#288579=CARTESIAN_POINT('Ctrl Pts',(-5.06254749600005,15.2,-10.05841162));
#288580=CARTESIAN_POINT('Ctrl Pts',(-5.06254749600005,11.6,-10.05841162));
#288581=CARTESIAN_POINT('Ctrl Pts',(-5.05987001900006,15.2,-10.05617026));
#288582=CARTESIAN_POINT('Ctrl Pts',(-5.05987001900006,11.6,-10.05617026));
#288583=CARTESIAN_POINT('Ctrl Pts',(-5.05719794700005,15.2,-10.053929867));
#288584=CARTESIAN_POINT('Ctrl Pts',(-5.05719794700005,11.6,-10.053929867));
#288585=CARTESIAN_POINT('Ctrl Pts',(-5.05453128300006,15.2,-10.051690451));
#288586=CARTESIAN_POINT('Ctrl Pts',(-5.05453128300006,11.6,-10.051690451));
#288587=CARTESIAN_POINT('Ctrl Pts',(-5.05187002900006,15.2,-10.049452021));
#288588=CARTESIAN_POINT('Ctrl Pts',(-5.05187002900006,11.6,-10.049452021));
#288589=CARTESIAN_POINT('Ctrl Pts',(-5.04921418500006,15.2,-10.047214585));
#288590=CARTESIAN_POINT('Ctrl Pts',(-5.04921418500006,11.6,-10.047214585));
#288591=CARTESIAN_POINT('Ctrl Pts',(-5.04656375500006,15.2,-10.044978156));
#288592=CARTESIAN_POINT('Ctrl Pts',(-5.04656375500006,11.6,-10.044978156));
#288593=CARTESIAN_POINT('Ctrl Pts',(-5.04391874100006,15.2,-10.042742742));
#288594=CARTESIAN_POINT('Ctrl Pts',(-5.04391874100006,11.6,-10.042742742));
#288595=CARTESIAN_POINT('Ctrl Pts',(-5.04127914400006,15.2,-10.040508355));
#288596=CARTESIAN_POINT('Ctrl Pts',(-5.04127914400006,11.6,-10.040508355));
#288597=CARTESIAN_POINT('Ctrl Pts',(-5.03864496600006,15.2,-10.038275001));
#288598=CARTESIAN_POINT('Ctrl Pts',(-5.03864496600006,11.6,-10.038275001));
#288599=CARTESIAN_POINT('Ctrl Pts',(-5.03601621000006,15.2,-10.036042694));
#288600=CARTESIAN_POINT('Ctrl Pts',(-5.03601621000006,11.6,-10.036042694));
#288601=CARTESIAN_POINT('Ctrl Pts',(-5.03339287600006,15.2,-10.033811442));
#288602=CARTESIAN_POINT('Ctrl Pts',(-5.03339287600006,11.6,-10.033811442));
#288603=CARTESIAN_POINT('Ctrl Pts',(-5.03077496800006,15.2,-10.031581256));
#288604=CARTESIAN_POINT('Ctrl Pts',(-5.03077496800006,11.6,-10.031581256));
#288605=CARTESIAN_POINT('Ctrl Pts',(-5.02816248700006,15.2,-10.029352144));
#288606=CARTESIAN_POINT('Ctrl Pts',(-5.02816248700006,11.6,-10.029352144));
#288607=CARTESIAN_POINT('Ctrl Pts',(-5.02555543600006,15.2,-10.027124119));
#288608=CARTESIAN_POINT('Ctrl Pts',(-5.02555543600006,11.6,-10.027124119));
#288609=CARTESIAN_POINT('Ctrl Pts',(-5.02295381500006,15.2,-10.024897189));
#288610=CARTESIAN_POINT('Ctrl Pts',(-5.02295381500006,11.6,-10.024897189));
#288611=CARTESIAN_POINT('Ctrl Pts',(-5.02035762800006,15.2,-10.022671365));
#288612=CARTESIAN_POINT('Ctrl Pts',(-5.02035762800006,11.6,-10.022671365));
#288613=CARTESIAN_POINT('Ctrl Pts',(-5.01776687500006,15.2,-10.020446656));
#288614=CARTESIAN_POINT('Ctrl Pts',(-5.01776687500006,11.6,-10.020446656));
#288615=CARTESIAN_POINT('Ctrl Pts',(-5.01518156100006,15.2,-10.018223073));
#288616=CARTESIAN_POINT('Ctrl Pts',(-5.01518156100006,11.6,-10.018223073));
#288617=CARTESIAN_POINT('Ctrl Pts',(-5.01260168500006,15.2,-10.016000626));
#288618=CARTESIAN_POINT('Ctrl Pts',(-5.01260168500006,11.6,-10.016000626));
#288619=CARTESIAN_POINT('Ctrl Pts',(-5.01002724900006,15.2,-10.013779325));
#288620=CARTESIAN_POINT('Ctrl Pts',(-5.01002724900006,11.6,-10.013779325));
#288621=CARTESIAN_POINT('Ctrl Pts',(-5.00745825700006,15.2,-10.011559181));
#288622=CARTESIAN_POINT('Ctrl Pts',(-5.00745825700006,11.6,-10.011559181));
#288623=CARTESIAN_POINT('Ctrl Pts',(-5.00489470900006,15.2,-10.009340204));
#288624=CARTESIAN_POINT('Ctrl Pts',(-5.00489470900006,11.6,-10.009340204));
#288625=CARTESIAN_POINT('Ctrl Pts',(-5.00233660800006,15.2,-10.007122403));
#288626=CARTESIAN_POINT('Ctrl Pts',(-5.00233660800006,11.6,-10.007122403));
#288627=CARTESIAN_POINT('Ctrl Pts',(-4.99978395600006,15.2,-10.004905789));
#288628=CARTESIAN_POINT('Ctrl Pts',(-4.99978395600006,11.6,-10.004905789));
#288629=CARTESIAN_POINT('Ctrl Pts',(-4.99723675400006,15.2,-10.002690373));
#288630=CARTESIAN_POINT('Ctrl Pts',(-4.99723675400006,11.6,-10.002690373));
#288631=CARTESIAN_POINT('Ctrl Pts',(-4.99469500400005,15.2,-10.000476165));
#288632=CARTESIAN_POINT('Ctrl Pts',(-4.99469500400005,11.6,-10.000476165));
#288633=CARTESIAN_POINT('Ctrl Pts',(-4.99215870900006,15.2,-9.99826317500001));
#288634=CARTESIAN_POINT('Ctrl Pts',(-4.99215870900006,11.6,-9.99826317500001));
#288635=CARTESIAN_POINT('Ctrl Pts',(-4.98962787100006,15.2,-9.99605141200002));
#288636=CARTESIAN_POINT('Ctrl Pts',(-4.98962787100006,11.6,-9.99605141200002));
#288637=CARTESIAN_POINT('Ctrl Pts',(-4.98710249000006,15.2,-9.99384088900001));
#288638=CARTESIAN_POINT('Ctrl Pts',(-4.98710249000006,11.6,-9.99384088900001));
#288639=CARTESIAN_POINT('Ctrl Pts',(-4.98458257000006,15.2,-9.99163161400001));
#288640=CARTESIAN_POINT('Ctrl Pts',(-4.98458257000006,11.6,-9.99163161400001));
#288641=CARTESIAN_POINT('Ctrl Pts',(-4.98206811000006,15.2,-9.98942360000001));
#288642=CARTESIAN_POINT('Ctrl Pts',(-4.98206811000006,11.6,-9.98942360000001));
#288643=CARTESIAN_POINT('Ctrl Pts',(-4.97955911600005,15.2,-9.98721685500001));
#288644=CARTESIAN_POINT('Ctrl Pts',(-4.97955911600005,11.6,-9.98721685500001));
#288645=CARTESIAN_POINT('Ctrl Pts',(-4.97705558700006,15.2,-9.98501139100001));
#288646=CARTESIAN_POINT('Ctrl Pts',(-4.97705558700006,11.6,-9.98501139100001));
#288647=CARTESIAN_POINT('Ctrl Pts',(-4.97455752500006,15.2,-9.98280721700001));
#288648=CARTESIAN_POINT('Ctrl Pts',(-4.97455752500006,11.6,-9.98280721700001));
#288649=CARTESIAN_POINT('Ctrl Pts',(-4.97206493300006,15.2,-9.98060434500001));
#288650=CARTESIAN_POINT('Ctrl Pts',(-4.97206493300006,11.6,-9.98060434500001));
#288651=CARTESIAN_POINT('Ctrl Pts',(-4.96957781200006,15.2,-9.97840278500002));
#288652=CARTESIAN_POINT('Ctrl Pts',(-4.96957781200006,11.6,-9.97840278500002));
#288653=CARTESIAN_POINT('Ctrl Pts',(-4.96709616400006,15.2,-9.97620254700001));
#288654=CARTESIAN_POINT('Ctrl Pts',(-4.96709616400006,11.6,-9.97620254700001));
#288655=CARTESIAN_POINT('Ctrl Pts',(-4.96461999100006,15.2,-9.97400364200001));
#288656=CARTESIAN_POINT('Ctrl Pts',(-4.96461999100006,11.6,-9.97400364200001));
#288657=CARTESIAN_POINT('Ctrl Pts',(-4.96214929500006,15.2,-9.97180608100001));
#288658=CARTESIAN_POINT('Ctrl Pts',(-4.96214929500006,11.6,-9.97180608100001));
#288659=CARTESIAN_POINT('Ctrl Pts',(-4.95968407800006,15.2,-9.96960987400001));
#288660=CARTESIAN_POINT('Ctrl Pts',(-4.95968407800006,11.6,-9.96960987400001));
#288661=CARTESIAN_POINT('Ctrl Pts',(-4.95722434300006,15.2,-9.96741503200001));
#288662=CARTESIAN_POINT('Ctrl Pts',(-4.95722434300006,11.6,-9.96741503200001));
#288663=CARTESIAN_POINT('Ctrl Pts',(-4.95477008900005,15.2,-9.96522156500001));
#288664=CARTESIAN_POINT('Ctrl Pts',(-4.95477008900005,11.6,-9.96522156500001));
#288665=CARTESIAN_POINT('Ctrl Pts',(-4.95232131800006,15.2,-9.96302948500001));
#288666=CARTESIAN_POINT('Ctrl Pts',(-4.95232131800006,11.6,-9.96302948500001));
#288667=CARTESIAN_POINT('Ctrl Pts',(-4.94987803400006,15.2,-9.96083880100001));
#288668=CARTESIAN_POINT('Ctrl Pts',(-4.94987803400006,11.6,-9.96083880100001));
#288669=CARTESIAN_POINT('Ctrl Pts',(-4.94744023900005,15.2,-9.95864952500001));
#288670=CARTESIAN_POINT('Ctrl Pts',(-4.94744023900005,11.6,-9.95864952500001));
#288671=CARTESIAN_POINT('Ctrl Pts',(-4.94500793300006,15.2,-9.95646166800001));
#288672=CARTESIAN_POINT('Ctrl Pts',(-4.94500793300006,11.6,-9.95646166800001));
#288673=CARTESIAN_POINT('Ctrl Pts',(-4.94258111800006,15.2,-9.95427523900001));
#288674=CARTESIAN_POINT('Ctrl Pts',(-4.94258111800006,11.6,-9.95427523900001));
#288675=CARTESIAN_POINT('Ctrl Pts',(-4.94015979700006,15.2,-9.95209025100001));
#288676=CARTESIAN_POINT('Ctrl Pts',(-4.94015979700006,11.6,-9.95209025100001));
#288677=CARTESIAN_POINT('Ctrl Pts',(-4.93774397100006,15.2,-9.94990671400001));
#288678=CARTESIAN_POINT('Ctrl Pts',(-4.93774397100006,11.6,-9.94990671400001));
#288679=CARTESIAN_POINT('Ctrl Pts',(-4.93533364100006,15.2,-9.94772463800001));
#288680=CARTESIAN_POINT('Ctrl Pts',(-4.93533364100006,11.6,-9.94772463800001));
#288681=CARTESIAN_POINT('Ctrl Pts',(-4.93292881100006,15.2,-9.94554403400001));
#288682=CARTESIAN_POINT('Ctrl Pts',(-4.93292881100006,11.6,-9.94554403400001));
#288683=CARTESIAN_POINT('Ctrl Pts',(-4.93052948000006,15.2,-9.94336491400001));
#288684=CARTESIAN_POINT('Ctrl Pts',(-4.93052948000006,11.6,-9.94336491400001));
#288685=CARTESIAN_POINT('Ctrl Pts',(-4.92813565300006,15.2,-9.94118728700001));
#288686=CARTESIAN_POINT('Ctrl Pts',(-4.92813565300006,11.6,-9.94118728700001));
#288687=CARTESIAN_POINT('Ctrl Pts',(-4.92574732900006,15.2,-9.93901116700001));
#288688=CARTESIAN_POINT('Ctrl Pts',(-4.92574732900006,11.6,-9.93901116700001));
#288689=CARTESIAN_POINT('Ctrl Pts',(-4.92336451200006,15.2,-9.93683656100002));
#288690=CARTESIAN_POINT('Ctrl Pts',(-4.92336451200006,11.6,-9.93683656100002));
#288691=CARTESIAN_POINT('Ctrl Pts',(-4.92098720200006,15.2,-9.93466348400001));
#288692=CARTESIAN_POINT('Ctrl Pts',(-4.92098720200006,11.6,-9.93466348400001));
#288693=CARTESIAN_POINT('Ctrl Pts',(-4.91861540100006,15.2,-9.93249194400001));
#288694=CARTESIAN_POINT('Ctrl Pts',(-4.91861540100006,11.6,-9.93249194400001));
#288695=CARTESIAN_POINT('Ctrl Pts',(-4.91624911200006,15.2,-9.93032195400001));
#288696=CARTESIAN_POINT('Ctrl Pts',(-4.91624911200006,11.6,-9.93032195400001));
#288697=CARTESIAN_POINT('Ctrl Pts',(-4.91388833500006,15.2,-9.92815352500001));
#288698=CARTESIAN_POINT('Ctrl Pts',(-4.91388833500006,11.6,-9.92815352500001));
#288699=CARTESIAN_POINT('Ctrl Pts',(-4.91153307300006,15.2,-9.92598666500001));
#288700=CARTESIAN_POINT('Ctrl Pts',(-4.91153307300006,11.6,-9.92598666500001));
#288701=CARTESIAN_POINT('Ctrl Pts',(-4.90918332700006,15.2,-9.92382138900001));
#288702=CARTESIAN_POINT('Ctrl Pts',(-4.90918332700006,11.6,-9.92382138900001));
#288703=CARTESIAN_POINT('Ctrl Pts',(-4.90683910000006,15.2,-9.92165770600001));
#288704=CARTESIAN_POINT('Ctrl Pts',(-4.90683910000006,11.6,-9.92165770600001));
#288705=CARTESIAN_POINT('Ctrl Pts',(-4.90450039200006,15.2,-9.91949562800001));
#288706=CARTESIAN_POINT('Ctrl Pts',(-4.90450039200006,11.6,-9.91949562800001));
#288707=CARTESIAN_POINT('Ctrl Pts',(-4.90216720600006,15.2,-9.91733516600001));
#288708=CARTESIAN_POINT('Ctrl Pts',(-4.90216720600006,11.6,-9.91733516600001));
#288709=CARTESIAN_POINT('Ctrl Pts',(-4.89983954300006,15.2,-9.91517633000001));
#288710=CARTESIAN_POINT('Ctrl Pts',(-4.89983954300006,11.6,-9.91517633000001));
#288711=CARTESIAN_POINT('Ctrl Pts',(-4.89751740600005,15.2,-9.91301913400001));
#288712=CARTESIAN_POINT('Ctrl Pts',(-4.89751740600005,11.6,-9.91301913400001));
#288713=CARTESIAN_POINT('Ctrl Pts',(-4.89520079400006,15.2,-9.91086358600001));
#288714=CARTESIAN_POINT('Ctrl Pts',(-4.89520079400006,11.6,-9.91086358600001));
#288715=CARTESIAN_POINT('Ctrl Pts',(-4.89288971100006,15.2,-9.90870970000001));
#288716=CARTESIAN_POINT('Ctrl Pts',(-4.89288971100006,11.6,-9.90870970000001));
#288717=CARTESIAN_POINT('Ctrl Pts',(-4.89058415900006,15.2,-9.90655748600001));
#288718=CARTESIAN_POINT('Ctrl Pts',(-4.89058415900006,11.6,-9.90655748600001));
#288719=CARTESIAN_POINT('Ctrl Pts',(-4.88828413900006,15.2,-9.90440695500001));
#288720=CARTESIAN_POINT('Ctrl Pts',(-4.88828413900006,11.6,-9.90440695500001));
#288721=CARTESIAN_POINT('Ctrl Pts',(-4.88598965300006,15.2,-9.90225811900001));
#288722=CARTESIAN_POINT('Ctrl Pts',(-4.88598965300006,11.6,-9.90225811900001));
#288723=CARTESIAN_POINT('Ctrl Pts',(-4.88370070000006,15.2,-9.90011099000001));
#288724=CARTESIAN_POINT('Ctrl Pts',(-4.88370070000006,11.6,-9.90011099000001));
#288725=CARTESIAN_POINT('Ctrl Pts',(-4.88141728600006,15.2,-9.89796557800001));
#288726=CARTESIAN_POINT('Ctrl Pts',(-4.88141728600006,11.6,-9.89796557800001));
#288727=CARTESIAN_POINT('Ctrl Pts',(-4.87913941000006,15.2,-9.89582189400001));
#288728=CARTESIAN_POINT('Ctrl Pts',(-4.87913941000006,11.6,-9.89582189400001));
#288729=CARTESIAN_POINT('Ctrl Pts',(-4.87686707400006,15.2,-9.89367995200001));
#288730=CARTESIAN_POINT('Ctrl Pts',(-4.87686707400006,11.6,-9.89367995200001));
#288731=CARTESIAN_POINT('Ctrl Pts',(-4.87460028000006,15.2,-9.89153976100001));
#288732=CARTESIAN_POINT('Ctrl Pts',(-4.87460028000006,11.6,-9.89153976100001));
#288733=CARTESIAN_POINT('Ctrl Pts',(-4.87233903000006,15.2,-9.88940133400001));
#288734=CARTESIAN_POINT('Ctrl Pts',(-4.87233903000006,11.6,-9.88940133400001));
#288735=CARTESIAN_POINT('Ctrl Pts',(-4.87008332400006,15.2,-9.88726468300001));
#288736=CARTESIAN_POINT('Ctrl Pts',(-4.87008332400006,11.6,-9.88726468300001));
#288737=CARTESIAN_POINT('Ctrl Pts',(-4.86783316600006,15.2,-9.88512981700001));
#288738=CARTESIAN_POINT('Ctrl Pts',(-4.86783316600006,11.6,-9.88512981700001));
#288739=CARTESIAN_POINT('Ctrl Pts',(-4.86558855600006,15.2,-9.88299675100001));
#288740=CARTESIAN_POINT('Ctrl Pts',(-4.86558855600006,11.6,-9.88299675100001));
#288741=CARTESIAN_POINT('Ctrl Pts',(-4.86334949700006,15.2,-9.88086549300001));
#288742=CARTESIAN_POINT('Ctrl Pts',(-4.86334949700006,11.6,-9.88086549300001));
#288743=CARTESIAN_POINT('Ctrl Pts',(-4.86111598900006,15.2,-9.87873605700001));
#288744=CARTESIAN_POINT('Ctrl Pts',(-4.86111598900006,11.6,-9.87873605700001));
#288745=CARTESIAN_POINT('Ctrl Pts',(-4.85888803500006,15.2,-9.87660845400001));
#288746=CARTESIAN_POINT('Ctrl Pts',(-4.85888803500006,11.6,-9.87660845400001));
#288747=CARTESIAN_POINT('Ctrl Pts',(-4.85666563600006,15.2,-9.87448269700001));
#288748=CARTESIAN_POINT('Ctrl Pts',(-4.85666563600006,11.6,-9.87448269700001));
#288749=CARTESIAN_POINT('Ctrl Pts',(-4.85444879300006,15.2,-9.87235879500002));
#288750=CARTESIAN_POINT('Ctrl Pts',(-4.85444879300006,11.6,-9.87235879500002));
#288751=CARTESIAN_POINT('Ctrl Pts',(-4.85223750900006,15.2,-9.87023676200001));
#288752=CARTESIAN_POINT('Ctrl Pts',(-4.85223750900006,11.6,-9.87023676200001));
#288753=CARTESIAN_POINT('Ctrl Pts',(-4.85003178500006,15.2,-9.86811660900001));
#288754=CARTESIAN_POINT('Ctrl Pts',(-4.85003178500006,11.6,-9.86811660900001));
#288755=CARTESIAN_POINT('Ctrl Pts',(-4.84783162200006,15.2,-9.86599834800001));
#288756=CARTESIAN_POINT('Ctrl Pts',(-4.84783162200006,11.6,-9.86599834800001));
#288757=CARTESIAN_POINT('Ctrl Pts',(-4.84563702200006,15.2,-9.86388199100001));
#288758=CARTESIAN_POINT('Ctrl Pts',(-4.84563702200006,11.6,-9.86388199100001));
#288759=CARTESIAN_POINT('Ctrl Pts',(-4.84344798800006,15.2,-9.86176755000001));
#288760=CARTESIAN_POINT('Ctrl Pts',(-4.84344798800006,11.6,-9.86176755000001));
#288761=CARTESIAN_POINT('Ctrl Pts',(-4.84126451900006,15.2,-9.85965503500001));
#288762=CARTESIAN_POINT('Ctrl Pts',(-4.84126451900006,11.6,-9.85965503500001));
#288763=CARTESIAN_POINT('Ctrl Pts',(-4.83908661800006,15.2,-9.85754446000001));
#288764=CARTESIAN_POINT('Ctrl Pts',(-4.83908661800006,11.6,-9.85754446000001));
#288765=CARTESIAN_POINT('Ctrl Pts',(-4.83691428700006,15.2,-9.85543583700001));
#288766=CARTESIAN_POINT('Ctrl Pts',(-4.83691428700006,11.6,-9.85543583700001));
#288767=CARTESIAN_POINT('Ctrl Pts',(-4.83474752500006,15.2,-9.85332917600001));
#288768=CARTESIAN_POINT('Ctrl Pts',(-4.83474752500006,11.6,-9.85332917600001));
#288769=CARTESIAN_POINT('Ctrl Pts',(-4.83258633700006,15.2,-9.85122449100001));
#288770=CARTESIAN_POINT('Ctrl Pts',(-4.83258633700006,11.6,-9.85122449100001));
#288771=CARTESIAN_POINT('Ctrl Pts',(-4.83043072400006,15.2,-9.84912179400001));
#288772=CARTESIAN_POINT('Ctrl Pts',(-4.83043072400006,11.6,-9.84912179400001));
#288773=CARTESIAN_POINT('Ctrl Pts',(-4.82828068600006,15.2,-9.84702109500001));
#288774=CARTESIAN_POINT('Ctrl Pts',(-4.82828068600006,11.6,-9.84702109500001));
#288775=CARTESIAN_POINT('Ctrl Pts',(-4.82613622400006,15.2,-9.84492240900001));
#288776=CARTESIAN_POINT('Ctrl Pts',(-4.82613622400006,11.6,-9.84492240900001));
#288777=CARTESIAN_POINT('Ctrl Pts',(-4.82399734200006,15.2,-9.84282574600002));
#288778=CARTESIAN_POINT('Ctrl Pts',(-4.82399734200006,11.6,-9.84282574600002));
#288779=CARTESIAN_POINT('Ctrl Pts',(-4.82186404000006,15.2,-9.84073111800001));
#288780=CARTESIAN_POINT('Ctrl Pts',(-4.82186404000006,11.6,-9.84073111800001));
#288781=CARTESIAN_POINT('Ctrl Pts',(-4.81973632000006,15.2,-9.83863853800001));
#288782=CARTESIAN_POINT('Ctrl Pts',(-4.81973632000006,11.6,-9.83863853800001));
#288783=CARTESIAN_POINT('Ctrl Pts',(-4.81761418300006,15.2,-9.83654801900001));
#288784=CARTESIAN_POINT('Ctrl Pts',(-4.81761418300006,11.6,-9.83654801900001));
#288785=CARTESIAN_POINT('Ctrl Pts',(-4.81549763100006,15.2,-9.83445957100001));
#288786=CARTESIAN_POINT('Ctrl Pts',(-4.81549763100006,11.6,-9.83445957100001));
#288787=CARTESIAN_POINT('Ctrl Pts',(-4.81338666500006,15.2,-9.83237320800001));
#288788=CARTESIAN_POINT('Ctrl Pts',(-4.81338666500006,11.6,-9.83237320800001));
#288789=CARTESIAN_POINT('Ctrl Pts',(-4.81128128700006,15.2,-9.83028894200001));
#288790=CARTESIAN_POINT('Ctrl Pts',(-4.81128128700006,11.6,-9.83028894200001));
#288791=CARTESIAN_POINT('Ctrl Pts',(-4.80918149800006,15.2,-9.82820678400001));
#288792=CARTESIAN_POINT('Ctrl Pts',(-4.80918149800006,11.6,-9.82820678400001));
#288793=CARTESIAN_POINT('Ctrl Pts',(-4.80708730100006,15.2,-9.82612674900001));
#288794=CARTESIAN_POINT('Ctrl Pts',(-4.80708730100006,11.6,-9.82612674900001));
#288795=CARTESIAN_POINT('Ctrl Pts',(-4.80499869400006,15.2,-9.82404884800001));
#288796=CARTESIAN_POINT('Ctrl Pts',(-4.80499869400006,11.6,-9.82404884800001));
#288797=CARTESIAN_POINT('Ctrl Pts',(-4.80291568400006,15.2,-9.82197309300001));
#288798=CARTESIAN_POINT('Ctrl Pts',(-4.80291568400006,11.6,-9.82197309300001));
#288799=CARTESIAN_POINT('Ctrl Pts',(-4.80083826700006,15.2,-9.81989949600001));
#288800=CARTESIAN_POINT('Ctrl Pts',(-4.80083826700006,11.6,-9.81989949600001));
#288801=CARTESIAN_POINT('Ctrl Pts',(-4.79876644700005,15.2,-9.81782807100001));
#288802=CARTESIAN_POINT('Ctrl Pts',(-4.79876644700005,11.6,-9.81782807100001));
#288803=CARTESIAN_POINT('Ctrl Pts',(-4.79670022500006,15.2,-9.81575882900001));
#288804=CARTESIAN_POINT('Ctrl Pts',(-4.79670022500006,11.6,-9.81575882900001));
#288805=CARTESIAN_POINT('Ctrl Pts',(-4.79463960400006,15.2,-9.81369178300001));
#288806=CARTESIAN_POINT('Ctrl Pts',(-4.79463960400006,11.6,-9.81369178300001));
#288807=CARTESIAN_POINT('Ctrl Pts',(-4.79258458200006,15.2,-9.81162694600001));
#288808=CARTESIAN_POINT('Ctrl Pts',(-4.79258458200006,11.6,-9.81162694600001));
#288809=CARTESIAN_POINT('Ctrl Pts',(-4.79053516300006,15.2,-9.80956433100001));
#288810=CARTESIAN_POINT('Ctrl Pts',(-4.79053516300006,11.6,-9.80956433100001));
#288811=CARTESIAN_POINT('Ctrl Pts',(-4.78849134900006,15.2,-9.80750394900001));
#288812=CARTESIAN_POINT('Ctrl Pts',(-4.78849134900006,11.6,-9.80750394900001));
#288813=CARTESIAN_POINT('Ctrl Pts',(-4.78645314000006,15.2,-9.80544581400001));
#288814=CARTESIAN_POINT('Ctrl Pts',(-4.78645314000006,11.6,-9.80544581400001));
#288815=CARTESIAN_POINT('Ctrl Pts',(-4.78442053800006,15.2,-9.80338993800001));
#288816=CARTESIAN_POINT('Ctrl Pts',(-4.78442053800006,11.6,-9.80338993800001));
#288817=CARTESIAN_POINT('Ctrl Pts',(-4.78239354400006,15.2,-9.80133633400001));
#288818=CARTESIAN_POINT('Ctrl Pts',(-4.78239354400006,11.6,-9.80133633400001));
#288819=CARTESIAN_POINT('Ctrl Pts',(-4.78037215900006,15.2,-9.79928501500001));
#288820=CARTESIAN_POINT('Ctrl Pts',(-4.78037215900006,11.6,-9.79928501500001));
#288821=CARTESIAN_POINT('Ctrl Pts',(-4.77835638600006,15.2,-9.79723599300001));
#288822=CARTESIAN_POINT('Ctrl Pts',(-4.77835638600006,11.6,-9.79723599300001));
#288823=CARTESIAN_POINT('Ctrl Pts',(-4.77634622500006,15.2,-9.79518928200001));
#288824=CARTESIAN_POINT('Ctrl Pts',(-4.77634622500006,11.6,-9.79518928200001));
#288825=CARTESIAN_POINT('Ctrl Pts',(-4.77434167800006,15.2,-9.79314489300001));
#288826=CARTESIAN_POINT('Ctrl Pts',(-4.77434167800006,11.6,-9.79314489300001));
#288827=CARTESIAN_POINT('Ctrl Pts',(-4.77234274700006,15.2,-9.79110284100001));
#288828=CARTESIAN_POINT('Ctrl Pts',(-4.77234274700006,11.6,-9.79110284100001));
#288829=CARTESIAN_POINT('Ctrl Pts',(-4.77034943200006,15.2,-9.78906313800001));
#288830=CARTESIAN_POINT('Ctrl Pts',(-4.77034943200006,11.6,-9.78906313800001));
#288831=CARTESIAN_POINT('Ctrl Pts',(-4.76836173400006,15.2,-9.78702579500001));
#288832=CARTESIAN_POINT('Ctrl Pts',(-4.76836173400006,11.6,-9.78702579500001));
#288833=CARTESIAN_POINT('Ctrl Pts',(-4.76637965600006,15.2,-9.78499082800001));
#288834=CARTESIAN_POINT('Ctrl Pts',(-4.76637965600006,11.6,-9.78499082800001));
#288835=CARTESIAN_POINT('Ctrl Pts',(-4.76440319900005,15.2,-9.78295824900002));
#288836=CARTESIAN_POINT('Ctrl Pts',(-4.76440319900005,11.6,-9.78295824900002));
#288837=CARTESIAN_POINT('Ctrl Pts',(-4.76243236400006,15.2,-9.78092807100001));
#288838=CARTESIAN_POINT('Ctrl Pts',(-4.76243236400006,11.6,-9.78092807100001));
#288839=CARTESIAN_POINT('Ctrl Pts',(-4.76046715200006,15.2,-9.77890030500001));
#288840=CARTESIAN_POINT('Ctrl Pts',(-4.76046715200006,11.6,-9.77890030500001));
#288841=CARTESIAN_POINT('Ctrl Pts',(-4.75850756600006,15.2,-9.77687496700001));
#288842=CARTESIAN_POINT('Ctrl Pts',(-4.75850756600006,11.6,-9.77687496700001));
#288843=CARTESIAN_POINT('Ctrl Pts',(-4.75655360400006,15.2,-9.77485207000001));
#288844=CARTESIAN_POINT('Ctrl Pts',(-4.75655360400006,11.6,-9.77485207000001));
#288845=CARTESIAN_POINT('Ctrl Pts',(-4.75460527100006,15.2,-9.77283162500001));
#288846=CARTESIAN_POINT('Ctrl Pts',(-4.75460527100006,11.6,-9.77283162500001));
#288847=CARTESIAN_POINT('Ctrl Pts',(-4.75266256600006,15.2,-9.77081364600001));
#288848=CARTESIAN_POINT('Ctrl Pts',(-4.75266256600006,11.6,-9.77081364600001));
#288849=CARTESIAN_POINT('Ctrl Pts',(-4.75072549100005,15.2,-9.76879814700001));
#288850=CARTESIAN_POINT('Ctrl Pts',(-4.75072549100005,11.6,-9.76879814700001));
#288851=CARTESIAN_POINT('Ctrl Pts',(-4.74879404800006,15.2,-9.76678514200001));
#288852=CARTESIAN_POINT('Ctrl Pts',(-4.74879404800006,11.6,-9.76678514200001));
#288853=CARTESIAN_POINT('Ctrl Pts',(-4.74686823700006,15.2,-9.76477464200001));
#288854=CARTESIAN_POINT('Ctrl Pts',(-4.74686823700006,11.6,-9.76477464200001));
#288855=CARTESIAN_POINT('Ctrl Pts',(-4.74494806000005,15.2,-9.76276666100001));
#288856=CARTESIAN_POINT('Ctrl Pts',(-4.74494806000005,11.6,-9.76276666100001));
#288857=CARTESIAN_POINT('Ctrl Pts',(-4.74303351900006,15.2,-9.76076121400001));
#288858=CARTESIAN_POINT('Ctrl Pts',(-4.74303351900006,11.6,-9.76076121400001));
#288859=CARTESIAN_POINT('Ctrl Pts',(-4.74112461300006,15.2,-9.75875831300001));
#288860=CARTESIAN_POINT('Ctrl Pts',(-4.74112461300006,11.6,-9.75875831300001));
#288861=CARTESIAN_POINT('Ctrl Pts',(-4.73922134700006,15.2,-9.75675797100001));
#288862=CARTESIAN_POINT('Ctrl Pts',(-4.73922134700006,11.6,-9.75675797100001));
#288863=CARTESIAN_POINT('Ctrl Pts',(-4.73732371800006,15.2,-9.75476020200001));
#288864=CARTESIAN_POINT('Ctrl Pts',(-4.73732371800006,11.6,-9.75476020200001));
#288865=CARTESIAN_POINT('Ctrl Pts',(-4.73543173000006,15.2,-9.75276502000001));
#288866=CARTESIAN_POINT('Ctrl Pts',(-4.73543173000006,11.6,-9.75276502000001));
#288867=CARTESIAN_POINT('Ctrl Pts',(-4.73354538400006,15.2,-9.75077243800001));
#288868=CARTESIAN_POINT('Ctrl Pts',(-4.73354538400006,11.6,-9.75077243800001));
#288869=CARTESIAN_POINT('Ctrl Pts',(-4.73166468000006,15.2,-9.74878247000001));
#288870=CARTESIAN_POINT('Ctrl Pts',(-4.73166468000006,11.6,-9.74878247000001));
#288871=CARTESIAN_POINT('Ctrl Pts',(-4.72978962100005,15.2,-9.74679512800001));
#288872=CARTESIAN_POINT('Ctrl Pts',(-4.72978962100005,11.6,-9.74679512800001));
#288873=CARTESIAN_POINT('Ctrl Pts',(-4.72792020700005,15.2,-9.74481042800001));
#288874=CARTESIAN_POINT('Ctrl Pts',(-4.72792020700005,11.6,-9.74481042800001));
#288875=CARTESIAN_POINT('Ctrl Pts',(-4.72605643800006,15.2,-9.74282838300001));
#288876=CARTESIAN_POINT('Ctrl Pts',(-4.72605643800006,11.6,-9.74282838300001));
#288877=CARTESIAN_POINT('Ctrl Pts',(-4.72419831900006,15.2,-9.74084900500001));
#288878=CARTESIAN_POINT('Ctrl Pts',(-4.72419831900006,11.6,-9.74084900500001));
#288879=CARTESIAN_POINT('Ctrl Pts',(-4.72234584800006,15.2,-9.73887231000001));
#288880=CARTESIAN_POINT('Ctrl Pts',(-4.72234584800006,11.6,-9.73887231000001));
#288881=CARTESIAN_POINT('Ctrl Pts',(-4.72049902600006,15.2,-9.73689831000001));
#288882=CARTESIAN_POINT('Ctrl Pts',(-4.72049902600006,11.6,-9.73689831000001));
#288883=CARTESIAN_POINT('Ctrl Pts',(-4.71865785700006,15.2,-9.73492702100001));
#288884=CARTESIAN_POINT('Ctrl Pts',(-4.71865785700006,11.6,-9.73492702100001));
#288885=CARTESIAN_POINT('Ctrl Pts',(-4.71682234000006,15.2,-9.73295845400001));
#288886=CARTESIAN_POINT('Ctrl Pts',(-4.71682234000006,11.6,-9.73295845400001));
#288887=CARTESIAN_POINT('Ctrl Pts',(-4.71499247600006,15.2,-9.73099262400001));
#288888=CARTESIAN_POINT('Ctrl Pts',(-4.71499247600006,11.6,-9.73099262400001));
#288889=CARTESIAN_POINT('Ctrl Pts',(-4.71316826800006,15.2,-9.72902954600001));
#288890=CARTESIAN_POINT('Ctrl Pts',(-4.71316826800006,11.6,-9.72902954600001));
#288891=CARTESIAN_POINT('Ctrl Pts',(-4.71134971600006,15.2,-9.72706923300001));
#288892=CARTESIAN_POINT('Ctrl Pts',(-4.71134971600006,11.6,-9.72706923300001));
#288893=CARTESIAN_POINT('Ctrl Pts',(-4.70953682100006,15.2,-9.72511169900001));
#288894=CARTESIAN_POINT('Ctrl Pts',(-4.70953682100006,11.6,-9.72511169900001));
#288895=CARTESIAN_POINT('Ctrl Pts',(-4.70772958400006,15.2,-9.72315696000001));
#288896=CARTESIAN_POINT('Ctrl Pts',(-4.70772958400006,11.6,-9.72315696000001));
#288897=CARTESIAN_POINT('Ctrl Pts',(-4.70592800700006,15.2,-9.72120502600001));
#288898=CARTESIAN_POINT('Ctrl Pts',(-4.70592800700006,11.6,-9.72120502600001));
#288899=CARTESIAN_POINT('Ctrl Pts',(-4.70413209100006,15.2,-9.71925591500001));
#288900=CARTESIAN_POINT('Ctrl Pts',(-4.70413209100006,11.6,-9.71925591500001));
#288901=CARTESIAN_POINT('Ctrl Pts',(-4.70234183600006,15.2,-9.71730963800001));
#288902=CARTESIAN_POINT('Ctrl Pts',(-4.70234183600006,11.6,-9.71730963800001));
#288903=CARTESIAN_POINT('Ctrl Pts',(-4.70055724400006,15.2,-9.71536621100001));
#288904=CARTESIAN_POINT('Ctrl Pts',(-4.70055724400006,11.6,-9.71536621100001));
#288905=CARTESIAN_POINT('Ctrl Pts',(-4.69877831600006,15.2,-9.71342564900001));
#288906=CARTESIAN_POINT('Ctrl Pts',(-4.69877831600006,11.6,-9.71342564900001));
#288907=CARTESIAN_POINT('Ctrl Pts',(-4.69700505400006,15.2,-9.71148796400001));
#288908=CARTESIAN_POINT('Ctrl Pts',(-4.69700505400006,11.6,-9.71148796400001));
#288909=CARTESIAN_POINT('Ctrl Pts',(-4.69523745700006,15.2,-9.70955317200001));
#288910=CARTESIAN_POINT('Ctrl Pts',(-4.69523745700006,11.6,-9.70955317200001));
#288911=CARTESIAN_POINT('Ctrl Pts',(-4.69347552900006,15.2,-9.70762128700001));
#288912=CARTESIAN_POINT('Ctrl Pts',(-4.69347552900006,11.6,-9.70762128700001));
#288913=CARTESIAN_POINT('Ctrl Pts',(-4.69171926900006,15.2,-9.70569232300001));
#288914=CARTESIAN_POINT('Ctrl Pts',(-4.69171926900006,11.6,-9.70569232300001));
#288915=CARTESIAN_POINT('Ctrl Pts',(-4.68996867800006,15.2,-9.70376629500001));
#288916=CARTESIAN_POINT('Ctrl Pts',(-4.68996867800006,11.6,-9.70376629500001));
#288917=CARTESIAN_POINT('Ctrl Pts',(-4.68822375800006,15.2,-9.70184321600001));
#288918=CARTESIAN_POINT('Ctrl Pts',(-4.68822375800006,11.6,-9.70184321600001));
#288919=CARTESIAN_POINT('Ctrl Pts',(-4.68648450900006,15.2,-9.69992310200001));
#288920=CARTESIAN_POINT('Ctrl Pts',(-4.68648450900006,11.6,-9.69992310200001));
#288921=CARTESIAN_POINT('Ctrl Pts',(-4.68475093300006,15.2,-9.69800596700001));
#288922=CARTESIAN_POINT('Ctrl Pts',(-4.68475093300006,11.6,-9.69800596700001));
#288923=CARTESIAN_POINT('Ctrl Pts',(-4.68302303100006,15.2,-9.69609182500001));
#288924=CARTESIAN_POINT('Ctrl Pts',(-4.68302303100006,11.6,-9.69609182500001));
#288925=CARTESIAN_POINT('Ctrl Pts',(-4.68130080400006,15.2,-9.69418069300001));
#288926=CARTESIAN_POINT('Ctrl Pts',(-4.68130080400006,11.6,-9.69418069300001));
#288927=CARTESIAN_POINT('Ctrl Pts',(-4.67958425200006,15.2,-9.69227258200001));
#288928=CARTESIAN_POINT('Ctrl Pts',(-4.67958425200006,11.6,-9.69227258200001));
#288929=CARTESIAN_POINT('Ctrl Pts',(-4.67787337700006,15.2,-9.69036751000001));
#288930=CARTESIAN_POINT('Ctrl Pts',(-4.67787337700006,11.6,-9.69036751000001));
#288931=CARTESIAN_POINT('Ctrl Pts',(-4.67616818100006,15.2,-9.68846548900001));
#288932=CARTESIAN_POINT('Ctrl Pts',(-4.67616818100006,11.6,-9.68846548900001));
#288933=CARTESIAN_POINT('Ctrl Pts',(-4.67446866400006,15.2,-9.68656653500001));
#288934=CARTESIAN_POINT('Ctrl Pts',(-4.67446866400006,11.6,-9.68656653500001));
#288935=CARTESIAN_POINT('Ctrl Pts',(-4.67277482600006,15.2,-9.68467066400001));
#288936=CARTESIAN_POINT('Ctrl Pts',(-4.67277482600006,11.6,-9.68467066400001));
#288937=CARTESIAN_POINT('Ctrl Pts',(-4.67108666900006,15.2,-9.68277788900001));
#288938=CARTESIAN_POINT('Ctrl Pts',(-4.67108666900006,11.6,-9.68277788900001));
#288939=CARTESIAN_POINT('Ctrl Pts',(-4.66940419400006,15.2,-9.68088822600001));
#288940=CARTESIAN_POINT('Ctrl Pts',(-4.66940419400006,11.6,-9.68088822600001));
#288941=CARTESIAN_POINT('Ctrl Pts',(-4.66772740200006,15.2,-9.67900168900002));
#288942=CARTESIAN_POINT('Ctrl Pts',(-4.66772740200006,11.6,-9.67900168900002));
#288943=CARTESIAN_POINT('Ctrl Pts',(-4.66605629400005,15.2,-9.67711829300001));
#288944=CARTESIAN_POINT('Ctrl Pts',(-4.66605629400005,11.6,-9.67711829300001));
#288945=CARTESIAN_POINT('Ctrl Pts',(-4.66439087100006,15.2,-9.67523805500001));
#288946=CARTESIAN_POINT('Ctrl Pts',(-4.66439087100006,11.6,-9.67523805500001));
#288947=CARTESIAN_POINT('Ctrl Pts',(-4.66273113300006,15.2,-9.67336098700001));
#288948=CARTESIAN_POINT('Ctrl Pts',(-4.66273113300006,11.6,-9.67336098700001));
#288949=CARTESIAN_POINT('Ctrl Pts',(-4.66107708300005,15.2,-9.67148710700001));
#288950=CARTESIAN_POINT('Ctrl Pts',(-4.66107708300005,11.6,-9.67148710700001));
#288951=CARTESIAN_POINT('Ctrl Pts',(-4.65942871900006,15.2,-9.66961642800001));
#288952=CARTESIAN_POINT('Ctrl Pts',(-4.65942871900006,11.6,-9.66961642800001));
#288953=CARTESIAN_POINT('Ctrl Pts',(-4.65778604600006,15.2,-9.66774896500001));
#288954=CARTESIAN_POINT('Ctrl Pts',(-4.65778604600006,11.6,-9.66774896500001));
#288955=CARTESIAN_POINT('Ctrl Pts',(-4.65614906000006,15.2,-9.66588473600001));
#288956=CARTESIAN_POINT('Ctrl Pts',(-4.65614906000006,11.6,-9.66588473600001));
#288957=CARTESIAN_POINT('Ctrl Pts',(-4.65451776600006,15.2,-9.66402375300001));
#288958=CARTESIAN_POINT('Ctrl Pts',(-4.65451776600006,11.6,-9.66402375300001));
#288959=CARTESIAN_POINT('Ctrl Pts',(-4.65289216200006,15.2,-9.66216603400001));
#288960=CARTESIAN_POINT('Ctrl Pts',(-4.65289216200006,11.6,-9.66216603400001));
#288961=CARTESIAN_POINT('Ctrl Pts',(-4.65127225200006,15.2,-9.66031159200002));
#288962=CARTESIAN_POINT('Ctrl Pts',(-4.65127225200006,11.6,-9.66031159200002));
#288963=CARTESIAN_POINT('Ctrl Pts',(-4.64965803500006,15.2,-9.65846044500001));
#288964=CARTESIAN_POINT('Ctrl Pts',(-4.64965803500006,11.6,-9.65846044500001));
#288965=CARTESIAN_POINT('Ctrl Pts',(-4.64804951100006,15.2,-9.65661260600001));
#288966=CARTESIAN_POINT('Ctrl Pts',(-4.64804951100006,11.6,-9.65661260600001));
#288967=CARTESIAN_POINT('Ctrl Pts',(-4.64644668200005,15.2,-9.65476809100001));
#288968=CARTESIAN_POINT('Ctrl Pts',(-4.64644668200005,11.6,-9.65476809100001));
#288969=CARTESIAN_POINT('Ctrl Pts',(-4.64484955000006,15.2,-9.65292691600001));
#288970=CARTESIAN_POINT('Ctrl Pts',(-4.64484955000006,11.6,-9.65292691600001));
#288971=CARTESIAN_POINT('Ctrl Pts',(-4.64325811300006,15.2,-9.65108909800002));
#288972=CARTESIAN_POINT('Ctrl Pts',(-4.64325811300006,11.6,-9.65108909800002));
#288973=CARTESIAN_POINT('Ctrl Pts',(-4.64167237400006,15.2,-9.64925464900002));
#288974=CARTESIAN_POINT('Ctrl Pts',(-4.64167237400006,11.6,-9.64925464900002));
#288975=CARTESIAN_POINT('Ctrl Pts',(-4.64009233400006,15.2,-9.64742358800001));
#288976=CARTESIAN_POINT('Ctrl Pts',(-4.64009233400006,11.6,-9.64742358800001));
#288977=CARTESIAN_POINT('Ctrl Pts',(-4.63851799300006,15.2,-9.64559593000001));
#288978=CARTESIAN_POINT('Ctrl Pts',(-4.63851799300006,11.6,-9.64559593000001));
#288979=CARTESIAN_POINT('Ctrl Pts',(-4.63694935100006,15.2,-9.64377169000001));
#288980=CARTESIAN_POINT('Ctrl Pts',(-4.63694935100006,11.6,-9.64377169000001));
#288981=CARTESIAN_POINT('Ctrl Pts',(-4.63538641100006,15.2,-9.64195088400002));
#288982=CARTESIAN_POINT('Ctrl Pts',(-4.63538641100006,11.6,-9.64195088400002));
#288983=CARTESIAN_POINT('Ctrl Pts',(-4.63382917200006,15.2,-9.64013352800002));
#288984=CARTESIAN_POINT('Ctrl Pts',(-4.63382917200006,11.6,-9.64013352800002));
#288985=CARTESIAN_POINT('Ctrl Pts',(-4.63227763500006,15.2,-9.63831963700001));
#288986=CARTESIAN_POINT('Ctrl Pts',(-4.63227763500006,11.6,-9.63831963700001));
#288987=CARTESIAN_POINT('Ctrl Pts',(-4.63073180200006,15.2,-9.63650922900002));
#288988=CARTESIAN_POINT('Ctrl Pts',(-4.63073180200006,11.6,-9.63650922900002));
#288989=CARTESIAN_POINT('Ctrl Pts',(-4.62919167300006,15.2,-9.63470231700001));
#288990=CARTESIAN_POINT('Ctrl Pts',(-4.62919167300006,11.6,-9.63470231700001));
#288991=CARTESIAN_POINT('Ctrl Pts',(-4.62765724900006,15.2,-9.63289892000001));
#288992=CARTESIAN_POINT('Ctrl Pts',(-4.62765724900006,11.6,-9.63289892000001));
#288993=CARTESIAN_POINT('Ctrl Pts',(-4.62612853000006,15.2,-9.63109905300002));
#288994=CARTESIAN_POINT('Ctrl Pts',(-4.62612853000006,11.6,-9.63109905300002));
#288995=CARTESIAN_POINT('Ctrl Pts',(-4.62460551700006,15.2,-9.62930273200002));
#288996=CARTESIAN_POINT('Ctrl Pts',(-4.62460551700006,11.6,-9.62930273200002));
#288997=CARTESIAN_POINT('Ctrl Pts',(-4.62308821200006,15.2,-9.62750997300001));
#288998=CARTESIAN_POINT('Ctrl Pts',(-4.62308821200006,11.6,-9.62750997300001));
#288999=CARTESIAN_POINT('Ctrl Pts',(-4.62157661300005,15.2,-9.62572079200001));
#289000=CARTESIAN_POINT('Ctrl Pts',(-4.62157661300005,11.6,-9.62572079200001));
#289001=CARTESIAN_POINT('Ctrl Pts',(-4.62007072500006,15.2,-9.62393520600001));
#289002=CARTESIAN_POINT('Ctrl Pts',(-4.62007072500006,11.6,-9.62393520600001));
#289003=CARTESIAN_POINT('Ctrl Pts',(-4.61857054400006,15.2,-9.62215323100001));
#289004=CARTESIAN_POINT('Ctrl Pts',(-4.61857054400006,11.6,-9.62215323100001));
#289005=CARTESIAN_POINT('Ctrl Pts',(-4.61707607400006,15.2,-9.62037488300002));
#289006=CARTESIAN_POINT('Ctrl Pts',(-4.61707607400006,11.6,-9.62037488300002));
#289007=CARTESIAN_POINT('Ctrl Pts',(-4.61558731500006,15.2,-9.61860017900002));
#289008=CARTESIAN_POINT('Ctrl Pts',(-4.61558731500006,11.6,-9.61860017900002));
#289009=CARTESIAN_POINT('Ctrl Pts',(-4.61410426600006,15.2,-9.61682913500002));
#289010=CARTESIAN_POINT('Ctrl Pts',(-4.61410426600006,11.6,-9.61682913500002));
#289011=CARTESIAN_POINT('Ctrl Pts',(-4.61262692900006,15.2,-9.61506176800001));
#289012=CARTESIAN_POINT('Ctrl Pts',(-4.61262692900006,11.6,-9.61506176800001));
#289013=CARTESIAN_POINT('Ctrl Pts',(-4.61115530500006,15.2,-9.61329809500001));
#289014=CARTESIAN_POINT('Ctrl Pts',(-4.61115530500006,11.6,-9.61329809500001));
#289015=CARTESIAN_POINT('Ctrl Pts',(-4.60968939500006,15.2,-9.61153813100001));
#289016=CARTESIAN_POINT('Ctrl Pts',(-4.60968939500006,11.6,-9.61153813100001));
#289017=CARTESIAN_POINT('Ctrl Pts',(-4.60822919900005,15.2,-9.60978189400001));
#289018=CARTESIAN_POINT('Ctrl Pts',(-4.60822919900005,11.6,-9.60978189400001));
#289019=CARTESIAN_POINT('Ctrl Pts',(-4.60677471800006,15.2,-9.60802939900002));
#289020=CARTESIAN_POINT('Ctrl Pts',(-4.60677471800006,11.6,-9.60802939900002));
#289021=CARTESIAN_POINT('Ctrl Pts',(-4.60532595100006,15.2,-9.60628066500002));
#289022=CARTESIAN_POINT('Ctrl Pts',(-4.60532595100006,11.6,-9.60628066500002));
#289023=CARTESIAN_POINT('Ctrl Pts',(-4.60388290000005,15.2,-9.60453570900001));
#289024=CARTESIAN_POINT('Ctrl Pts',(-4.60388290000005,11.6,-9.60453570900001));
#289025=CARTESIAN_POINT('Ctrl Pts',(-4.60244556700006,15.2,-9.60279454500002));
#289026=CARTESIAN_POINT('Ctrl Pts',(-4.60244556700006,11.6,-9.60279454500002));
#289027=CARTESIAN_POINT('Ctrl Pts',(-4.60101394900006,15.2,-9.60105719300002));
#289028=CARTESIAN_POINT('Ctrl Pts',(-4.60101394900006,11.6,-9.60105719300002));
#289029=CARTESIAN_POINT('Ctrl Pts',(-4.59958805000006,15.2,-9.59932366700002));
#289030=CARTESIAN_POINT('Ctrl Pts',(-4.59958805000006,11.6,-9.59932366700002));
#289031=CARTESIAN_POINT('Ctrl Pts',(-4.59816786800006,15.2,-9.59759398700001));
#289032=CARTESIAN_POINT('Ctrl Pts',(-4.59816786800006,11.6,-9.59759398700001));
#289033=CARTESIAN_POINT('Ctrl Pts',(-4.59675340700006,15.2,-9.59586816800002));
#289034=CARTESIAN_POINT('Ctrl Pts',(-4.59675340700006,11.6,-9.59586816800002));
#289035=CARTESIAN_POINT('Ctrl Pts',(-4.59534466400005,15.2,-9.59414622900002));
#289036=CARTESIAN_POINT('Ctrl Pts',(-4.59534466400005,11.6,-9.59414622900002));
#289037=CARTESIAN_POINT('Ctrl Pts',(-4.59394164100006,15.2,-9.59242818500002));
#289038=CARTESIAN_POINT('Ctrl Pts',(-4.59394164100006,11.6,-9.59242818500002));
#289039=CARTESIAN_POINT('Ctrl Pts',(-4.59254434000006,15.2,-9.59071405400002));
#289040=CARTESIAN_POINT('Ctrl Pts',(-4.59254434000006,11.6,-9.59071405400002));
#289041=CARTESIAN_POINT('Ctrl Pts',(-4.59115275800006,15.2,-9.58900385500002));
#289042=CARTESIAN_POINT('Ctrl Pts',(-4.59115275800006,11.6,-9.58900385500002));
#289043=CARTESIAN_POINT('Ctrl Pts',(-4.58976689900005,15.2,-9.58729760200002));
#289044=CARTESIAN_POINT('Ctrl Pts',(-4.58976689900005,11.6,-9.58729760200002));
#289045=CARTESIAN_POINT('Ctrl Pts',(-4.58838676200005,15.2,-9.58559531600002));
#289046=CARTESIAN_POINT('Ctrl Pts',(-4.58838676200005,11.6,-9.58559531600002));
#289047=CARTESIAN_POINT('Ctrl Pts',(-4.58701234700006,15.2,-9.58389701100002));
#289048=CARTESIAN_POINT('Ctrl Pts',(-4.58701234700006,11.6,-9.58389701100002));
#289049=CARTESIAN_POINT('Ctrl Pts',(-4.58564365600005,15.2,-9.58220270700001));
#289050=CARTESIAN_POINT('Ctrl Pts',(-4.58564365600005,11.6,-9.58220270700001));
#289051=CARTESIAN_POINT('Ctrl Pts',(-4.58428068800006,15.2,-9.58051242200002));
#289052=CARTESIAN_POINT('Ctrl Pts',(-4.58428068800006,11.6,-9.58051242200002));
#289053=CARTESIAN_POINT('Ctrl Pts',(-4.58292344400006,15.2,-9.57882617100001));
#289054=CARTESIAN_POINT('Ctrl Pts',(-4.58292344400006,11.6,-9.57882617100001));
#289055=CARTESIAN_POINT('Ctrl Pts',(-4.58157192500006,15.2,-9.57714397300002));
#289056=CARTESIAN_POINT('Ctrl Pts',(-4.58157192500006,11.6,-9.57714397300002));
#289057=CARTESIAN_POINT('Ctrl Pts',(-4.58022613100006,15.2,-9.57546584700001));
#289058=CARTESIAN_POINT('Ctrl Pts',(-4.58022613100006,11.6,-9.57546584700001));
#289059=CARTESIAN_POINT('Ctrl Pts',(-4.57888606300005,15.2,-9.57379180900002));
#289060=CARTESIAN_POINT('Ctrl Pts',(-4.57888606300005,11.6,-9.57379180900002));
#289061=CARTESIAN_POINT('Ctrl Pts',(-4.57755172000006,15.2,-9.57212187800002));
#289062=CARTESIAN_POINT('Ctrl Pts',(-4.57755172000006,11.6,-9.57212187800002));
#289063=CARTESIAN_POINT('Ctrl Pts',(-4.57622310400006,15.2,-9.57045607000002));
#289064=CARTESIAN_POINT('Ctrl Pts',(-4.57622310400006,11.6,-9.57045607000002));
#289065=CARTESIAN_POINT('Ctrl Pts',(-4.57490021400006,15.2,-9.56879440500002));
#289066=CARTESIAN_POINT('Ctrl Pts',(-4.57490021400006,11.6,-9.56879440500002));
#289067=CARTESIAN_POINT('Ctrl Pts',(-4.57358305300006,15.2,-9.56713690100001));
#289068=CARTESIAN_POINT('Ctrl Pts',(-4.57358305300006,11.6,-9.56713690100001));
#289069=CARTESIAN_POINT('Ctrl Pts',(-4.57227161800006,15.2,-9.56548357500001));
#289070=CARTESIAN_POINT('Ctrl Pts',(-4.57227161800006,11.6,-9.56548357500001));
#289071=CARTESIAN_POINT('Ctrl Pts',(-4.57096591100006,15.2,-9.56383444500002));
#289072=CARTESIAN_POINT('Ctrl Pts',(-4.57096591100006,11.6,-9.56383444500002));
#289073=CARTESIAN_POINT('Ctrl Pts',(-4.56966593300006,15.2,-9.56218953000001));
#289074=CARTESIAN_POINT('Ctrl Pts',(-4.56966593300006,11.6,-9.56218953000001));
#289075=CARTESIAN_POINT('Ctrl Pts',(-4.56837168400006,15.2,-9.56054884700002));
#289076=CARTESIAN_POINT('Ctrl Pts',(-4.56837168400006,11.6,-9.56054884700002));
#289077=CARTESIAN_POINT('Ctrl Pts',(-4.56708316400006,15.2,-9.55891241700002));
#289078=CARTESIAN_POINT('Ctrl Pts',(-4.56708316400006,11.6,-9.55891241700002));
#289079=CARTESIAN_POINT('Ctrl Pts',(-4.56580037200006,15.2,-9.55728025600001));
#289080=CARTESIAN_POINT('Ctrl Pts',(-4.56580037200006,11.6,-9.55728025600001));
#289081=CARTESIAN_POINT('Ctrl Pts',(-4.56452331100006,15.2,-9.55565238200002));
#289082=CARTESIAN_POINT('Ctrl Pts',(-4.56452331100006,11.6,-9.55565238200002));
#289083=CARTESIAN_POINT('Ctrl Pts',(-4.56325198000005,15.2,-9.55402881600002));
#289084=CARTESIAN_POINT('Ctrl Pts',(-4.56325198000005,11.6,-9.55402881600002));
#289085=CARTESIAN_POINT('Ctrl Pts',(-4.56198637900005,15.2,-9.55240957400001));
#289086=CARTESIAN_POINT('Ctrl Pts',(-4.56198637900005,11.6,-9.55240957400001));
#289087=CARTESIAN_POINT('Ctrl Pts',(-4.56072650900006,15.2,-9.55079467600001));
#289088=CARTESIAN_POINT('Ctrl Pts',(-4.56072650900006,11.6,-9.55079467600001));
#289089=CARTESIAN_POINT('Ctrl Pts',(-4.55947237000006,15.2,-9.54918414100002));
#289090=CARTESIAN_POINT('Ctrl Pts',(-4.55947237000006,11.6,-9.54918414100002));
#289091=CARTESIAN_POINT('Ctrl Pts',(-4.55822396200006,15.2,-9.54757798600001));
#289092=CARTESIAN_POINT('Ctrl Pts',(-4.55822396200006,11.6,-9.54757798600001));
#289093=CARTESIAN_POINT('Ctrl Pts',(-4.55698128600006,15.2,-9.54597623200002));
#289094=CARTESIAN_POINT('Ctrl Pts',(-4.55698128600006,11.6,-9.54597623200002));
#289095=CARTESIAN_POINT('Ctrl Pts',(-4.55574434200006,15.2,-9.54437889600002));
#289096=CARTESIAN_POINT('Ctrl Pts',(-4.55574434200006,11.6,-9.54437889600002));
#289097=CARTESIAN_POINT('Ctrl Pts',(-4.55451312900006,15.2,-9.54278599800002));
#289098=CARTESIAN_POINT('Ctrl Pts',(-4.55451312900006,11.6,-9.54278599800002));
#289099=CARTESIAN_POINT('Ctrl Pts',(-4.55328764900006,15.2,-9.54119755600002));
#289100=CARTESIAN_POINT('Ctrl Pts',(-4.55328764900006,11.6,-9.54119755600002));
#289101=CARTESIAN_POINT('Ctrl Pts',(-4.55206790200006,15.2,-9.53961359000001));
#289102=CARTESIAN_POINT('Ctrl Pts',(-4.55206790200006,11.6,-9.53961359000001));
#289103=CARTESIAN_POINT('Ctrl Pts',(-4.55085388600006,15.2,-9.53803412000001));
#289104=CARTESIAN_POINT('Ctrl Pts',(-4.55085388600006,11.6,-9.53803412000001));
#289105=CARTESIAN_POINT('Ctrl Pts',(-4.54964560400006,15.2,-9.53645916200001));
#289106=CARTESIAN_POINT('Ctrl Pts',(-4.54964560400006,11.6,-9.53645916200001));
#289107=CARTESIAN_POINT('Ctrl Pts',(-4.54844305500006,15.2,-9.53488873800002));
#289108=CARTESIAN_POINT('Ctrl Pts',(-4.54844305500006,11.6,-9.53488873800002));
#289109=CARTESIAN_POINT('Ctrl Pts',(-4.54724624000006,15.2,-9.53332286700002));
#289110=CARTESIAN_POINT('Ctrl Pts',(-4.54724624000006,11.6,-9.53332286700002));
#289111=CARTESIAN_POINT('Ctrl Pts',(-4.54605515800006,15.2,-9.53176156700002));
#289112=CARTESIAN_POINT('Ctrl Pts',(-4.54605515800006,11.6,-9.53176156700002));
#289113=CARTESIAN_POINT('Ctrl Pts',(-4.54486980900006,15.2,-9.53020485900002));
#289114=CARTESIAN_POINT('Ctrl Pts',(-4.54486980900006,11.6,-9.53020485900002));
#289115=CARTESIAN_POINT('Ctrl Pts',(-4.54369019500006,15.2,-9.52865276200002));
#289116=CARTESIAN_POINT('Ctrl Pts',(-4.54369019500006,11.6,-9.52865276200002));
#289117=CARTESIAN_POINT('Ctrl Pts',(-4.54251631400005,15.2,-9.52710529400001));
#289118=CARTESIAN_POINT('Ctrl Pts',(-4.54251631400005,11.6,-9.52710529400001));
#289119=CARTESIAN_POINT('Ctrl Pts',(-4.54134816700006,15.2,-9.52556247700001));
#289120=CARTESIAN_POINT('Ctrl Pts',(-4.54134816700006,11.6,-9.52556247700001));
#289121=CARTESIAN_POINT('Ctrl Pts',(-4.54018575500006,15.2,-9.52402433000002));
#289122=CARTESIAN_POINT('Ctrl Pts',(-4.54018575500006,11.6,-9.52402433000002));
#289123=CARTESIAN_POINT('Ctrl Pts',(-4.53902907600006,15.2,-9.52249087200002));
#289124=CARTESIAN_POINT('Ctrl Pts',(-4.53902907600006,11.6,-9.52249087200002));
#289125=CARTESIAN_POINT('Ctrl Pts',(-4.53787813200006,15.2,-9.52096212300001));
#289126=CARTESIAN_POINT('Ctrl Pts',(-4.53787813200006,11.6,-9.52096212300001));
#289127=CARTESIAN_POINT('Ctrl Pts',(-4.53673292200006,15.2,-9.51943810400002));
#289128=CARTESIAN_POINT('Ctrl Pts',(-4.53673292200006,11.6,-9.51943810400002));
#289129=CARTESIAN_POINT('Ctrl Pts',(-4.53559344600006,15.2,-9.51791883400002));
#289130=CARTESIAN_POINT('Ctrl Pts',(-4.53559344600006,11.6,-9.51791883400002));
#289131=CARTESIAN_POINT('Ctrl Pts',(-4.53445970600006,15.2,-9.51640433300001));
#289132=CARTESIAN_POINT('Ctrl Pts',(-4.53445970600006,11.6,-9.51640433300001));
#289133=CARTESIAN_POINT('Ctrl Pts',(-4.53333169900006,15.2,-9.51489462100002));
#289134=CARTESIAN_POINT('Ctrl Pts',(-4.53333169900006,11.6,-9.51489462100002));
#289135=CARTESIAN_POINT('Ctrl Pts',(-4.53220942700006,15.2,-9.51338972000002));
#289136=CARTESIAN_POINT('Ctrl Pts',(-4.53220942700006,11.6,-9.51338972000002));
#289137=CARTESIAN_POINT('Ctrl Pts',(-4.53109289000006,15.2,-9.51188964700002));
#289138=CARTESIAN_POINT('Ctrl Pts',(-4.53109289000006,11.6,-9.51188964700002));
#289139=CARTESIAN_POINT('Ctrl Pts',(-4.52998208700006,15.2,-9.51039442500001));
#289140=CARTESIAN_POINT('Ctrl Pts',(-4.52998208700006,11.6,-9.51039442500001));
#289141=CARTESIAN_POINT('Ctrl Pts',(-4.52887701900006,15.2,-9.50890407300001));
#289142=CARTESIAN_POINT('Ctrl Pts',(-4.52887701900006,11.6,-9.50890407300001));
#289143=CARTESIAN_POINT('Ctrl Pts',(-4.52777768500006,15.2,-9.50741861400001));
#289144=CARTESIAN_POINT('Ctrl Pts',(-4.52777768500006,11.6,-9.50741861400001));
#289145=CARTESIAN_POINT('Ctrl Pts',(-4.52668408500006,15.2,-9.50593806500001));
#289146=CARTESIAN_POINT('Ctrl Pts',(-4.52668408500006,11.6,-9.50593806500001));
#289147=CARTESIAN_POINT('Ctrl Pts',(-4.52559622100006,15.2,-9.50446244800002));
#289148=CARTESIAN_POINT('Ctrl Pts',(-4.52559622100006,11.6,-9.50446244800002));
#289149=CARTESIAN_POINT('Ctrl Pts',(-4.52451409000005,15.2,-9.50299178400002));
#289150=CARTESIAN_POINT('Ctrl Pts',(-4.52451409000005,11.6,-9.50299178400002));
#289151=CARTESIAN_POINT('Ctrl Pts',(-4.52343769400006,15.2,-9.50152609400002));
#289152=CARTESIAN_POINT('Ctrl Pts',(-4.52343769400006,11.6,-9.50152609400002));
#289153=CARTESIAN_POINT('Ctrl Pts',(-4.52236703200006,15.2,-9.50006539900001));
#289154=CARTESIAN_POINT('Ctrl Pts',(-4.52236703200006,11.6,-9.50006539900001));
#289155=CARTESIAN_POINT('Ctrl Pts',(-4.52130210400006,15.2,-9.49860971900002));
#289156=CARTESIAN_POINT('Ctrl Pts',(-4.52130210400006,11.6,-9.49860971900002));
#289157=CARTESIAN_POINT('Ctrl Pts',(-4.52024291000006,15.2,-9.49715907500002));
#289158=CARTESIAN_POINT('Ctrl Pts',(-4.52024291000006,11.6,-9.49715907500002));
#289159=CARTESIAN_POINT('Ctrl Pts',(-4.51918944900005,15.2,-9.49571348900001));
#289160=CARTESIAN_POINT('Ctrl Pts',(-4.51918944900005,11.6,-9.49571348900001));
#289161=CARTESIAN_POINT('Ctrl Pts',(-4.51814172300006,15.2,-9.49427298100002));
#289162=CARTESIAN_POINT('Ctrl Pts',(-4.51814172300006,11.6,-9.49427298100002));
#289163=CARTESIAN_POINT('Ctrl Pts',(-4.51709973000006,15.2,-9.49283757300002));
#289164=CARTESIAN_POINT('Ctrl Pts',(-4.51709973000006,11.6,-9.49283757300002));
#289165=CARTESIAN_POINT('Ctrl Pts',(-4.51606347100006,15.2,-9.49140728700002));
#289166=CARTESIAN_POINT('Ctrl Pts',(-4.51606347100006,11.6,-9.49140728700002));
#289167=CARTESIAN_POINT('Ctrl Pts',(-4.51503294500006,15.2,-9.48998214200002));
#289168=CARTESIAN_POINT('Ctrl Pts',(-4.51503294500006,11.6,-9.48998214200002));
#289169=CARTESIAN_POINT('Ctrl Pts',(-4.51400815100006,15.2,-9.48856216300002));
#289170=CARTESIAN_POINT('Ctrl Pts',(-4.51400815100006,11.6,-9.48856216300002));
#289171=CARTESIAN_POINT('Ctrl Pts',(-4.51298909100006,15.2,-9.48714736800002));
#289172=CARTESIAN_POINT('Ctrl Pts',(-4.51298909100006,11.6,-9.48714736800002));
#289173=CARTESIAN_POINT('Ctrl Pts',(-4.51197576300006,15.2,-9.48573778100002));
#289174=CARTESIAN_POINT('Ctrl Pts',(-4.51197576300006,11.6,-9.48573778100002));
#289175=CARTESIAN_POINT('Ctrl Pts',(-4.51096816800006,15.2,-9.48433342200002));
#289176=CARTESIAN_POINT('Ctrl Pts',(-4.51096816800006,11.6,-9.48433342200002));
#289177=CARTESIAN_POINT('Ctrl Pts',(-4.50996630400006,15.2,-9.48293431400002));
#289178=CARTESIAN_POINT('Ctrl Pts',(-4.50996630400006,11.6,-9.48293431400002));
#289179=CARTESIAN_POINT('Ctrl Pts',(-4.50897017100006,15.2,-9.48154047900001));
#289180=CARTESIAN_POINT('Ctrl Pts',(-4.50897017100006,11.6,-9.48154047900001));
#289181=CARTESIAN_POINT('Ctrl Pts',(-4.50797977200006,15.2,-9.48015193800002));
#289182=CARTESIAN_POINT('Ctrl Pts',(-4.50797977200006,11.6,-9.48015193800002));
#289183=CARTESIAN_POINT('Ctrl Pts',(-4.50699510300006,15.2,-9.47876871300002));
#289184=CARTESIAN_POINT('Ctrl Pts',(-4.50699510300006,11.6,-9.47876871300002));
#289185=CARTESIAN_POINT('Ctrl Pts',(-4.50601616600006,15.2,-9.47739082700001));
#289186=CARTESIAN_POINT('Ctrl Pts',(-4.50601616600006,11.6,-9.47739082700001));
#289187=CARTESIAN_POINT('Ctrl Pts',(-4.50504295800005,15.2,-9.47601830200002));
#289188=CARTESIAN_POINT('Ctrl Pts',(-4.50504295800005,11.6,-9.47601830200002));
#289189=CARTESIAN_POINT('Ctrl Pts',(-4.50407548200006,15.2,-9.47465116000001));
#289190=CARTESIAN_POINT('Ctrl Pts',(-4.50407548200006,11.6,-9.47465116000001));
#289191=CARTESIAN_POINT('Ctrl Pts',(-4.50311373400006,15.2,-9.47328942300001));
#289192=CARTESIAN_POINT('Ctrl Pts',(-4.50311373400006,11.6,-9.47328942300001));
#289193=CARTESIAN_POINT('Ctrl Pts',(-4.50215771700006,15.2,-9.47193311300002));
#289194=CARTESIAN_POINT('Ctrl Pts',(-4.50215771700006,11.6,-9.47193311300002));
#289195=CARTESIAN_POINT('Ctrl Pts',(-4.50120742900006,15.2,-9.47058225500001));
#289196=CARTESIAN_POINT('Ctrl Pts',(-4.50120742900006,11.6,-9.47058225500001));
#289197=CARTESIAN_POINT('Ctrl Pts',(-4.50026286900005,15.2,-9.46923686900002));
#289198=CARTESIAN_POINT('Ctrl Pts',(-4.50026286900005,11.6,-9.46923686900002));
#289199=CARTESIAN_POINT('Ctrl Pts',(-4.49932403800006,15.2,-9.46789697900002));
#289200=CARTESIAN_POINT('Ctrl Pts',(-4.49932403800006,11.6,-9.46789697900002));
#289201=CARTESIAN_POINT('Ctrl Pts',(-4.49839093600006,15.2,-9.46656260700001));
#289202=CARTESIAN_POINT('Ctrl Pts',(-4.49839093600006,11.6,-9.46656260700001));
#289203=CARTESIAN_POINT('Ctrl Pts',(-4.49746356100006,15.2,-9.46523377700002));
#289204=CARTESIAN_POINT('Ctrl Pts',(-4.49746356100006,11.6,-9.46523377700002));
#289205=CARTESIAN_POINT('Ctrl Pts',(-4.49654191300006,15.2,-9.46391051100001));
#289206=CARTESIAN_POINT('Ctrl Pts',(-4.49654191300006,11.6,-9.46391051100001));
#289207=CARTESIAN_POINT('Ctrl Pts',(-4.49562599200005,15.2,-9.46259283300002));
#289208=CARTESIAN_POINT('Ctrl Pts',(-4.49562599200005,11.6,-9.46259283300002));
#289209=CARTESIAN_POINT('Ctrl Pts',(-4.49471579600006,15.2,-9.46128076400001));
#289210=CARTESIAN_POINT('Ctrl Pts',(-4.49471579600006,11.6,-9.46128076400001));
#289211=CARTESIAN_POINT('Ctrl Pts',(-4.49381132700006,15.2,-9.45997433000001));
#289212=CARTESIAN_POINT('Ctrl Pts',(-4.49381132700006,11.6,-9.45997433000001));
#289213=CARTESIAN_POINT('Ctrl Pts',(-4.49291258300006,15.2,-9.45867355200001));
#289214=CARTESIAN_POINT('Ctrl Pts',(-4.49291258300006,11.6,-9.45867355200001));
#289215=CARTESIAN_POINT('Ctrl Pts',(-4.49201956400006,15.2,-9.45737845500001));
#289216=CARTESIAN_POINT('Ctrl Pts',(-4.49201956400006,11.6,-9.45737845500001));
#289217=CARTESIAN_POINT('Ctrl Pts',(-4.49113226700006,15.2,-9.45608906200002));
#289218=CARTESIAN_POINT('Ctrl Pts',(-4.49113226700006,11.6,-9.45608906200002));
#289219=CARTESIAN_POINT('Ctrl Pts',(-4.49025069600006,15.2,-9.45480539600002));
#289220=CARTESIAN_POINT('Ctrl Pts',(-4.49025069600006,11.6,-9.45480539600002));
#289221=CARTESIAN_POINT('Ctrl Pts',(-4.48937484700005,15.2,-9.45352748200002));
#289222=CARTESIAN_POINT('Ctrl Pts',(-4.48937484700005,11.6,-9.45352748200002));
#289223=CARTESIAN_POINT('Ctrl Pts',(-4.48850472100006,15.2,-9.45225534300001));
#289224=CARTESIAN_POINT('Ctrl Pts',(-4.48850472100006,11.6,-9.45225534300001));
#289225=CARTESIAN_POINT('Ctrl Pts',(-4.48764031700006,15.2,-9.45098900300002));
#289226=CARTESIAN_POINT('Ctrl Pts',(-4.48764031700006,11.6,-9.45098900300002));
#289227=CARTESIAN_POINT('Ctrl Pts',(-4.48678163300006,15.2,-9.44972848600001));
#289228=CARTESIAN_POINT('Ctrl Pts',(-4.48678163300006,11.6,-9.44972848600001));
#289229=CARTESIAN_POINT('Ctrl Pts',(-4.48592867100006,15.2,-9.44847381600002));
#289230=CARTESIAN_POINT('Ctrl Pts',(-4.48592867100006,11.6,-9.44847381600002));
#289231=CARTESIAN_POINT('Ctrl Pts',(-4.48508142900006,15.2,-9.44722501600002));
#289232=CARTESIAN_POINT('Ctrl Pts',(-4.48508142900006,11.6,-9.44722501600002));
#289233=CARTESIAN_POINT('Ctrl Pts',(-4.48423990500006,15.2,-9.44598211300002));
#289234=CARTESIAN_POINT('Ctrl Pts',(-4.48423990500006,11.6,-9.44598211300002));
#289235=CARTESIAN_POINT('Ctrl Pts',(-4.48340410100006,15.2,-9.44474512900002));
#289236=CARTESIAN_POINT('Ctrl Pts',(-4.48340410100006,11.6,-9.44474512900002));
#289237=CARTESIAN_POINT('Ctrl Pts',(-4.48257401400006,15.2,-9.44351408900001));
#289238=CARTESIAN_POINT('Ctrl Pts',(-4.48257401400006,11.6,-9.44351408900001));
#289239=CARTESIAN_POINT('Ctrl Pts',(-4.48174964500006,15.2,-9.44228901900001));
#289240=CARTESIAN_POINT('Ctrl Pts',(-4.48174964500006,11.6,-9.44228901900001));
#289241=CARTESIAN_POINT('Ctrl Pts',(-4.48093099200006,15.2,-9.44106994200002));
#289242=CARTESIAN_POINT('Ctrl Pts',(-4.48093099200006,11.6,-9.44106994200002));
#289243=CARTESIAN_POINT('Ctrl Pts',(-4.48011805500006,15.2,-9.43985688200002));
#289244=CARTESIAN_POINT('Ctrl Pts',(-4.48011805500006,11.6,-9.43985688200002));
#289245=CARTESIAN_POINT('Ctrl Pts',(-4.47931083300006,15.2,-9.43864986700002));
#289246=CARTESIAN_POINT('Ctrl Pts',(-4.47931083300006,11.6,-9.43864986700002));
#289247=CARTESIAN_POINT('Ctrl Pts',(-4.47850932400006,15.2,-9.43744891900002));
#289248=CARTESIAN_POINT('Ctrl Pts',(-4.47850932400006,11.6,-9.43744891900002));
#289249=CARTESIAN_POINT('Ctrl Pts',(-4.47771353000006,15.2,-9.43625406500002));
#289250=CARTESIAN_POINT('Ctrl Pts',(-4.47771353000006,11.6,-9.43625406500002));
#289251=CARTESIAN_POINT('Ctrl Pts',(-4.47692344800006,15.2,-9.43506533000001));
#289252=CARTESIAN_POINT('Ctrl Pts',(-4.47692344800006,11.6,-9.43506533000001));
#289253=CARTESIAN_POINT('Ctrl Pts',(-4.47613907800006,15.2,-9.43388273700002));
#289254=CARTESIAN_POINT('Ctrl Pts',(-4.47613907800006,11.6,-9.43388273700002));
#289255=CARTESIAN_POINT('Ctrl Pts',(-4.47536041800006,15.2,-9.43270631400001));
#289256=CARTESIAN_POINT('Ctrl Pts',(-4.47536041800006,11.6,-9.43270631400001));
#289257=CARTESIAN_POINT('Ctrl Pts',(-4.47458747000006,15.2,-9.43153608600002));
#289258=CARTESIAN_POINT('Ctrl Pts',(-4.47458747000006,11.6,-9.43153608600002));
#289259=CARTESIAN_POINT('Ctrl Pts',(-4.47382023000006,15.2,-9.43037207700002));
#289260=CARTESIAN_POINT('Ctrl Pts',(-4.47382023000006,11.6,-9.43037207700002));
#289261=CARTESIAN_POINT('Ctrl Pts',(-4.47305869800006,15.2,-9.42921431400002));
#289262=CARTESIAN_POINT('Ctrl Pts',(-4.47305869800006,11.6,-9.42921431400002));
#289263=CARTESIAN_POINT('Ctrl Pts',(-4.47230287400005,15.2,-9.42806282400002));
#289264=CARTESIAN_POINT('Ctrl Pts',(-4.47230287400005,11.6,-9.42806282400002));
#289265=CARTESIAN_POINT('Ctrl Pts',(-4.47155275700006,15.2,-9.42691763000001));
#289266=CARTESIAN_POINT('Ctrl Pts',(-4.47155275700006,11.6,-9.42691763000001));
#289267=CARTESIAN_POINT('Ctrl Pts',(-4.47080834500006,15.2,-9.42577876000002));
#289268=CARTESIAN_POINT('Ctrl Pts',(-4.47080834500006,11.6,-9.42577876000002));
#289269=CARTESIAN_POINT('Ctrl Pts',(-4.47006963800006,15.2,-9.42464624100002));
#289270=CARTESIAN_POINT('Ctrl Pts',(-4.47006963800006,11.6,-9.42464624100002));
#289271=CARTESIAN_POINT('Ctrl Pts',(-4.46933663400006,15.2,-9.42352009700001));
#289272=CARTESIAN_POINT('Ctrl Pts',(-4.46933663400006,11.6,-9.42352009700001));
#289273=CARTESIAN_POINT('Ctrl Pts',(-4.46860933200006,15.2,-9.42240035600001));
#289274=CARTESIAN_POINT('Ctrl Pts',(-4.46860933200006,11.6,-9.42240035600001));
#289275=CARTESIAN_POINT('Ctrl Pts',(-4.46788773300006,15.2,-9.42128704400002));
#289276=CARTESIAN_POINT('Ctrl Pts',(-4.46788773300006,11.6,-9.42128704400002));
#289277=CARTESIAN_POINT('Ctrl Pts',(-4.46717183400006,15.2,-9.42018018700002));
#289278=CARTESIAN_POINT('Ctrl Pts',(-4.46717183400006,11.6,-9.42018018700002));
#289279=CARTESIAN_POINT('Ctrl Pts',(-4.46646163400006,15.2,-9.41907981300002));
#289280=CARTESIAN_POINT('Ctrl Pts',(-4.46646163400006,11.6,-9.41907981300002));
#289281=CARTESIAN_POINT('Ctrl Pts',(-4.46575713300006,15.2,-9.41798594700002));
#289282=CARTESIAN_POINT('Ctrl Pts',(-4.46575713300006,11.6,-9.41798594700002));
#289283=CARTESIAN_POINT('Ctrl Pts',(-4.46505833000006,15.2,-9.41689861800001));
#289284=CARTESIAN_POINT('Ctrl Pts',(-4.46505833000006,11.6,-9.41689861800001));
#289285=CARTESIAN_POINT('Ctrl Pts',(-4.46436522200006,15.2,-9.41581785200002));
#289286=CARTESIAN_POINT('Ctrl Pts',(-4.46436522200006,11.6,-9.41581785200002));
#289287=CARTESIAN_POINT('Ctrl Pts',(-4.46367781000006,15.2,-9.41474367700001));
#289288=CARTESIAN_POINT('Ctrl Pts',(-4.46367781000006,11.6,-9.41474367700001));
#289289=CARTESIAN_POINT('Ctrl Pts',(-4.46299609100006,15.2,-9.41367611900001));
#289290=CARTESIAN_POINT('Ctrl Pts',(-4.46299609100006,11.6,-9.41367611900001));
#289291=CARTESIAN_POINT('Ctrl Pts',(-4.46232006500006,15.2,-9.41261520700002));
#289292=CARTESIAN_POINT('Ctrl Pts',(-4.46232006500006,11.6,-9.41261520700002));
#289293=CARTESIAN_POINT('Ctrl Pts',(-4.46164973200006,15.2,-9.41156096600002));
#289294=CARTESIAN_POINT('Ctrl Pts',(-4.46164973200006,11.6,-9.41156096600002));
#289295=CARTESIAN_POINT('Ctrl Pts',(-4.46098508800006,15.2,-9.41051342700002));
#289296=CARTESIAN_POINT('Ctrl Pts',(-4.46098508800006,11.6,-9.41051342700002));
#289297=CARTESIAN_POINT('Ctrl Pts',(-4.46032613400006,15.2,-9.40947261400002));
#289298=CARTESIAN_POINT('Ctrl Pts',(-4.46032613400006,11.6,-9.40947261400002));
#289299=CARTESIAN_POINT('Ctrl Pts',(-4.45967286700006,15.2,-9.40843855900001));
#289300=CARTESIAN_POINT('Ctrl Pts',(-4.45967286700006,11.6,-9.40843855900001));
#289301=CARTESIAN_POINT('Ctrl Pts',(-4.45902528800006,15.2,-9.40741128800001));
#289302=CARTESIAN_POINT('Ctrl Pts',(-4.45902528800006,11.6,-9.40741128800001));
#289303=CARTESIAN_POINT('Ctrl Pts',(-4.45838339400006,15.2,-9.40639082900002));
#289304=CARTESIAN_POINT('Ctrl Pts',(-4.45838339400006,11.6,-9.40639082900002));
#289305=CARTESIAN_POINT('Ctrl Pts',(-4.45774718400005,15.2,-9.40537720900002));
#289306=CARTESIAN_POINT('Ctrl Pts',(-4.45774718400005,11.6,-9.40537720900002));
#289307=CARTESIAN_POINT('Ctrl Pts',(-4.45711665600006,15.2,-9.40437046000002));
#289308=CARTESIAN_POINT('Ctrl Pts',(-4.45711665600006,11.6,-9.40437046000002));
#289309=CARTESIAN_POINT('Ctrl Pts',(-4.45649181000006,15.2,-9.40337060700001));
#289310=CARTESIAN_POINT('Ctrl Pts',(-4.45649181000006,11.6,-9.40337060700001));
#289311=CARTESIAN_POINT('Ctrl Pts',(-4.45587264400006,15.2,-9.40237768200002));
#289312=CARTESIAN_POINT('Ctrl Pts',(-4.45587264400006,11.6,-9.40237768200002));
#289313=CARTESIAN_POINT('Ctrl Pts',(-4.45525915700006,15.2,-9.40139171100002));
#289314=CARTESIAN_POINT('Ctrl Pts',(-4.45525915700006,11.6,-9.40139171100002));
#289315=CARTESIAN_POINT('Ctrl Pts',(-4.45465134800005,15.2,-9.40041272500002));
#289316=CARTESIAN_POINT('Ctrl Pts',(-4.45465134800005,11.6,-9.40041272500002));
#289317=CARTESIAN_POINT('Ctrl Pts',(-4.45404921300006,15.2,-9.39944075100002));
#289318=CARTESIAN_POINT('Ctrl Pts',(-4.45404921300006,11.6,-9.39944075100002));
#289319=CARTESIAN_POINT('Ctrl Pts',(-4.45345275400006,15.2,-9.39847582000001));
#289320=CARTESIAN_POINT('Ctrl Pts',(-4.45345275400006,11.6,-9.39847582000001));
#289321=CARTESIAN_POINT('Ctrl Pts',(-4.45286196800006,15.2,-9.39751796000002));
#289322=CARTESIAN_POINT('Ctrl Pts',(-4.45286196800006,11.6,-9.39751796000002));
#289323=CARTESIAN_POINT('Ctrl Pts',(-4.45227685400006,15.2,-9.39656720200002));
#289324=CARTESIAN_POINT('Ctrl Pts',(-4.45227685400006,11.6,-9.39656720200002));
#289325=CARTESIAN_POINT('Ctrl Pts',(-4.45169740800006,15.2,-9.39562357400002));
#289326=CARTESIAN_POINT('Ctrl Pts',(-4.45169740800006,11.6,-9.39562357400002));
#289327=CARTESIAN_POINT('Ctrl Pts',(-4.45112363200006,15.2,-9.39468710800002));
#289328=CARTESIAN_POINT('Ctrl Pts',(-4.45112363200006,11.6,-9.39468710800002));
#289329=CARTESIAN_POINT('Ctrl Pts',(-4.45055552300006,15.2,-9.39375783100001));
#289330=CARTESIAN_POINT('Ctrl Pts',(-4.45055552300006,11.6,-9.39375783100001));
#289331=CARTESIAN_POINT('Ctrl Pts',(-4.44999307900006,15.2,-9.39283577600002));
#289332=CARTESIAN_POINT('Ctrl Pts',(-4.44999307900006,11.6,-9.39283577600002));
#289333=CARTESIAN_POINT('Ctrl Pts',(-4.44943629900005,15.2,-9.39192097100002));
#289334=CARTESIAN_POINT('Ctrl Pts',(-4.44943629900005,11.6,-9.39192097100002));
#289335=CARTESIAN_POINT('Ctrl Pts',(-4.44888518000006,15.2,-9.39101344800001));
#289336=CARTESIAN_POINT('Ctrl Pts',(-4.44888518000006,11.6,-9.39101344800001));
#289337=CARTESIAN_POINT('Ctrl Pts',(-4.44833972300006,15.2,-9.39011323500001));
#289338=CARTESIAN_POINT('Ctrl Pts',(-4.44833972300006,11.6,-9.39011323500001));
#289339=CARTESIAN_POINT('Ctrl Pts',(-4.44779992500006,15.2,-9.38922036500001));
#289340=CARTESIAN_POINT('Ctrl Pts',(-4.44779992500006,11.6,-9.38922036500001));
#289341=CARTESIAN_POINT('Ctrl Pts',(-4.44726578300005,15.2,-9.38833486800002));
#289342=CARTESIAN_POINT('Ctrl Pts',(-4.44726578300005,11.6,-9.38833486800002));
#289343=CARTESIAN_POINT('Ctrl Pts',(-4.44673729800006,15.2,-9.38745677600001));
#289344=CARTESIAN_POINT('Ctrl Pts',(-4.44673729800006,11.6,-9.38745677600001));
#289345=CARTESIAN_POINT('Ctrl Pts',(-4.44621446600006,15.2,-9.38658611800001));
#289346=CARTESIAN_POINT('Ctrl Pts',(-4.44621446600006,11.6,-9.38658611800001));
#289347=CARTESIAN_POINT('Ctrl Pts',(-4.44569728500006,15.2,-9.38572292700002));
#289348=CARTESIAN_POINT('Ctrl Pts',(-4.44569728500006,11.6,-9.38572292700002));
#289349=CARTESIAN_POINT('Ctrl Pts',(-4.44518575600005,15.2,-9.38486723300001));
#289350=CARTESIAN_POINT('Ctrl Pts',(-4.44518575600005,11.6,-9.38486723300001));
#289351=CARTESIAN_POINT('Ctrl Pts',(-4.44467987500006,15.2,-9.38401906800001));
#289352=CARTESIAN_POINT('Ctrl Pts',(-4.44467987500006,11.6,-9.38401906800001));
#289353=CARTESIAN_POINT('Ctrl Pts',(-4.44417964000006,15.2,-9.38317846500002));
#289354=CARTESIAN_POINT('Ctrl Pts',(-4.44417964000006,11.6,-9.38317846500002));
#289355=CARTESIAN_POINT('Ctrl Pts',(-4.44368505200006,15.2,-9.38234545400002));
#289356=CARTESIAN_POINT('Ctrl Pts',(-4.44368505200006,11.6,-9.38234545400002));
#289357=CARTESIAN_POINT('Ctrl Pts',(-4.44319610500005,15.2,-9.38152006800001));
#289358=CARTESIAN_POINT('Ctrl Pts',(-4.44319610500005,11.6,-9.38152006800001));
#289359=CARTESIAN_POINT('Ctrl Pts',(-4.44271280000006,15.2,-9.38070233800002));
#289360=CARTESIAN_POINT('Ctrl Pts',(-4.44271280000006,11.6,-9.38070233800002));
#289361=CARTESIAN_POINT('Ctrl Pts',(-4.44223513400006,15.2,-9.37989229800002));
#289362=CARTESIAN_POINT('Ctrl Pts',(-4.44223513400006,11.6,-9.37989229800002));
#289363=CARTESIAN_POINT('Ctrl Pts',(-4.44176310600006,15.2,-9.37908998100001));
#289364=CARTESIAN_POINT('Ctrl Pts',(-4.44176310600006,11.6,-9.37908998100001));
#289365=CARTESIAN_POINT('Ctrl Pts',(-4.44129939900006,15.2,-9.37829999200002));
#289366=CARTESIAN_POINT('Ctrl Pts',(-4.44129939900006,11.6,-9.37829999200002));
#289367=CARTESIAN_POINT('Ctrl Pts',(-4.44093341100006,15.2,-9.37767505700002));
#289368=CARTESIAN_POINT('Ctrl Pts',(-4.44093341100006,11.6,-9.37767505700002));
#289369=CARTESIAN_POINT('Ctrl Pts',(-4.44066207100006,15.2,-9.37721094100001));
#289370=CARTESIAN_POINT('Ctrl Pts',(-4.44066207100006,11.6,-9.37721094100001));
#289371=CARTESIAN_POINT('Ctrl Pts',(-4.44048314800006,15.2,-9.37690455300002));
#289372=CARTESIAN_POINT('Ctrl Pts',(-4.44048314800006,11.6,-9.37690455300002));
#289373=CARTESIAN_POINT('Ctrl Pts',(-4.44039525800005,15.2,-9.37675396700002));
#289374=CARTESIAN_POINT('Ctrl Pts',(-4.44039525800005,11.6,-9.37675396700002));
#289375=CARTESIAN_POINT('',(-4.44039525809517,12.2,-9.3767539665342));
#289376=CARTESIAN_POINT('',(-4.44039525809517,15.2,-9.3767539665342));
#289377=CARTESIAN_POINT('',(-4.44039525800005,12.2,-9.37675396600002));
#289378=CARTESIAN_POINT('Ctrl Pts',(-5.26939701852072,12.2,-10.2217148786423));
#289379=CARTESIAN_POINT('Ctrl Pts',(-5.26633327357192,12.2,-10.2194283574115));
#289380=CARTESIAN_POINT('Ctrl Pts',(-5.26327740215982,12.2,-10.2171423379557));
#289381=CARTESIAN_POINT('Ctrl Pts',(-5.26022942034972,12.2,-10.2148568142835));
#289382=CARTESIAN_POINT('Ctrl Pts',(-5.25718143853964,12.2,-10.2125712906113));
#289383=CARTESIAN_POINT('Ctrl Pts',(-5.25414134151229,12.2,-10.2102862658399));
#289384=CARTESIAN_POINT('Ctrl Pts',(-5.25110913459507,12.2,-10.2080017554753));
#289385=CARTESIAN_POINT('Ctrl Pts',(-5.24807692767784,12.2,-10.2057172451108));
#289386=CARTESIAN_POINT('Ctrl Pts',(-5.2450526103324,12.2,-10.2034332511482));
#289387=CARTESIAN_POINT('Ctrl Pts',(-5.24203619464925,12.2,-10.2011498137311));
#289388=CARTESIAN_POINT('Ctrl Pts',(-5.23901977841812,12.2,-10.1988663758992));
#289389=CARTESIAN_POINT('Ctrl Pts',(-5.23601126359756,12.2,-10.1965834977174));
#289390=CARTESIAN_POINT('Ctrl Pts',(-5.23301066232921,12.2,-10.1943012257191));
#289391=CARTESIAN_POINT('Ctrl Pts',(-5.23001006160596,12.2,-10.1920189541355));
#289392=CARTESIAN_POINT('Ctrl Pts',(-5.227017373399,12.2,-10.1897372894851));
#289393=CARTESIAN_POINT('Ctrl Pts',(-5.22403260963313,12.2,-10.1874562692347));
#289394=CARTESIAN_POINT('Ctrl Pts',(-5.22104784586726,12.2,-10.1851752489843));
#289395=CARTESIAN_POINT('Ctrl Pts',(-5.21807100570288,12.2,-10.1828948727588));
#289396=CARTESIAN_POINT('Ctrl Pts',(-5.21510209700565,12.2,-10.1806151774979));
#289397=CARTESIAN_POINT('Ctrl Pts',(-5.21114355225578,12.2,-10.1775755839549));
#289398=CARTESIAN_POINT('Ctrl Pts',(-5.20719911047275,12.2,-10.1745371987484));
#289399=CARTESIAN_POINT('Ctrl Pts',(-5.20326879445928,12.2,-10.1715001199966));
#289400=CARTESIAN_POINT('Ctrl Pts',(-5.20032105677979,12.2,-10.1692223104154));
#289401=CARTESIAN_POINT('Ctrl Pts',(-5.1973812652192,12.2,-10.1669452356012));
#289402=CARTESIAN_POINT('Ctrl Pts',(-5.19444942958587,12.2,-10.1646689369788));
#289403=CARTESIAN_POINT('Ctrl Pts',(-5.19151759448515,12.2,-10.1623926387699));
#289404=CARTESIAN_POINT('Ctrl Pts',(-5.18859371667566,12.2,-10.1601171159194));
#289405=CARTESIAN_POINT('Ctrl Pts',(-5.1856778044073,12.2,-10.1578424087521));
#289406=CARTESIAN_POINT('Ctrl Pts',(-5.18276189213894,12.2,-10.1555677015848));
#289407=CARTESIAN_POINT('Ctrl Pts',(-5.17985394462181,12.2,-10.1532938106423));
#289408=CARTESIAN_POINT('Ctrl Pts',(-5.17695397425571,12.2,-10.1510207745063));
#289409=CARTESIAN_POINT('Ctrl Pts',(-5.17405400388961,12.2,-10.1487477383702));
#289410=CARTESIAN_POINT('Ctrl Pts',(-5.1711620077443,12.2,-10.1464755577132));
#289411=CARTESIAN_POINT('Ctrl Pts',(-5.16827799800262,12.2,-10.1442042744937));
#289412=CARTESIAN_POINT('Ctrl Pts',(-5.16539398826094,12.2,-10.1419329912743));
#289413=CARTESIAN_POINT('Ctrl Pts',(-5.16251796474257,12.2,-10.139662604215));
#289414=CARTESIAN_POINT('Ctrl Pts',(-5.15964993559609,12.2,-10.1373931555057));
#289415=CARTESIAN_POINT('Ctrl Pts',(-5.1567819064496,12.2,-10.1351237067964));
#289416=CARTESIAN_POINT('Ctrl Pts',(-5.15392187308588,12.2,-10.1328551959621));
#289417=CARTESIAN_POINT('Ctrl Pts',(-5.15106984485508,12.2,-10.1305876642943));
#289418=CARTESIAN_POINT('Ctrl Pts',(-5.14821781610616,12.2,-10.1283201322146));
#289419=CARTESIAN_POINT('Ctrl Pts',(-5.14537379164283,12.2,-10.1260535792519));
#289420=CARTESIAN_POINT('Ctrl Pts',(-5.14253778235676,12.2,-10.1237880462978));
#289421=CARTESIAN_POINT('Ctrl Pts',(-5.13875643750067,12.2,-10.1207673363783));
#289422=CARTESIAN_POINT('Ctrl Pts',(-5.13498934030452,12.2,-10.1177484413219));
#289423=CARTESIAN_POINT('Ctrl Pts',(-5.13123651476089,12.2,-10.1147314592771));
#289424=CARTESIAN_POINT('Ctrl Pts',(-5.12842189547534,12.2,-10.1124687226407));
#289425=CARTESIAN_POINT('Ctrl Pts',(-5.12561530227086,12.2,-10.1102070631311));
#289426=CARTESIAN_POINT('Ctrl Pts',(-5.12281674703851,12.2,-10.1079465215048));
#289427=CARTESIAN_POINT('Ctrl Pts',(-5.12001819180616,12.2,-10.1056859798785));
#289428=CARTESIAN_POINT('Ctrl Pts',(-5.11722767402325,12.2,-10.1034265563937));
#289429=CARTESIAN_POINT('Ctrl Pts',(-5.11444520183159,12.2,-10.1011682937673));
#289430=CARTESIAN_POINT('Ctrl Pts',(-5.11166272913444,12.2,-10.0989100307306));
#289431=CARTESIAN_POINT('Ctrl Pts',(-5.10888830266455,12.2,-10.0966529282692));
#289432=CARTESIAN_POINT('Ctrl Pts',(-5.10612193234694,12.2,-10.0943970292332));
#289433=CARTESIAN_POINT('Ctrl Pts',(-5.10335556253188,12.2,-10.092141130607));
#289434=CARTESIAN_POINT('Ctrl Pts',(-5.10059724754973,12.2,-10.0898864356391));
#289435=CARTESIAN_POINT('Ctrl Pts',(-5.09784699873369,12.2,-10.0876329860544));
#289436=CARTESIAN_POINT('Ctrl Pts',(-5.09509674991765,12.2,-10.0853795364697));
#289437=CARTESIAN_POINT('Ctrl Pts',(-5.09235456626056,12.2,-10.0831273331097));
#289438=CARTESIAN_POINT('Ctrl Pts',(-5.08962045651418,12.2,-10.080876418973));
#289439=CARTESIAN_POINT('Ctrl Pts',(-5.08688634676781,12.2,-10.0786255048362));
#289440=CARTESIAN_POINT('Ctrl Pts',(-5.08416031078277,12.2,-10.0763758791973));
#289441=CARTESIAN_POINT('Ctrl Pts',(-5.0814423590358,12.2,-10.0741275870187));
#289442=CARTESIAN_POINT('Ctrl Pts',(-5.07872440728883,12.2,-10.0718792948402));
#289443=CARTESIAN_POINT('Ctrl Pts',(-5.07601453924716,12.2,-10.0696323351633));
#289444=CARTESIAN_POINT('Ctrl Pts',(-5.07331276405296,12.2,-10.0673867514948));
#289445=CARTESIAN_POINT('Ctrl Pts',(-5.06971039680015,12.2,-10.0643926396648));
#289446=CARTESIAN_POINT('Ctrl Pts',(-5.0661224169907,12.2,-10.0614009741934));
#289447=CARTESIAN_POINT('Ctrl Pts',(-5.06254884624133,12.2,-10.0584118585307));
#289448=CARTESIAN_POINT('Ctrl Pts',(-5.05986866842275,12.2,-10.0561700219872));
#289449=CARTESIAN_POINT('Ctrl Pts',(-5.05719659431286,12.2,-10.0539296197101));
#289450=CARTESIAN_POINT('Ctrl Pts',(-5.05453263548092,12.2,-10.0516906974896));
#289451=CARTESIAN_POINT('Ctrl Pts',(-5.05186867664897,12.2,-10.0494517752691));
#289452=CARTESIAN_POINT('Ctrl Pts',(-5.04921283078493,12.2,-10.047214330381));
#289453=CARTESIAN_POINT('Ctrl Pts',(-5.04656510899407,12.2,-10.0449784097854));
#289454=CARTESIAN_POINT('Ctrl Pts',(-5.04391738720321,12.2,-10.0427424891898));
#289455=CARTESIAN_POINT('Ctrl Pts',(-5.04127778854206,12.2,-10.0405080924457));
#289456=CARTESIAN_POINT('Ctrl Pts',(-5.03864632176197,12.2,-10.0382752629434));
#289457=CARTESIAN_POINT('Ctrl Pts',(-5.03601485498187,12.2,-10.0360424334411));
#289458=CARTESIAN_POINT('Ctrl Pts',(-5.03339151957621,12.2,-10.0338111730719));
#289459=CARTESIAN_POINT('Ctrl Pts',(-5.03077632533678,12.2,-10.0315815250277));
#289460=CARTESIAN_POINT('Ctrl Pts',(-5.02816113062226,12.2,-10.0293518765785));
#289461=CARTESIAN_POINT('Ctrl Pts',(-5.02555407711005,12.2,-10.027123841488));
#289462=CARTESIAN_POINT('Ctrl Pts',(-5.02295517290011,12.2,-10.024897464998));
#289463=CARTESIAN_POINT('Ctrl Pts',(-5.02035626916231,12.2,-10.0226710889124));
#289464=CARTESIAN_POINT('Ctrl Pts',(-5.01776551501798,12.2,-10.0204463707667));
#289465=CARTESIAN_POINT('Ctrl Pts',(-5.0151829200254,12.2,-10.0182233565699));
#289466=CARTESIAN_POINT('Ctrl Pts',(-5.01260032503283,12.2,-10.0160003423732));
#289467=CARTESIAN_POINT('Ctrl Pts',(-5.01002588752645,12.2,-10.0137790321273));
#289468=CARTESIAN_POINT('Ctrl Pts',(-5.00745961774541,12.2,-10.0115594724998));
#289469=CARTESIAN_POINT('Ctrl Pts',(-5.00489334796437,12.2,-10.0093399128722));
#289470=CARTESIAN_POINT('Ctrl Pts',(-5.00233524529068,12.2,-10.0071221025362));
#289471=CARTESIAN_POINT('Ctrl Pts',(-4.99978531850833,12.2,-10.0049060884917));
#289472=CARTESIAN_POINT('Ctrl Pts',(-4.99723539172598,12.2,-10.0026900744472));
#289473=CARTESIAN_POINT('Ctrl Pts',(-4.99469363983496,12.2,-10.0004758575276));
#289474=CARTESIAN_POINT('Ctrl Pts',(-4.99216007350963,12.2,-9.99826348202451));
#289475=CARTESIAN_POINT('Ctrl Pts',(-4.9896265071843,12.2,-9.9960511065214));
#289476=CARTESIAN_POINT('Ctrl Pts',(-4.98710112537234,12.2,-9.99384057329098));
#289477=CARTESIAN_POINT('Ctrl Pts',(-4.98458393554543,12.2,-9.99163192963567));
#289478=CARTESIAN_POINT('Ctrl Pts',(-4.98206674571852,12.2,-9.98942328598036));
#289479=CARTESIAN_POINT('Ctrl Pts',(-4.97955774950544,12.2,-9.98721653205081));
#289480=CARTESIAN_POINT('Ctrl Pts',(-4.97705695430351,12.2,-9.98501171400565));
#289481=CARTESIAN_POINT('Ctrl Pts',(-4.97288896214887,12.2,-9.98133701713021));
#289482=CARTESIAN_POINT('Ctrl Pts',(-4.96874375134696,12.2,-9.97766769867996));
#289483=CARTESIAN_POINT('Ctrl Pts',(-4.96462136078907,12.2,-9.97400397847075));
#289484=CARTESIAN_POINT('Ctrl Pts',(-4.96132344816302,12.2,-9.97107300214364));
#289485=CARTESIAN_POINT('Ctrl Pts',(-4.95804014295738,12.2,-9.96814560872895));
#289486=CARTESIAN_POINT('Ctrl Pts',(-4.95477145976444,12.2,-9.96522191172301));
#289487=CARTESIAN_POINT('Ctrl Pts',(-4.95150277701685,12.2,-9.96229821511542));
#289488=CARTESIAN_POINT('Ctrl Pts',(-4.94824871974687,12.2,-9.95937821471655));
#289489=CARTESIAN_POINT('Ctrl Pts',(-4.94500930628799,12.2,-9.95646202551013));
#289490=CARTESIAN_POINT('Ctrl Pts',(-4.94176989238772,12.2,-9.95354583590638));
#289491=CARTESIAN_POINT('Ctrl Pts',(-4.93854512263328,12.2,-9.9506334582224));
#289492=CARTESIAN_POINT('Ctrl Pts',(-4.93533501595833,12.2,-9.94772500600833));
#289493=CARTESIAN_POINT('Ctrl Pts',(-4.93212490928337,12.2,-9.94481655379425));
#289494=CARTESIAN_POINT('Ctrl Pts',(-4.92892946581291,12.2,-9.94191202802787));
#289495=CARTESIAN_POINT('Ctrl Pts',(-4.92574870519662,12.2,-9.93901154509243));
#289496=CARTESIAN_POINT('Ctrl Pts',(-4.92256794501371,12.2,-9.93611106255218));
#289497=CARTESIAN_POINT('Ctrl Pts',(-4.91940186695056,12.2,-9.93321462228146));
#289498=CARTESIAN_POINT('Ctrl Pts',(-4.91625049002715,12.2,-9.93032234422697));
#289499=CARTESIAN_POINT('Ctrl Pts',(-4.91309911267437,12.2,-9.92743006577841));
#289500=CARTESIAN_POINT('Ctrl Pts',(-4.90996243593322,12.2,-9.92454194631578));
#289501=CARTESIAN_POINT('Ctrl Pts',(-4.90684047926456,12.2,-9.92165810677015));
#289502=CARTESIAN_POINT('Ctrl Pts',(-4.90371852302128,12.2,-9.91877426761745));
#289503=CARTESIAN_POINT('Ctrl Pts',(-4.90061128645942,12.2,-9.91589470749476));
#289504=CARTESIAN_POINT('Ctrl Pts',(-4.89751878754462,12.2,-9.91301954628508));
#289505=CARTESIAN_POINT('Ctrl Pts',(-4.89365316358509,12.2,-9.90942559447918));
#289506=CARTESIAN_POINT('Ctrl Pts',(-4.88981056848061,12.2,-9.90583851505712));
#289507=CARTESIAN_POINT('Ctrl Pts',(-4.88599103631042,12.2,-9.90225854573528));
#289508=CARTESIAN_POINT('Ctrl Pts',(-4.88293541040773,12.2,-9.89939457012172));
#289509=CARTESIAN_POINT('Ctrl Pts',(-4.8798945456131,12.2,-9.8965351435828));
#289510=CARTESIAN_POINT('Ctrl Pts',(-4.87686845900524,12.2,-9.89368038931658));
#289511=CARTESIAN_POINT('Ctrl Pts',(-4.87384237280968,12.2,-9.89082563543931));
#289512=CARTESIAN_POINT('Ctrl Pts',(-4.87083106485943,12.2,-9.88797555366423));
#289513=CARTESIAN_POINT('Ctrl Pts',(-4.86783455327011,12.2,-9.88513026717431));
#289514=CARTESIAN_POINT('Ctrl Pts',(-4.86483804127251,12.2,-9.88228498029672));
#289515=CARTESIAN_POINT('Ctrl Pts',(-4.86185632551708,12.2,-9.8794444874621));
#289516=CARTESIAN_POINT('Ctrl Pts',(-4.85888942331956,12.2,-9.87660891505523));
#289517=CARTESIAN_POINT('Ctrl Pts',(-4.85592252152629,12.2,-9.8737733430347));
#289518=CARTESIAN_POINT('Ctrl Pts',(-4.85297043309277,12.2,-9.87094269000036));
#289519=CARTESIAN_POINT('Ctrl Pts',(-4.8500331754986,12.2,-9.86811708223104));
#289520=CARTESIAN_POINT('Ctrl Pts',(-4.84709591750422,12.2,-9.86529147407672));
#289521=CARTESIAN_POINT('Ctrl Pts',(-4.84417349063382,12.2,-9.8624709117952));
#289522=CARTESIAN_POINT('Ctrl Pts',(-4.84126591075411,12.2,-9.85965551975322));
#289523=CARTESIAN_POINT('Ctrl Pts',(-4.83835833127056,12.2,-9.85684012809482));
#289524=CARTESIAN_POINT('Ctrl Pts',(-4.83546559825624,12.2,-9.85402990832429));
#289525=CARTESIAN_POINT('Ctrl Pts',(-4.8325877312122,12.2,-9.85122498844193));
#289526=CARTESIAN_POINT('Ctrl Pts',(-4.82970986377605,12.2,-9.84842006817742));
#289527=CARTESIAN_POINT('Ctrl Pts',(-4.82684685973839,12.2,-9.84562044753249));
#289528=CARTESIAN_POINT('Ctrl Pts',(-4.82399873701473,12.2,-9.84282625475642));
#289529=CARTESIAN_POINT('Ctrl Pts',(-4.82115061467911,12.2,-9.84003206236106));
#289530=CARTESIAN_POINT('Ctrl Pts',(-4.81831737290693,12.2,-9.83724329835031));
#289531=CARTESIAN_POINT('Ctrl Pts',(-4.81549902796914,12.2,-9.83446009268838));
#289532=CARTESIAN_POINT('Ctrl Pts',(-4.81268068264735,12.2,-9.83167688664724));
#289533=CARTESIAN_POINT('Ctrl Pts',(-4.80987723444919,12.2,-9.82889923871495));
#289534=CARTESIAN_POINT('Ctrl Pts',(-4.80708869857499,12.2,-9.82612728250832));
#289535=CARTESIAN_POINT('Ctrl Pts',(-4.8043001627008,12.2,-9.8233553263017));
#289536=CARTESIAN_POINT('Ctrl Pts',(-4.80152654065889,12.2,-9.82058905979851));
#289537=CARTESIAN_POINT('Ctrl Pts',(-4.79876784606562,12.2,-9.81782861631532));
#289538=CARTESIAN_POINT('Ctrl Pts',(-4.79600915184822,12.2,-9.81506817320825));
#289539=CARTESIAN_POINT('Ctrl Pts',(-4.79326538591345,12.2,-9.81231355234244));
#289540=CARTESIAN_POINT('Ctrl Pts',(-4.79053656423519,12.2,-9.80956488927686));
#289541=CARTESIAN_POINT('Ctrl Pts',(-4.78780774218513,12.2,-9.80681622583677));
#289542=CARTESIAN_POINT('Ctrl Pts',(-4.78509386508208,12.2,-9.80407351888719));
#289543=CARTESIAN_POINT('Ctrl Pts',(-4.7823949458254,12.2,-9.80133690479422));
#289544=CARTESIAN_POINT('Ctrl Pts',(-4.77969602693645,12.2,-9.7986002910741));
#289545=CARTESIAN_POINT('Ctrl Pts',(-4.77701206720667,12.2,-9.79586976972545));
#289546=CARTESIAN_POINT('Ctrl Pts',(-4.77434308220166,12.2,-9.79314547744776));
#289547=CARTESIAN_POINT('Ctrl Pts',(-4.771674096833,12.2,-9.79042118479888));
#289548=CARTESIAN_POINT('Ctrl Pts',(-4.76902008436373,12.2,-9.78770312084202));
#289549=CARTESIAN_POINT('Ctrl Pts',(-4.76638106086714,12.2,-9.78499142461487));
#289550=CARTESIAN_POINT('Ctrl Pts',(-4.76374203773012,12.2,-9.7822797287572));
#289551=CARTESIAN_POINT('Ctrl Pts',(-4.76111800389278,12.2,-9.77957439923381));
#289552=CARTESIAN_POINT('Ctrl Pts',(-4.75850897227176,12.2,-9.77687557745401));
#289553=CARTESIAN_POINT('Ctrl Pts',(-4.75589994029526,12.2,-9.7741767553065));
#289554=CARTESIAN_POINT('Ctrl Pts',(-4.7533059108011,12.2,-9.77148443834587));
#289555=CARTESIAN_POINT('Ctrl Pts',(-4.75072689877264,12.2,-9.7687987702555));
#289556=CARTESIAN_POINT('Ctrl Pts',(-4.74750313391277,12.2,-9.7654416853255));
#289557=CARTESIAN_POINT('Ctrl Pts',(-4.74430283258282,12.2,-9.76209498649535));
#289558=CARTESIAN_POINT('Ctrl Pts',(-4.74112602256463,12.2,-9.75875895237109));
#289559=CARTESIAN_POINT('Ctrl Pts',(-4.73858457475785,12.2,-9.75609012528987));
#289560=CARTESIAN_POINT('Ctrl Pts',(-4.73605816102612,12.2,-9.75342812337273));
#289561=CARTESIAN_POINT('Ctrl Pts',(-4.73354679473044,12.2,-9.75077309170043));
#289562=CARTESIAN_POINT('Ctrl Pts',(-4.73103542809259,12.2,-9.74811805966639));
#289563=CARTESIAN_POINT('Ctrl Pts',(-4.72853910887321,12.2,-9.74546999682206));
#289564=CARTESIAN_POINT('Ctrl Pts',(-4.72605785023896,12.2,-9.74282904956749));
#289565=CARTESIAN_POINT('Ctrl Pts',(-4.72357659194279,12.2,-9.74018810267274));
#289566=CARTESIAN_POINT('Ctrl Pts',(-4.72111039429581,12.2,-9.73755427105384));
#289567=CARTESIAN_POINT('Ctrl Pts',(-4.71865927037242,12.2,-9.73492770191449));
#289568=CARTESIAN_POINT('Ctrl Pts',(-4.71620814611507,12.2,-9.73230113241728));
#289569=CARTESIAN_POINT('Ctrl Pts',(-4.71377209473874,12.2,-9.72968182402841));
#289570=CARTESIAN_POINT('Ctrl Pts',(-4.71135113005222,12.2,-9.7270699275532));
#289571=CARTESIAN_POINT('Ctrl Pts',(-4.70893016569556,12.2,-9.72445803143386));
#289572=CARTESIAN_POINT('Ctrl Pts',(-4.70652428701922,12.2,-9.72185354758805));
#289573=CARTESIAN_POINT('Ctrl Pts',(-4.70413350665756,12.2,-9.71925662396625));
#289574=CARTESIAN_POINT('Ctrl Pts',(-4.70174272597016,12.2,-9.71665969999061));
#289575=CARTESIAN_POINT('Ctrl Pts',(-4.69936704292938,12.2,-9.71407033705063));
#289576=CARTESIAN_POINT('Ctrl Pts',(-4.69700647029006,12.2,-9.71148868723156));
#289577=CARTESIAN_POINT('Ctrl Pts',(-4.69464589797236,12.2,-9.70890703776424));
#289578=CARTESIAN_POINT('Ctrl Pts',(-4.69230043648095,12.2,-9.70633310220778));
#289579=CARTESIAN_POINT('Ctrl Pts',(-4.68997009611436,12.2,-9.70376703269454));
#289580=CARTESIAN_POINT('Ctrl Pts',(-4.68763975543026,12.2,-9.70120096283167));
#289581=CARTESIAN_POINT('Ctrl Pts',(-4.68532453581146,12.2,-9.69864275870007));
#289582=CARTESIAN_POINT('Ctrl Pts',(-4.68302444974166,12.2,-9.69609257744998));
#289583=CARTESIAN_POINT('Ctrl Pts',(-4.68072436367186,12.2,-9.69354239619989));
#289584=CARTESIAN_POINT('Ctrl Pts',(-4.67843940916771,12.2,-9.69100023702849));
#289585=CARTESIAN_POINT('Ctrl Pts',(-4.67616960037889,12.2,-9.68846625533568));
#289586=CARTESIAN_POINT('Ctrl Pts',(-4.67389979189934,12.2,-9.68593227398813));
#289587=CARTESIAN_POINT('Ctrl Pts',(-4.67164512580088,12.2,-9.68340647237124));
#289588=CARTESIAN_POINT('Ctrl Pts',(-4.66940561475152,12.2,-9.68088900751003));
#289589=CARTESIAN_POINT('Ctrl Pts',(-4.66716610339703,12.2,-9.67837154230581));
#289590=CARTESIAN_POINT('Ctrl Pts',(-4.66494174666043,12.2,-9.67586241396267));
#289591=CARTESIAN_POINT('Ctrl Pts',(-4.66273255459713,12.2,-9.67336178354946));
#289592=CARTESIAN_POINT('Ctrl Pts',(-4.65997106466851,12.2,-9.67023599570333));
#289593=CARTESIAN_POINT('Ctrl Pts',(-4.65723326972084,12.2,-9.66712348473242));
#289594=CARTESIAN_POINT('Ctrl Pts',(-4.654519188195,12.2,-9.66402456855298));
#289595=CARTESIAN_POINT('Ctrl Pts',(-4.651805106965,12.2,-9.66092565271133));
#289596=CARTESIAN_POINT('Ctrl Pts',(-4.64911474044341,12.2,-9.65784033211808));
#289597=CARTESIAN_POINT('Ctrl Pts',(-4.64644810656547,12.2,-9.65476892641006));
#289598=CARTESIAN_POINT('Ctrl Pts',(-4.64378147239686,12.2,-9.65169752036726));
#289599=CARTESIAN_POINT('Ctrl Pts',(-4.64113857041119,12.2,-9.64864003108809));
#289600=CARTESIAN_POINT('Ctrl Pts',(-4.63851941811759,12.2,-9.64559678490637));
#289601=CARTESIAN_POINT('Ctrl Pts',(-4.63590026582398,12.2,-9.64255353872465));
#289602=CARTESIAN_POINT('Ctrl Pts',(-4.6333048632772,12.2,-9.63952453455656));
#289603=CARTESIAN_POINT('Ctrl Pts',(-4.63073322834471,12.2,-9.63651010344427));
#289604=CARTESIAN_POINT('Ctrl Pts',(-4.62764726625754,12.2,-9.63289278591239));
#289605=CARTESIAN_POINT('Ctrl Pts',(-4.62459552761305,12.2,-9.62929645501804));
#289606=CARTESIAN_POINT('Ctrl Pts',(-4.62157804038318,12.2,-9.62572169039588));
#289607=CARTESIAN_POINT('Ctrl Pts',(-4.61906346782865,12.2,-9.62274272003977));
#289608=CARTESIAN_POINT('Ctrl Pts',(-4.61657268179206,12.2,-9.61977872733529));
#289609=CARTESIAN_POINT('Ctrl Pts',(-4.61410569366899,12.2,-9.61683005386429));
#289610=CARTESIAN_POINT('Ctrl Pts',(-4.61163870554591,12.2,-9.6138813803933));
#289611=CARTESIAN_POINT('Ctrl Pts',(-4.60919551947046,12.2,-9.6109480271837));
#289612=CARTESIAN_POINT('Ctrl Pts',(-4.60677614620855,12.2,-9.60803033885168));
#289613=CARTESIAN_POINT('Ctrl Pts',(-4.60435677321034,12.2,-9.60511265083768));
#289614=CARTESIAN_POINT('Ctrl Pts',(-4.60196121338143,12.2,-9.60221063109198));
#289615=CARTESIAN_POINT('Ctrl Pts',(-4.59958947961023,12.2,-9.5993246288358));
#289616=CARTESIAN_POINT('Ctrl Pts',(-4.59721774558051,12.2,-9.59643862626505));
#289617=CARTESIAN_POINT('Ctrl Pts',(-4.59486983921152,12.2,-9.5935686433746));
#289618=CARTESIAN_POINT('Ctrl Pts',(-4.59254577011232,12.2,-9.59071503733156));
#289619=CARTESIAN_POINT('Ctrl Pts',(-4.59022170101313,12.2,-9.58786143128853));
#289620=CARTESIAN_POINT('Ctrl Pts',(-4.58792146964639,12.2,-9.58502420073619));
#289621=CARTESIAN_POINT('Ctrl Pts',(-4.585645087031,12.2,-9.58220371205245));
#289622=CARTESIAN_POINT('Ctrl Pts',(-4.58336870441562,12.2,-9.57938322336871));
#289623=CARTESIAN_POINT('Ctrl Pts',(-4.58111617018602,12.2,-9.57657947431099));
#289624=CARTESIAN_POINT('Ctrl Pts',(-4.5788874944209,12.2,-9.57379283590732));
#289625=CARTESIAN_POINT('Ctrl Pts',(-4.57665881865576,12.2,-9.57100619750366));
#289626=CARTESIAN_POINT('Ctrl Pts',(-4.57445400159402,12.2,-9.56823666828653));
#289627=CARTESIAN_POINT('Ctrl Pts',(-4.57227305013444,12.2,-9.56548462418839));
#289628=CARTESIAN_POINT('Ctrl Pts',(-4.57009209867486,12.2,-9.56273258009026));
#289629=CARTESIAN_POINT('Ctrl Pts',(-4.56793501542203,12.2,-9.55999802091383));
#289630=CARTESIAN_POINT('Ctrl Pts',(-4.56580180471783,12.2,-9.55728132777645));
#289631=CARTESIAN_POINT('Ctrl Pts',(-4.56366859401363,12.2,-9.55456463463907));
#289632=CARTESIAN_POINT('Ctrl Pts',(-4.5615592585222,12.2,-9.55186580839441));
#289633=CARTESIAN_POINT('Ctrl Pts',(-4.55947380275833,12.2,-9.5491852360333));
#289634=CARTESIAN_POINT('Ctrl Pts',(-4.55738834699444,12.2,-9.54650466367219));
#289635=CARTESIAN_POINT('Ctrl Pts',(-4.55532677154696,12.2,-9.54384234556603));
#289636=CARTESIAN_POINT('Ctrl Pts',(-4.55328908223222,12.2,-9.54119867499853));
#289637=CARTESIAN_POINT('Ctrl Pts',(-4.55084385514338,12.2,-9.53802627043278));
#289638=CARTESIAN_POINT('Ctrl Pts',(-4.54843302214482,12.2,-9.53488071970793));
#289639=CARTESIAN_POINT('Ctrl Pts',(-4.54605659139632,12.2,-9.53176271515335));
#289640=CARTESIAN_POINT('Ctrl Pts',(-4.54368016043197,12.2,-9.52864471031555));
#289641=CARTESIAN_POINT('Ctrl Pts',(-4.54133813251356,12.2,-9.52555425267282));
#289642=CARTESIAN_POINT('Ctrl Pts',(-4.53903050947347,12.2,-9.52249204892452));
#289643=CARTESIAN_POINT('Ctrl Pts',(-4.53672288664299,12.2,-9.51942984545438));
#289644=CARTESIAN_POINT('Ctrl Pts',(-4.53444966962028,12.2,-9.51639589744254));
#289645=CARTESIAN_POINT('Ctrl Pts',(-4.5322108606198,12.2,-9.51339092688632));
#289646=CARTESIAN_POINT('Ctrl Pts',(-4.52997205161932,12.2,-9.51038595633012));
#289647=CARTESIAN_POINT('Ctrl Pts',(-4.52776764941607,12.2,-9.50740996380491));
#289648=CARTESIAN_POINT('Ctrl Pts',(-4.52559765441008,12.2,-9.50446368641068));
#289649=CARTESIAN_POINT('Ctrl Pts',(-4.5234276594041,12.2,-9.50151740901644));
#289650=CARTESIAN_POINT('Ctrl Pts',(-4.5212920698717,12.2,-9.49860084922844));
#289651=CARTESIAN_POINT('Ctrl Pts',(-4.5191908829457,12.2,-9.49571475883122));
#289652=CARTESIAN_POINT('Ctrl Pts',(-4.51708969582884,12.2,-9.49282866817185));
#289653=CARTESIAN_POINT('Ctrl Pts',(-4.51502291210698,12.2,-9.48997304829872));
#289654=CARTESIAN_POINT('Ctrl Pts',(-4.51299052391437,12.2,-9.48714866981283));
#289655=CARTESIAN_POINT('Ctrl Pts',(-4.51095813590639,12.2,-9.48432429158348));
#289656=CARTESIAN_POINT('Ctrl Pts',(-4.50896014198021,12.2,-9.48153115490518));
#289657=CARTESIAN_POINT('Ctrl Pts',(-4.50699653595922,12.2,-9.47877004774288));
#289658=CARTESIAN_POINT('Ctrl Pts',(-4.50503292993824,12.2,-9.47600894058059));
#289659=CARTESIAN_POINT('Ctrl Pts',(-4.50310370915668,12.2,-9.47327986356477));
#289660=CARTESIAN_POINT('Ctrl Pts',(-4.50120886122321,12.2,-9.47058362332719));
#289661=CARTESIAN_POINT('Ctrl Pts',(-4.49931401311762,12.2,-9.46788738284471));
#289662=CARTESIAN_POINT('Ctrl Pts',(-4.49745354028197,12.2,-9.46522397837363));
#289663=CARTESIAN_POINT('Ctrl Pts',(-4.49562742318395,12.2,-9.46259423514845));
#289664=CARTESIAN_POINT('Ctrl Pts',(-4.49380130625181,12.2,-9.45996449216213));
#289665=CARTESIAN_POINT('Ctrl Pts',(-4.49200954673666,12.2,-9.45736840990308));
#289666=CARTESIAN_POINT('Ctrl Pts',(-4.49025212654247,12.2,-9.45480683398446));
#289667=CARTESIAN_POINT('Ctrl Pts',(-4.48849470634826,12.2,-9.45224525806583));
#289668=CARTESIAN_POINT('Ctrl Pts',(-4.4867716246584,12.2,-9.44971818930846));
#289669=CARTESIAN_POINT('Ctrl Pts',(-4.48508285871741,12.2,-9.44722649047989));
#289670=CARTESIAN_POINT('Ctrl Pts',(-4.48339409262302,12.2,-9.444734791425));
#289671=CARTESIAN_POINT('Ctrl Pts',(-4.48173964300225,12.2,-9.44227846404994));
#289672=CARTESIAN_POINT('Ctrl Pts',(-4.48011948358502,12.2,-9.43985839296593));
#289673=CARTESIAN_POINT('Ctrl Pts',(-4.47849932431494,12.2,-9.43743832210177));
#289674=CARTESIAN_POINT('Ctrl Pts',(-4.47691345406029,12.2,-9.43505450957303));
#289675=CARTESIAN_POINT('Ctrl Pts',(-4.47536184594999,12.2,-9.43270786274161));
#289676=CARTESIAN_POINT('Ctrl Pts',(-4.47355163639402,12.2,-9.42997010796286));
#289677=CARTESIAN_POINT('Ctrl Pts',(-4.47178806018459,12.2,-9.42728293651277));
#289678=CARTESIAN_POINT('Ctrl Pts',(-4.47007106361604,12.2,-9.42464783456488));
#289679=CARTESIAN_POINT('Ctrl Pts',(-4.46859935234796,12.2,-9.42238917586963));
#289680=CARTESIAN_POINT('Ctrl Pts',(-4.46716186176567,12.2,-9.42016877156237));
#289681=CARTESIAN_POINT('Ctrl Pts',(-4.46575855748332,12.2,-9.41798758122494));
#289682=CARTESIAN_POINT('Ctrl Pts',(-4.46435525320098,12.2,-9.41580639088751));
#289683=CARTESIAN_POINT('Ctrl Pts',(-4.46298613169106,12.2,-9.41366441709268));
#289684=CARTESIAN_POINT('Ctrl Pts',(-4.46165115442089,12.2,-9.41156264164503));
#289685=CARTESIAN_POINT('Ctrl Pts',(-4.46031617702945,12.2,-9.40946086600647));
#289686=CARTESIAN_POINT('Ctrl Pts',(-4.45901534261198,12.2,-9.40739929082871));
#289687=CARTESIAN_POINT('Ctrl Pts',(-4.4577486043786,12.2,-9.4053789264714));
#289688=CARTESIAN_POINT('Ctrl Pts',(-4.45648186626027,12.2,-9.40335856229759));
#289689=CARTESIAN_POINT('Ctrl Pts',(-4.45524922600296,12.2,-9.40137941174577));
#289690=CARTESIAN_POINT('Ctrl Pts',(-4.4540506319578,12.2,-9.39944251172409));
#289691=CARTESIAN_POINT('Ctrl Pts',(-4.45285203791264,12.2,-9.39750561170241));
#289692=CARTESIAN_POINT('Ctrl Pts',(-4.4516874925305,12.2,-9.39561096341066));
#289693=CARTESIAN_POINT('Ctrl Pts',(-4.45055693932009,12.2,-9.39375963655935));
#289694=CARTESIAN_POINT('Ctrl Pts',(-4.44942638600698,12.2,-9.39190830953989));
#289695=CARTESIAN_POINT('Ctrl Pts',(-4.44832982439813,12.2,-9.3901003030425));
#289696=CARTESIAN_POINT('Ctrl Pts',(-4.44726719709251,12.2,-9.38833671903271));
#289697=CARTESIAN_POINT('Ctrl Pts',(-4.44620456988342,12.2,-9.38657313518314));
#289698=CARTESIAN_POINT('Ctrl Pts',(-4.44517587501664,12.2,-9.38485397162112));
#289699=CARTESIAN_POINT('Ctrl Pts',(-4.44418105163759,12.2,-9.38318036293392));
#289700=CARTESIAN_POINT('Ctrl Pts',(-4.44285939486153,12.2,-9.38095691673382));
#289701=CARTESIAN_POINT('Ctrl Pts',(-4.4415975258323,12.2,-9.3788138680557));
#289702=CARTESIAN_POINT('Ctrl Pts',(-4.44039525800005,12.2,-9.37675396700002));
#289703=CARTESIAN_POINT('Ctrl Pts',(-4.44039525800005,15.2,-9.37675396700002));
#289704=CARTESIAN_POINT('Ctrl Pts',(-4.44129587306896,15.2,-9.37829703243141));
#289705=CARTESIAN_POINT('Ctrl Pts',(-4.44222992933227,15.2,-9.37988675705661));
#289706=CARTESIAN_POINT('Ctrl Pts',(-4.44319751536069,15.2,-9.38152198184585));
#289707=CARTESIAN_POINT('Ctrl Pts',(-4.44416976757804,15.2,-9.38316509251559));
#289708=CARTESIAN_POINT('Ctrl Pts',(-4.44517586568178,15.2,-9.3848541409591));
#289709=CARTESIAN_POINT('Ctrl Pts',(-4.44621587887569,15.2,-9.38658798489277));
#289710=CARTESIAN_POINT('Ctrl Pts',(-4.44725589197513,15.2,-9.38832182866894));
#289711=CARTESIAN_POINT('Ctrl Pts',(-4.4483298151569,15.2,-9.3901004685328));
#289712=CARTESIAN_POINT('Ctrl Pts',(-4.44943771428333,15.2,-9.3919227914666));
#289713=CARTESIAN_POINT('Ctrl Pts',(-4.45054561340975,15.2,-9.39374511440041));
#289714=CARTESIAN_POINT('Ctrl Pts',(-4.45168748543062,15.2,-9.39561112218358));
#289715=CARTESIAN_POINT('Ctrl Pts',(-4.45286338586133,15.2,-9.39751973529041));
#289716=CARTESIAN_POINT('Ctrl Pts',(-4.45403928639883,15.2,-9.39942834857061));
#289717=CARTESIAN_POINT('Ctrl Pts',(-4.45524921782382,15.2,-9.40137956588904));
#289718=CARTESIAN_POINT('Ctrl Pts',(-4.45649323014394,15.2,-9.40337233916716));
#289719=CARTESIAN_POINT('Ctrl Pts',(-4.45773724235106,15.2,-9.40536511226427));
#289720=CARTESIAN_POINT('Ctrl Pts',(-4.4590153346589,15.2,-9.40739944035009));
#289721=CARTESIAN_POINT('Ctrl Pts',(-4.46032755578393,15.2,-9.40947430345089));
#289722=CARTESIAN_POINT('Ctrl Pts',(-4.46163977690896,15.2,-9.41154916655169));
#289723=CARTESIAN_POINT('Ctrl Pts',(-4.46298612577653,15.2,-9.41366456319599));
#289724=CARTESIAN_POINT('Ctrl Pts',(-4.46436664589157,15.2,-9.415819499616));
#289725=CARTESIAN_POINT('Ctrl Pts',(-4.46574716613199,15.2,-9.41797443623173));
#289726=CARTESIAN_POINT('Ctrl Pts',(-4.46716185662663,15.2,-9.42016891470236));
#289727=CARTESIAN_POINT('Ctrl Pts',(-4.4686107578746,15.2,-9.42240196349335));
#289728=CARTESIAN_POINT('Ctrl Pts',(-4.47005965899096,15.2,-9.42463501208151));
#289729=CARTESIAN_POINT('Ctrl Pts',(-4.47154276904483,15.2,-9.4269066335916));
#289730=CARTESIAN_POINT('Ctrl Pts',(-4.4730601250745,15.2,-9.42921588234262));
#289731=CARTESIAN_POINT('Ctrl Pts',(-4.47457748110417,15.2,-9.43152513109366));
#289732=CARTESIAN_POINT('Ctrl Pts',(-4.47612908174782,15.2,-9.43387200969173));
#289733=CARTESIAN_POINT('Ctrl Pts',(-4.47771495793871,15.2,-9.43625559460353));
#289734=CARTESIAN_POINT('Ctrl Pts',(-4.47930083412959,15.2,-9.43863917951534));
#289735=CARTESIAN_POINT('Ctrl Pts',(-4.48092098727379,15.2,-9.44105947538224));
#289736=CARTESIAN_POINT('Ctrl Pts',(-4.48257544329467,15.2,-9.44351558120724));
#289737=CARTESIAN_POINT('Ctrl Pts',(-4.48422989946583,15.2,-9.44597168725533));
#289738=CARTESIAN_POINT('Ctrl Pts',(-4.48591865903198,15.2,-9.44846360574858));
#289739=CARTESIAN_POINT('Ctrl Pts',(-4.48764174712739,15.2,-9.45099045888782));
#289740=CARTESIAN_POINT('Ctrl Pts',(-4.48936483506628,15.2,-9.45351731179754));
#289741=CARTESIAN_POINT('Ctrl Pts',(-4.49112225103122,15.2,-9.4560791013147));
#289742=CARTESIAN_POINT('Ctrl Pts',(-4.49291401422419,15.2,-9.45867497223211));
#289743=CARTESIAN_POINT('Ctrl Pts',(-4.49470577741715,15.2,-9.46127084314952));
#289744=CARTESIAN_POINT('Ctrl Pts',(-4.49653189046714,15.2,-9.46390079412535));
#289745=CARTESIAN_POINT('Ctrl Pts',(-4.49839236756388,15.2,-9.46656399219301));
#289746=CARTESIAN_POINT('Ctrl Pts',(-4.50025284482961,15.2,-9.46922719050256));
#289747=CARTESIAN_POINT('Ctrl Pts',(-4.50214768997363,15.2,-9.47192363591533));
#289748=CARTESIAN_POINT('Ctrl Pts',(-4.50407691416362,15.2,-9.47465251139882));
#289749=CARTESIAN_POINT('Ctrl Pts',(-4.50600613817835,15.2,-9.47738138663443));
#289750=CARTESIAN_POINT('Ctrl Pts',(-4.50796974008769,15.2,-9.48014269291256));
#289751=CARTESIAN_POINT('Ctrl Pts',(-4.50996773677409,15.2,-9.48293563224036));
#289752=CARTESIAN_POINT('Ctrl Pts',(-4.51196573346048,15.2,-9.48572857156816));
#289753=CARTESIAN_POINT('Ctrl Pts',(-4.51399811893549,15.2,-9.48855314476124));
#289754=CARTESIAN_POINT('Ctrl Pts',(-4.51606490402472,15.2,-9.49140857198872));
#289755=CARTESIAN_POINT('Ctrl Pts',(-4.51813168930169,15.2,-9.49426399947558));
#289756=CARTESIAN_POINT('Ctrl Pts',(-4.52023287548161,15.2,-9.49715028115079));
#289757=CARTESIAN_POINT('Ctrl Pts',(-4.52236846570667,15.2,-9.50006665304049));
#289758=CARTESIAN_POINT('Ctrl Pts',(-4.52450405573775,15.2,-9.50298302466529));
#289759=CARTESIAN_POINT('Ctrl Pts',(-4.52667405050507,15.2,-9.50592948864139));
#289760=CARTESIAN_POINT('Ctrl Pts',(-4.52887845250833,15.2,-9.50890529619996));
#289761=CARTESIAN_POINT('Ctrl Pts',(-4.53108285451158,15.2,-9.51188110375853));
#289762=CARTESIAN_POINT('Ctrl Pts',(-4.5333216636262,15.2,-9.5148862582502));
#289763=CARTESIAN_POINT('Ctrl Pts',(-4.53559487973851,15.2,-9.51792002595656));
#289764=CARTESIAN_POINT('Ctrl Pts',(-4.53786809605731,15.2,-9.52095379393847));
#289765=CARTESIAN_POINT('Ctrl Pts',(-4.54017571979194,15.2,-9.52401617530812));
#289766=CARTESIAN_POINT('Ctrl Pts',(-4.54251774775529,15.2,-9.52710645706181));
#289767=CARTESIAN_POINT('Ctrl Pts',(-4.54485977550589,15.2,-9.5301967385348));
#289768=CARTESIAN_POINT('Ctrl Pts',(-4.54723620634433,15.2,-9.533314916993));
#289769=CARTESIAN_POINT('Ctrl Pts',(-4.54964703726776,15.2,-9.5364602954764));
#289770=CARTESIAN_POINT('Ctrl Pts',(-4.55205786819119,15.2,-9.5396056739598));
#289771=CARTESIAN_POINT('Ctrl Pts',(-4.55450309886493,15.2,-9.54277824955146));
#289772=CARTESIAN_POINT('Ctrl Pts',(-4.55698271885667,15.2,-9.54597733635073));
#289773=CARTESIAN_POINT('Ctrl Pts',(-4.55904906892486,15.2,-9.54864324211365));
#289774=CARTESIAN_POINT('Ctrl Pts',(-4.5611393024409,15.2,-9.55132755935761));
#289775=CARTESIAN_POINT('Ctrl Pts',(-4.56325341237021,15.2,-9.55402989685668));
#289776=CARTESIAN_POINT('Ctrl Pts',(-4.56536752229952,15.2,-9.55673223435573));
#289777=CARTESIAN_POINT('Ctrl Pts',(-4.56750550940575,15.2,-9.559452592325));
#289778=CARTESIAN_POINT('Ctrl Pts',(-4.56966736524882,15.2,-9.56219058803181));
#289779=CARTESIAN_POINT('Ctrl Pts',(-4.57182922109189,15.2,-9.56492858373862));
#289780=CARTESIAN_POINT('Ctrl Pts',(-4.57401494733888,15.2,-9.56768421420552));
#289781=CARTESIAN_POINT('Ctrl Pts',(-4.57622453553333,15.2,-9.5704571057333));
#289782=CARTESIAN_POINT('Ctrl Pts',(-4.57843412372777,15.2,-9.57322999726108));
#289783=CARTESIAN_POINT('Ctrl Pts',(-4.58066757280202,15.2,-9.57602014604425));
#289784=CARTESIAN_POINT('Ctrl Pts',(-4.5829248752429,15.2,-9.57882718425151));
#289785=CARTESIAN_POINT('Ctrl Pts',(-4.58518217768378,15.2,-9.58163422245876));
#289786=CARTESIAN_POINT('Ctrl Pts',(-4.58746333292187,15.2,-9.58445814714054));
#289787=CARTESIAN_POINT('Ctrl Pts',(-4.58976832965921,15.2,-9.5872985938775));
#289788=CARTESIAN_POINT('Ctrl Pts',(-4.59207332639657,15.2,-9.59013904061447));
#289789=CARTESIAN_POINT('Ctrl Pts',(-4.59440216662497,15.2,-9.59299600884825));
#289790=CARTESIAN_POINT('Ctrl Pts',(-4.59675483669568,15.2,-9.59586913815465));
#289791=CARTESIAN_POINT('Ctrl Pts',(-4.59910750676638,15.2,-9.59874226746106));
#289792=CARTESIAN_POINT('Ctrl Pts',(-4.60148400954602,15.2,-9.60163155960212));
#289793=CARTESIAN_POINT('Ctrl Pts',(-4.60388432973706,15.2,-9.60453665738727));
#289794=CARTESIAN_POINT('Ctrl Pts',(-4.60676471386164,15.2,-9.60802277460278));
#289795=CARTESIAN_POINT('Ctrl Pts',(-4.60967939652379,15.2,-9.61153165427825));
#289796=CARTESIAN_POINT('Ctrl Pts',(-4.61262835724999,15.2,-9.61506269148331));
#289797=CARTESIAN_POINT('Ctrl Pts',(-4.61508582461112,15.2,-9.61800522259443));
#289798=CARTESIAN_POINT('Ctrl Pts',(-4.61756709430659,15.2,-9.62096314346027));
#289799=CARTESIAN_POINT('Ctrl Pts',(-4.62007215181803,15.2,-9.6239361087516));
#289800=CARTESIAN_POINT('Ctrl Pts',(-4.62307822072255,15.2,-9.62750366697158));
#289801=CARTESIAN_POINT('Ctrl Pts',(-4.62611854627076,15.2,-9.63109288948539));
#289802=CARTESIAN_POINT('Ctrl Pts',(-4.62919309907425,15.2,-9.63470319551998));
#289803=CARTESIAN_POINT('Ctrl Pts',(-4.63175522650357,15.2,-9.63771178399145));
#289804=CARTESIAN_POINT('Ctrl Pts',(-4.6343411247696,15.2,-9.64073501219105));
#289805=CARTESIAN_POINT('Ctrl Pts',(-4.63695077629614,15.2,-9.64377254830142));
#289806=CARTESIAN_POINT('Ctrl Pts',(-4.63956042782267,15.2,-9.64681008441177));
#289807=CARTESIAN_POINT('Ctrl Pts',(-4.64219383285538,15.2,-9.64986192952252));
#289808=CARTESIAN_POINT('Ctrl Pts',(-4.64485097361803,15.2,-9.65292775500789));
#289809=CARTESIAN_POINT('Ctrl Pts',(-4.64750811438069,15.2,-9.65599358049328));
#289810=CARTESIAN_POINT('Ctrl Pts',(-4.65018899065296,15.2,-9.65907338792872));
#289811=CARTESIAN_POINT('Ctrl Pts',(-4.65289358545686,15.2,-9.66216685328996));
#289812=CARTESIAN_POINT('Ctrl Pts',(-4.65559818026076,15.2,-9.66526031865121));
#289813=CARTESIAN_POINT('Ctrl Pts',(-4.65832649309999,15.2,-9.66836744337775));
#289814=CARTESIAN_POINT('Ctrl Pts',(-4.66107850455832,15.2,-9.67148790726664));
#289815=CARTESIAN_POINT('Ctrl Pts',(-4.66328011384498,15.2,-9.6739842785138));
#289816=CARTESIAN_POINT('Ctrl Pts',(-4.66549689001951,15.2,-9.67648918765086));
#289817=CARTESIAN_POINT('Ctrl Pts',(-4.66772882336492,15.2,-9.67900247467757));
#289818=CARTESIAN_POINT('Ctrl Pts',(-4.66996075640623,15.2,-9.68151576136185));
#289819=CARTESIAN_POINT('Ctrl Pts',(-4.67220784738428,15.2,-9.68403742419639));
#289820=CARTESIAN_POINT('Ctrl Pts',(-4.67447008376513,15.2,-9.68656730572326));
#289821=CARTESIAN_POINT('Ctrl Pts',(-4.6767323204542,15.2,-9.68909718759483));
#289822=CARTESIAN_POINT('Ctrl Pts',(-4.67900970379279,15.2,-9.69163528819614));
#289823=CARTESIAN_POINT('Ctrl Pts',(-4.6813022231415,15.2,-9.69418144872462));
#289824=CARTESIAN_POINT('Ctrl Pts',(-4.68359474217786,15.2,-9.69672760890619));
#289825=CARTESIAN_POINT('Ctrl Pts',(-4.68590239654558,15.2,-9.69928183023391));
#289826=CARTESIAN_POINT('Ctrl Pts',(-4.68822517557692,15.2,-9.70184395702393));
#289827=CARTESIAN_POINT('Ctrl Pts',(-4.69054795492474,15.2,-9.70440608416305));
#289828=CARTESIAN_POINT('Ctrl Pts',(-4.69288585780274,15.2,-9.70697611574302));
#289829=CARTESIAN_POINT('Ctrl Pts',(-4.69523887454985,15.2,-9.70955389912408));
#289830=CARTESIAN_POINT('Ctrl Pts',(-4.69759189097635,15.2,-9.7121316821539));
#289831=CARTESIAN_POINT('Ctrl Pts',(-4.69996002057612,15.2,-9.71471721621443));
#289832=CARTESIAN_POINT('Ctrl Pts',(-4.70234325154698,15.2,-9.71731035027974));
#289833=CARTESIAN_POINT('Ctrl Pts',(-4.70472648284255,15.2,-9.71990348469834));
#289834=CARTESIAN_POINT('Ctrl Pts',(-4.70712481440659,15.2,-9.72250421721508));
#289835=CARTESIAN_POINT('Ctrl Pts',(-4.70953823570577,15.2,-9.72511239791327));
#289836=CARTESIAN_POINT('Ctrl Pts',(-4.71195165667613,15.2,-9.72772057825609));
#289837=CARTESIAN_POINT('Ctrl Pts',(-4.71438016588005,15.2,-9.73033620828677));
#289838=CARTESIAN_POINT('Ctrl Pts',(-4.71682375291217,15.2,-9.73295913786943));
#289839=CARTESIAN_POINT('Ctrl Pts',(-4.71926734027724,15.2,-9.73558206780946));
#289840=CARTESIAN_POINT('Ctrl Pts',(-4.72172600436934,15.2,-9.73821229534368));
#289841=CARTESIAN_POINT('Ctrl Pts',(-4.72419973122737,15.2,-9.74084967593232));
#289842=CARTESIAN_POINT('Ctrl Pts',(-4.72667345774834,15.2,-9.74348705616163));
#289843=CARTESIAN_POINT('Ctrl Pts',(-4.72916224918853,15.2,-9.74613158787284));
#289844=CARTESIAN_POINT('Ctrl Pts',(-4.73166609081563,15.2,-9.7487831260998));
#289845=CARTESIAN_POINT('Ctrl Pts',(-4.73416993278388,15.2,-9.75143466468803));
#289846=CARTESIAN_POINT('Ctrl Pts',(-4.73668882621595,15.2,-9.75409320831662));
#289847=CARTESIAN_POINT('Ctrl Pts',(-4.73922275631006,15.2,-9.7567586142518));
#289848=CARTESIAN_POINT('Ctrl Pts',(-4.74175668605892,15.2,-9.75942401982382));
#289849=CARTESIAN_POINT('Ctrl Pts',(-4.74430565351416,15.2,-9.76209628581778));
#289850=CARTESIAN_POINT('Ctrl Pts',(-4.74686964508079,15.2,-9.76477527132031));
#289851=CARTESIAN_POINT('Ctrl Pts',(-4.74943363699677,15.2,-9.76745425718785));
#289852=CARTESIAN_POINT('Ctrl Pts',(-4.75201265260585,15.2,-9.77013996024215));
#289853=CARTESIAN_POINT('Ctrl Pts',(-4.75460667802499,15.2,-9.77283224149999));
#289854=CARTESIAN_POINT('Ctrl Pts',(-4.75720070344414,15.2,-9.77552452275782));
#289855=CARTESIAN_POINT('Ctrl Pts',(-4.75980973894005,15.2,-9.77822337983588));
#289856=CARTESIAN_POINT('Ctrl Pts',(-4.7624337701957,15.2,-9.78092867448397));
#289857=CARTESIAN_POINT('Ctrl Pts',(-4.76505780109382,15.2,-9.78363396876347));
#289858=CARTESIAN_POINT('Ctrl Pts',(-4.76769682802537,15.2,-9.78634569908302));
#289859=CARTESIAN_POINT('Ctrl Pts',(-4.77035083626486,15.2,-9.7890637280398));
#289860=CARTESIAN_POINT('Ctrl Pts',(-4.77300484486595,15.2,-9.79178175736693));
#289861=CARTESIAN_POINT('Ctrl Pts',(-4.77567383341881,15.2,-9.79450608374421));
#289862=CARTESIAN_POINT('Ctrl Pts',(-4.7783577894555,15.2,-9.79723657117143));
#289863=CARTESIAN_POINT('Ctrl Pts',(-4.7810417451265,15.2,-9.79996705822662));
#289864=CARTESIAN_POINT('Ctrl Pts',(-4.78374066790945,15.2,-9.80270370614766));
#289865=CARTESIAN_POINT('Ctrl Pts',(-4.78645454151995,15.2,-9.80544637853417));
#289866=CARTESIAN_POINT('Ctrl Pts',(-4.78984688381039,15.2,-9.80887471929756));
#289867=CARTESIAN_POINT('Ctrl Pts',(-4.793262589427,15.2,-9.81231247312136));
#289868=CARTESIAN_POINT('Ctrl Pts',(-4.79670162520646,15.2,-9.81575937799811));
#289869=CARTESIAN_POINT('Ctrl Pts',(-4.79945285397997,15.2,-9.81851690204981));
#289870=CARTESIAN_POINT('Ctrl Pts',(-4.80221901562662,15.2,-9.82128028213457));
#289871=CARTESIAN_POINT('Ctrl Pts',(-4.80500009361305,15.2,-9.82404938495274));
#289872=CARTESIAN_POINT('Ctrl Pts',(-4.80778117122055,15.2,-9.82681848739362));
#289873=CARTESIAN_POINT('Ctrl Pts',(-4.81057716615944,15.2,-9.82959331418652));
#289874=CARTESIAN_POINT('Ctrl Pts',(-4.81338806176202,15.2,-9.83237373201441));
#289875=CARTESIAN_POINT('Ctrl Pts',(-4.81619895774758,15.2,-9.83515415022114));
#289876=CARTESIAN_POINT('Ctrl Pts',(-4.81902475443926,15.2,-9.83794015955746));
#289877=CARTESIAN_POINT('Ctrl Pts',(-4.82186543590395,15.2,-9.84073163040508));
#289878=CARTESIAN_POINT('Ctrl Pts',(-4.82470611698159,15.2,-9.84352310087235));
#289879=CARTESIAN_POINT('Ctrl Pts',(-4.827561683815,15.2,-9.84632003093095));
#289880=CARTESIAN_POINT('Ctrl Pts',(-4.83043211752381,15.2,-9.84912229331263));
#289881=CARTESIAN_POINT('Ctrl Pts',(-4.83330255162373,15.2,-9.85192455607611));
#289882=CARTESIAN_POINT('Ctrl Pts',(-4.83618785594209,15.2,-9.85473215061525));
#289883=CARTESIAN_POINT('Ctrl Pts',(-4.83908801071222,15.2,-9.85754494821332));
#289884=CARTESIAN_POINT('Ctrl Pts',(-4.84198816508721,15.2,-9.86035774542816));
#289885=CARTESIAN_POINT('Ctrl Pts',(-4.84490317079812,15.2,-9.8631757464364));
#289886=CARTESIAN_POINT('Ctrl Pts',(-4.84783301227931,15.2,-9.86599882353843));
#289887=CARTESIAN_POINT('Ctrl Pts',(-4.85076285415969,15.2,-9.86882190102509));
#289888=CARTESIAN_POINT('Ctrl Pts',(-4.85370753039946,15.2,-9.87165005590408));
#289889=CARTESIAN_POINT('Ctrl Pts',(-4.85666702501868,15.2,-9.87448316079359));
#289890=CARTESIAN_POINT('Ctrl Pts',(-4.85962651923467,15.2,-9.87731626529708));
#289891=CARTESIAN_POINT('Ctrl Pts',(-4.86260083098215,15.2,-9.88015432137363));
#289892=CARTESIAN_POINT('Ctrl Pts',(-4.86558994323629,15.2,-9.88299720258519));
#289893=CARTESIAN_POINT('Ctrl Pts',(-4.86857905589768,15.2,-9.88584008418408));
#289894=CARTESIAN_POINT('Ctrl Pts',(-4.87158296992992,15.2,-9.8886877912251));
#289895=CARTESIAN_POINT('Ctrl Pts',(-4.87460166598333,15.2,-9.89154020199166));
#289896=CARTESIAN_POINT('Ctrl Pts',(-4.87837503584443,15.2,-9.89510571525555));
#289897=CARTESIAN_POINT('Ctrl Pts',(-4.88217150414023,15.2,-9.89867857641345));
#289898=CARTESIAN_POINT('Ctrl Pts',(-4.88599103631042,15.2,-9.90225854573528));
#289899=CARTESIAN_POINT('Ctrl Pts',(-4.88904666179677,15.2,-9.90512252095861));
#289900=CARTESIAN_POINT('Ctrl Pts',(-4.89211704631597,15.2,-9.90799104656559));
#289901=CARTESIAN_POINT('Ctrl Pts',(-4.89520217572892,15.2,-9.91086400099694));
#289902=CARTESIAN_POINT('Ctrl Pts',(-4.89828730556222,15.2,-9.91373695581972));
#289903=CARTESIAN_POINT('Ctrl Pts',(-4.90138717653582,15.2,-9.91661433966796));
#289904=CARTESIAN_POINT('Ctrl Pts',(-4.90450177248333,15.2,-9.91949603199166));
#289905=CARTESIAN_POINT('Ctrl Pts',(-4.90761636843084,15.2,-9.92237772431537));
#289906=CARTESIAN_POINT('Ctrl Pts',(-4.91074568829676,15.2,-9.92526372623405));
#289907=CARTESIAN_POINT('Ctrl Pts',(-4.91388971424739,15.2,-9.92815391778088));
#289908=CARTESIAN_POINT('Ctrl Pts',(-4.91703373976965,15.2,-9.93104410893392));
#289909=CARTESIAN_POINT('Ctrl Pts',(-4.92019247112068,15.2,-9.93393848935794));
#289910=CARTESIAN_POINT('Ctrl Pts',(-4.92336588876451,15.2,-9.93683694318969));
#289911=CARTESIAN_POINT('Ctrl Pts',(-4.92733266114358,15.2,-9.94046001077558));
#289912=CARTESIAN_POINT('Ctrl Pts',(-4.93132238283334,15.2,-9.94408944093889));
#289913=CARTESIAN_POINT('Ctrl Pts',(-4.93533501595833,15.2,-9.94772500600833));
#289914=CARTESIAN_POINT('Ctrl Pts',(-4.93854512263327,15.2,-9.95063345822239));
#289915=CARTESIAN_POINT('Ctrl Pts',(-4.94176989238772,15.2,-9.95354583590637));
#289916=CARTESIAN_POINT('Ctrl Pts',(-4.94500930628798,15.2,-9.95646202551013));
#289917=CARTESIAN_POINT('Ctrl Pts',(-4.94824871974687,15.2,-9.95937821471655));
#289918=CARTESIAN_POINT('Ctrl Pts',(-4.95150277701686,15.2,-9.96229821511542));
#289919=CARTESIAN_POINT('Ctrl Pts',(-4.95477145976444,15.2,-9.96522191172301));
#289920=CARTESIAN_POINT('Ctrl Pts',(-4.95804014295737,15.2,-9.96814560872894));
#289921=CARTESIAN_POINT('Ctrl Pts',(-4.96132344816353,15.2,-9.9710730021441));
#289922=CARTESIAN_POINT('Ctrl Pts',(-4.96462136078921,15.2,-9.97400397847088));
#289923=CARTESIAN_POINT('Ctrl Pts',(-4.96791927296556,15.2,-9.97693495439831));
#289924=CARTESIAN_POINT('Ctrl Pts',(-4.97123179003945,15.2,-9.97986951303868));
#289925=CARTESIAN_POINT('Ctrl Pts',(-4.97455889221133,15.2,-9.98280754224305));
#289926=CARTESIAN_POINT('Ctrl Pts',(-4.97705421895357,15.2,-9.9850110642464));
#289927=CARTESIAN_POINT('Ctrl Pts',(-4.97955774913085,15.2,-9.98721653815976));
#289928=CARTESIAN_POINT('Ctrl Pts',(-4.98206947595579,15.2,-9.98942391685628));
#289929=CARTESIAN_POINT('Ctrl Pts',(-4.98625568748279,15.2,-9.99310288148416));
#289930=CARTESIAN_POINT('Ctrl Pts',(-4.99046466364678,15.2,-9.99678713890346));
#289931=CARTESIAN_POINT('Ctrl Pts',(-4.99469636746505,15.2,-10.0004764692504));
#289932=CARTESIAN_POINT('Ctrl Pts',(-4.99723538966376,15.2,-10.0026900673782));
#289933=CARTESIAN_POINT('Ctrl Pts',(-4.99978259340357,15.2,-10.0049054927641));
#289934=CARTESIAN_POINT('Ctrl Pts',(-5.0023379696846,15.2,-10.0071226992667));
#289935=CARTESIAN_POINT('Ctrl Pts',(-5.00489334642986,15.2,-10.009339906172));
#289936=CARTESIAN_POINT('Ctrl Pts',(-5.0074568963191,15.2,-10.0115588927778));
#289937=CARTESIAN_POINT('Ctrl Pts',(-5.01002861052731,15.2,-10.0137796147258));
#289938=CARTESIAN_POINT('Ctrl Pts',(-5.0143147997842,15.2,-10.0174808170311));
#289939=CARTESIAN_POINT('Ctrl Pts',(-5.01862366698522,15.2,-10.0211868384584));
#289940=CARTESIAN_POINT('Ctrl Pts',(-5.02295517290012,15.2,-10.024897464998));
#289941=CARTESIAN_POINT('Ctrl Pts',(-5.02555407711004,15.2,-10.027123841488));
#289942=CARTESIAN_POINT('Ctrl Pts',(-5.02816113062227,15.2,-10.0293518765785));
#289943=CARTESIAN_POINT('Ctrl Pts',(-5.03077632533679,15.2,-10.0315815250277));
#289944=CARTESIAN_POINT('Ctrl Pts',(-5.03339151957621,15.2,-10.0338111730719));
#289945=CARTESIAN_POINT('Ctrl Pts',(-5.03601485498186,15.2,-10.0360424334411));
#289946=CARTESIAN_POINT('Ctrl Pts',(-5.03864632176197,15.2,-10.0382752629434));
#289947=CARTESIAN_POINT('Ctrl Pts',(-5.04127778854207,15.2,-10.0405080924458));
#289948=CARTESIAN_POINT('Ctrl Pts',(-5.04391738720321,15.2,-10.0427424891898));
#289949=CARTESIAN_POINT('Ctrl Pts',(-5.04656510899407,15.2,-10.0449784097854));
#289950=CARTESIAN_POINT('Ctrl Pts',(-5.04921283078493,15.2,-10.0472143303809));
#289951=CARTESIAN_POINT('Ctrl Pts',(-5.05186867664898,15.2,-10.0494517752692));
#289952=CARTESIAN_POINT('Ctrl Pts',(-5.05453263548092,15.2,-10.0516906974896));
#289953=CARTESIAN_POINT('Ctrl Pts',(-5.05719659431285,15.2,-10.0539296197101));
#289954=CARTESIAN_POINT('Ctrl Pts',(-5.05986866842276,15.2,-10.0561700219872));
#289955=CARTESIAN_POINT('Ctrl Pts',(-5.06254884624133,15.2,-10.0584118585307));
#289956=CARTESIAN_POINT('Ctrl Pts',(-5.0652290240599,15.2,-10.0606536950741));
#289957=CARTESIAN_POINT('Ctrl Pts',(-5.06791730711127,15.2,-10.0628969650424));
#289958=CARTESIAN_POINT('Ctrl Pts',(-5.07061368588719,15.2,-10.065141627044));
#289959=CARTESIAN_POINT('Ctrl Pts',(-5.07331006515296,15.2,-10.0673862894534));
#289960=CARTESIAN_POINT('Ctrl Pts',(-5.07601454037935,15.2,-10.0696323414965));
#289961=CARTESIAN_POINT('Ctrl Pts',(-5.07872710256635,15.2,-10.0718797409899));
#289962=CARTESIAN_POINT('Ctrl Pts',(-5.08143966426057,15.2,-10.0741271400751));
#289963=CARTESIAN_POINT('Ctrl Pts',(-5.08416031248991,15.2,-10.0763758862712));
#289964=CARTESIAN_POINT('Ctrl Pts',(-5.08688903877802,15.2,-10.0786259364687));
#289965=CARTESIAN_POINT('Ctrl Pts',(-5.08961776506613,15.2,-10.0808759866661));
#289966=CARTESIAN_POINT('Ctrl Pts',(-5.09235456784836,15.2,-10.0831273396106));
#289967=CARTESIAN_POINT('Ctrl Pts',(-5.09509943904099,15.2,-10.0853799536956));
#289968=CARTESIAN_POINT('Ctrl Pts',(-5.09784431023363,15.2,-10.0876325677805));
#289969=CARTESIAN_POINT('Ctrl Pts',(-5.10059724988364,15.2,-10.0898864421486));
#289970=CARTESIAN_POINT('Ctrl Pts',(-5.103358248575,15.2,-10.092141533775));
#289971=CARTESIAN_POINT('Ctrl Pts',(-5.10611924726635,15.2,-10.0943966254014));
#289972=CARTESIAN_POINT('Ctrl Pts',(-5.10888830443237,15.2,-10.0966529346028));
#289973=CARTESIAN_POINT('Ctrl Pts',(-5.11166541120576,15.2,-10.098910418729));
#289974=CARTESIAN_POINT('Ctrl Pts',(-5.11444251797916,15.2,-10.1011679028552));
#289975=CARTESIAN_POINT('Ctrl Pts',(-5.11722767457701,15.2,-10.103426561673));
#289976=CARTESIAN_POINT('Ctrl Pts',(-5.12002087039109,15.2,-10.1056863532574));
#289977=CARTESIAN_POINT('Ctrl Pts',(-5.1228140667126,15.2,-10.1079461452523));
#289978=CARTESIAN_POINT('Ctrl Pts',(-5.12561530416972,15.2,-10.1102070689309));
#289979=CARTESIAN_POINT('Ctrl Pts',(-5.12842457187077,15.2,-10.1124690834681));
#289980=CARTESIAN_POINT('Ctrl Pts',(-5.13123383906146,15.2,-10.1147310975944));
#289981=CARTESIAN_POINT('Ctrl Pts',(-5.13405113574062,15.2,-10.1169942029238));
#289982=CARTESIAN_POINT('Ctrl Pts',(-5.13687645453005,15.2,-10.1192583557464));
#289983=CARTESIAN_POINT('Ctrl Pts',(-5.13970177331947,15.2,-10.121522508569));
#289984=CARTESIAN_POINT('Ctrl Pts',(-5.14253511241238,15.2,-10.1237877102459));
#289985=CARTESIAN_POINT('Ctrl Pts',(-5.14537646355984,15.2,-10.126053917997));
#289986=CARTESIAN_POINT('Ctrl Pts',(-5.14821781470731,15.2,-10.1283201257481));
#289987=CARTESIAN_POINT('Ctrl Pts',(-5.15106717675381,15.2,-10.1305873404991));
#289988=CARTESIAN_POINT('Ctrl Pts',(-5.15392454052499,15.2,-10.1328555202083));
#289989=CARTESIAN_POINT('Ctrl Pts',(-5.15678190429618,15.2,-10.1351236999176));
#289990=CARTESIAN_POINT('Ctrl Pts',(-5.1596472709087,15.2,-10.1373928453518));
#289991=CARTESIAN_POINT('Ctrl Pts',(-5.16252062867861,15.2,-10.1396629149776));
#289992=CARTESIAN_POINT('Ctrl Pts',(-5.16539398644852,15.2,-10.1419329846034));
#289993=CARTESIAN_POINT('Ctrl Pts',(-5.16827533613595,15.2,-10.1442039780296));
#289994=CARTESIAN_POINT('Ctrl Pts',(-5.1711646689244,15.2,-10.1464758548105));
#289995=CARTESIAN_POINT('Ctrl Pts',(-5.17405400171285,15.2,-10.1487477315913));
#289996=CARTESIAN_POINT('Ctrl Pts',(-5.17695131542331,15.2,-10.1510204920538));
#289997=CARTESIAN_POINT('Ctrl Pts',(-5.17985660256666,15.2,-10.1532940937627));
#289998=CARTESIAN_POINT('Ctrl Pts',(-5.18276189023779,15.2,-10.1555676958847));
#289999=CARTESIAN_POINT('Ctrl Pts',(-5.18567515039454,15.2,-10.1578421401986));
#290000=CARTESIAN_POINT('Ctrl Pts',(-5.1885963726535,15.2,-10.1601173872377));
#290001=CARTESIAN_POINT('Ctrl Pts',(-5.19151759438178,15.2,-10.1623926338635));
#290002=CARTESIAN_POINT('Ctrl Pts',(-5.19444677960963,15.2,-10.1646686821308));
#290003=CARTESIAN_POINT('Ctrl Pts',(-5.19738391737861,15.2,-10.1669454932565));
#290004=CARTESIAN_POINT('Ctrl Pts',(-5.20130010089273,15.2,-10.1699812412862));
#290005=CARTESIAN_POINT('Ctrl Pts',(-5.2052304224238,15.2,-10.1730183444697));
#290006=CARTESIAN_POINT('Ctrl Pts',(-5.20917485868605,15.2,-10.1760567053175));
#290007=CARTESIAN_POINT('Ctrl Pts',(-5.21213318601711,15.2,-10.1783354760568));
#290008=CARTESIAN_POINT('Ctrl Pts',(-5.21509945316077,15.2,-10.1806149527859));
#290009=CARTESIAN_POINT('Ctrl Pts',(-5.2180736488433,15.2,-10.1828950979946));
#290010=CARTESIAN_POINT('Ctrl Pts',(-5.22104784506614,15.2,-10.1851752436176));
#290011=CARTESIAN_POINT('Ctrl Pts',(-5.22402996951621,15.2,-10.1874560576324));
#290012=CARTESIAN_POINT('Ctrl Pts',(-5.22702001566017,15.2,-10.1897375037557));
#290013=CARTESIAN_POINT('Ctrl Pts',(-5.2310067429468,15.2,-10.1927794312294));
#290014=CARTESIAN_POINT('Ctrl Pts',(-5.2350075501205,15.2,-10.1958224850945));
#290015=CARTESIAN_POINT('Ctrl Pts',(-5.23902241218025,15.2,-10.1988665637345));
#290016=CARTESIAN_POINT('Ctrl Pts',(-5.24203355886183,15.2,-10.2011496228182));
#290017=CARTESIAN_POINT('Ctrl Pts',(-5.24505261109078,15.2,-10.2034332566604));
#290018=CARTESIAN_POINT('Ctrl Pts',(-5.24807955692278,15.2,-10.2057174180248));
#290019=CARTESIAN_POINT('Ctrl Pts',(-5.25110650275477,15.2,-10.2080015793892));
#290020=CARTESIAN_POINT('Ctrl Pts',(-5.25414134106499,15.2,-10.2102862675516));
#290021=CARTESIAN_POINT('Ctrl Pts',(-5.25718406582836,15.2,-10.2125714567185));
#290022=CARTESIAN_POINT('Ctrl Pts',(-5.26124103254804,15.2,-10.2156183758845));
#290023=CARTESIAN_POINT('Ctrl Pts',(-5.2653120248846,15.2,-10.218666183391));
#290024=CARTESIAN_POINT('Ctrl Pts',(-5.26939701852072,15.2,-10.2217148786423));
#290025=CARTESIAN_POINT('Origin',(-5.66257110645729E-14,15.2,-1.77635683940025E-14));
#290026=CARTESIAN_POINT('',(-4.04260911704029,15.2,-9.55499537042844));
#290027=CARTESIAN_POINT('',(-4.04260911704029,12.2,-9.55499537042844));
#290028=CARTESIAN_POINT('',(-4.04260911700006,15.2,-9.55499537000001));
#290029=CARTESIAN_POINT('Origin',(-5.66257110645729E-14,12.2,-1.77635683940025E-14));
#290030=CARTESIAN_POINT('Origin',(-5.66257110645729E-14,15.2,-1.77635683940025E-14));
#290031=CARTESIAN_POINT('Origin',(-5.66257110645729E-14,15.2,-1.77635683940025E-14));
#290032=CARTESIAN_POINT('',(-4.12144986800006,15.2,-10.736091047));
#290033=CARTESIAN_POINT('',(-3.76106045600006,15.2,-10.867585944));
#290034=CARTESIAN_POINT('Origin',(-5.66257110645729E-14,15.2,-1.77635683940025E-14));
#290035=CARTESIAN_POINT('',(-3.76106045600006,12.2,-10.867585944));
#290036=CARTESIAN_POINT('',(-3.76106045600006,15.2,-10.867585944));
#290037=CARTESIAN_POINT('',(-4.12144986800006,12.2,-10.736091047));
#290038=CARTESIAN_POINT('Origin',(-5.66257110645729E-14,12.2,-1.77635683940025E-14));
#290039=CARTESIAN_POINT('',(-4.12144986800006,15.2,-10.736091047));
#290040=CARTESIAN_POINT('Ctrl Pts',(-3.76106045600006,15.2,-10.867585944));
#290041=CARTESIAN_POINT('Ctrl Pts',(-3.76106045600006,11.6,-10.867585944));
#290042=CARTESIAN_POINT('Ctrl Pts',(-3.76051902400006,15.2,-10.867046091));
#290043=CARTESIAN_POINT('Ctrl Pts',(-3.76051902400006,11.6,-10.867046091));
#290044=CARTESIAN_POINT('Ctrl Pts',(-3.75943667400006,15.2,-10.865966493));
#290045=CARTESIAN_POINT('Ctrl Pts',(-3.75943667400006,11.6,-10.865966493));
#290046=CARTESIAN_POINT('Ctrl Pts',(-3.75781469800006,15.2,-10.864347421));
#290047=CARTESIAN_POINT('Ctrl Pts',(-3.75781469800006,11.6,-10.864347421));
#290048=CARTESIAN_POINT('Ctrl Pts',(-3.75565515700006,15.2,-10.862189303));
#290049=CARTESIAN_POINT('Ctrl Pts',(-3.75565515700006,11.6,-10.862189303));
#290050=CARTESIAN_POINT('Ctrl Pts',(-3.75296088400006,15.2,-10.85949273));
#290051=CARTESIAN_POINT('Ctrl Pts',(-3.75296088400006,11.6,-10.85949273));
#290052=CARTESIAN_POINT('Ctrl Pts',(-3.75027176800006,15.2,-10.856797236));
#290053=CARTESIAN_POINT('Ctrl Pts',(-3.75027176800006,11.6,-10.856797236));
#290054=CARTESIAN_POINT('Ctrl Pts',(-3.74758780900006,15.2,-10.854102821));
#290055=CARTESIAN_POINT('Ctrl Pts',(-3.74758780900006,11.6,-10.854102821));
#290056=CARTESIAN_POINT('Ctrl Pts',(-3.74490900600006,15.2,-10.851409491));
#290057=CARTESIAN_POINT('Ctrl Pts',(-3.74490900600006,11.6,-10.851409491));
#290058=CARTESIAN_POINT('Ctrl Pts',(-3.74223536200006,15.2,-10.848717249));
#290059=CARTESIAN_POINT('Ctrl Pts',(-3.74223536200006,11.6,-10.848717249));
#290060=CARTESIAN_POINT('Ctrl Pts',(-3.73956687400006,15.2,-10.846026106));
#290061=CARTESIAN_POINT('Ctrl Pts',(-3.73956687400006,11.6,-10.846026106));
#290062=CARTESIAN_POINT('Ctrl Pts',(-3.73690354800006,15.2,-10.843336071));
#290063=CARTESIAN_POINT('Ctrl Pts',(-3.73690354800006,11.6,-10.843336071));
#290064=CARTESIAN_POINT('Ctrl Pts',(-3.73424538200006,15.2,-10.840647153));
#290065=CARTESIAN_POINT('Ctrl Pts',(-3.73424538200006,11.6,-10.840647153));
#290066=CARTESIAN_POINT('Ctrl Pts',(-3.73159237800006,15.2,-10.837959365));
#290067=CARTESIAN_POINT('Ctrl Pts',(-3.73159237800006,11.6,-10.837959365));
#290068=CARTESIAN_POINT('Ctrl Pts',(-3.72894453900006,15.2,-10.835272718));
#290069=CARTESIAN_POINT('Ctrl Pts',(-3.72894453900006,11.6,-10.835272718));
#290070=CARTESIAN_POINT('Ctrl Pts',(-3.72630186200006,15.2,-10.832587221));
#290071=CARTESIAN_POINT('Ctrl Pts',(-3.72630186200006,11.6,-10.832587221));
#290072=CARTESIAN_POINT('Ctrl Pts',(-3.72366435200005,15.2,-10.829902884));
#290073=CARTESIAN_POINT('Ctrl Pts',(-3.72366435200005,11.6,-10.829902884));
#290074=CARTESIAN_POINT('Ctrl Pts',(-3.72103200800006,15.2,-10.827219715));
#290075=CARTESIAN_POINT('Ctrl Pts',(-3.72103200800006,11.6,-10.827219715));
#290076=CARTESIAN_POINT('Ctrl Pts',(-3.71840483000006,15.2,-10.824537725));
#290077=CARTESIAN_POINT('Ctrl Pts',(-3.71840483000006,11.6,-10.824537725));
#290078=CARTESIAN_POINT('Ctrl Pts',(-3.71578282100006,15.2,-10.821856919));
#290079=CARTESIAN_POINT('Ctrl Pts',(-3.71578282100006,11.6,-10.821856919));
#290080=CARTESIAN_POINT('Ctrl Pts',(-3.71316598200006,15.2,-10.819177306));
#290081=CARTESIAN_POINT('Ctrl Pts',(-3.71316598200006,11.6,-10.819177306));
#290082=CARTESIAN_POINT('Ctrl Pts',(-3.71055431200006,15.2,-10.816498895));
#290083=CARTESIAN_POINT('Ctrl Pts',(-3.71055431200006,11.6,-10.816498895));
#290084=CARTESIAN_POINT('Ctrl Pts',(-3.70794781300006,15.2,-10.813821694));
#290085=CARTESIAN_POINT('Ctrl Pts',(-3.70794781300006,11.6,-10.813821694));
#290086=CARTESIAN_POINT('Ctrl Pts',(-3.70534648600006,15.2,-10.811145713));
#290087=CARTESIAN_POINT('Ctrl Pts',(-3.70534648600006,11.6,-10.811145713));
#290088=CARTESIAN_POINT('Ctrl Pts',(-3.70275033200006,15.2,-10.808470962));
#290089=CARTESIAN_POINT('Ctrl Pts',(-3.70275033200006,11.6,-10.808470962));
#290090=CARTESIAN_POINT('Ctrl Pts',(-3.70015935100006,15.2,-10.805797449));
#290091=CARTESIAN_POINT('Ctrl Pts',(-3.70015935100006,11.6,-10.805797449));
#290092=CARTESIAN_POINT('Ctrl Pts',(-3.69757354500006,15.2,-10.803125185));
#290093=CARTESIAN_POINT('Ctrl Pts',(-3.69757354500006,11.6,-10.803125185));
#290094=CARTESIAN_POINT('Ctrl Pts',(-3.69499291500006,15.2,-10.800454178));
#290095=CARTESIAN_POINT('Ctrl Pts',(-3.69499291500006,11.6,-10.800454178));
#290096=CARTESIAN_POINT('Ctrl Pts',(-3.69241746100006,15.2,-10.797784438));
#290097=CARTESIAN_POINT('Ctrl Pts',(-3.69241746100006,11.6,-10.797784438));
#290098=CARTESIAN_POINT('Ctrl Pts',(-3.68984718500006,15.2,-10.795115973));
#290099=CARTESIAN_POINT('Ctrl Pts',(-3.68984718500006,11.6,-10.795115973));
#290100=CARTESIAN_POINT('Ctrl Pts',(-3.68728208700006,15.2,-10.792448794));
#290101=CARTESIAN_POINT('Ctrl Pts',(-3.68728208700006,11.6,-10.792448794));
#290102=CARTESIAN_POINT('Ctrl Pts',(-3.68472216800006,15.2,-10.789782909));
#290103=CARTESIAN_POINT('Ctrl Pts',(-3.68472216800006,11.6,-10.789782909));
#290104=CARTESIAN_POINT('Ctrl Pts',(-3.68216742900006,15.2,-10.787118327));
#290105=CARTESIAN_POINT('Ctrl Pts',(-3.68216742900006,11.6,-10.787118327));
#290106=CARTESIAN_POINT('Ctrl Pts',(-3.67961787200006,15.2,-10.784455056));
#290107=CARTESIAN_POINT('Ctrl Pts',(-3.67961787200006,11.6,-10.784455056));
#290108=CARTESIAN_POINT('Ctrl Pts',(-3.67707349600006,15.2,-10.781793107));
#290109=CARTESIAN_POINT('Ctrl Pts',(-3.67707349600006,11.6,-10.781793107));
#290110=CARTESIAN_POINT('Ctrl Pts',(-3.67453430300006,15.2,-10.779132489));
#290111=CARTESIAN_POINT('Ctrl Pts',(-3.67453430300006,11.6,-10.779132489));
#290112=CARTESIAN_POINT('Ctrl Pts',(-3.67200029300006,15.2,-10.776473212));
#290113=CARTESIAN_POINT('Ctrl Pts',(-3.67200029300006,11.6,-10.776473212));
#290114=CARTESIAN_POINT('Ctrl Pts',(-3.66947146800006,15.2,-10.773815283));
#290115=CARTESIAN_POINT('Ctrl Pts',(-3.66947146800006,11.6,-10.773815283));
#290116=CARTESIAN_POINT('Ctrl Pts',(-3.66694782800006,15.2,-10.771158713));
#290117=CARTESIAN_POINT('Ctrl Pts',(-3.66694782800006,11.6,-10.771158713));
#290118=CARTESIAN_POINT('Ctrl Pts',(-3.66442937500006,15.2,-10.768503511));
#290119=CARTESIAN_POINT('Ctrl Pts',(-3.66442937500006,11.6,-10.768503511));
#290120=CARTESIAN_POINT('Ctrl Pts',(-3.66191610700006,15.2,-10.765849687));
#290121=CARTESIAN_POINT('Ctrl Pts',(-3.66191610700006,11.6,-10.765849687));
#290122=CARTESIAN_POINT('Ctrl Pts',(-3.65940802900006,15.2,-10.76319725));
#290123=CARTESIAN_POINT('Ctrl Pts',(-3.65940802900006,11.6,-10.76319725));
#290124=CARTESIAN_POINT('Ctrl Pts',(-3.65690513800006,15.2,-10.760546209));
#290125=CARTESIAN_POINT('Ctrl Pts',(-3.65690513800006,11.6,-10.760546209));
#290126=CARTESIAN_POINT('Ctrl Pts',(-3.65440743700006,15.2,-10.757896573));
#290127=CARTESIAN_POINT('Ctrl Pts',(-3.65440743700006,11.6,-10.757896573));
#290128=CARTESIAN_POINT('Ctrl Pts',(-3.65191492700006,15.2,-10.755248352));
#290129=CARTESIAN_POINT('Ctrl Pts',(-3.65191492700006,11.6,-10.755248352));
#290130=CARTESIAN_POINT('Ctrl Pts',(-3.64942760700006,15.2,-10.752601556));
#290131=CARTESIAN_POINT('Ctrl Pts',(-3.64942760700006,11.6,-10.752601556));
#290132=CARTESIAN_POINT('Ctrl Pts',(-3.64694547900006,15.2,-10.749956194));
#290133=CARTESIAN_POINT('Ctrl Pts',(-3.64694547900006,11.6,-10.749956194));
#290134=CARTESIAN_POINT('Ctrl Pts',(-3.64446854400006,15.2,-10.747312274));
#290135=CARTESIAN_POINT('Ctrl Pts',(-3.64446854400006,11.6,-10.747312274));
#290136=CARTESIAN_POINT('Ctrl Pts',(-3.64199680200006,15.2,-10.744669809));
#290137=CARTESIAN_POINT('Ctrl Pts',(-3.64199680200006,11.6,-10.744669809));
#290138=CARTESIAN_POINT('Ctrl Pts',(-3.63953025500006,15.2,-10.742028805));
#290139=CARTESIAN_POINT('Ctrl Pts',(-3.63953025500006,11.6,-10.742028805));
#290140=CARTESIAN_POINT('Ctrl Pts',(-3.63706890200006,15.2,-10.739389272));
#290141=CARTESIAN_POINT('Ctrl Pts',(-3.63706890200006,11.6,-10.739389272));
#290142=CARTESIAN_POINT('Ctrl Pts',(-3.63461274600006,15.2,-10.736751221));
#290143=CARTESIAN_POINT('Ctrl Pts',(-3.63461274600006,11.6,-10.736751221));
#290144=CARTESIAN_POINT('Ctrl Pts',(-3.63216178500006,15.2,-10.734114661));
#290145=CARTESIAN_POINT('Ctrl Pts',(-3.63216178500006,11.6,-10.734114661));
#290146=CARTESIAN_POINT('Ctrl Pts',(-3.62971602300005,15.2,-10.731479603));
#290147=CARTESIAN_POINT('Ctrl Pts',(-3.62971602300005,11.6,-10.731479603));
#290148=CARTESIAN_POINT('Ctrl Pts',(-3.62727545800006,15.2,-10.728846054));
#290149=CARTESIAN_POINT('Ctrl Pts',(-3.62727545800006,11.6,-10.728846054));
#290150=CARTESIAN_POINT('Ctrl Pts',(-3.62484009100006,15.2,-10.726214024));
#290151=CARTESIAN_POINT('Ctrl Pts',(-3.62484009100006,11.6,-10.726214024));
#290152=CARTESIAN_POINT('Ctrl Pts',(-3.62240992500006,15.2,-10.723583524));
#290153=CARTESIAN_POINT('Ctrl Pts',(-3.62240992500006,11.6,-10.723583524));
#290154=CARTESIAN_POINT('Ctrl Pts',(-3.61998495800006,15.2,-10.720954563));
#290155=CARTESIAN_POINT('Ctrl Pts',(-3.61998495800006,11.6,-10.720954563));
#290156=CARTESIAN_POINT('Ctrl Pts',(-3.61756519300005,15.2,-10.71832715));
#290157=CARTESIAN_POINT('Ctrl Pts',(-3.61756519300005,11.6,-10.71832715));
#290158=CARTESIAN_POINT('Ctrl Pts',(-3.61515062900006,15.2,-10.715701296));
#290159=CARTESIAN_POINT('Ctrl Pts',(-3.61515062900006,11.6,-10.715701296));
#290160=CARTESIAN_POINT('Ctrl Pts',(-3.61274126800006,15.2,-10.713077011));
#290161=CARTESIAN_POINT('Ctrl Pts',(-3.61274126800006,11.6,-10.713077011));
#290162=CARTESIAN_POINT('Ctrl Pts',(-3.61033711000006,15.2,-10.710454301));
#290163=CARTESIAN_POINT('Ctrl Pts',(-3.61033711000006,11.6,-10.710454301));
#290164=CARTESIAN_POINT('Ctrl Pts',(-3.60793815500006,15.2,-10.707833181));
#290165=CARTESIAN_POINT('Ctrl Pts',(-3.60793815500006,11.6,-10.707833181));
#290166=CARTESIAN_POINT('Ctrl Pts',(-3.60554440400006,15.2,-10.705213657));
#290167=CARTESIAN_POINT('Ctrl Pts',(-3.60554440400006,11.6,-10.705213657));
#290168=CARTESIAN_POINT('Ctrl Pts',(-3.60315586000006,15.2,-10.70259574));
#290169=CARTESIAN_POINT('Ctrl Pts',(-3.60315586000006,11.6,-10.70259574));
#290170=CARTESIAN_POINT('Ctrl Pts',(-3.60077252100006,15.2,-10.699979441));
#290171=CARTESIAN_POINT('Ctrl Pts',(-3.60077252100006,11.6,-10.699979441));
#290172=CARTESIAN_POINT('Ctrl Pts',(-3.59839438800006,15.2,-10.697364767));
#290173=CARTESIAN_POINT('Ctrl Pts',(-3.59839438800006,11.6,-10.697364767));
#290174=CARTESIAN_POINT('Ctrl Pts',(-3.59602146300006,15.2,-10.69475173));
#290175=CARTESIAN_POINT('Ctrl Pts',(-3.59602146300006,11.6,-10.69475173));
#290176=CARTESIAN_POINT('Ctrl Pts',(-3.59365374500006,15.2,-10.692140339));
#290177=CARTESIAN_POINT('Ctrl Pts',(-3.59365374500006,11.6,-10.692140339));
#290178=CARTESIAN_POINT('Ctrl Pts',(-3.59129123600006,15.2,-10.689530605));
#290179=CARTESIAN_POINT('Ctrl Pts',(-3.59129123600006,11.6,-10.689530605));
#290180=CARTESIAN_POINT('Ctrl Pts',(-3.58893393500006,15.2,-10.686922536));
#290181=CARTESIAN_POINT('Ctrl Pts',(-3.58893393500006,11.6,-10.686922536));
#290182=CARTESIAN_POINT('Ctrl Pts',(-3.58658184600006,15.2,-10.684316144));
#290183=CARTESIAN_POINT('Ctrl Pts',(-3.58658184600006,11.6,-10.684316144));
#290184=CARTESIAN_POINT('Ctrl Pts',(-3.58423496600006,15.2,-10.681711437));
#290185=CARTESIAN_POINT('Ctrl Pts',(-3.58423496600006,11.6,-10.681711437));
#290186=CARTESIAN_POINT('Ctrl Pts',(-3.58189329600005,15.2,-10.679108426));
#290187=CARTESIAN_POINT('Ctrl Pts',(-3.58189329600005,11.6,-10.679108426));
#290188=CARTESIAN_POINT('Ctrl Pts',(-3.57955683800006,15.2,-10.67650712));
#290189=CARTESIAN_POINT('Ctrl Pts',(-3.57955683800006,11.6,-10.67650712));
#290190=CARTESIAN_POINT('Ctrl Pts',(-3.57722559400006,15.2,-10.67390753));
#290191=CARTESIAN_POINT('Ctrl Pts',(-3.57722559400006,11.6,-10.67390753));
#290192=CARTESIAN_POINT('Ctrl Pts',(-3.57489956100006,15.2,-10.671309667));
#290193=CARTESIAN_POINT('Ctrl Pts',(-3.57489956100006,11.6,-10.671309667));
#290194=CARTESIAN_POINT('Ctrl Pts',(-3.57257874200006,15.2,-10.668713538));
#290195=CARTESIAN_POINT('Ctrl Pts',(-3.57257874200006,11.6,-10.668713538));
#290196=CARTESIAN_POINT('Ctrl Pts',(-3.57026313700006,15.2,-10.666119155));
#290197=CARTESIAN_POINT('Ctrl Pts',(-3.57026313700006,11.6,-10.666119155));
#290198=CARTESIAN_POINT('Ctrl Pts',(-3.56795274700006,15.2,-10.663526528));
#290199=CARTESIAN_POINT('Ctrl Pts',(-3.56795274700006,11.6,-10.663526528));
#290200=CARTESIAN_POINT('Ctrl Pts',(-3.56564757100006,15.2,-10.660935667));
#290201=CARTESIAN_POINT('Ctrl Pts',(-3.56564757100006,11.6,-10.660935667));
#290202=CARTESIAN_POINT('Ctrl Pts',(-3.56334761200006,15.2,-10.658346582));
#290203=CARTESIAN_POINT('Ctrl Pts',(-3.56334761200006,11.6,-10.658346582));
#290204=CARTESIAN_POINT('Ctrl Pts',(-3.56105286900006,15.2,-10.655759283));
#290205=CARTESIAN_POINT('Ctrl Pts',(-3.56105286900006,11.6,-10.655759283));
#290206=CARTESIAN_POINT('Ctrl Pts',(-3.55876334100006,15.2,-10.65317378));
#290207=CARTESIAN_POINT('Ctrl Pts',(-3.55876334100006,11.6,-10.65317378));
#290208=CARTESIAN_POINT('Ctrl Pts',(-3.55647903300006,15.2,-10.650590083));
#290209=CARTESIAN_POINT('Ctrl Pts',(-3.55647903300006,11.6,-10.650590083));
#290210=CARTESIAN_POINT('Ctrl Pts',(-3.55419994100005,15.2,-10.648008202));
#290211=CARTESIAN_POINT('Ctrl Pts',(-3.55419994100005,11.6,-10.648008202));
#290212=CARTESIAN_POINT('Ctrl Pts',(-3.55192606900006,15.2,-10.645428149));
#290213=CARTESIAN_POINT('Ctrl Pts',(-3.55192606900006,11.6,-10.645428149));
#290214=CARTESIAN_POINT('Ctrl Pts',(-3.54965741500005,15.2,-10.642849932));
#290215=CARTESIAN_POINT('Ctrl Pts',(-3.54965741500005,11.6,-10.642849932));
#290216=CARTESIAN_POINT('Ctrl Pts',(-3.54739398000006,15.2,-10.640273563));
#290217=CARTESIAN_POINT('Ctrl Pts',(-3.54739398000006,11.6,-10.640273563));
#290218=CARTESIAN_POINT('Ctrl Pts',(-3.54513576600006,15.2,-10.63769905));
#290219=CARTESIAN_POINT('Ctrl Pts',(-3.54513576600006,11.6,-10.63769905));
#290220=CARTESIAN_POINT('Ctrl Pts',(-3.54288277300006,15.2,-10.635126405));
#290221=CARTESIAN_POINT('Ctrl Pts',(-3.54288277300006,11.6,-10.635126405));
#290222=CARTESIAN_POINT('Ctrl Pts',(-3.54063499900006,15.2,-10.632555638));
#290223=CARTESIAN_POINT('Ctrl Pts',(-3.54063499900006,11.6,-10.632555638));
#290224=CARTESIAN_POINT('Ctrl Pts',(-3.53839244700006,15.2,-10.62998676));
#290225=CARTESIAN_POINT('Ctrl Pts',(-3.53839244700006,11.6,-10.62998676));
#290226=CARTESIAN_POINT('Ctrl Pts',(-3.53615511800006,15.2,-10.627419779));
#290227=CARTESIAN_POINT('Ctrl Pts',(-3.53615511800006,11.6,-10.627419779));
#290228=CARTESIAN_POINT('Ctrl Pts',(-3.53392301000006,15.2,-10.624854708));
#290229=CARTESIAN_POINT('Ctrl Pts',(-3.53392301000006,11.6,-10.624854708));
#290230=CARTESIAN_POINT('Ctrl Pts',(-3.53169612600006,15.2,-10.622291556));
#290231=CARTESIAN_POINT('Ctrl Pts',(-3.53169612600006,11.6,-10.622291556));
#290232=CARTESIAN_POINT('Ctrl Pts',(-3.52947446500006,15.2,-10.619730333));
#290233=CARTESIAN_POINT('Ctrl Pts',(-3.52947446500006,11.6,-10.619730333));
#290234=CARTESIAN_POINT('Ctrl Pts',(-3.52725802800006,15.2,-10.617171052));
#290235=CARTESIAN_POINT('Ctrl Pts',(-3.52725802800006,11.6,-10.617171052));
#290236=CARTESIAN_POINT('Ctrl Pts',(-3.52504681500006,15.2,-10.614613719));
#290237=CARTESIAN_POINT('Ctrl Pts',(-3.52504681500006,11.6,-10.614613719));
#290238=CARTESIAN_POINT('Ctrl Pts',(-3.52284082700006,15.2,-10.612058348));
#290239=CARTESIAN_POINT('Ctrl Pts',(-3.52284082700006,11.6,-10.612058348));
#290240=CARTESIAN_POINT('Ctrl Pts',(-3.52064006300006,15.2,-10.609504949));
#290241=CARTESIAN_POINT('Ctrl Pts',(-3.52064006300006,11.6,-10.609504949));
#290242=CARTESIAN_POINT('Ctrl Pts',(-3.51844452500006,15.2,-10.606953531));
#290243=CARTESIAN_POINT('Ctrl Pts',(-3.51844452500006,11.6,-10.606953531));
#290244=CARTESIAN_POINT('Ctrl Pts',(-3.51625421300006,15.2,-10.604404105));
#290245=CARTESIAN_POINT('Ctrl Pts',(-3.51625421300006,11.6,-10.604404105));
#290246=CARTESIAN_POINT('Ctrl Pts',(-3.51406912700006,15.2,-10.601856682));
#290247=CARTESIAN_POINT('Ctrl Pts',(-3.51406912700006,11.6,-10.601856682));
#290248=CARTESIAN_POINT('Ctrl Pts',(-3.51188926800006,15.2,-10.599311274));
#290249=CARTESIAN_POINT('Ctrl Pts',(-3.51188926800006,11.6,-10.599311274));
#290250=CARTESIAN_POINT('Ctrl Pts',(-3.50971463700006,15.2,-10.596767888));
#290251=CARTESIAN_POINT('Ctrl Pts',(-3.50971463700006,11.6,-10.596767888));
#290252=CARTESIAN_POINT('Ctrl Pts',(-3.50754523300006,15.2,-10.594226538));
#290253=CARTESIAN_POINT('Ctrl Pts',(-3.50754523300006,11.6,-10.594226538));
#290254=CARTESIAN_POINT('Ctrl Pts',(-3.50538105600006,15.2,-10.591687232));
#290255=CARTESIAN_POINT('Ctrl Pts',(-3.50538105600006,11.6,-10.591687232));
#290256=CARTESIAN_POINT('Ctrl Pts',(-3.50322210700006,15.2,-10.589149983));
#290257=CARTESIAN_POINT('Ctrl Pts',(-3.50322210700006,11.6,-10.589149983));
#290258=CARTESIAN_POINT('Ctrl Pts',(-3.50106838800006,15.2,-10.586614801));
#290259=CARTESIAN_POINT('Ctrl Pts',(-3.50106838800006,11.6,-10.586614801));
#290260=CARTESIAN_POINT('Ctrl Pts',(-3.49891989700006,15.2,-10.584081695));
#290261=CARTESIAN_POINT('Ctrl Pts',(-3.49891989700006,11.6,-10.584081695));
#290262=CARTESIAN_POINT('Ctrl Pts',(-3.49677663600006,15.2,-10.581550677));
#290263=CARTESIAN_POINT('Ctrl Pts',(-3.49677663600006,11.6,-10.581550677));
#290264=CARTESIAN_POINT('Ctrl Pts',(-3.49463860300005,15.2,-10.579021757));
#290265=CARTESIAN_POINT('Ctrl Pts',(-3.49463860300005,11.6,-10.579021757));
#290266=CARTESIAN_POINT('Ctrl Pts',(-3.49250580100006,15.2,-10.576494948));
#290267=CARTESIAN_POINT('Ctrl Pts',(-3.49250580100006,11.6,-10.576494948));
#290268=CARTESIAN_POINT('Ctrl Pts',(-3.49037822900006,15.2,-10.573970258));
#290269=CARTESIAN_POINT('Ctrl Pts',(-3.49037822900006,11.6,-10.573970258));
#290270=CARTESIAN_POINT('Ctrl Pts',(-3.48825588700006,15.2,-10.571447699));
#290271=CARTESIAN_POINT('Ctrl Pts',(-3.48825588700006,11.6,-10.571447699));
#290272=CARTESIAN_POINT('Ctrl Pts',(-3.48613877700005,15.2,-10.568927282));
#290273=CARTESIAN_POINT('Ctrl Pts',(-3.48613877700005,11.6,-10.568927282));
#290274=CARTESIAN_POINT('Ctrl Pts',(-3.48402689800006,15.2,-10.566409018));
#290275=CARTESIAN_POINT('Ctrl Pts',(-3.48402689800006,11.6,-10.566409018));
#290276=CARTESIAN_POINT('Ctrl Pts',(-3.48192025100006,15.2,-10.563892917));
#290277=CARTESIAN_POINT('Ctrl Pts',(-3.48192025100006,11.6,-10.563892917));
#290278=CARTESIAN_POINT('Ctrl Pts',(-3.47981883400006,15.2,-10.56137899));
#290279=CARTESIAN_POINT('Ctrl Pts',(-3.47981883400006,11.6,-10.56137899));
#290280=CARTESIAN_POINT('Ctrl Pts',(-3.47772265000006,15.2,-10.558867249));
#290281=CARTESIAN_POINT('Ctrl Pts',(-3.47772265000006,11.6,-10.558867249));
#290282=CARTESIAN_POINT('Ctrl Pts',(-3.47563169800006,15.2,-10.556357703));
#290283=CARTESIAN_POINT('Ctrl Pts',(-3.47563169800006,11.6,-10.556357703));
#290284=CARTESIAN_POINT('Ctrl Pts',(-3.47354597800006,15.2,-10.553850365));
#290285=CARTESIAN_POINT('Ctrl Pts',(-3.47354597800006,11.6,-10.553850365));
#290286=CARTESIAN_POINT('Ctrl Pts',(-3.47146549200006,15.2,-10.551345245));
#290287=CARTESIAN_POINT('Ctrl Pts',(-3.47146549200006,11.6,-10.551345245));
#290288=CARTESIAN_POINT('Ctrl Pts',(-3.46939023800005,15.2,-10.548842353));
#290289=CARTESIAN_POINT('Ctrl Pts',(-3.46939023800005,11.6,-10.548842353));
#290290=CARTESIAN_POINT('Ctrl Pts',(-3.46732021800006,15.2,-10.546341702));
#290291=CARTESIAN_POINT('Ctrl Pts',(-3.46732021800006,11.6,-10.546341702));
#290292=CARTESIAN_POINT('Ctrl Pts',(-3.46525543000006,15.2,-10.543843302));
#290293=CARTESIAN_POINT('Ctrl Pts',(-3.46525543000006,11.6,-10.543843302));
#290294=CARTESIAN_POINT('Ctrl Pts',(-3.46319587600005,15.2,-10.541347163));
#290295=CARTESIAN_POINT('Ctrl Pts',(-3.46319587600005,11.6,-10.541347163));
#290296=CARTESIAN_POINT('Ctrl Pts',(-3.46114155700006,15.2,-10.538853298));
#290297=CARTESIAN_POINT('Ctrl Pts',(-3.46114155700006,11.6,-10.538853298));
#290298=CARTESIAN_POINT('Ctrl Pts',(-3.45909247200006,15.2,-10.536361717));
#290299=CARTESIAN_POINT('Ctrl Pts',(-3.45909247200006,11.6,-10.536361717));
#290300=CARTESIAN_POINT('Ctrl Pts',(-3.45704862000006,15.2,-10.533872432));
#290301=CARTESIAN_POINT('Ctrl Pts',(-3.45704862000006,11.6,-10.533872432));
#290302=CARTESIAN_POINT('Ctrl Pts',(-3.45501000300006,15.2,-10.531385453));
#290303=CARTESIAN_POINT('Ctrl Pts',(-3.45501000300006,11.6,-10.531385453));
#290304=CARTESIAN_POINT('Ctrl Pts',(-3.45297662200006,15.2,-10.528900792));
#290305=CARTESIAN_POINT('Ctrl Pts',(-3.45297662200006,11.6,-10.528900792));
#290306=CARTESIAN_POINT('Ctrl Pts',(-3.45094847400006,15.2,-10.52641846));
#290307=CARTESIAN_POINT('Ctrl Pts',(-3.45094847400006,11.6,-10.52641846));
#290308=CARTESIAN_POINT('Ctrl Pts',(-3.44892556100006,15.2,-10.523938468));
#290309=CARTESIAN_POINT('Ctrl Pts',(-3.44892556100006,11.6,-10.523938468));
#290310=CARTESIAN_POINT('Ctrl Pts',(-3.44690788300006,15.2,-10.521460828));
#290311=CARTESIAN_POINT('Ctrl Pts',(-3.44690788300006,11.6,-10.521460828));
#290312=CARTESIAN_POINT('Ctrl Pts',(-3.44489544100006,15.2,-10.518985549));
#290313=CARTESIAN_POINT('Ctrl Pts',(-3.44489544100006,11.6,-10.518985549));
#290314=CARTESIAN_POINT('Ctrl Pts',(-3.44288823300006,15.2,-10.516512646));
#290315=CARTESIAN_POINT('Ctrl Pts',(-3.44288823300006,11.6,-10.516512646));
#290316=CARTESIAN_POINT('Ctrl Pts',(-3.44088626200006,15.2,-10.514042127));
#290317=CARTESIAN_POINT('Ctrl Pts',(-3.44088626200006,11.6,-10.514042127));
#290318=CARTESIAN_POINT('Ctrl Pts',(-3.43888952500006,15.2,-10.511574004));
#290319=CARTESIAN_POINT('Ctrl Pts',(-3.43888952500006,11.6,-10.511574004));
#290320=CARTESIAN_POINT('Ctrl Pts',(-3.43689802500006,15.2,-10.50910829));
#290321=CARTESIAN_POINT('Ctrl Pts',(-3.43689802500006,11.6,-10.50910829));
#290322=CARTESIAN_POINT('Ctrl Pts',(-3.43491176000006,15.2,-10.506644995));
#290323=CARTESIAN_POINT('Ctrl Pts',(-3.43491176000006,11.6,-10.506644995));
#290324=CARTESIAN_POINT('Ctrl Pts',(-3.43293073100006,15.2,-10.504184131));
#290325=CARTESIAN_POINT('Ctrl Pts',(-3.43293073100006,11.6,-10.504184131));
#290326=CARTESIAN_POINT('Ctrl Pts',(-3.43095493700006,15.2,-10.501725709));
#290327=CARTESIAN_POINT('Ctrl Pts',(-3.43095493700006,11.6,-10.501725709));
#290328=CARTESIAN_POINT('Ctrl Pts',(-3.42898438100006,15.2,-10.49926974));
#290329=CARTESIAN_POINT('Ctrl Pts',(-3.42898438100006,11.6,-10.49926974));
#290330=CARTESIAN_POINT('Ctrl Pts',(-3.42701905900006,15.2,-10.496816237));
#290331=CARTESIAN_POINT('Ctrl Pts',(-3.42701905900006,11.6,-10.496816237));
#290332=CARTESIAN_POINT('Ctrl Pts',(-3.42505897400006,15.2,-10.49436521));
#290333=CARTESIAN_POINT('Ctrl Pts',(-3.42505897400006,11.6,-10.49436521));
#290334=CARTESIAN_POINT('Ctrl Pts',(-3.42310412600006,15.2,-10.491916672));
#290335=CARTESIAN_POINT('Ctrl Pts',(-3.42310412600006,11.6,-10.491916672));
#290336=CARTESIAN_POINT('Ctrl Pts',(-3.42115451300006,15.2,-10.489470633));
#290337=CARTESIAN_POINT('Ctrl Pts',(-3.42115451300006,11.6,-10.489470633));
#290338=CARTESIAN_POINT('Ctrl Pts',(-3.41921013600006,15.2,-10.487027105));
#290339=CARTESIAN_POINT('Ctrl Pts',(-3.41921013600006,11.6,-10.487027105));
#290340=CARTESIAN_POINT('Ctrl Pts',(-3.41727099700006,15.2,-10.484586099));
#290341=CARTESIAN_POINT('Ctrl Pts',(-3.41727099700006,11.6,-10.484586099));
#290342=CARTESIAN_POINT('Ctrl Pts',(-3.41533709200006,15.2,-10.482147629));
#290343=CARTESIAN_POINT('Ctrl Pts',(-3.41533709200006,11.6,-10.482147629));
#290344=CARTESIAN_POINT('Ctrl Pts',(-3.41340842400006,15.2,-10.479711705));
#290345=CARTESIAN_POINT('Ctrl Pts',(-3.41340842400006,11.6,-10.479711705));
#290346=CARTESIAN_POINT('Ctrl Pts',(-3.41148499200005,15.2,-10.477278338));
#290347=CARTESIAN_POINT('Ctrl Pts',(-3.41148499200005,11.6,-10.477278338));
#290348=CARTESIAN_POINT('Ctrl Pts',(-3.40956679600006,15.2,-10.474847542));
#290349=CARTESIAN_POINT('Ctrl Pts',(-3.40956679600006,11.6,-10.474847542));
#290350=CARTESIAN_POINT('Ctrl Pts',(-3.40765383700006,15.2,-10.472419327));
#290351=CARTESIAN_POINT('Ctrl Pts',(-3.40765383700006,11.6,-10.472419327));
#290352=CARTESIAN_POINT('Ctrl Pts',(-3.40574611300006,15.2,-10.469993704));
#290353=CARTESIAN_POINT('Ctrl Pts',(-3.40574611300006,11.6,-10.469993704));
#290354=CARTESIAN_POINT('Ctrl Pts',(-3.40384362600005,15.2,-10.467570686));
#290355=CARTESIAN_POINT('Ctrl Pts',(-3.40384362600005,11.6,-10.467570686));
#290356=CARTESIAN_POINT('Ctrl Pts',(-3.40194637500006,15.2,-10.465150285));
#290357=CARTESIAN_POINT('Ctrl Pts',(-3.40194637500006,11.6,-10.465150285));
#290358=CARTESIAN_POINT('Ctrl Pts',(-3.40005435900005,15.2,-10.462732513));
#290359=CARTESIAN_POINT('Ctrl Pts',(-3.40005435900005,11.6,-10.462732513));
#290360=CARTESIAN_POINT('Ctrl Pts',(-3.39816757900006,15.2,-10.46031738));
#290361=CARTESIAN_POINT('Ctrl Pts',(-3.39816757900006,11.6,-10.46031738));
#290362=CARTESIAN_POINT('Ctrl Pts',(-3.39628603500006,15.2,-10.457904901));
#290363=CARTESIAN_POINT('Ctrl Pts',(-3.39628603500006,11.6,-10.457904901));
#290364=CARTESIAN_POINT('Ctrl Pts',(-3.39440972600006,15.2,-10.455495085));
#290365=CARTESIAN_POINT('Ctrl Pts',(-3.39440972600006,11.6,-10.455495085));
#290366=CARTESIAN_POINT('Ctrl Pts',(-3.39253865400006,15.2,-10.453087944));
#290367=CARTESIAN_POINT('Ctrl Pts',(-3.39253865400006,11.6,-10.453087944));
#290368=CARTESIAN_POINT('Ctrl Pts',(-3.39067281600005,15.2,-10.450683493));
#290369=CARTESIAN_POINT('Ctrl Pts',(-3.39067281600005,11.6,-10.450683493));
#290370=CARTESIAN_POINT('Ctrl Pts',(-3.38881221500006,15.2,-10.448281741));
#290371=CARTESIAN_POINT('Ctrl Pts',(-3.38881221500006,11.6,-10.448281741));
#290372=CARTESIAN_POINT('Ctrl Pts',(-3.38695684800005,15.2,-10.4458827));
#290373=CARTESIAN_POINT('Ctrl Pts',(-3.38695684800005,11.6,-10.4458827));
#290374=CARTESIAN_POINT('Ctrl Pts',(-3.38510671600006,15.2,-10.443486385));
#290375=CARTESIAN_POINT('Ctrl Pts',(-3.38510671600006,11.6,-10.443486385));
#290376=CARTESIAN_POINT('Ctrl Pts',(-3.38326181900006,15.2,-10.441092805));
#290377=CARTESIAN_POINT('Ctrl Pts',(-3.38326181900006,11.6,-10.441092805));
#290378=CARTESIAN_POINT('Ctrl Pts',(-3.38142215600006,15.2,-10.438701973));
#290379=CARTESIAN_POINT('Ctrl Pts',(-3.38142215600006,11.6,-10.438701973));
#290380=CARTESIAN_POINT('Ctrl Pts',(-3.37958772900006,15.2,-10.436313902));
#290381=CARTESIAN_POINT('Ctrl Pts',(-3.37958772900006,11.6,-10.436313902));
#290382=CARTESIAN_POINT('Ctrl Pts',(-3.37775853500006,15.2,-10.433928604));
#290383=CARTESIAN_POINT('Ctrl Pts',(-3.37775853500006,11.6,-10.433928604));
#290384=CARTESIAN_POINT('Ctrl Pts',(-3.37593457600006,15.2,-10.43154609));
#290385=CARTESIAN_POINT('Ctrl Pts',(-3.37593457600006,11.6,-10.43154609));
#290386=CARTESIAN_POINT('Ctrl Pts',(-3.37411585100006,15.2,-10.429166373));
#290387=CARTESIAN_POINT('Ctrl Pts',(-3.37411585100006,11.6,-10.429166373));
#290388=CARTESIAN_POINT('Ctrl Pts',(-3.37230235900006,15.2,-10.426789465));
#290389=CARTESIAN_POINT('Ctrl Pts',(-3.37230235900006,11.6,-10.426789465));
#290390=CARTESIAN_POINT('Ctrl Pts',(-3.37049410100006,15.2,-10.424415378));
#290391=CARTESIAN_POINT('Ctrl Pts',(-3.37049410100006,11.6,-10.424415378));
#290392=CARTESIAN_POINT('Ctrl Pts',(-3.36869107700006,15.2,-10.422044126));
#290393=CARTESIAN_POINT('Ctrl Pts',(-3.36869107700006,11.6,-10.422044126));
#290394=CARTESIAN_POINT('Ctrl Pts',(-3.36689328500006,15.2,-10.419675719));
#290395=CARTESIAN_POINT('Ctrl Pts',(-3.36689328500006,11.6,-10.419675719));
#290396=CARTESIAN_POINT('Ctrl Pts',(-3.36510072600006,15.2,-10.41731017));
#290397=CARTESIAN_POINT('Ctrl Pts',(-3.36510072600006,11.6,-10.41731017));
#290398=CARTESIAN_POINT('Ctrl Pts',(-3.36331340000006,15.2,-10.414947492));
#290399=CARTESIAN_POINT('Ctrl Pts',(-3.36331340000006,11.6,-10.414947492));
#290400=CARTESIAN_POINT('Ctrl Pts',(-3.36153130500006,15.2,-10.412587698));
#290401=CARTESIAN_POINT('Ctrl Pts',(-3.36153130500006,11.6,-10.412587698));
#290402=CARTESIAN_POINT('Ctrl Pts',(-3.35975444300006,15.2,-10.410230799));
#290403=CARTESIAN_POINT('Ctrl Pts',(-3.35975444300006,11.6,-10.410230799));
#290404=CARTESIAN_POINT('Ctrl Pts',(-3.35798281300006,15.2,-10.407876808));
#290405=CARTESIAN_POINT('Ctrl Pts',(-3.35798281300006,11.6,-10.407876808));
#290406=CARTESIAN_POINT('Ctrl Pts',(-3.35621641500006,15.2,-10.405525737));
#290407=CARTESIAN_POINT('Ctrl Pts',(-3.35621641500006,11.6,-10.405525737));
#290408=CARTESIAN_POINT('Ctrl Pts',(-3.35445524700006,15.2,-10.403177599));
#290409=CARTESIAN_POINT('Ctrl Pts',(-3.35445524700006,11.6,-10.403177599));
#290410=CARTESIAN_POINT('Ctrl Pts',(-3.35269931000005,15.2,-10.400832408));
#290411=CARTESIAN_POINT('Ctrl Pts',(-3.35269931000005,11.6,-10.400832408));
#290412=CARTESIAN_POINT('Ctrl Pts',(-3.35094860200006,15.2,-10.398490174));
#290413=CARTESIAN_POINT('Ctrl Pts',(-3.35094860200006,11.6,-10.398490174));
#290414=CARTESIAN_POINT('Ctrl Pts',(-3.34920312700006,15.2,-10.39615091));
#290415=CARTESIAN_POINT('Ctrl Pts',(-3.34920312700006,11.6,-10.39615091));
#290416=CARTESIAN_POINT('Ctrl Pts',(-3.34746288000006,15.2,-10.393814631));
#290417=CARTESIAN_POINT('Ctrl Pts',(-3.34746288000006,11.6,-10.393814631));
#290418=CARTESIAN_POINT('Ctrl Pts',(-3.34572786200006,15.2,-10.391481347));
#290419=CARTESIAN_POINT('Ctrl Pts',(-3.34572786200006,11.6,-10.391481347));
#290420=CARTESIAN_POINT('Ctrl Pts',(-3.34399807300006,15.2,-10.389151072));
#290421=CARTESIAN_POINT('Ctrl Pts',(-3.34399807300006,11.6,-10.389151072));
#290422=CARTESIAN_POINT('Ctrl Pts',(-3.34227351400005,15.2,-10.386823819));
#290423=CARTESIAN_POINT('Ctrl Pts',(-3.34227351400005,11.6,-10.386823819));
#290424=CARTESIAN_POINT('Ctrl Pts',(-3.34055418200006,15.2,-10.384499599));
#290425=CARTESIAN_POINT('Ctrl Pts',(-3.34055418200006,11.6,-10.384499599));
#290426=CARTESIAN_POINT('Ctrl Pts',(-3.33884007800005,15.2,-10.382178426));
#290427=CARTESIAN_POINT('Ctrl Pts',(-3.33884007800005,11.6,-10.382178426));
#290428=CARTESIAN_POINT('Ctrl Pts',(-3.33713120200006,15.2,-10.379860314));
#290429=CARTESIAN_POINT('Ctrl Pts',(-3.33713120200006,11.6,-10.379860314));
#290430=CARTESIAN_POINT('Ctrl Pts',(-3.33542755300006,15.2,-10.377545273));
#290431=CARTESIAN_POINT('Ctrl Pts',(-3.33542755300006,11.6,-10.377545273));
#290432=CARTESIAN_POINT('Ctrl Pts',(-3.33372912900006,15.2,-10.375233318));
#290433=CARTESIAN_POINT('Ctrl Pts',(-3.33372912900006,11.6,-10.375233318));
#290434=CARTESIAN_POINT('Ctrl Pts',(-3.33203593200006,15.2,-10.372924463));
#290435=CARTESIAN_POINT('Ctrl Pts',(-3.33203593200006,11.6,-10.372924463));
#290436=CARTESIAN_POINT('Ctrl Pts',(-3.33034796100006,15.2,-10.370618717));
#290437=CARTESIAN_POINT('Ctrl Pts',(-3.33034796100006,11.6,-10.370618717));
#290438=CARTESIAN_POINT('Ctrl Pts',(-3.32866521500006,15.2,-10.368316097));
#290439=CARTESIAN_POINT('Ctrl Pts',(-3.32866521500006,11.6,-10.368316097));
#290440=CARTESIAN_POINT('Ctrl Pts',(-3.32698769400006,15.2,-10.366016613));
#290441=CARTESIAN_POINT('Ctrl Pts',(-3.32698769400006,11.6,-10.366016613));
#290442=CARTESIAN_POINT('Ctrl Pts',(-3.32531539700006,15.2,-10.36372028));
#290443=CARTESIAN_POINT('Ctrl Pts',(-3.32531539700006,11.6,-10.36372028));
#290444=CARTESIAN_POINT('Ctrl Pts',(-3.32364832400006,15.2,-10.36142711));
#290445=CARTESIAN_POINT('Ctrl Pts',(-3.32364832400006,11.6,-10.36142711));
#290446=CARTESIAN_POINT('Ctrl Pts',(-3.32198647300006,15.2,-10.359137116));
#290447=CARTESIAN_POINT('Ctrl Pts',(-3.32198647300006,11.6,-10.359137116));
#290448=CARTESIAN_POINT('Ctrl Pts',(-3.32032984600006,15.2,-10.356850314));
#290449=CARTESIAN_POINT('Ctrl Pts',(-3.32032984600006,11.6,-10.356850314));
#290450=CARTESIAN_POINT('Ctrl Pts',(-3.31867844000006,15.2,-10.354566711));
#290451=CARTESIAN_POINT('Ctrl Pts',(-3.31867844000006,11.6,-10.354566711));
#290452=CARTESIAN_POINT('Ctrl Pts',(-3.31703225600006,15.2,-10.352286326));
#290453=CARTESIAN_POINT('Ctrl Pts',(-3.31703225600006,11.6,-10.352286326));
#290454=CARTESIAN_POINT('Ctrl Pts',(-3.31539129200006,15.2,-10.35000917));
#290455=CARTESIAN_POINT('Ctrl Pts',(-3.31539129200006,11.6,-10.35000917));
#290456=CARTESIAN_POINT('Ctrl Pts',(-3.31375555000006,15.2,-10.347735256));
#290457=CARTESIAN_POINT('Ctrl Pts',(-3.31375555000006,11.6,-10.347735256));
#290458=CARTESIAN_POINT('Ctrl Pts',(-3.31212502800006,15.2,-10.345464598));
#290459=CARTESIAN_POINT('Ctrl Pts',(-3.31212502800006,11.6,-10.345464598));
#290460=CARTESIAN_POINT('Ctrl Pts',(-3.31049972400006,15.2,-10.343197208));
#290461=CARTESIAN_POINT('Ctrl Pts',(-3.31049972400006,11.6,-10.343197208));
#290462=CARTESIAN_POINT('Ctrl Pts',(-3.30887963900006,15.2,-10.340933101));
#290463=CARTESIAN_POINT('Ctrl Pts',(-3.30887963900006,11.6,-10.340933101));
#290464=CARTESIAN_POINT('Ctrl Pts',(-3.30726477200006,15.2,-10.338672289));
#290465=CARTESIAN_POINT('Ctrl Pts',(-3.30726477200006,11.6,-10.338672289));
#290466=CARTESIAN_POINT('Ctrl Pts',(-3.30565512200006,15.2,-10.336414787));
#290467=CARTESIAN_POINT('Ctrl Pts',(-3.30565512200006,11.6,-10.336414787));
#290468=CARTESIAN_POINT('Ctrl Pts',(-3.30405069000005,15.2,-10.334160607));
#290469=CARTESIAN_POINT('Ctrl Pts',(-3.30405069000005,11.6,-10.334160607));
#290470=CARTESIAN_POINT('Ctrl Pts',(-3.30245147400006,15.2,-10.331909762));
#290471=CARTESIAN_POINT('Ctrl Pts',(-3.30245147400006,11.6,-10.331909762));
#290472=CARTESIAN_POINT('Ctrl Pts',(-3.30085747200005,15.2,-10.329662267));
#290473=CARTESIAN_POINT('Ctrl Pts',(-3.30085747200005,11.6,-10.329662267));
#290474=CARTESIAN_POINT('Ctrl Pts',(-3.29926868600006,15.2,-10.327418135));
#290475=CARTESIAN_POINT('Ctrl Pts',(-3.29926868600006,11.6,-10.327418135));
#290476=CARTESIAN_POINT('Ctrl Pts',(-3.29768511500005,15.2,-10.32517738));
#290477=CARTESIAN_POINT('Ctrl Pts',(-3.29768511500005,11.6,-10.32517738));
#290478=CARTESIAN_POINT('Ctrl Pts',(-3.29610675600006,15.2,-10.322940015));
#290479=CARTESIAN_POINT('Ctrl Pts',(-3.29610675600006,11.6,-10.322940015));
#290480=CARTESIAN_POINT('Ctrl Pts',(-3.29453360900006,15.2,-10.320706053));
#290481=CARTESIAN_POINT('Ctrl Pts',(-3.29453360900006,11.6,-10.320706053));
#290482=CARTESIAN_POINT('Ctrl Pts',(-3.29296567600006,15.2,-10.318475508));
#290483=CARTESIAN_POINT('Ctrl Pts',(-3.29296567600006,11.6,-10.318475508));
#290484=CARTESIAN_POINT('Ctrl Pts',(-3.29140295200005,15.2,-10.316248395));
#290485=CARTESIAN_POINT('Ctrl Pts',(-3.29140295200005,11.6,-10.316248395));
#290486=CARTESIAN_POINT('Ctrl Pts',(-3.28984544000006,15.2,-10.314024727));
#290487=CARTESIAN_POINT('Ctrl Pts',(-3.28984544000006,11.6,-10.314024727));
#290488=CARTESIAN_POINT('Ctrl Pts',(-3.28829313800005,15.2,-10.311804517));
#290489=CARTESIAN_POINT('Ctrl Pts',(-3.28829313800005,11.6,-10.311804517));
#290490=CARTESIAN_POINT('Ctrl Pts',(-3.28674604500006,15.2,-10.309587781));
#290491=CARTESIAN_POINT('Ctrl Pts',(-3.28674604500006,11.6,-10.309587781));
#290492=CARTESIAN_POINT('Ctrl Pts',(-3.28520415900006,15.2,-10.307374529));
#290493=CARTESIAN_POINT('Ctrl Pts',(-3.28520415900006,11.6,-10.307374529));
#290494=CARTESIAN_POINT('Ctrl Pts',(-3.28366748200006,15.2,-10.305164778));
#290495=CARTESIAN_POINT('Ctrl Pts',(-3.28366748200006,11.6,-10.305164778));
#290496=CARTESIAN_POINT('Ctrl Pts',(-3.28213601000006,15.2,-10.302958542));
#290497=CARTESIAN_POINT('Ctrl Pts',(-3.28213601000006,11.6,-10.302958542));
#290498=CARTESIAN_POINT('Ctrl Pts',(-3.28060974500006,15.2,-10.300755833));
#290499=CARTESIAN_POINT('Ctrl Pts',(-3.28060974500006,11.6,-10.300755833));
#290500=CARTESIAN_POINT('Ctrl Pts',(-3.27908868500006,15.2,-10.298556667));
#290501=CARTESIAN_POINT('Ctrl Pts',(-3.27908868500006,11.6,-10.298556667));
#290502=CARTESIAN_POINT('Ctrl Pts',(-3.27757282800006,15.2,-10.296361056));
#290503=CARTESIAN_POINT('Ctrl Pts',(-3.27757282800006,11.6,-10.296361056));
#290504=CARTESIAN_POINT('Ctrl Pts',(-3.27606217500006,15.2,-10.294169016));
#290505=CARTESIAN_POINT('Ctrl Pts',(-3.27606217500006,11.6,-10.294169016));
#290506=CARTESIAN_POINT('Ctrl Pts',(-3.27455672400006,15.2,-10.291980559));
#290507=CARTESIAN_POINT('Ctrl Pts',(-3.27455672400006,11.6,-10.291980559));
#290508=CARTESIAN_POINT('Ctrl Pts',(-3.27305647500005,15.2,-10.289795701));
#290509=CARTESIAN_POINT('Ctrl Pts',(-3.27305647500005,11.6,-10.289795701));
#290510=CARTESIAN_POINT('Ctrl Pts',(-3.27156142600006,15.2,-10.287614455));
#290511=CARTESIAN_POINT('Ctrl Pts',(-3.27156142600006,11.6,-10.287614455));
#290512=CARTESIAN_POINT('Ctrl Pts',(-3.27007157800006,15.2,-10.285436836));
#290513=CARTESIAN_POINT('Ctrl Pts',(-3.27007157800006,11.6,-10.285436836));
#290514=CARTESIAN_POINT('Ctrl Pts',(-3.26858692800006,15.2,-10.283262857));
#290515=CARTESIAN_POINT('Ctrl Pts',(-3.26858692800006,11.6,-10.283262857));
#290516=CARTESIAN_POINT('Ctrl Pts',(-3.26710747700006,15.2,-10.281092534));
#290517=CARTESIAN_POINT('Ctrl Pts',(-3.26710747700006,11.6,-10.281092534));
#290518=CARTESIAN_POINT('Ctrl Pts',(-3.26563322100006,15.2,-10.27892588));
#290519=CARTESIAN_POINT('Ctrl Pts',(-3.26563322100006,11.6,-10.27892588));
#290520=CARTESIAN_POINT('Ctrl Pts',(-3.26416416300006,15.2,-10.27676291));
#290521=CARTESIAN_POINT('Ctrl Pts',(-3.26416416300006,11.6,-10.27676291));
#290522=CARTESIAN_POINT('Ctrl Pts',(-3.26270029800006,15.2,-10.274603638));
#290523=CARTESIAN_POINT('Ctrl Pts',(-3.26270029800006,11.6,-10.274603638));
#290524=CARTESIAN_POINT('Ctrl Pts',(-3.26124162800005,15.2,-10.272448079));
#290525=CARTESIAN_POINT('Ctrl Pts',(-3.26124162800005,11.6,-10.272448079));
#290526=CARTESIAN_POINT('Ctrl Pts',(-3.25978815100005,15.2,-10.270296247));
#290527=CARTESIAN_POINT('Ctrl Pts',(-3.25978815100005,11.6,-10.270296247));
#290528=CARTESIAN_POINT('Ctrl Pts',(-3.25833986600006,15.2,-10.268148155));
#290529=CARTESIAN_POINT('Ctrl Pts',(-3.25833986600006,11.6,-10.268148155));
#290530=CARTESIAN_POINT('Ctrl Pts',(-3.25689677300006,15.2,-10.266003821));
#290531=CARTESIAN_POINT('Ctrl Pts',(-3.25689677300006,11.6,-10.266003821));
#290532=CARTESIAN_POINT('Ctrl Pts',(-3.25545886800006,15.2,-10.263863257));
#290533=CARTESIAN_POINT('Ctrl Pts',(-3.25545886800006,11.6,-10.263863257));
#290534=CARTESIAN_POINT('Ctrl Pts',(-3.25402615400006,15.2,-10.261726477));
#290535=CARTESIAN_POINT('Ctrl Pts',(-3.25402615400006,11.6,-10.261726477));
#290536=CARTESIAN_POINT('Ctrl Pts',(-3.25259862700006,15.2,-10.259593499));
#290537=CARTESIAN_POINT('Ctrl Pts',(-3.25259862700006,11.6,-10.259593499));
#290538=CARTESIAN_POINT('Ctrl Pts',(-3.25117628700006,15.2,-10.257464333));
#290539=CARTESIAN_POINT('Ctrl Pts',(-3.25117628700006,11.6,-10.257464333));
#290540=CARTESIAN_POINT('Ctrl Pts',(-3.24975913200006,15.2,-10.255338999));
#290541=CARTESIAN_POINT('Ctrl Pts',(-3.24975913200006,11.6,-10.255338999));
#290542=CARTESIAN_POINT('Ctrl Pts',(-3.24834716300006,15.2,-10.253217507));
#290543=CARTESIAN_POINT('Ctrl Pts',(-3.24834716300006,11.6,-10.253217507));
#290544=CARTESIAN_POINT('Ctrl Pts',(-3.24694037600006,15.2,-10.251099874));
#290545=CARTESIAN_POINT('Ctrl Pts',(-3.24694037600006,11.6,-10.251099874));
#290546=CARTESIAN_POINT('Ctrl Pts',(-3.24553877200006,15.2,-10.248986116));
#290547=CARTESIAN_POINT('Ctrl Pts',(-3.24553877200006,11.6,-10.248986116));
#290548=CARTESIAN_POINT('Ctrl Pts',(-3.24414235000006,15.2,-10.246876246));
#290549=CARTESIAN_POINT('Ctrl Pts',(-3.24414235000006,11.6,-10.246876246));
#290550=CARTESIAN_POINT('Ctrl Pts',(-3.24275110800006,15.2,-10.244770278));
#290551=CARTESIAN_POINT('Ctrl Pts',(-3.24275110800006,11.6,-10.244770278));
#290552=CARTESIAN_POINT('Ctrl Pts',(-3.24136504400005,15.2,-10.24266823));
#290553=CARTESIAN_POINT('Ctrl Pts',(-3.24136504400005,11.6,-10.24266823));
#290554=CARTESIAN_POINT('Ctrl Pts',(-3.23998415800005,15.2,-10.240570114));
#290555=CARTESIAN_POINT('Ctrl Pts',(-3.23998415800005,11.6,-10.240570114));
#290556=CARTESIAN_POINT('Ctrl Pts',(-3.23860844900006,15.2,-10.238475947));
#290557=CARTESIAN_POINT('Ctrl Pts',(-3.23860844900006,11.6,-10.238475947));
#290558=CARTESIAN_POINT('Ctrl Pts',(-3.23723791500006,15.2,-10.236385744));
#290559=CARTESIAN_POINT('Ctrl Pts',(-3.23723791500006,11.6,-10.236385744));
#290560=CARTESIAN_POINT('Ctrl Pts',(-3.23587255600006,15.2,-10.23429952));
#290561=CARTESIAN_POINT('Ctrl Pts',(-3.23587255600006,11.6,-10.23429952));
#290562=CARTESIAN_POINT('Ctrl Pts',(-3.23451236800006,15.2,-10.232217289));
#290563=CARTESIAN_POINT('Ctrl Pts',(-3.23451236800006,11.6,-10.232217289));
#290564=CARTESIAN_POINT('Ctrl Pts',(-3.23315735400006,15.2,-10.230139067));
#290565=CARTESIAN_POINT('Ctrl Pts',(-3.23315735400006,11.6,-10.230139067));
#290566=CARTESIAN_POINT('Ctrl Pts',(-3.23180750800006,15.2,-10.228064869));
#290567=CARTESIAN_POINT('Ctrl Pts',(-3.23180750800006,11.6,-10.228064869));
#290568=CARTESIAN_POINT('Ctrl Pts',(-3.23046283300005,15.2,-10.225994712));
#290569=CARTESIAN_POINT('Ctrl Pts',(-3.23046283300005,11.6,-10.225994712));
#290570=CARTESIAN_POINT('Ctrl Pts',(-3.22912332500006,15.2,-10.223928608));
#290571=CARTESIAN_POINT('Ctrl Pts',(-3.22912332500006,11.6,-10.223928608));
#290572=CARTESIAN_POINT('Ctrl Pts',(-3.22778898300006,15.2,-10.221866575));
#290573=CARTESIAN_POINT('Ctrl Pts',(-3.22778898300006,11.6,-10.221866575));
#290574=CARTESIAN_POINT('Ctrl Pts',(-3.22645980800006,15.2,-10.219808628));
#290575=CARTESIAN_POINT('Ctrl Pts',(-3.22645980800006,11.6,-10.219808628));
#290576=CARTESIAN_POINT('Ctrl Pts',(-3.22513579500006,15.2,-10.217754781));
#290577=CARTESIAN_POINT('Ctrl Pts',(-3.22513579500006,11.6,-10.217754781));
#290578=CARTESIAN_POINT('Ctrl Pts',(-3.22381694500006,15.2,-10.215705052));
#290579=CARTESIAN_POINT('Ctrl Pts',(-3.22381694500006,11.6,-10.215705052));
#290580=CARTESIAN_POINT('Ctrl Pts',(-3.22250325700006,15.2,-10.213659454));
#290581=CARTESIAN_POINT('Ctrl Pts',(-3.22250325700006,11.6,-10.213659454));
#290582=CARTESIAN_POINT('Ctrl Pts',(-3.22119472800006,15.2,-10.211618003));
#290583=CARTESIAN_POINT('Ctrl Pts',(-3.22119472800006,11.6,-10.211618003));
#290584=CARTESIAN_POINT('Ctrl Pts',(-3.21989135700006,15.2,-10.209580717));
#290585=CARTESIAN_POINT('Ctrl Pts',(-3.21989135700006,11.6,-10.209580717));
#290586=CARTESIAN_POINT('Ctrl Pts',(-3.21859314300006,15.2,-10.207547609));
#290587=CARTESIAN_POINT('Ctrl Pts',(-3.21859314300006,11.6,-10.207547609));
#290588=CARTESIAN_POINT('Ctrl Pts',(-3.21730008400006,15.2,-10.205518696));
#290589=CARTESIAN_POINT('Ctrl Pts',(-3.21730008400006,11.6,-10.205518696));
#290590=CARTESIAN_POINT('Ctrl Pts',(-3.21601218000006,15.2,-10.203493994));
#290591=CARTESIAN_POINT('Ctrl Pts',(-3.21601218000006,11.6,-10.203493994));
#290592=CARTESIAN_POINT('Ctrl Pts',(-3.21472942800006,15.2,-10.201473517));
#290593=CARTESIAN_POINT('Ctrl Pts',(-3.21472942800006,11.6,-10.201473517));
#290594=CARTESIAN_POINT('Ctrl Pts',(-3.21345182800005,15.2,-10.199457283));
#290595=CARTESIAN_POINT('Ctrl Pts',(-3.21345182800005,11.6,-10.199457283));
#290596=CARTESIAN_POINT('Ctrl Pts',(-3.21217937800006,15.2,-10.197445307));
#290597=CARTESIAN_POINT('Ctrl Pts',(-3.21217937800006,11.6,-10.197445307));
#290598=CARTESIAN_POINT('Ctrl Pts',(-3.21091207400006,15.2,-10.195437604));
#290599=CARTESIAN_POINT('Ctrl Pts',(-3.21091207400006,11.6,-10.195437604));
#290600=CARTESIAN_POINT('Ctrl Pts',(-3.20964991900006,15.2,-10.193434192));
#290601=CARTESIAN_POINT('Ctrl Pts',(-3.20964991900006,11.6,-10.193434192));
#290602=CARTESIAN_POINT('Ctrl Pts',(-3.20839290700006,15.2,-10.191435085));
#290603=CARTESIAN_POINT('Ctrl Pts',(-3.20839290700006,11.6,-10.191435085));
#290604=CARTESIAN_POINT('Ctrl Pts',(-3.20714104000006,15.2,-10.189440301));
#290605=CARTESIAN_POINT('Ctrl Pts',(-3.20714104000006,11.6,-10.189440301));
#290606=CARTESIAN_POINT('Ctrl Pts',(-3.20589431500005,15.2,-10.187449854));
#290607=CARTESIAN_POINT('Ctrl Pts',(-3.20589431500005,11.6,-10.187449854));
#290608=CARTESIAN_POINT('Ctrl Pts',(-3.20465273000006,15.2,-10.185463762));
#290609=CARTESIAN_POINT('Ctrl Pts',(-3.20465273000006,11.6,-10.185463762));
#290610=CARTESIAN_POINT('Ctrl Pts',(-3.20341628400006,15.2,-10.18348204));
#290611=CARTESIAN_POINT('Ctrl Pts',(-3.20341628400006,11.6,-10.18348204));
#290612=CARTESIAN_POINT('Ctrl Pts',(-3.20218497500006,15.2,-10.181504705));
#290613=CARTESIAN_POINT('Ctrl Pts',(-3.20218497500006,11.6,-10.181504705));
#290614=CARTESIAN_POINT('Ctrl Pts',(-3.20095880100005,15.2,-10.179531773));
#290615=CARTESIAN_POINT('Ctrl Pts',(-3.20095880100005,11.6,-10.179531773));
#290616=CARTESIAN_POINT('Ctrl Pts',(-3.19973776200006,15.2,-10.17756326));
#290617=CARTESIAN_POINT('Ctrl Pts',(-3.19973776200006,11.6,-10.17756326));
#290618=CARTESIAN_POINT('Ctrl Pts',(-3.19852185400006,15.2,-10.175599183));
#290619=CARTESIAN_POINT('Ctrl Pts',(-3.19852185400006,11.6,-10.175599183));
#290620=CARTESIAN_POINT('Ctrl Pts',(-3.19731107800005,15.2,-10.173639558));
#290621=CARTESIAN_POINT('Ctrl Pts',(-3.19731107800005,11.6,-10.173639558));
#290622=CARTESIAN_POINT('Ctrl Pts',(-3.19610543000006,15.2,-10.171684403));
#290623=CARTESIAN_POINT('Ctrl Pts',(-3.19610543000006,11.6,-10.171684403));
#290624=CARTESIAN_POINT('Ctrl Pts',(-3.19490490900006,15.2,-10.169733732));
#290625=CARTESIAN_POINT('Ctrl Pts',(-3.19490490900006,11.6,-10.169733732));
#290626=CARTESIAN_POINT('Ctrl Pts',(-3.19370951400006,15.2,-10.167787564));
#290627=CARTESIAN_POINT('Ctrl Pts',(-3.19370951400006,11.6,-10.167787564));
#290628=CARTESIAN_POINT('Ctrl Pts',(-3.19251924200006,15.2,-10.165845913));
#290629=CARTESIAN_POINT('Ctrl Pts',(-3.19251924200006,11.6,-10.165845913));
#290630=CARTESIAN_POINT('Ctrl Pts',(-3.19133409400005,15.2,-10.163908798));
#290631=CARTESIAN_POINT('Ctrl Pts',(-3.19133409400005,11.6,-10.163908798));
#290632=CARTESIAN_POINT('Ctrl Pts',(-3.19015406500006,15.2,-10.161976234));
#290633=CARTESIAN_POINT('Ctrl Pts',(-3.19015406500006,11.6,-10.161976234));
#290634=CARTESIAN_POINT('Ctrl Pts',(-3.18897915400006,15.2,-10.16004824));
#290635=CARTESIAN_POINT('Ctrl Pts',(-3.18897915400006,11.6,-10.16004824));
#290636=CARTESIAN_POINT('Ctrl Pts',(-3.18780936000006,15.2,-10.15812483));
#290637=CARTESIAN_POINT('Ctrl Pts',(-3.18780936000006,11.6,-10.15812483));
#290638=CARTESIAN_POINT('Ctrl Pts',(-3.18664468100006,15.2,-10.156206023));
#290639=CARTESIAN_POINT('Ctrl Pts',(-3.18664468100006,11.6,-10.156206023));
#290640=CARTESIAN_POINT('Ctrl Pts',(-3.18548511400006,15.2,-10.154291835));
#290641=CARTESIAN_POINT('Ctrl Pts',(-3.18548511400006,11.6,-10.154291835));
#290642=CARTESIAN_POINT('Ctrl Pts',(-3.18433065900006,15.2,-10.152382284));
#290643=CARTESIAN_POINT('Ctrl Pts',(-3.18433065900006,11.6,-10.152382284));
#290644=CARTESIAN_POINT('Ctrl Pts',(-3.18318131200006,15.2,-10.150477386));
#290645=CARTESIAN_POINT('Ctrl Pts',(-3.18318131200006,11.6,-10.150477386));
#290646=CARTESIAN_POINT('Ctrl Pts',(-3.18203707300006,15.2,-10.148577159));
#290647=CARTESIAN_POINT('Ctrl Pts',(-3.18203707300006,11.6,-10.148577159));
#290648=CARTESIAN_POINT('Ctrl Pts',(-3.18089794000006,15.2,-10.146681619));
#290649=CARTESIAN_POINT('Ctrl Pts',(-3.18089794000006,11.6,-10.146681619));
#290650=CARTESIAN_POINT('Ctrl Pts',(-3.17976391000005,15.2,-10.144790784));
#290651=CARTESIAN_POINT('Ctrl Pts',(-3.17976391000005,11.6,-10.144790784));
#290652=CARTESIAN_POINT('Ctrl Pts',(-3.17863498200006,15.2,-10.14290467));
#290653=CARTESIAN_POINT('Ctrl Pts',(-3.17863498200006,11.6,-10.14290467));
#290654=CARTESIAN_POINT('Ctrl Pts',(-3.17751115300006,15.2,-10.141023296));
#290655=CARTESIAN_POINT('Ctrl Pts',(-3.17751115300006,11.6,-10.141023296));
#290656=CARTESIAN_POINT('Ctrl Pts',(-3.17639242200006,15.2,-10.139146679));
#290657=CARTESIAN_POINT('Ctrl Pts',(-3.17639242200006,11.6,-10.139146679));
#290658=CARTESIAN_POINT('Ctrl Pts',(-3.17527878700006,15.2,-10.137274836));
#290659=CARTESIAN_POINT('Ctrl Pts',(-3.17527878700006,11.6,-10.137274836));
#290660=CARTESIAN_POINT('Ctrl Pts',(-3.17417024500006,15.2,-10.135407784));
#290661=CARTESIAN_POINT('Ctrl Pts',(-3.17417024500006,11.6,-10.135407784));
#290662=CARTESIAN_POINT('Ctrl Pts',(-3.17306679400006,15.2,-10.133545541));
#290663=CARTESIAN_POINT('Ctrl Pts',(-3.17306679400006,11.6,-10.133545541));
#290664=CARTESIAN_POINT('Ctrl Pts',(-3.17196843400006,15.2,-10.131688125));
#290665=CARTESIAN_POINT('Ctrl Pts',(-3.17196843400006,11.6,-10.131688125));
#290666=CARTESIAN_POINT('Ctrl Pts',(-3.17087516000006,15.2,-10.129835552));
#290667=CARTESIAN_POINT('Ctrl Pts',(-3.17087516000006,11.6,-10.129835552));
#290668=CARTESIAN_POINT('Ctrl Pts',(-3.16978697200006,15.2,-10.127987842));
#290669=CARTESIAN_POINT('Ctrl Pts',(-3.16978697200006,11.6,-10.127987842));
#290670=CARTESIAN_POINT('Ctrl Pts',(-3.16870386700006,15.2,-10.126145011));
#290671=CARTESIAN_POINT('Ctrl Pts',(-3.16870386700006,11.6,-10.126145011));
#290672=CARTESIAN_POINT('Ctrl Pts',(-3.16762584300006,15.2,-10.124307078));
#290673=CARTESIAN_POINT('Ctrl Pts',(-3.16762584300006,11.6,-10.124307078));
#290674=CARTESIAN_POINT('Ctrl Pts',(-3.16655289900006,15.2,-10.12247406));
#290675=CARTESIAN_POINT('Ctrl Pts',(-3.16655289900006,11.6,-10.12247406));
#290676=CARTESIAN_POINT('Ctrl Pts',(-3.16548503100006,15.2,-10.120645974));
#290677=CARTESIAN_POINT('Ctrl Pts',(-3.16548503100006,11.6,-10.120645974));
#290678=CARTESIAN_POINT('Ctrl Pts',(-3.16442223700005,15.2,-10.11882284));
#290679=CARTESIAN_POINT('Ctrl Pts',(-3.16442223700005,11.6,-10.11882284));
#290680=CARTESIAN_POINT('Ctrl Pts',(-3.16336451700006,15.2,-10.117004674));
#290681=CARTESIAN_POINT('Ctrl Pts',(-3.16336451700006,11.6,-10.117004674));
#290682=CARTESIAN_POINT('Ctrl Pts',(-3.16231186600006,15.2,-10.115191495));
#290683=CARTESIAN_POINT('Ctrl Pts',(-3.16231186600006,11.6,-10.115191495));
#290684=CARTESIAN_POINT('Ctrl Pts',(-3.16126428300006,15.2,-10.113383323));
#290685=CARTESIAN_POINT('Ctrl Pts',(-3.16126428300006,11.6,-10.113383323));
#290686=CARTESIAN_POINT('Ctrl Pts',(-3.16022176700006,15.2,-10.111580173));
#290687=CARTESIAN_POINT('Ctrl Pts',(-3.16022176700006,11.6,-10.111580173));
#290688=CARTESIAN_POINT('Ctrl Pts',(-3.15918431400006,15.2,-10.109782065));
#290689=CARTESIAN_POINT('Ctrl Pts',(-3.15918431400006,11.6,-10.109782065));
#290690=CARTESIAN_POINT('Ctrl Pts',(-3.15815192200006,15.2,-10.107989016));
#290691=CARTESIAN_POINT('Ctrl Pts',(-3.15815192200006,11.6,-10.107989016));
#290692=CARTESIAN_POINT('Ctrl Pts',(-3.15712458900005,15.2,-10.106201046));
#290693=CARTESIAN_POINT('Ctrl Pts',(-3.15712458900005,11.6,-10.106201046));
#290694=CARTESIAN_POINT('Ctrl Pts',(-3.15610231200006,15.2,-10.104418172));
#290695=CARTESIAN_POINT('Ctrl Pts',(-3.15610231200006,11.6,-10.104418172));
#290696=CARTESIAN_POINT('Ctrl Pts',(-3.15508508900006,15.2,-10.102640413));
#290697=CARTESIAN_POINT('Ctrl Pts',(-3.15508508900006,11.6,-10.102640413));
#290698=CARTESIAN_POINT('Ctrl Pts',(-3.15407291900006,15.2,-10.100867788));
#290699=CARTESIAN_POINT('Ctrl Pts',(-3.15407291900006,11.6,-10.100867788));
#290700=CARTESIAN_POINT('Ctrl Pts',(-3.15306579800006,15.2,-10.099100315));
#290701=CARTESIAN_POINT('Ctrl Pts',(-3.15306579800006,11.6,-10.099100315));
#290702=CARTESIAN_POINT('Ctrl Pts',(-3.15206372300006,15.2,-10.097338012));
#290703=CARTESIAN_POINT('Ctrl Pts',(-3.15206372300006,11.6,-10.097338012));
#290704=CARTESIAN_POINT('Ctrl Pts',(-3.15106669400006,15.2,-10.0955809));
#290705=CARTESIAN_POINT('Ctrl Pts',(-3.15106669400006,11.6,-10.0955809));
#290706=CARTESIAN_POINT('Ctrl Pts',(-3.15007470600006,15.2,-10.093828995));
#290707=CARTESIAN_POINT('Ctrl Pts',(-3.15007470600006,11.6,-10.093828995));
#290708=CARTESIAN_POINT('Ctrl Pts',(-3.14908775900005,15.2,-10.092082318));
#290709=CARTESIAN_POINT('Ctrl Pts',(-3.14908775900005,11.6,-10.092082318));
#290710=CARTESIAN_POINT('Ctrl Pts',(-3.14810584800005,15.2,-10.090340886));
#290711=CARTESIAN_POINT('Ctrl Pts',(-3.14810584800005,11.6,-10.090340886));
#290712=CARTESIAN_POINT('Ctrl Pts',(-3.14712897200006,15.2,-10.088604719));
#290713=CARTESIAN_POINT('Ctrl Pts',(-3.14712897200006,11.6,-10.088604719));
#290714=CARTESIAN_POINT('Ctrl Pts',(-3.14615712900005,15.2,-10.086873836));
#290715=CARTESIAN_POINT('Ctrl Pts',(-3.14615712900005,11.6,-10.086873836));
#290716=CARTESIAN_POINT('Ctrl Pts',(-3.14519031500006,15.2,-10.085148257));
#290717=CARTESIAN_POINT('Ctrl Pts',(-3.14519031500006,11.6,-10.085148257));
#290718=CARTESIAN_POINT('Ctrl Pts',(-3.14422852800006,15.2,-10.083427999));
#290719=CARTESIAN_POINT('Ctrl Pts',(-3.14422852800006,11.6,-10.083427999));
#290720=CARTESIAN_POINT('Ctrl Pts',(-3.14327176600006,15.2,-10.081713082));
#290721=CARTESIAN_POINT('Ctrl Pts',(-3.14327176600006,11.6,-10.081713082));
#290722=CARTESIAN_POINT('Ctrl Pts',(-3.14232002500006,15.2,-10.080003527));
#290723=CARTESIAN_POINT('Ctrl Pts',(-3.14232002500006,11.6,-10.080003527));
#290724=CARTESIAN_POINT('Ctrl Pts',(-3.14137330400006,15.2,-10.078299351));
#290725=CARTESIAN_POINT('Ctrl Pts',(-3.14137330400006,11.6,-10.078299351));
#290726=CARTESIAN_POINT('Ctrl Pts',(-3.14043159900006,15.2,-10.076600574));
#290727=CARTESIAN_POINT('Ctrl Pts',(-3.14043159900006,11.6,-10.076600574));
#290728=CARTESIAN_POINT('Ctrl Pts',(-3.13949490800006,15.2,-10.074907216));
#290729=CARTESIAN_POINT('Ctrl Pts',(-3.13949490800006,11.6,-10.074907216));
#290730=CARTESIAN_POINT('Ctrl Pts',(-3.13856322800006,15.2,-10.073219295));
#290731=CARTESIAN_POINT('Ctrl Pts',(-3.13856322800006,11.6,-10.073219295));
#290732=CARTESIAN_POINT('Ctrl Pts',(-3.13763655600006,15.2,-10.071536834));
#290733=CARTESIAN_POINT('Ctrl Pts',(-3.13763655600006,11.6,-10.071536834));
#290734=CARTESIAN_POINT('Ctrl Pts',(-3.13671489000006,15.2,-10.06985985));
#290735=CARTESIAN_POINT('Ctrl Pts',(-3.13671489000006,11.6,-10.06985985));
#290736=CARTESIAN_POINT('Ctrl Pts',(-3.13579822800006,15.2,-10.068188363));
#290737=CARTESIAN_POINT('Ctrl Pts',(-3.13579822800006,11.6,-10.068188363));
#290738=CARTESIAN_POINT('Ctrl Pts',(-3.13488656600006,15.2,-10.066522391));
#290739=CARTESIAN_POINT('Ctrl Pts',(-3.13488656600006,11.6,-10.066522391));
#290740=CARTESIAN_POINT('Ctrl Pts',(-3.13397990100006,15.2,-10.064861958));
#290741=CARTESIAN_POINT('Ctrl Pts',(-3.13397990100006,11.6,-10.064861958));
#290742=CARTESIAN_POINT('Ctrl Pts',(-3.13307823000006,15.2,-10.063207081));
#290743=CARTESIAN_POINT('Ctrl Pts',(-3.13307823000006,11.6,-10.063207081));
#290744=CARTESIAN_POINT('Ctrl Pts',(-3.13218155100006,15.2,-10.061557781));
#290745=CARTESIAN_POINT('Ctrl Pts',(-3.13218155100006,11.6,-10.061557781));
#290746=CARTESIAN_POINT('Ctrl Pts',(-3.13128986000006,15.2,-10.059914078));
#290747=CARTESIAN_POINT('Ctrl Pts',(-3.13128986000006,11.6,-10.059914078));
#290748=CARTESIAN_POINT('Ctrl Pts',(-3.13040315600006,15.2,-10.058275991));
#290749=CARTESIAN_POINT('Ctrl Pts',(-3.13040315600006,11.6,-10.058275991));
#290750=CARTESIAN_POINT('Ctrl Pts',(-3.12952143500006,15.2,-10.056643542));
#290751=CARTESIAN_POINT('Ctrl Pts',(-3.12952143500006,11.6,-10.056643542));
#290752=CARTESIAN_POINT('Ctrl Pts',(-3.12864469400005,15.2,-10.055016749));
#290753=CARTESIAN_POINT('Ctrl Pts',(-3.12864469400005,11.6,-10.055016749));
#290754=CARTESIAN_POINT('Ctrl Pts',(-3.12777293000006,15.2,-10.053395635));
#290755=CARTESIAN_POINT('Ctrl Pts',(-3.12777293000006,11.6,-10.053395635));
#290756=CARTESIAN_POINT('Ctrl Pts',(-3.12690614000006,15.2,-10.051780219));
#290757=CARTESIAN_POINT('Ctrl Pts',(-3.12690614000006,11.6,-10.051780219));
#290758=CARTESIAN_POINT('Ctrl Pts',(-3.12604432200006,15.2,-10.050170521));
#290759=CARTESIAN_POINT('Ctrl Pts',(-3.12604432200006,11.6,-10.050170521));
#290760=CARTESIAN_POINT('Ctrl Pts',(-3.12518747100006,15.2,-10.048566563));
#290761=CARTESIAN_POINT('Ctrl Pts',(-3.12518747100006,11.6,-10.048566563));
#290762=CARTESIAN_POINT('Ctrl Pts',(-3.12433558500006,15.2,-10.046968363));
#290763=CARTESIAN_POINT('Ctrl Pts',(-3.12433558500006,11.6,-10.046968363));
#290764=CARTESIAN_POINT('Ctrl Pts',(-3.12348866200006,15.2,-10.045375945));
#290765=CARTESIAN_POINT('Ctrl Pts',(-3.12348866200006,11.6,-10.045375945));
#290766=CARTESIAN_POINT('Ctrl Pts',(-3.12264669700005,15.2,-10.043789328));
#290767=CARTESIAN_POINT('Ctrl Pts',(-3.12264669700005,11.6,-10.043789328));
#290768=CARTESIAN_POINT('Ctrl Pts',(-3.12180968800006,15.2,-10.042208533));
#290769=CARTESIAN_POINT('Ctrl Pts',(-3.12180968800006,11.6,-10.042208533));
#290770=CARTESIAN_POINT('Ctrl Pts',(-3.12097763100006,15.2,-10.04063358));
#290771=CARTESIAN_POINT('Ctrl Pts',(-3.12097763100006,11.6,-10.04063358));
#290772=CARTESIAN_POINT('Ctrl Pts',(-3.12015052400006,15.2,-10.039064492));
#290773=CARTESIAN_POINT('Ctrl Pts',(-3.12015052400006,11.6,-10.039064492));
#290774=CARTESIAN_POINT('Ctrl Pts',(-3.11932836300006,15.2,-10.037501288));
#290775=CARTESIAN_POINT('Ctrl Pts',(-3.11932836300006,11.6,-10.037501288));
#290776=CARTESIAN_POINT('Ctrl Pts',(-3.11851114600006,15.2,-10.035943992));
#290777=CARTESIAN_POINT('Ctrl Pts',(-3.11851114600006,11.6,-10.035943992));
#290778=CARTESIAN_POINT('Ctrl Pts',(-3.11769886800006,15.2,-10.034392621));
#290779=CARTESIAN_POINT('Ctrl Pts',(-3.11769886800006,11.6,-10.034392621));
#290780=CARTESIAN_POINT('Ctrl Pts',(-3.11689152600006,15.2,-10.0328472));
#290781=CARTESIAN_POINT('Ctrl Pts',(-3.11689152600006,11.6,-10.0328472));
#290782=CARTESIAN_POINT('Ctrl Pts',(-3.11608911700006,15.2,-10.031307748));
#290783=CARTESIAN_POINT('Ctrl Pts',(-3.11608911700006,11.6,-10.031307748));
#290784=CARTESIAN_POINT('Ctrl Pts',(-3.11529163900006,15.2,-10.029774289));
#290785=CARTESIAN_POINT('Ctrl Pts',(-3.11529163900006,11.6,-10.029774289));
#290786=CARTESIAN_POINT('Ctrl Pts',(-3.11449908600005,15.2,-10.028246842));
#290787=CARTESIAN_POINT('Ctrl Pts',(-3.11449908600005,11.6,-10.028246842));
#290788=CARTESIAN_POINT('Ctrl Pts',(-3.11371145700006,15.2,-10.026725429));
#290789=CARTESIAN_POINT('Ctrl Pts',(-3.11371145700006,11.6,-10.026725429));
#290790=CARTESIAN_POINT('Ctrl Pts',(-3.11292874800006,15.2,-10.025210073));
#290791=CARTESIAN_POINT('Ctrl Pts',(-3.11292874800006,11.6,-10.025210073));
#290792=CARTESIAN_POINT('Ctrl Pts',(-3.11215095500006,15.2,-10.023700794));
#290793=CARTESIAN_POINT('Ctrl Pts',(-3.11215095500006,11.6,-10.023700794));
#290794=CARTESIAN_POINT('Ctrl Pts',(-3.11137807500006,15.2,-10.022197616));
#290795=CARTESIAN_POINT('Ctrl Pts',(-3.11137807500006,11.6,-10.022197616));
#290796=CARTESIAN_POINT('Ctrl Pts',(-3.11061010400006,15.2,-10.020700559));
#290797=CARTESIAN_POINT('Ctrl Pts',(-3.11061010400006,11.6,-10.020700559));
#290798=CARTESIAN_POINT('Ctrl Pts',(-3.10984704000006,15.2,-10.019209646));
#290799=CARTESIAN_POINT('Ctrl Pts',(-3.10984704000006,11.6,-10.019209646));
#290800=CARTESIAN_POINT('Ctrl Pts',(-3.10908887700006,15.2,-10.017724898));
#290801=CARTESIAN_POINT('Ctrl Pts',(-3.10908887700006,11.6,-10.017724898));
#290802=CARTESIAN_POINT('Ctrl Pts',(-3.10833561300006,15.2,-10.016246339));
#290803=CARTESIAN_POINT('Ctrl Pts',(-3.10833561300006,11.6,-10.016246339));
#290804=CARTESIAN_POINT('Ctrl Pts',(-3.10758724500006,15.2,-10.01477399));
#290805=CARTESIAN_POINT('Ctrl Pts',(-3.10758724500006,11.6,-10.01477399));
#290806=CARTESIAN_POINT('Ctrl Pts',(-3.10684376800006,15.2,-10.013307874));
#290807=CARTESIAN_POINT('Ctrl Pts',(-3.10684376800006,11.6,-10.013307874));
#290808=CARTESIAN_POINT('Ctrl Pts',(-3.10610518000006,15.2,-10.011848012));
#290809=CARTESIAN_POINT('Ctrl Pts',(-3.10610518000006,11.6,-10.011848012));
#290810=CARTESIAN_POINT('Ctrl Pts',(-3.10537147600006,15.2,-10.010394429));
#290811=CARTESIAN_POINT('Ctrl Pts',(-3.10537147600006,11.6,-10.010394429));
#290812=CARTESIAN_POINT('Ctrl Pts',(-3.10464265200005,15.2,-10.008947144));
#290813=CARTESIAN_POINT('Ctrl Pts',(-3.10464265200005,11.6,-10.008947144));
#290814=CARTESIAN_POINT('Ctrl Pts',(-3.10391870600006,15.2,-10.007506182));
#290815=CARTESIAN_POINT('Ctrl Pts',(-3.10391870600006,11.6,-10.007506182));
#290816=CARTESIAN_POINT('Ctrl Pts',(-3.10319963300006,15.2,-10.006071567));
#290817=CARTESIAN_POINT('Ctrl Pts',(-3.10319963300006,11.6,-10.006071567));
#290818=CARTESIAN_POINT('Ctrl Pts',(-3.10248542800006,15.2,-10.004643319));
#290819=CARTESIAN_POINT('Ctrl Pts',(-3.10248542800006,11.6,-10.004643319));
#290820=CARTESIAN_POINT('Ctrl Pts',(-3.10177609000006,15.2,-10.003221464));
#290821=CARTESIAN_POINT('Ctrl Pts',(-3.10177609000006,11.6,-10.003221464));
#290822=CARTESIAN_POINT('Ctrl Pts',(-3.10107161400006,15.2,-10.001806021));
#290823=CARTESIAN_POINT('Ctrl Pts',(-3.10107161400006,11.6,-10.001806021));
#290824=CARTESIAN_POINT('Ctrl Pts',(-3.10037199600006,15.2,-10.000397016));
#290825=CARTESIAN_POINT('Ctrl Pts',(-3.10037199600006,11.6,-10.000397016));
#290826=CARTESIAN_POINT('Ctrl Pts',(-3.09967723200006,15.2,-9.99899447200001));
#290827=CARTESIAN_POINT('Ctrl Pts',(-3.09967723200006,11.6,-9.99899447200001));
#290828=CARTESIAN_POINT('Ctrl Pts',(-3.09898731800006,15.2,-9.99759841200001));
#290829=CARTESIAN_POINT('Ctrl Pts',(-3.09898731800006,11.6,-9.99759841200001));
#290830=CARTESIAN_POINT('Ctrl Pts',(-3.09830225000006,15.2,-9.99620885900001));
#290831=CARTESIAN_POINT('Ctrl Pts',(-3.09830225000006,11.6,-9.99620885900001));
#290832=CARTESIAN_POINT('Ctrl Pts',(-3.09762202400006,15.2,-9.99482583600001));
#290833=CARTESIAN_POINT('Ctrl Pts',(-3.09762202400006,11.6,-9.99482583600001));
#290834=CARTESIAN_POINT('Ctrl Pts',(-3.09694663700005,15.2,-9.99344936800002));
#290835=CARTESIAN_POINT('Ctrl Pts',(-3.09694663700005,11.6,-9.99344936800002));
#290836=CARTESIAN_POINT('Ctrl Pts',(-3.09627608500006,15.2,-9.99207947800001));
#290837=CARTESIAN_POINT('Ctrl Pts',(-3.09627608500006,11.6,-9.99207947800001));
#290838=CARTESIAN_POINT('Ctrl Pts',(-3.09561036200006,15.2,-9.99071618900001));
#290839=CARTESIAN_POINT('Ctrl Pts',(-3.09561036200006,11.6,-9.99071618900001));
#290840=CARTESIAN_POINT('Ctrl Pts',(-3.09494946600006,15.2,-9.98935952600001));
#290841=CARTESIAN_POINT('Ctrl Pts',(-3.09494946600006,11.6,-9.98935952600001));
#290842=CARTESIAN_POINT('Ctrl Pts',(-3.09429339200006,15.2,-9.98800951200001));
#290843=CARTESIAN_POINT('Ctrl Pts',(-3.09429339200006,11.6,-9.98800951200001));
#290844=CARTESIAN_POINT('Ctrl Pts',(-3.09364213600006,15.2,-9.98666617100001));
#290845=CARTESIAN_POINT('Ctrl Pts',(-3.09364213600006,11.6,-9.98666617100001));
#290846=CARTESIAN_POINT('Ctrl Pts',(-3.09299569400005,15.2,-9.98532952800001));
#290847=CARTESIAN_POINT('Ctrl Pts',(-3.09299569400005,11.6,-9.98532952800001));
#290848=CARTESIAN_POINT('Ctrl Pts',(-3.09235406100006,15.2,-9.98399960700001));
#290849=CARTESIAN_POINT('Ctrl Pts',(-3.09235406100006,11.6,-9.98399960700001));
#290850=CARTESIAN_POINT('Ctrl Pts',(-3.09171723400006,15.2,-9.98267643200001));
#290851=CARTESIAN_POINT('Ctrl Pts',(-3.09171723400006,11.6,-9.98267643200001));
#290852=CARTESIAN_POINT('Ctrl Pts',(-3.09108520700006,15.2,-9.98136002700001));
#290853=CARTESIAN_POINT('Ctrl Pts',(-3.09108520700006,11.6,-9.98136002700001));
#290854=CARTESIAN_POINT('Ctrl Pts',(-3.09045797700006,15.2,-9.98005041700001));
#290855=CARTESIAN_POINT('Ctrl Pts',(-3.09045797700006,11.6,-9.98005041700001));
#290856=CARTESIAN_POINT('Ctrl Pts',(-3.08983554000006,15.2,-9.97874762700001));
#290857=CARTESIAN_POINT('Ctrl Pts',(-3.08983554000006,11.6,-9.97874762700001));
#290858=CARTESIAN_POINT('Ctrl Pts',(-3.08921789100005,15.2,-9.97745168100001));
#290859=CARTESIAN_POINT('Ctrl Pts',(-3.08921789100005,11.6,-9.97745168100001));
#290860=CARTESIAN_POINT('Ctrl Pts',(-3.08860502600006,15.2,-9.97616260400001));
#290861=CARTESIAN_POINT('Ctrl Pts',(-3.08860502600006,11.6,-9.97616260400001));
#290862=CARTESIAN_POINT('Ctrl Pts',(-3.08799694000006,15.2,-9.97488042200001));
#290863=CARTESIAN_POINT('Ctrl Pts',(-3.08799694000006,11.6,-9.97488042200001));
#290864=CARTESIAN_POINT('Ctrl Pts',(-3.08739362900006,15.2,-9.97360515800001));
#290865=CARTESIAN_POINT('Ctrl Pts',(-3.08739362900006,11.6,-9.97360515800001));
#290866=CARTESIAN_POINT('Ctrl Pts',(-3.08679508800005,15.2,-9.97233683800001));
#290867=CARTESIAN_POINT('Ctrl Pts',(-3.08679508800005,11.6,-9.97233683800001));
#290868=CARTESIAN_POINT('Ctrl Pts',(-3.08620131400006,15.2,-9.97107548900001));
#290869=CARTESIAN_POINT('Ctrl Pts',(-3.08620131400006,11.6,-9.97107548900001));
#290870=CARTESIAN_POINT('Ctrl Pts',(-3.08561230000006,15.2,-9.96982113300001));
#290871=CARTESIAN_POINT('Ctrl Pts',(-3.08561230000006,11.6,-9.96982113300001));
#290872=CARTESIAN_POINT('Ctrl Pts',(-3.08502804400006,15.2,-9.96857379800001));
#290873=CARTESIAN_POINT('Ctrl Pts',(-3.08502804400006,11.6,-9.96857379800001));
#290874=CARTESIAN_POINT('Ctrl Pts',(-3.08444854000005,15.2,-9.96733350900001));
#290875=CARTESIAN_POINT('Ctrl Pts',(-3.08444854000005,11.6,-9.96733350900001));
#290876=CARTESIAN_POINT('Ctrl Pts',(-3.08387378200006,15.2,-9.96610029000001));
#290877=CARTESIAN_POINT('Ctrl Pts',(-3.08387378200006,11.6,-9.96610029000001));
#290878=CARTESIAN_POINT('Ctrl Pts',(-3.08330376800006,15.2,-9.96487416900001));
#290879=CARTESIAN_POINT('Ctrl Pts',(-3.08330376800006,11.6,-9.96487416900001));
#290880=CARTESIAN_POINT('Ctrl Pts',(-3.08273849300006,15.2,-9.96365517000001));
#290881=CARTESIAN_POINT('Ctrl Pts',(-3.08273849300006,11.6,-9.96365517000001));
#290882=CARTESIAN_POINT('Ctrl Pts',(-3.08217795000005,15.2,-9.96244332100001));
#290883=CARTESIAN_POINT('Ctrl Pts',(-3.08217795000005,11.6,-9.96244332100001));
#290884=CARTESIAN_POINT('Ctrl Pts',(-3.08162213700006,15.2,-9.96123864600001));
#290885=CARTESIAN_POINT('Ctrl Pts',(-3.08162213700006,11.6,-9.96123864600001));
#290886=CARTESIAN_POINT('Ctrl Pts',(-3.08107104600006,15.2,-9.96004117200001));
#290887=CARTESIAN_POINT('Ctrl Pts',(-3.08107104600006,11.6,-9.96004117200001));
#290888=CARTESIAN_POINT('Ctrl Pts',(-3.08052467500006,15.2,-9.95885092700002));
#290889=CARTESIAN_POINT('Ctrl Pts',(-3.08052467500006,11.6,-9.95885092700002));
#290890=CARTESIAN_POINT('Ctrl Pts',(-3.07998301800006,15.2,-9.95766793500001));
#290891=CARTESIAN_POINT('Ctrl Pts',(-3.07998301800006,11.6,-9.95766793500001));
#290892=CARTESIAN_POINT('Ctrl Pts',(-3.07944607000006,15.2,-9.95649222300001));
#290893=CARTESIAN_POINT('Ctrl Pts',(-3.07944607000006,11.6,-9.95649222300001));
#290894=CARTESIAN_POINT('Ctrl Pts',(-3.07891382700006,15.2,-9.95532381800001));
#290895=CARTESIAN_POINT('Ctrl Pts',(-3.07891382700006,11.6,-9.95532381800001));
#290896=CARTESIAN_POINT('Ctrl Pts',(-3.07838628300006,15.2,-9.95416274700001));
#290897=CARTESIAN_POINT('Ctrl Pts',(-3.07838628300006,11.6,-9.95416274700001));
#290898=CARTESIAN_POINT('Ctrl Pts',(-3.07786343200006,15.2,-9.95300903700001));
#290899=CARTESIAN_POINT('Ctrl Pts',(-3.07786343200006,11.6,-9.95300903700001));
#290900=CARTESIAN_POINT('Ctrl Pts',(-3.07734527100005,15.2,-9.95186271400001));
#290901=CARTESIAN_POINT('Ctrl Pts',(-3.07734527100005,11.6,-9.95186271400001));
#290902=CARTESIAN_POINT('Ctrl Pts',(-3.07683179400006,15.2,-9.95072380600002));
#290903=CARTESIAN_POINT('Ctrl Pts',(-3.07683179400006,11.6,-9.95072380600002));
#290904=CARTESIAN_POINT('Ctrl Pts',(-3.07632299600006,15.2,-9.94959234000001));
#290905=CARTESIAN_POINT('Ctrl Pts',(-3.07632299600006,11.6,-9.94959234000001));
#290906=CARTESIAN_POINT('Ctrl Pts',(-3.07581887200006,15.2,-9.94846834300001));
#290907=CARTESIAN_POINT('Ctrl Pts',(-3.07581887200006,11.6,-9.94846834300001));
#290908=CARTESIAN_POINT('Ctrl Pts',(-3.07531941600006,15.2,-9.94735184300001));
#290909=CARTESIAN_POINT('Ctrl Pts',(-3.07531941600006,11.6,-9.94735184300001));
#290910=CARTESIAN_POINT('Ctrl Pts',(-3.07482462400006,15.2,-9.94624286700001));
#290911=CARTESIAN_POINT('Ctrl Pts',(-3.07482462400006,11.6,-9.94624286700001));
#290912=CARTESIAN_POINT('Ctrl Pts',(-3.07433449000006,15.2,-9.94514144400001));
#290913=CARTESIAN_POINT('Ctrl Pts',(-3.07433449000006,11.6,-9.94514144400001));
#290914=CARTESIAN_POINT('Ctrl Pts',(-3.07384900800006,15.2,-9.94404760000001));
#290915=CARTESIAN_POINT('Ctrl Pts',(-3.07384900800006,11.6,-9.94404760000001));
#290916=CARTESIAN_POINT('Ctrl Pts',(-3.07336817400006,15.2,-9.94296136400001));
#290917=CARTESIAN_POINT('Ctrl Pts',(-3.07336817400006,11.6,-9.94296136400001));
#290918=CARTESIAN_POINT('Ctrl Pts',(-3.07289198200006,15.2,-9.94188276500001));
#290919=CARTESIAN_POINT('Ctrl Pts',(-3.07289198200006,11.6,-9.94188276500001));
#290920=CARTESIAN_POINT('Ctrl Pts',(-3.07242042600006,15.2,-9.94081182900001));
#290921=CARTESIAN_POINT('Ctrl Pts',(-3.07242042600006,11.6,-9.94081182900001));
#290922=CARTESIAN_POINT('Ctrl Pts',(-3.07195350200006,15.2,-9.93974858600001));
#290923=CARTESIAN_POINT('Ctrl Pts',(-3.07195350200006,11.6,-9.93974858600001));
#290924=CARTESIAN_POINT('Ctrl Pts',(-3.07149120300005,15.2,-9.93869306300001));
#290925=CARTESIAN_POINT('Ctrl Pts',(-3.07149120300005,11.6,-9.93869306300001));
#290926=CARTESIAN_POINT('Ctrl Pts',(-3.07103352500006,15.2,-9.93764529100002));
#290927=CARTESIAN_POINT('Ctrl Pts',(-3.07103352500006,11.6,-9.93764529100002));
#290928=CARTESIAN_POINT('Ctrl Pts',(-3.07058046000006,15.2,-9.93660529500001));
#290929=CARTESIAN_POINT('Ctrl Pts',(-3.07058046000006,11.6,-9.93660529500001));
#290930=CARTESIAN_POINT('Ctrl Pts',(-3.07013200500006,15.2,-9.93557310800002));
#290931=CARTESIAN_POINT('Ctrl Pts',(-3.07013200500006,11.6,-9.93557310800002));
#290932=CARTESIAN_POINT('Ctrl Pts',(-3.06968815300006,15.2,-9.93454875700001));
#290933=CARTESIAN_POINT('Ctrl Pts',(-3.06968815300006,11.6,-9.93454875700001));
#290934=CARTESIAN_POINT('Ctrl Pts',(-3.06924889800006,15.2,-9.93353227000001));
#290935=CARTESIAN_POINT('Ctrl Pts',(-3.06924889800006,11.6,-9.93353227000001));
#290936=CARTESIAN_POINT('Ctrl Pts',(-3.06881423500006,15.2,-9.93252367900001));
#290937=CARTESIAN_POINT('Ctrl Pts',(-3.06881423500006,11.6,-9.93252367900001));
#290938=CARTESIAN_POINT('Ctrl Pts',(-3.06838415800006,15.2,-9.93152301000001));
#290939=CARTESIAN_POINT('Ctrl Pts',(-3.06838415800006,11.6,-9.93152301000001));
#290940=CARTESIAN_POINT('Ctrl Pts',(-3.06795866100006,15.2,-9.93053029600001));
#290941=CARTESIAN_POINT('Ctrl Pts',(-3.06795866100006,11.6,-9.93053029600001));
#290942=CARTESIAN_POINT('Ctrl Pts',(-3.06753773900006,15.2,-9.92954556400001));
#290943=CARTESIAN_POINT('Ctrl Pts',(-3.06753773900006,11.6,-9.92954556400001));
#290944=CARTESIAN_POINT('Ctrl Pts',(-3.06712138400006,15.2,-9.92856884600001));
#290945=CARTESIAN_POINT('Ctrl Pts',(-3.06712138400006,11.6,-9.92856884600001));
#290946=CARTESIAN_POINT('Ctrl Pts',(-3.06670959200006,15.2,-9.92760017000001));
#290947=CARTESIAN_POINT('Ctrl Pts',(-3.06670959200006,11.6,-9.92760017000001));
#290948=CARTESIAN_POINT('Ctrl Pts',(-3.06630235700006,15.2,-9.92663956700001));
#290949=CARTESIAN_POINT('Ctrl Pts',(-3.06630235700006,11.6,-9.92663956700001));
#290950=CARTESIAN_POINT('Ctrl Pts',(-3.06589967200006,15.2,-9.92568706800001));
#290951=CARTESIAN_POINT('Ctrl Pts',(-3.06589967200006,11.6,-9.92568706800001));
#290952=CARTESIAN_POINT('Ctrl Pts',(-3.06550153000006,15.2,-9.92474270100001));
#290953=CARTESIAN_POINT('Ctrl Pts',(-3.06550153000006,11.6,-9.92474270100001));
#290954=CARTESIAN_POINT('Ctrl Pts',(-3.06510792800006,15.2,-9.92380649800001));
#290955=CARTESIAN_POINT('Ctrl Pts',(-3.06510792800006,11.6,-9.92380649800001));
#290956=CARTESIAN_POINT('Ctrl Pts',(-3.06471885700006,15.2,-9.92287849000001));
#290957=CARTESIAN_POINT('Ctrl Pts',(-3.06471885700006,11.6,-9.92287849000001));
#290958=CARTESIAN_POINT('Ctrl Pts',(-3.06433431200006,15.2,-9.92195870800001));
#290959=CARTESIAN_POINT('Ctrl Pts',(-3.06433431200006,11.6,-9.92195870800001));
#290960=CARTESIAN_POINT('Ctrl Pts',(-3.06395428700006,15.2,-9.92104718300001));
#290961=CARTESIAN_POINT('Ctrl Pts',(-3.06395428700006,11.6,-9.92104718300001));
#290962=CARTESIAN_POINT('Ctrl Pts',(-3.06357877400006,15.2,-9.92014394500002));
#290963=CARTESIAN_POINT('Ctrl Pts',(-3.06357877400006,11.6,-9.92014394500002));
#290964=CARTESIAN_POINT('Ctrl Pts',(-3.06320776900006,15.2,-9.91924902500001));
#290965=CARTESIAN_POINT('Ctrl Pts',(-3.06320776900006,11.6,-9.91924902500001));
#290966=CARTESIAN_POINT('Ctrl Pts',(-3.06284126400006,15.2,-9.91836245500001));
#290967=CARTESIAN_POINT('Ctrl Pts',(-3.06284126400006,11.6,-9.91836245500001));
#290968=CARTESIAN_POINT('Ctrl Pts',(-3.06247925300006,15.2,-9.91748426800001));
#290969=CARTESIAN_POINT('Ctrl Pts',(-3.06247925300006,11.6,-9.91748426800001));
#290970=CARTESIAN_POINT('Ctrl Pts',(-3.06212173000006,15.2,-9.91661449400001));
#290971=CARTESIAN_POINT('Ctrl Pts',(-3.06212173000006,11.6,-9.91661449400001));
#290972=CARTESIAN_POINT('Ctrl Pts',(-3.06176868800006,15.2,-9.91575316500001));
#290973=CARTESIAN_POINT('Ctrl Pts',(-3.06176868800006,11.6,-9.91575316500001));
#290974=CARTESIAN_POINT('Ctrl Pts',(-3.06142212800005,15.2,-9.91490522700001));
#290975=CARTESIAN_POINT('Ctrl Pts',(-3.06142212800005,11.6,-9.91490522700001));
#290976=CARTESIAN_POINT('Ctrl Pts',(-3.06114880300006,15.2,-9.91423456700001));
#290977=CARTESIAN_POINT('Ctrl Pts',(-3.06114880300006,11.6,-9.91423456700001));
#290978=CARTESIAN_POINT('Ctrl Pts',(-3.06094627500006,15.2,-9.91373655900001));
#290979=CARTESIAN_POINT('Ctrl Pts',(-3.06094627500006,11.6,-9.91373655900001));
#290980=CARTESIAN_POINT('Ctrl Pts',(-3.06081277600006,15.2,-9.91340782600002));
#290981=CARTESIAN_POINT('Ctrl Pts',(-3.06081277600006,11.6,-9.91340782600002));
#290982=CARTESIAN_POINT('Ctrl Pts',(-3.06074721300006,15.2,-9.91324626500001));
#290983=CARTESIAN_POINT('Ctrl Pts',(-3.06074721300006,11.6,-9.91324626500001));
#290984=CARTESIAN_POINT('',(-3.06074721303514,12.2,-9.91324626444698));
#290985=CARTESIAN_POINT('',(-3.06074721303514,15.2,-9.91324626444698));
#290986=CARTESIAN_POINT('',(-3.06074721300006,12.2,-9.91324626400001));
#290987=CARTESIAN_POINT('Ctrl Pts',(-3.76106045600006,12.2,-10.867585944));
#290988=CARTESIAN_POINT('Ctrl Pts',(-3.75835329800824,12.2,-10.8648866810023));
#290989=CARTESIAN_POINT('Ctrl Pts',(-3.75565386775155,12.2,-10.8621890332137));
#290990=CARTESIAN_POINT('Ctrl Pts',(-3.75296217351105,12.2,-10.8594930000052));
#290991=CARTESIAN_POINT('Ctrl Pts',(-3.75027047927055,12.2,-10.8567969667966));
#290992=CARTESIAN_POINT('Ctrl Pts',(-3.74758651975522,12.2,-10.8541025490412));
#290993=CARTESIAN_POINT('Ctrl Pts',(-3.74491029621786,12.2,-10.8514097635877));
#290994=CARTESIAN_POINT('Ctrl Pts',(-3.74223407268051,12.2,-10.8487169781341));
#290995=CARTESIAN_POINT('Ctrl Pts',(-3.73956558451776,12.2,-10.8460258263555));
#290996=CARTESIAN_POINT('Ctrl Pts',(-3.73690483861338,12.2,-10.8433363508696));
#290997=CARTESIAN_POINT('Ctrl Pts',(-3.73424409222563,12.2,-10.8406468748952));
#290998=CARTESIAN_POINT('Ctrl Pts',(-3.73159108729007,12.2,-10.8379590765212));
#290999=CARTESIAN_POINT('Ctrl Pts',(-3.72894582899001,12.2,-10.8352730049228));
#291000=CARTESIAN_POINT('Ctrl Pts',(-3.72630057117051,12.2,-10.8325869338123));
#291001=CARTESIAN_POINT('Ctrl Pts',(-3.72366306001726,12.2,-10.8299025881433));
#291002=CARTESIAN_POINT('Ctrl Pts',(-3.72103329923849,12.2,-10.8272200094076));
#291003=CARTESIAN_POINT('Ctrl Pts',(-3.7175269516927,12.2,-10.8236432379225));
#291004=CARTESIAN_POINT('Ctrl Pts',(-3.7140343843038,12.2,-10.8200696049215));
#291005=CARTESIAN_POINT('Ctrl Pts',(-3.71055560524654,12.2,-10.8164991980348));
#291006=CARTESIAN_POINT('Ctrl Pts',(-3.7070768257153,12.2,-10.8129287906616));
#291007=CARTESIAN_POINT('Ctrl Pts',(-3.70361183581352,12.2,-10.8093616114055));
#291008=CARTESIAN_POINT('Ctrl Pts',(-3.70016064445966,12.2,-10.8057977609337));
#291009=CARTESIAN_POINT('Ctrl Pts',(-3.69757225117938,12.2,-10.8031248733226));
#291010=CARTESIAN_POINT('Ctrl Pts',(-3.69499162030653,12.2,-10.8004538583864));
#291011=CARTESIAN_POINT('Ctrl Pts',(-3.69241875548333,12.2,-10.797784756775));
#291012=CARTESIAN_POINT('Ctrl Pts',(-3.68984589066014,12.2,-10.7951156551636));
#291013=CARTESIAN_POINT('Ctrl Pts',(-3.68728079206997,12.2,-10.7924484677272));
#291014=CARTESIAN_POINT('Ctrl Pts',(-3.68472346328722,12.2,-10.7897832350322));
#291015=CARTESIAN_POINT('Ctrl Pts',(-3.68216613450446,12.2,-10.7871180023372));
#291016=CARTESIAN_POINT('Ctrl Pts',(-3.67961657667738,12.2,-10.7844547230181));
#291017=CARTESIAN_POINT('Ctrl Pts',(-3.67707479222519,12.2,-10.7817934402733));
#291018=CARTESIAN_POINT('Ctrl Pts',(-3.67453300777299,12.2,-10.7791321575284));
#291019=CARTESIAN_POINT('Ctrl Pts',(-3.67199899714333,12.2,-10.776472871883));
#291020=CARTESIAN_POINT('Ctrl Pts',(-3.66947276481739,12.2,-10.7738156233126));
#291021=CARTESIAN_POINT('Ctrl Pts',(-3.66694653203252,12.2,-10.7711583742595));
#291022=CARTESIAN_POINT('Ctrl Pts',(-3.66442807716651,12.2,-10.7685031633069));
#291023=CARTESIAN_POINT('Ctrl Pts',(-3.66191740388602,12.2,-10.7658500331716));
#291024=CARTESIAN_POINT('Ctrl Pts',(-3.65940673106163,12.2,-10.7631969035183));
#291025=CARTESIAN_POINT('Ctrl Pts',(-3.65690383987016,12.2,-10.7605458540315));
#291026=CARTESIAN_POINT('Ctrl Pts',(-3.6544087344615,12.2,-10.7578969264613));
#291027=CARTESIAN_POINT('Ctrl Pts',(-3.65191362905284,12.2,-10.7552479988911));
#291028=CARTESIAN_POINT('Ctrl Pts',(-3.64942630861889,12.2,-10.7526011945802));
#291029=CARTESIAN_POINT('Ctrl Pts',(-3.64694677723942,12.2,-10.7499565545393));
#291030=CARTESIAN_POINT('Ctrl Pts',(-3.64446724585995,12.2,-10.7473119144984));
#291031=CARTESIAN_POINT('Ctrl Pts',(-3.64199550337394,12.2,-10.7446694403018));
#291032=CARTESIAN_POINT('Ctrl Pts',(-3.63953155353558,12.2,-10.7420291727607));
#291033=CARTESIAN_POINT('Ctrl Pts',(-3.63706760369721,12.2,-10.7393889052197));
#291034=CARTESIAN_POINT('Ctrl Pts',(-3.63461144629539,12.2,-10.7367508449084));
#291035=CARTESIAN_POINT('Ctrl Pts',(-3.632163084967,12.2,-10.734115036754));
#291036=CARTESIAN_POINT('Ctrl Pts',(-3.62889860289929,12.2,-10.7306006255622));
#291037=CARTESIAN_POINT('Ctrl Pts',(-3.62564797998048,12.2,-10.7270902149876));
#291038=CARTESIAN_POINT('Ctrl Pts',(-3.62241122452719,12.2,-10.7235839084634));
#291039=CARTESIAN_POINT('Ctrl Pts',(-3.61998365815773,12.2,-10.7209541788091));
#291040=CARTESIAN_POINT('Ctrl Pts',(-3.61756389206236,12.2,-10.7183267569546));
#291041=CARTESIAN_POINT('Ctrl Pts',(-3.61515192973333,12.2,-10.7157016882167));
#291042=CARTESIAN_POINT('Ctrl Pts',(-3.6127399674043,12.2,-10.7130766194787));
#291043=CARTESIAN_POINT('Ctrl Pts',(-3.61033580902495,12.2,-10.710453901524));
#291044=CARTESIAN_POINT('Ctrl Pts',(-3.607939456278,12.2,-10.7078335803273));
#291045=CARTESIAN_POINT('Ctrl Pts',(-3.60554310353106,12.2,-10.7052132591306));
#291046=CARTESIAN_POINT('Ctrl Pts',(-3.60315455887737,12.2,-10.702595333542));
#291047=CARTESIAN_POINT('Ctrl Pts',(-3.60077382296903,12.2,-10.6999798477977));
#291048=CARTESIAN_POINT('Ctrl Pts',(-3.59839308706069,12.2,-10.6973643620535));
#291049=CARTESIAN_POINT('Ctrl Pts',(-3.59602016111406,12.2,-10.6947513154079));
#291050=CARTESIAN_POINT('Ctrl Pts',(-3.5936550477406,12.2,-10.6921407537941));
#291051=CARTESIAN_POINT('Ctrl Pts',(-3.59128993393748,12.2,-10.689530191706));
#291052=CARTESIAN_POINT('Ctrl Pts',(-3.58893263269488,12.2,-10.6869221137937));
#291053=CARTESIAN_POINT('Ctrl Pts',(-3.58658314777116,12.2,-10.684316564707));
#291054=CARTESIAN_POINT('Ctrl Pts',(-3.58423366327425,12.2,-10.6817110160937));
#291055=CARTESIAN_POINT('Ctrl Pts',(-3.58189199216026,12.2,-10.6791079957052));
#291056=CARTESIAN_POINT('Ctrl Pts',(-3.57955814120407,12.2,-10.6765075487166));
#291057=CARTESIAN_POINT('Ctrl Pts',(-3.57722429024789,12.2,-10.673907101728));
#291058=CARTESIAN_POINT('Ctrl Pts',(-3.57489825739083,12.2,-10.6713092294818));
#291059=CARTESIAN_POINT('Ctrl Pts',(-3.57258004550623,12.2,-10.668713974481));
#291060=CARTESIAN_POINT('Ctrl Pts',(-3.57026183362163,12.2,-10.6661187194802));
#291061=CARTESIAN_POINT('Ctrl Pts',(-3.56795144256226,12.2,-10.6635260830867));
#291062=CARTESIAN_POINT('Ctrl Pts',(-3.56564887521876,12.2,-10.6609361110023));
#291063=CARTESIAN_POINT('Ctrl Pts',(-3.56334630787527,12.2,-10.658346138918));
#291064=CARTESIAN_POINT('Ctrl Pts',(-3.56105156405033,12.2,-10.6557588308548));
#291065=CARTESIAN_POINT('Ctrl Pts',(-3.55876464617441,12.2,-10.6531742317818));
#291066=CARTESIAN_POINT('Ctrl Pts',(-3.55647772829848,12.2,-10.6505896327088));
#291067=CARTESIAN_POINT('Ctrl Pts',(-3.55419863698036,12.2,-10.6480077426689));
#291068=CARTESIAN_POINT('Ctrl Pts',(-3.55192737402014,12.2,-10.6454286085956));
#291069=CARTESIAN_POINT('Ctrl Pts',(-3.54965611064731,12.2,-10.6428494740537));
#291070=CARTESIAN_POINT('Ctrl Pts',(-3.5473926746517,12.2,-10.6402730948793));
#291071=CARTESIAN_POINT('Ctrl Pts',(-3.54513707074162,12.2,-10.6376995164223));
#291072=CARTESIAN_POINT('Ctrl Pts',(-3.54288146724131,12.2,-10.6351259384329));
#291073=CARTESIAN_POINT('Ctrl Pts',(-3.54063369286298,12.2,-10.6325551624545));
#291074=CARTESIAN_POINT('Ctrl Pts',(-3.5383937522917,12.2,-10.6299872337948));
#291075=CARTESIAN_POINT('Ctrl Pts',(-3.53615381172042,12.2,-10.6274193051352));
#291076=CARTESIAN_POINT('Ctrl Pts',(-3.53392170394285,12.2,-10.6248542244441));
#291077=CARTESIAN_POINT('Ctrl Pts',(-3.53169743152436,12.2,-10.6222920379958));
#291078=CARTESIAN_POINT('Ctrl Pts',(-3.52947315910586,12.2,-10.6197298515475));
#291079=CARTESIAN_POINT('Ctrl Pts',(-3.52725672165308,12.2,-10.6171705603738));
#291080=CARTESIAN_POINT('Ctrl Pts',(-3.52504812123333,12.2,-10.6146142094667));
#291081=CARTESIAN_POINT('Ctrl Pts',(-3.52136712039999,12.2,-10.6103536244667));
#291082=CARTESIAN_POINT('Ctrl Pts',(-3.51770788779226,12.2,-10.6061012102392));
#291083=CARTESIAN_POINT('Ctrl Pts',(-3.51407043374802,12.2,-10.601857185706));
#291084=CARTESIAN_POINT('Ctrl Pts',(-3.51188796140077,12.2,-10.5993107710786));
#291085=CARTESIAN_POINT('Ctrl Pts',(-3.50971333014979,12.2,-10.5967673760882));
#291086=CARTESIAN_POINT('Ctrl Pts',(-3.5075465397603,12.2,-10.594227049044));
#291087=CARTESIAN_POINT('Ctrl Pts',(-3.50465748564524,12.2,-10.5908399460106));
#291088=CARTESIAN_POINT('Ctrl Pts',(-3.50178237215338,12.2,-10.5874582980592));
#291089=CARTESIAN_POINT('Ctrl Pts',(-3.49892120399887,12.2,-10.5840822164313));
#291090=CARTESIAN_POINT('Ctrl Pts',(-3.4960600362342,12.2,-10.5807061352635));
#291091=CARTESIAN_POINT('Ctrl Pts',(-3.49321281240659,12.2,-10.577335622131));
#291092=CARTESIAN_POINT('Ctrl Pts',(-3.49037953674842,12.2,-10.5739707910168));
#291093=CARTESIAN_POINT('Ctrl Pts',(-3.48754626070421,12.2,-10.5706059594441));
#291094=CARTESIAN_POINT('Ctrl Pts',(-3.48472693437094,12.2,-10.5672468110938));
#291095=CARTESIAN_POINT('Ctrl Pts',(-3.48192155813467,12.2,-10.5638934600218));
#291096=CARTESIAN_POINT('Ctrl Pts',(-3.47911618228063,12.2,-10.5605401094067));
#291097=CARTESIAN_POINT('Ctrl Pts',(-3.47632475713438,12.2,-10.557192557056));
#291098=CARTESIAN_POINT('Ctrl Pts',(-3.47354728669386,12.2,-10.5538509197732));
#291099=CARTESIAN_POINT('Ctrl Pts',(-3.47076981587491,12.2,-10.5505092820352));
#291100=CARTESIAN_POINT('Ctrl Pts',(-3.46800629958263,12.2,-10.5471735585728));
#291101=CARTESIAN_POINT('Ctrl Pts',(-3.46525673826702,12.2,-10.5438438670028));
#291102=CARTESIAN_POINT('Ctrl Pts',(-3.46250717732603,12.2,-10.5405141758866));
#291103=CARTESIAN_POINT('Ctrl Pts',(-3.4597715748847,12.2,-10.5371905170043));
#291104=CARTESIAN_POINT('Ctrl Pts',(-3.45704992913667,12.2,-10.5338730089981));
#291105=CARTESIAN_POINT('Ctrl Pts',(-3.45432828301782,12.2,-10.5305555005399));
#291106=CARTESIAN_POINT('Ctrl Pts',(-3.45162059696194,12.2,-10.5272441427179));
#291107=CARTESIAN_POINT('Ctrl Pts',(-3.44892686953825,12.2,-10.5239390557049));
#291108=CARTESIAN_POINT('Ctrl Pts',(-3.44623314248158,12.2,-10.5206339691421));
#291109=CARTESIAN_POINT('Ctrl Pts',(-3.44355337610269,12.2,-10.5173351528892));
#291110=CARTESIAN_POINT('Ctrl Pts',(-3.44088757098587,12.2,-10.5140427265466));
#291111=CARTESIAN_POINT('Ctrl Pts',(-3.43822176550583,12.2,-10.5107502997554));
#291112=CARTESIAN_POINT('Ctrl Pts',(-3.43556992182613,12.2,-10.5074642644691));
#291113=CARTESIAN_POINT('Ctrl Pts',(-3.43293203978154,12.2,-10.5041847414978));
#291114=CARTESIAN_POINT('Ctrl Pts',(-3.43029415809635,12.2,-10.5009052189732));
#291115=CARTESIAN_POINT('Ctrl Pts',(-3.42767023889257,12.2,-10.4976322078816));
#291116=CARTESIAN_POINT('Ctrl Pts',(-3.42506028366007,12.2,-10.494365832759));
#291117=CARTESIAN_POINT('Ctrl Pts',(-3.42245032807196,12.2,-10.4910994571915));
#291118=CARTESIAN_POINT('Ctrl Pts',(-3.41985433508793,12.2,-10.4878397158106));
#291119=CARTESIAN_POINT('Ctrl Pts',(-3.41727230555833,12.2,-10.4845867329667));
#291120=CARTESIAN_POINT('Ctrl Pts',(-3.41469027602873,12.2,-10.4813337501227));
#291121=CARTESIAN_POINT('Ctrl Pts',(-3.41212220833408,12.2,-10.4780875264045));
#291122=CARTESIAN_POINT('Ctrl Pts',(-3.40956810480741,12.2,-10.4748481867287));
#291123=CARTESIAN_POINT('Ctrl Pts',(-3.40701400162875,12.2,-10.4716088474942));
#291124=CARTESIAN_POINT('Ctrl Pts',(-3.4044738615734,12.2,-10.468376389431));
#291125=CARTESIAN_POINT('Ctrl Pts',(-3.40194768376839,12.2,-10.4651509422355));
#291126=CARTESIAN_POINT('Ctrl Pts',(-3.39942150561919,12.2,-10.4619254946006));
#291127=CARTESIAN_POINT('Ctrl Pts',(-3.39690928899016,12.2,-10.4587070565909));
#291128=CARTESIAN_POINT('Ctrl Pts',(-3.39441103479988,12.2,-10.4554957532499));
#291129=CARTESIAN_POINT('Ctrl Pts',(-3.39191278094997,12.2,-10.4522844503465));
#291130=CARTESIAN_POINT('Ctrl Pts',(-3.38942848935381,12.2,-10.4490802841172));
#291131=CARTESIAN_POINT('Ctrl Pts',(-3.38695815694375,12.2,-10.4458833817114));
#291132=CARTESIAN_POINT('Ctrl Pts',(-3.3844878241971,12.2,-10.44268647887));
#291133=CARTESIAN_POINT('Ctrl Pts',(-3.38203145127989,12.2,-10.4394968398767));
#291134=CARTESIAN_POINT('Ctrl Pts',(-3.37958903709213,12.2,-10.4363145949816));
#291135=CARTESIAN_POINT('Ctrl Pts',(-3.37714662323716,12.2,-10.43313235052));
#291136=CARTESIAN_POINT('Ctrl Pts',(-3.37471816771099,12.2,-10.4299574991818));
#291137=CARTESIAN_POINT('Ctrl Pts',(-3.3723036678421,12.2,-10.4267901707263));
#291138=CARTESIAN_POINT('Ctrl Pts',(-3.36988916764423,12.2,-10.4236228418392));
#291139=CARTESIAN_POINT('Ctrl Pts',(-3.36748862427863,12.2,-10.4204630375525));
#291140=CARTESIAN_POINT('Ctrl Pts',(-3.36510203403836,12.2,-10.4173108874924));
#291141=CARTESIAN_POINT('Ctrl Pts',(-3.36271544412327,12.2,-10.4141587378617));
#291142=CARTESIAN_POINT('Ctrl Pts',(-3.36034280662203,12.2,-10.4110142448766));
#291143=CARTESIAN_POINT('Ctrl Pts',(-3.35798412136899,12.2,-10.4078775385212));
#291144=CARTESIAN_POINT('Ctrl Pts',(-3.35562543579457,12.2,-10.4047408317383));
#291145=CARTESIAN_POINT('Ctrl Pts',(-3.3532806990332,12.2,-10.4016119138099));
#291146=CARTESIAN_POINT('Ctrl Pts',(-3.35094991017341,12.2,-10.3984909165145));
#291147=CARTESIAN_POINT('Ctrl Pts',(-3.3486191216312,12.2,-10.3953699196444));
#291148=CARTESIAN_POINT('Ctrl Pts',(-3.34630227943413,12.2,-10.3922568450713));
#291149=CARTESIAN_POINT('Ctrl Pts',(-3.3439993808432,12.2,-10.389151827991));
#291150=CARTESIAN_POINT('Ctrl Pts',(-3.34169648193849,12.2,-10.3860468104876));
#291151=CARTESIAN_POINT('Ctrl Pts',(-3.33940752569898,12.2,-10.3829498492378));
#291152=CARTESIAN_POINT('Ctrl Pts',(-3.33713250874166,12.2,-10.3798610817916));
#291153=CARTESIAN_POINT('Ctrl Pts',(-3.33485749178434,12.2,-10.3767723143455));
#291154=CARTESIAN_POINT('Ctrl Pts',(-3.3325964117342,12.2,-10.3736917406059));
#291155=CARTESIAN_POINT('Ctrl Pts',(-3.33034926689093,12.2,-10.3706194979393));
#291156=CARTESIAN_POINT('Ctrl Pts',(-3.32810212235384,12.2,-10.3675472556913));
#291157=CARTESIAN_POINT('Ctrl Pts',(-3.32586891203021,12.2,-10.3644833448467));
#291158=CARTESIAN_POINT('Ctrl Pts',(-3.32364962953485,12.2,-10.3614279040271));
#291159=CARTESIAN_POINT('Ctrl Pts',(-3.32143034673711,12.2,-10.3583724627911));
#291160=CARTESIAN_POINT('Ctrl Pts',(-3.31922499279305,12.2,-10.3553254922679));
#291161=CARTESIAN_POINT('Ctrl Pts',(-3.31703356067505,12.2,-10.3522871327699));
#291162=CARTESIAN_POINT('Ctrl Pts',(-3.31484212885563,12.2,-10.3492487736858));
#291163=CARTESIAN_POINT('Ctrl Pts',(-3.31266462140105,12.2,-10.3462190252256));
#291164=CARTESIAN_POINT('Ctrl Pts',(-3.31050102891034,12.2,-10.343198028972));
#291165=CARTESIAN_POINT('Ctrl Pts',(-3.30833743612485,12.2,-10.3401770323068));
#291166=CARTESIAN_POINT('Ctrl Pts',(-3.30618775946761,12.2,-10.3371647890883));
#291167=CARTESIAN_POINT('Ctrl Pts',(-3.30405199369016,12.2,-10.3341614403309));
#291168=CARTESIAN_POINT('Ctrl Pts',(-3.30191622820371,12.2,-10.3311580919827));
#291169=CARTESIAN_POINT('Ctrl Pts',(-3.29979437152604,12.2,-10.3281636393895));
#291170=CARTESIAN_POINT('Ctrl Pts',(-3.29768641819746,12.2,-10.3251782277441));
#291171=CARTESIAN_POINT('Ctrl Pts',(-3.29557846458167,12.2,-10.3221928156919));
#291172=CARTESIAN_POINT('Ctrl Pts',(-3.29348441217865,12.2,-10.3192164420575));
#291173=CARTESIAN_POINT('Ctrl Pts',(-3.29140425478841,12.2,-10.3162492560075));
#291174=CARTESIAN_POINT('Ctrl Pts',(-3.28932409768159,12.2,-10.3132820703618));
#291175=CARTESIAN_POINT('Ctrl Pts',(-3.28725783687829,12.2,-10.3103240715044));
#291176=CARTESIAN_POINT('Ctrl Pts',(-3.28520546149789,12.2,-10.3073754046529));
#291177=CARTESIAN_POINT('Ctrl Pts',(-3.28315308583786,12.2,-10.3044267373996));
#291178=CARTESIAN_POINT('Ctrl Pts',(-3.28111459710795,12.2,-10.3014874054807));
#291179=CARTESIAN_POINT('Ctrl Pts',(-3.27908998560962,12.2,-10.2985575555439));
#291180=CARTESIAN_POINT('Ctrl Pts',(-3.27706537438714,12.2,-10.2956277060062));
#291181=CARTESIAN_POINT('Ctrl Pts',(-3.27505464057856,12.2,-10.2927073387));
#291182=CARTESIAN_POINT('Ctrl Pts',(-3.2730577753515,12.2,-10.2897966044926));
#291183=CARTESIAN_POINT('Ctrl Pts',(-3.27106090985235,12.2,-10.2868858698885));
#291184=CARTESIAN_POINT('Ctrl Pts',(-3.26907791397877,12.2,-10.2839847678798));
#291185=CARTESIAN_POINT('Ctrl Pts',(-3.267108775807,12.2,-10.2810934512647));
#291186=CARTESIAN_POINT('Ctrl Pts',(-3.26464735322643,12.2,-10.2774793056927));
#291187=CARTESIAN_POINT('Ctrl Pts',(-3.26220758391863,12.2,-10.2738804496538));
#291188=CARTESIAN_POINT('Ctrl Pts',(-3.25978944885032,12.2,-10.2702971818074));
#291189=CARTESIAN_POINT('Ctrl Pts',(-3.25785494095382,12.2,-10.2674305677646));
#291190=CARTESIAN_POINT('Ctrl Pts',(-3.2559342784962,12.2,-10.2645739314448));
#291191=CARTESIAN_POINT('Ctrl Pts',(-3.25402745109511,12.2,-10.2617274278987));
#291192=CARTESIAN_POINT('Ctrl Pts',(-3.25212062343421,12.2,-10.2588809239648));
#291193=CARTESIAN_POINT('Ctrl Pts',(-3.25022762948462,12.2,-10.2560445534066));
#291194=CARTESIAN_POINT('Ctrl Pts',(-3.24834845854039,12.2,-10.2532184717397));
#291195=CARTESIAN_POINT('Ctrl Pts',(-3.24646928785219,12.2,-10.2503923904579));
#291196=CARTESIAN_POINT('Ctrl Pts',(-3.24460394011389,12.2,-10.2475766005137));
#291197=CARTESIAN_POINT('Ctrl Pts',(-3.2427524028194,12.2,-10.2447712584087));
#291198=CARTESIAN_POINT('Ctrl Pts',(-3.24090086527264,12.2,-10.2419659159214));
#291199=CARTESIAN_POINT('Ctrl Pts',(-3.23906313770495,12.2,-10.2391710219489));
#291200=CARTESIAN_POINT('Ctrl Pts',(-3.23723920871666,12.2,-10.2363867387416));
#291201=CARTESIAN_POINT('Ctrl Pts',(-3.23495929760556,12.2,-10.2329063849222));
#291202=CARTESIAN_POINT('Ctrl Pts',(-3.23270094429777,12.2,-10.229442607397));
#291203=CARTESIAN_POINT('Ctrl Pts',(-3.23046412477379,12.2,-10.2259957252981));
#291204=CARTESIAN_POINT('Ctrl Pts',(-3.2282273052498,12.2,-10.2225488431992));
#291205=CARTESIAN_POINT('Ctrl Pts',(-3.22601201728332,12.2,-10.2191188550371));
#291206=CARTESIAN_POINT('Ctrl Pts',(-3.22381823533999,12.2,-10.2157060845519));
#291207=CARTESIAN_POINT('Ctrl Pts',(-3.22162445339668,12.2,-10.2122933140667));
#291208=CARTESIAN_POINT('Ctrl Pts',(-3.21945217529168,12.2,-10.2088977589283));
#291209=CARTESIAN_POINT('Ctrl Pts',(-3.21730137258447,12.2,-10.2055197485125));
#291210=CARTESIAN_POINT('Ctrl Pts',(-3.21515056987726,12.2,-10.2021417380967));
#291211=CARTESIAN_POINT('Ctrl Pts',(-3.21302124374448,12.2,-10.1987812701083));
#291212=CARTESIAN_POINT('Ctrl Pts',(-3.21091336103728,12.2,-10.1954386764981));
#291213=CARTESIAN_POINT('Ctrl Pts',(-3.20880547833007,12.2,-10.192096082888));
#291214=CARTESIAN_POINT('Ctrl Pts',(-3.20671904064537,12.2,-10.1887713637412));
#291215=CARTESIAN_POINT('Ctrl Pts',(-3.20465401450203,12.2,-10.1854648541329));
#291216=CARTESIAN_POINT('Ctrl Pts',(-3.20258898835869,12.2,-10.1821583445245));
#291217=CARTESIAN_POINT('Ctrl Pts',(-3.2005453735671,12.2,-10.178870044893));
#291218=CARTESIAN_POINT('Ctrl Pts',(-3.19852313669383,12.2,-10.175600295589));
#291219=CARTESIAN_POINT('Ctrl Pts',(-3.19650089982057,12.2,-10.1723305462849));
#291220=CARTESIAN_POINT('Ctrl Pts',(-3.1945000396338,12.2,-10.1690793491812));
#291221=CARTESIAN_POINT('Ctrl Pts',(-3.1925205226911,12.2,-10.1658470465439));
#291222=CARTESIAN_POINT('Ctrl Pts',(-3.19054100596417,12.2,-10.1626147442589));
#291223=CARTESIAN_POINT('Ctrl Pts',(-3.18858283094397,12.2,-10.1594013379767));
#291224=CARTESIAN_POINT('Ctrl Pts',(-3.18664595927835,12.2,-10.1562071781844));
#291225=CARTESIAN_POINT('Ctrl Pts',(-3.18470908740161,12.2,-10.153013018044));
#291226=CARTESIAN_POINT('Ctrl Pts',(-3.18279351879397,12.2,-10.1498381057865));
#291227=CARTESIAN_POINT('Ctrl Pts',(-3.18089921601445,12.2,-10.146682795646));
#291228=CARTESIAN_POINT('Ctrl Pts',(-3.17900491323494,12.2,-10.1435274855055));
#291229=CARTESIAN_POINT('Ctrl Pts',(-3.17713187508126,12.2,-10.1403917776799));
#291230=CARTESIAN_POINT('Ctrl Pts',(-3.17528006047338,12.2,-10.1372760341201));
#291231=CARTESIAN_POINT('Ctrl Pts',(-3.1734282458655,12.2,-10.1341602905602));
#291232=CARTESIAN_POINT('Ctrl Pts',(-3.17159765405846,12.2,-10.1310645103801));
#291233=CARTESIAN_POINT('Ctrl Pts',(-3.1697882428768,12.2,-10.1279890619762));
#291234=CARTESIAN_POINT('Ctrl Pts',(-3.16797883169514,12.2,-10.1249136135724));
#291235=CARTESIAN_POINT('Ctrl Pts',(-3.16619060092236,12.2,-10.1218584964608));
#291236=CARTESIAN_POINT('Ctrl Pts',(-3.16442350557403,12.2,-10.1188240822235));
#291237=CARTESIAN_POINT('Ctrl Pts',(-3.1626564102257,12.2,-10.1157896679863));
#291238=CARTESIAN_POINT('Ctrl Pts',(-3.16091045036994,12.2,-10.1127759580541));
#291239=CARTESIAN_POINT('Ctrl Pts',(-3.15918557925095,12.2,-10.1097833297766));
#291240=CARTESIAN_POINT('Ctrl Pts',(-3.15746070813195,12.2,-10.1067907014991));
#291241=CARTESIAN_POINT('Ctrl Pts',(-3.15575692424444,12.2,-10.1038191551666));
#291242=CARTESIAN_POINT('Ctrl Pts',(-3.15407418125833,12.2,-10.100869076));
#291243=CARTESIAN_POINT('Ctrl Pts',(-3.15239143827223,12.2,-10.0979189968333));
#291244=CARTESIAN_POINT('Ctrl Pts',(-3.1507297334565,12.2,-10.0949903842171));
#291245=CARTESIAN_POINT('Ctrl Pts',(-3.14908901803245,12.2,-10.0920836292734));
#291246=CARTESIAN_POINT('Ctrl Pts',(-3.14712015959512,12.2,-10.0885955234677));
#291247=CARTESIAN_POINT('Ctrl Pts',(-3.14518152472779,12.2,-10.0851388913637));
#291248=CARTESIAN_POINT('Ctrl Pts',(-3.14327302137914,12.2,-10.0817144226534));
#291249=CARTESIAN_POINT('Ctrl Pts',(-3.14136451785714,12.2,-10.078289953632));
#291250=CARTESIAN_POINT('Ctrl Pts',(-3.13948614573056,12.2,-10.0748976450063));
#291251=CARTESIAN_POINT('Ctrl Pts',(-3.13763780729854,12.2,-10.0715382029088));
#291252=CARTESIAN_POINT('Ctrl Pts',(-3.13578946903442,12.2,-10.0681787611164));
#291253=CARTESIAN_POINT('Ctrl Pts',(-3.13397116827805,12.2,-10.0648521796912));
#291254=CARTESIAN_POINT('Ctrl Pts',(-3.13218279792766,12.2,-10.0615591800623));
#291255=CARTESIAN_POINT('Ctrl Pts',(-3.13039442757727,12.2,-10.0582661804334));
#291256=CARTESIAN_POINT('Ctrl Pts',(-3.12863599159116,12.2,-10.0550067590768));
#291257=CARTESIAN_POINT('Ctrl Pts',(-3.12690738306934,12.2,-10.0517816486925));
#291258=CARTESIAN_POINT('Ctrl Pts',(-3.12517877454752,12.2,-10.0485565383082));
#291259=CARTESIAN_POINT('Ctrl Pts',(-3.12347999264,12.2,-10.0453657381733));
#291260=CARTESIAN_POINT('Ctrl Pts',(-3.1218109261986,12.2,-10.0422099938689));
#291261=CARTESIAN_POINT('Ctrl Pts',(-3.12014185960561,12.2,-10.0390542492779));
#291262=CARTESIAN_POINT('Ctrl Pts',(-3.11850251067384,12.2,-10.0359335617069));
#291263=CARTESIAN_POINT('Ctrl Pts',(-3.11689275917073,12.2,-10.0328486921236));
#291264=CARTESIAN_POINT('Ctrl Pts',(-3.11528300781385,12.2,-10.0297638228206));
#291265=CARTESIAN_POINT('Ctrl Pts',(-3.11370285677648,12.2,-10.0267147724556));
#291266=CARTESIAN_POINT('Ctrl Pts',(-3.11215218324238,12.2,-10.023702319218));
#291267=CARTESIAN_POINT('Ctrl Pts',(-3.11060150970829,12.2,-10.0206898659804));
#291268=CARTESIAN_POINT('Ctrl Pts',(-3.10908031346876,12.2,-10.0177140097827));
#291269=CARTESIAN_POINT('Ctrl Pts',(-3.10758846793762,12.2,-10.0147755485536));
#291270=CARTESIAN_POINT('Ctrl Pts',(-3.10609662227098,12.2,-10.0118370870575));
#291271=CARTESIAN_POINT('Ctrl Pts',(-3.10463412853219,12.2,-10.0089360179651));
#291272=CARTESIAN_POINT('Ctrl Pts',(-3.10320084995535,12.2,-10.0060731586441));
#291273=CARTESIAN_POINT('Ctrl Pts',(-3.10176757150868,12.2,-10.0032102995831));
#291274=CARTESIAN_POINT('Ctrl Pts',(-3.10036351212365,12.2,-10.0003856478294));
#291275=CARTESIAN_POINT('Ctrl Pts',(-3.09898852950063,12.2,-9.99760003875121));
#291276=CARTESIAN_POINT('Ctrl Pts',(-3.09761354687761,12.2,-9.99481442967302));
#291277=CARTESIAN_POINT('Ctrl Pts',(-3.09626764235601,12.2,-9.992067861541));
#291278=CARTESIAN_POINT('Ctrl Pts',(-3.0949506716519,12.2,-9.98936118855332));
#291279=CARTESIAN_POINT('Ctrl Pts',(-3.09363370082815,12.2,-9.98665451531976));
#291280=CARTESIAN_POINT('Ctrl Pts',(-3.09234566383313,12.2,-9.98398773660126));
#291281=CARTESIAN_POINT('Ctrl Pts',(-3.09108640611993,12.2,-9.98136172549601));
#291282=CARTESIAN_POINT('Ctrl Pts',(-3.08982714852112,12.2,-9.97873571462928));
#291283=CARTESIAN_POINT('Ctrl Pts',(-3.08859667413966,12.2,-9.97615047349918));
#291284=CARTESIAN_POINT('Ctrl Pts',(-3.08739482151667,12.2,-9.97360689400827));
#291285=CARTESIAN_POINT('Ctrl Pts',(-3.08619296889367,12.2,-9.97106331451735));
#291286=CARTESIAN_POINT('Ctrl Pts',(-3.0850197406864,12.2,-9.96856140040726));
#291287=CARTESIAN_POINT('Ctrl Pts',(-3.08387496808582,12.2,-9.96610206470462));
#291288=CARTESIAN_POINT('Ctrl Pts',(-3.08273019538126,12.2,-9.9636427287786));
#291289=CARTESIAN_POINT('Ctrl Pts',(-3.08161388236379,12.2,-9.96122597289263));
#291290=CARTESIAN_POINT('Ctrl Pts',(-3.08052585338975,12.2,-9.95885274001627));
#291291=CARTESIAN_POINT('Ctrl Pts',(-3.07943782451455,12.2,-9.95647950735548));
#291292=CARTESIAN_POINT('Ctrl Pts',(-3.07837808089167,12.2,-9.95414979408447));
#291293=CARTESIAN_POINT('Ctrl Pts',(-3.07734644200787,12.2,-9.95186456774057));
#291294=CARTESIAN_POINT('Ctrl Pts',(-3.07631480312407,12.2,-9.94957934139665));
#291295=CARTESIAN_POINT('Ctrl Pts',(-3.07531126986906,12.2,-9.94733860123363));
#291296=CARTESIAN_POINT('Ctrl Pts',(-3.07433565306996,12.2,-9.94514333889477));
#291297=CARTESIAN_POINT('Ctrl Pts',(-3.07336003618225,12.2,-9.94294807635649));
#291298=CARTESIAN_POINT('Ctrl Pts',(-3.07241233616466,12.2,-9.9407982909155));
#291299=CARTESIAN_POINT('Ctrl Pts',(-3.0714923581164,12.2,-9.93869500047068));
#291300=CARTESIAN_POINT('Ctrl Pts',(-3.07057238015171,12.2,-9.93659171021692));
#291301=CARTESIAN_POINT('Ctrl Pts',(-3.06968012242037,12.2,-9.9345349144572));
#291302=CARTESIAN_POINT('Ctrl Pts',(-3.06881538145299,12.2,-9.93252565944896));
#291303=CARTESIAN_POINT('Ctrl Pts',(-3.06795064048562,12.2,-9.9305164044407));
#291304=CARTESIAN_POINT('Ctrl Pts',(-3.06711341568285,12.2,-9.92855469009569));
#291305=CARTESIAN_POINT('Ctrl Pts',(-3.06630349454421,12.2,-9.92664159307927));
#291306=CARTESIAN_POINT('Ctrl Pts',(-3.06549357340558,12.2,-9.92472849606284));
#291307=CARTESIAN_POINT('Ctrl Pts',(-3.0647109540901,12.2,-9.9228640128102));
#291308=CARTESIAN_POINT('Ctrl Pts',(-3.0639554151157,12.2,-9.92104925495608));
#291309=CARTESIAN_POINT('Ctrl Pts',(-3.06282573262112,12.2,-9.91833582752322));
#291310=CARTESIAN_POINT('Ctrl Pts',(-3.06175657911663,12.2,-9.91573355507463));
#291311=CARTESIAN_POINT('Ctrl Pts',(-3.06074721300006,12.2,-9.91324626500001));
#291312=CARTESIAN_POINT('Ctrl Pts',(-3.06074721300006,15.2,-9.91324626500001));
#291313=CARTESIAN_POINT('Ctrl Pts',(-3.06141904375483,15.2,-9.91490179706191));
#291314=CARTESIAN_POINT('Ctrl Pts',(-3.06211736679865,15.2,-9.91660826837016));
#291315=CARTESIAN_POINT('Ctrl Pts',(-3.06284238742061,15.2,-9.91836455053259));
#291316=CARTESIAN_POINT('Ctrl Pts',(-3.06357090445848,15.2,-9.92012930237536));
#291317=CARTESIAN_POINT('Ctrl Pts',(-3.06432638660912,15.2,-9.92194434089947));
#291318=CARTESIAN_POINT('Ctrl Pts',(-3.06510906085912,15.2,-9.92380854693038));
#291319=CARTESIAN_POINT('Ctrl Pts',(-3.06589173503803,15.2,-9.92567275279196));
#291320=CARTESIAN_POINT('Ctrl Pts',(-3.06670160281363,15.2,-9.92758612253754));
#291321=CARTESIAN_POINT('Ctrl Pts',(-3.0675388807832,15.2,-9.92954756746627));
#291322=CARTESIAN_POINT('Ctrl Pts',(-3.06837615875278,15.2,-9.931509012395));
#291323=CARTESIAN_POINT('Ctrl Pts',(-3.0692408475782,15.2,-9.93351853336747));
#291324=CARTESIAN_POINT('Ctrl Pts',(-3.07013315567209,15.2,-9.93557506680944));
#291325=CARTESIAN_POINT('Ctrl Pts',(-3.07102546384703,15.2,-9.9376316004382));
#291326=CARTESIAN_POINT('Ctrl Pts',(-3.07194539223311,15.2,-9.93973515056398));
#291327=CARTESIAN_POINT('Ctrl Pts',(-3.07289314111998,15.2,-9.94188468101757));
#291328=CARTESIAN_POINT('Ctrl Pts',(-3.07384088992077,15.2,-9.94403421127591));
#291329=CARTESIAN_POINT('Ctrl Pts',(-3.07481645821564,15.2,-9.94622972489708));
#291330=CARTESIAN_POINT('Ctrl Pts',(-3.07582003901713,15.2,-9.94847021724262));
#291331=CARTESIAN_POINT('Ctrl Pts',(-3.07682361981862,15.2,-9.95071070958816));
#291332=CARTESIAN_POINT('Ctrl Pts',(-3.07785521373208,15.2,-9.95299617995969));
#291333=CARTESIAN_POINT('Ctrl Pts',(-3.07891500169237,15.2,-9.95532565137317));
#291334=CARTESIAN_POINT('Ctrl Pts',(-3.07997478974891,15.2,-9.95765512299823));
#291335=CARTESIAN_POINT('Ctrl Pts',(-3.08106277567559,15.2,-9.96002859490372));
#291336=CARTESIAN_POINT('Ctrl Pts',(-3.08217913257169,15.2,-9.96244511478835));
#291337=CARTESIAN_POINT('Ctrl Pts',(-3.0832954893664,15.2,-9.96486163445348));
#291338=CARTESIAN_POINT('Ctrl Pts',(-3.08444021890545,15.2,-9.9673212018672));
#291339=CARTESIAN_POINT('Ctrl Pts',(-3.08561348953074,15.2,-9.96982288836146));
#291340=CARTESIAN_POINT('Ctrl Pts',(-3.08678676015602,15.2,-9.97232457485573));
#291341=CARTESIAN_POINT('Ctrl Pts',(-3.08798857222068,15.2,-9.97486837946327));
#291342=CARTESIAN_POINT('Ctrl Pts',(-3.08921908692473,15.2,-9.97745339811756));
#291343=CARTESIAN_POINT('Ctrl Pts',(-3.09044960162878,15.2,-9.98003841677186));
#291344=CARTESIAN_POINT('Ctrl Pts',(-3.09170882050837,15.2,-9.98266464830892));
#291345=CARTESIAN_POINT('Ctrl Pts',(-3.09299689612628,15.2,-9.9853312082093));
#291346=CARTESIAN_POINT('Ctrl Pts',(-3.09428497186118,15.2,-9.98799776835189));
#291347=CARTESIAN_POINT('Ctrl Pts',(-3.09560190589886,15.2,-9.99070465833173));
#291348=CARTESIAN_POINT('Ctrl Pts',(-3.09694784580681,15.2,-9.99345101264978));
#291349=CARTESIAN_POINT('Ctrl Pts',(-3.0982937855925,15.2,-9.99619736671838));
#291350=CARTESIAN_POINT('Ctrl Pts',(-3.0996687338774,15.2,-9.99898318664687));
#291351=CARTESIAN_POINT('Ctrl Pts',(-3.10107282849937,15.2,-10.0018076304737));
#291352=CARTESIAN_POINT('Ctrl Pts',(-3.10247692312134,15.2,-10.0046320743005));
#291353=CARTESIAN_POINT('Ctrl Pts',(-3.1039101674124,15.2,-10.0074951390084));
#291354=CARTESIAN_POINT('Ctrl Pts',(-3.10537269585726,15.2,-10.0103960032338));
#291355=CARTESIAN_POINT('Ctrl Pts',(-3.10683522443497,15.2,-10.0132968677226));
#291356=CARTESIAN_POINT('Ctrl Pts',(-3.10832703761551,15.2,-10.0162355300235));
#291357=CARTESIAN_POINT('Ctrl Pts',(-3.10984826536637,15.2,-10.0192111874373));
#291358=CARTESIAN_POINT('Ctrl Pts',(-3.11136949297905,15.2,-10.0221868445808));
#291359=CARTESIAN_POINT('Ctrl Pts',(-3.11292013460792,15.2,-10.0251994943539));
#291360=CARTESIAN_POINT('Ctrl Pts',(-3.11450031697429,15.2,-10.0282483505069));
#291361=CARTESIAN_POINT('Ctrl Pts',(-3.11608049934065,15.2,-10.0312972066599));
#291362=CARTESIAN_POINT('Ctrl Pts',(-3.11769022027456,15.2,-10.034382268134));
#291363=CARTESIAN_POINT('Ctrl Pts',(-3.11932959879632,15.2,-10.0375027646015));
#291364=CARTESIAN_POINT('Ctrl Pts',(-3.12096897746699,15.2,-10.0406232613525));
#291365=CARTESIAN_POINT('Ctrl Pts',(-3.1226380161269,15.2,-10.043779194015));
#291366=CARTESIAN_POINT('Ctrl Pts',(-3.12433682588942,15.2,-10.046969808767));
#291367=CARTESIAN_POINT('Ctrl Pts',(-3.12603563549762,15.2,-10.0501604232292));
#291368=CARTESIAN_POINT('Ctrl Pts',(-3.12776421756389,15.2,-10.0533857175767));
#291369=CARTESIAN_POINT('Ctrl Pts',(-3.12952268,15.2,-10.0566449560416));
#291370=CARTESIAN_POINT('Ctrl Pts',(-3.13128114243611,15.2,-10.0599041945065));
#291371=CARTESIAN_POINT('Ctrl Pts',(-3.13306948755115,15.2,-10.0631973737432));
#291372=CARTESIAN_POINT('Ctrl Pts',(-3.13488781507418,15.2,-10.0665237753699));
#291373=CARTESIAN_POINT('Ctrl Pts',(-3.13670614276237,15.2,-10.0698501772988));
#291374=CARTESIAN_POINT('Ctrl Pts',(-3.13855445617533,15.2,-10.0732097970826));
#291375=CARTESIAN_POINT('Ctrl Pts',(-3.14043285269643,15.2,-10.076601929103));
#291376=CARTESIAN_POINT('Ctrl Pts',(-3.1423112490469,15.2,-10.0799940608154));
#291377=CARTESIAN_POINT('Ctrl Pts',(-3.14421972882912,15.2,-10.0834187031697));
#291378=CARTESIAN_POINT('Ctrl Pts',(-3.14615838626755,15.2,-10.0868751619765));
#291379=CARTESIAN_POINT('Ctrl Pts',(-3.14809704370598,15.2,-10.0903316207834));
#291380=CARTESIAN_POINT('Ctrl Pts',(-3.15006588000679,15.2,-10.0938198977291));
#291381=CARTESIAN_POINT('Ctrl Pts',(-3.15206498434951,15.2,-10.0973393095166));
#291382=CARTESIAN_POINT('Ctrl Pts',(-3.15373090469565,15.2,-10.1002721527794));
#291383=CARTESIAN_POINT('Ctrl Pts',(-3.1554178442173,15.2,-10.1032266189899));
#291384=CARTESIAN_POINT('Ctrl Pts',(-3.15712585289676,15.2,-10.1062023198221));
#291385=CARTESIAN_POINT('Ctrl Pts',(-3.15883386157622,15.2,-10.1091780206544));
#291386=CARTESIAN_POINT('Ctrl Pts',(-3.16056293785227,15.2,-10.1121749566236));
#291387=CARTESIAN_POINT('Ctrl Pts',(-3.16231313299905,15.2,-10.1151927467066));
#291388=CARTESIAN_POINT('Ctrl Pts',(-3.16406332814582,15.2,-10.1182105367897));
#291389=CARTESIAN_POINT('Ctrl Pts',(-3.16583463929444,15.2,-10.1212491832777));
#291390=CARTESIAN_POINT('Ctrl Pts',(-3.167627112975,15.2,-10.12430830675));
#291391=CARTESIAN_POINT('Ctrl Pts',(-3.16941958665556,15.2,-10.1273674302222));
#291392=CARTESIAN_POINT('Ctrl Pts',(-3.17123322385372,15.2,-10.1304470342486));
#291393=CARTESIAN_POINT('Ctrl Pts',(-3.17306806670934,15.2,-10.133546747735));
#291394=CARTESIAN_POINT('Ctrl Pts',(-3.17490290956495,15.2,-10.1366464612213));
#291395=CARTESIAN_POINT('Ctrl Pts',(-3.17675895911068,15.2,-10.1397662843544));
#291396=CARTESIAN_POINT('Ctrl Pts',(-3.17863625688957,15.2,-10.1429058551887));
#291397=CARTESIAN_POINT('Ctrl Pts',(-3.18051355466847,15.2,-10.1460454260231));
#291398=CARTESIAN_POINT('Ctrl Pts',(-3.18241210088013,15.2,-10.1492047423347));
#291399=CARTESIAN_POINT('Ctrl Pts',(-3.18433193615902,15.2,-10.1523834474746));
#291400=CARTESIAN_POINT('Ctrl Pts',(-3.18625177143792,15.2,-10.1555621526145));
#291401=CARTESIAN_POINT('Ctrl Pts',(-3.18819289448948,15.2,-10.1587602472948));
#291402=CARTESIAN_POINT('Ctrl Pts',(-3.19015534472789,15.2,-10.1619773768318));
#291403=CARTESIAN_POINT('Ctrl Pts',(-3.1921177949663,15.2,-10.1651945063689));
#291404=CARTESIAN_POINT('Ctrl Pts',(-3.19410157103831,15.2,-10.1684306717575));
#291405=CARTESIAN_POINT('Ctrl Pts',(-3.19610671201228,15.2,-10.1716855244674));
#291406=CARTESIAN_POINT('Ctrl Pts',(-3.19811185298625,15.2,-10.1749403771773));
#291407=CARTESIAN_POINT('Ctrl Pts',(-3.2001383563939,15.2,-10.1782139192346));
#291408=CARTESIAN_POINT('Ctrl Pts',(-3.20218625903454,15.2,-10.1815058061805));
#291409=CARTESIAN_POINT('Ctrl Pts',(-3.20423416145195,15.2,-10.1847976927677));
#291410=CARTESIAN_POINT('Ctrl Pts',(-3.20630346059506,15.2,-10.1881079253678));
#291411=CARTESIAN_POINT('Ctrl Pts',(-3.20839419293487,15.2,-10.1914361652813));
#291412=CARTESIAN_POINT('Ctrl Pts',(-3.21048492550257,15.2,-10.1947644055576));
#291413=CARTESIAN_POINT('Ctrl Pts',(-3.21259708890046,15.2,-10.1981106537447));
#291414=CARTESIAN_POINT('Ctrl Pts',(-3.21473071570426,15.2,-10.201474577285));
#291415=CARTESIAN_POINT('Ctrl Pts',(-3.21686434250806,15.2,-10.2048385008252));
#291416=CARTESIAN_POINT('Ctrl Pts',(-3.21901943374485,15.2,-10.2082200984179));
#291417=CARTESIAN_POINT('Ctrl Pts',(-3.22119601721531,15.2,-10.2116190437637));
#291418=CARTESIAN_POINT('Ctrl Pts',(-3.22337260068577,15.2,-10.2150179891095));
#291419=CARTESIAN_POINT('Ctrl Pts',(-3.22557067655524,15.2,-10.21843428127));
#291420=CARTESIAN_POINT('Ctrl Pts',(-3.22779027444242,15.2,-10.2218675960931));
#291421=CARTESIAN_POINT('Ctrl Pts',(-3.2300098723296,15.2,-10.2253009109163));
#291422=CARTESIAN_POINT('Ctrl Pts',(-3.23225099273662,15.2,-10.228751249002));
#291423=CARTESIAN_POINT('Ctrl Pts',(-3.23451366127715,15.2,-10.232218291015));
#291424=CARTESIAN_POINT('Ctrl Pts',(-3.23677632981768,15.2,-10.235685333028));
#291425=CARTESIAN_POINT('Ctrl Pts',(-3.23906054660602,15.2,-10.2391690781609));
#291426=CARTESIAN_POINT('Ctrl Pts',(-3.241366338341,15.2,-10.2426692128128));
#291427=CARTESIAN_POINT('Ctrl Pts',(-3.24321097182952,15.2,-10.245469320687));
#291428=CARTESIAN_POINT('Ctrl Pts',(-3.24506941114164,15.2,-10.2482799171166));
#291429=CARTESIAN_POINT('Ctrl Pts',(-3.24694167200509,15.2,-10.2511008431344));
#291430=CARTESIAN_POINT('Ctrl Pts',(-3.24881393261344,15.2,-10.2539217687678));
#291431=CARTESIAN_POINT('Ctrl Pts',(-3.25070001228992,15.2,-10.2567530244174));
#291432=CARTESIAN_POINT('Ctrl Pts',(-3.25259992357815,15.2,-10.2595944518511));
#291433=CARTESIAN_POINT('Ctrl Pts',(-3.25449983512524,15.2,-10.262435879672));
#291434=CARTESIAN_POINT('Ctrl Pts',(-3.25641357846286,15.2,-10.2652874788607));
#291435=CARTESIAN_POINT('Ctrl Pts',(-3.25834116412438,15.2,-10.268149094684));
#291436=CARTESIAN_POINT('Ctrl Pts',(-3.26026874952326,15.2,-10.2710107101174));
#291437=CARTESIAN_POINT('Ctrl Pts',(-3.26221017892137,15.2,-10.2738823411271));
#291438=CARTESIAN_POINT('Ctrl Pts',(-3.26416546102469,15.2,-10.2767638340902));
#291439=CARTESIAN_POINT('Ctrl Pts',(-3.26660956385364,15.2,-10.2803657005886));
#291440=CARTESIAN_POINT('Ctrl Pts',(-3.26907531174968,15.2,-10.283982975941));
#291441=CARTESIAN_POINT('Ctrl Pts',(-3.27156272605412,15.2,-10.2876153614958));
#291442=CARTESIAN_POINT('Ctrl Pts',(-3.27355265760613,15.2,-10.290521270098));
#291443=CARTESIAN_POINT('Ctrl Pts',(-3.27555645564032,15.2,-10.2934368496847));
#291444=CARTESIAN_POINT('Ctrl Pts',(-3.27757412914008,15.2,-10.2963619489559));
#291445=CARTESIAN_POINT('Ctrl Pts',(-3.27959180236493,15.2,-10.2992870478285));
#291446=CARTESIAN_POINT('Ctrl Pts',(-3.28162335029173,15.2,-10.3022216665117));
#291447=CARTESIAN_POINT('Ctrl Pts',(-3.28366878300327,15.2,-10.3051656563062));
#291448=CARTESIAN_POINT('Ctrl Pts',(-3.28571421599351,15.2,-10.3081096465018));
#291449=CARTESIAN_POINT('Ctrl Pts',(-3.28777353306405,15.2,-10.311063007883));
#291450=CARTESIAN_POINT('Ctrl Pts',(-3.28984674267795,15.2,-10.3140255917673));
#291451=CARTESIAN_POINT('Ctrl Pts',(-3.29191995200937,15.2,-10.3169881752479));
#291452=CARTESIAN_POINT('Ctrl Pts',(-3.29400705495745,15.2,-10.3199599823489));
#291453=CARTESIAN_POINT('Ctrl Pts',(-3.29610805867316,15.2,-10.3229408652709));
#291454=CARTESIAN_POINT('Ctrl Pts',(-3.29820906267513,15.2,-10.3259217485991));
#291455=CARTESIAN_POINT('Ctrl Pts',(-3.30032396540905,15.2,-10.3289117075305));
#291456=CARTESIAN_POINT('Ctrl Pts',(-3.30245277753479,15.2,-10.3319105994854));
#291457=CARTESIAN_POINT('Ctrl Pts',(-3.30458158937047,15.2,-10.3349094910316));
#291458=CARTESIAN_POINT('Ctrl Pts',(-3.30672430854734,15.2,-10.3379173133626));
#291459=CARTESIAN_POINT('Ctrl Pts',(-3.3088809431474,15.2,-10.3409339242818));
#291460=CARTESIAN_POINT('Ctrl Pts',(-3.3110375780413,15.2,-10.343950535612));
#291461=CARTESIAN_POINT('Ctrl Pts',(-3.31320812668095,15.2,-10.3469759351763));
#291462=CARTESIAN_POINT('Ctrl Pts',(-3.31539259746666,15.2,-10.3500099805083));
#291463=CARTESIAN_POINT('Ctrl Pts',(-3.31757706825238,15.2,-10.3530440258403));
#291464=CARTESIAN_POINT('Ctrl Pts',(-3.31977546047584,15.2,-10.3560867182011));
#291465=CARTESIAN_POINT('Ctrl Pts',(-3.32198777932005,15.2,-10.3591379144239));
#291466=CARTESIAN_POINT('Ctrl Pts',(-3.32420009786284,15.2,-10.3621891102308));
#291467=CARTESIAN_POINT('Ctrl Pts',(-3.32642634335759,15.2,-10.365248813332));
#291468=CARTESIAN_POINT('Ctrl Pts',(-3.32866652124014,15.2,-10.3683168810396));
#291469=CARTESIAN_POINT('Ctrl Pts',(-3.33090669942791,15.2,-10.3713849491651));
#291470=CARTESIAN_POINT('Ctrl Pts',(-3.33316081086247,15.2,-10.3744613824381));
#291471=CARTESIAN_POINT('Ctrl Pts',(-3.33542885965417,15.2,-10.377546044996));
#291472=CARTESIAN_POINT('Ctrl Pts',(-3.33769690813684,15.2,-10.3806307071335));
#291473=CARTESIAN_POINT('Ctrl Pts',(-3.33997889333993,15.2,-10.3837235966645));
#291474=CARTESIAN_POINT('Ctrl Pts',(-3.34227482059578,15.2,-10.3868245770216));
#291475=CARTESIAN_POINT('Ctrl Pts',(-3.3451447299002,15.2,-10.3907008027848));
#291476=CARTESIAN_POINT('Ctrl Pts',(-3.34803642425746,15.2,-10.3945896701079));
#291477=CARTESIAN_POINT('Ctrl Pts',(-3.35094991017342,15.2,-10.3984909165145));
#291478=CARTESIAN_POINT('Ctrl Pts',(-3.35328069903322,15.2,-10.4016119138099));
#291479=CARTESIAN_POINT('Ctrl Pts',(-3.35562543579456,15.2,-10.4047408317383));
#291480=CARTESIAN_POINT('Ctrl Pts',(-3.35798412136899,15.2,-10.4078775385212));
#291481=CARTESIAN_POINT('Ctrl Pts',(-3.36034280662204,15.2,-10.4110142448766));
#291482=CARTESIAN_POINT('Ctrl Pts',(-3.36271544412326,15.2,-10.4141587378617));
#291483=CARTESIAN_POINT('Ctrl Pts',(-3.36510203403836,15.2,-10.4173108874924));
#291484=CARTESIAN_POINT('Ctrl Pts',(-3.36748862427863,15.2,-10.4204630375525));
#291485=CARTESIAN_POINT('Ctrl Pts',(-3.36988916764422,15.2,-10.4236228418392));
#291486=CARTESIAN_POINT('Ctrl Pts',(-3.3723036678421,15.2,-10.4267901707263));
#291487=CARTESIAN_POINT('Ctrl Pts',(-3.37471816771101,15.2,-10.4299574991818));
#291488=CARTESIAN_POINT('Ctrl Pts',(-3.37714662323717,15.2,-10.43313235052));
#291489=CARTESIAN_POINT('Ctrl Pts',(-3.37958903709213,15.2,-10.4363145949816));
#291490=CARTESIAN_POINT('Ctrl Pts',(-3.38203145127987,15.2,-10.4394968398767));
#291491=CARTESIAN_POINT('Ctrl Pts',(-3.38448782419709,15.2,-10.44268647887));
#291492=CARTESIAN_POINT('Ctrl Pts',(-3.38695815694375,15.2,-10.4458833817114));
#291493=CARTESIAN_POINT('Ctrl Pts',(-3.38942848935382,15.2,-10.4490802841172));
#291494=CARTESIAN_POINT('Ctrl Pts',(-3.39191278094997,15.2,-10.4522844503465));
#291495=CARTESIAN_POINT('Ctrl Pts',(-3.39441103479988,15.2,-10.4554957532499));
#291496=CARTESIAN_POINT('Ctrl Pts',(-3.39690928899017,15.2,-10.4587070565909));
#291497=CARTESIAN_POINT('Ctrl Pts',(-3.39942150561919,15.2,-10.4619254946006));
#291498=CARTESIAN_POINT('Ctrl Pts',(-3.40194768376839,15.2,-10.4651509422355));
#291499=CARTESIAN_POINT('Ctrl Pts',(-3.4044738615734,15.2,-10.468376389431));
#291500=CARTESIAN_POINT('Ctrl Pts',(-3.40701400162874,15.2,-10.4716088474942));
#291501=CARTESIAN_POINT('Ctrl Pts',(-3.40956810480741,15.2,-10.4748481867287));
#291502=CARTESIAN_POINT('Ctrl Pts',(-3.41212220833408,15.2,-10.4780875264045));
#291503=CARTESIAN_POINT('Ctrl Pts',(-3.41469027602872,15.2,-10.4813337501227));
#291504=CARTESIAN_POINT('Ctrl Pts',(-3.41727230555833,15.2,-10.4845867329667));
#291505=CARTESIAN_POINT('Ctrl Pts',(-3.42049984229445,15.2,-10.4886529613));
#291506=CARTESIAN_POINT('Ctrl Pts',(-3.42374919592019,15.2,-10.4927297492725));
#291507=CARTESIAN_POINT('Ctrl Pts',(-3.42702036822679,15.2,-10.4968168560272));
#291508=CARTESIAN_POINT('Ctrl Pts',(-3.42963730585813,15.2,-10.5000865411637));
#291509=CARTESIAN_POINT('Ctrl Pts',(-3.43226820610188,15.2,-10.5033628310851));
#291510=CARTESIAN_POINT('Ctrl Pts',(-3.43491306855091,15.2,-10.5066456022049));
#291511=CARTESIAN_POINT('Ctrl Pts',(-3.4375579313603,15.2,-10.5099283737721));
#291512=CARTESIAN_POINT('Ctrl Pts',(-3.44021675605433,15.2,-10.5132176282981));
#291513=CARTESIAN_POINT('Ctrl Pts',(-3.4428895422,15.2,-10.5165132420333));
#291514=CARTESIAN_POINT('Ctrl Pts',(-3.44556232834566,15.2,-10.5198088557685));
#291515=CARTESIAN_POINT('Ctrl Pts',(-3.44824907580407,15.2,-10.5231108306461));
#291516=CARTESIAN_POINT('Ctrl Pts',(-3.45094978317491,15.2,-10.5264190455492));
#291517=CARTESIAN_POINT('Ctrl Pts',(-3.45365049017777,15.2,-10.5297272600016));
#291518=CARTESIAN_POINT('Ctrl Pts',(-3.45636515587275,15.2,-10.5330417151263));
#291519=CARTESIAN_POINT('Ctrl Pts',(-3.45909378027315,15.2,-10.5363622909811));
#291520=CARTESIAN_POINT('Ctrl Pts',(-3.46250456105248,15.2,-10.5405130111388));
#291521=CARTESIAN_POINT('Ctrl Pts',(-3.46593715146666,15.2,-10.5446732956555));
#291522=CARTESIAN_POINT('Ctrl Pts',(-3.46939154646666,15.2,-10.548842913225));
#291523=CARTESIAN_POINT('Ctrl Pts',(-3.47215506261727,15.2,-10.5521786074623));
#291524=CARTESIAN_POINT('Ctrl Pts',(-3.47493253425562,15.2,-10.5555202747032));
#291525=CARTESIAN_POINT('Ctrl Pts',(-3.47772395846474,15.2,-10.5588677983306));
#291526=CARTESIAN_POINT('Ctrl Pts',(-3.48051538229352,15.2,-10.562215321502));
#291527=CARTESIAN_POINT('Ctrl Pts',(-3.48332075898246,15.2,-10.5655687009987));
#291528=CARTESIAN_POINT('Ctrl Pts',(-3.48614008476475,15.2,-10.5689278202394));
#291529=CARTESIAN_POINT('Ctrl Pts',(-3.48895941093117,15.2,-10.5722869399377));
#291530=CARTESIAN_POINT('Ctrl Pts',(-3.49179268780338,15.2,-10.5756518002418));
#291531=CARTESIAN_POINT('Ctrl Pts',(-3.49463991118219,15.2,-10.5790222852594));
#291532=CARTESIAN_POINT('Ctrl Pts',(-3.49748713417307,15.2,-10.5823927698178));
#291533=CARTESIAN_POINT('Ctrl Pts',(-3.50034830246771,15.2,-10.585768880131));
#291534=CARTESIAN_POINT('Ctrl Pts',(-3.50322341423176,15.2,-10.5891504994653));
#291535=CARTESIAN_POINT('Ctrl Pts',(-3.50537974815274,15.2,-10.5916867140812));
#291536=CARTESIAN_POINT('Ctrl Pts',(-3.50754392576783,15.2,-10.5942260293405));
#291537=CARTESIAN_POINT('Ctrl Pts',(-3.50971594333818,15.2,-10.5967683964581));
#291538=CARTESIAN_POINT('Ctrl Pts',(-3.51333597275363,15.2,-10.6010056751415));
#291539=CARTESIAN_POINT('Ctrl Pts',(-3.5169777843839,15.2,-10.6052514312112));
#291540=CARTESIAN_POINT('Ctrl Pts',(-3.52064136924387,15.2,-10.6095054439885));
#291541=CARTESIAN_POINT('Ctrl Pts',(-3.52283952007998,15.2,-10.6120578515622));
#291542=CARTESIAN_POINT('Ctrl Pts',(-3.5250455086489,15.2,-10.6146132324356));
#291543=CARTESIAN_POINT('Ctrl Pts',(-3.52725933352573,15.2,-10.617171538509));
#291544=CARTESIAN_POINT('Ctrl Pts',(-3.52947315880474,15.2,-10.619729845047));
#291545=CARTESIAN_POINT('Ctrl Pts',(-3.53169482021096,15.2,-10.6222910772359));
#291546=CARTESIAN_POINT('Ctrl Pts',(-3.5339243164527,15.2,-10.6248551883173));
#291547=CARTESIAN_POINT('Ctrl Pts',(-3.53764014257722,15.2,-10.6291287056994));
#291548=CARTESIAN_POINT('Ctrl Pts',(-3.54137773184761,15.2,-10.6334102200849));
#291549=CARTESIAN_POINT('Ctrl Pts',(-3.54513707074162,15.2,-10.6376995164223));
#291550=CARTESIAN_POINT('Ctrl Pts',(-3.5473926746517,15.2,-10.6402730948793));
#291551=CARTESIAN_POINT('Ctrl Pts',(-3.54965611064733,15.2,-10.6428494740537));
#291552=CARTESIAN_POINT('Ctrl Pts',(-3.55192737402014,15.2,-10.6454286085956));
#291553=CARTESIAN_POINT('Ctrl Pts',(-3.55495572449621,15.2,-10.6488674538705));
#291554=CARTESIAN_POINT('Ctrl Pts',(-3.55799799235659,15.2,-10.6523111984448));
#291555=CARTESIAN_POINT('Ctrl Pts',(-3.56105417255029,15.2,-10.6557597317181));
#291556=CARTESIAN_POINT('Ctrl Pts',(-3.56334630779966,15.2,-10.6583461317906));
#291557=CARTESIAN_POINT('Ctrl Pts',(-3.56564626713971,15.2,-10.6609352257969));
#291558=CARTESIAN_POINT('Ctrl Pts',(-3.56795405008691,15.2,-10.6635269689986));
#291559=CARTESIAN_POINT('Ctrl Pts',(-3.57026183303412,15.2,-10.6661187122003));
#291560=CARTESIAN_POINT('Ctrl Pts',(-3.57257743817898,15.2,-10.6687131048619));
#291561=CARTESIAN_POINT('Ctrl Pts',(-3.5749008639685,15.2,-10.6713100999755));
#291562=CARTESIAN_POINT('Ctrl Pts',(-3.57722429018012,15.2,-10.6739070955609));
#291563=CARTESIAN_POINT('Ctrl Pts',(-3.57955553533558,15.2,-10.6765066947887));
#291564=CARTESIAN_POINT('Ctrl Pts',(-3.58189459950992,15.2,-10.6791088528339));
#291565=CARTESIAN_POINT('Ctrl Pts',(-3.58423366325934,15.2,-10.6817110104064));
#291566=CARTESIAN_POINT('Ctrl Pts',(-3.586580543325,15.2,-10.6843157259287));
#291567=CARTESIAN_POINT('Ctrl Pts',(-3.58893523819846,15.2,-10.6869229555009));
#291568=CARTESIAN_POINT('Ctrl Pts',(-3.59128993307192,15.2,-10.689530185073));
#291569=CARTESIAN_POINT('Ctrl Pts',(-3.59365244339414,15.2,-10.6921399284354));
#291570=CARTESIAN_POINT('Ctrl Pts',(-3.59602276477716,15.2,-10.694752141519));
#291571=CARTESIAN_POINT('Ctrl Pts',(-3.59839308616017,15.2,-10.6973643546027));
#291572=CARTESIAN_POINT('Ctrl Pts',(-3.60077121980706,15.2,-10.6999790372975));
#291573=CARTESIAN_POINT('Ctrl Pts',(-3.60315716127284,15.2,-10.7025961444643));
#291574=CARTESIAN_POINT('Ctrl Pts',(-3.60554310273861,15.2,-10.7052132516311));
#291575=CARTESIAN_POINT('Ctrl Pts',(-3.60793685412629,15.2,-10.7078327841097));
#291576=CARTESIAN_POINT('Ctrl Pts',(-3.61033841049669,15.2,-10.7104546981392));
#291577=CARTESIAN_POINT('Ctrl Pts',(-3.6127399668671,15.2,-10.7130766121688));
#291578=CARTESIAN_POINT('Ctrl Pts',(-3.61514932837862,15.2,-10.7157009066398));
#291579=CARTESIAN_POINT('Ctrl Pts',(-3.61756649274807,15.2,-10.7183275391691));
#291580=CARTESIAN_POINT('Ctrl Pts',(-3.61998365755664,15.2,-10.7209541721755));
#291581=CARTESIAN_POINT('Ctrl Pts',(-3.62240862492572,15.2,-10.7235831425075));
#291582=CARTESIAN_POINT('Ctrl Pts',(-3.62484139173869,15.2,-10.7262144070569));
#291583=CARTESIAN_POINT('Ctrl Pts',(-3.62808508008606,15.2,-10.7297227589928));
#291584=CARTESIAN_POINT('Ctrl Pts',(-3.63134263357882,15.2,-10.7332351875448));
#291585=CARTESIAN_POINT('Ctrl Pts',(-3.6346140445327,15.2,-10.7367515934792));
#291586=CARTESIAN_POINT('Ctrl Pts',(-3.63706760285953,15.2,-10.7393888980499));
#291587=CARTESIAN_POINT('Ctrl Pts',(-3.6395289557563,15.2,-10.7420284399032));
#291588=CARTESIAN_POINT('Ctrl Pts',(-3.64199810024736,15.2,-10.7446701737722));
#291589=CARTESIAN_POINT('Ctrl Pts',(-3.64446724473843,15.2,-10.7473119076413));
#291590=CARTESIAN_POINT('Ctrl Pts',(-3.64694418066634,15.2,-10.7499558357196));
#291591=CARTESIAN_POINT('Ctrl Pts',(-3.64942890445001,15.2,-10.7526019139148));
#291592=CARTESIAN_POINT('Ctrl Pts',(-3.65191362868507,15.2,-10.7552479925908));
#291593=CARTESIAN_POINT('Ctrl Pts',(-3.65440613983063,15.2,-10.7578962227423));
#291594=CARTESIAN_POINT('Ctrl Pts',(-3.65690643602841,15.2,-10.7605465608361));
#291595=CARTESIAN_POINT('Ctrl Pts',(-3.65940673177196,15.2,-10.7631968984484));
#291596=CARTESIAN_POINT('Ctrl Pts',(-3.66191481129844,15.2,-10.765849343669));
#291597=CARTESIAN_POINT('Ctrl Pts',(-3.66443067158269,15.2,-10.768503855781));
#291598=CARTESIAN_POINT('Ctrl Pts',(-3.66694653186695,15.2,-10.7711583678931));
#291599=CARTESIAN_POINT('Ctrl Pts',(-3.66947017189941,15.2,-10.7738149468703));
#291600=CARTESIAN_POINT('Ctrl Pts',(-3.67200158923564,15.2,-10.7764735490357));
#291601=CARTESIAN_POINT('Ctrl Pts',(-3.67453300657186,15.2,-10.7791321512012));
#291602=CARTESIAN_POINT('Ctrl Pts',(-3.67707220089537,15.2,-10.7817927773989));
#291603=CARTESIAN_POINT('Ctrl Pts',(-3.67961916727269,15.2,-10.7844553864809));
#291604=CARTESIAN_POINT('Ctrl Pts',(-3.68216613365002,15.2,-10.7871179955629));
#291605=CARTESIAN_POINT('Ctrl Pts',(-3.68472087314793,15.2,-10.7897825860231));
#291606=CARTESIAN_POINT('Ctrl Pts',(-3.68728338147082,15.2,-10.7924491172177));
#291607=CARTESIAN_POINT('Ctrl Pts',(-3.68984588979371,15.2,-10.7951156484123));
#291608=CARTESIAN_POINT('Ctrl Pts',(-3.69241616663272,15.2,-10.7977841214985));
#291609=CARTESIAN_POINT('Ctrl Pts',(-3.69499420845467,15.2,-10.8004544941512));
#291610=CARTESIAN_POINT('Ctrl Pts',(-3.69843159786283,15.2,-10.8040149913449));
#291611=CARTESIAN_POINT('Ctrl Pts',(-3.70188279176162,15.2,-10.8075788666085));
#291612=CARTESIAN_POINT('Ctrl Pts',(-3.70534777924403,15.2,-10.8111460204858));
#291613=CARTESIAN_POINT('Ctrl Pts',(-3.70794651961979,15.2,-10.8138213856507));
#291614=CARTESIAN_POINT('Ctrl Pts',(-3.71055301989745,15.2,-10.8164985952827));
#291615=CARTESIAN_POINT('Ctrl Pts',(-3.71316727427263,15.2,-10.8191776064892));
#291616=CARTESIAN_POINT('Ctrl Pts',(-3.71578152864781,15.2,-10.8218566176957));
#291617=CARTESIAN_POINT('Ctrl Pts',(-3.71840353845971,15.2,-10.8245374306719));
#291618=CARTESIAN_POINT('Ctrl Pts',(-3.72103329923849,15.2,-10.8272200094076));
#291619=CARTESIAN_POINT('Ctrl Pts',(-3.72366306001727,15.2,-10.8299025881434));
#291620=CARTESIAN_POINT('Ctrl Pts',(-3.72630057117052,15.2,-10.8325869338123));
#291621=CARTESIAN_POINT('Ctrl Pts',(-3.72894582899001,15.2,-10.8352730049228));
#291622=CARTESIAN_POINT('Ctrl Pts',(-3.73159108729005,15.2,-10.8379590765212));
#291623=CARTESIAN_POINT('Ctrl Pts',(-3.73424409222563,15.2,-10.8406468748952));
#291624=CARTESIAN_POINT('Ctrl Pts',(-3.73690483861338,15.2,-10.8433363508696));
#291625=CARTESIAN_POINT('Ctrl Pts',(-3.73956558451777,15.2,-10.8460258263555));
#291626=CARTESIAN_POINT('Ctrl Pts',(-3.7422340726805,15.2,-10.8487169781341));
#291627=CARTESIAN_POINT('Ctrl Pts',(-3.74491029621786,15.2,-10.8514097635877));
#291628=CARTESIAN_POINT('Ctrl Pts',(-3.74758651975522,15.2,-10.8541025490412));
#291629=CARTESIAN_POINT('Ctrl Pts',(-3.75027047927055,15.2,-10.8567969667966));
#291630=CARTESIAN_POINT('Ctrl Pts',(-3.75296217351105,15.2,-10.8594930000052));
#291631=CARTESIAN_POINT('Ctrl Pts',(-3.75565386775154,15.2,-10.8621890332137));
#291632=CARTESIAN_POINT('Ctrl Pts',(-3.75835329800824,15.2,-10.8648866810023));
#291633=CARTESIAN_POINT('Ctrl Pts',(-3.76106045600006,15.2,-10.867585944));
#291634=CARTESIAN_POINT('Ctrl Pts',(-4.04260911700006,15.2,-9.55499537100001));
#291635=CARTESIAN_POINT('Ctrl Pts',(-4.04260911700006,11.6,-9.55499537100001));
#291636=CARTESIAN_POINT('Ctrl Pts',(-4.04266300400006,15.2,-9.55516119200002));
#291637=CARTESIAN_POINT('Ctrl Pts',(-4.04266300400006,11.6,-9.55516119200002));
#291638=CARTESIAN_POINT('Ctrl Pts',(-4.04277258000006,15.2,-9.55549865500002));
#291639=CARTESIAN_POINT('Ctrl Pts',(-4.04277258000006,11.6,-9.55549865500002));
#291640=CARTESIAN_POINT('Ctrl Pts',(-4.04293835900006,15.2,-9.55601007100002));
#291641=CARTESIAN_POINT('Ctrl Pts',(-4.04293835900006,11.6,-9.55601007100002));
#291642=CARTESIAN_POINT('Ctrl Pts',(-4.04316116500006,15.2,-9.55669916200002));
#291643=CARTESIAN_POINT('Ctrl Pts',(-4.04316116500006,11.6,-9.55669916200002));
#291644=CARTESIAN_POINT('Ctrl Pts',(-4.04344211400006,15.2,-9.55757104100002));
#291645=CARTESIAN_POINT('Ctrl Pts',(-4.04344211400006,11.6,-9.55757104100002));
#291646=CARTESIAN_POINT('Ctrl Pts',(-4.04372672500006,15.2,-9.55845733800002));
#291647=CARTESIAN_POINT('Ctrl Pts',(-4.04372672500006,11.6,-9.55845733800002));
#291648=CARTESIAN_POINT('Ctrl Pts',(-4.04401334900006,15.2,-9.55935298200002));
#291649=CARTESIAN_POINT('Ctrl Pts',(-4.04401334900006,11.6,-9.55935298200002));
#291650=CARTESIAN_POINT('Ctrl Pts',(-4.04430195600006,15.2,-9.56025795100001));
#291651=CARTESIAN_POINT('Ctrl Pts',(-4.04430195600006,11.6,-9.56025795100001));
#291652=CARTESIAN_POINT('Ctrl Pts',(-4.04459252500006,15.2,-9.56117222800002));
#291653=CARTESIAN_POINT('Ctrl Pts',(-4.04459252500006,11.6,-9.56117222800002));
#291654=CARTESIAN_POINT('Ctrl Pts',(-4.04488502600006,15.2,-9.56209579100002));
#291655=CARTESIAN_POINT('Ctrl Pts',(-4.04488502600006,11.6,-9.56209579100002));
#291656=CARTESIAN_POINT('Ctrl Pts',(-4.04517943800006,15.2,-9.56302862000001));
#291657=CARTESIAN_POINT('Ctrl Pts',(-4.04517943800006,11.6,-9.56302862000001));
#291658=CARTESIAN_POINT('Ctrl Pts',(-4.04547573400006,15.2,-9.56397069600002));
#291659=CARTESIAN_POINT('Ctrl Pts',(-4.04547573400006,11.6,-9.56397069600002));
#291660=CARTESIAN_POINT('Ctrl Pts',(-4.04577389000006,15.2,-9.56492199900002));
#291661=CARTESIAN_POINT('Ctrl Pts',(-4.04577389000006,11.6,-9.56492199900002));
#291662=CARTESIAN_POINT('Ctrl Pts',(-4.04607388100006,15.2,-9.56588250900002));
#291663=CARTESIAN_POINT('Ctrl Pts',(-4.04607388100006,11.6,-9.56588250900002));
#291664=CARTESIAN_POINT('Ctrl Pts',(-4.04637568200005,15.2,-9.56685220700002));
#291665=CARTESIAN_POINT('Ctrl Pts',(-4.04637568200005,11.6,-9.56685220700002));
#291666=CARTESIAN_POINT('Ctrl Pts',(-4.04667926900006,15.2,-9.56783107300001));
#291667=CARTESIAN_POINT('Ctrl Pts',(-4.04667926900006,11.6,-9.56783107300001));
#291668=CARTESIAN_POINT('Ctrl Pts',(-4.04698461700006,15.2,-9.56881908900002));
#291669=CARTESIAN_POINT('Ctrl Pts',(-4.04698461700006,11.6,-9.56881908900002));
#291670=CARTESIAN_POINT('Ctrl Pts',(-4.04729170300006,15.2,-9.56981623200001));
#291671=CARTESIAN_POINT('Ctrl Pts',(-4.04729170300006,11.6,-9.56981623200001));
#291672=CARTESIAN_POINT('Ctrl Pts',(-4.04760050200006,15.2,-9.57082248800001));
#291673=CARTESIAN_POINT('Ctrl Pts',(-4.04760050200006,11.6,-9.57082248800001));
#291674=CARTESIAN_POINT('Ctrl Pts',(-4.04791099000006,15.2,-9.57183783400002));
#291675=CARTESIAN_POINT('Ctrl Pts',(-4.04791099000006,11.6,-9.57183783400002));
#291676=CARTESIAN_POINT('Ctrl Pts',(-4.04822314400006,15.2,-9.57286225100002));
#291677=CARTESIAN_POINT('Ctrl Pts',(-4.04822314400006,11.6,-9.57286225100002));
#291678=CARTESIAN_POINT('Ctrl Pts',(-4.04853693900006,15.2,-9.57389572300002));
#291679=CARTESIAN_POINT('Ctrl Pts',(-4.04853693900006,11.6,-9.57389572300002));
#291680=CARTESIAN_POINT('Ctrl Pts',(-4.04885235200005,15.2,-9.57493822800001));
#291681=CARTESIAN_POINT('Ctrl Pts',(-4.04885235200005,11.6,-9.57493822800001));
#291682=CARTESIAN_POINT('Ctrl Pts',(-4.04916936000006,15.2,-9.57598974800002));
#291683=CARTESIAN_POINT('Ctrl Pts',(-4.04916936000006,11.6,-9.57598974800002));
#291684=CARTESIAN_POINT('Ctrl Pts',(-4.04948794000005,15.2,-9.57705026500001));
#291685=CARTESIAN_POINT('Ctrl Pts',(-4.04948794000005,11.6,-9.57705026500001));
#291686=CARTESIAN_POINT('Ctrl Pts',(-4.04980806700006,15.2,-9.57811976000002));
#291687=CARTESIAN_POINT('Ctrl Pts',(-4.04980806700006,11.6,-9.57811976000002));
#291688=CARTESIAN_POINT('Ctrl Pts',(-4.05012971900006,15.2,-9.57919821400001));
#291689=CARTESIAN_POINT('Ctrl Pts',(-4.05012971900006,11.6,-9.57919821400001));
#291690=CARTESIAN_POINT('Ctrl Pts',(-4.05045287300006,15.2,-9.58028560900001));
#291691=CARTESIAN_POINT('Ctrl Pts',(-4.05045287300006,11.6,-9.58028560900001));
#291692=CARTESIAN_POINT('Ctrl Pts',(-4.05077750600006,15.2,-9.58138192600002));
#291693=CARTESIAN_POINT('Ctrl Pts',(-4.05077750600006,11.6,-9.58138192600002));
#291694=CARTESIAN_POINT('Ctrl Pts',(-4.05110359500005,15.2,-9.58248714700002));
#291695=CARTESIAN_POINT('Ctrl Pts',(-4.05110359500005,11.6,-9.58248714700002));
#291696=CARTESIAN_POINT('Ctrl Pts',(-4.05143111900006,15.2,-9.58360125300001));
#291697=CARTESIAN_POINT('Ctrl Pts',(-4.05143111900006,11.6,-9.58360125300001));
#291698=CARTESIAN_POINT('Ctrl Pts',(-4.05176005200006,15.2,-9.58472422800002));
#291699=CARTESIAN_POINT('Ctrl Pts',(-4.05176005200006,11.6,-9.58472422800002));
#291700=CARTESIAN_POINT('Ctrl Pts',(-4.05209037500006,15.2,-9.58585605000002));
#291701=CARTESIAN_POINT('Ctrl Pts',(-4.05209037500006,11.6,-9.58585605000002));
#291702=CARTESIAN_POINT('Ctrl Pts',(-4.05242206400006,15.2,-9.58699670600001));
#291703=CARTESIAN_POINT('Ctrl Pts',(-4.05242206400006,11.6,-9.58699670600001));
#291704=CARTESIAN_POINT('Ctrl Pts',(-4.05275509600005,15.2,-9.58814617300002));
#291705=CARTESIAN_POINT('Ctrl Pts',(-4.05275509600005,11.6,-9.58814617300002));
#291706=CARTESIAN_POINT('Ctrl Pts',(-4.05308945100006,15.2,-9.58930443500002));
#291707=CARTESIAN_POINT('Ctrl Pts',(-4.05308945100006,11.6,-9.58930443500002));
#291708=CARTESIAN_POINT('Ctrl Pts',(-4.05342510700006,15.2,-9.59047147500002));
#291709=CARTESIAN_POINT('Ctrl Pts',(-4.05342510700006,11.6,-9.59047147500002));
#291710=CARTESIAN_POINT('Ctrl Pts',(-4.05376204000006,15.2,-9.59164727400001));
#291711=CARTESIAN_POINT('Ctrl Pts',(-4.05376204000006,11.6,-9.59164727400001));
#291712=CARTESIAN_POINT('Ctrl Pts',(-4.05410023000006,15.2,-9.59283181500002));
#291713=CARTESIAN_POINT('Ctrl Pts',(-4.05410023000006,11.6,-9.59283181500002));
#291714=CARTESIAN_POINT('Ctrl Pts',(-4.05443965400006,15.2,-9.59402508100002));
#291715=CARTESIAN_POINT('Ctrl Pts',(-4.05443965400006,11.6,-9.59402508100002));
#291716=CARTESIAN_POINT('Ctrl Pts',(-4.05478029100006,15.2,-9.59522705200002));
#291717=CARTESIAN_POINT('Ctrl Pts',(-4.05478029100006,11.6,-9.59522705200002));
#291718=CARTESIAN_POINT('Ctrl Pts',(-4.05512211900006,15.2,-9.59643771300002));
#291719=CARTESIAN_POINT('Ctrl Pts',(-4.05512211900006,11.6,-9.59643771300002));
#291720=CARTESIAN_POINT('Ctrl Pts',(-4.05546511900006,15.2,-9.59765704600001));
#291721=CARTESIAN_POINT('Ctrl Pts',(-4.05546511900006,11.6,-9.59765704600001));
#291722=CARTESIAN_POINT('Ctrl Pts',(-4.05580926700006,15.2,-9.59888503200002));
#291723=CARTESIAN_POINT('Ctrl Pts',(-4.05580926700006,11.6,-9.59888503200002));
#291724=CARTESIAN_POINT('Ctrl Pts',(-4.05615454400006,15.2,-9.60012165500002));
#291725=CARTESIAN_POINT('Ctrl Pts',(-4.05615454400006,11.6,-9.60012165500002));
#291726=CARTESIAN_POINT('Ctrl Pts',(-4.05650092700006,15.2,-9.60136689800001));
#291727=CARTESIAN_POINT('Ctrl Pts',(-4.05650092700006,11.6,-9.60136689800001));
#291728=CARTESIAN_POINT('Ctrl Pts',(-4.05684839700006,15.2,-9.60262074300001));
#291729=CARTESIAN_POINT('Ctrl Pts',(-4.05684839700006,11.6,-9.60262074300001));
#291730=CARTESIAN_POINT('Ctrl Pts',(-4.05719693100006,15.2,-9.60388317400002));
#291731=CARTESIAN_POINT('Ctrl Pts',(-4.05719693100006,11.6,-9.60388317400002));
#291732=CARTESIAN_POINT('Ctrl Pts',(-4.05754650900006,15.2,-9.60515417200002));
#291733=CARTESIAN_POINT('Ctrl Pts',(-4.05754650900006,11.6,-9.60515417200002));
#291734=CARTESIAN_POINT('Ctrl Pts',(-4.05789711200006,15.2,-9.60643372300002));
#291735=CARTESIAN_POINT('Ctrl Pts',(-4.05789711200006,11.6,-9.60643372300002));
#291736=CARTESIAN_POINT('Ctrl Pts',(-4.05824871700006,15.2,-9.60772180700001));
#291737=CARTESIAN_POINT('Ctrl Pts',(-4.05824871700006,11.6,-9.60772180700001));
#291738=CARTESIAN_POINT('Ctrl Pts',(-4.05860130600006,15.2,-9.60901840800001));
#291739=CARTESIAN_POINT('Ctrl Pts',(-4.05860130600006,11.6,-9.60901840800001));
#291740=CARTESIAN_POINT('Ctrl Pts',(-4.05895485700006,15.2,-9.61032351000001));
#291741=CARTESIAN_POINT('Ctrl Pts',(-4.05895485700006,11.6,-9.61032351000001));
#291742=CARTESIAN_POINT('Ctrl Pts',(-4.05930934900006,15.2,-9.61163709600001));
#291743=CARTESIAN_POINT('Ctrl Pts',(-4.05930934900006,11.6,-9.61163709600001));
#291744=CARTESIAN_POINT('Ctrl Pts',(-4.05966476500006,15.2,-9.61295914900001));
#291745=CARTESIAN_POINT('Ctrl Pts',(-4.05966476500006,11.6,-9.61295914900001));
#291746=CARTESIAN_POINT('Ctrl Pts',(-4.06002108100005,15.2,-9.61428965300002));
#291747=CARTESIAN_POINT('Ctrl Pts',(-4.06002108100005,11.6,-9.61428965300002));
#291748=CARTESIAN_POINT('Ctrl Pts',(-4.06037827900006,15.2,-9.61562859000002));
#291749=CARTESIAN_POINT('Ctrl Pts',(-4.06037827900006,11.6,-9.61562859000002));
#291750=CARTESIAN_POINT('Ctrl Pts',(-4.06073634000006,15.2,-9.61697594500002));
#291751=CARTESIAN_POINT('Ctrl Pts',(-4.06073634000006,11.6,-9.61697594500002));
#291752=CARTESIAN_POINT('Ctrl Pts',(-4.06109524300006,15.2,-9.61833170100002));
#291753=CARTESIAN_POINT('Ctrl Pts',(-4.06109524300006,11.6,-9.61833170100002));
#291754=CARTESIAN_POINT('Ctrl Pts',(-4.06145496900006,15.2,-9.61969584100002));
#291755=CARTESIAN_POINT('Ctrl Pts',(-4.06145496900006,11.6,-9.61969584100002));
#291756=CARTESIAN_POINT('Ctrl Pts',(-4.06181549800006,15.2,-9.62106835000002));
#291757=CARTESIAN_POINT('Ctrl Pts',(-4.06181549800006,11.6,-9.62106835000002));
#291758=CARTESIAN_POINT('Ctrl Pts',(-4.06217680900006,15.2,-9.62244921100002));
#291759=CARTESIAN_POINT('Ctrl Pts',(-4.06217680900006,11.6,-9.62244921100002));
#291760=CARTESIAN_POINT('Ctrl Pts',(-4.06253888500006,15.2,-9.62383840700002));
#291761=CARTESIAN_POINT('Ctrl Pts',(-4.06253888500006,11.6,-9.62383840700002));
#291762=CARTESIAN_POINT('Ctrl Pts',(-4.06290170600006,15.2,-9.62523592300002));
#291763=CARTESIAN_POINT('Ctrl Pts',(-4.06290170600006,11.6,-9.62523592300002));
#291764=CARTESIAN_POINT('Ctrl Pts',(-4.06326525200006,15.2,-9.62664174300001));
#291765=CARTESIAN_POINT('Ctrl Pts',(-4.06326525200006,11.6,-9.62664174300001));
#291766=CARTESIAN_POINT('Ctrl Pts',(-4.06362950500006,15.2,-9.62805584900002));
#291767=CARTESIAN_POINT('Ctrl Pts',(-4.06362950500006,11.6,-9.62805584900002));
#291768=CARTESIAN_POINT('Ctrl Pts',(-4.06399444400006,15.2,-9.62947822800002));
#291769=CARTESIAN_POINT('Ctrl Pts',(-4.06399444400006,11.6,-9.62947822800002));
#291770=CARTESIAN_POINT('Ctrl Pts',(-4.06436005300006,15.2,-9.63090886200002));
#291771=CARTESIAN_POINT('Ctrl Pts',(-4.06436005300006,11.6,-9.63090886200002));
#291772=CARTESIAN_POINT('Ctrl Pts',(-4.06472631000006,15.2,-9.63234773600002));
#291773=CARTESIAN_POINT('Ctrl Pts',(-4.06472631000006,11.6,-9.63234773600002));
#291774=CARTESIAN_POINT('Ctrl Pts',(-4.06509319700006,15.2,-9.63379483400002));
#291775=CARTESIAN_POINT('Ctrl Pts',(-4.06509319700006,11.6,-9.63379483400002));
#291776=CARTESIAN_POINT('Ctrl Pts',(-4.06546069800005,15.2,-9.63525013900002));
#291777=CARTESIAN_POINT('Ctrl Pts',(-4.06546069800005,11.6,-9.63525013900002));
#291778=CARTESIAN_POINT('Ctrl Pts',(-4.06582879000006,15.2,-9.63671363800002));
#291779=CARTESIAN_POINT('Ctrl Pts',(-4.06582879000006,11.6,-9.63671363800002));
#291780=CARTESIAN_POINT('Ctrl Pts',(-4.06619745800006,15.2,-9.63818531300002));
#291781=CARTESIAN_POINT('Ctrl Pts',(-4.06619745800006,11.6,-9.63818531300002));
#291782=CARTESIAN_POINT('Ctrl Pts',(-4.06656668200006,15.2,-9.63966514900001));
#291783=CARTESIAN_POINT('Ctrl Pts',(-4.06656668200006,11.6,-9.63966514900001));
#291784=CARTESIAN_POINT('Ctrl Pts',(-4.06693644400006,15.2,-9.64115313000002));
#291785=CARTESIAN_POINT('Ctrl Pts',(-4.06693644400006,11.6,-9.64115313000002));
#291786=CARTESIAN_POINT('Ctrl Pts',(-4.06730672500006,15.2,-9.64264924100002));
#291787=CARTESIAN_POINT('Ctrl Pts',(-4.06730672500006,11.6,-9.64264924100002));
#291788=CARTESIAN_POINT('Ctrl Pts',(-4.06767750700006,15.2,-9.64415346700001));
#291789=CARTESIAN_POINT('Ctrl Pts',(-4.06767750700006,11.6,-9.64415346700001));
#291790=CARTESIAN_POINT('Ctrl Pts',(-4.06804877300006,15.2,-9.64566579300002));
#291791=CARTESIAN_POINT('Ctrl Pts',(-4.06804877300006,11.6,-9.64566579300002));
#291792=CARTESIAN_POINT('Ctrl Pts',(-4.06842050400006,15.2,-9.64718620200001));
#291793=CARTESIAN_POINT('Ctrl Pts',(-4.06842050400006,11.6,-9.64718620200001));
#291794=CARTESIAN_POINT('Ctrl Pts',(-4.06879268100006,15.2,-9.64871467800002));
#291795=CARTESIAN_POINT('Ctrl Pts',(-4.06879268100006,11.6,-9.64871467800002));
#291796=CARTESIAN_POINT('Ctrl Pts',(-4.06916528800005,15.2,-9.65025121000001));
#291797=CARTESIAN_POINT('Ctrl Pts',(-4.06916528800005,11.6,-9.65025121000001));
#291798=CARTESIAN_POINT('Ctrl Pts',(-4.06953830600005,15.2,-9.65179577800001));
#291799=CARTESIAN_POINT('Ctrl Pts',(-4.06953830600005,11.6,-9.65179577800001));
#291800=CARTESIAN_POINT('Ctrl Pts',(-4.06991171800006,15.2,-9.65334837100001));
#291801=CARTESIAN_POINT('Ctrl Pts',(-4.06991171800006,11.6,-9.65334837100001));
#291802=CARTESIAN_POINT('Ctrl Pts',(-4.07028550500006,15.2,-9.65490897100001));
#291803=CARTESIAN_POINT('Ctrl Pts',(-4.07028550500006,11.6,-9.65490897100001));
#291804=CARTESIAN_POINT('Ctrl Pts',(-4.07065965200006,15.2,-9.65647756300001));
#291805=CARTESIAN_POINT('Ctrl Pts',(-4.07065965200006,11.6,-9.65647756300001));
#291806=CARTESIAN_POINT('Ctrl Pts',(-4.07103413900006,15.2,-9.65805413300002));
#291807=CARTESIAN_POINT('Ctrl Pts',(-4.07103413900006,11.6,-9.65805413300002));
#291808=CARTESIAN_POINT('Ctrl Pts',(-4.07140894900006,15.2,-9.65963866700001));
#291809=CARTESIAN_POINT('Ctrl Pts',(-4.07140894900006,11.6,-9.65963866700001));
#291810=CARTESIAN_POINT('Ctrl Pts',(-4.07178406600006,15.2,-9.66123114900001));
#291811=CARTESIAN_POINT('Ctrl Pts',(-4.07178406600006,11.6,-9.66123114900001));
#291812=CARTESIAN_POINT('Ctrl Pts',(-4.07215947000005,15.2,-9.66283156300001));
#291813=CARTESIAN_POINT('Ctrl Pts',(-4.07215947000005,11.6,-9.66283156300001));
#291814=CARTESIAN_POINT('Ctrl Pts',(-4.07253514800006,15.2,-9.66443989500001));
#291815=CARTESIAN_POINT('Ctrl Pts',(-4.07253514800006,11.6,-9.66443989500001));
#291816=CARTESIAN_POINT('Ctrl Pts',(-4.07291107900006,15.2,-9.66605613100001));
#291817=CARTESIAN_POINT('Ctrl Pts',(-4.07291107900006,11.6,-9.66605613100001));
#291818=CARTESIAN_POINT('Ctrl Pts',(-4.07328724700006,15.2,-9.66768025600001));
#291819=CARTESIAN_POINT('Ctrl Pts',(-4.07328724700006,11.6,-9.66768025600001));
#291820=CARTESIAN_POINT('Ctrl Pts',(-4.07366363600006,15.2,-9.66931225500001));
#291821=CARTESIAN_POINT('Ctrl Pts',(-4.07366363600006,11.6,-9.66931225500001));
#291822=CARTESIAN_POINT('Ctrl Pts',(-4.07404022800006,15.2,-9.67095211400001));
#291823=CARTESIAN_POINT('Ctrl Pts',(-4.07404022800006,11.6,-9.67095211400001));
#291824=CARTESIAN_POINT('Ctrl Pts',(-4.07441700700006,15.2,-9.67259981700001));
#291825=CARTESIAN_POINT('Ctrl Pts',(-4.07441700700006,11.6,-9.67259981700001));
#291826=CARTESIAN_POINT('Ctrl Pts',(-4.07479395600006,15.2,-9.67425535100001));
#291827=CARTESIAN_POINT('Ctrl Pts',(-4.07479395600006,11.6,-9.67425535100001));
#291828=CARTESIAN_POINT('Ctrl Pts',(-4.07517105700006,15.2,-9.67591870100001));
#291829=CARTESIAN_POINT('Ctrl Pts',(-4.07517105700006,11.6,-9.67591870100001));
#291830=CARTESIAN_POINT('Ctrl Pts',(-4.07554829600006,15.2,-9.67758985300001));
#291831=CARTESIAN_POINT('Ctrl Pts',(-4.07554829600006,11.6,-9.67758985300001));
#291832=CARTESIAN_POINT('Ctrl Pts',(-4.07592565400006,15.2,-9.67926879100001));
#291833=CARTESIAN_POINT('Ctrl Pts',(-4.07592565400006,11.6,-9.67926879100001));
#291834=CARTESIAN_POINT('Ctrl Pts',(-4.07630311600006,15.2,-9.68095550200001));
#291835=CARTESIAN_POINT('Ctrl Pts',(-4.07630311600006,11.6,-9.68095550200001));
#291836=CARTESIAN_POINT('Ctrl Pts',(-4.07668066500006,15.2,-9.68264997100001));
#291837=CARTESIAN_POINT('Ctrl Pts',(-4.07668066500006,11.6,-9.68264997100001));
#291838=CARTESIAN_POINT('Ctrl Pts',(-4.07705828300006,15.2,-9.68435218600001));
#291839=CARTESIAN_POINT('Ctrl Pts',(-4.07705828300006,11.6,-9.68435218600001));
#291840=CARTESIAN_POINT('Ctrl Pts',(-4.07743595800006,15.2,-9.68606212900001));
#291841=CARTESIAN_POINT('Ctrl Pts',(-4.07743595800006,11.6,-9.68606212900001));
#291842=CARTESIAN_POINT('Ctrl Pts',(-4.07781367000006,15.2,-9.68777978900001));
#291843=CARTESIAN_POINT('Ctrl Pts',(-4.07781367000006,11.6,-9.68777978900001));
#291844=CARTESIAN_POINT('Ctrl Pts',(-4.07819140400006,15.2,-9.68950514900001));
#291845=CARTESIAN_POINT('Ctrl Pts',(-4.07819140400006,11.6,-9.68950514900001));
#291846=CARTESIAN_POINT('Ctrl Pts',(-4.07856914400006,15.2,-9.69123819800001));
#291847=CARTESIAN_POINT('Ctrl Pts',(-4.07856914400006,11.6,-9.69123819800001));
#291848=CARTESIAN_POINT('Ctrl Pts',(-4.07894687300006,15.2,-9.69297892000001));
#291849=CARTESIAN_POINT('Ctrl Pts',(-4.07894687300006,11.6,-9.69297892000001));
#291850=CARTESIAN_POINT('Ctrl Pts',(-4.07932457800006,15.2,-9.69472730100001));
#291851=CARTESIAN_POINT('Ctrl Pts',(-4.07932457800006,11.6,-9.69472730100001));
#291852=CARTESIAN_POINT('Ctrl Pts',(-4.07970224000006,15.2,-9.69648332900001));
#291853=CARTESIAN_POINT('Ctrl Pts',(-4.07970224000006,11.6,-9.69648332900001));
#291854=CARTESIAN_POINT('Ctrl Pts',(-4.08007984400006,15.2,-9.69824698600001));
#291855=CARTESIAN_POINT('Ctrl Pts',(-4.08007984400006,11.6,-9.69824698600001));
#291856=CARTESIAN_POINT('Ctrl Pts',(-4.08045737600006,15.2,-9.70001826300001));
#291857=CARTESIAN_POINT('Ctrl Pts',(-4.08045737600006,11.6,-9.70001826300001));
#291858=CARTESIAN_POINT('Ctrl Pts',(-4.08083481800006,15.2,-9.70179714300001));
#291859=CARTESIAN_POINT('Ctrl Pts',(-4.08083481800006,11.6,-9.70179714300001));
#291860=CARTESIAN_POINT('Ctrl Pts',(-4.08121215500006,15.2,-9.70358361200001));
#291861=CARTESIAN_POINT('Ctrl Pts',(-4.08121215500006,11.6,-9.70358361200001));
#291862=CARTESIAN_POINT('Ctrl Pts',(-4.08158937200006,15.2,-9.70537765900001));
#291863=CARTESIAN_POINT('Ctrl Pts',(-4.08158937200006,11.6,-9.70537765900001));
#291864=CARTESIAN_POINT('Ctrl Pts',(-4.08196645300006,15.2,-9.70717926800001));
#291865=CARTESIAN_POINT('Ctrl Pts',(-4.08196645300006,11.6,-9.70717926800001));
#291866=CARTESIAN_POINT('Ctrl Pts',(-4.08234338400006,15.2,-9.70898842600001));
#291867=CARTESIAN_POINT('Ctrl Pts',(-4.08234338400006,11.6,-9.70898842600001));
#291868=CARTESIAN_POINT('Ctrl Pts',(-4.08272014700006,15.2,-9.71080511800001));
#291869=CARTESIAN_POINT('Ctrl Pts',(-4.08272014700006,11.6,-9.71080511800001));
#291870=CARTESIAN_POINT('Ctrl Pts',(-4.08309672900006,15.2,-9.71262933200001));
#291871=CARTESIAN_POINT('Ctrl Pts',(-4.08309672900006,11.6,-9.71262933200001));
#291872=CARTESIAN_POINT('Ctrl Pts',(-4.08347311300005,15.2,-9.71446105500001));
#291873=CARTESIAN_POINT('Ctrl Pts',(-4.08347311300005,11.6,-9.71446105500001));
#291874=CARTESIAN_POINT('Ctrl Pts',(-4.08384928600006,15.2,-9.71630027200001));
#291875=CARTESIAN_POINT('Ctrl Pts',(-4.08384928600006,11.6,-9.71630027200001));
#291876=CARTESIAN_POINT('Ctrl Pts',(-4.08422523100006,15.2,-9.71814696900001));
#291877=CARTESIAN_POINT('Ctrl Pts',(-4.08422523100006,11.6,-9.71814696900001));
#291878=CARTESIAN_POINT('Ctrl Pts',(-4.08460093300006,15.2,-9.72000113500001));
#291879=CARTESIAN_POINT('Ctrl Pts',(-4.08460093300006,11.6,-9.72000113500001));
#291880=CARTESIAN_POINT('Ctrl Pts',(-4.08497637900005,15.2,-9.72186275400001));
#291881=CARTESIAN_POINT('Ctrl Pts',(-4.08497637900005,11.6,-9.72186275400001));
#291882=CARTESIAN_POINT('Ctrl Pts',(-4.08535155300005,15.2,-9.72373181400001));
#291883=CARTESIAN_POINT('Ctrl Pts',(-4.08535155300005,11.6,-9.72373181400001));
#291884=CARTESIAN_POINT('Ctrl Pts',(-4.08572643900006,15.2,-9.72560830200001));
#291885=CARTESIAN_POINT('Ctrl Pts',(-4.08572643900006,11.6,-9.72560830200001));
#291886=CARTESIAN_POINT('Ctrl Pts',(-4.08610102200006,15.2,-9.72749220300001));
#291887=CARTESIAN_POINT('Ctrl Pts',(-4.08610102200006,11.6,-9.72749220300001));
#291888=CARTESIAN_POINT('Ctrl Pts',(-4.08647528900006,15.2,-9.72938350500001));
#291889=CARTESIAN_POINT('Ctrl Pts',(-4.08647528900006,11.6,-9.72938350500001));
#291890=CARTESIAN_POINT('Ctrl Pts',(-4.08684922500006,15.2,-9.73128219600001));
#291891=CARTESIAN_POINT('Ctrl Pts',(-4.08684922500006,11.6,-9.73128219600001));
#291892=CARTESIAN_POINT('Ctrl Pts',(-4.08722281500006,15.2,-9.73318826000001));
#291893=CARTESIAN_POINT('Ctrl Pts',(-4.08722281500006,11.6,-9.73318826000001));
#291894=CARTESIAN_POINT('Ctrl Pts',(-4.08759604300006,15.2,-9.73510168500001));
#291895=CARTESIAN_POINT('Ctrl Pts',(-4.08759604300006,11.6,-9.73510168500001));
#291896=CARTESIAN_POINT('Ctrl Pts',(-4.08796889700006,15.2,-9.73702246000001));
#291897=CARTESIAN_POINT('Ctrl Pts',(-4.08796889700006,11.6,-9.73702246000001));
#291898=CARTESIAN_POINT('Ctrl Pts',(-4.08834136200006,15.2,-9.73895056800002));
#291899=CARTESIAN_POINT('Ctrl Pts',(-4.08834136200006,11.6,-9.73895056800002));
#291900=CARTESIAN_POINT('Ctrl Pts',(-4.08871342100006,15.2,-9.74088599900002));
#291901=CARTESIAN_POINT('Ctrl Pts',(-4.08871342100006,11.6,-9.74088599900002));
#291902=CARTESIAN_POINT('Ctrl Pts',(-4.08908506300006,15.2,-9.74282873800002));
#291903=CARTESIAN_POINT('Ctrl Pts',(-4.08908506300006,11.6,-9.74282873800002));
#291904=CARTESIAN_POINT('Ctrl Pts',(-4.08945627200006,15.2,-9.74477877400002));
#291905=CARTESIAN_POINT('Ctrl Pts',(-4.08945627200006,11.6,-9.74477877400002));
#291906=CARTESIAN_POINT('Ctrl Pts',(-4.08982703500006,15.2,-9.74673609300002));
#291907=CARTESIAN_POINT('Ctrl Pts',(-4.08982703500006,11.6,-9.74673609300002));
#291908=CARTESIAN_POINT('Ctrl Pts',(-4.09019733600006,15.2,-9.74870068100001));
#291909=CARTESIAN_POINT('Ctrl Pts',(-4.09019733600006,11.6,-9.74870068100001));
#291910=CARTESIAN_POINT('Ctrl Pts',(-4.09056716200006,15.2,-9.75067252700001));
#291911=CARTESIAN_POINT('Ctrl Pts',(-4.09056716200006,11.6,-9.75067252700001));
#291912=CARTESIAN_POINT('Ctrl Pts',(-4.09093649900006,15.2,-9.75265161800001));
#291913=CARTESIAN_POINT('Ctrl Pts',(-4.09093649900006,11.6,-9.75265161800001));
#291914=CARTESIAN_POINT('Ctrl Pts',(-4.09130533200006,15.2,-9.75463794000001));
#291915=CARTESIAN_POINT('Ctrl Pts',(-4.09130533200006,11.6,-9.75463794000001));
#291916=CARTESIAN_POINT('Ctrl Pts',(-4.09167364900005,15.2,-9.75663148100001));
#291917=CARTESIAN_POINT('Ctrl Pts',(-4.09167364900005,11.6,-9.75663148100001));
#291918=CARTESIAN_POINT('Ctrl Pts',(-4.09204143300006,15.2,-9.75863222700001));
#291919=CARTESIAN_POINT('Ctrl Pts',(-4.09204143300006,11.6,-9.75863222700001));
#291920=CARTESIAN_POINT('Ctrl Pts',(-4.09240867400006,15.2,-9.76064016800001));
#291921=CARTESIAN_POINT('Ctrl Pts',(-4.09240867400006,11.6,-9.76064016800001));
#291922=CARTESIAN_POINT('Ctrl Pts',(-4.09277535500006,15.2,-9.76265528900001));
#291923=CARTESIAN_POINT('Ctrl Pts',(-4.09277535500006,11.6,-9.76265528900001));
#291924=CARTESIAN_POINT('Ctrl Pts',(-4.09314146500006,15.2,-9.76467757800001));
#291925=CARTESIAN_POINT('Ctrl Pts',(-4.09314146500006,11.6,-9.76467757800001));
#291926=CARTESIAN_POINT('Ctrl Pts',(-4.09350698800006,15.2,-9.76670702200001));
#291927=CARTESIAN_POINT('Ctrl Pts',(-4.09350698800006,11.6,-9.76670702200001));
#291928=CARTESIAN_POINT('Ctrl Pts',(-4.09387191000006,15.2,-9.76874360900001));
#291929=CARTESIAN_POINT('Ctrl Pts',(-4.09387191000006,11.6,-9.76874360900001));
#291930=CARTESIAN_POINT('Ctrl Pts',(-4.09423622000006,15.2,-9.77078732700001));
#291931=CARTESIAN_POINT('Ctrl Pts',(-4.09423622000006,11.6,-9.77078732700001));
#291932=CARTESIAN_POINT('Ctrl Pts',(-4.09459990200006,15.2,-9.77283816200002));
#291933=CARTESIAN_POINT('Ctrl Pts',(-4.09459990200006,11.6,-9.77283816200002));
#291934=CARTESIAN_POINT('Ctrl Pts',(-4.09496294500006,15.2,-9.77489610300001));
#291935=CARTESIAN_POINT('Ctrl Pts',(-4.09496294500006,11.6,-9.77489610300001));
#291936=CARTESIAN_POINT('Ctrl Pts',(-4.09532533400006,15.2,-9.77696113700001));
#291937=CARTESIAN_POINT('Ctrl Pts',(-4.09532533400006,11.6,-9.77696113700001));
#291938=CARTESIAN_POINT('Ctrl Pts',(-4.09568705400006,15.2,-9.77903325100001));
#291939=CARTESIAN_POINT('Ctrl Pts',(-4.09568705400006,11.6,-9.77903325100001));
#291940=CARTESIAN_POINT('Ctrl Pts',(-4.09604809600006,15.2,-9.78111243300001));
#291941=CARTESIAN_POINT('Ctrl Pts',(-4.09604809600006,11.6,-9.78111243300001));
#291942=CARTESIAN_POINT('Ctrl Pts',(-4.09640844200006,15.2,-9.78319867000001));
#291943=CARTESIAN_POINT('Ctrl Pts',(-4.09640844200006,11.6,-9.78319867000001));
#291944=CARTESIAN_POINT('Ctrl Pts',(-4.09676808300006,15.2,-9.78529195200001));
#291945=CARTESIAN_POINT('Ctrl Pts',(-4.09676808300006,11.6,-9.78529195200001));
#291946=CARTESIAN_POINT('Ctrl Pts',(-4.09712700200005,15.2,-9.78739226400001));
#291947=CARTESIAN_POINT('Ctrl Pts',(-4.09712700200005,11.6,-9.78739226400001));
#291948=CARTESIAN_POINT('Ctrl Pts',(-4.09748518900006,15.2,-9.78949959400001));
#291949=CARTESIAN_POINT('Ctrl Pts',(-4.09748518900006,11.6,-9.78949959400001));
#291950=CARTESIAN_POINT('Ctrl Pts',(-4.09784262900006,15.2,-9.79161393200001));
#291951=CARTESIAN_POINT('Ctrl Pts',(-4.09784262900006,11.6,-9.79161393200001));
#291952=CARTESIAN_POINT('Ctrl Pts',(-4.09819930900006,15.2,-9.79373526400001));
#291953=CARTESIAN_POINT('Ctrl Pts',(-4.09819930900006,11.6,-9.79373526400001));
#291954=CARTESIAN_POINT('Ctrl Pts',(-4.09855521800006,15.2,-9.79586357800001));
#291955=CARTESIAN_POINT('Ctrl Pts',(-4.09855521800006,11.6,-9.79586357800001));
#291956=CARTESIAN_POINT('Ctrl Pts',(-4.09891034100006,15.2,-9.79799886300001));
#291957=CARTESIAN_POINT('Ctrl Pts',(-4.09891034100006,11.6,-9.79799886300001));
#291958=CARTESIAN_POINT('Ctrl Pts',(-4.09926466500006,15.2,-9.80014110500001));
#291959=CARTESIAN_POINT('Ctrl Pts',(-4.09926466500006,11.6,-9.80014110500001));
#291960=CARTESIAN_POINT('Ctrl Pts',(-4.09961817900006,15.2,-9.80229029300001));
#291961=CARTESIAN_POINT('Ctrl Pts',(-4.09961817900006,11.6,-9.80229029300001));
#291962=CARTESIAN_POINT('Ctrl Pts',(-4.09997086900006,15.2,-9.80444641500001));
#291963=CARTESIAN_POINT('Ctrl Pts',(-4.09997086900006,11.6,-9.80444641500001));
#291964=CARTESIAN_POINT('Ctrl Pts',(-4.10032272300006,15.2,-9.80660945800001));
#291965=CARTESIAN_POINT('Ctrl Pts',(-4.10032272300006,11.6,-9.80660945800001));
#291966=CARTESIAN_POINT('Ctrl Pts',(-4.10067372700006,15.2,-9.80877941200001));
#291967=CARTESIAN_POINT('Ctrl Pts',(-4.10067372700006,11.6,-9.80877941200001));
#291968=CARTESIAN_POINT('Ctrl Pts',(-4.10102386900006,15.2,-9.81095626300001));
#291969=CARTESIAN_POINT('Ctrl Pts',(-4.10102386900006,11.6,-9.81095626300001));
#291970=CARTESIAN_POINT('Ctrl Pts',(-4.10137313800006,15.2,-9.81314000000001));
#291971=CARTESIAN_POINT('Ctrl Pts',(-4.10137313800006,11.6,-9.81314000000001));
#291972=CARTESIAN_POINT('Ctrl Pts',(-4.10172152000006,15.2,-9.81533061200001));
#291973=CARTESIAN_POINT('Ctrl Pts',(-4.10172152000006,11.6,-9.81533061200001));
#291974=CARTESIAN_POINT('Ctrl Pts',(-4.10206900100006,15.2,-9.81752808500001));
#291975=CARTESIAN_POINT('Ctrl Pts',(-4.10206900100006,11.6,-9.81752808500001));
#291976=CARTESIAN_POINT('Ctrl Pts',(-4.10241557100006,15.2,-9.81973240900001));
#291977=CARTESIAN_POINT('Ctrl Pts',(-4.10241557100006,11.6,-9.81973240900001));
#291978=CARTESIAN_POINT('Ctrl Pts',(-4.10276121600006,15.2,-9.82194357100001));
#291979=CARTESIAN_POINT('Ctrl Pts',(-4.10276121600006,11.6,-9.82194357100001));
#291980=CARTESIAN_POINT('Ctrl Pts',(-4.10310592400006,15.2,-9.82416156000001));
#291981=CARTESIAN_POINT('Ctrl Pts',(-4.10310592400006,11.6,-9.82416156000001));
#291982=CARTESIAN_POINT('Ctrl Pts',(-4.10344968400006,15.2,-9.82638636200001));
#291983=CARTESIAN_POINT('Ctrl Pts',(-4.10344968400006,11.6,-9.82638636200001));
#291984=CARTESIAN_POINT('Ctrl Pts',(-4.10379248300006,15.2,-9.82861797000002));
#291985=CARTESIAN_POINT('Ctrl Pts',(-4.10379248300006,11.6,-9.82861797000002));
#291986=CARTESIAN_POINT('Ctrl Pts',(-4.10413430800006,15.2,-9.83085636800001));
#291987=CARTESIAN_POINT('Ctrl Pts',(-4.10413430800006,11.6,-9.83085636800001));
#291988=CARTESIAN_POINT('Ctrl Pts',(-4.10447514700006,15.2,-9.83310154500001));
#291989=CARTESIAN_POINT('Ctrl Pts',(-4.10447514700006,11.6,-9.83310154500001));
#291990=CARTESIAN_POINT('Ctrl Pts',(-4.10481498900006,15.2,-9.83535349100001));
#291991=CARTESIAN_POINT('Ctrl Pts',(-4.10481498900006,11.6,-9.83535349100001));
#291992=CARTESIAN_POINT('Ctrl Pts',(-4.10515382100006,15.2,-9.83761219400001));
#291993=CARTESIAN_POINT('Ctrl Pts',(-4.10515382100006,11.6,-9.83761219400001));
#291994=CARTESIAN_POINT('Ctrl Pts',(-4.10549163100006,15.2,-9.83987764100001));
#291995=CARTESIAN_POINT('Ctrl Pts',(-4.10549163100006,11.6,-9.83987764100001));
#291996=CARTESIAN_POINT('Ctrl Pts',(-4.10582840600005,15.2,-9.84214982100001));
#291997=CARTESIAN_POINT('Ctrl Pts',(-4.10582840600005,11.6,-9.84214982100001));
#291998=CARTESIAN_POINT('Ctrl Pts',(-4.10616413700006,15.2,-9.84442872300001));
#291999=CARTESIAN_POINT('Ctrl Pts',(-4.10616413700006,11.6,-9.84442872300001));
#292000=CARTESIAN_POINT('Ctrl Pts',(-4.10649880900006,15.2,-9.84671433500001));
#292001=CARTESIAN_POINT('Ctrl Pts',(-4.10649880900006,11.6,-9.84671433500001));
#292002=CARTESIAN_POINT('Ctrl Pts',(-4.10683241100006,15.2,-9.84900664600001));
#292003=CARTESIAN_POINT('Ctrl Pts',(-4.10683241100006,11.6,-9.84900664600001));
#292004=CARTESIAN_POINT('Ctrl Pts',(-4.10716493300006,15.2,-9.85130564400001));
#292005=CARTESIAN_POINT('Ctrl Pts',(-4.10716493300006,11.6,-9.85130564400001));
#292006=CARTESIAN_POINT('Ctrl Pts',(-4.10749636000006,15.2,-9.85361131800001));
#292007=CARTESIAN_POINT('Ctrl Pts',(-4.10749636000006,11.6,-9.85361131800001));
#292008=CARTESIAN_POINT('Ctrl Pts',(-4.10782668300006,15.2,-9.85592365600001));
#292009=CARTESIAN_POINT('Ctrl Pts',(-4.10782668300006,11.6,-9.85592365600001));
#292010=CARTESIAN_POINT('Ctrl Pts',(-4.10815588900006,15.2,-9.85824264700001));
#292011=CARTESIAN_POINT('Ctrl Pts',(-4.10815588900006,11.6,-9.85824264700001));
#292012=CARTESIAN_POINT('Ctrl Pts',(-4.10848396700006,15.2,-9.86056827900001));
#292013=CARTESIAN_POINT('Ctrl Pts',(-4.10848396700006,11.6,-9.86056827900001));
#292014=CARTESIAN_POINT('Ctrl Pts',(-4.10881090400006,15.2,-9.86290054200001));
#292015=CARTESIAN_POINT('Ctrl Pts',(-4.10881090400006,11.6,-9.86290054200001));
#292016=CARTESIAN_POINT('Ctrl Pts',(-4.10913669000006,15.2,-9.86523942300001));
#292017=CARTESIAN_POINT('Ctrl Pts',(-4.10913669000006,11.6,-9.86523942300001));
#292018=CARTESIAN_POINT('Ctrl Pts',(-4.10946131400006,15.2,-9.86758491300001));
#292019=CARTESIAN_POINT('Ctrl Pts',(-4.10946131400006,11.6,-9.86758491300001));
#292020=CARTESIAN_POINT('Ctrl Pts',(-4.10978476100006,15.2,-9.86993699800001));
#292021=CARTESIAN_POINT('Ctrl Pts',(-4.10978476100006,11.6,-9.86993699800001));
#292022=CARTESIAN_POINT('Ctrl Pts',(-4.11010702400006,15.2,-9.87229566900002));
#292023=CARTESIAN_POINT('Ctrl Pts',(-4.11010702400006,11.6,-9.87229566900002));
#292024=CARTESIAN_POINT('Ctrl Pts',(-4.11042808900006,15.2,-9.87466091300002));
#292025=CARTESIAN_POINT('Ctrl Pts',(-4.11042808900006,11.6,-9.87466091300002));
#292026=CARTESIAN_POINT('Ctrl Pts',(-4.11074794500006,15.2,-9.87703272000001));
#292027=CARTESIAN_POINT('Ctrl Pts',(-4.11074794500006,11.6,-9.87703272000001));
#292028=CARTESIAN_POINT('Ctrl Pts',(-4.11106658100006,15.2,-9.87941107800001));
#292029=CARTESIAN_POINT('Ctrl Pts',(-4.11106658100006,11.6,-9.87941107800001));
#292030=CARTESIAN_POINT('Ctrl Pts',(-4.11138398500006,15.2,-9.88179597800001));
#292031=CARTESIAN_POINT('Ctrl Pts',(-4.11138398500006,11.6,-9.88179597800001));
#292032=CARTESIAN_POINT('Ctrl Pts',(-4.11170014700006,15.2,-9.88418740500001));
#292033=CARTESIAN_POINT('Ctrl Pts',(-4.11170014700006,11.6,-9.88418740500001));
#292034=CARTESIAN_POINT('Ctrl Pts',(-4.11201505600006,15.2,-9.88658535100001));
#292035=CARTESIAN_POINT('Ctrl Pts',(-4.11201505600006,11.6,-9.88658535100001));
#292036=CARTESIAN_POINT('Ctrl Pts',(-4.11232869800005,15.2,-9.88898980400001));
#292037=CARTESIAN_POINT('Ctrl Pts',(-4.11232869800005,11.6,-9.88898980400001));
#292038=CARTESIAN_POINT('Ctrl Pts',(-4.11264106500006,15.2,-9.89140075300002));
#292039=CARTESIAN_POINT('Ctrl Pts',(-4.11264106500006,11.6,-9.89140075300002));
#292040=CARTESIAN_POINT('Ctrl Pts',(-4.11295214400006,15.2,-9.89381818800001));
#292041=CARTESIAN_POINT('Ctrl Pts',(-4.11295214400006,11.6,-9.89381818800001));
#292042=CARTESIAN_POINT('Ctrl Pts',(-4.11326192500006,15.2,-9.89624209500001));
#292043=CARTESIAN_POINT('Ctrl Pts',(-4.11326192500006,11.6,-9.89624209500001));
#292044=CARTESIAN_POINT('Ctrl Pts',(-4.11357039600006,15.2,-9.89867246600001));
#292045=CARTESIAN_POINT('Ctrl Pts',(-4.11357039600006,11.6,-9.89867246600001));
#292046=CARTESIAN_POINT('Ctrl Pts',(-4.11387754700006,15.2,-9.90110928800001));
#292047=CARTESIAN_POINT('Ctrl Pts',(-4.11387754700006,11.6,-9.90110928800001));
#292048=CARTESIAN_POINT('Ctrl Pts',(-4.11418336800006,15.2,-9.90355255300001));
#292049=CARTESIAN_POINT('Ctrl Pts',(-4.11418336800006,11.6,-9.90355255300001));
#292050=CARTESIAN_POINT('Ctrl Pts',(-4.11448784500006,15.2,-9.90600224700001));
#292051=CARTESIAN_POINT('Ctrl Pts',(-4.11448784500006,11.6,-9.90600224700001));
#292052=CARTESIAN_POINT('Ctrl Pts',(-4.11479097000006,15.2,-9.90845836000001));
#292053=CARTESIAN_POINT('Ctrl Pts',(-4.11479097000006,11.6,-9.90845836000001));
#292054=CARTESIAN_POINT('Ctrl Pts',(-4.11509273200005,15.2,-9.91092088100001));
#292055=CARTESIAN_POINT('Ctrl Pts',(-4.11509273200005,11.6,-9.91092088100001));
#292056=CARTESIAN_POINT('Ctrl Pts',(-4.11539311800006,15.2,-9.91338980100001));
#292057=CARTESIAN_POINT('Ctrl Pts',(-4.11539311800006,11.6,-9.91338980100001));
#292058=CARTESIAN_POINT('Ctrl Pts',(-4.11569211900006,15.2,-9.91586510600001));
#292059=CARTESIAN_POINT('Ctrl Pts',(-4.11569211900006,11.6,-9.91586510600001));
#292060=CARTESIAN_POINT('Ctrl Pts',(-4.11598972300006,15.2,-9.91834678800001));
#292061=CARTESIAN_POINT('Ctrl Pts',(-4.11598972300006,11.6,-9.91834678800001));
#292062=CARTESIAN_POINT('Ctrl Pts',(-4.11628592200006,15.2,-9.92083483500001));
#292063=CARTESIAN_POINT('Ctrl Pts',(-4.11628592200006,11.6,-9.92083483500001));
#292064=CARTESIAN_POINT('Ctrl Pts',(-4.11658070300006,15.2,-9.92332923600001));
#292065=CARTESIAN_POINT('Ctrl Pts',(-4.11658070300006,11.6,-9.92332923600001));
#292066=CARTESIAN_POINT('Ctrl Pts',(-4.11687405500006,15.2,-9.92582998100001));
#292067=CARTESIAN_POINT('Ctrl Pts',(-4.11687405500006,11.6,-9.92582998100001));
#292068=CARTESIAN_POINT('Ctrl Pts',(-4.11716597000006,15.2,-9.92833705900001));
#292069=CARTESIAN_POINT('Ctrl Pts',(-4.11716597000006,11.6,-9.92833705900001));
#292070=CARTESIAN_POINT('Ctrl Pts',(-4.11745643400006,15.2,-9.93085045900001));
#292071=CARTESIAN_POINT('Ctrl Pts',(-4.11745643400006,11.6,-9.93085045900001));
#292072=CARTESIAN_POINT('Ctrl Pts',(-4.11774544000005,15.2,-9.93337017000002));
#292073=CARTESIAN_POINT('Ctrl Pts',(-4.11774544000005,11.6,-9.93337017000002));
#292074=CARTESIAN_POINT('Ctrl Pts',(-4.11803297600006,15.2,-9.93589618200001));
#292075=CARTESIAN_POINT('Ctrl Pts',(-4.11803297600006,11.6,-9.93589618200001));
#292076=CARTESIAN_POINT('Ctrl Pts',(-4.11831903100006,15.2,-9.93842848500002));
#292077=CARTESIAN_POINT('Ctrl Pts',(-4.11831903100006,11.6,-9.93842848500002));
#292078=CARTESIAN_POINT('Ctrl Pts',(-4.11860359500006,15.2,-9.94096706700001));
#292079=CARTESIAN_POINT('Ctrl Pts',(-4.11860359500006,11.6,-9.94096706700001));
#292080=CARTESIAN_POINT('Ctrl Pts',(-4.11888665800006,15.2,-9.94351191900001));
#292081=CARTESIAN_POINT('Ctrl Pts',(-4.11888665800006,11.6,-9.94351191900001));
#292082=CARTESIAN_POINT('Ctrl Pts',(-4.11916821000006,15.2,-9.94606302900001));
#292083=CARTESIAN_POINT('Ctrl Pts',(-4.11916821000006,11.6,-9.94606302900001));
#292084=CARTESIAN_POINT('Ctrl Pts',(-4.11944823900006,15.2,-9.94862038700001));
#292085=CARTESIAN_POINT('Ctrl Pts',(-4.11944823900006,11.6,-9.94862038700001));
#292086=CARTESIAN_POINT('Ctrl Pts',(-4.11972673700006,15.2,-9.95118398200001));
#292087=CARTESIAN_POINT('Ctrl Pts',(-4.11972673700006,11.6,-9.95118398200001));
#292088=CARTESIAN_POINT('Ctrl Pts',(-4.12000369300006,15.2,-9.95375380500001));
#292089=CARTESIAN_POINT('Ctrl Pts',(-4.12000369300006,11.6,-9.95375380500001));
#292090=CARTESIAN_POINT('Ctrl Pts',(-4.12027909600006,15.2,-9.95632984300001));
#292091=CARTESIAN_POINT('Ctrl Pts',(-4.12027909600006,11.6,-9.95632984300001));
#292092=CARTESIAN_POINT('Ctrl Pts',(-4.12055293700006,15.2,-9.95891208800001));
#292093=CARTESIAN_POINT('Ctrl Pts',(-4.12055293700006,11.6,-9.95891208800001));
#292094=CARTESIAN_POINT('Ctrl Pts',(-4.12082520500006,15.2,-9.96150052900001));
#292095=CARTESIAN_POINT('Ctrl Pts',(-4.12082520500006,11.6,-9.96150052900001));
#292096=CARTESIAN_POINT('Ctrl Pts',(-4.12109589100006,15.2,-9.96409515500001));
#292097=CARTESIAN_POINT('Ctrl Pts',(-4.12109589100006,11.6,-9.96409515500001));
#292098=CARTESIAN_POINT('Ctrl Pts',(-4.12136498300006,15.2,-9.96669595500001));
#292099=CARTESIAN_POINT('Ctrl Pts',(-4.12136498300006,11.6,-9.96669595500001));
#292100=CARTESIAN_POINT('Ctrl Pts',(-4.12163247300006,15.2,-9.96930291900001));
#292101=CARTESIAN_POINT('Ctrl Pts',(-4.12163247300006,11.6,-9.96930291900001));
#292102=CARTESIAN_POINT('Ctrl Pts',(-4.12189835100006,15.2,-9.97191603900001));
#292103=CARTESIAN_POINT('Ctrl Pts',(-4.12189835100006,11.6,-9.97191603900001));
#292104=CARTESIAN_POINT('Ctrl Pts',(-4.12216260500006,15.2,-9.97453530100001));
#292105=CARTESIAN_POINT('Ctrl Pts',(-4.12216260500006,11.6,-9.97453530100001));
#292106=CARTESIAN_POINT('Ctrl Pts',(-4.12242522800006,15.2,-9.97716069700001));
#292107=CARTESIAN_POINT('Ctrl Pts',(-4.12242522800006,11.6,-9.97716069700001));
#292108=CARTESIAN_POINT('Ctrl Pts',(-4.12268620700006,15.2,-9.97979221700001));
#292109=CARTESIAN_POINT('Ctrl Pts',(-4.12268620700006,11.6,-9.97979221700001));
#292110=CARTESIAN_POINT('Ctrl Pts',(-4.12294553500006,15.2,-9.98242984900001));
#292111=CARTESIAN_POINT('Ctrl Pts',(-4.12294553500006,11.6,-9.98242984900001));
#292112=CARTESIAN_POINT('Ctrl Pts',(-4.12320320100005,15.2,-9.98507358300001));
#292113=CARTESIAN_POINT('Ctrl Pts',(-4.12320320100005,11.6,-9.98507358300001));
#292114=CARTESIAN_POINT('Ctrl Pts',(-4.12345919400006,15.2,-9.98772340900001));
#292115=CARTESIAN_POINT('Ctrl Pts',(-4.12345919400006,11.6,-9.98772340900001));
#292116=CARTESIAN_POINT('Ctrl Pts',(-4.12371350700006,15.2,-9.99037931800001));
#292117=CARTESIAN_POINT('Ctrl Pts',(-4.12371350700006,11.6,-9.99037931800001));
#292118=CARTESIAN_POINT('Ctrl Pts',(-4.12396612900006,15.2,-9.99304129900001));
#292119=CARTESIAN_POINT('Ctrl Pts',(-4.12396612900006,11.6,-9.99304129900001));
#292120=CARTESIAN_POINT('Ctrl Pts',(-4.12421704900006,15.2,-9.99570934200001));
#292121=CARTESIAN_POINT('Ctrl Pts',(-4.12421704900006,11.6,-9.99570934200001));
#292122=CARTESIAN_POINT('Ctrl Pts',(-4.12446625800006,15.2,-9.99838343600001));
#292123=CARTESIAN_POINT('Ctrl Pts',(-4.12446625800006,11.6,-9.99838343600001));
#292124=CARTESIAN_POINT('Ctrl Pts',(-4.12471374800006,15.2,-10.001063571));
#292125=CARTESIAN_POINT('Ctrl Pts',(-4.12471374800006,11.6,-10.001063571));
#292126=CARTESIAN_POINT('Ctrl Pts',(-4.12495950800006,15.2,-10.003749738));
#292127=CARTESIAN_POINT('Ctrl Pts',(-4.12495950800006,11.6,-10.003749738));
#292128=CARTESIAN_POINT('Ctrl Pts',(-4.12520352900006,15.2,-10.006441926));
#292129=CARTESIAN_POINT('Ctrl Pts',(-4.12520352900006,11.6,-10.006441926));
#292130=CARTESIAN_POINT('Ctrl Pts',(-4.12544580000006,15.2,-10.009140125));
#292131=CARTESIAN_POINT('Ctrl Pts',(-4.12544580000006,11.6,-10.009140125));
#292132=CARTESIAN_POINT('Ctrl Pts',(-4.12568631400006,15.2,-10.011844324));
#292133=CARTESIAN_POINT('Ctrl Pts',(-4.12568631400006,11.6,-10.011844324));
#292134=CARTESIAN_POINT('Ctrl Pts',(-4.12592506000006,15.2,-10.014554516));
#292135=CARTESIAN_POINT('Ctrl Pts',(-4.12592506000006,11.6,-10.014554516));
#292136=CARTESIAN_POINT('Ctrl Pts',(-4.12616203000006,15.2,-10.017270688));
#292137=CARTESIAN_POINT('Ctrl Pts',(-4.12616203000006,11.6,-10.017270688));
#292138=CARTESIAN_POINT('Ctrl Pts',(-4.12639721200006,15.2,-10.019992831));
#292139=CARTESIAN_POINT('Ctrl Pts',(-4.12639721200006,11.6,-10.019992831));
#292140=CARTESIAN_POINT('Ctrl Pts',(-4.12663059900006,15.2,-10.022720935));
#292141=CARTESIAN_POINT('Ctrl Pts',(-4.12663059900006,11.6,-10.022720935));
#292142=CARTESIAN_POINT('Ctrl Pts',(-4.12686218000006,15.2,-10.02545499));
#292143=CARTESIAN_POINT('Ctrl Pts',(-4.12686218000006,11.6,-10.02545499));
#292144=CARTESIAN_POINT('Ctrl Pts',(-4.12709194700006,15.2,-10.028194986));
#292145=CARTESIAN_POINT('Ctrl Pts',(-4.12709194700006,11.6,-10.028194986));
#292146=CARTESIAN_POINT('Ctrl Pts',(-4.12731989100006,15.2,-10.030940913));
#292147=CARTESIAN_POINT('Ctrl Pts',(-4.12731989100006,11.6,-10.030940913));
#292148=CARTESIAN_POINT('Ctrl Pts',(-4.12754600100006,15.2,-10.03369276));
#292149=CARTESIAN_POINT('Ctrl Pts',(-4.12754600100006,11.6,-10.03369276));
#292150=CARTESIAN_POINT('Ctrl Pts',(-4.12777027000006,15.2,-10.036450519));
#292151=CARTESIAN_POINT('Ctrl Pts',(-4.12777027000006,11.6,-10.036450519));
#292152=CARTESIAN_POINT('Ctrl Pts',(-4.12799268700006,15.2,-10.03921418));
#292153=CARTESIAN_POINT('Ctrl Pts',(-4.12799268700006,11.6,-10.03921418));
#292154=CARTESIAN_POINT('Ctrl Pts',(-4.12821324300006,15.2,-10.041983733));
#292155=CARTESIAN_POINT('Ctrl Pts',(-4.12821324300006,11.6,-10.041983733));
#292156=CARTESIAN_POINT('Ctrl Pts',(-4.12843193000006,15.2,-10.044759166));
#292157=CARTESIAN_POINT('Ctrl Pts',(-4.12843193000006,11.6,-10.044759166));
#292158=CARTESIAN_POINT('Ctrl Pts',(-4.12864873900006,15.2,-10.047540471));
#292159=CARTESIAN_POINT('Ctrl Pts',(-4.12864873900006,11.6,-10.047540471));
#292160=CARTESIAN_POINT('Ctrl Pts',(-4.12886366000006,15.2,-10.050327639));
#292161=CARTESIAN_POINT('Ctrl Pts',(-4.12886366000006,11.6,-10.050327639));
#292162=CARTESIAN_POINT('Ctrl Pts',(-4.12907668400006,15.2,-10.053120659));
#292163=CARTESIAN_POINT('Ctrl Pts',(-4.12907668400006,11.6,-10.053120659));
#292164=CARTESIAN_POINT('Ctrl Pts',(-4.12928780200006,15.2,-10.055919521));
#292165=CARTESIAN_POINT('Ctrl Pts',(-4.12928780200006,11.6,-10.055919521));
#292166=CARTESIAN_POINT('Ctrl Pts',(-4.12949700600006,15.2,-10.058724216));
#292167=CARTESIAN_POINT('Ctrl Pts',(-4.12949700600006,11.6,-10.058724216));
#292168=CARTESIAN_POINT('Ctrl Pts',(-4.12970428600006,15.2,-10.061534734));
#292169=CARTESIAN_POINT('Ctrl Pts',(-4.12970428600006,11.6,-10.061534734));
#292170=CARTESIAN_POINT('Ctrl Pts',(-4.12990963400006,15.2,-10.064351065));
#292171=CARTESIAN_POINT('Ctrl Pts',(-4.12990963400006,11.6,-10.064351065));
#292172=CARTESIAN_POINT('Ctrl Pts',(-4.13011304000006,15.2,-10.067173199));
#292173=CARTESIAN_POINT('Ctrl Pts',(-4.13011304000006,11.6,-10.067173199));
#292174=CARTESIAN_POINT('Ctrl Pts',(-4.13031449600005,15.2,-10.070001127));
#292175=CARTESIAN_POINT('Ctrl Pts',(-4.13031449600005,11.6,-10.070001127));
#292176=CARTESIAN_POINT('Ctrl Pts',(-4.13051399200006,15.2,-10.07283484));
#292177=CARTESIAN_POINT('Ctrl Pts',(-4.13051399200006,11.6,-10.07283484));
#292178=CARTESIAN_POINT('Ctrl Pts',(-4.13071152200006,15.2,-10.075674326));
#292179=CARTESIAN_POINT('Ctrl Pts',(-4.13071152200006,11.6,-10.075674326));
#292180=CARTESIAN_POINT('Ctrl Pts',(-4.13090707400006,15.2,-10.078519577));
#292181=CARTESIAN_POINT('Ctrl Pts',(-4.13090707400006,11.6,-10.078519577));
#292182=CARTESIAN_POINT('Ctrl Pts',(-4.13110064100006,15.2,-10.081370584));
#292183=CARTESIAN_POINT('Ctrl Pts',(-4.13110064100006,11.6,-10.081370584));
#292184=CARTESIAN_POINT('Ctrl Pts',(-4.13129221500006,15.2,-10.084227336));
#292185=CARTESIAN_POINT('Ctrl Pts',(-4.13129221500006,11.6,-10.084227336));
#292186=CARTESIAN_POINT('Ctrl Pts',(-4.13148178500006,15.2,-10.087089824));
#292187=CARTESIAN_POINT('Ctrl Pts',(-4.13148178500006,11.6,-10.087089824));
#292188=CARTESIAN_POINT('Ctrl Pts',(-4.13166934400006,15.2,-10.089958038));
#292189=CARTESIAN_POINT('Ctrl Pts',(-4.13166934400006,11.6,-10.089958038));
#292190=CARTESIAN_POINT('Ctrl Pts',(-4.13185488300006,15.2,-10.09283197));
#292191=CARTESIAN_POINT('Ctrl Pts',(-4.13185488300006,11.6,-10.09283197));
#292192=CARTESIAN_POINT('Ctrl Pts',(-4.13203839300006,15.2,-10.095711608));
#292193=CARTESIAN_POINT('Ctrl Pts',(-4.13203839300006,11.6,-10.095711608));
#292194=CARTESIAN_POINT('Ctrl Pts',(-4.13221986700006,15.2,-10.098596944));
#292195=CARTESIAN_POINT('Ctrl Pts',(-4.13221986700006,11.6,-10.098596944));
#292196=CARTESIAN_POINT('Ctrl Pts',(-4.13239929400006,15.2,-10.101487969));
#292197=CARTESIAN_POINT('Ctrl Pts',(-4.13239929400006,11.6,-10.101487969));
#292198=CARTESIAN_POINT('Ctrl Pts',(-4.13257666800006,15.2,-10.104384672));
#292199=CARTESIAN_POINT('Ctrl Pts',(-4.13257666800006,11.6,-10.104384672));
#292200=CARTESIAN_POINT('Ctrl Pts',(-4.13275197800006,15.2,-10.107287044));
#292201=CARTESIAN_POINT('Ctrl Pts',(-4.13275197800006,11.6,-10.107287044));
#292202=CARTESIAN_POINT('Ctrl Pts',(-4.13292521800006,15.2,-10.110195076));
#292203=CARTESIAN_POINT('Ctrl Pts',(-4.13292521800006,11.6,-10.110195076));
#292204=CARTESIAN_POINT('Ctrl Pts',(-4.13309637800006,15.2,-10.113108759));
#292205=CARTESIAN_POINT('Ctrl Pts',(-4.13309637800006,11.6,-10.113108759));
#292206=CARTESIAN_POINT('Ctrl Pts',(-4.13326545000006,15.2,-10.116028082));
#292207=CARTESIAN_POINT('Ctrl Pts',(-4.13326545000006,11.6,-10.116028082));
#292208=CARTESIAN_POINT('Ctrl Pts',(-4.13343242600006,15.2,-10.118953036));
#292209=CARTESIAN_POINT('Ctrl Pts',(-4.13343242600006,11.6,-10.118953036));
#292210=CARTESIAN_POINT('Ctrl Pts',(-4.13359729700006,15.2,-10.121883613));
#292211=CARTESIAN_POINT('Ctrl Pts',(-4.13359729700006,11.6,-10.121883613));
#292212=CARTESIAN_POINT('Ctrl Pts',(-4.13376005400006,15.2,-10.124819802));
#292213=CARTESIAN_POINT('Ctrl Pts',(-4.13376005400006,11.6,-10.124819802));
#292214=CARTESIAN_POINT('Ctrl Pts',(-4.13392069200006,15.2,-10.127761595));
#292215=CARTESIAN_POINT('Ctrl Pts',(-4.13392069200006,11.6,-10.127761595));
#292216=CARTESIAN_POINT('Ctrl Pts',(-4.13407919800005,15.2,-10.130708982));
#292217=CARTESIAN_POINT('Ctrl Pts',(-4.13407919800005,11.6,-10.130708982));
#292218=CARTESIAN_POINT('Ctrl Pts',(-4.13423556800006,15.2,-10.133661953));
#292219=CARTESIAN_POINT('Ctrl Pts',(-4.13423556800006,11.6,-10.133661953));
#292220=CARTESIAN_POINT('Ctrl Pts',(-4.13438979000006,15.2,-10.136620499));
#292221=CARTESIAN_POINT('Ctrl Pts',(-4.13438979000006,11.6,-10.136620499));
#292222=CARTESIAN_POINT('Ctrl Pts',(-4.13454185900005,15.2,-10.139584612));
#292223=CARTESIAN_POINT('Ctrl Pts',(-4.13454185900005,11.6,-10.139584612));
#292224=CARTESIAN_POINT('Ctrl Pts',(-4.13469176500006,15.2,-10.142554281));
#292225=CARTESIAN_POINT('Ctrl Pts',(-4.13469176500006,11.6,-10.142554281));
#292226=CARTESIAN_POINT('Ctrl Pts',(-4.13483950100006,15.2,-10.145529497));
#292227=CARTESIAN_POINT('Ctrl Pts',(-4.13483950100006,11.6,-10.145529497));
#292228=CARTESIAN_POINT('Ctrl Pts',(-4.13498505800006,15.2,-10.148510251));
#292229=CARTESIAN_POINT('Ctrl Pts',(-4.13498505800006,11.6,-10.148510251));
#292230=CARTESIAN_POINT('Ctrl Pts',(-4.13512842900006,15.2,-10.151496534));
#292231=CARTESIAN_POINT('Ctrl Pts',(-4.13512842900006,11.6,-10.151496534));
#292232=CARTESIAN_POINT('Ctrl Pts',(-4.13526960400006,15.2,-10.154488337));
#292233=CARTESIAN_POINT('Ctrl Pts',(-4.13526960400006,11.6,-10.154488337));
#292234=CARTESIAN_POINT('Ctrl Pts',(-4.13540857600006,15.2,-10.15748565));
#292235=CARTESIAN_POINT('Ctrl Pts',(-4.13540857600006,11.6,-10.15748565));
#292236=CARTESIAN_POINT('Ctrl Pts',(-4.13554533800006,15.2,-10.160488466));
#292237=CARTESIAN_POINT('Ctrl Pts',(-4.13554533800006,11.6,-10.160488466));
#292238=CARTESIAN_POINT('Ctrl Pts',(-4.13567988100006,15.2,-10.163496771));
#292239=CARTESIAN_POINT('Ctrl Pts',(-4.13567988100006,11.6,-10.163496771));
#292240=CARTESIAN_POINT('Ctrl Pts',(-4.13581219700006,15.2,-10.16651056));
#292241=CARTESIAN_POINT('Ctrl Pts',(-4.13581219700006,11.6,-10.16651056));
#292242=CARTESIAN_POINT('Ctrl Pts',(-4.13594227700006,15.2,-10.169529823));
#292243=CARTESIAN_POINT('Ctrl Pts',(-4.13594227700006,11.6,-10.169529823));
#292244=CARTESIAN_POINT('Ctrl Pts',(-4.13607011600006,15.2,-10.17255455));
#292245=CARTESIAN_POINT('Ctrl Pts',(-4.13607011600006,11.6,-10.17255455));
#292246=CARTESIAN_POINT('Ctrl Pts',(-4.13619570300006,15.2,-10.175584733));
#292247=CARTESIAN_POINT('Ctrl Pts',(-4.13619570300006,11.6,-10.175584733));
#292248=CARTESIAN_POINT('Ctrl Pts',(-4.13631903200006,15.2,-10.178620362));
#292249=CARTESIAN_POINT('Ctrl Pts',(-4.13631903200006,11.6,-10.178620362));
#292250=CARTESIAN_POINT('Ctrl Pts',(-4.13644009500006,15.2,-10.181661427));
#292251=CARTESIAN_POINT('Ctrl Pts',(-4.13644009500006,11.6,-10.181661427));
#292252=CARTESIAN_POINT('Ctrl Pts',(-4.13655888400006,15.2,-10.184707922));
#292253=CARTESIAN_POINT('Ctrl Pts',(-4.13655888400006,11.6,-10.184707922));
#292254=CARTESIAN_POINT('Ctrl Pts',(-4.13667539100006,15.2,-10.187759834));
#292255=CARTESIAN_POINT('Ctrl Pts',(-4.13667539100006,11.6,-10.187759834));
#292256=CARTESIAN_POINT('Ctrl Pts',(-4.13678960800006,15.2,-10.190817158));
#292257=CARTESIAN_POINT('Ctrl Pts',(-4.13678960800006,11.6,-10.190817158));
#292258=CARTESIAN_POINT('Ctrl Pts',(-4.13690152700006,15.2,-10.193879881));
#292259=CARTESIAN_POINT('Ctrl Pts',(-4.13690152700006,11.6,-10.193879881));
#292260=CARTESIAN_POINT('Ctrl Pts',(-4.13701114100006,15.2,-10.196947997));
#292261=CARTESIAN_POINT('Ctrl Pts',(-4.13701114100006,11.6,-10.196947997));
#292262=CARTESIAN_POINT('Ctrl Pts',(-4.13711844300006,15.2,-10.200021495));
#292263=CARTESIAN_POINT('Ctrl Pts',(-4.13711844300006,11.6,-10.200021495));
#292264=CARTESIAN_POINT('Ctrl Pts',(-4.13722342400006,15.2,-10.203100366));
#292265=CARTESIAN_POINT('Ctrl Pts',(-4.13722342400006,11.6,-10.203100366));
#292266=CARTESIAN_POINT('Ctrl Pts',(-4.13732607700006,15.2,-10.206184603));
#292267=CARTESIAN_POINT('Ctrl Pts',(-4.13732607700006,11.6,-10.206184603));
#292268=CARTESIAN_POINT('Ctrl Pts',(-4.13742639400006,15.2,-10.209274195));
#292269=CARTESIAN_POINT('Ctrl Pts',(-4.13742639400006,11.6,-10.209274195));
#292270=CARTESIAN_POINT('Ctrl Pts',(-4.13752436800006,15.2,-10.212369135));
#292271=CARTESIAN_POINT('Ctrl Pts',(-4.13752436800006,11.6,-10.212369135));
#292272=CARTESIAN_POINT('Ctrl Pts',(-4.13761999100006,15.2,-10.215469411));
#292273=CARTESIAN_POINT('Ctrl Pts',(-4.13761999100006,11.6,-10.215469411));
#292274=CARTESIAN_POINT('Ctrl Pts',(-4.13771325500006,15.2,-10.218575018));
#292275=CARTESIAN_POINT('Ctrl Pts',(-4.13771325500006,11.6,-10.218575018));
#292276=CARTESIAN_POINT('Ctrl Pts',(-4.13780415300006,15.2,-10.221685943));
#292277=CARTESIAN_POINT('Ctrl Pts',(-4.13780415300006,11.6,-10.221685943));
#292278=CARTESIAN_POINT('Ctrl Pts',(-4.13789267800006,15.2,-10.224802181));
#292279=CARTESIAN_POINT('Ctrl Pts',(-4.13789267800006,11.6,-10.224802181));
#292280=CARTESIAN_POINT('Ctrl Pts',(-4.13797882100006,15.2,-10.22792372));
#292281=CARTESIAN_POINT('Ctrl Pts',(-4.13797882100006,11.6,-10.22792372));
#292282=CARTESIAN_POINT('Ctrl Pts',(-4.13806257600006,15.2,-10.231050552));
#292283=CARTESIAN_POINT('Ctrl Pts',(-4.13806257600006,11.6,-10.231050552));
#292284=CARTESIAN_POINT('Ctrl Pts',(-4.13814393400005,15.2,-10.234182669));
#292285=CARTESIAN_POINT('Ctrl Pts',(-4.13814393400005,11.6,-10.234182669));
#292286=CARTESIAN_POINT('Ctrl Pts',(-4.13822289000006,15.2,-10.237320063));
#292287=CARTESIAN_POINT('Ctrl Pts',(-4.13822289000006,11.6,-10.237320063));
#292288=CARTESIAN_POINT('Ctrl Pts',(-4.13829943500006,15.2,-10.240462721));
#292289=CARTESIAN_POINT('Ctrl Pts',(-4.13829943500006,11.6,-10.240462721));
#292290=CARTESIAN_POINT('Ctrl Pts',(-4.13837356100006,15.2,-10.243610638));
#292291=CARTESIAN_POINT('Ctrl Pts',(-4.13837356100006,11.6,-10.243610638));
#292292=CARTESIAN_POINT('Ctrl Pts',(-4.13844526300006,15.2,-10.246763805));
#292293=CARTESIAN_POINT('Ctrl Pts',(-4.13844526300006,11.6,-10.246763805));
#292294=CARTESIAN_POINT('Ctrl Pts',(-4.13851453100006,15.2,-10.249922211));
#292295=CARTESIAN_POINT('Ctrl Pts',(-4.13851453100006,11.6,-10.249922211));
#292296=CARTESIAN_POINT('Ctrl Pts',(-4.13858135900006,15.2,-10.253085849));
#292297=CARTESIAN_POINT('Ctrl Pts',(-4.13858135900006,11.6,-10.253085849));
#292298=CARTESIAN_POINT('Ctrl Pts',(-4.13864573900006,15.2,-10.25625471));
#292299=CARTESIAN_POINT('Ctrl Pts',(-4.13864573900006,11.6,-10.25625471));
#292300=CARTESIAN_POINT('Ctrl Pts',(-4.13870766600006,15.2,-10.259428784));
#292301=CARTESIAN_POINT('Ctrl Pts',(-4.13870766600006,11.6,-10.259428784));
#292302=CARTESIAN_POINT('Ctrl Pts',(-4.13876712900006,15.2,-10.262608063));
#292303=CARTESIAN_POINT('Ctrl Pts',(-4.13876712900006,11.6,-10.262608063));
#292304=CARTESIAN_POINT('Ctrl Pts',(-4.13882412400006,15.2,-10.265792539));
#292305=CARTESIAN_POINT('Ctrl Pts',(-4.13882412400006,11.6,-10.265792539));
#292306=CARTESIAN_POINT('Ctrl Pts',(-4.13887864300006,15.2,-10.268982202));
#292307=CARTESIAN_POINT('Ctrl Pts',(-4.13887864300006,11.6,-10.268982202));
#292308=CARTESIAN_POINT('Ctrl Pts',(-4.13893067800006,15.2,-10.272177045));
#292309=CARTESIAN_POINT('Ctrl Pts',(-4.13893067800006,11.6,-10.272177045));
#292310=CARTESIAN_POINT('Ctrl Pts',(-4.13898022300006,15.2,-10.275377057));
#292311=CARTESIAN_POINT('Ctrl Pts',(-4.13898022300006,11.6,-10.275377057));
#292312=CARTESIAN_POINT('Ctrl Pts',(-4.13902726900006,15.2,-10.278582232));
#292313=CARTESIAN_POINT('Ctrl Pts',(-4.13902726900006,11.6,-10.278582232));
#292314=CARTESIAN_POINT('Ctrl Pts',(-4.13907181100006,15.2,-10.28179256));
#292315=CARTESIAN_POINT('Ctrl Pts',(-4.13907181100006,11.6,-10.28179256));
#292316=CARTESIAN_POINT('Ctrl Pts',(-4.13911384100006,15.2,-10.28500803));
#292317=CARTESIAN_POINT('Ctrl Pts',(-4.13911384100006,11.6,-10.28500803));
#292318=CARTESIAN_POINT('Ctrl Pts',(-4.13915335200006,15.2,-10.288228637));
#292319=CARTESIAN_POINT('Ctrl Pts',(-4.13915335200006,11.6,-10.288228637));
#292320=CARTESIAN_POINT('Ctrl Pts',(-4.13919033700005,15.2,-10.291454371));
#292321=CARTESIAN_POINT('Ctrl Pts',(-4.13919033700005,11.6,-10.291454371));
#292322=CARTESIAN_POINT('Ctrl Pts',(-4.13922478800006,15.2,-10.294685224));
#292323=CARTESIAN_POINT('Ctrl Pts',(-4.13922478800006,11.6,-10.294685224));
#292324=CARTESIAN_POINT('Ctrl Pts',(-4.13925670000006,15.2,-10.297921185));
#292325=CARTESIAN_POINT('Ctrl Pts',(-4.13925670000006,11.6,-10.297921185));
#292326=CARTESIAN_POINT('Ctrl Pts',(-4.13928606500006,15.2,-10.301162248));
#292327=CARTESIAN_POINT('Ctrl Pts',(-4.13928606500006,11.6,-10.301162248));
#292328=CARTESIAN_POINT('Ctrl Pts',(-4.13931287600006,15.2,-10.304408403));
#292329=CARTESIAN_POINT('Ctrl Pts',(-4.13931287600006,11.6,-10.304408403));
#292330=CARTESIAN_POINT('Ctrl Pts',(-4.13933712500006,15.2,-10.307659642));
#292331=CARTESIAN_POINT('Ctrl Pts',(-4.13933712500006,11.6,-10.307659642));
#292332=CARTESIAN_POINT('Ctrl Pts',(-4.13935880700006,15.2,-10.310915957));
#292333=CARTESIAN_POINT('Ctrl Pts',(-4.13935880700006,11.6,-10.310915957));
#292334=CARTESIAN_POINT('Ctrl Pts',(-4.13937791400006,15.2,-10.314177337));
#292335=CARTESIAN_POINT('Ctrl Pts',(-4.13937791400006,11.6,-10.314177337));
#292336=CARTESIAN_POINT('Ctrl Pts',(-4.13939443900006,15.2,-10.317443776));
#292337=CARTESIAN_POINT('Ctrl Pts',(-4.13939443900006,11.6,-10.317443776));
#292338=CARTESIAN_POINT('Ctrl Pts',(-4.13940837600006,15.2,-10.320715266));
#292339=CARTESIAN_POINT('Ctrl Pts',(-4.13940837600006,11.6,-10.320715266));
#292340=CARTESIAN_POINT('Ctrl Pts',(-4.13941971700006,15.2,-10.323991796));
#292341=CARTESIAN_POINT('Ctrl Pts',(-4.13941971700006,11.6,-10.323991796));
#292342=CARTESIAN_POINT('Ctrl Pts',(-4.13942845700006,15.2,-10.327273358));
#292343=CARTESIAN_POINT('Ctrl Pts',(-4.13942845700006,11.6,-10.327273358));
#292344=CARTESIAN_POINT('Ctrl Pts',(-4.13943458800006,15.2,-10.330559945));
#292345=CARTESIAN_POINT('Ctrl Pts',(-4.13943458800006,11.6,-10.330559945));
#292346=CARTESIAN_POINT('Ctrl Pts',(-4.13943810200006,15.2,-10.333851548));
#292347=CARTESIAN_POINT('Ctrl Pts',(-4.13943810200006,11.6,-10.333851548));
#292348=CARTESIAN_POINT('Ctrl Pts',(-4.13943899400006,15.2,-10.337148156));
#292349=CARTESIAN_POINT('Ctrl Pts',(-4.13943899400006,11.6,-10.337148156));
#292350=CARTESIAN_POINT('Ctrl Pts',(-4.13943725800006,15.2,-10.340449765));
#292351=CARTESIAN_POINT('Ctrl Pts',(-4.13943725800006,11.6,-10.340449765));
#292352=CARTESIAN_POINT('Ctrl Pts',(-4.13943288500006,15.2,-10.343756364));
#292353=CARTESIAN_POINT('Ctrl Pts',(-4.13943288500006,11.6,-10.343756364));
#292354=CARTESIAN_POINT('Ctrl Pts',(-4.13942587000006,15.2,-10.347067944));
#292355=CARTESIAN_POINT('Ctrl Pts',(-4.13942587000006,11.6,-10.347067944));
#292356=CARTESIAN_POINT('Ctrl Pts',(-4.13941620600006,15.2,-10.350384497));
#292357=CARTESIAN_POINT('Ctrl Pts',(-4.13941620600006,11.6,-10.350384497));
#292358=CARTESIAN_POINT('Ctrl Pts',(-4.13940388500006,15.2,-10.353706015));
#292359=CARTESIAN_POINT('Ctrl Pts',(-4.13940388500006,11.6,-10.353706015));
#292360=CARTESIAN_POINT('Ctrl Pts',(-4.13938890200006,15.2,-10.357032491));
#292361=CARTESIAN_POINT('Ctrl Pts',(-4.13938890200006,11.6,-10.357032491));
#292362=CARTESIAN_POINT('Ctrl Pts',(-4.13937125000006,15.2,-10.360363914));
#292363=CARTESIAN_POINT('Ctrl Pts',(-4.13937125000006,11.6,-10.360363914));
#292364=CARTESIAN_POINT('Ctrl Pts',(-4.13935092200005,15.2,-10.363700277));
#292365=CARTESIAN_POINT('Ctrl Pts',(-4.13935092200005,11.6,-10.363700277));
#292366=CARTESIAN_POINT('Ctrl Pts',(-4.13932791200006,15.2,-10.367041572));
#292367=CARTESIAN_POINT('Ctrl Pts',(-4.13932791200006,11.6,-10.367041572));
#292368=CARTESIAN_POINT('Ctrl Pts',(-4.13930221300006,15.2,-10.370387789));
#292369=CARTESIAN_POINT('Ctrl Pts',(-4.13930221300006,11.6,-10.370387789));
#292370=CARTESIAN_POINT('Ctrl Pts',(-4.13927381800006,15.2,-10.373738921));
#292371=CARTESIAN_POINT('Ctrl Pts',(-4.13927381800006,11.6,-10.373738921));
#292372=CARTESIAN_POINT('Ctrl Pts',(-4.13924272200005,15.2,-10.37709496));
#292373=CARTESIAN_POINT('Ctrl Pts',(-4.13924272200005,11.6,-10.37709496));
#292374=CARTESIAN_POINT('Ctrl Pts',(-4.13920891800006,15.2,-10.380455896));
#292375=CARTESIAN_POINT('Ctrl Pts',(-4.13920891800006,11.6,-10.380455896));
#292376=CARTESIAN_POINT('Ctrl Pts',(-4.13917239900006,15.2,-10.383821723));
#292377=CARTESIAN_POINT('Ctrl Pts',(-4.13917239900006,11.6,-10.383821723));
#292378=CARTESIAN_POINT('Ctrl Pts',(-4.13913315700006,15.2,-10.38719243));
#292379=CARTESIAN_POINT('Ctrl Pts',(-4.13913315700006,11.6,-10.38719243));
#292380=CARTESIAN_POINT('Ctrl Pts',(-4.13909119000006,15.2,-10.390568011));
#292381=CARTESIAN_POINT('Ctrl Pts',(-4.13909119000006,11.6,-10.390568011));
#292382=CARTESIAN_POINT('Ctrl Pts',(-4.13904648600006,15.2,-10.393948456));
#292383=CARTESIAN_POINT('Ctrl Pts',(-4.13904648600006,11.6,-10.393948456));
#292384=CARTESIAN_POINT('Ctrl Pts',(-4.13899904400005,15.2,-10.397333758));
#292385=CARTESIAN_POINT('Ctrl Pts',(-4.13899904400005,11.6,-10.397333758));
#292386=CARTESIAN_POINT('Ctrl Pts',(-4.13894885300006,15.2,-10.400723908));
#292387=CARTESIAN_POINT('Ctrl Pts',(-4.13894885300006,11.6,-10.400723908));
#292388=CARTESIAN_POINT('Ctrl Pts',(-4.13889591000006,15.2,-10.404118899));
#292389=CARTESIAN_POINT('Ctrl Pts',(-4.13889591000006,11.6,-10.404118899));
#292390=CARTESIAN_POINT('Ctrl Pts',(-4.13884020700006,15.2,-10.407518722));
#292391=CARTESIAN_POINT('Ctrl Pts',(-4.13884020700006,11.6,-10.407518722));
#292392=CARTESIAN_POINT('Ctrl Pts',(-4.13878173800006,15.2,-10.410923367));
#292393=CARTESIAN_POINT('Ctrl Pts',(-4.13878173800006,11.6,-10.410923367));
#292394=CARTESIAN_POINT('Ctrl Pts',(-4.13872049700006,15.2,-10.414332828));
#292395=CARTESIAN_POINT('Ctrl Pts',(-4.13872049700006,11.6,-10.414332828));
#292396=CARTESIAN_POINT('Ctrl Pts',(-4.13865647700006,15.2,-10.417747096));
#292397=CARTESIAN_POINT('Ctrl Pts',(-4.13865647700006,11.6,-10.417747096));
#292398=CARTESIAN_POINT('Ctrl Pts',(-4.13858967300006,15.2,-10.421166163));
#292399=CARTESIAN_POINT('Ctrl Pts',(-4.13858967300006,11.6,-10.421166163));
#292400=CARTESIAN_POINT('Ctrl Pts',(-4.13852007700005,15.2,-10.424590021));
#292401=CARTESIAN_POINT('Ctrl Pts',(-4.13852007700005,11.6,-10.424590021));
#292402=CARTESIAN_POINT('Ctrl Pts',(-4.13844768400006,15.2,-10.428018661));
#292403=CARTESIAN_POINT('Ctrl Pts',(-4.13844768400006,11.6,-10.428018661));
#292404=CARTESIAN_POINT('Ctrl Pts',(-4.13837248800006,15.2,-10.431452076));
#292405=CARTESIAN_POINT('Ctrl Pts',(-4.13837248800006,11.6,-10.431452076));
#292406=CARTESIAN_POINT('Ctrl Pts',(-4.13829448200006,15.2,-10.434890257));
#292407=CARTESIAN_POINT('Ctrl Pts',(-4.13829448200006,11.6,-10.434890257));
#292408=CARTESIAN_POINT('Ctrl Pts',(-4.13821365900006,15.2,-10.438333197));
#292409=CARTESIAN_POINT('Ctrl Pts',(-4.13821365900006,11.6,-10.438333197));
#292410=CARTESIAN_POINT('Ctrl Pts',(-4.13813001600006,15.2,-10.441780886));
#292411=CARTESIAN_POINT('Ctrl Pts',(-4.13813001600006,11.6,-10.441780886));
#292412=CARTESIAN_POINT('Ctrl Pts',(-4.13804354400006,15.2,-10.445233317));
#292413=CARTESIAN_POINT('Ctrl Pts',(-4.13804354400006,11.6,-10.445233317));
#292414=CARTESIAN_POINT('Ctrl Pts',(-4.13795423700006,15.2,-10.448690482));
#292415=CARTESIAN_POINT('Ctrl Pts',(-4.13795423700006,11.6,-10.448690482));
#292416=CARTESIAN_POINT('Ctrl Pts',(-4.13786209100006,15.2,-10.452152372));
#292417=CARTESIAN_POINT('Ctrl Pts',(-4.13786209100006,11.6,-10.452152372));
#292418=CARTESIAN_POINT('Ctrl Pts',(-4.13776709800006,15.2,-10.45561898));
#292419=CARTESIAN_POINT('Ctrl Pts',(-4.13776709800006,11.6,-10.45561898));
#292420=CARTESIAN_POINT('Ctrl Pts',(-4.13766925200005,15.2,-10.459090298));
#292421=CARTESIAN_POINT('Ctrl Pts',(-4.13766925200005,11.6,-10.459090298));
#292422=CARTESIAN_POINT('Ctrl Pts',(-4.13756854800006,15.2,-10.462566317));
#292423=CARTESIAN_POINT('Ctrl Pts',(-4.13756854800006,11.6,-10.462566317));
#292424=CARTESIAN_POINT('Ctrl Pts',(-4.13746498000005,15.2,-10.466047029));
#292425=CARTESIAN_POINT('Ctrl Pts',(-4.13746498000005,11.6,-10.466047029));
#292426=CARTESIAN_POINT('Ctrl Pts',(-4.13735854100006,15.2,-10.469532426));
#292427=CARTESIAN_POINT('Ctrl Pts',(-4.13735854100006,11.6,-10.469532426));
#292428=CARTESIAN_POINT('Ctrl Pts',(-4.13724922400006,15.2,-10.473022501));
#292429=CARTESIAN_POINT('Ctrl Pts',(-4.13724922400006,11.6,-10.473022501));
#292430=CARTESIAN_POINT('Ctrl Pts',(-4.13713702600006,15.2,-10.476517244));
#292431=CARTESIAN_POINT('Ctrl Pts',(-4.13713702600006,11.6,-10.476517244));
#292432=CARTESIAN_POINT('Ctrl Pts',(-4.13702193900006,15.2,-10.480016649));
#292433=CARTESIAN_POINT('Ctrl Pts',(-4.13702193900006,11.6,-10.480016649));
#292434=CARTESIAN_POINT('Ctrl Pts',(-4.13690395800006,15.2,-10.483520708));
#292435=CARTESIAN_POINT('Ctrl Pts',(-4.13690395800006,11.6,-10.483520708));
#292436=CARTESIAN_POINT('Ctrl Pts',(-4.13678307500006,15.2,-10.487029411));
#292437=CARTESIAN_POINT('Ctrl Pts',(-4.13678307500006,11.6,-10.487029411));
#292438=CARTESIAN_POINT('Ctrl Pts',(-4.13665928800006,15.2,-10.490542752));
#292439=CARTESIAN_POINT('Ctrl Pts',(-4.13665928800006,11.6,-10.490542752));
#292440=CARTESIAN_POINT('Ctrl Pts',(-4.13653258700006,15.2,-10.494060721));
#292441=CARTESIAN_POINT('Ctrl Pts',(-4.13653258700006,11.6,-10.494060721));
#292442=CARTESIAN_POINT('Ctrl Pts',(-4.13640296900006,15.2,-10.497583313));
#292443=CARTESIAN_POINT('Ctrl Pts',(-4.13640296900006,11.6,-10.497583313));
#292444=CARTESIAN_POINT('Ctrl Pts',(-4.13627042600006,15.2,-10.501110517));
#292445=CARTESIAN_POINT('Ctrl Pts',(-4.13627042600006,11.6,-10.501110517));
#292446=CARTESIAN_POINT('Ctrl Pts',(-4.13613495400006,15.2,-10.504642327));
#292447=CARTESIAN_POINT('Ctrl Pts',(-4.13613495400006,11.6,-10.504642327));
#292448=CARTESIAN_POINT('Ctrl Pts',(-4.13599654700006,15.2,-10.508178734));
#292449=CARTESIAN_POINT('Ctrl Pts',(-4.13599654700006,11.6,-10.508178734));
#292450=CARTESIAN_POINT('Ctrl Pts',(-4.13585519800006,15.2,-10.51171973));
#292451=CARTESIAN_POINT('Ctrl Pts',(-4.13585519800006,11.6,-10.51171973));
#292452=CARTESIAN_POINT('Ctrl Pts',(-4.13571090200006,15.2,-10.515265307));
#292453=CARTESIAN_POINT('Ctrl Pts',(-4.13571090200006,11.6,-10.515265307));
#292454=CARTESIAN_POINT('Ctrl Pts',(-4.13556365200006,15.2,-10.518815459));
#292455=CARTESIAN_POINT('Ctrl Pts',(-4.13556365200006,11.6,-10.518815459));
#292456=CARTESIAN_POINT('Ctrl Pts',(-4.13541344500006,15.2,-10.522370176));
#292457=CARTESIAN_POINT('Ctrl Pts',(-4.13541344500006,11.6,-10.522370176));
#292458=CARTESIAN_POINT('Ctrl Pts',(-4.13526027300006,15.2,-10.525929452));
#292459=CARTESIAN_POINT('Ctrl Pts',(-4.13526027300006,11.6,-10.525929452));
#292460=CARTESIAN_POINT('Ctrl Pts',(-4.13510413100005,15.2,-10.529493276));
#292461=CARTESIAN_POINT('Ctrl Pts',(-4.13510413100005,11.6,-10.529493276));
#292462=CARTESIAN_POINT('Ctrl Pts',(-4.13494501300006,15.2,-10.533061643));
#292463=CARTESIAN_POINT('Ctrl Pts',(-4.13494501300006,11.6,-10.533061643));
#292464=CARTESIAN_POINT('Ctrl Pts',(-4.13478291300006,15.2,-10.536634544));
#292465=CARTESIAN_POINT('Ctrl Pts',(-4.13478291300006,11.6,-10.536634544));
#292466=CARTESIAN_POINT('Ctrl Pts',(-4.13461782600006,15.2,-10.540211971));
#292467=CARTESIAN_POINT('Ctrl Pts',(-4.13461782600006,11.6,-10.540211971));
#292468=CARTESIAN_POINT('Ctrl Pts',(-4.13444974700006,15.2,-10.543793918));
#292469=CARTESIAN_POINT('Ctrl Pts',(-4.13444974700006,11.6,-10.543793918));
#292470=CARTESIAN_POINT('Ctrl Pts',(-4.13427866800006,15.2,-10.547380374));
#292471=CARTESIAN_POINT('Ctrl Pts',(-4.13427866800006,11.6,-10.547380374));
#292472=CARTESIAN_POINT('Ctrl Pts',(-4.13410458600006,15.2,-10.550971334));
#292473=CARTESIAN_POINT('Ctrl Pts',(-4.13410458600006,11.6,-10.550971334));
#292474=CARTESIAN_POINT('Ctrl Pts',(-4.13392749300006,15.2,-10.554566788));
#292475=CARTESIAN_POINT('Ctrl Pts',(-4.13392749300006,11.6,-10.554566788));
#292476=CARTESIAN_POINT('Ctrl Pts',(-4.13374738600006,15.2,-10.558166729));
#292477=CARTESIAN_POINT('Ctrl Pts',(-4.13374738600006,11.6,-10.558166729));
#292478=CARTESIAN_POINT('Ctrl Pts',(-4.13356425900006,15.2,-10.561771151));
#292479=CARTESIAN_POINT('Ctrl Pts',(-4.13356425900006,11.6,-10.561771151));
#292480=CARTESIAN_POINT('Ctrl Pts',(-4.13337810400006,15.2,-10.565380043));
#292481=CARTESIAN_POINT('Ctrl Pts',(-4.13337810400006,11.6,-10.565380043));
#292482=CARTESIAN_POINT('Ctrl Pts',(-4.13318891700006,15.2,-10.568993399));
#292483=CARTESIAN_POINT('Ctrl Pts',(-4.13318891700006,11.6,-10.568993399));
#292484=CARTESIAN_POINT('Ctrl Pts',(-4.13299669400006,15.2,-10.572611212));
#292485=CARTESIAN_POINT('Ctrl Pts',(-4.13299669400006,11.6,-10.572611212));
#292486=CARTESIAN_POINT('Ctrl Pts',(-4.13280142700006,15.2,-10.576233472));
#292487=CARTESIAN_POINT('Ctrl Pts',(-4.13280142700006,11.6,-10.576233472));
#292488=CARTESIAN_POINT('Ctrl Pts',(-4.13260311100006,15.2,-10.579860172));
#292489=CARTESIAN_POINT('Ctrl Pts',(-4.13260311100006,11.6,-10.579860172));
#292490=CARTESIAN_POINT('Ctrl Pts',(-4.13240174200006,15.2,-10.583491306));
#292491=CARTESIAN_POINT('Ctrl Pts',(-4.13240174200006,11.6,-10.583491306));
#292492=CARTESIAN_POINT('Ctrl Pts',(-4.13219731300006,15.2,-10.587126866));
#292493=CARTESIAN_POINT('Ctrl Pts',(-4.13219731300006,11.6,-10.587126866));
#292494=CARTESIAN_POINT('Ctrl Pts',(-4.13198981900006,15.2,-10.590766842));
#292495=CARTESIAN_POINT('Ctrl Pts',(-4.13198981900006,11.6,-10.590766842));
#292496=CARTESIAN_POINT('Ctrl Pts',(-4.13177925500006,15.2,-10.594411227));
#292497=CARTESIAN_POINT('Ctrl Pts',(-4.13177925500006,11.6,-10.594411227));
#292498=CARTESIAN_POINT('Ctrl Pts',(-4.13156561600006,15.2,-10.598060015));
#292499=CARTESIAN_POINT('Ctrl Pts',(-4.13156561600006,11.6,-10.598060015));
#292500=CARTESIAN_POINT('Ctrl Pts',(-4.13134889500006,15.2,-10.601713197));
#292501=CARTESIAN_POINT('Ctrl Pts',(-4.13134889500006,11.6,-10.601713197));
#292502=CARTESIAN_POINT('Ctrl Pts',(-4.13112908800006,15.2,-10.605370765));
#292503=CARTESIAN_POINT('Ctrl Pts',(-4.13112908800006,11.6,-10.605370765));
#292504=CARTESIAN_POINT('Ctrl Pts',(-4.13090618900006,15.2,-10.609032712));
#292505=CARTESIAN_POINT('Ctrl Pts',(-4.13090618900006,11.6,-10.609032712));
#292506=CARTESIAN_POINT('Ctrl Pts',(-4.13068019400006,15.2,-10.61269903));
#292507=CARTESIAN_POINT('Ctrl Pts',(-4.13068019400006,11.6,-10.61269903));
#292508=CARTESIAN_POINT('Ctrl Pts',(-4.13045109500006,15.2,-10.616369712));
#292509=CARTESIAN_POINT('Ctrl Pts',(-4.13045109500006,11.6,-10.616369712));
#292510=CARTESIAN_POINT('Ctrl Pts',(-4.13021888800006,15.2,-10.62004475));
#292511=CARTESIAN_POINT('Ctrl Pts',(-4.13021888800006,11.6,-10.62004475));
#292512=CARTESIAN_POINT('Ctrl Pts',(-4.12998356800006,15.2,-10.623724135));
#292513=CARTESIAN_POINT('Ctrl Pts',(-4.12998356800006,11.6,-10.623724135));
#292514=CARTESIAN_POINT('Ctrl Pts',(-4.12974513000006,15.2,-10.627407861));
#292515=CARTESIAN_POINT('Ctrl Pts',(-4.12974513000006,11.6,-10.627407861));
#292516=CARTESIAN_POINT('Ctrl Pts',(-4.12950356800006,15.2,-10.63109592));
#292517=CARTESIAN_POINT('Ctrl Pts',(-4.12950356800006,11.6,-10.63109592));
#292518=CARTESIAN_POINT('Ctrl Pts',(-4.12925887700006,15.2,-10.634788304));
#292519=CARTESIAN_POINT('Ctrl Pts',(-4.12925887700006,11.6,-10.634788304));
#292520=CARTESIAN_POINT('Ctrl Pts',(-4.12901105200006,15.2,-10.638485006));
#292521=CARTESIAN_POINT('Ctrl Pts',(-4.12901105200006,11.6,-10.638485006));
#292522=CARTESIAN_POINT('Ctrl Pts',(-4.12876008700006,15.2,-10.642186017));
#292523=CARTESIAN_POINT('Ctrl Pts',(-4.12876008700006,11.6,-10.642186017));
#292524=CARTESIAN_POINT('Ctrl Pts',(-4.12850597800006,15.2,-10.645891333));
#292525=CARTESIAN_POINT('Ctrl Pts',(-4.12850597800006,11.6,-10.645891333));
#292526=CARTESIAN_POINT('Ctrl Pts',(-4.12824872100006,15.2,-10.649600942));
#292527=CARTESIAN_POINT('Ctrl Pts',(-4.12824872100006,11.6,-10.649600942));
#292528=CARTESIAN_POINT('Ctrl Pts',(-4.12798830800006,15.2,-10.65331484));
#292529=CARTESIAN_POINT('Ctrl Pts',(-4.12798830800006,11.6,-10.65331484));
#292530=CARTESIAN_POINT('Ctrl Pts',(-4.12772473400006,15.2,-10.657033017));
#292531=CARTESIAN_POINT('Ctrl Pts',(-4.12772473400006,11.6,-10.657033017));
#292532=CARTESIAN_POINT('Ctrl Pts',(-4.12745799500006,15.2,-10.660755466));
#292533=CARTESIAN_POINT('Ctrl Pts',(-4.12745799500006,11.6,-10.660755466));
#292534=CARTESIAN_POINT('Ctrl Pts',(-4.12718808600006,15.2,-10.664482179));
#292535=CARTESIAN_POINT('Ctrl Pts',(-4.12718808600006,11.6,-10.664482179));
#292536=CARTESIAN_POINT('Ctrl Pts',(-4.12691499900006,15.2,-10.668213148));
#292537=CARTESIAN_POINT('Ctrl Pts',(-4.12691499900006,11.6,-10.668213148));
#292538=CARTESIAN_POINT('Ctrl Pts',(-4.12663873100006,15.2,-10.671948366));
#292539=CARTESIAN_POINT('Ctrl Pts',(-4.12663873100006,11.6,-10.671948366));
#292540=CARTESIAN_POINT('Ctrl Pts',(-4.12635927800006,15.2,-10.675687825));
#292541=CARTESIAN_POINT('Ctrl Pts',(-4.12635927800006,11.6,-10.675687825));
#292542=CARTESIAN_POINT('Ctrl Pts',(-4.12607663400006,15.2,-10.67943152));
#292543=CARTESIAN_POINT('Ctrl Pts',(-4.12607663400006,11.6,-10.67943152));
#292544=CARTESIAN_POINT('Ctrl Pts',(-4.12579079500006,15.2,-10.683179442));
#292545=CARTESIAN_POINT('Ctrl Pts',(-4.12579079500006,11.6,-10.683179442));
#292546=CARTESIAN_POINT('Ctrl Pts',(-4.12550175600006,15.2,-10.686931586));
#292547=CARTESIAN_POINT('Ctrl Pts',(-4.12550175600006,11.6,-10.686931586));
#292548=CARTESIAN_POINT('Ctrl Pts',(-4.12520951300006,15.2,-10.690687943));
#292549=CARTESIAN_POINT('Ctrl Pts',(-4.12520951300006,11.6,-10.690687943));
#292550=CARTESIAN_POINT('Ctrl Pts',(-4.12491405900006,15.2,-10.694448508));
#292551=CARTESIAN_POINT('Ctrl Pts',(-4.12491405900006,11.6,-10.694448508));
#292552=CARTESIAN_POINT('Ctrl Pts',(-4.12461539100006,15.2,-10.698213269));
#292553=CARTESIAN_POINT('Ctrl Pts',(-4.12461539100006,11.6,-10.698213269));
#292554=CARTESIAN_POINT('Ctrl Pts',(-4.12431350000006,15.2,-10.701982219));
#292555=CARTESIAN_POINT('Ctrl Pts',(-4.12431350000006,11.6,-10.701982219));
#292556=CARTESIAN_POINT('Ctrl Pts',(-4.12400838200006,15.2,-10.705755349));
#292557=CARTESIAN_POINT('Ctrl Pts',(-4.12400838200006,11.6,-10.705755349));
#292558=CARTESIAN_POINT('Ctrl Pts',(-4.12370002800006,15.2,-10.709532648));
#292559=CARTESIAN_POINT('Ctrl Pts',(-4.12370002800006,11.6,-10.709532648));
#292560=CARTESIAN_POINT('Ctrl Pts',(-4.12338843600006,15.2,-10.713314109));
#292561=CARTESIAN_POINT('Ctrl Pts',(-4.12338843600006,11.6,-10.713314109));
#292562=CARTESIAN_POINT('Ctrl Pts',(-4.12307360000006,15.2,-10.717099725));
#292563=CARTESIAN_POINT('Ctrl Pts',(-4.12307360000006,11.6,-10.717099725));
#292564=CARTESIAN_POINT('Ctrl Pts',(-4.12275551700006,15.2,-10.720889492));
#292565=CARTESIAN_POINT('Ctrl Pts',(-4.12275551700006,11.6,-10.720889492));
#292566=CARTESIAN_POINT('Ctrl Pts',(-4.12243418400006,15.2,-10.724683406));
#292567=CARTESIAN_POINT('Ctrl Pts',(-4.12243418400006,11.6,-10.724683406));
#292568=CARTESIAN_POINT('Ctrl Pts',(-4.12210960100006,15.2,-10.728481464));
#292569=CARTESIAN_POINT('Ctrl Pts',(-4.12210960100006,11.6,-10.728481464));
#292570=CARTESIAN_POINT('Ctrl Pts',(-4.12184733300006,15.2,-10.731523226));
#292571=CARTESIAN_POINT('Ctrl Pts',(-4.12184733300006,11.6,-10.731523226));
#292572=CARTESIAN_POINT('Ctrl Pts',(-4.12164917000006,15.2,-10.733806411));
#292573=CARTESIAN_POINT('Ctrl Pts',(-4.12164917000006,11.6,-10.733806411));
#292574=CARTESIAN_POINT('Ctrl Pts',(-4.12151641000006,15.2,-10.735329364));
#292575=CARTESIAN_POINT('Ctrl Pts',(-4.12151641000006,11.6,-10.735329364));
#292576=CARTESIAN_POINT('Ctrl Pts',(-4.12144986800006,15.2,-10.736091047));
#292577=CARTESIAN_POINT('Ctrl Pts',(-4.12144986800006,11.6,-10.736091047));
#292578=CARTESIAN_POINT('Ctrl Pts',(-4.04260911700006,15.2,-9.55499537100001));
#292579=CARTESIAN_POINT('Ctrl Pts',(-4.04316130262144,15.2,-9.55669455581129));
#292580=CARTESIAN_POINT('Ctrl Pts',(-4.04372605423532,15.2,-9.55844976611691));
#292581=CARTESIAN_POINT('Ctrl Pts',(-4.04430244636191,15.2,-9.56026027775997));
#292582=CARTESIAN_POINT('Ctrl Pts',(-4.04488161814269,15.2,-9.56207952060535));
#292583=CARTESIAN_POINT('Ctrl Pts',(-4.04547254558646,15.2,-9.56395460122364));
#292584=CARTESIAN_POINT('Ctrl Pts',(-4.04607433356661,15.2,-9.56588480617844));
#292585=CARTESIAN_POINT('Ctrl Pts',(-4.0466761214921,15.2,-9.56781501095792));
#292586=CARTESIAN_POINT('Ctrl Pts',(-4.047288768506,15.2,-9.5698003417657));
#292587=CARTESIAN_POINT('Ctrl Pts',(-4.04791140648337,15.2,-9.57184010177491));
#292588=CARTESIAN_POINT('Ctrl Pts',(-4.04853404446074,15.2,-9.57387986178411));
#292589=CARTESIAN_POINT('Ctrl Pts',(-4.04916667292143,15.1999999999999,
-9.57597405360779));
#292590=CARTESIAN_POINT('Ctrl Pts',(-4.04980844817965,15.2,-9.5781219995506));
#292591=CARTESIAN_POINT('Ctrl Pts',(-4.05045022349616,15.2,-9.58026994568851));
#292592=CARTESIAN_POINT('Ctrl Pts',(-4.05110114707708,15.2,-9.58247164586089));
#292593=CARTESIAN_POINT('Ctrl Pts',(-4.05176039953023,15.2,-9.5847264400707));
#292594=CARTESIAN_POINT('Ctrl Pts',(-4.0524196519235,15.2,-9.5869812340757));
#292595=CARTESIAN_POINT('Ctrl Pts',(-4.05308723483013,15.2,-9.58928912240923));
#292596=CARTESIAN_POINT('Ctrl Pts',(-4.05376235422535,15.2,-9.591649459501));
#292597=CARTESIAN_POINT('Ctrl Pts',(-4.05443747362059,15.2,-9.59400979659278));
#292598=CARTESIAN_POINT('Ctrl Pts',(-4.0551201277045,15.2,-9.59642258494927));
#292599=CARTESIAN_POINT('Ctrl Pts',(-4.05580954917917,15.2,-9.59888719110749));
#292600=CARTESIAN_POINT('Ctrl Pts',(-4.05649897071645,15.2,-9.60135179748957));
#292601=CARTESIAN_POINT('Ctrl Pts',(-4.05719515799624,15.2,-9.6038682244197));
#292602=CARTESIAN_POINT('Ctrl Pts',(-4.05789736261825,15.2,-9.60643585656314));
#292603=CARTESIAN_POINT('Ctrl Pts',(-4.05859956717648,15.2,-9.60900348847334));
#292604=CARTESIAN_POINT('Ctrl Pts',(-4.05930779063964,15.2,-9.61162232326542));
#292605=CARTESIAN_POINT('Ctrl Pts',(-4.06002130153062,15.2,-9.61429176142062));
#292606=CARTESIAN_POINT('Ctrl Pts',(-4.06073481242159,15.2,-9.61696119957584));
#292607=CARTESIAN_POINT('Ctrl Pts',(-4.06145361629545,15.2,-9.61968124038532));
#292608=CARTESIAN_POINT('Ctrl Pts',(-4.06217700018564,15.2,-9.62245129461584));
#292609=CARTESIAN_POINT('Ctrl Pts',(-4.06290038407583,15.2,-9.62522134884637));
#292610=CARTESIAN_POINT('Ctrl Pts',(-4.0636283523138,15.2,-9.6280414163698));
#292611=CARTESIAN_POINT('Ctrl Pts',(-4.06436021495361,15.2,-9.63091092167883));
#292612=CARTESIAN_POINT('Ctrl Pts',(-4.0650920776599,15.2,-9.63378042724854));
#292613=CARTESIAN_POINT('Ctrl Pts',(-4.06582783357492,15.2,-9.63669937083966));
#292614=CARTESIAN_POINT('Ctrl Pts',(-4.066566816532,15.2,-9.63966718542021));
#292615=CARTESIAN_POINT('Ctrl Pts',(-4.06730579942196,15.2,-9.64263499973116));
#292616=CARTESIAN_POINT('Ctrl Pts',(-4.06804800741506,15.2,-9.64565168660443));
#292617=CARTESIAN_POINT('Ctrl Pts',(-4.06879278847472,15.2,-9.64871669192355));
#292618=CARTESIAN_POINT('Ctrl Pts',(-4.06953756953436,15.2,-9.65178169724266));
#292619=CARTESIAN_POINT('Ctrl Pts',(-4.07028492545407,15.2,-9.65489502225683));
#292620=CARTESIAN_POINT('Ctrl Pts',(-4.07103421967672,15.2,-9.65805612363872));
#292621=CARTESIAN_POINT('Ctrl Pts',(-4.07178351396743,15.2,-9.66121722530775));
#292622=CARTESIAN_POINT('Ctrl Pts',(-4.07253474806667,15.2,-9.66442610292308));
#292623=CARTESIAN_POINT('Ctrl Pts',(-4.07328730227441,15.2,-9.66768222468592));
#292624=CARTESIAN_POINT('Ctrl Pts',(-4.07403985641379,15.2,-9.67093834615299));
#292625=CARTESIAN_POINT('Ctrl Pts',(-4.07479373164037,15.2,-9.67424171204671));
#292626=CARTESIAN_POINT('Ctrl Pts',(-4.07554832578305,15.2,-9.67759179952341));
#292627=CARTESIAN_POINT('Ctrl Pts',(-4.07630291992571,15.2,-9.68094188700013));
#292628=CARTESIAN_POINT('Ctrl Pts',(-4.07705823202017,15.2,-9.68433869613623));
#292629=CARTESIAN_POINT('Ctrl Pts',(-4.07781367540938,15.2,-9.68778171367465));
#292630=CARTESIAN_POINT('Ctrl Pts',(-4.07856911886721,15.2,-9.69122473152583));
#292631=CARTESIAN_POINT('Ctrl Pts',(-4.07932469262759,15.2,-9.69471395907011));
#292632=CARTESIAN_POINT('Ctrl Pts',(-4.08007982603977,15.2,-9.69824889127534));
#292633=CARTESIAN_POINT('Ctrl Pts',(-4.08083495938337,15.2,-9.70178382315949));
#292634=CARTESIAN_POINT('Ctrl Pts',(-4.08158965065244,15.2,-9.70536446190666));
#292635=CARTESIAN_POINT('Ctrl Pts',(-4.08234334204173,15.2,-9.70899030952492));
#292636=CARTESIAN_POINT('Ctrl Pts',(-4.0832226487082,15.2,-9.71322046529913));
#292637=CARTESIAN_POINT('Ctrl Pts',(-4.08410059079317,15.2,-9.7175121579116));
#292638=CARTESIAN_POINT('Ctrl Pts',(-4.08497631107267,15.2,-9.72186461460261));
#292639=CARTESIAN_POINT('Ctrl Pts',(-4.08572692841613,15.2,-9.72559529157269));
#292640=CARTESIAN_POINT('Ctrl Pts',(-4.08647590889386,15.2,-9.7293706133137));
#292641=CARTESIAN_POINT('Ctrl Pts',(-4.08722272453339,15.2,-9.73319010025826));
#292642=CARTESIAN_POINT('Ctrl Pts',(-4.08809400949141,15.2,-9.73764616859154));
#292643=CARTESIAN_POINT('Ctrl Pts',(-4.08896234769306,15.2,-9.74216235461556));
#292644=CARTESIAN_POINT('Ctrl Pts',(-4.08982691959674,15.2,-9.74673791065444));
#292645=CARTESIAN_POINT('Ctrl Pts',(-4.0904444709469,15.2,-9.75000616491704));
#292646=CARTESIAN_POINT('Ctrl Pts',(-4.09106010026381,15.2,-9.75330471188287));
#292647=CARTESIAN_POINT('Ctrl Pts',(-4.09167351588863,15.2,-9.75663328271865));
#292648=CARTESIAN_POINT('Ctrl Pts',(-4.09228693151345,15.2,-9.75996185355443));
#292649=CARTESIAN_POINT('Ctrl Pts',(-4.09289813542433,15.2,-9.76332045069072));
#292650=CARTESIAN_POINT('Ctrl Pts',(-4.09350683785468,15.2,-9.76670880819314));
#292651=CARTESIAN_POINT('Ctrl Pts',(-4.09411554021868,15.2,-9.77009716532623));
#292652=CARTESIAN_POINT('Ctrl Pts',(-4.09472174428668,15.2,-9.77351528533831));
#292653=CARTESIAN_POINT('Ctrl Pts',(-4.09532516672113,15.2,-9.77696290655733));
#292654=CARTESIAN_POINT('Ctrl Pts',(-4.09592858922136,15.2,-9.78041052815213));
#292655=CARTESIAN_POINT('Ctrl Pts',(-4.09652923228276,15.2,-9.78388765125482));
#292656=CARTESIAN_POINT('Ctrl Pts',(-4.09712681888023,15.2,-9.78739401805798));
#292657=CARTESIAN_POINT('Ctrl Pts',(-4.09784392283627,15.2,-9.7916016584511));
#292658=CARTESIAN_POINT('Ctrl Pts',(-4.0985566265532,15.2,-9.79585141337281));
#292659=CARTESIAN_POINT('Ctrl Pts',(-4.09926446254353,15.2,-9.80014284190685));
#292660=CARTESIAN_POINT('Ctrl Pts',(-4.09985432583665,15.2,-9.80371903215698));
#292661=CARTESIAN_POINT('Ctrl Pts',(-4.10044081003771,15.2,-9.80732416316734));
#292662=CARTESIAN_POINT('Ctrl Pts',(-4.1010236508013,15.2,-9.81095798497526));
#292663=CARTESIAN_POINT('Ctrl Pts',(-4.1016064915649,15.2,-9.81459180678317));
#292664=CARTESIAN_POINT('Ctrl Pts',(-4.10218568926452,15.2,-9.81825432077486));
#292665=CARTESIAN_POINT('Ctrl Pts',(-4.10276098183365,15.2,-9.82194527820773));
#292666=CARTESIAN_POINT('Ctrl Pts',(-4.10333627434006,15.2,-9.8256362352383));
#292667=CARTESIAN_POINT('Ctrl Pts',(-4.10390766522069,15.2,-9.82935563618167));
#292668=CARTESIAN_POINT('Ctrl Pts',(-4.1044748976592,15.2,-9.8331032367431));
#292669=CARTESIAN_POINT('Ctrl Pts',(-4.10504213015955,15.2,-9.83685083771302));
#292670=CARTESIAN_POINT('Ctrl Pts',(-4.10560520484884,15.2,-9.8406266399436));
#292671=CARTESIAN_POINT('Ctrl Pts',(-4.10616387221033,15.2,-9.84443040001075));
#292672=CARTESIAN_POINT('Ctrl Pts',(-4.1067225395718,15.2,-9.84823416007791));
#292673=CARTESIAN_POINT('Ctrl Pts',(-4.10727679784181,15.2,-9.85206587936669));
#292674=CARTESIAN_POINT('Ctrl Pts',(-4.10782640370292,15.2,-9.85592531879368));
#292675=CARTESIAN_POINT('Ctrl Pts',(-4.10859585192046,15.2,-9.86132853407562));
#292676=CARTESIAN_POINT('Ctrl Pts',(-4.10935617761061,15.2,-9.86678608025856));
#292677=CARTESIAN_POINT('Ctrl Pts',(-4.11010672452507,15.2,-9.87229731227494));
#292678=CARTESIAN_POINT('Ctrl Pts',(-4.11064282945563,15.2,-9.87623390651106));
#292679=CARTESIAN_POINT('Ctrl Pts',(-4.11117394296118,15.2,-9.88019789193882));
#292680=CARTESIAN_POINT('Ctrl Pts',(-4.11169983372507,15.2,-9.88418903471661));
#292681=CARTESIAN_POINT('Ctrl Pts',(-4.11222572448896,15.2,-9.88818017749438));
#292682=CARTESIAN_POINT('Ctrl Pts',(-4.11274638904247,15.2,-9.89219848073369));
#292683=CARTESIAN_POINT('Ctrl Pts',(-4.11326159751702,15.2,-9.89624371096049));
#292684=CARTESIAN_POINT('Ctrl Pts',(-4.11377680599157,15.2,-9.90028894118728));
#292685=CARTESIAN_POINT('Ctrl Pts',(-4.1142865584333,15.2,-9.90436110200566));
#292686=CARTESIAN_POINT('Ctrl Pts',(-4.11479062926633,15.2,-9.90845996228484));
#292687=CARTESIAN_POINT('Ctrl Pts',(-4.11529470009938,15.2,-9.91255882256402));
#292688=CARTESIAN_POINT('Ctrl Pts',(-4.11579308588255,15.2,-9.91668438523692));
#292689=CARTESIAN_POINT('Ctrl Pts',(-4.11628556754891,15.2,-9.92083642377998));
#292690=CARTESIAN_POINT('Ctrl Pts',(-4.11667955284979,15.2,-9.92415805434289));
#292691=CARTESIAN_POINT('Ctrl Pts',(-4.11706975713649,15.2,-9.92749663021293));
#292692=CARTESIAN_POINT('Ctrl Pts',(-4.11745606940233,15.2,-9.93085203627149));
#292693=CARTESIAN_POINT('Ctrl Pts',(-4.1178423817208,15.2,-9.93420744278723));
#292694=CARTESIAN_POINT('Ctrl Pts',(-4.11822480287172,15.2,-9.93757967973302));
#292695=CARTESIAN_POINT('Ctrl Pts',(-4.11860321978097,15.2,-9.94096863475215));
#292696=CARTESIAN_POINT('Ctrl Pts',(-4.11898163663866,15.2,-9.94435758930954));
#292697=CARTESIAN_POINT('Ctrl Pts',(-4.11935605002493,15.2,-9.94776326124409));
#292698=CARTESIAN_POINT('Ctrl Pts',(-4.11972635143953,15.2,-9.95118553840708));
#292699=CARTESIAN_POINT('Ctrl Pts',(-4.12009665290458,15.2,-9.95460781603635));
#292700=CARTESIAN_POINT('Ctrl Pts',(-4.1204628412873,15.2,-9.95804669827047));
#292701=CARTESIAN_POINT('Ctrl Pts',(-4.12082480947532,15.2,-9.9615020752523));
#292702=CARTESIAN_POINT('Ctrl Pts',(-4.12118677761402,15.2,-9.96495745176335));
#292703=CARTESIAN_POINT('Ctrl Pts',(-4.12154452473462,15.2,-9.96842932082201));
#292704=CARTESIAN_POINT('Ctrl Pts',(-4.12189794498395,15.2,-9.97191757397963));
#292705=CARTESIAN_POINT('Ctrl Pts',(-4.12225136528143,15.2,-9.97540582761253));
#292706=CARTESIAN_POINT('Ctrl Pts',(-4.12260045803685,15.2,-9.9789104647525));
#292707=CARTESIAN_POINT('Ctrl Pts',(-4.12294511950007,15.2,-9.98243137449994));
#292708=CARTESIAN_POINT('Ctrl Pts',(-4.1232897809633,15.2,-9.98595228424738));
#292709=CARTESIAN_POINT('Ctrl Pts',(-4.12363000999824,15.2,-9.9894894667106));
#292710=CARTESIAN_POINT('Ctrl Pts',(-4.12396570357162,15.2,-9.99304281507259));
#292711=CARTESIAN_POINT('Ctrl Pts',(-4.12430139709927,15.2,-9.99659616295044));
#292712=CARTESIAN_POINT('Ctrl Pts',(-4.12463255370282,15.2,-10.0001656746994));
#292713=CARTESIAN_POINT('Ctrl Pts',(-4.12495907323319,15.2,-10.0037512432558));
#292714=CARTESIAN_POINT('Ctrl Pts',(-4.12528559280803,15.2,-10.0073368123008));
#292715=CARTESIAN_POINT('Ctrl Pts',(-4.12560747311291,15.2,-10.0109384366482));
#292716=CARTESIAN_POINT('Ctrl Pts',(-4.12592461601859,15.2,-10.0145560116248));
#292717=CARTESIAN_POINT('Ctrl Pts',(-4.1263210446291,15.2,-10.019077980099));
#292718=CARTESIAN_POINT('Ctrl Pts',(-4.12671006683948,15.2,-10.0236248682959));
#292719=CARTESIAN_POINT('Ctrl Pts',(-4.1270914912833,15.2,-10.0281964693396));
#292720=CARTESIAN_POINT('Ctrl Pts',(-4.12739663081341,15.2,-10.0318537498756));
#292721=CARTESIAN_POINT('Ctrl Pts',(-4.1276969073921,15.2,-10.0355268451545));
#292722=CARTESIAN_POINT('Ctrl Pts',(-4.12799222175821,15.2,-10.0392156529808));
#292723=CARTESIAN_POINT('Ctrl Pts',(-4.12828753616455,15.2,-10.0429044613096));
#292724=CARTESIAN_POINT('Ctrl Pts',(-4.12857789011502,15.2,-10.0466089782455));
#292725=CARTESIAN_POINT('Ctrl Pts',(-4.12886318579672,15.2,-10.0503291026165));
#292726=CARTESIAN_POINT('Ctrl Pts',(-4.12921980537941,15.2,-10.0549792578269));
#292727=CARTESIAN_POINT('Ctrl Pts',(-4.12956852147862,15.2,-10.059653796857));
#292728=CARTESIAN_POINT('Ctrl Pts',(-4.12990914856129,15.2,-10.0643525163729));
#292729=CARTESIAN_POINT('Ctrl Pts',(-4.13018165020515,15.2,-10.0681114916783));
#292730=CARTESIAN_POINT('Ctrl Pts',(-4.13044897395067,15.2,-10.0718859438095));
#292731=CARTESIAN_POINT('Ctrl Pts',(-4.13071102754156,15.2,-10.075675767239));
#292732=CARTESIAN_POINT('Ctrl Pts',(-4.13097308116816,15.2,-10.079465591185));
#292733=CARTESIAN_POINT('Ctrl Pts',(-4.13122986381692,15.2,-10.0832707889315));
#292734=CARTESIAN_POINT('Ctrl Pts',(-4.13148128227451,15.2,-10.0870912561413));
#292735=CARTESIAN_POINT('Ctrl Pts',(-4.13173270069786,15.2,-10.0909117228305));
#292736=CARTESIAN_POINT('Ctrl Pts',(-4.13197875556911,15.2,-10.0947474600122));
#292737=CARTESIAN_POINT('Ctrl Pts',(-4.13221935527202,15.2,-10.0985983659186));
#292738=CARTESIAN_POINT('Ctrl Pts',(-4.13245995500772,15.2,-10.1024492723497));
#292739=CARTESIAN_POINT('Ctrl Pts',(-4.13269509902653,15.2,-10.1063153466676));
#292740=CARTESIAN_POINT('Ctrl Pts',(-4.13292469805003,15.2,-10.1101964892966));
#292741=CARTESIAN_POINT('Ctrl Pts',(-4.13315429704225,15.2,-10.1140776313967));
#292742=CARTESIAN_POINT('Ctrl Pts',(-4.1333783506441,15.2,-10.1179738397483));
#292743=CARTESIAN_POINT('Ctrl Pts',(-4.1335967685155,15.2,-10.1218850157054));
#292744=CARTESIAN_POINT('Ctrl Pts',(-4.13392439536725,15.2,-10.1277517804403));
#292745=CARTESIAN_POINT('Ctrl Pts',(-4.13423934470908,15.2,-10.1336522210044));
#292746=CARTESIAN_POINT('Ctrl Pts',(-4.13454131830799,15.2,-10.1395860016634));
#292747=CARTESIAN_POINT('Ctrl Pts',(-4.13474263401316,15.2,-10.1435418548971));
#292748=CARTESIAN_POINT('Ctrl Pts',(-4.13493818365069,15.2,-10.1475125246855));
#292749=CARTESIAN_POINT('Ctrl Pts',(-4.13512788002495,15.2,-10.1514979139889));
#292750=CARTESIAN_POINT('Ctrl Pts',(-4.13531757642506,15.2,-10.1554833038353));
#292751=CARTESIAN_POINT('Ctrl Pts',(-4.13550141920619,15.2,-10.1594834138944));
#292752=CARTESIAN_POINT('Ctrl Pts',(-4.13567932427083,15.2,-10.1634981426147));
#292753=CARTESIAN_POINT('Ctrl Pts',(-4.13590170558952,15.2,-10.1685165532416));
#292754=CARTESIAN_POINT('Ctrl Pts',(-4.1361148066386,15.2,-10.1735578111382));
#292755=CARTESIAN_POINT('Ctrl Pts',(-4.13631846552672,15.2,-10.1786217216957));
#292756=CARTESIAN_POINT('Ctrl Pts',(-4.13652212441483,15.2,-10.1836856322531));
#292757=CARTESIAN_POINT('Ctrl Pts',(-4.1367163409139,15.2,-10.1887721985553));
#292758=CARTESIAN_POINT('Ctrl Pts',(-4.13690095077422,15.2,-10.1938812298766));
#292759=CARTESIAN_POINT('Ctrl Pts',(-4.13704863865041,15.2,-10.1979684545994));
#292760=CARTESIAN_POINT('Ctrl Pts',(-4.13719018051875,15.2,-10.2020700570983));
#292761=CARTESIAN_POINT('Ctrl Pts',(-4.13732549300832,15.2,-10.2061859417805));
#292762=CARTESIAN_POINT('Ctrl Pts',(-4.13746080551633,15.2,-10.2103018270235));
#292763=CARTESIAN_POINT('Ctrl Pts',(-4.13758988962521,15.2,-10.2144319943503));
#292764=CARTESIAN_POINT('Ctrl Pts',(-4.13771266352015,15.2,-10.2185763482442));
#292765=CARTESIAN_POINT('Ctrl Pts',(-4.13786613088045,15.2,-10.2237567903293));
#292766=CARTESIAN_POINT('Ctrl Pts',(-4.13800973945726,15.2,-10.2289593978482));
#292767=CARTESIAN_POINT('Ctrl Pts',(-4.13814333348422,15.2,-10.2341839888917));
#292768=CARTESIAN_POINT('Ctrl Pts',(-4.13825020869705,15.2,-10.2383636613848));
#292769=CARTESIAN_POINT('Ctrl Pts',(-4.13835067542947,15.2,-10.242557400772));
#292770=CARTESIAN_POINT('Ctrl Pts',(-4.13844465453335,15.2,-10.2467651147804));
#292771=CARTESIAN_POINT('Ctrl Pts',(-4.13853863365003,15.2,-10.2509728293621));
#292772=CARTESIAN_POINT('Ctrl Pts',(-4.13862612423457,15.2,-10.2551945179324));
#292773=CARTESIAN_POINT('Ctrl Pts',(-4.13870705007164,15.2,-10.2594300859425));
#292774=CARTESIAN_POINT('Ctrl Pts',(-4.13880820736247,15.2,-10.2647245456665));
#292775=CARTESIAN_POINT('Ctrl Pts',(-4.13889910676701,15.2,-10.2700406936908));
#292776=CARTESIAN_POINT('Ctrl Pts',(-4.13897959829394,15.2,-10.2753783484148));
#292777=CARTESIAN_POINT('Ctrl Pts',(-4.13904399151022,15.2,-10.2796484718449));
#292778=CARTESIAN_POINT('Ctrl Pts',(-4.13910172399563,15.2,-10.2839323594289));
#292779=CARTESIAN_POINT('Ctrl Pts',(-4.13915272049171,15.2,-10.2882299187637));
#292780=CARTESIAN_POINT('Ctrl Pts',(-4.13920371699475,15.2,-10.2925274786841));
#292781=CARTESIAN_POINT('Ctrl Pts',(-4.13924797666319,15.2,-10.2968387104866));
#292782=CARTESIAN_POINT('Ctrl Pts',(-4.13928542649787,15.2,-10.3011635217237));
#292783=CARTESIAN_POINT('Ctrl Pts',(-4.13932287632744,15.2,-10.3054883323715));
#292784=CARTESIAN_POINT('Ctrl Pts',(-4.13935351456345,15.2,-10.3098267231787));
#292785=CARTESIAN_POINT('Ctrl Pts',(-4.13937726850641,15.2,-10.3141786013777));
#292786=CARTESIAN_POINT('Ctrl Pts',(-4.1394010224526,15.2,-10.3185304801695));
#292787=CARTESIAN_POINT('Ctrl Pts',(-4.13941789163994,15.2,-10.3228958492991));
#292788=CARTESIAN_POINT('Ctrl Pts',(-4.13942780475148,15.2,-10.3272746148687));
#292789=CARTESIAN_POINT('Ctrl Pts',(-4.13943771786167,15.2,-10.3316533798418));
#292790=CARTESIAN_POINT('Ctrl Pts',(-4.13944067222733,15.2,-10.3360455416287));
#292791=CARTESIAN_POINT('Ctrl Pts',(-4.13943659878368,15.2,-10.3404510121566));
#292792=CARTESIAN_POINT('Ctrl Pts',(-4.13943252533948,15.2,-10.3448564832847));
#292793=CARTESIAN_POINT('Ctrl Pts',(-4.13942142281665,15.2,-10.3492752595867));
#292794=CARTESIAN_POINT('Ctrl Pts',(-4.13940321948186,15.2,-10.3537072548291));
#292795=CARTESIAN_POINT('Ctrl Pts',(-4.13938046531462,15.2,-10.3592472485802));
#292796=CARTESIAN_POINT('Ctrl Pts',(-4.13934661818118,15.2,-10.3648078949844));
#292797=CARTESIAN_POINT('Ctrl Pts',(-4.13930153901148,15.2,-10.3703890183896));
#292798=CARTESIAN_POINT('Ctrl Pts',(-4.13927449151064,15.2,-10.3737376923111));
#292799=CARTESIAN_POINT('Ctrl Pts',(-4.13924340136193,15.2,-10.3770937384049));
#292800=CARTESIAN_POINT('Ctrl Pts',(-4.13920823923785,15.2,-10.380457119075));
#292801=CARTESIAN_POINT('Ctrl Pts',(-4.13917307711377,15.2,-10.3838204997451));
#292802=CARTESIAN_POINT('Ctrl Pts',(-4.13913384188185,15.2,-10.387191214856));
#292803=CARTESIAN_POINT('Ctrl Pts',(-4.13909050584175,15.2,-10.390569227025));
#292804=CARTESIAN_POINT('Ctrl Pts',(-4.13903272444971,15.2,-10.3950732436593));
#292805=CARTESIAN_POINT('Ctrl Pts',(-4.13896765145405,15.2,-10.3995902325396));
#292806=CARTESIAN_POINT('Ctrl Pts',(-4.13889522000491,15.2,-10.4041201077323));
#292807=CARTESIAN_POINT('Ctrl Pts',(-4.13884089642298,15.2,-10.4075175138181));
#292808=CARTESIAN_POINT('Ctrl Pts',(-4.13878243325593,15.2,-10.4109221665795));
#292809=CARTESIAN_POINT('Ctrl Pts',(-4.13871980225459,15.2,-10.4143340304185));
#292810=CARTESIAN_POINT('Ctrl Pts',(-4.13865717125326,15.2,-10.4177458942574));
#292811=CARTESIAN_POINT('Ctrl Pts',(-4.13859037269006,15.2,-10.4211649686807));
#292812=CARTESIAN_POINT('Ctrl Pts',(-4.13851937773394,15.2,-10.4245912168902));
#292813=CARTESIAN_POINT('Ctrl Pts',(-4.13844838277782,15.2,-10.4280174650997));
#292814=CARTESIAN_POINT('Ctrl Pts',(-4.1383731926972,15.2,-10.4314508870583));
#292815=CARTESIAN_POINT('Ctrl Pts',(-4.13829377778342,15.2,-10.434891446725));
#292816=CARTESIAN_POINT('Ctrl Pts',(-4.13821436286964,15.2,-10.4383320063916));
#292817=CARTESIAN_POINT('Ctrl Pts',(-4.13813072518937,15.2,-10.4417797029497));
#292818=CARTESIAN_POINT('Ctrl Pts',(-4.13804283527626,15.2,-10.4452345001152));
#292819=CARTESIAN_POINT('Ctrl Pts',(-4.13792564871481,15.2,-10.4498408967543));
#292820=CARTESIAN_POINT('Ctrl Pts',(-4.13780090476477,15.2,-10.45445991639));
#292821=CARTESIAN_POINT('Ctrl Pts',(-4.1376685374725,15.2,-10.4590914739304));
#292822=CARTESIAN_POINT('Ctrl Pts',(-4.13756926201232,15.2,-10.4625651417702));
#292823=CARTESIAN_POINT('Ctrl Pts',(-4.13746569993471,15.2,-10.4660458606897));
#292824=CARTESIAN_POINT('Ctrl Pts',(-4.13735782152159,15.2,-10.4695335958552));
#292825=CARTESIAN_POINT('Ctrl Pts',(-4.13724994310846,15.2,-10.4730213310208));
#292826=CARTESIAN_POINT('Ctrl Pts',(-4.13713775001252,15.2,-10.4765160813605));
#292827=CARTESIAN_POINT('Ctrl Pts',(-4.13702121547509,15.2,-10.4800178124833));
#292828=CARTESIAN_POINT('Ctrl Pts',(-4.13686583607773,15.2,-10.4846867877378));
#292829=CARTESIAN_POINT('Ctrl Pts',(-4.13670273763503,15.2,-10.4893681707659));
#292830=CARTESIAN_POINT('Ctrl Pts',(-4.13653185768048,15.2,-10.4940618774674));
#292831=CARTESIAN_POINT('Ctrl Pts',(-4.1364036977262,15.2,-10.4975821571738));
#292832=CARTESIAN_POINT('Ctrl Pts',(-4.13627116025926,15.2,-10.5011093691015));
#292833=CARTESIAN_POINT('Ctrl Pts',(-4.13613422021522,15.2,-10.5046434769421));
#292834=CARTESIAN_POINT('Ctrl Pts',(-4.13599728017117,15.2,-10.5081775847828));
#292835=CARTESIAN_POINT('Ctrl Pts',(-4.13585593692921,15.2,-10.5117185873984));
#292836=CARTESIAN_POINT('Ctrl Pts',(-4.13571016351746,15.2,-10.5152664511035));
#292837=CARTESIAN_POINT('Ctrl Pts',(-4.1355643901057,15.2,-10.5188143148085));
#292838=CARTESIAN_POINT('Ctrl Pts',(-4.13541418794447,15.2,-10.522369039846));
#292839=CARTESIAN_POINT('Ctrl Pts',(-4.13525953049176,15.2,-10.52593058905));
#292840=CARTESIAN_POINT('Ctrl Pts',(-4.13505332053607,15.2,-10.5306793217532));
#292841=CARTESIAN_POINT('Ctrl Pts',(-4.13483918934058,15.2,-10.5354401864218));
#292842=CARTESIAN_POINT('Ctrl Pts',(-4.13461707793877,15.2,-10.5402131017387));
#292843=CARTESIAN_POINT('Ctrl Pts',(-4.13445049440254,15.2,-10.5437927879012));
#292844=CARTESIAN_POINT('Ctrl Pts',(-4.13427942122489,15.2,-10.547379251755));
#292845=CARTESIAN_POINT('Ctrl Pts',(-4.13410383327254,15.2,-10.5509724579167));
#292846=CARTESIAN_POINT('Ctrl Pts',(-4.13392824532019,15.2,-10.5545656640784));
#292847=CARTESIAN_POINT('Ctrl Pts',(-4.1337481435274,15.2,-10.5581656123679));
#292848=CARTESIAN_POINT('Ctrl Pts',(-4.13356350203325,15.2,-10.5617722685449));
#292849=CARTESIAN_POINT('Ctrl Pts',(-4.1333788605391,15.2,-10.565378924722));
#292850=CARTESIAN_POINT('Ctrl Pts',(-4.13318967856075,15.2,-10.5689922880951));
#292851=CARTESIAN_POINT('Ctrl Pts',(-4.13299593302526,15.2,-10.5726123237717));
#292852=CARTESIAN_POINT('Ctrl Pts',(-4.13267302378771,15.2,-10.5786457167852));
#292853=CARTESIAN_POINT('Ctrl Pts',(-4.1323374338612,15.2,-10.5846976443278));
#292854=CARTESIAN_POINT('Ctrl Pts',(-4.13198905150009,15.2,-10.5907679442583));
#292855=CARTESIAN_POINT('Ctrl Pts',(-4.13171034559601,15.2,-10.5956241844674));
#292856=CARTESIAN_POINT('Ctrl Pts',(-4.13142345287431,15.2,-10.600492184439));
#292857=CARTESIAN_POINT('Ctrl Pts',(-4.1311283149685,15.2,-10.6053718605395));
#292858=CARTESIAN_POINT('Ctrl Pts',(-4.13090696155924,15.2,-10.6090316172824));
#292859=CARTESIAN_POINT('Ctrl Pts',(-4.13068097132577,15.2,-10.6126979423598));
#292860=CARTESIAN_POINT('Ctrl Pts',(-4.13045031794709,15.2,-10.6163708017023));
#292861=CARTESIAN_POINT('Ctrl Pts',(-4.1302196645684,15.2,-10.6200436610448));
#292862=CARTESIAN_POINT('Ctrl Pts',(-4.12998434943221,15.2,-10.6237230529518));
#292863=CARTESIAN_POINT('Ctrl Pts',(-4.12974434898218,15.2,-10.6274089446518));
#292864=CARTESIAN_POINT('Ctrl Pts',(-4.12950434853216,15.2,-10.6310948363518));
#292865=CARTESIAN_POINT('Ctrl Pts',(-4.12925966242436,15.2,-10.6347872274677));
#292866=CARTESIAN_POINT('Ctrl Pts',(-4.12901026701676,15.2,-10.6384860832916));
#292867=CARTESIAN_POINT('Ctrl Pts',(-4.12859460798898,15.2,-10.6446508432222));
#292868=CARTESIAN_POINT('Ctrl Pts',(-4.12816587086856,15.2,-10.6508335643418));
#292869=CARTESIAN_POINT('Ctrl Pts',(-4.12772394274151,15.2,-10.657034084995));
#292870=CARTESIAN_POINT('Ctrl Pts',(-4.12745878587492,15.2,-10.6607543972518));
#292871=CARTESIAN_POINT('Ctrl Pts',(-4.12718888152492,15.2,-10.664481117482));
#292872=CARTESIAN_POINT('Ctrl Pts',(-4.126914203742,15.2,-10.6682142102382));
#292873=CARTESIAN_POINT('Ctrl Pts',(-4.12663952595909,15.2,-10.6719473029945));
#292874=CARTESIAN_POINT('Ctrl Pts',(-4.12636007713692,15.2,-10.6756867685951));
#292875=CARTESIAN_POINT('Ctrl Pts',(-4.12607583527266,15.2,-10.6794325763751));
#292876=CARTESIAN_POINT('Ctrl Pts',(-4.1257915934084,15.2,-10.6831783841551));
#292877=CARTESIAN_POINT('Ctrl Pts',(-4.12550255925281,15.2,-10.6869305339681));
#292878=CARTESIAN_POINT('Ctrl Pts',(-4.12520871034748,15.2,-10.6906889941223));
#292879=CARTESIAN_POINT('Ctrl Pts',(-4.12491486138876,15.2,-10.6944474549593));
#292880=CARTESIAN_POINT('Ctrl Pts',(-4.12461619822869,15.2,-10.6982122250898));
#292881=CARTESIAN_POINT('Ctrl Pts',(-4.12431269314226,15.2,-10.7019832648054));
#292882=CARTESIAN_POINT('Ctrl Pts',(-4.12400918811096,15.2,-10.7057543038359));
#292883=CARTESIAN_POINT('Ctrl Pts',(-4.12370083934428,15.2,-10.7095316104131));
#292884=CARTESIAN_POINT('Ctrl Pts',(-4.12338762496444,15.2,-10.713315148507));
#292885=CARTESIAN_POINT('Ctrl Pts',(-4.12307441058461,15.2,-10.717098686601));
#292886=CARTESIAN_POINT('Ctrl Pts',(-4.12275632951957,15.2,-10.7208884566915));
#292887=CARTESIAN_POINT('Ctrl Pts',(-4.12243337144829,15.2,-10.7246844424413));
#292888=CARTESIAN_POINT('Ctrl Pts',(-4.12211041337701,15.2,-10.7284804281911));
#292889=CARTESIAN_POINT('Ctrl Pts',(-4.1217825780605,15.2,-10.7322826313081));
#292890=CARTESIAN_POINT('Ctrl Pts',(-4.12144986800006,15.2,-10.736091047));
#292891=CARTESIAN_POINT('Ctrl Pts',(-4.04260911700006,12.2,-9.55499537100001));
#292892=CARTESIAN_POINT('Ctrl Pts',(-4.04316130262144,12.2,-9.55669455581129));
#292893=CARTESIAN_POINT('Ctrl Pts',(-4.04372605423532,12.2,-9.55844976611691));
#292894=CARTESIAN_POINT('Ctrl Pts',(-4.04430244636191,12.2,-9.56026027775997));
#292895=CARTESIAN_POINT('Ctrl Pts',(-4.04488161814269,12.2,-9.56207952060535));
#292896=CARTESIAN_POINT('Ctrl Pts',(-4.04547254558646,12.2,-9.56395460122364));
#292897=CARTESIAN_POINT('Ctrl Pts',(-4.04607433356661,12.2,-9.56588480617844));
#292898=CARTESIAN_POINT('Ctrl Pts',(-4.0466761214921,12.2,-9.56781501095792));
#292899=CARTESIAN_POINT('Ctrl Pts',(-4.047288768506,12.2,-9.5698003417657));
#292900=CARTESIAN_POINT('Ctrl Pts',(-4.04791140648337,12.2,-9.57184010177491));
#292901=CARTESIAN_POINT('Ctrl Pts',(-4.04853404446074,12.2,-9.57387986178411));
#292902=CARTESIAN_POINT('Ctrl Pts',(-4.04916667292143,12.2,-9.57597405360779));
#292903=CARTESIAN_POINT('Ctrl Pts',(-4.04980844817965,12.2,-9.5781219995506));
#292904=CARTESIAN_POINT('Ctrl Pts',(-4.05045022349616,12.2,-9.58026994568851));
#292905=CARTESIAN_POINT('Ctrl Pts',(-4.05110114707708,12.2,-9.58247164586089));
#292906=CARTESIAN_POINT('Ctrl Pts',(-4.05176039953023,12.2,-9.5847264400707));
#292907=CARTESIAN_POINT('Ctrl Pts',(-4.0524196519235,12.2,-9.5869812340757));
#292908=CARTESIAN_POINT('Ctrl Pts',(-4.05308723483013,12.2,-9.58928912240923));
#292909=CARTESIAN_POINT('Ctrl Pts',(-4.05376235422535,12.2,-9.591649459501));
#292910=CARTESIAN_POINT('Ctrl Pts',(-4.05443747362059,12.2,-9.59400979659278));
#292911=CARTESIAN_POINT('Ctrl Pts',(-4.0551201277045,12.2,-9.59642258494927));
#292912=CARTESIAN_POINT('Ctrl Pts',(-4.05580954917917,12.2,-9.59888719110749));
#292913=CARTESIAN_POINT('Ctrl Pts',(-4.05649897071645,12.2,-9.60135179748957));
#292914=CARTESIAN_POINT('Ctrl Pts',(-4.05719515799624,12.2,-9.6038682244197));
#292915=CARTESIAN_POINT('Ctrl Pts',(-4.05789736261825,12.2,-9.60643585656314));
#292916=CARTESIAN_POINT('Ctrl Pts',(-4.05859956717648,12.2,-9.60900348847334));
#292917=CARTESIAN_POINT('Ctrl Pts',(-4.05930779063965,12.2,-9.61162232326542));
#292918=CARTESIAN_POINT('Ctrl Pts',(-4.06002130153062,12.2,-9.61429176142063));
#292919=CARTESIAN_POINT('Ctrl Pts',(-4.0607348124216,12.2,-9.61696119957584));
#292920=CARTESIAN_POINT('Ctrl Pts',(-4.06145361629545,12.2,-9.61968124038532));
#292921=CARTESIAN_POINT('Ctrl Pts',(-4.06217700018564,12.2,-9.62245129461584));
#292922=CARTESIAN_POINT('Ctrl Pts',(-4.06290038407583,12.2,-9.62522134884637));
#292923=CARTESIAN_POINT('Ctrl Pts',(-4.0636283523138,12.2,-9.6280414163698));
#292924=CARTESIAN_POINT('Ctrl Pts',(-4.06436021495361,12.2,-9.63091092167883));
#292925=CARTESIAN_POINT('Ctrl Pts',(-4.0650920776599,12.2,-9.63378042724854));
#292926=CARTESIAN_POINT('Ctrl Pts',(-4.06582783357492,12.2,-9.63669937083967));
#292927=CARTESIAN_POINT('Ctrl Pts',(-4.066566816532,12.2,-9.63966718542021));
#292928=CARTESIAN_POINT('Ctrl Pts',(-4.06730579942196,12.2,-9.64263499973117));
#292929=CARTESIAN_POINT('Ctrl Pts',(-4.06804800741506,12.2,-9.64565168660443));
#292930=CARTESIAN_POINT('Ctrl Pts',(-4.06879278847471,12.2,-9.64871669192354));
#292931=CARTESIAN_POINT('Ctrl Pts',(-4.06953756953436,12.2,-9.65178169724265));
#292932=CARTESIAN_POINT('Ctrl Pts',(-4.07028492545407,12.2,-9.65489502225683));
#292933=CARTESIAN_POINT('Ctrl Pts',(-4.07103421967672,12.2,-9.65805612363872));
#292934=CARTESIAN_POINT('Ctrl Pts',(-4.07178351396743,12.2,-9.66121722530775));
#292935=CARTESIAN_POINT('Ctrl Pts',(-4.07253474806667,12.2,-9.66442610292308));
#292936=CARTESIAN_POINT('Ctrl Pts',(-4.07328730227441,12.2,-9.66768222468592));
#292937=CARTESIAN_POINT('Ctrl Pts',(-4.07403985641379,12.2,-9.67093834615299));
#292938=CARTESIAN_POINT('Ctrl Pts',(-4.07479373164037,12.2,-9.6742417120467));
#292939=CARTESIAN_POINT('Ctrl Pts',(-4.07554832578304,12.2,-9.6775917995234));
#292940=CARTESIAN_POINT('Ctrl Pts',(-4.07630291992571,12.2,-9.68094188700012));
#292941=CARTESIAN_POINT('Ctrl Pts',(-4.07705823202017,12.2,-9.68433869613623));
#292942=CARTESIAN_POINT('Ctrl Pts',(-4.07781367540938,12.2,-9.68778171367465));
#292943=CARTESIAN_POINT('Ctrl Pts',(-4.07856911886721,12.2,-9.69122473152582));
#292944=CARTESIAN_POINT('Ctrl Pts',(-4.07932469262759,12.2,-9.6947139590701));
#292945=CARTESIAN_POINT('Ctrl Pts',(-4.08007982603977,12.2,-9.69824889127533));
#292946=CARTESIAN_POINT('Ctrl Pts',(-4.08083495938336,12.2,-9.70178382315948));
#292947=CARTESIAN_POINT('Ctrl Pts',(-4.08158965065244,12.2,-9.70536446190665));
#292948=CARTESIAN_POINT('Ctrl Pts',(-4.08234334204172,12.2,-9.70899030952491));
#292949=CARTESIAN_POINT('Ctrl Pts',(-4.08309703343101,12.2,-9.71261615714318));
#292950=CARTESIAN_POINT('Ctrl Pts',(-4.08384972330873,12.2,-9.71628721520919));
#292951=CARTESIAN_POINT('Ctrl Pts',(-4.08460086890239,12.2,-9.72000299792392));
#292952=CARTESIAN_POINT('Ctrl Pts',(-4.08535201456428,12.2,-9.72371878097617));
#292953=CARTESIAN_POINT('Ctrl Pts',(-4.08610161511594,12.2,-9.72747928682096));
#292954=CARTESIAN_POINT('Ctrl Pts',(-4.08684913857321,12.2,-9.73128403969801));
#292955=CARTESIAN_POINT('Ctrl Pts',(-4.08759666196258,12.2,-9.73508879222945));
#292956=CARTESIAN_POINT('Ctrl Pts',(-4.08834210621569,12.2,-9.7389377894337));
#292957=CARTESIAN_POINT('Ctrl Pts',(-4.0890849547754,12.2,-9.74283056222672));
#292958=CARTESIAN_POINT('Ctrl Pts',(-4.08982780333511,12.2,-9.74672333501973));
#292959=CARTESIAN_POINT('Ctrl Pts',(-4.09056805536152,12.2,-9.75065988382971));
#292960=CARTESIAN_POINT('Ctrl Pts',(-4.09130520291821,12.2,-9.75463974451655));
#292961=CARTESIAN_POINT('Ctrl Pts',(-4.09191949257109,12.2,-9.75795629520942));
#292962=CARTESIAN_POINT('Ctrl Pts',(-4.09253162614338,12.2,-9.76130292410865));
#292963=CARTESIAN_POINT('Ctrl Pts',(-4.09314131822684,12.2,-9.76467936653764));
#292964=CARTESIAN_POINT('Ctrl Pts',(-4.0937510103103,12.2,-9.76805580896661));
#292965=CARTESIAN_POINT('Ctrl Pts',(-4.09435825691365,12.2,-9.77146206553812));
#292966=CARTESIAN_POINT('Ctrl Pts',(-4.09496278149974,12.2,-9.77489787624809));
#292967=CARTESIAN_POINT('Ctrl Pts',(-4.09556730608582,12.2,-9.77833368695805));
#292968=CARTESIAN_POINT('Ctrl Pts',(-4.0961691044334,12.2,-9.78179904973328));
#292969=CARTESIAN_POINT('Ctrl Pts',(-4.0967679025584,12.2,-9.78529370952493));
#292970=CARTESIAN_POINT('Ctrl Pts',(-4.09736670068339,12.2,-9.78878836931659));
#292971=CARTESIAN_POINT('Ctrl Pts',(-4.09796249679215,12.2,-9.79231232328012));
#292972=CARTESIAN_POINT('Ctrl Pts',(-4.09855502151705,12.2,-9.79586532072688));
#292973=CARTESIAN_POINT('Ctrl Pts',(-4.09914754624196,12.2,-9.79941831817364));
#292974=CARTESIAN_POINT('Ctrl Pts',(-4.09973679736076,12.2,-9.80300035678474));
#292975=CARTESIAN_POINT('Ctrl Pts',(-4.10032251055502,12.2,-9.80661118595292));
#292976=CARTESIAN_POINT('Ctrl Pts',(-4.10090822374928,12.2,-9.81022201512111));
#292977=CARTESIAN_POINT('Ctrl Pts',(-4.10149039908807,12.2,-9.81386163539408));
#292978=CARTESIAN_POINT('Ctrl Pts',(-4.10206877325454,12.2,-9.81752979796501));
#292979=CARTESIAN_POINT('Ctrl Pts',(-4.102647147421,12.2,-9.82119796053593));
#292980=CARTESIAN_POINT('Ctrl Pts',(-4.10322172128251,12.2,-9.82489466466107));
#292981=CARTESIAN_POINT('Ctrl Pts',(-4.10379223957461,12.2,-9.82861966797413));
#292982=CARTESIAN_POINT('Ctrl Pts',(-4.10436275786672,12.2,-9.83234467128718));
#292983=CARTESIAN_POINT('Ctrl Pts',(-4.10492921971839,12.2,-9.8360979704367));
#292984=CARTESIAN_POINT('Ctrl Pts',(-4.10549137235693,12.2,-9.83987932474456));
#292985=CARTESIAN_POINT('Ctrl Pts',(-4.10605352499546,12.2,-9.84366067905241));
#292986=CARTESIAN_POINT('Ctrl Pts',(-4.10661137020614,12.2,-9.84747008842182));
#292987=CARTESIAN_POINT('Ctrl Pts',(-4.10716465937244,12.2,-9.85130731349353));
#292988=CARTESIAN_POINT('Ctrl Pts',(-4.10771794847843,12.2,-9.855144538147));
#292989=CARTESIAN_POINT('Ctrl Pts',(-4.10826668185449,12.2,-9.85900957797845));
#292990=CARTESIAN_POINT('Ctrl Pts',(-4.10881061617059,12.2,-9.86290219602413));
#292991=CARTESIAN_POINT('Ctrl Pts',(-4.10946333745663,12.2,-9.86757333844268));
#292992=CARTESIAN_POINT('Ctrl Pts',(-4.1101091499087,12.2,-9.87228419452342));
#292993=CARTESIAN_POINT('Ctrl Pts',(-4.1107476400265,12.2,-9.87703435803399));
#292994=CARTESIAN_POINT('Ctrl Pts',(-4.11127971509568,12.2,-9.88099282741039));
#292995=CARTESIAN_POINT('Ctrl Pts',(-4.11180670653443,12.2,-9.88497859472781));
#292996=CARTESIAN_POINT('Ctrl Pts',(-4.11232837924249,12.2,-9.88899142827089));
#292997=CARTESIAN_POINT('Ctrl Pts',(-4.11285005195055,12.2,-9.89300426181397));
#292998=CARTESIAN_POINT('Ctrl Pts',(-4.11336640616755,12.2,-9.8970441613282));
#292999=CARTESIAN_POINT('Ctrl Pts',(-4.11387721452601,12.2,-9.90111089917212));
#293000=CARTESIAN_POINT('Ctrl Pts',(-4.11438802288448,12.2,-9.90517763701604));
#293001=CARTESIAN_POINT('Ctrl Pts',(-4.11489328408254,12.2,-9.90927121186446));
#293002=CARTESIAN_POINT('Ctrl Pts',(-4.1153927717904,12.2,-9.91339139783888));
#293003=CARTESIAN_POINT('Ctrl Pts',(-4.11579236192403,12.2,-9.91668754634894));
#293004=CARTESIAN_POINT('Ctrl Pts',(-4.11618825816368,12.2,-9.92000072582621));
#293005=CARTESIAN_POINT('Ctrl Pts',(-4.11658034574298,12.2,-9.92333082171954));
#293006=CARTESIAN_POINT('Ctrl Pts',(-4.11697243337571,12.2,-9.92666091806659));
#293007=CARTESIAN_POINT('Ctrl Pts',(-4.1173607124688,12.2,-9.93000793116309));
#293008=CARTESIAN_POINT('Ctrl Pts',(-4.11774507256416,12.2,-9.93337174573815));
#293009=CARTESIAN_POINT('Ctrl Pts',(-4.11812943260715,12.2,-9.9367355598549));
#293010=CARTESIAN_POINT('Ctrl Pts',(-4.11850987145533,12.2,-9.94011617674009));
#293011=CARTESIAN_POINT('Ctrl Pts',(-4.1188862802026,12.2,-9.94351348323904));
#293012=CARTESIAN_POINT('Ctrl Pts',(-4.11926268900115,12.2,-9.94691079020087));
#293013=CARTESIAN_POINT('Ctrl Pts',(-4.11963506655479,12.2,-9.95032478605084));
#293014=CARTESIAN_POINT('Ctrl Pts',(-4.1200033047968,12.2,-9.95375535907222));
#293015=CARTESIAN_POINT('Ctrl Pts',(-4.12037154298865,12.2,-9.95718593162619));
#293016=CARTESIAN_POINT('Ctrl Pts',(-4.12073564160335,12.2,-9.96063308195066));
#293017=CARTESIAN_POINT('Ctrl Pts',(-4.12109549248117,12.2,-9.96409669800578));
#293018=CARTESIAN_POINT('Ctrl Pts',(-4.12145534340801,12.2,-9.96756031453283));
#293019=CARTESIAN_POINT('Ctrl Pts',(-4.12181094698766,12.2,-9.97104039691098));
#293020=CARTESIAN_POINT('Ctrl Pts',(-4.12216219722875,12.2,-9.97453683476927));
#293021=CARTESIAN_POINT('Ctrl Pts',(-4.12251344742197,12.2,-9.97803327215117));
#293022=CARTESIAN_POINT('Ctrl Pts',(-4.12286034442162,12.2,-9.98154606677697));
#293023=CARTESIAN_POINT('Ctrl Pts',(-4.12320278272741,12.2,-9.98507510543128));
#293024=CARTESIAN_POINT('Ctrl Pts',(-4.12354522107987,12.2,-9.98860414456644));
#293025=CARTESIAN_POINT('Ctrl Pts',(-4.12388320285007,12.2,-9.99214943105037));
#293026=CARTESIAN_POINT('Ctrl Pts',(-4.12421662125863,12.2,-9.99571085476071));
#293027=CARTESIAN_POINT('Ctrl Pts',(-4.12455003962177,12.2,-9.99927227798581));
#293028=CARTESIAN_POINT('Ctrl Pts',(-4.12487889783976,12.2,-10.0028498382828));
#293029=CARTESIAN_POINT('Ctrl Pts',(-4.1252030914804,12.2,-10.0064434281541));
#293030=CARTESIAN_POINT('Ctrl Pts',(-4.12552728516521,12.2,-10.010037018515));
#293031=CARTESIAN_POINT('Ctrl Pts',(-4.12584681608015,12.2,-10.0136466382662));
#293032=CARTESIAN_POINT('Ctrl Pts',(-4.12616158304174,12.2,-10.0172721807416));
#293033=CARTESIAN_POINT('Ctrl Pts',(-4.12647635000334,12.2,-10.020897723217));
#293034=CARTESIAN_POINT('Ctrl Pts',(-4.12678635171161,12.2,-10.0245391883053));
#293035=CARTESIAN_POINT('Ctrl Pts',(-4.1270914912833,12.2,-10.0281964693396));
#293036=CARTESIAN_POINT('Ctrl Pts',(-4.12739663081341,12.2,-10.0318537498756));
#293037=CARTESIAN_POINT('Ctrl Pts',(-4.1276969073921,12.2,-10.0355268451545));
#293038=CARTESIAN_POINT('Ctrl Pts',(-4.12799222175821,12.2,-10.0392156529808));
#293039=CARTESIAN_POINT('Ctrl Pts',(-4.12828753616455,12.2,-10.0429044613096));
#293040=CARTESIAN_POINT('Ctrl Pts',(-4.12857789011502,12.2,-10.0466089782455));
#293041=CARTESIAN_POINT('Ctrl Pts',(-4.12886318579672,12.2,-10.0503291026165));
#293042=CARTESIAN_POINT('Ctrl Pts',(-4.12914848143955,12.2,-10.0540492264807));
#293043=CARTESIAN_POINT('Ctrl Pts',(-4.12942871864969,12.2,-10.0577849556955));
#293044=CARTESIAN_POINT('Ctrl Pts',(-4.12970380296087,12.2,-10.0615361869434));
#293045=CARTESIAN_POINT('Ctrl Pts',(-4.12997888730953,12.2,-10.0652874187024));
#293046=CARTESIAN_POINT('Ctrl Pts',(-4.13024881746126,12.2,-10.0690541518802));
#293047=CARTESIAN_POINT('Ctrl Pts',(-4.13051350048845,12.2,-10.0728362838322));
#293048=CARTESIAN_POINT('Ctrl Pts',(-4.13077818347958,12.2,-10.0766184152688));
#293049=CARTESIAN_POINT('Ctrl Pts',(-4.13103761903301,12.2,-10.0804159443817));
#293050=CARTESIAN_POINT('Ctrl Pts',(-4.13129171401259,12.2,-10.0842287696801));
#293051=CARTESIAN_POINT('Ctrl Pts',(-4.13154580902679,12.2,-10.088041595498));
#293052=CARTESIAN_POINT('Ctrl Pts',(-4.13179456230701,12.2,-10.09186971754));
#293053=CARTESIAN_POINT('Ctrl Pts',(-4.13203788398658,12.2,-10.095713032806));
#293054=CARTESIAN_POINT('Ctrl Pts',(-4.13228120563301,12.2,-10.0995563475483));
#293055=CARTESIAN_POINT('Ctrl Pts',(-4.13251909466213,12.2,-10.1034148568957));
#293056=CARTESIAN_POINT('Ctrl Pts',(-4.132751460433,12.2,-10.107288458438));
#293057=CARTESIAN_POINT('Ctrl Pts',(-4.13298382623553,12.2,-10.1111620605079));
#293058=CARTESIAN_POINT('Ctrl Pts',(-4.13321066942309,12.2,-10.1150507555527));
#293059=CARTESIAN_POINT('Ctrl Pts',(-4.13343189976811,12.2,-10.1189544420442));
#293060=CARTESIAN_POINT('Ctrl Pts',(-4.13365313008299,12.2,-10.1228581280039));
#293061=CARTESIAN_POINT('Ctrl Pts',(-4.13386874747122,12.2,-10.1267768067438));
#293062=CARTESIAN_POINT('Ctrl Pts',(-4.13407866389909,12.2,-10.1307103773652));
#293063=CARTESIAN_POINT('Ctrl Pts',(-4.13428858035556,12.2,-10.1346439485225));
#293064=CARTESIAN_POINT('Ctrl Pts',(-4.13449279536074,12.2,-10.138592411852));
#293065=CARTESIAN_POINT('Ctrl Pts',(-4.13469122248355,12.2,-10.1425556677527));
#293066=CARTESIAN_POINT('Ctrl Pts',(-4.13488964957932,12.2,-10.1465189231134));
#293067=CARTESIAN_POINT('Ctrl Pts',(-4.13508228934532,12.2,-10.1504969711445));
#293068=CARTESIAN_POINT('Ctrl Pts',(-4.13526905321954,12.2,-10.1544897138722));
#293069=CARTESIAN_POINT('Ctrl Pts',(-4.13545581711921,12.2,-10.1584824571438));
#293070=CARTESIAN_POINT('Ctrl Pts',(-4.13563670813499,12.2,-10.1624898947252));
#293071=CARTESIAN_POINT('Ctrl Pts',(-4.13581163803341,12.2,-10.1665119285));
#293072=CARTESIAN_POINT('Ctrl Pts',(-4.13598656793184,12.2,-10.1705339622747));
#293073=CARTESIAN_POINT('Ctrl Pts',(-4.13615553840734,12.2,-10.1745705930289));
#293074=CARTESIAN_POINT('Ctrl Pts',(-4.13631846552672,12.2,-10.1786217216956));
#293075=CARTESIAN_POINT('Ctrl Pts',(-4.13648139262389,12.2,-10.1826728498104));
#293076=CARTESIAN_POINT('Ctrl Pts',(-4.13663827700795,12.2,-10.1867384775316));
#293077=CARTESIAN_POINT('Ctrl Pts',(-4.13678903349603,12.2,-10.1908185074749));
#293078=CARTESIAN_POINT('Ctrl Pts',(-4.13693979000465,12.2,-10.1948985379741));
#293079=CARTESIAN_POINT('Ctrl Pts',(-4.13708442016454,12.2,-10.1989929699658));
#293080=CARTESIAN_POINT('Ctrl Pts',(-4.1372228420118,12.2,-10.2031017080629));
#293081=CARTESIAN_POINT('Ctrl Pts',(-4.13736126384019,12.2,-10.2072104456002));
#293082=CARTESIAN_POINT('Ctrl Pts',(-4.13749347742461,12.2,-10.211333489351));
#293083=CARTESIAN_POINT('Ctrl Pts',(-4.13761940124806,12.2,-10.2154707433452));
#293084=CARTESIAN_POINT('Ctrl Pts',(-4.13774532508867,12.2,-10.2196079979031));
#293085=CARTESIAN_POINT('Ctrl Pts',(-4.13786495947852,12.2,-10.2237594635849));
#293086=CARTESIAN_POINT('Ctrl Pts',(-4.13797822398428,12.2,-10.2279250435906));
#293087=CARTESIAN_POINT('Ctrl Pts',(-4.1380914884746,12.2,-10.2320906230288));
#293088=CARTESIAN_POINT('Ctrl Pts',(-4.13819838365199,12.2,-10.2362703193538));
#293089=CARTESIAN_POINT('Ctrl Pts',(-4.13829883026047,12.2,-10.2404640351082));
#293090=CARTESIAN_POINT('Ctrl Pts',(-4.13842438853133,12.2,-10.2457061802296));
#293091=CARTESIAN_POINT('Ctrl Pts',(-4.13853987097038,12.2,-10.2509702350055));
#293092=CARTESIAN_POINT('Ctrl Pts',(-4.13864512569314,12.2,-10.2562560129211));
#293093=CARTESIAN_POINT('Ctrl Pts',(-4.13872932947593,12.2,-10.260484635484));
#293094=CARTESIAN_POINT('Ctrl Pts',(-4.13880698679683,12.2,-10.2647271607485));
#293095=CARTESIAN_POINT('Ctrl Pts',(-4.13887802202249,12.2,-10.2689834973147));
#293096=CARTESIAN_POINT('Ctrl Pts',(-4.13894905723848,12.2,-10.273239833301));
#293097=CARTESIAN_POINT('Ctrl Pts',(-4.13901346916792,12.2,-10.2775099806213));
#293098=CARTESIAN_POINT('Ctrl Pts',(-4.139071183,12.2,-10.2817938449284));
#293099=CARTESIAN_POINT('Ctrl Pts',(-4.13912889683995,12.2,-10.2860777098192));
#293100=CARTESIAN_POINT('Ctrl Pts',(-4.13917991194888,12.2,-10.2903752927694));
#293101=CARTESIAN_POINT('Ctrl Pts',(-4.13922415322864,12.2,-10.2946865013942));
#293102=CARTESIAN_POINT('Ctrl Pts',(-4.13926839450235,12.2,-10.2989977094316));
#293103=CARTESIAN_POINT('Ctrl Pts',(-4.13930586327743,12.2,-10.3033225423439));
#293104=CARTESIAN_POINT('Ctrl Pts',(-4.13933648322007,12.2,-10.3076609102656));
#293105=CARTESIAN_POINT('Ctrl Pts',(-4.13936710316689,12.2,-10.3119992787785));
#293106=CARTESIAN_POINT('Ctrl Pts',(-4.13939087574634,12.2,-10.316351180159));
#293107=CARTESIAN_POINT('Ctrl Pts',(-4.13940772702509,12.2,-10.3207165260279));
#293108=CARTESIAN_POINT('Ctrl Pts',(-4.13942457830155,12.2,-10.325081871302));
#293109=CARTESIAN_POINT('Ctrl Pts',(-4.13943450976857,12.2,-10.3294606591173));
#293110=CARTESIAN_POINT('Ctrl Pts',(-4.13943744649127,12.2,-10.3338527985902));
#293111=CARTESIAN_POINT('Ctrl Pts',(-4.13944038321436,12.2,-10.3382449386615));
#293112=CARTESIAN_POINT('Ctrl Pts',(-4.13943632790903,12.2,-10.3426504325647));
#293113=CARTESIAN_POINT('Ctrl Pts',(-4.13942520774175,12.2,-10.34706918725));
#293114=CARTESIAN_POINT('Ctrl Pts',(-4.13941408757448,12.2,-10.3514879419352));
#293115=CARTESIAN_POINT('Ctrl Pts',(-4.13939590172861,12.2,-10.3559199596415));
#293116=CARTESIAN_POINT('Ctrl Pts',(-4.13937058100427,12.2,-10.3603651497184));
#293117=CARTESIAN_POINT('Ctrl Pts',(-4.13935159046275,12.2,-10.3636990419733));
#293118=CARTESIAN_POINT('Ctrl Pts',(-4.13932858651232,12.2,-10.3670403444681));
#293119=CARTESIAN_POINT('Ctrl Pts',(-4.13930153901148,12.2,-10.3703890183896));
#293120=CARTESIAN_POINT('Ctrl Pts',(-4.13926547567867,12.2,-10.3748539167488));
#293121=CARTESIAN_POINT('Ctrl Pts',(-4.13922222618843,12.2,-10.3793319213204));
#293122=CARTESIAN_POINT('Ctrl Pts',(-4.13917171830415,12.2,-10.3838229426746));
#293123=CARTESIAN_POINT('Ctrl Pts',(-4.13912121041298,12.2,-10.3883139646407));
#293124=CARTESIAN_POINT('Ctrl Pts',(-4.13906344625983,12.2,-10.3928180030279));
#293125=CARTESIAN_POINT('Ctrl Pts',(-4.13899835681136,12.2,-10.397334970386));
#293126=CARTESIAN_POINT('Ctrl Pts',(-4.13894953972944,12.2,-10.4007226955969));
#293127=CARTESIAN_POINT('Ctrl Pts',(-4.13889660199824,12.2,-10.4041176943112));
#293128=CARTESIAN_POINT('Ctrl Pts',(-4.13883951550003,12.2,-10.4075199275364));
#293129=CARTESIAN_POINT('Ctrl Pts',(-4.1387443713329,12.2,-10.4131903164511));
#293130=CARTESIAN_POINT('Ctrl Pts',(-4.13863770266511,12.2,-10.4188808030003));
#293131=CARTESIAN_POINT('Ctrl Pts',(-4.13851937773394,12.2,-10.4245912168902));
#293132=CARTESIAN_POINT('Ctrl Pts',(-4.13844838277782,12.2,-10.4280174650997));
#293133=CARTESIAN_POINT('Ctrl Pts',(-4.1383731926972,12.2,-10.4314508870583));
#293134=CARTESIAN_POINT('Ctrl Pts',(-4.13829377778342,12.2,-10.434891446725));
#293135=CARTESIAN_POINT('Ctrl Pts',(-4.13821436286964,12.2,-10.4383320063916));
#293136=CARTESIAN_POINT('Ctrl Pts',(-4.13813072518937,12.2,-10.4417797029497));
#293137=CARTESIAN_POINT('Ctrl Pts',(-4.13804283527626,12.2,-10.4452345001152));
#293138=CARTESIAN_POINT('Ctrl Pts',(-4.13795494536316,12.2,-10.4486892972807));
#293139=CARTESIAN_POINT('Ctrl Pts',(-4.13786280473618,12.2,-10.4521511944824));
#293140=CARTESIAN_POINT('Ctrl Pts',(-4.13776638477703,12.2,-10.4556201568205));
#293141=CARTESIAN_POINT('Ctrl Pts',(-4.13766996481788,12.2,-10.4590891191587));
#293142=CARTESIAN_POINT('Ctrl Pts',(-4.13756926635191,12.2,-10.4625651457515));
#293143=CARTESIAN_POINT('Ctrl Pts',(-4.13746426227297,12.2,-10.466048199499));
#293144=CARTESIAN_POINT('Ctrl Pts',(-4.13735925817497,12.2,-10.4695312538792));
#293145=CARTESIAN_POINT('Ctrl Pts',(-4.13724994680908,12.2,-10.4730213363198));
#293146=CARTESIAN_POINT('Ctrl Pts',(-4.13713630375031,12.2,-10.4765184102457));
#293147=CARTESIAN_POINT('Ctrl Pts',(-4.13702266071218,12.2,-10.4800154835362));
#293148=CARTESIAN_POINT('Ctrl Pts',(-4.13690468441595,12.2,-10.4835195496431));
#293149=CARTESIAN_POINT('Ctrl Pts',(-4.13678234892001,12.2,-10.4870305708495));
#293150=CARTESIAN_POINT('Ctrl Pts',(-4.13666001342408,12.2,-10.4905415920558));
#293151=CARTESIAN_POINT('Ctrl Pts',(-4.13653331877915,12.2,-10.4940595688652));
#293152=CARTESIAN_POINT('Ctrl Pts',(-4.1364022377833,12.2,-10.4975844660448));
#293153=CARTESIAN_POINT('Ctrl Pts',(-4.13627115678745,12.2,-10.5011093632245));
#293154=CARTESIAN_POINT('Ctrl Pts',(-4.13613569001241,12.2,-10.504641180526));
#293155=CARTESIAN_POINT('Ctrl Pts',(-4.13599581151688,12.2,-10.5081798812467));
#293156=CARTESIAN_POINT('Ctrl Pts',(-4.13585593302135,12.2,-10.5117185819676));
#293157=CARTESIAN_POINT('Ctrl Pts',(-4.1357116416771,12.2,-10.5152641661925));
#293158=CARTESIAN_POINT('Ctrl Pts',(-4.13556291272456,12.2,-10.5188165998962));
#293159=CARTESIAN_POINT('Ctrl Pts',(-4.13541418377201,12.2,-10.5223690335999));
#293160=CARTESIAN_POINT('Ctrl Pts',(-4.13526101752811,12.2,-10.5259283161531));
#293161=CARTESIAN_POINT('Ctrl Pts',(-4.13510338703445,12.2,-10.5294944109392));
#293162=CARTESIAN_POINT('Ctrl Pts',(-4.13494575651215,12.2,-10.5330605063732));
#293163=CARTESIAN_POINT('Ctrl Pts',(-4.13478366150526,12.2,-10.5366334149258));
#293164=CARTESIAN_POINT('Ctrl Pts',(-4.13461707793877,12.2,-10.5402131017387));
#293165=CARTESIAN_POINT('Ctrl Pts',(-4.13445049440254,12.2,-10.5437927879012));
#293166=CARTESIAN_POINT('Ctrl Pts',(-4.13427942122489,12.2,-10.547379251755));
#293167=CARTESIAN_POINT('Ctrl Pts',(-4.13410383327254,12.2,-10.5509724579167));
#293168=CARTESIAN_POINT('Ctrl Pts',(-4.13392824532019,12.2,-10.5545656640784));
#293169=CARTESIAN_POINT('Ctrl Pts',(-4.1337481435274,12.2,-10.5581656123679));
#293170=CARTESIAN_POINT('Ctrl Pts',(-4.13356350203325,12.2,-10.5617722685449));
#293171=CARTESIAN_POINT('Ctrl Pts',(-4.1333788605391,12.2,-10.565378924722));
#293172=CARTESIAN_POINT('Ctrl Pts',(-4.13318967856075,12.2,-10.5689922880951));
#293173=CARTESIAN_POINT('Ctrl Pts',(-4.13299593302526,12.2,-10.5726123237717));
#293174=CARTESIAN_POINT('Ctrl Pts',(-4.13280218748977,12.2,-10.5762323594483));
#293175=CARTESIAN_POINT('Ctrl Pts',(-4.13260387653102,12.2,-10.57985906597));
#293176=CARTESIAN_POINT('Ctrl Pts',(-4.13240097703879,12.2,-10.5834924120874));
#293177=CARTESIAN_POINT('Ctrl Pts',(-4.13219807754657,12.2,-10.5871257582048));
#293178=CARTESIAN_POINT('Ctrl Pts',(-4.13199058827132,12.2,-10.5907657411884));
#293179=CARTESIAN_POINT('Ctrl Pts',(-4.13177848627966,12.2,-10.59441232693));
#293180=CARTESIAN_POINT('Ctrl Pts',(-4.13156638424946,12.2,-10.5980589133341));
#293181=CARTESIAN_POINT('Ctrl Pts',(-4.13134966841797,12.2,-10.6017121031317));
#293182=CARTESIAN_POINT('Ctrl Pts',(-4.1311283149685,12.2,-10.6053718605395));
#293183=CARTESIAN_POINT('Ctrl Pts',(-4.13090696155924,12.2,-10.6090316172824));
#293184=CARTESIAN_POINT('Ctrl Pts',(-4.13068097132577,12.2,-10.6126979423598));
#293185=CARTESIAN_POINT('Ctrl Pts',(-4.13045031794708,12.2,-10.6163708017023));
#293186=CARTESIAN_POINT('Ctrl Pts',(-4.1302196645684,12.2,-10.6200436610448));
#293187=CARTESIAN_POINT('Ctrl Pts',(-4.12998434943221,12.2,-10.6237230529518));
#293188=CARTESIAN_POINT('Ctrl Pts',(-4.12974434898218,12.2,-10.6274089446518));
#293189=CARTESIAN_POINT('Ctrl Pts',(-4.12950434853216,12.2,-10.6310948363518));
#293190=CARTESIAN_POINT('Ctrl Pts',(-4.12925966242436,12.2,-10.6347872274677));
#293191=CARTESIAN_POINT('Ctrl Pts',(-4.12901026701676,12.2,-10.6384860832916));
#293192=CARTESIAN_POINT('Ctrl Pts',(-4.12876087160915,12.2,-10.6421849391156));
#293193=CARTESIAN_POINT('Ctrl Pts',(-4.12850676758507,12.2,-10.6458902610143));
#293194=CARTESIAN_POINT('Ctrl Pts',(-4.12824793205322,12.2,-10.6496020137955));
#293195=CARTESIAN_POINT('Ctrl Pts',(-4.12781653948446,12.2,-10.6557882686557));
#293196=CARTESIAN_POINT('Ctrl Pts',(-4.12737200006349,12.2,-10.6619923887517));
#293197=CARTESIAN_POINT('Ctrl Pts',(-4.126914203742,12.2,-10.6682142102382));
#293198=CARTESIAN_POINT('Ctrl Pts',(-4.12663952595909,12.2,-10.6719473029945));
#293199=CARTESIAN_POINT('Ctrl Pts',(-4.12636007713692,12.2,-10.6756867685951));
#293200=CARTESIAN_POINT('Ctrl Pts',(-4.12607583527266,12.2,-10.6794325763751));
#293201=CARTESIAN_POINT('Ctrl Pts',(-4.12569684608589,12.2,-10.6844269872021));
#293202=CARTESIAN_POINT('Ctrl Pts',(-4.12530933743978,12.2,-10.6894326742333));
#293203=CARTESIAN_POINT('Ctrl Pts',(-4.12491325541763,12.2,-10.6944495574519));
#293204=CARTESIAN_POINT('Ctrl Pts',(-4.124616193928,12.2,-10.6982122195241));
#293205=CARTESIAN_POINT('Ctrl Pts',(-4.12431430950675,12.2,-10.7019811776567));
#293206=CARTESIAN_POINT('Ctrl Pts',(-4.12400757305814,12.2,-10.7057563912867));
#293207=CARTESIAN_POINT('Ctrl Pts',(-4.12370083660954,12.2,-10.7095316049168));
#293208=CARTESIAN_POINT('Ctrl Pts',(-4.12338924799029,12.2,-10.7133130717003));
#293209=CARTESIAN_POINT('Ctrl Pts',(-4.12307278825038,12.2,-10.7171007627465));
#293210=CARTESIAN_POINT('Ctrl Pts',(-4.12254535533135,12.2,-10.7234135813863));
#293211=CARTESIAN_POINT('Ctrl Pts',(-4.12200438478762,12.2,-10.7297436872829));
#293212=CARTESIAN_POINT('Ctrl Pts',(-4.12144986800006,12.2,-10.736091047));
#293213=CARTESIAN_POINT('Origin',(-5.66257110645729E-14,15.2,-1.77635683940025E-14));
#293214=CARTESIAN_POINT('',(-2.64164356403319,15.2,-10.0330625574592));
#293215=CARTESIAN_POINT('',(-2.64164356403319,12.2,-10.0330625574592));
#293216=CARTESIAN_POINT('',(-2.64164356400005,15.2,-10.033062557));
#293217=CARTESIAN_POINT('Origin',(-5.66257110645729E-14,12.2,-1.77635683940025E-14));
#293218=CARTESIAN_POINT('Origin',(-5.66257110645729E-14,15.2,-1.77635683940025E-14));
#293219=CARTESIAN_POINT('Origin',(-5.66257110645729E-14,15.2,-1.77635683940025E-14));
#293220=CARTESIAN_POINT('',(-2.55159439100006,15.2,-11.213356592));
#293221=CARTESIAN_POINT('',(-2.17615954800006,15.2,-11.292224299));
#293222=CARTESIAN_POINT('Origin',(-5.66257110645729E-14,15.2,-1.77635683940025E-14));
#293223=CARTESIAN_POINT('',(-2.17615954800006,12.2,-11.292224299));
#293224=CARTESIAN_POINT('',(-2.17615954800006,15.2,-11.292224299));
#293225=CARTESIAN_POINT('',(-2.55159439100006,12.2,-11.213356592));
#293226=CARTESIAN_POINT('Origin',(-5.66257110645729E-14,12.2,-1.77635683940025E-14));
#293227=CARTESIAN_POINT('',(-2.55159439100006,15.2,-11.213356592));
#293228=CARTESIAN_POINT('Ctrl Pts',(-2.64164356400005,15.2,-10.033062558));
#293229=CARTESIAN_POINT('Ctrl Pts',(-2.64164356400005,11.6,-10.033062558));
#293230=CARTESIAN_POINT('Ctrl Pts',(-2.64167330500006,15.2,-10.03323436));
#293231=CARTESIAN_POINT('Ctrl Pts',(-2.64167330500006,11.6,-10.03323436));
#293232=CARTESIAN_POINT('Ctrl Pts',(-2.64173373800006,15.2,-10.033583981));
#293233=CARTESIAN_POINT('Ctrl Pts',(-2.64173373800006,11.6,-10.033583981));
#293234=CARTESIAN_POINT('Ctrl Pts',(-2.64182504800006,15.2,-10.034113785));
#293235=CARTESIAN_POINT('Ctrl Pts',(-2.64182504800006,11.6,-10.034113785));
#293236=CARTESIAN_POINT('Ctrl Pts',(-2.64194752000006,15.2,-10.034827572));
#293237=CARTESIAN_POINT('Ctrl Pts',(-2.64194752000006,11.6,-10.034827572));
#293238=CARTESIAN_POINT('Ctrl Pts',(-2.64210152600006,15.2,-10.03573056));
#293239=CARTESIAN_POINT('Ctrl Pts',(-2.64210152600006,11.6,-10.03573056));
#293240=CARTESIAN_POINT('Ctrl Pts',(-2.64225710800006,15.2,-10.03664834));
#293241=CARTESIAN_POINT('Ctrl Pts',(-2.64225710800006,11.6,-10.03664834));
#293242=CARTESIAN_POINT('Ctrl Pts',(-2.64241335000006,15.2,-10.037575657));
#293243=CARTESIAN_POINT('Ctrl Pts',(-2.64241335000006,11.6,-10.037575657));
#293244=CARTESIAN_POINT('Ctrl Pts',(-2.64257023000006,15.2,-10.038512489));
#293245=CARTESIAN_POINT('Ctrl Pts',(-2.64257023000006,11.6,-10.038512489));
#293246=CARTESIAN_POINT('Ctrl Pts',(-2.64272772500005,15.2,-10.039458811));
#293247=CARTESIAN_POINT('Ctrl Pts',(-2.64272772500005,11.6,-10.039458811));
#293248=CARTESIAN_POINT('Ctrl Pts',(-2.64288581300006,15.2,-10.040414601));
#293249=CARTESIAN_POINT('Ctrl Pts',(-2.64288581300006,11.6,-10.040414601));
#293250=CARTESIAN_POINT('Ctrl Pts',(-2.64304447300006,15.2,-10.041379835));
#293251=CARTESIAN_POINT('Ctrl Pts',(-2.64304447300006,11.6,-10.041379835));
#293252=CARTESIAN_POINT('Ctrl Pts',(-2.64320368100006,15.2,-10.042354489));
#293253=CARTESIAN_POINT('Ctrl Pts',(-2.64320368100006,11.6,-10.042354489));
#293254=CARTESIAN_POINT('Ctrl Pts',(-2.64336341800006,15.2,-10.043338542));
#293255=CARTESIAN_POINT('Ctrl Pts',(-2.64336341800006,11.6,-10.043338542));
#293256=CARTESIAN_POINT('Ctrl Pts',(-2.64352366100006,15.2,-10.044331968));
#293257=CARTESIAN_POINT('Ctrl Pts',(-2.64352366100006,11.6,-10.044331968));
#293258=CARTESIAN_POINT('Ctrl Pts',(-2.64368438700005,15.2,-10.045334746));
#293259=CARTESIAN_POINT('Ctrl Pts',(-2.64368438700005,11.6,-10.045334746));
#293260=CARTESIAN_POINT('Ctrl Pts',(-2.64384557700006,15.2,-10.046346854));
#293261=CARTESIAN_POINT('Ctrl Pts',(-2.64384557700006,11.6,-10.046346854));
#293262=CARTESIAN_POINT('Ctrl Pts',(-2.64400720800006,15.2,-10.047368268));
#293263=CARTESIAN_POINT('Ctrl Pts',(-2.64400720800006,11.6,-10.047368268));
#293264=CARTESIAN_POINT('Ctrl Pts',(-2.64416926000006,15.2,-10.048398967));
#293265=CARTESIAN_POINT('Ctrl Pts',(-2.64416926000006,11.6,-10.048398967));
#293266=CARTESIAN_POINT('Ctrl Pts',(-2.64433171100006,15.2,-10.049438925));
#293267=CARTESIAN_POINT('Ctrl Pts',(-2.64433171100006,11.6,-10.049438925));
#293268=CARTESIAN_POINT('Ctrl Pts',(-2.64449454000005,15.2,-10.050488124));
#293269=CARTESIAN_POINT('Ctrl Pts',(-2.64449454000005,11.6,-10.050488124));
#293270=CARTESIAN_POINT('Ctrl Pts',(-2.64465772700006,15.2,-10.051546539));
#293271=CARTESIAN_POINT('Ctrl Pts',(-2.64465772700006,11.6,-10.051546539));
#293272=CARTESIAN_POINT('Ctrl Pts',(-2.64482124900006,15.2,-10.052614149));
#293273=CARTESIAN_POINT('Ctrl Pts',(-2.64482124900006,11.6,-10.052614149));
#293274=CARTESIAN_POINT('Ctrl Pts',(-2.64498508800005,15.2,-10.05369093));
#293275=CARTESIAN_POINT('Ctrl Pts',(-2.64498508800005,11.6,-10.05369093));
#293276=CARTESIAN_POINT('Ctrl Pts',(-2.64514922300005,15.2,-10.054776863));
#293277=CARTESIAN_POINT('Ctrl Pts',(-2.64514922300005,11.6,-10.054776863));
#293278=CARTESIAN_POINT('Ctrl Pts',(-2.64531363200006,15.2,-10.055871923));
#293279=CARTESIAN_POINT('Ctrl Pts',(-2.64531363200006,11.6,-10.055871923));
#293280=CARTESIAN_POINT('Ctrl Pts',(-2.64547829600006,15.2,-10.056976091));
#293281=CARTESIAN_POINT('Ctrl Pts',(-2.64547829600006,11.6,-10.056976091));
#293282=CARTESIAN_POINT('Ctrl Pts',(-2.64564319300006,15.2,-10.058089344));
#293283=CARTESIAN_POINT('Ctrl Pts',(-2.64564319300006,11.6,-10.058089344));
#293284=CARTESIAN_POINT('Ctrl Pts',(-2.64580830600006,15.2,-10.059211661));
#293285=CARTESIAN_POINT('Ctrl Pts',(-2.64580830600006,11.6,-10.059211661));
#293286=CARTESIAN_POINT('Ctrl Pts',(-2.64597361300006,15.2,-10.060343019));
#293287=CARTESIAN_POINT('Ctrl Pts',(-2.64597361300006,11.6,-10.060343019));
#293288=CARTESIAN_POINT('Ctrl Pts',(-2.64613909300006,15.2,-10.061483397));
#293289=CARTESIAN_POINT('Ctrl Pts',(-2.64613909300006,11.6,-10.061483397));
#293290=CARTESIAN_POINT('Ctrl Pts',(-2.64630472900006,15.2,-10.062632776));
#293291=CARTESIAN_POINT('Ctrl Pts',(-2.64630472900006,11.6,-10.062632776));
#293292=CARTESIAN_POINT('Ctrl Pts',(-2.64647049900006,15.2,-10.063791132));
#293293=CARTESIAN_POINT('Ctrl Pts',(-2.64647049900006,11.6,-10.063791132));
#293294=CARTESIAN_POINT('Ctrl Pts',(-2.64663638300005,15.2,-10.064958444));
#293295=CARTESIAN_POINT('Ctrl Pts',(-2.64663638300005,11.6,-10.064958444));
#293296=CARTESIAN_POINT('Ctrl Pts',(-2.64680236500006,15.2,-10.066134693));
#293297=CARTESIAN_POINT('Ctrl Pts',(-2.64680236500006,11.6,-10.066134693));
#293298=CARTESIAN_POINT('Ctrl Pts',(-2.64696842100005,15.2,-10.067319856));
#293299=CARTESIAN_POINT('Ctrl Pts',(-2.64696842100005,11.6,-10.067319856));
#293300=CARTESIAN_POINT('Ctrl Pts',(-2.64713453500006,15.2,-10.068513912));
#293301=CARTESIAN_POINT('Ctrl Pts',(-2.64713453500006,11.6,-10.068513912));
#293302=CARTESIAN_POINT('Ctrl Pts',(-2.64730068700006,15.2,-10.069716842));
#293303=CARTESIAN_POINT('Ctrl Pts',(-2.64730068700006,11.6,-10.069716842));
#293304=CARTESIAN_POINT('Ctrl Pts',(-2.64746685600006,15.2,-10.070928624));
#293305=CARTESIAN_POINT('Ctrl Pts',(-2.64746685600006,11.6,-10.070928624));
#293306=CARTESIAN_POINT('Ctrl Pts',(-2.64763302600006,15.2,-10.072149237));
#293307=CARTESIAN_POINT('Ctrl Pts',(-2.64763302600006,11.6,-10.072149237));
#293308=CARTESIAN_POINT('Ctrl Pts',(-2.64779917600006,15.2,-10.073378662));
#293309=CARTESIAN_POINT('Ctrl Pts',(-2.64779917600006,11.6,-10.073378662));
#293310=CARTESIAN_POINT('Ctrl Pts',(-2.64796528800006,15.2,-10.074616877));
#293311=CARTESIAN_POINT('Ctrl Pts',(-2.64796528800006,11.6,-10.074616877));
#293312=CARTESIAN_POINT('Ctrl Pts',(-2.64813134300006,15.2,-10.075863863));
#293313=CARTESIAN_POINT('Ctrl Pts',(-2.64813134300006,11.6,-10.075863863));
#293314=CARTESIAN_POINT('Ctrl Pts',(-2.64829732200006,15.2,-10.077119598));
#293315=CARTESIAN_POINT('Ctrl Pts',(-2.64829732200006,11.6,-10.077119598));
#293316=CARTESIAN_POINT('Ctrl Pts',(-2.64846320600005,15.2,-10.078384063));
#293317=CARTESIAN_POINT('Ctrl Pts',(-2.64846320600005,11.6,-10.078384063));
#293318=CARTESIAN_POINT('Ctrl Pts',(-2.64862897800006,15.2,-10.079657237));
#293319=CARTESIAN_POINT('Ctrl Pts',(-2.64862897800006,11.6,-10.079657237));
#293320=CARTESIAN_POINT('Ctrl Pts',(-2.64879462000006,15.2,-10.0809391));
#293321=CARTESIAN_POINT('Ctrl Pts',(-2.64879462000006,11.6,-10.0809391));
#293322=CARTESIAN_POINT('Ctrl Pts',(-2.64896011100006,15.2,-10.082229633));
#293323=CARTESIAN_POINT('Ctrl Pts',(-2.64896011100006,11.6,-10.082229633));
#293324=CARTESIAN_POINT('Ctrl Pts',(-2.64912543500006,15.2,-10.083528816));
#293325=CARTESIAN_POINT('Ctrl Pts',(-2.64912543500006,11.6,-10.083528816));
#293326=CARTESIAN_POINT('Ctrl Pts',(-2.64929057300006,15.2,-10.084836628));
#293327=CARTESIAN_POINT('Ctrl Pts',(-2.64929057300006,11.6,-10.084836628));
#293328=CARTESIAN_POINT('Ctrl Pts',(-2.64945550900006,15.2,-10.086153049));
#293329=CARTESIAN_POINT('Ctrl Pts',(-2.64945550900006,11.6,-10.086153049));
#293330=CARTESIAN_POINT('Ctrl Pts',(-2.64962022200006,15.2,-10.087478061));
#293331=CARTESIAN_POINT('Ctrl Pts',(-2.64962022200006,11.6,-10.087478061));
#293332=CARTESIAN_POINT('Ctrl Pts',(-2.64978469600006,15.2,-10.088811644));
#293333=CARTESIAN_POINT('Ctrl Pts',(-2.64978469600006,11.6,-10.088811644));
#293334=CARTESIAN_POINT('Ctrl Pts',(-2.64994891300006,15.2,-10.090153778));
#293335=CARTESIAN_POINT('Ctrl Pts',(-2.64994891300006,11.6,-10.090153778));
#293336=CARTESIAN_POINT('Ctrl Pts',(-2.65011285400006,15.2,-10.091504443));
#293337=CARTESIAN_POINT('Ctrl Pts',(-2.65011285400006,11.6,-10.091504443));
#293338=CARTESIAN_POINT('Ctrl Pts',(-2.65027650300006,15.2,-10.09286362));
#293339=CARTESIAN_POINT('Ctrl Pts',(-2.65027650300006,11.6,-10.09286362));
#293340=CARTESIAN_POINT('Ctrl Pts',(-2.65043984300006,15.2,-10.09423129));
#293341=CARTESIAN_POINT('Ctrl Pts',(-2.65043984300006,11.6,-10.09423129));
#293342=CARTESIAN_POINT('Ctrl Pts',(-2.65060285500006,15.2,-10.095607434));
#293343=CARTESIAN_POINT('Ctrl Pts',(-2.65060285500006,11.6,-10.095607434));
#293344=CARTESIAN_POINT('Ctrl Pts',(-2.65076552300005,15.2,-10.096992032));
#293345=CARTESIAN_POINT('Ctrl Pts',(-2.65076552300005,11.6,-10.096992032));
#293346=CARTESIAN_POINT('Ctrl Pts',(-2.65092782900005,15.2,-10.098385065));
#293347=CARTESIAN_POINT('Ctrl Pts',(-2.65092782900005,11.6,-10.098385065));
#293348=CARTESIAN_POINT('Ctrl Pts',(-2.65108975500006,15.2,-10.099786515));
#293349=CARTESIAN_POINT('Ctrl Pts',(-2.65108975500006,11.6,-10.099786515));
#293350=CARTESIAN_POINT('Ctrl Pts',(-2.65125128600005,15.2,-10.101196362));
#293351=CARTESIAN_POINT('Ctrl Pts',(-2.65125128600005,11.6,-10.101196362));
#293352=CARTESIAN_POINT('Ctrl Pts',(-2.65141240300005,15.2,-10.102614588));
#293353=CARTESIAN_POINT('Ctrl Pts',(-2.65141240300005,11.6,-10.102614588));
#293354=CARTESIAN_POINT('Ctrl Pts',(-2.65157309100006,15.2,-10.104041173));
#293355=CARTESIAN_POINT('Ctrl Pts',(-2.65157309100006,11.6,-10.104041173));
#293356=CARTESIAN_POINT('Ctrl Pts',(-2.65173333100006,15.2,-10.105476099));
#293357=CARTESIAN_POINT('Ctrl Pts',(-2.65173333100006,11.6,-10.105476099));
#293358=CARTESIAN_POINT('Ctrl Pts',(-2.65189310800006,15.2,-10.106919347));
#293359=CARTESIAN_POINT('Ctrl Pts',(-2.65189310800006,11.6,-10.106919347));
#293360=CARTESIAN_POINT('Ctrl Pts',(-2.65205240400006,15.2,-10.108370899));
#293361=CARTESIAN_POINT('Ctrl Pts',(-2.65205240400006,11.6,-10.108370899));
#293362=CARTESIAN_POINT('Ctrl Pts',(-2.65221120300006,15.2,-10.109830736));
#293363=CARTESIAN_POINT('Ctrl Pts',(-2.65221120300006,11.6,-10.109830736));
#293364=CARTESIAN_POINT('Ctrl Pts',(-2.65236949000006,15.2,-10.11129884));
#293365=CARTESIAN_POINT('Ctrl Pts',(-2.65236949000006,11.6,-10.11129884));
#293366=CARTESIAN_POINT('Ctrl Pts',(-2.65252724700006,15.2,-10.112775192));
#293367=CARTESIAN_POINT('Ctrl Pts',(-2.65252724700006,11.6,-10.112775192));
#293368=CARTESIAN_POINT('Ctrl Pts',(-2.65268445700006,15.2,-10.114259774));
#293369=CARTESIAN_POINT('Ctrl Pts',(-2.65268445700006,11.6,-10.114259774));
#293370=CARTESIAN_POINT('Ctrl Pts',(-2.65284110500006,15.2,-10.115752567));
#293371=CARTESIAN_POINT('Ctrl Pts',(-2.65284110500006,11.6,-10.115752567));
#293372=CARTESIAN_POINT('Ctrl Pts',(-2.65299717300006,15.2,-10.117253555));
#293373=CARTESIAN_POINT('Ctrl Pts',(-2.65299717300006,11.6,-10.117253555));
#293374=CARTESIAN_POINT('Ctrl Pts',(-2.65315264700006,15.2,-10.118762717));
#293375=CARTESIAN_POINT('Ctrl Pts',(-2.65315264700006,11.6,-10.118762717));
#293376=CARTESIAN_POINT('Ctrl Pts',(-2.65330751000006,15.2,-10.120280036));
#293377=CARTESIAN_POINT('Ctrl Pts',(-2.65330751000006,11.6,-10.120280036));
#293378=CARTESIAN_POINT('Ctrl Pts',(-2.65346174600006,15.2,-10.121805494));
#293379=CARTESIAN_POINT('Ctrl Pts',(-2.65346174600006,11.6,-10.121805494));
#293380=CARTESIAN_POINT('Ctrl Pts',(-2.65361534000006,15.2,-10.123339074));
#293381=CARTESIAN_POINT('Ctrl Pts',(-2.65361534000006,11.6,-10.123339074));
#293382=CARTESIAN_POINT('Ctrl Pts',(-2.65376827400006,15.2,-10.124880757));
#293383=CARTESIAN_POINT('Ctrl Pts',(-2.65376827400006,11.6,-10.124880757));
#293384=CARTESIAN_POINT('Ctrl Pts',(-2.65392053400006,15.2,-10.126430526));
#293385=CARTESIAN_POINT('Ctrl Pts',(-2.65392053400006,11.6,-10.126430526));
#293386=CARTESIAN_POINT('Ctrl Pts',(-2.65407210500006,15.2,-10.127988362));
#293387=CARTESIAN_POINT('Ctrl Pts',(-2.65407210500006,11.6,-10.127988362));
#293388=CARTESIAN_POINT('Ctrl Pts',(-2.65422296900006,15.2,-10.129554248));
#293389=CARTESIAN_POINT('Ctrl Pts',(-2.65422296900006,11.6,-10.129554248));
#293390=CARTESIAN_POINT('Ctrl Pts',(-2.65437311200006,15.2,-10.131128167));
#293391=CARTESIAN_POINT('Ctrl Pts',(-2.65437311200006,11.6,-10.131128167));
#293392=CARTESIAN_POINT('Ctrl Pts',(-2.65452251800005,15.2,-10.1327101));
#293393=CARTESIAN_POINT('Ctrl Pts',(-2.65452251800005,11.6,-10.1327101));
#293394=CARTESIAN_POINT('Ctrl Pts',(-2.65467117300005,15.2,-10.134300032));
#293395=CARTESIAN_POINT('Ctrl Pts',(-2.65467117300005,11.6,-10.134300032));
#293396=CARTESIAN_POINT('Ctrl Pts',(-2.65481906000006,15.2,-10.135897942));
#293397=CARTESIAN_POINT('Ctrl Pts',(-2.65481906000006,11.6,-10.135897942));
#293398=CARTESIAN_POINT('Ctrl Pts',(-2.65496616300006,15.2,-10.137503815));
#293399=CARTESIAN_POINT('Ctrl Pts',(-2.65496616300006,11.6,-10.137503815));
#293400=CARTESIAN_POINT('Ctrl Pts',(-2.65511246900005,15.2,-10.139117634));
#293401=CARTESIAN_POINT('Ctrl Pts',(-2.65511246900005,11.6,-10.139117634));
#293402=CARTESIAN_POINT('Ctrl Pts',(-2.65525796200006,15.2,-10.14073938));
#293403=CARTESIAN_POINT('Ctrl Pts',(-2.65525796200006,11.6,-10.14073938));
#293404=CARTESIAN_POINT('Ctrl Pts',(-2.65540262700006,15.2,-10.142369036));
#293405=CARTESIAN_POINT('Ctrl Pts',(-2.65540262700006,11.6,-10.142369036));
#293406=CARTESIAN_POINT('Ctrl Pts',(-2.65554644800006,15.2,-10.144006586));
#293407=CARTESIAN_POINT('Ctrl Pts',(-2.65554644800006,11.6,-10.144006586));
#293408=CARTESIAN_POINT('Ctrl Pts',(-2.65568941100006,15.2,-10.145652013));
#293409=CARTESIAN_POINT('Ctrl Pts',(-2.65568941100006,11.6,-10.145652013));
#293410=CARTESIAN_POINT('Ctrl Pts',(-2.65583150100006,15.2,-10.147305299));
#293411=CARTESIAN_POINT('Ctrl Pts',(-2.65583150100006,11.6,-10.147305299));
#293412=CARTESIAN_POINT('Ctrl Pts',(-2.65597270400006,15.2,-10.148966426));
#293413=CARTESIAN_POINT('Ctrl Pts',(-2.65597270400006,11.6,-10.148966426));
#293414=CARTESIAN_POINT('Ctrl Pts',(-2.65611300400006,15.2,-10.15063538));
#293415=CARTESIAN_POINT('Ctrl Pts',(-2.65611300400006,11.6,-10.15063538));
#293416=CARTESIAN_POINT('Ctrl Pts',(-2.65625238700005,15.2,-10.152312142));
#293417=CARTESIAN_POINT('Ctrl Pts',(-2.65625238700005,11.6,-10.152312142));
#293418=CARTESIAN_POINT('Ctrl Pts',(-2.65639083700006,15.2,-10.153996696));
#293419=CARTESIAN_POINT('Ctrl Pts',(-2.65639083700006,11.6,-10.153996696));
#293420=CARTESIAN_POINT('Ctrl Pts',(-2.65652834300006,15.2,-10.155689024));
#293421=CARTESIAN_POINT('Ctrl Pts',(-2.65652834300006,11.6,-10.155689024));
#293422=CARTESIAN_POINT('Ctrl Pts',(-2.65666488600006,15.2,-10.157389111));
#293423=CARTESIAN_POINT('Ctrl Pts',(-2.65666488600006,11.6,-10.157389111));
#293424=CARTESIAN_POINT('Ctrl Pts',(-2.65680045600006,15.2,-10.159096939));
#293425=CARTESIAN_POINT('Ctrl Pts',(-2.65680045600006,11.6,-10.159096939));
#293426=CARTESIAN_POINT('Ctrl Pts',(-2.65693503500006,15.2,-10.160812491));
#293427=CARTESIAN_POINT('Ctrl Pts',(-2.65693503500006,11.6,-10.160812491));
#293428=CARTESIAN_POINT('Ctrl Pts',(-2.65706861100006,15.2,-10.162535753));
#293429=CARTESIAN_POINT('Ctrl Pts',(-2.65706861100006,11.6,-10.162535753));
#293430=CARTESIAN_POINT('Ctrl Pts',(-2.65720116900006,15.2,-10.164266706));
#293431=CARTESIAN_POINT('Ctrl Pts',(-2.65720116900006,11.6,-10.164266706));
#293432=CARTESIAN_POINT('Ctrl Pts',(-2.65733269400006,15.2,-10.166005334));
#293433=CARTESIAN_POINT('Ctrl Pts',(-2.65733269400006,11.6,-10.166005334));
#293434=CARTESIAN_POINT('Ctrl Pts',(-2.65746317300006,15.2,-10.167751622));
#293435=CARTESIAN_POINT('Ctrl Pts',(-2.65746317300006,11.6,-10.167751622));
#293436=CARTESIAN_POINT('Ctrl Pts',(-2.65759259200005,15.2,-10.169505551));
#293437=CARTESIAN_POINT('Ctrl Pts',(-2.65759259200005,11.6,-10.169505551));
#293438=CARTESIAN_POINT('Ctrl Pts',(-2.65772093700006,15.2,-10.171267108));
#293439=CARTESIAN_POINT('Ctrl Pts',(-2.65772093700006,11.6,-10.171267108));
#293440=CARTESIAN_POINT('Ctrl Pts',(-2.65784819400006,15.2,-10.173036275));
#293441=CARTESIAN_POINT('Ctrl Pts',(-2.65784819400006,11.6,-10.173036275));
#293442=CARTESIAN_POINT('Ctrl Pts',(-2.65797434800006,15.2,-10.174813035));
#293443=CARTESIAN_POINT('Ctrl Pts',(-2.65797434800006,11.6,-10.174813035));
#293444=CARTESIAN_POINT('Ctrl Pts',(-2.65809938700006,15.2,-10.176597374));
#293445=CARTESIAN_POINT('Ctrl Pts',(-2.65809938700006,11.6,-10.176597374));
#293446=CARTESIAN_POINT('Ctrl Pts',(-2.65822329700006,15.2,-10.178389273));
#293447=CARTESIAN_POINT('Ctrl Pts',(-2.65822329700006,11.6,-10.178389273));
#293448=CARTESIAN_POINT('Ctrl Pts',(-2.65834606300006,15.2,-10.18018872));
#293449=CARTESIAN_POINT('Ctrl Pts',(-2.65834606300006,11.6,-10.18018872));
#293450=CARTESIAN_POINT('Ctrl Pts',(-2.65846767200005,15.2,-10.181995694));
#293451=CARTESIAN_POINT('Ctrl Pts',(-2.65846767200005,11.6,-10.181995694));
#293452=CARTESIAN_POINT('Ctrl Pts',(-2.65858811200005,15.2,-10.183810184));
#293453=CARTESIAN_POINT('Ctrl Pts',(-2.65858811200005,11.6,-10.183810184));
#293454=CARTESIAN_POINT('Ctrl Pts',(-2.65870736700006,15.2,-10.185632171));
#293455=CARTESIAN_POINT('Ctrl Pts',(-2.65870736700006,11.6,-10.185632171));
#293456=CARTESIAN_POINT('Ctrl Pts',(-2.65882542500006,15.2,-10.18746164));
#293457=CARTESIAN_POINT('Ctrl Pts',(-2.65882542500006,11.6,-10.18746164));
#293458=CARTESIAN_POINT('Ctrl Pts',(-2.65894227300006,15.2,-10.189298575));
#293459=CARTESIAN_POINT('Ctrl Pts',(-2.65894227300006,11.6,-10.189298575));
#293460=CARTESIAN_POINT('Ctrl Pts',(-2.65905789700006,15.2,-10.191142961));
#293461=CARTESIAN_POINT('Ctrl Pts',(-2.65905789700006,11.6,-10.191142961));
#293462=CARTESIAN_POINT('Ctrl Pts',(-2.65917228200005,15.2,-10.192994781));
#293463=CARTESIAN_POINT('Ctrl Pts',(-2.65917228200005,11.6,-10.192994781));
#293464=CARTESIAN_POINT('Ctrl Pts',(-2.65928541900006,15.2,-10.194854021));
#293465=CARTESIAN_POINT('Ctrl Pts',(-2.65928541900006,11.6,-10.194854021));
#293466=CARTESIAN_POINT('Ctrl Pts',(-2.65939729100006,15.2,-10.196720664));
#293467=CARTESIAN_POINT('Ctrl Pts',(-2.65939729100006,11.6,-10.196720664));
#293468=CARTESIAN_POINT('Ctrl Pts',(-2.65950788700006,15.2,-10.198594695));
#293469=CARTESIAN_POINT('Ctrl Pts',(-2.65950788700006,11.6,-10.198594695));
#293470=CARTESIAN_POINT('Ctrl Pts',(-2.65961719400006,15.2,-10.200476098));
#293471=CARTESIAN_POINT('Ctrl Pts',(-2.65961719400006,11.6,-10.200476098));
#293472=CARTESIAN_POINT('Ctrl Pts',(-2.65972519700005,15.2,-10.202364859));
#293473=CARTESIAN_POINT('Ctrl Pts',(-2.65972519700005,11.6,-10.202364859));
#293474=CARTESIAN_POINT('Ctrl Pts',(-2.65983188500006,15.2,-10.204260961));
#293475=CARTESIAN_POINT('Ctrl Pts',(-2.65983188500006,11.6,-10.204260961));
#293476=CARTESIAN_POINT('Ctrl Pts',(-2.65993724400006,15.2,-10.20616439));
#293477=CARTESIAN_POINT('Ctrl Pts',(-2.65993724400006,11.6,-10.20616439));
#293478=CARTESIAN_POINT('Ctrl Pts',(-2.66004126100006,15.2,-10.208075129));
#293479=CARTESIAN_POINT('Ctrl Pts',(-2.66004126100006,11.6,-10.208075129));
#293480=CARTESIAN_POINT('Ctrl Pts',(-2.66014392500006,15.2,-10.209993165));
#293481=CARTESIAN_POINT('Ctrl Pts',(-2.66014392500006,11.6,-10.209993165));
#293482=CARTESIAN_POINT('Ctrl Pts',(-2.66024522200006,15.2,-10.21191848));
#293483=CARTESIAN_POINT('Ctrl Pts',(-2.66024522200006,11.6,-10.21191848));
#293484=CARTESIAN_POINT('Ctrl Pts',(-2.66034514100005,15.2,-10.213851061));
#293485=CARTESIAN_POINT('Ctrl Pts',(-2.66034514100005,11.6,-10.213851061));
#293486=CARTESIAN_POINT('Ctrl Pts',(-2.66044366600005,15.2,-10.215790891));
#293487=CARTESIAN_POINT('Ctrl Pts',(-2.66044366600005,11.6,-10.215790891));
#293488=CARTESIAN_POINT('Ctrl Pts',(-2.66054078800006,15.2,-10.217737957));
#293489=CARTESIAN_POINT('Ctrl Pts',(-2.66054078800006,11.6,-10.217737957));
#293490=CARTESIAN_POINT('Ctrl Pts',(-2.66063649100006,15.2,-10.219692242));
#293491=CARTESIAN_POINT('Ctrl Pts',(-2.66063649100006,11.6,-10.219692242));
#293492=CARTESIAN_POINT('Ctrl Pts',(-2.66073076600006,15.2,-10.221653734));
#293493=CARTESIAN_POINT('Ctrl Pts',(-2.66073076600006,11.6,-10.221653734));
#293494=CARTESIAN_POINT('Ctrl Pts',(-2.66082359900006,15.2,-10.223622414));
#293495=CARTESIAN_POINT('Ctrl Pts',(-2.66082359900006,11.6,-10.223622414));
#293496=CARTESIAN_POINT('Ctrl Pts',(-2.66091497700006,15.2,-10.225598269));
#293497=CARTESIAN_POINT('Ctrl Pts',(-2.66091497700006,11.6,-10.225598269));
#293498=CARTESIAN_POINT('Ctrl Pts',(-2.66100488900006,15.2,-10.227581285));
#293499=CARTESIAN_POINT('Ctrl Pts',(-2.66100488900006,11.6,-10.227581285));
#293500=CARTESIAN_POINT('Ctrl Pts',(-2.66109332200006,15.2,-10.229571446));
#293501=CARTESIAN_POINT('Ctrl Pts',(-2.66109332200006,11.6,-10.229571446));
#293502=CARTESIAN_POINT('Ctrl Pts',(-2.66118026300005,15.2,-10.231568737));
#293503=CARTESIAN_POINT('Ctrl Pts',(-2.66118026300005,11.6,-10.231568737));
#293504=CARTESIAN_POINT('Ctrl Pts',(-2.66126570200006,15.2,-10.233573145));
#293505=CARTESIAN_POINT('Ctrl Pts',(-2.66126570200006,11.6,-10.233573145));
#293506=CARTESIAN_POINT('Ctrl Pts',(-2.66134962600006,15.2,-10.235584653));
#293507=CARTESIAN_POINT('Ctrl Pts',(-2.66134962600006,11.6,-10.235584653));
#293508=CARTESIAN_POINT('Ctrl Pts',(-2.66143202200006,15.2,-10.237603248));
#293509=CARTESIAN_POINT('Ctrl Pts',(-2.66143202200006,11.6,-10.237603248));
#293510=CARTESIAN_POINT('Ctrl Pts',(-2.66151287900006,15.2,-10.239628914));
#293511=CARTESIAN_POINT('Ctrl Pts',(-2.66151287900006,11.6,-10.239628914));
#293512=CARTESIAN_POINT('Ctrl Pts',(-2.66159218500006,15.2,-10.241661637));
#293513=CARTESIAN_POINT('Ctrl Pts',(-2.66159218500006,11.6,-10.241661637));
#293514=CARTESIAN_POINT('Ctrl Pts',(-2.66166992800006,15.2,-10.243701403));
#293515=CARTESIAN_POINT('Ctrl Pts',(-2.66166992800006,11.6,-10.243701403));
#293516=CARTESIAN_POINT('Ctrl Pts',(-2.66174609500006,15.2,-10.245748197));
#293517=CARTESIAN_POINT('Ctrl Pts',(-2.66174609500006,11.6,-10.245748197));
#293518=CARTESIAN_POINT('Ctrl Pts',(-2.66182067500006,15.2,-10.247802005));
#293519=CARTESIAN_POINT('Ctrl Pts',(-2.66182067500006,11.6,-10.247802005));
#293520=CARTESIAN_POINT('Ctrl Pts',(-2.66189365800006,15.2,-10.249862812));
#293521=CARTESIAN_POINT('Ctrl Pts',(-2.66189365800006,11.6,-10.249862812));
#293522=CARTESIAN_POINT('Ctrl Pts',(-2.66196503000006,15.2,-10.251930603));
#293523=CARTESIAN_POINT('Ctrl Pts',(-2.66196503000006,11.6,-10.251930603));
#293524=CARTESIAN_POINT('Ctrl Pts',(-2.66203478000006,15.2,-10.254005366));
#293525=CARTESIAN_POINT('Ctrl Pts',(-2.66203478000006,11.6,-10.254005366));
#293526=CARTESIAN_POINT('Ctrl Pts',(-2.66210289700005,15.2,-10.256087084));
#293527=CARTESIAN_POINT('Ctrl Pts',(-2.66210289700005,11.6,-10.256087084));
#293528=CARTESIAN_POINT('Ctrl Pts',(-2.66216936800005,15.2,-10.258175744));
#293529=CARTESIAN_POINT('Ctrl Pts',(-2.66216936800005,11.6,-10.258175744));
#293530=CARTESIAN_POINT('Ctrl Pts',(-2.66223418300005,15.2,-10.260271331));
#293531=CARTESIAN_POINT('Ctrl Pts',(-2.66223418300005,11.6,-10.260271331));
#293532=CARTESIAN_POINT('Ctrl Pts',(-2.66229733100006,15.2,-10.262373833));
#293533=CARTESIAN_POINT('Ctrl Pts',(-2.66229733100006,11.6,-10.262373833));
#293534=CARTESIAN_POINT('Ctrl Pts',(-2.66235879800006,15.2,-10.264483233));
#293535=CARTESIAN_POINT('Ctrl Pts',(-2.66235879800006,11.6,-10.264483233));
#293536=CARTESIAN_POINT('Ctrl Pts',(-2.66241857500006,15.2,-10.266599519));
#293537=CARTESIAN_POINT('Ctrl Pts',(-2.66241857500006,11.6,-10.266599519));
#293538=CARTESIAN_POINT('Ctrl Pts',(-2.66247664900006,15.2,-10.268722675));
#293539=CARTESIAN_POINT('Ctrl Pts',(-2.66247664900006,11.6,-10.268722675));
#293540=CARTESIAN_POINT('Ctrl Pts',(-2.66253301000006,15.2,-10.270852689));
#293541=CARTESIAN_POINT('Ctrl Pts',(-2.66253301000006,11.6,-10.270852689));
#293542=CARTESIAN_POINT('Ctrl Pts',(-2.66258764600006,15.2,-10.272989546));
#293543=CARTESIAN_POINT('Ctrl Pts',(-2.66258764600006,11.6,-10.272989546));
#293544=CARTESIAN_POINT('Ctrl Pts',(-2.66264054600006,15.2,-10.275133231));
#293545=CARTESIAN_POINT('Ctrl Pts',(-2.66264054600006,11.6,-10.275133231));
#293546=CARTESIAN_POINT('Ctrl Pts',(-2.66269169900006,15.2,-10.277283732));
#293547=CARTESIAN_POINT('Ctrl Pts',(-2.66269169900006,11.6,-10.277283732));
#293548=CARTESIAN_POINT('Ctrl Pts',(-2.66274109400006,15.2,-10.279441034));
#293549=CARTESIAN_POINT('Ctrl Pts',(-2.66274109400006,11.6,-10.279441034));
#293550=CARTESIAN_POINT('Ctrl Pts',(-2.66278872000006,15.2,-10.281605123));
#293551=CARTESIAN_POINT('Ctrl Pts',(-2.66278872000006,11.6,-10.281605123));
#293552=CARTESIAN_POINT('Ctrl Pts',(-2.66283456500005,15.2,-10.283775986));
#293553=CARTESIAN_POINT('Ctrl Pts',(-2.66283456500005,11.6,-10.283775986));
#293554=CARTESIAN_POINT('Ctrl Pts',(-2.66287862000006,15.2,-10.28595361));
#293555=CARTESIAN_POINT('Ctrl Pts',(-2.66287862000006,11.6,-10.28595361));
#293556=CARTESIAN_POINT('Ctrl Pts',(-2.66292087200006,15.2,-10.288137978));
#293557=CARTESIAN_POINT('Ctrl Pts',(-2.66292087200006,11.6,-10.288137978));
#293558=CARTESIAN_POINT('Ctrl Pts',(-2.66296131100006,15.2,-10.290329079));
#293559=CARTESIAN_POINT('Ctrl Pts',(-2.66296131100006,11.6,-10.290329079));
#293560=CARTESIAN_POINT('Ctrl Pts',(-2.66299992500006,15.2,-10.292526898));
#293561=CARTESIAN_POINT('Ctrl Pts',(-2.66299992500006,11.6,-10.292526898));
#293562=CARTESIAN_POINT('Ctrl Pts',(-2.66303670700006,15.2,-10.294731423));
#293563=CARTESIAN_POINT('Ctrl Pts',(-2.66303670700006,11.6,-10.294731423));
#293564=CARTESIAN_POINT('Ctrl Pts',(-2.66307164100006,15.2,-10.296942639));
#293565=CARTESIAN_POINT('Ctrl Pts',(-2.66307164100006,11.6,-10.296942639));
#293566=CARTESIAN_POINT('Ctrl Pts',(-2.66310472000006,15.2,-10.299160533));
#293567=CARTESIAN_POINT('Ctrl Pts',(-2.66310472000006,11.6,-10.299160533));
#293568=CARTESIAN_POINT('Ctrl Pts',(-2.66313593100006,15.2,-10.301385092));
#293569=CARTESIAN_POINT('Ctrl Pts',(-2.66313593100006,11.6,-10.301385092));
#293570=CARTESIAN_POINT('Ctrl Pts',(-2.66316526600006,15.2,-10.3036163));
#293571=CARTESIAN_POINT('Ctrl Pts',(-2.66316526600006,11.6,-10.3036163));
#293572=CARTESIAN_POINT('Ctrl Pts',(-2.66319271200006,15.2,-10.305854147));
#293573=CARTESIAN_POINT('Ctrl Pts',(-2.66319271200006,11.6,-10.305854147));
#293574=CARTESIAN_POINT('Ctrl Pts',(-2.66321825900006,15.2,-10.308098617));
#293575=CARTESIAN_POINT('Ctrl Pts',(-2.66321825900006,11.6,-10.308098617));
#293576=CARTESIAN_POINT('Ctrl Pts',(-2.66324189700006,15.2,-10.310349696));
#293577=CARTESIAN_POINT('Ctrl Pts',(-2.66324189700006,11.6,-10.310349696));
#293578=CARTESIAN_POINT('Ctrl Pts',(-2.66326361600006,15.2,-10.312607374));
#293579=CARTESIAN_POINT('Ctrl Pts',(-2.66326361600006,11.6,-10.312607374));
#293580=CARTESIAN_POINT('Ctrl Pts',(-2.66328340400006,15.2,-10.314871635));
#293581=CARTESIAN_POINT('Ctrl Pts',(-2.66328340400006,11.6,-10.314871635));
#293582=CARTESIAN_POINT('Ctrl Pts',(-2.66330125200006,15.2,-10.317142467));
#293583=CARTESIAN_POINT('Ctrl Pts',(-2.66330125200006,11.6,-10.317142467));
#293584=CARTESIAN_POINT('Ctrl Pts',(-2.66331714900006,15.2,-10.319419855));
#293585=CARTESIAN_POINT('Ctrl Pts',(-2.66331714900006,11.6,-10.319419855));
#293586=CARTESIAN_POINT('Ctrl Pts',(-2.66333108600006,15.2,-10.321703788));
#293587=CARTESIAN_POINT('Ctrl Pts',(-2.66333108600006,11.6,-10.321703788));
#293588=CARTESIAN_POINT('Ctrl Pts',(-2.66334305100006,15.2,-10.323994252));
#293589=CARTESIAN_POINT('Ctrl Pts',(-2.66334305100006,11.6,-10.323994252));
#293590=CARTESIAN_POINT('Ctrl Pts',(-2.66335303300006,15.2,-10.326291233));
#293591=CARTESIAN_POINT('Ctrl Pts',(-2.66335303300006,11.6,-10.326291233));
#293592=CARTESIAN_POINT('Ctrl Pts',(-2.66336102400006,15.2,-10.328594718));
#293593=CARTESIAN_POINT('Ctrl Pts',(-2.66336102400006,11.6,-10.328594718));
#293594=CARTESIAN_POINT('Ctrl Pts',(-2.66336701400005,15.2,-10.330904695));
#293595=CARTESIAN_POINT('Ctrl Pts',(-2.66336701400005,11.6,-10.330904695));
#293596=CARTESIAN_POINT('Ctrl Pts',(-2.66337099100005,15.2,-10.33322115));
#293597=CARTESIAN_POINT('Ctrl Pts',(-2.66337099100005,11.6,-10.33322115));
#293598=CARTESIAN_POINT('Ctrl Pts',(-2.66337294600006,15.2,-10.33554407));
#293599=CARTESIAN_POINT('Ctrl Pts',(-2.66337294600006,11.6,-10.33554407));
#293600=CARTESIAN_POINT('Ctrl Pts',(-2.66337286800006,15.2,-10.337873443));
#293601=CARTESIAN_POINT('Ctrl Pts',(-2.66337286800006,11.6,-10.337873443));
#293602=CARTESIAN_POINT('Ctrl Pts',(-2.66337074900005,15.2,-10.340209254));
#293603=CARTESIAN_POINT('Ctrl Pts',(-2.66337074900005,11.6,-10.340209254));
#293604=CARTESIAN_POINT('Ctrl Pts',(-2.66336657800006,15.2,-10.342551492));
#293605=CARTESIAN_POINT('Ctrl Pts',(-2.66336657800006,11.6,-10.342551492));
#293606=CARTESIAN_POINT('Ctrl Pts',(-2.66336034400006,15.2,-10.344900143));
#293607=CARTESIAN_POINT('Ctrl Pts',(-2.66336034400006,11.6,-10.344900143));
#293608=CARTESIAN_POINT('Ctrl Pts',(-2.66335203800006,15.2,-10.347255195));
#293609=CARTESIAN_POINT('Ctrl Pts',(-2.66335203800006,11.6,-10.347255195));
#293610=CARTESIAN_POINT('Ctrl Pts',(-2.66334165000006,15.2,-10.349616635));
#293611=CARTESIAN_POINT('Ctrl Pts',(-2.66334165000006,11.6,-10.349616635));
#293612=CARTESIAN_POINT('Ctrl Pts',(-2.66332917200006,15.2,-10.351984448));
#293613=CARTESIAN_POINT('Ctrl Pts',(-2.66332917200006,11.6,-10.351984448));
#293614=CARTESIAN_POINT('Ctrl Pts',(-2.66331459100006,15.2,-10.354358625));
#293615=CARTESIAN_POINT('Ctrl Pts',(-2.66331459100006,11.6,-10.354358625));
#293616=CARTESIAN_POINT('Ctrl Pts',(-2.66329789900006,15.2,-10.35673915));
#293617=CARTESIAN_POINT('Ctrl Pts',(-2.66329789900006,11.6,-10.35673915));
#293618=CARTESIAN_POINT('Ctrl Pts',(-2.66327908700006,15.2,-10.359126011));
#293619=CARTESIAN_POINT('Ctrl Pts',(-2.66327908700006,11.6,-10.359126011));
#293620=CARTESIAN_POINT('Ctrl Pts',(-2.66325814400005,15.2,-10.361519197));
#293621=CARTESIAN_POINT('Ctrl Pts',(-2.66325814400005,11.6,-10.361519197));
#293622=CARTESIAN_POINT('Ctrl Pts',(-2.66323506000006,15.2,-10.363918694));
#293623=CARTESIAN_POINT('Ctrl Pts',(-2.66323506000006,11.6,-10.363918694));
#293624=CARTESIAN_POINT('Ctrl Pts',(-2.66320982800006,15.2,-10.36632449));
#293625=CARTESIAN_POINT('Ctrl Pts',(-2.66320982800006,11.6,-10.36632449));
#293626=CARTESIAN_POINT('Ctrl Pts',(-2.66318243600006,15.2,-10.36873657));
#293627=CARTESIAN_POINT('Ctrl Pts',(-2.66318243600006,11.6,-10.36873657));
#293628=CARTESIAN_POINT('Ctrl Pts',(-2.66315287500006,15.2,-10.371154926));
#293629=CARTESIAN_POINT('Ctrl Pts',(-2.66315287500006,11.6,-10.371154926));
#293630=CARTESIAN_POINT('Ctrl Pts',(-2.66312113600006,15.2,-10.37357954));
#293631=CARTESIAN_POINT('Ctrl Pts',(-2.66312113600006,11.6,-10.37357954));
#293632=CARTESIAN_POINT('Ctrl Pts',(-2.66308721000006,15.2,-10.376010404));
#293633=CARTESIAN_POINT('Ctrl Pts',(-2.66308721000006,11.6,-10.376010404));
#293634=CARTESIAN_POINT('Ctrl Pts',(-2.66305108600006,15.2,-10.378447503));
#293635=CARTESIAN_POINT('Ctrl Pts',(-2.66305108600006,11.6,-10.378447503));
#293636=CARTESIAN_POINT('Ctrl Pts',(-2.66301275600005,15.2,-10.380890826));
#293637=CARTESIAN_POINT('Ctrl Pts',(-2.66301275600005,11.6,-10.380890826));
#293638=CARTESIAN_POINT('Ctrl Pts',(-2.66297221000006,15.2,-10.383340359));
#293639=CARTESIAN_POINT('Ctrl Pts',(-2.66297221000006,11.6,-10.383340359));
#293640=CARTESIAN_POINT('Ctrl Pts',(-2.66292943900006,15.2,-10.38579609));
#293641=CARTESIAN_POINT('Ctrl Pts',(-2.66292943900006,11.6,-10.38579609));
#293642=CARTESIAN_POINT('Ctrl Pts',(-2.66288443400006,15.2,-10.388258008));
#293643=CARTESIAN_POINT('Ctrl Pts',(-2.66288443400006,11.6,-10.388258008));
#293644=CARTESIAN_POINT('Ctrl Pts',(-2.66283718400006,15.2,-10.390726099));
#293645=CARTESIAN_POINT('Ctrl Pts',(-2.66283718400006,11.6,-10.390726099));
#293646=CARTESIAN_POINT('Ctrl Pts',(-2.66278768300006,15.2,-10.393200352));
#293647=CARTESIAN_POINT('Ctrl Pts',(-2.66278768300006,11.6,-10.393200352));
#293648=CARTESIAN_POINT('Ctrl Pts',(-2.66273591900006,15.2,-10.395680753));
#293649=CARTESIAN_POINT('Ctrl Pts',(-2.66273591900006,11.6,-10.395680753));
#293650=CARTESIAN_POINT('Ctrl Pts',(-2.66268188400006,15.2,-10.398167292));
#293651=CARTESIAN_POINT('Ctrl Pts',(-2.66268188400006,11.6,-10.398167292));
#293652=CARTESIAN_POINT('Ctrl Pts',(-2.66262556800006,15.2,-10.400659955));
#293653=CARTESIAN_POINT('Ctrl Pts',(-2.66262556800006,11.6,-10.400659955));
#293654=CARTESIAN_POINT('Ctrl Pts',(-2.66256696400006,15.2,-10.403158731));
#293655=CARTESIAN_POINT('Ctrl Pts',(-2.66256696400006,11.6,-10.403158731));
#293656=CARTESIAN_POINT('Ctrl Pts',(-2.66250606100006,15.2,-10.405663606));
#293657=CARTESIAN_POINT('Ctrl Pts',(-2.66250606100006,11.6,-10.405663606));
#293658=CARTESIAN_POINT('Ctrl Pts',(-2.66244285200006,15.2,-10.40817457));
#293659=CARTESIAN_POINT('Ctrl Pts',(-2.66244285200006,11.6,-10.40817457));
#293660=CARTESIAN_POINT('Ctrl Pts',(-2.66237732500006,15.2,-10.410691609));
#293661=CARTESIAN_POINT('Ctrl Pts',(-2.66237732500006,11.6,-10.410691609));
#293662=CARTESIAN_POINT('Ctrl Pts',(-2.66230947400006,15.2,-10.413214712));
#293663=CARTESIAN_POINT('Ctrl Pts',(-2.66230947400006,11.6,-10.413214712));
#293664=CARTESIAN_POINT('Ctrl Pts',(-2.66223928800006,15.2,-10.415743867));
#293665=CARTESIAN_POINT('Ctrl Pts',(-2.66223928800006,11.6,-10.415743867));
#293666=CARTESIAN_POINT('Ctrl Pts',(-2.66216676000006,15.2,-10.41827906));
#293667=CARTESIAN_POINT('Ctrl Pts',(-2.66216676000006,11.6,-10.41827906));
#293668=CARTESIAN_POINT('Ctrl Pts',(-2.66209187900006,15.2,-10.420820282));
#293669=CARTESIAN_POINT('Ctrl Pts',(-2.66209187900006,11.6,-10.420820282));
#293670=CARTESIAN_POINT('Ctrl Pts',(-2.66201463800006,15.2,-10.423367519));
#293671=CARTESIAN_POINT('Ctrl Pts',(-2.66201463800006,11.6,-10.423367519));
#293672=CARTESIAN_POINT('Ctrl Pts',(-2.66193502800005,15.2,-10.42592076));
#293673=CARTESIAN_POINT('Ctrl Pts',(-2.66193502800005,11.6,-10.42592076));
#293674=CARTESIAN_POINT('Ctrl Pts',(-2.66185304000006,15.2,-10.428479993));
#293675=CARTESIAN_POINT('Ctrl Pts',(-2.66185304000006,11.6,-10.428479993));
#293676=CARTESIAN_POINT('Ctrl Pts',(-2.66176866500006,15.2,-10.431045206));
#293677=CARTESIAN_POINT('Ctrl Pts',(-2.66176866500006,11.6,-10.431045206));
#293678=CARTESIAN_POINT('Ctrl Pts',(-2.66168189500006,15.2,-10.433616386));
#293679=CARTESIAN_POINT('Ctrl Pts',(-2.66168189500006,11.6,-10.433616386));
#293680=CARTESIAN_POINT('Ctrl Pts',(-2.66159272000006,15.2,-10.436193522));
#293681=CARTESIAN_POINT('Ctrl Pts',(-2.66159272000006,11.6,-10.436193522));
#293682=CARTESIAN_POINT('Ctrl Pts',(-2.66150113200006,15.2,-10.438776602));
#293683=CARTESIAN_POINT('Ctrl Pts',(-2.66150113200006,11.6,-10.438776602));
#293684=CARTESIAN_POINT('Ctrl Pts',(-2.66140712500006,15.2,-10.441365614));
#293685=CARTESIAN_POINT('Ctrl Pts',(-2.66140712500006,11.6,-10.441365614));
#293686=CARTESIAN_POINT('Ctrl Pts',(-2.66131068600005,15.2,-10.443960548));
#293687=CARTESIAN_POINT('Ctrl Pts',(-2.66131068600005,11.6,-10.443960548));
#293688=CARTESIAN_POINT('Ctrl Pts',(-2.66121180900006,15.2,-10.446561389));
#293689=CARTESIAN_POINT('Ctrl Pts',(-2.66121180900006,11.6,-10.446561389));
#293690=CARTESIAN_POINT('Ctrl Pts',(-2.66111048600005,15.2,-10.449168128));
#293691=CARTESIAN_POINT('Ctrl Pts',(-2.66111048600005,11.6,-10.449168128));
#293692=CARTESIAN_POINT('Ctrl Pts',(-2.66100670800005,15.2,-10.451780752));
#293693=CARTESIAN_POINT('Ctrl Pts',(-2.66100670800005,11.6,-10.451780752));
#293694=CARTESIAN_POINT('Ctrl Pts',(-2.66090046500006,15.2,-10.45439925));
#293695=CARTESIAN_POINT('Ctrl Pts',(-2.66090046500006,11.6,-10.45439925));
#293696=CARTESIAN_POINT('Ctrl Pts',(-2.66079175100006,15.2,-10.457023609));
#293697=CARTESIAN_POINT('Ctrl Pts',(-2.66079175100006,11.6,-10.457023609));
#293698=CARTESIAN_POINT('Ctrl Pts',(-2.66068055500006,15.2,-10.459653819));
#293699=CARTESIAN_POINT('Ctrl Pts',(-2.66068055500006,11.6,-10.459653819));
#293700=CARTESIAN_POINT('Ctrl Pts',(-2.66056687200006,15.2,-10.462289867));
#293701=CARTESIAN_POINT('Ctrl Pts',(-2.66056687200006,11.6,-10.462289867));
#293702=CARTESIAN_POINT('Ctrl Pts',(-2.66045069100006,15.2,-10.464931742));
#293703=CARTESIAN_POINT('Ctrl Pts',(-2.66045069100006,11.6,-10.464931742));
#293704=CARTESIAN_POINT('Ctrl Pts',(-2.66033200500006,15.2,-10.467579434));
#293705=CARTESIAN_POINT('Ctrl Pts',(-2.66033200500006,11.6,-10.467579434));
#293706=CARTESIAN_POINT('Ctrl Pts',(-2.66021080500006,15.2,-10.470232928));
#293707=CARTESIAN_POINT('Ctrl Pts',(-2.66021080500006,11.6,-10.470232928));
#293708=CARTESIAN_POINT('Ctrl Pts',(-2.66008708400005,15.2,-10.472892215));
#293709=CARTESIAN_POINT('Ctrl Pts',(-2.66008708400005,11.6,-10.472892215));
#293710=CARTESIAN_POINT('Ctrl Pts',(-2.65996083200006,15.2,-10.475557283));
#293711=CARTESIAN_POINT('Ctrl Pts',(-2.65996083200006,11.6,-10.475557283));
#293712=CARTESIAN_POINT('Ctrl Pts',(-2.65983204300006,15.2,-10.47822812));
#293713=CARTESIAN_POINT('Ctrl Pts',(-2.65983204300006,11.6,-10.47822812));
#293714=CARTESIAN_POINT('Ctrl Pts',(-2.65970070700006,15.2,-10.480904716));
#293715=CARTESIAN_POINT('Ctrl Pts',(-2.65970070700006,11.6,-10.480904716));
#293716=CARTESIAN_POINT('Ctrl Pts',(-2.65956681800006,15.2,-10.483587058));
#293717=CARTESIAN_POINT('Ctrl Pts',(-2.65956681800006,11.6,-10.483587058));
#293718=CARTESIAN_POINT('Ctrl Pts',(-2.65943036500006,15.2,-10.486275134));
#293719=CARTESIAN_POINT('Ctrl Pts',(-2.65943036500006,11.6,-10.486275134));
#293720=CARTESIAN_POINT('Ctrl Pts',(-2.65929134200006,15.2,-10.488968935));
#293721=CARTESIAN_POINT('Ctrl Pts',(-2.65929134200006,11.6,-10.488968935));
#293722=CARTESIAN_POINT('Ctrl Pts',(-2.65914974000005,15.2,-10.491668449));
#293723=CARTESIAN_POINT('Ctrl Pts',(-2.65914974000005,11.6,-10.491668449));
#293724=CARTESIAN_POINT('Ctrl Pts',(-2.65900555300006,15.2,-10.494373662));
#293725=CARTESIAN_POINT('Ctrl Pts',(-2.65900555300006,11.6,-10.494373662));
#293726=CARTESIAN_POINT('Ctrl Pts',(-2.65885877000006,15.2,-10.497084566));
#293727=CARTESIAN_POINT('Ctrl Pts',(-2.65885877000006,11.6,-10.497084566));
#293728=CARTESIAN_POINT('Ctrl Pts',(-2.65870938700006,15.2,-10.499801149));
#293729=CARTESIAN_POINT('Ctrl Pts',(-2.65870938700006,11.6,-10.499801149));
#293730=CARTESIAN_POINT('Ctrl Pts',(-2.65855739200005,15.2,-10.502523398));
#293731=CARTESIAN_POINT('Ctrl Pts',(-2.65855739200005,11.6,-10.502523398));
#293732=CARTESIAN_POINT('Ctrl Pts',(-2.65840277900006,15.2,-10.505251303));
#293733=CARTESIAN_POINT('Ctrl Pts',(-2.65840277900006,11.6,-10.505251303));
#293734=CARTESIAN_POINT('Ctrl Pts',(-2.65824554000006,15.2,-10.507984854));
#293735=CARTESIAN_POINT('Ctrl Pts',(-2.65824554000006,11.6,-10.507984854));
#293736=CARTESIAN_POINT('Ctrl Pts',(-2.65808566800006,15.2,-10.510724037));
#293737=CARTESIAN_POINT('Ctrl Pts',(-2.65808566800006,11.6,-10.510724037));
#293738=CARTESIAN_POINT('Ctrl Pts',(-2.65792315500006,15.2,-10.513468843));
#293739=CARTESIAN_POINT('Ctrl Pts',(-2.65792315500006,11.6,-10.513468843));
#293740=CARTESIAN_POINT('Ctrl Pts',(-2.65775799200005,15.2,-10.51621926));
#293741=CARTESIAN_POINT('Ctrl Pts',(-2.65775799200005,11.6,-10.51621926));
#293742=CARTESIAN_POINT('Ctrl Pts',(-2.65759017200006,15.2,-10.518975277));
#293743=CARTESIAN_POINT('Ctrl Pts',(-2.65759017200006,11.6,-10.518975277));
#293744=CARTESIAN_POINT('Ctrl Pts',(-2.65741968700006,15.2,-10.521736883));
#293745=CARTESIAN_POINT('Ctrl Pts',(-2.65741968700006,11.6,-10.521736883));
#293746=CARTESIAN_POINT('Ctrl Pts',(-2.65724653100006,15.2,-10.524504067));
#293747=CARTESIAN_POINT('Ctrl Pts',(-2.65724653100006,11.6,-10.524504067));
#293748=CARTESIAN_POINT('Ctrl Pts',(-2.65707069400006,15.2,-10.527276817));
#293749=CARTESIAN_POINT('Ctrl Pts',(-2.65707069400006,11.6,-10.527276817));
#293750=CARTESIAN_POINT('Ctrl Pts',(-2.65689217000005,15.2,-10.530055124));
#293751=CARTESIAN_POINT('Ctrl Pts',(-2.65689217000005,11.6,-10.530055124));
#293752=CARTESIAN_POINT('Ctrl Pts',(-2.65671095000005,15.2,-10.532838975));
#293753=CARTESIAN_POINT('Ctrl Pts',(-2.65671095000005,11.6,-10.532838975));
#293754=CARTESIAN_POINT('Ctrl Pts',(-2.65652702800006,15.2,-10.535628359));
#293755=CARTESIAN_POINT('Ctrl Pts',(-2.65652702800006,11.6,-10.535628359));
#293756=CARTESIAN_POINT('Ctrl Pts',(-2.65634039600006,15.2,-10.538423267));
#293757=CARTESIAN_POINT('Ctrl Pts',(-2.65634039600006,11.6,-10.538423267));
#293758=CARTESIAN_POINT('Ctrl Pts',(-2.65615104500006,15.2,-10.541223686));
#293759=CARTESIAN_POINT('Ctrl Pts',(-2.65615104500006,11.6,-10.541223686));
#293760=CARTESIAN_POINT('Ctrl Pts',(-2.65595897100006,15.2,-10.544029605));
#293761=CARTESIAN_POINT('Ctrl Pts',(-2.65595897100006,11.6,-10.544029605));
#293762=CARTESIAN_POINT('Ctrl Pts',(-2.65576416300005,15.2,-10.546841016));
#293763=CARTESIAN_POINT('Ctrl Pts',(-2.65576416300005,11.6,-10.546841016));
#293764=CARTESIAN_POINT('Ctrl Pts',(-2.65556661400006,15.2,-10.549657904));
#293765=CARTESIAN_POINT('Ctrl Pts',(-2.65556661400006,11.6,-10.549657904));
#293766=CARTESIAN_POINT('Ctrl Pts',(-2.65536631800006,15.2,-10.552480261));
#293767=CARTESIAN_POINT('Ctrl Pts',(-2.65536631800006,11.6,-10.552480261));
#293768=CARTESIAN_POINT('Ctrl Pts',(-2.65516326800005,15.2,-10.555308075));
#293769=CARTESIAN_POINT('Ctrl Pts',(-2.65516326800005,11.6,-10.555308075));
#293770=CARTESIAN_POINT('Ctrl Pts',(-2.65495745400006,15.2,-10.558141335));
#293771=CARTESIAN_POINT('Ctrl Pts',(-2.65495745400006,11.6,-10.558141335));
#293772=CARTESIAN_POINT('Ctrl Pts',(-2.65474887200006,15.2,-10.560980032));
#293773=CARTESIAN_POINT('Ctrl Pts',(-2.65474887200006,11.6,-10.560980032));
#293774=CARTESIAN_POINT('Ctrl Pts',(-2.65453751300006,15.2,-10.563824152));
#293775=CARTESIAN_POINT('Ctrl Pts',(-2.65453751300006,11.6,-10.563824152));
#293776=CARTESIAN_POINT('Ctrl Pts',(-2.65432336900006,15.2,-10.566673688));
#293777=CARTESIAN_POINT('Ctrl Pts',(-2.65432336900006,11.6,-10.566673688));
#293778=CARTESIAN_POINT('Ctrl Pts',(-2.65410643400006,15.2,-10.569528625));
#293779=CARTESIAN_POINT('Ctrl Pts',(-2.65410643400006,11.6,-10.569528625));
#293780=CARTESIAN_POINT('Ctrl Pts',(-2.65388670100006,15.2,-10.572388956));
#293781=CARTESIAN_POINT('Ctrl Pts',(-2.65388670100006,11.6,-10.572388956));
#293782=CARTESIAN_POINT('Ctrl Pts',(-2.65366416100006,15.2,-10.575254669));
#293783=CARTESIAN_POINT('Ctrl Pts',(-2.65366416100006,11.6,-10.575254669));
#293784=CARTESIAN_POINT('Ctrl Pts',(-2.65343880900006,15.2,-10.578125752));
#293785=CARTESIAN_POINT('Ctrl Pts',(-2.65343880900006,11.6,-10.578125752));
#293786=CARTESIAN_POINT('Ctrl Pts',(-2.65321063600005,15.2,-10.581002197));
#293787=CARTESIAN_POINT('Ctrl Pts',(-2.65321063600005,11.6,-10.581002197));
#293788=CARTESIAN_POINT('Ctrl Pts',(-2.65297963600006,15.2,-10.58388399));
#293789=CARTESIAN_POINT('Ctrl Pts',(-2.65297963600006,11.6,-10.58388399));
#293790=CARTESIAN_POINT('Ctrl Pts',(-2.65274580100006,15.2,-10.586771123));
#293791=CARTESIAN_POINT('Ctrl Pts',(-2.65274580100006,11.6,-10.586771123));
#293792=CARTESIAN_POINT('Ctrl Pts',(-2.65250912600006,15.2,-10.589663585));
#293793=CARTESIAN_POINT('Ctrl Pts',(-2.65250912600006,11.6,-10.589663585));
#293794=CARTESIAN_POINT('Ctrl Pts',(-2.65226960100006,15.2,-10.592561365));
#293795=CARTESIAN_POINT('Ctrl Pts',(-2.65226960100006,11.6,-10.592561365));
#293796=CARTESIAN_POINT('Ctrl Pts',(-2.65202722100006,15.2,-10.595464452));
#293797=CARTESIAN_POINT('Ctrl Pts',(-2.65202722100006,11.6,-10.595464452));
#293798=CARTESIAN_POINT('Ctrl Pts',(-2.65178197900005,15.2,-10.598372836));
#293799=CARTESIAN_POINT('Ctrl Pts',(-2.65178197900005,11.6,-10.598372836));
#293800=CARTESIAN_POINT('Ctrl Pts',(-2.65153386700006,15.2,-10.601286506));
#293801=CARTESIAN_POINT('Ctrl Pts',(-2.65153386700006,11.6,-10.601286506));
#293802=CARTESIAN_POINT('Ctrl Pts',(-2.65128287800006,15.2,-10.604205452));
#293803=CARTESIAN_POINT('Ctrl Pts',(-2.65128287800006,11.6,-10.604205452));
#293804=CARTESIAN_POINT('Ctrl Pts',(-2.65102900700006,15.2,-10.607129663));
#293805=CARTESIAN_POINT('Ctrl Pts',(-2.65102900700006,11.6,-10.607129663));
#293806=CARTESIAN_POINT('Ctrl Pts',(-2.65077224500006,15.2,-10.610059129));
#293807=CARTESIAN_POINT('Ctrl Pts',(-2.65077224500006,11.6,-10.610059129));
#293808=CARTESIAN_POINT('Ctrl Pts',(-2.65051258500006,15.2,-10.61299384));
#293809=CARTESIAN_POINT('Ctrl Pts',(-2.65051258500006,11.6,-10.61299384));
#293810=CARTESIAN_POINT('Ctrl Pts',(-2.65025002300006,15.2,-10.615933785));
#293811=CARTESIAN_POINT('Ctrl Pts',(-2.65025002300006,11.6,-10.615933785));
#293812=CARTESIAN_POINT('Ctrl Pts',(-2.64998454800006,15.2,-10.618878952));
#293813=CARTESIAN_POINT('Ctrl Pts',(-2.64998454800006,11.6,-10.618878952));
#293814=CARTESIAN_POINT('Ctrl Pts',(-2.64971615600006,15.2,-10.621829333));
#293815=CARTESIAN_POINT('Ctrl Pts',(-2.64971615600006,11.6,-10.621829333));
#293816=CARTESIAN_POINT('Ctrl Pts',(-2.64944484000006,15.2,-10.624784916));
#293817=CARTESIAN_POINT('Ctrl Pts',(-2.64944484000006,11.6,-10.624784916));
#293818=CARTESIAN_POINT('Ctrl Pts',(-2.64917059300006,15.2,-10.627745692));
#293819=CARTESIAN_POINT('Ctrl Pts',(-2.64917059300006,11.6,-10.627745692));
#293820=CARTESIAN_POINT('Ctrl Pts',(-2.64889340700006,15.2,-10.63071165));
#293821=CARTESIAN_POINT('Ctrl Pts',(-2.64889340700006,11.6,-10.63071165));
#293822=CARTESIAN_POINT('Ctrl Pts',(-2.64861327700005,15.2,-10.63368278));
#293823=CARTESIAN_POINT('Ctrl Pts',(-2.64861327700005,11.6,-10.63368278));
#293824=CARTESIAN_POINT('Ctrl Pts',(-2.64833019600006,15.2,-10.636659071));
#293825=CARTESIAN_POINT('Ctrl Pts',(-2.64833019600006,11.6,-10.636659071));
#293826=CARTESIAN_POINT('Ctrl Pts',(-2.64804415600006,15.2,-10.639640512));
#293827=CARTESIAN_POINT('Ctrl Pts',(-2.64804415600006,11.6,-10.639640512));
#293828=CARTESIAN_POINT('Ctrl Pts',(-2.64775515200005,15.2,-10.642627095));
#293829=CARTESIAN_POINT('Ctrl Pts',(-2.64775515200005,11.6,-10.642627095));
#293830=CARTESIAN_POINT('Ctrl Pts',(-2.64746317600005,15.2,-10.645618808));
#293831=CARTESIAN_POINT('Ctrl Pts',(-2.64746317600005,11.6,-10.645618808));
#293832=CARTESIAN_POINT('Ctrl Pts',(-2.64716822300006,15.2,-10.648615642));
#293833=CARTESIAN_POINT('Ctrl Pts',(-2.64716822300006,11.6,-10.648615642));
#293834=CARTESIAN_POINT('Ctrl Pts',(-2.64687028500005,15.2,-10.651617586));
#293835=CARTESIAN_POINT('Ctrl Pts',(-2.64687028500005,11.6,-10.651617586));
#293836=CARTESIAN_POINT('Ctrl Pts',(-2.64656935600006,15.2,-10.654624629));
#293837=CARTESIAN_POINT('Ctrl Pts',(-2.64656935600006,11.6,-10.654624629));
#293838=CARTESIAN_POINT('Ctrl Pts',(-2.64626543000006,15.2,-10.657636763));
#293839=CARTESIAN_POINT('Ctrl Pts',(-2.64626543000006,11.6,-10.657636763));
#293840=CARTESIAN_POINT('Ctrl Pts',(-2.64595849900005,15.2,-10.660653975));
#293841=CARTESIAN_POINT('Ctrl Pts',(-2.64595849900005,11.6,-10.660653975));
#293842=CARTESIAN_POINT('Ctrl Pts',(-2.64564855800006,15.2,-10.663676257));
#293843=CARTESIAN_POINT('Ctrl Pts',(-2.64564855800006,11.6,-10.663676257));
#293844=CARTESIAN_POINT('Ctrl Pts',(-2.64533560000006,15.2,-10.666703598));
#293845=CARTESIAN_POINT('Ctrl Pts',(-2.64533560000006,11.6,-10.666703598));
#293846=CARTESIAN_POINT('Ctrl Pts',(-2.64501961800006,15.2,-10.669735989));
#293847=CARTESIAN_POINT('Ctrl Pts',(-2.64501961800006,11.6,-10.669735989));
#293848=CARTESIAN_POINT('Ctrl Pts',(-2.64470060600006,15.2,-10.672773418));
#293849=CARTESIAN_POINT('Ctrl Pts',(-2.64470060600006,11.6,-10.672773418));
#293850=CARTESIAN_POINT('Ctrl Pts',(-2.64437855800006,15.2,-10.675815877));
#293851=CARTESIAN_POINT('Ctrl Pts',(-2.64437855800006,11.6,-10.675815877));
#293852=CARTESIAN_POINT('Ctrl Pts',(-2.64405346800006,15.2,-10.678863354));
#293853=CARTESIAN_POINT('Ctrl Pts',(-2.64405346800006,11.6,-10.678863354));
#293854=CARTESIAN_POINT('Ctrl Pts',(-2.64372532800006,15.2,-10.681915841));
#293855=CARTESIAN_POINT('Ctrl Pts',(-2.64372532800006,11.6,-10.681915841));
#293856=CARTESIAN_POINT('Ctrl Pts',(-2.64339413300006,15.2,-10.684973325));
#293857=CARTESIAN_POINT('Ctrl Pts',(-2.64339413300006,11.6,-10.684973325));
#293858=CARTESIAN_POINT('Ctrl Pts',(-2.64305987700005,15.2,-10.688035798));
#293859=CARTESIAN_POINT('Ctrl Pts',(-2.64305987700005,11.6,-10.688035798));
#293860=CARTESIAN_POINT('Ctrl Pts',(-2.64272255200006,15.2,-10.691103251));
#293861=CARTESIAN_POINT('Ctrl Pts',(-2.64272255200006,11.6,-10.691103251));
#293862=CARTESIAN_POINT('Ctrl Pts',(-2.64238215300006,15.2,-10.694175673));
#293863=CARTESIAN_POINT('Ctrl Pts',(-2.64238215300006,11.6,-10.694175673));
#293864=CARTESIAN_POINT('Ctrl Pts',(-2.64203867400005,15.2,-10.697253053));
#293865=CARTESIAN_POINT('Ctrl Pts',(-2.64203867400005,11.6,-10.697253053));
#293866=CARTESIAN_POINT('Ctrl Pts',(-2.64169210800006,15.2,-10.700335382));
#293867=CARTESIAN_POINT('Ctrl Pts',(-2.64169210800006,11.6,-10.700335382));
#293868=CARTESIAN_POINT('Ctrl Pts',(-2.64134244900006,15.2,-10.703422651));
#293869=CARTESIAN_POINT('Ctrl Pts',(-2.64134244900006,11.6,-10.703422651));
#293870=CARTESIAN_POINT('Ctrl Pts',(-2.64098969100006,15.2,-10.706514848));
#293871=CARTESIAN_POINT('Ctrl Pts',(-2.64098969100006,11.6,-10.706514848));
#293872=CARTESIAN_POINT('Ctrl Pts',(-2.64063382800006,15.2,-10.709611965));
#293873=CARTESIAN_POINT('Ctrl Pts',(-2.64063382800006,11.6,-10.709611965));
#293874=CARTESIAN_POINT('Ctrl Pts',(-2.64027485200006,15.2,-10.712713991));
#293875=CARTESIAN_POINT('Ctrl Pts',(-2.64027485200006,11.6,-10.712713991));
#293876=CARTESIAN_POINT('Ctrl Pts',(-2.63991276100006,15.2,-10.715820916));
#293877=CARTESIAN_POINT('Ctrl Pts',(-2.63991276100006,11.6,-10.715820916));
#293878=CARTESIAN_POINT('Ctrl Pts',(-2.63954754500006,15.2,-10.718932731));
#293879=CARTESIAN_POINT('Ctrl Pts',(-2.63954754500006,11.6,-10.718932731));
#293880=CARTESIAN_POINT('Ctrl Pts',(-2.63917919900006,15.2,-10.722049426));
#293881=CARTESIAN_POINT('Ctrl Pts',(-2.63917919900006,11.6,-10.722049426));
#293882=CARTESIAN_POINT('Ctrl Pts',(-2.63880771700005,15.2,-10.725170991));
#293883=CARTESIAN_POINT('Ctrl Pts',(-2.63880771700005,11.6,-10.725170991));
#293884=CARTESIAN_POINT('Ctrl Pts',(-2.63843309400006,15.2,-10.728297416));
#293885=CARTESIAN_POINT('Ctrl Pts',(-2.63843309400006,11.6,-10.728297416));
#293886=CARTESIAN_POINT('Ctrl Pts',(-2.63805532400006,15.2,-10.731428692));
#293887=CARTESIAN_POINT('Ctrl Pts',(-2.63805532400006,11.6,-10.731428692));
#293888=CARTESIAN_POINT('Ctrl Pts',(-2.63767439800006,15.2,-10.734564808));
#293889=CARTESIAN_POINT('Ctrl Pts',(-2.63767439800006,11.6,-10.734564808));
#293890=CARTESIAN_POINT('Ctrl Pts',(-2.63729031400006,15.2,-10.737705755));
#293891=CARTESIAN_POINT('Ctrl Pts',(-2.63729031400006,11.6,-10.737705755));
#293892=CARTESIAN_POINT('Ctrl Pts',(-2.63690306200006,15.2,-10.740851524));
#293893=CARTESIAN_POINT('Ctrl Pts',(-2.63690306200006,11.6,-10.740851524));
#293894=CARTESIAN_POINT('Ctrl Pts',(-2.63651264000006,15.2,-10.744002104));
#293895=CARTESIAN_POINT('Ctrl Pts',(-2.63651264000006,11.6,-10.744002104));
#293896=CARTESIAN_POINT('Ctrl Pts',(-2.63611904100005,15.2,-10.747157485));
#293897=CARTESIAN_POINT('Ctrl Pts',(-2.63611904100005,11.6,-10.747157485));
#293898=CARTESIAN_POINT('Ctrl Pts',(-2.63572225700006,15.2,-10.750317658));
#293899=CARTESIAN_POINT('Ctrl Pts',(-2.63572225700006,11.6,-10.750317658));
#293900=CARTESIAN_POINT('Ctrl Pts',(-2.63532228500006,15.2,-10.753482615));
#293901=CARTESIAN_POINT('Ctrl Pts',(-2.63532228500006,11.6,-10.753482615));
#293902=CARTESIAN_POINT('Ctrl Pts',(-2.63491911700005,15.2,-10.756652345));
#293903=CARTESIAN_POINT('Ctrl Pts',(-2.63491911700005,11.6,-10.756652345));
#293904=CARTESIAN_POINT('Ctrl Pts',(-2.63451274800006,15.2,-10.759826836));
#293905=CARTESIAN_POINT('Ctrl Pts',(-2.63451274800006,11.6,-10.759826836));
#293906=CARTESIAN_POINT('Ctrl Pts',(-2.63410317200006,15.2,-10.763006082));
#293907=CARTESIAN_POINT('Ctrl Pts',(-2.63410317200006,11.6,-10.763006082));
#293908=CARTESIAN_POINT('Ctrl Pts',(-2.63369038300006,15.2,-10.766190071));
#293909=CARTESIAN_POINT('Ctrl Pts',(-2.63369038300006,11.6,-10.766190071));
#293910=CARTESIAN_POINT('Ctrl Pts',(-2.63327437600006,15.2,-10.769378796));
#293911=CARTESIAN_POINT('Ctrl Pts',(-2.63327437600006,11.6,-10.769378796));
#293912=CARTESIAN_POINT('Ctrl Pts',(-2.63285514500006,15.2,-10.772572244));
#293913=CARTESIAN_POINT('Ctrl Pts',(-2.63285514500006,11.6,-10.772572244));
#293914=CARTESIAN_POINT('Ctrl Pts',(-2.63243268300006,15.2,-10.775770408));
#293915=CARTESIAN_POINT('Ctrl Pts',(-2.63243268300006,11.6,-10.775770408));
#293916=CARTESIAN_POINT('Ctrl Pts',(-2.63200698600006,15.2,-10.778973278));
#293917=CARTESIAN_POINT('Ctrl Pts',(-2.63200698600006,11.6,-10.778973278));
#293918=CARTESIAN_POINT('Ctrl Pts',(-2.63157804800006,15.2,-10.782180844));
#293919=CARTESIAN_POINT('Ctrl Pts',(-2.63157804800006,11.6,-10.782180844));
#293920=CARTESIAN_POINT('Ctrl Pts',(-2.63114586200006,15.2,-10.785393096));
#293921=CARTESIAN_POINT('Ctrl Pts',(-2.63114586200006,11.6,-10.785393096));
#293922=CARTESIAN_POINT('Ctrl Pts',(-2.63071042300006,15.2,-10.788610025));
#293923=CARTESIAN_POINT('Ctrl Pts',(-2.63071042300006,11.6,-10.788610025));
#293924=CARTESIAN_POINT('Ctrl Pts',(-2.63027172600005,15.2,-10.791831622));
#293925=CARTESIAN_POINT('Ctrl Pts',(-2.63027172600005,11.6,-10.791831622));
#293926=CARTESIAN_POINT('Ctrl Pts',(-2.62982976500005,15.2,-10.795057878));
#293927=CARTESIAN_POINT('Ctrl Pts',(-2.62982976500005,11.6,-10.795057878));
#293928=CARTESIAN_POINT('Ctrl Pts',(-2.62938453600006,15.2,-10.798288782));
#293929=CARTESIAN_POINT('Ctrl Pts',(-2.62938453600006,11.6,-10.798288782));
#293930=CARTESIAN_POINT('Ctrl Pts',(-2.62893603000005,15.2,-10.801524326));
#293931=CARTESIAN_POINT('Ctrl Pts',(-2.62893603000005,11.6,-10.801524326));
#293932=CARTESIAN_POINT('Ctrl Pts',(-2.62848424300006,15.2,-10.804764499));
#293933=CARTESIAN_POINT('Ctrl Pts',(-2.62848424300006,11.6,-10.804764499));
#293934=CARTESIAN_POINT('Ctrl Pts',(-2.62802917100006,15.2,-10.808009292));
#293935=CARTESIAN_POINT('Ctrl Pts',(-2.62802917100006,11.6,-10.808009292));
#293936=CARTESIAN_POINT('Ctrl Pts',(-2.62757080600006,15.2,-10.811258697));
#293937=CARTESIAN_POINT('Ctrl Pts',(-2.62757080600006,11.6,-10.811258697));
#293938=CARTESIAN_POINT('Ctrl Pts',(-2.62710914400006,15.2,-10.814512704));
#293939=CARTESIAN_POINT('Ctrl Pts',(-2.62710914400006,11.6,-10.814512704));
#293940=CARTESIAN_POINT('Ctrl Pts',(-2.62664417900006,15.2,-10.817771302));
#293941=CARTESIAN_POINT('Ctrl Pts',(-2.62664417900006,11.6,-10.817771302));
#293942=CARTESIAN_POINT('Ctrl Pts',(-2.62617590600006,15.2,-10.821034484));
#293943=CARTESIAN_POINT('Ctrl Pts',(-2.62617590600006,11.6,-10.821034484));
#293944=CARTESIAN_POINT('Ctrl Pts',(-2.62570431900006,15.2,-10.82430224));
#293945=CARTESIAN_POINT('Ctrl Pts',(-2.62570431900006,11.6,-10.82430224));
#293946=CARTESIAN_POINT('Ctrl Pts',(-2.62522941300006,15.2,-10.82757456));
#293947=CARTESIAN_POINT('Ctrl Pts',(-2.62522941300006,11.6,-10.82757456));
#293948=CARTESIAN_POINT('Ctrl Pts',(-2.62475118200005,15.2,-10.830851435));
#293949=CARTESIAN_POINT('Ctrl Pts',(-2.62475118200005,11.6,-10.830851435));
#293950=CARTESIAN_POINT('Ctrl Pts',(-2.62426962100006,15.2,-10.834132855));
#293951=CARTESIAN_POINT('Ctrl Pts',(-2.62426962100006,11.6,-10.834132855));
#293952=CARTESIAN_POINT('Ctrl Pts',(-2.62378472400006,15.2,-10.837418812));
#293953=CARTESIAN_POINT('Ctrl Pts',(-2.62378472400006,11.6,-10.837418812));
#293954=CARTESIAN_POINT('Ctrl Pts',(-2.62329648700006,15.2,-10.840709295));
#293955=CARTESIAN_POINT('Ctrl Pts',(-2.62329648700006,11.6,-10.840709295));
#293956=CARTESIAN_POINT('Ctrl Pts',(-2.62280490400005,15.2,-10.844004298));
#293957=CARTESIAN_POINT('Ctrl Pts',(-2.62280490400005,11.6,-10.844004298));
#293958=CARTESIAN_POINT('Ctrl Pts',(-2.62230997000006,15.2,-10.847303808));
#293959=CARTESIAN_POINT('Ctrl Pts',(-2.62230997000006,11.6,-10.847303808));
#293960=CARTESIAN_POINT('Ctrl Pts',(-2.62181167800006,15.2,-10.850607819));
#293961=CARTESIAN_POINT('Ctrl Pts',(-2.62181167800006,11.6,-10.850607819));
#293962=CARTESIAN_POINT('Ctrl Pts',(-2.62131002400006,15.2,-10.853916319));
#293963=CARTESIAN_POINT('Ctrl Pts',(-2.62131002400006,11.6,-10.853916319));
#293964=CARTESIAN_POINT('Ctrl Pts',(-2.62080500300006,15.2,-10.857229301));
#293965=CARTESIAN_POINT('Ctrl Pts',(-2.62080500300006,11.6,-10.857229301));
#293966=CARTESIAN_POINT('Ctrl Pts',(-2.62029660900006,15.2,-10.860546754));
#293967=CARTESIAN_POINT('Ctrl Pts',(-2.62029660900006,11.6,-10.860546754));
#293968=CARTESIAN_POINT('Ctrl Pts',(-2.61978483700006,15.2,-10.863868671));
#293969=CARTESIAN_POINT('Ctrl Pts',(-2.61978483700006,11.6,-10.863868671));
#293970=CARTESIAN_POINT('Ctrl Pts',(-2.61926968300005,15.2,-10.86719504));
#293971=CARTESIAN_POINT('Ctrl Pts',(-2.61926968300005,11.6,-10.86719504));
#293972=CARTESIAN_POINT('Ctrl Pts',(-2.61875114000006,15.2,-10.870525854));
#293973=CARTESIAN_POINT('Ctrl Pts',(-2.61875114000006,11.6,-10.870525854));
#293974=CARTESIAN_POINT('Ctrl Pts',(-2.61822920300005,15.2,-10.873861104));
#293975=CARTESIAN_POINT('Ctrl Pts',(-2.61822920300005,11.6,-10.873861104));
#293976=CARTESIAN_POINT('Ctrl Pts',(-2.61770386800006,15.2,-10.877200779));
#293977=CARTESIAN_POINT('Ctrl Pts',(-2.61770386800006,11.6,-10.877200779));
#293978=CARTESIAN_POINT('Ctrl Pts',(-2.61717512900006,15.2,-10.880544872));
#293979=CARTESIAN_POINT('Ctrl Pts',(-2.61717512900006,11.6,-10.880544872));
#293980=CARTESIAN_POINT('Ctrl Pts',(-2.61664298100006,15.2,-10.883893373));
#293981=CARTESIAN_POINT('Ctrl Pts',(-2.61664298100006,11.6,-10.883893373));
#293982=CARTESIAN_POINT('Ctrl Pts',(-2.61610741900005,15.2,-10.887246272));
#293983=CARTESIAN_POINT('Ctrl Pts',(-2.61610741900005,11.6,-10.887246272));
#293984=CARTESIAN_POINT('Ctrl Pts',(-2.61556843800005,15.2,-10.890603561));
#293985=CARTESIAN_POINT('Ctrl Pts',(-2.61556843800005,11.6,-10.890603561));
#293986=CARTESIAN_POINT('Ctrl Pts',(-2.61502603200006,15.2,-10.893965232));
#293987=CARTESIAN_POINT('Ctrl Pts',(-2.61502603200006,11.6,-10.893965232));
#293988=CARTESIAN_POINT('Ctrl Pts',(-2.61448019800006,15.2,-10.897331274));
#293989=CARTESIAN_POINT('Ctrl Pts',(-2.61448019800006,11.6,-10.897331274));
#293990=CARTESIAN_POINT('Ctrl Pts',(-2.61393092800006,15.2,-10.900701679));
#293991=CARTESIAN_POINT('Ctrl Pts',(-2.61393092800006,11.6,-10.900701679));
#293992=CARTESIAN_POINT('Ctrl Pts',(-2.61337822000006,15.2,-10.904076438));
#293993=CARTESIAN_POINT('Ctrl Pts',(-2.61337822000006,11.6,-10.904076438));
#293994=CARTESIAN_POINT('Ctrl Pts',(-2.61282206700006,15.2,-10.907455541));
#293995=CARTESIAN_POINT('Ctrl Pts',(-2.61282206700006,11.6,-10.907455541));
#293996=CARTESIAN_POINT('Ctrl Pts',(-2.61226246400006,15.2,-10.91083898));
#293997=CARTESIAN_POINT('Ctrl Pts',(-2.61226246400006,11.6,-10.91083898));
#293998=CARTESIAN_POINT('Ctrl Pts',(-2.61169940800006,15.2,-10.914226746));
#293999=CARTESIAN_POINT('Ctrl Pts',(-2.61169940800006,11.6,-10.914226746));
#294000=CARTESIAN_POINT('Ctrl Pts',(-2.61113289100006,15.2,-10.91761883));
#294001=CARTESIAN_POINT('Ctrl Pts',(-2.61113289100006,11.6,-10.91761883));
#294002=CARTESIAN_POINT('Ctrl Pts',(-2.61056291100005,15.2,-10.921015223));
#294003=CARTESIAN_POINT('Ctrl Pts',(-2.61056291100005,11.6,-10.921015223));
#294004=CARTESIAN_POINT('Ctrl Pts',(-2.60998946100006,15.2,-10.924415916));
#294005=CARTESIAN_POINT('Ctrl Pts',(-2.60998946100006,11.6,-10.924415916));
#294006=CARTESIAN_POINT('Ctrl Pts',(-2.60941253700006,15.2,-10.9278209));
#294007=CARTESIAN_POINT('Ctrl Pts',(-2.60941253700006,11.6,-10.9278209));
#294008=CARTESIAN_POINT('Ctrl Pts',(-2.60883213400006,15.2,-10.931230167));
#294009=CARTESIAN_POINT('Ctrl Pts',(-2.60883213400006,11.6,-10.931230167));
#294010=CARTESIAN_POINT('Ctrl Pts',(-2.60824824700005,15.2,-10.934643706));
#294011=CARTESIAN_POINT('Ctrl Pts',(-2.60824824700005,11.6,-10.934643706));
#294012=CARTESIAN_POINT('Ctrl Pts',(-2.60766087100006,15.2,-10.93806151));
#294013=CARTESIAN_POINT('Ctrl Pts',(-2.60766087100006,11.6,-10.93806151));
#294014=CARTESIAN_POINT('Ctrl Pts',(-2.60707000100005,15.2,-10.94148357));
#294015=CARTESIAN_POINT('Ctrl Pts',(-2.60707000100005,11.6,-10.94148357));
#294016=CARTESIAN_POINT('Ctrl Pts',(-2.60647563300005,15.2,-10.944909876));
#294017=CARTESIAN_POINT('Ctrl Pts',(-2.60647563300005,11.6,-10.944909876));
#294018=CARTESIAN_POINT('Ctrl Pts',(-2.60587776200006,15.2,-10.948340421));
#294019=CARTESIAN_POINT('Ctrl Pts',(-2.60587776200006,11.6,-10.948340421));
#294020=CARTESIAN_POINT('Ctrl Pts',(-2.60527638100006,15.2,-10.951775194));
#294021=CARTESIAN_POINT('Ctrl Pts',(-2.60527638100006,11.6,-10.951775194));
#294022=CARTESIAN_POINT('Ctrl Pts',(-2.60467148900006,15.2,-10.955214187));
#294023=CARTESIAN_POINT('Ctrl Pts',(-2.60467148900006,11.6,-10.955214187));
#294024=CARTESIAN_POINT('Ctrl Pts',(-2.60406307900006,15.2,-10.958657392));
#294025=CARTESIAN_POINT('Ctrl Pts',(-2.60406307900006,11.6,-10.958657392));
#294026=CARTESIAN_POINT('Ctrl Pts',(-2.60345114600006,15.2,-10.9621048));
#294027=CARTESIAN_POINT('Ctrl Pts',(-2.60345114600006,11.6,-10.9621048));
#294028=CARTESIAN_POINT('Ctrl Pts',(-2.60283568600005,15.2,-10.965556401));
#294029=CARTESIAN_POINT('Ctrl Pts',(-2.60283568600005,11.6,-10.965556401));
#294030=CARTESIAN_POINT('Ctrl Pts',(-2.60221669300006,15.2,-10.969012188));
#294031=CARTESIAN_POINT('Ctrl Pts',(-2.60221669300006,11.6,-10.969012188));
#294032=CARTESIAN_POINT('Ctrl Pts',(-2.60159416500006,15.2,-10.972472151));
#294033=CARTESIAN_POINT('Ctrl Pts',(-2.60159416500006,11.6,-10.972472151));
#294034=CARTESIAN_POINT('Ctrl Pts',(-2.60096809500005,15.2,-10.975936281));
#294035=CARTESIAN_POINT('Ctrl Pts',(-2.60096809500005,11.6,-10.975936281));
#294036=CARTESIAN_POINT('Ctrl Pts',(-2.60033847900006,15.2,-10.979404571));
#294037=CARTESIAN_POINT('Ctrl Pts',(-2.60033847900006,11.6,-10.979404571));
#294038=CARTESIAN_POINT('Ctrl Pts',(-2.59970531300006,15.2,-10.98287701));
#294039=CARTESIAN_POINT('Ctrl Pts',(-2.59970531300006,11.6,-10.98287701));
#294040=CARTESIAN_POINT('Ctrl Pts',(-2.59906859000006,15.2,-10.986353591));
#294041=CARTESIAN_POINT('Ctrl Pts',(-2.59906859000006,11.6,-10.986353591));
#294042=CARTESIAN_POINT('Ctrl Pts',(-2.59842830800005,15.2,-10.989834305));
#294043=CARTESIAN_POINT('Ctrl Pts',(-2.59842830800005,11.6,-10.989834305));
#294044=CARTESIAN_POINT('Ctrl Pts',(-2.59778446200006,15.2,-10.993319143));
#294045=CARTESIAN_POINT('Ctrl Pts',(-2.59778446200006,11.6,-10.993319143));
#294046=CARTESIAN_POINT('Ctrl Pts',(-2.59713704700005,15.2,-10.996808096));
#294047=CARTESIAN_POINT('Ctrl Pts',(-2.59713704700005,11.6,-10.996808096));
#294048=CARTESIAN_POINT('Ctrl Pts',(-2.59648605700006,15.2,-11.000301157));
#294049=CARTESIAN_POINT('Ctrl Pts',(-2.59648605700006,11.6,-11.000301157));
#294050=CARTESIAN_POINT('Ctrl Pts',(-2.59583148900006,15.2,-11.003798315));
#294051=CARTESIAN_POINT('Ctrl Pts',(-2.59583148900006,11.6,-11.003798315));
#294052=CARTESIAN_POINT('Ctrl Pts',(-2.59517333800006,15.2,-11.007299564));
#294053=CARTESIAN_POINT('Ctrl Pts',(-2.59517333800006,11.6,-11.007299564));
#294054=CARTESIAN_POINT('Ctrl Pts',(-2.59451160000005,15.2,-11.010804893));
#294055=CARTESIAN_POINT('Ctrl Pts',(-2.59451160000005,11.6,-11.010804893));
#294056=CARTESIAN_POINT('Ctrl Pts',(-2.59384627000005,15.2,-11.014314294));
#294057=CARTESIAN_POINT('Ctrl Pts',(-2.59384627000005,11.6,-11.014314294));
#294058=CARTESIAN_POINT('Ctrl Pts',(-2.59317734300006,15.2,-11.017827759));
#294059=CARTESIAN_POINT('Ctrl Pts',(-2.59317734300006,11.6,-11.017827759));
#294060=CARTESIAN_POINT('Ctrl Pts',(-2.59250481600006,15.2,-11.021345279));
#294061=CARTESIAN_POINT('Ctrl Pts',(-2.59250481600006,11.6,-11.021345279));
#294062=CARTESIAN_POINT('Ctrl Pts',(-2.59182868400006,15.2,-11.024866846));
#294063=CARTESIAN_POINT('Ctrl Pts',(-2.59182868400006,11.6,-11.024866846));
#294064=CARTESIAN_POINT('Ctrl Pts',(-2.59114894000006,15.2,-11.02839245));
#294065=CARTESIAN_POINT('Ctrl Pts',(-2.59114894000006,11.6,-11.02839245));
#294066=CARTESIAN_POINT('Ctrl Pts',(-2.59046558300006,15.2,-11.031922084));
#294067=CARTESIAN_POINT('Ctrl Pts',(-2.59046558300006,11.6,-11.031922084));
#294068=CARTESIAN_POINT('Ctrl Pts',(-2.58977860700006,15.2,-11.035455739));
#294069=CARTESIAN_POINT('Ctrl Pts',(-2.58977860700006,11.6,-11.035455739));
#294070=CARTESIAN_POINT('Ctrl Pts',(-2.58908800800006,15.2,-11.038993407));
#294071=CARTESIAN_POINT('Ctrl Pts',(-2.58908800800006,11.6,-11.038993407));
#294072=CARTESIAN_POINT('Ctrl Pts',(-2.58839378100005,15.2,-11.042535078));
#294073=CARTESIAN_POINT('Ctrl Pts',(-2.58839378100005,11.6,-11.042535078));
#294074=CARTESIAN_POINT('Ctrl Pts',(-2.58769592300006,15.2,-11.046080744));
#294075=CARTESIAN_POINT('Ctrl Pts',(-2.58769592300006,11.6,-11.046080744));
#294076=CARTESIAN_POINT('Ctrl Pts',(-2.58699442800005,15.2,-11.049630398));
#294077=CARTESIAN_POINT('Ctrl Pts',(-2.58699442800005,11.6,-11.049630398));
#294078=CARTESIAN_POINT('Ctrl Pts',(-2.58628929200006,15.2,-11.05318403));
#294079=CARTESIAN_POINT('Ctrl Pts',(-2.58628929200006,11.6,-11.05318403));
#294080=CARTESIAN_POINT('Ctrl Pts',(-2.58558051100006,15.2,-11.056741631));
#294081=CARTESIAN_POINT('Ctrl Pts',(-2.58558051100006,11.6,-11.056741631));
#294082=CARTESIAN_POINT('Ctrl Pts',(-2.58486808100006,15.2,-11.060303195));
#294083=CARTESIAN_POINT('Ctrl Pts',(-2.58486808100006,11.6,-11.060303195));
#294084=CARTESIAN_POINT('Ctrl Pts',(-2.58415199700006,15.2,-11.063868711));
#294085=CARTESIAN_POINT('Ctrl Pts',(-2.58415199700006,11.6,-11.063868711));
#294086=CARTESIAN_POINT('Ctrl Pts',(-2.58343225500006,15.2,-11.067438171));
#294087=CARTESIAN_POINT('Ctrl Pts',(-2.58343225500006,11.6,-11.067438171));
#294088=CARTESIAN_POINT('Ctrl Pts',(-2.58270885100006,15.2,-11.071011569));
#294089=CARTESIAN_POINT('Ctrl Pts',(-2.58270885100006,11.6,-11.071011569));
#294090=CARTESIAN_POINT('Ctrl Pts',(-2.58198178000006,15.2,-11.074588893));
#294091=CARTESIAN_POINT('Ctrl Pts',(-2.58198178000006,11.6,-11.074588893));
#294092=CARTESIAN_POINT('Ctrl Pts',(-2.58125103800006,15.2,-11.078170137));
#294093=CARTESIAN_POINT('Ctrl Pts',(-2.58125103800006,11.6,-11.078170137));
#294094=CARTESIAN_POINT('Ctrl Pts',(-2.58051662100006,15.2,-11.081755292));
#294095=CARTESIAN_POINT('Ctrl Pts',(-2.58051662100006,11.6,-11.081755292));
#294096=CARTESIAN_POINT('Ctrl Pts',(-2.57977852500006,15.2,-11.08534435));
#294097=CARTESIAN_POINT('Ctrl Pts',(-2.57977852500006,11.6,-11.08534435));
#294098=CARTESIAN_POINT('Ctrl Pts',(-2.57903674600006,15.2,-11.088937302));
#294099=CARTESIAN_POINT('Ctrl Pts',(-2.57903674600006,11.6,-11.088937302));
#294100=CARTESIAN_POINT('Ctrl Pts',(-2.57829127900005,15.2,-11.09253414));
#294101=CARTESIAN_POINT('Ctrl Pts',(-2.57829127900005,11.6,-11.09253414));
#294102=CARTESIAN_POINT('Ctrl Pts',(-2.57754212000005,15.2,-11.096134855));
#294103=CARTESIAN_POINT('Ctrl Pts',(-2.57754212000005,11.6,-11.096134855));
#294104=CARTESIAN_POINT('Ctrl Pts',(-2.57678926400006,15.2,-11.099739441));
#294105=CARTESIAN_POINT('Ctrl Pts',(-2.57678926400006,11.6,-11.099739441));
#294106=CARTESIAN_POINT('Ctrl Pts',(-2.57603270800006,15.2,-11.103347885));
#294107=CARTESIAN_POINT('Ctrl Pts',(-2.57603270800006,11.6,-11.103347885));
#294108=CARTESIAN_POINT('Ctrl Pts',(-2.57527244700006,15.2,-11.106960183));
#294109=CARTESIAN_POINT('Ctrl Pts',(-2.57527244700006,11.6,-11.106960183));
#294110=CARTESIAN_POINT('Ctrl Pts',(-2.57450847900006,15.2,-11.110576324));
#294111=CARTESIAN_POINT('Ctrl Pts',(-2.57450847900006,11.6,-11.110576324));
#294112=CARTESIAN_POINT('Ctrl Pts',(-2.57374079800006,15.2,-11.114196302));
#294113=CARTESIAN_POINT('Ctrl Pts',(-2.57374079800006,11.6,-11.114196302));
#294114=CARTESIAN_POINT('Ctrl Pts',(-2.57296940000006,15.2,-11.117820108));
#294115=CARTESIAN_POINT('Ctrl Pts',(-2.57296940000006,11.6,-11.117820108));
#294116=CARTESIAN_POINT('Ctrl Pts',(-2.57219428000006,15.2,-11.121447733));
#294117=CARTESIAN_POINT('Ctrl Pts',(-2.57219428000006,11.6,-11.121447733));
#294118=CARTESIAN_POINT('Ctrl Pts',(-2.57141543700006,15.2,-11.125079169));
#294119=CARTESIAN_POINT('Ctrl Pts',(-2.57141543700006,11.6,-11.125079169));
#294120=CARTESIAN_POINT('Ctrl Pts',(-2.57063286500005,15.2,-11.128714409));
#294121=CARTESIAN_POINT('Ctrl Pts',(-2.57063286500005,11.6,-11.128714409));
#294122=CARTESIAN_POINT('Ctrl Pts',(-2.56984656000005,15.2,-11.132353444));
#294123=CARTESIAN_POINT('Ctrl Pts',(-2.56984656000005,11.6,-11.132353444));
#294124=CARTESIAN_POINT('Ctrl Pts',(-2.56905651800006,15.2,-11.135996266));
#294125=CARTESIAN_POINT('Ctrl Pts',(-2.56905651800006,11.6,-11.135996266));
#294126=CARTESIAN_POINT('Ctrl Pts',(-2.56826273400006,15.2,-11.139642864));
#294127=CARTESIAN_POINT('Ctrl Pts',(-2.56826273400006,11.6,-11.139642864));
#294128=CARTESIAN_POINT('Ctrl Pts',(-2.56746520400006,15.2,-11.143293232));
#294129=CARTESIAN_POINT('Ctrl Pts',(-2.56746520400006,11.6,-11.143293232));
#294130=CARTESIAN_POINT('Ctrl Pts',(-2.56666392600006,15.2,-11.146947361));
#294131=CARTESIAN_POINT('Ctrl Pts',(-2.56666392600006,11.6,-11.146947361));
#294132=CARTESIAN_POINT('Ctrl Pts',(-2.56585889400006,15.2,-11.150605243));
#294133=CARTESIAN_POINT('Ctrl Pts',(-2.56585889400006,11.6,-11.150605243));
#294134=CARTESIAN_POINT('Ctrl Pts',(-2.56505010400006,15.2,-11.15426687));
#294135=CARTESIAN_POINT('Ctrl Pts',(-2.56505010400006,11.6,-11.15426687));
#294136=CARTESIAN_POINT('Ctrl Pts',(-2.56423755400006,15.2,-11.157932234));
#294137=CARTESIAN_POINT('Ctrl Pts',(-2.56423755400006,11.6,-11.157932234));
#294138=CARTESIAN_POINT('Ctrl Pts',(-2.56342123900006,15.2,-11.161601329));
#294139=CARTESIAN_POINT('Ctrl Pts',(-2.56342123900006,11.6,-11.161601329));
#294140=CARTESIAN_POINT('Ctrl Pts',(-2.56260115700006,15.2,-11.165274147));
#294141=CARTESIAN_POINT('Ctrl Pts',(-2.56260115700006,11.6,-11.165274147));
#294142=CARTESIAN_POINT('Ctrl Pts',(-2.56177730200006,15.2,-11.16895068));
#294143=CARTESIAN_POINT('Ctrl Pts',(-2.56177730200006,11.6,-11.16895068));
#294144=CARTESIAN_POINT('Ctrl Pts',(-2.56094967200006,15.2,-11.172630919));
#294145=CARTESIAN_POINT('Ctrl Pts',(-2.56094967200006,11.6,-11.172630919));
#294146=CARTESIAN_POINT('Ctrl Pts',(-2.56011826200006,15.2,-11.176314856));
#294147=CARTESIAN_POINT('Ctrl Pts',(-2.56011826200006,11.6,-11.176314856));
#294148=CARTESIAN_POINT('Ctrl Pts',(-2.55928306700006,15.2,-11.18000248));
#294149=CARTESIAN_POINT('Ctrl Pts',(-2.55928306700006,11.6,-11.18000248));
#294150=CARTESIAN_POINT('Ctrl Pts',(-2.55844408200006,15.2,-11.183693781));
#294151=CARTESIAN_POINT('Ctrl Pts',(-2.55844408200006,11.6,-11.183693781));
#294152=CARTESIAN_POINT('Ctrl Pts',(-2.55760130200006,15.2,-11.18738875));
#294153=CARTESIAN_POINT('Ctrl Pts',(-2.55760130200006,11.6,-11.18738875));
#294154=CARTESIAN_POINT('Ctrl Pts',(-2.55675472300006,15.2,-11.191087378));
#294155=CARTESIAN_POINT('Ctrl Pts',(-2.55675472300006,11.6,-11.191087378));
#294156=CARTESIAN_POINT('Ctrl Pts',(-2.55590434200006,15.2,-11.194789656));
#294157=CARTESIAN_POINT('Ctrl Pts',(-2.55590434200006,11.6,-11.194789656));
#294158=CARTESIAN_POINT('Ctrl Pts',(-2.55505015600006,15.2,-11.198495579));
#294159=CARTESIAN_POINT('Ctrl Pts',(-2.55505015600006,11.6,-11.198495579));
#294160=CARTESIAN_POINT('Ctrl Pts',(-2.55419216400006,15.2,-11.202205146));
#294161=CARTESIAN_POINT('Ctrl Pts',(-2.55419216400006,11.6,-11.202205146));
#294162=CARTESIAN_POINT('Ctrl Pts',(-2.55333036400006,15.2,-11.205918353));
#294163=CARTESIAN_POINT('Ctrl Pts',(-2.55333036400006,11.6,-11.205918353));
#294164=CARTESIAN_POINT('Ctrl Pts',(-2.55263787800006,15.2,-11.20889183));
#294165=CARTESIAN_POINT('Ctrl Pts',(-2.55263787800006,11.6,-11.20889183));
#294166=CARTESIAN_POINT('Ctrl Pts',(-2.55211680100006,15.2,-11.211123574));
#294167=CARTESIAN_POINT('Ctrl Pts',(-2.55211680100006,11.6,-11.211123574));
#294168=CARTESIAN_POINT('Ctrl Pts',(-2.55176865500006,15.2,-11.212612131));
#294169=CARTESIAN_POINT('Ctrl Pts',(-2.55176865500006,11.6,-11.212612131));
#294170=CARTESIAN_POINT('Ctrl Pts',(-2.55159439100006,15.2,-11.213356592));
#294171=CARTESIAN_POINT('Ctrl Pts',(-2.55159439100006,11.6,-11.213356592));
#294172=CARTESIAN_POINT('Ctrl Pts',(-2.64164356400005,15.2,-10.033062558));
#294173=CARTESIAN_POINT('Ctrl Pts',(-2.64194832280646,15.2,-10.0348230291495));
#294174=CARTESIAN_POINT('Ctrl Pts',(-2.64225752123829,15.2,-10.0366407490542));
#294175=CARTESIAN_POINT('Ctrl Pts',(-2.64257038372412,15.2,-10.0385148613197));
#294176=CARTESIAN_POINT('Ctrl Pts',(-2.642884754991,15.2,-10.0403980115018));
#294177=CARTESIAN_POINT('Ctrl Pts',(-2.64320281628075,15.2,-10.0423381055564));
#294178=CARTESIAN_POINT('Ctrl Pts',(-2.64352378181444,15.2,-10.0443343061848));
#294179=CARTESIAN_POINT('Ctrl Pts',(-2.64384474731898,15.2,-10.046330506632));
#294180=CARTESIAN_POINT('Ctrl Pts',(-2.64416861707023,15.2,-10.0483828179432));
#294181=CARTESIAN_POINT('Ctrl Pts',(-2.64449462947505,15.2,-10.0504904280332));
#294182=CARTESIAN_POINT('Ctrl Pts',(-2.64482064187987,15.2,-10.0525980381233));
#294183=CARTESIAN_POINT('Ctrl Pts',(-2.64514879650543,15.1999999999999,
-10.0547609446918));
#294184=CARTESIAN_POINT('Ctrl Pts',(-2.64547835425984,15.2,-10.0569783620522));
#294185=CARTESIAN_POINT('Ctrl Pts',(-2.64580791204419,15.2,-10.059195779614));
#294186=CARTESIAN_POINT('Ctrl Pts',(-2.64613887655142,15.2,-10.061467706473));
#294187=CARTESIAN_POINT('Ctrl Pts',(-2.64647052756954,15.2,-10.0637933712701));
#294188=CARTESIAN_POINT('Ctrl Pts',(-2.64680217855753,15.2,-10.0661190358559));
#294189=CARTESIAN_POINT('Ctrl Pts',(-2.64713452030244,15.2,-10.0684984401782));
#294190=CARTESIAN_POINT('Ctrl Pts',(-2.64746685620854,15.2,-10.0709308317677));
#294191=CARTESIAN_POINT('Ctrl Pts',(-2.64779919211464,15.2,-10.0733632233572));
#294192=CARTESIAN_POINT('Ctrl Pts',(-2.64813152490233,15.2,-10.0758486046313));
#294193=CARTESIAN_POINT('Ctrl Pts',(-2.64846317797365,15.2,-10.0783862401202));
#294194=CARTESIAN_POINT('Ctrl Pts',(-2.64879483107508,15.2,-10.0809238758395));
#294195=CARTESIAN_POINT('Ctrl Pts',(-2.64912580739311,15.2,-10.0835137670404));
#294196=CARTESIAN_POINT('Ctrl Pts',(-2.64945545332766,15.2,-10.0861551970212));
#294197=CARTESIAN_POINT('Ctrl Pts',(-2.64978509923225,15.2,-10.088796626762));
#294198=CARTESIAN_POINT('Ctrl Pts',(-2.65011341197145,15.2,-10.0914895979888));
#294199=CARTESIAN_POINT('Ctrl Pts',(-2.65043976104284,15.2,-10.0942334086413));
#294200=CARTESIAN_POINT('Ctrl Pts',(-2.65076611011422,15.2,-10.0969772192938));
#294201=CARTESIAN_POINT('Ctrl Pts',(-2.65109049354409,15.2,-10.099771869884));
#294202=CARTESIAN_POINT('Ctrl Pts',(-2.65141229569918,15.2,-10.1026166776118));
#294203=CARTESIAN_POINT('Ctrl Pts',(-2.65173409785426,15.2,-10.1054614853395));
#294204=CARTESIAN_POINT('Ctrl Pts',(-2.65205331640188,15.2,-10.108356448881));
#294205=CARTESIAN_POINT('Ctrl Pts',(-2.65236935747395,15.2,-10.1113009016873));
#294206=CARTESIAN_POINT('Ctrl Pts',(-2.65268539857472,15.2,-10.1142453547611));
#294207=CARTESIAN_POINT('Ctrl Pts',(-2.65299825684187,15.2,-10.117239296673));
#294208=CARTESIAN_POINT('Ctrl Pts',(-2.65330735327523,15.2,-10.1202820709243));
#294209=CARTESIAN_POINT('Ctrl Pts',(-2.6536164496805,15.2,-10.1233248448992));
#294210=CARTESIAN_POINT('Ctrl Pts',(-2.65392178424282,15.2,-10.1264164543317));
#294211=CARTESIAN_POINT('Ctrl Pts',(-2.65422278873326,15.2,-10.1295562562318));
#294212=CARTESIAN_POINT('Ctrl Pts',(-2.6545237932237,15.2,-10.1326960581319));
#294213=CARTESIAN_POINT('Ctrl Pts',(-2.6548204693202,15.2,-10.1358840535347));
#294214=CARTESIAN_POINT('Ctrl Pts',(-2.65511226572659,15.2,-10.1391196154139));
#294215=CARTESIAN_POINT('Ctrl Pts',(-2.65540406215949,15.2,-10.142355177587));
#294216=CARTESIAN_POINT('Ctrl Pts',(-2.65569097776695,15.2,-10.1456383044564));
#294217=CARTESIAN_POINT('Ctrl Pts',(-2.65597247828205,15.2,-10.1489683828899));
#294218=CARTESIAN_POINT('Ctrl Pts',(-2.65625397877158,15.2,-10.152298461021));
#294219=CARTESIAN_POINT('Ctrl Pts',(-2.65653006180852,15.2,-10.1556754927156));
#294220=CARTESIAN_POINT('Ctrl Pts',(-2.65680020829994,15.2,-10.1590988700234));
#294221=CARTESIAN_POINT('Ctrl Pts',(-2.65707035479137,15.2,-10.1625222473311));
#294222=CARTESIAN_POINT('Ctrl Pts',(-2.65733456181423,15.2,-10.1659919742893));
#294223=CARTESIAN_POINT('Ctrl Pts',(-2.65759232347197,15.2,-10.1695074575751));
#294224=CARTESIAN_POINT('Ctrl Pts',(-2.65785008515312,15.2,-10.1730229411802));
#294225=CARTESIAN_POINT('Ctrl Pts',(-2.65810140084023,15.2,-10.1765841834696));
#294226=CARTESIAN_POINT('Ctrl Pts',(-2.65834577378202,15.2,-10.1801906021823));
#294227=CARTESIAN_POINT('Ctrl Pts',(-2.65859014670161,15.2,-10.1837970205673));
#294228=CARTESIAN_POINT('Ctrl Pts',(-2.65882758030843,15.2,-10.1874486162425));
#294229=CARTESIAN_POINT('Ctrl Pts',(-2.65905758730007,15.2,-10.1911448195249));
#294230=CARTESIAN_POINT('Ctrl Pts',(-2.65928759429171,15.2,-10.1948410228073));
#294231=CARTESIAN_POINT('Ctrl Pts',(-2.65951017928423,15.2,-10.1985818334432));
#294232=CARTESIAN_POINT('Ctrl Pts',(-2.65972486820428,15.2,-10.2023666939089));
#294233=CARTESIAN_POINT('Ctrl Pts',(-2.65993955714384,15.2,-10.2061515547184));
#294234=CARTESIAN_POINT('Ctrl Pts',(-2.66014635065311,15.2,-10.2099804649914));
#294235=CARTESIAN_POINT('Ctrl Pts',(-2.66034479258003,15.2,-10.2138528737054));
#294236=CARTESIAN_POINT('Ctrl Pts',(-2.66054323448892,15.2,-10.2177252820677));
#294237=CARTESIAN_POINT('Ctrl Pts',(-2.66073332248927,15.2,-10.2216411908608));
#294238=CARTESIAN_POINT('Ctrl Pts',(-2.66091461048349,15.2,-10.2256000592351));
#294239=CARTESIAN_POINT('Ctrl Pts',(-2.66109589847771,15.2,-10.2295589276093));
#294240=CARTESIAN_POINT('Ctrl Pts',(-2.661268386155,15.2,-10.2335607571951));
#294241=CARTESIAN_POINT('Ctrl Pts',(-2.6614316372328,15.2,-10.2376050155464));
#294242=CARTESIAN_POINT('Ctrl Pts',(-2.66156767980258,15.2,-10.2409752309615));
#294243=CARTESIAN_POINT('Ctrl Pts',(-2.66169730820831,15.2,-10.2443749107774));
#294244=CARTESIAN_POINT('Ctrl Pts',(-2.66182027570866,15.2,-10.2478037545259));
#294245=CARTESIAN_POINT('Ctrl Pts',(-2.661943243209,15.2,-10.2512325982743));
#294246=CARTESIAN_POINT('Ctrl Pts',(-2.6620595504495,15.2,-10.2546906051323));
#294247=CARTESIAN_POINT('Ctrl Pts',(-2.66216895399168,15.2,-10.258177475773));
#294248=CARTESIAN_POINT('Ctrl Pts',(-2.66227835753386,15.2,-10.2616643464138));
#294249=CARTESIAN_POINT('Ctrl Pts',(-2.66238085976118,15.2,-10.2651800830166));
#294250=CARTESIAN_POINT('Ctrl Pts',(-2.66247622073341,15.2,-10.2687243894749));
#294251=CARTESIAN_POINT('Ctrl Pts',(-2.66257158170563,15.2,-10.2722686959333));
#294252=CARTESIAN_POINT('Ctrl Pts',(-2.66265980250532,15.2,-10.2758415734521));
#294253=CARTESIAN_POINT('Ctrl Pts',(-2.66274065174178,15.2,-10.2794427307602));
#294254=CARTESIAN_POINT('Ctrl Pts',(-2.66282150097824,15.2,-10.2830438880684));
#294255=CARTESIAN_POINT('Ctrl Pts',(-2.66289497861584,15.2,-10.2866733273045));
#294256=CARTESIAN_POINT('Ctrl Pts',(-2.662960854796,15.2,-10.2903307587643));
#294257=CARTESIAN_POINT('Ctrl Pts',(-2.66302673097616,15.2,-10.2939881902241));
#294258=CARTESIAN_POINT('Ctrl Pts',(-2.6630850084204,15.2,-10.2976736171804));
#294259=CARTESIAN_POINT('Ctrl Pts',(-2.66313546196166,15.2,-10.301386754543));
#294260=CARTESIAN_POINT('Ctrl Pts',(-2.66318591550292,15.2,-10.3050998919055));
#294261=CARTESIAN_POINT('Ctrl Pts',(-2.66322854556956,15.2,-10.3088407394751));
#294262=CARTESIAN_POINT('Ctrl Pts',(-2.66326313327906,15.2,-10.3126090202208));
#294263=CARTESIAN_POINT('Ctrl Pts',(-2.66329772098856,15.2,-10.3163773009665));
#294264=CARTESIAN_POINT('Ctrl Pts',(-2.66332426743092,15.2,-10.3201730127978));
#294265=CARTESIAN_POINT('Ctrl Pts',(-2.66334255527747,15.2,-10.3239958817583));
#294266=CARTESIAN_POINT('Ctrl Pts',(-2.66336084312401,15.2,-10.3278187507189));
#294267=CARTESIAN_POINT('Ctrl Pts',(-2.66337087492875,15.2,-10.3316687747715));
#294268=CARTESIAN_POINT('Ctrl Pts',(-2.66337243777528,15.2,-10.3355456837321));
#294269=CARTESIAN_POINT('Ctrl Pts',(-2.66337400062164,15.2,-10.33942259227));
#294270=CARTESIAN_POINT('Ctrl Pts',(-2.66336709709971,15.2,-10.3433263838442));
#294271=CARTESIAN_POINT('Ctrl Pts',(-2.66335151751878,15.2,-10.3472567914692));
#294272=CARTESIAN_POINT('Ctrl Pts',(-2.66333282201861,15.2,-10.3519732813903));
#294273=CARTESIAN_POINT('Ctrl Pts',(-2.66330163719225,15.2,-10.3567280939318));
#294274=CARTESIAN_POINT('Ctrl Pts',(-2.66325760877262,15.2,-10.361520775028));
#294275=CARTESIAN_POINT('Ctrl Pts',(-2.66322091842494,15.2,-10.3655146757238));
#294276=CARTESIAN_POINT('Ctrl Pts',(-2.66317531145247,15.2,-10.3695348726356));
#294277=CARTESIAN_POINT('Ctrl Pts',(-2.66312058922978,15.2,-10.3735811027064));
#294278=CARTESIAN_POINT('Ctrl Pts',(-2.66306586700708,15.2,-10.3776273327772));
#294279=CARTESIAN_POINT('Ctrl Pts',(-2.66300202853475,15.2,-10.381699597897));
#294280=CARTESIAN_POINT('Ctrl Pts',(-2.66292888047489,15.2,-10.3857976372008));
#294281=CARTESIAN_POINT('Ctrl Pts',(-2.66285573241503,15.2,-10.3898956765045));
#294282=CARTESIAN_POINT('Ctrl Pts',(-2.66277327411105,15.2,-10.3940194903017));
#294283=CARTESIAN_POINT('Ctrl Pts',(-2.66268131376305,15.2,-10.3981688235677));
#294284=CARTESIAN_POINT('Ctrl Pts',(-2.66260774549067,15.2,-10.4014882899091));
#294285=CARTESIAN_POINT('Ctrl Pts',(-2.66252809754961,15.2,-10.404824088165));
#294286=CARTESIAN_POINT('Ctrl Pts',(-2.66244227255704,15.2,-10.4081760885011));
#294287=CARTESIAN_POINT('Ctrl Pts',(-2.66235644755276,15.2,-10.4115280892938));
#294288=CARTESIAN_POINT('Ctrl Pts',(-2.6622644454466,15.2,-10.4148962919556));
#294289=CARTESIAN_POINT('Ctrl Pts',(-2.66216617176912,15.2,-10.4182805676994));
#294290=CARTESIAN_POINT('Ctrl Pts',(-2.66206789810503,15.2,-10.4216648429821));
#294291=CARTESIAN_POINT('Ctrl Pts',(-2.66196335286905,15.2,-10.4250651920484));
#294292=CARTESIAN_POINT('Ctrl Pts',(-2.66185244326742,15.2,-10.4284814877125));
#294293=CARTESIAN_POINT('Ctrl Pts',(-2.66174153365068,15.2,-10.4318977838421));
#294294=CARTESIAN_POINT('Ctrl Pts',(-2.66162425824429,15.2,-10.4353300249986));
#294295=CARTESIAN_POINT('Ctrl Pts',(-2.66150052718157,15.2,-10.4387780852986));
#294296=CARTESIAN_POINT('Ctrl Pts',(-2.6613458633616,15.2,-10.4430881604388));
#294297=CARTESIAN_POINT('Ctrl Pts',(-2.66118111038363,15.2,-10.4474229541032));
#294298=CARTESIAN_POINT('Ctrl Pts',(-2.66100609176306,15.2,-10.4517822209894));
#294299=CARTESIAN_POINT('Ctrl Pts',(-2.66086607687805,15.2,-10.4552696342132));
#294300=CARTESIAN_POINT('Ctrl Pts',(-2.66071949119958,15.2,-10.4587727095928));
#294301=CARTESIAN_POINT('Ctrl Pts',(-2.66056624754588,15.2,-10.4622913234708));
#294302=CARTESIAN_POINT('Ctrl Pts',(-2.66041300387129,15.2,-10.4658099378282));
#294303=CARTESIAN_POINT('Ctrl Pts',(-2.6602531008348,15.2,-10.4693440916791));
#294304=CARTESIAN_POINT('Ctrl Pts',(-2.66008645126973,15.2,-10.4728936605403));
#294305=CARTESIAN_POINT('Ctrl Pts',(-2.65991980172736,15.2,-10.4764432289178));
#294306=CARTESIAN_POINT('Ctrl Pts',(-2.65974640600598,15.2,-10.4800082136206));
#294307=CARTESIAN_POINT('Ctrl Pts',(-2.65956617706786,15.2,-10.4835884910055));
#294308=CARTESIAN_POINT('Ctrl Pts',(-2.65938594810519,15.2,-10.4871687688782));
#294309=CARTESIAN_POINT('Ctrl Pts',(-2.65919888488685,15.2,-10.4907643412586));
#294310=CARTESIAN_POINT('Ctrl Pts',(-2.65900490404249,15.2,-10.4943750850119));
#294311=CARTESIAN_POINT('Ctrl Pts',(-2.65881092322457,15.2,-10.4979858282733));
#294312=CARTESIAN_POINT('Ctrl Pts',(-2.65861002469136,15.2,-10.5016117448372));
#294313=CARTESIAN_POINT('Ctrl Pts',(-2.6584021225424,15.2,-10.5052527138713));
#294314=CARTESIAN_POINT('Ctrl Pts',(-2.65819422036513,15.2,-10.5088936834015));
#294315=CARTESIAN_POINT('Ctrl Pts',(-2.65797931725473,15.2,-10.5125497050079));
#294316=CARTESIAN_POINT('Ctrl Pts',(-2.6577573277416,15.2,-10.5162206600025));
#294317=CARTESIAN_POINT('Ctrl Pts',(-2.65753533825871,15.2,-10.5198916144969));
#294318=CARTESIAN_POINT('Ctrl Pts',(-2.65730626374366,15.2,-10.5235775024712));
#294319=CARTESIAN_POINT('Ctrl Pts',(-2.65707002226371,15.2,-10.5272782056116));
#294320=CARTESIAN_POINT('Ctrl Pts',(-2.65683378075156,15.2,-10.5309789092562));
#294321=CARTESIAN_POINT('Ctrl Pts',(-2.65659037236097,15.2,-10.5346944278967));
#294322=CARTESIAN_POINT('Ctrl Pts',(-2.65633971629175,15.2,-10.5384246447666));
#294323=CARTESIAN_POINT('Ctrl Pts',(-2.65608906022254,15.2,-10.5421548616366));
#294324=CARTESIAN_POINT('Ctrl Pts',(-2.65583115793581,15.2,-10.5458997760694));
#294325=CARTESIAN_POINT('Ctrl Pts',(-2.65556592719838,15.2,-10.5496592718313));
#294326=CARTESIAN_POINT('Ctrl Pts',(-2.65530069649709,15.2,-10.553418767081));
#294327=CARTESIAN_POINT('Ctrl Pts',(-2.65502813934808,15.2,-10.5571928445983));
#294328=CARTESIAN_POINT('Ctrl Pts',(-2.65474817775861,15.2,-10.5609813878057));
#294329=CARTESIAN_POINT('Ctrl Pts',(-2.65446821613099,15.2,-10.5647699315293));
#294330=CARTESIAN_POINT('Ctrl Pts',(-2.65418084869649,15.2,-10.5685729405813));
#294331=CARTESIAN_POINT('Ctrl Pts',(-2.65388599923521,15.2,-10.5723903021241));
#294332=CARTESIAN_POINT('Ctrl Pts',(-2.6535911498141,15.2,-10.5762076631468));
#294333=CARTESIAN_POINT('Ctrl Pts',(-2.65328881799674,15.2,-10.5800393753649));
#294334=CARTESIAN_POINT('Ctrl Pts',(-2.65297892730035,15.2,-10.5838853246607));
#294335=CARTESIAN_POINT('Ctrl Pts',(-2.65266903656173,15.2,-10.5877312744805));
#294336=CARTESIAN_POINT('Ctrl Pts',(-2.65235158764583,15.2,-10.5915914635646));
#294337=CARTESIAN_POINT('Ctrl Pts',(-2.65202650544454,15.2,-10.5954657768039));
#294338=CARTESIAN_POINT('Ctrl Pts',(-2.65170142328754,15.2,-10.5993400895153));
#294339=CARTESIAN_POINT('Ctrl Pts',(-2.65136870715507,15.2,-10.6032285265288));
#294340=CARTESIAN_POINT('Ctrl Pts',(-2.65102828429451,15.2,-10.6071309764311));
#294341=CARTESIAN_POINT('Ctrl Pts',(-2.6505176499341,15.2,-10.612984652082));
#294342=CARTESIAN_POINT('Ctrl Pts',(-2.64998967146322,15.2,-10.6188698572203));
#294343=CARTESIAN_POINT('Ctrl Pts',(-2.64944410718228,15.2,-10.6247862148782));
#294344=CARTESIAN_POINT('Ctrl Pts',(-2.64908039771122,15.2,-10.6287304527794));
#294345=CARTESIAN_POINT('Ctrl Pts',(-2.64870887096825,15.2,-10.6326885385512));
#294346=CARTESIAN_POINT('Ctrl Pts',(-2.64832945627534,15.2,-10.6366603585223));
#294347=CARTESIAN_POINT('Ctrl Pts',(-2.64795004153075,15.2,-10.6406321790345));
#294348=CARTESIAN_POINT('Ctrl Pts',(-2.64756273816892,15.2,-10.6446177358234));
#294349=CARTESIAN_POINT('Ctrl Pts',(-2.64716747670212,15.2,-10.6486169201538));
#294350=CARTESIAN_POINT('Ctrl Pts',(-2.64677221528918,15.2,-10.6526161039394));
#294351=CARTESIAN_POINT('Ctrl Pts',(-2.64636899514949,15.2,-10.6566289141982));
#294352=CARTESIAN_POINT('Ctrl Pts',(-2.64595774651696,15.2,-10.6606552421459));
#294353=CARTESIAN_POINT('Ctrl Pts',(-2.64534087348413,15.2,-10.6666947348904));
#294354=CARTESIAN_POINT('Ctrl Pts',(-2.64470593657406,15.2,-10.6727646445387));
#294355=CARTESIAN_POINT('Ctrl Pts',(-2.64405270545388,15.2,-10.6788646071232));
#294356=CARTESIAN_POINT('Ctrl Pts',(-2.64361721809977,15.2,-10.6829312482921));
#294357=CARTESIAN_POINT('Ctrl Pts',(-2.64317360006826,15.2,-10.6870112447855));
#294358=CARTESIAN_POINT('Ctrl Pts',(-2.64272178349206,15.2,-10.6911044932472));
#294359=CARTESIAN_POINT('Ctrl Pts',(-2.6422699668543,15.2,-10.6951977422666));
#294360=CARTESIAN_POINT('Ctrl Pts',(-2.64180995286655,15.2,-10.6993042405921));
#294361=CARTESIAN_POINT('Ctrl Pts',(-2.64134167417352,15.2,-10.7034238837069));
#294362=CARTESIAN_POINT('Ctrl Pts',(-2.64087339554429,15.2,-10.7075435262603));
#294363=CARTESIAN_POINT('Ctrl Pts',(-2.6403968519578,15.2,-10.7116763128815));
#294364=CARTESIAN_POINT('Ctrl Pts',(-2.63991197983132,15.2,-10.7158221381528));
#294365=CARTESIAN_POINT('Ctrl Pts',(-2.63942710763877,15.2,-10.719967963989));
#294366=CARTESIAN_POINT('Ctrl Pts',(-2.63893390337205,15.2,-10.7241268293463));
#294367=CARTESIAN_POINT('Ctrl Pts',(-2.63843230715226,15.2,-10.7282986293387));
#294368=CARTESIAN_POINT('Ctrl Pts',(-2.63780531191169,15.2,-10.7335133790451));
#294369=CARTESIAN_POINT('Ctrl Pts',(-2.63716519753237,15.2,-10.7387483387635));
#294370=CARTESIAN_POINT('Ctrl Pts',(-2.63651184565629,15.2,-10.7440033049456));
#294371=CARTESIAN_POINT('Ctrl Pts',(-2.63598916419815,15.2,-10.7482072775477));
#294372=CARTESIAN_POINT('Ctrl Pts',(-2.63545800868556,15.2,-10.7524240556342));
#294373=CARTESIAN_POINT('Ctrl Pts',(-2.63491831678579,15.2,-10.7566535349543));
#294374=CARTESIAN_POINT('Ctrl Pts',(-2.63437862481249,15.2,-10.7608830148507));
#294375=CARTESIAN_POINT('Ctrl Pts',(-2.63383039602538,15.2,-10.765125196083));
#294376=CARTESIAN_POINT('Ctrl Pts',(-2.63327356991091,15.2,-10.7693799774174));
#294377=CARTESIAN_POINT('Ctrl Pts',(-2.63271674387231,15.2,-10.7736347581721));
#294378=CARTESIAN_POINT('Ctrl Pts',(-2.63215131934944,15.2,-10.7779021378981));
#294379=CARTESIAN_POINT('Ctrl Pts',(-2.63157723606361,15.2,-10.7821820151585));
#294380=CARTESIAN_POINT('Ctrl Pts',(-2.63100315269955,15.2,-10.7864618930021));
#294381=CARTESIAN_POINT('Ctrl Pts',(-2.63042040866501,15.2,-10.7907542678638));
#294382=CARTESIAN_POINT('Ctrl Pts',(-2.62982894790999,15.2,-10.795059040377));
#294383=CARTESIAN_POINT('Ctrl Pts',(-2.6290896220065,15.2,-10.8004400057252));
#294384=CARTESIAN_POINT('Ctrl Pts',(-2.62833667154474,15.2,-10.8058403393071));
#294385=CARTESIAN_POINT('Ctrl Pts',(-2.62756998164437,15.2,-10.8112598481208));
#294386=CARTESIAN_POINT('Ctrl Pts',(-2.62695662977422,15.2,-10.8155954548174));
#294387=CARTESIAN_POINT('Ctrl Pts',(-2.62633448518554,15.2,-10.8199433313981));
#294388=CARTESIAN_POINT('Ctrl Pts',(-2.62570348929326,15.2,-10.824303380652));
#294389=CARTESIAN_POINT('Ctrl Pts',(-2.625072493315,15.2,-10.8286634305));
#294390=CARTESIAN_POINT('Ctrl Pts',(-2.6244326455218,15.2,-10.8330356512715));
#294391=CARTESIAN_POINT('Ctrl Pts',(-2.6237838889303,15.2,-10.8374199439002));
#294392=CARTESIAN_POINT('Ctrl Pts',(-2.62297294323513,15.2,-10.8429003093873));
#294393=CARTESIAN_POINT('Ctrl Pts',(-2.62214807878443,15.2,-10.8483995394136));
#294394=CARTESIAN_POINT('Ctrl Pts',(-2.62130918214433,15.2,-10.8539174401072));
#294395=CARTESIAN_POINT('Ctrl Pts',(-2.62080584417855,15.2,-10.8572281804031));
#294396=CARTESIAN_POINT('Ctrl Pts',(-2.62029745485916,15.2,-10.8605456423159));
#294397=CARTESIAN_POINT('Ctrl Pts',(-2.61978399141904,15.2,-10.8638697844041));
#294398=CARTESIAN_POINT('Ctrl Pts',(-2.61927052797892,15.2,-10.8671939264922));
#294399=CARTESIAN_POINT('Ctrl Pts',(-2.61875198988107,15.2,-10.8705247486546));
#294400=CARTESIAN_POINT('Ctrl Pts',(-2.61822835348343,15.2,-10.8738622102833));
#294401=CARTESIAN_POINT('Ctrl Pts',(-2.61753017155649,15.2,-10.8783121595258));
#294402=CARTESIAN_POINT('Ctrl Pts',(-2.61682292677571,15.2,-10.8827739122086));
#294403=CARTESIAN_POINT('Ctrl Pts',(-2.61610656412463,15.2,-10.8872473702314));
#294404=CARTESIAN_POINT('Ctrl Pts',(-2.61556929218512,15.2,-10.8906024634437));
#294405=CARTESIAN_POINT('Ctrl Pts',(-2.61502689136883,15.2,-10.893964142555));
#294406=CARTESIAN_POINT('Ctrl Pts',(-2.6144793389441,15.2,-10.8973323653934));
#294407=CARTESIAN_POINT('Ctrl Pts',(-2.61393178651938,15.2,-10.9007005882317));
#294408=CARTESIAN_POINT('Ctrl Pts',(-2.61337908276938,15.2,-10.9040753551909));
#294409=CARTESIAN_POINT('Ctrl Pts',(-2.61282120445586,15.2,-10.9074566253603));
#294410=CARTESIAN_POINT('Ctrl Pts',(-2.61226332614235,15.2,-10.9108378955297));
#294411=CARTESIAN_POINT('Ctrl Pts',(-2.61170027406278,15.2,-10.9142256696233));
#294412=CARTESIAN_POINT('Ctrl Pts',(-2.61113202520843,15.2,-10.91761990725));
#294413=CARTESIAN_POINT('Ctrl Pts',(-2.61037436000046,15.2,-10.92214555783));
#294414=CARTESIAN_POINT('Ctrl Pts',(-2.60960745680532,15.2,-10.9266826991946));
#294415=CARTESIAN_POINT('Ctrl Pts',(-2.60883126287318,15.2,-10.931231235777));
#294416=CARTESIAN_POINT('Ctrl Pts',(-2.60824911747695,15.2,-10.9346426379039));
#294417=CARTESIAN_POINT('Ctrl Pts',(-2.60766174576073,15.2,-10.9380604498485));
#294418=CARTESIAN_POINT('Ctrl Pts',(-2.60706912637705,15.2,-10.9414846321875));
#294419=CARTESIAN_POINT('Ctrl Pts',(-2.60647650699337,15.2,-10.9449088145266));
#294420=CARTESIAN_POINT('Ctrl Pts',(-2.60587863994614,15.2,-10.9483393671657));
#294421=CARTESIAN_POINT('Ctrl Pts',(-2.60527550313426,15.2,-10.9517762493747));
#294422=CARTESIAN_POINT('Ctrl Pts',(-2.60467236632238,15.2,-10.9552131315837));
#294423=CARTESIAN_POINT('Ctrl Pts',(-2.6040639611278,15.2,-10.9586563446086));
#294424=CARTESIAN_POINT('Ctrl Pts',(-2.60345026423343,15.2,-10.962105848275));
#294425=CARTESIAN_POINT('Ctrl Pts',(-2.60283656733906,15.2,-10.9655553519413));
#294426=CARTESIAN_POINT('Ctrl Pts',(-2.60221757902824,15.2,-10.9690111466824));
#294427=CARTESIAN_POINT('Ctrl Pts',(-2.60159327959305,15.2,-10.9724731923894));
#294428=CARTESIAN_POINT('Ctrl Pts',(-2.60096898015786,15.2,-10.9759352380964));
#294429=CARTESIAN_POINT('Ctrl Pts',(-2.60033936879759,15.2,-10.9794035354312));
#294430=CARTESIAN_POINT('Ctrl Pts',(-2.59970442391455,15.2,-10.9828780448111));
#294431=CARTESIAN_POINT('Ctrl Pts',(-2.59906947903152,15.2,-10.9863525541911));
#294432=CARTESIAN_POINT('Ctrl Pts',(-2.59842920081665,15.2,-10.9898332763007));
#294433=CARTESIAN_POINT('Ctrl Pts',(-2.5977835698825,15.2,-10.9933201710065));
#294434=CARTESIAN_POINT('Ctrl Pts',(-2.59713793883107,15.2,-10.9968070663458));
#294435=CARTESIAN_POINT('Ctrl Pts',(-2.59648695308646,15.2,-11.0003001351701));
#294436=CARTESIAN_POINT('Ctrl Pts',(-2.59583059311534,15.2,-11.0037993384711));
#294437=CARTESIAN_POINT('Ctrl Pts',(-2.5947366599891,15.2,-11.0096313431253));
#294438=CARTESIAN_POINT('Ctrl Pts',(-2.59362779792098,15.2,-11.0154803869159));
#294439=CARTESIAN_POINT('Ctrl Pts',(-2.59250391458642,15.2,-11.0213462915006));
#294440=CARTESIAN_POINT('Ctrl Pts',(-2.59182958461018,15.2,-11.0248658341235));
#294441=CARTESIAN_POINT('Ctrl Pts',(-2.59114984508423,15.2,-11.0283914459795));
#294442=CARTESIAN_POINT('Ctrl Pts',(-2.59046467819199,15.2,-11.0319230896434));
#294443=CARTESIAN_POINT('Ctrl Pts',(-2.58977951129974,15.2,-11.0354547333072));
#294444=CARTESIAN_POINT('Ctrl Pts',(-2.58908891607736,15.2,-11.0389924089991));
#294445=CARTESIAN_POINT('Ctrl Pts',(-2.58839287322446,15.2,-11.0425360767615));
#294446=CARTESIAN_POINT('Ctrl Pts',(-2.58769683037156,15.2,-11.0460797445239));
#294447=CARTESIAN_POINT('Ctrl Pts',(-2.58699533956157,15.2,-11.0496294065098));
#294448=CARTESIAN_POINT('Ctrl Pts',(-2.58628838075073,15.2,-11.0531850222717));
#294449=CARTESIAN_POINT('Ctrl Pts',(-2.5851101160232,15.2,-11.059111048757));
#294450=CARTESIAN_POINT('Ctrl Pts',(-2.58391666405009,15.2,-11.0650536168));
#294451=CARTESIAN_POINT('Ctrl Pts',(-2.58270793425843,15.2,-11.07101255055));
#294452=CARTESIAN_POINT('Ctrl Pts',(-2.5817409503724,15.2,-11.0757796978098));
#294453=CARTESIAN_POINT('Ctrl Pts',(-2.58076418796855,15.2,-11.0805573183069));
#294454=CARTESIAN_POINT('Ctrl Pts',(-2.57977760408045,15.2,-11.0853453242911));
#294455=CARTESIAN_POINT('Ctrl Pts',(-2.57903766623159,15.2,-11.0889363284531));
#294456=CARTESIAN_POINT('Ctrl Pts',(-2.57829220346561,15.2,-11.0925331736306));
#294457=CARTESIAN_POINT('Ctrl Pts',(-2.5775411956214,15.2,-11.0961358233887));
#294458=CARTESIAN_POINT('Ctrl Pts',(-2.5767901877772,15.2,-11.0997384731468));
#294459=CARTESIAN_POINT('Ctrl Pts',(-2.57603363493972,15.2,-11.1033469255248));
#294460=CARTESIAN_POINT('Ctrl Pts',(-2.5752715201336,15.2,-11.1069611441857));
#294461=CARTESIAN_POINT('Ctrl Pts',(-2.57450940532747,15.2,-11.1105753628465));
#294462=CARTESIAN_POINT('Ctrl Pts',(-2.57374172875534,15.2,-11.1141953480984));
#294463=CARTESIAN_POINT('Ctrl Pts',(-2.57296846953343,15.2,-11.1178210627583));
#294464=CARTESIAN_POINT('Ctrl Pts',(-2.57219521031153,15.2,-11.1214467774182));
#294465=CARTESIAN_POINT('Ctrl Pts',(-2.57141637063985,15.2,-11.1250782207029));
#294466=CARTESIAN_POINT('Ctrl Pts',(-2.5706319318355,15.2,-11.128715357362));
#294467=CARTESIAN_POINT('Ctrl Pts',(-2.56984749303116,15.2,-11.132352494021));
#294468=CARTESIAN_POINT('Ctrl Pts',(-2.56905745493083,15.2,-11.1359953233451));
#294469=CARTESIAN_POINT('Ctrl Pts',(-2.56826179767065,15.2,-11.1396438057691));
#294470=CARTESIAN_POINT('Ctrl Pts',(-2.56720092122736,15.2,-11.1445084494431));
#294471=CARTESIAN_POINT('Ctrl Pts',(-2.56613005766842,15.2,-11.1493831445103));
#294472=CARTESIAN_POINT('Ctrl Pts',(-2.56504916388664,15.2,-11.1542678046661));
#294473=CARTESIAN_POINT('Ctrl Pts',(-2.56423849362394,15.2,-11.1579312994501));
#294474=CARTESIAN_POINT('Ctrl Pts',(-2.5634221825869,15.2,-11.1616004010835));
#294475=CARTESIAN_POINT('Ctrl Pts',(-2.56260021378343,15.2,-11.1652750757416));
#294476=CARTESIAN_POINT('Ctrl Pts',(-2.56177824497996,15.2,-11.1689497503998));
#294477=CARTESIAN_POINT('Ctrl Pts',(-2.56095061872672,15.2,-11.172629997866));
#294478=CARTESIAN_POINT('Ctrl Pts',(-2.56011731584083,15.2,-11.1763157773567));
#294479=CARTESIAN_POINT('Ctrl Pts',(-2.55928401295493,15.2,-11.1800015568473));
#294480=CARTESIAN_POINT('Ctrl Pts',(-2.55844503222431,15.2,-11.183692866235));
#294481=CARTESIAN_POINT('Ctrl Pts',(-2.5576003524218,15.2,-11.1873896640348));
#294482=CARTESIAN_POINT('Ctrl Pts',(-2.55675567261928,15.2,-11.1910864618345));
#294483=CARTESIAN_POINT('Ctrl Pts',(-2.5559052937715,15.2,-11.1947887445105));
#294484=CARTESIAN_POINT('Ctrl Pts',(-2.55504920467839,15.2,-11.1984964891667));
#294485=CARTESIAN_POINT('Ctrl Pts',(-2.55390775245054,15.2,-11.2034401491574));
#294486=CARTESIAN_POINT('Ctrl Pts',(-2.55275615131663,15.2,-11.2083935173142));
#294487=CARTESIAN_POINT('Ctrl Pts',(-2.55159439100006,15.2,-11.213356592));
#294488=CARTESIAN_POINT('Ctrl Pts',(-2.64164356400005,12.2,-10.033062558));
#294489=CARTESIAN_POINT('Ctrl Pts',(-2.64194832280646,12.2,-10.0348230291495));
#294490=CARTESIAN_POINT('Ctrl Pts',(-2.64225752123829,12.2,-10.0366407490542));
#294491=CARTESIAN_POINT('Ctrl Pts',(-2.64257038372412,12.2,-10.0385148613197));
#294492=CARTESIAN_POINT('Ctrl Pts',(-2.642884754991,12.2,-10.0403980115018));
#294493=CARTESIAN_POINT('Ctrl Pts',(-2.64320281628075,12.2,-10.0423381055564));
#294494=CARTESIAN_POINT('Ctrl Pts',(-2.64352378181444,12.2,-10.0443343061848));
#294495=CARTESIAN_POINT('Ctrl Pts',(-2.64384474731898,12.2,-10.046330506632));
#294496=CARTESIAN_POINT('Ctrl Pts',(-2.64416861707023,12.2,-10.0483828179432));
#294497=CARTESIAN_POINT('Ctrl Pts',(-2.64449462947505,12.2,-10.0504904280332));
#294498=CARTESIAN_POINT('Ctrl Pts',(-2.64482064187987,12.2,-10.0525980381233));
#294499=CARTESIAN_POINT('Ctrl Pts',(-2.64514879650543,12.2,-10.0547609446918));
#294500=CARTESIAN_POINT('Ctrl Pts',(-2.64547835425984,12.2,-10.0569783620522));
#294501=CARTESIAN_POINT('Ctrl Pts',(-2.64580791204419,12.2,-10.059195779614));
#294502=CARTESIAN_POINT('Ctrl Pts',(-2.64613887655142,12.2,-10.061467706473));
#294503=CARTESIAN_POINT('Ctrl Pts',(-2.64647052756954,12.2,-10.0637933712701));
#294504=CARTESIAN_POINT('Ctrl Pts',(-2.64680217855753,12.2,-10.0661190358559));
#294505=CARTESIAN_POINT('Ctrl Pts',(-2.64713452030244,12.2,-10.0684984401782));
#294506=CARTESIAN_POINT('Ctrl Pts',(-2.64746685620854,12.2,-10.0709308317677));
#294507=CARTESIAN_POINT('Ctrl Pts',(-2.64779919211464,12.2,-10.0733632233572));
#294508=CARTESIAN_POINT('Ctrl Pts',(-2.64813152490233,12.2,-10.0758486046313));
#294509=CARTESIAN_POINT('Ctrl Pts',(-2.64846317797365,12.2,-10.0783862401202));
#294510=CARTESIAN_POINT('Ctrl Pts',(-2.64879483107508,12.2,-10.0809238758395));
#294511=CARTESIAN_POINT('Ctrl Pts',(-2.64912580739311,12.2,-10.0835137670404));
#294512=CARTESIAN_POINT('Ctrl Pts',(-2.64945545332766,12.2,-10.0861551970212));
#294513=CARTESIAN_POINT('Ctrl Pts',(-2.64978509923225,12.2,-10.088796626762));
#294514=CARTESIAN_POINT('Ctrl Pts',(-2.65011341197145,12.2,-10.0914895979888));
#294515=CARTESIAN_POINT('Ctrl Pts',(-2.65043976104284,12.2,-10.0942334086413));
#294516=CARTESIAN_POINT('Ctrl Pts',(-2.65076611011422,12.2,-10.0969772192938));
#294517=CARTESIAN_POINT('Ctrl Pts',(-2.65109049354409,12.2,-10.099771869884));
#294518=CARTESIAN_POINT('Ctrl Pts',(-2.65141229569918,12.2,-10.1026166776118));
#294519=CARTESIAN_POINT('Ctrl Pts',(-2.65173409785426,12.2,-10.1054614853395));
#294520=CARTESIAN_POINT('Ctrl Pts',(-2.65205331640188,12.2,-10.108356448881));
#294521=CARTESIAN_POINT('Ctrl Pts',(-2.65236935747395,12.2,-10.1113009016873));
#294522=CARTESIAN_POINT('Ctrl Pts',(-2.65268539857472,12.2,-10.1142453547611));
#294523=CARTESIAN_POINT('Ctrl Pts',(-2.65299825684187,12.2,-10.117239296673));
#294524=CARTESIAN_POINT('Ctrl Pts',(-2.65330735327523,12.2,-10.1202820709243));
#294525=CARTESIAN_POINT('Ctrl Pts',(-2.6536164496805,12.2,-10.1233248448992));
#294526=CARTESIAN_POINT('Ctrl Pts',(-2.65392178424282,12.2,-10.1264164543318));
#294527=CARTESIAN_POINT('Ctrl Pts',(-2.65422278873326,12.2,-10.1295562562319));
#294528=CARTESIAN_POINT('Ctrl Pts',(-2.6545237932237,12.2,-10.1326960581319));
#294529=CARTESIAN_POINT('Ctrl Pts',(-2.6548204693202,12.2,-10.1358840535347));
#294530=CARTESIAN_POINT('Ctrl Pts',(-2.65511226572659,12.2,-10.1391196154139));
#294531=CARTESIAN_POINT('Ctrl Pts',(-2.65540406215949,12.2,-10.142355177587));
#294532=CARTESIAN_POINT('Ctrl Pts',(-2.65569097776695,12.2,-10.1456383044564));
#294533=CARTESIAN_POINT('Ctrl Pts',(-2.65597247828205,12.2,-10.14896838289));
#294534=CARTESIAN_POINT('Ctrl Pts',(-2.65625397877158,12.2,-10.152298461021));
#294535=CARTESIAN_POINT('Ctrl Pts',(-2.65653006180852,12.2,-10.1556754927156));
#294536=CARTESIAN_POINT('Ctrl Pts',(-2.65680020829994,12.2,-10.1590988700234));
#294537=CARTESIAN_POINT('Ctrl Pts',(-2.65707035479137,12.2,-10.1625222473311));
#294538=CARTESIAN_POINT('Ctrl Pts',(-2.65733456181423,12.2,-10.1659919742893));
#294539=CARTESIAN_POINT('Ctrl Pts',(-2.65759232347197,12.2,-10.1695074575751));
#294540=CARTESIAN_POINT('Ctrl Pts',(-2.65785008515312,12.2,-10.1730229411802));
#294541=CARTESIAN_POINT('Ctrl Pts',(-2.65810140084023,12.2,-10.1765841834696));
#294542=CARTESIAN_POINT('Ctrl Pts',(-2.65834577378202,12.2,-10.1801906021823));
#294543=CARTESIAN_POINT('Ctrl Pts',(-2.65859014670162,12.2,-10.1837970205673));
#294544=CARTESIAN_POINT('Ctrl Pts',(-2.65882758030843,12.2,-10.1874486162425));
#294545=CARTESIAN_POINT('Ctrl Pts',(-2.65905758730007,12.2,-10.1911448195249));
#294546=CARTESIAN_POINT('Ctrl Pts',(-2.65928759429171,12.2,-10.1948410228073));
#294547=CARTESIAN_POINT('Ctrl Pts',(-2.65951017928423,12.2,-10.1985818334432));
#294548=CARTESIAN_POINT('Ctrl Pts',(-2.65972486820428,12.2,-10.2023666939089));
#294549=CARTESIAN_POINT('Ctrl Pts',(-2.65993955714384,12.2,-10.2061515547184));
#294550=CARTESIAN_POINT('Ctrl Pts',(-2.66014635065312,12.2,-10.2099804649914));
#294551=CARTESIAN_POINT('Ctrl Pts',(-2.66034479258003,12.2,-10.2138528737054));
#294552=CARTESIAN_POINT('Ctrl Pts',(-2.66054323448892,12.2,-10.2177252820677));
#294553=CARTESIAN_POINT('Ctrl Pts',(-2.66073332248927,12.2,-10.2216411908608));
#294554=CARTESIAN_POINT('Ctrl Pts',(-2.66091461048349,12.2,-10.2256000592351));
#294555=CARTESIAN_POINT('Ctrl Pts',(-2.66109589847771,12.2,-10.2295589276093));
#294556=CARTESIAN_POINT('Ctrl Pts',(-2.661268386155,12.2,-10.2335607571951));
#294557=CARTESIAN_POINT('Ctrl Pts',(-2.6614316372328,12.2,-10.2376050155464));
#294558=CARTESIAN_POINT('Ctrl Pts',(-2.66156767980258,12.2,-10.2409752309615));
#294559=CARTESIAN_POINT('Ctrl Pts',(-2.66169730820831,12.2,-10.2443749107774));
#294560=CARTESIAN_POINT('Ctrl Pts',(-2.66182027570866,12.2,-10.2478037545259));
#294561=CARTESIAN_POINT('Ctrl Pts',(-2.661943243209,12.2,-10.2512325982743));
#294562=CARTESIAN_POINT('Ctrl Pts',(-2.6620595504495,12.2,-10.2546906051323));
#294563=CARTESIAN_POINT('Ctrl Pts',(-2.66216895399168,12.2,-10.258177475773));
#294564=CARTESIAN_POINT('Ctrl Pts',(-2.66227835753386,12.2,-10.2616643464138));
#294565=CARTESIAN_POINT('Ctrl Pts',(-2.66238085976118,12.2,-10.2651800830166));
#294566=CARTESIAN_POINT('Ctrl Pts',(-2.66247622073341,12.2,-10.2687243894749));
#294567=CARTESIAN_POINT('Ctrl Pts',(-2.66257158170563,12.2,-10.2722686959333));
#294568=CARTESIAN_POINT('Ctrl Pts',(-2.66265980250532,12.2,-10.2758415734521));
#294569=CARTESIAN_POINT('Ctrl Pts',(-2.66274065174178,12.2,-10.2794427307602));
#294570=CARTESIAN_POINT('Ctrl Pts',(-2.66282150097824,12.2,-10.2830438880684));
#294571=CARTESIAN_POINT('Ctrl Pts',(-2.66289497861584,12.2,-10.2866733273045));
#294572=CARTESIAN_POINT('Ctrl Pts',(-2.662960854796,12.2,-10.2903307587643));
#294573=CARTESIAN_POINT('Ctrl Pts',(-2.66302673097616,12.2,-10.2939881902241));
#294574=CARTESIAN_POINT('Ctrl Pts',(-2.6630850084204,12.2,-10.2976736171804));
#294575=CARTESIAN_POINT('Ctrl Pts',(-2.66313546196166,12.2,-10.301386754543));
#294576=CARTESIAN_POINT('Ctrl Pts',(-2.66318591550292,12.2,-10.3050998919055));
#294577=CARTESIAN_POINT('Ctrl Pts',(-2.66322854556956,12.2,-10.3088407394751));
#294578=CARTESIAN_POINT('Ctrl Pts',(-2.66326313327906,12.2,-10.3126090202208));
#294579=CARTESIAN_POINT('Ctrl Pts',(-2.66329772098856,12.2,-10.3163773009665));
#294580=CARTESIAN_POINT('Ctrl Pts',(-2.66332426743092,12.2,-10.3201730127977));
#294581=CARTESIAN_POINT('Ctrl Pts',(-2.66334255527747,12.2,-10.3239958817583));
#294582=CARTESIAN_POINT('Ctrl Pts',(-2.66336084312401,12.2,-10.3278187507189));
#294583=CARTESIAN_POINT('Ctrl Pts',(-2.66337087492875,12.2,-10.3316687747715));
#294584=CARTESIAN_POINT('Ctrl Pts',(-2.66337243777528,12.2,-10.3355456837321));
#294585=CARTESIAN_POINT('Ctrl Pts',(-2.66337400062164,12.2,-10.33942259227));
#294586=CARTESIAN_POINT('Ctrl Pts',(-2.66336709709971,12.2,-10.3433263838442));
#294587=CARTESIAN_POINT('Ctrl Pts',(-2.66335151751878,12.2,-10.3472567914692));
#294588=CARTESIAN_POINT('Ctrl Pts',(-2.66333282201861,12.2,-10.3519732813903));
#294589=CARTESIAN_POINT('Ctrl Pts',(-2.66330163719225,12.2,-10.3567280939318));
#294590=CARTESIAN_POINT('Ctrl Pts',(-2.66325760877262,12.2,-10.361520775028));
#294591=CARTESIAN_POINT('Ctrl Pts',(-2.66322091842494,12.2,-10.3655146757238));
#294592=CARTESIAN_POINT('Ctrl Pts',(-2.66317531145247,12.2,-10.3695348726356));
#294593=CARTESIAN_POINT('Ctrl Pts',(-2.66312058922978,12.2,-10.3735811027064));
#294594=CARTESIAN_POINT('Ctrl Pts',(-2.66306586700708,12.2,-10.3776273327772));
#294595=CARTESIAN_POINT('Ctrl Pts',(-2.66300202853475,12.2,-10.381699597897));
#294596=CARTESIAN_POINT('Ctrl Pts',(-2.66292888047489,12.2,-10.3857976372008));
#294597=CARTESIAN_POINT('Ctrl Pts',(-2.66285573241503,12.2,-10.3898956765045));
#294598=CARTESIAN_POINT('Ctrl Pts',(-2.66277327411105,12.2,-10.3940194903017));
#294599=CARTESIAN_POINT('Ctrl Pts',(-2.66268131376305,12.2,-10.3981688235677));
#294600=CARTESIAN_POINT('Ctrl Pts',(-2.66260774549067,12.2,-10.4014882899091));
#294601=CARTESIAN_POINT('Ctrl Pts',(-2.66252809754961,12.2,-10.404824088165));
#294602=CARTESIAN_POINT('Ctrl Pts',(-2.66244227255704,12.2,-10.4081760885011));
#294603=CARTESIAN_POINT('Ctrl Pts',(-2.66233499130754,12.2,-10.4123660892637));
#294604=CARTESIAN_POINT('Ctrl Pts',(-2.66221805842847,12.2,-10.4165814049896));
#294605=CARTESIAN_POINT('Ctrl Pts',(-2.66209128898348,12.2,-10.4208217857726));
#294606=CARTESIAN_POINT('Ctrl Pts',(-2.66198987342196,12.2,-10.424214090584));
#294607=CARTESIAN_POINT('Ctrl Pts',(-2.66188216388829,12.2,-10.4276224374716));
#294608=CARTESIAN_POINT('Ctrl Pts',(-2.66176806621476,12.2,-10.4310466983265));
#294609=CARTESIAN_POINT('Ctrl Pts',(-2.6616254441306,12.2,-10.4353270241618));
#294610=CARTESIAN_POINT('Ctrl Pts',(-2.66147284076851,12.2,-10.439632214531));
#294611=CARTESIAN_POINT('Ctrl Pts',(-2.66131007646212,12.2,-10.4439620253663));
#294612=CARTESIAN_POINT('Ctrl Pts',(-2.66117986502765,12.2,-10.4474258737514));
#294613=CARTESIAN_POINT('Ctrl Pts',(-2.66104315280853,12.2,-10.4509054788203));
#294614=CARTESIAN_POINT('Ctrl Pts',(-2.66089984720851,12.2,-10.4544007152726));
#294615=CARTESIAN_POINT('Ctrl Pts',(-2.66075654158896,12.2,-10.4578959522011));
#294616=CARTESIAN_POINT('Ctrl Pts',(-2.66060664360592,12.2,-10.46140681998));
#294617=CARTESIAN_POINT('Ctrl Pts',(-2.66045006470781,12.2,-10.4649331967849));
#294618=CARTESIAN_POINT('Ctrl Pts',(-2.66029348583104,12.2,-10.4684595731093));
#294619=CARTESIAN_POINT('Ctrl Pts',(-2.66013022593846,12.2,-10.47200145649));
#294620=CARTESIAN_POINT('Ctrl Pts',(-2.65996019773058,12.2,-10.475558724976));
#294621=CARTESIAN_POINT('Ctrl Pts',(-2.65979016949954,12.2,-10.4791159939466));
#294622=CARTESIAN_POINT('Ctrl Pts',(-2.65961337396817,12.2,-10.4826886485362));
#294623=CARTESIAN_POINT('Ctrl Pts',(-2.6594297224484,12.2,-10.4862765657457));
#294624=CARTESIAN_POINT('Ctrl Pts',(-2.65924607095364,12.2,-10.4898644824663));
#294625=CARTESIAN_POINT('Ctrl Pts',(-2.65905556482179,12.2,-10.493467662465));
#294626=CARTESIAN_POINT('Ctrl Pts',(-2.65885811994949,12.2,-10.497085985446));
#294627=CARTESIAN_POINT('Ctrl Pts',(-2.6586606750503,12.2,-10.5007043089199));
#294628=CARTESIAN_POINT('Ctrl Pts',(-2.65845628990305,12.2,-10.5043377740846));
#294629=CARTESIAN_POINT('Ctrl Pts',(-2.6582448817244,12.2,-10.50798626234));
#294630=CARTESIAN_POINT('Ctrl Pts',(-2.6579806215155,12.2,-10.5125468724107));
#294631=CARTESIAN_POINT('Ctrl Pts',(-2.65770538780966,12.2,-10.517130954392));
#294632=CARTESIAN_POINT('Ctrl Pts',(-2.65741901918347,12.2,-10.5217382780265));
#294633=CARTESIAN_POINT('Ctrl Pts',(-2.65718992430124,12.2,-10.5254241366329));
#294634=CARTESIAN_POINT('Ctrl Pts',(-2.65695370326065,12.2,-10.5291248693788));
#294635=CARTESIAN_POINT('Ctrl Pts',(-2.65671027450325,12.2,-10.532840357963));
#294636=CARTESIAN_POINT('Ctrl Pts',(-2.65646684571267,12.2,-10.5365558470534));
#294637=CARTESIAN_POINT('Ctrl Pts',(-2.65621620986013,12.2,-10.540286092654));
#294638=CARTESIAN_POINT('Ctrl Pts',(-2.65595828751226,12.2,-10.5440309782479));
#294639=CARTESIAN_POINT('Ctrl Pts',(-2.65570036519954,12.2,-10.5477758633316));
#294640=CARTESIAN_POINT('Ctrl Pts',(-2.65543515385807,12.2,-10.5515353878681));
#294641=CARTESIAN_POINT('Ctrl Pts',(-2.6551625770896,12.2,-10.5553094359691));
#294642=CARTESIAN_POINT('Ctrl Pts',(-2.65489000028398,12.2,-10.5590834845843));
#294643=CARTESIAN_POINT('Ctrl Pts',(-2.65461005795656,12.2,-10.5628720576417));
#294644=CARTESIAN_POINT('Ctrl Pts',(-2.65432267121819,12.2,-10.5666750386277));
#294645=CARTESIAN_POINT('Ctrl Pts',(-2.65403528451897,12.2,-10.5704780190955));
#294646=CARTESIAN_POINT('Ctrl Pts',(-2.65374045463237,12.2,-10.5742954080271));
#294647=CARTESIAN_POINT('Ctrl Pts',(-2.65343810382452,12.2,-10.5781270918235));
#294648=CARTESIAN_POINT('Ctrl Pts',(-2.65313575297547,12.2,-10.581958776142));
#294649=CARTESIAN_POINT('Ctrl Pts',(-2.65282588106031,12.2,-10.5858047541635));
#294650=CARTESIAN_POINT('Ctrl Pts',(-2.65250841354154,12.2,-10.5896649145026));
#294651=CARTESIAN_POINT('Ctrl Pts',(-2.65219094606602,12.2,-10.5935250743157));
#294652=CARTESIAN_POINT('Ctrl Pts',(-2.65186588245983,12.2,-10.5973994151752));
#294653=CARTESIAN_POINT('Ctrl Pts',(-2.65153314782115,12.2,-10.6012878243559));
#294654=CARTESIAN_POINT('Ctrl Pts',(-2.6511172294888,12.2,-10.6061483362291));
#294655=CARTESIAN_POINT('Ctrl Pts',(-2.65068932673998,12.2,-10.6110308312825));
#294656=CARTESIAN_POINT('Ctrl Pts',(-2.65024929486597,12.2,-10.6159350898918));
#294657=CARTESIAN_POINT('Ctrl Pts',(-2.64989726934758,12.2,-10.6198584969931));
#294658=CARTESIAN_POINT('Ctrl Pts',(-2.64953748101879,12.2,-10.6237958324443));
#294659=CARTESIAN_POINT('Ctrl Pts',(-2.64916985827483,12.2,-10.627746987511));
#294660=CARTESIAN_POINT('Ctrl Pts',(-2.64880223558097,12.2,-10.6316981420393));
#294661=CARTESIAN_POINT('Ctrl Pts',(-2.64842677839451,12.2,-10.6356631155872));
#294662=CARTESIAN_POINT('Ctrl Pts',(-2.64804341503776,12.2,-10.6396417968161));
#294663=CARTESIAN_POINT('Ctrl Pts',(-2.64766005162879,12.2,-10.6436204785871));
#294664=CARTESIAN_POINT('Ctrl Pts',(-2.64726878260518,12.2,-10.6476128702788));
#294665=CARTESIAN_POINT('Ctrl Pts',(-2.64686953725009,12.2,-10.6516188607749));
#294666=CARTESIAN_POINT('Ctrl Pts',(-2.646470291895,12.2,-10.6556248512711));
#294667=CARTESIAN_POINT('Ctrl Pts',(-2.64606307048342,12.2,-10.659644441316));
#294668=CARTESIAN_POINT('Ctrl Pts',(-2.64564780368219,12.2,-10.663677522426));
#294669=CARTESIAN_POINT('Ctrl Pts',(-2.64523253693753,12.2,-10.6677106029866));
#294670=CARTESIAN_POINT('Ctrl Pts',(-2.64480922359393,12.2,-10.6717571753121));
#294671=CARTESIAN_POINT('Ctrl Pts',(-2.64437779751861,12.2,-10.6758171312015));
#294672=CARTESIAN_POINT('Ctrl Pts',(-2.64394637138452,12.2,-10.6798770876441));
#294673=CARTESIAN_POINT('Ctrl Pts',(-2.64350683114644,12.2,-10.6839504269261));
#294674=CARTESIAN_POINT('Ctrl Pts',(-2.64305910971007,12.2,-10.6880370435764));
#294675=CARTESIAN_POINT('Ctrl Pts',(-2.64261138833471,12.2,-10.6921236596698));
#294676=CARTESIAN_POINT('Ctrl Pts',(-2.64215548541614,12.2,-10.6962235528093));
#294677=CARTESIAN_POINT('Ctrl Pts',(-2.64169133478795,12.2,-10.7003366166388));
#294678=CARTESIAN_POINT('Ctrl Pts',(-2.64111114645529,12.2,-10.7054779468461));
#294679=CARTESIAN_POINT('Ctrl Pts',(-2.64051807003897,12.2,-10.71063985614));
#294680=CARTESIAN_POINT('Ctrl Pts',(-2.63991197983132,12.2,-10.7158221381528));
#294681=CARTESIAN_POINT('Ctrl Pts',(-2.63942710763877,12.2,-10.719967963989));
#294682=CARTESIAN_POINT('Ctrl Pts',(-2.63893390337205,12.2,-10.7241268293463));
#294683=CARTESIAN_POINT('Ctrl Pts',(-2.63843230715226,12.2,-10.7282986293387));
#294684=CARTESIAN_POINT('Ctrl Pts',(-2.63793071100081,12.2,-10.7324704287628));
#294685=CARTESIAN_POINT('Ctrl Pts',(-2.63742071929113,12.2,-10.7366551619259));
#294686=CARTESIAN_POINT('Ctrl Pts',(-2.63690226950073,12.2,-10.7408527264153));
#294687=CARTESIAN_POINT('Ctrl Pts',(-2.63638381963969,12.2,-10.7450502914765));
#294688=CARTESIAN_POINT('Ctrl Pts',(-2.63585691339987,12.2,-10.7492606849671));
#294689=CARTESIAN_POINT('Ctrl Pts',(-2.63532148598124,12.2,-10.753483808587));
#294690=CARTESIAN_POINT('Ctrl Pts',(-2.63478605863556,12.2,-10.7577069316315));
#294691=CARTESIAN_POINT('Ctrl Pts',(-2.63424210983135,12.2,-10.7619427795808));
#294692=CARTESIAN_POINT('Ctrl Pts',(-2.63368957857189,12.2,-10.7661912543336));
#294693=CARTESIAN_POINT('Ctrl Pts',(-2.63299891444108,12.2,-10.7715018482086));
#294694=CARTESIAN_POINT('Ctrl Pts',(-2.63229484022956,12.2,-10.7768321681457));
#294695=CARTESIAN_POINT('Ctrl Pts',(-2.63157723606361,12.2,-10.7821820151585));
#294696=CARTESIAN_POINT('Ctrl Pts',(-2.63085963189765,12.2,-10.7875318621714));
#294697=CARTESIAN_POINT('Ctrl Pts',(-2.63012849690911,12.2,-10.7929012362764));
#294698=CARTESIAN_POINT('Ctrl Pts',(-2.62938371684038,12.2,-10.7982899416227));
#294699=CARTESIAN_POINT('Ctrl Pts',(-2.62878789275292,12.2,-10.8026009061346));
#294700=CARTESIAN_POINT('Ctrl Pts',(-2.62818333359809,12.2,-10.8069242408335));
#294701=CARTESIAN_POINT('Ctrl Pts',(-2.62756998164437,12.2,-10.8112598481208));
#294702=CARTESIAN_POINT('Ctrl Pts',(-2.62695662977422,12.2,-10.8155954548174));
#294703=CARTESIAN_POINT('Ctrl Pts',(-2.62633448518554,12.2,-10.8199433313981));
#294704=CARTESIAN_POINT('Ctrl Pts',(-2.62570348929326,12.2,-10.824303380652));
#294705=CARTESIAN_POINT('Ctrl Pts',(-2.62491474436342,12.2,-10.8297534426649));
#294706=CARTESIAN_POINT('Ctrl Pts',(-2.62411216799157,12.2,-10.8352225209033));
#294707=CARTESIAN_POINT('Ctrl Pts',(-2.62329565056174,12.2,-10.8407104245828));
#294708=CARTESIAN_POINT('Ctrl Pts',(-2.62280574012164,12.2,-10.8440031666709));
#294709=CARTESIAN_POINT('Ctrl Pts',(-2.62231081096967,12.2,-10.8473026858994));
#294710=CARTESIAN_POINT('Ctrl Pts',(-2.62181083758844,12.2,-10.850608940652));
#294711=CARTESIAN_POINT('Ctrl Pts',(-2.62131086420721,12.2,-10.8539151954046));
#294712=CARTESIAN_POINT('Ctrl Pts',(-2.6208058479754,12.2,-10.8572281851478));
#294713=CARTESIAN_POINT('Ctrl Pts',(-2.62029576461962,12.2,-10.8605478692346));
#294714=CARTESIAN_POINT('Ctrl Pts',(-2.61978568117117,12.2,-10.8638675539245));
#294715=CARTESIAN_POINT('Ctrl Pts',(-2.61927053184631,12.2,-10.867193932058));
#294716=CARTESIAN_POINT('Ctrl Pts',(-2.61875029139501,12.2,-10.8705269637099));
#294717=CARTESIAN_POINT('Ctrl Pts',(-2.61823005103822,12.2,-10.8738599947564));
#294718=CARTESIAN_POINT('Ctrl Pts',(-2.61770472059003,12.2,-10.8771996783192));
#294719=CARTESIAN_POINT('Ctrl Pts',(-2.61717427669219,12.2,-10.8805459743648));
#294720=CARTESIAN_POINT('Ctrl Pts',(-2.61664383279435,12.2,-10.8838922704105));
#294721=CARTESIAN_POINT('Ctrl Pts',(-2.61610827563243,12.2,-10.8872451773764));
#294722=CARTESIAN_POINT('Ctrl Pts',(-2.6155675817746,12.2,-10.890604656478));
#294723=CARTESIAN_POINT('Ctrl Pts',(-2.61502688791676,12.2,-10.8939641355796));
#294724=CARTESIAN_POINT('Ctrl Pts',(-2.61448105781638,12.2,-10.8973301863875));
#294725=CARTESIAN_POINT('Ctrl Pts',(-2.61393006845892,12.2,-10.9007027674886));
#294726=CARTESIAN_POINT('Ctrl Pts',(-2.61337907910146,12.2,-10.9040753485896));
#294727=CARTESIAN_POINT('Ctrl Pts',(-2.61282293070701,12.2,-10.9074544597546));
#294728=CARTESIAN_POINT('Ctrl Pts',(-2.61226160076952,12.2,-10.910840061381));
#294729=CARTESIAN_POINT('Ctrl Pts',(-2.61170027083203,12.2,-10.9142256630075));
#294730=CARTESIAN_POINT('Ctrl Pts',(-2.61113375908657,12.2,-10.9176177551335));
#294731=CARTESIAN_POINT('Ctrl Pts',(-2.61056204364972,12.2,-10.9210162972591));
#294732=CARTESIAN_POINT('Ctrl Pts',(-2.609990328109,12.2,-10.9244148400021));
#294733=CARTESIAN_POINT('Ctrl Pts',(-2.60941340837517,12.2,-10.9278198330303));
#294734=CARTESIAN_POINT('Ctrl Pts',(-2.60883126287318,12.2,-10.931231235777));
#294735=CARTESIAN_POINT('Ctrl Pts',(-2.60824911747695,12.2,-10.9346426379039));
#294736=CARTESIAN_POINT('Ctrl Pts',(-2.60766174576073,12.2,-10.9380604498485));
#294737=CARTESIAN_POINT('Ctrl Pts',(-2.60706912637705,12.2,-10.9414846321875));
#294738=CARTESIAN_POINT('Ctrl Pts',(-2.60647650699336,12.2,-10.9449088145266));
#294739=CARTESIAN_POINT('Ctrl Pts',(-2.60587863994614,12.2,-10.9483393671657));
#294740=CARTESIAN_POINT('Ctrl Pts',(-2.60527550313426,12.2,-10.9517762493747));
#294741=CARTESIAN_POINT('Ctrl Pts',(-2.60467236632238,12.2,-10.9552131315837));
#294742=CARTESIAN_POINT('Ctrl Pts',(-2.6040639611278,12.2,-10.9586563446086));
#294743=CARTESIAN_POINT('Ctrl Pts',(-2.60345026423343,12.2,-10.962105848275));
#294744=CARTESIAN_POINT('Ctrl Pts',(-2.60283656733906,12.2,-10.9655553519413));
#294745=CARTESIAN_POINT('Ctrl Pts',(-2.60221757902824,12.2,-10.9690111466824));
#294746=CARTESIAN_POINT('Ctrl Pts',(-2.60159327959305,12.2,-10.9724731923894));
#294747=CARTESIAN_POINT('Ctrl Pts',(-2.60096898015786,12.2,-10.9759352380964));
#294748=CARTESIAN_POINT('Ctrl Pts',(-2.60033936879759,12.2,-10.9794035354312));
#294749=CARTESIAN_POINT('Ctrl Pts',(-2.59970442391456,12.2,-10.9828780448111));
#294750=CARTESIAN_POINT('Ctrl Pts',(-2.59906947903152,12.2,-10.9863525541911));
#294751=CARTESIAN_POINT('Ctrl Pts',(-2.59842920081665,12.2,-10.9898332763007));
#294752=CARTESIAN_POINT('Ctrl Pts',(-2.5977835698825,12.2,-10.9933201710065));
#294753=CARTESIAN_POINT('Ctrl Pts',(-2.59713793883106,12.2,-10.9968070663458));
#294754=CARTESIAN_POINT('Ctrl Pts',(-2.59648695308646,12.2,-11.0003001351701));
#294755=CARTESIAN_POINT('Ctrl Pts',(-2.59583059311534,12.2,-11.0037993384711));
#294756=CARTESIAN_POINT('Ctrl Pts',(-2.59495544668589,12.2,-11.0084649418131));
#294757=CARTESIAN_POINT('Ctrl Pts',(-2.59407074609382,12.2,-11.0131414503702));
#294758=CARTESIAN_POINT('Ctrl Pts',(-2.59317644305645,12.2,-11.0178287723752));
#294759=CARTESIAN_POINT('Ctrl Pts',(-2.59250571574795,12.2,-11.0213442640386));
#294760=CARTESIAN_POINT('Ctrl Pts',(-2.59182958762317,12.2,-11.0248658385099));
#294761=CARTESIAN_POINT('Ctrl Pts',(-2.591148036857,12.2,-11.0283934567143));
#294762=CARTESIAN_POINT('Ctrl Pts',(-2.59046648596702,12.2,-11.0319210755595));
#294763=CARTESIAN_POINT('Ctrl Pts',(-2.58977951430051,12.2,-11.0354547392731));
#294764=CARTESIAN_POINT('Ctrl Pts',(-2.58908710086581,12.2,-11.0389944085383));
#294765=CARTESIAN_POINT('Ctrl Pts',(-2.58793307876814,12.2,-11.0448938558133));
#294766=CARTESIAN_POINT('Ctrl Pts',(-2.58676394189133,12.2,-11.0508099852608));
#294767=CARTESIAN_POINT('Ctrl Pts',(-2.58557959889667,12.2,-11.0567426209323));
#294768=CARTESIAN_POINT('Ctrl Pts',(-2.58439525577291,12.2,-11.0626752572504));
#294769=CARTESIAN_POINT('Ctrl Pts',(-2.58319570712997,12.2,-11.0686243999043));
#294770=CARTESIAN_POINT('Ctrl Pts',(-2.58198086240899,12.2,-11.0745898721947));
#294771=CARTESIAN_POINT('Ctrl Pts',(-2.58125195547047,12.2,-11.0781691560891));
#294772=CARTESIAN_POINT('Ctrl Pts',(-2.58051754206374,12.2,-11.0817543194768));
#294773=CARTESIAN_POINT('Ctrl Pts',(-2.57977760408045,12.2,-11.0853453242911));
#294774=CARTESIAN_POINT('Ctrl Pts',(-2.57903766623159,12.2,-11.0889363284531));
#294775=CARTESIAN_POINT('Ctrl Pts',(-2.57829220346561,12.2,-11.0925331736306));
#294776=CARTESIAN_POINT('Ctrl Pts',(-2.5775411956214,12.2,-11.0961358233887));
#294777=CARTESIAN_POINT('Ctrl Pts',(-2.5767901877772,12.2,-11.0997384731468));
#294778=CARTESIAN_POINT('Ctrl Pts',(-2.57603363493972,12.2,-11.1033469255248));
#294779=CARTESIAN_POINT('Ctrl Pts',(-2.5752715201336,12.2,-11.1069611441857));
#294780=CARTESIAN_POINT('Ctrl Pts',(-2.57450940532747,12.2,-11.1105753628466));
#294781=CARTESIAN_POINT('Ctrl Pts',(-2.57374172875534,12.2,-11.1141953480984));
#294782=CARTESIAN_POINT('Ctrl Pts',(-2.57296846953343,12.2,-11.1178210627583));
#294783=CARTESIAN_POINT('Ctrl Pts',(-2.57219521031153,12.2,-11.1214467774182));
#294784=CARTESIAN_POINT('Ctrl Pts',(-2.57141637063985,12.2,-11.1250782207029));
#294785=CARTESIAN_POINT('Ctrl Pts',(-2.5706319318355,12.2,-11.128715357362));
#294786=CARTESIAN_POINT('Ctrl Pts',(-2.56984749303116,12.2,-11.132352494021));
#294787=CARTESIAN_POINT('Ctrl Pts',(-2.56905745493083,12.2,-11.1359953233451));
#294788=CARTESIAN_POINT('Ctrl Pts',(-2.56826179767065,12.2,-11.1396438057691));
#294789=CARTESIAN_POINT('Ctrl Pts',(-2.56746614041046,12.2,-11.1432922881932));
#294790=CARTESIAN_POINT('Ctrl Pts',(-2.56666486591258,12.2,-11.1469464247525));
#294791=CARTESIAN_POINT('Ctrl Pts',(-2.56585795469266,12.2,-11.1506061784522));
#294792=CARTESIAN_POINT('Ctrl Pts',(-2.56478207296838,12.2,-11.1554858504949));
#294793=CARTESIAN_POINT('Ctrl Pts',(-2.56369617228761,12.2,-11.1603755090857));
#294794=CARTESIAN_POINT('Ctrl Pts',(-2.56260021378343,12.2,-11.1652750757416));
#294795=CARTESIAN_POINT('Ctrl Pts',(-2.56177824497996,12.2,-11.1689497503998));
#294796=CARTESIAN_POINT('Ctrl Pts',(-2.56095061872672,12.2,-11.172629997866));
#294797=CARTESIAN_POINT('Ctrl Pts',(-2.56011731584083,12.2,-11.1763157773567));
#294798=CARTESIAN_POINT('Ctrl Pts',(-2.55928401295493,12.2,-11.1800015568472));
#294799=CARTESIAN_POINT('Ctrl Pts',(-2.55844503222431,12.2,-11.183692866235));
#294800=CARTESIAN_POINT('Ctrl Pts',(-2.5576003524218,12.2,-11.1873896640348));
#294801=CARTESIAN_POINT('Ctrl Pts',(-2.5564741125828,12.2,-11.1923187282155));
#294802=CARTESIAN_POINT('Ctrl Pts',(-2.55533774007136,12.2,-11.1972575404348));
#294803=CARTESIAN_POINT('Ctrl Pts',(-2.5541912119275,12.2,-11.20220605643));
#294804=CARTESIAN_POINT('Ctrl Pts',(-2.55333131589771,12.2,-11.2059174430893));
#294805=CARTESIAN_POINT('Ctrl Pts',(-2.55246571115834,12.2,-11.2096342863238));
#294806=CARTESIAN_POINT('Ctrl Pts',(-2.55159439100006,12.2,-11.213356592));
#294807=CARTESIAN_POINT('Ctrl Pts',(-2.17615954800006,15.2,-11.292224299));
#294808=CARTESIAN_POINT('Ctrl Pts',(-2.17615954800006,11.6,-11.292224299));
#294809=CARTESIAN_POINT('Ctrl Pts',(-2.17570045500006,15.2,-11.291612887));
#294810=CARTESIAN_POINT('Ctrl Pts',(-2.17570045500006,11.6,-11.291612887));
#294811=CARTESIAN_POINT('Ctrl Pts',(-2.17478276600006,15.2,-11.290390245));
#294812=CARTESIAN_POINT('Ctrl Pts',(-2.17478276600006,11.6,-11.290390245));
#294813=CARTESIAN_POINT('Ctrl Pts',(-2.17340771700006,15.2,-11.28855682));
#294814=CARTESIAN_POINT('Ctrl Pts',(-2.17340771700006,11.6,-11.28855682));
#294815=CARTESIAN_POINT('Ctrl Pts',(-2.17157728800006,15.2,-11.286113334));
#294816=CARTESIAN_POINT('Ctrl Pts',(-2.17157728800006,11.6,-11.286113334));
#294817=CARTESIAN_POINT('Ctrl Pts',(-2.16929420200006,15.2,-11.283060773));
#294818=CARTESIAN_POINT('Ctrl Pts',(-2.16929420200006,11.6,-11.283060773));
#294819=CARTESIAN_POINT('Ctrl Pts',(-2.16701606700005,15.2,-11.280010015));
#294820=CARTESIAN_POINT('Ctrl Pts',(-2.16701606700005,11.6,-11.280010015));
#294821=CARTESIAN_POINT('Ctrl Pts',(-2.16474288100006,15.2,-11.276961058));
#294822=CARTESIAN_POINT('Ctrl Pts',(-2.16474288100006,11.6,-11.276961058));
#294823=CARTESIAN_POINT('Ctrl Pts',(-2.16247464600006,15.2,-11.273913908));
#294824=CARTESIAN_POINT('Ctrl Pts',(-2.16247464600006,11.6,-11.273913908));
#294825=CARTESIAN_POINT('Ctrl Pts',(-2.16021136000006,15.2,-11.27086857));
#294826=CARTESIAN_POINT('Ctrl Pts',(-2.16021136000006,11.6,-11.27086857));
#294827=CARTESIAN_POINT('Ctrl Pts',(-2.15795302500006,15.2,-11.267825054));
#294828=CARTESIAN_POINT('Ctrl Pts',(-2.15795302500006,11.6,-11.267825054));
#294829=CARTESIAN_POINT('Ctrl Pts',(-2.15569963800006,15.2,-11.264783368));
#294830=CARTESIAN_POINT('Ctrl Pts',(-2.15569963800006,11.6,-11.264783368));
#294831=CARTESIAN_POINT('Ctrl Pts',(-2.15345120200006,15.2,-11.261743524));
#294832=CARTESIAN_POINT('Ctrl Pts',(-2.15345120200006,11.6,-11.261743524));
#294833=CARTESIAN_POINT('Ctrl Pts',(-2.15120771500006,15.2,-11.258705531));
#294834=CARTESIAN_POINT('Ctrl Pts',(-2.15120771500006,11.6,-11.258705531));
#294835=CARTESIAN_POINT('Ctrl Pts',(-2.14896917600006,15.2,-11.255669403));
#294836=CARTESIAN_POINT('Ctrl Pts',(-2.14896917600006,11.6,-11.255669403));
#294837=CARTESIAN_POINT('Ctrl Pts',(-2.14673558400006,15.2,-11.252635149));
#294838=CARTESIAN_POINT('Ctrl Pts',(-2.14673558400006,11.6,-11.252635149));
#294839=CARTESIAN_POINT('Ctrl Pts',(-2.14450694000006,15.2,-11.249602777));
#294840=CARTESIAN_POINT('Ctrl Pts',(-2.14450694000006,11.6,-11.249602777));
#294841=CARTESIAN_POINT('Ctrl Pts',(-2.14228324400006,15.2,-11.246572299));
#294842=CARTESIAN_POINT('Ctrl Pts',(-2.14228324400006,11.6,-11.246572299));
#294843=CARTESIAN_POINT('Ctrl Pts',(-2.14006449500005,15.2,-11.243543721));
#294844=CARTESIAN_POINT('Ctrl Pts',(-2.14006449500005,11.6,-11.243543721));
#294845=CARTESIAN_POINT('Ctrl Pts',(-2.13785069300005,15.2,-11.24051705));
#294846=CARTESIAN_POINT('Ctrl Pts',(-2.13785069300005,11.6,-11.24051705));
#294847=CARTESIAN_POINT('Ctrl Pts',(-2.13564183800006,15.2,-11.237492297));
#294848=CARTESIAN_POINT('Ctrl Pts',(-2.13564183800006,11.6,-11.237492297));
#294849=CARTESIAN_POINT('Ctrl Pts',(-2.13343792800006,15.2,-11.234469469));
#294850=CARTESIAN_POINT('Ctrl Pts',(-2.13343792800006,11.6,-11.234469469));
#294851=CARTESIAN_POINT('Ctrl Pts',(-2.13123896500006,15.2,-11.231448574));
#294852=CARTESIAN_POINT('Ctrl Pts',(-2.13123896500006,11.6,-11.231448574));
#294853=CARTESIAN_POINT('Ctrl Pts',(-2.12904494800005,15.2,-11.228429624));
#294854=CARTESIAN_POINT('Ctrl Pts',(-2.12904494800005,11.6,-11.228429624));
#294855=CARTESIAN_POINT('Ctrl Pts',(-2.12685587600005,15.2,-11.225412626));
#294856=CARTESIAN_POINT('Ctrl Pts',(-2.12685587600005,11.6,-11.225412626));
#294857=CARTESIAN_POINT('Ctrl Pts',(-2.12467174800006,15.2,-11.222397592));
#294858=CARTESIAN_POINT('Ctrl Pts',(-2.12467174800006,11.6,-11.222397592));
#294859=CARTESIAN_POINT('Ctrl Pts',(-2.12249256500006,15.2,-11.219384528));
#294860=CARTESIAN_POINT('Ctrl Pts',(-2.12249256500006,11.6,-11.219384528));
#294861=CARTESIAN_POINT('Ctrl Pts',(-2.12031832600006,15.2,-11.216373446));
#294862=CARTESIAN_POINT('Ctrl Pts',(-2.12031832600006,11.6,-11.216373446));
#294863=CARTESIAN_POINT('Ctrl Pts',(-2.11814903000006,15.2,-11.213364356));
#294864=CARTESIAN_POINT('Ctrl Pts',(-2.11814903000006,11.6,-11.213364356));
#294865=CARTESIAN_POINT('Ctrl Pts',(-2.11598467700005,15.2,-11.210357264));
#294866=CARTESIAN_POINT('Ctrl Pts',(-2.11598467700005,11.6,-11.210357264));
#294867=CARTESIAN_POINT('Ctrl Pts',(-2.11382526700006,15.2,-11.207352181));
#294868=CARTESIAN_POINT('Ctrl Pts',(-2.11382526700006,11.6,-11.207352181));
#294869=CARTESIAN_POINT('Ctrl Pts',(-2.11167080000005,15.2,-11.204349116));
#294870=CARTESIAN_POINT('Ctrl Pts',(-2.11167080000005,11.6,-11.204349116));
#294871=CARTESIAN_POINT('Ctrl Pts',(-2.10952127400006,15.2,-11.201348078));
#294872=CARTESIAN_POINT('Ctrl Pts',(-2.10952127400006,11.6,-11.201348078));
#294873=CARTESIAN_POINT('Ctrl Pts',(-2.10737669000005,15.2,-11.198349076));
#294874=CARTESIAN_POINT('Ctrl Pts',(-2.10737669000005,11.6,-11.198349076));
#294875=CARTESIAN_POINT('Ctrl Pts',(-2.10523704700006,15.2,-11.19535212));
#294876=CARTESIAN_POINT('Ctrl Pts',(-2.10523704700006,11.6,-11.19535212));
#294877=CARTESIAN_POINT('Ctrl Pts',(-2.10310234500006,15.2,-11.192357218));
#294878=CARTESIAN_POINT('Ctrl Pts',(-2.10310234500006,11.6,-11.192357218));
#294879=CARTESIAN_POINT('Ctrl Pts',(-2.10097258200005,15.2,-11.18936438));
#294880=CARTESIAN_POINT('Ctrl Pts',(-2.10097258200005,11.6,-11.18936438));
#294881=CARTESIAN_POINT('Ctrl Pts',(-2.09884776000006,15.2,-11.186373616));
#294882=CARTESIAN_POINT('Ctrl Pts',(-2.09884776000006,11.6,-11.186373616));
#294883=CARTESIAN_POINT('Ctrl Pts',(-2.09672787600006,15.2,-11.183384935));
#294884=CARTESIAN_POINT('Ctrl Pts',(-2.09672787600006,11.6,-11.183384935));
#294885=CARTESIAN_POINT('Ctrl Pts',(-2.09461293200006,15.2,-11.180398346));
#294886=CARTESIAN_POINT('Ctrl Pts',(-2.09461293200006,11.6,-11.180398346));
#294887=CARTESIAN_POINT('Ctrl Pts',(-2.09250292400006,15.2,-11.177413859));
#294888=CARTESIAN_POINT('Ctrl Pts',(-2.09250292400006,11.6,-11.177413859));
#294889=CARTESIAN_POINT('Ctrl Pts',(-2.09039785500006,15.2,-11.174431482));
#294890=CARTESIAN_POINT('Ctrl Pts',(-2.09039785500006,11.6,-11.174431482));
#294891=CARTESIAN_POINT('Ctrl Pts',(-2.08829772300006,15.2,-11.171451227));
#294892=CARTESIAN_POINT('Ctrl Pts',(-2.08829772300006,11.6,-11.171451227));
#294893=CARTESIAN_POINT('Ctrl Pts',(-2.08620252700006,15.2,-11.1684731));
#294894=CARTESIAN_POINT('Ctrl Pts',(-2.08620252700006,11.6,-11.1684731));
#294895=CARTESIAN_POINT('Ctrl Pts',(-2.08411226900005,15.2,-11.165497114));
#294896=CARTESIAN_POINT('Ctrl Pts',(-2.08411226900005,11.6,-11.165497114));
#294897=CARTESIAN_POINT('Ctrl Pts',(-2.08202694500006,15.2,-11.162523276));
#294898=CARTESIAN_POINT('Ctrl Pts',(-2.08202694500006,11.6,-11.162523276));
#294899=CARTESIAN_POINT('Ctrl Pts',(-2.07994655600006,15.2,-11.159551596));
#294900=CARTESIAN_POINT('Ctrl Pts',(-2.07994655600006,11.6,-11.159551596));
#294901=CARTESIAN_POINT('Ctrl Pts',(-2.07787110100006,15.2,-11.156582084));
#294902=CARTESIAN_POINT('Ctrl Pts',(-2.07787110100006,11.6,-11.156582084));
#294903=CARTESIAN_POINT('Ctrl Pts',(-2.07580058000006,15.2,-11.153614748));
#294904=CARTESIAN_POINT('Ctrl Pts',(-2.07580058000006,11.6,-11.153614748));
#294905=CARTESIAN_POINT('Ctrl Pts',(-2.07373499200005,15.2,-11.1506496));
#294906=CARTESIAN_POINT('Ctrl Pts',(-2.07373499200005,11.6,-11.1506496));
#294907=CARTESIAN_POINT('Ctrl Pts',(-2.07167433800006,15.2,-11.147686647));
#294908=CARTESIAN_POINT('Ctrl Pts',(-2.07167433800006,11.6,-11.147686647));
#294909=CARTESIAN_POINT('Ctrl Pts',(-2.06961861500006,15.2,-11.1447259));
#294910=CARTESIAN_POINT('Ctrl Pts',(-2.06961861500006,11.6,-11.1447259));
#294911=CARTESIAN_POINT('Ctrl Pts',(-2.06756782400006,15.2,-11.141767369));
#294912=CARTESIAN_POINT('Ctrl Pts',(-2.06756782400006,11.6,-11.141767369));
#294913=CARTESIAN_POINT('Ctrl Pts',(-2.06552196300006,15.2,-11.138811062));
#294914=CARTESIAN_POINT('Ctrl Pts',(-2.06552196300006,11.6,-11.138811062));
#294915=CARTESIAN_POINT('Ctrl Pts',(-2.06348103200006,15.2,-11.13585699));
#294916=CARTESIAN_POINT('Ctrl Pts',(-2.06348103200006,11.6,-11.13585699));
#294917=CARTESIAN_POINT('Ctrl Pts',(-2.06144503200006,15.2,-11.132905162));
#294918=CARTESIAN_POINT('Ctrl Pts',(-2.06144503200006,11.6,-11.132905162));
#294919=CARTESIAN_POINT('Ctrl Pts',(-2.05941396000005,15.2,-11.129955589));
#294920=CARTESIAN_POINT('Ctrl Pts',(-2.05941396000005,11.6,-11.129955589));
#294921=CARTESIAN_POINT('Ctrl Pts',(-2.05738781600005,15.2,-11.127008278));
#294922=CARTESIAN_POINT('Ctrl Pts',(-2.05738781600005,11.6,-11.127008278));
#294923=CARTESIAN_POINT('Ctrl Pts',(-2.05536660000006,15.2,-11.12406324));
#294924=CARTESIAN_POINT('Ctrl Pts',(-2.05536660000006,11.6,-11.12406324));
#294925=CARTESIAN_POINT('Ctrl Pts',(-2.05335031200006,15.2,-11.121120485));
#294926=CARTESIAN_POINT('Ctrl Pts',(-2.05335031200006,11.6,-11.121120485));
#294927=CARTESIAN_POINT('Ctrl Pts',(-2.05133894900006,15.2,-11.118180023));
#294928=CARTESIAN_POINT('Ctrl Pts',(-2.05133894900006,11.6,-11.118180023));
#294929=CARTESIAN_POINT('Ctrl Pts',(-2.04933251100006,15.2,-11.115241862));
#294930=CARTESIAN_POINT('Ctrl Pts',(-2.04933251100006,11.6,-11.115241862));
#294931=CARTESIAN_POINT('Ctrl Pts',(-2.04733100000006,15.2,-11.112306013));
#294932=CARTESIAN_POINT('Ctrl Pts',(-2.04733100000006,11.6,-11.112306013));
#294933=CARTESIAN_POINT('Ctrl Pts',(-2.04533441100006,15.2,-11.109372486));
#294934=CARTESIAN_POINT('Ctrl Pts',(-2.04533441100006,11.6,-11.109372486));
#294935=CARTESIAN_POINT('Ctrl Pts',(-2.04334274700006,15.2,-11.106441291));
#294936=CARTESIAN_POINT('Ctrl Pts',(-2.04334274700006,11.6,-11.106441291));
#294937=CARTESIAN_POINT('Ctrl Pts',(-2.04135600500006,15.2,-11.103512437));
#294938=CARTESIAN_POINT('Ctrl Pts',(-2.04135600500006,11.6,-11.103512437));
#294939=CARTESIAN_POINT('Ctrl Pts',(-2.03937418400006,15.2,-11.100585934));
#294940=CARTESIAN_POINT('Ctrl Pts',(-2.03937418400006,11.6,-11.100585934));
#294941=CARTESIAN_POINT('Ctrl Pts',(-2.03739728600006,15.2,-11.097661791));
#294942=CARTESIAN_POINT('Ctrl Pts',(-2.03739728600006,11.6,-11.097661791));
#294943=CARTESIAN_POINT('Ctrl Pts',(-2.03542530900005,15.2,-11.094740019));
#294944=CARTESIAN_POINT('Ctrl Pts',(-2.03542530900005,11.6,-11.094740019));
#294945=CARTESIAN_POINT('Ctrl Pts',(-2.03345825000006,15.2,-11.091820627));
#294946=CARTESIAN_POINT('Ctrl Pts',(-2.03345825000006,11.6,-11.091820627));
#294947=CARTESIAN_POINT('Ctrl Pts',(-2.03149611100006,15.2,-11.088903627));
#294948=CARTESIAN_POINT('Ctrl Pts',(-2.03149611100006,11.6,-11.088903627));
#294949=CARTESIAN_POINT('Ctrl Pts',(-2.02953889000006,15.2,-11.085989026));
#294950=CARTESIAN_POINT('Ctrl Pts',(-2.02953889000006,11.6,-11.085989026));
#294951=CARTESIAN_POINT('Ctrl Pts',(-2.02758658500006,15.2,-11.083076836));
#294952=CARTESIAN_POINT('Ctrl Pts',(-2.02758658500006,11.6,-11.083076836));
#294953=CARTESIAN_POINT('Ctrl Pts',(-2.02563919900005,15.2,-11.080167065));
#294954=CARTESIAN_POINT('Ctrl Pts',(-2.02563919900005,11.6,-11.080167065));
#294955=CARTESIAN_POINT('Ctrl Pts',(-2.02369672800006,15.2,-11.077259724));
#294956=CARTESIAN_POINT('Ctrl Pts',(-2.02369672800006,11.6,-11.077259724));
#294957=CARTESIAN_POINT('Ctrl Pts',(-2.02175917100006,15.2,-11.074354824));
#294958=CARTESIAN_POINT('Ctrl Pts',(-2.02175917100006,11.6,-11.074354824));
#294959=CARTESIAN_POINT('Ctrl Pts',(-2.01982652900006,15.2,-11.071452373));
#294960=CARTESIAN_POINT('Ctrl Pts',(-2.01982652900006,11.6,-11.071452373));
#294961=CARTESIAN_POINT('Ctrl Pts',(-2.01789880000006,15.2,-11.068552382));
#294962=CARTESIAN_POINT('Ctrl Pts',(-2.01789880000006,11.6,-11.068552382));
#294963=CARTESIAN_POINT('Ctrl Pts',(-2.01597598400005,15.2,-11.065654863));
#294964=CARTESIAN_POINT('Ctrl Pts',(-2.01597598400005,11.6,-11.065654863));
#294965=CARTESIAN_POINT('Ctrl Pts',(-2.01405807900006,15.2,-11.062759821));
#294966=CARTESIAN_POINT('Ctrl Pts',(-2.01405807900006,11.6,-11.062759821));
#294967=CARTESIAN_POINT('Ctrl Pts',(-2.01214508600006,15.2,-11.059867271));
#294968=CARTESIAN_POINT('Ctrl Pts',(-2.01214508600006,11.6,-11.059867271));
#294969=CARTESIAN_POINT('Ctrl Pts',(-2.01023700100006,15.2,-11.056977221));
#294970=CARTESIAN_POINT('Ctrl Pts',(-2.01023700100006,11.6,-11.056977221));
#294971=CARTESIAN_POINT('Ctrl Pts',(-2.00833382600006,15.2,-11.054089681));
#294972=CARTESIAN_POINT('Ctrl Pts',(-2.00833382600006,11.6,-11.054089681));
#294973=CARTESIAN_POINT('Ctrl Pts',(-2.00643555900006,15.2,-11.05120466));
#294974=CARTESIAN_POINT('Ctrl Pts',(-2.00643555900006,11.6,-11.05120466));
#294975=CARTESIAN_POINT('Ctrl Pts',(-2.00454219900006,15.2,-11.048322171));
#294976=CARTESIAN_POINT('Ctrl Pts',(-2.00454219900006,11.6,-11.048322171));
#294977=CARTESIAN_POINT('Ctrl Pts',(-2.00265374600006,15.2,-11.045442222));
#294978=CARTESIAN_POINT('Ctrl Pts',(-2.00265374600006,11.6,-11.045442222));
#294979=CARTESIAN_POINT('Ctrl Pts',(-2.00077019700006,15.2,-11.042564824));
#294980=CARTESIAN_POINT('Ctrl Pts',(-2.00077019700006,11.6,-11.042564824));
#294981=CARTESIAN_POINT('Ctrl Pts',(-1.99889155400006,15.2,-11.039689987));
#294982=CARTESIAN_POINT('Ctrl Pts',(-1.99889155400006,11.6,-11.039689987));
#294983=CARTESIAN_POINT('Ctrl Pts',(-1.99701781300006,15.2,-11.03681772));
#294984=CARTESIAN_POINT('Ctrl Pts',(-1.99701781300006,11.6,-11.03681772));
#294985=CARTESIAN_POINT('Ctrl Pts',(-1.99514897500006,15.2,-11.033948035));
#294986=CARTESIAN_POINT('Ctrl Pts',(-1.99514897500006,11.6,-11.033948035));
#294987=CARTESIAN_POINT('Ctrl Pts',(-1.99328503900006,15.2,-11.031080942));
#294988=CARTESIAN_POINT('Ctrl Pts',(-1.99328503900006,11.6,-11.031080942));
#294989=CARTESIAN_POINT('Ctrl Pts',(-1.99142600300006,15.2,-11.02821645));
#294990=CARTESIAN_POINT('Ctrl Pts',(-1.99142600300006,11.6,-11.02821645));
#294991=CARTESIAN_POINT('Ctrl Pts',(-1.98957186800006,15.2,-11.025354571));
#294992=CARTESIAN_POINT('Ctrl Pts',(-1.98957186800006,11.6,-11.025354571));
#294993=CARTESIAN_POINT('Ctrl Pts',(-1.98772263100006,15.2,-11.022495313));
#294994=CARTESIAN_POINT('Ctrl Pts',(-1.98772263100006,11.6,-11.022495313));
#294995=CARTESIAN_POINT('Ctrl Pts',(-1.98587829000005,15.2,-11.019638689));
#294996=CARTESIAN_POINT('Ctrl Pts',(-1.98587829000005,11.6,-11.019638689));
#294997=CARTESIAN_POINT('Ctrl Pts',(-1.98403884700005,15.2,-11.016784707));
#294998=CARTESIAN_POINT('Ctrl Pts',(-1.98403884700005,11.6,-11.016784707));
#294999=CARTESIAN_POINT('Ctrl Pts',(-1.98220430000006,15.2,-11.013933379));
#295000=CARTESIAN_POINT('Ctrl Pts',(-1.98220430000006,11.6,-11.013933379));
#295001=CARTESIAN_POINT('Ctrl Pts',(-1.98037464600006,15.2,-11.011084714));
#295002=CARTESIAN_POINT('Ctrl Pts',(-1.98037464600006,11.6,-11.011084714));
#295003=CARTESIAN_POINT('Ctrl Pts',(-1.97854988600006,15.2,-11.008238724));
#295004=CARTESIAN_POINT('Ctrl Pts',(-1.97854988600006,11.6,-11.008238724));
#295005=CARTESIAN_POINT('Ctrl Pts',(-1.97673001900006,15.2,-11.005395418));
#295006=CARTESIAN_POINT('Ctrl Pts',(-1.97673001900006,11.6,-11.005395418));
#295007=CARTESIAN_POINT('Ctrl Pts',(-1.97491504200005,15.2,-11.002554807));
#295008=CARTESIAN_POINT('Ctrl Pts',(-1.97491504200005,11.6,-11.002554807));
#295009=CARTESIAN_POINT('Ctrl Pts',(-1.97310495700005,15.2,-10.999716901));
#295010=CARTESIAN_POINT('Ctrl Pts',(-1.97310495700005,11.6,-10.999716901));
#295011=CARTESIAN_POINT('Ctrl Pts',(-1.97129976000005,15.2,-10.996881712));
#295012=CARTESIAN_POINT('Ctrl Pts',(-1.97129976000005,11.6,-10.996881712));
#295013=CARTESIAN_POINT('Ctrl Pts',(-1.96949945100006,15.2,-10.994049247));
#295014=CARTESIAN_POINT('Ctrl Pts',(-1.96949945100006,11.6,-10.994049247));
#295015=CARTESIAN_POINT('Ctrl Pts',(-1.96770402900006,15.2,-10.99121952));
#295016=CARTESIAN_POINT('Ctrl Pts',(-1.96770402900006,11.6,-10.99121952));
#295017=CARTESIAN_POINT('Ctrl Pts',(-1.96591349400005,15.2,-10.988392541));
#295018=CARTESIAN_POINT('Ctrl Pts',(-1.96591349400005,11.6,-10.988392541));
#295019=CARTESIAN_POINT('Ctrl Pts',(-1.96412784300006,15.2,-10.985568319));
#295020=CARTESIAN_POINT('Ctrl Pts',(-1.96412784300006,11.6,-10.985568319));
#295021=CARTESIAN_POINT('Ctrl Pts',(-1.96234707500006,15.2,-10.982746866));
#295022=CARTESIAN_POINT('Ctrl Pts',(-1.96234707500006,11.6,-10.982746866));
#295023=CARTESIAN_POINT('Ctrl Pts',(-1.96057119000006,15.2,-10.979928192));
#295024=CARTESIAN_POINT('Ctrl Pts',(-1.96057119000006,11.6,-10.979928192));
#295025=CARTESIAN_POINT('Ctrl Pts',(-1.95880018600006,15.2,-10.977112307));
#295026=CARTESIAN_POINT('Ctrl Pts',(-1.95880018600006,11.6,-10.977112307));
#295027=CARTESIAN_POINT('Ctrl Pts',(-1.95703406200006,15.2,-10.974299223));
#295028=CARTESIAN_POINT('Ctrl Pts',(-1.95703406200006,11.6,-10.974299223));
#295029=CARTESIAN_POINT('Ctrl Pts',(-1.95527281700006,15.2,-10.971488949));
#295030=CARTESIAN_POINT('Ctrl Pts',(-1.95527281700006,11.6,-10.971488949));
#295031=CARTESIAN_POINT('Ctrl Pts',(-1.95351645100006,15.2,-10.968681498));
#295032=CARTESIAN_POINT('Ctrl Pts',(-1.95351645100006,11.6,-10.968681498));
#295033=CARTESIAN_POINT('Ctrl Pts',(-1.95176495900005,15.2,-10.965876877));
#295034=CARTESIAN_POINT('Ctrl Pts',(-1.95176495900005,11.6,-10.965876877));
#295035=CARTESIAN_POINT('Ctrl Pts',(-1.95001834500005,15.2,-10.963075101));
#295036=CARTESIAN_POINT('Ctrl Pts',(-1.95001834500005,11.6,-10.963075101));
#295037=CARTESIAN_POINT('Ctrl Pts',(-1.94827660300006,15.2,-10.960276177));
#295038=CARTESIAN_POINT('Ctrl Pts',(-1.94827660300006,11.6,-10.960276177));
#295039=CARTESIAN_POINT('Ctrl Pts',(-1.94653973400006,15.2,-10.957480118));
#295040=CARTESIAN_POINT('Ctrl Pts',(-1.94653973400006,11.6,-10.957480118));
#295041=CARTESIAN_POINT('Ctrl Pts',(-1.94480773800006,15.2,-10.954686934));
#295042=CARTESIAN_POINT('Ctrl Pts',(-1.94480773800006,11.6,-10.954686934));
#295043=CARTESIAN_POINT('Ctrl Pts',(-1.94308061000006,15.2,-10.951896636));
#295044=CARTESIAN_POINT('Ctrl Pts',(-1.94308061000006,11.6,-10.951896636));
#295045=CARTESIAN_POINT('Ctrl Pts',(-1.94135835200006,15.2,-10.949109235));
#295046=CARTESIAN_POINT('Ctrl Pts',(-1.94135835200006,11.6,-10.949109235));
#295047=CARTESIAN_POINT('Ctrl Pts',(-1.93964096300005,15.2,-10.946324741));
#295048=CARTESIAN_POINT('Ctrl Pts',(-1.93964096300005,11.6,-10.946324741));
#295049=CARTESIAN_POINT('Ctrl Pts',(-1.93792843900006,15.2,-10.943543166));
#295050=CARTESIAN_POINT('Ctrl Pts',(-1.93792843900006,11.6,-10.943543166));
#295051=CARTESIAN_POINT('Ctrl Pts',(-1.93622078100006,15.2,-10.940764519));
#295052=CARTESIAN_POINT('Ctrl Pts',(-1.93622078100006,11.6,-10.940764519));
#295053=CARTESIAN_POINT('Ctrl Pts',(-1.93451798600006,15.2,-10.937988814));
#295054=CARTESIAN_POINT('Ctrl Pts',(-1.93451798600006,11.6,-10.937988814));
#295055=CARTESIAN_POINT('Ctrl Pts',(-1.93282005500006,15.2,-10.935216058));
#295056=CARTESIAN_POINT('Ctrl Pts',(-1.93282005500006,11.6,-10.935216058));
#295057=CARTESIAN_POINT('Ctrl Pts',(-1.93112698400005,15.2,-10.932446266));
#295058=CARTESIAN_POINT('Ctrl Pts',(-1.93112698400005,11.6,-10.932446266));
#295059=CARTESIAN_POINT('Ctrl Pts',(-1.92943877200005,15.2,-10.929679446));
#295060=CARTESIAN_POINT('Ctrl Pts',(-1.92943877200005,11.6,-10.929679446));
#295061=CARTESIAN_POINT('Ctrl Pts',(-1.92775541900006,15.2,-10.92691561));
#295062=CARTESIAN_POINT('Ctrl Pts',(-1.92775541900006,11.6,-10.92691561));
#295063=CARTESIAN_POINT('Ctrl Pts',(-1.92607692400005,15.2,-10.924154768));
#295064=CARTESIAN_POINT('Ctrl Pts',(-1.92607692400005,11.6,-10.924154768));
#295065=CARTESIAN_POINT('Ctrl Pts',(-1.92440328400005,15.2,-10.921396933));
#295066=CARTESIAN_POINT('Ctrl Pts',(-1.92440328400005,11.6,-10.921396933));
#295067=CARTESIAN_POINT('Ctrl Pts',(-1.92273449900005,15.2,-10.918642115));
#295068=CARTESIAN_POINT('Ctrl Pts',(-1.92273449900005,11.6,-10.918642115));
#295069=CARTESIAN_POINT('Ctrl Pts',(-1.92107056600005,15.2,-10.915890324));
#295070=CARTESIAN_POINT('Ctrl Pts',(-1.92107056600005,11.6,-10.915890324));
#295071=CARTESIAN_POINT('Ctrl Pts',(-1.91941148400006,15.2,-10.913141573));
#295072=CARTESIAN_POINT('Ctrl Pts',(-1.91941148400006,11.6,-10.913141573));
#295073=CARTESIAN_POINT('Ctrl Pts',(-1.91775725300006,15.2,-10.910395872));
#295074=CARTESIAN_POINT('Ctrl Pts',(-1.91775725300006,11.6,-10.910395872));
#295075=CARTESIAN_POINT('Ctrl Pts',(-1.91610787000006,15.2,-10.907653232));
#295076=CARTESIAN_POINT('Ctrl Pts',(-1.91610787000006,11.6,-10.907653232));
#295077=CARTESIAN_POINT('Ctrl Pts',(-1.91446333500006,15.2,-10.904913664));
#295078=CARTESIAN_POINT('Ctrl Pts',(-1.91446333500006,11.6,-10.904913664));
#295079=CARTESIAN_POINT('Ctrl Pts',(-1.91282364500006,15.2,-10.902177181));
#295080=CARTESIAN_POINT('Ctrl Pts',(-1.91282364500006,11.6,-10.902177181));
#295081=CARTESIAN_POINT('Ctrl Pts',(-1.91118879900006,15.2,-10.899443792));
#295082=CARTESIAN_POINT('Ctrl Pts',(-1.91118879900006,11.6,-10.899443792));
#295083=CARTESIAN_POINT('Ctrl Pts',(-1.90955879600006,15.2,-10.89671351));
#295084=CARTESIAN_POINT('Ctrl Pts',(-1.90955879600006,11.6,-10.89671351));
#295085=CARTESIAN_POINT('Ctrl Pts',(-1.90793363400006,15.2,-10.893986344));
#295086=CARTESIAN_POINT('Ctrl Pts',(-1.90793363400006,11.6,-10.893986344));
#295087=CARTESIAN_POINT('Ctrl Pts',(-1.90631331200006,15.2,-10.891262307));
#295088=CARTESIAN_POINT('Ctrl Pts',(-1.90631331200006,11.6,-10.891262307));
#295089=CARTESIAN_POINT('Ctrl Pts',(-1.90469782800006,15.2,-10.888541409));
#295090=CARTESIAN_POINT('Ctrl Pts',(-1.90469782800006,11.6,-10.888541409));
#295091=CARTESIAN_POINT('Ctrl Pts',(-1.90308718100006,15.2,-10.885823664));
#295092=CARTESIAN_POINT('Ctrl Pts',(-1.90308718100006,11.6,-10.885823664));
#295093=CARTESIAN_POINT('Ctrl Pts',(-1.90148136800006,15.2,-10.88310908));
#295094=CARTESIAN_POINT('Ctrl Pts',(-1.90148136800006,11.6,-10.88310908));
#295095=CARTESIAN_POINT('Ctrl Pts',(-1.89988038900006,15.2,-10.880397671));
#295096=CARTESIAN_POINT('Ctrl Pts',(-1.89988038900006,11.6,-10.880397671));
#295097=CARTESIAN_POINT('Ctrl Pts',(-1.89828424200006,15.2,-10.877689446));
#295098=CARTESIAN_POINT('Ctrl Pts',(-1.89828424200006,11.6,-10.877689446));
#295099=CARTESIAN_POINT('Ctrl Pts',(-1.89669292500006,15.2,-10.874984418));
#295100=CARTESIAN_POINT('Ctrl Pts',(-1.89669292500006,11.6,-10.874984418));
#295101=CARTESIAN_POINT('Ctrl Pts',(-1.89510643700005,15.2,-10.872282597));
#295102=CARTESIAN_POINT('Ctrl Pts',(-1.89510643700005,11.6,-10.872282597));
#295103=CARTESIAN_POINT('Ctrl Pts',(-1.89352477600006,15.2,-10.869583997));
#295104=CARTESIAN_POINT('Ctrl Pts',(-1.89352477600006,11.6,-10.869583997));
#295105=CARTESIAN_POINT('Ctrl Pts',(-1.89194794100006,15.2,-10.866888627));
#295106=CARTESIAN_POINT('Ctrl Pts',(-1.89194794100006,11.6,-10.866888627));
#295107=CARTESIAN_POINT('Ctrl Pts',(-1.89037592900006,15.2,-10.8641965));
#295108=CARTESIAN_POINT('Ctrl Pts',(-1.89037592900006,11.6,-10.8641965));
#295109=CARTESIAN_POINT('Ctrl Pts',(-1.88880874000006,15.2,-10.861507626));
#295110=CARTESIAN_POINT('Ctrl Pts',(-1.88880874000006,11.6,-10.861507626));
#295111=CARTESIAN_POINT('Ctrl Pts',(-1.88724637200006,15.2,-10.858822018));
#295112=CARTESIAN_POINT('Ctrl Pts',(-1.88724637200006,11.6,-10.858822018));
#295113=CARTESIAN_POINT('Ctrl Pts',(-1.88568882100005,15.2,-10.856139687));
#295114=CARTESIAN_POINT('Ctrl Pts',(-1.88568882100005,11.6,-10.856139687));
#295115=CARTESIAN_POINT('Ctrl Pts',(-1.88413608800006,15.2,-10.853460644));
#295116=CARTESIAN_POINT('Ctrl Pts',(-1.88413608800006,11.6,-10.853460644));
#295117=CARTESIAN_POINT('Ctrl Pts',(-1.88258817100006,15.2,-10.850784903));
#295118=CARTESIAN_POINT('Ctrl Pts',(-1.88258817100006,11.6,-10.850784903));
#295119=CARTESIAN_POINT('Ctrl Pts',(-1.88104506800005,15.2,-10.848112472));
#295120=CARTESIAN_POINT('Ctrl Pts',(-1.88104506800005,11.6,-10.848112472));
#295121=CARTESIAN_POINT('Ctrl Pts',(-1.87950677700006,15.2,-10.845443365));
#295122=CARTESIAN_POINT('Ctrl Pts',(-1.87950677700006,11.6,-10.845443365));
#295123=CARTESIAN_POINT('Ctrl Pts',(-1.87797329500006,15.2,-10.842777593));
#295124=CARTESIAN_POINT('Ctrl Pts',(-1.87797329500006,11.6,-10.842777593));
#295125=CARTESIAN_POINT('Ctrl Pts',(-1.87644462200006,15.2,-10.840115167));
#295126=CARTESIAN_POINT('Ctrl Pts',(-1.87644462200006,11.6,-10.840115167));
#295127=CARTESIAN_POINT('Ctrl Pts',(-1.87492075700006,15.2,-10.837456101));
#295128=CARTESIAN_POINT('Ctrl Pts',(-1.87492075700006,11.6,-10.837456101));
#295129=CARTESIAN_POINT('Ctrl Pts',(-1.87340169600006,15.2,-10.834800405));
#295130=CARTESIAN_POINT('Ctrl Pts',(-1.87340169600006,11.6,-10.834800405));
#295131=CARTESIAN_POINT('Ctrl Pts',(-1.87188743800006,15.2,-10.832148091));
#295132=CARTESIAN_POINT('Ctrl Pts',(-1.87188743800006,11.6,-10.832148091));
#295133=CARTESIAN_POINT('Ctrl Pts',(-1.87037798200006,15.2,-10.829499171));
#295134=CARTESIAN_POINT('Ctrl Pts',(-1.87037798200006,11.6,-10.829499171));
#295135=CARTESIAN_POINT('Ctrl Pts',(-1.86887332500006,15.2,-10.826853656));
#295136=CARTESIAN_POINT('Ctrl Pts',(-1.86887332500006,11.6,-10.826853656));
#295137=CARTESIAN_POINT('Ctrl Pts',(-1.86737346700005,15.2,-10.82421156));
#295138=CARTESIAN_POINT('Ctrl Pts',(-1.86737346700005,11.6,-10.82421156));
#295139=CARTESIAN_POINT('Ctrl Pts',(-1.86587840400006,15.2,-10.821572893));
#295140=CARTESIAN_POINT('Ctrl Pts',(-1.86587840400006,11.6,-10.821572893));
#295141=CARTESIAN_POINT('Ctrl Pts',(-1.86438813500006,15.2,-10.818937666));
#295142=CARTESIAN_POINT('Ctrl Pts',(-1.86438813500006,11.6,-10.818937666));
#295143=CARTESIAN_POINT('Ctrl Pts',(-1.86290265800006,15.2,-10.816305894));
#295144=CARTESIAN_POINT('Ctrl Pts',(-1.86290265800006,11.6,-10.816305894));
#295145=CARTESIAN_POINT('Ctrl Pts',(-1.86142197200006,15.2,-10.813677586));
#295146=CARTESIAN_POINT('Ctrl Pts',(-1.86142197200006,11.6,-10.813677586));
#295147=CARTESIAN_POINT('Ctrl Pts',(-1.85994607300006,15.2,-10.811052755));
#295148=CARTESIAN_POINT('Ctrl Pts',(-1.85994607300006,11.6,-10.811052755));
#295149=CARTESIAN_POINT('Ctrl Pts',(-1.85847496200006,15.2,-10.808431414));
#295150=CARTESIAN_POINT('Ctrl Pts',(-1.85847496200006,11.6,-10.808431414));
#295151=CARTESIAN_POINT('Ctrl Pts',(-1.85700863500006,15.2,-10.805813575));
#295152=CARTESIAN_POINT('Ctrl Pts',(-1.85700863500006,11.6,-10.805813575));
#295153=CARTESIAN_POINT('Ctrl Pts',(-1.85554709100006,15.2,-10.803199248));
#295154=CARTESIAN_POINT('Ctrl Pts',(-1.85554709100006,11.6,-10.803199248));
#295155=CARTESIAN_POINT('Ctrl Pts',(-1.85409032800006,15.2,-10.800588447));
#295156=CARTESIAN_POINT('Ctrl Pts',(-1.85409032800006,11.6,-10.800588447));
#295157=CARTESIAN_POINT('Ctrl Pts',(-1.85263834300006,15.2,-10.797981184));
#295158=CARTESIAN_POINT('Ctrl Pts',(-1.85263834300006,11.6,-10.797981184));
#295159=CARTESIAN_POINT('Ctrl Pts',(-1.85119113400006,15.2,-10.795377469));
#295160=CARTESIAN_POINT('Ctrl Pts',(-1.85119113400006,11.6,-10.795377469));
#295161=CARTESIAN_POINT('Ctrl Pts',(-1.84974870200006,15.2,-10.792777317));
#295162=CARTESIAN_POINT('Ctrl Pts',(-1.84974870200006,11.6,-10.792777317));
#295163=CARTESIAN_POINT('Ctrl Pts',(-1.84831104100006,15.2,-10.790180739));
#295164=CARTESIAN_POINT('Ctrl Pts',(-1.84831104100006,11.6,-10.790180739));
#295165=CARTESIAN_POINT('Ctrl Pts',(-1.84687815100005,15.2,-10.787587746));
#295166=CARTESIAN_POINT('Ctrl Pts',(-1.84687815100005,11.6,-10.787587746));
#295167=CARTESIAN_POINT('Ctrl Pts',(-1.84545003000005,15.2,-10.784998353));
#295168=CARTESIAN_POINT('Ctrl Pts',(-1.84545003000005,11.6,-10.784998353));
#295169=CARTESIAN_POINT('Ctrl Pts',(-1.84402667500006,15.2,-10.78241257));
#295170=CARTESIAN_POINT('Ctrl Pts',(-1.84402667500006,11.6,-10.78241257));
#295171=CARTESIAN_POINT('Ctrl Pts',(-1.84260808600006,15.2,-10.77983041));
#295172=CARTESIAN_POINT('Ctrl Pts',(-1.84260808600006,11.6,-10.77983041));
#295173=CARTESIAN_POINT('Ctrl Pts',(-1.84119425800006,15.2,-10.777251885));
#295174=CARTESIAN_POINT('Ctrl Pts',(-1.84119425800006,11.6,-10.777251885));
#295175=CARTESIAN_POINT('Ctrl Pts',(-1.83978519200006,15.2,-10.774677008));
#295176=CARTESIAN_POINT('Ctrl Pts',(-1.83978519200006,11.6,-10.774677008));
#295177=CARTESIAN_POINT('Ctrl Pts',(-1.83838088300006,15.2,-10.77210579));
#295178=CARTESIAN_POINT('Ctrl Pts',(-1.83838088300006,11.6,-10.77210579));
#295179=CARTESIAN_POINT('Ctrl Pts',(-1.83698133100005,15.2,-10.769538245));
#295180=CARTESIAN_POINT('Ctrl Pts',(-1.83698133100005,11.6,-10.769538245));
#295181=CARTESIAN_POINT('Ctrl Pts',(-1.83558653300006,15.2,-10.766974386));
#295182=CARTESIAN_POINT('Ctrl Pts',(-1.83558653300006,11.6,-10.766974386));
#295183=CARTESIAN_POINT('Ctrl Pts',(-1.83419648600006,15.2,-10.764414223));
#295184=CARTESIAN_POINT('Ctrl Pts',(-1.83419648600006,11.6,-10.764414223));
#295185=CARTESIAN_POINT('Ctrl Pts',(-1.83281119000006,15.2,-10.76185777));
#295186=CARTESIAN_POINT('Ctrl Pts',(-1.83281119000006,11.6,-10.76185777));
#295187=CARTESIAN_POINT('Ctrl Pts',(-1.83143064100005,15.2,-10.759305039));
#295188=CARTESIAN_POINT('Ctrl Pts',(-1.83143064100005,11.6,-10.759305039));
#295189=CARTESIAN_POINT('Ctrl Pts',(-1.83005483700006,15.2,-10.756756043));
#295190=CARTESIAN_POINT('Ctrl Pts',(-1.83005483700006,11.6,-10.756756043));
#295191=CARTESIAN_POINT('Ctrl Pts',(-1.82868377600006,15.2,-10.754210794));
#295192=CARTESIAN_POINT('Ctrl Pts',(-1.82868377600006,11.6,-10.754210794));
#295193=CARTESIAN_POINT('Ctrl Pts',(-1.82731745700006,15.2,-10.751669306));
#295194=CARTESIAN_POINT('Ctrl Pts',(-1.82731745700006,11.6,-10.751669306));
#295195=CARTESIAN_POINT('Ctrl Pts',(-1.82595587600006,15.2,-10.749131589));
#295196=CARTESIAN_POINT('Ctrl Pts',(-1.82595587600006,11.6,-10.749131589));
#295197=CARTESIAN_POINT('Ctrl Pts',(-1.82459903200006,15.2,-10.746597658));
#295198=CARTESIAN_POINT('Ctrl Pts',(-1.82459903200006,11.6,-10.746597658));
#295199=CARTESIAN_POINT('Ctrl Pts',(-1.82324692200006,15.2,-10.744067526));
#295200=CARTESIAN_POINT('Ctrl Pts',(-1.82324692200006,11.6,-10.744067526));
#295201=CARTESIAN_POINT('Ctrl Pts',(-1.82189954400006,15.2,-10.741541203));
#295202=CARTESIAN_POINT('Ctrl Pts',(-1.82189954400006,11.6,-10.741541203));
#295203=CARTESIAN_POINT('Ctrl Pts',(-1.82055689600006,15.2,-10.739018703));
#295204=CARTESIAN_POINT('Ctrl Pts',(-1.82055689600006,11.6,-10.739018703));
#295205=CARTESIAN_POINT('Ctrl Pts',(-1.81921897500006,15.2,-10.73650004));
#295206=CARTESIAN_POINT('Ctrl Pts',(-1.81921897500006,11.6,-10.73650004));
#295207=CARTESIAN_POINT('Ctrl Pts',(-1.81788577800006,15.2,-10.733985227));
#295208=CARTESIAN_POINT('Ctrl Pts',(-1.81788577800006,11.6,-10.733985227));
#295209=CARTESIAN_POINT('Ctrl Pts',(-1.81655730500006,15.2,-10.731474274));
#295210=CARTESIAN_POINT('Ctrl Pts',(-1.81655730500006,11.6,-10.731474274));
#295211=CARTESIAN_POINT('Ctrl Pts',(-1.81523355200006,15.2,-10.728967196));
#295212=CARTESIAN_POINT('Ctrl Pts',(-1.81523355200006,11.6,-10.728967196));
#295213=CARTESIAN_POINT('Ctrl Pts',(-1.81391451700006,15.2,-10.726464005));
#295214=CARTESIAN_POINT('Ctrl Pts',(-1.81391451700006,11.6,-10.726464005));
#295215=CARTESIAN_POINT('Ctrl Pts',(-1.81260019800006,15.2,-10.723964715));
#295216=CARTESIAN_POINT('Ctrl Pts',(-1.81260019800006,11.6,-10.723964715));
#295217=CARTESIAN_POINT('Ctrl Pts',(-1.81129059100006,15.2,-10.721469338));
#295218=CARTESIAN_POINT('Ctrl Pts',(-1.81129059100006,11.6,-10.721469338));
#295219=CARTESIAN_POINT('Ctrl Pts',(-1.80998569500006,15.2,-10.718977888));
#295220=CARTESIAN_POINT('Ctrl Pts',(-1.80998569500006,11.6,-10.718977888));
#295221=CARTESIAN_POINT('Ctrl Pts',(-1.80868550800006,15.2,-10.716490376));
#295222=CARTESIAN_POINT('Ctrl Pts',(-1.80868550800006,11.6,-10.716490376));
#295223=CARTESIAN_POINT('Ctrl Pts',(-1.80739002700005,15.2,-10.714006817));
#295224=CARTESIAN_POINT('Ctrl Pts',(-1.80739002700005,11.6,-10.714006817));
#295225=CARTESIAN_POINT('Ctrl Pts',(-1.80609924900006,15.2,-10.711527223));
#295226=CARTESIAN_POINT('Ctrl Pts',(-1.80609924900006,11.6,-10.711527223));
#295227=CARTESIAN_POINT('Ctrl Pts',(-1.80481317200006,15.2,-10.709051608));
#295228=CARTESIAN_POINT('Ctrl Pts',(-1.80481317200006,11.6,-10.709051608));
#295229=CARTESIAN_POINT('Ctrl Pts',(-1.80353179300006,15.2,-10.706579983));
#295230=CARTESIAN_POINT('Ctrl Pts',(-1.80353179300006,11.6,-10.706579983));
#295231=CARTESIAN_POINT('Ctrl Pts',(-1.80225511100006,15.2,-10.704112363));
#295232=CARTESIAN_POINT('Ctrl Pts',(-1.80225511100006,11.6,-10.704112363));
#295233=CARTESIAN_POINT('Ctrl Pts',(-1.80098312100006,15.2,-10.701648762));
#295234=CARTESIAN_POINT('Ctrl Pts',(-1.80098312100006,11.6,-10.701648762));
#295235=CARTESIAN_POINT('Ctrl Pts',(-1.79971582300006,15.2,-10.699189192));
#295236=CARTESIAN_POINT('Ctrl Pts',(-1.79971582300006,11.6,-10.699189192));
#295237=CARTESIAN_POINT('Ctrl Pts',(-1.79845321300005,15.2,-10.696733666));
#295238=CARTESIAN_POINT('Ctrl Pts',(-1.79845321300005,11.6,-10.696733666));
#295239=CARTESIAN_POINT('Ctrl Pts',(-1.79719528800006,15.2,-10.694282196));
#295240=CARTESIAN_POINT('Ctrl Pts',(-1.79719528800006,11.6,-10.694282196));
#295241=CARTESIAN_POINT('Ctrl Pts',(-1.79594204700006,15.2,-10.691834799));
#295242=CARTESIAN_POINT('Ctrl Pts',(-1.79594204700006,11.6,-10.691834799));
#295243=CARTESIAN_POINT('Ctrl Pts',(-1.79469348600006,15.2,-10.689391486));
#295244=CARTESIAN_POINT('Ctrl Pts',(-1.79469348600006,11.6,-10.689391486));
#295245=CARTESIAN_POINT('Ctrl Pts',(-1.79344960300006,15.2,-10.686952269));
#295246=CARTESIAN_POINT('Ctrl Pts',(-1.79344960300006,11.6,-10.686952269));
#295247=CARTESIAN_POINT('Ctrl Pts',(-1.79221039500006,15.2,-10.684517164));
#295248=CARTESIAN_POINT('Ctrl Pts',(-1.79221039500006,11.6,-10.684517164));
#295249=CARTESIAN_POINT('Ctrl Pts',(-1.79097586000006,15.2,-10.682086183));
#295250=CARTESIAN_POINT('Ctrl Pts',(-1.79097586000006,11.6,-10.682086183));
#295251=CARTESIAN_POINT('Ctrl Pts',(-1.78974599400005,15.2,-10.67965934));
#295252=CARTESIAN_POINT('Ctrl Pts',(-1.78974599400005,11.6,-10.67965934));
#295253=CARTESIAN_POINT('Ctrl Pts',(-1.78852079600006,15.2,-10.677236648));
#295254=CARTESIAN_POINT('Ctrl Pts',(-1.78852079600006,11.6,-10.677236648));
#295255=CARTESIAN_POINT('Ctrl Pts',(-1.78730026300005,15.2,-10.674818122));
#295256=CARTESIAN_POINT('Ctrl Pts',(-1.78730026300005,11.6,-10.674818122));
#295257=CARTESIAN_POINT('Ctrl Pts',(-1.78608439100006,15.2,-10.672403774));
#295258=CARTESIAN_POINT('Ctrl Pts',(-1.78608439100006,11.6,-10.672403774));
#295259=CARTESIAN_POINT('Ctrl Pts',(-1.78487317800006,15.2,-10.669993617));
#295260=CARTESIAN_POINT('Ctrl Pts',(-1.78487317800006,11.6,-10.669993617));
#295261=CARTESIAN_POINT('Ctrl Pts',(-1.78366662300005,15.2,-10.667587667));
#295262=CARTESIAN_POINT('Ctrl Pts',(-1.78366662300005,11.6,-10.667587667));
#295263=CARTESIAN_POINT('Ctrl Pts',(-1.78246472000006,15.2,-10.665185935));
#295264=CARTESIAN_POINT('Ctrl Pts',(-1.78246472000006,11.6,-10.665185935));
#295265=CARTESIAN_POINT('Ctrl Pts',(-1.78126746700006,15.2,-10.662788437));
#295266=CARTESIAN_POINT('Ctrl Pts',(-1.78126746700006,11.6,-10.662788437));
#295267=CARTESIAN_POINT('Ctrl Pts',(-1.78007486300006,15.2,-10.660395184));
#295268=CARTESIAN_POINT('Ctrl Pts',(-1.78007486300006,11.6,-10.660395184));
#295269=CARTESIAN_POINT('Ctrl Pts',(-1.77888690400006,15.2,-10.658006194));
#295270=CARTESIAN_POINT('Ctrl Pts',(-1.77888690400006,11.6,-10.658006194));
#295271=CARTESIAN_POINT('Ctrl Pts',(-1.77770358700006,15.2,-10.655621476));
#295272=CARTESIAN_POINT('Ctrl Pts',(-1.77770358700006,11.6,-10.655621476));
#295273=CARTESIAN_POINT('Ctrl Pts',(-1.77652491000006,15.2,-10.653241047));
#295274=CARTESIAN_POINT('Ctrl Pts',(-1.77652491000006,11.6,-10.653241047));
#295275=CARTESIAN_POINT('Ctrl Pts',(-1.77535086900006,15.2,-10.65086492));
#295276=CARTESIAN_POINT('Ctrl Pts',(-1.77535086900006,11.6,-10.65086492));
#295277=CARTESIAN_POINT('Ctrl Pts',(-1.77418146100006,15.2,-10.648493108));
#295278=CARTESIAN_POINT('Ctrl Pts',(-1.77418146100006,11.6,-10.648493108));
#295279=CARTESIAN_POINT('Ctrl Pts',(-1.77301668500006,15.2,-10.646125627));
#295280=CARTESIAN_POINT('Ctrl Pts',(-1.77301668500006,11.6,-10.646125627));
#295281=CARTESIAN_POINT('Ctrl Pts',(-1.77185653500006,15.2,-10.643762488));
#295282=CARTESIAN_POINT('Ctrl Pts',(-1.77185653500006,11.6,-10.643762488));
#295283=CARTESIAN_POINT('Ctrl Pts',(-1.77070101200006,15.2,-10.641403708));
#295284=CARTESIAN_POINT('Ctrl Pts',(-1.77070101200006,11.6,-10.641403708));
#295285=CARTESIAN_POINT('Ctrl Pts',(-1.76955010900006,15.2,-10.639049299));
#295286=CARTESIAN_POINT('Ctrl Pts',(-1.76955010900006,11.6,-10.639049299));
#295287=CARTESIAN_POINT('Ctrl Pts',(-1.76840382600005,15.2,-10.636699276));
#295288=CARTESIAN_POINT('Ctrl Pts',(-1.76840382600005,11.6,-10.636699276));
#295289=CARTESIAN_POINT('Ctrl Pts',(-1.76726215900006,15.2,-10.634353653));
#295290=CARTESIAN_POINT('Ctrl Pts',(-1.76726215900006,11.6,-10.634353653));
#295291=CARTESIAN_POINT('Ctrl Pts',(-1.76612510400005,15.2,-10.632012444));
#295292=CARTESIAN_POINT('Ctrl Pts',(-1.76612510400005,11.6,-10.632012444));
#295293=CARTESIAN_POINT('Ctrl Pts',(-1.76499265900006,15.2,-10.629675663));
#295294=CARTESIAN_POINT('Ctrl Pts',(-1.76499265900006,11.6,-10.629675663));
#295295=CARTESIAN_POINT('Ctrl Pts',(-1.76386482100006,15.2,-10.627343324));
#295296=CARTESIAN_POINT('Ctrl Pts',(-1.76386482100006,11.6,-10.627343324));
#295297=CARTESIAN_POINT('Ctrl Pts',(-1.76274158600006,15.2,-10.625015442));
#295298=CARTESIAN_POINT('Ctrl Pts',(-1.76274158600006,11.6,-10.625015442));
#295299=CARTESIAN_POINT('Ctrl Pts',(-1.76162295200006,15.2,-10.622692031));
#295300=CARTESIAN_POINT('Ctrl Pts',(-1.76162295200006,11.6,-10.622692031));
#295301=CARTESIAN_POINT('Ctrl Pts',(-1.76050891600006,15.2,-10.620373104));
#295302=CARTESIAN_POINT('Ctrl Pts',(-1.76050891600006,11.6,-10.620373104));
#295303=CARTESIAN_POINT('Ctrl Pts',(-1.75939947300006,15.2,-10.618058678));
#295304=CARTESIAN_POINT('Ctrl Pts',(-1.75939947300006,11.6,-10.618058678));
#295305=CARTESIAN_POINT('Ctrl Pts',(-1.75829462200006,15.2,-10.615748764));
#295306=CARTESIAN_POINT('Ctrl Pts',(-1.75829462200006,11.6,-10.615748764));
#295307=CARTESIAN_POINT('Ctrl Pts',(-1.75719435900006,15.2,-10.61344338));
#295308=CARTESIAN_POINT('Ctrl Pts',(-1.75719435900006,11.6,-10.61344338));
#295309=CARTESIAN_POINT('Ctrl Pts',(-1.75609868000006,15.2,-10.611142538));
#295310=CARTESIAN_POINT('Ctrl Pts',(-1.75609868000006,11.6,-10.611142538));
#295311=CARTESIAN_POINT('Ctrl Pts',(-1.75500758400006,15.2,-10.608846253));
#295312=CARTESIAN_POINT('Ctrl Pts',(-1.75500758400006,11.6,-10.608846253));
#295313=CARTESIAN_POINT('Ctrl Pts',(-1.75392106600006,15.2,-10.60655454));
#295314=CARTESIAN_POINT('Ctrl Pts',(-1.75392106600006,11.6,-10.60655454));
#295315=CARTESIAN_POINT('Ctrl Pts',(-1.75283912300006,15.2,-10.604267414));
#295316=CARTESIAN_POINT('Ctrl Pts',(-1.75283912300006,11.6,-10.604267414));
#295317=CARTESIAN_POINT('Ctrl Pts',(-1.75176175100006,15.2,-10.601984888));
#295318=CARTESIAN_POINT('Ctrl Pts',(-1.75176175100006,11.6,-10.601984888));
#295319=CARTESIAN_POINT('Ctrl Pts',(-1.75068894900006,15.2,-10.599706978));
#295320=CARTESIAN_POINT('Ctrl Pts',(-1.75068894900006,11.6,-10.599706978));
#295321=CARTESIAN_POINT('Ctrl Pts',(-1.74962071200006,15.2,-10.597433698));
#295322=CARTESIAN_POINT('Ctrl Pts',(-1.74962071200006,11.6,-10.597433698));
#295323=CARTESIAN_POINT('Ctrl Pts',(-1.74855703600006,15.2,-10.595165063));
#295324=CARTESIAN_POINT('Ctrl Pts',(-1.74855703600006,11.6,-10.595165063));
#295325=CARTESIAN_POINT('Ctrl Pts',(-1.74749792000006,15.2,-10.592901087));
#295326=CARTESIAN_POINT('Ctrl Pts',(-1.74749792000006,11.6,-10.592901087));
#295327=CARTESIAN_POINT('Ctrl Pts',(-1.74644335700005,15.2,-10.590641786));
#295328=CARTESIAN_POINT('Ctrl Pts',(-1.74644335700005,11.6,-10.590641786));
#295329=CARTESIAN_POINT('Ctrl Pts',(-1.74539334800006,15.2,-10.588387175));
#295330=CARTESIAN_POINT('Ctrl Pts',(-1.74539334800006,11.6,-10.588387175));
#295331=CARTESIAN_POINT('Ctrl Pts',(-1.74434788700006,15.2,-10.586137267));
#295332=CARTESIAN_POINT('Ctrl Pts',(-1.74434788700006,11.6,-10.586137267));
#295333=CARTESIAN_POINT('Ctrl Pts',(-1.74330697100005,15.2,-10.58389208));
#295334=CARTESIAN_POINT('Ctrl Pts',(-1.74330697100005,11.6,-10.58389208));
#295335=CARTESIAN_POINT('Ctrl Pts',(-1.74227059600006,15.2,-10.581651626));
#295336=CARTESIAN_POINT('Ctrl Pts',(-1.74227059600006,11.6,-10.581651626));
#295337=CARTESIAN_POINT('Ctrl Pts',(-1.74123875900006,15.2,-10.57941592));
#295338=CARTESIAN_POINT('Ctrl Pts',(-1.74123875900006,11.6,-10.57941592));
#295339=CARTESIAN_POINT('Ctrl Pts',(-1.74021145800005,15.2,-10.577184979));
#295340=CARTESIAN_POINT('Ctrl Pts',(-1.74021145800005,11.6,-10.577184979));
#295341=CARTESIAN_POINT('Ctrl Pts',(-1.73918868600006,15.2,-10.574958817));
#295342=CARTESIAN_POINT('Ctrl Pts',(-1.73918868600006,11.6,-10.574958817));
#295343=CARTESIAN_POINT('Ctrl Pts',(-1.73817044300006,15.2,-10.572737449));
#295344=CARTESIAN_POINT('Ctrl Pts',(-1.73817044300006,11.6,-10.572737449));
#295345=CARTESIAN_POINT('Ctrl Pts',(-1.73715672500005,15.2,-10.570520891));
#295346=CARTESIAN_POINT('Ctrl Pts',(-1.73715672500005,11.6,-10.570520891));
#295347=CARTESIAN_POINT('Ctrl Pts',(-1.73614752700006,15.2,-10.568309157));
#295348=CARTESIAN_POINT('Ctrl Pts',(-1.73614752700006,11.6,-10.568309157));
#295349=CARTESIAN_POINT('Ctrl Pts',(-1.73514284500006,15.2,-10.566102263));
#295350=CARTESIAN_POINT('Ctrl Pts',(-1.73514284500006,11.6,-10.566102263));
#295351=CARTESIAN_POINT('Ctrl Pts',(-1.73414267600006,15.2,-10.563900224));
#295352=CARTESIAN_POINT('Ctrl Pts',(-1.73414267600006,11.6,-10.563900224));
#295353=CARTESIAN_POINT('Ctrl Pts',(-1.73314701900006,15.2,-10.561703056));
#295354=CARTESIAN_POINT('Ctrl Pts',(-1.73314701900006,11.6,-10.561703056));
#295355=CARTESIAN_POINT('Ctrl Pts',(-1.73215586600006,15.2,-10.559510773));
#295356=CARTESIAN_POINT('Ctrl Pts',(-1.73215586600006,11.6,-10.559510773));
#295357=CARTESIAN_POINT('Ctrl Pts',(-1.73116921600006,15.2,-10.55732339));
#295358=CARTESIAN_POINT('Ctrl Pts',(-1.73116921600006,11.6,-10.55732339));
#295359=CARTESIAN_POINT('Ctrl Pts',(-1.73018706500006,15.2,-10.555140925));
#295360=CARTESIAN_POINT('Ctrl Pts',(-1.73018706500006,11.6,-10.555140925));
#295361=CARTESIAN_POINT('Ctrl Pts',(-1.72920940800006,15.2,-10.552963391));
#295362=CARTESIAN_POINT('Ctrl Pts',(-1.72920940800006,11.6,-10.552963391));
#295363=CARTESIAN_POINT('Ctrl Pts',(-1.72823624300006,15.2,-10.550790805));
#295364=CARTESIAN_POINT('Ctrl Pts',(-1.72823624300006,11.6,-10.550790805));
#295365=CARTESIAN_POINT('Ctrl Pts',(-1.72726756600006,15.2,-10.548623183));
#295366=CARTESIAN_POINT('Ctrl Pts',(-1.72726756600006,11.6,-10.548623183));
#295367=CARTESIAN_POINT('Ctrl Pts',(-1.72630337200005,15.2,-10.546460538));
#295368=CARTESIAN_POINT('Ctrl Pts',(-1.72630337200005,11.6,-10.546460538));
#295369=CARTESIAN_POINT('Ctrl Pts',(-1.72534365800006,15.2,-10.544302889));
#295370=CARTESIAN_POINT('Ctrl Pts',(-1.72534365800006,11.6,-10.544302889));
#295371=CARTESIAN_POINT('Ctrl Pts',(-1.72438842000005,15.2,-10.542150249));
#295372=CARTESIAN_POINT('Ctrl Pts',(-1.72438842000005,11.6,-10.542150249));
#295373=CARTESIAN_POINT('Ctrl Pts',(-1.72343765400006,15.2,-10.540002635));
#295374=CARTESIAN_POINT('Ctrl Pts',(-1.72343765400006,11.6,-10.540002635));
#295375=CARTESIAN_POINT('Ctrl Pts',(-1.72249135800006,15.2,-10.537860062));
#295376=CARTESIAN_POINT('Ctrl Pts',(-1.72249135800006,11.6,-10.537860062));
#295377=CARTESIAN_POINT('Ctrl Pts',(-1.72154952600006,15.2,-10.535722547));
#295378=CARTESIAN_POINT('Ctrl Pts',(-1.72154952600006,11.6,-10.535722547));
#295379=CARTESIAN_POINT('Ctrl Pts',(-1.72061215300006,15.2,-10.533590105));
#295380=CARTESIAN_POINT('Ctrl Pts',(-1.72061215300006,11.6,-10.533590105));
#295381=CARTESIAN_POINT('Ctrl Pts',(-1.71967923800006,15.2,-10.531462752));
#295382=CARTESIAN_POINT('Ctrl Pts',(-1.71967923800006,11.6,-10.531462752));
#295383=CARTESIAN_POINT('Ctrl Pts',(-1.71875077600005,15.2,-10.529340504));
#295384=CARTESIAN_POINT('Ctrl Pts',(-1.71875077600005,11.6,-10.529340504));
#295385=CARTESIAN_POINT('Ctrl Pts',(-1.71782676200006,15.2,-10.527223376));
#295386=CARTESIAN_POINT('Ctrl Pts',(-1.71782676200006,11.6,-10.527223376));
#295387=CARTESIAN_POINT('Ctrl Pts',(-1.71690719200006,15.2,-10.525111386));
#295388=CARTESIAN_POINT('Ctrl Pts',(-1.71690719200006,11.6,-10.525111386));
#295389=CARTESIAN_POINT('Ctrl Pts',(-1.71599206400006,15.2,-10.523004549));
#295390=CARTESIAN_POINT('Ctrl Pts',(-1.71599206400006,11.6,-10.523004549));
#295391=CARTESIAN_POINT('Ctrl Pts',(-1.71508137200005,15.2,-10.520902882));
#295392=CARTESIAN_POINT('Ctrl Pts',(-1.71508137200005,11.6,-10.520902882));
#295393=CARTESIAN_POINT('Ctrl Pts',(-1.71417511300006,15.2,-10.5188064));
#295394=CARTESIAN_POINT('Ctrl Pts',(-1.71417511300006,11.6,-10.5188064));
#295395=CARTESIAN_POINT('Ctrl Pts',(-1.71327328300006,15.2,-10.516715119));
#295396=CARTESIAN_POINT('Ctrl Pts',(-1.71327328300006,11.6,-10.516715119));
#295397=CARTESIAN_POINT('Ctrl Pts',(-1.71237587800006,15.2,-10.514629056));
#295398=CARTESIAN_POINT('Ctrl Pts',(-1.71237587800006,11.6,-10.514629056));
#295399=CARTESIAN_POINT('Ctrl Pts',(-1.71148289100006,15.2,-10.512548228));
#295400=CARTESIAN_POINT('Ctrl Pts',(-1.71148289100006,11.6,-10.512548228));
#295401=CARTESIAN_POINT('Ctrl Pts',(-1.71059432200006,15.2,-10.510472651));
#295402=CARTESIAN_POINT('Ctrl Pts',(-1.71059432200006,11.6,-10.510472651));
#295403=CARTESIAN_POINT('Ctrl Pts',(-1.70971016400005,15.2,-10.50840234));
#295404=CARTESIAN_POINT('Ctrl Pts',(-1.70971016400005,11.6,-10.50840234));
#295405=CARTESIAN_POINT('Ctrl Pts',(-1.70883041500006,15.2,-10.506337312));
#295406=CARTESIAN_POINT('Ctrl Pts',(-1.70883041500006,11.6,-10.506337312));
#295407=CARTESIAN_POINT('Ctrl Pts',(-1.70795506800005,15.2,-10.504277584));
#295408=CARTESIAN_POINT('Ctrl Pts',(-1.70795506800005,11.6,-10.504277584));
#295409=CARTESIAN_POINT('Ctrl Pts',(-1.70708412100006,15.2,-10.502223174));
#295410=CARTESIAN_POINT('Ctrl Pts',(-1.70708412100006,11.6,-10.502223174));
#295411=CARTESIAN_POINT('Ctrl Pts',(-1.70621756900006,15.2,-10.500174096));
#295412=CARTESIAN_POINT('Ctrl Pts',(-1.70621756900006,11.6,-10.500174096));
#295413=CARTESIAN_POINT('Ctrl Pts',(-1.70535540700006,15.2,-10.498130368));
#295414=CARTESIAN_POINT('Ctrl Pts',(-1.70535540700006,11.6,-10.498130368));
#295415=CARTESIAN_POINT('Ctrl Pts',(-1.70449763200006,15.2,-10.496092006));
#295416=CARTESIAN_POINT('Ctrl Pts',(-1.70449763200006,11.6,-10.496092006));
#295417=CARTESIAN_POINT('Ctrl Pts',(-1.70364423900006,15.2,-10.494059027));
#295418=CARTESIAN_POINT('Ctrl Pts',(-1.70364423900006,11.6,-10.494059027));
#295419=CARTESIAN_POINT('Ctrl Pts',(-1.70279522300006,15.2,-10.492031449));
#295420=CARTESIAN_POINT('Ctrl Pts',(-1.70279522300006,11.6,-10.492031449));
#295421=CARTESIAN_POINT('Ctrl Pts',(-1.70195058100005,15.2,-10.490009287));
#295422=CARTESIAN_POINT('Ctrl Pts',(-1.70195058100005,11.6,-10.490009287));
#295423=CARTESIAN_POINT('Ctrl Pts',(-1.70111030700005,15.2,-10.487992559));
#295424=CARTESIAN_POINT('Ctrl Pts',(-1.70111030700005,11.6,-10.487992559));
#295425=CARTESIAN_POINT('Ctrl Pts',(-1.70027439800006,15.2,-10.485981281));
#295426=CARTESIAN_POINT('Ctrl Pts',(-1.70027439800006,11.6,-10.485981281));
#295427=CARTESIAN_POINT('Ctrl Pts',(-1.69944284900006,15.2,-10.483975472));
#295428=CARTESIAN_POINT('Ctrl Pts',(-1.69944284900006,11.6,-10.483975472));
#295429=CARTESIAN_POINT('Ctrl Pts',(-1.69861565500006,15.2,-10.481975146));
#295430=CARTESIAN_POINT('Ctrl Pts',(-1.69861565500006,11.6,-10.481975146));
#295431=CARTESIAN_POINT('Ctrl Pts',(-1.69779281100006,15.2,-10.479980323));
#295432=CARTESIAN_POINT('Ctrl Pts',(-1.69779281100006,11.6,-10.479980323));
#295433=CARTESIAN_POINT('Ctrl Pts',(-1.69697431500006,15.2,-10.477991019));
#295434=CARTESIAN_POINT('Ctrl Pts',(-1.69697431500006,11.6,-10.477991019));
#295435=CARTESIAN_POINT('Ctrl Pts',(-1.69616015900006,15.2,-10.476007249));
#295436=CARTESIAN_POINT('Ctrl Pts',(-1.69616015900006,11.6,-10.476007249));
#295437=CARTESIAN_POINT('Ctrl Pts',(-1.69535034100006,15.2,-10.474029034));
#295438=CARTESIAN_POINT('Ctrl Pts',(-1.69535034100006,11.6,-10.474029034));
#295439=CARTESIAN_POINT('Ctrl Pts',(-1.69454485500005,15.2,-10.47205639));
#295440=CARTESIAN_POINT('Ctrl Pts',(-1.69454485500005,11.6,-10.47205639));
#295441=CARTESIAN_POINT('Ctrl Pts',(-1.69374369700006,15.2,-10.470089332));
#295442=CARTESIAN_POINT('Ctrl Pts',(-1.69374369700006,11.6,-10.470089332));
#295443=CARTESIAN_POINT('Ctrl Pts',(-1.69294686200006,15.2,-10.468127881));
#295444=CARTESIAN_POINT('Ctrl Pts',(-1.69294686200006,11.6,-10.468127881));
#295445=CARTESIAN_POINT('Ctrl Pts',(-1.69215434600006,15.2,-10.466172052));
#295446=CARTESIAN_POINT('Ctrl Pts',(-1.69215434600006,11.6,-10.466172052));
#295447=CARTESIAN_POINT('Ctrl Pts',(-1.69136614300006,15.2,-10.464221864));
#295448=CARTESIAN_POINT('Ctrl Pts',(-1.69136614300006,11.6,-10.464221864));
#295449=CARTESIAN_POINT('Ctrl Pts',(-1.69058224900006,15.2,-10.462277333));
#295450=CARTESIAN_POINT('Ctrl Pts',(-1.69058224900006,11.6,-10.462277333));
#295451=CARTESIAN_POINT('Ctrl Pts',(-1.68980265900006,15.2,-10.460338479));
#295452=CARTESIAN_POINT('Ctrl Pts',(-1.68980265900006,11.6,-10.460338479));
#295453=CARTESIAN_POINT('Ctrl Pts',(-1.68902736900006,15.2,-10.458405316));
#295454=CARTESIAN_POINT('Ctrl Pts',(-1.68902736900006,11.6,-10.458405316));
#295455=CARTESIAN_POINT('Ctrl Pts',(-1.68825637300006,15.2,-10.456477865));
#295456=CARTESIAN_POINT('Ctrl Pts',(-1.68825637300006,11.6,-10.456477865));
#295457=CARTESIAN_POINT('Ctrl Pts',(-1.68748966700006,15.2,-10.454556142));
#295458=CARTESIAN_POINT('Ctrl Pts',(-1.68748966700006,11.6,-10.454556142));
#295459=CARTESIAN_POINT('Ctrl Pts',(-1.68672724500006,15.2,-10.452640166));
#295460=CARTESIAN_POINT('Ctrl Pts',(-1.68672724500006,11.6,-10.452640166));
#295461=CARTESIAN_POINT('Ctrl Pts',(-1.68596910300006,15.2,-10.450729954));
#295462=CARTESIAN_POINT('Ctrl Pts',(-1.68596910300006,11.6,-10.450729954));
#295463=CARTESIAN_POINT('Ctrl Pts',(-1.68521523600006,15.2,-10.448825525));
#295464=CARTESIAN_POINT('Ctrl Pts',(-1.68521523600006,11.6,-10.448825525));
#295465=CARTESIAN_POINT('Ctrl Pts',(-1.68446563900006,15.2,-10.446926896));
#295466=CARTESIAN_POINT('Ctrl Pts',(-1.68446563900006,11.6,-10.446926896));
#295467=CARTESIAN_POINT('Ctrl Pts',(-1.68372030600006,15.2,-10.445034085));
#295468=CARTESIAN_POINT('Ctrl Pts',(-1.68372030600006,11.6,-10.445034085));
#295469=CARTESIAN_POINT('Ctrl Pts',(-1.68297923400006,15.2,-10.44314711));
#295470=CARTESIAN_POINT('Ctrl Pts',(-1.68297923400006,11.6,-10.44314711));
#295471=CARTESIAN_POINT('Ctrl Pts',(-1.68224241500006,15.2,-10.44126599));
#295472=CARTESIAN_POINT('Ctrl Pts',(-1.68224241500006,11.6,-10.44126599));
#295473=CARTESIAN_POINT('Ctrl Pts',(-1.68150984700006,15.2,-10.439390743));
#295474=CARTESIAN_POINT('Ctrl Pts',(-1.68150984700006,11.6,-10.439390743));
#295475=CARTESIAN_POINT('Ctrl Pts',(-1.68078152300006,15.2,-10.437521386));
#295476=CARTESIAN_POINT('Ctrl Pts',(-1.68078152300006,11.6,-10.437521386));
#295477=CARTESIAN_POINT('Ctrl Pts',(-1.68005743900005,15.2,-10.435657939));
#295478=CARTESIAN_POINT('Ctrl Pts',(-1.68005743900005,11.6,-10.435657939));
#295479=CARTESIAN_POINT('Ctrl Pts',(-1.67933758800005,15.2,-10.433800421));
#295480=CARTESIAN_POINT('Ctrl Pts',(-1.67933758800005,11.6,-10.433800421));
#295481=CARTESIAN_POINT('Ctrl Pts',(-1.67862196700006,15.2,-10.431948849));
#295482=CARTESIAN_POINT('Ctrl Pts',(-1.67862196700006,11.6,-10.431948849));
#295483=CARTESIAN_POINT('Ctrl Pts',(-1.67791057000006,15.2,-10.430103241));
#295484=CARTESIAN_POINT('Ctrl Pts',(-1.67791057000006,11.6,-10.430103241));
#295485=CARTESIAN_POINT('Ctrl Pts',(-1.67720339000006,15.2,-10.428263616));
#295486=CARTESIAN_POINT('Ctrl Pts',(-1.67720339000006,11.6,-10.428263616));
#295487=CARTESIAN_POINT('Ctrl Pts',(-1.67650042400005,15.2,-10.426429993));
#295488=CARTESIAN_POINT('Ctrl Pts',(-1.67650042400005,11.6,-10.426429993));
#295489=CARTESIAN_POINT('Ctrl Pts',(-1.67580166700006,15.2,-10.424602391));
#295490=CARTESIAN_POINT('Ctrl Pts',(-1.67580166700006,11.6,-10.424602391));
#295491=CARTESIAN_POINT('Ctrl Pts',(-1.67510711100005,15.2,-10.422780829));
#295492=CARTESIAN_POINT('Ctrl Pts',(-1.67510711100005,11.6,-10.422780829));
#295493=CARTESIAN_POINT('Ctrl Pts',(-1.67441675200006,15.2,-10.420965325));
#295494=CARTESIAN_POINT('Ctrl Pts',(-1.67441675200006,11.6,-10.420965325));
#295495=CARTESIAN_POINT('Ctrl Pts',(-1.67373058500006,15.2,-10.419155897));
#295496=CARTESIAN_POINT('Ctrl Pts',(-1.67373058500006,11.6,-10.419155897));
#295497=CARTESIAN_POINT('Ctrl Pts',(-1.67304860500006,15.2,-10.417352566));
#295498=CARTESIAN_POINT('Ctrl Pts',(-1.67304860500006,11.6,-10.417352566));
#295499=CARTESIAN_POINT('Ctrl Pts',(-1.67237080500006,15.2,-10.41555535));
#295500=CARTESIAN_POINT('Ctrl Pts',(-1.67237080500006,11.6,-10.41555535));
#295501=CARTESIAN_POINT('Ctrl Pts',(-1.67169718000005,15.2,-10.413764268));
#295502=CARTESIAN_POINT('Ctrl Pts',(-1.67169718000005,11.6,-10.413764268));
#295503=CARTESIAN_POINT('Ctrl Pts',(-1.67102772500006,15.2,-10.411979339));
#295504=CARTESIAN_POINT('Ctrl Pts',(-1.67102772500006,11.6,-10.411979339));
#295505=CARTESIAN_POINT('Ctrl Pts',(-1.67036243400006,15.2,-10.410200583));
#295506=CARTESIAN_POINT('Ctrl Pts',(-1.67036243400006,11.6,-10.410200583));
#295507=CARTESIAN_POINT('Ctrl Pts',(-1.66970130200006,15.2,-10.408428019));
#295508=CARTESIAN_POINT('Ctrl Pts',(-1.66970130200006,11.6,-10.408428019));
#295509=CARTESIAN_POINT('Ctrl Pts',(-1.66904432300006,15.2,-10.406661664));
#295510=CARTESIAN_POINT('Ctrl Pts',(-1.66904432300006,11.6,-10.406661664));
#295511=CARTESIAN_POINT('Ctrl Pts',(-1.66839149100006,15.2,-10.404901541));
#295512=CARTESIAN_POINT('Ctrl Pts',(-1.66839149100006,11.6,-10.404901541));
#295513=CARTESIAN_POINT('Ctrl Pts',(-1.66774280000005,15.2,-10.403147668));
#295514=CARTESIAN_POINT('Ctrl Pts',(-1.66774280000005,11.6,-10.403147668));
#295515=CARTESIAN_POINT('Ctrl Pts',(-1.66709824500006,15.2,-10.401400063));
#295516=CARTESIAN_POINT('Ctrl Pts',(-1.66709824500006,11.6,-10.401400063));
#295517=CARTESIAN_POINT('Ctrl Pts',(-1.66645782000006,15.2,-10.399658748));
#295518=CARTESIAN_POINT('Ctrl Pts',(-1.66645782000006,11.6,-10.399658748));
#295519=CARTESIAN_POINT('Ctrl Pts',(-1.66582152000006,15.2,-10.397923741));
#295520=CARTESIAN_POINT('Ctrl Pts',(-1.66582152000006,11.6,-10.397923741));
#295521=CARTESIAN_POINT('Ctrl Pts',(-1.66518933800006,15.2,-10.396195062));
#295522=CARTESIAN_POINT('Ctrl Pts',(-1.66518933800006,11.6,-10.396195062));
#295523=CARTESIAN_POINT('Ctrl Pts',(-1.66456126800006,15.2,-10.394472732));
#295524=CARTESIAN_POINT('Ctrl Pts',(-1.66456126800006,11.6,-10.394472732));
#295525=CARTESIAN_POINT('Ctrl Pts',(-1.66393730600006,15.2,-10.392756769));
#295526=CARTESIAN_POINT('Ctrl Pts',(-1.66393730600006,11.6,-10.392756769));
#295527=CARTESIAN_POINT('Ctrl Pts',(-1.66331744300006,15.2,-10.391047193));
#295528=CARTESIAN_POINT('Ctrl Pts',(-1.66331744300006,11.6,-10.391047193));
#295529=CARTESIAN_POINT('Ctrl Pts',(-1.66270167700006,15.2,-10.389344026));
#295530=CARTESIAN_POINT('Ctrl Pts',(-1.66270167700006,11.6,-10.389344026));
#295531=CARTESIAN_POINT('Ctrl Pts',(-1.66208999800005,15.2,-10.387647286));
#295532=CARTESIAN_POINT('Ctrl Pts',(-1.66208999800005,11.6,-10.387647286));
#295533=CARTESIAN_POINT('Ctrl Pts',(-1.66148240300006,15.2,-10.385956994));
#295534=CARTESIAN_POINT('Ctrl Pts',(-1.66148240300006,11.6,-10.385956994));
#295535=CARTESIAN_POINT('Ctrl Pts',(-1.66087888400006,15.2,-10.38427317));
#295536=CARTESIAN_POINT('Ctrl Pts',(-1.66087888400006,11.6,-10.38427317));
#295537=CARTESIAN_POINT('Ctrl Pts',(-1.66027943500006,15.2,-10.382595835));
#295538=CARTESIAN_POINT('Ctrl Pts',(-1.66027943500006,11.6,-10.382595835));
#295539=CARTESIAN_POINT('Ctrl Pts',(-1.65968405200006,15.2,-10.380925008));
#295540=CARTESIAN_POINT('Ctrl Pts',(-1.65968405200006,11.6,-10.380925008));
#295541=CARTESIAN_POINT('Ctrl Pts',(-1.65909272600006,15.2,-10.37926071));
#295542=CARTESIAN_POINT('Ctrl Pts',(-1.65909272600006,11.6,-10.37926071));
#295543=CARTESIAN_POINT('Ctrl Pts',(-1.65850545200006,15.2,-10.377602961));
#295544=CARTESIAN_POINT('Ctrl Pts',(-1.65850545200006,11.6,-10.377602961));
#295545=CARTESIAN_POINT('Ctrl Pts',(-1.65792222600006,15.2,-10.375951783));
#295546=CARTESIAN_POINT('Ctrl Pts',(-1.65792222600006,11.6,-10.375951783));
#295547=CARTESIAN_POINT('Ctrl Pts',(-1.65734303700006,15.2,-10.374307195));
#295548=CARTESIAN_POINT('Ctrl Pts',(-1.65734303700006,11.6,-10.374307195));
#295549=CARTESIAN_POINT('Ctrl Pts',(-1.65676788300006,15.2,-10.372669218));
#295550=CARTESIAN_POINT('Ctrl Pts',(-1.65676788300006,11.6,-10.372669218));
#295551=CARTESIAN_POINT('Ctrl Pts',(-1.65619675600006,15.2,-10.371037873));
#295552=CARTESIAN_POINT('Ctrl Pts',(-1.65619675600006,11.6,-10.371037873));
#295553=CARTESIAN_POINT('Ctrl Pts',(-1.65562964900006,15.2,-10.369413181));
#295554=CARTESIAN_POINT('Ctrl Pts',(-1.65562964900006,11.6,-10.369413181));
#295555=CARTESIAN_POINT('Ctrl Pts',(-1.65506655700006,15.2,-10.367795164));
#295556=CARTESIAN_POINT('Ctrl Pts',(-1.65506655700006,11.6,-10.367795164));
#295557=CARTESIAN_POINT('Ctrl Pts',(-1.65450747200006,15.2,-10.36618384));
#295558=CARTESIAN_POINT('Ctrl Pts',(-1.65450747200006,11.6,-10.36618384));
#295559=CARTESIAN_POINT('Ctrl Pts',(-1.65395238800006,15.2,-10.364579233));
#295560=CARTESIAN_POINT('Ctrl Pts',(-1.65395238800006,11.6,-10.364579233));
#295561=CARTESIAN_POINT('Ctrl Pts',(-1.65340130000006,15.2,-10.362981362));
#295562=CARTESIAN_POINT('Ctrl Pts',(-1.65340130000006,11.6,-10.362981362));
#295563=CARTESIAN_POINT('Ctrl Pts',(-1.65285419900006,15.2,-10.361390249));
#295564=CARTESIAN_POINT('Ctrl Pts',(-1.65285419900006,11.6,-10.361390249));
#295565=CARTESIAN_POINT('Ctrl Pts',(-1.65231108000006,15.2,-10.359805917));
#295566=CARTESIAN_POINT('Ctrl Pts',(-1.65231108000006,11.6,-10.359805917));
#295567=CARTESIAN_POINT('Ctrl Pts',(-1.65177193600006,15.2,-10.358228384));
#295568=CARTESIAN_POINT('Ctrl Pts',(-1.65177193600006,11.6,-10.358228384));
#295569=CARTESIAN_POINT('Ctrl Pts',(-1.65123676100006,15.2,-10.356657674));
#295570=CARTESIAN_POINT('Ctrl Pts',(-1.65123676100006,11.6,-10.356657674));
#295571=CARTESIAN_POINT('Ctrl Pts',(-1.65070554700006,15.2,-10.355093807));
#295572=CARTESIAN_POINT('Ctrl Pts',(-1.65070554700006,11.6,-10.355093807));
#295573=CARTESIAN_POINT('Ctrl Pts',(-1.65017828800006,15.2,-10.353536807));
#295574=CARTESIAN_POINT('Ctrl Pts',(-1.65017828800006,11.6,-10.353536807));
#295575=CARTESIAN_POINT('Ctrl Pts',(-1.64965497700006,15.2,-10.351986691));
#295576=CARTESIAN_POINT('Ctrl Pts',(-1.64965497700006,11.6,-10.351986691));
#295577=CARTESIAN_POINT('Ctrl Pts',(-1.64913560800006,15.2,-10.350443486));
#295578=CARTESIAN_POINT('Ctrl Pts',(-1.64913560800006,11.6,-10.350443486));
#295579=CARTESIAN_POINT('Ctrl Pts',(-1.64862017200006,15.2,-10.348907211));
#295580=CARTESIAN_POINT('Ctrl Pts',(-1.64862017200006,11.6,-10.348907211));
#295581=CARTESIAN_POINT('Ctrl Pts',(-1.64810866500006,15.2,-10.347377888));
#295582=CARTESIAN_POINT('Ctrl Pts',(-1.64810866500006,11.6,-10.347377888));
#295583=CARTESIAN_POINT('Ctrl Pts',(-1.64760107800005,15.2,-10.34585554));
#295584=CARTESIAN_POINT('Ctrl Pts',(-1.64760107800005,11.6,-10.34585554));
#295585=CARTESIAN_POINT('Ctrl Pts',(-1.64709740400005,15.2,-10.344340188));
#295586=CARTESIAN_POINT('Ctrl Pts',(-1.64709740400005,11.6,-10.344340188));
#295587=CARTESIAN_POINT('Ctrl Pts',(-1.64659763700006,15.2,-10.342831854));
#295588=CARTESIAN_POINT('Ctrl Pts',(-1.64659763700006,11.6,-10.342831854));
#295589=CARTESIAN_POINT('Ctrl Pts',(-1.64610177000006,15.2,-10.341330563));
#295590=CARTESIAN_POINT('Ctrl Pts',(-1.64610177000006,11.6,-10.341330563));
#295591=CARTESIAN_POINT('Ctrl Pts',(-1.64560979500005,15.2,-10.339836333));
#295592=CARTESIAN_POINT('Ctrl Pts',(-1.64560979500005,11.6,-10.339836333));
#295593=CARTESIAN_POINT('Ctrl Pts',(-1.64512170500006,15.2,-10.33834919));
#295594=CARTESIAN_POINT('Ctrl Pts',(-1.64512170500006,11.6,-10.33834919));
#295595=CARTESIAN_POINT('Ctrl Pts',(-1.64463749400006,15.2,-10.336869154));
#295596=CARTESIAN_POINT('Ctrl Pts',(-1.64463749400006,11.6,-10.336869154));
#295597=CARTESIAN_POINT('Ctrl Pts',(-1.64415715300006,15.2,-10.33539625));
#295598=CARTESIAN_POINT('Ctrl Pts',(-1.64415715300006,11.6,-10.33539625));
#295599=CARTESIAN_POINT('Ctrl Pts',(-1.64368067600006,15.2,-10.333930498));
#295600=CARTESIAN_POINT('Ctrl Pts',(-1.64368067600006,11.6,-10.333930498));
#295601=CARTESIAN_POINT('Ctrl Pts',(-1.64320805500005,15.2,-10.332471923));
#295602=CARTESIAN_POINT('Ctrl Pts',(-1.64320805500005,11.6,-10.332471923));
#295603=CARTESIAN_POINT('Ctrl Pts',(-1.64273928400006,15.2,-10.331020547));
#295604=CARTESIAN_POINT('Ctrl Pts',(-1.64273928400006,11.6,-10.331020547));
#295605=CARTESIAN_POINT('Ctrl Pts',(-1.64227435300006,15.2,-10.329576392));
#295606=CARTESIAN_POINT('Ctrl Pts',(-1.64227435300006,11.6,-10.329576392));
#295607=CARTESIAN_POINT('Ctrl Pts',(-1.64181325800006,15.2,-10.328139482));
#295608=CARTESIAN_POINT('Ctrl Pts',(-1.64181325800006,11.6,-10.328139482));
#295609=CARTESIAN_POINT('Ctrl Pts',(-1.64135598800006,15.2,-10.32670984));
#295610=CARTESIAN_POINT('Ctrl Pts',(-1.64135598800006,11.6,-10.32670984));
#295611=CARTESIAN_POINT('Ctrl Pts',(-1.64090253900006,15.2,-10.325287489));
#295612=CARTESIAN_POINT('Ctrl Pts',(-1.64090253900006,11.6,-10.325287489));
#295613=CARTESIAN_POINT('Ctrl Pts',(-1.64045290000006,15.2,-10.323872454));
#295614=CARTESIAN_POINT('Ctrl Pts',(-1.64045290000006,11.6,-10.323872454));
#295615=CARTESIAN_POINT('Ctrl Pts',(-1.64000706600006,15.2,-10.322464755));
#295616=CARTESIAN_POINT('Ctrl Pts',(-1.64000706600006,11.6,-10.322464755));
#295617=CARTESIAN_POINT('Ctrl Pts',(-1.63956502700006,15.2,-10.321064418));
#295618=CARTESIAN_POINT('Ctrl Pts',(-1.63956502700006,11.6,-10.321064418));
#295619=CARTESIAN_POINT('Ctrl Pts',(-1.63912677800006,15.2,-10.319671466));
#295620=CARTESIAN_POINT('Ctrl Pts',(-1.63912677800006,11.6,-10.319671466));
#295621=CARTESIAN_POINT('Ctrl Pts',(-1.63869231000006,15.2,-10.318285921));
#295622=CARTESIAN_POINT('Ctrl Pts',(-1.63869231000006,11.6,-10.318285921));
#295623=CARTESIAN_POINT('Ctrl Pts',(-1.63826161500006,15.2,-10.316907809));
#295624=CARTESIAN_POINT('Ctrl Pts',(-1.63826161500006,11.6,-10.316907809));
#295625=CARTESIAN_POINT('Ctrl Pts',(-1.63783468500006,15.2,-10.315537154));
#295626=CARTESIAN_POINT('Ctrl Pts',(-1.63783468500006,11.6,-10.315537154));
#295627=CARTESIAN_POINT('Ctrl Pts',(-1.63741151300006,15.2,-10.314173978));
#295628=CARTESIAN_POINT('Ctrl Pts',(-1.63741151300006,11.6,-10.314173978));
#295629=CARTESIAN_POINT('Ctrl Pts',(-1.63699208900006,15.2,-10.312818307));
#295630=CARTESIAN_POINT('Ctrl Pts',(-1.63699208900006,11.6,-10.312818307));
#295631=CARTESIAN_POINT('Ctrl Pts',(-1.63657640900006,15.2,-10.311470164));
#295632=CARTESIAN_POINT('Ctrl Pts',(-1.63657640900006,11.6,-10.311470164));
#295633=CARTESIAN_POINT('Ctrl Pts',(-1.63616446000006,15.2,-10.310129573));
#295634=CARTESIAN_POINT('Ctrl Pts',(-1.63616446000006,11.6,-10.310129573));
#295635=CARTESIAN_POINT('Ctrl Pts',(-1.63575623900006,15.2,-10.308796558));
#295636=CARTESIAN_POINT('Ctrl Pts',(-1.63575623900006,11.6,-10.308796558));
#295637=CARTESIAN_POINT('Ctrl Pts',(-1.63535173400006,15.2,-10.307471145));
#295638=CARTESIAN_POINT('Ctrl Pts',(-1.63535173400006,11.6,-10.307471145));
#295639=CARTESIAN_POINT('Ctrl Pts',(-1.63495093900006,15.2,-10.306153358));
#295640=CARTESIAN_POINT('Ctrl Pts',(-1.63495093900006,11.6,-10.306153358));
#295641=CARTESIAN_POINT('Ctrl Pts',(-1.63455384500006,15.2,-10.30484322));
#295642=CARTESIAN_POINT('Ctrl Pts',(-1.63455384500006,11.6,-10.30484322));
#295643=CARTESIAN_POINT('Ctrl Pts',(-1.63416044300006,15.2,-10.303540757));
#295644=CARTESIAN_POINT('Ctrl Pts',(-1.63416044300006,11.6,-10.303540757));
#295645=CARTESIAN_POINT('Ctrl Pts',(-1.63377072600006,15.2,-10.302245994));
#295646=CARTESIAN_POINT('Ctrl Pts',(-1.63377072600006,11.6,-10.302245994));
#295647=CARTESIAN_POINT('Ctrl Pts',(-1.63338468600006,15.2,-10.300958957));
#295648=CARTESIAN_POINT('Ctrl Pts',(-1.63338468600006,11.6,-10.300958957));
#295649=CARTESIAN_POINT('Ctrl Pts',(-1.63300231200005,15.2,-10.299679669));
#295650=CARTESIAN_POINT('Ctrl Pts',(-1.63300231200005,11.6,-10.299679669));
#295651=CARTESIAN_POINT('Ctrl Pts',(-1.63262359900005,15.2,-10.298408156));
#295652=CARTESIAN_POINT('Ctrl Pts',(-1.63262359900005,11.6,-10.298408156));
#295653=CARTESIAN_POINT('Ctrl Pts',(-1.63224853600005,15.2,-10.297144443));
#295654=CARTESIAN_POINT('Ctrl Pts',(-1.63224853600005,11.6,-10.297144443));
#295655=CARTESIAN_POINT('Ctrl Pts',(-1.63187711600006,15.2,-10.295888554));
#295656=CARTESIAN_POINT('Ctrl Pts',(-1.63187711600006,11.6,-10.295888554));
#295657=CARTESIAN_POINT('Ctrl Pts',(-1.63150933000006,15.2,-10.294640518));
#295658=CARTESIAN_POINT('Ctrl Pts',(-1.63150933000006,11.6,-10.294640518));
#295659=CARTESIAN_POINT('Ctrl Pts',(-1.63114516900006,15.2,-10.293400358));
#295660=CARTESIAN_POINT('Ctrl Pts',(-1.63114516900006,11.6,-10.293400358));
#295661=CARTESIAN_POINT('Ctrl Pts',(-1.63078462400006,15.2,-10.292168099));
#295662=CARTESIAN_POINT('Ctrl Pts',(-1.63078462400006,11.6,-10.292168099));
#295663=CARTESIAN_POINT('Ctrl Pts',(-1.63042768700006,15.2,-10.290943769));
#295664=CARTESIAN_POINT('Ctrl Pts',(-1.63042768700006,11.6,-10.290943769));
#295665=CARTESIAN_POINT('Ctrl Pts',(-1.63007434900006,15.2,-10.289727392));
#295666=CARTESIAN_POINT('Ctrl Pts',(-1.63007434900006,11.6,-10.289727392));
#295667=CARTESIAN_POINT('Ctrl Pts',(-1.62972460000006,15.2,-10.288518995));
#295668=CARTESIAN_POINT('Ctrl Pts',(-1.62972460000006,11.6,-10.288518995));
#295669=CARTESIAN_POINT('Ctrl Pts',(-1.62937843400006,15.2,-10.287318604));
#295670=CARTESIAN_POINT('Ctrl Pts',(-1.62937843400006,11.6,-10.287318604));
#295671=CARTESIAN_POINT('Ctrl Pts',(-1.62903583800006,15.2,-10.286126246));
#295672=CARTESIAN_POINT('Ctrl Pts',(-1.62903583800006,11.6,-10.286126246));
#295673=CARTESIAN_POINT('Ctrl Pts',(-1.62869680700006,15.2,-10.284941945));
#295674=CARTESIAN_POINT('Ctrl Pts',(-1.62869680700006,11.6,-10.284941945));
#295675=CARTESIAN_POINT('Ctrl Pts',(-1.62836133000006,15.2,-10.283765729));
#295676=CARTESIAN_POINT('Ctrl Pts',(-1.62836133000006,11.6,-10.283765729));
#295677=CARTESIAN_POINT('Ctrl Pts',(-1.62802939800006,15.2,-10.282597626));
#295678=CARTESIAN_POINT('Ctrl Pts',(-1.62802939800006,11.6,-10.282597626));
#295679=CARTESIAN_POINT('Ctrl Pts',(-1.62770100100006,15.2,-10.281437659));
#295680=CARTESIAN_POINT('Ctrl Pts',(-1.62770100100006,11.6,-10.281437659));
#295681=CARTESIAN_POINT('Ctrl Pts',(-1.62737613100005,15.2,-10.280285858));
#295682=CARTESIAN_POINT('Ctrl Pts',(-1.62737613100005,11.6,-10.280285858));
#295683=CARTESIAN_POINT('Ctrl Pts',(-1.62705477800006,15.2,-10.279142249));
#295684=CARTESIAN_POINT('Ctrl Pts',(-1.62705477800006,11.6,-10.279142249));
#295685=CARTESIAN_POINT('Ctrl Pts',(-1.62673693500006,15.2,-10.278006858));
#295686=CARTESIAN_POINT('Ctrl Pts',(-1.62673693500006,11.6,-10.278006858));
#295687=CARTESIAN_POINT('Ctrl Pts',(-1.62642258900005,15.2,-10.276879714));
#295688=CARTESIAN_POINT('Ctrl Pts',(-1.62642258900005,11.6,-10.276879714));
#295689=CARTESIAN_POINT('Ctrl Pts',(-1.62611173300005,15.2,-10.275760843));
#295690=CARTESIAN_POINT('Ctrl Pts',(-1.62611173300005,11.6,-10.275760843));
#295691=CARTESIAN_POINT('Ctrl Pts',(-1.62580435500006,15.2,-10.274650272));
#295692=CARTESIAN_POINT('Ctrl Pts',(-1.62580435500006,11.6,-10.274650272));
#295693=CARTESIAN_POINT('Ctrl Pts',(-1.62550044800006,15.2,-10.27354803));
#295694=CARTESIAN_POINT('Ctrl Pts',(-1.62550044800006,11.6,-10.27354803));
#295695=CARTESIAN_POINT('Ctrl Pts',(-1.62520000300006,15.2,-10.272454143));
#295696=CARTESIAN_POINT('Ctrl Pts',(-1.62520000300006,11.6,-10.272454143));
#295697=CARTESIAN_POINT('Ctrl Pts',(-1.62490300800005,15.2,-10.27136864));
#295698=CARTESIAN_POINT('Ctrl Pts',(-1.62490300800005,11.6,-10.27136864));
#295699=CARTESIAN_POINT('Ctrl Pts',(-1.62460945300006,15.2,-10.270291548));
#295700=CARTESIAN_POINT('Ctrl Pts',(-1.62460945300006,11.6,-10.270291548));
#295701=CARTESIAN_POINT('Ctrl Pts',(-1.62431933100006,15.2,-10.269222895));
#295702=CARTESIAN_POINT('Ctrl Pts',(-1.62431933100006,11.6,-10.269222895));
#295703=CARTESIAN_POINT('Ctrl Pts',(-1.62403263000006,15.2,-10.268162711));
#295704=CARTESIAN_POINT('Ctrl Pts',(-1.62403263000006,11.6,-10.268162711));
#295705=CARTESIAN_POINT('Ctrl Pts',(-1.62374934000006,15.2,-10.267111021));
#295706=CARTESIAN_POINT('Ctrl Pts',(-1.62374934000006,11.6,-10.267111021));
#295707=CARTESIAN_POINT('Ctrl Pts',(-1.62346945200006,15.2,-10.266067857));
#295708=CARTESIAN_POINT('Ctrl Pts',(-1.62346945200006,11.6,-10.266067857));
#295709=CARTESIAN_POINT('Ctrl Pts',(-1.62319295600006,15.2,-10.265033246));
#295710=CARTESIAN_POINT('Ctrl Pts',(-1.62319295600006,11.6,-10.265033246));
#295711=CARTESIAN_POINT('Ctrl Pts',(-1.62291984100006,15.2,-10.264007214));
#295712=CARTESIAN_POINT('Ctrl Pts',(-1.62291984100006,11.6,-10.264007214));
#295713=CARTESIAN_POINT('Ctrl Pts',(-1.62265009700006,15.2,-10.262989795));
#295714=CARTESIAN_POINT('Ctrl Pts',(-1.62265009700006,11.6,-10.262989795));
#295715=CARTESIAN_POINT('Ctrl Pts',(-1.62238371500006,15.2,-10.261981014));
#295716=CARTESIAN_POINT('Ctrl Pts',(-1.62238371500006,11.6,-10.261981014));
#295717=CARTESIAN_POINT('Ctrl Pts',(-1.62212068400006,15.2,-10.260980901));
#295718=CARTESIAN_POINT('Ctrl Pts',(-1.62212068400006,11.6,-10.260980901));
#295719=CARTESIAN_POINT('Ctrl Pts',(-1.62186099300006,15.2,-10.259989485));
#295720=CARTESIAN_POINT('Ctrl Pts',(-1.62186099300006,11.6,-10.259989485));
#295721=CARTESIAN_POINT('Ctrl Pts',(-1.62160463200005,15.2,-10.259006796));
#295722=CARTESIAN_POINT('Ctrl Pts',(-1.62160463200005,11.6,-10.259006796));
#295723=CARTESIAN_POINT('Ctrl Pts',(-1.62135159100006,15.2,-10.258032864));
#295724=CARTESIAN_POINT('Ctrl Pts',(-1.62135159100006,11.6,-10.258032864));
#295725=CARTESIAN_POINT('Ctrl Pts',(-1.62110185800006,15.2,-10.257067717));
#295726=CARTESIAN_POINT('Ctrl Pts',(-1.62110185800006,11.6,-10.257067717));
#295727=CARTESIAN_POINT('Ctrl Pts',(-1.62085542500006,15.2,-10.256111386));
#295728=CARTESIAN_POINT('Ctrl Pts',(-1.62085542500006,11.6,-10.256111386));
#295729=CARTESIAN_POINT('Ctrl Pts',(-1.62061227900006,15.2,-10.255163901));
#295730=CARTESIAN_POINT('Ctrl Pts',(-1.62061227900006,11.6,-10.255163901));
#295731=CARTESIAN_POINT('Ctrl Pts',(-1.62037241000006,15.2,-10.254225291));
#295732=CARTESIAN_POINT('Ctrl Pts',(-1.62037241000006,11.6,-10.254225291));
#295733=CARTESIAN_POINT('Ctrl Pts',(-1.62013580800005,15.2,-10.253295586));
#295734=CARTESIAN_POINT('Ctrl Pts',(-1.62013580800005,11.6,-10.253295586));
#295735=CARTESIAN_POINT('Ctrl Pts',(-1.61990246100005,15.2,-10.252374817));
#295736=CARTESIAN_POINT('Ctrl Pts',(-1.61990246100005,11.6,-10.252374817));
#295737=CARTESIAN_POINT('Ctrl Pts',(-1.61967235800006,15.2,-10.251463016));
#295738=CARTESIAN_POINT('Ctrl Pts',(-1.61967235800006,11.6,-10.251463016));
#295739=CARTESIAN_POINT('Ctrl Pts',(-1.61944548900005,15.2,-10.250560211));
#295740=CARTESIAN_POINT('Ctrl Pts',(-1.61944548900005,11.6,-10.250560211));
#295741=CARTESIAN_POINT('Ctrl Pts',(-1.61922313100006,15.2,-10.249671582));
#295742=CARTESIAN_POINT('Ctrl Pts',(-1.61922313100006,11.6,-10.249671582));
#295743=CARTESIAN_POINT('Ctrl Pts',(-1.61904803300006,15.2,-10.248968851));
#295744=CARTESIAN_POINT('Ctrl Pts',(-1.61904803300006,11.6,-10.248968851));
#295745=CARTESIAN_POINT('Ctrl Pts',(-1.61891844100006,15.2,-10.24844709));
#295746=CARTESIAN_POINT('Ctrl Pts',(-1.61891844100006,11.6,-10.24844709));
#295747=CARTESIAN_POINT('Ctrl Pts',(-1.61883308400005,15.2,-10.248102703));
#295748=CARTESIAN_POINT('Ctrl Pts',(-1.61883308400005,11.6,-10.248102703));
#295749=CARTESIAN_POINT('Ctrl Pts',(-1.61879118000006,15.2,-10.247933456));
#295750=CARTESIAN_POINT('Ctrl Pts',(-1.61879118000006,11.6,-10.247933456));
#295751=CARTESIAN_POINT('',(-1.61879117999241,12.2,-10.2479334556183));
#295752=CARTESIAN_POINT('',(-1.61879117999241,15.2,-10.2479334556183));
#295753=CARTESIAN_POINT('',(-1.61879118000006,12.2,-10.247933455));
#295754=CARTESIAN_POINT('Ctrl Pts',(-2.17615954800006,12.2,-11.292224299));
#295755=CARTESIAN_POINT('Ctrl Pts',(-2.17570045500006,12.2,-11.291612887));
#295756=CARTESIAN_POINT('Ctrl Pts',(-2.17478276600006,12.2,-11.290390245));
#295757=CARTESIAN_POINT('Ctrl Pts',(-2.17340771700006,12.2,-11.28855682));
#295758=CARTESIAN_POINT('Ctrl Pts',(-2.17157728800006,12.2,-11.286113334));
#295759=CARTESIAN_POINT('Ctrl Pts',(-2.16929420200006,12.2,-11.283060773));
#295760=CARTESIAN_POINT('Ctrl Pts',(-2.16701606700005,12.2,-11.280010015));
#295761=CARTESIAN_POINT('Ctrl Pts',(-2.16474288100006,12.2,-11.276961058));
#295762=CARTESIAN_POINT('Ctrl Pts',(-2.16247464600006,12.2,-11.273913908));
#295763=CARTESIAN_POINT('Ctrl Pts',(-2.16021136000006,12.2,-11.27086857));
#295764=CARTESIAN_POINT('Ctrl Pts',(-2.15795302500006,12.2,-11.267825054));
#295765=CARTESIAN_POINT('Ctrl Pts',(-2.15569963800006,12.2,-11.264783368));
#295766=CARTESIAN_POINT('Ctrl Pts',(-2.15345120200006,12.2,-11.261743524));
#295767=CARTESIAN_POINT('Ctrl Pts',(-2.15120771500006,12.2,-11.258705531));
#295768=CARTESIAN_POINT('Ctrl Pts',(-2.14896917600006,12.2,-11.255669403));
#295769=CARTESIAN_POINT('Ctrl Pts',(-2.14673558400006,12.2,-11.252635149));
#295770=CARTESIAN_POINT('Ctrl Pts',(-2.14450694000006,12.2,-11.249602777));
#295771=CARTESIAN_POINT('Ctrl Pts',(-2.14228324400006,12.2,-11.246572299));
#295772=CARTESIAN_POINT('Ctrl Pts',(-2.14006449500005,12.2,-11.243543721));
#295773=CARTESIAN_POINT('Ctrl Pts',(-2.13785069300005,12.2,-11.24051705));
#295774=CARTESIAN_POINT('Ctrl Pts',(-2.13564183800006,12.2,-11.237492297));
#295775=CARTESIAN_POINT('Ctrl Pts',(-2.13343792800006,12.2,-11.234469469));
#295776=CARTESIAN_POINT('Ctrl Pts',(-2.13123896500006,12.2,-11.231448574));
#295777=CARTESIAN_POINT('Ctrl Pts',(-2.12904494800005,12.2,-11.228429624));
#295778=CARTESIAN_POINT('Ctrl Pts',(-2.12685587600005,12.2,-11.225412626));
#295779=CARTESIAN_POINT('Ctrl Pts',(-2.12467174800006,12.2,-11.222397592));
#295780=CARTESIAN_POINT('Ctrl Pts',(-2.12249256500006,12.2,-11.219384528));
#295781=CARTESIAN_POINT('Ctrl Pts',(-2.12031832600006,12.2,-11.216373446));
#295782=CARTESIAN_POINT('Ctrl Pts',(-2.11814903000006,12.2,-11.213364356));
#295783=CARTESIAN_POINT('Ctrl Pts',(-2.11598467700005,12.2,-11.210357264));
#295784=CARTESIAN_POINT('Ctrl Pts',(-2.11382526700006,12.2,-11.207352181));
#295785=CARTESIAN_POINT('Ctrl Pts',(-2.11167080000005,12.2,-11.204349116));
#295786=CARTESIAN_POINT('Ctrl Pts',(-2.10952127400006,12.2,-11.201348078));
#295787=CARTESIAN_POINT('Ctrl Pts',(-2.10737669000005,12.2,-11.198349076));
#295788=CARTESIAN_POINT('Ctrl Pts',(-2.10523704700006,12.2,-11.19535212));
#295789=CARTESIAN_POINT('Ctrl Pts',(-2.10310234500006,12.2,-11.192357218));
#295790=CARTESIAN_POINT('Ctrl Pts',(-2.10097258200005,12.2,-11.18936438));
#295791=CARTESIAN_POINT('Ctrl Pts',(-2.09884776000006,12.2,-11.186373616));
#295792=CARTESIAN_POINT('Ctrl Pts',(-2.09672787600006,12.2,-11.183384935));
#295793=CARTESIAN_POINT('Ctrl Pts',(-2.09461293200006,12.2,-11.180398346));
#295794=CARTESIAN_POINT('Ctrl Pts',(-2.09250292400006,12.2,-11.177413859));
#295795=CARTESIAN_POINT('Ctrl Pts',(-2.09039785500006,12.2,-11.174431482));
#295796=CARTESIAN_POINT('Ctrl Pts',(-2.08829772300006,12.2,-11.171451227));
#295797=CARTESIAN_POINT('Ctrl Pts',(-2.08620252700006,12.2,-11.1684731));
#295798=CARTESIAN_POINT('Ctrl Pts',(-2.08411226900005,12.2,-11.165497114));
#295799=CARTESIAN_POINT('Ctrl Pts',(-2.08202694500006,12.2,-11.162523276));
#295800=CARTESIAN_POINT('Ctrl Pts',(-2.07994655600006,12.2,-11.159551596));
#295801=CARTESIAN_POINT('Ctrl Pts',(-2.07787110100006,12.2,-11.156582084));
#295802=CARTESIAN_POINT('Ctrl Pts',(-2.07580058000006,12.2,-11.153614748));
#295803=CARTESIAN_POINT('Ctrl Pts',(-2.07373499200005,12.2,-11.1506496));
#295804=CARTESIAN_POINT('Ctrl Pts',(-2.07167433800006,12.2,-11.147686647));
#295805=CARTESIAN_POINT('Ctrl Pts',(-2.06961861500006,12.2,-11.1447259));
#295806=CARTESIAN_POINT('Ctrl Pts',(-2.06756782400006,12.2,-11.141767369));
#295807=CARTESIAN_POINT('Ctrl Pts',(-2.06552196300006,12.2,-11.138811062));
#295808=CARTESIAN_POINT('Ctrl Pts',(-2.06348103200006,12.2,-11.13585699));
#295809=CARTESIAN_POINT('Ctrl Pts',(-2.06144503200006,12.2,-11.132905162));
#295810=CARTESIAN_POINT('Ctrl Pts',(-2.05941396000005,12.2,-11.129955589));
#295811=CARTESIAN_POINT('Ctrl Pts',(-2.05738781600005,12.2,-11.127008278));
#295812=CARTESIAN_POINT('Ctrl Pts',(-2.05536660000006,12.2,-11.12406324));
#295813=CARTESIAN_POINT('Ctrl Pts',(-2.05335031200006,12.2,-11.121120485));
#295814=CARTESIAN_POINT('Ctrl Pts',(-2.05133894900006,12.2,-11.118180023));
#295815=CARTESIAN_POINT('Ctrl Pts',(-2.04933251100006,12.2,-11.115241862));
#295816=CARTESIAN_POINT('Ctrl Pts',(-2.04733100000006,12.2,-11.112306013));
#295817=CARTESIAN_POINT('Ctrl Pts',(-2.04533441100006,12.2,-11.109372486));
#295818=CARTESIAN_POINT('Ctrl Pts',(-2.04334274700006,12.2,-11.106441291));
#295819=CARTESIAN_POINT('Ctrl Pts',(-2.04135600500006,12.2,-11.103512437));
#295820=CARTESIAN_POINT('Ctrl Pts',(-2.03937418400006,12.2,-11.100585934));
#295821=CARTESIAN_POINT('Ctrl Pts',(-2.03739728600006,12.2,-11.097661791));
#295822=CARTESIAN_POINT('Ctrl Pts',(-2.03542530900005,12.2,-11.094740019));
#295823=CARTESIAN_POINT('Ctrl Pts',(-2.03345825000006,12.2,-11.091820627));
#295824=CARTESIAN_POINT('Ctrl Pts',(-2.03149611100006,12.2,-11.088903627));
#295825=CARTESIAN_POINT('Ctrl Pts',(-2.02953889000006,12.2,-11.085989026));
#295826=CARTESIAN_POINT('Ctrl Pts',(-2.02758658500006,12.2,-11.083076836));
#295827=CARTESIAN_POINT('Ctrl Pts',(-2.02563919900005,12.2,-11.080167065));
#295828=CARTESIAN_POINT('Ctrl Pts',(-2.02369672800006,12.2,-11.077259724));
#295829=CARTESIAN_POINT('Ctrl Pts',(-2.02175917100006,12.2,-11.074354824));
#295830=CARTESIAN_POINT('Ctrl Pts',(-2.01982652900006,12.2,-11.071452373));
#295831=CARTESIAN_POINT('Ctrl Pts',(-2.01789880000006,12.2,-11.068552382));
#295832=CARTESIAN_POINT('Ctrl Pts',(-2.01597598400005,12.2,-11.065654863));
#295833=CARTESIAN_POINT('Ctrl Pts',(-2.01405807900006,12.2,-11.062759821));
#295834=CARTESIAN_POINT('Ctrl Pts',(-2.01214508600006,12.2,-11.059867271));
#295835=CARTESIAN_POINT('Ctrl Pts',(-2.01023700100006,12.2,-11.056977221));
#295836=CARTESIAN_POINT('Ctrl Pts',(-2.00833382600006,12.2,-11.054089681));
#295837=CARTESIAN_POINT('Ctrl Pts',(-2.00643555900006,12.2,-11.05120466));
#295838=CARTESIAN_POINT('Ctrl Pts',(-2.00454219900006,12.2,-11.048322171));
#295839=CARTESIAN_POINT('Ctrl Pts',(-2.00265374600006,12.2,-11.045442222));
#295840=CARTESIAN_POINT('Ctrl Pts',(-2.00077019700006,12.2,-11.042564824));
#295841=CARTESIAN_POINT('Ctrl Pts',(-1.99889155400006,12.2,-11.039689987));
#295842=CARTESIAN_POINT('Ctrl Pts',(-1.99701781300006,12.2,-11.03681772));
#295843=CARTESIAN_POINT('Ctrl Pts',(-1.99514897500006,12.2,-11.033948035));
#295844=CARTESIAN_POINT('Ctrl Pts',(-1.99328503900006,12.2,-11.031080942));
#295845=CARTESIAN_POINT('Ctrl Pts',(-1.99142600300006,12.2,-11.02821645));
#295846=CARTESIAN_POINT('Ctrl Pts',(-1.98957186800006,12.2,-11.025354571));
#295847=CARTESIAN_POINT('Ctrl Pts',(-1.98772263100006,12.2,-11.022495313));
#295848=CARTESIAN_POINT('Ctrl Pts',(-1.98587829000005,12.2,-11.019638689));
#295849=CARTESIAN_POINT('Ctrl Pts',(-1.98403884700005,12.2,-11.016784707));
#295850=CARTESIAN_POINT('Ctrl Pts',(-1.98220430000006,12.2,-11.013933379));
#295851=CARTESIAN_POINT('Ctrl Pts',(-1.98037464600006,12.2,-11.011084714));
#295852=CARTESIAN_POINT('Ctrl Pts',(-1.97854988600006,12.2,-11.008238724));
#295853=CARTESIAN_POINT('Ctrl Pts',(-1.97673001900006,12.2,-11.005395418));
#295854=CARTESIAN_POINT('Ctrl Pts',(-1.97491504200005,12.2,-11.002554807));
#295855=CARTESIAN_POINT('Ctrl Pts',(-1.97310495700005,12.2,-10.999716901));
#295856=CARTESIAN_POINT('Ctrl Pts',(-1.97129976000005,12.2,-10.996881712));
#295857=CARTESIAN_POINT('Ctrl Pts',(-1.96949945100006,12.2,-10.994049247));
#295858=CARTESIAN_POINT('Ctrl Pts',(-1.96770402900006,12.2,-10.99121952));
#295859=CARTESIAN_POINT('Ctrl Pts',(-1.96591349400005,12.2,-10.988392541));
#295860=CARTESIAN_POINT('Ctrl Pts',(-1.96412784300006,12.2,-10.985568319));
#295861=CARTESIAN_POINT('Ctrl Pts',(-1.96234707500006,12.2,-10.982746866));
#295862=CARTESIAN_POINT('Ctrl Pts',(-1.96057119000006,12.2,-10.979928192));
#295863=CARTESIAN_POINT('Ctrl Pts',(-1.95880018600006,12.2,-10.977112307));
#295864=CARTESIAN_POINT('Ctrl Pts',(-1.95703406200006,12.2,-10.974299223));
#295865=CARTESIAN_POINT('Ctrl Pts',(-1.95527281700006,12.2,-10.971488949));
#295866=CARTESIAN_POINT('Ctrl Pts',(-1.95351645100006,12.2,-10.968681498));
#295867=CARTESIAN_POINT('Ctrl Pts',(-1.95176495900005,12.2,-10.965876877));
#295868=CARTESIAN_POINT('Ctrl Pts',(-1.95001834500005,12.2,-10.963075101));
#295869=CARTESIAN_POINT('Ctrl Pts',(-1.94827660300006,12.2,-10.960276177));
#295870=CARTESIAN_POINT('Ctrl Pts',(-1.94653973400006,12.2,-10.957480118));
#295871=CARTESIAN_POINT('Ctrl Pts',(-1.94480773800006,12.2,-10.954686934));
#295872=CARTESIAN_POINT('Ctrl Pts',(-1.94308061000006,12.2,-10.951896636));
#295873=CARTESIAN_POINT('Ctrl Pts',(-1.94135835200006,12.2,-10.949109235));
#295874=CARTESIAN_POINT('Ctrl Pts',(-1.93964096300005,12.2,-10.946324741));
#295875=CARTESIAN_POINT('Ctrl Pts',(-1.93792843900006,12.2,-10.943543166));
#295876=CARTESIAN_POINT('Ctrl Pts',(-1.93622078100006,12.2,-10.940764519));
#295877=CARTESIAN_POINT('Ctrl Pts',(-1.93451798600006,12.2,-10.937988814));
#295878=CARTESIAN_POINT('Ctrl Pts',(-1.93282005500006,12.2,-10.935216058));
#295879=CARTESIAN_POINT('Ctrl Pts',(-1.93112698400005,12.2,-10.932446266));
#295880=CARTESIAN_POINT('Ctrl Pts',(-1.92943877200005,12.2,-10.929679446));
#295881=CARTESIAN_POINT('Ctrl Pts',(-1.92775541900006,12.2,-10.92691561));
#295882=CARTESIAN_POINT('Ctrl Pts',(-1.92607692400005,12.2,-10.924154768));
#295883=CARTESIAN_POINT('Ctrl Pts',(-1.92440328400005,12.2,-10.921396933));
#295884=CARTESIAN_POINT('Ctrl Pts',(-1.92273449900005,12.2,-10.918642115));
#295885=CARTESIAN_POINT('Ctrl Pts',(-1.92107056600005,12.2,-10.915890324));
#295886=CARTESIAN_POINT('Ctrl Pts',(-1.91941148400006,12.2,-10.913141573));
#295887=CARTESIAN_POINT('Ctrl Pts',(-1.91775725300006,12.2,-10.910395872));
#295888=CARTESIAN_POINT('Ctrl Pts',(-1.91610787000006,12.2,-10.907653232));
#295889=CARTESIAN_POINT('Ctrl Pts',(-1.91446333500006,12.2,-10.904913664));
#295890=CARTESIAN_POINT('Ctrl Pts',(-1.91282364500006,12.2,-10.902177181));
#295891=CARTESIAN_POINT('Ctrl Pts',(-1.91118879900006,12.2,-10.899443792));
#295892=CARTESIAN_POINT('Ctrl Pts',(-1.90955879600006,12.2,-10.89671351));
#295893=CARTESIAN_POINT('Ctrl Pts',(-1.90793363400006,12.2,-10.893986344));
#295894=CARTESIAN_POINT('Ctrl Pts',(-1.90631331200006,12.2,-10.891262307));
#295895=CARTESIAN_POINT('Ctrl Pts',(-1.90469782800006,12.2,-10.888541409));
#295896=CARTESIAN_POINT('Ctrl Pts',(-1.90308718100006,12.2,-10.885823664));
#295897=CARTESIAN_POINT('Ctrl Pts',(-1.90148136800006,12.2,-10.88310908));
#295898=CARTESIAN_POINT('Ctrl Pts',(-1.89988038900006,12.2,-10.880397671));
#295899=CARTESIAN_POINT('Ctrl Pts',(-1.89828424200006,12.2,-10.877689446));
#295900=CARTESIAN_POINT('Ctrl Pts',(-1.89669292500006,12.2,-10.874984418));
#295901=CARTESIAN_POINT('Ctrl Pts',(-1.89510643700005,12.2,-10.872282597));
#295902=CARTESIAN_POINT('Ctrl Pts',(-1.89352477600006,12.2,-10.869583997));
#295903=CARTESIAN_POINT('Ctrl Pts',(-1.89194794100006,12.2,-10.866888627));
#295904=CARTESIAN_POINT('Ctrl Pts',(-1.89037592900006,12.2,-10.8641965));
#295905=CARTESIAN_POINT('Ctrl Pts',(-1.88880874000006,12.2,-10.861507626));
#295906=CARTESIAN_POINT('Ctrl Pts',(-1.88724637200006,12.2,-10.858822018));
#295907=CARTESIAN_POINT('Ctrl Pts',(-1.88568882100005,12.2,-10.856139687));
#295908=CARTESIAN_POINT('Ctrl Pts',(-1.88413608800006,12.2,-10.853460644));
#295909=CARTESIAN_POINT('Ctrl Pts',(-1.88258817100006,12.2,-10.850784903));
#295910=CARTESIAN_POINT('Ctrl Pts',(-1.88104506800005,12.2,-10.848112472));
#295911=CARTESIAN_POINT('Ctrl Pts',(-1.87950677700006,12.2,-10.845443365));
#295912=CARTESIAN_POINT('Ctrl Pts',(-1.87797329500006,12.2,-10.842777593));
#295913=CARTESIAN_POINT('Ctrl Pts',(-1.87644462200006,12.2,-10.840115167));
#295914=CARTESIAN_POINT('Ctrl Pts',(-1.87492075700006,12.2,-10.837456101));
#295915=CARTESIAN_POINT('Ctrl Pts',(-1.87340169600006,12.2,-10.834800405));
#295916=CARTESIAN_POINT('Ctrl Pts',(-1.87188743800006,12.2,-10.832148091));
#295917=CARTESIAN_POINT('Ctrl Pts',(-1.87037798200006,12.2,-10.829499171));
#295918=CARTESIAN_POINT('Ctrl Pts',(-1.86887332500006,12.2,-10.826853656));
#295919=CARTESIAN_POINT('Ctrl Pts',(-1.86737346700005,12.2,-10.82421156));
#295920=CARTESIAN_POINT('Ctrl Pts',(-1.86587840400006,12.2,-10.821572893));
#295921=CARTESIAN_POINT('Ctrl Pts',(-1.86438813500006,12.2,-10.818937666));
#295922=CARTESIAN_POINT('Ctrl Pts',(-1.86290265800006,12.2,-10.816305894));
#295923=CARTESIAN_POINT('Ctrl Pts',(-1.86142197200006,12.2,-10.813677586));
#295924=CARTESIAN_POINT('Ctrl Pts',(-1.85994607300006,12.2,-10.811052755));
#295925=CARTESIAN_POINT('Ctrl Pts',(-1.85847496200006,12.2,-10.808431414));
#295926=CARTESIAN_POINT('Ctrl Pts',(-1.85700863500006,12.2,-10.805813575));
#295927=CARTESIAN_POINT('Ctrl Pts',(-1.85554709100006,12.2,-10.803199248));
#295928=CARTESIAN_POINT('Ctrl Pts',(-1.85409032800006,12.2,-10.800588447));
#295929=CARTESIAN_POINT('Ctrl Pts',(-1.85263834300006,12.2,-10.797981184));
#295930=CARTESIAN_POINT('Ctrl Pts',(-1.85119113400006,12.2,-10.795377469));
#295931=CARTESIAN_POINT('Ctrl Pts',(-1.84974870200006,12.2,-10.792777317));
#295932=CARTESIAN_POINT('Ctrl Pts',(-1.84831104100006,12.2,-10.790180739));
#295933=CARTESIAN_POINT('Ctrl Pts',(-1.84687815100005,12.2,-10.787587746));
#295934=CARTESIAN_POINT('Ctrl Pts',(-1.84545003000005,12.2,-10.784998353));
#295935=CARTESIAN_POINT('Ctrl Pts',(-1.84402667500006,12.2,-10.78241257));
#295936=CARTESIAN_POINT('Ctrl Pts',(-1.84260808600006,12.2,-10.77983041));
#295937=CARTESIAN_POINT('Ctrl Pts',(-1.84119425800006,12.2,-10.777251885));
#295938=CARTESIAN_POINT('Ctrl Pts',(-1.83978519200006,12.2,-10.774677008));
#295939=CARTESIAN_POINT('Ctrl Pts',(-1.83838088300006,12.2,-10.77210579));
#295940=CARTESIAN_POINT('Ctrl Pts',(-1.83698133100005,12.2,-10.769538245));
#295941=CARTESIAN_POINT('Ctrl Pts',(-1.83558653300006,12.2,-10.766974386));
#295942=CARTESIAN_POINT('Ctrl Pts',(-1.83419648600006,12.2,-10.764414223));
#295943=CARTESIAN_POINT('Ctrl Pts',(-1.83281119000006,12.2,-10.76185777));
#295944=CARTESIAN_POINT('Ctrl Pts',(-1.83143064100005,12.2,-10.759305039));
#295945=CARTESIAN_POINT('Ctrl Pts',(-1.83005483700006,12.2,-10.756756043));
#295946=CARTESIAN_POINT('Ctrl Pts',(-1.82868377600006,12.2,-10.754210794));
#295947=CARTESIAN_POINT('Ctrl Pts',(-1.82731745700006,12.2,-10.751669306));
#295948=CARTESIAN_POINT('Ctrl Pts',(-1.82595587600006,12.2,-10.749131589));
#295949=CARTESIAN_POINT('Ctrl Pts',(-1.82459903200006,12.2,-10.746597658));
#295950=CARTESIAN_POINT('Ctrl Pts',(-1.82324692200006,12.2,-10.744067526));
#295951=CARTESIAN_POINT('Ctrl Pts',(-1.82189954400006,12.2,-10.741541203));
#295952=CARTESIAN_POINT('Ctrl Pts',(-1.82055689600006,12.2,-10.739018703));
#295953=CARTESIAN_POINT('Ctrl Pts',(-1.81921897500006,12.2,-10.73650004));
#295954=CARTESIAN_POINT('Ctrl Pts',(-1.81788577800006,12.2,-10.733985227));
#295955=CARTESIAN_POINT('Ctrl Pts',(-1.81655730500006,12.2,-10.731474274));
#295956=CARTESIAN_POINT('Ctrl Pts',(-1.81523355200006,12.2,-10.728967196));
#295957=CARTESIAN_POINT('Ctrl Pts',(-1.81391451700006,12.2,-10.726464005));
#295958=CARTESIAN_POINT('Ctrl Pts',(-1.81260019800006,12.2,-10.723964715));
#295959=CARTESIAN_POINT('Ctrl Pts',(-1.81129059100006,12.2,-10.721469338));
#295960=CARTESIAN_POINT('Ctrl Pts',(-1.80998569500006,12.2,-10.718977888));
#295961=CARTESIAN_POINT('Ctrl Pts',(-1.80868550800006,12.2,-10.716490376));
#295962=CARTESIAN_POINT('Ctrl Pts',(-1.80739002700005,12.2,-10.714006817));
#295963=CARTESIAN_POINT('Ctrl Pts',(-1.80609924900006,12.2,-10.711527223));
#295964=CARTESIAN_POINT('Ctrl Pts',(-1.80481317200006,12.2,-10.709051608));
#295965=CARTESIAN_POINT('Ctrl Pts',(-1.80353179300006,12.2,-10.706579983));
#295966=CARTESIAN_POINT('Ctrl Pts',(-1.80225511100006,12.2,-10.704112363));
#295967=CARTESIAN_POINT('Ctrl Pts',(-1.80098312100006,12.2,-10.701648762));
#295968=CARTESIAN_POINT('Ctrl Pts',(-1.79971582300006,12.2,-10.699189192));
#295969=CARTESIAN_POINT('Ctrl Pts',(-1.79845321300005,12.2,-10.696733666));
#295970=CARTESIAN_POINT('Ctrl Pts',(-1.79719528800006,12.2,-10.694282196));
#295971=CARTESIAN_POINT('Ctrl Pts',(-1.79594204700006,12.2,-10.691834799));
#295972=CARTESIAN_POINT('Ctrl Pts',(-1.79469348600006,12.2,-10.689391486));
#295973=CARTESIAN_POINT('Ctrl Pts',(-1.79344960300006,12.2,-10.686952269));
#295974=CARTESIAN_POINT('Ctrl Pts',(-1.79221039500006,12.2,-10.684517164));
#295975=CARTESIAN_POINT('Ctrl Pts',(-1.79097586000006,12.2,-10.682086183));
#295976=CARTESIAN_POINT('Ctrl Pts',(-1.78974599400005,12.2,-10.67965934));
#295977=CARTESIAN_POINT('Ctrl Pts',(-1.78852079600006,12.2,-10.677236648));
#295978=CARTESIAN_POINT('Ctrl Pts',(-1.78730026300005,12.2,-10.674818122));
#295979=CARTESIAN_POINT('Ctrl Pts',(-1.78608439100006,12.2,-10.672403774));
#295980=CARTESIAN_POINT('Ctrl Pts',(-1.78487317800006,12.2,-10.669993617));
#295981=CARTESIAN_POINT('Ctrl Pts',(-1.78366662300005,12.2,-10.667587667));
#295982=CARTESIAN_POINT('Ctrl Pts',(-1.78246472000006,12.2,-10.665185935));
#295983=CARTESIAN_POINT('Ctrl Pts',(-1.78126746700006,12.2,-10.662788437));
#295984=CARTESIAN_POINT('Ctrl Pts',(-1.78007486300006,12.2,-10.660395184));
#295985=CARTESIAN_POINT('Ctrl Pts',(-1.77888690400006,12.2,-10.658006194));
#295986=CARTESIAN_POINT('Ctrl Pts',(-1.77770358700006,12.2,-10.655621476));
#295987=CARTESIAN_POINT('Ctrl Pts',(-1.77652491000006,12.2,-10.653241047));
#295988=CARTESIAN_POINT('Ctrl Pts',(-1.77535086900006,12.2,-10.65086492));
#295989=CARTESIAN_POINT('Ctrl Pts',(-1.77418146100006,12.2,-10.648493108));
#295990=CARTESIAN_POINT('Ctrl Pts',(-1.77301668500006,12.2,-10.646125627));
#295991=CARTESIAN_POINT('Ctrl Pts',(-1.77185653500006,12.2,-10.643762488));
#295992=CARTESIAN_POINT('Ctrl Pts',(-1.77070101200006,12.2,-10.641403708));
#295993=CARTESIAN_POINT('Ctrl Pts',(-1.76955010900006,12.2,-10.639049299));
#295994=CARTESIAN_POINT('Ctrl Pts',(-1.76840382600005,12.2,-10.636699276));
#295995=CARTESIAN_POINT('Ctrl Pts',(-1.76726215900006,12.2,-10.634353653));
#295996=CARTESIAN_POINT('Ctrl Pts',(-1.76612510400005,12.2,-10.632012444));
#295997=CARTESIAN_POINT('Ctrl Pts',(-1.76499265900006,12.2,-10.629675663));
#295998=CARTESIAN_POINT('Ctrl Pts',(-1.76386482100006,12.2,-10.627343324));
#295999=CARTESIAN_POINT('Ctrl Pts',(-1.76274158600006,12.2,-10.625015442));
#296000=CARTESIAN_POINT('Ctrl Pts',(-1.76162295200006,12.2,-10.622692031));
#296001=CARTESIAN_POINT('Ctrl Pts',(-1.76050891600006,12.2,-10.620373104));
#296002=CARTESIAN_POINT('Ctrl Pts',(-1.75939947300006,12.2,-10.618058678));
#296003=CARTESIAN_POINT('Ctrl Pts',(-1.75829462200006,12.2,-10.615748764));
#296004=CARTESIAN_POINT('Ctrl Pts',(-1.75719435900006,12.2,-10.61344338));
#296005=CARTESIAN_POINT('Ctrl Pts',(-1.75609868000006,12.2,-10.611142538));
#296006=CARTESIAN_POINT('Ctrl Pts',(-1.75500758400006,12.2,-10.608846253));
#296007=CARTESIAN_POINT('Ctrl Pts',(-1.75392106600006,12.2,-10.60655454));
#296008=CARTESIAN_POINT('Ctrl Pts',(-1.75283912300006,12.2,-10.604267414));
#296009=CARTESIAN_POINT('Ctrl Pts',(-1.75176175100006,12.2,-10.601984888));
#296010=CARTESIAN_POINT('Ctrl Pts',(-1.75068894900006,12.2,-10.599706978));
#296011=CARTESIAN_POINT('Ctrl Pts',(-1.74962071200006,12.2,-10.597433698));
#296012=CARTESIAN_POINT('Ctrl Pts',(-1.74855703600006,12.2,-10.595165063));
#296013=CARTESIAN_POINT('Ctrl Pts',(-1.74749792000006,12.2,-10.592901087));
#296014=CARTESIAN_POINT('Ctrl Pts',(-1.74644335700005,12.2,-10.590641786));
#296015=CARTESIAN_POINT('Ctrl Pts',(-1.74539334800006,12.2,-10.588387175));
#296016=CARTESIAN_POINT('Ctrl Pts',(-1.74434788700006,12.2,-10.586137267));
#296017=CARTESIAN_POINT('Ctrl Pts',(-1.74330697100005,12.2,-10.58389208));
#296018=CARTESIAN_POINT('Ctrl Pts',(-1.74227059600006,12.2,-10.581651626));
#296019=CARTESIAN_POINT('Ctrl Pts',(-1.74123875900006,12.2,-10.57941592));
#296020=CARTESIAN_POINT('Ctrl Pts',(-1.74021145800005,12.2,-10.577184979));
#296021=CARTESIAN_POINT('Ctrl Pts',(-1.73918868600006,12.2,-10.574958817));
#296022=CARTESIAN_POINT('Ctrl Pts',(-1.73817044300006,12.2,-10.572737449));
#296023=CARTESIAN_POINT('Ctrl Pts',(-1.73715672500005,12.2,-10.570520891));
#296024=CARTESIAN_POINT('Ctrl Pts',(-1.73614752700006,12.2,-10.568309157));
#296025=CARTESIAN_POINT('Ctrl Pts',(-1.73514284500006,12.2,-10.566102263));
#296026=CARTESIAN_POINT('Ctrl Pts',(-1.73414267600006,12.2,-10.563900224));
#296027=CARTESIAN_POINT('Ctrl Pts',(-1.73314701900006,12.2,-10.561703056));
#296028=CARTESIAN_POINT('Ctrl Pts',(-1.73215586600006,12.2,-10.559510773));
#296029=CARTESIAN_POINT('Ctrl Pts',(-1.73116921600006,12.2,-10.55732339));
#296030=CARTESIAN_POINT('Ctrl Pts',(-1.73018706500006,12.2,-10.555140925));
#296031=CARTESIAN_POINT('Ctrl Pts',(-1.72920940800006,12.2,-10.552963391));
#296032=CARTESIAN_POINT('Ctrl Pts',(-1.72823624300006,12.2,-10.550790805));
#296033=CARTESIAN_POINT('Ctrl Pts',(-1.72726756600006,12.2,-10.548623183));
#296034=CARTESIAN_POINT('Ctrl Pts',(-1.72630337200005,12.2,-10.546460538));
#296035=CARTESIAN_POINT('Ctrl Pts',(-1.72534365800006,12.2,-10.544302889));
#296036=CARTESIAN_POINT('Ctrl Pts',(-1.72438842000005,12.2,-10.542150249));
#296037=CARTESIAN_POINT('Ctrl Pts',(-1.72343765400006,12.2,-10.540002635));
#296038=CARTESIAN_POINT('Ctrl Pts',(-1.72249135800006,12.2,-10.537860062));
#296039=CARTESIAN_POINT('Ctrl Pts',(-1.72154952600006,12.2,-10.535722547));
#296040=CARTESIAN_POINT('Ctrl Pts',(-1.72061215300006,12.2,-10.533590105));
#296041=CARTESIAN_POINT('Ctrl Pts',(-1.71967923800006,12.2,-10.531462752));
#296042=CARTESIAN_POINT('Ctrl Pts',(-1.71875077600005,12.2,-10.529340504));
#296043=CARTESIAN_POINT('Ctrl Pts',(-1.71782676200006,12.2,-10.527223376));
#296044=CARTESIAN_POINT('Ctrl Pts',(-1.71690719200006,12.2,-10.525111386));
#296045=CARTESIAN_POINT('Ctrl Pts',(-1.71599206400006,12.2,-10.523004549));
#296046=CARTESIAN_POINT('Ctrl Pts',(-1.71508137200005,12.2,-10.520902882));
#296047=CARTESIAN_POINT('Ctrl Pts',(-1.71417511300006,12.2,-10.5188064));
#296048=CARTESIAN_POINT('Ctrl Pts',(-1.71327328300006,12.2,-10.516715119));
#296049=CARTESIAN_POINT('Ctrl Pts',(-1.71237587800006,12.2,-10.514629056));
#296050=CARTESIAN_POINT('Ctrl Pts',(-1.71148289100006,12.2,-10.512548228));
#296051=CARTESIAN_POINT('Ctrl Pts',(-1.71059432200006,12.2,-10.510472651));
#296052=CARTESIAN_POINT('Ctrl Pts',(-1.70971016400005,12.2,-10.50840234));
#296053=CARTESIAN_POINT('Ctrl Pts',(-1.70883041500006,12.2,-10.506337312));
#296054=CARTESIAN_POINT('Ctrl Pts',(-1.70795506800005,12.2,-10.504277584));
#296055=CARTESIAN_POINT('Ctrl Pts',(-1.70708412100006,12.2,-10.502223174));
#296056=CARTESIAN_POINT('Ctrl Pts',(-1.70621756900006,12.2,-10.500174096));
#296057=CARTESIAN_POINT('Ctrl Pts',(-1.70535540700006,12.2,-10.498130368));
#296058=CARTESIAN_POINT('Ctrl Pts',(-1.70449763200006,12.2,-10.496092006));
#296059=CARTESIAN_POINT('Ctrl Pts',(-1.70364423900006,12.2,-10.494059027));
#296060=CARTESIAN_POINT('Ctrl Pts',(-1.70279522300006,12.2,-10.492031449));
#296061=CARTESIAN_POINT('Ctrl Pts',(-1.70195058100005,12.2,-10.490009287));
#296062=CARTESIAN_POINT('Ctrl Pts',(-1.70111030700005,12.2,-10.487992559));
#296063=CARTESIAN_POINT('Ctrl Pts',(-1.70027439800006,12.2,-10.485981281));
#296064=CARTESIAN_POINT('Ctrl Pts',(-1.69944284900006,12.2,-10.483975472));
#296065=CARTESIAN_POINT('Ctrl Pts',(-1.69861565500006,12.2,-10.481975146));
#296066=CARTESIAN_POINT('Ctrl Pts',(-1.69779281100006,12.2,-10.479980323));
#296067=CARTESIAN_POINT('Ctrl Pts',(-1.69697431500006,12.2,-10.477991019));
#296068=CARTESIAN_POINT('Ctrl Pts',(-1.69616015900006,12.2,-10.476007249));
#296069=CARTESIAN_POINT('Ctrl Pts',(-1.69535034100006,12.2,-10.474029034));
#296070=CARTESIAN_POINT('Ctrl Pts',(-1.69454485500005,12.2,-10.47205639));
#296071=CARTESIAN_POINT('Ctrl Pts',(-1.69374369700006,12.2,-10.470089332));
#296072=CARTESIAN_POINT('Ctrl Pts',(-1.69294686200006,12.2,-10.468127881));
#296073=CARTESIAN_POINT('Ctrl Pts',(-1.69215434600006,12.2,-10.466172052));
#296074=CARTESIAN_POINT('Ctrl Pts',(-1.69136614300006,12.2,-10.464221864));
#296075=CARTESIAN_POINT('Ctrl Pts',(-1.69058224900006,12.2,-10.462277333));
#296076=CARTESIAN_POINT('Ctrl Pts',(-1.68980265900006,12.2,-10.460338479));
#296077=CARTESIAN_POINT('Ctrl Pts',(-1.68902736900006,12.2,-10.458405316));
#296078=CARTESIAN_POINT('Ctrl Pts',(-1.68825637300006,12.2,-10.456477865));
#296079=CARTESIAN_POINT('Ctrl Pts',(-1.68748966700006,12.2,-10.454556142));
#296080=CARTESIAN_POINT('Ctrl Pts',(-1.68672724500006,12.2,-10.452640166));
#296081=CARTESIAN_POINT('Ctrl Pts',(-1.68596910300006,12.2,-10.450729954));
#296082=CARTESIAN_POINT('Ctrl Pts',(-1.68521523600006,12.2,-10.448825525));
#296083=CARTESIAN_POINT('Ctrl Pts',(-1.68446563900006,12.2,-10.446926896));
#296084=CARTESIAN_POINT('Ctrl Pts',(-1.68372030600006,12.2,-10.445034085));
#296085=CARTESIAN_POINT('Ctrl Pts',(-1.68297923400006,12.2,-10.44314711));
#296086=CARTESIAN_POINT('Ctrl Pts',(-1.68224241500006,12.2,-10.44126599));
#296087=CARTESIAN_POINT('Ctrl Pts',(-1.68150984700006,12.2,-10.439390743));
#296088=CARTESIAN_POINT('Ctrl Pts',(-1.68078152300006,12.2,-10.437521386));
#296089=CARTESIAN_POINT('Ctrl Pts',(-1.68005743900005,12.2,-10.435657939));
#296090=CARTESIAN_POINT('Ctrl Pts',(-1.67933758800005,12.2,-10.433800421));
#296091=CARTESIAN_POINT('Ctrl Pts',(-1.67862196700006,12.2,-10.431948849));
#296092=CARTESIAN_POINT('Ctrl Pts',(-1.67791057000006,12.2,-10.430103241));
#296093=CARTESIAN_POINT('Ctrl Pts',(-1.67720339000006,12.2,-10.428263616));
#296094=CARTESIAN_POINT('Ctrl Pts',(-1.67650042400005,12.2,-10.426429993));
#296095=CARTESIAN_POINT('Ctrl Pts',(-1.67580166700006,12.2,-10.424602391));
#296096=CARTESIAN_POINT('Ctrl Pts',(-1.67510711100005,12.2,-10.422780829));
#296097=CARTESIAN_POINT('Ctrl Pts',(-1.67441675200006,12.2,-10.420965325));
#296098=CARTESIAN_POINT('Ctrl Pts',(-1.67373058500006,12.2,-10.419155897));
#296099=CARTESIAN_POINT('Ctrl Pts',(-1.67304860500006,12.2,-10.417352566));
#296100=CARTESIAN_POINT('Ctrl Pts',(-1.67237080500006,12.2,-10.41555535));
#296101=CARTESIAN_POINT('Ctrl Pts',(-1.67169718000005,12.2,-10.413764268));
#296102=CARTESIAN_POINT('Ctrl Pts',(-1.67102772500006,12.2,-10.411979339));
#296103=CARTESIAN_POINT('Ctrl Pts',(-1.67036243400006,12.2,-10.410200583));
#296104=CARTESIAN_POINT('Ctrl Pts',(-1.66970130200006,12.2,-10.408428019));
#296105=CARTESIAN_POINT('Ctrl Pts',(-1.66904432300006,12.2,-10.406661664));
#296106=CARTESIAN_POINT('Ctrl Pts',(-1.66839149100006,12.2,-10.404901541));
#296107=CARTESIAN_POINT('Ctrl Pts',(-1.66774280000005,12.2,-10.403147668));
#296108=CARTESIAN_POINT('Ctrl Pts',(-1.66709824500006,12.2,-10.401400063));
#296109=CARTESIAN_POINT('Ctrl Pts',(-1.66645782000006,12.2,-10.399658748));
#296110=CARTESIAN_POINT('Ctrl Pts',(-1.66582152000006,12.2,-10.397923741));
#296111=CARTESIAN_POINT('Ctrl Pts',(-1.66518933800006,12.2,-10.396195062));
#296112=CARTESIAN_POINT('Ctrl Pts',(-1.66456126800006,12.2,-10.394472732));
#296113=CARTESIAN_POINT('Ctrl Pts',(-1.66393730600006,12.2,-10.392756769));
#296114=CARTESIAN_POINT('Ctrl Pts',(-1.66331744300006,12.2,-10.391047193));
#296115=CARTESIAN_POINT('Ctrl Pts',(-1.66270167700006,12.2,-10.389344026));
#296116=CARTESIAN_POINT('Ctrl Pts',(-1.66208999800005,12.2,-10.387647286));
#296117=CARTESIAN_POINT('Ctrl Pts',(-1.66148240300006,12.2,-10.385956994));
#296118=CARTESIAN_POINT('Ctrl Pts',(-1.66087888400006,12.2,-10.38427317));
#296119=CARTESIAN_POINT('Ctrl Pts',(-1.66027943500006,12.2,-10.382595835));
#296120=CARTESIAN_POINT('Ctrl Pts',(-1.65968405200006,12.2,-10.380925008));
#296121=CARTESIAN_POINT('Ctrl Pts',(-1.65909272600006,12.2,-10.37926071));
#296122=CARTESIAN_POINT('Ctrl Pts',(-1.65850545200006,12.2,-10.377602961));
#296123=CARTESIAN_POINT('Ctrl Pts',(-1.65792222600006,12.2,-10.375951783));
#296124=CARTESIAN_POINT('Ctrl Pts',(-1.65734303700006,12.2,-10.374307195));
#296125=CARTESIAN_POINT('Ctrl Pts',(-1.65676788300006,12.2,-10.372669218));
#296126=CARTESIAN_POINT('Ctrl Pts',(-1.65619675600006,12.2,-10.371037873));
#296127=CARTESIAN_POINT('Ctrl Pts',(-1.65562964900006,12.2,-10.369413181));
#296128=CARTESIAN_POINT('Ctrl Pts',(-1.65506655700006,12.2,-10.367795164));
#296129=CARTESIAN_POINT('Ctrl Pts',(-1.65450747200006,12.2,-10.36618384));
#296130=CARTESIAN_POINT('Ctrl Pts',(-1.65395238800006,12.2,-10.364579233));
#296131=CARTESIAN_POINT('Ctrl Pts',(-1.65340130000006,12.2,-10.362981362));
#296132=CARTESIAN_POINT('Ctrl Pts',(-1.65285419900006,12.2,-10.361390249));
#296133=CARTESIAN_POINT('Ctrl Pts',(-1.65231108000006,12.2,-10.359805917));
#296134=CARTESIAN_POINT('Ctrl Pts',(-1.65177193600006,12.2,-10.358228384));
#296135=CARTESIAN_POINT('Ctrl Pts',(-1.65123676100006,12.2,-10.356657674));
#296136=CARTESIAN_POINT('Ctrl Pts',(-1.65070554700006,12.2,-10.355093807));
#296137=CARTESIAN_POINT('Ctrl Pts',(-1.65017828800006,12.2,-10.353536807));
#296138=CARTESIAN_POINT('Ctrl Pts',(-1.64965497700006,12.2,-10.351986691));
#296139=CARTESIAN_POINT('Ctrl Pts',(-1.64913560800006,12.2,-10.350443486));
#296140=CARTESIAN_POINT('Ctrl Pts',(-1.64862017200006,12.2,-10.348907211));
#296141=CARTESIAN_POINT('Ctrl Pts',(-1.64810866500006,12.2,-10.347377888));
#296142=CARTESIAN_POINT('Ctrl Pts',(-1.64760107800005,12.2,-10.34585554));
#296143=CARTESIAN_POINT('Ctrl Pts',(-1.64709740400005,12.2,-10.344340188));
#296144=CARTESIAN_POINT('Ctrl Pts',(-1.64659763700006,12.2,-10.342831854));
#296145=CARTESIAN_POINT('Ctrl Pts',(-1.64610177000006,12.2,-10.341330563));
#296146=CARTESIAN_POINT('Ctrl Pts',(-1.64560979500005,12.2,-10.339836333));
#296147=CARTESIAN_POINT('Ctrl Pts',(-1.64512170500006,12.2,-10.33834919));
#296148=CARTESIAN_POINT('Ctrl Pts',(-1.64463749400006,12.2,-10.336869154));
#296149=CARTESIAN_POINT('Ctrl Pts',(-1.64415715300006,12.2,-10.33539625));
#296150=CARTESIAN_POINT('Ctrl Pts',(-1.64368067600006,12.2,-10.333930498));
#296151=CARTESIAN_POINT('Ctrl Pts',(-1.64320805500005,12.2,-10.332471923));
#296152=CARTESIAN_POINT('Ctrl Pts',(-1.64273928400006,12.2,-10.331020547));
#296153=CARTESIAN_POINT('Ctrl Pts',(-1.64227435300006,12.2,-10.329576392));
#296154=CARTESIAN_POINT('Ctrl Pts',(-1.64181325800006,12.2,-10.328139482));
#296155=CARTESIAN_POINT('Ctrl Pts',(-1.64135598800006,12.2,-10.32670984));
#296156=CARTESIAN_POINT('Ctrl Pts',(-1.64090253900006,12.2,-10.325287489));
#296157=CARTESIAN_POINT('Ctrl Pts',(-1.64045290000006,12.2,-10.323872454));
#296158=CARTESIAN_POINT('Ctrl Pts',(-1.64000706600006,12.2,-10.322464755));
#296159=CARTESIAN_POINT('Ctrl Pts',(-1.63956502700006,12.2,-10.321064418));
#296160=CARTESIAN_POINT('Ctrl Pts',(-1.63912677800006,12.2,-10.319671466));
#296161=CARTESIAN_POINT('Ctrl Pts',(-1.63869231000006,12.2,-10.318285921));
#296162=CARTESIAN_POINT('Ctrl Pts',(-1.63826161500006,12.2,-10.316907809));
#296163=CARTESIAN_POINT('Ctrl Pts',(-1.63783468500006,12.2,-10.315537154));
#296164=CARTESIAN_POINT('Ctrl Pts',(-1.63741151300006,12.2,-10.314173978));
#296165=CARTESIAN_POINT('Ctrl Pts',(-1.63699208900006,12.2,-10.312818307));
#296166=CARTESIAN_POINT('Ctrl Pts',(-1.63657640900006,12.2,-10.311470164));
#296167=CARTESIAN_POINT('Ctrl Pts',(-1.63616446000006,12.2,-10.310129573));
#296168=CARTESIAN_POINT('Ctrl Pts',(-1.63575623900006,12.2,-10.308796558));
#296169=CARTESIAN_POINT('Ctrl Pts',(-1.63535173400006,12.2,-10.307471145));
#296170=CARTESIAN_POINT('Ctrl Pts',(-1.63495093900006,12.2,-10.306153358));
#296171=CARTESIAN_POINT('Ctrl Pts',(-1.63455384500006,12.2,-10.30484322));
#296172=CARTESIAN_POINT('Ctrl Pts',(-1.63416044300006,12.2,-10.303540757));
#296173=CARTESIAN_POINT('Ctrl Pts',(-1.63377072600006,12.2,-10.302245994));
#296174=CARTESIAN_POINT('Ctrl Pts',(-1.63338468600006,12.2,-10.300958957));
#296175=CARTESIAN_POINT('Ctrl Pts',(-1.63300231200005,12.2,-10.299679669));
#296176=CARTESIAN_POINT('Ctrl Pts',(-1.63262359900005,12.2,-10.298408156));
#296177=CARTESIAN_POINT('Ctrl Pts',(-1.63224853600005,12.2,-10.297144443));
#296178=CARTESIAN_POINT('Ctrl Pts',(-1.63187711600006,12.2,-10.295888554));
#296179=CARTESIAN_POINT('Ctrl Pts',(-1.63150933000006,12.2,-10.294640518));
#296180=CARTESIAN_POINT('Ctrl Pts',(-1.63114516900006,12.2,-10.293400358));
#296181=CARTESIAN_POINT('Ctrl Pts',(-1.63078462400006,12.2,-10.292168099));
#296182=CARTESIAN_POINT('Ctrl Pts',(-1.63042768700006,12.2,-10.290943769));
#296183=CARTESIAN_POINT('Ctrl Pts',(-1.63007434900006,12.2,-10.289727392));
#296184=CARTESIAN_POINT('Ctrl Pts',(-1.62972460000006,12.2,-10.288518995));
#296185=CARTESIAN_POINT('Ctrl Pts',(-1.62937843400006,12.2,-10.287318604));
#296186=CARTESIAN_POINT('Ctrl Pts',(-1.62903583800006,12.2,-10.286126246));
#296187=CARTESIAN_POINT('Ctrl Pts',(-1.62869680700006,12.2,-10.284941945));
#296188=CARTESIAN_POINT('Ctrl Pts',(-1.62836133000006,12.2,-10.283765729));
#296189=CARTESIAN_POINT('Ctrl Pts',(-1.62802939800006,12.2,-10.282597626));
#296190=CARTESIAN_POINT('Ctrl Pts',(-1.62770100100006,12.2,-10.281437659));
#296191=CARTESIAN_POINT('Ctrl Pts',(-1.62737613100005,12.2,-10.280285858));
#296192=CARTESIAN_POINT('Ctrl Pts',(-1.62705477800006,12.2,-10.279142249));
#296193=CARTESIAN_POINT('Ctrl Pts',(-1.62673693500006,12.2,-10.278006858));
#296194=CARTESIAN_POINT('Ctrl Pts',(-1.62642258900005,12.2,-10.276879714));
#296195=CARTESIAN_POINT('Ctrl Pts',(-1.62611173300005,12.2,-10.275760843));
#296196=CARTESIAN_POINT('Ctrl Pts',(-1.62580435500006,12.2,-10.274650272));
#296197=CARTESIAN_POINT('Ctrl Pts',(-1.62550044800006,12.2,-10.27354803));
#296198=CARTESIAN_POINT('Ctrl Pts',(-1.62520000300006,12.2,-10.272454143));
#296199=CARTESIAN_POINT('Ctrl Pts',(-1.62490300800005,12.2,-10.27136864));
#296200=CARTESIAN_POINT('Ctrl Pts',(-1.62460945300006,12.2,-10.270291548));
#296201=CARTESIAN_POINT('Ctrl Pts',(-1.62431933100006,12.2,-10.269222895));
#296202=CARTESIAN_POINT('Ctrl Pts',(-1.62403263000006,12.2,-10.268162711));
#296203=CARTESIAN_POINT('Ctrl Pts',(-1.62374934000006,12.2,-10.267111021));
#296204=CARTESIAN_POINT('Ctrl Pts',(-1.62346945200006,12.2,-10.266067857));
#296205=CARTESIAN_POINT('Ctrl Pts',(-1.62319295600006,12.2,-10.265033246));
#296206=CARTESIAN_POINT('Ctrl Pts',(-1.62291984100006,12.2,-10.264007214));
#296207=CARTESIAN_POINT('Ctrl Pts',(-1.62265009700006,12.2,-10.262989795));
#296208=CARTESIAN_POINT('Ctrl Pts',(-1.62238371500006,12.2,-10.261981014));
#296209=CARTESIAN_POINT('Ctrl Pts',(-1.62212068400006,12.2,-10.260980901));
#296210=CARTESIAN_POINT('Ctrl Pts',(-1.62186099300006,12.2,-10.259989485));
#296211=CARTESIAN_POINT('Ctrl Pts',(-1.62160463200005,12.2,-10.259006796));
#296212=CARTESIAN_POINT('Ctrl Pts',(-1.62135159100006,12.2,-10.258032864));
#296213=CARTESIAN_POINT('Ctrl Pts',(-1.62110185800006,12.2,-10.257067717));
#296214=CARTESIAN_POINT('Ctrl Pts',(-1.62085542500006,12.2,-10.256111386));
#296215=CARTESIAN_POINT('Ctrl Pts',(-1.62061227900006,12.2,-10.255163901));
#296216=CARTESIAN_POINT('Ctrl Pts',(-1.62037241000006,12.2,-10.254225291));
#296217=CARTESIAN_POINT('Ctrl Pts',(-1.62013580800005,12.2,-10.253295586));
#296218=CARTESIAN_POINT('Ctrl Pts',(-1.61990246100005,12.2,-10.252374817));
#296219=CARTESIAN_POINT('Ctrl Pts',(-1.61967235800006,12.2,-10.251463016));
#296220=CARTESIAN_POINT('Ctrl Pts',(-1.61944548900005,12.2,-10.250560211));
#296221=CARTESIAN_POINT('Ctrl Pts',(-1.61922313100006,12.2,-10.249671582));
#296222=CARTESIAN_POINT('Ctrl Pts',(-1.61904803300006,12.2,-10.248968851));
#296223=CARTESIAN_POINT('Ctrl Pts',(-1.61891844100006,12.2,-10.248447089));
#296224=CARTESIAN_POINT('Ctrl Pts',(-1.61883308400005,12.2,-10.248102703));
#296225=CARTESIAN_POINT('Ctrl Pts',(-1.61879118000006,12.2,-10.247933456));
#296226=CARTESIAN_POINT('Ctrl Pts',(-1.61879118000006,15.2,-10.247933456));
#296227=CARTESIAN_POINT('Ctrl Pts',(-1.61883308400005,15.2,-10.248102703));
#296228=CARTESIAN_POINT('Ctrl Pts',(-1.61891844100006,15.2,-10.248447089));
#296229=CARTESIAN_POINT('Ctrl Pts',(-1.61904803300006,15.2,-10.248968851));
#296230=CARTESIAN_POINT('Ctrl Pts',(-1.61922313100006,15.2,-10.249671582));
#296231=CARTESIAN_POINT('Ctrl Pts',(-1.61944548900005,15.2,-10.250560211));
#296232=CARTESIAN_POINT('Ctrl Pts',(-1.61967235800006,15.2,-10.251463016));
#296233=CARTESIAN_POINT('Ctrl Pts',(-1.61990246100005,15.2,-10.252374817));
#296234=CARTESIAN_POINT('Ctrl Pts',(-1.62013580800005,15.2,-10.253295586));
#296235=CARTESIAN_POINT('Ctrl Pts',(-1.62037241000006,15.2,-10.254225291));
#296236=CARTESIAN_POINT('Ctrl Pts',(-1.62061227900006,15.2,-10.255163901));
#296237=CARTESIAN_POINT('Ctrl Pts',(-1.62085542500006,15.2,-10.256111386));
#296238=CARTESIAN_POINT('Ctrl Pts',(-1.62110185800006,15.2,-10.257067717));
#296239=CARTESIAN_POINT('Ctrl Pts',(-1.62135159100006,15.2,-10.258032864));
#296240=CARTESIAN_POINT('Ctrl Pts',(-1.62160463200005,15.2,-10.259006796));
#296241=CARTESIAN_POINT('Ctrl Pts',(-1.62186099300006,15.2,-10.259989485));
#296242=CARTESIAN_POINT('Ctrl Pts',(-1.62212068400006,15.2,-10.260980901));
#296243=CARTESIAN_POINT('Ctrl Pts',(-1.62238371500006,15.2,-10.261981014));
#296244=CARTESIAN_POINT('Ctrl Pts',(-1.62265009700006,15.2,-10.262989795));
#296245=CARTESIAN_POINT('Ctrl Pts',(-1.62291984100006,15.2,-10.264007214));
#296246=CARTESIAN_POINT('Ctrl Pts',(-1.62319295600006,15.2,-10.265033246));
#296247=CARTESIAN_POINT('Ctrl Pts',(-1.62346945200006,15.2,-10.266067857));
#296248=CARTESIAN_POINT('Ctrl Pts',(-1.62374934000006,15.2,-10.267111021));
#296249=CARTESIAN_POINT('Ctrl Pts',(-1.62403263000006,15.2,-10.268162711));
#296250=CARTESIAN_POINT('Ctrl Pts',(-1.62431933100006,15.2,-10.269222895));
#296251=CARTESIAN_POINT('Ctrl Pts',(-1.62460945300006,15.2,-10.270291548));
#296252=CARTESIAN_POINT('Ctrl Pts',(-1.62490300800005,15.2,-10.27136864));
#296253=CARTESIAN_POINT('Ctrl Pts',(-1.62520000300006,15.2,-10.272454143));
#296254=CARTESIAN_POINT('Ctrl Pts',(-1.62550044800006,15.2,-10.27354803));
#296255=CARTESIAN_POINT('Ctrl Pts',(-1.62580435500006,15.2,-10.274650272));
#296256=CARTESIAN_POINT('Ctrl Pts',(-1.62611173300005,15.2,-10.275760843));
#296257=CARTESIAN_POINT('Ctrl Pts',(-1.62642258900005,15.2,-10.276879714));
#296258=CARTESIAN_POINT('Ctrl Pts',(-1.62673693500006,15.2,-10.278006858));
#296259=CARTESIAN_POINT('Ctrl Pts',(-1.62705477800006,15.2,-10.279142249));
#296260=CARTESIAN_POINT('Ctrl Pts',(-1.62737613100005,15.2,-10.280285858));
#296261=CARTESIAN_POINT('Ctrl Pts',(-1.62770100100006,15.2,-10.281437659));
#296262=CARTESIAN_POINT('Ctrl Pts',(-1.62802939800006,15.2,-10.282597626));
#296263=CARTESIAN_POINT('Ctrl Pts',(-1.62836133000006,15.2,-10.283765729));
#296264=CARTESIAN_POINT('Ctrl Pts',(-1.62869680700006,15.2,-10.284941945));
#296265=CARTESIAN_POINT('Ctrl Pts',(-1.62903583800006,15.2,-10.286126246));
#296266=CARTESIAN_POINT('Ctrl Pts',(-1.62937843400006,15.2,-10.287318604));
#296267=CARTESIAN_POINT('Ctrl Pts',(-1.62972460000006,15.2,-10.288518995));
#296268=CARTESIAN_POINT('Ctrl Pts',(-1.63007434900006,15.2,-10.289727392));
#296269=CARTESIAN_POINT('Ctrl Pts',(-1.63042768700006,15.2,-10.290943769));
#296270=CARTESIAN_POINT('Ctrl Pts',(-1.63078462400006,15.2,-10.292168099));
#296271=CARTESIAN_POINT('Ctrl Pts',(-1.63114516900006,15.2,-10.293400358));
#296272=CARTESIAN_POINT('Ctrl Pts',(-1.63150933000006,15.2,-10.294640518));
#296273=CARTESIAN_POINT('Ctrl Pts',(-1.63187711600006,15.2,-10.295888554));
#296274=CARTESIAN_POINT('Ctrl Pts',(-1.63224853600005,15.2,-10.297144443));
#296275=CARTESIAN_POINT('Ctrl Pts',(-1.63262359900005,15.2,-10.298408156));
#296276=CARTESIAN_POINT('Ctrl Pts',(-1.63300231200005,15.2,-10.299679669));
#296277=CARTESIAN_POINT('Ctrl Pts',(-1.63338468600006,15.2,-10.300958957));
#296278=CARTESIAN_POINT('Ctrl Pts',(-1.63377072600006,15.2,-10.302245994));
#296279=CARTESIAN_POINT('Ctrl Pts',(-1.63416044300006,15.2,-10.303540757));
#296280=CARTESIAN_POINT('Ctrl Pts',(-1.63455384500006,15.2,-10.30484322));
#296281=CARTESIAN_POINT('Ctrl Pts',(-1.63495093900006,15.2,-10.306153358));
#296282=CARTESIAN_POINT('Ctrl Pts',(-1.63535173400006,15.2,-10.307471145));
#296283=CARTESIAN_POINT('Ctrl Pts',(-1.63575623900006,15.2,-10.308796558));
#296284=CARTESIAN_POINT('Ctrl Pts',(-1.63616446000006,15.2,-10.310129573));
#296285=CARTESIAN_POINT('Ctrl Pts',(-1.63657640900006,15.2,-10.311470164));
#296286=CARTESIAN_POINT('Ctrl Pts',(-1.63699208900006,15.2,-10.312818307));
#296287=CARTESIAN_POINT('Ctrl Pts',(-1.63741151300006,15.2,-10.314173978));
#296288=CARTESIAN_POINT('Ctrl Pts',(-1.63783468500006,15.2,-10.315537154));
#296289=CARTESIAN_POINT('Ctrl Pts',(-1.63826161500006,15.2,-10.316907809));
#296290=CARTESIAN_POINT('Ctrl Pts',(-1.63869231000006,15.2,-10.318285921));
#296291=CARTESIAN_POINT('Ctrl Pts',(-1.63912677800006,15.2,-10.319671466));
#296292=CARTESIAN_POINT('Ctrl Pts',(-1.63956502700006,15.2,-10.321064418));
#296293=CARTESIAN_POINT('Ctrl Pts',(-1.64000706600006,15.2,-10.322464755));
#296294=CARTESIAN_POINT('Ctrl Pts',(-1.64045290000006,15.2,-10.323872454));
#296295=CARTESIAN_POINT('Ctrl Pts',(-1.64090253900006,15.2,-10.325287489));
#296296=CARTESIAN_POINT('Ctrl Pts',(-1.64135598800006,15.2,-10.32670984));
#296297=CARTESIAN_POINT('Ctrl Pts',(-1.64181325800006,15.2,-10.328139482));
#296298=CARTESIAN_POINT('Ctrl Pts',(-1.64227435300006,15.2,-10.329576392));
#296299=CARTESIAN_POINT('Ctrl Pts',(-1.64273928400006,15.2,-10.331020547));
#296300=CARTESIAN_POINT('Ctrl Pts',(-1.64320805500005,15.2,-10.332471923));
#296301=CARTESIAN_POINT('Ctrl Pts',(-1.64368067600006,15.2,-10.333930498));
#296302=CARTESIAN_POINT('Ctrl Pts',(-1.64415715300006,15.2,-10.33539625));
#296303=CARTESIAN_POINT('Ctrl Pts',(-1.64463749400006,15.2,-10.336869154));
#296304=CARTESIAN_POINT('Ctrl Pts',(-1.64512170500006,15.2,-10.33834919));
#296305=CARTESIAN_POINT('Ctrl Pts',(-1.64560979500005,15.2,-10.339836333));
#296306=CARTESIAN_POINT('Ctrl Pts',(-1.64610177000006,15.2,-10.341330563));
#296307=CARTESIAN_POINT('Ctrl Pts',(-1.64659763700006,15.2,-10.342831854));
#296308=CARTESIAN_POINT('Ctrl Pts',(-1.64709740400005,15.2,-10.344340188));
#296309=CARTESIAN_POINT('Ctrl Pts',(-1.64760107800005,15.2,-10.34585554));
#296310=CARTESIAN_POINT('Ctrl Pts',(-1.64810866500006,15.2,-10.347377888));
#296311=CARTESIAN_POINT('Ctrl Pts',(-1.64862017200006,15.2,-10.348907211));
#296312=CARTESIAN_POINT('Ctrl Pts',(-1.64913560800006,15.2,-10.350443486));
#296313=CARTESIAN_POINT('Ctrl Pts',(-1.64965497700006,15.2,-10.351986691));
#296314=CARTESIAN_POINT('Ctrl Pts',(-1.65017828800006,15.2,-10.353536807));
#296315=CARTESIAN_POINT('Ctrl Pts',(-1.65070554700006,15.2,-10.355093807));
#296316=CARTESIAN_POINT('Ctrl Pts',(-1.65123676100006,15.2,-10.356657674));
#296317=CARTESIAN_POINT('Ctrl Pts',(-1.65177193600006,15.2,-10.358228384));
#296318=CARTESIAN_POINT('Ctrl Pts',(-1.65231108000006,15.2,-10.359805917));
#296319=CARTESIAN_POINT('Ctrl Pts',(-1.65285419900006,15.2,-10.361390249));
#296320=CARTESIAN_POINT('Ctrl Pts',(-1.65340130000006,15.2,-10.362981362));
#296321=CARTESIAN_POINT('Ctrl Pts',(-1.65395238800006,15.2,-10.364579233));
#296322=CARTESIAN_POINT('Ctrl Pts',(-1.65450747200006,15.2,-10.36618384));
#296323=CARTESIAN_POINT('Ctrl Pts',(-1.65506655700006,15.2,-10.367795164));
#296324=CARTESIAN_POINT('Ctrl Pts',(-1.65562964900006,15.2,-10.369413181));
#296325=CARTESIAN_POINT('Ctrl Pts',(-1.65619675600006,15.2,-10.371037873));
#296326=CARTESIAN_POINT('Ctrl Pts',(-1.65676788300006,15.2,-10.372669218));
#296327=CARTESIAN_POINT('Ctrl Pts',(-1.65734303700006,15.2,-10.374307195));
#296328=CARTESIAN_POINT('Ctrl Pts',(-1.65792222600006,15.2,-10.375951783));
#296329=CARTESIAN_POINT('Ctrl Pts',(-1.65850545200006,15.2,-10.377602961));
#296330=CARTESIAN_POINT('Ctrl Pts',(-1.65909272600006,15.2,-10.37926071));
#296331=CARTESIAN_POINT('Ctrl Pts',(-1.65968405200006,15.2,-10.380925008));
#296332=CARTESIAN_POINT('Ctrl Pts',(-1.66027943500006,15.2,-10.382595835));
#296333=CARTESIAN_POINT('Ctrl Pts',(-1.66087888400006,15.2,-10.38427317));
#296334=CARTESIAN_POINT('Ctrl Pts',(-1.66148240300006,15.2,-10.385956994));
#296335=CARTESIAN_POINT('Ctrl Pts',(-1.66208999800005,15.2,-10.387647286));
#296336=CARTESIAN_POINT('Ctrl Pts',(-1.66270167700006,15.2,-10.389344026));
#296337=CARTESIAN_POINT('Ctrl Pts',(-1.66331744300006,15.2,-10.391047193));
#296338=CARTESIAN_POINT('Ctrl Pts',(-1.66393730600006,15.2,-10.392756769));
#296339=CARTESIAN_POINT('Ctrl Pts',(-1.66456126800006,15.2,-10.394472732));
#296340=CARTESIAN_POINT('Ctrl Pts',(-1.66518933800006,15.2,-10.396195062));
#296341=CARTESIAN_POINT('Ctrl Pts',(-1.66582152000006,15.2,-10.397923741));
#296342=CARTESIAN_POINT('Ctrl Pts',(-1.66645782000006,15.2,-10.399658748));
#296343=CARTESIAN_POINT('Ctrl Pts',(-1.66709824500006,15.2,-10.401400063));
#296344=CARTESIAN_POINT('Ctrl Pts',(-1.66774280000005,15.2,-10.403147668));
#296345=CARTESIAN_POINT('Ctrl Pts',(-1.66839149100006,15.2,-10.404901541));
#296346=CARTESIAN_POINT('Ctrl Pts',(-1.66904432300006,15.2,-10.406661664));
#296347=CARTESIAN_POINT('Ctrl Pts',(-1.66970130200006,15.2,-10.408428019));
#296348=CARTESIAN_POINT('Ctrl Pts',(-1.67036243400006,15.2,-10.410200583));
#296349=CARTESIAN_POINT('Ctrl Pts',(-1.67102772500006,15.2,-10.411979339));
#296350=CARTESIAN_POINT('Ctrl Pts',(-1.67169718000005,15.2,-10.413764268));
#296351=CARTESIAN_POINT('Ctrl Pts',(-1.67237080500006,15.2,-10.41555535));
#296352=CARTESIAN_POINT('Ctrl Pts',(-1.67304860500006,15.2,-10.417352566));
#296353=CARTESIAN_POINT('Ctrl Pts',(-1.67373058500006,15.2,-10.419155897));
#296354=CARTESIAN_POINT('Ctrl Pts',(-1.67441675200006,15.2,-10.420965325));
#296355=CARTESIAN_POINT('Ctrl Pts',(-1.67510711100005,15.2,-10.422780829));
#296356=CARTESIAN_POINT('Ctrl Pts',(-1.67580166700006,15.2,-10.424602391));
#296357=CARTESIAN_POINT('Ctrl Pts',(-1.67650042400005,15.2,-10.426429993));
#296358=CARTESIAN_POINT('Ctrl Pts',(-1.67720339000006,15.2,-10.428263616));
#296359=CARTESIAN_POINT('Ctrl Pts',(-1.67791057000006,15.2,-10.430103241));
#296360=CARTESIAN_POINT('Ctrl Pts',(-1.67862196700006,15.2,-10.431948849));
#296361=CARTESIAN_POINT('Ctrl Pts',(-1.67933758800005,15.2,-10.433800421));
#296362=CARTESIAN_POINT('Ctrl Pts',(-1.68005743900005,15.2,-10.435657939));
#296363=CARTESIAN_POINT('Ctrl Pts',(-1.68078152300006,15.2,-10.437521386));
#296364=CARTESIAN_POINT('Ctrl Pts',(-1.68150984700006,15.2,-10.439390743));
#296365=CARTESIAN_POINT('Ctrl Pts',(-1.68224241500006,15.2,-10.44126599));
#296366=CARTESIAN_POINT('Ctrl Pts',(-1.68297923400006,15.2,-10.44314711));
#296367=CARTESIAN_POINT('Ctrl Pts',(-1.68372030600006,15.2,-10.445034085));
#296368=CARTESIAN_POINT('Ctrl Pts',(-1.68446563900006,15.2,-10.446926896));
#296369=CARTESIAN_POINT('Ctrl Pts',(-1.68521523600006,15.2,-10.448825525));
#296370=CARTESIAN_POINT('Ctrl Pts',(-1.68596910300006,15.2,-10.450729954));
#296371=CARTESIAN_POINT('Ctrl Pts',(-1.68672724500006,15.2,-10.452640166));
#296372=CARTESIAN_POINT('Ctrl Pts',(-1.68748966700006,15.2,-10.454556142));
#296373=CARTESIAN_POINT('Ctrl Pts',(-1.68825637300006,15.2,-10.456477865));
#296374=CARTESIAN_POINT('Ctrl Pts',(-1.68902736900006,15.2,-10.458405316));
#296375=CARTESIAN_POINT('Ctrl Pts',(-1.68980265900006,15.2,-10.460338479));
#296376=CARTESIAN_POINT('Ctrl Pts',(-1.69058224900006,15.2,-10.462277333));
#296377=CARTESIAN_POINT('Ctrl Pts',(-1.69136614300006,15.2,-10.464221864));
#296378=CARTESIAN_POINT('Ctrl Pts',(-1.69215434600006,15.2,-10.466172052));
#296379=CARTESIAN_POINT('Ctrl Pts',(-1.69294686200006,15.2,-10.468127881));
#296380=CARTESIAN_POINT('Ctrl Pts',(-1.69374369700006,15.2,-10.470089332));
#296381=CARTESIAN_POINT('Ctrl Pts',(-1.69454485500005,15.2,-10.47205639));
#296382=CARTESIAN_POINT('Ctrl Pts',(-1.69535034100006,15.2,-10.474029034));
#296383=CARTESIAN_POINT('Ctrl Pts',(-1.69616015900006,15.2,-10.476007249));
#296384=CARTESIAN_POINT('Ctrl Pts',(-1.69697431500006,15.2,-10.477991019));
#296385=CARTESIAN_POINT('Ctrl Pts',(-1.69779281100006,15.2,-10.479980323));
#296386=CARTESIAN_POINT('Ctrl Pts',(-1.69861565500006,15.2,-10.481975146));
#296387=CARTESIAN_POINT('Ctrl Pts',(-1.69944284900006,15.2,-10.483975472));
#296388=CARTESIAN_POINT('Ctrl Pts',(-1.70027439800006,15.2,-10.485981281));
#296389=CARTESIAN_POINT('Ctrl Pts',(-1.70111030700005,15.2,-10.487992559));
#296390=CARTESIAN_POINT('Ctrl Pts',(-1.70195058100005,15.2,-10.490009287));
#296391=CARTESIAN_POINT('Ctrl Pts',(-1.70279522300006,15.2,-10.492031449));
#296392=CARTESIAN_POINT('Ctrl Pts',(-1.70364423900006,15.2,-10.494059027));
#296393=CARTESIAN_POINT('Ctrl Pts',(-1.70449763200006,15.2,-10.496092006));
#296394=CARTESIAN_POINT('Ctrl Pts',(-1.70535540700006,15.2,-10.498130368));
#296395=CARTESIAN_POINT('Ctrl Pts',(-1.70621756900006,15.2,-10.500174096));
#296396=CARTESIAN_POINT('Ctrl Pts',(-1.70708412100006,15.2,-10.502223174));
#296397=CARTESIAN_POINT('Ctrl Pts',(-1.70795506800005,15.2,-10.504277584));
#296398=CARTESIAN_POINT('Ctrl Pts',(-1.70883041500006,15.2,-10.506337312));
#296399=CARTESIAN_POINT('Ctrl Pts',(-1.70971016400005,15.2,-10.50840234));
#296400=CARTESIAN_POINT('Ctrl Pts',(-1.71059432200006,15.2,-10.510472651));
#296401=CARTESIAN_POINT('Ctrl Pts',(-1.71148289100006,15.2,-10.512548228));
#296402=CARTESIAN_POINT('Ctrl Pts',(-1.71237587800006,15.2,-10.514629056));
#296403=CARTESIAN_POINT('Ctrl Pts',(-1.71327328300006,15.2,-10.516715119));
#296404=CARTESIAN_POINT('Ctrl Pts',(-1.71417511300006,15.2,-10.5188064));
#296405=CARTESIAN_POINT('Ctrl Pts',(-1.71508137200005,15.2,-10.520902882));
#296406=CARTESIAN_POINT('Ctrl Pts',(-1.71599206400006,15.2,-10.523004549));
#296407=CARTESIAN_POINT('Ctrl Pts',(-1.71690719200006,15.2,-10.525111386));
#296408=CARTESIAN_POINT('Ctrl Pts',(-1.71782676200006,15.2,-10.527223376));
#296409=CARTESIAN_POINT('Ctrl Pts',(-1.71875077600005,15.2,-10.529340504));
#296410=CARTESIAN_POINT('Ctrl Pts',(-1.71967923800006,15.2,-10.531462752));
#296411=CARTESIAN_POINT('Ctrl Pts',(-1.72061215300006,15.2,-10.533590105));
#296412=CARTESIAN_POINT('Ctrl Pts',(-1.72154952600006,15.2,-10.535722547));
#296413=CARTESIAN_POINT('Ctrl Pts',(-1.72249135800006,15.2,-10.537860062));
#296414=CARTESIAN_POINT('Ctrl Pts',(-1.72343765400006,15.2,-10.540002635));
#296415=CARTESIAN_POINT('Ctrl Pts',(-1.72438842000005,15.2,-10.542150249));
#296416=CARTESIAN_POINT('Ctrl Pts',(-1.72534365800006,15.2,-10.544302889));
#296417=CARTESIAN_POINT('Ctrl Pts',(-1.72630337200005,15.2,-10.546460538));
#296418=CARTESIAN_POINT('Ctrl Pts',(-1.72726756600006,15.2,-10.548623183));
#296419=CARTESIAN_POINT('Ctrl Pts',(-1.72823624300006,15.2,-10.550790805));
#296420=CARTESIAN_POINT('Ctrl Pts',(-1.72920940800006,15.2,-10.552963391));
#296421=CARTESIAN_POINT('Ctrl Pts',(-1.73018706500006,15.2,-10.555140925));
#296422=CARTESIAN_POINT('Ctrl Pts',(-1.73116921600006,15.2,-10.55732339));
#296423=CARTESIAN_POINT('Ctrl Pts',(-1.73215586600006,15.2,-10.559510773));
#296424=CARTESIAN_POINT('Ctrl Pts',(-1.73314701900006,15.2,-10.561703056));
#296425=CARTESIAN_POINT('Ctrl Pts',(-1.73414267600006,15.2,-10.563900224));
#296426=CARTESIAN_POINT('Ctrl Pts',(-1.73514284500006,15.2,-10.566102263));
#296427=CARTESIAN_POINT('Ctrl Pts',(-1.73614752700006,15.2,-10.568309157));
#296428=CARTESIAN_POINT('Ctrl Pts',(-1.73715672500005,15.2,-10.570520891));
#296429=CARTESIAN_POINT('Ctrl Pts',(-1.73817044300006,15.2,-10.572737449));
#296430=CARTESIAN_POINT('Ctrl Pts',(-1.73918868600006,15.2,-10.574958817));
#296431=CARTESIAN_POINT('Ctrl Pts',(-1.74021145800005,15.2,-10.577184979));
#296432=CARTESIAN_POINT('Ctrl Pts',(-1.74123875900006,15.2,-10.57941592));
#296433=CARTESIAN_POINT('Ctrl Pts',(-1.74227059600006,15.2,-10.581651626));
#296434=CARTESIAN_POINT('Ctrl Pts',(-1.74330697100005,15.2,-10.58389208));
#296435=CARTESIAN_POINT('Ctrl Pts',(-1.74434788700006,15.2,-10.586137267));
#296436=CARTESIAN_POINT('Ctrl Pts',(-1.74539334800006,15.2,-10.588387175));
#296437=CARTESIAN_POINT('Ctrl Pts',(-1.74644335700005,15.2,-10.590641786));
#296438=CARTESIAN_POINT('Ctrl Pts',(-1.74749792000006,15.2,-10.592901087));
#296439=CARTESIAN_POINT('Ctrl Pts',(-1.74855703600006,15.2,-10.595165063));
#296440=CARTESIAN_POINT('Ctrl Pts',(-1.74962071200006,15.2,-10.597433698));
#296441=CARTESIAN_POINT('Ctrl Pts',(-1.75068894900006,15.2,-10.599706978));
#296442=CARTESIAN_POINT('Ctrl Pts',(-1.75176175100006,15.2,-10.601984888));
#296443=CARTESIAN_POINT('Ctrl Pts',(-1.75283912300006,15.2,-10.604267414));
#296444=CARTESIAN_POINT('Ctrl Pts',(-1.75392106600006,15.2,-10.60655454));
#296445=CARTESIAN_POINT('Ctrl Pts',(-1.75500758400006,15.2,-10.608846253));
#296446=CARTESIAN_POINT('Ctrl Pts',(-1.75609868000006,15.2,-10.611142538));
#296447=CARTESIAN_POINT('Ctrl Pts',(-1.75719435900006,15.2,-10.61344338));
#296448=CARTESIAN_POINT('Ctrl Pts',(-1.75829462200006,15.2,-10.615748764));
#296449=CARTESIAN_POINT('Ctrl Pts',(-1.75939947300006,15.2,-10.618058678));
#296450=CARTESIAN_POINT('Ctrl Pts',(-1.76050891600006,15.2,-10.620373104));
#296451=CARTESIAN_POINT('Ctrl Pts',(-1.76162295200006,15.2,-10.622692031));
#296452=CARTESIAN_POINT('Ctrl Pts',(-1.76274158600006,15.2,-10.625015442));
#296453=CARTESIAN_POINT('Ctrl Pts',(-1.76386482100006,15.2,-10.627343324));
#296454=CARTESIAN_POINT('Ctrl Pts',(-1.76499265900006,15.2,-10.629675663));
#296455=CARTESIAN_POINT('Ctrl Pts',(-1.76612510400005,15.2,-10.632012444));
#296456=CARTESIAN_POINT('Ctrl Pts',(-1.76726215900006,15.2,-10.634353653));
#296457=CARTESIAN_POINT('Ctrl Pts',(-1.76840382600005,15.2,-10.636699276));
#296458=CARTESIAN_POINT('Ctrl Pts',(-1.76955010900006,15.2,-10.639049299));
#296459=CARTESIAN_POINT('Ctrl Pts',(-1.77070101200006,15.2,-10.641403708));
#296460=CARTESIAN_POINT('Ctrl Pts',(-1.77185653500006,15.2,-10.643762488));
#296461=CARTESIAN_POINT('Ctrl Pts',(-1.77301668500006,15.2,-10.646125627));
#296462=CARTESIAN_POINT('Ctrl Pts',(-1.77418146100006,15.2,-10.648493108));
#296463=CARTESIAN_POINT('Ctrl Pts',(-1.77535086900006,15.2,-10.65086492));
#296464=CARTESIAN_POINT('Ctrl Pts',(-1.77652491000006,15.2,-10.653241047));
#296465=CARTESIAN_POINT('Ctrl Pts',(-1.77770358700006,15.2,-10.655621476));
#296466=CARTESIAN_POINT('Ctrl Pts',(-1.77888690400006,15.2,-10.658006194));
#296467=CARTESIAN_POINT('Ctrl Pts',(-1.78007486300006,15.2,-10.660395184));
#296468=CARTESIAN_POINT('Ctrl Pts',(-1.78126746700006,15.2,-10.662788437));
#296469=CARTESIAN_POINT('Ctrl Pts',(-1.78246472000006,15.2,-10.665185935));
#296470=CARTESIAN_POINT('Ctrl Pts',(-1.78366662300005,15.2,-10.667587667));
#296471=CARTESIAN_POINT('Ctrl Pts',(-1.78487317800006,15.2,-10.669993617));
#296472=CARTESIAN_POINT('Ctrl Pts',(-1.78608439100006,15.2,-10.672403774));
#296473=CARTESIAN_POINT('Ctrl Pts',(-1.78730026300005,15.2,-10.674818122));
#296474=CARTESIAN_POINT('Ctrl Pts',(-1.78852079600006,15.2,-10.677236648));
#296475=CARTESIAN_POINT('Ctrl Pts',(-1.78974599400005,15.2,-10.67965934));
#296476=CARTESIAN_POINT('Ctrl Pts',(-1.79097586000006,15.2,-10.682086183));
#296477=CARTESIAN_POINT('Ctrl Pts',(-1.79221039500006,15.2,-10.684517164));
#296478=CARTESIAN_POINT('Ctrl Pts',(-1.79344960300006,15.2,-10.686952269));
#296479=CARTESIAN_POINT('Ctrl Pts',(-1.79469348600006,15.2,-10.689391486));
#296480=CARTESIAN_POINT('Ctrl Pts',(-1.79594204700006,15.2,-10.691834799));
#296481=CARTESIAN_POINT('Ctrl Pts',(-1.79719528800006,15.2,-10.694282196));
#296482=CARTESIAN_POINT('Ctrl Pts',(-1.79845321300005,15.2,-10.696733666));
#296483=CARTESIAN_POINT('Ctrl Pts',(-1.79971582300006,15.2,-10.699189192));
#296484=CARTESIAN_POINT('Ctrl Pts',(-1.80098312100006,15.2,-10.701648762));
#296485=CARTESIAN_POINT('Ctrl Pts',(-1.80225511100006,15.2,-10.704112363));
#296486=CARTESIAN_POINT('Ctrl Pts',(-1.80353179300006,15.2,-10.706579983));
#296487=CARTESIAN_POINT('Ctrl Pts',(-1.80481317200006,15.2,-10.709051608));
#296488=CARTESIAN_POINT('Ctrl Pts',(-1.80609924900006,15.2,-10.711527223));
#296489=CARTESIAN_POINT('Ctrl Pts',(-1.80739002700005,15.2,-10.714006817));
#296490=CARTESIAN_POINT('Ctrl Pts',(-1.80868550800006,15.2,-10.716490376));
#296491=CARTESIAN_POINT('Ctrl Pts',(-1.80998569500006,15.2,-10.718977888));
#296492=CARTESIAN_POINT('Ctrl Pts',(-1.81129059100006,15.2,-10.721469338));
#296493=CARTESIAN_POINT('Ctrl Pts',(-1.81260019800006,15.2,-10.723964715));
#296494=CARTESIAN_POINT('Ctrl Pts',(-1.81391451700006,15.2,-10.726464005));
#296495=CARTESIAN_POINT('Ctrl Pts',(-1.81523355200006,15.2,-10.728967196));
#296496=CARTESIAN_POINT('Ctrl Pts',(-1.81655730500006,15.2,-10.731474274));
#296497=CARTESIAN_POINT('Ctrl Pts',(-1.81788577800006,15.2,-10.733985227));
#296498=CARTESIAN_POINT('Ctrl Pts',(-1.81921897500006,15.2,-10.73650004));
#296499=CARTESIAN_POINT('Ctrl Pts',(-1.82055689600006,15.2,-10.739018703));
#296500=CARTESIAN_POINT('Ctrl Pts',(-1.82189954400006,15.2,-10.741541203));
#296501=CARTESIAN_POINT('Ctrl Pts',(-1.82324692200006,15.2,-10.744067526));
#296502=CARTESIAN_POINT('Ctrl Pts',(-1.82459903200006,15.2,-10.746597658));
#296503=CARTESIAN_POINT('Ctrl Pts',(-1.82595587600006,15.2,-10.749131589));
#296504=CARTESIAN_POINT('Ctrl Pts',(-1.82731745700006,15.2,-10.751669306));
#296505=CARTESIAN_POINT('Ctrl Pts',(-1.82868377600006,15.2,-10.754210794));
#296506=CARTESIAN_POINT('Ctrl Pts',(-1.83005483700006,15.2,-10.756756043));
#296507=CARTESIAN_POINT('Ctrl Pts',(-1.83143064100005,15.2,-10.759305039));
#296508=CARTESIAN_POINT('Ctrl Pts',(-1.83281119000006,15.2,-10.76185777));
#296509=CARTESIAN_POINT('Ctrl Pts',(-1.83419648600006,15.2,-10.764414223));
#296510=CARTESIAN_POINT('Ctrl Pts',(-1.83558653300006,15.2,-10.766974386));
#296511=CARTESIAN_POINT('Ctrl Pts',(-1.83698133100005,15.2,-10.769538245));
#296512=CARTESIAN_POINT('Ctrl Pts',(-1.83838088300006,15.2,-10.77210579));
#296513=CARTESIAN_POINT('Ctrl Pts',(-1.83978519200006,15.2,-10.774677008));
#296514=CARTESIAN_POINT('Ctrl Pts',(-1.84119425800006,15.2,-10.777251885));
#296515=CARTESIAN_POINT('Ctrl Pts',(-1.84260808600006,15.2,-10.77983041));
#296516=CARTESIAN_POINT('Ctrl Pts',(-1.84402667500006,15.2,-10.78241257));
#296517=CARTESIAN_POINT('Ctrl Pts',(-1.84545003000005,15.2,-10.784998353));
#296518=CARTESIAN_POINT('Ctrl Pts',(-1.84687815100005,15.2,-10.787587746));
#296519=CARTESIAN_POINT('Ctrl Pts',(-1.84831104100006,15.2,-10.790180739));
#296520=CARTESIAN_POINT('Ctrl Pts',(-1.84974870200006,15.2,-10.792777317));
#296521=CARTESIAN_POINT('Ctrl Pts',(-1.85119113400006,15.2,-10.795377469));
#296522=CARTESIAN_POINT('Ctrl Pts',(-1.85263834300006,15.2,-10.797981184));
#296523=CARTESIAN_POINT('Ctrl Pts',(-1.85409032800006,15.2,-10.800588447));
#296524=CARTESIAN_POINT('Ctrl Pts',(-1.85554709100006,15.2,-10.803199248));
#296525=CARTESIAN_POINT('Ctrl Pts',(-1.85700863500006,15.2,-10.805813575));
#296526=CARTESIAN_POINT('Ctrl Pts',(-1.85847496200006,15.2,-10.808431414));
#296527=CARTESIAN_POINT('Ctrl Pts',(-1.85994607300006,15.2,-10.811052755));
#296528=CARTESIAN_POINT('Ctrl Pts',(-1.86142197200006,15.2,-10.813677586));
#296529=CARTESIAN_POINT('Ctrl Pts',(-1.86290265800006,15.2,-10.816305894));
#296530=CARTESIAN_POINT('Ctrl Pts',(-1.86438813500006,15.2,-10.818937666));
#296531=CARTESIAN_POINT('Ctrl Pts',(-1.86587840400006,15.2,-10.821572893));
#296532=CARTESIAN_POINT('Ctrl Pts',(-1.86737346700005,15.2,-10.82421156));
#296533=CARTESIAN_POINT('Ctrl Pts',(-1.86887332500006,15.2,-10.826853656));
#296534=CARTESIAN_POINT('Ctrl Pts',(-1.87037798200006,15.2,-10.829499171));
#296535=CARTESIAN_POINT('Ctrl Pts',(-1.87188743800006,15.2,-10.832148091));
#296536=CARTESIAN_POINT('Ctrl Pts',(-1.87340169600006,15.2,-10.834800405));
#296537=CARTESIAN_POINT('Ctrl Pts',(-1.87492075700006,15.2,-10.837456101));
#296538=CARTESIAN_POINT('Ctrl Pts',(-1.87644462200006,15.2,-10.840115167));
#296539=CARTESIAN_POINT('Ctrl Pts',(-1.87797329500006,15.2,-10.842777593));
#296540=CARTESIAN_POINT('Ctrl Pts',(-1.87950677700006,15.2,-10.845443365));
#296541=CARTESIAN_POINT('Ctrl Pts',(-1.88104506800005,15.2,-10.848112472));
#296542=CARTESIAN_POINT('Ctrl Pts',(-1.88258817100006,15.2,-10.850784903));
#296543=CARTESIAN_POINT('Ctrl Pts',(-1.88413608800006,15.2,-10.853460644));
#296544=CARTESIAN_POINT('Ctrl Pts',(-1.88568882100005,15.2,-10.856139687));
#296545=CARTESIAN_POINT('Ctrl Pts',(-1.88724637200006,15.2,-10.858822018));
#296546=CARTESIAN_POINT('Ctrl Pts',(-1.88880874000006,15.2,-10.861507626));
#296547=CARTESIAN_POINT('Ctrl Pts',(-1.89037592900006,15.2,-10.8641965));
#296548=CARTESIAN_POINT('Ctrl Pts',(-1.89194794100006,15.2,-10.866888627));
#296549=CARTESIAN_POINT('Ctrl Pts',(-1.89352477600006,15.2,-10.869583997));
#296550=CARTESIAN_POINT('Ctrl Pts',(-1.89510643700005,15.2,-10.872282597));
#296551=CARTESIAN_POINT('Ctrl Pts',(-1.89669292500006,15.2,-10.874984418));
#296552=CARTESIAN_POINT('Ctrl Pts',(-1.89828424200006,15.2,-10.877689446));
#296553=CARTESIAN_POINT('Ctrl Pts',(-1.89988038900006,15.2,-10.880397671));
#296554=CARTESIAN_POINT('Ctrl Pts',(-1.90148136800006,15.2,-10.88310908));
#296555=CARTESIAN_POINT('Ctrl Pts',(-1.90308718100006,15.2,-10.885823664));
#296556=CARTESIAN_POINT('Ctrl Pts',(-1.90469782800006,15.2,-10.888541409));
#296557=CARTESIAN_POINT('Ctrl Pts',(-1.90631331200006,15.2,-10.891262307));
#296558=CARTESIAN_POINT('Ctrl Pts',(-1.90793363400006,15.2,-10.893986344));
#296559=CARTESIAN_POINT('Ctrl Pts',(-1.90955879600006,15.2,-10.89671351));
#296560=CARTESIAN_POINT('Ctrl Pts',(-1.91118879900006,15.2,-10.899443792));
#296561=CARTESIAN_POINT('Ctrl Pts',(-1.91282364500006,15.2,-10.902177181));
#296562=CARTESIAN_POINT('Ctrl Pts',(-1.91446333500006,15.2,-10.904913664));
#296563=CARTESIAN_POINT('Ctrl Pts',(-1.91610787000006,15.2,-10.907653232));
#296564=CARTESIAN_POINT('Ctrl Pts',(-1.91775725300006,15.2,-10.910395872));
#296565=CARTESIAN_POINT('Ctrl Pts',(-1.91941148400006,15.2,-10.913141573));
#296566=CARTESIAN_POINT('Ctrl Pts',(-1.92107056600005,15.2,-10.915890324));
#296567=CARTESIAN_POINT('Ctrl Pts',(-1.92273449900005,15.2,-10.918642115));
#296568=CARTESIAN_POINT('Ctrl Pts',(-1.92440328400005,15.2,-10.921396933));
#296569=CARTESIAN_POINT('Ctrl Pts',(-1.92607692400005,15.2,-10.924154768));
#296570=CARTESIAN_POINT('Ctrl Pts',(-1.92775541900006,15.2,-10.92691561));
#296571=CARTESIAN_POINT('Ctrl Pts',(-1.92943877200005,15.2,-10.929679446));
#296572=CARTESIAN_POINT('Ctrl Pts',(-1.93112698400005,15.2,-10.932446266));
#296573=CARTESIAN_POINT('Ctrl Pts',(-1.93282005500006,15.2,-10.935216058));
#296574=CARTESIAN_POINT('Ctrl Pts',(-1.93451798600006,15.2,-10.937988814));
#296575=CARTESIAN_POINT('Ctrl Pts',(-1.93622078100006,15.2,-10.940764519));
#296576=CARTESIAN_POINT('Ctrl Pts',(-1.93792843900006,15.2,-10.943543166));
#296577=CARTESIAN_POINT('Ctrl Pts',(-1.93964096300005,15.2,-10.946324741));
#296578=CARTESIAN_POINT('Ctrl Pts',(-1.94135835200006,15.2,-10.949109235));
#296579=CARTESIAN_POINT('Ctrl Pts',(-1.94308061000006,15.2,-10.951896636));
#296580=CARTESIAN_POINT('Ctrl Pts',(-1.94480773800006,15.2,-10.954686934));
#296581=CARTESIAN_POINT('Ctrl Pts',(-1.94653973400006,15.2,-10.957480118));
#296582=CARTESIAN_POINT('Ctrl Pts',(-1.94827660300006,15.2,-10.960276177));
#296583=CARTESIAN_POINT('Ctrl Pts',(-1.95001834500005,15.2,-10.963075101));
#296584=CARTESIAN_POINT('Ctrl Pts',(-1.95176495900005,15.2,-10.965876877));
#296585=CARTESIAN_POINT('Ctrl Pts',(-1.95351645100006,15.2,-10.968681498));
#296586=CARTESIAN_POINT('Ctrl Pts',(-1.95527281700006,15.2,-10.971488949));
#296587=CARTESIAN_POINT('Ctrl Pts',(-1.95703406200006,15.2,-10.974299223));
#296588=CARTESIAN_POINT('Ctrl Pts',(-1.95880018600006,15.2,-10.977112307));
#296589=CARTESIAN_POINT('Ctrl Pts',(-1.96057119000006,15.2,-10.979928192));
#296590=CARTESIAN_POINT('Ctrl Pts',(-1.96234707500006,15.2,-10.982746866));
#296591=CARTESIAN_POINT('Ctrl Pts',(-1.96412784300006,15.2,-10.985568319));
#296592=CARTESIAN_POINT('Ctrl Pts',(-1.96591349400005,15.2,-10.988392541));
#296593=CARTESIAN_POINT('Ctrl Pts',(-1.96770402900006,15.2,-10.99121952));
#296594=CARTESIAN_POINT('Ctrl Pts',(-1.96949945100006,15.2,-10.994049247));
#296595=CARTESIAN_POINT('Ctrl Pts',(-1.97129976000005,15.2,-10.996881712));
#296596=CARTESIAN_POINT('Ctrl Pts',(-1.97310495700005,15.2,-10.999716901));
#296597=CARTESIAN_POINT('Ctrl Pts',(-1.97491504200005,15.2,-11.002554807));
#296598=CARTESIAN_POINT('Ctrl Pts',(-1.97673001900006,15.2,-11.005395418));
#296599=CARTESIAN_POINT('Ctrl Pts',(-1.97854988600006,15.2,-11.008238724));
#296600=CARTESIAN_POINT('Ctrl Pts',(-1.98037464600006,15.2,-11.011084714));
#296601=CARTESIAN_POINT('Ctrl Pts',(-1.98220430000006,15.2,-11.013933379));
#296602=CARTESIAN_POINT('Ctrl Pts',(-1.98403884700005,15.2,-11.016784707));
#296603=CARTESIAN_POINT('Ctrl Pts',(-1.98587829000005,15.2,-11.019638689));
#296604=CARTESIAN_POINT('Ctrl Pts',(-1.98772263100006,15.2,-11.022495313));
#296605=CARTESIAN_POINT('Ctrl Pts',(-1.98957186800006,15.2,-11.025354571));
#296606=CARTESIAN_POINT('Ctrl Pts',(-1.99142600300006,15.2,-11.02821645));
#296607=CARTESIAN_POINT('Ctrl Pts',(-1.99328503900006,15.2,-11.031080942));
#296608=CARTESIAN_POINT('Ctrl Pts',(-1.99514897500006,15.2,-11.033948035));
#296609=CARTESIAN_POINT('Ctrl Pts',(-1.99701781300006,15.2,-11.03681772));
#296610=CARTESIAN_POINT('Ctrl Pts',(-1.99889155400006,15.2,-11.039689987));
#296611=CARTESIAN_POINT('Ctrl Pts',(-2.00077019700006,15.2,-11.042564824));
#296612=CARTESIAN_POINT('Ctrl Pts',(-2.00265374600006,15.2,-11.045442222));
#296613=CARTESIAN_POINT('Ctrl Pts',(-2.00454219900006,15.2,-11.048322171));
#296614=CARTESIAN_POINT('Ctrl Pts',(-2.00643555900006,15.2,-11.05120466));
#296615=CARTESIAN_POINT('Ctrl Pts',(-2.00833382600006,15.2,-11.054089681));
#296616=CARTESIAN_POINT('Ctrl Pts',(-2.01023700100006,15.2,-11.056977221));
#296617=CARTESIAN_POINT('Ctrl Pts',(-2.01214508600006,15.2,-11.059867271));
#296618=CARTESIAN_POINT('Ctrl Pts',(-2.01405807900006,15.2,-11.062759821));
#296619=CARTESIAN_POINT('Ctrl Pts',(-2.01597598400005,15.2,-11.065654863));
#296620=CARTESIAN_POINT('Ctrl Pts',(-2.01789880000006,15.2,-11.068552382));
#296621=CARTESIAN_POINT('Ctrl Pts',(-2.01982652900006,15.2,-11.071452373));
#296622=CARTESIAN_POINT('Ctrl Pts',(-2.02175917100006,15.2,-11.074354824));
#296623=CARTESIAN_POINT('Ctrl Pts',(-2.02369672800006,15.2,-11.077259724));
#296624=CARTESIAN_POINT('Ctrl Pts',(-2.02563919900005,15.2,-11.080167065));
#296625=CARTESIAN_POINT('Ctrl Pts',(-2.02758658500006,15.2,-11.083076836));
#296626=CARTESIAN_POINT('Ctrl Pts',(-2.02953889000006,15.2,-11.085989026));
#296627=CARTESIAN_POINT('Ctrl Pts',(-2.03149611100006,15.2,-11.088903627));
#296628=CARTESIAN_POINT('Ctrl Pts',(-2.03345825000006,15.2,-11.091820627));
#296629=CARTESIAN_POINT('Ctrl Pts',(-2.03542530900005,15.2,-11.094740019));
#296630=CARTESIAN_POINT('Ctrl Pts',(-2.03739728600006,15.2,-11.097661791));
#296631=CARTESIAN_POINT('Ctrl Pts',(-2.03937418400006,15.2,-11.100585934));
#296632=CARTESIAN_POINT('Ctrl Pts',(-2.04135600500006,15.2,-11.103512437));
#296633=CARTESIAN_POINT('Ctrl Pts',(-2.04334274700006,15.2,-11.106441291));
#296634=CARTESIAN_POINT('Ctrl Pts',(-2.04533441100006,15.2,-11.109372486));
#296635=CARTESIAN_POINT('Ctrl Pts',(-2.04733100000006,15.2,-11.112306013));
#296636=CARTESIAN_POINT('Ctrl Pts',(-2.04933251100006,15.2,-11.115241862));
#296637=CARTESIAN_POINT('Ctrl Pts',(-2.05133894900006,15.2,-11.118180023));
#296638=CARTESIAN_POINT('Ctrl Pts',(-2.05335031200006,15.2,-11.121120485));
#296639=CARTESIAN_POINT('Ctrl Pts',(-2.05536660000006,15.2,-11.12406324));
#296640=CARTESIAN_POINT('Ctrl Pts',(-2.05738781600005,15.2,-11.127008278));
#296641=CARTESIAN_POINT('Ctrl Pts',(-2.05941396000005,15.2,-11.129955589));
#296642=CARTESIAN_POINT('Ctrl Pts',(-2.06144503200006,15.2,-11.132905162));
#296643=CARTESIAN_POINT('Ctrl Pts',(-2.06348103200006,15.2,-11.13585699));
#296644=CARTESIAN_POINT('Ctrl Pts',(-2.06552196300006,15.2,-11.138811062));
#296645=CARTESIAN_POINT('Ctrl Pts',(-2.06756782400006,15.2,-11.141767369));
#296646=CARTESIAN_POINT('Ctrl Pts',(-2.06961861500006,15.2,-11.1447259));
#296647=CARTESIAN_POINT('Ctrl Pts',(-2.07167433800006,15.2,-11.147686647));
#296648=CARTESIAN_POINT('Ctrl Pts',(-2.07373499200005,15.2,-11.1506496));
#296649=CARTESIAN_POINT('Ctrl Pts',(-2.07580058000006,15.2,-11.153614748));
#296650=CARTESIAN_POINT('Ctrl Pts',(-2.07787110100006,15.2,-11.156582084));
#296651=CARTESIAN_POINT('Ctrl Pts',(-2.07994655600006,15.2,-11.159551596));
#296652=CARTESIAN_POINT('Ctrl Pts',(-2.08202694500006,15.2,-11.162523276));
#296653=CARTESIAN_POINT('Ctrl Pts',(-2.08411226900005,15.2,-11.165497114));
#296654=CARTESIAN_POINT('Ctrl Pts',(-2.08620252700006,15.2,-11.1684731));
#296655=CARTESIAN_POINT('Ctrl Pts',(-2.08829772300006,15.2,-11.171451227));
#296656=CARTESIAN_POINT('Ctrl Pts',(-2.09039785500006,15.2,-11.174431482));
#296657=CARTESIAN_POINT('Ctrl Pts',(-2.09250292400006,15.2,-11.177413859));
#296658=CARTESIAN_POINT('Ctrl Pts',(-2.09461293200006,15.2,-11.180398346));
#296659=CARTESIAN_POINT('Ctrl Pts',(-2.09672787600006,15.2,-11.183384935));
#296660=CARTESIAN_POINT('Ctrl Pts',(-2.09884776000006,15.2,-11.186373616));
#296661=CARTESIAN_POINT('Ctrl Pts',(-2.10097258200005,15.2,-11.18936438));
#296662=CARTESIAN_POINT('Ctrl Pts',(-2.10310234500006,15.2,-11.192357218));
#296663=CARTESIAN_POINT('Ctrl Pts',(-2.10523704700006,15.2,-11.19535212));
#296664=CARTESIAN_POINT('Ctrl Pts',(-2.10737669000005,15.2,-11.198349076));
#296665=CARTESIAN_POINT('Ctrl Pts',(-2.10952127400006,15.2,-11.201348078));
#296666=CARTESIAN_POINT('Ctrl Pts',(-2.11167080000005,15.2,-11.204349116));
#296667=CARTESIAN_POINT('Ctrl Pts',(-2.11382526700006,15.2,-11.207352181));
#296668=CARTESIAN_POINT('Ctrl Pts',(-2.11598467700005,15.2,-11.210357264));
#296669=CARTESIAN_POINT('Ctrl Pts',(-2.11814903000006,15.2,-11.213364356));
#296670=CARTESIAN_POINT('Ctrl Pts',(-2.12031832600006,15.2,-11.216373446));
#296671=CARTESIAN_POINT('Ctrl Pts',(-2.12249256500006,15.2,-11.219384528));
#296672=CARTESIAN_POINT('Ctrl Pts',(-2.12467174800006,15.2,-11.222397592));
#296673=CARTESIAN_POINT('Ctrl Pts',(-2.12685587600005,15.2,-11.225412626));
#296674=CARTESIAN_POINT('Ctrl Pts',(-2.12904494800005,15.2,-11.228429624));
#296675=CARTESIAN_POINT('Ctrl Pts',(-2.13123896500006,15.2,-11.231448574));
#296676=CARTESIAN_POINT('Ctrl Pts',(-2.13343792800006,15.2,-11.234469469));
#296677=CARTESIAN_POINT('Ctrl Pts',(-2.13564183800006,15.2,-11.237492297));
#296678=CARTESIAN_POINT('Ctrl Pts',(-2.13785069300005,15.2,-11.24051705));
#296679=CARTESIAN_POINT('Ctrl Pts',(-2.14006449500005,15.2,-11.243543721));
#296680=CARTESIAN_POINT('Ctrl Pts',(-2.14228324400006,15.2,-11.246572299));
#296681=CARTESIAN_POINT('Ctrl Pts',(-2.14450694000006,15.2,-11.249602777));
#296682=CARTESIAN_POINT('Ctrl Pts',(-2.14673558400006,15.2,-11.252635149));
#296683=CARTESIAN_POINT('Ctrl Pts',(-2.14896917600006,15.2,-11.255669403));
#296684=CARTESIAN_POINT('Ctrl Pts',(-2.15120771500006,15.2,-11.258705531));
#296685=CARTESIAN_POINT('Ctrl Pts',(-2.15345120200006,15.2,-11.261743524));
#296686=CARTESIAN_POINT('Ctrl Pts',(-2.15569963800006,15.2,-11.264783368));
#296687=CARTESIAN_POINT('Ctrl Pts',(-2.15795302500006,15.2,-11.267825054));
#296688=CARTESIAN_POINT('Ctrl Pts',(-2.16021136000006,15.2,-11.27086857));
#296689=CARTESIAN_POINT('Ctrl Pts',(-2.16247464600006,15.2,-11.273913908));
#296690=CARTESIAN_POINT('Ctrl Pts',(-2.16474288100006,15.2,-11.276961058));
#296691=CARTESIAN_POINT('Ctrl Pts',(-2.16701606700005,15.2,-11.280010015));
#296692=CARTESIAN_POINT('Ctrl Pts',(-2.16929420200006,15.2,-11.283060773));
#296693=CARTESIAN_POINT('Ctrl Pts',(-2.17157728800006,15.2,-11.286113334));
#296694=CARTESIAN_POINT('Ctrl Pts',(-2.17340771700006,15.2,-11.28855682));
#296695=CARTESIAN_POINT('Ctrl Pts',(-2.17478276600006,15.2,-11.290390245));
#296696=CARTESIAN_POINT('Ctrl Pts',(-2.17570045500006,15.2,-11.291612887));
#296697=CARTESIAN_POINT('Ctrl Pts',(-2.17615954800006,15.2,-11.292224299));
#296698=CARTESIAN_POINT('Origin',(-5.66257110645729E-14,15.2,-1.77635683940025E-14));
#296699=CARTESIAN_POINT('',(-1.18690176602512,15.2,-10.306885523551));
#296700=CARTESIAN_POINT('Origin',(-5.66257110645729E-14,15.2,-1.77635683940025E-14));
#296701=CARTESIAN_POINT('',(-0.143881228002569,15.2,-10.3740022745144));
#296702=CARTESIAN_POINT('Origin',(-5.66257110645729E-14,15.2,-1.77635683940025E-14));
#296703=CARTESIAN_POINT('',(-0.546958306000055,15.2,-11.486985532));
#296704=CARTESIAN_POINT('Ctrl Pts',(-0.143881228000057,15.2,-10.374002275));
#296705=CARTESIAN_POINT('Ctrl Pts',(-0.143898619000057,15.2,-10.374175763));
#296706=CARTESIAN_POINT('Ctrl Pts',(-0.143934095000056,15.2,-10.37452879));
#296707=CARTESIAN_POINT('Ctrl Pts',(-0.143988114000055,15.2,-10.375063685));
#296708=CARTESIAN_POINT('Ctrl Pts',(-0.144061421000057,15.2,-10.375784183));
#296709=CARTESIAN_POINT('Ctrl Pts',(-0.144155050000055,15.2,-10.376695412));
#296710=CARTESIAN_POINT('Ctrl Pts',(-0.144251127000056,15.2,-10.377621314));
#296711=CARTESIAN_POINT('Ctrl Pts',(-0.144349125000056,15.2,-10.378556581));
#296712=CARTESIAN_POINT('Ctrl Pts',(-0.144449058000056,15.2,-10.379501186));
#296713=CARTESIAN_POINT('Ctrl Pts',(-0.144550942000056,15.2,-10.380455099));
#296714=CARTESIAN_POINT('Ctrl Pts',(-0.144654791000055,15.2,-10.381418293));
#296715=CARTESIAN_POINT('Ctrl Pts',(-0.144760620000056,15.2,-10.382390738));
#296716=CARTESIAN_POINT('Ctrl Pts',(-0.144868446000055,15.2,-10.383372406));
#296717=CARTESIAN_POINT('Ctrl Pts',(-0.144978281000055,15.2,-10.38436327));
#296718=CARTESIAN_POINT('Ctrl Pts',(-0.145090142000056,15.2,-10.3853633));
#296719=CARTESIAN_POINT('Ctrl Pts',(-0.145204042000057,15.2,-10.38637247));
#296720=CARTESIAN_POINT('Ctrl Pts',(-0.145319997000056,15.2,-10.387390753));
#296721=CARTESIAN_POINT('Ctrl Pts',(-0.145438020000055,15.2,-10.388418119));
#296722=CARTESIAN_POINT('Ctrl Pts',(-0.145558126000056,15.2,-10.389454543));
#296723=CARTESIAN_POINT('Ctrl Pts',(-0.145680330000056,15.2,-10.390499995));
#296724=CARTESIAN_POINT('Ctrl Pts',(-0.145804646000055,15.2,-10.39155445));
#296725=CARTESIAN_POINT('Ctrl Pts',(-0.145931087000056,15.2,-10.392617881));
#296726=CARTESIAN_POINT('Ctrl Pts',(-0.146059668000056,15.2,-10.39369026));
#296727=CARTESIAN_POINT('Ctrl Pts',(-0.146190404000055,15.2,-10.394771561));
#296728=CARTESIAN_POINT('Ctrl Pts',(-0.146323306000056,15.2,-10.395861756));
#296729=CARTESIAN_POINT('Ctrl Pts',(-0.146458391000056,15.2,-10.39696082));
#296730=CARTESIAN_POINT('Ctrl Pts',(-0.146595671000057,15.2,-10.398068726));
#296731=CARTESIAN_POINT('Ctrl Pts',(-0.146735160000055,15.2,-10.399185446));
#296732=CARTESIAN_POINT('Ctrl Pts',(-0.146876872000057,15.2,-10.400310957));
#296733=CARTESIAN_POINT('Ctrl Pts',(-0.147020820000057,15.2,-10.401445231));
#296734=CARTESIAN_POINT('Ctrl Pts',(-0.147167017000056,15.2,-10.402588242));
#296735=CARTESIAN_POINT('Ctrl Pts',(-0.147315478000056,15.2,-10.403739965));
#296736=CARTESIAN_POINT('Ctrl Pts',(-0.147466215000056,15.2,-10.404900372));
#296737=CARTESIAN_POINT('Ctrl Pts',(-0.147619240000055,15.2,-10.40606944));
#296738=CARTESIAN_POINT('Ctrl Pts',(-0.147774569000055,15.2,-10.407247142));
#296739=CARTESIAN_POINT('Ctrl Pts',(-0.147932214000056,15.2,-10.408433454));
#296740=CARTESIAN_POINT('Ctrl Pts',(-0.148092187000056,15.2,-10.409628348));
#296741=CARTESIAN_POINT('Ctrl Pts',(-0.148254502000055,15.2,-10.410831802));
#296742=CARTESIAN_POINT('Ctrl Pts',(-0.148419173000055,15.2,-10.412043788));
#296743=CARTESIAN_POINT('Ctrl Pts',(-0.148586210000056,15.2,-10.413264283));
#296744=CARTESIAN_POINT('Ctrl Pts',(-0.148755627000057,15.2,-10.414493262));
#296745=CARTESIAN_POINT('Ctrl Pts',(-0.148927437000056,15.2,-10.4157307));
#296746=CARTESIAN_POINT('Ctrl Pts',(-0.149101652000055,15.2,-10.416976571));
#296747=CARTESIAN_POINT('Ctrl Pts',(-0.149278286000056,15.2,-10.418230852));
#296748=CARTESIAN_POINT('Ctrl Pts',(-0.149457350000055,15.2,-10.419493518));
#296749=CARTESIAN_POINT('Ctrl Pts',(-0.149638856000056,15.2,-10.420764545));
#296750=CARTESIAN_POINT('Ctrl Pts',(-0.149822818000055,15.2,-10.422043907));
#296751=CARTESIAN_POINT('Ctrl Pts',(-0.150009246000057,15.2,-10.423331583));
#296752=CARTESIAN_POINT('Ctrl Pts',(-0.150198154000056,15.2,-10.424627545));
#296753=CARTESIAN_POINT('Ctrl Pts',(-0.150389553000055,15.2,-10.425931773));
#296754=CARTESIAN_POINT('Ctrl Pts',(-0.150583457000056,15.2,-10.427244241));
#296755=CARTESIAN_POINT('Ctrl Pts',(-0.150779876000057,15.2,-10.428564925));
#296756=CARTESIAN_POINT('Ctrl Pts',(-0.150978823000055,15.2,-10.429893802));
#296757=CARTESIAN_POINT('Ctrl Pts',(-0.151180310000055,15.2,-10.431230848));
#296758=CARTESIAN_POINT('Ctrl Pts',(-0.151384347000055,15.2,-10.43257604));
#296759=CARTESIAN_POINT('Ctrl Pts',(-0.151590948000055,15.2,-10.433929354));
#296760=CARTESIAN_POINT('Ctrl Pts',(-0.151800122000055,15.2,-10.435290769));
#296761=CARTESIAN_POINT('Ctrl Pts',(-0.152011884000055,15.2,-10.436660258));
#296762=CARTESIAN_POINT('Ctrl Pts',(-0.152226243000056,15.2,-10.4380378));
#296763=CARTESIAN_POINT('Ctrl Pts',(-0.152443212000056,15.2,-10.439423372));
#296764=CARTESIAN_POINT('Ctrl Pts',(-0.152662802000056,15.2,-10.440816951));
#296765=CARTESIAN_POINT('Ctrl Pts',(-0.152885022000057,15.2,-10.442218514));
#296766=CARTESIAN_POINT('Ctrl Pts',(-0.153109888000056,15.2,-10.443628038));
#296767=CARTESIAN_POINT('Ctrl Pts',(-0.153337407000055,15.2,-10.4450455));
#296768=CARTESIAN_POINT('Ctrl Pts',(-0.153567593000057,15.2,-10.446470879));
#296769=CARTESIAN_POINT('Ctrl Pts',(-0.153800456000056,15.2,-10.447904152));
#296770=CARTESIAN_POINT('Ctrl Pts',(-0.154036006000055,15.2,-10.449345296));
#296771=CARTESIAN_POINT('Ctrl Pts',(-0.154274256000055,15.2,-10.450794288));
#296772=CARTESIAN_POINT('Ctrl Pts',(-0.154515216000056,15.2,-10.452251106));
#296773=CARTESIAN_POINT('Ctrl Pts',(-0.154758897000056,15.2,-10.45371573));
#296774=CARTESIAN_POINT('Ctrl Pts',(-0.155005310000057,15.2,-10.455188136));
#296775=CARTESIAN_POINT('Ctrl Pts',(-0.155254466000055,15.2,-10.456668302));
#296776=CARTESIAN_POINT('Ctrl Pts',(-0.155506375000056,15.2,-10.458156207));
#296777=CARTESIAN_POINT('Ctrl Pts',(-0.155761048000055,15.2,-10.459651829));
#296778=CARTESIAN_POINT('Ctrl Pts',(-0.156018496000057,15.2,-10.461155145));
#296779=CARTESIAN_POINT('Ctrl Pts',(-0.156278730000056,15.2,-10.462666135));
#296780=CARTESIAN_POINT('Ctrl Pts',(-0.156541758000056,15.2,-10.464184778));
#296781=CARTESIAN_POINT('Ctrl Pts',(-0.156807594000057,15.2,-10.46571105));
#296782=CARTESIAN_POINT('Ctrl Pts',(-0.157076245000055,15.2,-10.467244931));
#296783=CARTESIAN_POINT('Ctrl Pts',(-0.157347725000055,15.2,-10.4687864));
#296784=CARTESIAN_POINT('Ctrl Pts',(-0.157622041000056,15.2,-10.470335435));
#296785=CARTESIAN_POINT('Ctrl Pts',(-0.157899205000056,15.2,-10.471892016));
#296786=CARTESIAN_POINT('Ctrl Pts',(-0.158179227000056,15.2,-10.473456121));
#296787=CARTESIAN_POINT('Ctrl Pts',(-0.158462117000056,15.2,-10.475027729));
#296788=CARTESIAN_POINT('Ctrl Pts',(-0.158747884000056,15.2,-10.476606819));
#296789=CARTESIAN_POINT('Ctrl Pts',(-0.159036540000056,15.2,-10.478193371));
#296790=CARTESIAN_POINT('Ctrl Pts',(-0.159328094000056,15.2,-10.479787363));
#296791=CARTESIAN_POINT('Ctrl Pts',(-0.159622556000055,15.2,-10.481388775));
#296792=CARTESIAN_POINT('Ctrl Pts',(-0.159919937000056,15.2,-10.482997586));
#296793=CARTESIAN_POINT('Ctrl Pts',(-0.160220245000057,15.2,-10.484613776));
#296794=CARTESIAN_POINT('Ctrl Pts',(-0.160523489000056,15.2,-10.486237324));
#296795=CARTESIAN_POINT('Ctrl Pts',(-0.160829682000055,15.2,-10.487868211));
#296796=CARTESIAN_POINT('Ctrl Pts',(-0.161138833000055,15.2,-10.489506414));
#296797=CARTESIAN_POINT('Ctrl Pts',(-0.161450949000056,15.2,-10.491151915));
#296798=CARTESIAN_POINT('Ctrl Pts',(-0.161766042000057,15.2,-10.492804693));
#296799=CARTESIAN_POINT('Ctrl Pts',(-0.162084120000056,15.2,-10.494464728));
#296800=CARTESIAN_POINT('Ctrl Pts',(-0.162405194000056,15.2,-10.496131999));
#296801=CARTESIAN_POINT('Ctrl Pts',(-0.162729274000055,15.2,-10.497806488));
#296802=CARTESIAN_POINT('Ctrl Pts',(-0.163056366000056,15.2,-10.499488173));
#296803=CARTESIAN_POINT('Ctrl Pts',(-0.163386483000056,15.2,-10.501177036));
#296804=CARTESIAN_POINT('Ctrl Pts',(-0.163719632000056,15.2,-10.502873055));
#296805=CARTESIAN_POINT('Ctrl Pts',(-0.164055824000057,15.2,-10.504576212));
#296806=CARTESIAN_POINT('Ctrl Pts',(-0.164395067000056,15.2,-10.506286487));
#296807=CARTESIAN_POINT('Ctrl Pts',(-0.164737371000055,15.2,-10.508003862));
#296808=CARTESIAN_POINT('Ctrl Pts',(-0.165082744000056,15.2,-10.509728314));
#296809=CARTESIAN_POINT('Ctrl Pts',(-0.165431198000056,15.2,-10.511459826));
#296810=CARTESIAN_POINT('Ctrl Pts',(-0.165782737000055,15.2,-10.513198378));
#296811=CARTESIAN_POINT('Ctrl Pts',(-0.166137374000056,15.2,-10.514943952));
#296812=CARTESIAN_POINT('Ctrl Pts',(-0.166495117000055,15.2,-10.516696527));
#296813=CARTESIAN_POINT('Ctrl Pts',(-0.166855974000055,15.2,-10.518456084));
#296814=CARTESIAN_POINT('Ctrl Pts',(-0.167219956000055,15.2,-10.520222604));
#296815=CARTESIAN_POINT('Ctrl Pts',(-0.167587069000056,15.2,-10.521996069));
#296816=CARTESIAN_POINT('Ctrl Pts',(-0.167957324000056,15.2,-10.523776458));
#296817=CARTESIAN_POINT('Ctrl Pts',(-0.168330729000056,15.2,-10.525563754));
#296818=CARTESIAN_POINT('Ctrl Pts',(-0.168707293000055,15.2,-10.527357938));
#296819=CARTESIAN_POINT('Ctrl Pts',(-0.169087023000056,15.2,-10.529158991));
#296820=CARTESIAN_POINT('Ctrl Pts',(-0.169469930000057,15.2,-10.530966892));
#296821=CARTESIAN_POINT('Ctrl Pts',(-0.169856021000055,15.2,-10.532781626));
#296822=CARTESIAN_POINT('Ctrl Pts',(-0.170245305000056,15.2,-10.534603171));
#296823=CARTESIAN_POINT('Ctrl Pts',(-0.170637791000056,15.2,-10.536431511));
#296824=CARTESIAN_POINT('Ctrl Pts',(-0.171033486000055,15.2,-10.538266627));
#296825=CARTESIAN_POINT('Ctrl Pts',(-0.171432400000056,15.2,-10.5401085));
#296826=CARTESIAN_POINT('Ctrl Pts',(-0.171834541000055,15.2,-10.541957111));
#296827=CARTESIAN_POINT('Ctrl Pts',(-0.172239916000055,15.2,-10.543812443));
#296828=CARTESIAN_POINT('Ctrl Pts',(-0.172648536000055,15.2,-10.545674477));
#296829=CARTESIAN_POINT('Ctrl Pts',(-0.173060406000056,15.2,-10.547543195));
#296830=CARTESIAN_POINT('Ctrl Pts',(-0.173475537000056,15.2,-10.549418579));
#296831=CARTESIAN_POINT('Ctrl Pts',(-0.173893934000056,15.2,-10.551300611));
#296832=CARTESIAN_POINT('Ctrl Pts',(-0.174315609000055,15.2,-10.553189273));
#296833=CARTESIAN_POINT('Ctrl Pts',(-0.174740568000056,15.2,-10.555084546));
#296834=CARTESIAN_POINT('Ctrl Pts',(-0.175168818000057,15.2,-10.556986413));
#296835=CARTESIAN_POINT('Ctrl Pts',(-0.175600369000056,15.2,-10.558894856));
#296836=CARTESIAN_POINT('Ctrl Pts',(-0.176035228000057,15.2,-10.560809857));
#296837=CARTESIAN_POINT('Ctrl Pts',(-0.176473403000056,15.2,-10.562731399));
#296838=CARTESIAN_POINT('Ctrl Pts',(-0.176914903000055,15.2,-10.564659465));
#296839=CARTESIAN_POINT('Ctrl Pts',(-0.177359734000057,15.2,-10.566594035));
#296840=CARTESIAN_POINT('Ctrl Pts',(-0.177807905000057,15.2,-10.568535092));
#296841=CARTESIAN_POINT('Ctrl Pts',(-0.178259423000057,15.2,-10.570482619));
#296842=CARTESIAN_POINT('Ctrl Pts',(-0.178714296000055,15.2,-10.572436599));
#296843=CARTESIAN_POINT('Ctrl Pts',(-0.179172532000056,15.2,-10.574397014));
#296844=CARTESIAN_POINT('Ctrl Pts',(-0.179634139000056,15.2,-10.576363848));
#296845=CARTESIAN_POINT('Ctrl Pts',(-0.180099125000056,15.2,-10.578337081));
#296846=CARTESIAN_POINT('Ctrl Pts',(-0.180567496000055,15.2,-10.580316698));
#296847=CARTESIAN_POINT('Ctrl Pts',(-0.181039260000055,15.2,-10.582302681));
#296848=CARTESIAN_POINT('Ctrl Pts',(-0.181514425000057,15.2,-10.584295012));
#296849=CARTESIAN_POINT('Ctrl Pts',(-0.181992998000055,15.2,-10.586293676));
#296850=CARTESIAN_POINT('Ctrl Pts',(-0.182474988000055,15.2,-10.588298654));
#296851=CARTESIAN_POINT('Ctrl Pts',(-0.182960401000055,15.2,-10.59030993));
#296852=CARTESIAN_POINT('Ctrl Pts',(-0.183449244000055,15.2,-10.592327487));
#296853=CARTESIAN_POINT('Ctrl Pts',(-0.183941526000057,15.2,-10.594351307));
#296854=CARTESIAN_POINT('Ctrl Pts',(-0.184437253000055,15.2,-10.596381375));
#296855=CARTESIAN_POINT('Ctrl Pts',(-0.184936432000056,15.2,-10.598417672));
#296856=CARTESIAN_POINT('Ctrl Pts',(-0.185439071000056,15.2,-10.600460183));
#296857=CARTESIAN_POINT('Ctrl Pts',(-0.185945177000055,15.2,-10.602508892));
#296858=CARTESIAN_POINT('Ctrl Pts',(-0.186454758000056,15.2,-10.60456378));
#296859=CARTESIAN_POINT('Ctrl Pts',(-0.186967820000056,15.2,-10.606624832));
#296860=CARTESIAN_POINT('Ctrl Pts',(-0.187484370000056,15.2,-10.60869203));
#296861=CARTESIAN_POINT('Ctrl Pts',(-0.188004417000055,15.2,-10.610765359));
#296862=CARTESIAN_POINT('Ctrl Pts',(-0.188527965000055,15.2,-10.612844802));
#296863=CARTESIAN_POINT('Ctrl Pts',(-0.189055024000057,15.2,-10.614930343));
#296864=CARTESIAN_POINT('Ctrl Pts',(-0.189585599000056,15.2,-10.617021965));
#296865=CARTESIAN_POINT('Ctrl Pts',(-0.190119697000056,15.2,-10.619119652));
#296866=CARTESIAN_POINT('Ctrl Pts',(-0.190657326000055,15.2,-10.621223388));
#296867=CARTESIAN_POINT('Ctrl Pts',(-0.191198493000057,15.2,-10.623333156));
#296868=CARTESIAN_POINT('Ctrl Pts',(-0.191743203000057,15.2,-10.62544894));
#296869=CARTESIAN_POINT('Ctrl Pts',(-0.192291464000055,15.2,-10.627570723));
#296870=CARTESIAN_POINT('Ctrl Pts',(-0.192843283000055,15.2,-10.629698492));
#296871=CARTESIAN_POINT('Ctrl Pts',(-0.193398667000055,15.2,-10.631832228));
#296872=CARTESIAN_POINT('Ctrl Pts',(-0.193957623000056,15.2,-10.633971916));
#296873=CARTESIAN_POINT('Ctrl Pts',(-0.194520156000056,15.2,-10.636117541));
#296874=CARTESIAN_POINT('Ctrl Pts',(-0.195086274000056,15.2,-10.638269086));
#296875=CARTESIAN_POINT('Ctrl Pts',(-0.195655982000057,15.2,-10.640426534));
#296876=CARTESIAN_POINT('Ctrl Pts',(-0.196229289000056,15.2,-10.642589871));
#296877=CARTESIAN_POINT('Ctrl Pts',(-0.196806201000056,15.2,-10.644759081));
#296878=CARTESIAN_POINT('Ctrl Pts',(-0.197386723000056,15.2,-10.646934148));
#296879=CARTESIAN_POINT('Ctrl Pts',(-0.197970862000056,15.2,-10.649115056));
#296880=CARTESIAN_POINT('Ctrl Pts',(-0.198558626000055,15.2,-10.651301789));
#296881=CARTESIAN_POINT('Ctrl Pts',(-0.199150020000056,15.2,-10.653494333));
#296882=CARTESIAN_POINT('Ctrl Pts',(-0.199745051000055,15.2,-10.655692671));
#296883=CARTESIAN_POINT('Ctrl Pts',(-0.200343725000056,15.2,-10.657896788));
#296884=CARTESIAN_POINT('Ctrl Pts',(-0.200946049000056,15.2,-10.660106669));
#296885=CARTESIAN_POINT('Ctrl Pts',(-0.201552028000057,15.2,-10.662322297));
#296886=CARTESIAN_POINT('Ctrl Pts',(-0.202161670000055,15.2,-10.664543659));
#296887=CARTESIAN_POINT('Ctrl Pts',(-0.202774980000056,15.2,-10.666770738));
#296888=CARTESIAN_POINT('Ctrl Pts',(-0.203391965000056,15.2,-10.669003519));
#296889=CARTESIAN_POINT('Ctrl Pts',(-0.204012631000056,15.2,-10.671241986));
#296890=CARTESIAN_POINT('Ctrl Pts',(-0.204636983000055,15.2,-10.673486125));
#296891=CARTESIAN_POINT('Ctrl Pts',(-0.205265029000056,15.2,-10.67573592));
#296892=CARTESIAN_POINT('Ctrl Pts',(-0.205896774000056,15.2,-10.677991357));
#296893=CARTESIAN_POINT('Ctrl Pts',(-0.206532225000055,15.2,-10.68025242));
#296894=CARTESIAN_POINT('Ctrl Pts',(-0.207171387000056,15.2,-10.682519093));
#296895=CARTESIAN_POINT('Ctrl Pts',(-0.207814267000056,15.2,-10.684791362));
#296896=CARTESIAN_POINT('Ctrl Pts',(-0.208460870000057,15.2,-10.687069213));
#296897=CARTESIAN_POINT('Ctrl Pts',(-0.209111203000055,15.2,-10.68935263));
#296898=CARTESIAN_POINT('Ctrl Pts',(-0.209765271000055,15.2,-10.691641597));
#296899=CARTESIAN_POINT('Ctrl Pts',(-0.210423081000056,15.2,-10.693936102));
#296900=CARTESIAN_POINT('Ctrl Pts',(-0.211084639000055,15.2,-10.696236127));
#296901=CARTESIAN_POINT('Ctrl Pts',(-0.211749948000056,15.2,-10.69854166));
#296902=CARTESIAN_POINT('Ctrl Pts',(-0.212419019000055,15.2,-10.700852684));
#296903=CARTESIAN_POINT('Ctrl Pts',(-0.213091853000057,15.2,-10.703169187));
#296904=CARTESIAN_POINT('Ctrl Pts',(-0.213903779044305,15.2,-10.7059555439519));
#296905=CARTESIAN_POINT('Ctrl Pts',(-0.214721369015063,15.2,-10.708750071151));
#296906=CARTESIAN_POINT('Ctrl Pts',(-0.21554463698505,15.2,-10.711552744849));
#296907=CARTESIAN_POINT('Ctrl Pts',(-0.21637359103007,15.2,-10.714363529302));
#296908=CARTESIAN_POINT('Ctrl Pts',(-0.217208245000055,15.2,-10.7171824));
#296909=CARTESIAN_POINT('Ctrl Pts',(-0.217907594000056,15.2,-10.719536833));
#296910=CARTESIAN_POINT('Ctrl Pts',(-0.218610753000055,15.2,-10.721896628));
#296911=CARTESIAN_POINT('Ctrl Pts',(-0.219317730000055,15.2,-10.724261768));
#296912=CARTESIAN_POINT('Ctrl Pts',(-0.220028527000055,15.2,-10.726632241));
#296913=CARTESIAN_POINT('Ctrl Pts',(-0.220743152000056,15.2,-10.729008033));
#296914=CARTESIAN_POINT('Ctrl Pts',(-0.221461609000055,15.2,-10.731389127));
#296915=CARTESIAN_POINT('Ctrl Pts',(-0.222183905000056,15.2,-10.733775512));
#296916=CARTESIAN_POINT('Ctrl Pts',(-0.222910044000055,15.2,-10.736167171));
#296917=CARTESIAN_POINT('Ctrl Pts',(-0.223640033000055,15.2,-10.738564091));
#296918=CARTESIAN_POINT('Ctrl Pts',(-0.224373875000056,15.2,-10.740966259));
#296919=CARTESIAN_POINT('Ctrl Pts',(-0.225111578000057,15.2,-10.743373659));
#296920=CARTESIAN_POINT('Ctrl Pts',(-0.225853145000056,15.2,-10.745786278));
#296921=CARTESIAN_POINT('Ctrl Pts',(-0.226598585000056,15.2,-10.748204102));
#296922=CARTESIAN_POINT('Ctrl Pts',(-0.227347899000057,15.2,-10.750627116));
#296923=CARTESIAN_POINT('Ctrl Pts',(-0.228101094000056,15.2,-10.753055307));
#296924=CARTESIAN_POINT('Ctrl Pts',(-0.228858176000056,15.2,-10.75548866));
#296925=CARTESIAN_POINT('Ctrl Pts',(-0.229619150000057,15.2,-10.757927163));
#296926=CARTESIAN_POINT('Ctrl Pts',(-0.230384020000055,15.2,-10.760370801));
#296927=CARTESIAN_POINT('Ctrl Pts',(-0.231152793000057,15.2,-10.76281956));
#296928=CARTESIAN_POINT('Ctrl Pts',(-0.231925472000055,15.2,-10.765273428));
#296929=CARTESIAN_POINT('Ctrl Pts',(-0.232702064000057,15.2,-10.767732388));
#296930=CARTESIAN_POINT('Ctrl Pts',(-0.233482574000057,15.2,-10.770196429));
#296931=CARTESIAN_POINT('Ctrl Pts',(-0.234267006000056,15.2,-10.772665536));
#296932=CARTESIAN_POINT('Ctrl Pts',(-0.235055365000055,15.2,-10.775139696));
#296933=CARTESIAN_POINT('Ctrl Pts',(-0.235847657000056,15.2,-10.777618895));
#296934=CARTESIAN_POINT('Ctrl Pts',(-0.236643888000057,15.2,-10.780103119));
#296935=CARTESIAN_POINT('Ctrl Pts',(-0.237444060000056,15.2,-10.782592355));
#296936=CARTESIAN_POINT('Ctrl Pts',(-0.238248181000056,15.2,-10.78508659));
#296937=CARTESIAN_POINT('Ctrl Pts',(-0.239056253000056,15.2,-10.78758581));
#296938=CARTESIAN_POINT('Ctrl Pts',(-0.239868284000057,15.2,-10.790090001));
#296939=CARTESIAN_POINT('Ctrl Pts',(-0.240684278000056,15.2,-10.79259915));
#296940=CARTESIAN_POINT('Ctrl Pts',(-0.241504238000055,15.2,-10.795113244));
#296941=CARTESIAN_POINT('Ctrl Pts',(-0.242328171000056,15.2,-10.797632269));
#296942=CARTESIAN_POINT('Ctrl Pts',(-0.243156080000055,15.2,-10.800156212));
#296943=CARTESIAN_POINT('Ctrl Pts',(-0.243987973000056,15.2,-10.80268506));
#296944=CARTESIAN_POINT('Ctrl Pts',(-0.244823851000057,15.2,-10.805218799));
#296945=CARTESIAN_POINT('Ctrl Pts',(-0.245663721000057,15.2,-10.807757416));
#296946=CARTESIAN_POINT('Ctrl Pts',(-0.246507587000057,15.2,-10.810300898));
#296947=CARTESIAN_POINT('Ctrl Pts',(-0.247355454000056,15.2,-10.812849232));
#296948=CARTESIAN_POINT('Ctrl Pts',(-0.248207327000056,15.2,-10.815402404));
#296949=CARTESIAN_POINT('Ctrl Pts',(-0.249063210000056,15.2,-10.817960403));
#296950=CARTESIAN_POINT('Ctrl Pts',(-0.249923109000055,15.2,-10.820523213));
#296951=CARTESIAN_POINT('Ctrl Pts',(-0.250787027000056,15.2,-10.823090823));
#296952=CARTESIAN_POINT('Ctrl Pts',(-0.251654969000056,15.2,-10.825663219));
#296953=CARTESIAN_POINT('Ctrl Pts',(-0.252526940000056,15.2,-10.828240388));
#296954=CARTESIAN_POINT('Ctrl Pts',(-0.253402945000056,15.2,-10.830822318));
#296955=CARTESIAN_POINT('Ctrl Pts',(-0.254282988000056,15.2,-10.833408995));
#296956=CARTESIAN_POINT('Ctrl Pts',(-0.255167073000055,15.2,-10.836000406));
#296957=CARTESIAN_POINT('Ctrl Pts',(-0.256055206000055,15.2,-10.838596538));
#296958=CARTESIAN_POINT('Ctrl Pts',(-0.256947390000055,15.2,-10.84119738));
#296959=CARTESIAN_POINT('Ctrl Pts',(-0.257843631000056,15.2,-10.843802918));
#296960=CARTESIAN_POINT('Ctrl Pts',(-0.258743931000056,15.2,-10.846413139));
#296961=CARTESIAN_POINT('Ctrl Pts',(-0.259648297000057,15.2,-10.84902803));
#296962=CARTESIAN_POINT('Ctrl Pts',(-0.260556733000056,15.2,-10.851647578));
#296963=CARTESIAN_POINT('Ctrl Pts',(-0.261469242000055,15.2,-10.854271772));
#296964=CARTESIAN_POINT('Ctrl Pts',(-0.262385828000056,15.2,-10.856900598));
#296965=CARTESIAN_POINT('Ctrl Pts',(-0.263306498000055,15.2,-10.859534042));
#296966=CARTESIAN_POINT('Ctrl Pts',(-0.264231255000055,15.2,-10.862172095));
#296967=CARTESIAN_POINT('Ctrl Pts',(-0.265160103000056,15.2,-10.864814742));
#296968=CARTESIAN_POINT('Ctrl Pts',(-0.266093047000057,15.2,-10.86746197));
#296969=CARTESIAN_POINT('Ctrl Pts',(-0.267030089000055,15.2,-10.870113767));
#296970=CARTESIAN_POINT('Ctrl Pts',(-0.267971237000056,15.2,-10.872770121));
#296971=CARTESIAN_POINT('Ctrl Pts',(-0.268916493000055,15.2,-10.87543102));
#296972=CARTESIAN_POINT('Ctrl Pts',(-0.269865860000056,15.2,-10.878096449));
#296973=CARTESIAN_POINT('Ctrl Pts',(-0.270819345000056,15.2,-10.880766398));
#296974=CARTESIAN_POINT('Ctrl Pts',(-0.271776951000057,15.2,-10.883440854));
#296975=CARTESIAN_POINT('Ctrl Pts',(-0.272738681000056,15.2,-10.886119805));
#296976=CARTESIAN_POINT('Ctrl Pts',(-0.273704541000056,15.2,-10.888803238));
#296977=CARTESIAN_POINT('Ctrl Pts',(-0.274674534000056,15.2,-10.891491141));
#296978=CARTESIAN_POINT('Ctrl Pts',(-0.275648666000056,15.2,-10.8941835));
#296979=CARTESIAN_POINT('Ctrl Pts',(-0.276626937000056,15.2,-10.896880306));
#296980=CARTESIAN_POINT('Ctrl Pts',(-0.277609355000056,15.2,-10.899581544));
#296981=CARTESIAN_POINT('Ctrl Pts',(-0.278595921000055,15.2,-10.902287203));
#296982=CARTESIAN_POINT('Ctrl Pts',(-0.279586642000057,15.2,-10.904997271));
#296983=CARTESIAN_POINT('Ctrl Pts',(-0.280581520000055,15.2,-10.907711734));
#296984=CARTESIAN_POINT('Ctrl Pts',(-0.281580560000056,15.2,-10.910430583));
#296985=CARTESIAN_POINT('Ctrl Pts',(-0.282583766000055,15.2,-10.913153802));
#296986=CARTESIAN_POINT('Ctrl Pts',(-0.283591141000056,15.2,-10.915881383));
#296987=CARTESIAN_POINT('Ctrl Pts',(-0.284602690000056,15.2,-10.918613312));
#296988=CARTESIAN_POINT('Ctrl Pts',(-0.285618416000055,15.2,-10.921349576));
#296989=CARTESIAN_POINT('Ctrl Pts',(-0.286638323000057,15.2,-10.924090164));
#296990=CARTESIAN_POINT('Ctrl Pts',(-0.287662415000056,15.2,-10.926835064));
#296991=CARTESIAN_POINT('Ctrl Pts',(-0.288690696000057,15.2,-10.929584264));
#296992=CARTESIAN_POINT('Ctrl Pts',(-0.289723171000055,15.2,-10.932337751));
#296993=CARTESIAN_POINT('Ctrl Pts',(-0.290759842000057,15.2,-10.935095515));
#296994=CARTESIAN_POINT('Ctrl Pts',(-0.291800713000056,15.2,-10.937857543));
#296995=CARTESIAN_POINT('Ctrl Pts',(-0.292845789000056,15.2,-10.940623823));
#296996=CARTESIAN_POINT('Ctrl Pts',(-0.293895073000057,15.2,-10.943394344));
#296997=CARTESIAN_POINT('Ctrl Pts',(-0.294948568000055,15.2,-10.946169093));
#296998=CARTESIAN_POINT('Ctrl Pts',(-0.296006280000055,15.2,-10.948948059));
#296999=CARTESIAN_POINT('Ctrl Pts',(-0.297068210000055,15.2,-10.951731231));
#297000=CARTESIAN_POINT('Ctrl Pts',(-0.298134363000055,15.2,-10.954518595));
#297001=CARTESIAN_POINT('Ctrl Pts',(-0.299204743000056,15.2,-10.957310141));
#297002=CARTESIAN_POINT('Ctrl Pts',(-0.300279354000056,15.2,-10.960105857));
#297003=CARTESIAN_POINT('Ctrl Pts',(-0.301358198000056,15.2,-10.962905731));
#297004=CARTESIAN_POINT('Ctrl Pts',(-0.302441280000056,15.2,-10.965709752));
#297005=CARTESIAN_POINT('Ctrl Pts',(-0.303528603000055,15.2,-10.968517907));
#297006=CARTESIAN_POINT('Ctrl Pts',(-0.304620171000056,15.2,-10.971330186));
#297007=CARTESIAN_POINT('Ctrl Pts',(-0.305715987000056,15.2,-10.974146576));
#297008=CARTESIAN_POINT('Ctrl Pts',(-0.306816056000055,15.2,-10.976967067));
#297009=CARTESIAN_POINT('Ctrl Pts',(-0.307920380000055,15.2,-10.979791646));
#297010=CARTESIAN_POINT('Ctrl Pts',(-0.309028962000056,15.2,-10.982620303));
#297011=CARTESIAN_POINT('Ctrl Pts',(-0.310141808000056,15.2,-10.985453024));
#297012=CARTESIAN_POINT('Ctrl Pts',(-0.311258919000055,15.2,-10.988289801));
#297013=CARTESIAN_POINT('Ctrl Pts',(-0.312380301000056,15.2,-10.991130619));
#297014=CARTESIAN_POINT('Ctrl Pts',(-0.313505954000056,15.2,-10.993975469));
#297015=CARTESIAN_POINT('Ctrl Pts',(-0.314635885000056,15.2,-10.996824339));
#297016=CARTESIAN_POINT('Ctrl Pts',(-0.315770096000056,15.2,-10.999677217));
#297017=CARTESIAN_POINT('Ctrl Pts',(-0.316908589000056,15.2,-11.002534092));
#297018=CARTESIAN_POINT('Ctrl Pts',(-0.318051369000055,15.2,-11.005394953));
#297019=CARTESIAN_POINT('Ctrl Pts',(-0.319198440000056,15.2,-11.008259788));
#297020=CARTESIAN_POINT('Ctrl Pts',(-0.320349803000056,15.2,-11.011128588));
#297021=CARTESIAN_POINT('Ctrl Pts',(-0.321505465000056,15.2,-11.014001338));
#297022=CARTESIAN_POINT('Ctrl Pts',(-0.322665426000055,15.2,-11.01687803));
#297023=CARTESIAN_POINT('Ctrl Pts',(-0.323829689000057,15.2,-11.01975865));
#297024=CARTESIAN_POINT('Ctrl Pts',(-0.324998260000056,15.2,-11.022643189));
#297025=CARTESIAN_POINT('Ctrl Pts',(-0.326171142000057,15.2,-11.025531635));
#297026=CARTESIAN_POINT('Ctrl Pts',(-0.327348336000056,15.2,-11.028423977));
#297027=CARTESIAN_POINT('Ctrl Pts',(-0.328529847000055,15.2,-11.031320204));
#297028=CARTESIAN_POINT('Ctrl Pts',(-0.329715678000057,15.2,-11.034220304));
#297029=CARTESIAN_POINT('Ctrl Pts',(-0.330905831000056,15.2,-11.037124266));
#297030=CARTESIAN_POINT('Ctrl Pts',(-0.332100311000056,15.2,-11.040032081));
#297031=CARTESIAN_POINT('Ctrl Pts',(-0.333299121000056,15.2,-11.042943735));
#297032=CARTESIAN_POINT('Ctrl Pts',(-0.334502263000056,15.2,-11.045859219));
#297033=CARTESIAN_POINT('Ctrl Pts',(-0.335709740000055,15.2,-11.048778521));
#297034=CARTESIAN_POINT('Ctrl Pts',(-0.336921557000055,15.2,-11.051701631));
#297035=CARTESIAN_POINT('Ctrl Pts',(-0.338137716000055,15.2,-11.054628537));
#297036=CARTESIAN_POINT('Ctrl Pts',(-0.339358220000056,15.2,-11.057559229));
#297037=CARTESIAN_POINT('Ctrl Pts',(-0.340583073000056,15.2,-11.060493695));
#297038=CARTESIAN_POINT('Ctrl Pts',(-0.341812276000055,15.2,-11.063431925));
#297039=CARTESIAN_POINT('Ctrl Pts',(-0.343045833000056,15.2,-11.066373907));
#297040=CARTESIAN_POINT('Ctrl Pts',(-0.344283750000055,15.2,-11.069319632));
#297041=CARTESIAN_POINT('Ctrl Pts',(-0.345526025000057,15.2,-11.072269087));
#297042=CARTESIAN_POINT('Ctrl Pts',(-0.346772665000056,15.2,-11.075222262));
#297043=CARTESIAN_POINT('Ctrl Pts',(-0.348023671000056,15.2,-11.078179147));
#297044=CARTESIAN_POINT('Ctrl Pts',(-0.349279047000056,15.2,-11.08113973));
#297045=CARTESIAN_POINT('Ctrl Pts',(-0.350538795000055,15.2,-11.084104002));
#297046=CARTESIAN_POINT('Ctrl Pts',(-0.351802919000056,15.2,-11.08707195));
#297047=CARTESIAN_POINT('Ctrl Pts',(-0.353071422000056,15.2,-11.090043565));
#297048=CARTESIAN_POINT('Ctrl Pts',(-0.354344305000056,15.2,-11.093018835));
#297049=CARTESIAN_POINT('Ctrl Pts',(-0.355621573000056,15.2,-11.09599775));
#297050=CARTESIAN_POINT('Ctrl Pts',(-0.356903229000055,15.2,-11.0989803));
#297051=CARTESIAN_POINT('Ctrl Pts',(-0.358189274000056,15.2,-11.101966474));
#297052=CARTESIAN_POINT('Ctrl Pts',(-0.359479712000056,15.2,-11.104956259));
#297053=CARTESIAN_POINT('Ctrl Pts',(-0.360774547000055,15.2,-11.107949648));
#297054=CARTESIAN_POINT('Ctrl Pts',(-0.362073780000056,15.2,-11.110946628));
#297055=CARTESIAN_POINT('Ctrl Pts',(-0.363377414000056,15.2,-11.11394719));
#297056=CARTESIAN_POINT('Ctrl Pts',(-0.364685453000057,15.2,-11.116951323));
#297057=CARTESIAN_POINT('Ctrl Pts',(-0.365997899000057,15.2,-11.119959015));
#297058=CARTESIAN_POINT('Ctrl Pts',(-0.367314756000056,15.2,-11.122970257));
#297059=CARTESIAN_POINT('Ctrl Pts',(-0.368636025000055,15.2,-11.125985039));
#297060=CARTESIAN_POINT('Ctrl Pts',(-0.369961710000055,15.2,-11.129003349));
#297061=CARTESIAN_POINT('Ctrl Pts',(-0.371291813000055,15.2,-11.132025177));
#297062=CARTESIAN_POINT('Ctrl Pts',(-0.372626336000056,15.2,-11.135050513));
#297063=CARTESIAN_POINT('Ctrl Pts',(-0.373965284000055,15.2,-11.138079346));
#297064=CARTESIAN_POINT('Ctrl Pts',(-0.375308659000056,15.2,-11.141111667));
#297065=CARTESIAN_POINT('Ctrl Pts',(-0.376656462000057,15.2,-11.144147464));
#297066=CARTESIAN_POINT('Ctrl Pts',(-0.378008697000055,15.2,-11.147186726));
#297067=CARTESIAN_POINT('Ctrl Pts',(-0.379365367000055,15.2,-11.150229445));
#297068=CARTESIAN_POINT('Ctrl Pts',(-0.380726475000056,15.2,-11.153275611));
#297069=CARTESIAN_POINT('Ctrl Pts',(-0.382092022000055,15.2,-11.156325211));
#297070=CARTESIAN_POINT('Ctrl Pts',(-0.383462012000055,15.2,-11.159378235));
#297071=CARTESIAN_POINT('Ctrl Pts',(-0.384836446000056,15.2,-11.162434675));
#297072=CARTESIAN_POINT('Ctrl Pts',(-0.386215329000056,15.2,-11.165494519));
#297073=CARTESIAN_POINT('Ctrl Pts',(-0.387598661000055,15.2,-11.168557756));
#297074=CARTESIAN_POINT('Ctrl Pts',(-0.388986447000056,15.2,-11.171624379));
#297075=CARTESIAN_POINT('Ctrl Pts',(-0.390378688000055,15.2,-11.174694374));
#297076=CARTESIAN_POINT('Ctrl Pts',(-0.391775388000056,15.2,-11.177767733));
#297077=CARTESIAN_POINT('Ctrl Pts',(-0.393176547000056,15.2,-11.180844447));
#297078=CARTESIAN_POINT('Ctrl Pts',(-0.394582170000056,15.2,-11.183924502));
#297079=CARTESIAN_POINT('Ctrl Pts',(-0.395992258000056,15.2,-11.187007892));
#297080=CARTESIAN_POINT('Ctrl Pts',(-0.397406814000056,15.2,-11.190094604));
#297081=CARTESIAN_POINT('Ctrl Pts',(-0.398825842000056,15.2,-11.193184629));
#297082=CARTESIAN_POINT('Ctrl Pts',(-0.400249343000055,15.2,-11.196277957));
#297083=CARTESIAN_POINT('Ctrl Pts',(-0.401677318000055,15.2,-11.199374578));
#297084=CARTESIAN_POINT('Ctrl Pts',(-0.403109771000055,15.2,-11.202474481));
#297085=CARTESIAN_POINT('Ctrl Pts',(-0.404546705000056,15.2,-11.205577658));
#297086=CARTESIAN_POINT('Ctrl Pts',(-0.405988122000055,15.2,-11.208684097));
#297087=CARTESIAN_POINT('Ctrl Pts',(-0.407434025000055,15.2,-11.211793789));
#297088=CARTESIAN_POINT('Ctrl Pts',(-0.408884415000056,15.2,-11.214906723));
#297089=CARTESIAN_POINT('Ctrl Pts',(-0.410339295000056,15.2,-11.21802289));
#297090=CARTESIAN_POINT('Ctrl Pts',(-0.411798667000056,15.2,-11.221142281));
#297091=CARTESIAN_POINT('Ctrl Pts',(-0.413262534000056,15.2,-11.224264883));
#297092=CARTESIAN_POINT('Ctrl Pts',(-0.414730899000055,15.2,-11.22739069));
#297093=CARTESIAN_POINT('Ctrl Pts',(-0.416203762000055,15.2,-11.230519688));
#297094=CARTESIAN_POINT('Ctrl Pts',(-0.417681127000057,15.2,-11.233651872));
#297095=CARTESIAN_POINT('Ctrl Pts',(-0.419162997000055,15.2,-11.236787227));
#297096=CARTESIAN_POINT('Ctrl Pts',(-0.420649373000056,15.2,-11.239925747));
#297097=CARTESIAN_POINT('Ctrl Pts',(-0.422140258000056,15.2,-11.243067421));
#297098=CARTESIAN_POINT('Ctrl Pts',(-0.423635654000056,15.2,-11.246212238));
#297099=CARTESIAN_POINT('Ctrl Pts',(-0.425135562000056,15.2,-11.249360189));
#297100=CARTESIAN_POINT('Ctrl Pts',(-0.426639987000056,15.2,-11.252511265));
#297101=CARTESIAN_POINT('Ctrl Pts',(-0.428148929000055,15.2,-11.255665455));
#297102=CARTESIAN_POINT('Ctrl Pts',(-0.429662391000055,15.2,-11.258822751));
#297103=CARTESIAN_POINT('Ctrl Pts',(-0.431180374000055,15.2,-11.261983141));
#297104=CARTESIAN_POINT('Ctrl Pts',(-0.432702884000056,15.2,-11.265146617));
#297105=CARTESIAN_POINT('Ctrl Pts',(-0.434229918000056,15.2,-11.268313169));
#297106=CARTESIAN_POINT('Ctrl Pts',(-0.435761482000055,15.2,-11.271482787));
#297107=CARTESIAN_POINT('Ctrl Pts',(-0.437297576000055,15.2,-11.274655461));
#297108=CARTESIAN_POINT('Ctrl Pts',(-0.438838204000056,15.2,-11.277831182));
#297109=CARTESIAN_POINT('Ctrl Pts',(-0.440383367000056,15.2,-11.281009939));
#297110=CARTESIAN_POINT('Ctrl Pts',(-0.441933068000055,15.2,-11.284191725));
#297111=CARTESIAN_POINT('Ctrl Pts',(-0.443487307000057,15.2,-11.287376529));
#297112=CARTESIAN_POINT('Ctrl Pts',(-0.445046088000056,15.2,-11.290564341));
#297113=CARTESIAN_POINT('Ctrl Pts',(-0.446609414000055,15.2,-11.293755152));
#297114=CARTESIAN_POINT('Ctrl Pts',(-0.448177284000056,15.2,-11.296948952));
#297115=CARTESIAN_POINT('Ctrl Pts',(-0.449749702000056,15.2,-11.300145731));
#297116=CARTESIAN_POINT('Ctrl Pts',(-0.451326671000055,15.2,-11.303345481));
#297117=CARTESIAN_POINT('Ctrl Pts',(-0.452908191000055,15.2,-11.306548191));
#297118=CARTESIAN_POINT('Ctrl Pts',(-0.454494265000056,15.2,-11.309753853));
#297119=CARTESIAN_POINT('Ctrl Pts',(-0.456084896000055,15.2,-11.312962457));
#297120=CARTESIAN_POINT('Ctrl Pts',(-0.457680085000056,15.2,-11.316173992));
#297121=CARTESIAN_POINT('Ctrl Pts',(-0.459279833000057,15.2,-11.319388451));
#297122=CARTESIAN_POINT('Ctrl Pts',(-0.460884143000057,15.2,-11.322605822));
#297123=CARTESIAN_POINT('Ctrl Pts',(-0.462493018000056,15.2,-11.325826098));
#297124=CARTESIAN_POINT('Ctrl Pts',(-0.464106457000056,15.2,-11.329049269));
#297125=CARTESIAN_POINT('Ctrl Pts',(-0.465724466000056,15.2,-11.332275325));
#297126=CARTESIAN_POINT('Ctrl Pts',(-0.467347044000055,15.2,-11.335504256));
#297127=CARTESIAN_POINT('Ctrl Pts',(-0.468974194000056,15.2,-11.338736054));
#297128=CARTESIAN_POINT('Ctrl Pts',(-0.470605918000055,15.2,-11.341970709));
#297129=CARTESIAN_POINT('Ctrl Pts',(-0.472242218000056,15.2,-11.345208212));
#297130=CARTESIAN_POINT('Ctrl Pts',(-0.473883095000056,15.2,-11.348448553));
#297131=CARTESIAN_POINT('Ctrl Pts',(-0.475528552000055,15.2,-11.351691723));
#297132=CARTESIAN_POINT('Ctrl Pts',(-0.477178589000056,15.2,-11.354937714));
#297133=CARTESIAN_POINT('Ctrl Pts',(-0.478833210000056,15.2,-11.358186515));
#297134=CARTESIAN_POINT('Ctrl Pts',(-0.480492416000056,15.2,-11.361438118));
#297135=CARTESIAN_POINT('Ctrl Pts',(-0.482156209000056,15.2,-11.364692512));
#297136=CARTESIAN_POINT('Ctrl Pts',(-0.483824592000056,15.2,-11.367949691));
#297137=CARTESIAN_POINT('Ctrl Pts',(-0.485497564000056,15.2,-11.371209642));
#297138=CARTESIAN_POINT('Ctrl Pts',(-0.487175129000056,15.2,-11.374472358));
#297139=CARTESIAN_POINT('Ctrl Pts',(-0.488857288000055,15.2,-11.377737829));
#297140=CARTESIAN_POINT('Ctrl Pts',(-0.490544043000056,15.2,-11.381006047));
#297141=CARTESIAN_POINT('Ctrl Pts',(-0.492235397000057,15.2,-11.384277003));
#297142=CARTESIAN_POINT('Ctrl Pts',(-0.493931349000055,15.2,-11.387550685));
#297143=CARTESIAN_POINT('Ctrl Pts',(-0.495631904000057,15.2,-11.390827086));
#297144=CARTESIAN_POINT('Ctrl Pts',(-0.497337060000056,15.2,-11.394106196));
#297145=CARTESIAN_POINT('Ctrl Pts',(-0.499046823000056,15.2,-11.397388008));
#297146=CARTESIAN_POINT('Ctrl Pts',(-0.500761192000055,15.2,-11.400672511));
#297147=CARTESIAN_POINT('Ctrl Pts',(-0.502480169000057,15.2,-11.403959697));
#297148=CARTESIAN_POINT('Ctrl Pts',(-0.504203756000056,15.2,-11.407249556));
#297149=CARTESIAN_POINT('Ctrl Pts',(-0.505931954000056,15.2,-11.410542081));
#297150=CARTESIAN_POINT('Ctrl Pts',(-0.507664766000057,15.2,-11.413837262));
#297151=CARTESIAN_POINT('Ctrl Pts',(-0.509402194000056,15.2,-11.417135088));
#297152=CARTESIAN_POINT('Ctrl Pts',(-0.511144239000056,15.2,-11.420435551));
#297153=CARTESIAN_POINT('Ctrl Pts',(-0.512890901000055,15.2,-11.423738642));
#297154=CARTESIAN_POINT('Ctrl Pts',(-0.514642185000056,15.2,-11.427044351));
#297155=CARTESIAN_POINT('Ctrl Pts',(-0.516398090000055,15.2,-11.43035267));
#297156=CARTESIAN_POINT('Ctrl Pts',(-0.518158619000056,15.2,-11.433663589));
#297157=CARTESIAN_POINT('Ctrl Pts',(-0.519923771000055,15.2,-11.436977103));
#297158=CARTESIAN_POINT('Ctrl Pts',(-0.521693552000055,15.2,-11.4402932));
#297159=CARTESIAN_POINT('Ctrl Pts',(-0.523467959000056,15.2,-11.443611875));
#297160=CARTESIAN_POINT('Ctrl Pts',(-0.525246997000056,15.2,-11.446933118));
#297161=CARTESIAN_POINT('Ctrl Pts',(-0.527030665000057,15.2,-11.450256921));
#297162=CARTESIAN_POINT('Ctrl Pts',(-0.528818965000056,15.2,-11.453583273));
#297163=CARTESIAN_POINT('Ctrl Pts',(-0.530611902000055,15.2,-11.456912162));
#297164=CARTESIAN_POINT('Ctrl Pts',(-0.532409474000056,15.2,-11.460243578));
#297165=CARTESIAN_POINT('Ctrl Pts',(-0.534211686000056,15.2,-11.46357751));
#297166=CARTESIAN_POINT('Ctrl Pts',(-0.536018537000055,15.2,-11.466913949));
#297167=CARTESIAN_POINT('Ctrl Pts',(-0.537830030000055,15.2,-11.470252887));
#297168=CARTESIAN_POINT('Ctrl Pts',(-0.539646167000055,15.2,-11.473594318));
#297169=CARTESIAN_POINT('Ctrl Pts',(-0.541466946000057,15.2,-11.476938237));
#297170=CARTESIAN_POINT('Ctrl Pts',(-0.543292369000056,15.2,-11.480284643));
#297171=CARTESIAN_POINT('Ctrl Pts',(-0.544756421000056,15.2,-11.482963757));
#297172=CARTESIAN_POINT('Ctrl Pts',(-0.545856551000057,15.2,-11.484974209));
#297173=CARTESIAN_POINT('Ctrl Pts',(-0.546590899000057,15.2,-11.486315008));
#297174=CARTESIAN_POINT('Ctrl Pts',(-0.546958306000055,15.2,-11.486985532));
#297175=CARTESIAN_POINT('',(-0.929795809014353,15.2,-11.4623505335096));
#297176=CARTESIAN_POINT('Origin',(-5.66257110645729E-14,15.2,-1.77635683940025E-14));
#297177=CARTESIAN_POINT('Ctrl Pts',(-1.18690176600006,15.2,-10.306885524));
#297178=CARTESIAN_POINT('Ctrl Pts',(-1.18695287825247,15.2,-10.3086714504511));
#297179=CARTESIAN_POINT('Ctrl Pts',(-1.18700024431844,15.2,-10.3105146700777));
#297180=CARTESIAN_POINT('Ctrl Pts',(-1.18704320796202,15.2,-10.3124142312835));
#297181=CARTESIAN_POINT('Ctrl Pts',(-1.18708637879801,15.2,-10.3143229531337));
#297182=CARTESIAN_POINT('Ctrl Pts',(-1.18712509994175,15.2,-10.3162885639395));
#297183=CARTESIAN_POINT('Ctrl Pts',(-1.1871587090283,15.2,-10.3183101249039));
#297184=CARTESIAN_POINT('Ctrl Pts',(-1.1871923181118,15.2,-10.3203316856847));
#297185=CARTESIAN_POINT('Ctrl Pts',(-1.18722081733423,15.2,-10.322409198819));
#297186=CARTESIAN_POINT('Ctrl Pts',(-1.18724356650007,15.2,-10.3245417524916));
#297187=CARTESIAN_POINT('Ctrl Pts',(-1.18726631566591,15.2,-10.3266743061641));
#297188=CARTESIAN_POINT('Ctrl Pts',(-1.18728331741518,15.1999999999999,
-10.3288618993474));
#297189=CARTESIAN_POINT('Ctrl Pts',(-1.18729394974902,15.2,-10.3311036472915));
#297190=CARTESIAN_POINT('Ctrl Pts',(-1.18730458208384,15.2,-10.3333453954392));
#297191=CARTESIAN_POINT('Ctrl Pts',(-1.18730884758373,15.2,-10.335641298191));
#297192=CARTESIAN_POINT('Ctrl Pts',(-1.18730614774977,15.2,-10.3379904903227));
#297193=CARTESIAN_POINT('Ctrl Pts',(-1.18730344791606,15.2,-10.3403396822409));
#297194=CARTESIAN_POINT('Ctrl Pts',(-1.18729378039953,15.2,-10.3427421643207));
#297195=CARTESIAN_POINT('Ctrl Pts',(-1.18727656873339,15.2,-10.3451970944927));
#297196=CARTESIAN_POINT('Ctrl Pts',(-1.18725935706726,15.2,-10.3476520246647));
#297197=CARTESIAN_POINT('Ctrl Pts',(-1.18723459815028,15.2,-10.3501594023475));
#297198=CARTESIAN_POINT('Ctrl Pts',(-1.18720173348516,15.2,-10.3527184083357));
#297199=CARTESIAN_POINT('Ctrl Pts',(-1.18716886881705,15.2,-10.3552774145562));
#297200=CARTESIAN_POINT('Ctrl Pts',(-1.18712789608962,15.2,-10.3578880464332));
#297201=CARTESIAN_POINT('Ctrl Pts',(-1.18707827150299,15.2,-10.3605495048317));
#297202=CARTESIAN_POINT('Ctrl Pts',(-1.18702864692087,15.2,-10.3632109629885));
#297203=CARTESIAN_POINT('Ctrl Pts',(-1.18697036877764,15.2,-10.3659232462155));
#297204=CARTESIAN_POINT('Ctrl Pts',(-1.18690291127969,15.2,-10.3686855726173));
#297205=CARTESIAN_POINT('Ctrl Pts',(-1.18683545378174,15.2,-10.3714478990192));
#297206=CARTESIAN_POINT('Ctrl Pts',(-1.18675881418451,15.2,-10.3742602688836));
#297207=CARTESIAN_POINT('Ctrl Pts',(-1.18667248268807,15.2,-10.3771219181108));
#297208=CARTESIAN_POINT('Ctrl Pts',(-1.18658615119163,15.2,-10.379983567338));
#297209=CARTESIAN_POINT('Ctrl Pts',(-1.18649012644043,15.2,-10.3828944944465));
#297210=CARTESIAN_POINT('Ctrl Pts',(-1.18638390927832,15.2,-10.385853953919));
#297211=CARTESIAN_POINT('Ctrl Pts',(-1.18627769210655,15.2,-10.3888134136604));
#297212=CARTESIAN_POINT('Ctrl Pts',(-1.18616128558383,15.2,-10.3918214053147));
#297213=CARTESIAN_POINT('Ctrl Pts',(-1.1860342042431,15.2,-10.39487719815));
#297214=CARTESIAN_POINT('Ctrl Pts',(-1.18590712291392,15.2,-10.3979329907077));
#297215=CARTESIAN_POINT('Ctrl Pts',(-1.18576936691205,15.2,-10.4010365852655));
#297216=CARTESIAN_POINT('Ctrl Pts',(-1.18562046775014,15.2,-10.4041872659985));
#297217=CARTESIAN_POINT('Ctrl Pts',(-1.18547156858824,15.2,-10.4073379467315));
#297218=CARTESIAN_POINT('Ctrl Pts',(-1.18531152576172,15.2,-10.410535714918));
#297219=CARTESIAN_POINT('Ctrl Pts',(-1.18513988276875,15.2,-10.4137798696303));
#297220=CARTESIAN_POINT('Ctrl Pts',(-1.18496823976018,15.2,-10.4170240246374));
#297221=CARTESIAN_POINT('Ctrl Pts',(-1.18478499820055,15.2,-10.4203145675565));
#297222=CARTESIAN_POINT('Ctrl Pts',(-1.18458971402272,15.2,-10.423650812657));
#297223=CARTESIAN_POINT('Ctrl Pts',(-1.18439442986262,15.2,-10.4269870574544));
#297224=CARTESIAN_POINT('Ctrl Pts',(-1.18418710221816,15.2,-10.4303690046824));
#297225=CARTESIAN_POINT('Ctrl Pts',(-1.18396730047518,15.2,-10.43379598349));
#297226=CARTESIAN_POINT('Ctrl Pts',(-1.18374749873219,15.2,-10.4372229622977));
#297227=CARTESIAN_POINT('Ctrl Pts',(-1.18351522376701,15.2,-10.4406949718391));
#297228=CARTESIAN_POINT('Ctrl Pts',(-1.1832700567768,15.2,-10.444211356625));
#297229=CARTESIAN_POINT('Ctrl Pts',(-1.18302488976432,15.2,-10.4477277417303));
#297230=CARTESIAN_POINT('Ctrl Pts',(-1.18276682798624,15.2,-10.4512885011113));
#297231=CARTESIAN_POINT('Ctrl Pts',(-1.18249546795713,15.2,-10.4548929895737));
#297232=CARTESIAN_POINT('Ctrl Pts',(-1.18222410795266,15.2,-10.4584974777087));
#297233=CARTESIAN_POINT('Ctrl Pts',(-1.18193944638091,15.2,-10.4621456945924));
#297234=CARTESIAN_POINT('Ctrl Pts',(-1.18164108847508,15.2,-10.4658370095416));
#297235=CARTESIAN_POINT('Ctrl Pts',(-1.18124327792495,15.2,-10.4707587629189));
#297236=CARTESIAN_POINT('Ctrl Pts',(-1.1808211147739,15.2,-10.4757571319861));
#297237=CARTESIAN_POINT('Ctrl Pts',(-1.18037369100023,15.2,-10.4808306522732));
#297238=CARTESIAN_POINT('Ctrl Pts',(-1.1800381231776,15.2,-10.4846357924021));
#297239=CARTESIAN_POINT('Ctrl Pts',(-1.17968834555056,15.2,-10.4884832053535));
#297240=CARTESIAN_POINT('Ctrl Pts',(-1.17932398598146,15.2,-10.492372285376));
#297241=CARTESIAN_POINT('Ctrl Pts',(-1.17895962637926,15.2,-10.4962613657518));
#297242=CARTESIAN_POINT('Ctrl Pts',(-1.17858068606229,15.2,-10.5001921147587));
#297243=CARTESIAN_POINT('Ctrl Pts',(-1.17818680043694,15.2,-10.5041639364259));
#297244=CARTESIAN_POINT('Ctrl Pts',(-1.17785856243371,15.2,-10.5074737876349));
#297245=CARTESIAN_POINT('Ctrl Pts',(-1.1775199460886,15.2,-10.5108121629491));
#297246=CARTESIAN_POINT('Ctrl Pts',(-1.17717074796274,15.2,-10.5141787224653));
#297247=CARTESIAN_POINT('Ctrl Pts',(-1.17682154983687,15.2,-10.5175452819815));
#297248=CARTESIAN_POINT('Ctrl Pts',(-1.17646176907471,15.2,-10.520940028212));
#297249=CARTESIAN_POINT('Ctrl Pts',(-1.17609120372661,15.2,-10.5243626244643));
#297250=CARTESIAN_POINT('Ctrl Pts',(-1.1757206384189,15.2,-10.5277852203435));
#297251=CARTESIAN_POINT('Ctrl Pts',(-1.17533929147996,15.2,-10.5312356701097));
#297252=CARTESIAN_POINT('Ctrl Pts',(-1.1749469643014,15.2,-10.5347136418117));
#297253=CARTESIAN_POINT('Ctrl Pts',(-1.17455463708007,15.2,-10.5381916138928));
#297254=CARTESIAN_POINT('Ctrl Pts',(-1.1741513308756,15.2,-10.541697109029));
#297255=CARTESIAN_POINT('Ctrl Pts',(-1.17373685302929,15.2,-10.5452298043045));
#297256=CARTESIAN_POINT('Ctrl Pts',(-1.17332237518299,15.2,-10.5487624995801));
#297257=CARTESIAN_POINT('Ctrl Pts',(-1.17289672702737,15.2,-10.5523223925563));
#297258=CARTESIAN_POINT('Ctrl Pts',(-1.17245971832577,15.2,-10.5559091671087));
#297259=CARTESIAN_POINT('Ctrl Pts',(-1.17202270962417,15.2,-10.559495941661));
#297260=CARTESIAN_POINT('Ctrl Pts',(-1.17157434308505,15.2,-10.563109595319));
#297261=CARTESIAN_POINT('Ctrl Pts',(-1.17111443273843,15.2,-10.5667498133037));
#297262=CARTESIAN_POINT('Ctrl Pts',(-1.17056254029241,15.2,-10.5711180751234));
#297263=CARTESIAN_POINT('Ctrl Pts',(-1.16999402641933,15.2,-10.5755245905979));
#297264=CARTESIAN_POINT('Ctrl Pts',(-1.1694085782196,15.2,-10.579968822426));
#297265=CARTESIAN_POINT('Ctrl Pts',(-1.16892070479959,15.2,-10.583672348344));
#297266=CARTESIAN_POINT('Ctrl Pts',(-1.16842107412137,15.2,-10.5874020667535));
#297267=CARTESIAN_POINT('Ctrl Pts',(-1.167909508067,15.2,-10.5911576717587));
#297268=CARTESIAN_POINT('Ctrl Pts',(-1.16739794195686,15.2,-10.5949132771732));
#297269=CARTESIAN_POINT('Ctrl Pts',(-1.16687444269685,15.2,-10.5986947696602));
#297270=CARTESIAN_POINT('Ctrl Pts',(-1.16633883658673,15.2,-10.6025018445192));
#297271=CARTESIAN_POINT('Ctrl Pts',(-1.16569610921955,15.2,-10.6070703345991));
#297272=CARTESIAN_POINT('Ctrl Pts',(-1.16503595023964,15.2,-10.6116756682454));
#297273=CARTESIAN_POINT('Ctrl Pts',(-1.16435806500113,15.2,-10.6163173283991));
#297274=CARTESIAN_POINT('Ctrl Pts',(-1.1637931606665,15.2,-10.6201853783163));
#297275=CARTESIAN_POINT('Ctrl Pts',(-1.16321594966842,15.2,-10.6240786547382));
#297276=CARTESIAN_POINT('Ctrl Pts',(-1.16262626688962,15.2,-10.6279968652958));
#297277=CARTESIAN_POINT('Ctrl Pts',(-1.16203658411082,15.2,-10.6319150758534));
#297278=CARTESIAN_POINT('Ctrl Pts',(-1.16143442917626,15.2,-10.6358582204114));
#297279=CARTESIAN_POINT('Ctrl Pts',(-1.160819640703,15.2,-10.6398260084689));
#297280=CARTESIAN_POINT('Ctrl Pts',(-1.16020485222975,15.2,-10.6437937965265));
#297281=CARTESIAN_POINT('Ctrl Pts',(-1.15957743160628,15.2,-10.6477862292234));
#297282=CARTESIAN_POINT('Ctrl Pts',(-1.15893722042468,15.2,-10.651803019017));
#297283=CARTESIAN_POINT('Ctrl Pts',(-1.15816896703467,15.2,-10.6566231665943));
#297284=CARTESIAN_POINT('Ctrl Pts',(-1.15738229466934,15.2,-10.6614783887011));
#297285=CARTESIAN_POINT('Ctrl Pts',(-1.15657693744778,15.2,-10.6663681982749));
#297286=CARTESIAN_POINT('Ctrl Pts',(-1.15590580640544,15.2,-10.6704430397345));
#297287=CARTESIAN_POINT('Ctrl Pts',(-1.15522170016621,15.2,-10.6745418988963));
#297288=CARTESIAN_POINT('Ctrl Pts',(-1.15452446822108,15.2,-10.6786644979947));
#297289=CARTESIAN_POINT('Ctrl Pts',(-1.15396668271057,15.2,-10.6819625770039));
#297290=CARTESIAN_POINT('Ctrl Pts',(-1.15340049515609,15.2,-10.6852758510325));
#297291=CARTESIAN_POINT('Ctrl Pts',(-1.15282583234176,15.2,-10.6886041767588));
#297292=CARTESIAN_POINT('Ctrl Pts',(-1.15225116944913,15.2,-10.6919325029384));
#297293=CARTESIAN_POINT('Ctrl Pts',(-1.15166802957889,15.2,-10.6952758802129));
#297294=CARTESIAN_POINT('Ctrl Pts',(-1.15107633943497,15.2,-10.698634171508));
#297295=CARTESIAN_POINT('Ctrl Pts',(-1.15033672679538,15.2,-10.7028320353981));
#297296=CARTESIAN_POINT('Ctrl Pts',(-1.1495837529728,15.2,-10.7070531990154));
#297297=CARTESIAN_POINT('Ctrl Pts',(-1.14881727470821,15.2,-10.7112973930443));
#297298=CARTESIAN_POINT('Ctrl Pts',(-1.14805079644363,15.2,-10.7155415870733));
#297299=CARTESIAN_POINT('Ctrl Pts',(-1.14727081541518,15.2,-10.7198088116099));
#297300=CARTESIAN_POINT('Ctrl Pts',(-1.14647719016625,15.2,-10.7240987992564));
#297301=CARTESIAN_POINT('Ctrl Pts',(-1.14584229001901,15.2,-10.7275307890929));
#297302=CARTESIAN_POINT('Ctrl Pts',(-1.1451986568661,15.2,-10.7309773469649));
#297303=CARTESIAN_POINT('Ctrl Pts',(-1.14454622158668,15.2,-10.7344383379588));
#297304=CARTESIAN_POINT('Ctrl Pts',(-1.14389378621836,15.2,-10.7378993294243));
#297305=CARTESIAN_POINT('Ctrl Pts',(-1.14323254940177,15.2,-10.7413747540387));
#297306=CARTESIAN_POINT('Ctrl Pts',(-1.14256243942023,15.2,-10.7448644767854));
#297307=CARTESIAN_POINT('Ctrl Pts',(-1.14189232952998,15.2,-10.7483541990566));
#297308=CARTESIAN_POINT('Ctrl Pts',(-1.14121334901333,15.2,-10.7518582199831));
#297309=CARTESIAN_POINT('Ctrl Pts',(-1.14052542709153,15.2,-10.7553764064812));
#297310=CARTESIAN_POINT('Ctrl Pts',(-1.139837505076,15.2,-10.7588945934586));
#297311=CARTESIAN_POINT('Ctrl Pts',(-1.13914064425914,15.2,-10.7624269452319));
#297312=CARTESIAN_POINT('Ctrl Pts',(-1.1384347754423,15.2,-10.765973330815));
#297313=CARTESIAN_POINT('Ctrl Pts',(-1.13772890672164,15.2,-10.7695197159149));
#297314=CARTESIAN_POINT('Ctrl Pts',(-1.13701403064168,15.2,-10.773080135087));
#297315=CARTESIAN_POINT('Ctrl Pts',(-1.13629008136845,15.2,-10.7766544566822));
#297316=CARTESIAN_POINT('Ctrl Pts',(-1.13538514470294,15.2,-10.7811223590416));
#297317=CARTESIAN_POINT('Ctrl Pts',(-1.13446602963737,15.2,-10.7856119837191));
#297318=CARTESIAN_POINT('Ctrl Pts',(-1.13353261209173,15.2,-10.790123078943));
#297319=CARTESIAN_POINT('Ctrl Pts',(-1.13278587801452,15.2,-10.7937319553188));
#297320=CARTESIAN_POINT('Ctrl Pts',(-1.13202998984642,15.2,-10.7973545722789));
#297321=CARTESIAN_POINT('Ctrl Pts',(-1.13126488247079,15.2,-10.8009908017557));
#297322=CARTESIAN_POINT('Ctrl Pts',(-1.1304997751994,15.2,-10.8046270307371));
#297323=CARTESIAN_POINT('Ctrl Pts',(-1.12972545059653,15.2,-10.8082768706824));
#297324=CARTESIAN_POINT('Ctrl Pts',(-1.12894184466154,15.2,-10.8119401976594));
#297325=CARTESIAN_POINT('Ctrl Pts',(-1.12815823861978,15.2,-10.8156035251354));
#297326=CARTESIAN_POINT('Ctrl Pts',(-1.12736534972472,15.2,-10.819280336279));
#297327=CARTESIAN_POINT('Ctrl Pts',(-1.12656312023288,15.2,-10.8229705077191));
#297328=CARTESIAN_POINT('Ctrl Pts',(-1.12576089085034,15.2,-10.8266606786565));
#297329=CARTESIAN_POINT('Ctrl Pts',(-1.1249493176718,15.2,-10.8303642080502));
#297330=CARTESIAN_POINT('Ctrl Pts',(-1.12412834118432,15.2,-10.8340809711339));
#297331=CARTESIAN_POINT('Ctrl Pts',(-1.12330736458498,15.2,-10.8377977347241));
#297332=CARTESIAN_POINT('Ctrl Pts',(-1.12247698474864,15.2,-10.8415277334043));
#297333=CARTESIAN_POINT('Ctrl Pts',(-1.12163714075843,15.2,-10.845270839775));
#297334=CARTESIAN_POINT('Ctrl Pts',(-1.12079729676822,15.2,-10.8490139461456));
#297335=CARTESIAN_POINT('Ctrl Pts',(-1.11994799076579,15.2,-10.8527701631317));
#297336=CARTESIAN_POINT('Ctrl Pts',(-1.11908916088467,15.2,-10.8565393661162));
#297337=CARTESIAN_POINT('Ctrl Pts',(-1.11823033112057,15.2,-10.8603085685872));
#297338=CARTESIAN_POINT('Ctrl Pts',(-1.1173619804551,15.2,-10.8640907580737));
#297339=CARTESIAN_POINT('Ctrl Pts',(-1.11648404796736,15.2,-10.8678858117807));
#297340=CARTESIAN_POINT('Ctrl Pts',(-1.11560611536,15.2,-10.8716808660047));
#297341=CARTESIAN_POINT('Ctrl Pts',(-1.1147186030644,15.2,-10.8754887839373));
#297342=CARTESIAN_POINT('Ctrl Pts',(-1.11382145257007,15.2,-10.8793094449246));
#297343=CARTESIAN_POINT('Ctrl Pts',(-1.11292430219798,15.2,-10.8831301053914));
#297344=CARTESIAN_POINT('Ctrl Pts',(-1.11201751551881,15.2,-10.8869635091092));
#297345=CARTESIAN_POINT('Ctrl Pts',(-1.11110103431659,15.2,-10.8908095349607));
#297346=CARTESIAN_POINT('Ctrl Pts',(-1.1101845529895,15.2,-10.8946555613361));
#297347=CARTESIAN_POINT('Ctrl Pts',(-1.10925837840729,15.2,-10.8985142115119));
#297348=CARTESIAN_POINT('Ctrl Pts',(-1.10832245386423,15.2,-10.9023853640284));
#297349=CARTESIAN_POINT('Ctrl Pts',(-1.1073865294487,15.2,-10.9062565160176));
#297350=CARTESIAN_POINT('Ctrl Pts',(-1.10644085710492,15.2,-10.9101401728953));
#297351=CARTESIAN_POINT('Ctrl Pts',(-1.10548538062811,15.2,-10.9140362134649));
#297352=CARTESIAN_POINT('Ctrl Pts',(-1.10452990402112,15.2,-10.9179322545654));
#297353=CARTESIAN_POINT('Ctrl Pts',(-1.10356462468796,15.2,-10.9218406810645));
#297354=CARTESIAN_POINT('Ctrl Pts',(-1.10258948691195,15.2,-10.9257613741123));
#297355=CARTESIAN_POINT('Ctrl Pts',(-1.10161434926881,15.2,-10.9296820666259));
#297356=CARTESIAN_POINT('Ctrl Pts',(-1.10062935524985,15.2,-10.9336150266954));
#297357=CARTESIAN_POINT('Ctrl Pts',(-1.09963445138776,15.2,-10.9375601383716));
#297358=CARTESIAN_POINT('Ctrl Pts',(-1.0986395473901,15.2,-10.9415052505854));
#297359=CARTESIAN_POINT('Ctrl Pts',(-1.09763473318157,15.2,-10.9454625118544));
#297360=CARTESIAN_POINT('Ctrl Pts',(-1.09661995723274,15.2,-10.9494318094777));
#297361=CARTESIAN_POINT('Ctrl Pts',(-1.09560518142216,15.2,-10.9534011065601));
#297362=CARTESIAN_POINT('Ctrl Pts',(-1.0945804442281,15.2,-10.9573824381109));
#297363=CARTESIAN_POINT('Ctrl Pts',(-1.09354569320261,15.2,-10.9613756898387));
#297364=CARTESIAN_POINT('Ctrl Pts',(-1.09251094203613,15.2,-10.9653689421107));
#297365=CARTESIAN_POINT('Ctrl Pts',(-1.09146617741037,15.2,-10.9693741141449));
#297366=CARTESIAN_POINT('Ctrl Pts',(-1.09041135074177,15.2,-10.973391091975));
#297367=CARTESIAN_POINT('Ctrl Pts',(-1.08935652407317,15.2,-10.977408069805));
#297368=CARTESIAN_POINT('Ctrl Pts',(-1.08829163310617,15.2,-10.9814368537948));
#297369=CARTESIAN_POINT('Ctrl Pts',(-1.08721662982433,15.2,-10.9854773301273));
#297370=CARTESIAN_POINT('Ctrl Pts',(-1.08614162668895,15.2,-10.9895178059093));
#297371=CARTESIAN_POINT('Ctrl Pts',(-1.08505651033569,15.2,-10.9935699738332));
#297372=CARTESIAN_POINT('Ctrl Pts',(-1.08396123247584,15.2,-10.9976337229639));
#297373=CARTESIAN_POINT('Ctrl Pts',(-1.08286595446676,15.2,-11.0016974726482));
#297374=CARTESIAN_POINT('Ctrl Pts',(-1.08176051414342,15.2,-11.0057728019692));
#297375=CARTESIAN_POINT('Ctrl Pts',(-1.08064486435935,15.2,-11.0098595996932));
#297376=CARTESIAN_POINT('Ctrl Pts',(-1.07952921472728,15.2,-11.0139463968603));
#297377=CARTESIAN_POINT('Ctrl Pts',(-1.07840335555766,15.2,-11.0180446622591));
#297378=CARTESIAN_POINT('Ctrl Pts',(-1.07726723915121,15.2,-11.0221542854225));
#297379=CARTESIAN_POINT('Ctrl Pts',(-1.07613112258996,15.2,-11.0262639091457));
#297380=CARTESIAN_POINT('Ctrl Pts',(-1.07498474934558,15.2,-11.0303848909948));
#297381=CARTESIAN_POINT('Ctrl Pts',(-1.0738280720572,15.2,-11.0345171196496));
#297382=CARTESIAN_POINT('Ctrl Pts',(-1.07238222552552,15.2,-11.0396824051867));
#297383=CARTESIAN_POINT('Ctrl Pts',(-1.07092027880252,15.2,-11.0448652644399));
#297384=CARTESIAN_POINT('Ctrl Pts',(-1.06944214477342,15.2,-11.0500654854135));
#297385=CARTESIAN_POINT('Ctrl Pts',(-1.06796401074431,15.2,-11.0552657063871));
#297386=CARTESIAN_POINT('Ctrl Pts',(-1.06646968679268,15.2,-11.0604832869279));
#297387=CARTESIAN_POINT('Ctrl Pts',(-1.06495908706919,15.2,-11.0657180179013));
#297388=CARTESIAN_POINT('Ctrl Pts',(-1.06375060738919,15.2,-11.0699058023376));
#297389=CARTESIAN_POINT('Ctrl Pts',(-1.06253171105598,15.2,-11.0741045619194));
#297390=CARTESIAN_POINT('Ctrl Pts',(-1.06130235348427,15.2,-11.0783141892054));
#297391=CARTESIAN_POINT('Ctrl Pts',(-1.06007299574505,15.2,-11.0825238170651));
#297392=CARTESIAN_POINT('Ctrl Pts',(-1.05883317762321,15.2,-11.0867443131629));
#297393=CARTESIAN_POINT('Ctrl Pts',(-1.057582855054,15.2,-11.0909755714501));
#297394=CARTESIAN_POINT('Ctrl Pts',(-1.05633253265514,15.2,-11.0952068291609));
#297395=CARTESIAN_POINT('Ctrl Pts',(-1.05507170624375,15.2,-11.0994488459952));
#297396=CARTESIAN_POINT('Ctrl Pts',(-1.0538003325706,15.2,-11.1037015198691));
#297397=CARTESIAN_POINT('Ctrl Pts',(-1.05252895872422,15.2,-11.1079541943224));
#297398=CARTESIAN_POINT('Ctrl Pts',(-1.05124703809842,15.2,-11.1122175233006));
#297399=CARTESIAN_POINT('Ctrl Pts',(-1.04995452829582,15.2,-11.1164914026369));
#297400=CARTESIAN_POINT('Ctrl Pts',(-1.04898514603192,15.2,-11.1196968118479));
#297401=CARTESIAN_POINT('Ctrl Pts',(-1.04800980859123,15.2,-11.1229081555005));
#297402=CARTESIAN_POINT('Ctrl Pts',(-1.04702849637637,15.2,-11.1261253890924));
#297403=CARTESIAN_POINT('Ctrl Pts',(-1.0460471841615,15.2,-11.1293426226844));
#297404=CARTESIAN_POINT('Ctrl Pts',(-1.04505989848068,15.2,-11.1325657464673));
#297405=CARTESIAN_POINT('Ctrl Pts',(-1.0440666217251,15.2,-11.135794716475));
#297406=CARTESIAN_POINT('Ctrl Pts',(-1.04307334496953,15.2,-11.1390236864826));
#297407=CARTESIAN_POINT('Ctrl Pts',(-1.04207407795586,15.2,-11.1422585019317));
#297408=CARTESIAN_POINT('Ctrl Pts',(-1.0410688026179,15.2,-11.1454991204385));
#297409=CARTESIAN_POINT('Ctrl Pts',(-1.04006352727995,15.2,-11.1487397389453));
#297410=CARTESIAN_POINT('Ctrl Pts',(-1.03905224281003,15.2,-11.1519861597272));
#297411=CARTESIAN_POINT('Ctrl Pts',(-1.03803493396353,15.2,-11.1552383398958));
#297412=CARTESIAN_POINT('Ctrl Pts',(-1.03701762511703,15.2,-11.1584905200645));
#297413=CARTESIAN_POINT('Ctrl Pts',(-1.03599429145294,15.2,-11.1617484580745));
#297414=CARTESIAN_POINT('Ctrl Pts',(-1.03496491624116,15.2,-11.1650121125802));
#297415=CARTESIAN_POINT('Ctrl Pts',(-1.03393554084238,15.2,-11.1682757676787));
#297416=CARTESIAN_POINT('Ctrl Pts',(-1.03290012460857,15.2,-11.1715451375205));
#297417=CARTESIAN_POINT('Ctrl Pts',(-1.03185864924805,15.2,-11.1748201802056));
#297418=CARTESIAN_POINT('Ctrl Pts',(-1.03081717407673,15.2,-11.1780952222957));
#297419=CARTESIAN_POINT('Ctrl Pts',(-1.02976964141406,15.2,-11.1813759363939));
#297420=CARTESIAN_POINT('Ctrl Pts',(-1.02871603461848,15.2,-11.1846622800666));
#297421=CARTESIAN_POINT('Ctrl Pts',(-1.0276624278229,15.2,-11.1879486237394));
#297422=CARTESIAN_POINT('Ctrl Pts',(-1.02660274653194,15.2,-11.1912405979911));
#297423=CARTESIAN_POINT('Ctrl Pts',(-1.02553697477413,15.2,-11.194538157678));
#297424=CARTESIAN_POINT('Ctrl Pts',(-1.02447120301632,15.2,-11.1978357173648));
#297425=CARTESIAN_POINT('Ctrl Pts',(-1.02339934128344,15.2,-11.2011388652189));
#297426=CARTESIAN_POINT('Ctrl Pts',(-1.02232137302608,15.2,-11.2044475567803));
#297427=CARTESIAN_POINT('Ctrl Pts',(-1.02124340476871,15.2,-11.2077562483417));
#297428=CARTESIAN_POINT('Ctrl Pts',(-1.02015932972868,15.2,-11.2110704833093));
#297429=CARTESIAN_POINT('Ctrl Pts',(-1.01906913385216,15.2,-11.2143902208549));
#297430=CARTESIAN_POINT('Ctrl Pts',(-1.01797893797563,15.2,-11.2177099584005));
#297431=CARTESIAN_POINT('Ctrl Pts',(-1.01688261859954,15.2,-11.2210351971956));
#297432=CARTESIAN_POINT('Ctrl Pts',(-1.01578016326543,15.2,-11.2243658962822));
#297433=CARTESIAN_POINT('Ctrl Pts',(-1.01467770773104,15.2,-11.2276965959739));
#297434=CARTESIAN_POINT('Ctrl Pts',(-1.01356911463659,15.2,-11.2310327557087));
#297435=CARTESIAN_POINT('Ctrl Pts',(-1.01245436826541,15.2,-11.2343743329451));
#297436=CARTESIAN_POINT('Ctrl Pts',(-1.01133962209675,15.2,-11.2377159095744));
#297437=CARTESIAN_POINT('Ctrl Pts',(-1.01021872428139,15.2,-11.2410629044357));
#297438=CARTESIAN_POINT('Ctrl Pts',(-1.00909165755698,15.2,-11.2444152756486));
#297439=CARTESIAN_POINT('Ctrl Pts',(-1.00796459083257,15.2,-11.2477676468616));
#297440=CARTESIAN_POINT('Ctrl Pts',(-1.00683135638494,15.2,-11.251125393055));
#297441=CARTESIAN_POINT('Ctrl Pts',(-1.00569193959246,15.2,-11.2544884746));
#297442=CARTESIAN_POINT('Ctrl Pts',(-1.00455252279999,15.2,-11.2578515561449));
#297443=CARTESIAN_POINT('Ctrl Pts',(-1.00340692262492,15.2,-11.2612199716726));
#297444=CARTESIAN_POINT('Ctrl Pts',(-1.00225512579177,15.2,-11.2645936812583));
#297445=CARTESIAN_POINT('Ctrl Pts',(-1.0007193965414,15.2,-11.2690919611146));
#297446=CARTESIAN_POINT('Ctrl Pts',(-0.9991726478092,15.2,-11.2735996508886));
#297447=CARTESIAN_POINT('Ctrl Pts',(-0.997614847945394,15.2,-11.2781166527468));
#297448=CARTESIAN_POINT('Ctrl Pts',(-0.996446498153664,15.2,-11.2815044038328));
#297449=CARTESIAN_POINT('Ctrl Pts',(-0.995271930628931,15.2,-11.2848973936268));
#297450=CARTESIAN_POINT('Ctrl Pts',(-0.994091132379621,15.2,-11.2882955811705));
#297451=CARTESIAN_POINT('Ctrl Pts',(-0.992910334130311,15.2,-11.2916937687141));
#297452=CARTESIAN_POINT('Ctrl Pts',(-0.991723304977775,15.2,-11.2950971526781));
#297453=CARTESIAN_POINT('Ctrl Pts',(-0.990530030224015,15.2,-11.2985056942781));
#297454=CARTESIAN_POINT('Ctrl Pts',(-0.989336755470255,15.2,-11.3019142358781));
#297455=CARTESIAN_POINT('Ctrl Pts',(-0.988137235029497,15.2,-11.3053279337889));
#297456=CARTESIAN_POINT('Ctrl Pts',(-0.986931455317859,15.2,-11.3087467479719));
#297457=CARTESIAN_POINT('Ctrl Pts',(-0.984921822392114,15.2,-11.3144447718172));
#297458=CARTESIAN_POINT('Ctrl Pts',(-0.982894802494541,15.2,-11.3201570080722));
#297459=CARTESIAN_POINT('Ctrl Pts',(-0.980850330550103,15.2,-11.325883267725));
#297460=CARTESIAN_POINT('Ctrl Pts',(-0.979623647428009,15.2,-11.3293190233918));
#297461=CARTESIAN_POINT('Ctrl Pts',(-0.97839068277283,15.2,-11.3327598287168));
#297462=CARTESIAN_POINT('Ctrl Pts',(-0.97715142165174,15.2,-11.3362056423828));
#297463=CARTESIAN_POINT('Ctrl Pts',(-0.97591216053065,15.2,-11.3396514560488));
#297464=CARTESIAN_POINT('Ctrl Pts',(-0.974666603441903,15.2,-11.3431022787682));
#297465=CARTESIAN_POINT('Ctrl Pts',(-0.973414737175575,15.2,-11.3465580705648));
#297466=CARTESIAN_POINT('Ctrl Pts',(-0.972162870909247,15.2,-11.3500138623613));
#297467=CARTESIAN_POINT('Ctrl Pts',(-0.970904695512286,15.2,-11.3534746229377));
#297468=CARTESIAN_POINT('Ctrl Pts',(-0.969640197309088,15.2,-11.3569403125195));
#297469=CARTESIAN_POINT('Ctrl Pts',(-0.968375698876172,15.2,-11.3604060027308));
#297470=CARTESIAN_POINT('Ctrl Pts',(-0.967104878474818,15.2,-11.3638766210019));
#297471=CARTESIAN_POINT('Ctrl Pts',(-0.965827722496673,15.2,-11.3673521297576));
#297472=CARTESIAN_POINT('Ctrl Pts',(-0.964550566750545,15.2,-11.370827637882));
#297473=CARTESIAN_POINT('Ctrl Pts',(-0.963267074113089,15.2,-11.3743080363062));
#297474=CARTESIAN_POINT('Ctrl Pts',(-0.961977234867734,15.2,-11.37779328543));
#297475=CARTESIAN_POINT('Ctrl Pts',(-0.96068739562238,15.2,-11.3812785345537));
#297476=CARTESIAN_POINT('Ctrl Pts',(-0.959391207590864,15.2,-11.3847686341476));
#297477=CARTESIAN_POINT('Ctrl Pts',(-0.958088658423916,15.2,-11.3882635447448));
#297478=CARTESIAN_POINT('Ctrl Pts',(-0.956786109256967,15.2,-11.3917584553421));
#297479=CARTESIAN_POINT('Ctrl Pts',(-0.955477199409448,15.2,-11.3952581757582));
#297480=CARTESIAN_POINT('Ctrl Pts',(-0.95416191474296,15.2,-11.3987626660218));
#297481=CARTESIAN_POINT('Ctrl Pts',(-0.952846630076473,15.2,-11.4022671562854));
#297482=CARTESIAN_POINT('Ctrl Pts',(-0.951524971795942,15.2,-11.4057764180618));
#297483=CARTESIAN_POINT('Ctrl Pts',(-0.950196927678083,15.2,-11.4092904138504));
#297484=CARTESIAN_POINT('Ctrl Pts',(-0.948868883560225,15.2,-11.4128044096389));
#297485=CARTESIAN_POINT('Ctrl Pts',(-0.947534454142807,15.2,-11.4163231416439));
#297486=CARTESIAN_POINT('Ctrl Pts',(-0.946193627484058,15.2,-11.4198465707652));
#297487=CARTESIAN_POINT('Ctrl Pts',(-0.944852800581726,15.2,-11.4233700005267));
#297488=CARTESIAN_POINT('Ctrl Pts',(-0.943505576719271,15.2,-11.4268981283394));
#297489=CARTESIAN_POINT('Ctrl Pts',(-0.942151941188334,15.2,-11.4304309065618));
#297490=CARTESIAN_POINT('Ctrl Pts',(-0.940798305903308,15.2,-11.4339636841424));
#297491=CARTESIAN_POINT('Ctrl Pts',(-0.939438257755021,15.2,-11.4375011121365));
#297492=CARTESIAN_POINT('Ctrl Pts',(-0.93807178498566,15.2,-11.441043147727));
#297493=CARTESIAN_POINT('Ctrl Pts',(-0.936705312216299,15.2,-11.4445851833174));
#297494=CARTESIAN_POINT('Ctrl Pts',(-0.935332413680909,15.2,-11.4481318270889));
#297495=CARTESIAN_POINT('Ctrl Pts',(-0.933953085108609,15.2,-11.4516830608689));
#297496=CARTESIAN_POINT('Ctrl Pts',(-0.932573756536309,15.2,-11.4552342946488));
#297497=CARTESIAN_POINT('Ctrl Pts',(-0.931187997895759,15.2,-11.4587901218222));
#297498=CARTESIAN_POINT('Ctrl Pts',(-0.929795809339219,15.2,-11.4623505331326));
#297499=CARTESIAN_POINT('',(-3.28892417320473,15.2,-1.19707050039253));
#297500=CARTESIAN_POINT('Origin',(-5.66257110645729E-14,15.2,-1.77635683940025E-14));
#297501=CARTESIAN_POINT('Origin',(-5.66257110645729E-14,15.2,-1.77635683940025E-14));
#297502=CARTESIAN_POINT('',(-0.143881228002569,12.2,-10.3740022745144));
#297503=CARTESIAN_POINT('',(-0.143881228000057,12.2,-10.374002274));
#297504=CARTESIAN_POINT('Origin',(-5.66257110645729E-14,12.2,-1.77635683940025E-14));
#297505=CARTESIAN_POINT('Origin',(-5.66257110645729E-14,15.2,-1.77635683940025E-14));
#297506=CARTESIAN_POINT('',(-1.18690176602512,12.2,-10.306885523551));
#297507=CARTESIAN_POINT('',(-1.18690176600006,15.2,-10.306885523));
#297508=CARTESIAN_POINT('Origin',(-5.66257110645729E-14,12.2,-1.77635683940025E-14));
#297509=CARTESIAN_POINT('Origin',(-5.66257110645729E-14,15.2,-1.77635683940025E-14));
#297510=CARTESIAN_POINT('',(-0.546958306000055,12.2,-11.486985532));
#297511=CARTESIAN_POINT('',(-0.546958306000055,15.2,-11.486985532));
#297512=CARTESIAN_POINT('',(-0.929795809000057,12.2,-11.462350533));
#297513=CARTESIAN_POINT('Origin',(-5.66257110645729E-14,12.2,-1.77635683940025E-14));
#297514=CARTESIAN_POINT('',(-0.929795809000057,15.2,-11.462350533));
#297515=CARTESIAN_POINT('Ctrl Pts',(-0.546958306000055,15.2,-11.486985532));
#297516=CARTESIAN_POINT('Ctrl Pts',(-0.546958306000055,11.6,-11.486985532));
#297517=CARTESIAN_POINT('Ctrl Pts',(-0.546590899000057,15.2,-11.486315008));
#297518=CARTESIAN_POINT('Ctrl Pts',(-0.546590899000057,11.6,-11.486315008));
#297519=CARTESIAN_POINT('Ctrl Pts',(-0.545856551000057,15.2,-11.484974209));
#297520=CARTESIAN_POINT('Ctrl Pts',(-0.545856551000057,11.6,-11.484974209));
#297521=CARTESIAN_POINT('Ctrl Pts',(-0.544756421000056,15.2,-11.482963757));
#297522=CARTESIAN_POINT('Ctrl Pts',(-0.544756421000056,11.6,-11.482963757));
#297523=CARTESIAN_POINT('Ctrl Pts',(-0.543292369000056,15.2,-11.480284643));
#297524=CARTESIAN_POINT('Ctrl Pts',(-0.543292369000056,11.6,-11.480284643));
#297525=CARTESIAN_POINT('Ctrl Pts',(-0.541466946000057,15.2,-11.476938237));
#297526=CARTESIAN_POINT('Ctrl Pts',(-0.541466946000057,11.6,-11.476938237));
#297527=CARTESIAN_POINT('Ctrl Pts',(-0.539646167000055,15.2,-11.473594318));
#297528=CARTESIAN_POINT('Ctrl Pts',(-0.539646167000055,11.6,-11.473594318));
#297529=CARTESIAN_POINT('Ctrl Pts',(-0.537830030000055,15.2,-11.470252887));
#297530=CARTESIAN_POINT('Ctrl Pts',(-0.537830030000055,11.6,-11.470252887));
#297531=CARTESIAN_POINT('Ctrl Pts',(-0.536018537000055,15.2,-11.466913949));
#297532=CARTESIAN_POINT('Ctrl Pts',(-0.536018537000055,11.6,-11.466913949));
#297533=CARTESIAN_POINT('Ctrl Pts',(-0.534211686000056,15.2,-11.46357751));
#297534=CARTESIAN_POINT('Ctrl Pts',(-0.534211686000056,11.6,-11.46357751));
#297535=CARTESIAN_POINT('Ctrl Pts',(-0.532409474000056,15.2,-11.460243578));
#297536=CARTESIAN_POINT('Ctrl Pts',(-0.532409474000056,11.6,-11.460243578));
#297537=CARTESIAN_POINT('Ctrl Pts',(-0.530611902000055,15.2,-11.456912162));
#297538=CARTESIAN_POINT('Ctrl Pts',(-0.530611902000055,11.6,-11.456912162));
#297539=CARTESIAN_POINT('Ctrl Pts',(-0.528818965000056,15.2,-11.453583273));
#297540=CARTESIAN_POINT('Ctrl Pts',(-0.528818965000056,11.6,-11.453583273));
#297541=CARTESIAN_POINT('Ctrl Pts',(-0.527030665000057,15.2,-11.450256921));
#297542=CARTESIAN_POINT('Ctrl Pts',(-0.527030665000057,11.6,-11.450256921));
#297543=CARTESIAN_POINT('Ctrl Pts',(-0.525246997000056,15.2,-11.446933118));
#297544=CARTESIAN_POINT('Ctrl Pts',(-0.525246997000056,11.6,-11.446933118));
#297545=CARTESIAN_POINT('Ctrl Pts',(-0.523467959000056,15.2,-11.443611875));
#297546=CARTESIAN_POINT('Ctrl Pts',(-0.523467959000056,11.6,-11.443611875));
#297547=CARTESIAN_POINT('Ctrl Pts',(-0.521693552000055,15.2,-11.4402932));
#297548=CARTESIAN_POINT('Ctrl Pts',(-0.521693552000055,11.6,-11.4402932));
#297549=CARTESIAN_POINT('Ctrl Pts',(-0.519923771000055,15.2,-11.436977103));
#297550=CARTESIAN_POINT('Ctrl Pts',(-0.519923771000055,11.6,-11.436977103));
#297551=CARTESIAN_POINT('Ctrl Pts',(-0.518158619000056,15.2,-11.433663589));
#297552=CARTESIAN_POINT('Ctrl Pts',(-0.518158619000056,11.6,-11.433663589));
#297553=CARTESIAN_POINT('Ctrl Pts',(-0.516398090000055,15.2,-11.43035267));
#297554=CARTESIAN_POINT('Ctrl Pts',(-0.516398090000055,11.6,-11.43035267));
#297555=CARTESIAN_POINT('Ctrl Pts',(-0.514642185000056,15.2,-11.427044351));
#297556=CARTESIAN_POINT('Ctrl Pts',(-0.514642185000056,11.6,-11.427044351));
#297557=CARTESIAN_POINT('Ctrl Pts',(-0.512890901000055,15.2,-11.423738642));
#297558=CARTESIAN_POINT('Ctrl Pts',(-0.512890901000055,11.6,-11.423738642));
#297559=CARTESIAN_POINT('Ctrl Pts',(-0.511144239000056,15.2,-11.420435551));
#297560=CARTESIAN_POINT('Ctrl Pts',(-0.511144239000056,11.6,-11.420435551));
#297561=CARTESIAN_POINT('Ctrl Pts',(-0.509402194000056,15.2,-11.417135088));
#297562=CARTESIAN_POINT('Ctrl Pts',(-0.509402194000056,11.6,-11.417135088));
#297563=CARTESIAN_POINT('Ctrl Pts',(-0.507664766000057,15.2,-11.413837262));
#297564=CARTESIAN_POINT('Ctrl Pts',(-0.507664766000057,11.6,-11.413837262));
#297565=CARTESIAN_POINT('Ctrl Pts',(-0.505931954000056,15.2,-11.410542081));
#297566=CARTESIAN_POINT('Ctrl Pts',(-0.505931954000056,11.6,-11.410542081));
#297567=CARTESIAN_POINT('Ctrl Pts',(-0.504203756000056,15.2,-11.407249556));
#297568=CARTESIAN_POINT('Ctrl Pts',(-0.504203756000056,11.6,-11.407249556));
#297569=CARTESIAN_POINT('Ctrl Pts',(-0.502480169000057,15.2,-11.403959697));
#297570=CARTESIAN_POINT('Ctrl Pts',(-0.502480169000057,11.6,-11.403959697));
#297571=CARTESIAN_POINT('Ctrl Pts',(-0.500761192000055,15.2,-11.400672511));
#297572=CARTESIAN_POINT('Ctrl Pts',(-0.500761192000055,11.6,-11.400672511));
#297573=CARTESIAN_POINT('Ctrl Pts',(-0.499046823000056,15.2,-11.397388008));
#297574=CARTESIAN_POINT('Ctrl Pts',(-0.499046823000056,11.6,-11.397388008));
#297575=CARTESIAN_POINT('Ctrl Pts',(-0.497337060000056,15.2,-11.394106196));
#297576=CARTESIAN_POINT('Ctrl Pts',(-0.497337060000056,11.6,-11.394106196));
#297577=CARTESIAN_POINT('Ctrl Pts',(-0.495631904000057,15.2,-11.390827086));
#297578=CARTESIAN_POINT('Ctrl Pts',(-0.495631904000057,11.6,-11.390827086));
#297579=CARTESIAN_POINT('Ctrl Pts',(-0.493931349000055,15.2,-11.387550685));
#297580=CARTESIAN_POINT('Ctrl Pts',(-0.493931349000055,11.6,-11.387550685));
#297581=CARTESIAN_POINT('Ctrl Pts',(-0.492235397000057,15.2,-11.384277003));
#297582=CARTESIAN_POINT('Ctrl Pts',(-0.492235397000057,11.6,-11.384277003));
#297583=CARTESIAN_POINT('Ctrl Pts',(-0.490544043000056,15.2,-11.381006047));
#297584=CARTESIAN_POINT('Ctrl Pts',(-0.490544043000056,11.6,-11.381006047));
#297585=CARTESIAN_POINT('Ctrl Pts',(-0.488857288000055,15.2,-11.377737829));
#297586=CARTESIAN_POINT('Ctrl Pts',(-0.488857288000055,11.6,-11.377737829));
#297587=CARTESIAN_POINT('Ctrl Pts',(-0.487175129000056,15.2,-11.374472358));
#297588=CARTESIAN_POINT('Ctrl Pts',(-0.487175129000056,11.6,-11.374472358));
#297589=CARTESIAN_POINT('Ctrl Pts',(-0.485497564000056,15.2,-11.371209642));
#297590=CARTESIAN_POINT('Ctrl Pts',(-0.485497564000056,11.6,-11.371209642));
#297591=CARTESIAN_POINT('Ctrl Pts',(-0.483824592000056,15.2,-11.367949691));
#297592=CARTESIAN_POINT('Ctrl Pts',(-0.483824592000056,11.6,-11.367949691));
#297593=CARTESIAN_POINT('Ctrl Pts',(-0.482156209000056,15.2,-11.364692512));
#297594=CARTESIAN_POINT('Ctrl Pts',(-0.482156209000056,11.6,-11.364692512));
#297595=CARTESIAN_POINT('Ctrl Pts',(-0.480492416000056,15.2,-11.361438118));
#297596=CARTESIAN_POINT('Ctrl Pts',(-0.480492416000056,11.6,-11.361438118));
#297597=CARTESIAN_POINT('Ctrl Pts',(-0.478833210000056,15.2,-11.358186515));
#297598=CARTESIAN_POINT('Ctrl Pts',(-0.478833210000056,11.6,-11.358186515));
#297599=CARTESIAN_POINT('Ctrl Pts',(-0.477178589000056,15.2,-11.354937714));
#297600=CARTESIAN_POINT('Ctrl Pts',(-0.477178589000056,11.6,-11.354937714));
#297601=CARTESIAN_POINT('Ctrl Pts',(-0.475528552000055,15.2,-11.351691723));
#297602=CARTESIAN_POINT('Ctrl Pts',(-0.475528552000055,11.6,-11.351691723));
#297603=CARTESIAN_POINT('Ctrl Pts',(-0.473883095000056,15.2,-11.348448553));
#297604=CARTESIAN_POINT('Ctrl Pts',(-0.473883095000056,11.6,-11.348448553));
#297605=CARTESIAN_POINT('Ctrl Pts',(-0.472242218000056,15.2,-11.345208212));
#297606=CARTESIAN_POINT('Ctrl Pts',(-0.472242218000056,11.6,-11.345208212));
#297607=CARTESIAN_POINT('Ctrl Pts',(-0.470605918000055,15.2,-11.341970709));
#297608=CARTESIAN_POINT('Ctrl Pts',(-0.470605918000055,11.6,-11.341970709));
#297609=CARTESIAN_POINT('Ctrl Pts',(-0.468974194000056,15.2,-11.338736054));
#297610=CARTESIAN_POINT('Ctrl Pts',(-0.468974194000056,11.6,-11.338736054));
#297611=CARTESIAN_POINT('Ctrl Pts',(-0.467347044000055,15.2,-11.335504256));
#297612=CARTESIAN_POINT('Ctrl Pts',(-0.467347044000055,11.6,-11.335504256));
#297613=CARTESIAN_POINT('Ctrl Pts',(-0.465724466000056,15.2,-11.332275325));
#297614=CARTESIAN_POINT('Ctrl Pts',(-0.465724466000056,11.6,-11.332275325));
#297615=CARTESIAN_POINT('Ctrl Pts',(-0.464106457000056,15.2,-11.329049269));
#297616=CARTESIAN_POINT('Ctrl Pts',(-0.464106457000056,11.6,-11.329049269));
#297617=CARTESIAN_POINT('Ctrl Pts',(-0.462493018000056,15.2,-11.325826098));
#297618=CARTESIAN_POINT('Ctrl Pts',(-0.462493018000056,11.6,-11.325826098));
#297619=CARTESIAN_POINT('Ctrl Pts',(-0.460884143000057,15.2,-11.322605822));
#297620=CARTESIAN_POINT('Ctrl Pts',(-0.460884143000057,11.6,-11.322605822));
#297621=CARTESIAN_POINT('Ctrl Pts',(-0.459279833000057,15.2,-11.319388451));
#297622=CARTESIAN_POINT('Ctrl Pts',(-0.459279833000057,11.6,-11.319388451));
#297623=CARTESIAN_POINT('Ctrl Pts',(-0.457680085000056,15.2,-11.316173992));
#297624=CARTESIAN_POINT('Ctrl Pts',(-0.457680085000056,11.6,-11.316173992));
#297625=CARTESIAN_POINT('Ctrl Pts',(-0.456084896000055,15.2,-11.312962457));
#297626=CARTESIAN_POINT('Ctrl Pts',(-0.456084896000055,11.6,-11.312962457));
#297627=CARTESIAN_POINT('Ctrl Pts',(-0.454494265000056,15.2,-11.309753853));
#297628=CARTESIAN_POINT('Ctrl Pts',(-0.454494265000056,11.6,-11.309753853));
#297629=CARTESIAN_POINT('Ctrl Pts',(-0.452908191000055,15.2,-11.306548191));
#297630=CARTESIAN_POINT('Ctrl Pts',(-0.452908191000055,11.6,-11.306548191));
#297631=CARTESIAN_POINT('Ctrl Pts',(-0.451326671000055,15.2,-11.303345481));
#297632=CARTESIAN_POINT('Ctrl Pts',(-0.451326671000055,11.6,-11.303345481));
#297633=CARTESIAN_POINT('Ctrl Pts',(-0.449749702000056,15.2,-11.300145731));
#297634=CARTESIAN_POINT('Ctrl Pts',(-0.449749702000056,11.6,-11.300145731));
#297635=CARTESIAN_POINT('Ctrl Pts',(-0.448177284000056,15.2,-11.296948952));
#297636=CARTESIAN_POINT('Ctrl Pts',(-0.448177284000056,11.6,-11.296948952));
#297637=CARTESIAN_POINT('Ctrl Pts',(-0.446609414000055,15.2,-11.293755152));
#297638=CARTESIAN_POINT('Ctrl Pts',(-0.446609414000055,11.6,-11.293755152));
#297639=CARTESIAN_POINT('Ctrl Pts',(-0.445046088000056,15.2,-11.290564341));
#297640=CARTESIAN_POINT('Ctrl Pts',(-0.445046088000056,11.6,-11.290564341));
#297641=CARTESIAN_POINT('Ctrl Pts',(-0.443487307000057,15.2,-11.287376529));
#297642=CARTESIAN_POINT('Ctrl Pts',(-0.443487307000057,11.6,-11.287376529));
#297643=CARTESIAN_POINT('Ctrl Pts',(-0.441933068000055,15.2,-11.284191725));
#297644=CARTESIAN_POINT('Ctrl Pts',(-0.441933068000055,11.6,-11.284191725));
#297645=CARTESIAN_POINT('Ctrl Pts',(-0.440383367000056,15.2,-11.281009939));
#297646=CARTESIAN_POINT('Ctrl Pts',(-0.440383367000056,11.6,-11.281009939));
#297647=CARTESIAN_POINT('Ctrl Pts',(-0.438838204000056,15.2,-11.277831182));
#297648=CARTESIAN_POINT('Ctrl Pts',(-0.438838204000056,11.6,-11.277831182));
#297649=CARTESIAN_POINT('Ctrl Pts',(-0.437297576000055,15.2,-11.274655461));
#297650=CARTESIAN_POINT('Ctrl Pts',(-0.437297576000055,11.6,-11.274655461));
#297651=CARTESIAN_POINT('Ctrl Pts',(-0.435761482000055,15.2,-11.271482787));
#297652=CARTESIAN_POINT('Ctrl Pts',(-0.435761482000055,11.6,-11.271482787));
#297653=CARTESIAN_POINT('Ctrl Pts',(-0.434229918000056,15.2,-11.268313169));
#297654=CARTESIAN_POINT('Ctrl Pts',(-0.434229918000056,11.6,-11.268313169));
#297655=CARTESIAN_POINT('Ctrl Pts',(-0.432702884000056,15.2,-11.265146617));
#297656=CARTESIAN_POINT('Ctrl Pts',(-0.432702884000056,11.6,-11.265146617));
#297657=CARTESIAN_POINT('Ctrl Pts',(-0.431180374000055,15.2,-11.261983141));
#297658=CARTESIAN_POINT('Ctrl Pts',(-0.431180374000055,11.6,-11.261983141));
#297659=CARTESIAN_POINT('Ctrl Pts',(-0.429662391000055,15.2,-11.258822751));
#297660=CARTESIAN_POINT('Ctrl Pts',(-0.429662391000055,11.6,-11.258822751));
#297661=CARTESIAN_POINT('Ctrl Pts',(-0.428148929000055,15.2,-11.255665455));
#297662=CARTESIAN_POINT('Ctrl Pts',(-0.428148929000055,11.6,-11.255665455));
#297663=CARTESIAN_POINT('Ctrl Pts',(-0.426639987000056,15.2,-11.252511265));
#297664=CARTESIAN_POINT('Ctrl Pts',(-0.426639987000056,11.6,-11.252511265));
#297665=CARTESIAN_POINT('Ctrl Pts',(-0.425135562000056,15.2,-11.249360189));
#297666=CARTESIAN_POINT('Ctrl Pts',(-0.425135562000056,11.6,-11.249360189));
#297667=CARTESIAN_POINT('Ctrl Pts',(-0.423635654000056,15.2,-11.246212238));
#297668=CARTESIAN_POINT('Ctrl Pts',(-0.423635654000056,11.6,-11.246212238));
#297669=CARTESIAN_POINT('Ctrl Pts',(-0.422140258000056,15.2,-11.243067421));
#297670=CARTESIAN_POINT('Ctrl Pts',(-0.422140258000056,11.6,-11.243067421));
#297671=CARTESIAN_POINT('Ctrl Pts',(-0.420649373000056,15.2,-11.239925747));
#297672=CARTESIAN_POINT('Ctrl Pts',(-0.420649373000056,11.6,-11.239925747));
#297673=CARTESIAN_POINT('Ctrl Pts',(-0.419162997000055,15.2,-11.236787227));
#297674=CARTESIAN_POINT('Ctrl Pts',(-0.419162997000055,11.6,-11.236787227));
#297675=CARTESIAN_POINT('Ctrl Pts',(-0.417681127000057,15.2,-11.233651872));
#297676=CARTESIAN_POINT('Ctrl Pts',(-0.417681127000057,11.6,-11.233651872));
#297677=CARTESIAN_POINT('Ctrl Pts',(-0.416203762000055,15.2,-11.230519688));
#297678=CARTESIAN_POINT('Ctrl Pts',(-0.416203762000055,11.6,-11.230519688));
#297679=CARTESIAN_POINT('Ctrl Pts',(-0.414730899000055,15.2,-11.22739069));
#297680=CARTESIAN_POINT('Ctrl Pts',(-0.414730899000055,11.6,-11.22739069));
#297681=CARTESIAN_POINT('Ctrl Pts',(-0.413262534000056,15.2,-11.224264883));
#297682=CARTESIAN_POINT('Ctrl Pts',(-0.413262534000056,11.6,-11.224264883));
#297683=CARTESIAN_POINT('Ctrl Pts',(-0.411798667000056,15.2,-11.221142281));
#297684=CARTESIAN_POINT('Ctrl Pts',(-0.411798667000056,11.6,-11.221142281));
#297685=CARTESIAN_POINT('Ctrl Pts',(-0.410339295000056,15.2,-11.21802289));
#297686=CARTESIAN_POINT('Ctrl Pts',(-0.410339295000056,11.6,-11.21802289));
#297687=CARTESIAN_POINT('Ctrl Pts',(-0.408884415000056,15.2,-11.214906723));
#297688=CARTESIAN_POINT('Ctrl Pts',(-0.408884415000056,11.6,-11.214906723));
#297689=CARTESIAN_POINT('Ctrl Pts',(-0.407434025000055,15.2,-11.211793789));
#297690=CARTESIAN_POINT('Ctrl Pts',(-0.407434025000055,11.6,-11.211793789));
#297691=CARTESIAN_POINT('Ctrl Pts',(-0.405988122000055,15.2,-11.208684097));
#297692=CARTESIAN_POINT('Ctrl Pts',(-0.405988122000055,11.6,-11.208684097));
#297693=CARTESIAN_POINT('Ctrl Pts',(-0.404546705000056,15.2,-11.205577658));
#297694=CARTESIAN_POINT('Ctrl Pts',(-0.404546705000056,11.6,-11.205577658));
#297695=CARTESIAN_POINT('Ctrl Pts',(-0.403109771000055,15.2,-11.202474481));
#297696=CARTESIAN_POINT('Ctrl Pts',(-0.403109771000055,11.6,-11.202474481));
#297697=CARTESIAN_POINT('Ctrl Pts',(-0.401677318000055,15.2,-11.199374578));
#297698=CARTESIAN_POINT('Ctrl Pts',(-0.401677318000055,11.6,-11.199374578));
#297699=CARTESIAN_POINT('Ctrl Pts',(-0.400249343000055,15.2,-11.196277957));
#297700=CARTESIAN_POINT('Ctrl Pts',(-0.400249343000055,11.6,-11.196277957));
#297701=CARTESIAN_POINT('Ctrl Pts',(-0.398825842000056,15.2,-11.193184629));
#297702=CARTESIAN_POINT('Ctrl Pts',(-0.398825842000056,11.6,-11.193184629));
#297703=CARTESIAN_POINT('Ctrl Pts',(-0.397406814000056,15.2,-11.190094604));
#297704=CARTESIAN_POINT('Ctrl Pts',(-0.397406814000056,11.6,-11.190094604));
#297705=CARTESIAN_POINT('Ctrl Pts',(-0.395992258000056,15.2,-11.187007892));
#297706=CARTESIAN_POINT('Ctrl Pts',(-0.395992258000056,11.6,-11.187007892));
#297707=CARTESIAN_POINT('Ctrl Pts',(-0.394582170000056,15.2,-11.183924502));
#297708=CARTESIAN_POINT('Ctrl Pts',(-0.394582170000056,11.6,-11.183924502));
#297709=CARTESIAN_POINT('Ctrl Pts',(-0.393176547000056,15.2,-11.180844447));
#297710=CARTESIAN_POINT('Ctrl Pts',(-0.393176547000056,11.6,-11.180844447));
#297711=CARTESIAN_POINT('Ctrl Pts',(-0.391775388000056,15.2,-11.177767733));
#297712=CARTESIAN_POINT('Ctrl Pts',(-0.391775388000056,11.6,-11.177767733));
#297713=CARTESIAN_POINT('Ctrl Pts',(-0.390378688000055,15.2,-11.174694374));
#297714=CARTESIAN_POINT('Ctrl Pts',(-0.390378688000055,11.6,-11.174694374));
#297715=CARTESIAN_POINT('Ctrl Pts',(-0.388986447000056,15.2,-11.171624379));
#297716=CARTESIAN_POINT('Ctrl Pts',(-0.388986447000056,11.6,-11.171624379));
#297717=CARTESIAN_POINT('Ctrl Pts',(-0.387598661000055,15.2,-11.168557756));
#297718=CARTESIAN_POINT('Ctrl Pts',(-0.387598661000055,11.6,-11.168557756));
#297719=CARTESIAN_POINT('Ctrl Pts',(-0.386215329000056,15.2,-11.165494519));
#297720=CARTESIAN_POINT('Ctrl Pts',(-0.386215329000056,11.6,-11.165494519));
#297721=CARTESIAN_POINT('Ctrl Pts',(-0.384836446000056,15.2,-11.162434675));
#297722=CARTESIAN_POINT('Ctrl Pts',(-0.384836446000056,11.6,-11.162434675));
#297723=CARTESIAN_POINT('Ctrl Pts',(-0.383462012000055,15.2,-11.159378235));
#297724=CARTESIAN_POINT('Ctrl Pts',(-0.383462012000055,11.6,-11.159378235));
#297725=CARTESIAN_POINT('Ctrl Pts',(-0.382092022000055,15.2,-11.156325211));
#297726=CARTESIAN_POINT('Ctrl Pts',(-0.382092022000055,11.6,-11.156325211));
#297727=CARTESIAN_POINT('Ctrl Pts',(-0.380726475000056,15.2,-11.153275611));
#297728=CARTESIAN_POINT('Ctrl Pts',(-0.380726475000056,11.6,-11.153275611));
#297729=CARTESIAN_POINT('Ctrl Pts',(-0.379365367000055,15.2,-11.150229445));
#297730=CARTESIAN_POINT('Ctrl Pts',(-0.379365367000055,11.6,-11.150229445));
#297731=CARTESIAN_POINT('Ctrl Pts',(-0.378008697000055,15.2,-11.147186726));
#297732=CARTESIAN_POINT('Ctrl Pts',(-0.378008697000055,11.6,-11.147186726));
#297733=CARTESIAN_POINT('Ctrl Pts',(-0.376656462000057,15.2,-11.144147464));
#297734=CARTESIAN_POINT('Ctrl Pts',(-0.376656462000057,11.6,-11.144147464));
#297735=CARTESIAN_POINT('Ctrl Pts',(-0.375308659000056,15.2,-11.141111667));
#297736=CARTESIAN_POINT('Ctrl Pts',(-0.375308659000056,11.6,-11.141111667));
#297737=CARTESIAN_POINT('Ctrl Pts',(-0.373965284000055,15.2,-11.138079346));
#297738=CARTESIAN_POINT('Ctrl Pts',(-0.373965284000055,11.6,-11.138079346));
#297739=CARTESIAN_POINT('Ctrl Pts',(-0.372626336000056,15.2,-11.135050513));
#297740=CARTESIAN_POINT('Ctrl Pts',(-0.372626336000056,11.6,-11.135050513));
#297741=CARTESIAN_POINT('Ctrl Pts',(-0.371291813000055,15.2,-11.132025177));
#297742=CARTESIAN_POINT('Ctrl Pts',(-0.371291813000055,11.6,-11.132025177));
#297743=CARTESIAN_POINT('Ctrl Pts',(-0.369961710000055,15.2,-11.129003349));
#297744=CARTESIAN_POINT('Ctrl Pts',(-0.369961710000055,11.6,-11.129003349));
#297745=CARTESIAN_POINT('Ctrl Pts',(-0.368636025000055,15.2,-11.125985039));
#297746=CARTESIAN_POINT('Ctrl Pts',(-0.368636025000055,11.6,-11.125985039));
#297747=CARTESIAN_POINT('Ctrl Pts',(-0.367314756000056,15.2,-11.122970257));
#297748=CARTESIAN_POINT('Ctrl Pts',(-0.367314756000056,11.6,-11.122970257));
#297749=CARTESIAN_POINT('Ctrl Pts',(-0.365997899000057,15.2,-11.119959015));
#297750=CARTESIAN_POINT('Ctrl Pts',(-0.365997899000057,11.6,-11.119959015));
#297751=CARTESIAN_POINT('Ctrl Pts',(-0.364685453000057,15.2,-11.116951323));
#297752=CARTESIAN_POINT('Ctrl Pts',(-0.364685453000057,11.6,-11.116951323));
#297753=CARTESIAN_POINT('Ctrl Pts',(-0.363377414000056,15.2,-11.11394719));
#297754=CARTESIAN_POINT('Ctrl Pts',(-0.363377414000056,11.6,-11.11394719));
#297755=CARTESIAN_POINT('Ctrl Pts',(-0.362073780000056,15.2,-11.110946628));
#297756=CARTESIAN_POINT('Ctrl Pts',(-0.362073780000056,11.6,-11.110946628));
#297757=CARTESIAN_POINT('Ctrl Pts',(-0.360774547000055,15.2,-11.107949648));
#297758=CARTESIAN_POINT('Ctrl Pts',(-0.360774547000055,11.6,-11.107949648));
#297759=CARTESIAN_POINT('Ctrl Pts',(-0.359479712000056,15.2,-11.104956259));
#297760=CARTESIAN_POINT('Ctrl Pts',(-0.359479712000056,11.6,-11.104956259));
#297761=CARTESIAN_POINT('Ctrl Pts',(-0.358189274000056,15.2,-11.101966474));
#297762=CARTESIAN_POINT('Ctrl Pts',(-0.358189274000056,11.6,-11.101966474));
#297763=CARTESIAN_POINT('Ctrl Pts',(-0.356903229000055,15.2,-11.0989803));
#297764=CARTESIAN_POINT('Ctrl Pts',(-0.356903229000055,11.6,-11.0989803));
#297765=CARTESIAN_POINT('Ctrl Pts',(-0.355621573000056,15.2,-11.09599775));
#297766=CARTESIAN_POINT('Ctrl Pts',(-0.355621573000056,11.6,-11.09599775));
#297767=CARTESIAN_POINT('Ctrl Pts',(-0.354344305000056,15.2,-11.093018835));
#297768=CARTESIAN_POINT('Ctrl Pts',(-0.354344305000056,11.6,-11.093018835));
#297769=CARTESIAN_POINT('Ctrl Pts',(-0.353071422000056,15.2,-11.090043565));
#297770=CARTESIAN_POINT('Ctrl Pts',(-0.353071422000056,11.6,-11.090043565));
#297771=CARTESIAN_POINT('Ctrl Pts',(-0.351802919000056,15.2,-11.08707195));
#297772=CARTESIAN_POINT('Ctrl Pts',(-0.351802919000056,11.6,-11.08707195));
#297773=CARTESIAN_POINT('Ctrl Pts',(-0.350538795000055,15.2,-11.084104002));
#297774=CARTESIAN_POINT('Ctrl Pts',(-0.350538795000055,11.6,-11.084104002));
#297775=CARTESIAN_POINT('Ctrl Pts',(-0.349279047000056,15.2,-11.08113973));
#297776=CARTESIAN_POINT('Ctrl Pts',(-0.349279047000056,11.6,-11.08113973));
#297777=CARTESIAN_POINT('Ctrl Pts',(-0.348023671000056,15.2,-11.078179147));
#297778=CARTESIAN_POINT('Ctrl Pts',(-0.348023671000056,11.6,-11.078179147));
#297779=CARTESIAN_POINT('Ctrl Pts',(-0.346772665000056,15.2,-11.075222262));
#297780=CARTESIAN_POINT('Ctrl Pts',(-0.346772665000056,11.6,-11.075222262));
#297781=CARTESIAN_POINT('Ctrl Pts',(-0.345526025000057,15.2,-11.072269087));
#297782=CARTESIAN_POINT('Ctrl Pts',(-0.345526025000057,11.6,-11.072269087));
#297783=CARTESIAN_POINT('Ctrl Pts',(-0.344283750000055,15.2,-11.069319632));
#297784=CARTESIAN_POINT('Ctrl Pts',(-0.344283750000055,11.6,-11.069319632));
#297785=CARTESIAN_POINT('Ctrl Pts',(-0.343045833000056,15.2,-11.066373907));
#297786=CARTESIAN_POINT('Ctrl Pts',(-0.343045833000056,11.6,-11.066373907));
#297787=CARTESIAN_POINT('Ctrl Pts',(-0.341812276000055,15.2,-11.063431925));
#297788=CARTESIAN_POINT('Ctrl Pts',(-0.341812276000055,11.6,-11.063431925));
#297789=CARTESIAN_POINT('Ctrl Pts',(-0.340583073000056,15.2,-11.060493695));
#297790=CARTESIAN_POINT('Ctrl Pts',(-0.340583073000056,11.6,-11.060493695));
#297791=CARTESIAN_POINT('Ctrl Pts',(-0.339358220000056,15.2,-11.057559229));
#297792=CARTESIAN_POINT('Ctrl Pts',(-0.339358220000056,11.6,-11.057559229));
#297793=CARTESIAN_POINT('Ctrl Pts',(-0.338137716000055,15.2,-11.054628537));
#297794=CARTESIAN_POINT('Ctrl Pts',(-0.338137716000055,11.6,-11.054628537));
#297795=CARTESIAN_POINT('Ctrl Pts',(-0.336921557000055,15.2,-11.051701631));
#297796=CARTESIAN_POINT('Ctrl Pts',(-0.336921557000055,11.6,-11.051701631));
#297797=CARTESIAN_POINT('Ctrl Pts',(-0.335709740000055,15.2,-11.048778521));
#297798=CARTESIAN_POINT('Ctrl Pts',(-0.335709740000055,11.6,-11.048778521));
#297799=CARTESIAN_POINT('Ctrl Pts',(-0.334502263000056,15.2,-11.045859219));
#297800=CARTESIAN_POINT('Ctrl Pts',(-0.334502263000056,11.6,-11.045859219));
#297801=CARTESIAN_POINT('Ctrl Pts',(-0.333299121000056,15.2,-11.042943735));
#297802=CARTESIAN_POINT('Ctrl Pts',(-0.333299121000056,11.6,-11.042943735));
#297803=CARTESIAN_POINT('Ctrl Pts',(-0.332100311000056,15.2,-11.040032081));
#297804=CARTESIAN_POINT('Ctrl Pts',(-0.332100311000056,11.6,-11.040032081));
#297805=CARTESIAN_POINT('Ctrl Pts',(-0.330905831000056,15.2,-11.037124266));
#297806=CARTESIAN_POINT('Ctrl Pts',(-0.330905831000056,11.6,-11.037124266));
#297807=CARTESIAN_POINT('Ctrl Pts',(-0.329715678000057,15.2,-11.034220304));
#297808=CARTESIAN_POINT('Ctrl Pts',(-0.329715678000057,11.6,-11.034220304));
#297809=CARTESIAN_POINT('Ctrl Pts',(-0.328529847000055,15.2,-11.031320204));
#297810=CARTESIAN_POINT('Ctrl Pts',(-0.328529847000055,11.6,-11.031320204));
#297811=CARTESIAN_POINT('Ctrl Pts',(-0.327348336000056,15.2,-11.028423977));
#297812=CARTESIAN_POINT('Ctrl Pts',(-0.327348336000056,11.6,-11.028423977));
#297813=CARTESIAN_POINT('Ctrl Pts',(-0.326171142000057,15.2,-11.025531635));
#297814=CARTESIAN_POINT('Ctrl Pts',(-0.326171142000057,11.6,-11.025531635));
#297815=CARTESIAN_POINT('Ctrl Pts',(-0.324998260000056,15.2,-11.022643189));
#297816=CARTESIAN_POINT('Ctrl Pts',(-0.324998260000056,11.6,-11.022643189));
#297817=CARTESIAN_POINT('Ctrl Pts',(-0.323829689000057,15.2,-11.01975865));
#297818=CARTESIAN_POINT('Ctrl Pts',(-0.323829689000057,11.6,-11.01975865));
#297819=CARTESIAN_POINT('Ctrl Pts',(-0.322665426000055,15.2,-11.01687803));
#297820=CARTESIAN_POINT('Ctrl Pts',(-0.322665426000055,11.6,-11.01687803));
#297821=CARTESIAN_POINT('Ctrl Pts',(-0.321505465000056,15.2,-11.014001338));
#297822=CARTESIAN_POINT('Ctrl Pts',(-0.321505465000056,11.6,-11.014001338));
#297823=CARTESIAN_POINT('Ctrl Pts',(-0.320349803000056,15.2,-11.011128588));
#297824=CARTESIAN_POINT('Ctrl Pts',(-0.320349803000056,11.6,-11.011128588));
#297825=CARTESIAN_POINT('Ctrl Pts',(-0.319198440000056,15.2,-11.008259788));
#297826=CARTESIAN_POINT('Ctrl Pts',(-0.319198440000056,11.6,-11.008259788));
#297827=CARTESIAN_POINT('Ctrl Pts',(-0.318051369000055,15.2,-11.005394953));
#297828=CARTESIAN_POINT('Ctrl Pts',(-0.318051369000055,11.6,-11.005394953));
#297829=CARTESIAN_POINT('Ctrl Pts',(-0.316908589000056,15.2,-11.002534092));
#297830=CARTESIAN_POINT('Ctrl Pts',(-0.316908589000056,11.6,-11.002534092));
#297831=CARTESIAN_POINT('Ctrl Pts',(-0.315770096000056,15.2,-10.999677217));
#297832=CARTESIAN_POINT('Ctrl Pts',(-0.315770096000056,11.6,-10.999677217));
#297833=CARTESIAN_POINT('Ctrl Pts',(-0.314635885000056,15.2,-10.996824339));
#297834=CARTESIAN_POINT('Ctrl Pts',(-0.314635885000056,11.6,-10.996824339));
#297835=CARTESIAN_POINT('Ctrl Pts',(-0.313505954000056,15.2,-10.993975469));
#297836=CARTESIAN_POINT('Ctrl Pts',(-0.313505954000056,11.6,-10.993975469));
#297837=CARTESIAN_POINT('Ctrl Pts',(-0.312380301000056,15.2,-10.991130619));
#297838=CARTESIAN_POINT('Ctrl Pts',(-0.312380301000056,11.6,-10.991130619));
#297839=CARTESIAN_POINT('Ctrl Pts',(-0.311258919000055,15.2,-10.988289801));
#297840=CARTESIAN_POINT('Ctrl Pts',(-0.311258919000055,11.6,-10.988289801));
#297841=CARTESIAN_POINT('Ctrl Pts',(-0.310141808000056,15.2,-10.985453024));
#297842=CARTESIAN_POINT('Ctrl Pts',(-0.310141808000056,11.6,-10.985453024));
#297843=CARTESIAN_POINT('Ctrl Pts',(-0.309028962000056,15.2,-10.982620303));
#297844=CARTESIAN_POINT('Ctrl Pts',(-0.309028962000056,11.6,-10.982620303));
#297845=CARTESIAN_POINT('Ctrl Pts',(-0.307920380000055,15.2,-10.979791646));
#297846=CARTESIAN_POINT('Ctrl Pts',(-0.307920380000055,11.6,-10.979791646));
#297847=CARTESIAN_POINT('Ctrl Pts',(-0.306816056000055,15.2,-10.976967067));
#297848=CARTESIAN_POINT('Ctrl Pts',(-0.306816056000055,11.6,-10.976967067));
#297849=CARTESIAN_POINT('Ctrl Pts',(-0.305715987000056,15.2,-10.974146576));
#297850=CARTESIAN_POINT('Ctrl Pts',(-0.305715987000056,11.6,-10.974146576));
#297851=CARTESIAN_POINT('Ctrl Pts',(-0.304620171000056,15.2,-10.971330186));
#297852=CARTESIAN_POINT('Ctrl Pts',(-0.304620171000056,11.6,-10.971330186));
#297853=CARTESIAN_POINT('Ctrl Pts',(-0.303528603000055,15.2,-10.968517907));
#297854=CARTESIAN_POINT('Ctrl Pts',(-0.303528603000055,11.6,-10.968517907));
#297855=CARTESIAN_POINT('Ctrl Pts',(-0.302441280000056,15.2,-10.965709752));
#297856=CARTESIAN_POINT('Ctrl Pts',(-0.302441280000056,11.6,-10.965709752));
#297857=CARTESIAN_POINT('Ctrl Pts',(-0.301358198000056,15.2,-10.962905731));
#297858=CARTESIAN_POINT('Ctrl Pts',(-0.301358198000056,11.6,-10.962905731));
#297859=CARTESIAN_POINT('Ctrl Pts',(-0.300279354000056,15.2,-10.960105857));
#297860=CARTESIAN_POINT('Ctrl Pts',(-0.300279354000056,11.6,-10.960105857));
#297861=CARTESIAN_POINT('Ctrl Pts',(-0.299204743000056,15.2,-10.957310141));
#297862=CARTESIAN_POINT('Ctrl Pts',(-0.299204743000056,11.6,-10.957310141));
#297863=CARTESIAN_POINT('Ctrl Pts',(-0.298134363000055,15.2,-10.954518595));
#297864=CARTESIAN_POINT('Ctrl Pts',(-0.298134363000055,11.6,-10.954518595));
#297865=CARTESIAN_POINT('Ctrl Pts',(-0.297068210000055,15.2,-10.951731231));
#297866=CARTESIAN_POINT('Ctrl Pts',(-0.297068210000055,11.6,-10.951731231));
#297867=CARTESIAN_POINT('Ctrl Pts',(-0.296006280000055,15.2,-10.948948059));
#297868=CARTESIAN_POINT('Ctrl Pts',(-0.296006280000055,11.6,-10.948948059));
#297869=CARTESIAN_POINT('Ctrl Pts',(-0.294948568000055,15.2,-10.946169093));
#297870=CARTESIAN_POINT('Ctrl Pts',(-0.294948568000055,11.6,-10.946169093));
#297871=CARTESIAN_POINT('Ctrl Pts',(-0.293895073000057,15.2,-10.943394344));
#297872=CARTESIAN_POINT('Ctrl Pts',(-0.293895073000057,11.6,-10.943394344));
#297873=CARTESIAN_POINT('Ctrl Pts',(-0.292845789000056,15.2,-10.940623823));
#297874=CARTESIAN_POINT('Ctrl Pts',(-0.292845789000056,11.6,-10.940623823));
#297875=CARTESIAN_POINT('Ctrl Pts',(-0.291800713000056,15.2,-10.937857543));
#297876=CARTESIAN_POINT('Ctrl Pts',(-0.291800713000056,11.6,-10.937857543));
#297877=CARTESIAN_POINT('Ctrl Pts',(-0.290759842000057,15.2,-10.935095515));
#297878=CARTESIAN_POINT('Ctrl Pts',(-0.290759842000057,11.6,-10.935095515));
#297879=CARTESIAN_POINT('Ctrl Pts',(-0.289723171000055,15.2,-10.932337751));
#297880=CARTESIAN_POINT('Ctrl Pts',(-0.289723171000055,11.6,-10.932337751));
#297881=CARTESIAN_POINT('Ctrl Pts',(-0.288690696000057,15.2,-10.929584264));
#297882=CARTESIAN_POINT('Ctrl Pts',(-0.288690696000057,11.6,-10.929584264));
#297883=CARTESIAN_POINT('Ctrl Pts',(-0.287662415000056,15.2,-10.926835064));
#297884=CARTESIAN_POINT('Ctrl Pts',(-0.287662415000056,11.6,-10.926835064));
#297885=CARTESIAN_POINT('Ctrl Pts',(-0.286638323000057,15.2,-10.924090164));
#297886=CARTESIAN_POINT('Ctrl Pts',(-0.286638323000057,11.6,-10.924090164));
#297887=CARTESIAN_POINT('Ctrl Pts',(-0.285618416000055,15.2,-10.921349576));
#297888=CARTESIAN_POINT('Ctrl Pts',(-0.285618416000055,11.6,-10.921349576));
#297889=CARTESIAN_POINT('Ctrl Pts',(-0.284602690000056,15.2,-10.918613312));
#297890=CARTESIAN_POINT('Ctrl Pts',(-0.284602690000056,11.6,-10.918613312));
#297891=CARTESIAN_POINT('Ctrl Pts',(-0.283591141000056,15.2,-10.915881383));
#297892=CARTESIAN_POINT('Ctrl Pts',(-0.283591141000056,11.6,-10.915881383));
#297893=CARTESIAN_POINT('Ctrl Pts',(-0.282583766000055,15.2,-10.913153802));
#297894=CARTESIAN_POINT('Ctrl Pts',(-0.282583766000055,11.6,-10.913153802));
#297895=CARTESIAN_POINT('Ctrl Pts',(-0.281580560000056,15.2,-10.910430583));
#297896=CARTESIAN_POINT('Ctrl Pts',(-0.281580560000056,11.6,-10.910430583));
#297897=CARTESIAN_POINT('Ctrl Pts',(-0.280581520000055,15.2,-10.907711734));
#297898=CARTESIAN_POINT('Ctrl Pts',(-0.280581520000055,11.6,-10.907711734));
#297899=CARTESIAN_POINT('Ctrl Pts',(-0.279586642000057,15.2,-10.904997271));
#297900=CARTESIAN_POINT('Ctrl Pts',(-0.279586642000057,11.6,-10.904997271));
#297901=CARTESIAN_POINT('Ctrl Pts',(-0.278595921000055,15.2,-10.902287203));
#297902=CARTESIAN_POINT('Ctrl Pts',(-0.278595921000055,11.6,-10.902287203));
#297903=CARTESIAN_POINT('Ctrl Pts',(-0.277609355000056,15.2,-10.899581544));
#297904=CARTESIAN_POINT('Ctrl Pts',(-0.277609355000056,11.6,-10.899581544));
#297905=CARTESIAN_POINT('Ctrl Pts',(-0.276626937000056,15.2,-10.896880306));
#297906=CARTESIAN_POINT('Ctrl Pts',(-0.276626937000056,11.6,-10.896880306));
#297907=CARTESIAN_POINT('Ctrl Pts',(-0.275648666000056,15.2,-10.8941835));
#297908=CARTESIAN_POINT('Ctrl Pts',(-0.275648666000056,11.6,-10.8941835));
#297909=CARTESIAN_POINT('Ctrl Pts',(-0.274674534000056,15.2,-10.891491141));
#297910=CARTESIAN_POINT('Ctrl Pts',(-0.274674534000056,11.6,-10.891491141));
#297911=CARTESIAN_POINT('Ctrl Pts',(-0.273704541000056,15.2,-10.888803238));
#297912=CARTESIAN_POINT('Ctrl Pts',(-0.273704541000056,11.6,-10.888803238));
#297913=CARTESIAN_POINT('Ctrl Pts',(-0.272738681000056,15.2,-10.886119805));
#297914=CARTESIAN_POINT('Ctrl Pts',(-0.272738681000056,11.6,-10.886119805));
#297915=CARTESIAN_POINT('Ctrl Pts',(-0.271776951000057,15.2,-10.883440854));
#297916=CARTESIAN_POINT('Ctrl Pts',(-0.271776951000057,11.6,-10.883440854));
#297917=CARTESIAN_POINT('Ctrl Pts',(-0.270819345000056,15.2,-10.880766398));
#297918=CARTESIAN_POINT('Ctrl Pts',(-0.270819345000056,11.6,-10.880766398));
#297919=CARTESIAN_POINT('Ctrl Pts',(-0.269865860000056,15.2,-10.878096449));
#297920=CARTESIAN_POINT('Ctrl Pts',(-0.269865860000056,11.6,-10.878096449));
#297921=CARTESIAN_POINT('Ctrl Pts',(-0.268916493000055,15.2,-10.87543102));
#297922=CARTESIAN_POINT('Ctrl Pts',(-0.268916493000055,11.6,-10.87543102));
#297923=CARTESIAN_POINT('Ctrl Pts',(-0.267971237000056,15.2,-10.872770121));
#297924=CARTESIAN_POINT('Ctrl Pts',(-0.267971237000056,11.6,-10.872770121));
#297925=CARTESIAN_POINT('Ctrl Pts',(-0.267030089000055,15.2,-10.870113767));
#297926=CARTESIAN_POINT('Ctrl Pts',(-0.267030089000055,11.6,-10.870113767));
#297927=CARTESIAN_POINT('Ctrl Pts',(-0.266093047000057,15.2,-10.86746197));
#297928=CARTESIAN_POINT('Ctrl Pts',(-0.266093047000057,11.6,-10.86746197));
#297929=CARTESIAN_POINT('Ctrl Pts',(-0.265160103000056,15.2,-10.864814742));
#297930=CARTESIAN_POINT('Ctrl Pts',(-0.265160103000056,11.6,-10.864814742));
#297931=CARTESIAN_POINT('Ctrl Pts',(-0.264231255000055,15.2,-10.862172095));
#297932=CARTESIAN_POINT('Ctrl Pts',(-0.264231255000055,11.6,-10.862172095));
#297933=CARTESIAN_POINT('Ctrl Pts',(-0.263306498000055,15.2,-10.859534042));
#297934=CARTESIAN_POINT('Ctrl Pts',(-0.263306498000055,11.6,-10.859534042));
#297935=CARTESIAN_POINT('Ctrl Pts',(-0.262385828000056,15.2,-10.856900598));
#297936=CARTESIAN_POINT('Ctrl Pts',(-0.262385828000056,11.6,-10.856900598));
#297937=CARTESIAN_POINT('Ctrl Pts',(-0.261469242000055,15.2,-10.854271772));
#297938=CARTESIAN_POINT('Ctrl Pts',(-0.261469242000055,11.6,-10.854271772));
#297939=CARTESIAN_POINT('Ctrl Pts',(-0.260556733000056,15.2,-10.851647578));
#297940=CARTESIAN_POINT('Ctrl Pts',(-0.260556733000056,11.6,-10.851647578));
#297941=CARTESIAN_POINT('Ctrl Pts',(-0.259648297000057,15.2,-10.84902803));
#297942=CARTESIAN_POINT('Ctrl Pts',(-0.259648297000057,11.6,-10.84902803));
#297943=CARTESIAN_POINT('Ctrl Pts',(-0.258743931000056,15.2,-10.846413139));
#297944=CARTESIAN_POINT('Ctrl Pts',(-0.258743931000056,11.6,-10.846413139));
#297945=CARTESIAN_POINT('Ctrl Pts',(-0.257843631000056,15.2,-10.843802918));
#297946=CARTESIAN_POINT('Ctrl Pts',(-0.257843631000056,11.6,-10.843802918));
#297947=CARTESIAN_POINT('Ctrl Pts',(-0.256947390000055,15.2,-10.84119738));
#297948=CARTESIAN_POINT('Ctrl Pts',(-0.256947390000055,11.6,-10.84119738));
#297949=CARTESIAN_POINT('Ctrl Pts',(-0.256055206000055,15.2,-10.838596538));
#297950=CARTESIAN_POINT('Ctrl Pts',(-0.256055206000055,11.6,-10.838596538));
#297951=CARTESIAN_POINT('Ctrl Pts',(-0.255167073000055,15.2,-10.836000406));
#297952=CARTESIAN_POINT('Ctrl Pts',(-0.255167073000055,11.6,-10.836000406));
#297953=CARTESIAN_POINT('Ctrl Pts',(-0.254282988000056,15.2,-10.833408995));
#297954=CARTESIAN_POINT('Ctrl Pts',(-0.254282988000056,11.6,-10.833408995));
#297955=CARTESIAN_POINT('Ctrl Pts',(-0.253402945000056,15.2,-10.830822318));
#297956=CARTESIAN_POINT('Ctrl Pts',(-0.253402945000056,11.6,-10.830822318));
#297957=CARTESIAN_POINT('Ctrl Pts',(-0.252526940000056,15.2,-10.828240388));
#297958=CARTESIAN_POINT('Ctrl Pts',(-0.252526940000056,11.6,-10.828240388));
#297959=CARTESIAN_POINT('Ctrl Pts',(-0.251654969000056,15.2,-10.825663219));
#297960=CARTESIAN_POINT('Ctrl Pts',(-0.251654969000056,11.6,-10.825663219));
#297961=CARTESIAN_POINT('Ctrl Pts',(-0.250787027000056,15.2,-10.823090823));
#297962=CARTESIAN_POINT('Ctrl Pts',(-0.250787027000056,11.6,-10.823090823));
#297963=CARTESIAN_POINT('Ctrl Pts',(-0.249923109000055,15.2,-10.820523213));
#297964=CARTESIAN_POINT('Ctrl Pts',(-0.249923109000055,11.6,-10.820523213));
#297965=CARTESIAN_POINT('Ctrl Pts',(-0.249063210000056,15.2,-10.817960403));
#297966=CARTESIAN_POINT('Ctrl Pts',(-0.249063210000056,11.6,-10.817960403));
#297967=CARTESIAN_POINT('Ctrl Pts',(-0.248207327000056,15.2,-10.815402404));
#297968=CARTESIAN_POINT('Ctrl Pts',(-0.248207327000056,11.6,-10.815402404));
#297969=CARTESIAN_POINT('Ctrl Pts',(-0.247355454000056,15.2,-10.812849232));
#297970=CARTESIAN_POINT('Ctrl Pts',(-0.247355454000056,11.6,-10.812849232));
#297971=CARTESIAN_POINT('Ctrl Pts',(-0.246507587000057,15.2,-10.810300898));
#297972=CARTESIAN_POINT('Ctrl Pts',(-0.246507587000057,11.6,-10.810300898));
#297973=CARTESIAN_POINT('Ctrl Pts',(-0.245663721000057,15.2,-10.807757416));
#297974=CARTESIAN_POINT('Ctrl Pts',(-0.245663721000057,11.6,-10.807757416));
#297975=CARTESIAN_POINT('Ctrl Pts',(-0.244823851000057,15.2,-10.805218799));
#297976=CARTESIAN_POINT('Ctrl Pts',(-0.244823851000057,11.6,-10.805218799));
#297977=CARTESIAN_POINT('Ctrl Pts',(-0.243987973000056,15.2,-10.80268506));
#297978=CARTESIAN_POINT('Ctrl Pts',(-0.243987973000056,11.6,-10.80268506));
#297979=CARTESIAN_POINT('Ctrl Pts',(-0.243156080000055,15.2,-10.800156212));
#297980=CARTESIAN_POINT('Ctrl Pts',(-0.243156080000055,11.6,-10.800156212));
#297981=CARTESIAN_POINT('Ctrl Pts',(-0.242328171000056,15.2,-10.797632269));
#297982=CARTESIAN_POINT('Ctrl Pts',(-0.242328171000056,11.6,-10.797632269));
#297983=CARTESIAN_POINT('Ctrl Pts',(-0.241504238000055,15.2,-10.795113244));
#297984=CARTESIAN_POINT('Ctrl Pts',(-0.241504238000055,11.6,-10.795113244));
#297985=CARTESIAN_POINT('Ctrl Pts',(-0.240684278000056,15.2,-10.79259915));
#297986=CARTESIAN_POINT('Ctrl Pts',(-0.240684278000056,11.6,-10.79259915));
#297987=CARTESIAN_POINT('Ctrl Pts',(-0.239868284000057,15.2,-10.790090001));
#297988=CARTESIAN_POINT('Ctrl Pts',(-0.239868284000057,11.6,-10.790090001));
#297989=CARTESIAN_POINT('Ctrl Pts',(-0.239056253000056,15.2,-10.78758581));
#297990=CARTESIAN_POINT('Ctrl Pts',(-0.239056253000056,11.6,-10.78758581));
#297991=CARTESIAN_POINT('Ctrl Pts',(-0.238248181000056,15.2,-10.78508659));
#297992=CARTESIAN_POINT('Ctrl Pts',(-0.238248181000056,11.6,-10.78508659));
#297993=CARTESIAN_POINT('Ctrl Pts',(-0.237444060000056,15.2,-10.782592355));
#297994=CARTESIAN_POINT('Ctrl Pts',(-0.237444060000056,11.6,-10.782592355));
#297995=CARTESIAN_POINT('Ctrl Pts',(-0.236643888000057,15.2,-10.780103119));
#297996=CARTESIAN_POINT('Ctrl Pts',(-0.236643888000057,11.6,-10.780103119));
#297997=CARTESIAN_POINT('Ctrl Pts',(-0.235847657000056,15.2,-10.777618895));
#297998=CARTESIAN_POINT('Ctrl Pts',(-0.235847657000056,11.6,-10.777618895));
#297999=CARTESIAN_POINT('Ctrl Pts',(-0.235055365000055,15.2,-10.775139696));
#298000=CARTESIAN_POINT('Ctrl Pts',(-0.235055365000055,11.6,-10.775139696));
#298001=CARTESIAN_POINT('Ctrl Pts',(-0.234267006000056,15.2,-10.772665536));
#298002=CARTESIAN_POINT('Ctrl Pts',(-0.234267006000056,11.6,-10.772665536));
#298003=CARTESIAN_POINT('Ctrl Pts',(-0.233482574000057,15.2,-10.770196429));
#298004=CARTESIAN_POINT('Ctrl Pts',(-0.233482574000057,11.6,-10.770196429));
#298005=CARTESIAN_POINT('Ctrl Pts',(-0.232702064000057,15.2,-10.767732388));
#298006=CARTESIAN_POINT('Ctrl Pts',(-0.232702064000057,11.6,-10.767732388));
#298007=CARTESIAN_POINT('Ctrl Pts',(-0.231925472000055,15.2,-10.765273428));
#298008=CARTESIAN_POINT('Ctrl Pts',(-0.231925472000055,11.6,-10.765273428));
#298009=CARTESIAN_POINT('Ctrl Pts',(-0.231152793000057,15.2,-10.76281956));
#298010=CARTESIAN_POINT('Ctrl Pts',(-0.231152793000057,11.6,-10.76281956));
#298011=CARTESIAN_POINT('Ctrl Pts',(-0.230384020000055,15.2,-10.760370801));
#298012=CARTESIAN_POINT('Ctrl Pts',(-0.230384020000055,11.6,-10.760370801));
#298013=CARTESIAN_POINT('Ctrl Pts',(-0.229619150000057,15.2,-10.757927163));
#298014=CARTESIAN_POINT('Ctrl Pts',(-0.229619150000057,11.6,-10.757927163));
#298015=CARTESIAN_POINT('Ctrl Pts',(-0.228858176000056,15.2,-10.75548866));
#298016=CARTESIAN_POINT('Ctrl Pts',(-0.228858176000056,11.6,-10.75548866));
#298017=CARTESIAN_POINT('Ctrl Pts',(-0.228101094000056,15.2,-10.753055307));
#298018=CARTESIAN_POINT('Ctrl Pts',(-0.228101094000056,11.6,-10.753055307));
#298019=CARTESIAN_POINT('Ctrl Pts',(-0.227347899000057,15.2,-10.750627116));
#298020=CARTESIAN_POINT('Ctrl Pts',(-0.227347899000057,11.6,-10.750627116));
#298021=CARTESIAN_POINT('Ctrl Pts',(-0.226598585000056,15.2,-10.748204102));
#298022=CARTESIAN_POINT('Ctrl Pts',(-0.226598585000056,11.6,-10.748204102));
#298023=CARTESIAN_POINT('Ctrl Pts',(-0.225853145000056,15.2,-10.745786278));
#298024=CARTESIAN_POINT('Ctrl Pts',(-0.225853145000056,11.6,-10.745786278));
#298025=CARTESIAN_POINT('Ctrl Pts',(-0.225111578000057,15.2,-10.743373659));
#298026=CARTESIAN_POINT('Ctrl Pts',(-0.225111578000057,11.6,-10.743373659));
#298027=CARTESIAN_POINT('Ctrl Pts',(-0.224373875000056,15.2,-10.740966259));
#298028=CARTESIAN_POINT('Ctrl Pts',(-0.224373875000056,11.6,-10.740966259));
#298029=CARTESIAN_POINT('Ctrl Pts',(-0.223640033000055,15.2,-10.738564091));
#298030=CARTESIAN_POINT('Ctrl Pts',(-0.223640033000055,11.6,-10.738564091));
#298031=CARTESIAN_POINT('Ctrl Pts',(-0.222910044000055,15.2,-10.736167171));
#298032=CARTESIAN_POINT('Ctrl Pts',(-0.222910044000055,11.6,-10.736167171));
#298033=CARTESIAN_POINT('Ctrl Pts',(-0.222183905000056,15.2,-10.733775512));
#298034=CARTESIAN_POINT('Ctrl Pts',(-0.222183905000056,11.6,-10.733775512));
#298035=CARTESIAN_POINT('Ctrl Pts',(-0.221461609000055,15.2,-10.731389127));
#298036=CARTESIAN_POINT('Ctrl Pts',(-0.221461609000055,11.6,-10.731389127));
#298037=CARTESIAN_POINT('Ctrl Pts',(-0.220743152000056,15.2,-10.729008033));
#298038=CARTESIAN_POINT('Ctrl Pts',(-0.220743152000056,11.6,-10.729008033));
#298039=CARTESIAN_POINT('Ctrl Pts',(-0.220028527000055,15.2,-10.726632241));
#298040=CARTESIAN_POINT('Ctrl Pts',(-0.220028527000055,11.6,-10.726632241));
#298041=CARTESIAN_POINT('Ctrl Pts',(-0.219317730000055,15.2,-10.724261768));
#298042=CARTESIAN_POINT('Ctrl Pts',(-0.219317730000055,11.6,-10.724261768));
#298043=CARTESIAN_POINT('Ctrl Pts',(-0.218610753000055,15.2,-10.721896628));
#298044=CARTESIAN_POINT('Ctrl Pts',(-0.218610753000055,11.6,-10.721896628));
#298045=CARTESIAN_POINT('Ctrl Pts',(-0.217907594000056,15.2,-10.719536833));
#298046=CARTESIAN_POINT('Ctrl Pts',(-0.217907594000056,11.6,-10.719536833));
#298047=CARTESIAN_POINT('Ctrl Pts',(-0.217208245000055,15.2,-10.7171824));
#298048=CARTESIAN_POINT('Ctrl Pts',(-0.217208245000055,11.6,-10.7171824));
#298049=CARTESIAN_POINT('Ctrl Pts',(-0.216512700000056,15.2,-10.714833341));
#298050=CARTESIAN_POINT('Ctrl Pts',(-0.216512700000056,11.6,-10.714833341));
#298051=CARTESIAN_POINT('Ctrl Pts',(-0.215820955000057,15.2,-10.712489673));
#298052=CARTESIAN_POINT('Ctrl Pts',(-0.215820955000057,11.6,-10.712489673));
#298053=CARTESIAN_POINT('Ctrl Pts',(-0.215133003000056,15.2,-10.710151408));
#298054=CARTESIAN_POINT('Ctrl Pts',(-0.215133003000056,11.6,-10.710151408));
#298055=CARTESIAN_POINT('Ctrl Pts',(-0.214448839000055,15.2,-10.707818562));
#298056=CARTESIAN_POINT('Ctrl Pts',(-0.214448839000055,11.6,-10.707818562));
#298057=CARTESIAN_POINT('Ctrl Pts',(-0.213768458000055,15.2,-10.705491151));
#298058=CARTESIAN_POINT('Ctrl Pts',(-0.213768458000055,11.6,-10.705491151));
#298059=CARTESIAN_POINT('Ctrl Pts',(-0.213091853000057,15.2,-10.703169187));
#298060=CARTESIAN_POINT('Ctrl Pts',(-0.213091853000057,11.6,-10.703169187));
#298061=CARTESIAN_POINT('Ctrl Pts',(-0.212419019000055,15.2,-10.700852684));
#298062=CARTESIAN_POINT('Ctrl Pts',(-0.212419019000055,11.6,-10.700852684));
#298063=CARTESIAN_POINT('Ctrl Pts',(-0.211749948000056,15.2,-10.69854166));
#298064=CARTESIAN_POINT('Ctrl Pts',(-0.211749948000056,11.6,-10.69854166));
#298065=CARTESIAN_POINT('Ctrl Pts',(-0.211084639000055,15.2,-10.696236127));
#298066=CARTESIAN_POINT('Ctrl Pts',(-0.211084639000055,11.6,-10.696236127));
#298067=CARTESIAN_POINT('Ctrl Pts',(-0.210423081000056,15.2,-10.693936102));
#298068=CARTESIAN_POINT('Ctrl Pts',(-0.210423081000056,11.6,-10.693936102));
#298069=CARTESIAN_POINT('Ctrl Pts',(-0.209765271000055,15.2,-10.691641597));
#298070=CARTESIAN_POINT('Ctrl Pts',(-0.209765271000055,11.6,-10.691641597));
#298071=CARTESIAN_POINT('Ctrl Pts',(-0.209111203000055,15.2,-10.68935263));
#298072=CARTESIAN_POINT('Ctrl Pts',(-0.209111203000055,11.6,-10.68935263));
#298073=CARTESIAN_POINT('Ctrl Pts',(-0.208460870000057,15.2,-10.687069213));
#298074=CARTESIAN_POINT('Ctrl Pts',(-0.208460870000057,11.6,-10.687069213));
#298075=CARTESIAN_POINT('Ctrl Pts',(-0.207814267000056,15.2,-10.684791362));
#298076=CARTESIAN_POINT('Ctrl Pts',(-0.207814267000056,11.6,-10.684791362));
#298077=CARTESIAN_POINT('Ctrl Pts',(-0.207171387000056,15.2,-10.682519093));
#298078=CARTESIAN_POINT('Ctrl Pts',(-0.207171387000056,11.6,-10.682519093));
#298079=CARTESIAN_POINT('Ctrl Pts',(-0.206532225000055,15.2,-10.68025242));
#298080=CARTESIAN_POINT('Ctrl Pts',(-0.206532225000055,11.6,-10.68025242));
#298081=CARTESIAN_POINT('Ctrl Pts',(-0.205896774000056,15.2,-10.677991357));
#298082=CARTESIAN_POINT('Ctrl Pts',(-0.205896774000056,11.6,-10.677991357));
#298083=CARTESIAN_POINT('Ctrl Pts',(-0.205265029000056,15.2,-10.67573592));
#298084=CARTESIAN_POINT('Ctrl Pts',(-0.205265029000056,11.6,-10.67573592));
#298085=CARTESIAN_POINT('Ctrl Pts',(-0.204636983000055,15.2,-10.673486125));
#298086=CARTESIAN_POINT('Ctrl Pts',(-0.204636983000055,11.6,-10.673486125));
#298087=CARTESIAN_POINT('Ctrl Pts',(-0.204012631000056,15.2,-10.671241986));
#298088=CARTESIAN_POINT('Ctrl Pts',(-0.204012631000056,11.6,-10.671241986));
#298089=CARTESIAN_POINT('Ctrl Pts',(-0.203391965000056,15.2,-10.669003519));
#298090=CARTESIAN_POINT('Ctrl Pts',(-0.203391965000056,11.6,-10.669003519));
#298091=CARTESIAN_POINT('Ctrl Pts',(-0.202774980000056,15.2,-10.666770738));
#298092=CARTESIAN_POINT('Ctrl Pts',(-0.202774980000056,11.6,-10.666770738));
#298093=CARTESIAN_POINT('Ctrl Pts',(-0.202161670000055,15.2,-10.664543659));
#298094=CARTESIAN_POINT('Ctrl Pts',(-0.202161670000055,11.6,-10.664543659));
#298095=CARTESIAN_POINT('Ctrl Pts',(-0.201552028000057,15.2,-10.662322297));
#298096=CARTESIAN_POINT('Ctrl Pts',(-0.201552028000057,11.6,-10.662322297));
#298097=CARTESIAN_POINT('Ctrl Pts',(-0.200946049000056,15.2,-10.660106669));
#298098=CARTESIAN_POINT('Ctrl Pts',(-0.200946049000056,11.6,-10.660106669));
#298099=CARTESIAN_POINT('Ctrl Pts',(-0.200343725000056,15.2,-10.657896788));
#298100=CARTESIAN_POINT('Ctrl Pts',(-0.200343725000056,11.6,-10.657896788));
#298101=CARTESIAN_POINT('Ctrl Pts',(-0.199745051000055,15.2,-10.655692671));
#298102=CARTESIAN_POINT('Ctrl Pts',(-0.199745051000055,11.6,-10.655692671));
#298103=CARTESIAN_POINT('Ctrl Pts',(-0.199150020000056,15.2,-10.653494333));
#298104=CARTESIAN_POINT('Ctrl Pts',(-0.199150020000056,11.6,-10.653494333));
#298105=CARTESIAN_POINT('Ctrl Pts',(-0.198558626000055,15.2,-10.651301789));
#298106=CARTESIAN_POINT('Ctrl Pts',(-0.198558626000055,11.6,-10.651301789));
#298107=CARTESIAN_POINT('Ctrl Pts',(-0.197970862000056,15.2,-10.649115056));
#298108=CARTESIAN_POINT('Ctrl Pts',(-0.197970862000056,11.6,-10.649115056));
#298109=CARTESIAN_POINT('Ctrl Pts',(-0.197386723000056,15.2,-10.646934148));
#298110=CARTESIAN_POINT('Ctrl Pts',(-0.197386723000056,11.6,-10.646934148));
#298111=CARTESIAN_POINT('Ctrl Pts',(-0.196806201000056,15.2,-10.644759081));
#298112=CARTESIAN_POINT('Ctrl Pts',(-0.196806201000056,11.6,-10.644759081));
#298113=CARTESIAN_POINT('Ctrl Pts',(-0.196229289000056,15.2,-10.642589871));
#298114=CARTESIAN_POINT('Ctrl Pts',(-0.196229289000056,11.6,-10.642589871));
#298115=CARTESIAN_POINT('Ctrl Pts',(-0.195655982000057,15.2,-10.640426534));
#298116=CARTESIAN_POINT('Ctrl Pts',(-0.195655982000057,11.6,-10.640426534));
#298117=CARTESIAN_POINT('Ctrl Pts',(-0.195086274000056,15.2,-10.638269086));
#298118=CARTESIAN_POINT('Ctrl Pts',(-0.195086274000056,11.6,-10.638269086));
#298119=CARTESIAN_POINT('Ctrl Pts',(-0.194520156000056,15.2,-10.636117541));
#298120=CARTESIAN_POINT('Ctrl Pts',(-0.194520156000056,11.6,-10.636117541));
#298121=CARTESIAN_POINT('Ctrl Pts',(-0.193957623000056,15.2,-10.633971916));
#298122=CARTESIAN_POINT('Ctrl Pts',(-0.193957623000056,11.6,-10.633971916));
#298123=CARTESIAN_POINT('Ctrl Pts',(-0.193398667000055,15.2,-10.631832228));
#298124=CARTESIAN_POINT('Ctrl Pts',(-0.193398667000055,11.6,-10.631832228));
#298125=CARTESIAN_POINT('Ctrl Pts',(-0.192843283000055,15.2,-10.629698492));
#298126=CARTESIAN_POINT('Ctrl Pts',(-0.192843283000055,11.6,-10.629698492));
#298127=CARTESIAN_POINT('Ctrl Pts',(-0.192291464000055,15.2,-10.627570723));
#298128=CARTESIAN_POINT('Ctrl Pts',(-0.192291464000055,11.6,-10.627570723));
#298129=CARTESIAN_POINT('Ctrl Pts',(-0.191743203000057,15.2,-10.62544894));
#298130=CARTESIAN_POINT('Ctrl Pts',(-0.191743203000057,11.6,-10.62544894));
#298131=CARTESIAN_POINT('Ctrl Pts',(-0.191198493000057,15.2,-10.623333156));
#298132=CARTESIAN_POINT('Ctrl Pts',(-0.191198493000057,11.6,-10.623333156));
#298133=CARTESIAN_POINT('Ctrl Pts',(-0.190657326000055,15.2,-10.621223388));
#298134=CARTESIAN_POINT('Ctrl Pts',(-0.190657326000055,11.6,-10.621223388));
#298135=CARTESIAN_POINT('Ctrl Pts',(-0.190119697000056,15.2,-10.619119652));
#298136=CARTESIAN_POINT('Ctrl Pts',(-0.190119697000056,11.6,-10.619119652));
#298137=CARTESIAN_POINT('Ctrl Pts',(-0.189585599000056,15.2,-10.617021965));
#298138=CARTESIAN_POINT('Ctrl Pts',(-0.189585599000056,11.6,-10.617021965));
#298139=CARTESIAN_POINT('Ctrl Pts',(-0.189055024000057,15.2,-10.614930343));
#298140=CARTESIAN_POINT('Ctrl Pts',(-0.189055024000057,11.6,-10.614930343));
#298141=CARTESIAN_POINT('Ctrl Pts',(-0.188527965000055,15.2,-10.612844802));
#298142=CARTESIAN_POINT('Ctrl Pts',(-0.188527965000055,11.6,-10.612844802));
#298143=CARTESIAN_POINT('Ctrl Pts',(-0.188004417000055,15.2,-10.610765359));
#298144=CARTESIAN_POINT('Ctrl Pts',(-0.188004417000055,11.6,-10.610765359));
#298145=CARTESIAN_POINT('Ctrl Pts',(-0.187484370000056,15.2,-10.60869203));
#298146=CARTESIAN_POINT('Ctrl Pts',(-0.187484370000056,11.6,-10.60869203));
#298147=CARTESIAN_POINT('Ctrl Pts',(-0.186967820000056,15.2,-10.606624832));
#298148=CARTESIAN_POINT('Ctrl Pts',(-0.186967820000056,11.6,-10.606624832));
#298149=CARTESIAN_POINT('Ctrl Pts',(-0.186454758000056,15.2,-10.60456378));
#298150=CARTESIAN_POINT('Ctrl Pts',(-0.186454758000056,11.6,-10.60456378));
#298151=CARTESIAN_POINT('Ctrl Pts',(-0.185945177000055,15.2,-10.602508892));
#298152=CARTESIAN_POINT('Ctrl Pts',(-0.185945177000055,11.6,-10.602508892));
#298153=CARTESIAN_POINT('Ctrl Pts',(-0.185439071000056,15.2,-10.600460183));
#298154=CARTESIAN_POINT('Ctrl Pts',(-0.185439071000056,11.6,-10.600460183));
#298155=CARTESIAN_POINT('Ctrl Pts',(-0.184936432000056,15.2,-10.598417672));
#298156=CARTESIAN_POINT('Ctrl Pts',(-0.184936432000056,11.6,-10.598417672));
#298157=CARTESIAN_POINT('Ctrl Pts',(-0.184437253000055,15.2,-10.596381375));
#298158=CARTESIAN_POINT('Ctrl Pts',(-0.184437253000055,11.6,-10.596381375));
#298159=CARTESIAN_POINT('Ctrl Pts',(-0.183941526000057,15.2,-10.594351307));
#298160=CARTESIAN_POINT('Ctrl Pts',(-0.183941526000057,11.6,-10.594351307));
#298161=CARTESIAN_POINT('Ctrl Pts',(-0.183449244000055,15.2,-10.592327487));
#298162=CARTESIAN_POINT('Ctrl Pts',(-0.183449244000055,11.6,-10.592327487));
#298163=CARTESIAN_POINT('Ctrl Pts',(-0.182960401000055,15.2,-10.59030993));
#298164=CARTESIAN_POINT('Ctrl Pts',(-0.182960401000055,11.6,-10.59030993));
#298165=CARTESIAN_POINT('Ctrl Pts',(-0.182474988000055,15.2,-10.588298654));
#298166=CARTESIAN_POINT('Ctrl Pts',(-0.182474988000055,11.6,-10.588298654));
#298167=CARTESIAN_POINT('Ctrl Pts',(-0.181992998000055,15.2,-10.586293676));
#298168=CARTESIAN_POINT('Ctrl Pts',(-0.181992998000055,11.6,-10.586293676));
#298169=CARTESIAN_POINT('Ctrl Pts',(-0.181514425000057,15.2,-10.584295012));
#298170=CARTESIAN_POINT('Ctrl Pts',(-0.181514425000057,11.6,-10.584295012));
#298171=CARTESIAN_POINT('Ctrl Pts',(-0.181039260000055,15.2,-10.582302681));
#298172=CARTESIAN_POINT('Ctrl Pts',(-0.181039260000055,11.6,-10.582302681));
#298173=CARTESIAN_POINT('Ctrl Pts',(-0.180567496000055,15.2,-10.580316698));
#298174=CARTESIAN_POINT('Ctrl Pts',(-0.180567496000055,11.6,-10.580316698));
#298175=CARTESIAN_POINT('Ctrl Pts',(-0.180099125000056,15.2,-10.578337081));
#298176=CARTESIAN_POINT('Ctrl Pts',(-0.180099125000056,11.6,-10.578337081));
#298177=CARTESIAN_POINT('Ctrl Pts',(-0.179634139000056,15.2,-10.576363848));
#298178=CARTESIAN_POINT('Ctrl Pts',(-0.179634139000056,11.6,-10.576363848));
#298179=CARTESIAN_POINT('Ctrl Pts',(-0.179172532000056,15.2,-10.574397014));
#298180=CARTESIAN_POINT('Ctrl Pts',(-0.179172532000056,11.6,-10.574397014));
#298181=CARTESIAN_POINT('Ctrl Pts',(-0.178714296000055,15.2,-10.572436599));
#298182=CARTESIAN_POINT('Ctrl Pts',(-0.178714296000055,11.6,-10.572436599));
#298183=CARTESIAN_POINT('Ctrl Pts',(-0.178259423000057,15.2,-10.570482619));
#298184=CARTESIAN_POINT('Ctrl Pts',(-0.178259423000057,11.6,-10.570482619));
#298185=CARTESIAN_POINT('Ctrl Pts',(-0.177807905000057,15.2,-10.568535092));
#298186=CARTESIAN_POINT('Ctrl Pts',(-0.177807905000057,11.6,-10.568535092));
#298187=CARTESIAN_POINT('Ctrl Pts',(-0.177359734000057,15.2,-10.566594035));
#298188=CARTESIAN_POINT('Ctrl Pts',(-0.177359734000057,11.6,-10.566594035));
#298189=CARTESIAN_POINT('Ctrl Pts',(-0.176914903000055,15.2,-10.564659465));
#298190=CARTESIAN_POINT('Ctrl Pts',(-0.176914903000055,11.6,-10.564659465));
#298191=CARTESIAN_POINT('Ctrl Pts',(-0.176473403000056,15.2,-10.562731399));
#298192=CARTESIAN_POINT('Ctrl Pts',(-0.176473403000056,11.6,-10.562731399));
#298193=CARTESIAN_POINT('Ctrl Pts',(-0.176035228000057,15.2,-10.560809857));
#298194=CARTESIAN_POINT('Ctrl Pts',(-0.176035228000057,11.6,-10.560809857));
#298195=CARTESIAN_POINT('Ctrl Pts',(-0.175600369000056,15.2,-10.558894856));
#298196=CARTESIAN_POINT('Ctrl Pts',(-0.175600369000056,11.6,-10.558894856));
#298197=CARTESIAN_POINT('Ctrl Pts',(-0.175168818000057,15.2,-10.556986413));
#298198=CARTESIAN_POINT('Ctrl Pts',(-0.175168818000057,11.6,-10.556986413));
#298199=CARTESIAN_POINT('Ctrl Pts',(-0.174740568000056,15.2,-10.555084546));
#298200=CARTESIAN_POINT('Ctrl Pts',(-0.174740568000056,11.6,-10.555084546));
#298201=CARTESIAN_POINT('Ctrl Pts',(-0.174315609000055,15.2,-10.553189273));
#298202=CARTESIAN_POINT('Ctrl Pts',(-0.174315609000055,11.6,-10.553189273));
#298203=CARTESIAN_POINT('Ctrl Pts',(-0.173893934000056,15.2,-10.551300611));
#298204=CARTESIAN_POINT('Ctrl Pts',(-0.173893934000056,11.6,-10.551300611));
#298205=CARTESIAN_POINT('Ctrl Pts',(-0.173475537000056,15.2,-10.549418579));
#298206=CARTESIAN_POINT('Ctrl Pts',(-0.173475537000056,11.6,-10.549418579));
#298207=CARTESIAN_POINT('Ctrl Pts',(-0.173060406000056,15.2,-10.547543195));
#298208=CARTESIAN_POINT('Ctrl Pts',(-0.173060406000056,11.6,-10.547543195));
#298209=CARTESIAN_POINT('Ctrl Pts',(-0.172648536000055,15.2,-10.545674477));
#298210=CARTESIAN_POINT('Ctrl Pts',(-0.172648536000055,11.6,-10.545674477));
#298211=CARTESIAN_POINT('Ctrl Pts',(-0.172239916000055,15.2,-10.543812443));
#298212=CARTESIAN_POINT('Ctrl Pts',(-0.172239916000055,11.6,-10.543812443));
#298213=CARTESIAN_POINT('Ctrl Pts',(-0.171834541000055,15.2,-10.541957111));
#298214=CARTESIAN_POINT('Ctrl Pts',(-0.171834541000055,11.6,-10.541957111));
#298215=CARTESIAN_POINT('Ctrl Pts',(-0.171432400000056,15.2,-10.5401085));
#298216=CARTESIAN_POINT('Ctrl Pts',(-0.171432400000056,11.6,-10.5401085));
#298217=CARTESIAN_POINT('Ctrl Pts',(-0.171033486000055,15.2,-10.538266627));
#298218=CARTESIAN_POINT('Ctrl Pts',(-0.171033486000055,11.6,-10.538266627));
#298219=CARTESIAN_POINT('Ctrl Pts',(-0.170637791000056,15.2,-10.536431511));
#298220=CARTESIAN_POINT('Ctrl Pts',(-0.170637791000056,11.6,-10.536431511));
#298221=CARTESIAN_POINT('Ctrl Pts',(-0.170245305000056,15.2,-10.534603171));
#298222=CARTESIAN_POINT('Ctrl Pts',(-0.170245305000056,11.6,-10.534603171));
#298223=CARTESIAN_POINT('Ctrl Pts',(-0.169856021000055,15.2,-10.532781626));
#298224=CARTESIAN_POINT('Ctrl Pts',(-0.169856021000055,11.6,-10.532781626));
#298225=CARTESIAN_POINT('Ctrl Pts',(-0.169469930000057,15.2,-10.530966892));
#298226=CARTESIAN_POINT('Ctrl Pts',(-0.169469930000057,11.6,-10.530966892));
#298227=CARTESIAN_POINT('Ctrl Pts',(-0.169087023000056,15.2,-10.529158991));
#298228=CARTESIAN_POINT('Ctrl Pts',(-0.169087023000056,11.6,-10.529158991));
#298229=CARTESIAN_POINT('Ctrl Pts',(-0.168707293000055,15.2,-10.527357938));
#298230=CARTESIAN_POINT('Ctrl Pts',(-0.168707293000055,11.6,-10.527357938));
#298231=CARTESIAN_POINT('Ctrl Pts',(-0.168330729000056,15.2,-10.525563754));
#298232=CARTESIAN_POINT('Ctrl Pts',(-0.168330729000056,11.6,-10.525563754));
#298233=CARTESIAN_POINT('Ctrl Pts',(-0.167957324000056,15.2,-10.523776458));
#298234=CARTESIAN_POINT('Ctrl Pts',(-0.167957324000056,11.6,-10.523776458));
#298235=CARTESIAN_POINT('Ctrl Pts',(-0.167587069000056,15.2,-10.521996069));
#298236=CARTESIAN_POINT('Ctrl Pts',(-0.167587069000056,11.6,-10.521996069));
#298237=CARTESIAN_POINT('Ctrl Pts',(-0.167219956000055,15.2,-10.520222604));
#298238=CARTESIAN_POINT('Ctrl Pts',(-0.167219956000055,11.6,-10.520222604));
#298239=CARTESIAN_POINT('Ctrl Pts',(-0.166855974000055,15.2,-10.518456084));
#298240=CARTESIAN_POINT('Ctrl Pts',(-0.166855974000055,11.6,-10.518456084));
#298241=CARTESIAN_POINT('Ctrl Pts',(-0.166495117000055,15.2,-10.516696527));
#298242=CARTESIAN_POINT('Ctrl Pts',(-0.166495117000055,11.6,-10.516696527));
#298243=CARTESIAN_POINT('Ctrl Pts',(-0.166137374000056,15.2,-10.514943952));
#298244=CARTESIAN_POINT('Ctrl Pts',(-0.166137374000056,11.6,-10.514943952));
#298245=CARTESIAN_POINT('Ctrl Pts',(-0.165782737000055,15.2,-10.513198378));
#298246=CARTESIAN_POINT('Ctrl Pts',(-0.165782737000055,11.6,-10.513198378));
#298247=CARTESIAN_POINT('Ctrl Pts',(-0.165431198000056,15.2,-10.511459826));
#298248=CARTESIAN_POINT('Ctrl Pts',(-0.165431198000056,11.6,-10.511459826));
#298249=CARTESIAN_POINT('Ctrl Pts',(-0.165082744000056,15.2,-10.509728314));
#298250=CARTESIAN_POINT('Ctrl Pts',(-0.165082744000056,11.6,-10.509728314));
#298251=CARTESIAN_POINT('Ctrl Pts',(-0.164737371000055,15.2,-10.508003862));
#298252=CARTESIAN_POINT('Ctrl Pts',(-0.164737371000055,11.6,-10.508003862));
#298253=CARTESIAN_POINT('Ctrl Pts',(-0.164395067000056,15.2,-10.506286487));
#298254=CARTESIAN_POINT('Ctrl Pts',(-0.164395067000056,11.6,-10.506286487));
#298255=CARTESIAN_POINT('Ctrl Pts',(-0.164055824000057,15.2,-10.504576212));
#298256=CARTESIAN_POINT('Ctrl Pts',(-0.164055824000057,11.6,-10.504576212));
#298257=CARTESIAN_POINT('Ctrl Pts',(-0.163719632000056,15.2,-10.502873055));
#298258=CARTESIAN_POINT('Ctrl Pts',(-0.163719632000056,11.6,-10.502873055));
#298259=CARTESIAN_POINT('Ctrl Pts',(-0.163386483000056,15.2,-10.501177036));
#298260=CARTESIAN_POINT('Ctrl Pts',(-0.163386483000056,11.6,-10.501177036));
#298261=CARTESIAN_POINT('Ctrl Pts',(-0.163056366000056,15.2,-10.499488173));
#298262=CARTESIAN_POINT('Ctrl Pts',(-0.163056366000056,11.6,-10.499488173));
#298263=CARTESIAN_POINT('Ctrl Pts',(-0.162729274000055,15.2,-10.497806488));
#298264=CARTESIAN_POINT('Ctrl Pts',(-0.162729274000055,11.6,-10.497806488));
#298265=CARTESIAN_POINT('Ctrl Pts',(-0.162405194000056,15.2,-10.496131999));
#298266=CARTESIAN_POINT('Ctrl Pts',(-0.162405194000056,11.6,-10.496131999));
#298267=CARTESIAN_POINT('Ctrl Pts',(-0.162084120000056,15.2,-10.494464728));
#298268=CARTESIAN_POINT('Ctrl Pts',(-0.162084120000056,11.6,-10.494464728));
#298269=CARTESIAN_POINT('Ctrl Pts',(-0.161766042000057,15.2,-10.492804693));
#298270=CARTESIAN_POINT('Ctrl Pts',(-0.161766042000057,11.6,-10.492804693));
#298271=CARTESIAN_POINT('Ctrl Pts',(-0.161450949000056,15.2,-10.491151915));
#298272=CARTESIAN_POINT('Ctrl Pts',(-0.161450949000056,11.6,-10.491151915));
#298273=CARTESIAN_POINT('Ctrl Pts',(-0.161138833000055,15.2,-10.489506414));
#298274=CARTESIAN_POINT('Ctrl Pts',(-0.161138833000055,11.6,-10.489506414));
#298275=CARTESIAN_POINT('Ctrl Pts',(-0.160829682000055,15.2,-10.487868211));
#298276=CARTESIAN_POINT('Ctrl Pts',(-0.160829682000055,11.6,-10.487868211));
#298277=CARTESIAN_POINT('Ctrl Pts',(-0.160523489000056,15.2,-10.486237324));
#298278=CARTESIAN_POINT('Ctrl Pts',(-0.160523489000056,11.6,-10.486237324));
#298279=CARTESIAN_POINT('Ctrl Pts',(-0.160220245000057,15.2,-10.484613776));
#298280=CARTESIAN_POINT('Ctrl Pts',(-0.160220245000057,11.6,-10.484613776));
#298281=CARTESIAN_POINT('Ctrl Pts',(-0.159919937000056,15.2,-10.482997586));
#298282=CARTESIAN_POINT('Ctrl Pts',(-0.159919937000056,11.6,-10.482997586));
#298283=CARTESIAN_POINT('Ctrl Pts',(-0.159622556000055,15.2,-10.481388775));
#298284=CARTESIAN_POINT('Ctrl Pts',(-0.159622556000055,11.6,-10.481388775));
#298285=CARTESIAN_POINT('Ctrl Pts',(-0.159328094000056,15.2,-10.479787363));
#298286=CARTESIAN_POINT('Ctrl Pts',(-0.159328094000056,11.6,-10.479787363));
#298287=CARTESIAN_POINT('Ctrl Pts',(-0.159036540000056,15.2,-10.478193371));
#298288=CARTESIAN_POINT('Ctrl Pts',(-0.159036540000056,11.6,-10.478193371));
#298289=CARTESIAN_POINT('Ctrl Pts',(-0.158747884000056,15.2,-10.476606819));
#298290=CARTESIAN_POINT('Ctrl Pts',(-0.158747884000056,11.6,-10.476606819));
#298291=CARTESIAN_POINT('Ctrl Pts',(-0.158462117000056,15.2,-10.475027729));
#298292=CARTESIAN_POINT('Ctrl Pts',(-0.158462117000056,11.6,-10.475027729));
#298293=CARTESIAN_POINT('Ctrl Pts',(-0.158179227000056,15.2,-10.473456121));
#298294=CARTESIAN_POINT('Ctrl Pts',(-0.158179227000056,11.6,-10.473456121));
#298295=CARTESIAN_POINT('Ctrl Pts',(-0.157899205000056,15.2,-10.471892016));
#298296=CARTESIAN_POINT('Ctrl Pts',(-0.157899205000056,11.6,-10.471892016));
#298297=CARTESIAN_POINT('Ctrl Pts',(-0.157622041000056,15.2,-10.470335435));
#298298=CARTESIAN_POINT('Ctrl Pts',(-0.157622041000056,11.6,-10.470335435));
#298299=CARTESIAN_POINT('Ctrl Pts',(-0.157347725000055,15.2,-10.4687864));
#298300=CARTESIAN_POINT('Ctrl Pts',(-0.157347725000055,11.6,-10.4687864));
#298301=CARTESIAN_POINT('Ctrl Pts',(-0.157076245000055,15.2,-10.467244931));
#298302=CARTESIAN_POINT('Ctrl Pts',(-0.157076245000055,11.6,-10.467244931));
#298303=CARTESIAN_POINT('Ctrl Pts',(-0.156807594000057,15.2,-10.46571105));
#298304=CARTESIAN_POINT('Ctrl Pts',(-0.156807594000057,11.6,-10.46571105));
#298305=CARTESIAN_POINT('Ctrl Pts',(-0.156541758000056,15.2,-10.464184778));
#298306=CARTESIAN_POINT('Ctrl Pts',(-0.156541758000056,11.6,-10.464184778));
#298307=CARTESIAN_POINT('Ctrl Pts',(-0.156278730000056,15.2,-10.462666135));
#298308=CARTESIAN_POINT('Ctrl Pts',(-0.156278730000056,11.6,-10.462666135));
#298309=CARTESIAN_POINT('Ctrl Pts',(-0.156018496000057,15.2,-10.461155145));
#298310=CARTESIAN_POINT('Ctrl Pts',(-0.156018496000057,11.6,-10.461155145));
#298311=CARTESIAN_POINT('Ctrl Pts',(-0.155761048000055,15.2,-10.459651829));
#298312=CARTESIAN_POINT('Ctrl Pts',(-0.155761048000055,11.6,-10.459651829));
#298313=CARTESIAN_POINT('Ctrl Pts',(-0.155506375000056,15.2,-10.458156207));
#298314=CARTESIAN_POINT('Ctrl Pts',(-0.155506375000056,11.6,-10.458156207));
#298315=CARTESIAN_POINT('Ctrl Pts',(-0.155254466000055,15.2,-10.456668302));
#298316=CARTESIAN_POINT('Ctrl Pts',(-0.155254466000055,11.6,-10.456668302));
#298317=CARTESIAN_POINT('Ctrl Pts',(-0.155005310000057,15.2,-10.455188136));
#298318=CARTESIAN_POINT('Ctrl Pts',(-0.155005310000057,11.6,-10.455188136));
#298319=CARTESIAN_POINT('Ctrl Pts',(-0.154758897000056,15.2,-10.45371573));
#298320=CARTESIAN_POINT('Ctrl Pts',(-0.154758897000056,11.6,-10.45371573));
#298321=CARTESIAN_POINT('Ctrl Pts',(-0.154515216000056,15.2,-10.452251106));
#298322=CARTESIAN_POINT('Ctrl Pts',(-0.154515216000056,11.6,-10.452251106));
#298323=CARTESIAN_POINT('Ctrl Pts',(-0.154274256000055,15.2,-10.450794288));
#298324=CARTESIAN_POINT('Ctrl Pts',(-0.154274256000055,11.6,-10.450794288));
#298325=CARTESIAN_POINT('Ctrl Pts',(-0.154036006000055,15.2,-10.449345296));
#298326=CARTESIAN_POINT('Ctrl Pts',(-0.154036006000055,11.6,-10.449345296));
#298327=CARTESIAN_POINT('Ctrl Pts',(-0.153800456000056,15.2,-10.447904152));
#298328=CARTESIAN_POINT('Ctrl Pts',(-0.153800456000056,11.6,-10.447904152));
#298329=CARTESIAN_POINT('Ctrl Pts',(-0.153567593000057,15.2,-10.446470879));
#298330=CARTESIAN_POINT('Ctrl Pts',(-0.153567593000057,11.6,-10.446470879));
#298331=CARTESIAN_POINT('Ctrl Pts',(-0.153337407000055,15.2,-10.4450455));
#298332=CARTESIAN_POINT('Ctrl Pts',(-0.153337407000055,11.6,-10.4450455));
#298333=CARTESIAN_POINT('Ctrl Pts',(-0.153109888000056,15.2,-10.443628038));
#298334=CARTESIAN_POINT('Ctrl Pts',(-0.153109888000056,11.6,-10.443628038));
#298335=CARTESIAN_POINT('Ctrl Pts',(-0.152885022000057,15.2,-10.442218514));
#298336=CARTESIAN_POINT('Ctrl Pts',(-0.152885022000057,11.6,-10.442218514));
#298337=CARTESIAN_POINT('Ctrl Pts',(-0.152662802000056,15.2,-10.440816951));
#298338=CARTESIAN_POINT('Ctrl Pts',(-0.152662802000056,11.6,-10.440816951));
#298339=CARTESIAN_POINT('Ctrl Pts',(-0.152443212000056,15.2,-10.439423372));
#298340=CARTESIAN_POINT('Ctrl Pts',(-0.152443212000056,11.6,-10.439423372));
#298341=CARTESIAN_POINT('Ctrl Pts',(-0.152226243000056,15.2,-10.4380378));
#298342=CARTESIAN_POINT('Ctrl Pts',(-0.152226243000056,11.6,-10.4380378));
#298343=CARTESIAN_POINT('Ctrl Pts',(-0.152011884000055,15.2,-10.436660258));
#298344=CARTESIAN_POINT('Ctrl Pts',(-0.152011884000055,11.6,-10.436660258));
#298345=CARTESIAN_POINT('Ctrl Pts',(-0.151800122000055,15.2,-10.435290769));
#298346=CARTESIAN_POINT('Ctrl Pts',(-0.151800122000055,11.6,-10.435290769));
#298347=CARTESIAN_POINT('Ctrl Pts',(-0.151590948000055,15.2,-10.433929354));
#298348=CARTESIAN_POINT('Ctrl Pts',(-0.151590948000055,11.6,-10.433929354));
#298349=CARTESIAN_POINT('Ctrl Pts',(-0.151384347000055,15.2,-10.43257604));
#298350=CARTESIAN_POINT('Ctrl Pts',(-0.151384347000055,11.6,-10.43257604));
#298351=CARTESIAN_POINT('Ctrl Pts',(-0.151180310000055,15.2,-10.431230848));
#298352=CARTESIAN_POINT('Ctrl Pts',(-0.151180310000055,11.6,-10.431230848));
#298353=CARTESIAN_POINT('Ctrl Pts',(-0.150978823000055,15.2,-10.429893802));
#298354=CARTESIAN_POINT('Ctrl Pts',(-0.150978823000055,11.6,-10.429893802));
#298355=CARTESIAN_POINT('Ctrl Pts',(-0.150779876000057,15.2,-10.428564925));
#298356=CARTESIAN_POINT('Ctrl Pts',(-0.150779876000057,11.6,-10.428564925));
#298357=CARTESIAN_POINT('Ctrl Pts',(-0.150583457000056,15.2,-10.427244241));
#298358=CARTESIAN_POINT('Ctrl Pts',(-0.150583457000056,11.6,-10.427244241));
#298359=CARTESIAN_POINT('Ctrl Pts',(-0.150389553000055,15.2,-10.425931773));
#298360=CARTESIAN_POINT('Ctrl Pts',(-0.150389553000055,11.6,-10.425931773));
#298361=CARTESIAN_POINT('Ctrl Pts',(-0.150198154000056,15.2,-10.424627545));
#298362=CARTESIAN_POINT('Ctrl Pts',(-0.150198154000056,11.6,-10.424627545));
#298363=CARTESIAN_POINT('Ctrl Pts',(-0.150009246000057,15.2,-10.423331583));
#298364=CARTESIAN_POINT('Ctrl Pts',(-0.150009246000057,11.6,-10.423331583));
#298365=CARTESIAN_POINT('Ctrl Pts',(-0.149822818000055,15.2,-10.422043907));
#298366=CARTESIAN_POINT('Ctrl Pts',(-0.149822818000055,11.6,-10.422043907));
#298367=CARTESIAN_POINT('Ctrl Pts',(-0.149638856000056,15.2,-10.420764545));
#298368=CARTESIAN_POINT('Ctrl Pts',(-0.149638856000056,11.6,-10.420764545));
#298369=CARTESIAN_POINT('Ctrl Pts',(-0.149457350000055,15.2,-10.419493518));
#298370=CARTESIAN_POINT('Ctrl Pts',(-0.149457350000055,11.6,-10.419493518));
#298371=CARTESIAN_POINT('Ctrl Pts',(-0.149278286000056,15.2,-10.418230852));
#298372=CARTESIAN_POINT('Ctrl Pts',(-0.149278286000056,11.6,-10.418230852));
#298373=CARTESIAN_POINT('Ctrl Pts',(-0.149101652000055,15.2,-10.416976571));
#298374=CARTESIAN_POINT('Ctrl Pts',(-0.149101652000055,11.6,-10.416976571));
#298375=CARTESIAN_POINT('Ctrl Pts',(-0.148927437000056,15.2,-10.4157307));
#298376=CARTESIAN_POINT('Ctrl Pts',(-0.148927437000056,11.6,-10.4157307));
#298377=CARTESIAN_POINT('Ctrl Pts',(-0.148755627000057,15.2,-10.414493262));
#298378=CARTESIAN_POINT('Ctrl Pts',(-0.148755627000057,11.6,-10.414493262));
#298379=CARTESIAN_POINT('Ctrl Pts',(-0.148586210000056,15.2,-10.413264283));
#298380=CARTESIAN_POINT('Ctrl Pts',(-0.148586210000056,11.6,-10.413264283));
#298381=CARTESIAN_POINT('Ctrl Pts',(-0.148419173000055,15.2,-10.412043788));
#298382=CARTESIAN_POINT('Ctrl Pts',(-0.148419173000055,11.6,-10.412043788));
#298383=CARTESIAN_POINT('Ctrl Pts',(-0.148254502000055,15.2,-10.410831802));
#298384=CARTESIAN_POINT('Ctrl Pts',(-0.148254502000055,11.6,-10.410831802));
#298385=CARTESIAN_POINT('Ctrl Pts',(-0.148092187000056,15.2,-10.409628348));
#298386=CARTESIAN_POINT('Ctrl Pts',(-0.148092187000056,11.6,-10.409628348));
#298387=CARTESIAN_POINT('Ctrl Pts',(-0.147932214000056,15.2,-10.408433454));
#298388=CARTESIAN_POINT('Ctrl Pts',(-0.147932214000056,11.6,-10.408433454));
#298389=CARTESIAN_POINT('Ctrl Pts',(-0.147774569000055,15.2,-10.407247142));
#298390=CARTESIAN_POINT('Ctrl Pts',(-0.147774569000055,11.6,-10.407247142));
#298391=CARTESIAN_POINT('Ctrl Pts',(-0.147619240000055,15.2,-10.40606944));
#298392=CARTESIAN_POINT('Ctrl Pts',(-0.147619240000055,11.6,-10.40606944));
#298393=CARTESIAN_POINT('Ctrl Pts',(-0.147466215000056,15.2,-10.404900372));
#298394=CARTESIAN_POINT('Ctrl Pts',(-0.147466215000056,11.6,-10.404900372));
#298395=CARTESIAN_POINT('Ctrl Pts',(-0.147315478000056,15.2,-10.403739965));
#298396=CARTESIAN_POINT('Ctrl Pts',(-0.147315478000056,11.6,-10.403739965));
#298397=CARTESIAN_POINT('Ctrl Pts',(-0.147167017000056,15.2,-10.402588242));
#298398=CARTESIAN_POINT('Ctrl Pts',(-0.147167017000056,11.6,-10.402588242));
#298399=CARTESIAN_POINT('Ctrl Pts',(-0.147020820000057,15.2,-10.401445231));
#298400=CARTESIAN_POINT('Ctrl Pts',(-0.147020820000057,11.6,-10.401445231));
#298401=CARTESIAN_POINT('Ctrl Pts',(-0.146876872000057,15.2,-10.400310957));
#298402=CARTESIAN_POINT('Ctrl Pts',(-0.146876872000057,11.6,-10.400310957));
#298403=CARTESIAN_POINT('Ctrl Pts',(-0.146735160000055,15.2,-10.399185446));
#298404=CARTESIAN_POINT('Ctrl Pts',(-0.146735160000055,11.6,-10.399185446));
#298405=CARTESIAN_POINT('Ctrl Pts',(-0.146595671000057,15.2,-10.398068726));
#298406=CARTESIAN_POINT('Ctrl Pts',(-0.146595671000057,11.6,-10.398068726));
#298407=CARTESIAN_POINT('Ctrl Pts',(-0.146458391000056,15.2,-10.39696082));
#298408=CARTESIAN_POINT('Ctrl Pts',(-0.146458391000056,11.6,-10.39696082));
#298409=CARTESIAN_POINT('Ctrl Pts',(-0.146323306000056,15.2,-10.395861756));
#298410=CARTESIAN_POINT('Ctrl Pts',(-0.146323306000056,11.6,-10.395861756));
#298411=CARTESIAN_POINT('Ctrl Pts',(-0.146190404000055,15.2,-10.394771561));
#298412=CARTESIAN_POINT('Ctrl Pts',(-0.146190404000055,11.6,-10.394771561));
#298413=CARTESIAN_POINT('Ctrl Pts',(-0.146059668000056,15.2,-10.39369026));
#298414=CARTESIAN_POINT('Ctrl Pts',(-0.146059668000056,11.6,-10.39369026));
#298415=CARTESIAN_POINT('Ctrl Pts',(-0.145931087000056,15.2,-10.392617881));
#298416=CARTESIAN_POINT('Ctrl Pts',(-0.145931087000056,11.6,-10.392617881));
#298417=CARTESIAN_POINT('Ctrl Pts',(-0.145804646000055,15.2,-10.39155445));
#298418=CARTESIAN_POINT('Ctrl Pts',(-0.145804646000055,11.6,-10.39155445));
#298419=CARTESIAN_POINT('Ctrl Pts',(-0.145680330000056,15.2,-10.390499995));
#298420=CARTESIAN_POINT('Ctrl Pts',(-0.145680330000056,11.6,-10.390499995));
#298421=CARTESIAN_POINT('Ctrl Pts',(-0.145558126000056,15.2,-10.389454543));
#298422=CARTESIAN_POINT('Ctrl Pts',(-0.145558126000056,11.6,-10.389454543));
#298423=CARTESIAN_POINT('Ctrl Pts',(-0.145438020000055,15.2,-10.388418119));
#298424=CARTESIAN_POINT('Ctrl Pts',(-0.145438020000055,11.6,-10.388418119));
#298425=CARTESIAN_POINT('Ctrl Pts',(-0.145319997000056,15.2,-10.387390753));
#298426=CARTESIAN_POINT('Ctrl Pts',(-0.145319997000056,11.6,-10.387390753));
#298427=CARTESIAN_POINT('Ctrl Pts',(-0.145204042000057,15.2,-10.38637247));
#298428=CARTESIAN_POINT('Ctrl Pts',(-0.145204042000057,11.6,-10.38637247));
#298429=CARTESIAN_POINT('Ctrl Pts',(-0.145090142000056,15.2,-10.3853633));
#298430=CARTESIAN_POINT('Ctrl Pts',(-0.145090142000056,11.6,-10.3853633));
#298431=CARTESIAN_POINT('Ctrl Pts',(-0.144978281000055,15.2,-10.38436327));
#298432=CARTESIAN_POINT('Ctrl Pts',(-0.144978281000055,11.6,-10.38436327));
#298433=CARTESIAN_POINT('Ctrl Pts',(-0.144868446000055,15.2,-10.383372406));
#298434=CARTESIAN_POINT('Ctrl Pts',(-0.144868446000055,11.6,-10.383372406));
#298435=CARTESIAN_POINT('Ctrl Pts',(-0.144760620000056,15.2,-10.382390738));
#298436=CARTESIAN_POINT('Ctrl Pts',(-0.144760620000056,11.6,-10.382390738));
#298437=CARTESIAN_POINT('Ctrl Pts',(-0.144654791000055,15.2,-10.381418293));
#298438=CARTESIAN_POINT('Ctrl Pts',(-0.144654791000055,11.6,-10.381418293));
#298439=CARTESIAN_POINT('Ctrl Pts',(-0.144550942000056,15.2,-10.380455099));
#298440=CARTESIAN_POINT('Ctrl Pts',(-0.144550942000056,11.6,-10.380455099));
#298441=CARTESIAN_POINT('Ctrl Pts',(-0.144449058000056,15.2,-10.379501186));
#298442=CARTESIAN_POINT('Ctrl Pts',(-0.144449058000056,11.6,-10.379501186));
#298443=CARTESIAN_POINT('Ctrl Pts',(-0.144349125000056,15.2,-10.378556581));
#298444=CARTESIAN_POINT('Ctrl Pts',(-0.144349125000056,11.6,-10.378556581));
#298445=CARTESIAN_POINT('Ctrl Pts',(-0.144251127000056,15.2,-10.377621314));
#298446=CARTESIAN_POINT('Ctrl Pts',(-0.144251127000056,11.6,-10.377621314));
#298447=CARTESIAN_POINT('Ctrl Pts',(-0.144155050000055,15.2,-10.376695412));
#298448=CARTESIAN_POINT('Ctrl Pts',(-0.144155050000055,11.6,-10.376695412));
#298449=CARTESIAN_POINT('Ctrl Pts',(-0.144061421000057,15.2,-10.375784183));
#298450=CARTESIAN_POINT('Ctrl Pts',(-0.144061421000057,11.6,-10.375784183));
#298451=CARTESIAN_POINT('Ctrl Pts',(-0.143988114000055,15.2,-10.375063685));
#298452=CARTESIAN_POINT('Ctrl Pts',(-0.143988114000055,11.6,-10.375063685));
#298453=CARTESIAN_POINT('Ctrl Pts',(-0.143934095000056,15.2,-10.374528791));
#298454=CARTESIAN_POINT('Ctrl Pts',(-0.143934095000056,11.6,-10.374528791));
#298455=CARTESIAN_POINT('Ctrl Pts',(-0.143898619000057,15.2,-10.374175764));
#298456=CARTESIAN_POINT('Ctrl Pts',(-0.143898619000057,11.6,-10.374175764));
#298457=CARTESIAN_POINT('Ctrl Pts',(-0.143881228000057,15.2,-10.374002275));
#298458=CARTESIAN_POINT('Ctrl Pts',(-0.143881228000057,11.6,-10.374002275));
#298459=CARTESIAN_POINT('Ctrl Pts',(-0.546958306000055,12.2,-11.486985532));
#298460=CARTESIAN_POINT('Ctrl Pts',(-0.546590899000057,12.2,-11.486315008));
#298461=CARTESIAN_POINT('Ctrl Pts',(-0.545856551000057,12.2,-11.484974209));
#298462=CARTESIAN_POINT('Ctrl Pts',(-0.544756421000056,12.2,-11.482963757));
#298463=CARTESIAN_POINT('Ctrl Pts',(-0.543292369000056,12.2,-11.480284643));
#298464=CARTESIAN_POINT('Ctrl Pts',(-0.541466946000057,12.2,-11.476938237));
#298465=CARTESIAN_POINT('Ctrl Pts',(-0.539646167000055,12.2,-11.473594318));
#298466=CARTESIAN_POINT('Ctrl Pts',(-0.537830030000055,12.2,-11.470252887));
#298467=CARTESIAN_POINT('Ctrl Pts',(-0.536018537000055,12.2,-11.466913949));
#298468=CARTESIAN_POINT('Ctrl Pts',(-0.534211686000056,12.2,-11.46357751));
#298469=CARTESIAN_POINT('Ctrl Pts',(-0.532409474000056,12.2,-11.460243578));
#298470=CARTESIAN_POINT('Ctrl Pts',(-0.530611902000055,12.2,-11.456912162));
#298471=CARTESIAN_POINT('Ctrl Pts',(-0.528818965000056,12.2,-11.453583273));
#298472=CARTESIAN_POINT('Ctrl Pts',(-0.527030665000057,12.2,-11.450256921));
#298473=CARTESIAN_POINT('Ctrl Pts',(-0.525246997000056,12.2,-11.446933118));
#298474=CARTESIAN_POINT('Ctrl Pts',(-0.523467959000056,12.2,-11.443611875));
#298475=CARTESIAN_POINT('Ctrl Pts',(-0.521693552000055,12.2,-11.4402932));
#298476=CARTESIAN_POINT('Ctrl Pts',(-0.519923771000055,12.2,-11.436977103));
#298477=CARTESIAN_POINT('Ctrl Pts',(-0.518158619000056,12.2,-11.433663589));
#298478=CARTESIAN_POINT('Ctrl Pts',(-0.516398090000055,12.2,-11.43035267));
#298479=CARTESIAN_POINT('Ctrl Pts',(-0.514642185000056,12.2,-11.427044351));
#298480=CARTESIAN_POINT('Ctrl Pts',(-0.512890901000055,12.2,-11.423738642));
#298481=CARTESIAN_POINT('Ctrl Pts',(-0.511144239000056,12.2,-11.420435551));
#298482=CARTESIAN_POINT('Ctrl Pts',(-0.509402194000056,12.2,-11.417135088));
#298483=CARTESIAN_POINT('Ctrl Pts',(-0.507664766000057,12.2,-11.413837262));
#298484=CARTESIAN_POINT('Ctrl Pts',(-0.505931954000056,12.2,-11.410542081));
#298485=CARTESIAN_POINT('Ctrl Pts',(-0.504203756000056,12.2,-11.407249556));
#298486=CARTESIAN_POINT('Ctrl Pts',(-0.502480169000057,12.2,-11.403959697));
#298487=CARTESIAN_POINT('Ctrl Pts',(-0.500761192000055,12.2,-11.400672511));
#298488=CARTESIAN_POINT('Ctrl Pts',(-0.499046823000056,12.2,-11.397388008));
#298489=CARTESIAN_POINT('Ctrl Pts',(-0.497337060000056,12.2,-11.394106196));
#298490=CARTESIAN_POINT('Ctrl Pts',(-0.495631904000057,12.2,-11.390827086));
#298491=CARTESIAN_POINT('Ctrl Pts',(-0.493931349000055,12.2,-11.387550685));
#298492=CARTESIAN_POINT('Ctrl Pts',(-0.492235397000057,12.2,-11.384277003));
#298493=CARTESIAN_POINT('Ctrl Pts',(-0.490544043000056,12.2,-11.381006047));
#298494=CARTESIAN_POINT('Ctrl Pts',(-0.488857288000055,12.2,-11.377737829));
#298495=CARTESIAN_POINT('Ctrl Pts',(-0.487175129000056,12.2,-11.374472358));
#298496=CARTESIAN_POINT('Ctrl Pts',(-0.485497564000056,12.2,-11.371209642));
#298497=CARTESIAN_POINT('Ctrl Pts',(-0.483824592000056,12.2,-11.367949691));
#298498=CARTESIAN_POINT('Ctrl Pts',(-0.482156209000056,12.2,-11.364692512));
#298499=CARTESIAN_POINT('Ctrl Pts',(-0.480492416000056,12.2,-11.361438118));
#298500=CARTESIAN_POINT('Ctrl Pts',(-0.478833210000056,12.2,-11.358186515));
#298501=CARTESIAN_POINT('Ctrl Pts',(-0.477178589000056,12.2,-11.354937714));
#298502=CARTESIAN_POINT('Ctrl Pts',(-0.475528552000055,12.2,-11.351691723));
#298503=CARTESIAN_POINT('Ctrl Pts',(-0.473883095000056,12.2,-11.348448553));
#298504=CARTESIAN_POINT('Ctrl Pts',(-0.472242218000056,12.2,-11.345208212));
#298505=CARTESIAN_POINT('Ctrl Pts',(-0.470605918000055,12.2,-11.341970709));
#298506=CARTESIAN_POINT('Ctrl Pts',(-0.468974194000056,12.2,-11.338736054));
#298507=CARTESIAN_POINT('Ctrl Pts',(-0.467347044000055,12.2,-11.335504256));
#298508=CARTESIAN_POINT('Ctrl Pts',(-0.465724466000056,12.2,-11.332275325));
#298509=CARTESIAN_POINT('Ctrl Pts',(-0.464106457000056,12.2,-11.329049269));
#298510=CARTESIAN_POINT('Ctrl Pts',(-0.462493018000056,12.2,-11.325826098));
#298511=CARTESIAN_POINT('Ctrl Pts',(-0.460884143000057,12.2,-11.322605822));
#298512=CARTESIAN_POINT('Ctrl Pts',(-0.459279833000057,12.2,-11.319388451));
#298513=CARTESIAN_POINT('Ctrl Pts',(-0.457680085000056,12.2,-11.316173992));
#298514=CARTESIAN_POINT('Ctrl Pts',(-0.456084896000055,12.2,-11.312962457));
#298515=CARTESIAN_POINT('Ctrl Pts',(-0.454494265000056,12.2,-11.309753853));
#298516=CARTESIAN_POINT('Ctrl Pts',(-0.452908191000055,12.2,-11.306548191));
#298517=CARTESIAN_POINT('Ctrl Pts',(-0.451326671000055,12.2,-11.303345481));
#298518=CARTESIAN_POINT('Ctrl Pts',(-0.449749702000056,12.2,-11.300145731));
#298519=CARTESIAN_POINT('Ctrl Pts',(-0.448177284000056,12.2,-11.296948952));
#298520=CARTESIAN_POINT('Ctrl Pts',(-0.446609414000055,12.2,-11.293755152));
#298521=CARTESIAN_POINT('Ctrl Pts',(-0.445046088000056,12.2,-11.290564341));
#298522=CARTESIAN_POINT('Ctrl Pts',(-0.443487307000057,12.2,-11.287376529));
#298523=CARTESIAN_POINT('Ctrl Pts',(-0.441933068000055,12.2,-11.284191725));
#298524=CARTESIAN_POINT('Ctrl Pts',(-0.440383367000056,12.2,-11.281009939));
#298525=CARTESIAN_POINT('Ctrl Pts',(-0.438838204000056,12.2,-11.277831182));
#298526=CARTESIAN_POINT('Ctrl Pts',(-0.437297576000055,12.2,-11.274655461));
#298527=CARTESIAN_POINT('Ctrl Pts',(-0.435761482000055,12.2,-11.271482787));
#298528=CARTESIAN_POINT('Ctrl Pts',(-0.434229918000056,12.2,-11.268313169));
#298529=CARTESIAN_POINT('Ctrl Pts',(-0.432702884000056,12.2,-11.265146617));
#298530=CARTESIAN_POINT('Ctrl Pts',(-0.431180374000055,12.2,-11.261983141));
#298531=CARTESIAN_POINT('Ctrl Pts',(-0.429662391000055,12.2,-11.258822751));
#298532=CARTESIAN_POINT('Ctrl Pts',(-0.428148929000055,12.2,-11.255665455));
#298533=CARTESIAN_POINT('Ctrl Pts',(-0.426639987000056,12.2,-11.252511265));
#298534=CARTESIAN_POINT('Ctrl Pts',(-0.425135562000056,12.2,-11.249360189));
#298535=CARTESIAN_POINT('Ctrl Pts',(-0.423635654000056,12.2,-11.246212238));
#298536=CARTESIAN_POINT('Ctrl Pts',(-0.422140258000056,12.2,-11.243067421));
#298537=CARTESIAN_POINT('Ctrl Pts',(-0.420649373000056,12.2,-11.239925747));
#298538=CARTESIAN_POINT('Ctrl Pts',(-0.419162997000055,12.2,-11.236787227));
#298539=CARTESIAN_POINT('Ctrl Pts',(-0.417681127000057,12.2,-11.233651872));
#298540=CARTESIAN_POINT('Ctrl Pts',(-0.416203762000055,12.2,-11.230519688));
#298541=CARTESIAN_POINT('Ctrl Pts',(-0.414730899000055,12.2,-11.22739069));
#298542=CARTESIAN_POINT('Ctrl Pts',(-0.413262534000056,12.2,-11.224264883));
#298543=CARTESIAN_POINT('Ctrl Pts',(-0.411798667000056,12.2,-11.221142281));
#298544=CARTESIAN_POINT('Ctrl Pts',(-0.410339295000056,12.2,-11.21802289));
#298545=CARTESIAN_POINT('Ctrl Pts',(-0.408884415000056,12.2,-11.214906723));
#298546=CARTESIAN_POINT('Ctrl Pts',(-0.407434025000055,12.2,-11.211793789));
#298547=CARTESIAN_POINT('Ctrl Pts',(-0.405988122000055,12.2,-11.208684097));
#298548=CARTESIAN_POINT('Ctrl Pts',(-0.404546705000056,12.2,-11.205577658));
#298549=CARTESIAN_POINT('Ctrl Pts',(-0.403109771000055,12.2,-11.202474481));
#298550=CARTESIAN_POINT('Ctrl Pts',(-0.401677318000055,12.2,-11.199374578));
#298551=CARTESIAN_POINT('Ctrl Pts',(-0.400249343000055,12.2,-11.196277957));
#298552=CARTESIAN_POINT('Ctrl Pts',(-0.398825842000056,12.2,-11.193184629));
#298553=CARTESIAN_POINT('Ctrl Pts',(-0.397406814000056,12.2,-11.190094604));
#298554=CARTESIAN_POINT('Ctrl Pts',(-0.395992258000056,12.2,-11.187007892));
#298555=CARTESIAN_POINT('Ctrl Pts',(-0.394582170000056,12.2,-11.183924502));
#298556=CARTESIAN_POINT('Ctrl Pts',(-0.393176547000056,12.2,-11.180844447));
#298557=CARTESIAN_POINT('Ctrl Pts',(-0.391775388000056,12.2,-11.177767733));
#298558=CARTESIAN_POINT('Ctrl Pts',(-0.390378688000055,12.2,-11.174694374));
#298559=CARTESIAN_POINT('Ctrl Pts',(-0.388986447000056,12.2,-11.171624379));
#298560=CARTESIAN_POINT('Ctrl Pts',(-0.387598661000055,12.2,-11.168557756));
#298561=CARTESIAN_POINT('Ctrl Pts',(-0.386215329000056,12.2,-11.165494519));
#298562=CARTESIAN_POINT('Ctrl Pts',(-0.384836446000056,12.2,-11.162434675));
#298563=CARTESIAN_POINT('Ctrl Pts',(-0.383462012000055,12.2,-11.159378235));
#298564=CARTESIAN_POINT('Ctrl Pts',(-0.382092022000055,12.2,-11.156325211));
#298565=CARTESIAN_POINT('Ctrl Pts',(-0.380726475000056,12.2,-11.153275611));
#298566=CARTESIAN_POINT('Ctrl Pts',(-0.379365367000055,12.2,-11.150229445));
#298567=CARTESIAN_POINT('Ctrl Pts',(-0.378008697000055,12.2,-11.147186726));
#298568=CARTESIAN_POINT('Ctrl Pts',(-0.376656462000057,12.2,-11.144147464));
#298569=CARTESIAN_POINT('Ctrl Pts',(-0.375308659000056,12.2,-11.141111667));
#298570=CARTESIAN_POINT('Ctrl Pts',(-0.373965284000055,12.2,-11.138079346));
#298571=CARTESIAN_POINT('Ctrl Pts',(-0.372626336000056,12.2,-11.135050513));
#298572=CARTESIAN_POINT('Ctrl Pts',(-0.371291813000055,12.2,-11.132025177));
#298573=CARTESIAN_POINT('Ctrl Pts',(-0.369961710000055,12.2,-11.129003349));
#298574=CARTESIAN_POINT('Ctrl Pts',(-0.368636025000055,12.2,-11.125985039));
#298575=CARTESIAN_POINT('Ctrl Pts',(-0.367314756000056,12.2,-11.122970257));
#298576=CARTESIAN_POINT('Ctrl Pts',(-0.365997899000057,12.2,-11.119959015));
#298577=CARTESIAN_POINT('Ctrl Pts',(-0.364685453000057,12.2,-11.116951323));
#298578=CARTESIAN_POINT('Ctrl Pts',(-0.363377414000056,12.2,-11.11394719));
#298579=CARTESIAN_POINT('Ctrl Pts',(-0.362073780000056,12.2,-11.110946628));
#298580=CARTESIAN_POINT('Ctrl Pts',(-0.360774547000055,12.2,-11.107949648));
#298581=CARTESIAN_POINT('Ctrl Pts',(-0.359479712000056,12.2,-11.104956259));
#298582=CARTESIAN_POINT('Ctrl Pts',(-0.358189274000056,12.2,-11.101966474));
#298583=CARTESIAN_POINT('Ctrl Pts',(-0.356903229000055,12.2,-11.0989803));
#298584=CARTESIAN_POINT('Ctrl Pts',(-0.355621573000056,12.2,-11.09599775));
#298585=CARTESIAN_POINT('Ctrl Pts',(-0.354344305000056,12.2,-11.093018835));
#298586=CARTESIAN_POINT('Ctrl Pts',(-0.353071422000056,12.2,-11.090043565));
#298587=CARTESIAN_POINT('Ctrl Pts',(-0.351802919000056,12.2,-11.08707195));
#298588=CARTESIAN_POINT('Ctrl Pts',(-0.350538795000055,12.2,-11.084104002));
#298589=CARTESIAN_POINT('Ctrl Pts',(-0.349279047000056,12.2,-11.08113973));
#298590=CARTESIAN_POINT('Ctrl Pts',(-0.348023671000056,12.2,-11.078179147));
#298591=CARTESIAN_POINT('Ctrl Pts',(-0.346772665000056,12.2,-11.075222262));
#298592=CARTESIAN_POINT('Ctrl Pts',(-0.345526025000057,12.2,-11.072269087));
#298593=CARTESIAN_POINT('Ctrl Pts',(-0.344283750000055,12.2,-11.069319632));
#298594=CARTESIAN_POINT('Ctrl Pts',(-0.343045833000056,12.2,-11.066373907));
#298595=CARTESIAN_POINT('Ctrl Pts',(-0.341812276000055,12.2,-11.063431925));
#298596=CARTESIAN_POINT('Ctrl Pts',(-0.340583073000056,12.2,-11.060493695));
#298597=CARTESIAN_POINT('Ctrl Pts',(-0.339358220000056,12.2,-11.057559229));
#298598=CARTESIAN_POINT('Ctrl Pts',(-0.338137716000055,12.2,-11.054628537));
#298599=CARTESIAN_POINT('Ctrl Pts',(-0.336921557000055,12.2,-11.051701631));
#298600=CARTESIAN_POINT('Ctrl Pts',(-0.335709740000055,12.2,-11.048778521));
#298601=CARTESIAN_POINT('Ctrl Pts',(-0.334502263000056,12.2,-11.045859219));
#298602=CARTESIAN_POINT('Ctrl Pts',(-0.333299121000056,12.2,-11.042943735));
#298603=CARTESIAN_POINT('Ctrl Pts',(-0.332100311000056,12.2,-11.040032081));
#298604=CARTESIAN_POINT('Ctrl Pts',(-0.330905831000056,12.2,-11.037124266));
#298605=CARTESIAN_POINT('Ctrl Pts',(-0.329715678000057,12.2,-11.034220304));
#298606=CARTESIAN_POINT('Ctrl Pts',(-0.328529847000055,12.2,-11.031320204));
#298607=CARTESIAN_POINT('Ctrl Pts',(-0.327348336000056,12.2,-11.028423977));
#298608=CARTESIAN_POINT('Ctrl Pts',(-0.326171142000057,12.2,-11.025531635));
#298609=CARTESIAN_POINT('Ctrl Pts',(-0.324998260000056,12.2,-11.022643189));
#298610=CARTESIAN_POINT('Ctrl Pts',(-0.323829689000057,12.2,-11.01975865));
#298611=CARTESIAN_POINT('Ctrl Pts',(-0.322665426000055,12.2,-11.01687803));
#298612=CARTESIAN_POINT('Ctrl Pts',(-0.321505465000056,12.2,-11.014001338));
#298613=CARTESIAN_POINT('Ctrl Pts',(-0.320349803000056,12.2,-11.011128588));
#298614=CARTESIAN_POINT('Ctrl Pts',(-0.319198440000056,12.2,-11.008259788));
#298615=CARTESIAN_POINT('Ctrl Pts',(-0.318051369000055,12.2,-11.005394953));
#298616=CARTESIAN_POINT('Ctrl Pts',(-0.316908589000056,12.2,-11.002534092));
#298617=CARTESIAN_POINT('Ctrl Pts',(-0.315770096000056,12.2,-10.999677217));
#298618=CARTESIAN_POINT('Ctrl Pts',(-0.314635885000056,12.2,-10.996824339));
#298619=CARTESIAN_POINT('Ctrl Pts',(-0.313505954000056,12.2,-10.993975469));
#298620=CARTESIAN_POINT('Ctrl Pts',(-0.312380301000056,12.2,-10.991130619));
#298621=CARTESIAN_POINT('Ctrl Pts',(-0.311258919000055,12.2,-10.988289801));
#298622=CARTESIAN_POINT('Ctrl Pts',(-0.310141808000056,12.2,-10.985453024));
#298623=CARTESIAN_POINT('Ctrl Pts',(-0.309028962000056,12.2,-10.982620303));
#298624=CARTESIAN_POINT('Ctrl Pts',(-0.307920380000055,12.2,-10.979791646));
#298625=CARTESIAN_POINT('Ctrl Pts',(-0.306816056000055,12.2,-10.976967067));
#298626=CARTESIAN_POINT('Ctrl Pts',(-0.305715987000056,12.2,-10.974146576));
#298627=CARTESIAN_POINT('Ctrl Pts',(-0.304620171000056,12.2,-10.971330186));
#298628=CARTESIAN_POINT('Ctrl Pts',(-0.303528603000055,12.2,-10.968517907));
#298629=CARTESIAN_POINT('Ctrl Pts',(-0.302441280000056,12.2,-10.965709752));
#298630=CARTESIAN_POINT('Ctrl Pts',(-0.301358198000056,12.2,-10.962905731));
#298631=CARTESIAN_POINT('Ctrl Pts',(-0.300279354000056,12.2,-10.960105857));
#298632=CARTESIAN_POINT('Ctrl Pts',(-0.299204743000056,12.2,-10.957310141));
#298633=CARTESIAN_POINT('Ctrl Pts',(-0.298134363000055,12.2,-10.954518595));
#298634=CARTESIAN_POINT('Ctrl Pts',(-0.297068210000055,12.2,-10.951731231));
#298635=CARTESIAN_POINT('Ctrl Pts',(-0.296006280000055,12.2,-10.948948059));
#298636=CARTESIAN_POINT('Ctrl Pts',(-0.294948568000055,12.2,-10.946169093));
#298637=CARTESIAN_POINT('Ctrl Pts',(-0.293895073000057,12.2,-10.943394344));
#298638=CARTESIAN_POINT('Ctrl Pts',(-0.292845789000056,12.2,-10.940623823));
#298639=CARTESIAN_POINT('Ctrl Pts',(-0.291800713000056,12.2,-10.937857543));
#298640=CARTESIAN_POINT('Ctrl Pts',(-0.290759842000057,12.2,-10.935095515));
#298641=CARTESIAN_POINT('Ctrl Pts',(-0.289723171000055,12.2,-10.932337751));
#298642=CARTESIAN_POINT('Ctrl Pts',(-0.288690696000057,12.2,-10.929584264));
#298643=CARTESIAN_POINT('Ctrl Pts',(-0.287662415000056,12.2,-10.926835064));
#298644=CARTESIAN_POINT('Ctrl Pts',(-0.286638323000057,12.2,-10.924090164));
#298645=CARTESIAN_POINT('Ctrl Pts',(-0.285618416000055,12.2,-10.921349576));
#298646=CARTESIAN_POINT('Ctrl Pts',(-0.284602690000056,12.2,-10.918613312));
#298647=CARTESIAN_POINT('Ctrl Pts',(-0.283591141000056,12.2,-10.915881383));
#298648=CARTESIAN_POINT('Ctrl Pts',(-0.282583766000055,12.2,-10.913153802));
#298649=CARTESIAN_POINT('Ctrl Pts',(-0.281580560000056,12.2,-10.910430583));
#298650=CARTESIAN_POINT('Ctrl Pts',(-0.280581520000055,12.2,-10.907711734));
#298651=CARTESIAN_POINT('Ctrl Pts',(-0.279586642000057,12.2,-10.904997271));
#298652=CARTESIAN_POINT('Ctrl Pts',(-0.278595921000055,12.2,-10.902287203));
#298653=CARTESIAN_POINT('Ctrl Pts',(-0.277609355000056,12.2,-10.899581544));
#298654=CARTESIAN_POINT('Ctrl Pts',(-0.276626937000056,12.2,-10.896880306));
#298655=CARTESIAN_POINT('Ctrl Pts',(-0.275648666000056,12.2,-10.8941835));
#298656=CARTESIAN_POINT('Ctrl Pts',(-0.274674534000056,12.2,-10.891491141));
#298657=CARTESIAN_POINT('Ctrl Pts',(-0.273704541000056,12.2,-10.888803238));
#298658=CARTESIAN_POINT('Ctrl Pts',(-0.272738681000056,12.2,-10.886119805));
#298659=CARTESIAN_POINT('Ctrl Pts',(-0.271776951000057,12.2,-10.883440854));
#298660=CARTESIAN_POINT('Ctrl Pts',(-0.270819345000056,12.2,-10.880766398));
#298661=CARTESIAN_POINT('Ctrl Pts',(-0.269865860000056,12.2,-10.878096449));
#298662=CARTESIAN_POINT('Ctrl Pts',(-0.268916493000055,12.2,-10.87543102));
#298663=CARTESIAN_POINT('Ctrl Pts',(-0.267971237000056,12.2,-10.872770121));
#298664=CARTESIAN_POINT('Ctrl Pts',(-0.267030089000055,12.2,-10.870113767));
#298665=CARTESIAN_POINT('Ctrl Pts',(-0.266093047000057,12.2,-10.86746197));
#298666=CARTESIAN_POINT('Ctrl Pts',(-0.265160103000056,12.2,-10.864814742));
#298667=CARTESIAN_POINT('Ctrl Pts',(-0.264231255000055,12.2,-10.862172095));
#298668=CARTESIAN_POINT('Ctrl Pts',(-0.263306498000055,12.2,-10.859534042));
#298669=CARTESIAN_POINT('Ctrl Pts',(-0.262385828000056,12.2,-10.856900598));
#298670=CARTESIAN_POINT('Ctrl Pts',(-0.261469242000055,12.2,-10.854271772));
#298671=CARTESIAN_POINT('Ctrl Pts',(-0.260556733000056,12.2,-10.851647578));
#298672=CARTESIAN_POINT('Ctrl Pts',(-0.259648297000057,12.2,-10.84902803));
#298673=CARTESIAN_POINT('Ctrl Pts',(-0.258743931000056,12.2,-10.846413139));
#298674=CARTESIAN_POINT('Ctrl Pts',(-0.257843631000056,12.2,-10.843802918));
#298675=CARTESIAN_POINT('Ctrl Pts',(-0.256947390000055,12.2,-10.84119738));
#298676=CARTESIAN_POINT('Ctrl Pts',(-0.256055206000055,12.2,-10.838596538));
#298677=CARTESIAN_POINT('Ctrl Pts',(-0.255167073000055,12.2,-10.836000406));
#298678=CARTESIAN_POINT('Ctrl Pts',(-0.254282988000056,12.2,-10.833408995));
#298679=CARTESIAN_POINT('Ctrl Pts',(-0.253402945000056,12.2,-10.830822318));
#298680=CARTESIAN_POINT('Ctrl Pts',(-0.252526940000056,12.2,-10.828240388));
#298681=CARTESIAN_POINT('Ctrl Pts',(-0.251654969000056,12.2,-10.825663219));
#298682=CARTESIAN_POINT('Ctrl Pts',(-0.250787027000056,12.2,-10.823090823));
#298683=CARTESIAN_POINT('Ctrl Pts',(-0.249923109000055,12.2,-10.820523213));
#298684=CARTESIAN_POINT('Ctrl Pts',(-0.249063210000056,12.2,-10.817960403));
#298685=CARTESIAN_POINT('Ctrl Pts',(-0.248207327000056,12.2,-10.815402404));
#298686=CARTESIAN_POINT('Ctrl Pts',(-0.247355454000056,12.2,-10.812849232));
#298687=CARTESIAN_POINT('Ctrl Pts',(-0.246507587000057,12.2,-10.810300898));
#298688=CARTESIAN_POINT('Ctrl Pts',(-0.245663721000057,12.2,-10.807757416));
#298689=CARTESIAN_POINT('Ctrl Pts',(-0.244823851000057,12.2,-10.805218799));
#298690=CARTESIAN_POINT('Ctrl Pts',(-0.243987973000056,12.2,-10.80268506));
#298691=CARTESIAN_POINT('Ctrl Pts',(-0.243156080000055,12.2,-10.800156212));
#298692=CARTESIAN_POINT('Ctrl Pts',(-0.242328171000056,12.2,-10.797632269));
#298693=CARTESIAN_POINT('Ctrl Pts',(-0.241504238000055,12.2,-10.795113244));
#298694=CARTESIAN_POINT('Ctrl Pts',(-0.240684278000056,12.2,-10.79259915));
#298695=CARTESIAN_POINT('Ctrl Pts',(-0.239868284000057,12.2,-10.790090001));
#298696=CARTESIAN_POINT('Ctrl Pts',(-0.239056253000056,12.2,-10.78758581));
#298697=CARTESIAN_POINT('Ctrl Pts',(-0.238248181000056,12.2,-10.78508659));
#298698=CARTESIAN_POINT('Ctrl Pts',(-0.237444060000056,12.2,-10.782592355));
#298699=CARTESIAN_POINT('Ctrl Pts',(-0.236643888000057,12.2,-10.780103119));
#298700=CARTESIAN_POINT('Ctrl Pts',(-0.235847657000056,12.2,-10.777618895));
#298701=CARTESIAN_POINT('Ctrl Pts',(-0.235055365000055,12.2,-10.775139696));
#298702=CARTESIAN_POINT('Ctrl Pts',(-0.234267006000056,12.2,-10.772665536));
#298703=CARTESIAN_POINT('Ctrl Pts',(-0.233482574000057,12.2,-10.770196429));
#298704=CARTESIAN_POINT('Ctrl Pts',(-0.232702064000057,12.2,-10.767732388));
#298705=CARTESIAN_POINT('Ctrl Pts',(-0.231925472000055,12.2,-10.765273428));
#298706=CARTESIAN_POINT('Ctrl Pts',(-0.231152793000057,12.2,-10.76281956));
#298707=CARTESIAN_POINT('Ctrl Pts',(-0.230384020000055,12.2,-10.760370801));
#298708=CARTESIAN_POINT('Ctrl Pts',(-0.229619150000057,12.2,-10.757927163));
#298709=CARTESIAN_POINT('Ctrl Pts',(-0.228858176000056,12.2,-10.75548866));
#298710=CARTESIAN_POINT('Ctrl Pts',(-0.228101094000056,12.2,-10.753055307));
#298711=CARTESIAN_POINT('Ctrl Pts',(-0.227347899000057,12.2,-10.750627116));
#298712=CARTESIAN_POINT('Ctrl Pts',(-0.226598585000056,12.2,-10.748204102));
#298713=CARTESIAN_POINT('Ctrl Pts',(-0.225853145000056,12.2,-10.745786278));
#298714=CARTESIAN_POINT('Ctrl Pts',(-0.225111578000057,12.2,-10.743373659));
#298715=CARTESIAN_POINT('Ctrl Pts',(-0.224373875000056,12.2,-10.740966259));
#298716=CARTESIAN_POINT('Ctrl Pts',(-0.223640033000055,12.2,-10.738564091));
#298717=CARTESIAN_POINT('Ctrl Pts',(-0.222910044000055,12.2,-10.736167171));
#298718=CARTESIAN_POINT('Ctrl Pts',(-0.222183905000056,12.2,-10.733775512));
#298719=CARTESIAN_POINT('Ctrl Pts',(-0.221461609000055,12.2,-10.731389127));
#298720=CARTESIAN_POINT('Ctrl Pts',(-0.220743152000056,12.2,-10.729008033));
#298721=CARTESIAN_POINT('Ctrl Pts',(-0.220028527000055,12.2,-10.726632241));
#298722=CARTESIAN_POINT('Ctrl Pts',(-0.219317730000055,12.2,-10.724261768));
#298723=CARTESIAN_POINT('Ctrl Pts',(-0.218610753000055,12.2,-10.721896628));
#298724=CARTESIAN_POINT('Ctrl Pts',(-0.217907594000056,12.2,-10.719536833));
#298725=CARTESIAN_POINT('Ctrl Pts',(-0.217208245000055,12.2,-10.7171824));
#298726=CARTESIAN_POINT('Ctrl Pts',(-0.216373591030381,12.2,-10.7143635293024));
#298727=CARTESIAN_POINT('Ctrl Pts',(-0.215544636984895,12.2,-10.7115527448488));
#298728=CARTESIAN_POINT('Ctrl Pts',(-0.214721369015218,12.2,-10.7087500711512));
#298729=CARTESIAN_POINT('Ctrl Pts',(-0.213903779043993,12.2,-10.7059555439514));
#298730=CARTESIAN_POINT('Ctrl Pts',(-0.213091853000057,12.2,-10.703169187));
#298731=CARTESIAN_POINT('Ctrl Pts',(-0.212419019000055,12.2,-10.700852684));
#298732=CARTESIAN_POINT('Ctrl Pts',(-0.211749948000056,12.2,-10.69854166));
#298733=CARTESIAN_POINT('Ctrl Pts',(-0.211084639000055,12.2,-10.696236127));
#298734=CARTESIAN_POINT('Ctrl Pts',(-0.210423081000056,12.2,-10.693936102));
#298735=CARTESIAN_POINT('Ctrl Pts',(-0.209765271000055,12.2,-10.691641597));
#298736=CARTESIAN_POINT('Ctrl Pts',(-0.209111203000055,12.2,-10.68935263));
#298737=CARTESIAN_POINT('Ctrl Pts',(-0.208460870000057,12.2,-10.687069213));
#298738=CARTESIAN_POINT('Ctrl Pts',(-0.207814267000056,12.2,-10.684791362));
#298739=CARTESIAN_POINT('Ctrl Pts',(-0.207171387000056,12.2,-10.682519093));
#298740=CARTESIAN_POINT('Ctrl Pts',(-0.206532225000055,12.2,-10.68025242));
#298741=CARTESIAN_POINT('Ctrl Pts',(-0.205896774000056,12.2,-10.677991357));
#298742=CARTESIAN_POINT('Ctrl Pts',(-0.205265029000056,12.2,-10.67573592));
#298743=CARTESIAN_POINT('Ctrl Pts',(-0.204636983000055,12.2,-10.673486125));
#298744=CARTESIAN_POINT('Ctrl Pts',(-0.204012631000056,12.2,-10.671241986));
#298745=CARTESIAN_POINT('Ctrl Pts',(-0.203391965000056,12.2,-10.669003519));
#298746=CARTESIAN_POINT('Ctrl Pts',(-0.202774980000056,12.2,-10.666770738));
#298747=CARTESIAN_POINT('Ctrl Pts',(-0.202161670000055,12.2,-10.664543659));
#298748=CARTESIAN_POINT('Ctrl Pts',(-0.201552028000057,12.2,-10.662322297));
#298749=CARTESIAN_POINT('Ctrl Pts',(-0.200946049000056,12.2,-10.660106669));
#298750=CARTESIAN_POINT('Ctrl Pts',(-0.200343725000056,12.2,-10.657896788));
#298751=CARTESIAN_POINT('Ctrl Pts',(-0.199745051000055,12.2,-10.655692671));
#298752=CARTESIAN_POINT('Ctrl Pts',(-0.199150020000056,12.2,-10.653494333));
#298753=CARTESIAN_POINT('Ctrl Pts',(-0.198558626000055,12.2,-10.651301789));
#298754=CARTESIAN_POINT('Ctrl Pts',(-0.197970862000056,12.2,-10.649115056));
#298755=CARTESIAN_POINT('Ctrl Pts',(-0.197386723000056,12.2,-10.646934148));
#298756=CARTESIAN_POINT('Ctrl Pts',(-0.196806201000056,12.2,-10.644759081));
#298757=CARTESIAN_POINT('Ctrl Pts',(-0.196229289000056,12.2,-10.642589871));
#298758=CARTESIAN_POINT('Ctrl Pts',(-0.195655982000057,12.2,-10.640426534));
#298759=CARTESIAN_POINT('Ctrl Pts',(-0.195086274000056,12.2,-10.638269086));
#298760=CARTESIAN_POINT('Ctrl Pts',(-0.194520156000056,12.2,-10.636117541));
#298761=CARTESIAN_POINT('Ctrl Pts',(-0.193957623000056,12.2,-10.633971916));
#298762=CARTESIAN_POINT('Ctrl Pts',(-0.193398667000055,12.2,-10.631832228));
#298763=CARTESIAN_POINT('Ctrl Pts',(-0.192843283000055,12.2,-10.629698492));
#298764=CARTESIAN_POINT('Ctrl Pts',(-0.192291464000055,12.2,-10.627570723));
#298765=CARTESIAN_POINT('Ctrl Pts',(-0.191743203000057,12.2,-10.62544894));
#298766=CARTESIAN_POINT('Ctrl Pts',(-0.191198493000057,12.2,-10.623333156));
#298767=CARTESIAN_POINT('Ctrl Pts',(-0.190657326000055,12.2,-10.621223388));
#298768=CARTESIAN_POINT('Ctrl Pts',(-0.190119697000056,12.2,-10.619119652));
#298769=CARTESIAN_POINT('Ctrl Pts',(-0.189585599000056,12.2,-10.617021965));
#298770=CARTESIAN_POINT('Ctrl Pts',(-0.189055024000057,12.2,-10.614930343));
#298771=CARTESIAN_POINT('Ctrl Pts',(-0.188527965000055,12.2,-10.612844802));
#298772=CARTESIAN_POINT('Ctrl Pts',(-0.188004417000055,12.2,-10.610765359));
#298773=CARTESIAN_POINT('Ctrl Pts',(-0.187484370000056,12.2,-10.60869203));
#298774=CARTESIAN_POINT('Ctrl Pts',(-0.186967820000056,12.2,-10.606624832));
#298775=CARTESIAN_POINT('Ctrl Pts',(-0.186454758000056,12.2,-10.60456378));
#298776=CARTESIAN_POINT('Ctrl Pts',(-0.185945177000055,12.2,-10.602508892));
#298777=CARTESIAN_POINT('Ctrl Pts',(-0.185439071000056,12.2,-10.600460183));
#298778=CARTESIAN_POINT('Ctrl Pts',(-0.184936432000056,12.2,-10.598417672));
#298779=CARTESIAN_POINT('Ctrl Pts',(-0.184437253000055,12.2,-10.596381375));
#298780=CARTESIAN_POINT('Ctrl Pts',(-0.183941526000057,12.2,-10.594351307));
#298781=CARTESIAN_POINT('Ctrl Pts',(-0.183449244000055,12.2,-10.592327487));
#298782=CARTESIAN_POINT('Ctrl Pts',(-0.182960401000055,12.2,-10.59030993));
#298783=CARTESIAN_POINT('Ctrl Pts',(-0.182474988000055,12.2,-10.588298654));
#298784=CARTESIAN_POINT('Ctrl Pts',(-0.181992998000055,12.2,-10.586293676));
#298785=CARTESIAN_POINT('Ctrl Pts',(-0.181514425000057,12.2,-10.584295012));
#298786=CARTESIAN_POINT('Ctrl Pts',(-0.181039260000055,12.2,-10.582302681));
#298787=CARTESIAN_POINT('Ctrl Pts',(-0.180567496000055,12.2,-10.580316698));
#298788=CARTESIAN_POINT('Ctrl Pts',(-0.180099125000056,12.2,-10.578337081));
#298789=CARTESIAN_POINT('Ctrl Pts',(-0.179634139000056,12.2,-10.576363848));
#298790=CARTESIAN_POINT('Ctrl Pts',(-0.179172532000056,12.2,-10.574397014));
#298791=CARTESIAN_POINT('Ctrl Pts',(-0.178714296000055,12.2,-10.572436599));
#298792=CARTESIAN_POINT('Ctrl Pts',(-0.178259423000057,12.2,-10.570482619));
#298793=CARTESIAN_POINT('Ctrl Pts',(-0.177807905000057,12.2,-10.568535092));
#298794=CARTESIAN_POINT('Ctrl Pts',(-0.177359734000057,12.2,-10.566594035));
#298795=CARTESIAN_POINT('Ctrl Pts',(-0.176914903000055,12.2,-10.564659465));
#298796=CARTESIAN_POINT('Ctrl Pts',(-0.176473403000056,12.2,-10.562731399));
#298797=CARTESIAN_POINT('Ctrl Pts',(-0.176035228000057,12.2,-10.560809857));
#298798=CARTESIAN_POINT('Ctrl Pts',(-0.175600369000056,12.2,-10.558894856));
#298799=CARTESIAN_POINT('Ctrl Pts',(-0.175168818000057,12.2,-10.556986413));
#298800=CARTESIAN_POINT('Ctrl Pts',(-0.174740568000056,12.2,-10.555084546));
#298801=CARTESIAN_POINT('Ctrl Pts',(-0.174315609000055,12.2,-10.553189273));
#298802=CARTESIAN_POINT('Ctrl Pts',(-0.173893934000056,12.2,-10.551300611));
#298803=CARTESIAN_POINT('Ctrl Pts',(-0.173475537000056,12.2,-10.549418579));
#298804=CARTESIAN_POINT('Ctrl Pts',(-0.173060406000056,12.2,-10.547543195));
#298805=CARTESIAN_POINT('Ctrl Pts',(-0.172648536000055,12.2,-10.545674477));
#298806=CARTESIAN_POINT('Ctrl Pts',(-0.172239916000055,12.2,-10.543812443));
#298807=CARTESIAN_POINT('Ctrl Pts',(-0.171834541000055,12.2,-10.541957111));
#298808=CARTESIAN_POINT('Ctrl Pts',(-0.171432400000056,12.2,-10.5401085));
#298809=CARTESIAN_POINT('Ctrl Pts',(-0.171033486000055,12.2,-10.538266627));
#298810=CARTESIAN_POINT('Ctrl Pts',(-0.170637791000056,12.2,-10.536431511));
#298811=CARTESIAN_POINT('Ctrl Pts',(-0.170245305000056,12.2,-10.534603171));
#298812=CARTESIAN_POINT('Ctrl Pts',(-0.169856021000055,12.2,-10.532781626));
#298813=CARTESIAN_POINT('Ctrl Pts',(-0.169469930000057,12.2,-10.530966892));
#298814=CARTESIAN_POINT('Ctrl Pts',(-0.169087023000056,12.2,-10.529158991));
#298815=CARTESIAN_POINT('Ctrl Pts',(-0.168707293000055,12.2,-10.527357938));
#298816=CARTESIAN_POINT('Ctrl Pts',(-0.168330729000056,12.2,-10.525563754));
#298817=CARTESIAN_POINT('Ctrl Pts',(-0.167957324000056,12.2,-10.523776458));
#298818=CARTESIAN_POINT('Ctrl Pts',(-0.167587069000056,12.2,-10.521996069));
#298819=CARTESIAN_POINT('Ctrl Pts',(-0.167219956000055,12.2,-10.520222604));
#298820=CARTESIAN_POINT('Ctrl Pts',(-0.166855974000055,12.2,-10.518456084));
#298821=CARTESIAN_POINT('Ctrl Pts',(-0.166495117000055,12.2,-10.516696527));
#298822=CARTESIAN_POINT('Ctrl Pts',(-0.166137374000056,12.2,-10.514943952));
#298823=CARTESIAN_POINT('Ctrl Pts',(-0.165782737000055,12.2,-10.513198378));
#298824=CARTESIAN_POINT('Ctrl Pts',(-0.165431198000056,12.2,-10.511459826));
#298825=CARTESIAN_POINT('Ctrl Pts',(-0.165082744000056,12.2,-10.509728314));
#298826=CARTESIAN_POINT('Ctrl Pts',(-0.164737371000055,12.2,-10.508003862));
#298827=CARTESIAN_POINT('Ctrl Pts',(-0.164395067000056,12.2,-10.506286487));
#298828=CARTESIAN_POINT('Ctrl Pts',(-0.164055824000057,12.2,-10.504576212));
#298829=CARTESIAN_POINT('Ctrl Pts',(-0.163719632000056,12.2,-10.502873055));
#298830=CARTESIAN_POINT('Ctrl Pts',(-0.163386483000056,12.2,-10.501177036));
#298831=CARTESIAN_POINT('Ctrl Pts',(-0.163056366000056,12.2,-10.499488173));
#298832=CARTESIAN_POINT('Ctrl Pts',(-0.162729274000055,12.2,-10.497806488));
#298833=CARTESIAN_POINT('Ctrl Pts',(-0.162405194000056,12.2,-10.496131999));
#298834=CARTESIAN_POINT('Ctrl Pts',(-0.162084120000056,12.2,-10.494464728));
#298835=CARTESIAN_POINT('Ctrl Pts',(-0.161766042000057,12.2,-10.492804693));
#298836=CARTESIAN_POINT('Ctrl Pts',(-0.161450949000056,12.2,-10.491151915));
#298837=CARTESIAN_POINT('Ctrl Pts',(-0.161138833000055,12.2,-10.489506414));
#298838=CARTESIAN_POINT('Ctrl Pts',(-0.160829682000055,12.2,-10.487868211));
#298839=CARTESIAN_POINT('Ctrl Pts',(-0.160523489000056,12.2,-10.486237324));
#298840=CARTESIAN_POINT('Ctrl Pts',(-0.160220245000057,12.2,-10.484613776));
#298841=CARTESIAN_POINT('Ctrl Pts',(-0.159919937000056,12.2,-10.482997586));
#298842=CARTESIAN_POINT('Ctrl Pts',(-0.159622556000055,12.2,-10.481388775));
#298843=CARTESIAN_POINT('Ctrl Pts',(-0.159328094000056,12.2,-10.479787363));
#298844=CARTESIAN_POINT('Ctrl Pts',(-0.159036540000056,12.2,-10.478193371));
#298845=CARTESIAN_POINT('Ctrl Pts',(-0.158747884000056,12.2,-10.476606819));
#298846=CARTESIAN_POINT('Ctrl Pts',(-0.158462117000056,12.2,-10.475027729));
#298847=CARTESIAN_POINT('Ctrl Pts',(-0.158179227000056,12.2,-10.473456121));
#298848=CARTESIAN_POINT('Ctrl Pts',(-0.157899205000056,12.2,-10.471892016));
#298849=CARTESIAN_POINT('Ctrl Pts',(-0.157622041000056,12.2,-10.470335435));
#298850=CARTESIAN_POINT('Ctrl Pts',(-0.157347725000055,12.2,-10.4687864));
#298851=CARTESIAN_POINT('Ctrl Pts',(-0.157076245000055,12.2,-10.467244931));
#298852=CARTESIAN_POINT('Ctrl Pts',(-0.156807594000057,12.2,-10.46571105));
#298853=CARTESIAN_POINT('Ctrl Pts',(-0.156541758000056,12.2,-10.464184778));
#298854=CARTESIAN_POINT('Ctrl Pts',(-0.156278730000056,12.2,-10.462666135));
#298855=CARTESIAN_POINT('Ctrl Pts',(-0.156018496000057,12.2,-10.461155145));
#298856=CARTESIAN_POINT('Ctrl Pts',(-0.155761048000055,12.2,-10.459651829));
#298857=CARTESIAN_POINT('Ctrl Pts',(-0.155506375000056,12.2,-10.458156207));
#298858=CARTESIAN_POINT('Ctrl Pts',(-0.155254466000055,12.2,-10.456668302));
#298859=CARTESIAN_POINT('Ctrl Pts',(-0.155005310000057,12.2,-10.455188136));
#298860=CARTESIAN_POINT('Ctrl Pts',(-0.154758897000056,12.2,-10.45371573));
#298861=CARTESIAN_POINT('Ctrl Pts',(-0.154515216000056,12.2,-10.452251106));
#298862=CARTESIAN_POINT('Ctrl Pts',(-0.154274256000055,12.2,-10.450794288));
#298863=CARTESIAN_POINT('Ctrl Pts',(-0.154036006000055,12.2,-10.449345296));
#298864=CARTESIAN_POINT('Ctrl Pts',(-0.153800456000056,12.2,-10.447904152));
#298865=CARTESIAN_POINT('Ctrl Pts',(-0.153567593000057,12.2,-10.446470879));
#298866=CARTESIAN_POINT('Ctrl Pts',(-0.153337407000055,12.2,-10.4450455));
#298867=CARTESIAN_POINT('Ctrl Pts',(-0.153109888000056,12.2,-10.443628038));
#298868=CARTESIAN_POINT('Ctrl Pts',(-0.152885022000057,12.2,-10.442218514));
#298869=CARTESIAN_POINT('Ctrl Pts',(-0.152662802000056,12.2,-10.440816951));
#298870=CARTESIAN_POINT('Ctrl Pts',(-0.152443212000056,12.2,-10.439423372));
#298871=CARTESIAN_POINT('Ctrl Pts',(-0.152226243000056,12.2,-10.4380378));
#298872=CARTESIAN_POINT('Ctrl Pts',(-0.152011884000055,12.2,-10.436660258));
#298873=CARTESIAN_POINT('Ctrl Pts',(-0.151800122000055,12.2,-10.435290769));
#298874=CARTESIAN_POINT('Ctrl Pts',(-0.151590948000055,12.2,-10.433929354));
#298875=CARTESIAN_POINT('Ctrl Pts',(-0.151384347000055,12.2,-10.43257604));
#298876=CARTESIAN_POINT('Ctrl Pts',(-0.151180310000055,12.2,-10.431230848));
#298877=CARTESIAN_POINT('Ctrl Pts',(-0.150978823000055,12.2,-10.429893802));
#298878=CARTESIAN_POINT('Ctrl Pts',(-0.150779876000057,12.2,-10.428564925));
#298879=CARTESIAN_POINT('Ctrl Pts',(-0.150583457000056,12.2,-10.427244241));
#298880=CARTESIAN_POINT('Ctrl Pts',(-0.150389553000055,12.2,-10.425931773));
#298881=CARTESIAN_POINT('Ctrl Pts',(-0.150198154000056,12.2,-10.424627545));
#298882=CARTESIAN_POINT('Ctrl Pts',(-0.150009246000057,12.2,-10.423331583));
#298883=CARTESIAN_POINT('Ctrl Pts',(-0.149822818000055,12.2,-10.422043907));
#298884=CARTESIAN_POINT('Ctrl Pts',(-0.149638856000056,12.2,-10.420764545));
#298885=CARTESIAN_POINT('Ctrl Pts',(-0.149457350000055,12.2,-10.419493518));
#298886=CARTESIAN_POINT('Ctrl Pts',(-0.149278286000056,12.2,-10.418230852));
#298887=CARTESIAN_POINT('Ctrl Pts',(-0.149101652000055,12.2,-10.416976571));
#298888=CARTESIAN_POINT('Ctrl Pts',(-0.148927437000056,12.2,-10.4157307));
#298889=CARTESIAN_POINT('Ctrl Pts',(-0.148755627000057,12.2,-10.414493262));
#298890=CARTESIAN_POINT('Ctrl Pts',(-0.148586210000056,12.2,-10.413264283));
#298891=CARTESIAN_POINT('Ctrl Pts',(-0.148419173000055,12.2,-10.412043788));
#298892=CARTESIAN_POINT('Ctrl Pts',(-0.148254502000055,12.2,-10.410831802));
#298893=CARTESIAN_POINT('Ctrl Pts',(-0.148092187000056,12.2,-10.409628348));
#298894=CARTESIAN_POINT('Ctrl Pts',(-0.147932214000056,12.2,-10.408433454));
#298895=CARTESIAN_POINT('Ctrl Pts',(-0.147774569000055,12.2,-10.407247142));
#298896=CARTESIAN_POINT('Ctrl Pts',(-0.147619240000055,12.2,-10.40606944));
#298897=CARTESIAN_POINT('Ctrl Pts',(-0.147466215000056,12.2,-10.404900372));
#298898=CARTESIAN_POINT('Ctrl Pts',(-0.147315478000056,12.2,-10.403739965));
#298899=CARTESIAN_POINT('Ctrl Pts',(-0.147167017000056,12.2,-10.402588242));
#298900=CARTESIAN_POINT('Ctrl Pts',(-0.147020820000057,12.2,-10.401445231));
#298901=CARTESIAN_POINT('Ctrl Pts',(-0.146876872000057,12.2,-10.400310957));
#298902=CARTESIAN_POINT('Ctrl Pts',(-0.146735160000055,12.2,-10.399185446));
#298903=CARTESIAN_POINT('Ctrl Pts',(-0.146595671000057,12.2,-10.398068726));
#298904=CARTESIAN_POINT('Ctrl Pts',(-0.146458391000056,12.2,-10.39696082));
#298905=CARTESIAN_POINT('Ctrl Pts',(-0.146323306000056,12.2,-10.395861756));
#298906=CARTESIAN_POINT('Ctrl Pts',(-0.146190404000055,12.2,-10.394771561));
#298907=CARTESIAN_POINT('Ctrl Pts',(-0.146059668000056,12.2,-10.39369026));
#298908=CARTESIAN_POINT('Ctrl Pts',(-0.145931087000056,12.2,-10.392617881));
#298909=CARTESIAN_POINT('Ctrl Pts',(-0.145804646000055,12.2,-10.39155445));
#298910=CARTESIAN_POINT('Ctrl Pts',(-0.145680330000056,12.2,-10.390499995));
#298911=CARTESIAN_POINT('Ctrl Pts',(-0.145558126000056,12.2,-10.389454543));
#298912=CARTESIAN_POINT('Ctrl Pts',(-0.145438020000055,12.2,-10.388418119));
#298913=CARTESIAN_POINT('Ctrl Pts',(-0.145319997000056,12.2,-10.387390753));
#298914=CARTESIAN_POINT('Ctrl Pts',(-0.145204042000057,12.2,-10.38637247));
#298915=CARTESIAN_POINT('Ctrl Pts',(-0.145090142000056,12.2,-10.3853633));
#298916=CARTESIAN_POINT('Ctrl Pts',(-0.144978281000055,12.2,-10.38436327));
#298917=CARTESIAN_POINT('Ctrl Pts',(-0.144868446000055,12.2,-10.383372406));
#298918=CARTESIAN_POINT('Ctrl Pts',(-0.144760620000056,12.2,-10.382390738));
#298919=CARTESIAN_POINT('Ctrl Pts',(-0.144654791000055,12.2,-10.381418293));
#298920=CARTESIAN_POINT('Ctrl Pts',(-0.144550942000056,12.2,-10.380455099));
#298921=CARTESIAN_POINT('Ctrl Pts',(-0.144449058000056,12.2,-10.379501186));
#298922=CARTESIAN_POINT('Ctrl Pts',(-0.144349125000056,12.2,-10.378556581));
#298923=CARTESIAN_POINT('Ctrl Pts',(-0.144251127000056,12.2,-10.377621314));
#298924=CARTESIAN_POINT('Ctrl Pts',(-0.144155050000055,12.2,-10.376695412));
#298925=CARTESIAN_POINT('Ctrl Pts',(-0.144061421000057,12.2,-10.375784183));
#298926=CARTESIAN_POINT('Ctrl Pts',(-0.143988114000055,12.2,-10.375063685));
#298927=CARTESIAN_POINT('Ctrl Pts',(-0.143934095000056,12.2,-10.37452879));
#298928=CARTESIAN_POINT('Ctrl Pts',(-0.143898619000057,12.2,-10.374175763));
#298929=CARTESIAN_POINT('Ctrl Pts',(-0.143881228000057,12.2,-10.374002275));
#298930=CARTESIAN_POINT('Ctrl Pts',(-1.18690176600006,15.2,-10.306885524));
#298931=CARTESIAN_POINT('Ctrl Pts',(-1.18690176600006,11.6,-10.306885524));
#298932=CARTESIAN_POINT('Ctrl Pts',(-1.18690675400006,15.2,-10.307059811));
#298933=CARTESIAN_POINT('Ctrl Pts',(-1.18690675400006,11.6,-10.307059811));
#298934=CARTESIAN_POINT('Ctrl Pts',(-1.18691681600006,15.2,-10.307414474));
#298935=CARTESIAN_POINT('Ctrl Pts',(-1.18691681600006,11.6,-10.307414474));
#298936=CARTESIAN_POINT('Ctrl Pts',(-1.18693179800006,15.2,-10.30795188));
#298937=CARTESIAN_POINT('Ctrl Pts',(-1.18693179800006,11.6,-10.30795188));
#298938=CARTESIAN_POINT('Ctrl Pts',(-1.18695144000006,15.2,-10.30867583));
#298939=CARTESIAN_POINT('Ctrl Pts',(-1.18695144000006,11.6,-10.30867583));
#298940=CARTESIAN_POINT('Ctrl Pts',(-1.18697537100006,15.2,-10.309591544));
#298941=CARTESIAN_POINT('Ctrl Pts',(-1.18697537100006,11.6,-10.309591544));
#298942=CARTESIAN_POINT('Ctrl Pts',(-1.18699875600006,15.2,-10.310522124));
#298943=CARTESIAN_POINT('Ctrl Pts',(-1.18699875600006,11.6,-10.310522124));
#298944=CARTESIAN_POINT('Ctrl Pts',(-1.18702143600006,15.2,-10.311462239));
#298945=CARTESIAN_POINT('Ctrl Pts',(-1.18702143600006,11.6,-10.311462239));
#298946=CARTESIAN_POINT('Ctrl Pts',(-1.18704339300006,15.2,-10.312411861));
#298947=CARTESIAN_POINT('Ctrl Pts',(-1.18704339300006,11.6,-10.312411861));
#298948=CARTESIAN_POINT('Ctrl Pts',(-1.18706461000005,15.2,-10.313370965));
#298949=CARTESIAN_POINT('Ctrl Pts',(-1.18706461000005,11.6,-10.313370965));
#298950=CARTESIAN_POINT('Ctrl Pts',(-1.18708506600006,15.2,-10.314339525));
#298951=CARTESIAN_POINT('Ctrl Pts',(-1.18708506600006,11.6,-10.314339525));
#298952=CARTESIAN_POINT('Ctrl Pts',(-1.18710474400006,15.2,-10.315317513));
#298953=CARTESIAN_POINT('Ctrl Pts',(-1.18710474400006,11.6,-10.315317513));
#298954=CARTESIAN_POINT('Ctrl Pts',(-1.18712362500006,15.2,-10.316304905));
#298955=CARTESIAN_POINT('Ctrl Pts',(-1.18712362500006,11.6,-10.316304905));
#298956=CARTESIAN_POINT('Ctrl Pts',(-1.18714169000006,15.2,-10.317301674));
#298957=CARTESIAN_POINT('Ctrl Pts',(-1.18714169000006,11.6,-10.317301674));
#298958=CARTESIAN_POINT('Ctrl Pts',(-1.18715892200006,15.2,-10.318307793));
#298959=CARTESIAN_POINT('Ctrl Pts',(-1.18715892200006,11.6,-10.318307793));
#298960=CARTESIAN_POINT('Ctrl Pts',(-1.18717530200006,15.2,-10.319323239));
#298961=CARTESIAN_POINT('Ctrl Pts',(-1.18717530200006,11.6,-10.319323239));
#298962=CARTESIAN_POINT('Ctrl Pts',(-1.18719081400006,15.2,-10.320347984));
#298963=CARTESIAN_POINT('Ctrl Pts',(-1.18719081400006,11.6,-10.320347984));
#298964=CARTESIAN_POINT('Ctrl Pts',(-1.18720543700006,15.2,-10.321382005));
#298965=CARTESIAN_POINT('Ctrl Pts',(-1.18720543700006,11.6,-10.321382005));
#298966=CARTESIAN_POINT('Ctrl Pts',(-1.18721915500006,15.2,-10.322425274));
#298967=CARTESIAN_POINT('Ctrl Pts',(-1.18721915500006,11.6,-10.322425274));
#298968=CARTESIAN_POINT('Ctrl Pts',(-1.18723195100006,15.2,-10.323477767));
#298969=CARTESIAN_POINT('Ctrl Pts',(-1.18723195100006,11.6,-10.323477767));
#298970=CARTESIAN_POINT('Ctrl Pts',(-1.18724380600006,15.2,-10.324539459));
#298971=CARTESIAN_POINT('Ctrl Pts',(-1.18724380600006,11.6,-10.324539459));
#298972=CARTESIAN_POINT('Ctrl Pts',(-1.18725470300006,15.2,-10.325610325));
#298973=CARTESIAN_POINT('Ctrl Pts',(-1.18725470300006,11.6,-10.325610325));
#298974=CARTESIAN_POINT('Ctrl Pts',(-1.18726462500006,15.2,-10.326690339));
#298975=CARTESIAN_POINT('Ctrl Pts',(-1.18726462500006,11.6,-10.326690339));
#298976=CARTESIAN_POINT('Ctrl Pts',(-1.18727355500006,15.2,-10.327779477));
#298977=CARTESIAN_POINT('Ctrl Pts',(-1.18727355500006,11.6,-10.327779477));
#298978=CARTESIAN_POINT('Ctrl Pts',(-1.18728147400006,15.2,-10.328877716));
#298979=CARTESIAN_POINT('Ctrl Pts',(-1.18728147400006,11.6,-10.328877716));
#298980=CARTESIAN_POINT('Ctrl Pts',(-1.18728836700006,15.2,-10.329985028));
#298981=CARTESIAN_POINT('Ctrl Pts',(-1.18728836700006,11.6,-10.329985028));
#298982=CARTESIAN_POINT('Ctrl Pts',(-1.18729421500006,15.2,-10.331101391));
#298983=CARTESIAN_POINT('Ctrl Pts',(-1.18729421500006,11.6,-10.331101391));
#298984=CARTESIAN_POINT('Ctrl Pts',(-1.18729900200006,15.2,-10.33222678));
#298985=CARTESIAN_POINT('Ctrl Pts',(-1.18729900200006,11.6,-10.33222678));
#298986=CARTESIAN_POINT('Ctrl Pts',(-1.18730271200006,15.2,-10.333361171));
#298987=CARTESIAN_POINT('Ctrl Pts',(-1.18730271200006,11.6,-10.333361171));
#298988=CARTESIAN_POINT('Ctrl Pts',(-1.18730532700006,15.2,-10.33450454));
#298989=CARTESIAN_POINT('Ctrl Pts',(-1.18730532700006,11.6,-10.33450454));
#298990=CARTESIAN_POINT('Ctrl Pts',(-1.18730683000006,15.2,-10.335656862));
#298991=CARTESIAN_POINT('Ctrl Pts',(-1.18730683000006,11.6,-10.335656862));
#298992=CARTESIAN_POINT('Ctrl Pts',(-1.18730720600006,15.2,-10.336818112));
#298993=CARTESIAN_POINT('Ctrl Pts',(-1.18730720600006,11.6,-10.336818112));
#298994=CARTESIAN_POINT('Ctrl Pts',(-1.18730643800006,15.2,-10.33798827));
#298995=CARTESIAN_POINT('Ctrl Pts',(-1.18730643800006,11.6,-10.33798827));
#298996=CARTESIAN_POINT('Ctrl Pts',(-1.18730450900006,15.2,-10.339167308));
#298997=CARTESIAN_POINT('Ctrl Pts',(-1.18730450900006,11.6,-10.339167308));
#298998=CARTESIAN_POINT('Ctrl Pts',(-1.18730140200006,15.2,-10.340355206));
#298999=CARTESIAN_POINT('Ctrl Pts',(-1.18730140200006,11.6,-10.340355206));
#299000=CARTESIAN_POINT('Ctrl Pts',(-1.18729710300006,15.2,-10.341551938));
#299001=CARTESIAN_POINT('Ctrl Pts',(-1.18729710300006,11.6,-10.341551938));
#299002=CARTESIAN_POINT('Ctrl Pts',(-1.18729159300006,15.2,-10.342757481));
#299003=CARTESIAN_POINT('Ctrl Pts',(-1.18729159300006,11.6,-10.342757481));
#299004=CARTESIAN_POINT('Ctrl Pts',(-1.18728485900006,15.2,-10.343971813));
#299005=CARTESIAN_POINT('Ctrl Pts',(-1.18728485900006,11.6,-10.343971813));
#299006=CARTESIAN_POINT('Ctrl Pts',(-1.18727688300006,15.2,-10.345194909));
#299007=CARTESIAN_POINT('Ctrl Pts',(-1.18727688300006,11.6,-10.345194909));
#299008=CARTESIAN_POINT('Ctrl Pts',(-1.18726765000006,15.2,-10.346426747));
#299009=CARTESIAN_POINT('Ctrl Pts',(-1.18726765000006,11.6,-10.346426747));
#299010=CARTESIAN_POINT('Ctrl Pts',(-1.18725714300006,15.2,-10.347667304));
#299011=CARTESIAN_POINT('Ctrl Pts',(-1.18725714300006,11.6,-10.347667304));
#299012=CARTESIAN_POINT('Ctrl Pts',(-1.18724534800006,15.2,-10.348916556));
#299013=CARTESIAN_POINT('Ctrl Pts',(-1.18724534800006,11.6,-10.348916556));
#299014=CARTESIAN_POINT('Ctrl Pts',(-1.18723224800006,15.2,-10.350174481));
#299015=CARTESIAN_POINT('Ctrl Pts',(-1.18723224800006,11.6,-10.350174481));
#299016=CARTESIAN_POINT('Ctrl Pts',(-1.18721782700006,15.2,-10.351441055));
#299017=CARTESIAN_POINT('Ctrl Pts',(-1.18721782700006,11.6,-10.351441055));
#299018=CARTESIAN_POINT('Ctrl Pts',(-1.18720207100006,15.2,-10.352716257));
#299019=CARTESIAN_POINT('Ctrl Pts',(-1.18720207100006,11.6,-10.352716257));
#299020=CARTESIAN_POINT('Ctrl Pts',(-1.18718496500006,15.2,-10.354000065));
#299021=CARTESIAN_POINT('Ctrl Pts',(-1.18718496500006,11.6,-10.354000065));
#299022=CARTESIAN_POINT('Ctrl Pts',(-1.18716649200006,15.2,-10.355292454));
#299023=CARTESIAN_POINT('Ctrl Pts',(-1.18716649200006,11.6,-10.355292454));
#299024=CARTESIAN_POINT('Ctrl Pts',(-1.18714663700006,15.2,-10.356593403));
#299025=CARTESIAN_POINT('Ctrl Pts',(-1.18714663700006,11.6,-10.356593403));
#299026=CARTESIAN_POINT('Ctrl Pts',(-1.18712538600006,15.2,-10.35790289));
#299027=CARTESIAN_POINT('Ctrl Pts',(-1.18712538600006,11.6,-10.35790289));
#299028=CARTESIAN_POINT('Ctrl Pts',(-1.18710272200006,15.2,-10.359220891));
#299029=CARTESIAN_POINT('Ctrl Pts',(-1.18710272200006,11.6,-10.359220891));
#299030=CARTESIAN_POINT('Ctrl Pts',(-1.18707863200005,15.2,-10.360547387));
#299031=CARTESIAN_POINT('Ctrl Pts',(-1.18707863200005,11.6,-10.360547387));
#299032=CARTESIAN_POINT('Ctrl Pts',(-1.18705310000006,15.2,-10.361882353));
#299033=CARTESIAN_POINT('Ctrl Pts',(-1.18705310000006,11.6,-10.361882353));
#299034=CARTESIAN_POINT('Ctrl Pts',(-1.18702611100006,15.2,-10.363225769));
#299035=CARTESIAN_POINT('Ctrl Pts',(-1.18702611100006,11.6,-10.363225769));
#299036=CARTESIAN_POINT('Ctrl Pts',(-1.18699765000006,15.2,-10.364577611));
#299037=CARTESIAN_POINT('Ctrl Pts',(-1.18699765000006,11.6,-10.364577611));
#299038=CARTESIAN_POINT('Ctrl Pts',(-1.18696770400006,15.2,-10.36593786));
#299039=CARTESIAN_POINT('Ctrl Pts',(-1.18696770400006,11.6,-10.36593786));
#299040=CARTESIAN_POINT('Ctrl Pts',(-1.18693625600006,15.2,-10.367306493));
#299041=CARTESIAN_POINT('Ctrl Pts',(-1.18693625600006,11.6,-10.367306493));
#299042=CARTESIAN_POINT('Ctrl Pts',(-1.18690329400006,15.2,-10.368683487));
#299043=CARTESIAN_POINT('Ctrl Pts',(-1.18690329400006,11.6,-10.368683487));
#299044=CARTESIAN_POINT('Ctrl Pts',(-1.18686880100006,15.2,-10.370068823));
#299045=CARTESIAN_POINT('Ctrl Pts',(-1.18686880100006,11.6,-10.370068823));
#299046=CARTESIAN_POINT('Ctrl Pts',(-1.18683276400006,15.2,-10.371462478));
#299047=CARTESIAN_POINT('Ctrl Pts',(-1.18683276400006,11.6,-10.371462478));
#299048=CARTESIAN_POINT('Ctrl Pts',(-1.18679516800006,15.2,-10.372864431));
#299049=CARTESIAN_POINT('Ctrl Pts',(-1.18679516800006,11.6,-10.372864431));
#299050=CARTESIAN_POINT('Ctrl Pts',(-1.18675600000006,15.2,-10.374274661));
#299051=CARTESIAN_POINT('Ctrl Pts',(-1.18675600000006,11.6,-10.374274661));
#299052=CARTESIAN_POINT('Ctrl Pts',(-1.18671524400006,15.2,-10.375693145));
#299053=CARTESIAN_POINT('Ctrl Pts',(-1.18671524400006,11.6,-10.375693145));
#299054=CARTESIAN_POINT('Ctrl Pts',(-1.18667288600006,15.2,-10.377119865));
#299055=CARTESIAN_POINT('Ctrl Pts',(-1.18667288600006,11.6,-10.377119865));
#299056=CARTESIAN_POINT('Ctrl Pts',(-1.18662891500006,15.2,-10.378554798));
#299057=CARTESIAN_POINT('Ctrl Pts',(-1.18662891500006,11.6,-10.378554798));
#299058=CARTESIAN_POINT('Ctrl Pts',(-1.18658331200006,15.2,-10.379997923));
#299059=CARTESIAN_POINT('Ctrl Pts',(-1.18658331200006,11.6,-10.379997923));
#299060=CARTESIAN_POINT('Ctrl Pts',(-1.18653606700006,15.2,-10.38144922));
#299061=CARTESIAN_POINT('Ctrl Pts',(-1.18653606700006,11.6,-10.38144922));
#299062=CARTESIAN_POINT('Ctrl Pts',(-1.18648716500006,15.2,-10.382908667));
#299063=CARTESIAN_POINT('Ctrl Pts',(-1.18648716500006,11.6,-10.382908667));
#299064=CARTESIAN_POINT('Ctrl Pts',(-1.18643659200006,15.2,-10.384376245));
#299065=CARTESIAN_POINT('Ctrl Pts',(-1.18643659200006,11.6,-10.384376245));
#299066=CARTESIAN_POINT('Ctrl Pts',(-1.18638433400006,15.2,-10.385851932));
#299067=CARTESIAN_POINT('Ctrl Pts',(-1.18638433400006,11.6,-10.385851932));
#299068=CARTESIAN_POINT('Ctrl Pts',(-1.18633037700006,15.2,-10.387335708));
#299069=CARTESIAN_POINT('Ctrl Pts',(-1.18633037700006,11.6,-10.387335708));
#299070=CARTESIAN_POINT('Ctrl Pts',(-1.18627470900006,15.2,-10.388827552));
#299071=CARTESIAN_POINT('Ctrl Pts',(-1.18627470900006,11.6,-10.388827552));
#299072=CARTESIAN_POINT('Ctrl Pts',(-1.18621731600006,15.2,-10.390327444));
#299073=CARTESIAN_POINT('Ctrl Pts',(-1.18621731600006,11.6,-10.390327444));
#299074=CARTESIAN_POINT('Ctrl Pts',(-1.18615818400006,15.2,-10.391835365));
#299075=CARTESIAN_POINT('Ctrl Pts',(-1.18615818400006,11.6,-10.391835365));
#299076=CARTESIAN_POINT('Ctrl Pts',(-1.18609729900006,15.2,-10.393351292));
#299077=CARTESIAN_POINT('Ctrl Pts',(-1.18609729900006,11.6,-10.393351292));
#299078=CARTESIAN_POINT('Ctrl Pts',(-1.18603464900006,15.2,-10.394875206));
#299079=CARTESIAN_POINT('Ctrl Pts',(-1.18603464900006,11.6,-10.394875206));
#299080=CARTESIAN_POINT('Ctrl Pts',(-1.18597022000006,15.2,-10.396407088));
#299081=CARTESIAN_POINT('Ctrl Pts',(-1.18597022000006,11.6,-10.396407088));
#299082=CARTESIAN_POINT('Ctrl Pts',(-1.18590399800006,15.2,-10.397946917));
#299083=CARTESIAN_POINT('Ctrl Pts',(-1.18590399800006,11.6,-10.397946917));
#299084=CARTESIAN_POINT('Ctrl Pts',(-1.18583597200006,15.2,-10.399494673));
#299085=CARTESIAN_POINT('Ctrl Pts',(-1.18583597200006,11.6,-10.399494673));
#299086=CARTESIAN_POINT('Ctrl Pts',(-1.18576612800006,15.2,-10.401050335));
#299087=CARTESIAN_POINT('Ctrl Pts',(-1.18576612800006,11.6,-10.401050335));
#299088=CARTESIAN_POINT('Ctrl Pts',(-1.18569445200006,15.2,-10.402613886));
#299089=CARTESIAN_POINT('Ctrl Pts',(-1.18569445200006,11.6,-10.402613886));
#299090=CARTESIAN_POINT('Ctrl Pts',(-1.18562093200006,15.2,-10.404185304));
#299091=CARTESIAN_POINT('Ctrl Pts',(-1.18562093200006,11.6,-10.404185304));
#299092=CARTESIAN_POINT('Ctrl Pts',(-1.18554555500006,15.2,-10.40576457));
#299093=CARTESIAN_POINT('Ctrl Pts',(-1.18554555500006,11.6,-10.40576457));
#299094=CARTESIAN_POINT('Ctrl Pts',(-1.18546830800006,15.2,-10.407351665));
#299095=CARTESIAN_POINT('Ctrl Pts',(-1.18546830800006,11.6,-10.407351665));
#299096=CARTESIAN_POINT('Ctrl Pts',(-1.18538917800006,15.2,-10.408946568));
#299097=CARTESIAN_POINT('Ctrl Pts',(-1.18538917800006,11.6,-10.408946568));
#299098=CARTESIAN_POINT('Ctrl Pts',(-1.18530815300006,15.2,-10.410549261));
#299099=CARTESIAN_POINT('Ctrl Pts',(-1.18530815300006,11.6,-10.410549261));
#299100=CARTESIAN_POINT('Ctrl Pts',(-1.18522522000006,15.2,-10.412159724));
#299101=CARTESIAN_POINT('Ctrl Pts',(-1.18522522000006,11.6,-10.412159724));
#299102=CARTESIAN_POINT('Ctrl Pts',(-1.18514036600006,15.2,-10.413777937));
#299103=CARTESIAN_POINT('Ctrl Pts',(-1.18514036600006,11.6,-10.413777937));
#299104=CARTESIAN_POINT('Ctrl Pts',(-1.18505357900006,15.2,-10.415403882));
#299105=CARTESIAN_POINT('Ctrl Pts',(-1.18505357900006,11.6,-10.415403882));
#299106=CARTESIAN_POINT('Ctrl Pts',(-1.18496484700006,15.2,-10.417037539));
#299107=CARTESIAN_POINT('Ctrl Pts',(-1.18496484700006,11.6,-10.417037539));
#299108=CARTESIAN_POINT('Ctrl Pts',(-1.18487415700006,15.2,-10.418678889));
#299109=CARTESIAN_POINT('Ctrl Pts',(-1.18487415700006,11.6,-10.418678889));
#299110=CARTESIAN_POINT('Ctrl Pts',(-1.18478149700006,15.2,-10.420327913));
#299111=CARTESIAN_POINT('Ctrl Pts',(-1.18478149700006,11.6,-10.420327913));
#299112=CARTESIAN_POINT('Ctrl Pts',(-1.18468685300006,15.2,-10.421984593));
#299113=CARTESIAN_POINT('Ctrl Pts',(-1.18468685300006,11.6,-10.421984593));
#299114=CARTESIAN_POINT('Ctrl Pts',(-1.18459021600006,15.2,-10.423648908));
#299115=CARTESIAN_POINT('Ctrl Pts',(-1.18459021600006,11.6,-10.423648908));
#299116=CARTESIAN_POINT('Ctrl Pts',(-1.18449157100006,15.2,-10.425320841));
#299117=CARTESIAN_POINT('Ctrl Pts',(-1.18449157100006,11.6,-10.425320841));
#299118=CARTESIAN_POINT('Ctrl Pts',(-1.18439090700006,15.2,-10.427000372));
#299119=CARTESIAN_POINT('Ctrl Pts',(-1.18439090700006,11.6,-10.427000372));
#299120=CARTESIAN_POINT('Ctrl Pts',(-1.18428821200006,15.2,-10.428687482));
#299121=CARTESIAN_POINT('Ctrl Pts',(-1.18428821200006,11.6,-10.428687482));
#299122=CARTESIAN_POINT('Ctrl Pts',(-1.18418347300006,15.2,-10.430382155));
#299123=CARTESIAN_POINT('Ctrl Pts',(-1.18418347300006,11.6,-10.430382155));
#299124=CARTESIAN_POINT('Ctrl Pts',(-1.18407668100006,15.2,-10.432084369));
#299125=CARTESIAN_POINT('Ctrl Pts',(-1.18407668100006,11.6,-10.432084369));
#299126=CARTESIAN_POINT('Ctrl Pts',(-1.18396782000006,15.2,-10.433794107));
#299127=CARTESIAN_POINT('Ctrl Pts',(-1.18396782000006,11.6,-10.433794107));
#299128=CARTESIAN_POINT('Ctrl Pts',(-1.18385688100005,15.2,-10.435511351));
#299129=CARTESIAN_POINT('Ctrl Pts',(-1.18385688100005,11.6,-10.435511351));
#299130=CARTESIAN_POINT('Ctrl Pts',(-1.18374385200006,15.2,-10.437236082));
#299131=CARTESIAN_POINT('Ctrl Pts',(-1.18374385200006,11.6,-10.437236082));
#299132=CARTESIAN_POINT('Ctrl Pts',(-1.18362872000006,15.2,-10.438968281));
#299133=CARTESIAN_POINT('Ctrl Pts',(-1.18362872000006,11.6,-10.438968281));
#299134=CARTESIAN_POINT('Ctrl Pts',(-1.18351147300006,15.2,-10.440707931));
#299135=CARTESIAN_POINT('Ctrl Pts',(-1.18351147300006,11.6,-10.440707931));
#299136=CARTESIAN_POINT('Ctrl Pts',(-1.18339210200006,15.2,-10.442455012));
#299137=CARTESIAN_POINT('Ctrl Pts',(-1.18339210200006,11.6,-10.442455012));
#299138=CARTESIAN_POINT('Ctrl Pts',(-1.18327059400006,15.2,-10.444209508));
#299139=CARTESIAN_POINT('Ctrl Pts',(-1.18327059400006,11.6,-10.444209508));
#299140=CARTESIAN_POINT('Ctrl Pts',(-1.18314693700006,15.2,-10.4459714));
#299141=CARTESIAN_POINT('Ctrl Pts',(-1.18314693700006,11.6,-10.4459714));
#299142=CARTESIAN_POINT('Ctrl Pts',(-1.18302111900006,15.2,-10.44774067));
#299143=CARTESIAN_POINT('Ctrl Pts',(-1.18302111900006,11.6,-10.44774067));
#299144=CARTESIAN_POINT('Ctrl Pts',(-1.18289313000006,15.2,-10.449517299));
#299145=CARTESIAN_POINT('Ctrl Pts',(-1.18289313000006,11.6,-10.449517299));
#299146=CARTESIAN_POINT('Ctrl Pts',(-1.18276295900006,15.2,-10.45130127));
#299147=CARTESIAN_POINT('Ctrl Pts',(-1.18276295900006,11.6,-10.45130127));
#299148=CARTESIAN_POINT('Ctrl Pts',(-1.18263059300006,15.2,-10.453092566));
#299149=CARTESIAN_POINT('Ctrl Pts',(-1.18263059300006,11.6,-10.453092566));
#299150=CARTESIAN_POINT('Ctrl Pts',(-1.18249602200006,15.2,-10.454891167));
#299151=CARTESIAN_POINT('Ctrl Pts',(-1.18249602200006,11.6,-10.454891167));
#299152=CARTESIAN_POINT('Ctrl Pts',(-1.18235923500006,15.2,-10.456697057));
#299153=CARTESIAN_POINT('Ctrl Pts',(-1.18235923500006,11.6,-10.456697057));
#299154=CARTESIAN_POINT('Ctrl Pts',(-1.18222021900006,15.2,-10.458510217));
#299155=CARTESIAN_POINT('Ctrl Pts',(-1.18222021900006,11.6,-10.458510217));
#299156=CARTESIAN_POINT('Ctrl Pts',(-1.18207896500006,15.2,-10.460330631));
#299157=CARTESIAN_POINT('Ctrl Pts',(-1.18207896500006,11.6,-10.460330631));
#299158=CARTESIAN_POINT('Ctrl Pts',(-1.18193546100006,15.2,-10.46215828));
#299159=CARTESIAN_POINT('Ctrl Pts',(-1.18193546100006,11.6,-10.46215828));
#299160=CARTESIAN_POINT('Ctrl Pts',(-1.18178969600006,15.2,-10.463993146));
#299161=CARTESIAN_POINT('Ctrl Pts',(-1.18178969600006,11.6,-10.463993146));
#299162=CARTESIAN_POINT('Ctrl Pts',(-1.18164165900006,15.2,-10.465835214));
#299163=CARTESIAN_POINT('Ctrl Pts',(-1.18164165900006,11.6,-10.465835214));
#299164=CARTESIAN_POINT('Ctrl Pts',(-1.18149134000006,15.2,-10.467684464));
#299165=CARTESIAN_POINT('Ctrl Pts',(-1.18149134000006,11.6,-10.467684464));
#299166=CARTESIAN_POINT('Ctrl Pts',(-1.18133872600006,15.2,-10.469540881));
#299167=CARTESIAN_POINT('Ctrl Pts',(-1.18133872600006,11.6,-10.469540881));
#299168=CARTESIAN_POINT('Ctrl Pts',(-1.18118380900005,15.2,-10.471404445));
#299169=CARTESIAN_POINT('Ctrl Pts',(-1.18118380900005,11.6,-10.471404445));
#299170=CARTESIAN_POINT('Ctrl Pts',(-1.18102657700006,15.2,-10.473275141));
#299171=CARTESIAN_POINT('Ctrl Pts',(-1.18102657700006,11.6,-10.473275141));
#299172=CARTESIAN_POINT('Ctrl Pts',(-1.18086701900006,15.2,-10.475152951));
#299173=CARTESIAN_POINT('Ctrl Pts',(-1.18086701900006,11.6,-10.475152951));
#299174=CARTESIAN_POINT('Ctrl Pts',(-1.18070512400006,15.2,-10.477037856));
#299175=CARTESIAN_POINT('Ctrl Pts',(-1.18070512400006,11.6,-10.477037856));
#299176=CARTESIAN_POINT('Ctrl Pts',(-1.18054088200006,15.2,-10.478929842));
#299177=CARTESIAN_POINT('Ctrl Pts',(-1.18054088200006,11.6,-10.478929842));
#299178=CARTESIAN_POINT('Ctrl Pts',(-1.18037428300006,15.2,-10.480828891));
#299179=CARTESIAN_POINT('Ctrl Pts',(-1.18037428300006,11.6,-10.480828891));
#299180=CARTESIAN_POINT('Ctrl Pts',(-1.18020531600005,15.2,-10.482734985));
#299181=CARTESIAN_POINT('Ctrl Pts',(-1.18020531600005,11.6,-10.482734985));
#299182=CARTESIAN_POINT('Ctrl Pts',(-1.18003397000006,15.2,-10.484648109));
#299183=CARTESIAN_POINT('Ctrl Pts',(-1.18003397000006,11.6,-10.484648109));
#299184=CARTESIAN_POINT('Ctrl Pts',(-1.17986023500006,15.2,-10.486568243));
#299185=CARTESIAN_POINT('Ctrl Pts',(-1.17986023500006,11.6,-10.486568243));
#299186=CARTESIAN_POINT('Ctrl Pts',(-1.17968410100006,15.2,-10.488495373));
#299187=CARTESIAN_POINT('Ctrl Pts',(-1.17968410100006,11.6,-10.488495373));
#299188=CARTESIAN_POINT('Ctrl Pts',(-1.17950555800006,15.2,-10.49042948));
#299189=CARTESIAN_POINT('Ctrl Pts',(-1.17950555800006,11.6,-10.49042948));
#299190=CARTESIAN_POINT('Ctrl Pts',(-1.17932459300006,15.2,-10.49237055));
#299191=CARTESIAN_POINT('Ctrl Pts',(-1.17932459300006,11.6,-10.49237055));
#299192=CARTESIAN_POINT('Ctrl Pts',(-1.17914120000005,15.2,-10.494318563));
#299193=CARTESIAN_POINT('Ctrl Pts',(-1.17914120000005,11.6,-10.494318563));
#299194=CARTESIAN_POINT('Ctrl Pts',(-1.17895536600006,15.2,-10.496273505));
#299195=CARTESIAN_POINT('Ctrl Pts',(-1.17895536600006,11.6,-10.496273505));
#299196=CARTESIAN_POINT('Ctrl Pts',(-1.17876708000006,15.2,-10.498235359));
#299197=CARTESIAN_POINT('Ctrl Pts',(-1.17876708000006,11.6,-10.498235359));
#299198=CARTESIAN_POINT('Ctrl Pts',(-1.17857633500006,15.2,-10.500204108));
#299199=CARTESIAN_POINT('Ctrl Pts',(-1.17857633500006,11.6,-10.500204108));
#299200=CARTESIAN_POINT('Ctrl Pts',(-1.17838312000006,15.2,-10.502179735));
#299201=CARTESIAN_POINT('Ctrl Pts',(-1.17838312000006,11.6,-10.502179735));
#299202=CARTESIAN_POINT('Ctrl Pts',(-1.17818742300006,15.2,-10.504162225));
#299203=CARTESIAN_POINT('Ctrl Pts',(-1.17818742300006,11.6,-10.504162225));
#299204=CARTESIAN_POINT('Ctrl Pts',(-1.17798923600006,15.2,-10.506151559));
#299205=CARTESIAN_POINT('Ctrl Pts',(-1.17798923600006,11.6,-10.506151559));
#299206=CARTESIAN_POINT('Ctrl Pts',(-1.17778854800005,15.2,-10.508147723));
#299207=CARTESIAN_POINT('Ctrl Pts',(-1.17778854800005,11.6,-10.508147723));
#299208=CARTESIAN_POINT('Ctrl Pts',(-1.17758535000006,15.2,-10.510150702));
#299209=CARTESIAN_POINT('Ctrl Pts',(-1.17758535000006,11.6,-10.510150702));
#299210=CARTESIAN_POINT('Ctrl Pts',(-1.17737963100006,15.2,-10.512160476));
#299211=CARTESIAN_POINT('Ctrl Pts',(-1.17737963100006,11.6,-10.512160476));
#299212=CARTESIAN_POINT('Ctrl Pts',(-1.17717138300006,15.2,-10.514177031));
#299213=CARTESIAN_POINT('Ctrl Pts',(-1.17717138300006,11.6,-10.514177031));
#299214=CARTESIAN_POINT('Ctrl Pts',(-1.17696059500006,15.2,-10.51620035));
#299215=CARTESIAN_POINT('Ctrl Pts',(-1.17696059500006,11.6,-10.51620035));
#299216=CARTESIAN_POINT('Ctrl Pts',(-1.17674725700006,15.2,-10.518230419));
#299217=CARTESIAN_POINT('Ctrl Pts',(-1.17674725700006,11.6,-10.518230419));
#299218=CARTESIAN_POINT('Ctrl Pts',(-1.17653136000005,15.2,-10.520267219));
#299219=CARTESIAN_POINT('Ctrl Pts',(-1.17653136000005,11.6,-10.520267219));
#299220=CARTESIAN_POINT('Ctrl Pts',(-1.17631289500006,15.2,-10.522310736));
#299221=CARTESIAN_POINT('Ctrl Pts',(-1.17631289500006,11.6,-10.522310736));
#299222=CARTESIAN_POINT('Ctrl Pts',(-1.17609185100006,15.2,-10.524360953));
#299223=CARTESIAN_POINT('Ctrl Pts',(-1.17609185100006,11.6,-10.524360953));
#299224=CARTESIAN_POINT('Ctrl Pts',(-1.17586821800006,15.2,-10.526417854));
#299225=CARTESIAN_POINT('Ctrl Pts',(-1.17586821800006,11.6,-10.526417854));
#299226=CARTESIAN_POINT('Ctrl Pts',(-1.17564198900006,15.2,-10.528481425));
#299227=CARTESIAN_POINT('Ctrl Pts',(-1.17564198900006,11.6,-10.528481425));
#299228=CARTESIAN_POINT('Ctrl Pts',(-1.17541315400006,15.2,-10.530551648));
#299229=CARTESIAN_POINT('Ctrl Pts',(-1.17541315400006,11.6,-10.530551648));
#299230=CARTESIAN_POINT('Ctrl Pts',(-1.17518170100006,15.2,-10.532628509));
#299231=CARTESIAN_POINT('Ctrl Pts',(-1.17518170100006,11.6,-10.532628509));
#299232=CARTESIAN_POINT('Ctrl Pts',(-1.17494762300006,15.2,-10.534711991));
#299233=CARTESIAN_POINT('Ctrl Pts',(-1.17494762300006,11.6,-10.534711991));
#299234=CARTESIAN_POINT('Ctrl Pts',(-1.17471091000006,15.2,-10.536802078));
#299235=CARTESIAN_POINT('Ctrl Pts',(-1.17471091000006,11.6,-10.536802078));
#299236=CARTESIAN_POINT('Ctrl Pts',(-1.17447155200006,15.2,-10.538898756));
#299237=CARTESIAN_POINT('Ctrl Pts',(-1.17447155200006,11.6,-10.538898756));
#299238=CARTESIAN_POINT('Ctrl Pts',(-1.17422954200006,15.2,-10.541002007));
#299239=CARTESIAN_POINT('Ctrl Pts',(-1.17422954200006,11.6,-10.541002007));
#299240=CARTESIAN_POINT('Ctrl Pts',(-1.17398486900006,15.2,-10.543111818));
#299241=CARTESIAN_POINT('Ctrl Pts',(-1.17398486900006,11.6,-10.543111818));
#299242=CARTESIAN_POINT('Ctrl Pts',(-1.17373752300006,15.2,-10.545228173));
#299243=CARTESIAN_POINT('Ctrl Pts',(-1.17373752300006,11.6,-10.545228173));
#299244=CARTESIAN_POINT('Ctrl Pts',(-1.17348749700006,15.2,-10.547351055));
#299245=CARTESIAN_POINT('Ctrl Pts',(-1.17348749700006,11.6,-10.547351055));
#299246=CARTESIAN_POINT('Ctrl Pts',(-1.17323478100006,15.2,-10.549480449));
#299247=CARTESIAN_POINT('Ctrl Pts',(-1.17323478100006,11.6,-10.549480449));
#299248=CARTESIAN_POINT('Ctrl Pts',(-1.17297936500006,15.2,-10.551616341));
#299249=CARTESIAN_POINT('Ctrl Pts',(-1.17297936500006,11.6,-10.551616341));
#299250=CARTESIAN_POINT('Ctrl Pts',(-1.17272124100006,15.2,-10.553758714));
#299251=CARTESIAN_POINT('Ctrl Pts',(-1.17272124100006,11.6,-10.553758714));
#299252=CARTESIAN_POINT('Ctrl Pts',(-1.17246040000005,15.2,-10.555907555));
#299253=CARTESIAN_POINT('Ctrl Pts',(-1.17246040000005,11.6,-10.555907555));
#299254=CARTESIAN_POINT('Ctrl Pts',(-1.17219683200006,15.2,-10.558062846));
#299255=CARTESIAN_POINT('Ctrl Pts',(-1.17219683200006,11.6,-10.558062846));
#299256=CARTESIAN_POINT('Ctrl Pts',(-1.17193053000006,15.2,-10.560224572));
#299257=CARTESIAN_POINT('Ctrl Pts',(-1.17193053000006,11.6,-10.560224572));
#299258=CARTESIAN_POINT('Ctrl Pts',(-1.17166148400006,15.2,-10.562392721));
#299259=CARTESIAN_POINT('Ctrl Pts',(-1.17166148400006,11.6,-10.562392721));
#299260=CARTESIAN_POINT('Ctrl Pts',(-1.17138968600006,15.2,-10.564567275));
#299261=CARTESIAN_POINT('Ctrl Pts',(-1.17138968600006,11.6,-10.564567275));
#299262=CARTESIAN_POINT('Ctrl Pts',(-1.17111512500006,15.2,-10.56674822));
#299263=CARTESIAN_POINT('Ctrl Pts',(-1.17111512500006,11.6,-10.56674822));
#299264=CARTESIAN_POINT('Ctrl Pts',(-1.17083779500006,15.2,-10.568935539));
#299265=CARTESIAN_POINT('Ctrl Pts',(-1.17083779500006,11.6,-10.568935539));
#299266=CARTESIAN_POINT('Ctrl Pts',(-1.17055768500006,15.2,-10.57112922));
#299267=CARTESIAN_POINT('Ctrl Pts',(-1.17055768500006,11.6,-10.57112922));
#299268=CARTESIAN_POINT('Ctrl Pts',(-1.17027478800006,15.2,-10.573329247));
#299269=CARTESIAN_POINT('Ctrl Pts',(-1.17027478800006,11.6,-10.573329247));
#299270=CARTESIAN_POINT('Ctrl Pts',(-1.16998909400006,15.2,-10.575535603));
#299271=CARTESIAN_POINT('Ctrl Pts',(-1.16998909400006,11.6,-10.575535603));
#299272=CARTESIAN_POINT('Ctrl Pts',(-1.16970059600006,15.2,-10.577748277));
#299273=CARTESIAN_POINT('Ctrl Pts',(-1.16970059600006,11.6,-10.577748277));
#299274=CARTESIAN_POINT('Ctrl Pts',(-1.16940928400005,15.2,-10.57996725));
#299275=CARTESIAN_POINT('Ctrl Pts',(-1.16940928400005,11.6,-10.57996725));
#299276=CARTESIAN_POINT('Ctrl Pts',(-1.16911514900006,15.2,-10.582192511));
#299277=CARTESIAN_POINT('Ctrl Pts',(-1.16911514900006,11.6,-10.582192511));
#299278=CARTESIAN_POINT('Ctrl Pts',(-1.16881818600006,15.2,-10.584424042));
#299279=CARTESIAN_POINT('Ctrl Pts',(-1.16881818600006,11.6,-10.584424042));
#299280=CARTESIAN_POINT('Ctrl Pts',(-1.16851838200006,15.2,-10.586661831));
#299281=CARTESIAN_POINT('Ctrl Pts',(-1.16851838200006,11.6,-10.586661831));
#299282=CARTESIAN_POINT('Ctrl Pts',(-1.16821573100006,15.2,-10.588905861));
#299283=CARTESIAN_POINT('Ctrl Pts',(-1.16821573100006,11.6,-10.588905861));
#299284=CARTESIAN_POINT('Ctrl Pts',(-1.16791022400006,15.2,-10.591156119));
#299285=CARTESIAN_POINT('Ctrl Pts',(-1.16791022400006,11.6,-10.591156119));
#299286=CARTESIAN_POINT('Ctrl Pts',(-1.16760185300006,15.2,-10.59341259));
#299287=CARTESIAN_POINT('Ctrl Pts',(-1.16760185300006,11.6,-10.59341259));
#299288=CARTESIAN_POINT('Ctrl Pts',(-1.16729061000005,15.2,-10.595675259));
#299289=CARTESIAN_POINT('Ctrl Pts',(-1.16729061000005,11.6,-10.595675259));
#299290=CARTESIAN_POINT('Ctrl Pts',(-1.16697648600006,15.2,-10.597944112));
#299291=CARTESIAN_POINT('Ctrl Pts',(-1.16697648600006,11.6,-10.597944112));
#299292=CARTESIAN_POINT('Ctrl Pts',(-1.16665947300006,15.2,-10.600219134));
#299293=CARTESIAN_POINT('Ctrl Pts',(-1.16665947300006,11.6,-10.600219134));
#299294=CARTESIAN_POINT('Ctrl Pts',(-1.16633956300006,15.2,-10.60250031));
#299295=CARTESIAN_POINT('Ctrl Pts',(-1.16633956300006,11.6,-10.60250031));
#299296=CARTESIAN_POINT('Ctrl Pts',(-1.16601674700005,15.2,-10.604787626));
#299297=CARTESIAN_POINT('Ctrl Pts',(-1.16601674700005,11.6,-10.604787626));
#299298=CARTESIAN_POINT('Ctrl Pts',(-1.16569101800006,15.2,-10.60708107));
#299299=CARTESIAN_POINT('Ctrl Pts',(-1.16569101800006,11.6,-10.60708107));
#299300=CARTESIAN_POINT('Ctrl Pts',(-1.16536236700005,15.2,-10.609380624));
#299301=CARTESIAN_POINT('Ctrl Pts',(-1.16536236700005,11.6,-10.609380624));
#299302=CARTESIAN_POINT('Ctrl Pts',(-1.16503078700006,15.2,-10.611686275));
#299303=CARTESIAN_POINT('Ctrl Pts',(-1.16503078700006,11.6,-10.611686275));
#299304=CARTESIAN_POINT('Ctrl Pts',(-1.16469626800005,15.2,-10.613998011));
#299305=CARTESIAN_POINT('Ctrl Pts',(-1.16469626800005,11.6,-10.613998011));
#299306=CARTESIAN_POINT('Ctrl Pts',(-1.16435880400006,15.2,-10.616315814));
#299307=CARTESIAN_POINT('Ctrl Pts',(-1.16435880400006,11.6,-10.616315814));
#299308=CARTESIAN_POINT('Ctrl Pts',(-1.16401838400006,15.2,-10.618639673));
#299309=CARTESIAN_POINT('Ctrl Pts',(-1.16401838400006,11.6,-10.618639673));
#299310=CARTESIAN_POINT('Ctrl Pts',(-1.16367500500006,15.2,-10.620969571));
#299311=CARTESIAN_POINT('Ctrl Pts',(-1.16367500500006,11.6,-10.620969571));
#299312=CARTESIAN_POINT('Ctrl Pts',(-1.16332865500006,15.2,-10.623305496));
#299313=CARTESIAN_POINT('Ctrl Pts',(-1.16332865500006,11.6,-10.623305496));
#299314=CARTESIAN_POINT('Ctrl Pts',(-1.16297932800006,15.2,-10.625647433));
#299315=CARTESIAN_POINT('Ctrl Pts',(-1.16297932800006,11.6,-10.625647433));
#299316=CARTESIAN_POINT('Ctrl Pts',(-1.16262701500006,15.2,-10.627995369));
#299317=CARTESIAN_POINT('Ctrl Pts',(-1.16262701500006,11.6,-10.627995369));
#299318=CARTESIAN_POINT('Ctrl Pts',(-1.16227171000006,15.2,-10.630349288));
#299319=CARTESIAN_POINT('Ctrl Pts',(-1.16227171000006,11.6,-10.630349288));
#299320=CARTESIAN_POINT('Ctrl Pts',(-1.16191340300006,15.2,-10.632709178));
#299321=CARTESIAN_POINT('Ctrl Pts',(-1.16191340300006,11.6,-10.632709178));
#299322=CARTESIAN_POINT('Ctrl Pts',(-1.16155208700006,15.2,-10.635075024));
#299323=CARTESIAN_POINT('Ctrl Pts',(-1.16155208700006,11.6,-10.635075024));
#299324=CARTESIAN_POINT('Ctrl Pts',(-1.16118775500005,15.2,-10.637446813));
#299325=CARTESIAN_POINT('Ctrl Pts',(-1.16118775500005,11.6,-10.637446813));
#299326=CARTESIAN_POINT('Ctrl Pts',(-1.16082039900006,15.2,-10.639824529));
#299327=CARTESIAN_POINT('Ctrl Pts',(-1.16082039900006,11.6,-10.639824529));
#299328=CARTESIAN_POINT('Ctrl Pts',(-1.16045001000006,15.2,-10.642208161));
#299329=CARTESIAN_POINT('Ctrl Pts',(-1.16045001000006,11.6,-10.642208161));
#299330=CARTESIAN_POINT('Ctrl Pts',(-1.16007658300005,15.2,-10.644597692));
#299331=CARTESIAN_POINT('Ctrl Pts',(-1.16007658300005,11.6,-10.644597692));
#299332=CARTESIAN_POINT('Ctrl Pts',(-1.15970010900006,15.2,-10.646993112));
#299333=CARTESIAN_POINT('Ctrl Pts',(-1.15970010900006,11.6,-10.646993112));
#299334=CARTESIAN_POINT('Ctrl Pts',(-1.15932057900006,15.2,-10.649394405));
#299335=CARTESIAN_POINT('Ctrl Pts',(-1.15932057900006,11.6,-10.649394405));
#299336=CARTESIAN_POINT('Ctrl Pts',(-1.15893798800006,15.2,-10.651801557));
#299337=CARTESIAN_POINT('Ctrl Pts',(-1.15893798800006,11.6,-10.651801557));
#299338=CARTESIAN_POINT('Ctrl Pts',(-1.15855232700006,15.2,-10.654214555));
#299339=CARTESIAN_POINT('Ctrl Pts',(-1.15855232700006,11.6,-10.654214555));
#299340=CARTESIAN_POINT('Ctrl Pts',(-1.15816358800006,15.2,-10.656633385));
#299341=CARTESIAN_POINT('Ctrl Pts',(-1.15816358800006,11.6,-10.656633385));
#299342=CARTESIAN_POINT('Ctrl Pts',(-1.15777176600006,15.2,-10.659058034));
#299343=CARTESIAN_POINT('Ctrl Pts',(-1.15777176600006,11.6,-10.659058034));
#299344=CARTESIAN_POINT('Ctrl Pts',(-1.15737685100005,15.2,-10.661488487));
#299345=CARTESIAN_POINT('Ctrl Pts',(-1.15737685100005,11.6,-10.661488487));
#299346=CARTESIAN_POINT('Ctrl Pts',(-1.15697883700006,15.2,-10.663924733));
#299347=CARTESIAN_POINT('Ctrl Pts',(-1.15697883700006,11.6,-10.663924733));
#299348=CARTESIAN_POINT('Ctrl Pts',(-1.15657771600006,15.2,-10.666366757));
#299349=CARTESIAN_POINT('Ctrl Pts',(-1.15657771600006,11.6,-10.666366757));
#299350=CARTESIAN_POINT('Ctrl Pts',(-1.15617348100006,15.2,-10.668814545));
#299351=CARTESIAN_POINT('Ctrl Pts',(-1.15617348100006,11.6,-10.668814545));
#299352=CARTESIAN_POINT('Ctrl Pts',(-1.15576612400006,15.2,-10.671268084));
#299353=CARTESIAN_POINT('Ctrl Pts',(-1.15576612400006,11.6,-10.671268084));
#299354=CARTESIAN_POINT('Ctrl Pts',(-1.15535564000006,15.2,-10.673727361));
#299355=CARTESIAN_POINT('Ctrl Pts',(-1.15535564000006,11.6,-10.673727361));
#299356=CARTESIAN_POINT('Ctrl Pts',(-1.15494201900006,15.2,-10.676192362));
#299357=CARTESIAN_POINT('Ctrl Pts',(-1.15494201900006,11.6,-10.676192362));
#299358=CARTESIAN_POINT('Ctrl Pts',(-1.15452525600006,15.2,-10.678663073));
#299359=CARTESIAN_POINT('Ctrl Pts',(-1.15452525600006,11.6,-10.678663073));
#299360=CARTESIAN_POINT('Ctrl Pts',(-1.15410534200006,15.2,-10.681139483));
#299361=CARTESIAN_POINT('Ctrl Pts',(-1.15410534200006,11.6,-10.681139483));
#299362=CARTESIAN_POINT('Ctrl Pts',(-1.15368227000006,15.2,-10.683621578));
#299363=CARTESIAN_POINT('Ctrl Pts',(-1.15368227000006,11.6,-10.683621578));
#299364=CARTESIAN_POINT('Ctrl Pts',(-1.15325603400006,15.2,-10.686109343));
#299365=CARTESIAN_POINT('Ctrl Pts',(-1.15325603400006,11.6,-10.686109343));
#299366=CARTESIAN_POINT('Ctrl Pts',(-1.15282662700006,15.2,-10.688602766));
#299367=CARTESIAN_POINT('Ctrl Pts',(-1.15282662700006,11.6,-10.688602766));
#299368=CARTESIAN_POINT('Ctrl Pts',(-1.15239404100006,15.2,-10.691101834));
#299369=CARTESIAN_POINT('Ctrl Pts',(-1.15239404100006,11.6,-10.691101834));
#299370=CARTESIAN_POINT('Ctrl Pts',(-1.15195826900006,15.2,-10.693606533));
#299371=CARTESIAN_POINT('Ctrl Pts',(-1.15195826900006,11.6,-10.693606533));
#299372=CARTESIAN_POINT('Ctrl Pts',(-1.15151930500006,15.2,-10.69611685));
#299373=CARTESIAN_POINT('Ctrl Pts',(-1.15151930500006,11.6,-10.69611685));
#299374=CARTESIAN_POINT('Ctrl Pts',(-1.15107714100006,15.2,-10.698632773));
#299375=CARTESIAN_POINT('Ctrl Pts',(-1.15107714100006,11.6,-10.698632773));
#299376=CARTESIAN_POINT('Ctrl Pts',(-1.15063177100006,15.2,-10.701154289));
#299377=CARTESIAN_POINT('Ctrl Pts',(-1.15063177100006,11.6,-10.701154289));
#299378=CARTESIAN_POINT('Ctrl Pts',(-1.15018318700006,15.2,-10.703681383));
#299379=CARTESIAN_POINT('Ctrl Pts',(-1.15018318700006,11.6,-10.703681383));
#299380=CARTESIAN_POINT('Ctrl Pts',(-1.14973138200006,15.2,-10.706214044));
#299381=CARTESIAN_POINT('Ctrl Pts',(-1.14973138200006,11.6,-10.706214044));
#299382=CARTESIAN_POINT('Ctrl Pts',(-1.14927635100006,15.2,-10.708752257));
#299383=CARTESIAN_POINT('Ctrl Pts',(-1.14927635100006,11.6,-10.708752257));
#299384=CARTESIAN_POINT('Ctrl Pts',(-1.14881808500006,15.2,-10.711296011));
#299385=CARTESIAN_POINT('Ctrl Pts',(-1.14881808500006,11.6,-10.711296011));
#299386=CARTESIAN_POINT('Ctrl Pts',(-1.14835657800006,15.2,-10.713845292));
#299387=CARTESIAN_POINT('Ctrl Pts',(-1.14835657800006,11.6,-10.713845292));
#299388=CARTESIAN_POINT('Ctrl Pts',(-1.14789182500005,15.2,-10.716400088));
#299389=CARTESIAN_POINT('Ctrl Pts',(-1.14789182500005,11.6,-10.716400088));
#299390=CARTESIAN_POINT('Ctrl Pts',(-1.14742381600006,15.2,-10.718960385));
#299391=CARTESIAN_POINT('Ctrl Pts',(-1.14742381600006,11.6,-10.718960385));
#299392=CARTESIAN_POINT('Ctrl Pts',(-1.14695254600006,15.2,-10.721526171));
#299393=CARTESIAN_POINT('Ctrl Pts',(-1.14695254600006,11.6,-10.721526171));
#299394=CARTESIAN_POINT('Ctrl Pts',(-1.14647800900006,15.2,-10.724097433));
#299395=CARTESIAN_POINT('Ctrl Pts',(-1.14647800900006,11.6,-10.724097433));
#299396=CARTESIAN_POINT('Ctrl Pts',(-1.14600019700006,15.2,-10.726674158));
#299397=CARTESIAN_POINT('Ctrl Pts',(-1.14600019700006,11.6,-10.726674158));
#299398=CARTESIAN_POINT('Ctrl Pts',(-1.14551910300006,15.2,-10.729256334));
#299399=CARTESIAN_POINT('Ctrl Pts',(-1.14551910300006,11.6,-10.729256334));
#299400=CARTESIAN_POINT('Ctrl Pts',(-1.14503472200005,15.2,-10.731843947));
#299401=CARTESIAN_POINT('Ctrl Pts',(-1.14503472200005,11.6,-10.731843947));
#299402=CARTESIAN_POINT('Ctrl Pts',(-1.14454704700006,15.2,-10.734436985));
#299403=CARTESIAN_POINT('Ctrl Pts',(-1.14454704700006,11.6,-10.734436985));
#299404=CARTESIAN_POINT('Ctrl Pts',(-1.14405607000006,15.2,-10.737035436));
#299405=CARTESIAN_POINT('Ctrl Pts',(-1.14405607000006,11.6,-10.737035436));
#299406=CARTESIAN_POINT('Ctrl Pts',(-1.14356178700006,15.2,-10.739639287));
#299407=CARTESIAN_POINT('Ctrl Pts',(-1.14356178700006,11.6,-10.739639287));
#299408=CARTESIAN_POINT('Ctrl Pts',(-1.14306419000005,15.2,-10.742248524));
#299409=CARTESIAN_POINT('Ctrl Pts',(-1.14306419000005,11.6,-10.742248524));
#299410=CARTESIAN_POINT('Ctrl Pts',(-1.14256327100006,15.2,-10.744863136));
#299411=CARTESIAN_POINT('Ctrl Pts',(-1.14256327100006,11.6,-10.744863136));
#299412=CARTESIAN_POINT('Ctrl Pts',(-1.14205902600006,15.2,-10.74748311));
#299413=CARTESIAN_POINT('Ctrl Pts',(-1.14205902600006,11.6,-10.74748311));
#299414=CARTESIAN_POINT('Ctrl Pts',(-1.14155144800006,15.2,-10.750108433));
#299415=CARTESIAN_POINT('Ctrl Pts',(-1.14155144800006,11.6,-10.750108433));
#299416=CARTESIAN_POINT('Ctrl Pts',(-1.14104053000006,15.2,-10.752739094));
#299417=CARTESIAN_POINT('Ctrl Pts',(-1.14104053000006,11.6,-10.752739094));
#299418=CARTESIAN_POINT('Ctrl Pts',(-1.14052626500006,15.2,-10.755375079));
#299419=CARTESIAN_POINT('Ctrl Pts',(-1.14052626500006,11.6,-10.755375079));
#299420=CARTESIAN_POINT('Ctrl Pts',(-1.14000864800005,15.2,-10.758016376));
#299421=CARTESIAN_POINT('Ctrl Pts',(-1.14000864800005,11.6,-10.758016376));
#299422=CARTESIAN_POINT('Ctrl Pts',(-1.13948767300006,15.2,-10.760662972));
#299423=CARTESIAN_POINT('Ctrl Pts',(-1.13948767300006,11.6,-10.760662972));
#299424=CARTESIAN_POINT('Ctrl Pts',(-1.13896333200006,15.2,-10.763314856));
#299425=CARTESIAN_POINT('Ctrl Pts',(-1.13896333200006,11.6,-10.763314856));
#299426=CARTESIAN_POINT('Ctrl Pts',(-1.13843562000006,15.2,-10.765972015));
#299427=CARTESIAN_POINT('Ctrl Pts',(-1.13843562000006,11.6,-10.765972015));
#299428=CARTESIAN_POINT('Ctrl Pts',(-1.13790453000005,15.2,-10.768634436));
#299429=CARTESIAN_POINT('Ctrl Pts',(-1.13790453000005,11.6,-10.768634436));
#299430=CARTESIAN_POINT('Ctrl Pts',(-1.13737005500006,15.2,-10.771302109));
#299431=CARTESIAN_POINT('Ctrl Pts',(-1.13737005500006,11.6,-10.771302109));
#299432=CARTESIAN_POINT('Ctrl Pts',(-1.13683219200006,15.2,-10.773975018));
#299433=CARTESIAN_POINT('Ctrl Pts',(-1.13683219200006,11.6,-10.773975018));
#299434=CARTESIAN_POINT('Ctrl Pts',(-1.13629093200006,15.2,-10.776653154));
#299435=CARTESIAN_POINT('Ctrl Pts',(-1.13629093200006,11.6,-10.776653154));
#299436=CARTESIAN_POINT('Ctrl Pts',(-1.13574626900006,15.2,-10.779336503));
#299437=CARTESIAN_POINT('Ctrl Pts',(-1.13574626900006,11.6,-10.779336503));
#299438=CARTESIAN_POINT('Ctrl Pts',(-1.13519819700006,15.2,-10.782025053));
#299439=CARTESIAN_POINT('Ctrl Pts',(-1.13519819700006,11.6,-10.782025053));
#299440=CARTESIAN_POINT('Ctrl Pts',(-1.13464671100005,15.2,-10.784718793));
#299441=CARTESIAN_POINT('Ctrl Pts',(-1.13464671100005,11.6,-10.784718793));
#299442=CARTESIAN_POINT('Ctrl Pts',(-1.13409180400006,15.2,-10.78741771));
#299443=CARTESIAN_POINT('Ctrl Pts',(-1.13409180400006,11.6,-10.78741771));
#299444=CARTESIAN_POINT('Ctrl Pts',(-1.13353347000006,15.2,-10.790121791));
#299445=CARTESIAN_POINT('Ctrl Pts',(-1.13353347000006,11.6,-10.790121791));
#299446=CARTESIAN_POINT('Ctrl Pts',(-1.13297170400006,15.2,-10.792831026));
#299447=CARTESIAN_POINT('Ctrl Pts',(-1.13297170400006,11.6,-10.792831026));
#299448=CARTESIAN_POINT('Ctrl Pts',(-1.13240649900006,15.2,-10.795545401));
#299449=CARTESIAN_POINT('Ctrl Pts',(-1.13240649900006,11.6,-10.795545401));
#299450=CARTESIAN_POINT('Ctrl Pts',(-1.13183784800006,15.2,-10.798264905));
#299451=CARTESIAN_POINT('Ctrl Pts',(-1.13183784800006,11.6,-10.798264905));
#299452=CARTESIAN_POINT('Ctrl Pts',(-1.13126574700006,15.2,-10.800989525));
#299453=CARTESIAN_POINT('Ctrl Pts',(-1.13126574700006,11.6,-10.800989525));
#299454=CARTESIAN_POINT('Ctrl Pts',(-1.13069018800006,15.2,-10.803719251));
#299455=CARTESIAN_POINT('Ctrl Pts',(-1.13069018800006,11.6,-10.803719251));
#299456=CARTESIAN_POINT('Ctrl Pts',(-1.13011116700006,15.2,-10.806454068));
#299457=CARTESIAN_POINT('Ctrl Pts',(-1.13011116700006,11.6,-10.806454068));
#299458=CARTESIAN_POINT('Ctrl Pts',(-1.12952867800006,15.2,-10.809193966));
#299459=CARTESIAN_POINT('Ctrl Pts',(-1.12952867800006,11.6,-10.809193966));
#299460=CARTESIAN_POINT('Ctrl Pts',(-1.12894271500006,15.2,-10.811938934));
#299461=CARTESIAN_POINT('Ctrl Pts',(-1.12894271500006,11.6,-10.811938934));
#299462=CARTESIAN_POINT('Ctrl Pts',(-1.12835327000006,15.2,-10.814688959));
#299463=CARTESIAN_POINT('Ctrl Pts',(-1.12835327000006,11.6,-10.814688959));
#299464=CARTESIAN_POINT('Ctrl Pts',(-1.12776033900006,15.2,-10.817444029));
#299465=CARTESIAN_POINT('Ctrl Pts',(-1.12776033900006,11.6,-10.817444029));
#299466=CARTESIAN_POINT('Ctrl Pts',(-1.12716391600006,15.2,-10.820204131));
#299467=CARTESIAN_POINT('Ctrl Pts',(-1.12716391600006,11.6,-10.820204131));
#299468=CARTESIAN_POINT('Ctrl Pts',(-1.12656399600006,15.2,-10.822969255));
#299469=CARTESIAN_POINT('Ctrl Pts',(-1.12656399600006,11.6,-10.822969255));
#299470=CARTESIAN_POINT('Ctrl Pts',(-1.12596057300006,15.2,-10.82573939));
#299471=CARTESIAN_POINT('Ctrl Pts',(-1.12596057300006,11.6,-10.82573939));
#299472=CARTESIAN_POINT('Ctrl Pts',(-1.12535363900006,15.2,-10.828514521));
#299473=CARTESIAN_POINT('Ctrl Pts',(-1.12535363900006,11.6,-10.828514521));
#299474=CARTESIAN_POINT('Ctrl Pts',(-1.12474319100005,15.2,-10.831294639));
#299475=CARTESIAN_POINT('Ctrl Pts',(-1.12474319100005,11.6,-10.831294639));
#299476=CARTESIAN_POINT('Ctrl Pts',(-1.12412922300006,15.2,-10.834079731));
#299477=CARTESIAN_POINT('Ctrl Pts',(-1.12412922300006,11.6,-10.834079731));
#299478=CARTESIAN_POINT('Ctrl Pts',(-1.12351172700005,15.2,-10.836869786));
#299479=CARTESIAN_POINT('Ctrl Pts',(-1.12351172700005,11.6,-10.836869786));
#299480=CARTESIAN_POINT('Ctrl Pts',(-1.12289070100006,15.2,-10.839664792));
#299481=CARTESIAN_POINT('Ctrl Pts',(-1.12289070100006,11.6,-10.839664792));
#299482=CARTESIAN_POINT('Ctrl Pts',(-1.12226613600006,15.2,-10.842464738));
#299483=CARTESIAN_POINT('Ctrl Pts',(-1.12226613600006,11.6,-10.842464738));
#299484=CARTESIAN_POINT('Ctrl Pts',(-1.12163802800006,15.2,-10.845269611));
#299485=CARTESIAN_POINT('Ctrl Pts',(-1.12163802800006,11.6,-10.845269611));
#299486=CARTESIAN_POINT('Ctrl Pts',(-1.12100637100006,15.2,-10.848079399));
#299487=CARTESIAN_POINT('Ctrl Pts',(-1.12100637100006,11.6,-10.848079399));
#299488=CARTESIAN_POINT('Ctrl Pts',(-1.12037116000006,15.2,-10.850894093));
#299489=CARTESIAN_POINT('Ctrl Pts',(-1.12037116000006,11.6,-10.850894093));
#299490=CARTESIAN_POINT('Ctrl Pts',(-1.11973239000006,15.2,-10.85371368));
#299491=CARTESIAN_POINT('Ctrl Pts',(-1.11973239000006,11.6,-10.85371368));
#299492=CARTESIAN_POINT('Ctrl Pts',(-1.11909005400006,15.2,-10.856538148));
#299493=CARTESIAN_POINT('Ctrl Pts',(-1.11909005400006,11.6,-10.856538148));
#299494=CARTESIAN_POINT('Ctrl Pts',(-1.11844414600006,15.2,-10.859367486));
#299495=CARTESIAN_POINT('Ctrl Pts',(-1.11844414600006,11.6,-10.859367486));
#299496=CARTESIAN_POINT('Ctrl Pts',(-1.11779466300006,15.2,-10.862201683));
#299497=CARTESIAN_POINT('Ctrl Pts',(-1.11779466300006,11.6,-10.862201683));
#299498=CARTESIAN_POINT('Ctrl Pts',(-1.11714159900006,15.2,-10.865040726));
#299499=CARTESIAN_POINT('Ctrl Pts',(-1.11714159900006,11.6,-10.865040726));
#299500=CARTESIAN_POINT('Ctrl Pts',(-1.11648494600006,15.2,-10.867884606));
#299501=CARTESIAN_POINT('Ctrl Pts',(-1.11648494600006,11.6,-10.867884606));
#299502=CARTESIAN_POINT('Ctrl Pts',(-1.11582470100006,15.2,-10.870733309));
#299503=CARTESIAN_POINT('Ctrl Pts',(-1.11582470100006,11.6,-10.870733309));
#299504=CARTESIAN_POINT('Ctrl Pts',(-1.11516085700006,15.2,-10.873586825));
#299505=CARTESIAN_POINT('Ctrl Pts',(-1.11516085700006,11.6,-10.873586825));
#299506=CARTESIAN_POINT('Ctrl Pts',(-1.11449341200006,15.2,-10.876445142));
#299507=CARTESIAN_POINT('Ctrl Pts',(-1.11449341200006,11.6,-10.876445142));
#299508=CARTESIAN_POINT('Ctrl Pts',(-1.11382235600006,15.2,-10.87930825));
#299509=CARTESIAN_POINT('Ctrl Pts',(-1.11382235600006,11.6,-10.87930825));
#299510=CARTESIAN_POINT('Ctrl Pts',(-1.11314768700006,15.2,-10.882176135));
#299511=CARTESIAN_POINT('Ctrl Pts',(-1.11314768700006,11.6,-10.882176135));
#299512=CARTESIAN_POINT('Ctrl Pts',(-1.11246939900006,15.2,-10.885048789));
#299513=CARTESIAN_POINT('Ctrl Pts',(-1.11246939900006,11.6,-10.885048789));
#299514=CARTESIAN_POINT('Ctrl Pts',(-1.11178748600006,15.2,-10.887926198));
#299515=CARTESIAN_POINT('Ctrl Pts',(-1.11178748600006,11.6,-10.887926198));
#299516=CARTESIAN_POINT('Ctrl Pts',(-1.11110194300006,15.2,-10.890808352));
#299517=CARTESIAN_POINT('Ctrl Pts',(-1.11110194300006,11.6,-10.890808352));
#299518=CARTESIAN_POINT('Ctrl Pts',(-1.11041276500006,15.2,-10.893695239));
#299519=CARTESIAN_POINT('Ctrl Pts',(-1.11041276500006,11.6,-10.893695239));
#299520=CARTESIAN_POINT('Ctrl Pts',(-1.10971994600006,15.2,-10.89658685));
#299521=CARTESIAN_POINT('Ctrl Pts',(-1.10971994600006,11.6,-10.89658685));
#299522=CARTESIAN_POINT('Ctrl Pts',(-1.10902348300006,15.2,-10.899483171));
#299523=CARTESIAN_POINT('Ctrl Pts',(-1.10902348300006,11.6,-10.899483171));
#299524=CARTESIAN_POINT('Ctrl Pts',(-1.10832336800006,15.2,-10.902384191));
#299525=CARTESIAN_POINT('Ctrl Pts',(-1.10832336800006,11.6,-10.902384191));
#299526=CARTESIAN_POINT('Ctrl Pts',(-1.10761959700006,15.2,-10.905289901));
#299527=CARTESIAN_POINT('Ctrl Pts',(-1.10761959700006,11.6,-10.905289901));
#299528=CARTESIAN_POINT('Ctrl Pts',(-1.10691216600006,15.2,-10.908200288));
#299529=CARTESIAN_POINT('Ctrl Pts',(-1.10691216600006,11.6,-10.908200288));
#299530=CARTESIAN_POINT('Ctrl Pts',(-1.10620106800006,15.2,-10.911115343));
#299531=CARTESIAN_POINT('Ctrl Pts',(-1.10620106800006,11.6,-10.911115343));
#299532=CARTESIAN_POINT('Ctrl Pts',(-1.10548630000006,15.2,-10.914035053));
#299533=CARTESIAN_POINT('Ctrl Pts',(-1.10548630000006,11.6,-10.914035053));
#299534=CARTESIAN_POINT('Ctrl Pts',(-1.10476785400005,15.2,-10.916959406));
#299535=CARTESIAN_POINT('Ctrl Pts',(-1.10476785400005,11.6,-10.916959406));
#299536=CARTESIAN_POINT('Ctrl Pts',(-1.10404572800006,15.2,-10.919888394));
#299537=CARTESIAN_POINT('Ctrl Pts',(-1.10404572800006,11.6,-10.919888394));
#299538=CARTESIAN_POINT('Ctrl Pts',(-1.10331991600006,15.2,-10.922822003));
#299539=CARTESIAN_POINT('Ctrl Pts',(-1.10331991600006,11.6,-10.922822003));
#299540=CARTESIAN_POINT('Ctrl Pts',(-1.10259041100006,15.2,-10.925760224));
#299541=CARTESIAN_POINT('Ctrl Pts',(-1.10259041100006,11.6,-10.925760224));
#299542=CARTESIAN_POINT('Ctrl Pts',(-1.10185721000006,15.2,-10.928703044));
#299543=CARTESIAN_POINT('Ctrl Pts',(-1.10185721000006,11.6,-10.928703044));
#299544=CARTESIAN_POINT('Ctrl Pts',(-1.10112030900006,15.2,-10.931650455));
#299545=CARTESIAN_POINT('Ctrl Pts',(-1.10112030900006,11.6,-10.931650455));
#299546=CARTESIAN_POINT('Ctrl Pts',(-1.10037970000006,15.2,-10.934602443));
#299547=CARTESIAN_POINT('Ctrl Pts',(-1.10037970000006,11.6,-10.934602443));
#299548=CARTESIAN_POINT('Ctrl Pts',(-1.09963538000006,15.2,-10.937559));
#299549=CARTESIAN_POINT('Ctrl Pts',(-1.09963538000006,11.6,-10.937559));
#299550=CARTESIAN_POINT('Ctrl Pts',(-1.09888734500006,15.2,-10.940520113));
#299551=CARTESIAN_POINT('Ctrl Pts',(-1.09888734500006,11.6,-10.940520113));
#299552=CARTESIAN_POINT('Ctrl Pts',(-1.09813558800006,15.2,-10.943485771));
#299553=CARTESIAN_POINT('Ctrl Pts',(-1.09813558800006,11.6,-10.943485771));
#299554=CARTESIAN_POINT('Ctrl Pts',(-1.09738010500006,15.2,-10.946455964));
#299555=CARTESIAN_POINT('Ctrl Pts',(-1.09738010500006,11.6,-10.946455964));
#299556=CARTESIAN_POINT('Ctrl Pts',(-1.09662089100006,15.2,-10.949430681));
#299557=CARTESIAN_POINT('Ctrl Pts',(-1.09662089100006,11.6,-10.949430681));
#299558=CARTESIAN_POINT('Ctrl Pts',(-1.09585794200005,15.2,-10.952409912));
#299559=CARTESIAN_POINT('Ctrl Pts',(-1.09585794200005,11.6,-10.952409912));
#299560=CARTESIAN_POINT('Ctrl Pts',(-1.09509125200006,15.2,-10.955393644));
#299561=CARTESIAN_POINT('Ctrl Pts',(-1.09509125200006,11.6,-10.955393644));
#299562=CARTESIAN_POINT('Ctrl Pts',(-1.09432081700006,15.2,-10.958381868));
#299563=CARTESIAN_POINT('Ctrl Pts',(-1.09432081700006,11.6,-10.958381868));
#299564=CARTESIAN_POINT('Ctrl Pts',(-1.09354663200006,15.2,-10.961374573));
#299565=CARTESIAN_POINT('Ctrl Pts',(-1.09354663200006,11.6,-10.961374573));
#299566=CARTESIAN_POINT('Ctrl Pts',(-1.09276869100006,15.2,-10.964371748));
#299567=CARTESIAN_POINT('Ctrl Pts',(-1.09276869100006,11.6,-10.964371748));
#299568=CARTESIAN_POINT('Ctrl Pts',(-1.09198699200006,15.2,-10.967373381));
#299569=CARTESIAN_POINT('Ctrl Pts',(-1.09198699200006,11.6,-10.967373381));
#299570=CARTESIAN_POINT('Ctrl Pts',(-1.09120152700006,15.2,-10.970379465));
#299571=CARTESIAN_POINT('Ctrl Pts',(-1.09120152700006,11.6,-10.970379465));
#299572=CARTESIAN_POINT('Ctrl Pts',(-1.09041229400006,15.2,-10.973389985));
#299573=CARTESIAN_POINT('Ctrl Pts',(-1.09041229400006,11.6,-10.973389985));
#299574=CARTESIAN_POINT('Ctrl Pts',(-1.08961928800006,15.2,-10.976404933));
#299575=CARTESIAN_POINT('Ctrl Pts',(-1.08961928800006,11.6,-10.976404933));
#299576=CARTESIAN_POINT('Ctrl Pts',(-1.08882250300006,15.2,-10.979424298));
#299577=CARTESIAN_POINT('Ctrl Pts',(-1.08882250300006,11.6,-10.979424298));
#299578=CARTESIAN_POINT('Ctrl Pts',(-1.08802193400006,15.2,-10.982448068));
#299579=CARTESIAN_POINT('Ctrl Pts',(-1.08802193400006,11.6,-10.982448068));
#299580=CARTESIAN_POINT('Ctrl Pts',(-1.08721757800006,15.2,-10.985476233));
#299581=CARTESIAN_POINT('Ctrl Pts',(-1.08721757800006,11.6,-10.985476233));
#299582=CARTESIAN_POINT('Ctrl Pts',(-1.08640943000006,15.2,-10.988508784));
#299583=CARTESIAN_POINT('Ctrl Pts',(-1.08640943000006,11.6,-10.988508784));
#299584=CARTESIAN_POINT('Ctrl Pts',(-1.08559748500006,15.2,-10.991545708));
#299585=CARTESIAN_POINT('Ctrl Pts',(-1.08559748500006,11.6,-10.991545708));
#299586=CARTESIAN_POINT('Ctrl Pts',(-1.08478173800005,15.2,-10.994586996));
#299587=CARTESIAN_POINT('Ctrl Pts',(-1.08478173800005,11.6,-10.994586996));
#299588=CARTESIAN_POINT('Ctrl Pts',(-1.08396218500006,15.2,-10.997632637));
#299589=CARTESIAN_POINT('Ctrl Pts',(-1.08396218500006,11.6,-10.997632637));
#299590=CARTESIAN_POINT('Ctrl Pts',(-1.08313882200005,15.2,-11.000682622));
#299591=CARTESIAN_POINT('Ctrl Pts',(-1.08313882200005,11.6,-11.000682622));
#299592=CARTESIAN_POINT('Ctrl Pts',(-1.08231164200006,15.2,-11.003736938));
#299593=CARTESIAN_POINT('Ctrl Pts',(-1.08231164200006,11.6,-11.003736938));
#299594=CARTESIAN_POINT('Ctrl Pts',(-1.08148064400006,15.2,-11.006795575));
#299595=CARTESIAN_POINT('Ctrl Pts',(-1.08148064400006,11.6,-11.006795575));
#299596=CARTESIAN_POINT('Ctrl Pts',(-1.08064582200006,15.2,-11.009858524));
#299597=CARTESIAN_POINT('Ctrl Pts',(-1.08064582200006,11.6,-11.009858524));
#299598=CARTESIAN_POINT('Ctrl Pts',(-1.07980717000006,15.2,-11.012925773));
#299599=CARTESIAN_POINT('Ctrl Pts',(-1.07980717000006,11.6,-11.012925773));
#299600=CARTESIAN_POINT('Ctrl Pts',(-1.07896468700006,15.2,-11.015997313));
#299601=CARTESIAN_POINT('Ctrl Pts',(-1.07896468700006,11.6,-11.015997313));
#299602=CARTESIAN_POINT('Ctrl Pts',(-1.07811836400006,15.2,-11.019073132));
#299603=CARTESIAN_POINT('Ctrl Pts',(-1.07811836400006,11.6,-11.019073132));
#299604=CARTESIAN_POINT('Ctrl Pts',(-1.07726820100006,15.2,-11.022153221));
#299605=CARTESIAN_POINT('Ctrl Pts',(-1.07726820100006,11.6,-11.022153221));
#299606=CARTESIAN_POINT('Ctrl Pts',(-1.07641419000006,15.2,-11.025237569));
#299607=CARTESIAN_POINT('Ctrl Pts',(-1.07641419000006,11.6,-11.025237569));
#299608=CARTESIAN_POINT('Ctrl Pts',(-1.07555633000006,15.2,-11.028326166));
#299609=CARTESIAN_POINT('Ctrl Pts',(-1.07555633000006,11.6,-11.028326166));
#299610=CARTESIAN_POINT('Ctrl Pts',(-1.07469461400005,15.2,-11.031419001));
#299611=CARTESIAN_POINT('Ctrl Pts',(-1.07469461400005,11.6,-11.031419001));
#299612=CARTESIAN_POINT('Ctrl Pts',(-1.07382903800006,15.2,-11.034516065));
#299613=CARTESIAN_POINT('Ctrl Pts',(-1.07382903800006,11.6,-11.034516065));
#299614=CARTESIAN_POINT('Ctrl Pts',(-1.07295959900006,15.2,-11.037617345));
#299615=CARTESIAN_POINT('Ctrl Pts',(-1.07295959900006,11.6,-11.037617345));
#299616=CARTESIAN_POINT('Ctrl Pts',(-1.07208629100006,15.2,-11.040722834));
#299617=CARTESIAN_POINT('Ctrl Pts',(-1.07208629100006,11.6,-11.040722834));
#299618=CARTESIAN_POINT('Ctrl Pts',(-1.07120911100006,15.2,-11.04383252));
#299619=CARTESIAN_POINT('Ctrl Pts',(-1.07120911100006,11.6,-11.04383252));
#299620=CARTESIAN_POINT('Ctrl Pts',(-1.07032805400006,15.2,-11.046946393));
#299621=CARTESIAN_POINT('Ctrl Pts',(-1.07032805400006,11.6,-11.046946393));
#299622=CARTESIAN_POINT('Ctrl Pts',(-1.06944311600006,15.2,-11.050064443));
#299623=CARTESIAN_POINT('Ctrl Pts',(-1.06944311600006,11.6,-11.050064443));
#299624=CARTESIAN_POINT('Ctrl Pts',(-1.06855429400005,15.2,-11.05318666));
#299625=CARTESIAN_POINT('Ctrl Pts',(-1.06855429400005,11.6,-11.05318666));
#299626=CARTESIAN_POINT('Ctrl Pts',(-1.06766158100006,15.2,-11.056313032));
#299627=CARTESIAN_POINT('Ctrl Pts',(-1.06766158100006,11.6,-11.056313032));
#299628=CARTESIAN_POINT('Ctrl Pts',(-1.06676497400006,15.2,-11.059443552));
#299629=CARTESIAN_POINT('Ctrl Pts',(-1.06676497400006,11.6,-11.059443552));
#299630=CARTESIAN_POINT('Ctrl Pts',(-1.06586447000006,15.2,-11.062578207));
#299631=CARTESIAN_POINT('Ctrl Pts',(-1.06586447000006,11.6,-11.062578207));
#299632=CARTESIAN_POINT('Ctrl Pts',(-1.06496006400006,15.2,-11.065716988));
#299633=CARTESIAN_POINT('Ctrl Pts',(-1.06496006400006,11.6,-11.065716988));
#299634=CARTESIAN_POINT('Ctrl Pts',(-1.06405175100006,15.2,-11.068859886));
#299635=CARTESIAN_POINT('Ctrl Pts',(-1.06405175100006,11.6,-11.068859886));
#299636=CARTESIAN_POINT('Ctrl Pts',(-1.06313952800006,15.2,-11.072006888));
#299637=CARTESIAN_POINT('Ctrl Pts',(-1.06313952800006,11.6,-11.072006888));
#299638=CARTESIAN_POINT('Ctrl Pts',(-1.06222339100006,15.2,-11.075157987));
#299639=CARTESIAN_POINT('Ctrl Pts',(-1.06222339100006,11.6,-11.075157987));
#299640=CARTESIAN_POINT('Ctrl Pts',(-1.06130333400006,15.2,-11.07831317));
#299641=CARTESIAN_POINT('Ctrl Pts',(-1.06130333400006,11.6,-11.07831317));
#299642=CARTESIAN_POINT('Ctrl Pts',(-1.06037935500006,15.2,-11.08147243));
#299643=CARTESIAN_POINT('Ctrl Pts',(-1.06037935500006,11.6,-11.08147243));
#299644=CARTESIAN_POINT('Ctrl Pts',(-1.05945145000006,15.2,-11.084635755));
#299645=CARTESIAN_POINT('Ctrl Pts',(-1.05945145000006,11.6,-11.084635755));
#299646=CARTESIAN_POINT('Ctrl Pts',(-1.05851961200006,15.2,-11.087803135));
#299647=CARTESIAN_POINT('Ctrl Pts',(-1.05851961200006,11.6,-11.087803135));
#299648=CARTESIAN_POINT('Ctrl Pts',(-1.05758384000006,15.2,-11.090974562));
#299649=CARTESIAN_POINT('Ctrl Pts',(-1.05758384000006,11.6,-11.090974562));
#299650=CARTESIAN_POINT('Ctrl Pts',(-1.05664412900005,15.2,-11.094150024));
#299651=CARTESIAN_POINT('Ctrl Pts',(-1.05664412900005,11.6,-11.094150024));
#299652=CARTESIAN_POINT('Ctrl Pts',(-1.05570047500006,15.2,-11.09732951));
#299653=CARTESIAN_POINT('Ctrl Pts',(-1.05570047500006,11.6,-11.09732951));
#299654=CARTESIAN_POINT('Ctrl Pts',(-1.05475287400006,15.2,-11.100513013));
#299655=CARTESIAN_POINT('Ctrl Pts',(-1.05475287400006,11.6,-11.100513013));
#299656=CARTESIAN_POINT('Ctrl Pts',(-1.05380132100006,15.2,-11.103700521));
#299657=CARTESIAN_POINT('Ctrl Pts',(-1.05380132100006,11.6,-11.103700521));
#299658=CARTESIAN_POINT('Ctrl Pts',(-1.05284581400006,15.2,-11.106892026));
#299659=CARTESIAN_POINT('Ctrl Pts',(-1.05284581400006,11.6,-11.106892026));
#299660=CARTESIAN_POINT('Ctrl Pts',(-1.05188634700006,15.2,-11.110087516));
#299661=CARTESIAN_POINT('Ctrl Pts',(-1.05188634700006,11.6,-11.110087516));
#299662=CARTESIAN_POINT('Ctrl Pts',(-1.05092291800006,15.2,-11.113286981));
#299663=CARTESIAN_POINT('Ctrl Pts',(-1.05092291800006,11.6,-11.113286981));
#299664=CARTESIAN_POINT('Ctrl Pts',(-1.04995552100006,15.2,-11.116490413));
#299665=CARTESIAN_POINT('Ctrl Pts',(-1.04995552100006,11.6,-11.116490413));
#299666=CARTESIAN_POINT('Ctrl Pts',(-1.04898415400006,15.2,-11.119697801));
#299667=CARTESIAN_POINT('Ctrl Pts',(-1.04898415400006,11.6,-11.119697801));
#299668=CARTESIAN_POINT('Ctrl Pts',(-1.04800881300006,15.2,-11.122909136));
#299669=CARTESIAN_POINT('Ctrl Pts',(-1.04800881300006,11.6,-11.122909136));
#299670=CARTESIAN_POINT('Ctrl Pts',(-1.04702949200006,15.2,-11.126124407));
#299671=CARTESIAN_POINT('Ctrl Pts',(-1.04702949200006,11.6,-11.126124407));
#299672=CARTESIAN_POINT('Ctrl Pts',(-1.04604618900005,15.2,-11.129343605));
#299673=CARTESIAN_POINT('Ctrl Pts',(-1.04604618900005,11.6,-11.129343605));
#299674=CARTESIAN_POINT('Ctrl Pts',(-1.04505890000006,15.2,-11.13256672));
#299675=CARTESIAN_POINT('Ctrl Pts',(-1.04505890000006,11.6,-11.13256672));
#299676=CARTESIAN_POINT('Ctrl Pts',(-1.04406762000006,15.2,-11.135793742));
#299677=CARTESIAN_POINT('Ctrl Pts',(-1.04406762000006,11.6,-11.135793742));
#299678=CARTESIAN_POINT('Ctrl Pts',(-1.04307234700006,15.2,-11.139024662));
#299679=CARTESIAN_POINT('Ctrl Pts',(-1.04307234700006,11.6,-11.139024662));
#299680=CARTESIAN_POINT('Ctrl Pts',(-1.04207307600006,15.2,-11.142259468));
#299681=CARTESIAN_POINT('Ctrl Pts',(-1.04207307600006,11.6,-11.142259468));
#299682=CARTESIAN_POINT('Ctrl Pts',(-1.04106980400006,15.2,-11.145498154));
#299683=CARTESIAN_POINT('Ctrl Pts',(-1.04106980400006,11.6,-11.145498154));
#299684=CARTESIAN_POINT('Ctrl Pts',(-1.04006252600006,15.2,-11.148740707));
#299685=CARTESIAN_POINT('Ctrl Pts',(-1.04006252600006,11.6,-11.148740707));
#299686=CARTESIAN_POINT('Ctrl Pts',(-1.03905123800006,15.2,-11.151987119));
#299687=CARTESIAN_POINT('Ctrl Pts',(-1.03905123800006,11.6,-11.151987119));
#299688=CARTESIAN_POINT('Ctrl Pts',(-1.03803593800005,15.2,-11.155237381));
#299689=CARTESIAN_POINT('Ctrl Pts',(-1.03803593800005,11.6,-11.155237381));
#299690=CARTESIAN_POINT('Ctrl Pts',(-1.03701662100006,15.2,-11.158491481));
#299691=CARTESIAN_POINT('Ctrl Pts',(-1.03701662100006,11.6,-11.158491481));
#299692=CARTESIAN_POINT('Ctrl Pts',(-1.03599328400006,15.2,-11.16174941));
#299693=CARTESIAN_POINT('Ctrl Pts',(-1.03599328400006,11.6,-11.16174941));
#299694=CARTESIAN_POINT('Ctrl Pts',(-1.03496592300006,15.2,-11.165011161));
#299695=CARTESIAN_POINT('Ctrl Pts',(-1.03496592300006,11.6,-11.165011161));
#299696=CARTESIAN_POINT('Ctrl Pts',(-1.03393453400005,15.2,-11.168276721));
#299697=CARTESIAN_POINT('Ctrl Pts',(-1.03393453400005,11.6,-11.168276721));
#299698=CARTESIAN_POINT('Ctrl Pts',(-1.03289911500006,15.2,-11.171546082));
#299699=CARTESIAN_POINT('Ctrl Pts',(-1.03289911500006,11.6,-11.171546082));
#299700=CARTESIAN_POINT('Ctrl Pts',(-1.03185965900006,15.2,-11.174819234));
#299701=CARTESIAN_POINT('Ctrl Pts',(-1.03185965900006,11.6,-11.174819234));
#299702=CARTESIAN_POINT('Ctrl Pts',(-1.03081616500006,15.2,-11.178096168));
#299703=CARTESIAN_POINT('Ctrl Pts',(-1.03081616500006,11.6,-11.178096168));
#299704=CARTESIAN_POINT('Ctrl Pts',(-1.02976862900006,15.2,-11.181376874));
#299705=CARTESIAN_POINT('Ctrl Pts',(-1.02976862900006,11.6,-11.181376874));
#299706=CARTESIAN_POINT('Ctrl Pts',(-1.02871704700006,15.2,-11.184661341));
#299707=CARTESIAN_POINT('Ctrl Pts',(-1.02871704700006,11.6,-11.184661341));
#299708=CARTESIAN_POINT('Ctrl Pts',(-1.02766141600006,15.2,-11.187949563));
#299709=CARTESIAN_POINT('Ctrl Pts',(-1.02766141600006,11.6,-11.187949563));
#299710=CARTESIAN_POINT('Ctrl Pts',(-1.02660173100006,15.2,-11.191241529));
#299711=CARTESIAN_POINT('Ctrl Pts',(-1.02660173100006,11.6,-11.191241529));
#299712=CARTESIAN_POINT('Ctrl Pts',(-1.02553799000005,15.2,-11.194537226));
#299713=CARTESIAN_POINT('Ctrl Pts',(-1.02553799000005,11.6,-11.194537226));
#299714=CARTESIAN_POINT('Ctrl Pts',(-1.02447018800006,15.2,-11.19783665));
#299715=CARTESIAN_POINT('Ctrl Pts',(-1.02447018800006,11.6,-11.19783665));
#299716=CARTESIAN_POINT('Ctrl Pts',(-1.02339832300006,15.2,-11.201139788));
#299717=CARTESIAN_POINT('Ctrl Pts',(-1.02339832300006,11.6,-11.201139788));
#299718=CARTESIAN_POINT('Ctrl Pts',(-1.02232239100006,15.2,-11.204446633));
#299719=CARTESIAN_POINT('Ctrl Pts',(-1.02232239100006,11.6,-11.204446633));
#299720=CARTESIAN_POINT('Ctrl Pts',(-1.02124238700006,15.2,-11.207757173));
#299721=CARTESIAN_POINT('Ctrl Pts',(-1.02124238700006,11.6,-11.207757173));
#299722=CARTESIAN_POINT('Ctrl Pts',(-1.02015830900006,15.2,-11.2110714));
#299723=CARTESIAN_POINT('Ctrl Pts',(-1.02015830900006,11.6,-11.2110714));
#299724=CARTESIAN_POINT('Ctrl Pts',(-1.01907015400006,15.2,-11.214389304));
#299725=CARTESIAN_POINT('Ctrl Pts',(-1.01907015400006,11.6,-11.214389304));
#299726=CARTESIAN_POINT('Ctrl Pts',(-1.01797791800006,15.2,-11.217710877));
#299727=CARTESIAN_POINT('Ctrl Pts',(-1.01797791800006,11.6,-11.217710877));
#299728=CARTESIAN_POINT('Ctrl Pts',(-1.01688159500006,15.2,-11.221036107));
#299729=CARTESIAN_POINT('Ctrl Pts',(-1.01688159500006,11.6,-11.221036107));
#299730=CARTESIAN_POINT('Ctrl Pts',(-1.01578118600006,15.2,-11.224364987));
#299731=CARTESIAN_POINT('Ctrl Pts',(-1.01578118600006,11.6,-11.224364987));
#299732=CARTESIAN_POINT('Ctrl Pts',(-1.01467668500006,15.2,-11.227697507));
#299733=CARTESIAN_POINT('Ctrl Pts',(-1.01467668500006,11.6,-11.227697507));
#299734=CARTESIAN_POINT('Ctrl Pts',(-1.01356808900006,15.2,-11.231033658));
#299735=CARTESIAN_POINT('Ctrl Pts',(-1.01356808900006,11.6,-11.231033658));
#299736=CARTESIAN_POINT('Ctrl Pts',(-1.01245539400006,15.2,-11.234373429));
#299737=CARTESIAN_POINT('Ctrl Pts',(-1.01245539400006,11.6,-11.234373429));
#299738=CARTESIAN_POINT('Ctrl Pts',(-1.01133859700006,15.2,-11.237716813));
#299739=CARTESIAN_POINT('Ctrl Pts',(-1.01133859700006,11.6,-11.237716813));
#299740=CARTESIAN_POINT('Ctrl Pts',(-1.01021769600006,15.2,-11.241063799));
#299741=CARTESIAN_POINT('Ctrl Pts',(-1.01021769600006,11.6,-11.241063799));
#299742=CARTESIAN_POINT('Ctrl Pts',(-1.00909268600006,15.2,-11.244414379));
#299743=CARTESIAN_POINT('Ctrl Pts',(-1.00909268600006,11.6,-11.244414379));
#299744=CARTESIAN_POINT('Ctrl Pts',(-1.00796356300005,15.2,-11.247768543));
#299745=CARTESIAN_POINT('Ctrl Pts',(-1.00796356300005,11.6,-11.247768543));
#299746=CARTESIAN_POINT('Ctrl Pts',(-1.00683032600006,15.2,-11.251126281));
#299747=CARTESIAN_POINT('Ctrl Pts',(-1.00683032600006,11.6,-11.251126281));
#299748=CARTESIAN_POINT('Ctrl Pts',(-1.00569297000005,15.2,-11.254487585));
#299749=CARTESIAN_POINT('Ctrl Pts',(-1.00569297000005,11.6,-11.254487585));
#299750=CARTESIAN_POINT('Ctrl Pts',(-1.00455149300006,15.2,-11.257852446));
#299751=CARTESIAN_POINT('Ctrl Pts',(-1.00455149300006,11.6,-11.257852446));
#299752=CARTESIAN_POINT('Ctrl Pts',(-1.00340588900006,15.2,-11.261220853));
#299753=CARTESIAN_POINT('Ctrl Pts',(-1.00340588900006,11.6,-11.261220853));
#299754=CARTESIAN_POINT('Ctrl Pts',(-1.00225615900006,15.2,-11.264592799));
#299755=CARTESIAN_POINT('Ctrl Pts',(-1.00225615900006,11.6,-11.264592799));
#299756=CARTESIAN_POINT('Ctrl Pts',(-1.00110229600006,15.2,-11.267968274));
#299757=CARTESIAN_POINT('Ctrl Pts',(-1.00110229600006,11.6,-11.267968274));
#299758=CARTESIAN_POINT('Ctrl Pts',(-0.999944298000056,15.2,-11.271347269));
#299759=CARTESIAN_POINT('Ctrl Pts',(-0.999944298000056,11.6,-11.271347269));
#299760=CARTESIAN_POINT('Ctrl Pts',(-0.998782162000056,15.2,-11.274729773));
#299761=CARTESIAN_POINT('Ctrl Pts',(-0.998782162000056,11.6,-11.274729773));
#299762=CARTESIAN_POINT('Ctrl Pts',(-0.997615884000057,15.2,-11.278115779));
#299763=CARTESIAN_POINT('Ctrl Pts',(-0.997615884000057,11.6,-11.278115779));
#299764=CARTESIAN_POINT('Ctrl Pts',(-0.996445463000055,15.2,-11.281505277));
#299765=CARTESIAN_POINT('Ctrl Pts',(-0.996445463000055,11.6,-11.281505277));
#299766=CARTESIAN_POINT('Ctrl Pts',(-0.995270892000055,15.2,-11.284898258));
#299767=CARTESIAN_POINT('Ctrl Pts',(-0.995270892000055,11.6,-11.284898258));
#299768=CARTESIAN_POINT('Ctrl Pts',(-0.994092171000055,15.2,-11.288294715));
#299769=CARTESIAN_POINT('Ctrl Pts',(-0.994092171000055,11.6,-11.288294715));
#299770=CARTESIAN_POINT('Ctrl Pts',(-0.992909296000055,15.2,-11.291694635));
#299771=CARTESIAN_POINT('Ctrl Pts',(-0.992909296000055,11.6,-11.291694635));
#299772=CARTESIAN_POINT('Ctrl Pts',(-0.991722264000057,15.2,-11.295098011));
#299773=CARTESIAN_POINT('Ctrl Pts',(-0.991722264000057,11.6,-11.295098011));
#299774=CARTESIAN_POINT('Ctrl Pts',(-0.990531071000056,15.2,-11.298504835));
#299775=CARTESIAN_POINT('Ctrl Pts',(-0.990531071000056,11.6,-11.298504835));
#299776=CARTESIAN_POINT('Ctrl Pts',(-0.989335715000056,15.2,-11.301915096));
#299777=CARTESIAN_POINT('Ctrl Pts',(-0.989335715000056,11.6,-11.301915096));
#299778=CARTESIAN_POINT('Ctrl Pts',(-0.988136191000055,15.2,-11.305328786));
#299779=CARTESIAN_POINT('Ctrl Pts',(-0.988136191000055,11.6,-11.305328786));
#299780=CARTESIAN_POINT('Ctrl Pts',(-0.986932499000056,15.2,-11.308745895));
#299781=CARTESIAN_POINT('Ctrl Pts',(-0.986932499000056,11.6,-11.308745895));
#299782=CARTESIAN_POINT('Ctrl Pts',(-0.985724632000055,15.2,-11.312166416));
#299783=CARTESIAN_POINT('Ctrl Pts',(-0.985724632000055,11.6,-11.312166416));
#299784=CARTESIAN_POINT('Ctrl Pts',(-0.984512591000056,15.2,-11.315590339));
#299785=CARTESIAN_POINT('Ctrl Pts',(-0.984512591000056,11.6,-11.315590339));
#299786=CARTESIAN_POINT('Ctrl Pts',(-0.983296369000056,15.2,-11.319017654));
#299787=CARTESIAN_POINT('Ctrl Pts',(-0.983296369000056,11.6,-11.319017654));
#299788=CARTESIAN_POINT('Ctrl Pts',(-0.982075966000057,15.2,-11.322448353));
#299789=CARTESIAN_POINT('Ctrl Pts',(-0.982075966000057,11.6,-11.322448353));
#299790=CARTESIAN_POINT('Ctrl Pts',(-0.980851378000055,15.2,-11.325882426));
#299791=CARTESIAN_POINT('Ctrl Pts',(-0.980851378000055,11.6,-11.325882426));
#299792=CARTESIAN_POINT('Ctrl Pts',(-0.979622600000055,15.2,-11.329319866));
#299793=CARTESIAN_POINT('Ctrl Pts',(-0.979622600000055,11.6,-11.329319866));
#299794=CARTESIAN_POINT('Ctrl Pts',(-0.978389633000055,15.2,-11.332760663));
#299795=CARTESIAN_POINT('Ctrl Pts',(-0.978389633000055,11.6,-11.332760663));
#299796=CARTESIAN_POINT('Ctrl Pts',(-0.977152471000055,15.2,-11.336204808));
#299797=CARTESIAN_POINT('Ctrl Pts',(-0.977152471000055,11.6,-11.336204808));
#299798=CARTESIAN_POINT('Ctrl Pts',(-0.975911111000055,15.2,-11.339652292));
#299799=CARTESIAN_POINT('Ctrl Pts',(-0.975911111000055,11.6,-11.339652292));
#299800=CARTESIAN_POINT('Ctrl Pts',(-0.974665552000056,15.2,-11.343103107));
#299801=CARTESIAN_POINT('Ctrl Pts',(-0.974665552000056,11.6,-11.343103107));
#299802=CARTESIAN_POINT('Ctrl Pts',(-0.973415788000055,15.2,-11.346557243));
#299803=CARTESIAN_POINT('Ctrl Pts',(-0.973415788000055,11.6,-11.346557243));
#299804=CARTESIAN_POINT('Ctrl Pts',(-0.972161820000055,15.2,-11.350014692));
#299805=CARTESIAN_POINT('Ctrl Pts',(-0.972161820000055,11.6,-11.350014692));
#299806=CARTESIAN_POINT('Ctrl Pts',(-0.970903641000056,15.2,-11.353475444));
#299807=CARTESIAN_POINT('Ctrl Pts',(-0.970903641000056,11.6,-11.353475444));
#299808=CARTESIAN_POINT('Ctrl Pts',(-0.969641251000055,15.2,-11.356939492));
#299809=CARTESIAN_POINT('Ctrl Pts',(-0.969641251000055,11.6,-11.356939492));
#299810=CARTESIAN_POINT('Ctrl Pts',(-0.968374645000055,15.2,-11.360406825));
#299811=CARTESIAN_POINT('Ctrl Pts',(-0.968374645000055,11.6,-11.360406825));
#299812=CARTESIAN_POINT('Ctrl Pts',(-0.967103822000055,15.2,-11.363877435));
#299813=CARTESIAN_POINT('Ctrl Pts',(-0.967103822000055,11.6,-11.363877435));
#299814=CARTESIAN_POINT('Ctrl Pts',(-0.965828779000055,15.2,-11.367351314));
#299815=CARTESIAN_POINT('Ctrl Pts',(-0.965828779000055,11.6,-11.367351314));
#299816=CARTESIAN_POINT('Ctrl Pts',(-0.964549511000056,15.2,-11.370828453));
#299817=CARTESIAN_POINT('Ctrl Pts',(-0.964549511000056,11.6,-11.370828453));
#299818=CARTESIAN_POINT('Ctrl Pts',(-0.963266016000055,15.2,-11.374308843));
#299819=CARTESIAN_POINT('Ctrl Pts',(-0.963266016000055,11.6,-11.374308843));
#299820=CARTESIAN_POINT('Ctrl Pts',(-0.961978293000056,15.2,-11.377792477));
#299821=CARTESIAN_POINT('Ctrl Pts',(-0.961978293000056,11.6,-11.377792477));
#299822=CARTESIAN_POINT('Ctrl Pts',(-0.960686338000055,15.2,-11.381279343));
#299823=CARTESIAN_POINT('Ctrl Pts',(-0.960686338000055,11.6,-11.381279343));
#299824=CARTESIAN_POINT('Ctrl Pts',(-0.959390148000056,15.2,-11.384769435));
#299825=CARTESIAN_POINT('Ctrl Pts',(-0.959390148000056,11.6,-11.384769435));
#299826=CARTESIAN_POINT('Ctrl Pts',(-0.958089718000057,15.2,-11.388262743));
#299827=CARTESIAN_POINT('Ctrl Pts',(-0.958089718000057,11.6,-11.388262743));
#299828=CARTESIAN_POINT('Ctrl Pts',(-0.956785050000055,15.2,-11.391759258));
#299829=CARTESIAN_POINT('Ctrl Pts',(-0.956785050000055,11.6,-11.391759258));
#299830=CARTESIAN_POINT('Ctrl Pts',(-0.955476137000056,15.2,-11.39525897));
#299831=CARTESIAN_POINT('Ctrl Pts',(-0.955476137000056,11.6,-11.39525897));
#299832=CARTESIAN_POINT('Ctrl Pts',(-0.954162977000056,15.2,-11.398761871));
#299833=CARTESIAN_POINT('Ctrl Pts',(-0.954162977000056,11.6,-11.398761871));
#299834=CARTESIAN_POINT('Ctrl Pts',(-0.952845568000056,15.2,-11.402267952));
#299835=CARTESIAN_POINT('Ctrl Pts',(-0.952845568000056,11.6,-11.402267952));
#299836=CARTESIAN_POINT('Ctrl Pts',(-0.951523907000055,15.2,-11.405777207));
#299837=CARTESIAN_POINT('Ctrl Pts',(-0.951523907000055,11.6,-11.405777207));
#299838=CARTESIAN_POINT('Ctrl Pts',(-0.950197992000056,15.2,-11.409289625));
#299839=CARTESIAN_POINT('Ctrl Pts',(-0.950197992000056,11.6,-11.409289625));
#299840=CARTESIAN_POINT('Ctrl Pts',(-0.948867819000055,15.2,-11.4128052));
#299841=CARTESIAN_POINT('Ctrl Pts',(-0.948867819000055,11.6,-11.4128052));
#299842=CARTESIAN_POINT('Ctrl Pts',(-0.947533388000057,15.2,-11.416323924));
#299843=CARTESIAN_POINT('Ctrl Pts',(-0.947533388000057,11.6,-11.416323924));
#299844=CARTESIAN_POINT('Ctrl Pts',(-0.946194693000055,15.2,-11.419845789));
#299845=CARTESIAN_POINT('Ctrl Pts',(-0.946194693000055,11.6,-11.419845789));
#299846=CARTESIAN_POINT('Ctrl Pts',(-0.944851735000055,15.2,-11.423370784));
#299847=CARTESIAN_POINT('Ctrl Pts',(-0.944851735000055,11.6,-11.423370784));
#299848=CARTESIAN_POINT('Ctrl Pts',(-0.943504508000055,15.2,-11.426898902));
#299849=CARTESIAN_POINT('Ctrl Pts',(-0.943504508000055,11.6,-11.426898902));
#299850=CARTESIAN_POINT('Ctrl Pts',(-0.942153010000055,15.2,-11.430430131));
#299851=CARTESIAN_POINT('Ctrl Pts',(-0.942153010000055,11.6,-11.430430131));
#299852=CARTESIAN_POINT('Ctrl Pts',(-0.940797238000056,15.2,-11.433964459));
#299853=CARTESIAN_POINT('Ctrl Pts',(-0.940797238000056,11.6,-11.433964459));
#299854=CARTESIAN_POINT('Ctrl Pts',(-0.939437187000056,15.2,-11.437501879));
#299855=CARTESIAN_POINT('Ctrl Pts',(-0.939437187000056,11.6,-11.437501879));
#299856=CARTESIAN_POINT('Ctrl Pts',(-0.938072856000056,15.2,-11.441042379));
#299857=CARTESIAN_POINT('Ctrl Pts',(-0.938072856000056,11.6,-11.441042379));
#299858=CARTESIAN_POINT('Ctrl Pts',(-0.936704242000056,15.2,-11.444585951));
#299859=CARTESIAN_POINT('Ctrl Pts',(-0.936704242000056,11.6,-11.444585951));
#299860=CARTESIAN_POINT('Ctrl Pts',(-0.935331342000056,15.2,-11.448132592));
#299861=CARTESIAN_POINT('Ctrl Pts',(-0.935331342000056,11.6,-11.448132592));
#299862=CARTESIAN_POINT('Ctrl Pts',(-0.933954157000055,15.2,-11.451682295));
#299863=CARTESIAN_POINT('Ctrl Pts',(-0.933954157000055,11.6,-11.451682295));
#299864=CARTESIAN_POINT('Ctrl Pts',(-0.932572685000055,15.2,-11.45523506));
#299865=CARTESIAN_POINT('Ctrl Pts',(-0.932572685000055,11.6,-11.45523506));
#299866=CARTESIAN_POINT('Ctrl Pts',(-0.931464077000056,15.2,-11.45807972));
#299867=CARTESIAN_POINT('Ctrl Pts',(-0.931464077000056,11.6,-11.45807972));
#299868=CARTESIAN_POINT('Ctrl Pts',(-0.930630693000056,15.2,-11.460214591));
#299869=CARTESIAN_POINT('Ctrl Pts',(-0.930630693000056,11.6,-11.460214591));
#299870=CARTESIAN_POINT('Ctrl Pts',(-0.930074247000056,15.2,-11.461638451));
#299871=CARTESIAN_POINT('Ctrl Pts',(-0.930074247000056,11.6,-11.461638451));
#299872=CARTESIAN_POINT('Ctrl Pts',(-0.929795809000057,15.2,-11.462350534));
#299873=CARTESIAN_POINT('Ctrl Pts',(-0.929795809000057,11.6,-11.462350534));
#299874=CARTESIAN_POINT('Ctrl Pts',(-1.18690176600006,12.2,-10.306885524));
#299875=CARTESIAN_POINT('Ctrl Pts',(-1.18695287825247,12.2,-10.3086714504511));
#299876=CARTESIAN_POINT('Ctrl Pts',(-1.18700024431844,12.2,-10.3105146700777));
#299877=CARTESIAN_POINT('Ctrl Pts',(-1.18704320796202,12.2,-10.3124142312835));
#299878=CARTESIAN_POINT('Ctrl Pts',(-1.18708637879801,12.2,-10.3143229531337));
#299879=CARTESIAN_POINT('Ctrl Pts',(-1.18712509994175,12.2,-10.3162885639395));
#299880=CARTESIAN_POINT('Ctrl Pts',(-1.1871587090283,12.2,-10.3183101249039));
#299881=CARTESIAN_POINT('Ctrl Pts',(-1.1871923181118,12.2,-10.3203316856847));
#299882=CARTESIAN_POINT('Ctrl Pts',(-1.18722081733423,12.2,-10.322409198819));
#299883=CARTESIAN_POINT('Ctrl Pts',(-1.18724356650007,12.2,-10.3245417524916));
#299884=CARTESIAN_POINT('Ctrl Pts',(-1.18726631566591,12.2,-10.3266743061641));
#299885=CARTESIAN_POINT('Ctrl Pts',(-1.18728331741518,12.2,-10.3288618993474));
#299886=CARTESIAN_POINT('Ctrl Pts',(-1.18729394974902,12.2,-10.3311036472915));
#299887=CARTESIAN_POINT('Ctrl Pts',(-1.18730458208384,12.2,-10.3333453954392));
#299888=CARTESIAN_POINT('Ctrl Pts',(-1.18730884758373,12.2,-10.335641298191));
#299889=CARTESIAN_POINT('Ctrl Pts',(-1.18730614774977,12.2,-10.3379904903227));
#299890=CARTESIAN_POINT('Ctrl Pts',(-1.18730344791606,12.2,-10.3403396822409));
#299891=CARTESIAN_POINT('Ctrl Pts',(-1.18729378039953,12.2,-10.3427421643207));
#299892=CARTESIAN_POINT('Ctrl Pts',(-1.18727656873339,12.2,-10.3451970944927));
#299893=CARTESIAN_POINT('Ctrl Pts',(-1.18725935706726,12.2,-10.3476520246647));
#299894=CARTESIAN_POINT('Ctrl Pts',(-1.18723459815028,12.2,-10.3501594023475));
#299895=CARTESIAN_POINT('Ctrl Pts',(-1.18720173348516,12.2,-10.3527184083357));
#299896=CARTESIAN_POINT('Ctrl Pts',(-1.18716886881705,12.2,-10.3552774145562));
#299897=CARTESIAN_POINT('Ctrl Pts',(-1.18712789608962,12.2,-10.3578880464332));
#299898=CARTESIAN_POINT('Ctrl Pts',(-1.18707827150299,12.2,-10.3605495048317));
#299899=CARTESIAN_POINT('Ctrl Pts',(-1.18702864692087,12.2,-10.3632109629885));
#299900=CARTESIAN_POINT('Ctrl Pts',(-1.18697036877764,12.2,-10.3659232462155));
#299901=CARTESIAN_POINT('Ctrl Pts',(-1.18690291127969,12.2,-10.3686855726173));
#299902=CARTESIAN_POINT('Ctrl Pts',(-1.18683545378174,12.2,-10.3714478990192));
#299903=CARTESIAN_POINT('Ctrl Pts',(-1.18675881418451,12.2,-10.3742602688836));
#299904=CARTESIAN_POINT('Ctrl Pts',(-1.18667248268807,12.2,-10.3771219181108));
#299905=CARTESIAN_POINT('Ctrl Pts',(-1.18658615119163,12.2,-10.379983567338));
#299906=CARTESIAN_POINT('Ctrl Pts',(-1.18649012644043,12.2,-10.3828944944465));
#299907=CARTESIAN_POINT('Ctrl Pts',(-1.18638390927832,12.2,-10.385853953919));
#299908=CARTESIAN_POINT('Ctrl Pts',(-1.18627769210655,12.2,-10.3888134136604));
#299909=CARTESIAN_POINT('Ctrl Pts',(-1.18616128558383,12.2,-10.3918214053147));
#299910=CARTESIAN_POINT('Ctrl Pts',(-1.1860342042431,12.2,-10.39487719815));
#299911=CARTESIAN_POINT('Ctrl Pts',(-1.18590712291392,12.2,-10.3979329907077));
#299912=CARTESIAN_POINT('Ctrl Pts',(-1.18576936691205,12.2,-10.4010365852655));
#299913=CARTESIAN_POINT('Ctrl Pts',(-1.18562046775014,12.2,-10.4041872659985));
#299914=CARTESIAN_POINT('Ctrl Pts',(-1.18547156858824,12.2,-10.4073379467315));
#299915=CARTESIAN_POINT('Ctrl Pts',(-1.18531152576172,12.2,-10.410535714918));
#299916=CARTESIAN_POINT('Ctrl Pts',(-1.18513988276875,12.2,-10.4137798696303));
#299917=CARTESIAN_POINT('Ctrl Pts',(-1.18496823976018,12.2,-10.4170240246374));
#299918=CARTESIAN_POINT('Ctrl Pts',(-1.18478499820055,12.2,-10.4203145675565));
#299919=CARTESIAN_POINT('Ctrl Pts',(-1.18458971402272,12.2,-10.423650812657));
#299920=CARTESIAN_POINT('Ctrl Pts',(-1.18439442986262,12.2,-10.4269870574544));
#299921=CARTESIAN_POINT('Ctrl Pts',(-1.18418710221816,12.2,-10.4303690046824));
#299922=CARTESIAN_POINT('Ctrl Pts',(-1.18396730047518,12.2,-10.43379598349));
#299923=CARTESIAN_POINT('Ctrl Pts',(-1.18374749873219,12.2,-10.4372229622977));
#299924=CARTESIAN_POINT('Ctrl Pts',(-1.18351522376701,12.2,-10.4406949718391));
#299925=CARTESIAN_POINT('Ctrl Pts',(-1.1832700567768,12.2,-10.444211356625));
#299926=CARTESIAN_POINT('Ctrl Pts',(-1.18302488976432,12.2,-10.4477277417303));
#299927=CARTESIAN_POINT('Ctrl Pts',(-1.18276682798624,12.2,-10.4512885011114));
#299928=CARTESIAN_POINT('Ctrl Pts',(-1.18249546795713,12.2,-10.4548929895738));
#299929=CARTESIAN_POINT('Ctrl Pts',(-1.18222410795266,12.2,-10.4584974777087));
#299930=CARTESIAN_POINT('Ctrl Pts',(-1.18193944638091,12.2,-10.4621456945924));
#299931=CARTESIAN_POINT('Ctrl Pts',(-1.18164108847508,12.2,-10.4658370095416));
#299932=CARTESIAN_POINT('Ctrl Pts',(-1.18134273056926,12.2,-10.4695283244908));
#299933=CARTESIAN_POINT('Ctrl Pts',(-1.18103067595189,12.2,-10.473262737469));
#299934=CARTESIAN_POINT('Ctrl Pts',(-1.1807045372816,12.2,-10.4770396258513));
#299935=CARTESIAN_POINT('Ctrl Pts',(-1.18037839858167,12.2,-10.4808165145767));
#299936=CARTESIAN_POINT('Ctrl Pts',(-1.1800381776234,12.2,-10.4846358832492));
#299937=CARTESIAN_POINT('Ctrl Pts',(-1.17968349868642,12.2,-10.4884971177125));
#299938=CARTESIAN_POINT('Ctrl Pts',(-1.17932881978165,12.2,-10.4923583518251));
#299939=CARTESIAN_POINT('Ctrl Pts',(-1.17895967939607,12.2,-10.4962614543104));
#299940=CARTESIAN_POINT('Ctrl Pts',(-1.17857571749157,12.2,-10.5002058275184));
#299941=CARTESIAN_POINT('Ctrl Pts',(-1.17819175558708,12.2,-10.5041502007264));
#299942=CARTESIAN_POINT('Ctrl Pts',(-1.17779296731521,12.2,-10.5081358447371));
#299943=CARTESIAN_POINT('Ctrl Pts',(-1.17737899874758,12.2,-10.5121621710057));
#299944=CARTESIAN_POINT('Ctrl Pts',(-1.17703402492869,12.2,-10.5155174430181));
#299945=CARTESIAN_POINT('Ctrl Pts',(-1.17667850924008,12.2,-10.5189009680785));
#299946=CARTESIAN_POINT('Ctrl Pts',(-1.1763122502823,12.2,-10.5223124107853));
#299947=CARTESIAN_POINT('Ctrl Pts',(-1.17594599132453,12.2,-10.5257238534922));
#299948=CARTESIAN_POINT('Ctrl Pts',(-1.17556898840758,12.2,-10.5291632140324));
#299949=CARTESIAN_POINT('Ctrl Pts',(-1.17518104472529,12.2,-10.5326301642564));
#299950=CARTESIAN_POINT('Ctrl Pts',(-1.17479310104301,12.2,-10.5360971144804));
#299951=CARTESIAN_POINT('Ctrl Pts',(-1.17439421778898,12.2,-10.5395916512833));
#299952=CARTESIAN_POINT('Ctrl Pts',(-1.17398420077509,12.2,-10.5431134539916));
#299953=CARTESIAN_POINT('Ctrl Pts',(-1.1735741837612,12.2,-10.5466352566999));
#299954=CARTESIAN_POINT('Ctrl Pts',(-1.17315303389629,12.2,-10.55018432143));
#299955=CARTESIAN_POINT('Ctrl Pts',(-1.17272056174151,12.2,-10.5537603309602));
#299956=CARTESIAN_POINT('Ctrl Pts',(-1.17228808958674,12.2,-10.5573363404904));
#299957=CARTESIAN_POINT('Ctrl Pts',(-1.17184429560973,12.2,-10.5609392926138));
#299958=CARTESIAN_POINT('Ctrl Pts',(-1.17138899526191,12.2,-10.5645688729625));
#299959=CARTESIAN_POINT('Ctrl Pts',(-1.17093369491408,12.2,-10.5681984533111));
#299960=CARTESIAN_POINT('Ctrl Pts',(-1.17046688745822,12.2,-10.5718546597562));
#299961=CARTESIAN_POINT('Ctrl Pts',(-1.16998839294372,12.2,-10.5755371826743));
#299962=CARTESIAN_POINT('Ctrl Pts',(-1.16950989842922,12.2,-10.5792197055923));
#299963=CARTESIAN_POINT('Ctrl Pts',(-1.16901971706767,12.2,-10.5829285444452));
#299964=CARTESIAN_POINT('Ctrl Pts',(-1.16851767016676,12.2,-10.5866633917169));
#299965=CARTESIAN_POINT('Ctrl Pts',(-1.16791521390756,12.2,-10.5911452082802));
#299966=CARTESIAN_POINT('Ctrl Pts',(-1.16729567313537,12.2,-10.5956644770899));
#299967=CARTESIAN_POINT('Ctrl Pts',(-1.16665874874172,12.2,-10.6002206725085));
#299968=CARTESIAN_POINT('Ctrl Pts',(-1.1661279783944,12.2,-10.604017502162));
#299969=CARTESIAN_POINT('Ctrl Pts',(-1.16558513589678,12.2,-10.6078399757678));
#299970=CARTESIAN_POINT('Ctrl Pts',(-1.16503005228311,12.2,-10.6116877962021));
#299971=CARTESIAN_POINT('Ctrl Pts',(-1.16447496866945,12.2,-10.6155356166363));
#299972=CARTESIAN_POINT('Ctrl Pts',(-1.16390764256274,12.2,-10.6194087828815));
#299973=CARTESIAN_POINT('Ctrl Pts',(-1.1633279106871,12.2,-10.6233069992717));
#299974=CARTESIAN_POINT('Ctrl Pts',(-1.16274817881145,12.2,-10.6272052156619));
#299975=CARTESIAN_POINT('Ctrl Pts',(-1.16215604066112,12.2,-10.6311284828292));
#299976=CARTESIAN_POINT('Ctrl Pts',(-1.16155133295213,12.2,-10.6350765099833));
#299977=CARTESIAN_POINT('Ctrl Pts',(-1.16094662524314,12.2,-10.6390245371374));
#299978=CARTESIAN_POINT('Ctrl Pts',(-1.16032934929836,12.2,-10.6429973217769));
#299979=CARTESIAN_POINT('Ctrl Pts',(-1.15969934499214,12.2,-10.6469945805282));
#299980=CARTESIAN_POINT('Ctrl Pts',(-1.15906934068592,12.2,-10.6509918392795));
#299981=CARTESIAN_POINT('Ctrl Pts',(-1.1584266080187,12.2,-10.6550135687715));
#299982=CARTESIAN_POINT('Ctrl Pts',(-1.15777099270727,12.2,-10.659059485503));
#299983=CARTESIAN_POINT('Ctrl Pts',(-1.15711537739584,12.2,-10.6631054022346));
#299984=CARTESIAN_POINT('Ctrl Pts',(-1.15644687732867,12.2,-10.6671755075668));
#299985=CARTESIAN_POINT('Ctrl Pts',(-1.15576534211927,12.2,-10.6712695190271));
#299986=CARTESIAN_POINT('Ctrl Pts',(-1.15522011399633,12.2,-10.6745447279276));
#299987=CARTESIAN_POINT('Ctrl Pts',(-1.15466654389668,12.2,-10.6778352358539));
#299988=CARTESIAN_POINT('Ctrl Pts',(-1.15410455255429,12.2,-10.6811409039715));
#299989=CARTESIAN_POINT('Ctrl Pts',(-1.15354256113532,12.2,-10.6844465725396));
#299990=CARTESIAN_POINT('Ctrl Pts',(-1.15297215054114,12.2,-10.687767398726));
#299991=CARTESIAN_POINT('Ctrl Pts',(-1.15239324442437,12.2,-10.6911032422424));
#299992=CARTESIAN_POINT('Ctrl Pts',(-1.15166961181785,12.2,-10.6952730464107));
#299993=CARTESIAN_POINT('Ctrl Pts',(-1.15093270666971,12.2,-10.6994663145718));
#299994=CARTESIAN_POINT('Ctrl Pts',(-1.15018238166861,12.2,-10.7036827752681));
#299995=CARTESIAN_POINT('Ctrl Pts',(-1.1495821217168,12.2,-10.7070559435494));
#299996=CARTESIAN_POINT('Ctrl Pts',(-1.14897327395778,12.2,-10.7104439541788));
#299997=CARTESIAN_POINT('Ctrl Pts',(-1.14835576650882,12.2,-10.7138466704553));
#299998=CARTESIAN_POINT('Ctrl Pts',(-1.14773825897573,12.2,-10.7172493871953));
#299999=CARTESIAN_POINT('Ctrl Pts',(-1.14711209039999,12.2,-10.7206668089522));
#300000=CARTESIAN_POINT('Ctrl Pts',(-1.14647719016625,12.2,-10.7240987992564));
#300001=CARTESIAN_POINT('Ctrl Pts',(-1.14584229001901,12.2,-10.727530789093));
#300002=CARTESIAN_POINT('Ctrl Pts',(-1.1451986568661,12.2,-10.7309773469649));
#300003=CARTESIAN_POINT('Ctrl Pts',(-1.14454622158668,12.2,-10.7344383379588));
#300004=CARTESIAN_POINT('Ctrl Pts',(-1.14389378621836,12.2,-10.7378993294243));
#300005=CARTESIAN_POINT('Ctrl Pts',(-1.14323254940177,12.2,-10.7413747540387));
#300006=CARTESIAN_POINT('Ctrl Pts',(-1.14256243942022,12.2,-10.7448644767854));
#300007=CARTESIAN_POINT('Ctrl Pts',(-1.14189232952998,12.2,-10.7483541990566));
#300008=CARTESIAN_POINT('Ctrl Pts',(-1.14121334901333,12.2,-10.7518582199831));
#300009=CARTESIAN_POINT('Ctrl Pts',(-1.14052542709153,12.2,-10.7553764064812));
#300010=CARTESIAN_POINT('Ctrl Pts',(-1.139837505076,12.2,-10.7588945934586));
#300011=CARTESIAN_POINT('Ctrl Pts',(-1.13914064425914,12.2,-10.7624269452319));
#300012=CARTESIAN_POINT('Ctrl Pts',(-1.1384347754423,12.2,-10.765973330815));
#300013=CARTESIAN_POINT('Ctrl Pts',(-1.13772890672163,12.2,-10.7695197159149));
#300014=CARTESIAN_POINT('Ctrl Pts',(-1.13701403064168,12.2,-10.773080135087));
#300015=CARTESIAN_POINT('Ctrl Pts',(-1.13629008136845,12.2,-10.7766544566822));
#300016=CARTESIAN_POINT('Ctrl Pts',(-1.13556613199659,12.2,-10.7802287787645));
#300017=CARTESIAN_POINT('Ctrl Pts',(-1.13483310857954,12.2,-10.7838170034258));
#300018=CARTESIAN_POINT('Ctrl Pts',(-1.13409094725792,12.2,-10.7874190010274));
#300019=CARTESIAN_POINT('Ctrl Pts',(-1.13334878603741,12.2,-10.7910209981382));
#300020=CARTESIAN_POINT('Ctrl Pts',(-1.13259748752799,12.2,-10.7946367690074));
#300021=CARTESIAN_POINT('Ctrl Pts',(-1.1318369855911,12.2,-10.7982661834316));
#300022=CARTESIAN_POINT('Ctrl Pts',(-1.13107648355059,12.2,-10.8018955983502));
#300023=CARTESIAN_POINT('Ctrl Pts',(-1.13030677830366,12.2,-10.805538657284));
#300024=CARTESIAN_POINT('Ctrl Pts',(-1.12952780948343,12.2,-10.8091952334833));
#300025=CARTESIAN_POINT('Ctrl Pts',(-1.1287488406632,12.2,-10.8128518096826));
#300026=CARTESIAN_POINT('Ctrl Pts',(-1.12796060426689,12.2,-10.8165219040584));
#300027=CARTESIAN_POINT('Ctrl Pts',(-1.12716304161135,12.2,-10.8202053870939));
#300028=CARTESIAN_POINT('Ctrl Pts',(-1.12636547906449,12.2,-10.8238888696274));
#300029=CARTESIAN_POINT('Ctrl Pts',(-1.12555858903203,12.2,-10.8275857441339));
#300030=CARTESIAN_POINT('Ctrl Pts',(-1.12474231098398,12.2,-10.8312958825141));
#300031=CARTESIAN_POINT('Ctrl Pts',(-1.12392603282471,12.2,-10.8350060213998));
#300032=CARTESIAN_POINT('Ctrl Pts',(-1.12310036603225,12.2,-10.8387294255531));
#300033=CARTESIAN_POINT('Ctrl Pts',(-1.12226525009688,12.2,-10.8424659703692));
#300034=CARTESIAN_POINT('Ctrl Pts',(-1.12143013427529,12.2,-10.8462025146762));
#300035=CARTESIAN_POINT('Ctrl Pts',(-1.12058556989661,12.2,-10.8499521982037));
#300036=CARTESIAN_POINT('Ctrl Pts',(-1.11973149857816,12.2,-10.8537148999508));
#300037=CARTESIAN_POINT('Ctrl Pts',(-1.11887742714334,12.2,-10.8574776022106));
#300038=CARTESIAN_POINT('Ctrl Pts',(-1.11801384703482,12.2,-10.8612533213057));
#300039=CARTESIAN_POINT('Ctrl Pts',(-1.11714070166501,12.2,-10.8650419357581));
#300040=CARTESIAN_POINT('Ctrl Pts',(-1.11626755641416,12.2,-10.8688305496943));
#300041=CARTESIAN_POINT('Ctrl Pts',(-1.11538484398271,12.2,-10.8726320577176));
#300042=CARTESIAN_POINT('Ctrl Pts',(-1.11449250938962,12.2,-10.8764463394049));
#300043=CARTESIAN_POINT('Ctrl Pts',(-1.11360017467495,12.2,-10.880260621612));
#300044=CARTESIAN_POINT('Ctrl Pts',(-1.11269821636468,12.2,-10.8840876768928));
#300045=CARTESIAN_POINT('Ctrl Pts',(-1.11178657842548,12.2,-10.8879273845473));
#300046=CARTESIAN_POINT('Ctrl Pts',(-1.11087494061048,12.2,-10.8917670916787));
#300047=CARTESIAN_POINT('Ctrl Pts',(-1.10995362280469,12.2,-10.895619452441));
#300048=CARTESIAN_POINT('Ctrl Pts',(-1.10902257016848,12.2,-10.8994843452059));
#300049=CARTESIAN_POINT('Ctrl Pts',(-1.1080915174054,12.2,-10.9033492384974));
#300050=CARTESIAN_POINT('Ctrl Pts',(-1.10715072837752,12.2,-10.9072266649192));
#300051=CARTESIAN_POINT('Ctrl Pts',(-1.10620015038063,12.2,-10.9111165070764));
#300052=CARTESIAN_POINT('Ctrl Pts',(-1.10524957251325,12.2,-10.9150063487037));
#300053=CARTESIAN_POINT('Ctrl Pts',(-1.10428920475062,12.2,-10.9189086035368));
#300054=CARTESIAN_POINT('Ctrl Pts',(-1.10331899294205,12.2,-10.9228231553266));
#300055=CARTESIAN_POINT('Ctrl Pts',(-1.1021062280822,12.2,-10.9277163454639));
#300056=CARTESIAN_POINT('Ctrl Pts',(-1.10087808131704,12.2,-10.9326287483732));
#300057=CARTESIAN_POINT('Ctrl Pts',(-1.09963445138776,12.2,-10.9375601383716));
#300058=CARTESIAN_POINT('Ctrl Pts',(-1.0986395473901,12.2,-10.9415052505854));
#300059=CARTESIAN_POINT('Ctrl Pts',(-1.09763473318157,12.2,-10.9454625118544));
#300060=CARTESIAN_POINT('Ctrl Pts',(-1.09661995723274,12.2,-10.9494318094777));
#300061=CARTESIAN_POINT('Ctrl Pts',(-1.09535148736582,12.2,-10.9543934312364));
#300062=CARTESIAN_POINT('Ctrl Pts',(-1.09406745206026,12.2,-10.9593738575205));
#300063=CARTESIAN_POINT('Ctrl Pts',(-1.092767751365,12.2,-10.9643728628687));
#300064=CARTESIAN_POINT('Ctrl Pts',(-1.09120811058736,12.2,-10.9703716690685));
#300065=CARTESIAN_POINT('Ctrl Pts',(-1.08962591292817,12.2,-10.9763972332329));
#300066=CARTESIAN_POINT('Ctrl Pts',(-1.0880209873208,12.2,-10.9824491664286));
#300067=CARTESIAN_POINT('Ctrl Pts',(-1.0869510368187,12.2,-10.9864837889255));
#300068=CARTESIAN_POINT('Ctrl Pts',(-1.08587098690105,12.2,-10.9905301328751));
#300069=CARTESIAN_POINT('Ctrl Pts',(-1.08478078634185,12.2,-10.9945880848555));
#300070=CARTESIAN_POINT('Ctrl Pts',(-1.08369058593118,12.2,-10.9986460362831));
#300071=CARTESIAN_POINT('Ctrl Pts',(-1.08259023533267,12.2,-11.0027155968092));
#300072=CARTESIAN_POINT('Ctrl Pts',(-1.08147968809079,12.2,-11.0067966526415));
#300073=CARTESIAN_POINT('Ctrl Pts',(-1.08036914069759,12.2,-11.0108777090298));
#300074=CARTESIAN_POINT('Ctrl Pts',(-1.07924839501429,12.2,-11.0149702620389));
#300075=CARTESIAN_POINT('Ctrl Pts',(-1.07811740384087,12.2,-11.0190741998189));
#300076=CARTESIAN_POINT('Ctrl Pts',(-1.07698641282155,12.2,-11.0231781370397));
#300077=CARTESIAN_POINT('Ctrl Pts',(-1.07584517752686,12.2,-11.0272934596389));
#300078=CARTESIAN_POINT('Ctrl Pts',(-1.07469364917547,12.2,-11.0314200576179));
#300079=CARTESIAN_POINT('Ctrl Pts',(-1.07354212066718,12.2,-11.0355466561591));
#300080=CARTESIAN_POINT('Ctrl Pts',(-1.07238030022707,12.2,-11.0396845286402));
#300081=CARTESIAN_POINT('Ctrl Pts',(-1.07120814166251,12.2,-11.0438335670893));
#300082=CARTESIAN_POINT('Ctrl Pts',(-1.07003598325766,12.2,-11.047982604973));
#300083=CARTESIAN_POINT('Ctrl Pts',(-1.06885348792987,12.2,-11.0521428083879));
#300084=CARTESIAN_POINT('Ctrl Pts',(-1.06766060769512,12.2,-11.056314068268));
#300085=CARTESIAN_POINT('Ctrl Pts',(-1.06646772729784,12.2,-11.0604853287164));
#300086=CARTESIAN_POINT('Ctrl Pts',(-1.06526446461823,12.2,-11.0646676462495));
#300087=CARTESIAN_POINT('Ctrl Pts',(-1.06405077349099,12.2,-11.0688609120526));
#300088=CARTESIAN_POINT('Ctrl Pts',(-1.06283708252911,12.2,-11.0730541772845));
#300089=CARTESIAN_POINT('Ctrl Pts',(-1.0616129635194,12.2,-11.0772583904787));
#300090=CARTESIAN_POINT('Ctrl Pts',(-1.06037837367695,12.2,-11.0814734455775));
#300091=CARTESIAN_POINT('Ctrl Pts',(-1.05914378366628,12.2,-11.0856885012506));
#300092=CARTESIAN_POINT('Ctrl Pts',(-1.05789872042964,12.2,-11.0899143988024));
#300093=CARTESIAN_POINT('Ctrl Pts',(-1.0566431432501,12.2,-11.0941510300333));
#300094=CARTESIAN_POINT('Ctrl Pts',(-1.05538756607056,12.2,-11.0983876612642));
#300095=CARTESIAN_POINT('Ctrl Pts',(-1.05412147367313,12.2,-11.1026350272852));
#300096=CARTESIAN_POINT('Ctrl Pts',(-1.05284482382469,12.2,-11.1068930229628));
#300097=CARTESIAN_POINT('Ctrl Pts',(-1.05188733652533,12.2,-11.110086519431));
#300098=CARTESIAN_POINT('Ctrl Pts',(-1.05092391055972,12.2,-11.1132859934258));
#300099=CARTESIAN_POINT('Ctrl Pts',(-1.04995452829582,12.2,-11.1164914026369));
#300100=CARTESIAN_POINT('Ctrl Pts',(-1.04898514603192,12.2,-11.1196968118479));
#300101=CARTESIAN_POINT('Ctrl Pts',(-1.04800980859123,12.2,-11.1229081555005));
#300102=CARTESIAN_POINT('Ctrl Pts',(-1.04702849637637,12.2,-11.1261253890924));
#300103=CARTESIAN_POINT('Ctrl Pts',(-1.0460471841615,12.2,-11.1293426226844));
#300104=CARTESIAN_POINT('Ctrl Pts',(-1.04505989848068,12.2,-11.1325657464673));
#300105=CARTESIAN_POINT('Ctrl Pts',(-1.0440666217251,12.2,-11.135794716475));
#300106=CARTESIAN_POINT('Ctrl Pts',(-1.04307334496953,12.2,-11.1390236864826));
#300107=CARTESIAN_POINT('Ctrl Pts',(-1.04207407795586,12.2,-11.1422585019318));
#300108=CARTESIAN_POINT('Ctrl Pts',(-1.0410688026179,12.2,-11.1454991204385));
#300109=CARTESIAN_POINT('Ctrl Pts',(-1.04006352727995,12.2,-11.1487397389453));
#300110=CARTESIAN_POINT('Ctrl Pts',(-1.03905224281003,12.2,-11.1519861597272));
#300111=CARTESIAN_POINT('Ctrl Pts',(-1.03803493396353,12.2,-11.1552383398958));
#300112=CARTESIAN_POINT('Ctrl Pts',(-1.03667852204499,12.2,-11.1595745805146));
#300113=CARTESIAN_POINT('Ctrl Pts',(-1.03531139892148,12.2,-11.1639210583515));
#300114=CARTESIAN_POINT('Ctrl Pts',(-1.03393352634569,12.2,-11.1682776715896));
#300115=CARTESIAN_POINT('Ctrl Pts',(-1.03290012200771,12.2,-11.1715451312213));
#300116=CARTESIAN_POINT('Ctrl Pts',(-1.03186066979545,12.2,-11.1748182919858));
#300117=CARTESIAN_POINT('Ctrl Pts',(-1.0308151545001,12.2,-11.1780971109916));
#300118=CARTESIAN_POINT('Ctrl Pts',(-1.02976963920475,12.2,-11.1813759299975));
#300119=CARTESIAN_POINT('Ctrl Pts',(-1.02871806089299,12.2,-11.1846604057448));
#300120=CARTESIAN_POINT('Ctrl Pts',(-1.02766040264028,12.2,-11.1879504986248));
#300121=CARTESIAN_POINT('Ctrl Pts',(-1.02660274438757,12.2,-11.1912405915048));
#300122=CARTESIAN_POINT('Ctrl Pts',(-1.02553900620423,12.2,-11.1945362977003));
#300123=CARTESIAN_POINT('Ctrl Pts',(-1.02446917244036,12.2,-11.1978375779113));
#300124=CARTESIAN_POINT('Ctrl Pts',(-1.02339933867648,12.2,-11.2011388581223));
#300125=CARTESIAN_POINT('Ctrl Pts',(-1.02232340989583,12.2,-11.2044457113823));
#300126=CARTESIAN_POINT('Ctrl Pts',(-1.02124136872764,12.2,-11.2077580940112));
#300127=CARTESIAN_POINT('Ctrl Pts',(-1.02015932736289,12.2,-11.2110704772419));
#300128=CARTESIAN_POINT('Ctrl Pts',(-1.01907117593808,12.2,-11.2143883908241));
#300129=CARTESIAN_POINT('Ctrl Pts',(-1.01797689606987,12.2,-11.2177117920161));
#300130=CARTESIAN_POINT('Ctrl Pts',(-1.01688261640046,12.2,-11.2210351926045));
#300131=CARTESIAN_POINT('Ctrl Pts',(-1.01578220987305,12.2,-11.2243640805508));
#300132=CARTESIAN_POINT('Ctrl Pts',(-1.01467566112105,12.2,-11.2276984150968));
#300133=CARTESIAN_POINT('Ctrl Pts',(-1.01356911236905,12.2,-11.2310327496428));
#300134=CARTESIAN_POINT('Ctrl Pts',(-1.01245642023021,12.2,-11.234372529426));
#300135=CARTESIAN_POINT('Ctrl Pts',(-1.01133757097408,12.2,-11.237717713528));
#300136=CARTESIAN_POINT('Ctrl Pts',(-1.01021872171795,12.2,-11.24106289763));
#300137=CARTESIAN_POINT('Ctrl Pts',(-1.0090937146818,12.2,-11.2444134863703));
#300138=CARTESIAN_POINT('Ctrl Pts',(-1.00796253446779,12.2,-11.2477694365136));
#300139=CARTESIAN_POINT('Ctrl Pts',(-1.00683135425378,12.2,-11.2511253866569));
#300140=CARTESIAN_POINT('Ctrl Pts',(-1.00569400209922,12.2,-11.2544866990392));
#300141=CARTESIAN_POINT('Ctrl Pts',(-1.00455046143297,12.2,-11.2578533321664));
#300142=CARTESIAN_POINT('Ctrl Pts',(-1.00340692076673,12.2,-11.2612199652937));
#300143=CARTESIAN_POINT('Ctrl Pts',(-1.00225719315924,12.2,-11.2645919192038));
#300144=CARTESIAN_POINT('Ctrl Pts',(-1.00110126249375,12.2,-11.2679691532471));
#300145=CARTESIAN_POINT('Ctrl Pts',(-0.999945331618268,12.2,-11.2713463879039));
#300146=CARTESIAN_POINT('Ctrl Pts',(-0.998783197949374,12.2,-11.2747289010454));
#300147=CARTESIAN_POINT('Ctrl Pts',(-0.997614847945394,12.2,-11.2781166527468));
#300148=CARTESIAN_POINT('Ctrl Pts',(-0.996446498153665,12.2,-11.2815044038328));
#300149=CARTESIAN_POINT('Ctrl Pts',(-0.99527193062893,12.2,-11.2848973936268));
#300150=CARTESIAN_POINT('Ctrl Pts',(-0.99409113237962,12.2,-11.2882955811705));
#300151=CARTESIAN_POINT('Ctrl Pts',(-0.992910334130311,12.2,-11.2916937687141));
#300152=CARTESIAN_POINT('Ctrl Pts',(-0.991723304977775,12.2,-11.2950971526781));
#300153=CARTESIAN_POINT('Ctrl Pts',(-0.990530030224015,12.2,-11.2985056942781));
#300154=CARTESIAN_POINT('Ctrl Pts',(-0.988938997291261,12.2,-11.303050416205));
#300155=CARTESIAN_POINT('Ctrl Pts',(-0.987336860897517,12.2,-11.3076043045723));
#300156=CARTESIAN_POINT('Ctrl Pts',(-0.985723588697198,12.2,-11.3121672657539));
#300157=CARTESIAN_POINT('Ctrl Pts',(-0.98411031627707,12.2,-11.3167302275573));
#300158=CARTESIAN_POINT('Ctrl Pts',(-0.982485908194793,12.2,-11.3213022597531));
#300159=CARTESIAN_POINT('Ctrl Pts',(-0.980850330550103,12.2,-11.325883267725));
#300160=CARTESIAN_POINT('Ctrl Pts',(-0.979623647428009,12.2,-11.3293190233918));
#300161=CARTESIAN_POINT('Ctrl Pts',(-0.97839068277283,12.2,-11.3327598287168));
#300162=CARTESIAN_POINT('Ctrl Pts',(-0.97715142165174,12.2,-11.3362056423828));
#300163=CARTESIAN_POINT('Ctrl Pts',(-0.97591216053065,12.2,-11.3396514560488));
#300164=CARTESIAN_POINT('Ctrl Pts',(-0.974666603441903,12.2,-11.3431022787682));
#300165=CARTESIAN_POINT('Ctrl Pts',(-0.973414737175575,12.2,-11.3465580705648));
#300166=CARTESIAN_POINT('Ctrl Pts',(-0.972162870909247,12.2,-11.3500138623613));
#300167=CARTESIAN_POINT('Ctrl Pts',(-0.970904695512285,12.2,-11.3534746229377));
#300168=CARTESIAN_POINT('Ctrl Pts',(-0.969640197309087,12.2,-11.3569403125195));
#300169=CARTESIAN_POINT('Ctrl Pts',(-0.968375698876171,12.2,-11.3604060027308));
#300170=CARTESIAN_POINT('Ctrl Pts',(-0.967104878474818,12.2,-11.3638766210019));
#300171=CARTESIAN_POINT('Ctrl Pts',(-0.965827722496673,12.2,-11.3673521297576));
#300172=CARTESIAN_POINT('Ctrl Pts',(-0.964550566750545,12.2,-11.370827637882));
#300173=CARTESIAN_POINT('Ctrl Pts',(-0.963267074113089,12.2,-11.3743080363062));
#300174=CARTESIAN_POINT('Ctrl Pts',(-0.961977234867734,12.2,-11.37779328543));
#300175=CARTESIAN_POINT('Ctrl Pts',(-0.96068739562238,12.2,-11.3812785345537));
#300176=CARTESIAN_POINT('Ctrl Pts',(-0.959391207590864,12.2,-11.3847686341476));
#300177=CARTESIAN_POINT('Ctrl Pts',(-0.958088658423916,12.2,-11.3882635447448));
#300178=CARTESIAN_POINT('Ctrl Pts',(-0.956786109256967,12.2,-11.3917584553421));
#300179=CARTESIAN_POINT('Ctrl Pts',(-0.955477199409448,12.2,-11.3952581757582));
#300180=CARTESIAN_POINT('Ctrl Pts',(-0.95416191474296,12.2,-11.3987626660218));
#300181=CARTESIAN_POINT('Ctrl Pts',(-0.952846630076473,12.2,-11.4022671562854));
#300182=CARTESIAN_POINT('Ctrl Pts',(-0.951524971795942,12.2,-11.4057764180618));
#300183=CARTESIAN_POINT('Ctrl Pts',(-0.950196927678083,12.2,-11.4092904138504));
#300184=CARTESIAN_POINT('Ctrl Pts',(-0.948426202026765,12.2,-11.4139757419941));
#300185=CARTESIAN_POINT('Ctrl Pts',(-0.946644124846304,12.2,-11.4186694905582));
#300186=CARTESIAN_POINT('Ctrl Pts',(-0.944850667636712,12.2,-11.4233715650928));
#300187=CARTESIAN_POINT('Ctrl Pts',(-0.943505574851696,12.2,-11.4268981206734));
#300188=CARTESIAN_POINT('Ctrl Pts',(-0.942154079989061,12.2,-11.4304293588656));
#300189=CARTESIAN_POINT('Ctrl Pts',(-0.940796168282198,12.2,-11.4339652319615));
#300190=CARTESIAN_POINT('Ctrl Pts',(-0.939438256575334,12.2,-11.4375011050575));
#300191=CARTESIAN_POINT('Ctrl Pts',(-0.938073927574405,12.2,-11.4410416122428));
#300192=CARTESIAN_POINT('Ctrl Pts',(-0.936703170534677,12.2,-11.4445867182134));
#300193=CARTESIAN_POINT('Ctrl Pts',(-0.934418575385458,12.2,-11.4504952283791));
#300194=CARTESIAN_POINT('Ctrl Pts',(-0.932116123684424,12.2,-11.4564165140663));
#300195=CARTESIAN_POINT('Ctrl Pts',(-0.929795809339219,12.2,-11.4623505331326));
#300196=CARTESIAN_POINT('Origin',(-5.66257110645729E-14,15.4,-1.77635683940025E-14));
#300197=CARTESIAN_POINT('',(-3.28892417320473,12.2,-1.19707050039253));
#300198=CARTESIAN_POINT('',(-3.28892417320473,15.4,-1.19707050039253));
#300199=CARTESIAN_POINT('Origin',(-5.66257110645729E-14,12.2,-1.77635683940025E-14));
#300200=CARTESIAN_POINT('Origin',(2.60871324108541E-9,12.2,-1.77635683940025E-14));
#300201=CARTESIAN_POINT('Origin',(-5.66300478732629E-14,15.4,-1.77635683940025E-14));
#300202=CARTESIAN_POINT('',(1.49999999999995,17.9,-1.77635683940025E-14));
#300203=CARTESIAN_POINT('Origin',(-5.55198248486377E-14,17.9,-1.77635683940025E-14));
#300204=CARTESIAN_POINT('',(1.49999999999994,15.4,-1.79472654138746E-14));
#300205=CARTESIAN_POINT('',(1.49999999999994,15.4,-1.79472654138746E-14));
#300206=CARTESIAN_POINT('Origin',(-5.66300478732629E-14,15.4,-1.77635683940025E-14));
#300207=CARTESIAN_POINT('Origin',(-5.66300478732629E-14,15.4,-1.77635683940025E-14));
#300208=CARTESIAN_POINT('',(1.49999999999994,2.4,-1.91719121435528E-14));
#300209=CARTESIAN_POINT('Origin',(-6.24032076013137E-14,2.4,-1.93556091634249E-14));
#300210=CARTESIAN_POINT('',(1.49999999999994,-0.100000000000001,-1.11022302462516E-14));
#300211=CARTESIAN_POINT('',(1.49999999999994,15.4,-1.79472654138746E-14));
#300212=CARTESIAN_POINT('Origin',(-6.4401609045639E-14,-0.100000000000001,
-1.11022302462516E-14));
#300213=CARTESIAN_POINT('Origin',(-6.4401609045639E-14,-0.100000000000001,
-1.11022302462516E-14));
#300214=CARTESIAN_POINT('Origin',(-5.55198248486377E-14,17.9,-1.77635683940025E-14));
#300215=CARTESIAN_POINT('Origin',(-5.66300478732629E-14,12.2,-1.77635683940025E-14));
#300216=CARTESIAN_POINT('',(1.33499935591029,12.2,-3.76399246382145));
#300217=CARTESIAN_POINT('',(1.21174315076912,12.2,-3.41647530879655));
#300218=CARTESIAN_POINT('',(1.33499941799994,12.2,-3.76399244200002));
#300219=CARTESIAN_POINT('',(0.669813182999944,12.2,-3.56257986500002));
#300220=CARTESIAN_POINT('Origin',(-5.66300478732629E-14,12.2,-1.77635683940025E-14));
#300221=CARTESIAN_POINT('',(0.737948320677355,12.2,-3.92497529182648));
#300222=CARTESIAN_POINT('',(0.669813182999944,12.2,-3.56257986500002));
#300223=CARTESIAN_POINT('',(0.540411127999944,12.2,-4.71915837900001));
#300224=CARTESIAN_POINT('Ctrl Pts',(0.737948221040922,12.2,-3.92497531022196));
#300225=CARTESIAN_POINT('Ctrl Pts',(0.738035737340575,12.2,-3.92544932936902));
#300226=CARTESIAN_POINT('Ctrl Pts',(0.738181018754199,12.2,-3.92631728138919));
#300227=CARTESIAN_POINT('Ctrl Pts',(0.738670587243213,12.2,-3.92956818688039));
#300228=CARTESIAN_POINT('Ctrl Pts',(0.738954729183831,12.1999999999079,
-3.93174223113599));
#300229=CARTESIAN_POINT('Ctrl Pts',(0.740093274189603,12.1999999999079,
-3.94128424531577));
#300230=CARTESIAN_POINT('Ctrl Pts',(0.740740501657956,12.1999999999079,
-3.94930810735695));
#300231=CARTESIAN_POINT('Ctrl Pts',(0.742798149505974,12.1999999999079,
-3.98426650826332));
#300232=CARTESIAN_POINT('Ctrl Pts',(0.742372759528698,12.2,-4.01357561888738));
#300233=CARTESIAN_POINT('Ctrl Pts',(0.736437186727589,12.2,-4.119388050933));
#300234=CARTESIAN_POINT('Ctrl Pts',(0.721506350180841,12.2,-4.21805492592019));
#300235=CARTESIAN_POINT('Ctrl Pts',(0.653099662777896,12.2,-4.46559806981985));
#300236=CARTESIAN_POINT('Ctrl Pts',(0.601738439484085,12.2,-4.59476663244512));
#300237=CARTESIAN_POINT('Ctrl Pts',(0.540411128396557,12.2,-4.71915837919555));
#300238=CARTESIAN_POINT('',(0.204481245999943,12.2,-4.74559663400001));
#300239=CARTESIAN_POINT('Origin',(-5.66300478732629E-14,12.2,-1.77635683940025E-14));
#300240=CARTESIAN_POINT('',(-0.114861198664522,12.2,-3.99208010934835));
#300241=CARTESIAN_POINT('Ctrl Pts',(0.204481245999943,12.2,-4.74559663400001));
#300242=CARTESIAN_POINT('Ctrl Pts',(0.172553443581559,12.2,-4.7004103209369));
#300243=CARTESIAN_POINT('Ctrl Pts',(0.143344934273432,12.2,-4.65597464923193));
#300244=CARTESIAN_POINT('Ctrl Pts',(0.116780339324946,12.2,-4.61263536275873));
#300245=CARTESIAN_POINT('Ctrl Pts',(0.089774485485458,12.2,-4.56857617652711));
#300246=CARTESIAN_POINT('Ctrl Pts',(0.0655014911131988,12.2,-4.52565083217712));
#300247=CARTESIAN_POINT('Ctrl Pts',(0.0438412949943011,12.2,-4.48424707603364));
#300248=CARTESIAN_POINT('Ctrl Pts',(0.0230828477657351,12.2,-4.44456702501974));
#300249=CARTESIAN_POINT('Ctrl Pts',(0.00472433924867187,12.2000000000001,
-4.40628451809031));
#300250=CARTESIAN_POINT('Ctrl Pts',(-0.0113809795912018,12.2,-4.36976156125905));
#300251=CARTESIAN_POINT('Ctrl Pts',(-0.0270142158296342,12.1999999999999,
-4.33430917326561));
#300252=CARTESIAN_POINT('Ctrl Pts',(-0.0405241706954382,12.2,-4.30051460941323));
#300253=CARTESIAN_POINT('Ctrl Pts',(-0.0520879448806814,12.2,-4.26872928236361));
#300254=CARTESIAN_POINT('Ctrl Pts',(-0.06314037611749,12.2,-4.23834948283383));
#300255=CARTESIAN_POINT('Ctrl Pts',(-0.0724147466109138,12.2,-4.20980510629708));
#300256=CARTESIAN_POINT('Ctrl Pts',(-0.0801088059519884,12.2,-4.18342243520099));
#300257=CARTESIAN_POINT('Ctrl Pts',(-0.0874725000263822,12.2,-4.15817257550991));
#300258=CARTESIAN_POINT('Ctrl Pts',(-0.0933884292815516,12.1999999999999,
-4.13490270492306));
#300259=CARTESIAN_POINT('Ctrl Pts',(-0.0980736177886704,12.2,-4.11391792531568));
#300260=CARTESIAN_POINT('Ctrl Pts',(-0.102420051223164,12.2000000000001,
-4.09445041668451));
#300261=CARTESIAN_POINT('Ctrl Pts',(-0.105707231633019,12.2,-4.07694951907395));
#300262=CARTESIAN_POINT('Ctrl Pts',(-0.108148552352073,12.2,-4.06167605561997));
#300263=CARTESIAN_POINT('Ctrl Pts',(-0.110505994223923,12.2,-4.04692735751014));
#300264=CARTESIAN_POINT('Ctrl Pts',(-0.112074334131715,12.1999999999999,
-4.03425550678305));
#300265=CARTESIAN_POINT('Ctrl Pts',(-0.113087970038994,12.2,-4.02391341293629));
#300266=CARTESIAN_POINT('Ctrl Pts',(-0.114055851981257,12.2000000000001,
-4.01403814529079));
#300267=CARTESIAN_POINT('Ctrl Pts',(-0.114517612985473,12.2,-4.00628689124919));
#300268=CARTESIAN_POINT('Ctrl Pts',(-0.114721610728504,12.2,-4.0008988960201));
#300269=CARTESIAN_POINT('Ctrl Pts',(-0.11482360960002,12.2,-3.99820489840556));
#300270=CARTESIAN_POINT('Ctrl Pts',(-0.114861911538468,12.2,-3.99610203167409));
#300271=CARTESIAN_POINT('Ctrl Pts',(-0.114872546484935,12.2,-3.99462238128286));
#300272=CARTESIAN_POINT('Ctrl Pts',(-0.114877863958168,12.2,-3.99388255608725));
#300273=CARTESIAN_POINT('Ctrl Pts',(-0.11487632054625,12.2,-3.99329856060513));
#300274=CARTESIAN_POINT('Ctrl Pts',(-0.11487279171893,12.2,-3.99287456748994));
#300275=CARTESIAN_POINT('Ctrl Pts',(-0.114871027305269,12.2,-3.99266257093235));
#300276=CARTESIAN_POINT('Ctrl Pts',(-0.114868725248524,12.2,-3.99249054033208));
#300277=CARTESIAN_POINT('Ctrl Pts',(-0.114866622243977,12.2,-3.99235909393692));
#300278=CARTESIAN_POINT('Ctrl Pts',(-0.114865070454561,12.2,-3.99226210074452));
#300279=CARTESIAN_POINT('Ctrl Pts',(-0.114863611222235,12.2,-3.99218545762677));
#300280=CARTESIAN_POINT('Ctrl Pts',(-0.114862439806823,12.2,-3.99213426766888));
#300281=CARTESIAN_POINT('Ctrl Pts',(-0.114862023705324,12.2,-3.99211608435154));
#300282=CARTESIAN_POINT('Ctrl Pts',(-0.1148616317576,12.2,-3.99210051805137));
#300283=CARTESIAN_POINT('Ctrl Pts',(-0.11486123084618,12.2,-3.99208443600385));
#300284=CARTESIAN_POINT('',(-0.104256396000055,12.2,-3.62350046200001));
#300285=CARTESIAN_POINT('',(-0.114861017000055,12.2,-3.99207578600001));
#300286=CARTESIAN_POINT('',(-0.662370095000057,12.2,-3.56397122000002));
#300287=CARTESIAN_POINT('Origin',(-5.66300478732629E-14,12.2,-1.77635683940025E-14));
#300288=CARTESIAN_POINT('',(-0.729748298404982,12.2,-3.92650814146157));
#300289=CARTESIAN_POINT('',(-0.662370095000057,12.2,-3.56397122000002));
#300290=CARTESIAN_POINT('',(-1.20083826600006,12.2,-4.59570315100001));
#300291=CARTESIAN_POINT('Ctrl Pts',(-0.729748397137909,12.2,-3.92650812272649));
#300292=CARTESIAN_POINT('Ctrl Pts',(-0.729798979329332,12.2,-3.92677468824178));
#300293=CARTESIAN_POINT('Ctrl Pts',(-0.729853590824242,12.1999999999997,
-3.92704048095005));
#300294=CARTESIAN_POINT('Ctrl Pts',(-0.730025582708951,12.1999999999997,
-3.92786938784101));
#300295=CARTESIAN_POINT('Ctrl Pts',(-0.730155150278449,12.2,-3.92846502942454));
#300296=CARTESIAN_POINT('Ctrl Pts',(-0.730733246668206,12.2,-3.93104867134671));
#300297=CARTESIAN_POINT('Ctrl Pts',(-0.731253196319109,12.1999999999077,
-3.93317718551181));
#300298=CARTESIAN_POINT('Ctrl Pts',(-0.733639815031661,12.1999999999077,
-3.94249120885481));
#300299=CARTESIAN_POINT('Ctrl Pts',(-0.735934859520536,12.1999999999077,
-3.95020698257531));
#300300=CARTESIAN_POINT('Ctrl Pts',(-0.746644516032087,12.1999999999077,
-3.98354780293642));
#300301=CARTESIAN_POINT('Ctrl Pts',(-0.757632863640905,12.2,-4.01073278352797));
#300302=CARTESIAN_POINT('Ctrl Pts',(-0.801179313012322,12.2,-4.10678792979713));
#300303=CARTESIAN_POINT('Ctrl Pts',(-0.850601354606886,12.2,-4.19338450992101));
#300304=CARTESIAN_POINT('Ctrl Pts',(-1.00417815028429,12.2,-4.39999394708107));
#300305=CARTESIAN_POINT('Ctrl Pts',(-1.09878737824146,12.2,-4.50193041233648));
#300306=CARTESIAN_POINT('Ctrl Pts',(-1.20083826600006,12.2,-4.59570315100001));
#300307=CARTESIAN_POINT('',(-1.5236341523253,12.2,-4.49900421997614));
#300308=CARTESIAN_POINT('Origin',(-5.66300478732629E-14,12.2,-1.77635683940025E-14));
#300309=CARTESIAN_POINT('',(-1.54921060157246,12.2,-3.68101131236159));
#300310=CARTESIAN_POINT('Ctrl Pts',(-1.52363415300006,12.2,-4.49900422000002));
#300311=CARTESIAN_POINT('Ctrl Pts',(-1.53068793708627,12.2,-4.47085469189399));
#300312=CARTESIAN_POINT('Ctrl Pts',(-1.53711977389706,12.2,-4.4431686191827));
#300313=CARTESIAN_POINT('Ctrl Pts',(-1.54295573603177,12.2,-4.41598726777904));
#300314=CARTESIAN_POINT('Ctrl Pts',(-1.55441407633895,12.2,-4.36261934536915));
#300315=CARTESIAN_POINT('Ctrl Pts',(-1.56357351051339,12.2,-4.3111985843265));
#300316=CARTESIAN_POINT('Ctrl Pts',(-1.57067315083765,12.2,-4.26205308021928));
#300317=CARTESIAN_POINT('Ctrl Pts',(-1.57747688850023,12.2,-4.21495588909847));
#300318=CARTESIAN_POINT('Ctrl Pts',(-1.58238883909617,12.1999999999999,
-4.16994832068129));
#300319=CARTESIAN_POINT('Ctrl Pts',(-1.58566442677365,12.2,-4.127324038995));
#300320=CARTESIAN_POINT('Ctrl Pts',(-1.58883259252429,12.2,-4.0860976079907));
#300321=CARTESIAN_POINT('Ctrl Pts',(-1.59046974502133,12.2,-4.04710078678771));
#300322=CARTESIAN_POINT('Ctrl Pts',(-1.59085264474885,12.2,-4.01060305274178));
#300323=CARTESIAN_POINT('Ctrl Pts',(-1.59122369863281,12.2,-3.97523445621444));
#300324=CARTESIAN_POINT('Ctrl Pts',(-1.59041660073962,12.2,-3.94221277590855));
#300325=CARTESIAN_POINT('Ctrl Pts',(-1.58873062606297,12.2,-3.911786232773));
#300326=CARTESIAN_POINT('Ctrl Pts',(-1.58714775742718,12.2,-3.88322042956623));
#300327=CARTESIAN_POINT('Ctrl Pts',(-1.58479013109599,12.2,-3.85694208153543));
#300328=CARTESIAN_POINT('Ctrl Pts',(-1.58195002843682,12.2,-3.83315875411321));
#300329=CARTESIAN_POINT('Ctrl Pts',(-1.57910981659426,12.2,-3.80937451237743));
#300330=CARTESIAN_POINT('Ctrl Pts',(-1.57578641439816,12.1999999999999,
-3.7880854732337));
#300331=CARTESIAN_POINT('Ctrl Pts',(-1.5723245407617,12.2,-3.7695012212912));
#300332=CARTESIAN_POINT('Ctrl Pts',(-1.56921114460368,12.2000000000001,
-3.75278768848402));
#300333=CARTESIAN_POINT('Ctrl Pts',(-1.56598590621646,12.2,-3.73826182817511));
#300334=CARTESIAN_POINT('Ctrl Pts',(-1.56294413362489,12.2,-3.72607762949063));
#300335=CARTESIAN_POINT('Ctrl Pts',(-1.56002764522756,12.2,-3.71439527223861));
#300336=CARTESIAN_POINT('Ctrl Pts',(-1.55727941358539,12.2,-3.70486562365225));
#300337=CARTESIAN_POINT('Ctrl Pts',(-1.5550051743708,12.2,-3.69762600726247));
#300338=CARTESIAN_POINT('Ctrl Pts',(-1.55337212957192,12.2,-3.69242751371117));
#300339=CARTESIAN_POINT('Ctrl Pts',(-1.55198432092636,12.2,-3.6884098225594));
#300340=CARTESIAN_POINT('Ctrl Pts',(-1.55097251090944,12.2,-3.68562445599079));
#300341=CARTESIAN_POINT('Ctrl Pts',(-1.55046660590099,12.2,-3.68423177270649));
#300342=CARTESIAN_POINT('Ctrl Pts',(-1.55005495419322,12.2,-3.68314718213396));
#300343=CARTESIAN_POINT('Ctrl Pts',(-1.54975552508367,12.2,-3.68237719584491));
#300344=CARTESIAN_POINT('Ctrl Pts',(-1.5496058105289,12.2,-3.68199220270039));
#300345=CARTESIAN_POINT('Ctrl Pts',(-1.54948420123509,12.2,-3.68168586978067));
#300346=CARTESIAN_POINT('Ctrl Pts',(-1.54939298287873,12.2,-3.68145899258006));
#300347=CARTESIAN_POINT('Ctrl Pts',(-1.54933878915026,12.2,-3.68132420258933));
#300348=CARTESIAN_POINT('Ctrl Pts',(-1.54929551285811,12.2,-3.68121780149236));
#300349=CARTESIAN_POINT('Ctrl Pts',(-1.54926322330182,12.2,-3.68113891519218));
#300350=CARTESIAN_POINT('Ctrl Pts',(-1.54924619322756,12.2,-3.68109730918379));
#300351=CARTESIAN_POINT('Ctrl Pts',(-1.54923273601866,12.2,-3.68106468916976));
#300352=CARTESIAN_POINT('Ctrl Pts',(-1.54922180885574,12.2,-3.68103843225446));
#300353=CARTESIAN_POINT('Ctrl Pts',(-1.54921858151565,12.2,-3.68103067726846));
#300354=CARTESIAN_POINT('Ctrl Pts',(-1.54921541865686,12.2,-3.68102308221307));
#300355=CARTESIAN_POINT('Ctrl Pts',(-1.54921224493634,12.2,-3.68101546102655));
#300356=CARTESIAN_POINT('',(-1.40617553966606,12.2,-3.34115179986312));
#300357=CARTESIAN_POINT('',(-1.54920881800006,12.2,-3.68100722300001));
#300358=CARTESIAN_POINT('',(-1.90509662000005,12.2,-3.08402851200002));
#300359=CARTESIAN_POINT('Origin',(-5.66300478732629E-14,12.2,-1.77635683940025E-14));
#300360=CARTESIAN_POINT('',(-2.0988883662473,12.2,-3.39774430965258));
#300361=CARTESIAN_POINT('',(-1.90509662000005,12.2,-3.08402851200002));
#300362=CARTESIAN_POINT('',(-2.77990780000006,12.2,-3.85157274700001));
#300363=CARTESIAN_POINT('Ctrl Pts',(-2.09888845211281,12.2,-3.39774425618107));
#300364=CARTESIAN_POINT('Ctrl Pts',(-2.09903187832741,12.2,-3.39797457253771));
#300365=CARTESIAN_POINT('Ctrl Pts',(-2.09917885578644,12.1999999999997,
-3.39820266771551));
#300366=CARTESIAN_POINT('Ctrl Pts',(-2.09963895812251,12.1999999999997,
-3.39891392611081));
#300367=CARTESIAN_POINT('Ctrl Pts',(-2.09997452956103,12.2,-3.39942189887948));
#300368=CARTESIAN_POINT('Ctrl Pts',(-2.1014481628405,12.2,-3.40162410246599));
#300369=CARTESIAN_POINT('Ctrl Pts',(-2.10270249498751,12.1999999999079,
-3.40342177907669));
#300370=CARTESIAN_POINT('Ctrl Pts',(-2.10829027509302,12.1999999999079,
-3.41124149475554));
#300371=CARTESIAN_POINT('Ctrl Pts',(-2.11321950204324,12.1999999999079,
-3.41760963109163));
#300372=CARTESIAN_POINT('Ctrl Pts',(-2.13524297057016,12.1999999999079,
-3.44482145366327));
#300373=CARTESIAN_POINT('Ctrl Pts',(-2.15530017599741,12.2,-3.46619350428762));
#300374=CARTESIAN_POINT('Ctrl Pts',(-2.23100372376674,12.2,-3.54042209052579));
#300375=CARTESIAN_POINT('Ctrl Pts',(-2.30852269436843,12.2,-3.6032793024282));
#300376=CARTESIAN_POINT('Ctrl Pts',(-2.52588006333986,12.2,-3.74015282700682));
#300377=CARTESIAN_POINT('Ctrl Pts',(-2.65150240933442,12.2,-3.80124396329853));
#300378=CARTESIAN_POINT('Ctrl Pts',(-2.77990780000006,12.2,-3.85157274700001));
#300379=CARTESIAN_POINT('',(-3.04597431500006,12.2,-3.64479635500001));
#300380=CARTESIAN_POINT('Origin',(-5.66300478732629E-14,12.2,-1.77635683940025E-14));
#300381=CARTESIAN_POINT('',(-2.77433052545124,12.2,-2.87280140881169));
#300382=CARTESIAN_POINT('Ctrl Pts',(-3.04597431500006,12.2,-3.64479635500001));
#300383=CARTESIAN_POINT('Ctrl Pts',(-3.04202932086791,12.2,-3.61316355471933));
#300384=CARTESIAN_POINT('Ctrl Pts',(-3.03758633189924,12.2,-3.5823231881441));
#300385=CARTESIAN_POINT('Ctrl Pts',(-3.03269790848834,12.2,-3.55231409881095));
#300386=CARTESIAN_POINT('Ctrl Pts',(-3.02400453989956,12.2,-3.49894718423372));
#300387=CARTESIAN_POINT('Ctrl Pts',(-3.01390127476584,12.2,-3.44821094171571));
#300388=CARTESIAN_POINT('Ctrl Pts',(-3.0027266806269,12.2,-3.4003210931824));
#300389=CARTESIAN_POINT('Ctrl Pts',(-2.991920980653,12.2,-3.35401217774325));
#300390=CARTESIAN_POINT('Ctrl Pts',(-2.98011337707264,12.1999999999999,
-3.31036493482041));
#300391=CARTESIAN_POINT('Ctrl Pts',(-2.96765450987006,12.2,-3.26956247204393));
#300392=CARTESIAN_POINT('Ctrl Pts',(-2.95566474553295,12.2000000000001,
-3.2302963088279));
#300393=CARTESIAN_POINT('Ctrl Pts',(-2.94307169437058,12.2,-3.19366484089195));
#300394=CARTESIAN_POINT('Ctrl Pts',(-2.93023205633515,12.2,-3.15981818093772));
#300395=CARTESIAN_POINT('Ctrl Pts',(-2.91788975284348,12.2,-3.12728254806535));
#300396=CARTESIAN_POINT('Ctrl Pts',(-2.90531940526358,12.2,-3.09732026810663));
#300397=CARTESIAN_POINT('Ctrl Pts',(-2.89288201802745,12.2,-3.07005062301657));
#300398=CARTESIAN_POINT('Ctrl Pts',(-2.88095667512664,12.2,-3.04390366286261));
#300399=CARTESIAN_POINT('Ctrl Pts',(-2.869153369637,12.2,-3.02023230347142));
#300400=CARTESIAN_POINT('Ctrl Pts',(-2.85783471947781,12.2,-2.99912683090921));
#300401=CARTESIAN_POINT('Ctrl Pts',(-2.84681464370975,12.2,-2.97857809908297));
#300402=CARTESIAN_POINT('Ctrl Pts',(-2.83625357808533,12.2,-2.9604618568326));
#300403=CARTESIAN_POINT('Ctrl Pts',(-2.82653408044394,12.2,-2.94484495350539));
#300404=CARTESIAN_POINT('Ctrl Pts',(-2.81760443123926,12.2,-2.93049714732027));
#300405=CARTESIAN_POINT('Ctrl Pts',(-2.80938510198816,12.2,-2.91825898115459));
#300406=CARTESIAN_POINT('Ctrl Pts',(-2.80221596360782,12.2,-2.90816727129479));
#300407=CARTESIAN_POINT('Ctrl Pts',(-2.79537498136305,12.2,-2.89853749372491));
#300408=CARTESIAN_POINT('Ctrl Pts',(-2.78948989273483,12.2,-2.89086226716769));
#300409=CARTESIAN_POINT('Ctrl Pts',(-2.78489987364489,12.2,-2.88515831797985));
#300410=CARTESIAN_POINT('Ctrl Pts',(-2.78174647474832,12.2,-2.88123963556861));
#300411=CARTESIAN_POINT('Ctrl Pts',(-2.77920517936183,12.2,-2.87825107637023));
#300412=CARTESIAN_POINT('Ctrl Pts',(-2.77740054731802,12.2,-2.87619306749039));
#300413=CARTESIAN_POINT('Ctrl Pts',(-2.77649823129612,12.2,-2.87516406305046));
#300414=CARTESIAN_POINT('Ctrl Pts',(-2.77578028206434,12.2,-2.87436762379733));
#300415=CARTESIAN_POINT('Ctrl Pts',(-2.77526359373549,12.2,-2.87380336028058));
#300416=CARTESIAN_POINT('Ctrl Pts',(-2.77500524957107,12.2,-2.8735212285222));
#300417=CARTESIAN_POINT('Ctrl Pts',(-2.77479725418726,12.2,-2.87329713551082));
#300418=CARTESIAN_POINT('Ctrl Pts',(-2.77464175442408,12.2,-2.87313100117707));
#300419=CARTESIAN_POINT('Ctrl Pts',(-2.77454713595653,12.2,-2.87302991178797));
#300420=CARTESIAN_POINT('Ctrl Pts',(-2.77447240241418,12.2,-2.87295067082362));
#300421=CARTESIAN_POINT('Ctrl Pts',(-2.77441676535422,12.2,-2.87289196756005));
#300422=CARTESIAN_POINT('Ctrl Pts',(-2.77438698189278,12.2,-2.87286054270784));
#300423=CARTESIAN_POINT('Ctrl Pts',(-2.77436463441682,12.2,-2.87283711775074));
#300424=CARTESIAN_POINT('Ctrl Pts',(-2.77434525405922,12.2,-2.87281688981085));
#300425=CARTESIAN_POINT('Ctrl Pts',(-2.77434133962869,12.2,-2.87281280418626));
#300426=CARTESIAN_POINT('Ctrl Pts',(-2.77433745035311,12.2,-2.87280874625328));
#300427=CARTESIAN_POINT('Ctrl Pts',(-2.77433355875055,12.2,-2.87280468523913));
#300428=CARTESIAN_POINT('',(-2.51818288326644,12.2,-2.6075620736151));
#300429=CARTESIAN_POINT('',(-2.77432738300006,12.2,-2.87279823700001));
#300430=CARTESIAN_POINT('',(-2.89052929200006,12.2,-2.18757066500002));
#300431=CARTESIAN_POINT('Origin',(-5.66300478732629E-14,12.2,-1.77635683940025E-14));
#300432=CARTESIAN_POINT('',(-3.18456193007282,12.2,-2.41009628089888));
#300433=CARTESIAN_POINT('',(-2.89052929200006,12.2,-2.18757066500002));
#300434=CARTESIAN_POINT('',(-3.98353538000006,12.2,-2.58726610100001));
#300435=CARTESIAN_POINT('Ctrl Pts',(-3.18456199052765,12.2,-2.41009620039622));
#300436=CARTESIAN_POINT('Ctrl Pts',(-3.1847789483277,12.2,-2.41025912851954));
#300437=CARTESIAN_POINT('Ctrl Pts',(-3.18499837884731,12.1999999999997,
-2.41041875026477));
#300438=CARTESIAN_POINT('Ctrl Pts',(-3.18568371131526,12.1999999999997,
-2.41091530622894));
#300439=CARTESIAN_POINT('Ctrl Pts',(-3.18618024732525,12.2,-2.41126785644461));
#300440=CARTESIAN_POINT('Ctrl Pts',(-3.18834989044632,12.2,-2.41278901397985));
#300441=CARTESIAN_POINT('Ctrl Pts',(-3.19016802488907,12.1999999999079,
-2.41401161234104));
#300442=CARTESIAN_POINT('Ctrl Pts',(-3.19820687861432,12.1999999999079,
-2.41928710817222));
#300443=CARTESIAN_POINT('Ctrl Pts',(-3.20510075911968,12.1999999999079,
-2.42344270161732));
#300444=CARTESIAN_POINT('Ctrl Pts',(-3.23547872372625,12.1999999999079,
-2.44086791092227));
#300445=CARTESIAN_POINT('Ctrl Pts',(-3.26191056113451,12.2,-2.45355331330479));
#300446=CARTESIAN_POINT('Ctrl Pts',(-3.35901835635599,12.2,-2.49529406440199));
#300447=CARTESIAN_POINT('Ctrl Pts',(-3.45393334803369,12.2,-2.52595419545077));
#300448=CARTESIAN_POINT('Ctrl Pts',(-3.70638249798277,12.2,-2.57512980517529));
#300449=CARTESIAN_POINT('Ctrl Pts',(-3.84524313000394,12.2,-2.58671966873636));
#300450=CARTESIAN_POINT('Ctrl Pts',(-3.98353538000006,12.2,-2.58726610100001));
#300451=CARTESIAN_POINT('',(-4.15693876900006,12.2,-2.29833854600002));
#300452=CARTESIAN_POINT('Origin',(-5.66300478732629E-14,12.2,-1.77635683940025E-14));
#300453=CARTESIAN_POINT('',(-3.62476174783278,12.2,-1.676603759906));
#300454=CARTESIAN_POINT('Ctrl Pts',(-4.15693876900006,12.2,-2.29833854600002));
#300455=CARTESIAN_POINT('Ctrl Pts',(-4.14220958485318,12.2,-2.27096656816286));
#300456=CARTESIAN_POINT('Ctrl Pts',(-4.12731111776242,12.2,-2.24446827238719));
#300457=CARTESIAN_POINT('Ctrl Pts',(-4.11230167253419,12.2,-2.21885949074597));
#300458=CARTESIAN_POINT('Ctrl Pts',(-4.08477741829449,12.2,-2.17189822029633));
#300459=CARTESIAN_POINT('Ctrl Pts',(-4.05687943548038,12.2,-2.12793053560342));
#300460=CARTESIAN_POINT('Ctrl Pts',(-4.02900743847548,12.2,-2.08703684650124));
#300461=CARTESIAN_POINT('Ctrl Pts',(-4.00217614217277,12.2,-2.04767006955237));
#300462=CARTESIAN_POINT('Ctrl Pts',(-3.97536882407247,12.2,-2.01115220162154));
#300463=CARTESIAN_POINT('Ctrl Pts',(-3.94897945960632,12.2,-1.97752765018928));
#300464=CARTESIAN_POINT('Ctrl Pts',(-3.92350771750221,12.2,-1.94507230616052));
#300465=CARTESIAN_POINT('Ctrl Pts',(-3.89842521272531,12.2,-1.9153127559376));
#300466=CARTESIAN_POINT('Ctrl Pts',(-3.87412319315574,12.2,-1.88826042636132));
#300467=CARTESIAN_POINT('Ctrl Pts',(-3.85061722051365,12.2,-1.86209423399593));
#300468=CARTESIAN_POINT('Ctrl Pts',(-3.8278412423737,12.2,-1.83846102204754));
#300469=CARTESIAN_POINT('Ctrl Pts',(-3.80618677108186,12.2,-1.81734097964565));
#300470=CARTESIAN_POINT('Ctrl Pts',(-3.78529621739538,12.2,-1.79696600148473));
#300471=CARTESIAN_POINT('Ctrl Pts',(-3.76544921024321,12.2,-1.77893023451589));
#300472=CARTESIAN_POINT('Ctrl Pts',(-3.74703567838489,12.2,-1.76318404897607));
#300473=CARTESIAN_POINT('Ctrl Pts',(-3.72949948546344,12.2,-1.74818811286084));
#300474=CARTESIAN_POINT('Ctrl Pts',(-3.71326322431709,12.2,-1.73526896265244));
#300475=CARTESIAN_POINT('Ctrl Pts',(-3.69870203620881,12.2,-1.72435135611523));
#300476=CARTESIAN_POINT('Ctrl Pts',(-3.68525234134329,12.2,-1.71426711879234));
#300477=CARTESIAN_POINT('Ctrl Pts',(-3.67323171741993,12.2,-1.70589056673568));
#300478=CARTESIAN_POINT('Ctrl Pts',(-3.66297061081925,12.2,-1.69913275840808));
#300479=CARTESIAN_POINT('Ctrl Pts',(-3.6531381669103,12.2,-1.69265726079223));
#300480=CARTESIAN_POINT('Ctrl Pts',(-3.6449209883424,12.2,-1.68766836640196));
#300481=CARTESIAN_POINT('Ctrl Pts',(-3.63864585579863,12.2,-1.68405720735998));
#300482=CARTESIAN_POINT('Ctrl Pts',(-3.63442292860184,12.2,-1.68162703371441));
#300483=CARTESIAN_POINT('Ctrl Pts',(-3.63108021443716,12.2,-1.67982022145482));
#300484=CARTESIAN_POINT('Ctrl Pts',(-3.62872851541058,12.2,-1.6785941477588));
#300485=CARTESIAN_POINT('Ctrl Pts',(-3.62755266589729,12.2,-1.67798111091079));
#300486=CARTESIAN_POINT('Ctrl Pts',(-3.62662472212591,12.2,-1.67751313883082));
#300487=CARTESIAN_POINT('Ctrl Pts',(-3.62595954395709,12.2,-1.67718405449576));
#300488=CARTESIAN_POINT('Ctrl Pts',(-3.62562695487268,12.2,-1.67701951232824));
#300489=CARTESIAN_POINT('Ctrl Pts',(-3.62536007978653,12.2,-1.67688967842754));
#300490=CARTESIAN_POINT('Ctrl Pts',(-3.62516080538803,12.2,-1.67679374434236));
#300491=CARTESIAN_POINT('Ctrl Pts',(-3.62503846121203,12.2,-1.67673484577491));
#300492=CARTESIAN_POINT('Ctrl Pts',(-3.62494219413518,12.2,-1.67668893681862));
#300493=CARTESIAN_POINT('Ctrl Pts',(-3.62487062783168,12.2,-1.67665503599103));
#300494=CARTESIAN_POINT('Ctrl Pts',(-3.62483104884004,12.2,-1.67663628749479));
#300495=CARTESIAN_POINT('Ctrl Pts',(-3.62480232555704,12.2,-1.67662280367348));
#300496=CARTESIAN_POINT('Ctrl Pts',(-3.62477640670851,12.2,-1.67661069179204));
#300497=CARTESIAN_POINT('Ctrl Pts',(-3.62477285602412,12.2,-1.67660903255675));
#300498=CARTESIAN_POINT('Ctrl Pts',(-3.62476931425303,12.2,-1.6766073779349));
#300499=CARTESIAN_POINT('Ctrl Pts',(-3.62476577205416,12.2,-1.67660572288421));
#300500=CARTESIAN_POINT('',(-3.29009567465824,12.2,-1.52180664071691));
#300501=CARTESIAN_POINT('',(-3.62475766100006,12.2,-1.67660193100001));
#300502=CARTESIAN_POINT('',(-3.48557996500006,12.2,-0.995669277000015));
#300503=CARTESIAN_POINT('Origin',(-5.66300478732629E-14,12.2,-1.77635683940025E-14));
#300504=CARTESIAN_POINT('',(-3.84014275842517,12.2,-1.0969513940623));
#300505=CARTESIAN_POINT('',(-3.48557996500006,12.2,-0.995669277000015));
#300506=CARTESIAN_POINT('',(-4.64916443400006,12.2,-0.973534832000014));
#300507=CARTESIAN_POINT('Ctrl Pts',(-3.84014278600006,12.2,-1.09695129700001));
#300508=CARTESIAN_POINT('Ctrl Pts',(-3.84030898991399,12.2,-1.09699816032842));
#300509=CARTESIAN_POINT('Ctrl Pts',(-3.84140226785887,12.2,-1.0972932841756));
#300510=CARTESIAN_POINT('Ctrl Pts',(-3.84464780527484,12.2,-1.0980939631551));
#300511=CARTESIAN_POINT('Ctrl Pts',(-3.84678446778506,12.199999999908,-1.0985771363248));
#300512=CARTESIAN_POINT('Ctrl Pts',(-3.85618709028379,12.199999999908,-1.10059260222741));
#300513=CARTESIAN_POINT('Ctrl Pts',(-3.86411569097725,12.199999999908,-1.10197705056623));
#300514=CARTESIAN_POINT('Ctrl Pts',(-3.89873881818786,12.199999999908,-1.10725203377565));
#300515=CARTESIAN_POINT('Ctrl Pts',(-3.92796253029191,12.2,-1.10953219114214));
#300516=CARTESIAN_POINT('Ctrl Pts',(-4.0336650704685,12.2,-1.11337750310591));
#300517=CARTESIAN_POINT('Ctrl Pts',(-4.13324208872044,12.2,-1.10766588628757));
#300518=CARTESIAN_POINT('Ctrl Pts',(-4.38630470364963,12.2,-1.06234400779285));
#300519=CARTESIAN_POINT('Ctrl Pts',(-4.51963188083663,12.2,-1.02312808333993));
#300520=CARTESIAN_POINT('Ctrl Pts',(-4.64916443400006,12.2,-0.973534832000014));
#300521=CARTESIAN_POINT('',(-4.70648560700006,12.2,-0.641477381000013));
#300522=CARTESIAN_POINT('Origin',(-5.66300478732629E-14,12.2,-1.77635683940025E-14));
#300523=CARTESIAN_POINT('',(-3.98564879651336,12.2,-0.253971471173062));
#300524=CARTESIAN_POINT('Ctrl Pts',(-4.70648560700006,12.2,-0.641477381000013));
#300525=CARTESIAN_POINT('Ctrl Pts',(-4.67739030276498,12.2,-0.616593939557199));
#300526=CARTESIAN_POINT('Ctrl Pts',(-4.64853374448598,12.2,-0.593039396638165));
#300527=CARTESIAN_POINT('Ctrl Pts',(-4.62002995111684,12.2,-0.570801237698567));
#300528=CARTESIAN_POINT('Ctrl Pts',(-4.57760782927771,12.2,-0.537704243351314));
#300529=CARTESIAN_POINT('Ctrl Pts',(-4.53596732202362,12.2,-0.50752499617894));
#300530=CARTESIAN_POINT('Ctrl Pts',(-4.49551314177239,12.2,-0.480188970837284));
#300531=CARTESIAN_POINT('Ctrl Pts',(-4.45659866038684,12.2,-0.453893363246007));
#300532=CARTESIAN_POINT('Ctrl Pts',(-4.4187819253462,12.2,-0.430228847080283));
#300533=CARTESIAN_POINT('Ctrl Pts',(-4.38244840783252,12.2,-0.409089430305889));
#300534=CARTESIAN_POINT('Ctrl Pts',(-4.34725263625644,12.2,-0.388611972163751));
#300535=CARTESIAN_POINT('Ctrl Pts',(-4.31344857123307,12.2,-0.370504213207233));
#300536=CARTESIAN_POINT('Ctrl Pts',(-4.28141134962896,12.2,-0.354628570095604));
#300537=CARTESIAN_POINT('Ctrl Pts',(-4.2509814919226,12.2,-0.339549435991728));
#300538=CARTESIAN_POINT('Ctrl Pts',(-4.22214561332269,12.2,-0.326484236774195));
#300539=CARTESIAN_POINT('Ctrl Pts',(-4.19524842022594,12.2,-0.31527462050277));
#300540=CARTESIAN_POINT('Ctrl Pts',(-4.16917658132024,12.2,-0.304408977066588));
#300541=CARTESIAN_POINT('Ctrl Pts',(-4.14492611508931,12.2,-0.295287111378102));
#300542=CARTESIAN_POINT('Ctrl Pts',(-4.12283468744088,12.2,-0.287722175954538));
#300543=CARTESIAN_POINT('Ctrl Pts',(-4.10223155113375,12.2,-0.280666887443235));
#300544=CARTESIAN_POINT('Ctrl Pts',(-4.08350632160541,12.2,-0.274965900155463));
#300545=CARTESIAN_POINT('Ctrl Pts',(-4.06695477888446,12.2,-0.27042749044276));
#300546=CARTESIAN_POINT('Ctrl Pts',(-4.05123986161395,12.2,-0.26611848225076));
#300547=CARTESIAN_POINT('Ctrl Pts',(-4.03748433107584,12.2,-0.262857737210549));
#300548=CARTESIAN_POINT('Ctrl Pts',(-4.02596291487887,12.2,-0.260441305594084));
#300549=CARTESIAN_POINT('Ctrl Pts',(-4.01484311445685,12.2,-0.25810910642263));
#300550=CARTESIAN_POINT('Ctrl Pts',(-4.00580415854497,12.2,-0.256563801725764));
#300551=CARTESIAN_POINT('Ctrl Pts',(-3.9991163289497,12.2,-0.255579178475452));
#300552=CARTESIAN_POINT('Ctrl Pts',(-3.99497751304969,12.2,-0.254969836639529));
#300553=CARTESIAN_POINT('Ctrl Pts',(-3.99173960011373,12.2,-0.254574381557754));
#300554=CARTESIAN_POINT('Ctrl Pts',(-3.98947213811192,12.2,-0.25432920431917));
#300555=CARTESIAN_POINT('Ctrl Pts',(-3.98833840711101,12.2,-0.254206615699878));
#300556=CARTESIAN_POINT('Ctrl Pts',(-3.98744734802868,12.2,-0.254121478293377));
#300557=CARTESIAN_POINT('Ctrl Pts',(-3.98680815864947,12.2,-0.254064967079465));
#300558=CARTESIAN_POINT('Ctrl Pts',(-3.98648856395987,12.2,-0.254036711472509));
#300559=CARTESIAN_POINT('Ctrl Pts',(-3.9862319212959,12.2,-0.254015618895323));
#300560=CARTESIAN_POINT('Ctrl Pts',(-3.98603942619645,12.2,-0.254000520323441));
#300561=CARTESIAN_POINT('Ctrl Pts',(-3.98591562691842,12.2,-0.253990809986381));
#300562=CARTESIAN_POINT('Ctrl Pts',(-3.98581889125066,12.2,-0.253983577985231));
#300563=CARTESIAN_POINT('Ctrl Pts',(-3.98574755264139,12.2,-0.25397838826675));
#300564=CARTESIAN_POINT('Ctrl Pts',(-3.98570796707643,12.2,-0.253975508508647));
#300565=CARTESIAN_POINT('Ctrl Pts',(-3.98568085248347,12.2,-0.253973712859757));
#300566=CARTESIAN_POINT('Ctrl Pts',(-3.98565325097426,12.2,-0.2539718483819));
#300567=CARTESIAN_POINT('',(-3.61766281507283,12.2,-0.230522786376999));
#300568=CARTESIAN_POINT('',(-3.98564433200006,12.2,-0.253971243000013));
#300569=CARTESIAN_POINT('',(-3.60988374900006,12.2,0.330702762999984));
#300570=CARTESIAN_POINT('Origin',(-5.66300478732629E-14,12.2,-1.77635683940025E-14));
#300571=CARTESIAN_POINT('',(-3.9770910289505,12.2,0.364342856252411));
#300572=CARTESIAN_POINT('',(-3.60988374900006,12.2,0.330702762999984));
#300573=CARTESIAN_POINT('',(-4.68689806900006,12.2,0.771677711999987));
#300574=CARTESIAN_POINT('Ctrl Pts',(-3.97709101934974,12.2,0.364342957033298));
#300575=CARTESIAN_POINT('Ctrl Pts',(-3.97736112094161,12.2,0.364368687912379));
#300576=CARTESIAN_POINT('Ctrl Pts',(-3.97763081754438,12.1999999999997,
0.364398582405285));
#300577=CARTESIAN_POINT('Ctrl Pts',(-3.97847249976144,12.1999999999997,
0.364493406994217));
#300578=CARTESIAN_POINT('Ctrl Pts',(-3.97907662749092,12.2,0.364567350873792));
#300579=CARTESIAN_POINT('Ctrl Pts',(-3.98170542410654,12.2,0.364904961265897));
#300580=CARTESIAN_POINT('Ctrl Pts',(-3.98387379409812,12.199999999908,0.365226521130628));
#300581=CARTESIAN_POINT('Ctrl Pts',(-3.99336397358853,12.199999999908,0.366742885520348));
#300582=CARTESIAN_POINT('Ctrl Pts',(-4.0012579760989,12.199999999908,0.368316009283327));
#300583=CARTESIAN_POINT('Ctrl Pts',(-4.03544701617339,12.199999999908,0.375904201720463));
#300584=CARTESIAN_POINT('Ctrl Pts',(-4.06352360252377,12.2,0.384335203288191));
#300585=CARTESIAN_POINT('Ctrl Pts',(-4.16348965587543,12.2,0.418937988494843));
#300586=CARTESIAN_POINT('Ctrl Pts',(-4.25429273351133,12.2,0.460246281843015));
#300587=CARTESIAN_POINT('Ctrl Pts',(-4.47387858189227,12.2,0.593914841213743));
#300588=CARTESIAN_POINT('Ctrl Pts',(-4.5841592272997,12.2,0.67875964775583));
#300589=CARTESIAN_POINT('Ctrl Pts',(-4.68689806900006,12.2,0.771677711999987));
#300590=CARTESIAN_POINT('',(-4.62039548500006,12.2,1.10201885899999));
#300591=CARTESIAN_POINT('Origin',(-5.66300478732629E-14,12.2,-1.77635683940025E-14));
#300592=CARTESIAN_POINT('',(-3.80824764648564,12.2,1.20295971278735));
#300593=CARTESIAN_POINT('Ctrl Pts',(-4.62039548500006,12.2,1.10201885899999));
#300594=CARTESIAN_POINT('Ctrl Pts',(-4.49008798165083,12.2,1.14780973418869));
#300595=CARTESIAN_POINT('Ctrl Pts',(-4.35566622701388,12.2,1.18338092348667));
#300596=CARTESIAN_POINT('Ctrl Pts',(-4.10115788280569,12.2,1.22181532284944));
#300597=CARTESIAN_POINT('Ctrl Pts',(-4.00118301828606,12.2,1.22475245377806));
#300598=CARTESIAN_POINT('Ctrl Pts',(-3.89557234472372,12.2,1.21796341587231));
#300599=CARTESIAN_POINT('Ctrl Pts',(-3.86637307317564,12.2000000000748,
1.21486437588036));
#300600=CARTESIAN_POINT('Ctrl Pts',(-3.83190572787353,12.2000000000748,
1.20861681729509));
#300601=CARTESIAN_POINT('Ctrl Pts',(-3.82403373441455,12.2000000000748,
1.20701284847675));
#300602=CARTESIAN_POINT('Ctrl Pts',(-3.81473210800609,12.2000000000748,
1.20474214283786));
#300603=CARTESIAN_POINT('Ctrl Pts',(-3.81262693390849,12.2,1.2042031454596));
#300604=CARTESIAN_POINT('Ctrl Pts',(-3.81010330907745,12.2,1.20350407609351));
#300605=CARTESIAN_POINT('Ctrl Pts',(-3.80952866324519,12.2000000000005,
1.2033412192238));
#300606=CARTESIAN_POINT('Ctrl Pts',(-3.80885139391262,12.2000000000005,
1.20314218456492));
#300607=CARTESIAN_POINT('Ctrl Pts',(-3.80853382233514,12.2,1.20304885187476));
#300608=CARTESIAN_POINT('Ctrl Pts',(-3.80828031400006,12.2,1.20296984599999));
#300609=CARTESIAN_POINT('',(-3.45664454600006,12.2,1.09189444699998));
#300610=CARTESIAN_POINT('',(-3.80824765200006,12.2,1.20295966899999));
#300611=CARTESIAN_POINT('',(-3.24665273100006,12.2,1.61241156299999));
#300612=CARTESIAN_POINT('Origin',(-5.66300478732629E-14,12.2,-1.77635683940025E-14));
#300613=CARTESIAN_POINT('',(-3.57691111715103,12.2,1.7764305847426));
#300614=CARTESIAN_POINT('',(-3.24665273100006,12.2,1.61241156299999));
#300615=CARTESIAN_POINT('',(-4.09164014900006,12.2,2.41267090399998));
#300616=CARTESIAN_POINT('Ctrl Pts',(-3.57691107200006,12.2,1.77643067499998));
#300617=CARTESIAN_POINT('Ctrl Pts',(-3.57715363087875,12.2,1.77655225603397));
#300618=CARTESIAN_POINT('Ctrl Pts',(-3.57739432442841,12.1999999999997,
1.7766775413267));
#300619=CARTESIAN_POINT('Ctrl Pts',(-3.57814397713914,12.1999999999997,
1.77706952294413));
#300620=CARTESIAN_POINT('Ctrl Pts',(-3.57868088758371,12.2,1.77735684826631));
#300621=CARTESIAN_POINT('Ctrl Pts',(-3.58100948595218,12.2,1.77862090122509));
#300622=CARTESIAN_POINT('Ctrl Pts',(-3.58291519327722,12.1999999999079,
1.77970395294905));
#300623=CARTESIAN_POINT('Ctrl Pts',(-3.5912174593958,12.1999999999079,1.78454657405624));
#300624=CARTESIAN_POINT('Ctrl Pts',(-3.5980079172033,12.1999999999079,1.78886359039074));
#300625=CARTESIAN_POINT('Ctrl Pts',(-3.62715509725334,12.1999999999079,
1.80829521478595));
#300626=CARTESIAN_POINT('Ctrl Pts',(-3.65029150305341,12.2,1.82630146689454));
#300627=CARTESIAN_POINT('Ctrl Pts',(-3.73111669954928,12.2,1.89477220755472));
#300628=CARTESIAN_POINT('Ctrl Pts',(-3.8008635540934,12.2,1.96614323281364));
#300629=CARTESIAN_POINT('Ctrl Pts',(-3.95725251061657,12.2,2.17000168930957));
#300630=CARTESIAN_POINT('Ctrl Pts',(-4.02964978479197,12.2,2.28940052844448));
#300631=CARTESIAN_POINT('Ctrl Pts',(-4.09164014979821,12.2,2.41267090359861));
#300632=CARTESIAN_POINT('',(-3.91029535000006,12.2,2.69668134599998));
#300633=CARTESIAN_POINT('Origin',(-5.66300478732629E-14,12.2,-1.77635683940025E-14));
#300634=CARTESIAN_POINT('',(-3.11652947055878,12.2,2.49742704586989));
#300635=CARTESIAN_POINT('Ctrl Pts',(-3.91029535000006,12.2,2.69668134599998));
#300636=CARTESIAN_POINT('Ctrl Pts',(-3.87704667375992,12.2,2.69562795448002));
#300637=CARTESIAN_POINT('Ctrl Pts',(-3.844607186862,12.2,2.69395488001898));
#300638=CARTESIAN_POINT('Ctrl Pts',(-3.81302641540527,12.2,2.69171777261672));
#300639=CARTESIAN_POINT('Ctrl Pts',(-3.75925183787251,12.2,2.68790850831115));
#300640=CARTESIAN_POINT('Ctrl Pts',(-3.70796856982792,12.2,2.68246255129163));
#300641=CARTESIAN_POINT('Ctrl Pts',(-3.65942186526007,12.2,2.67569751949168));
#300642=CARTESIAN_POINT('Ctrl Pts',(-3.61272377880615,12.2,2.66919009447346));
#300643=CARTESIAN_POINT('Ctrl Pts',(-3.56855790143124,12.2,2.66146197193717));
#300644=CARTESIAN_POINT('Ctrl Pts',(-3.52713481762616,12.2,2.65284046259447));
#300645=CARTESIAN_POINT('Ctrl Pts',(-3.48684973136383,12.2,2.644455808057));
#300646=CARTESIAN_POINT('Ctrl Pts',(-3.44915895619017,12.2,2.63522588786816));
#300647=CARTESIAN_POINT('Ctrl Pts',(-3.41424704813716,12.2,2.62549768671105));
#300648=CARTESIAN_POINT('Ctrl Pts',(-3.38050173090573,12.2,2.6160945560188));
#300649=CARTESIAN_POINT('Ctrl Pts',(-3.34935281231531,12.2,2.60622559506111));
#300650=CARTESIAN_POINT('Ctrl Pts',(-3.32095662401592,12.2,2.59625133524797));
#300651=CARTESIAN_POINT('Ctrl Pts',(-3.29395175854877,12.2,2.58676578241432));
#300652=CARTESIAN_POINT('Ctrl Pts',(-3.26943656002086,12.2,2.57718480265262));
#300653=CARTESIAN_POINT('Ctrl Pts',(-3.24753462597801,12.2,2.56786486200729));
#300654=CARTESIAN_POINT('Ctrl Pts',(-3.22645411420113,12.2,2.5588944615783));
#300655=CARTESIAN_POINT('Ctrl Pts',(-3.20779462551826,12.2,2.5501655301266));
#300656=CARTESIAN_POINT('Ctrl Pts',(-3.19165465935819,12.2,2.54204381384399));
#300657=CARTESIAN_POINT('Ctrl Pts',(-3.176799307833,12.2,2.53456852243573));
#300658=CARTESIAN_POINT('Ctrl Pts',(-3.16407839268306,12.2,2.52760760821054));
#300659=CARTESIAN_POINT('Ctrl Pts',(-3.15355800067279,12.2,2.52148949437163));
#300660=CARTESIAN_POINT('Ctrl Pts',(-3.14350736635935,12.2,2.51564456722226));
#300661=CARTESIAN_POINT('Ctrl Pts',(-3.13546519137256,12.2,2.5105685062388));
#300662=CARTESIAN_POINT('Ctrl Pts',(-3.12947823622448,12.2,2.50659179575057));
#300663=CARTESIAN_POINT('Ctrl Pts',(-3.12539205517989,12.2,2.50387763494345));
#300664=CARTESIAN_POINT('Ctrl Pts',(-3.12226302098882,12.2,2.50167644123223));
#300665=CARTESIAN_POINT('Ctrl Pts',(-3.12010253332815,12.2,2.50010760672021));
#300666=CARTESIAN_POINT('Ctrl Pts',(-3.11902228949781,12.2,2.4993231894642));
#300667=CARTESIAN_POINT('Ctrl Pts',(-3.11818413389332,12.2,2.49869705722392));
#300668=CARTESIAN_POINT('Ctrl Pts',(-3.11758918392009,12.2,2.49824543008379));
#300669=CARTESIAN_POINT('Ctrl Pts',(-3.11729170893347,12.2,2.49801961651373));
#300670=CARTESIAN_POINT('Ctrl Pts',(-3.11705503249409,12.2,2.49783745985302));
#300671=CARTESIAN_POINT('Ctrl Pts',(-3.11687927028665,12.2,2.49770102503292));
#300672=CARTESIAN_POINT('Ctrl Pts',(-3.11677151728329,12.2,2.49761738212787));
#300673=CARTESIAN_POINT('Ctrl Pts',(-3.11668713186045,12.2,2.49755136519769));
#300674=CARTESIAN_POINT('Ctrl Pts',(-3.11662457182833,12.2,2.49750218397371));
#300675=CARTESIAN_POINT('Ctrl Pts',(-3.11659040942531,12.2,2.49747532738912));
#300676=CARTESIAN_POINT('Ctrl Pts',(-3.11656553206438,12.2,2.49745561966817));
#300677=CARTESIAN_POINT('Ctrl Pts',(-3.11654335547073,12.2,2.49743798830104));
#300678=CARTESIAN_POINT('Ctrl Pts',(-3.11653990011135,12.2,2.49743524113839));
#300679=CARTESIAN_POINT('Ctrl Pts',(-3.11653645629695,12.2,2.4974325028997));
#300680=CARTESIAN_POINT('Ctrl Pts',(-3.11653301183405,12.2,2.49742976420877));
#300681=CARTESIAN_POINT('',(-2.82878727700006,12.2,2.26684528399999));
#300682=CARTESIAN_POINT('',(-3.11652602300006,12.2,2.49742420999999));
#300683=CARTESIAN_POINT('',(-2.44494327000006,12.2,2.67635524699998));
#300684=CARTESIAN_POINT('Origin',(-5.66300478732629E-14,12.2,-1.77635683940025E-14));
#300685=CARTESIAN_POINT('',(-2.69364953994162,12.2,2.94860152033068));
#300686=CARTESIAN_POINT('',(-2.44494327000006,12.2,2.67635524699998));
#300687=CARTESIAN_POINT('',(-2.94378355400006,12.2,3.72781952199999));
#300688=CARTESIAN_POINT('Ctrl Pts',(-2.69364946515999,12.2,2.94860158817627));
#300689=CARTESIAN_POINT('Ctrl Pts',(-2.69383177439424,12.2,2.94880253537606));
#300690=CARTESIAN_POINT('Ctrl Pts',(-2.69401090483053,12.1999999999997,
2.94900635440571));
#300691=CARTESIAN_POINT('Ctrl Pts',(-2.69456846309778,12.1999999999997,
2.94964281651214));
#300692=CARTESIAN_POINT('Ctrl Pts',(-2.69496497063731,12.2,2.95010428156435));
#300693=CARTESIAN_POINT('Ctrl Pts',(-2.69668033191381,12.2,2.95212492184448));
#300694=CARTESIAN_POINT('Ctrl Pts',(-2.69806509480641,12.1999999999079,
2.95382201005389));
#300695=CARTESIAN_POINT('Ctrl Pts',(-2.70406029290256,12.1999999999079,
2.96134042105594));
#300696=CARTESIAN_POINT('Ctrl Pts',(-2.70883395520956,12.1999999999079,
2.96782105431918));
#300697=CARTESIAN_POINT('Ctrl Pts',(-2.72898834256397,12.1999999999079,
2.99646249251351));
#300698=CARTESIAN_POINT('Ctrl Pts',(-2.74405879664829,12.2,3.02161189257851));
#300699=CARTESIAN_POINT('Ctrl Pts',(-2.79448036335615,12.2,3.11426835608687));
#300700=CARTESIAN_POINT('Ctrl Pts',(-2.83379571846681,12.2,3.2058879483145));
#300701=CARTESIAN_POINT('Ctrl Pts',(-2.90612983688009,12.2,3.45297987201336));
#300702=CARTESIAN_POINT('Ctrl Pts',(-2.9304772130833,12.2,3.59014359399116));
#300703=CARTESIAN_POINT('Ctrl Pts',(-2.94378355400006,12.2,3.72781952199999));
#300704=CARTESIAN_POINT('',(-2.67208816000006,12.2,3.92714207399998));
#300705=CARTESIAN_POINT('Origin',(-5.66300478732629E-14,12.2,-1.77635683940025E-14));
#300706=CARTESIAN_POINT('',(-2.00390023382555,12.2,3.45459781463392));
#300707=CARTESIAN_POINT('Ctrl Pts',(-2.67208816000006,12.2,3.92714207399998));
#300708=CARTESIAN_POINT('Ctrl Pts',(-2.54470272548118,12.2,3.87309341167482));
#300709=CARTESIAN_POINT('Ctrl Pts',(-2.42161063813132,12.2,3.80890442524401));
#300710=CARTESIAN_POINT('Ctrl Pts',(-2.20787373403996,12.2,3.66600708574621));
#300711=CARTESIAN_POINT('Ctrl Pts',(-2.13195690805562,12.2,3.60084568574312));
#300712=CARTESIAN_POINT('Ctrl Pts',(-2.0583252666406,12.2,3.52451513065958));
#300713=CARTESIAN_POINT('Ctrl Pts',(-2.0388379215194,12.2000000000748,3.50255771474838));
#300714=CARTESIAN_POINT('Ctrl Pts',(-2.01046851767774,12.2000000000748,
3.46541597332446));
#300715=CARTESIAN_POINT('Ctrl Pts',(-2.00486827616945,12.2,3.45625245717719));
#300716=CARTESIAN_POINT('Ctrl Pts',(-2.00390029233317,12.2,3.45459778040704));
#300717=CARTESIAN_POINT('',(-1.81888661200006,12.2,3.13564610499999));
#300718=CARTESIAN_POINT('',(-2.00390028500005,12.2,3.45459777499999));
#300719=CARTESIAN_POINT('',(-1.31303067400006,12.2,3.37884232399999));
#300720=CARTESIAN_POINT('Origin',(-5.66300478732629E-14,12.2,-1.77635683940025E-14));
#300721=CARTESIAN_POINT('',(-1.44659566557757,12.2,3.72254748089793));
#300722=CARTESIAN_POINT('',(-1.31303067400006,12.2,3.37884232399999));
#300723=CARTESIAN_POINT('',(-1.39835267900006,12.2,4.53950545599999));
#300724=CARTESIAN_POINT('Ctrl Pts',(-1.44659557109088,12.2,3.72254751723615));
#300725=CARTESIAN_POINT('Ctrl Pts',(-1.44669296442588,12.2,3.72280075945341));
#300726=CARTESIAN_POINT('Ctrl Pts',(-1.4467863863064,12.1999999999997,3.72305551966744));
#300727=CARTESIAN_POINT('Ctrl Pts',(-1.44707664467613,12.1999999999997,
3.72385115239218));
#300728=CARTESIAN_POINT('Ctrl Pts',(-1.44727952399059,12.2,3.72442428851802));
#300729=CARTESIAN_POINT('Ctrl Pts',(-1.44814961145563,12.2,3.72692957023441));
#300730=CARTESIAN_POINT('Ctrl Pts',(-1.44882811640487,12.199999999908,3.72901348813528));
#300731=CARTESIAN_POINT('Ctrl Pts',(-1.45170124179413,12.199999999908,3.73818584407418));
#300732=CARTESIAN_POINT('Ctrl Pts',(-1.45381079932822,12.199999999908,3.74595029799757));
#300733=CARTESIAN_POINT('Ctrl Pts',(-1.46226030946429,12.199999999908,3.77994874903547));
#300734=CARTESIAN_POINT('Ctrl Pts',(-1.46722768673953,12.2,3.80884656437798));
#300735=CARTESIAN_POINT('Ctrl Pts',(-1.48078731749073,12.2,3.91357120575646));
#300736=CARTESIAN_POINT('Ctrl Pts',(-1.4843227561384,12.2,4.01323730435706));
#300737=CARTESIAN_POINT('Ctrl Pts',(-1.46252018784725,12.2,4.26968072123177));
#300738=CARTESIAN_POINT('Ctrl Pts',(-1.43552455444774,12.2,4.40687162494879));
#300739=CARTESIAN_POINT('Ctrl Pts',(-1.39835267900006,12.2,4.53950545599998));
#300740=CARTESIAN_POINT('',(-1.07300065765139,12.2,4.62722050353667));
#300741=CARTESIAN_POINT('Origin',(-5.66300478732629E-14,12.2,-1.77635683940025E-14));
#300742=CARTESIAN_POINT('',(-0.620636653770277,12.2,3.9452088280328));
#300743=CARTESIAN_POINT('Ctrl Pts',(-1.07300065706596,12.2,4.62722050309264));
#300744=CARTESIAN_POINT('Ctrl Pts',(-1.0507849572306,12.2,4.60564108152845));
#300745=CARTESIAN_POINT('Ctrl Pts',(-1.02944940026969,12.2,4.58413736641884));
#300746=CARTESIAN_POINT('Ctrl Pts',(-1.00899345236455,12.2,4.56276913341815));
#300747=CARTESIAN_POINT('Ctrl Pts',(-0.971388421889957,12.2,4.52348701083426));
#300748=CARTESIAN_POINT('Ctrl Pts',(-0.936758198137158,12.2,4.48466285825686));
#300749=CARTESIAN_POINT('Ctrl Pts',(-0.905070969024602,12.2,4.44670166000136));
#300750=CARTESIAN_POINT('Ctrl Pts',(-0.874654520745516,12.2,4.41026285308488));
#300751=CARTESIAN_POINT('Ctrl Pts',(-0.846949885617722,12.2,4.37461914823072));
#300752=CARTESIAN_POINT('Ctrl Pts',(-0.821892991659933,12.2,4.34015678120677));
#300753=CARTESIAN_POINT('Ctrl Pts',(-0.797601978032624,12.2,4.30674777894103));
#300754=CARTESIAN_POINT('Ctrl Pts',(-0.77579954999807,12.2,4.27444890333346));
#300755=CARTESIAN_POINT('Ctrl Pts',(-0.756389823805907,12.2,4.24363974821588));
#300756=CARTESIAN_POINT('Ctrl Pts',(-0.737708294855191,12.2,4.21398646420878));
#300757=CARTESIAN_POINT('Ctrl Pts',(-0.721243540586764,12.2,4.18571311401967));
#300758=CARTESIAN_POINT('Ctrl Pts',(-0.706871483729886,12.2,4.15918547425683));
#300759=CARTESIAN_POINT('Ctrl Pts',(-0.693077220900548,12.2,4.13372431453733));
#300760=CARTESIAN_POINT('Ctrl Pts',(-0.681211010007532,12.2,4.10987120057421));
#300761=CARTESIAN_POINT('Ctrl Pts',(-0.671123604797768,12.2,4.08797668630482));
#300762=CARTESIAN_POINT('Ctrl Pts',(-0.66135402368667,12.2,4.06677200297993));
#300763=CARTESIAN_POINT('Ctrl Pts',(-0.653253266385538,12.2,4.04740423646243));
#300764=CARTESIAN_POINT('Ctrl Pts',(-0.646643456602352,12.2,4.03022032450418));
#300765=CARTESIAN_POINT('Ctrl Pts',(-0.640601123809652,12.2,4.01451171591513));
#300766=CARTESIAN_POINT('Ctrl Pts',(-0.635804690486196,12.2,4.00062807843892));
#300767=CARTESIAN_POINT('Ctrl Pts',(-0.632080686925434,12.2,3.98885955077024));
#300768=CARTESIAN_POINT('Ctrl Pts',(-0.628517809363524,12.2,3.97760021052436));
#300769=CARTESIAN_POINT('Ctrl Pts',(-0.625936885444006,12.2,3.9682766719032));
#300770=CARTESIAN_POINT('Ctrl Pts',(-0.624147610493951,12.2,3.96116869451554));
#300771=CARTESIAN_POINT('Ctrl Pts',(-0.622908591722011,12.2,3.95624663521237));
#300772=CARTESIAN_POINT('Ctrl Pts',(-0.622048443669106,12.2,3.95238744701319));
#300773=CARTESIAN_POINT('Ctrl Pts',(-0.621490912601253,12.2,3.94969285919901));
#300774=CARTESIAN_POINT('Ctrl Pts',(-0.621212147067327,12.2,3.94834556529192));
#300775=CARTESIAN_POINT('Ctrl Pts',(-0.621008857541319,12.2,3.94728953113019));
#300776=CARTESIAN_POINT('Ctrl Pts',(-0.620870323783881,12.2,3.94653829591385));
#300777=CARTESIAN_POINT('Ctrl Pts',(-0.620801056905161,12.2,3.94616267830568));
#300778=CARTESIAN_POINT('Ctrl Pts',(-0.620747955427695,12.2,3.94586327661587));
#300779=CARTESIAN_POINT('Ctrl Pts',(-0.620709628879688,12.2,3.94564180448601));
#300780=CARTESIAN_POINT('Ctrl Pts',(-0.620685910104493,12.2,3.94550474419926));
#300781=CARTESIAN_POINT('Ctrl Pts',(-0.620667909838897,12.2,3.94539829416118));
#300782=CARTESIAN_POINT('Ctrl Pts',(-0.620654939939172,12.2,3.94532036311127));
#300783=CARTESIAN_POINT('Ctrl Pts',(-0.620646952117413,12.2,3.94527236741744));
#300784=CARTESIAN_POINT('Ctrl Pts',(-0.620641950349572,12.2,3.94524125295544));
#300785=CARTESIAN_POINT('Ctrl Pts',(-0.620636729615096,12.2,3.94520886906205));
#300786=CARTESIAN_POINT('',(-0.563335230000056,12.2,3.58096054499998));
#300787=CARTESIAN_POINT('',(-0.620636721000055,12.2,3.94520881799998));
#300788=CARTESIAN_POINT('',(-0.00378600900005522,12.2,3.62499802299999));
#300789=CARTESIAN_POINT('Origin',(-5.66300478732629E-14,12.2,-1.77635683940025E-14));
#300790=CARTESIAN_POINT('',(-0.0041710307407783,12.2,3.99374277690018));
#300791=CARTESIAN_POINT('',(-0.00378600900005522,12.2,3.62499802299999));
#300792=CARTESIAN_POINT('',(0.335933474325597,12.2,4.73810602455833));
#300793=CARTESIAN_POINT('Ctrl Pts',(-0.00417093000005587,12.2,3.99374277699999));
#300794=CARTESIAN_POINT('Ctrl Pts',(-0.00417024165288169,12.2,3.99401409886674));
#300795=CARTESIAN_POINT('Ctrl Pts',(-0.00416534981364848,12.1999999999997,
3.99428540196681));
#300796=CARTESIAN_POINT('Ctrl Pts',(-0.00414859876650465,12.1999999999997,
3.99513161023346));
#300797=CARTESIAN_POINT('Ctrl Pts',(-0.00413071236587515,12.2,3.99574033513076));
#300798=CARTESIAN_POINT('Ctrl Pts',(-0.0040371607748202,12.2,3.99838724109435));
#300799=CARTESIAN_POINT('Ctrl Pts',(-0.00391727435201773,12.1999999999079,
4.00057359205342));
#300800=CARTESIAN_POINT('Ctrl Pts',(-0.00328249533119052,12.1999999999079,
4.01017095407316));
#300801=CARTESIAN_POINT('Ctrl Pts',(-0.0024444871704632,12.1999999999079,
4.01817466079553));
#300802=CARTESIAN_POINT('Ctrl Pts',(0.00195733879072123,12.1999999999079,
4.05292260177391));
#300803=CARTESIAN_POINT('Ctrl Pts',(0.00776259300637182,12.2,4.08165749006985));
#300804=CARTESIAN_POINT('Ctrl Pts',(0.0330060981399338,12.2,4.18443935972204));
#300805=CARTESIAN_POINT('Ctrl Pts',(0.0657739729375395,12.2,4.27866713336303));
#300806=CARTESIAN_POINT('Ctrl Pts',(0.178614829390611,12.2,4.50965703821246));
#300807=CARTESIAN_POINT('Ctrl Pts',(0.253251233611231,12.2,4.62771303457587));
#300808=CARTESIAN_POINT('Ctrl Pts',(0.335933474999944,12.2,4.73810602399999));
#300809=CARTESIAN_POINT('',(0.671001528968269,12.2,4.70236716444468));
#300810=CARTESIAN_POINT('Origin',(-5.66300478732629E-14,12.2,-1.77635683940025E-14));
#300811=CARTESIAN_POINT('',(0.846447363903509,12.2,3.90299749089007));
#300812=CARTESIAN_POINT('Ctrl Pts',(0.671001528999944,12.2,4.70236716399998));
#300813=CARTESIAN_POINT('Ctrl Pts',(0.689750617970205,12.2,4.66152111816135));
#300814=CARTESIAN_POINT('Ctrl Pts',(0.706827850453991,12.2,4.62149223703923));
#300815=CARTESIAN_POINT('Ctrl Pts',(0.722304674338832,12.2,4.58245379874695));
#300816=CARTESIAN_POINT('Ctrl Pts',(0.741807263919132,12.2,4.53326084769089));
#300817=CARTESIAN_POINT('Ctrl Pts',(0.758767324969944,12.2,4.48564127013701));
#300818=CARTESIAN_POINT('Ctrl Pts',(0.773369417859129,12.2,4.43995898600264));
#300819=CARTESIAN_POINT('Ctrl Pts',(0.787377131758578,12.2,4.39613620174263));
#300820=CARTESIAN_POINT('Ctrl Pts',(0.79921477102076,12.2,4.35409623312068));
#300821=CARTESIAN_POINT('Ctrl Pts',(0.809089552047529,12.2,4.31417337674083));
#300822=CARTESIAN_POINT('Ctrl Pts',(0.818602810828708,12.2,4.2757121224613));
#300823=CARTESIAN_POINT('Ctrl Pts',(0.826294080583583,12.2,4.23921581476659));
#300824=CARTESIAN_POINT('Ctrl Pts',(0.832393390803862,12.2,4.20499530620236));
#300825=CARTESIAN_POINT('Ctrl Pts',(0.838252673463236,12.2,4.17212148519901));
#300826=CARTESIAN_POINT('Ctrl Pts',(0.842642574720562,12.2,4.14134786481141));
#300827=CARTESIAN_POINT('Ctrl Pts',(0.845812337415013,12.2,4.11296125522075));
#300828=CARTESIAN_POINT('Ctrl Pts',(0.848839496067851,12.2,4.0858517271171));
#300829=CARTESIAN_POINT('Ctrl Pts',(0.850753570419483,12.2,4.06091921258366));
#300830=CARTESIAN_POINT('Ctrl Pts',(0.851817032964709,12.2,4.03842413570375));
#300831=CARTESIAN_POINT('Ctrl Pts',(0.852808803672242,12.2,4.01744553291857));
#300832=CARTESIAN_POINT('Ctrl Pts',(0.853060701605771,12.2,3.99858680463442));
#300833=CARTESIAN_POINT('Ctrl Pts',(0.852827866970706,12.2,3.98206865845845));
#300834=CARTESIAN_POINT('Ctrl Pts',(0.852604043162,12.2,3.96618977347707));
#300835=CARTESIAN_POINT('Ctrl Pts',(0.85193190637898,12.2,3.95247375923966));
#300836=CARTESIAN_POINT('Ctrl Pts',(0.851081822358656,12.2,3.94112639931417));
#300837=CARTESIAN_POINT('Ctrl Pts',(0.850268518793122,12.2,3.93027000386836));
#300838=CARTESIAN_POINT('Ctrl Pts',(0.849291970755508,12.2,3.92158163117595));
#300839=CARTESIAN_POINT('Ctrl Pts',(0.848434785939518,12.2,3.91525181550474));
#300840=CARTESIAN_POINT('Ctrl Pts',(0.84791939618732,12.2,3.91144595932368));
#300841=CARTESIAN_POINT('Ctrl Pts',(0.847448067511482,12.2,3.90849293832927));
#300842=CARTESIAN_POINT('Ctrl Pts',(0.847091867570908,12.2,3.90643638947668));
#300843=CARTESIAN_POINT('Ctrl Pts',(0.846913767600621,12.2,3.90540811505039));
#300844=CARTESIAN_POINT('Ctrl Pts',(0.846764561790633,12.2,3.90460397331201));
#300845=CARTESIAN_POINT('Ctrl Pts',(0.846653981297917,12.2,3.90402963828343));
#300846=CARTESIAN_POINT('Ctrl Pts',(0.846598691051559,12.2,3.90374247076914));
#300847=CARTESIAN_POINT('Ctrl Pts',(0.846553019198255,12.2,3.90351273146421));
#300848=CARTESIAN_POINT('Ctrl Pts',(0.846518305619912,12.2,3.90334117504919));
#300849=CARTESIAN_POINT('Ctrl Pts',(0.846494840731448,12.2,3.90322521027874));
#300850=CARTESIAN_POINT('Ctrl Pts',(0.846476253679565,12.2,3.90313481853468));
#300851=CARTESIAN_POINT('Ctrl Pts',(0.846463233076636,12.2,3.90307263461551));
#300852=CARTESIAN_POINT('Ctrl Pts',(0.84645699120915,12.2,3.90304282464548));
#300853=CARTESIAN_POINT('Ctrl Pts',(0.846452319816075,12.2,3.90302108760437));
#300854=CARTESIAN_POINT('Ctrl Pts',(0.846447309728966,12.2,3.90299755605768));
#300855=CARTESIAN_POINT('',(0.768297694750895,12.2,3.54264641972273));
#300856=CARTESIAN_POINT('',(0.846447299999944,12.2,3.90299750499998));
#300857=CARTESIAN_POINT('',(1.30596997799994,12.2,3.38157765299999));
#300858=CARTESIAN_POINT('Origin',(-5.66300478732629E-14,12.2,-1.77635683940025E-14));
#300859=CARTESIAN_POINT('',(1.43881692432775,12.2,3.72556098059384));
#300860=CARTESIAN_POINT('',(1.30596997799994,12.2,3.38157765299999));
#300861=CARTESIAN_POINT('',(2.02484994999994,12.2,4.29679911999998));
#300862=CARTESIAN_POINT('Ctrl Pts',(1.43881701800443,12.2,3.72556094401147));
#300863=CARTESIAN_POINT('Ctrl Pts',(1.43891571542436,12.2,3.72581367906159));
#300864=CARTESIAN_POINT('Ctrl Pts',(1.43901824239838,12.1999999999997,3.72606491060791));
#300865=CARTESIAN_POINT('Ctrl Pts',(1.43933918812595,12.1999999999997,3.72684706398779));
#300866=CARTESIAN_POINT('Ctrl Pts',(1.43957531344741,12.2,3.72740719862251));
#300867=CARTESIAN_POINT('Ctrl Pts',(1.44062068239649,12.2,3.72984614017064));
#300868=CARTESIAN_POINT('Ctrl Pts',(1.44152373669993,12.1999999999078,3.73184446484589));
#300869=CARTESIAN_POINT('Ctrl Pts',(1.44557809881245,12.1999999999078,3.74055478896382));
#300870=CARTESIAN_POINT('Ctrl Pts',(1.44925055570118,12.1999999999078,3.74771538267329));
#300871=CARTESIAN_POINT('Ctrl Pts',(1.46590832509403,12.1999999999078,3.77852819662625));
#300872=CARTESIAN_POINT('Ctrl Pts',(1.48170041768112,12.2,3.80322417128525));
#300873=CARTESIAN_POINT('Ctrl Pts',(1.54222286540467,12.2,3.88973841319805));
#300874=CARTESIAN_POINT('Ctrl Pts',(1.60672952262203,12.2,3.96575969106281));
#300875=CARTESIAN_POINT('Ctrl Pts',(1.79561314049852,12.2,4.14059190618597));
#300876=CARTESIAN_POINT('Ctrl Pts',(1.9075685457603,12.2,4.22353887709006));
#300877=CARTESIAN_POINT('Ctrl Pts',(2.02484995028062,12.2,4.29679911955065));
#300878=CARTESIAN_POINT('',(2.32438124132219,12.2,4.14243308298023));
#300879=CARTESIAN_POINT('Origin',(-5.66300478732629E-14,12.2,-1.77635683940025E-14));
#300880=CARTESIAN_POINT('',(2.19921397760577,12.2,3.33366471456779));
#300881=CARTESIAN_POINT('Ctrl Pts',(2.32438124099994,12.2,4.14243308299998));
#300882=CARTESIAN_POINT('Ctrl Pts',(2.33276945463597,12.2,4.00447590820319));
#300883=CARTESIAN_POINT('Ctrl Pts',(2.33018902391579,12.2,3.86552790147597));
#300884=CARTESIAN_POINT('Ctrl Pts',(2.29756209278249,12.2,3.61065448254086));
#300885=CARTESIAN_POINT('Ctrl Pts',(2.27310042612445,12.2,3.51362648008036));
#300886=CARTESIAN_POINT('Ctrl Pts',(2.2375381345951,12.2,3.41353790557386));
#300887=CARTESIAN_POINT('Ctrl Pts',(2.22657068478963,12.2000000000756,3.38631279890763));
#300888=CARTESIAN_POINT('Ctrl Pts',(2.21112646047588,12.2000000000756,3.35486547673215));
#300889=CARTESIAN_POINT('Ctrl Pts',(2.20743003282668,12.2000000000756,3.34773476935894));
#300890=CARTESIAN_POINT('Ctrl Pts',(2.20270375929611,12.2000000000756,3.33941537254005));
#300891=CARTESIAN_POINT('Ctrl Pts',(2.20160840104712,12.2,3.33753660556523));
#300892=CARTESIAN_POINT('Ctrl Pts',(2.20024479446,12.2,3.33529963498368));
#300893=CARTESIAN_POINT('Ctrl Pts',(2.19993114734272,12.2000000000005,3.33479192891932));
#300894=CARTESIAN_POINT('Ctrl Pts',(2.19957309575045,12.2000000000005,3.33422465248725));
#300895=CARTESIAN_POINT('Ctrl Pts',(2.19936920503646,12.2,3.33390204975526));
#300896=CARTESIAN_POINT('Ctrl Pts',(2.19921392137674,12.2,3.33366475136423));
#300897=CARTESIAN_POINT('',(1.99616775954023,12.2,3.02587826526674));
#300898=CARTESIAN_POINT('',(2.19921392199994,12.2,3.33366475199998));
#300899=CARTESIAN_POINT('',(2.43934748299994,12.2,2.68145648099999));
#300900=CARTESIAN_POINT('Origin',(-5.66300478732629E-14,12.2,-1.77635683940025E-14));
#300901=CARTESIAN_POINT('',(2.68748468083623,12.2,2.9542215299112));
#300902=CARTESIAN_POINT('',(2.43934748299994,12.2,2.68145648099999));
#300903=CARTESIAN_POINT('',(3.44029922199995,12.2,3.27518568399999));
#300904=CARTESIAN_POINT('Ctrl Pts',(2.68748475499994,12.2,2.95422146199999));
#300905=CARTESIAN_POINT('Ctrl Pts',(2.68766810418239,12.2,2.95442145981663));
#300906=CARTESIAN_POINT('Ctrl Pts',(2.68785444461358,12.1999999999997,2.95461870580728));
#300907=CARTESIAN_POINT('Ctrl Pts',(2.68843649977677,12.1999999999997,2.95523235155731));
#300908=CARTESIAN_POINT('Ctrl Pts',(2.68885952550013,12.2,2.95566986667335));
#300909=CARTESIAN_POINT('Ctrl Pts',(2.6907140028693,12.2,2.95756511229716));
#300910=CARTESIAN_POINT('Ctrl Pts',(2.69227789133226,12.1999999999079,2.95910224681046));
#300911=CARTESIAN_POINT('Ctrl Pts',(2.69920541755507,12.1999999999079,2.96576016437954));
#300912=CARTESIAN_POINT('Ctrl Pts',(2.70521670352856,12.1999999999079,2.97111070509354));
#300913=CARTESIAN_POINT('Ctrl Pts',(2.73188047686284,12.1999999999079,2.99382533939136));
#300914=CARTESIAN_POINT('Ctrl Pts',(2.75552513406558,12.2,3.01114739782507));
#300915=CARTESIAN_POINT('Ctrl Pts',(2.84363361994914,12.2,3.07023822782865));
#300916=CARTESIAN_POINT('Ctrl Pts',(2.93139608331567,12.2,3.11776816464238));
#300917=CARTESIAN_POINT('Ctrl Pts',(3.17016487496149,12.2,3.21235683542494));
#300918=CARTESIAN_POINT('Ctrl Pts',(3.30518397689249,12.2,3.24937563452363));
#300919=CARTESIAN_POINT('Ctrl Pts',(3.44029922199995,12.2,3.27518568399999));
#300920=CARTESIAN_POINT('',(3.66384038699994,12.2,3.02304045899999));
#300921=CARTESIAN_POINT('Origin',(-5.66300478732629E-14,12.2,-1.77635683940025E-14));
#300922=CARTESIAN_POINT('',(3.25496455695711,12.2,2.31410204699751));
#300923=CARTESIAN_POINT('Ctrl Pts',(3.66384038663958,12.2,3.0230404588706));
#300924=CARTESIAN_POINT('Ctrl Pts',(3.65004021639256,12.2,2.97979079468028));
#300925=CARTESIAN_POINT('Ctrl Pts',(3.6355410673424,12.2,2.93830654304683));
#300926=CARTESIAN_POINT('Ctrl Pts',(3.62051781872112,12.2,2.89867000875219));
#300927=CARTESIAN_POINT('Ctrl Pts',(3.60181539509289,12.2,2.84932653623033));
#300928=CARTESIAN_POINT('Ctrl Pts',(3.58230031128659,12.2,2.80284793622846));
#300929=CARTESIAN_POINT('Ctrl Pts',(3.56235203927954,12.2,2.75937773445781));
#300930=CARTESIAN_POINT('Ctrl Pts',(3.54321245661152,12.2,2.71766978501283));
#300931=CARTESIAN_POINT('Ctrl Pts',(3.52367400370563,12.2,2.67873141952692));
#300932=CARTESIAN_POINT('Ctrl Pts',(3.50411306518538,12.2,2.64266933700222));
#300933=CARTESIAN_POINT('Ctrl Pts',(3.48530900365763,12.2,2.60800261495761));
#300934=CARTESIAN_POINT('Ctrl Pts',(3.46648405527645,12.2,2.57599404382551));
#300935=CARTESIAN_POINT('Ctrl Pts',(3.4480130972279,12.2,2.54671742996617));
#300936=CARTESIAN_POINT('Ctrl Pts',(3.43017328439979,12.2,2.51844118624785));
#300937=CARTESIAN_POINT('Ctrl Pts',(3.41266347568383,12.2,2.49271356238918));
#300938=CARTESIAN_POINT('Ctrl Pts',(3.39586256226689,12.2,2.46957875447664));
#300939=CARTESIAN_POINT('Ctrl Pts',(3.37963335056515,12.2,2.44723117812919));
#300940=CARTESIAN_POINT('Ctrl Pts',(3.36406534738878,12.2,2.42730316202406));
#300941=CARTESIAN_POINT('Ctrl Pts',(3.3495426582697,12.2,2.40981071661852));
#300942=CARTESIAN_POINT('Ctrl Pts',(3.33613594551948,12.2,2.39366245448001));
#300943=CARTESIAN_POINT('Ctrl Pts',(3.32362008334591,12.2,2.37958984249667));
#300944=CARTESIAN_POINT('Ctrl Pts',(3.3123355631942,12.2,2.36758366996853));
#300945=CARTESIAN_POINT('Ctrl Pts',(3.30155454011509,12.2,2.35611319347705));
#300946=CARTESIAN_POINT('Ctrl Pts',(3.29189718479154,12.2,2.34652900741971));
#300947=CARTESIAN_POINT('Ctrl Pts',(3.28369897633022,12.2,2.33880100197491));
#300948=CARTESIAN_POINT('Ctrl Pts',(3.27585943539416,12.2,2.33141109290826));
#300949=CARTESIAN_POINT('Ctrl Pts',(3.26935383400655,12.2,2.3257186557819));
#300950=CARTESIAN_POINT('Ctrl Pts',(3.26451584584619,12.2,2.32167436186622));
#300951=CARTESIAN_POINT('Ctrl Pts',(3.26162365731134,12.2,2.31925665018384));
#300952=CARTESIAN_POINT('Ctrl Pts',(3.25932822240677,12.2,2.31742748566471));
#300953=CARTESIAN_POINT('Ctrl Pts',(3.25770916214891,12.2,2.31617162237947));
#300954=CARTESIAN_POINT('Ctrl Pts',(3.25689963201998,12.2,2.31554369073685));
#300955=CARTESIAN_POINT('Ctrl Pts',(3.25625928522045,12.2,2.3150590283412));
#300956=CARTESIAN_POINT('Ctrl Pts',(3.25579882407171,12.2,2.31471533066125));
#300957=CARTESIAN_POINT('Ctrl Pts',(3.25556859349734,12.2,2.31454348182128));
#300958=CARTESIAN_POINT('Ctrl Pts',(3.25538328548142,12.2,2.31440688227762));
#300959=CARTESIAN_POINT('Ctrl Pts',(3.2552443668341,12.2,2.31430519881979));
#300960=CARTESIAN_POINT('Ctrl Pts',(3.25514984661369,12.2,2.31423601341501));
#300961=CARTESIAN_POINT('Ctrl Pts',(3.25507590025553,12.2,2.31418223108013));
#300962=CARTESIAN_POINT('Ctrl Pts',(3.25502519035787,12.2,2.31414564573923));
#300963=CARTESIAN_POINT('Ctrl Pts',(3.25500137069604,12.2,2.31412846072234));
#300964=CARTESIAN_POINT('Ctrl Pts',(3.25498365476425,12.2,2.31411582124383));
#300965=CARTESIAN_POINT('Ctrl Pts',(3.25496456102782,12.2,2.3141021319611));
#300966=CARTESIAN_POINT('',(2.95444430678277,12.2,2.10044848453536));
#300967=CARTESIAN_POINT('',(3.25496451799994,12.2,2.31410210199999));
#300968=CARTESIAN_POINT('',(3.24327759199994,12.2,1.61918975399999));
#300969=CARTESIAN_POINT('Origin',(-5.66300478732629E-14,12.2,-1.77635683940025E-14));
#300970=CARTESIAN_POINT('',(3.57319274026315,12.2,1.78389809210464));
#300971=CARTESIAN_POINT('',(3.24327759199994,12.2,1.61918975399999));
#300972=CARTESIAN_POINT('',(4.39111701799995,12.2,1.81124027399999));
#300973=CARTESIAN_POINT('Ctrl Pts',(3.57320811899994,12.2,1.78390558399999));
#300974=CARTESIAN_POINT('Ctrl Pts',(3.573471434563,12.2,1.78403581721233));
#300975=CARTESIAN_POINT('Ctrl Pts',(3.57385384963781,12.1999999999998,1.78421671185872));
#300976=CARTESIAN_POINT('Ctrl Pts',(3.57444583390415,12.1999999999998,1.78449699969217));
#300977=CARTESIAN_POINT('Ctrl Pts',(3.57499885979161,12.2,1.78475240106916));
#300978=CARTESIAN_POINT('Ctrl Pts',(3.57741451025376,12.2,1.78585050902155));
#300979=CARTESIAN_POINT('Ctrl Pts',(3.57942953936059,12.1999999999353,1.78671951455766));
#300980=CARTESIAN_POINT('Ctrl Pts',(3.58830406673956,12.1999999999353,1.79042908219111));
#300981=CARTESIAN_POINT('Ctrl Pts',(3.59584781630494,12.1999999999353,1.79324846166707));
#300982=CARTESIAN_POINT('Ctrl Pts',(3.62895086887599,12.1999999999353,1.80480706665112));
#300983=CARTESIAN_POINT('Ctrl Pts',(3.65729094241754,12.2,1.81242373874791));
#300984=CARTESIAN_POINT('Ctrl Pts',(3.76042940298413,12.2,1.83560201230679));
#300985=CARTESIAN_POINT('Ctrl Pts',(3.85943144621604,12.2,1.84831099332293));
#300986=CARTESIAN_POINT('Ctrl Pts',(4.11673089669352,12.2,1.85021299219715));
#300987=CARTESIAN_POINT('Ctrl Pts',(4.2554861848505,12.2,1.83603990528381));
#300988=CARTESIAN_POINT('Ctrl Pts',(4.39111701799995,12.2,1.81124027399999));
#300989=CARTESIAN_POINT('',(4.50847758599994,12.2,1.49536946999998));
#300990=CARTESIAN_POINT('Origin',(-5.66300478732629E-14,12.2,-1.77635683940025E-14));
#300991=CARTESIAN_POINT('',(3.87111413641841,12.2,0.982007073016362));
#300992=CARTESIAN_POINT('Ctrl Pts',(4.50847758599994,12.2,1.49536947099998));
#300993=CARTESIAN_POINT('Ctrl Pts',(4.42189143693061,12.2,1.38796023687308));
#300994=CARTESIAN_POINT('Ctrl Pts',(4.32625365229783,12.2,1.28685002287302));
#300995=CARTESIAN_POINT('Ctrl Pts',(4.13004445467292,12.2,1.12014543536591));
#300996=CARTESIAN_POINT('Ctrl Pts',(4.04660568678907,12.2,1.06503627533653));
#300997=CARTESIAN_POINT('Ctrl Pts',(3.95325368265746,12.2,1.01521924022475));
#300998=CARTESIAN_POINT('Ctrl Pts',(3.92680090281939,12.2000000000757,1.00248483664623));
#300999=CARTESIAN_POINT('Ctrl Pts',(3.89420290683788,12.2000000000757,0.989650213179769));
#301000=CARTESIAN_POINT('Ctrl Pts',(3.88666701235301,12.2000000000757,0.98687056215581));
#301001=CARTESIAN_POINT('Ctrl Pts',(3.8775671417713,12.2000000000757,0.983905758842116));
#301002=CARTESIAN_POINT('Ctrl Pts',(3.87549245275233,12.2,0.983255419398263));
#301003=CARTESIAN_POINT('Ctrl Pts',(3.87297812162379,12.2,0.982521063410915));
#301004=CARTESIAN_POINT('Ctrl Pts',(3.87240393490892,12.2000000000005,0.982357051593943));
#301005=CARTESIAN_POINT('Ctrl Pts',(3.87161345090973,12.2000000000005,0.982139498976519));
#301006=CARTESIAN_POINT('Ctrl Pts',(3.87136421885209,12.2,0.982071645256235));
#301007=CARTESIAN_POINT('Ctrl Pts',(3.87111411939993,12.2,0.982007138999299));
#301008=CARTESIAN_POINT('',(3.51370678013976,12.2,0.891341496431592));
#301009=CARTESIAN_POINT('',(3.87111411999994,12.2,0.982007138999985));
#301010=CARTESIAN_POINT('',(3.60918509199994,12.2,0.338242477999984));
#301011=CARTESIAN_POINT('Origin',(-5.66300478732629E-14,12.2,-1.77635683940025E-14));
#301012=CARTESIAN_POINT('',(3.97632131980427,12.2,0.372649332160937));
#301013=CARTESIAN_POINT('',(3.60918509199994,12.2,0.338242477999984));
#301014=CARTESIAN_POINT('',(4.74889012999994,12.2,0.102676828999986));
#301015=CARTESIAN_POINT('Ctrl Pts',(3.97632132878368,12.2,0.372649232070297));
#301016=CARTESIAN_POINT('Ctrl Pts',(3.97659156631608,12.2,0.372673475831972));
#301017=CARTESIAN_POINT('Ctrl Pts',(3.97686215349336,12.1999999999997,0.372693740160113));
#301018=CARTESIAN_POINT('Ctrl Pts',(3.97770753758359,12.1999999999997,0.372755234620468));
#301019=CARTESIAN_POINT('Ctrl Pts',(3.97831516441626,12.2,0.372793558096753));
#301020=CARTESIAN_POINT('Ctrl Pts',(3.98096065091767,12.2,0.372944703878524));
#301021=CARTESIAN_POINT('Ctrl Pts',(3.98315053462491,12.1999999999078,0.373027030774091));
#301022=CARTESIAN_POINT('Ctrl Pts',(3.99275999528421,12.1999999999078,0.373280365470712));
#301023=CARTESIAN_POINT('Ctrl Pts',(4.00080741751491,12.1999999999078,0.373184467362426));
#301024=CARTESIAN_POINT('Ctrl Pts',(4.03581303640557,12.1999999999078,0.372007587291399));
#301025=CARTESIAN_POINT('Ctrl Pts',(4.06496098547899,12.2,0.368878531427779));
#301026=CARTESIAN_POINT('Ctrl Pts',(4.16957554102918,12.2,0.353234892688601));
#301027=CARTESIAN_POINT('Ctrl Pts',(4.26641642627047,12.2,0.329317758609609));
#301028=CARTESIAN_POINT('Ctrl Pts',(4.5068681474629,12.2,0.238257898338845));
#301029=CARTESIAN_POINT('Ctrl Pts',(4.63107293515098,12.2,0.174983763566832));
#301030=CARTESIAN_POINT('Ctrl Pts',(4.74889012955414,12.2,0.102676828273587));
#301031=CARTESIAN_POINT('',(4.74421990499994,12.2,-0.234259451000014));
#301032=CARTESIAN_POINT('Origin',(-5.66300478732629E-14,12.2,-1.77635683940025E-14));
#301033=CARTESIAN_POINT('',(3.9644482997684,12.2,-0.482713394198715));
#301034=CARTESIAN_POINT('Ctrl Pts',(4.74421990499994,12.2,-0.234259451000014));
#301035=CARTESIAN_POINT('Ctrl Pts',(4.71280838274439,12.2,-0.252358422706553));
#301036=CARTESIAN_POINT('Ctrl Pts',(4.68182628481682,12.2,-0.269325626376228));
#301037=CARTESIAN_POINT('Ctrl Pts',(4.65136663428666,12.2,-0.285188901941369));
#301038=CARTESIAN_POINT('Ctrl Pts',(4.60376418654431,12.2,-0.309980084143681));
#301039=CARTESIAN_POINT('Ctrl Pts',(4.55743821394982,12.2,-0.33207332577565));
#301040=CARTESIAN_POINT('Ctrl Pts',(4.51276566604218,12.2,-0.351611995871092));
#301041=CARTESIAN_POINT('Ctrl Pts',(4.46966970825717,12.2,-0.370461104351526));
#301042=CARTESIAN_POINT('Ctrl Pts',(4.42811254063867,12.2,-0.386932586665946));
#301043=CARTESIAN_POINT('Ctrl Pts',(4.38844978019863,12.2,-0.40119795231803));
#301044=CARTESIAN_POINT('Ctrl Pts',(4.35014417590209,12.2,-0.414975194389727));
#301045=CARTESIAN_POINT('Ctrl Pts',(4.31360554684493,12.2,-0.426694489899858));
#301046=CARTESIAN_POINT('Ctrl Pts',(4.27917057492761,12.2,-0.436554070185109));
#301047=CARTESIAN_POINT('Ctrl Pts',(4.24599813772591,12.2,-0.446052155696343));
#301048=CARTESIAN_POINT('Ctrl Pts',(4.21477788342143,12.2,-0.453824144641168));
#301049=CARTESIAN_POINT('Ctrl Pts',(4.18582653151251,12.2,-0.460092073302094));
#301050=CARTESIAN_POINT('Ctrl Pts',(4.15829129016377,12.2,-0.466053415935704));
#301051=CARTESIAN_POINT('Ctrl Pts',(4.13280837037226,12.2,-0.470654038415366));
#301052=CARTESIAN_POINT('Ctrl Pts',(4.10966513089301,12.2,-0.474129271609313));
#301053=CARTESIAN_POINT('Ctrl Pts',(4.08747104362572,12.2,-0.477461978288073));
#301054=CARTESIAN_POINT('Ctrl Pts',(4.06742854151838,12.2,-0.47975942539362));
#301055=CARTESIAN_POINT('Ctrl Pts',(4.04980584225301,12.2,-0.48127457959937));
#301056=CARTESIAN_POINT('Ctrl Pts',(4.03332992873515,12.2,-0.482691136125943));
#301057=CARTESIAN_POINT('Ctrl Pts',(4.01896907893941,12.2,-0.483423742151229));
#301058=CARTESIAN_POINT('Ctrl Pts',(4.00695638984246,12.2,-0.483722451718041));
#301059=CARTESIAN_POINT('Ctrl Pts',(3.99549310337372,12.2,-0.484007499745812));
#301060=CARTESIAN_POINT('Ctrl Pts',(3.98616799207043,12.2,-0.483897081035411));
#301061=CARTESIAN_POINT('Ctrl Pts',(3.97919795030351,12.2,-0.483652861953002));
#301062=CARTESIAN_POINT('Ctrl Pts',(3.97461628623507,12.2,-0.483492327793793));
#301063=CARTESIAN_POINT('Ctrl Pts',(3.97105251234585,12.2,-0.483274855533071));
#301064=CARTESIAN_POINT('Ctrl Pts',(3.96857238495118,12.2,-0.483087409556649));
#301065=CARTESIAN_POINT('Ctrl Pts',(3.96733232125385,12.2,-0.482993686568438));
#301066=CARTESIAN_POINT('Ctrl Pts',(3.96636321862757,12.2,-0.482907633051564));
#301067=CARTESIAN_POINT('Ctrl Pts',(3.96567368282888,12.2,-0.482841249840966));
#301068=CARTESIAN_POINT('Ctrl Pts',(3.96532891492954,12.2,-0.482808058235667));
#301069=CARTESIAN_POINT('Ctrl Pts',(3.965054037478,12.2,-0.482779787357501));
#301070=CARTESIAN_POINT('Ctrl Pts',(3.96485014744288,12.2,-0.48275801329454));
#301071=CARTESIAN_POINT('Ctrl Pts',(3.96472015919018,12.2,-0.482744131437113));
#301072=CARTESIAN_POINT('Ctrl Pts',(3.96461946383355,12.2,-0.482732997352684));
#301073=CARTESIAN_POINT('Ctrl Pts',(3.96454657132337,12.2,-0.482724755568015));
#301074=CARTESIAN_POINT('Ctrl Pts',(3.96450512999067,12.2,-0.482720069894005));
#301075=CARTESIAN_POINT('Ctrl Pts',(3.96447771970708,12.2,-0.482716794149493));
#301076=CARTESIAN_POINT('Ctrl Pts',(3.96444835997019,12.2,-0.482713334252444));
#301077=CARTESIAN_POINT('',(3.5984236820905,12.2,-0.438146098542558));
#301078=CARTESIAN_POINT('',(3.96444830899994,12.2,-0.482713328000015));
#301079=CARTESIAN_POINT('',(3.48765214499994,12.2,-0.988386318000014));
#301080=CARTESIAN_POINT('Origin',(-5.66300478732629E-14,12.2,-1.77635683940025E-14));
#301081=CARTESIAN_POINT('',(3.84242567103147,12.2,-1.0889277859801));
#301082=CARTESIAN_POINT('',(3.48765214499994,12.2,-0.988386318000014));
#301083=CARTESIAN_POINT('',(4.46529931499995,12.2,-1.61975369200002));
#301084=CARTESIAN_POINT('Ctrl Pts',(3.84242564315659,12.2,-1.088927883045));
#301085=CARTESIAN_POINT('Ctrl Pts',(3.84268642756792,12.2,-1.0890027745344));
#301086=CARTESIAN_POINT('Ctrl Pts',(3.84294603075642,12.1999999999997,-1.089081747968));
#301087=CARTESIAN_POINT('Ctrl Pts',(3.84375517486719,12.1999999999997,-1.08932937765328));
#301088=CARTESIAN_POINT('Ctrl Pts',(3.84433532277453,12.2,-1.08951302470086));
#301089=CARTESIAN_POINT('Ctrl Pts',(3.84685853713855,12.2,-1.09032831431401));
#301090=CARTESIAN_POINT('Ctrl Pts',(3.84893005724474,12.1999999999081,-1.09104255104995));
#301091=CARTESIAN_POINT('Ctrl Pts',(3.85798372485354,12.1999999999081,-1.09427822963628));
#301092=CARTESIAN_POINT('Ctrl Pts',(3.86545613666242,12.1999999999081,-1.09727610859554));
#301093=CARTESIAN_POINT('Ctrl Pts',(3.89766100957131,12.1999999999081,-1.111014062726));
#301094=CARTESIAN_POINT('Ctrl Pts',(3.92371080997547,12.2,-1.12446042846844));
#301095=CARTESIAN_POINT('Ctrl Pts',(4.01543103001572,12.2,-1.17673704252015));
#301096=CARTESIAN_POINT('Ctrl Pts',(4.09709048001922,12.2,-1.2339590057417));
#301097=CARTESIAN_POINT('Ctrl Pts',(4.28857034295747,12.2,-1.40587505111375));
#301098=CARTESIAN_POINT('Ctrl Pts',(4.38130822209624,12.2,-1.50944072497096));
#301099=CARTESIAN_POINT('Ctrl Pts',(4.46529931499995,12.2,-1.61975369200002));
#301100=CARTESIAN_POINT('',(4.33922903699994,12.2,-1.93225033600001));
#301101=CARTESIAN_POINT('Origin',(-5.66300478732629E-14,12.2,-1.77635683940025E-14));
#301102=CARTESIAN_POINT('',(3.52236175392628,12.2,-1.88224074466015));
#301103=CARTESIAN_POINT('Ctrl Pts',(4.33922903699994,12.2,-1.93225033600001));
#301104=CARTESIAN_POINT('Ctrl Pts',(4.29900656514174,12.2,-1.93845813259177));
#301105=CARTESIAN_POINT('Ctrl Pts',(4.25980390494279,12.2,-1.94353103969836));
#301106=CARTESIAN_POINT('Ctrl Pts',(4.22172995537545,12.2,-1.94755436125775));
#301107=CARTESIAN_POINT('Ctrl Pts',(4.16871119947665,12.2,-1.95315691907179));
#301108=CARTESIAN_POINT('Ctrl Pts',(4.11788223931045,12.2,-1.9567229568601));
#301109=CARTESIAN_POINT('Ctrl Pts',(4.06954307521643,12.2,-1.95852644618014));
#301110=CARTESIAN_POINT('Ctrl Pts',(4.02325836860018,12.2,-1.96025328559965));
#301111=CARTESIAN_POINT('Ctrl Pts',(3.97925644296878,12.2,-1.96036409029778));
#301112=CARTESIAN_POINT('Ctrl Pts',(3.93780116827124,12.2,-1.95914487990857));
#301113=CARTESIAN_POINT('Ctrl Pts',(3.89739186390891,12.2,-1.95795643177842));
#301114=CARTESIAN_POINT('Ctrl Pts',(3.8594024213275,12.2,-1.95550391043724));
#301115=CARTESIAN_POINT('Ctrl Pts',(3.82407655579394,12.2,-1.95209965533137));
#301116=CARTESIAN_POINT('Ctrl Pts',(3.78997061682712,12.2,-1.94881296114527));
#301117=CARTESIAN_POINT('Ctrl Pts',(3.75834756381887,12.2,-1.94463885468989));
#301118=CARTESIAN_POINT('Ctrl Pts',(3.72942509982425,12.2,-1.9399073151758));
#301119=CARTESIAN_POINT('Ctrl Pts',(3.70208784783339,12.2,-1.9354351067213));
#301120=CARTESIAN_POINT('Ctrl Pts',(3.67716330263961,12.2,-1.93046473194123));
#301121=CARTESIAN_POINT('Ctrl Pts',(3.65483308074296,12.2,-1.92532209267641));
#301122=CARTESIAN_POINT('Ctrl Pts',(3.63387548666265,12.2,-1.92049556893149));
#301123=CARTESIAN_POINT('Ctrl Pts',(3.61520310657084,12.2,-1.91551717163214));
#301124=CARTESIAN_POINT('Ctrl Pts',(3.59896359240005,12.2,-1.91070096211013));
#301125=CARTESIAN_POINT('Ctrl Pts',(3.58357139066594,12.2,-1.9061360430013));
#301126=CARTESIAN_POINT('Ctrl Pts',(3.57036483791297,12.2,-1.90171657509177));
#301127=CARTESIAN_POINT('Ctrl Pts',(3.55946707966078,12.2,-1.89775407406141));
#301128=CARTESIAN_POINT('Ctrl Pts',(3.54893209458809,12.2,-1.89392347989339));
#301129=CARTESIAN_POINT('Ctrl Pts',(3.54055478815737,12.2,-1.89051943439848));
#301130=CARTESIAN_POINT('Ctrl Pts',(3.53444369477347,12.2,-1.88787100387636));
#301131=CARTESIAN_POINT('Ctrl Pts',(3.53065572913985,12.2,-1.88622937231052));
#301132=CARTESIAN_POINT('Ctrl Pts',(3.52773843948522,12.2,-1.88487898787886));
#301133=CARTESIAN_POINT('Ctrl Pts',(3.52571707879089,12.2,-1.88390942517561));
#301134=CARTESIAN_POINT('Ctrl Pts',(3.52470639844372,12.2,-1.88342464382399));
#301135=CARTESIAN_POINT('Ctrl Pts',(3.52391969356645,12.2,-1.88303518981985));
#301136=CARTESIAN_POINT('Ctrl Pts',(3.52336008261798,12.2,-1.88275326165307));
#301137=CARTESIAN_POINT('Ctrl Pts',(3.52308027714375,12.2,-1.88261229756968));
#301138=CARTESIAN_POINT('Ctrl Pts',(3.52285723827716,12.2,-1.88249818746355));
#301139=CARTESIAN_POINT('Ctrl Pts',(3.52269136250471,12.2,-1.88241256318214));
#301140=CARTESIAN_POINT('Ctrl Pts',(3.52258193395062,12.2,-1.88235607668522));
#301141=CARTESIAN_POINT('Ctrl Pts',(3.52249703884443,12.2,-1.88231188564555));
#301142=CARTESIAN_POINT('Ctrl Pts',(3.52243726950848,12.2,-1.88228053212193));
#301143=CARTESIAN_POINT('Ctrl Pts',(3.52240643831652,12.2,-1.88226435883692));
#301144=CARTESIAN_POINT('Ctrl Pts',(3.5223850376344,12.2,-1.88225299025455));
#301145=CARTESIAN_POINT('Ctrl Pts',(3.52236183191156,12.2,-1.88224071016707));
#301146=CARTESIAN_POINT('',(3.19715352623975,12.2,-1.70845963654418));
#301147=CARTESIAN_POINT('',(3.52236178599994,12.2,-1.88224068600002));
#301148=CARTESIAN_POINT('',(2.89509245023569,12.2,-2.18152806526552));
#301149=CARTESIAN_POINT('Origin',(-5.66300478732629E-14,12.2,-1.77635683940025E-14));
#301150=CARTESIAN_POINT('',(3.1895891437794,12.2,-2.40343917166473));
#301151=CARTESIAN_POINT('',(2.89509244999994,12.2,-2.18152806500001));
#301152=CARTESIAN_POINT('',(3.57864508499994,12.2,-3.12342750100001));
#301153=CARTESIAN_POINT('Ctrl Pts',(3.18958908299994,12.2,-2.40343925200001));
#301154=CARTESIAN_POINT('Ctrl Pts',(3.18972664483265,12.2,-2.40354363799686));
#301155=CARTESIAN_POINT('Ctrl Pts',(3.19053877007493,12.2,-2.40417145281639));
#301156=CARTESIAN_POINT('Ctrl Pts',(3.19321480642603,12.2,-2.40634490153556));
#301157=CARTESIAN_POINT('Ctrl Pts',(3.19488796455418,12.1999999999079,-2.40775871102333));
#301158=CARTESIAN_POINT('Ctrl Pts',(3.20216212621672,12.1999999999079,-2.41404710203839));
#301159=CARTESIAN_POINT('Ctrl Pts',(3.20804455305006,12.1999999999079,-2.41953932649126));
#301160=CARTESIAN_POINT('Ctrl Pts',(3.23312051415152,12.1999999999079,-2.44399161344329));
#301161=CARTESIAN_POINT('Ctrl Pts',(3.25255277588417,12.2,-2.46594012204941));
#301162=CARTESIAN_POINT('Ctrl Pts',(3.31934274303239,12.2,-2.54800138031337));
#301163=CARTESIAN_POINT('Ctrl Pts',(3.37479477908212,12.2,-2.63092698918229));
#301164=CARTESIAN_POINT('Ctrl Pts',(3.49112749819354,12.2,-2.86017974548445));
#301165=CARTESIAN_POINT('Ctrl Pts',(3.54028648814989,12.2,-2.99060729942287));
#301166=CARTESIAN_POINT('Ctrl Pts',(3.57864508499994,12.2,-3.12342750100001));
#301167=CARTESIAN_POINT('',(3.34820124399994,12.2,-3.36928010500001));
#301168=CARTESIAN_POINT('Origin',(-5.66300478732629E-14,12.2,-1.77635683940025E-14));
#301169=CARTESIAN_POINT('',(2.60456073403712,12.2,-3.02756105307893));
#301170=CARTESIAN_POINT('Ctrl Pts',(3.34820124399994,12.2,-3.36928010500001));
#301171=CARTESIAN_POINT('Ctrl Pts',(3.31610338031493,12.2,-3.36222132135304));
#301172=CARTESIAN_POINT('Ctrl Pts',(3.28489316543702,12.2,-3.35471299742094));
#301173=CARTESIAN_POINT('Ctrl Pts',(3.25460746644452,12.2,-3.34681680642958));
#301174=CARTESIAN_POINT('Ctrl Pts',(3.20231260989431,12.2,-3.33318231262812));
#301175=CARTESIAN_POINT('Ctrl Pts',(3.15277628079259,12.2,-3.31839009953227));
#301176=CARTESIAN_POINT('Ctrl Pts',(3.10618228623555,12.2,-3.30279915010095));
#301177=CARTESIAN_POINT('Ctrl Pts',(3.06109729991451,12.2,-3.28771313422004));
#301178=CARTESIAN_POINT('Ctrl Pts',(3.01876729021624,12.2000000000001,-3.27187911778594));
#301179=CARTESIAN_POINT('Ctrl Pts',(2.97934262927457,12.2,-3.2556658918671));
#301180=CARTESIAN_POINT('Ctrl Pts',(2.94147455473056,12.1999999999999,-3.2400928055544));
#301181=CARTESIAN_POINT('Ctrl Pts',(2.90628704421913,12.2,-3.22416976229994));
#301182=CARTESIAN_POINT('Ctrl Pts',(2.87389618604026,12.2,-3.20826646750966));
#301183=CARTESIAN_POINT('Ctrl Pts',(2.84258537401118,12.2,-3.19289345481974));
#301184=CARTESIAN_POINT('Ctrl Pts',(2.81388796074758,12.2,-3.17753868749481));
#301185=CARTESIAN_POINT('Ctrl Pts',(2.78789027600534,12.2,-3.16257980667675));
#301186=CARTESIAN_POINT('Ctrl Pts',(2.76293364575501,12.2,-3.14821994112579));
#301187=CARTESIAN_POINT('Ctrl Pts',(2.74046502013137,12.1999999999999,-3.13422463962054));
#301188=CARTESIAN_POINT('Ctrl Pts',(2.72054127763874,12.2,-3.12097215534773));
#301189=CARTESIAN_POINT('Ctrl Pts',(2.70141897153072,12.2000000000001,-3.1082527548109));
#301190=CARTESIAN_POINT('Ctrl Pts',(2.68464109606858,12.2,-3.0962173287529));
#301191=CARTESIAN_POINT('Ctrl Pts',(2.67023747516043,12.2,-3.08524559523614));
#301192=CARTESIAN_POINT('Ctrl Pts',(2.65700458237695,12.2,-3.0751656456039));
#301193=CARTESIAN_POINT('Ctrl Pts',(2.64577568833732,12.2,-3.06598350134236));
#301194=CARTESIAN_POINT('Ctrl Pts',(2.63655542330602,12.2,-3.05803422841789));
#301195=CARTESIAN_POINT('Ctrl Pts',(2.6277125659735,12.2,-3.050410338418));
#301196=CARTESIAN_POINT('Ctrl Pts',(2.62071741312198,12.2,-3.04392007669833));
#301197=CARTESIAN_POINT('Ctrl Pts',(2.61555497849679,12.2,-3.03890099424192));
#301198=CARTESIAN_POINT('Ctrl Pts',(2.61203910333727,12.2,-3.03548274905079));
#301199=CARTESIAN_POINT('Ctrl Pts',(2.60937292520829,12.2,-3.032747694406));
#301200=CARTESIAN_POINT('Ctrl Pts',(2.60754559550129,12.2,-3.03081602249089));
#301201=CARTESIAN_POINT('Ctrl Pts',(2.60663193064778,12.2,-3.02985018653334));
#301202=CARTESIAN_POINT('Ctrl Pts',(2.6059279015729,12.2,-3.02908537937573));
#301203=CARTESIAN_POINT('Ctrl Pts',(2.60543160098027,12.2,-3.02853785707786));
#301204=CARTESIAN_POINT('Ctrl Pts',(2.60518345068395,12.2,-3.02826409592892));
#301205=CARTESIAN_POINT('Ctrl Pts',(2.60498722709952,12.2,-3.02804467705542));
#301206=CARTESIAN_POINT('Ctrl Pts',(2.60484265807629,12.2,-3.02788168440645));
#301207=CARTESIAN_POINT('Ctrl Pts',(2.60475225973617,12.2,-3.02777976585854));
#301208=CARTESIAN_POINT('Ctrl Pts',(2.60468246168515,12.2,-3.02770047411044));
#301209=CARTESIAN_POINT('Ctrl Pts',(2.60463169836712,12.2,-3.02764248669049));
#301210=CARTESIAN_POINT('Ctrl Pts',(2.60460127874204,12.2,-3.02760773806407));
#301211=CARTESIAN_POINT('Ctrl Pts',(2.60458156576711,12.2,-3.0275849736035));
#301212=CARTESIAN_POINT('Ctrl Pts',(2.60456081971581,12.2,-3.02756104824639));
#301213=CARTESIAN_POINT('',(2.36409006999994,12.2,-2.74803623300001));
#301214=CARTESIAN_POINT('',(2.60456078499995,12.2,-3.02756100900002));
#301215=CARTESIAN_POINT('',(1.91153447899994,12.2,-3.08004235900002));
#301216=CARTESIAN_POINT('Origin',(-5.66300478732629E-14,12.2,-1.77635683940025E-14));
#301217=CARTESIAN_POINT('',(2.10598092973928,12.2,-3.39335277979123));
#301218=CARTESIAN_POINT('',(1.91153447899994,12.2,-3.08004235900002));
#301219=CARTESIAN_POINT('',(2.20867500599994,12.2,-4.20526511800002));
#301220=CARTESIAN_POINT('Ctrl Pts',(2.10598084399995,12.2,-3.39335283300001));
#301221=CARTESIAN_POINT('Ctrl Pts',(2.10612311054997,12.2,-3.39358400226231));
#301222=CARTESIAN_POINT('Ctrl Pts',(2.10626187270212,12.1999999999997,-3.39381731953339));
#301223=CARTESIAN_POINT('Ctrl Pts',(2.10669328388901,12.1999999999997,-3.39454590594761));
#301224=CARTESIAN_POINT('Ctrl Pts',(2.10699833127559,12.2,-3.39507253151456));
#301225=CARTESIAN_POINT('Ctrl Pts',(2.1083141818034,12.2,-3.39737572880188));
#301226=CARTESIAN_POINT('Ctrl Pts',(2.10936495438345,12.199999999924,-3.39930115367447));
#301227=CARTESIAN_POINT('Ctrl Pts',(2.11387550924077,12.199999999924,-3.40779148964373));
#301228=CARTESIAN_POINT('Ctrl Pts',(2.11737859461051,12.199999999924,-3.41504199950801));
#301229=CARTESIAN_POINT('Ctrl Pts',(2.13193416739489,12.199999999924,-3.44691753809593));
#301230=CARTESIAN_POINT('Ctrl Pts',(2.14212952196091,12.2,-3.47441825103592));
#301231=CARTESIAN_POINT('Ctrl Pts',(2.17477097005074,12.2,-3.57510296880395));
#301232=CARTESIAN_POINT('Ctrl Pts',(2.19652755494506,12.2,-3.67250735829484));
#301233=CARTESIAN_POINT('Ctrl Pts',(2.2221638801155,12.2,-3.92833258330708));
#301234=CARTESIAN_POINT('Ctrl Pts',(2.22086610698297,12.2,-4.06779136454917));
#301235=CARTESIAN_POINT('Ctrl Pts',(2.20867500608793,12.2,-4.20526511800782));
#301236=CARTESIAN_POINT('',(1.90498031899994,12.2,-4.35126992700001));
#301237=CARTESIAN_POINT('Origin',(-5.66300478732629E-14,12.2,-1.77635683940025E-14));
#301238=CARTESIAN_POINT('Ctrl Pts',(1.90498031853915,12.2,-4.3512699276941));
#301239=CARTESIAN_POINT('Ctrl Pts',(1.87731122367178,12.2,-4.33290102593718));
#301240=CARTESIAN_POINT('Ctrl Pts',(1.85065313309167,12.2,-4.31443155952546));
#301241=CARTESIAN_POINT('Ctrl Pts',(1.82501865469772,12.2,-4.29593456725834));
#301242=CARTESIAN_POINT('Ctrl Pts',(1.7814207545479,12.2,-4.26447576362908));
#301243=CARTESIAN_POINT('Ctrl Pts',(1.74078589202437,12.2,-4.23293703601144));
#301244=CARTESIAN_POINT('Ctrl Pts',(1.70315507361045,12.2,-4.20171407893944));
#301245=CARTESIAN_POINT('Ctrl Pts',(1.66677641164637,12.2,-4.17153005826926));
#301246=CARTESIAN_POINT('Ctrl Pts',(1.63320539722488,12.2000000000001,-4.14164105433643));
#301247=CARTESIAN_POINT('Ctrl Pts',(1.60244892133047,12.2,-4.11243861538496));
#301248=CARTESIAN_POINT('Ctrl Pts',(1.57273511323079,12.1999999999999,-4.08422616120049));
#301249=CARTESIAN_POINT('Ctrl Pts',(1.54564845580195,12.2,-4.0566544282747));
#301250=CARTESIAN_POINT('Ctrl Pts',(1.52116372005999,12.2,-4.03011018221668));
#301251=CARTESIAN_POINT('Ctrl Pts',(1.49762025163875,12.2,-4.004586377287));
#301252=CARTESIAN_POINT('Ctrl Pts',(1.47648269596018,12.2,-3.98001248487298));
#301253=CARTESIAN_POINT('Ctrl Pts',(1.45769623267052,12.2,-3.95676577818292));
#301254=CARTESIAN_POINT('Ctrl Pts',(1.43938836702436,12.2,-3.93411129680262));
#301255=CARTESIAN_POINT('Ctrl Pts',(1.42331361287325,12.1999999999999,-3.91271697766841));
#301256=CARTESIAN_POINT('Ctrl Pts',(1.40938606434272,12.2,-3.8929672821972));
#301257=CARTESIAN_POINT('Ctrl Pts',(1.39615307577568,12.2000000000001,-3.87420249428061));
#301258=CARTESIAN_POINT('Ctrl Pts',(1.38485861700844,12.2,-3.85692219250991));
#301259=CARTESIAN_POINT('Ctrl Pts',(1.37539340264988,12.2,-3.84149117465438));
#301260=CARTESIAN_POINT('Ctrl Pts',(1.36665980231613,12.2,-3.82725289778206));
#301261=CARTESIAN_POINT('Ctrl Pts',(1.3594835944762,12.2,-3.81458902219661));
#301262=CARTESIAN_POINT('Ctrl Pts',(1.35374651900545,12.2,-3.803817745772));
#301263=CARTESIAN_POINT('Ctrl Pts',(1.34830700444303,12.2,-3.79360513565971));
#301264=CARTESIAN_POINT('Ctrl Pts',(1.34416138735862,12.2,-3.78509367744774));
#301265=CARTESIAN_POINT('Ctrl Pts',(1.34117666537531,12.2,-3.7785860725486));
#301266=CARTESIAN_POINT('Ctrl Pts',(1.3391254676793,12.2,-3.77411383551939));
#301267=CARTESIAN_POINT('Ctrl Pts',(1.33762190934237,12.2,-3.77058860390923));
#301268=CARTESIAN_POINT('Ctrl Pts',(1.33661222385445,12.2,-3.76811909717029));
#301269=CARTESIAN_POINT('Ctrl Pts',(1.33610738111049,12.2,-3.76688434380082));
#301270=CARTESIAN_POINT('Ctrl Pts',(1.33572585904822,12.2,-3.76591366201497));
#301271=CARTESIAN_POINT('Ctrl Pts',(1.33545997377132,12.2,-3.76522160098899));
#301272=CARTESIAN_POINT('Ctrl Pts',(1.33532703113287,12.2,-3.764875570476));
#301273=CARTESIAN_POINT('Ctrl Pts',(1.33522298535505,12.2,-3.76459921215659));
#301274=CARTESIAN_POINT('Ctrl Pts',(1.33514682354475,12.2,-3.7643943808242));
#301275=CARTESIAN_POINT('Ctrl Pts',(1.33509927145191,12.2,-3.76426649312701));
#301276=CARTESIAN_POINT('Ctrl Pts',(1.33506277162764,12.2,-3.76416716393628));
#301277=CARTESIAN_POINT('Ctrl Pts',(1.33503630943865,12.2,-3.76409459607695));
#301278=CARTESIAN_POINT('Ctrl Pts',(1.3350203884622,12.2,-3.76405093562315));
#301279=CARTESIAN_POINT('Ctrl Pts',(1.33501018614367,12.2,-3.76402242543819));
#301280=CARTESIAN_POINT('Ctrl Pts',(1.33499943628452,12.2,-3.76399249025695));
#301281=CARTESIAN_POINT('',(-3.28892417320473,12.2,-1.19707050039253));
#301282=CARTESIAN_POINT('Origin',(-5.66300478732629E-14,12.2,-1.77635683940025E-14));
#301283=CARTESIAN_POINT('Origin',(-5.66300478732629E-14,5.2,-1.77635683940025E-14));
#301284=CARTESIAN_POINT('',(0.235377287932295,2.4,-2.99075200114047));
#301285=CARTESIAN_POINT('Origin',(-5.66300478732629E-14,2.4,-1.81064694828012E-14));
#301286=CARTESIAN_POINT('',(0.235377287932295,2.7,-2.99075200114047));
#301287=CARTESIAN_POINT('',(0.235377287932296,5.2,-2.99075200114047));
#301288=CARTESIAN_POINT('Origin',(-5.66300478732629E-14,2.7,-1.80697300804299E-14));
#301289=CARTESIAN_POINT('Origin',(-5.66300478732629E-14,2.4,-1.77268289916312E-14));
#301290=CARTESIAN_POINT('Origin',(-5.66300478732629E-14,15.2,-1.77635683940025E-14));
#301291=CARTESIAN_POINT('',(-1.39835267900006,2.7,4.53950545599999));
#301292=CARTESIAN_POINT('',(-1.39835267900006,12.2,4.53950545599999));
#301293=CARTESIAN_POINT('',(-1.07300065800006,2.7,4.62722050399999));
#301294=CARTESIAN_POINT('Origin',(-5.66300478732629E-14,2.7,-1.92943768261394E-14));
#301295=CARTESIAN_POINT('',(-1.07300065800006,12.2,4.62722050399999));
#301296=CARTESIAN_POINT('Ctrl Pts',(-1.39835267900006,12.2,4.53950545599999));
#301297=CARTESIAN_POINT('Ctrl Pts',(-1.39835267900006,5.2,4.53950545599999));
#301298=CARTESIAN_POINT('Ctrl Pts',(-1.39835267900006,2.2,4.53950545599999));
#301299=CARTESIAN_POINT('Ctrl Pts',(-1.39849651400006,12.2,4.53899223499998));
#301300=CARTESIAN_POINT('Ctrl Pts',(-1.39849651400006,5.2,4.53899223499998));
#301301=CARTESIAN_POINT('Ctrl Pts',(-1.39849651400006,2.2,4.53899223499998));
#301302=CARTESIAN_POINT('Ctrl Pts',(-1.39878382700006,12.2,4.53796604699999));
#301303=CARTESIAN_POINT('Ctrl Pts',(-1.39878382700006,5.2,4.53796604699999));
#301304=CARTESIAN_POINT('Ctrl Pts',(-1.39878382700006,2.2,4.53796604699999));
#301305=CARTESIAN_POINT('Ctrl Pts',(-1.39921373200006,12.2,4.53642752199999));
#301306=CARTESIAN_POINT('Ctrl Pts',(-1.39921373200006,5.2,4.53642752199999));
#301307=CARTESIAN_POINT('Ctrl Pts',(-1.39921373200006,2.2,4.53642752199999));
#301308=CARTESIAN_POINT('Ctrl Pts',(-1.39978480400006,12.2,4.53437767499998));
#301309=CARTESIAN_POINT('Ctrl Pts',(-1.39978480400006,5.2,4.53437767499998));
#301310=CARTESIAN_POINT('Ctrl Pts',(-1.39978480400006,2.2,4.53437767499998));
#301311=CARTESIAN_POINT('Ctrl Pts',(-1.40049509300006,12.2,4.53181789599999));
#301312=CARTESIAN_POINT('Ctrl Pts',(-1.40049509300006,5.2,4.53181789599999));
#301313=CARTESIAN_POINT('Ctrl Pts',(-1.40049509300006,2.2,4.53181789599999));
#301314=CARTESIAN_POINT('Ctrl Pts',(-1.40120182900006,12.2,4.52926064799998));
#301315=CARTESIAN_POINT('Ctrl Pts',(-1.40120182900006,5.2,4.52926064799998));
#301316=CARTESIAN_POINT('Ctrl Pts',(-1.40120182900006,2.2,4.52926064799998));
#301317=CARTESIAN_POINT('Ctrl Pts',(-1.40190501200006,12.2,4.52670593299998));
#301318=CARTESIAN_POINT('Ctrl Pts',(-1.40190501200006,5.2,4.52670593299998));
#301319=CARTESIAN_POINT('Ctrl Pts',(-1.40190501200006,2.2,4.52670593299998));
#301320=CARTESIAN_POINT('Ctrl Pts',(-1.40260464700006,12.2,4.52415375599998));
#301321=CARTESIAN_POINT('Ctrl Pts',(-1.40260464700006,5.2,4.52415375599998));
#301322=CARTESIAN_POINT('Ctrl Pts',(-1.40260464700006,2.2,4.52415375599998));
#301323=CARTESIAN_POINT('Ctrl Pts',(-1.40330073300006,12.2,4.52160412099998));
#301324=CARTESIAN_POINT('Ctrl Pts',(-1.40330073300006,5.2,4.52160412099998));
#301325=CARTESIAN_POINT('Ctrl Pts',(-1.40330073300006,2.2,4.52160412099998));
#301326=CARTESIAN_POINT('Ctrl Pts',(-1.40399327800006,12.2,4.51905703499998));
#301327=CARTESIAN_POINT('Ctrl Pts',(-1.40399327800006,5.2,4.51905703499998));
#301328=CARTESIAN_POINT('Ctrl Pts',(-1.40399327800006,2.2,4.51905703499998));
#301329=CARTESIAN_POINT('Ctrl Pts',(-1.40468228400006,12.2,4.51651250799999));
#301330=CARTESIAN_POINT('Ctrl Pts',(-1.40468228400006,5.2,4.51651250799999));
#301331=CARTESIAN_POINT('Ctrl Pts',(-1.40468228400006,2.2,4.51651250799999));
#301332=CARTESIAN_POINT('Ctrl Pts',(-1.40536775800006,12.2,4.51397054699999));
#301333=CARTESIAN_POINT('Ctrl Pts',(-1.40536775800006,5.2,4.51397054699999));
#301334=CARTESIAN_POINT('Ctrl Pts',(-1.40536775800006,2.2,4.51397054699999));
#301335=CARTESIAN_POINT('Ctrl Pts',(-1.40604970300006,12.2,4.51143116199999));
#301336=CARTESIAN_POINT('Ctrl Pts',(-1.40604970300006,5.2,4.51143116199999));
#301337=CARTESIAN_POINT('Ctrl Pts',(-1.40604970300006,2.2,4.51143116199999));
#301338=CARTESIAN_POINT('Ctrl Pts',(-1.40672812800006,12.2,4.50889436399999));
#301339=CARTESIAN_POINT('Ctrl Pts',(-1.40672812800006,5.2,4.50889436399999));
#301340=CARTESIAN_POINT('Ctrl Pts',(-1.40672812800006,2.2,4.50889436399999));
#301341=CARTESIAN_POINT('Ctrl Pts',(-1.40740303600006,12.2,4.50636015799999));
#301342=CARTESIAN_POINT('Ctrl Pts',(-1.40740303600006,5.2,4.50636015799999));
#301343=CARTESIAN_POINT('Ctrl Pts',(-1.40740303600006,2.2,4.50636015799999));
#301344=CARTESIAN_POINT('Ctrl Pts',(-1.40807443200006,12.2,4.50382855499999));
#301345=CARTESIAN_POINT('Ctrl Pts',(-1.40807443200006,5.2,4.50382855499999));
#301346=CARTESIAN_POINT('Ctrl Pts',(-1.40807443200006,2.2,4.50382855499999));
#301347=CARTESIAN_POINT('Ctrl Pts',(-1.40874231900006,12.2,4.50129955899998));
#301348=CARTESIAN_POINT('Ctrl Pts',(-1.40874231900006,5.2,4.50129955899998));
#301349=CARTESIAN_POINT('Ctrl Pts',(-1.40874231900006,2.2,4.50129955899998));
#301350=CARTESIAN_POINT('Ctrl Pts',(-1.40940670100006,12.2,4.49877317899999));
#301351=CARTESIAN_POINT('Ctrl Pts',(-1.40940670100006,5.2,4.49877317899999));
#301352=CARTESIAN_POINT('Ctrl Pts',(-1.40940670100006,2.2,4.49877317899999));
#301353=CARTESIAN_POINT('Ctrl Pts',(-1.41006758200006,12.2,4.49624941999998));
#301354=CARTESIAN_POINT('Ctrl Pts',(-1.41006758200006,5.2,4.49624941999998));
#301355=CARTESIAN_POINT('Ctrl Pts',(-1.41006758200006,2.2,4.49624941999998));
#301356=CARTESIAN_POINT('Ctrl Pts',(-1.41072496700006,12.2,4.49372828999999));
#301357=CARTESIAN_POINT('Ctrl Pts',(-1.41072496700006,5.2,4.49372828999999));
#301358=CARTESIAN_POINT('Ctrl Pts',(-1.41072496700006,2.2,4.49372828999999));
#301359=CARTESIAN_POINT('Ctrl Pts',(-1.41137886000006,12.2,4.49120979499998));
#301360=CARTESIAN_POINT('Ctrl Pts',(-1.41137886000006,5.2,4.49120979499998));
#301361=CARTESIAN_POINT('Ctrl Pts',(-1.41137886000006,2.2,4.49120979499998));
#301362=CARTESIAN_POINT('Ctrl Pts',(-1.41202926500006,12.2,4.48869394399999));
#301363=CARTESIAN_POINT('Ctrl Pts',(-1.41202926500006,5.2,4.48869394399999));
#301364=CARTESIAN_POINT('Ctrl Pts',(-1.41202926500006,2.2,4.48869394399999));
#301365=CARTESIAN_POINT('Ctrl Pts',(-1.41267618800006,12.2,4.48618074299999));
#301366=CARTESIAN_POINT('Ctrl Pts',(-1.41267618800006,5.2,4.48618074299999));
#301367=CARTESIAN_POINT('Ctrl Pts',(-1.41267618800006,2.2,4.48618074299999));
#301368=CARTESIAN_POINT('Ctrl Pts',(-1.41331963200006,12.2,4.48367020199999));
#301369=CARTESIAN_POINT('Ctrl Pts',(-1.41331963200006,5.2,4.48367020199999));
#301370=CARTESIAN_POINT('Ctrl Pts',(-1.41331963200006,2.2,4.48367020199999));
#301371=CARTESIAN_POINT('Ctrl Pts',(-1.41395960300006,12.2,4.48116232799999));
#301372=CARTESIAN_POINT('Ctrl Pts',(-1.41395960300006,5.2,4.48116232799999));
#301373=CARTESIAN_POINT('Ctrl Pts',(-1.41395960300006,2.2,4.48116232799999));
#301374=CARTESIAN_POINT('Ctrl Pts',(-1.41459610500006,12.2,4.47865712799998));
#301375=CARTESIAN_POINT('Ctrl Pts',(-1.41459610500006,5.2,4.47865712799998));
#301376=CARTESIAN_POINT('Ctrl Pts',(-1.41459610500006,2.2,4.47865712799998));
#301377=CARTESIAN_POINT('Ctrl Pts',(-1.41522914200006,12.2,4.47615460999998));
#301378=CARTESIAN_POINT('Ctrl Pts',(-1.41522914200006,5.2,4.47615460999998));
#301379=CARTESIAN_POINT('Ctrl Pts',(-1.41522914200006,2.2,4.47615460999998));
#301380=CARTESIAN_POINT('Ctrl Pts',(-1.41585872000006,12.2,4.47365478099999));
#301381=CARTESIAN_POINT('Ctrl Pts',(-1.41585872000006,5.2,4.47365478099999));
#301382=CARTESIAN_POINT('Ctrl Pts',(-1.41585872000006,2.2,4.47365478099999));
#301383=CARTESIAN_POINT('Ctrl Pts',(-1.41648484200006,12.2,4.47115764999998));
#301384=CARTESIAN_POINT('Ctrl Pts',(-1.41648484200006,5.2,4.47115764999998));
#301385=CARTESIAN_POINT('Ctrl Pts',(-1.41648484200006,2.2,4.47115764999998));
#301386=CARTESIAN_POINT('Ctrl Pts',(-1.41710751400006,12.2,4.46866322199998));
#301387=CARTESIAN_POINT('Ctrl Pts',(-1.41710751400006,5.2,4.46866322199998));
#301388=CARTESIAN_POINT('Ctrl Pts',(-1.41710751400006,2.2,4.46866322199998));
#301389=CARTESIAN_POINT('Ctrl Pts',(-1.41772673900006,12.2,4.46617150599998));
#301390=CARTESIAN_POINT('Ctrl Pts',(-1.41772673900006,5.2,4.46617150599998));
#301391=CARTESIAN_POINT('Ctrl Pts',(-1.41772673900006,2.2,4.46617150599998));
#301392=CARTESIAN_POINT('Ctrl Pts',(-1.41834252300006,12.2,4.46368250799999));
#301393=CARTESIAN_POINT('Ctrl Pts',(-1.41834252300006,5.2,4.46368250799999));
#301394=CARTESIAN_POINT('Ctrl Pts',(-1.41834252300006,2.2,4.46368250799999));
#301395=CARTESIAN_POINT('Ctrl Pts',(-1.41895486900006,12.2,4.46119623799999));
#301396=CARTESIAN_POINT('Ctrl Pts',(-1.41895486900006,5.2,4.46119623799999));
#301397=CARTESIAN_POINT('Ctrl Pts',(-1.41895486900006,2.2,4.46119623799999));
#301398=CARTESIAN_POINT('Ctrl Pts',(-1.41956378300006,12.2,4.45871269999999));
#301399=CARTESIAN_POINT('Ctrl Pts',(-1.41956378300006,5.2,4.45871269999999));
#301400=CARTESIAN_POINT('Ctrl Pts',(-1.41956378300006,2.2,4.45871269999999));
#301401=CARTESIAN_POINT('Ctrl Pts',(-1.42016927000006,12.2,4.45623190599999));
#301402=CARTESIAN_POINT('Ctrl Pts',(-1.42016927000006,5.2,4.45623190599999));
#301403=CARTESIAN_POINT('Ctrl Pts',(-1.42016927000006,2.2,4.45623190599999));
#301404=CARTESIAN_POINT('Ctrl Pts',(-1.42077133300006,12.2,4.45375385999998));
#301405=CARTESIAN_POINT('Ctrl Pts',(-1.42077133300006,5.2,4.45375385999998));
#301406=CARTESIAN_POINT('Ctrl Pts',(-1.42077133300006,2.2,4.45375385999998));
#301407=CARTESIAN_POINT('Ctrl Pts',(-1.42136997900006,12.2,4.45127857099998));
#301408=CARTESIAN_POINT('Ctrl Pts',(-1.42136997900006,5.2,4.45127857099998));
#301409=CARTESIAN_POINT('Ctrl Pts',(-1.42136997900006,2.2,4.45127857099998));
#301410=CARTESIAN_POINT('Ctrl Pts',(-1.42196521100006,12.2,4.44880604699998));
#301411=CARTESIAN_POINT('Ctrl Pts',(-1.42196521100006,5.2,4.44880604699998));
#301412=CARTESIAN_POINT('Ctrl Pts',(-1.42196521100006,2.2,4.44880604699998));
#301413=CARTESIAN_POINT('Ctrl Pts',(-1.42255703400005,12.2,4.44633629399998));
#301414=CARTESIAN_POINT('Ctrl Pts',(-1.42255703400005,5.2,4.44633629399998));
#301415=CARTESIAN_POINT('Ctrl Pts',(-1.42255703400005,2.2,4.44633629399998));
#301416=CARTESIAN_POINT('Ctrl Pts',(-1.42314545400006,12.2,4.44386931899999));
#301417=CARTESIAN_POINT('Ctrl Pts',(-1.42314545400006,5.2,4.44386931899999));
#301418=CARTESIAN_POINT('Ctrl Pts',(-1.42314545400006,2.2,4.44386931899999));
#301419=CARTESIAN_POINT('Ctrl Pts',(-1.42373047400006,12.2,4.44140513299998));
#301420=CARTESIAN_POINT('Ctrl Pts',(-1.42373047400006,5.2,4.44140513299998));
#301421=CARTESIAN_POINT('Ctrl Pts',(-1.42373047400006,2.2,4.44140513299998));
#301422=CARTESIAN_POINT('Ctrl Pts',(-1.42431210000006,12.2,4.43894374199999));
#301423=CARTESIAN_POINT('Ctrl Pts',(-1.42431210000006,5.2,4.43894374199999));
#301424=CARTESIAN_POINT('Ctrl Pts',(-1.42431210000006,2.2,4.43894374199999));
#301425=CARTESIAN_POINT('Ctrl Pts',(-1.42489033600006,12.2,4.43648515099999));
#301426=CARTESIAN_POINT('Ctrl Pts',(-1.42489033600006,5.2,4.43648515099999));
#301427=CARTESIAN_POINT('Ctrl Pts',(-1.42489033600006,2.2,4.43648515099999));
#301428=CARTESIAN_POINT('Ctrl Pts',(-1.42546518700006,12.2,4.43402936999998));
#301429=CARTESIAN_POINT('Ctrl Pts',(-1.42546518700006,5.2,4.43402936999998));
#301430=CARTESIAN_POINT('Ctrl Pts',(-1.42546518700006,2.2,4.43402936999998));
#301431=CARTESIAN_POINT('Ctrl Pts',(-1.42603665900006,12.2,4.43157640599999));
#301432=CARTESIAN_POINT('Ctrl Pts',(-1.42603665900006,5.2,4.43157640599999));
#301433=CARTESIAN_POINT('Ctrl Pts',(-1.42603665900006,2.2,4.43157640599999));
#301434=CARTESIAN_POINT('Ctrl Pts',(-1.42660475600006,12.2,4.42912626699999));
#301435=CARTESIAN_POINT('Ctrl Pts',(-1.42660475600006,5.2,4.42912626699999));
#301436=CARTESIAN_POINT('Ctrl Pts',(-1.42660475600006,2.2,4.42912626699999));
#301437=CARTESIAN_POINT('Ctrl Pts',(-1.42716948100006,12.2,4.42667895999998));
#301438=CARTESIAN_POINT('Ctrl Pts',(-1.42716948100006,5.2,4.42667895999998));
#301439=CARTESIAN_POINT('Ctrl Pts',(-1.42716948100006,2.2,4.42667895999998));
#301440=CARTESIAN_POINT('Ctrl Pts',(-1.42773084300006,12.2,4.42423449199998));
#301441=CARTESIAN_POINT('Ctrl Pts',(-1.42773084300006,5.2,4.42423449199998));
#301442=CARTESIAN_POINT('Ctrl Pts',(-1.42773084300006,2.2,4.42423449199998));
#301443=CARTESIAN_POINT('Ctrl Pts',(-1.42828884300006,12.2,4.42179287099999));
#301444=CARTESIAN_POINT('Ctrl Pts',(-1.42828884300006,5.2,4.42179287099999));
#301445=CARTESIAN_POINT('Ctrl Pts',(-1.42828884300006,2.2,4.42179287099999));
#301446=CARTESIAN_POINT('Ctrl Pts',(-1.42884348800006,12.2,4.41935410599999));
#301447=CARTESIAN_POINT('Ctrl Pts',(-1.42884348800006,5.2,4.41935410599999));
#301448=CARTESIAN_POINT('Ctrl Pts',(-1.42884348800006,2.2,4.41935410599999));
#301449=CARTESIAN_POINT('Ctrl Pts',(-1.42939478200006,12.2,4.41691820299998));
#301450=CARTESIAN_POINT('Ctrl Pts',(-1.42939478200006,5.2,4.41691820299998));
#301451=CARTESIAN_POINT('Ctrl Pts',(-1.42939478200006,2.2,4.41691820299998));
#301452=CARTESIAN_POINT('Ctrl Pts',(-1.42994273000006,12.2,4.41448516999999));
#301453=CARTESIAN_POINT('Ctrl Pts',(-1.42994273000006,5.2,4.41448516999999));
#301454=CARTESIAN_POINT('Ctrl Pts',(-1.42994273000006,2.2,4.41448516999999));
#301455=CARTESIAN_POINT('Ctrl Pts',(-1.43048733900006,12.2,4.41205501499999));
#301456=CARTESIAN_POINT('Ctrl Pts',(-1.43048733900006,5.2,4.41205501499999));
#301457=CARTESIAN_POINT('Ctrl Pts',(-1.43048733900006,2.2,4.41205501499999));
#301458=CARTESIAN_POINT('Ctrl Pts',(-1.43102861100005,12.2,4.40962774299998));
#301459=CARTESIAN_POINT('Ctrl Pts',(-1.43102861100005,5.2,4.40962774299998));
#301460=CARTESIAN_POINT('Ctrl Pts',(-1.43102861100005,2.2,4.40962774299998));
#301461=CARTESIAN_POINT('Ctrl Pts',(-1.43156655300006,12.2,4.40720336599998));
#301462=CARTESIAN_POINT('Ctrl Pts',(-1.43156655300006,5.2,4.40720336599998));
#301463=CARTESIAN_POINT('Ctrl Pts',(-1.43156655300006,2.2,4.40720336599998));
#301464=CARTESIAN_POINT('Ctrl Pts',(-1.43210116800006,12.2,4.40478188799998));
#301465=CARTESIAN_POINT('Ctrl Pts',(-1.43210116800006,5.2,4.40478188799998));
#301466=CARTESIAN_POINT('Ctrl Pts',(-1.43210116800006,2.2,4.40478188799998));
#301467=CARTESIAN_POINT('Ctrl Pts',(-1.43263246300006,12.2,4.40236331799999));
#301468=CARTESIAN_POINT('Ctrl Pts',(-1.43263246300006,5.2,4.40236331799999));
#301469=CARTESIAN_POINT('Ctrl Pts',(-1.43263246300006,2.2,4.40236331799999));
#301470=CARTESIAN_POINT('Ctrl Pts',(-1.43316044400006,12.2,4.39994766299999));
#301471=CARTESIAN_POINT('Ctrl Pts',(-1.43316044400006,5.2,4.39994766299999));
#301472=CARTESIAN_POINT('Ctrl Pts',(-1.43316044400006,2.2,4.39994766299999));
#301473=CARTESIAN_POINT('Ctrl Pts',(-1.43368511200006,12.2,4.39753493199999));
#301474=CARTESIAN_POINT('Ctrl Pts',(-1.43368511200006,5.2,4.39753493199999));
#301475=CARTESIAN_POINT('Ctrl Pts',(-1.43368511200006,2.2,4.39753493199999));
#301476=CARTESIAN_POINT('Ctrl Pts',(-1.43420647600006,12.2,4.39512513099999));
#301477=CARTESIAN_POINT('Ctrl Pts',(-1.43420647600006,5.2,4.39512513099999));
#301478=CARTESIAN_POINT('Ctrl Pts',(-1.43420647600006,2.2,4.39512513099999));
#301479=CARTESIAN_POINT('Ctrl Pts',(-1.43472454000006,12.2,4.39271826799998));
#301480=CARTESIAN_POINT('Ctrl Pts',(-1.43472454000006,5.2,4.39271826799998));
#301481=CARTESIAN_POINT('Ctrl Pts',(-1.43472454000006,2.2,4.39271826799998));
#301482=CARTESIAN_POINT('Ctrl Pts',(-1.43523930800006,12.2,4.39031435099999));
#301483=CARTESIAN_POINT('Ctrl Pts',(-1.43523930800006,5.2,4.39031435099999));
#301484=CARTESIAN_POINT('Ctrl Pts',(-1.43523930800006,2.2,4.39031435099999));
#301485=CARTESIAN_POINT('Ctrl Pts',(-1.43575078600006,12.2,4.38791338599999));
#301486=CARTESIAN_POINT('Ctrl Pts',(-1.43575078600006,5.2,4.38791338599999));
#301487=CARTESIAN_POINT('Ctrl Pts',(-1.43575078600006,2.2,4.38791338599999));
#301488=CARTESIAN_POINT('Ctrl Pts',(-1.43625898000006,12.2,4.38551538399999));
#301489=CARTESIAN_POINT('Ctrl Pts',(-1.43625898000006,5.2,4.38551538399999));
#301490=CARTESIAN_POINT('Ctrl Pts',(-1.43625898000006,2.2,4.38551538399999));
#301491=CARTESIAN_POINT('Ctrl Pts',(-1.43676389300005,12.2,4.38312034899998));
#301492=CARTESIAN_POINT('Ctrl Pts',(-1.43676389300005,5.2,4.38312034899998));
#301493=CARTESIAN_POINT('Ctrl Pts',(-1.43676389300005,2.2,4.38312034899998));
#301494=CARTESIAN_POINT('Ctrl Pts',(-1.43726553200006,12.2,4.38072828999999));
#301495=CARTESIAN_POINT('Ctrl Pts',(-1.43726553200006,5.2,4.38072828999999));
#301496=CARTESIAN_POINT('Ctrl Pts',(-1.43726553200006,2.2,4.38072828999999));
#301497=CARTESIAN_POINT('Ctrl Pts',(-1.43776390200006,12.2,4.37833921599999));
#301498=CARTESIAN_POINT('Ctrl Pts',(-1.43776390200006,5.2,4.37833921599999));
#301499=CARTESIAN_POINT('Ctrl Pts',(-1.43776390200006,2.2,4.37833921599999));
#301500=CARTESIAN_POINT('Ctrl Pts',(-1.43825900700006,12.2,4.37595313299998));
#301501=CARTESIAN_POINT('Ctrl Pts',(-1.43825900700006,5.2,4.37595313299998));
#301502=CARTESIAN_POINT('Ctrl Pts',(-1.43825900700006,2.2,4.37595313299998));
#301503=CARTESIAN_POINT('Ctrl Pts',(-1.43875085400005,12.2,4.37357004899999));
#301504=CARTESIAN_POINT('Ctrl Pts',(-1.43875085400005,5.2,4.37357004899999));
#301505=CARTESIAN_POINT('Ctrl Pts',(-1.43875085400005,2.2,4.37357004899999));
#301506=CARTESIAN_POINT('Ctrl Pts',(-1.43923944700005,12.2,4.37118997099999));
#301507=CARTESIAN_POINT('Ctrl Pts',(-1.43923944700005,5.2,4.37118997099999));
#301508=CARTESIAN_POINT('Ctrl Pts',(-1.43923944700005,2.2,4.37118997099999));
#301509=CARTESIAN_POINT('Ctrl Pts',(-1.43972479200006,12.2,4.36881290699999));
#301510=CARTESIAN_POINT('Ctrl Pts',(-1.43972479200006,5.2,4.36881290699999));
#301511=CARTESIAN_POINT('Ctrl Pts',(-1.43972479200006,2.2,4.36881290699999));
#301512=CARTESIAN_POINT('Ctrl Pts',(-1.44020689300006,12.2,4.36643886499999));
#301513=CARTESIAN_POINT('Ctrl Pts',(-1.44020689300006,5.2,4.36643886499999));
#301514=CARTESIAN_POINT('Ctrl Pts',(-1.44020689300006,2.2,4.36643886499999));
#301515=CARTESIAN_POINT('Ctrl Pts',(-1.44068575700006,12.2,4.36406785199999));
#301516=CARTESIAN_POINT('Ctrl Pts',(-1.44068575700006,5.2,4.36406785199999));
#301517=CARTESIAN_POINT('Ctrl Pts',(-1.44068575700006,2.2,4.36406785199999));
#301518=CARTESIAN_POINT('Ctrl Pts',(-1.44116138800006,12.2,4.36169987799998));
#301519=CARTESIAN_POINT('Ctrl Pts',(-1.44116138800006,5.2,4.36169987799998));
#301520=CARTESIAN_POINT('Ctrl Pts',(-1.44116138800006,2.2,4.36169987799998));
#301521=CARTESIAN_POINT('Ctrl Pts',(-1.44163379200006,12.2,4.35933494699999));
#301522=CARTESIAN_POINT('Ctrl Pts',(-1.44163379200006,5.2,4.35933494699999));
#301523=CARTESIAN_POINT('Ctrl Pts',(-1.44163379200006,2.2,4.35933494699999));
#301524=CARTESIAN_POINT('Ctrl Pts',(-1.44210297400006,12.2,4.35697306899999));
#301525=CARTESIAN_POINT('Ctrl Pts',(-1.44210297400006,5.2,4.35697306899999));
#301526=CARTESIAN_POINT('Ctrl Pts',(-1.44210297400006,2.2,4.35697306899999));
#301527=CARTESIAN_POINT('Ctrl Pts',(-1.44256894100006,12.2,4.35461424899999));
#301528=CARTESIAN_POINT('Ctrl Pts',(-1.44256894100006,5.2,4.35461424899999));
#301529=CARTESIAN_POINT('Ctrl Pts',(-1.44256894100006,2.2,4.35461424899999));
#301530=CARTESIAN_POINT('Ctrl Pts',(-1.44303169500006,12.2,4.35225849899999));
#301531=CARTESIAN_POINT('Ctrl Pts',(-1.44303169500006,5.2,4.35225849899999));
#301532=CARTESIAN_POINT('Ctrl Pts',(-1.44303169500006,2.2,4.35225849899999));
#301533=CARTESIAN_POINT('Ctrl Pts',(-1.44349124500006,12.2,4.34990582299999));
#301534=CARTESIAN_POINT('Ctrl Pts',(-1.44349124500006,5.2,4.34990582299999));
#301535=CARTESIAN_POINT('Ctrl Pts',(-1.44349124500006,2.2,4.34990582299999));
#301536=CARTESIAN_POINT('Ctrl Pts',(-1.44394759500006,12.2,4.34755622899999));
#301537=CARTESIAN_POINT('Ctrl Pts',(-1.44394759500006,5.2,4.34755622899999));
#301538=CARTESIAN_POINT('Ctrl Pts',(-1.44394759500006,2.2,4.34755622899999));
#301539=CARTESIAN_POINT('Ctrl Pts',(-1.44440074900006,12.2,4.34520972699998));
#301540=CARTESIAN_POINT('Ctrl Pts',(-1.44440074900006,5.2,4.34520972699998));
#301541=CARTESIAN_POINT('Ctrl Pts',(-1.44440074900006,2.2,4.34520972699998));
#301542=CARTESIAN_POINT('Ctrl Pts',(-1.44485071400006,12.2,4.34286632199999));
#301543=CARTESIAN_POINT('Ctrl Pts',(-1.44485071400006,5.2,4.34286632199999));
#301544=CARTESIAN_POINT('Ctrl Pts',(-1.44485071400006,2.2,4.34286632199999));
#301545=CARTESIAN_POINT('Ctrl Pts',(-1.44529749600006,12.2,4.34052602399999));
#301546=CARTESIAN_POINT('Ctrl Pts',(-1.44529749600006,5.2,4.34052602399999));
#301547=CARTESIAN_POINT('Ctrl Pts',(-1.44529749600006,2.2,4.34052602399999));
#301548=CARTESIAN_POINT('Ctrl Pts',(-1.44574109900006,12.2,4.33818883899999));
#301549=CARTESIAN_POINT('Ctrl Pts',(-1.44574109900006,5.2,4.33818883899999));
#301550=CARTESIAN_POINT('Ctrl Pts',(-1.44574109900006,2.2,4.33818883899999));
#301551=CARTESIAN_POINT('Ctrl Pts',(-1.44618153000006,12.2,4.33585477399999));
#301552=CARTESIAN_POINT('Ctrl Pts',(-1.44618153000006,5.2,4.33585477399999));
#301553=CARTESIAN_POINT('Ctrl Pts',(-1.44618153000006,2.2,4.33585477399999));
#301554=CARTESIAN_POINT('Ctrl Pts',(-1.44661879400006,12.2,4.33352383899998));
#301555=CARTESIAN_POINT('Ctrl Pts',(-1.44661879400006,5.2,4.33352383899998));
#301556=CARTESIAN_POINT('Ctrl Pts',(-1.44661879400006,2.2,4.33352383899998));
#301557=CARTESIAN_POINT('Ctrl Pts',(-1.44705289500005,12.2,4.33119603999998));
#301558=CARTESIAN_POINT('Ctrl Pts',(-1.44705289500005,5.2,4.33119603999998));
#301559=CARTESIAN_POINT('Ctrl Pts',(-1.44705289500005,2.2,4.33119603999998));
#301560=CARTESIAN_POINT('Ctrl Pts',(-1.44748384100006,12.2,4.32887138499999));
#301561=CARTESIAN_POINT('Ctrl Pts',(-1.44748384100006,5.2,4.32887138499999));
#301562=CARTESIAN_POINT('Ctrl Pts',(-1.44748384100006,2.2,4.32887138499999));
#301563=CARTESIAN_POINT('Ctrl Pts',(-1.44791163700006,12.2,4.32654988099999));
#301564=CARTESIAN_POINT('Ctrl Pts',(-1.44791163700006,5.2,4.32654988099999));
#301565=CARTESIAN_POINT('Ctrl Pts',(-1.44791163700006,2.2,4.32654988099999));
#301566=CARTESIAN_POINT('Ctrl Pts',(-1.44833628700006,12.2,4.32423153699999));
#301567=CARTESIAN_POINT('Ctrl Pts',(-1.44833628700006,5.2,4.32423153699999));
#301568=CARTESIAN_POINT('Ctrl Pts',(-1.44833628700006,2.2,4.32423153699999));
#301569=CARTESIAN_POINT('Ctrl Pts',(-1.44875779800006,12.2,4.32191636099999));
#301570=CARTESIAN_POINT('Ctrl Pts',(-1.44875779800006,5.2,4.32191636099999));
#301571=CARTESIAN_POINT('Ctrl Pts',(-1.44875779800006,2.2,4.32191636099999));
#301572=CARTESIAN_POINT('Ctrl Pts',(-1.44917617600006,12.2,4.31960435799999));
#301573=CARTESIAN_POINT('Ctrl Pts',(-1.44917617600006,5.2,4.31960435799999));
#301574=CARTESIAN_POINT('Ctrl Pts',(-1.44917617600006,2.2,4.31960435799999));
#301575=CARTESIAN_POINT('Ctrl Pts',(-1.44959142400006,12.2,4.31729553799999));
#301576=CARTESIAN_POINT('Ctrl Pts',(-1.44959142400006,5.2,4.31729553799999));
#301577=CARTESIAN_POINT('Ctrl Pts',(-1.44959142400006,2.2,4.31729553799999));
#301578=CARTESIAN_POINT('Ctrl Pts',(-1.45000355200006,12.2,4.31498990799999));
#301579=CARTESIAN_POINT('Ctrl Pts',(-1.45000355200006,5.2,4.31498990799999));
#301580=CARTESIAN_POINT('Ctrl Pts',(-1.45000355200006,2.2,4.31498990799999));
#301581=CARTESIAN_POINT('Ctrl Pts',(-1.45041256300006,12.2,4.31268747599999));
#301582=CARTESIAN_POINT('Ctrl Pts',(-1.45041256300006,5.2,4.31268747599999));
#301583=CARTESIAN_POINT('Ctrl Pts',(-1.45041256300006,2.2,4.31268747599999));
#301584=CARTESIAN_POINT('Ctrl Pts',(-1.45081846300006,12.2,4.31038824899999));
#301585=CARTESIAN_POINT('Ctrl Pts',(-1.45081846300006,5.2,4.31038824899999));
#301586=CARTESIAN_POINT('Ctrl Pts',(-1.45081846300006,2.2,4.31038824899999));
#301587=CARTESIAN_POINT('Ctrl Pts',(-1.45122125700005,12.2,4.30809223499999));
#301588=CARTESIAN_POINT('Ctrl Pts',(-1.45122125700005,5.2,4.30809223499999));
#301589=CARTESIAN_POINT('Ctrl Pts',(-1.45122125700005,2.2,4.30809223499999));
#301590=CARTESIAN_POINT('Ctrl Pts',(-1.45162095300006,12.2,4.30579944199999));
#301591=CARTESIAN_POINT('Ctrl Pts',(-1.45162095300006,5.2,4.30579944199999));
#301592=CARTESIAN_POINT('Ctrl Pts',(-1.45162095300006,2.2,4.30579944199999));
#301593=CARTESIAN_POINT('Ctrl Pts',(-1.45201755400006,12.2,4.30350987799999));
#301594=CARTESIAN_POINT('Ctrl Pts',(-1.45201755400006,5.2,4.30350987799999));
#301595=CARTESIAN_POINT('Ctrl Pts',(-1.45201755400006,2.2,4.30350987799999));
#301596=CARTESIAN_POINT('Ctrl Pts',(-1.45241106800006,12.2,4.30122354899999));
#301597=CARTESIAN_POINT('Ctrl Pts',(-1.45241106800006,5.2,4.30122354899999));
#301598=CARTESIAN_POINT('Ctrl Pts',(-1.45241106800006,2.2,4.30122354899999));
#301599=CARTESIAN_POINT('Ctrl Pts',(-1.45280150000006,12.2,4.29894046499999));
#301600=CARTESIAN_POINT('Ctrl Pts',(-1.45280150000006,5.2,4.29894046499999));
#301601=CARTESIAN_POINT('Ctrl Pts',(-1.45280150000006,2.2,4.29894046499999));
#301602=CARTESIAN_POINT('Ctrl Pts',(-1.45318885600005,12.2,4.29666063199999));
#301603=CARTESIAN_POINT('Ctrl Pts',(-1.45318885600005,5.2,4.29666063199999));
#301604=CARTESIAN_POINT('Ctrl Pts',(-1.45318885600005,2.2,4.29666063199999));
#301605=CARTESIAN_POINT('Ctrl Pts',(-1.45357314000006,12.2,4.29438405699998));
#301606=CARTESIAN_POINT('Ctrl Pts',(-1.45357314000006,5.2,4.29438405699998));
#301607=CARTESIAN_POINT('Ctrl Pts',(-1.45357314000006,2.2,4.29438405699998));
#301608=CARTESIAN_POINT('Ctrl Pts',(-1.45395436100006,12.2,4.29211075099998));
#301609=CARTESIAN_POINT('Ctrl Pts',(-1.45395436100006,5.2,4.29211075099998));
#301610=CARTESIAN_POINT('Ctrl Pts',(-1.45395436100006,2.2,4.29211075099998));
#301611=CARTESIAN_POINT('Ctrl Pts',(-1.45433252400006,12.2,4.28984071899999));
#301612=CARTESIAN_POINT('Ctrl Pts',(-1.45433252400006,5.2,4.28984071899999));
#301613=CARTESIAN_POINT('Ctrl Pts',(-1.45433252400006,2.2,4.28984071899999));
#301614=CARTESIAN_POINT('Ctrl Pts',(-1.45470763300006,12.2,4.28757396799998));
#301615=CARTESIAN_POINT('Ctrl Pts',(-1.45470763300006,5.2,4.28757396799998));
#301616=CARTESIAN_POINT('Ctrl Pts',(-1.45470763300006,2.2,4.28757396799998));
#301617=CARTESIAN_POINT('Ctrl Pts',(-1.45507969700006,12.2,4.28531050899998));
#301618=CARTESIAN_POINT('Ctrl Pts',(-1.45507969700006,5.2,4.28531050899998));
#301619=CARTESIAN_POINT('Ctrl Pts',(-1.45507969700006,2.2,4.28531050899998));
#301620=CARTESIAN_POINT('Ctrl Pts',(-1.45544871800006,12.2,4.28305034699999));
#301621=CARTESIAN_POINT('Ctrl Pts',(-1.45544871800006,5.2,4.28305034699999));
#301622=CARTESIAN_POINT('Ctrl Pts',(-1.45544871800006,2.2,4.28305034699999));
#301623=CARTESIAN_POINT('Ctrl Pts',(-1.45581470400006,12.2,4.28079348999999));
#301624=CARTESIAN_POINT('Ctrl Pts',(-1.45581470400006,5.2,4.28079348999999));
#301625=CARTESIAN_POINT('Ctrl Pts',(-1.45581470400006,2.2,4.28079348999999));
#301626=CARTESIAN_POINT('Ctrl Pts',(-1.45617766300006,12.2,4.27853994599998));
#301627=CARTESIAN_POINT('Ctrl Pts',(-1.45617766300006,5.2,4.27853994599998));
#301628=CARTESIAN_POINT('Ctrl Pts',(-1.45617766300006,2.2,4.27853994599998));
#301629=CARTESIAN_POINT('Ctrl Pts',(-1.45653759900006,12.2,4.27628972399998));
#301630=CARTESIAN_POINT('Ctrl Pts',(-1.45653759900006,5.2,4.27628972399998));
#301631=CARTESIAN_POINT('Ctrl Pts',(-1.45653759900006,2.2,4.27628972399998));
#301632=CARTESIAN_POINT('Ctrl Pts',(-1.45689451600005,12.2,4.27404282999999));
#301633=CARTESIAN_POINT('Ctrl Pts',(-1.45689451600005,5.2,4.27404282999999));
#301634=CARTESIAN_POINT('Ctrl Pts',(-1.45689451600005,2.2,4.27404282999999));
#301635=CARTESIAN_POINT('Ctrl Pts',(-1.45724842400006,12.2,4.27179927199998));
#301636=CARTESIAN_POINT('Ctrl Pts',(-1.45724842400006,5.2,4.27179927199998));
#301637=CARTESIAN_POINT('Ctrl Pts',(-1.45724842400006,2.2,4.27179927199998));
#301638=CARTESIAN_POINT('Ctrl Pts',(-1.45759932700006,12.2,4.26955905899998));
#301639=CARTESIAN_POINT('Ctrl Pts',(-1.45759932700006,5.2,4.26955905899998));
#301640=CARTESIAN_POINT('Ctrl Pts',(-1.45759932700006,2.2,4.26955905899998));
#301641=CARTESIAN_POINT('Ctrl Pts',(-1.45794723000006,12.2,4.26732219699999));
#301642=CARTESIAN_POINT('Ctrl Pts',(-1.45794723000006,5.2,4.26732219699999));
#301643=CARTESIAN_POINT('Ctrl Pts',(-1.45794723000006,2.2,4.26732219699999));
#301644=CARTESIAN_POINT('Ctrl Pts',(-1.45829214100006,12.2,4.26508869499998));
#301645=CARTESIAN_POINT('Ctrl Pts',(-1.45829214100006,5.2,4.26508869499998));
#301646=CARTESIAN_POINT('Ctrl Pts',(-1.45829214100006,2.2,4.26508869499998));
#301647=CARTESIAN_POINT('Ctrl Pts',(-1.45863406500006,12.2,4.26285855999998));
#301648=CARTESIAN_POINT('Ctrl Pts',(-1.45863406500006,5.2,4.26285855999998));
#301649=CARTESIAN_POINT('Ctrl Pts',(-1.45863406500006,2.2,4.26285855999998));
#301650=CARTESIAN_POINT('Ctrl Pts',(-1.45897301000006,12.2,4.26063179999999));
#301651=CARTESIAN_POINT('Ctrl Pts',(-1.45897301000006,5.2,4.26063179999999));
#301652=CARTESIAN_POINT('Ctrl Pts',(-1.45897301000006,2.2,4.26063179999999));
#301653=CARTESIAN_POINT('Ctrl Pts',(-1.45930898000006,12.2,4.25840842299999));
#301654=CARTESIAN_POINT('Ctrl Pts',(-1.45930898000006,5.2,4.25840842299999));
#301655=CARTESIAN_POINT('Ctrl Pts',(-1.45930898000006,2.2,4.25840842299999));
#301656=CARTESIAN_POINT('Ctrl Pts',(-1.45964198100006,12.2,4.25618843599998));
#301657=CARTESIAN_POINT('Ctrl Pts',(-1.45964198100006,5.2,4.25618843599998));
#301658=CARTESIAN_POINT('Ctrl Pts',(-1.45964198100006,2.2,4.25618843599998));
#301659=CARTESIAN_POINT('Ctrl Pts',(-1.45997202100006,12.2,4.25397184699998));
#301660=CARTESIAN_POINT('Ctrl Pts',(-1.45997202100006,5.2,4.25397184699998));
#301661=CARTESIAN_POINT('Ctrl Pts',(-1.45997202100006,2.2,4.25397184699998));
#301662=CARTESIAN_POINT('Ctrl Pts',(-1.46029910500006,12.2,4.25175866399999));
#301663=CARTESIAN_POINT('Ctrl Pts',(-1.46029910500006,5.2,4.25175866399999));
#301664=CARTESIAN_POINT('Ctrl Pts',(-1.46029910500006,2.2,4.25175866399999));
#301665=CARTESIAN_POINT('Ctrl Pts',(-1.46062324000006,12.2,4.24954889499999));
#301666=CARTESIAN_POINT('Ctrl Pts',(-1.46062324000006,5.2,4.24954889499999));
#301667=CARTESIAN_POINT('Ctrl Pts',(-1.46062324000006,2.2,4.24954889499999));
#301668=CARTESIAN_POINT('Ctrl Pts',(-1.46094443100006,12.2,4.24734254799999));
#301669=CARTESIAN_POINT('Ctrl Pts',(-1.46094443100006,5.2,4.24734254799999));
#301670=CARTESIAN_POINT('Ctrl Pts',(-1.46094443100006,2.2,4.24734254799999));
#301671=CARTESIAN_POINT('Ctrl Pts',(-1.46126268600006,12.2,4.24513962999999));
#301672=CARTESIAN_POINT('Ctrl Pts',(-1.46126268600006,5.2,4.24513962999999));
#301673=CARTESIAN_POINT('Ctrl Pts',(-1.46126268600006,2.2,4.24513962999999));
#301674=CARTESIAN_POINT('Ctrl Pts',(-1.46157800900006,12.2,4.24294014899999));
#301675=CARTESIAN_POINT('Ctrl Pts',(-1.46157800900006,5.2,4.24294014899999));
#301676=CARTESIAN_POINT('Ctrl Pts',(-1.46157800900006,2.2,4.24294014899999));
#301677=CARTESIAN_POINT('Ctrl Pts',(-1.46189040800005,12.2,4.24074411199998));
#301678=CARTESIAN_POINT('Ctrl Pts',(-1.46189040800005,5.2,4.24074411199998));
#301679=CARTESIAN_POINT('Ctrl Pts',(-1.46189040800005,2.2,4.24074411199998));
#301680=CARTESIAN_POINT('Ctrl Pts',(-1.46219988800006,12.2,4.23855152799998));
#301681=CARTESIAN_POINT('Ctrl Pts',(-1.46219988800006,5.2,4.23855152799998));
#301682=CARTESIAN_POINT('Ctrl Pts',(-1.46219988800006,2.2,4.23855152799998));
#301683=CARTESIAN_POINT('Ctrl Pts',(-1.46250645800006,12.2,4.23636240399999));
#301684=CARTESIAN_POINT('Ctrl Pts',(-1.46250645800006,5.2,4.23636240399999));
#301685=CARTESIAN_POINT('Ctrl Pts',(-1.46250645800006,2.2,4.23636240399999));
#301686=CARTESIAN_POINT('Ctrl Pts',(-1.46281012200006,12.2,4.23417674899999));
#301687=CARTESIAN_POINT('Ctrl Pts',(-1.46281012200006,5.2,4.23417674899999));
#301688=CARTESIAN_POINT('Ctrl Pts',(-1.46281012200006,2.2,4.23417674899999));
#301689=CARTESIAN_POINT('Ctrl Pts',(-1.46311088700006,12.2,4.23199456799999));
#301690=CARTESIAN_POINT('Ctrl Pts',(-1.46311088700006,5.2,4.23199456799999));
#301691=CARTESIAN_POINT('Ctrl Pts',(-1.46311088700006,2.2,4.23199456799999));
#301692=CARTESIAN_POINT('Ctrl Pts',(-1.46340875900006,12.2,4.22981587199998));
#301693=CARTESIAN_POINT('Ctrl Pts',(-1.46340875900006,5.2,4.22981587199998));
#301694=CARTESIAN_POINT('Ctrl Pts',(-1.46340875900006,2.2,4.22981587199998));
#301695=CARTESIAN_POINT('Ctrl Pts',(-1.46370374500005,12.2,4.22764066699998));
#301696=CARTESIAN_POINT('Ctrl Pts',(-1.46370374500005,5.2,4.22764066699998));
#301697=CARTESIAN_POINT('Ctrl Pts',(-1.46370374500005,2.2,4.22764066699998));
#301698=CARTESIAN_POINT('Ctrl Pts',(-1.46399585200006,12.2,4.22546895999999));
#301699=CARTESIAN_POINT('Ctrl Pts',(-1.46399585200006,5.2,4.22546895999999));
#301700=CARTESIAN_POINT('Ctrl Pts',(-1.46399585200006,2.2,4.22546895999999));
#301701=CARTESIAN_POINT('Ctrl Pts',(-1.46428508500006,12.2,4.22330076099998));
#301702=CARTESIAN_POINT('Ctrl Pts',(-1.46428508500006,5.2,4.22330076099998));
#301703=CARTESIAN_POINT('Ctrl Pts',(-1.46428508500006,2.2,4.22330076099998));
#301704=CARTESIAN_POINT('Ctrl Pts',(-1.46457145100006,12.2,4.22113607699998));
#301705=CARTESIAN_POINT('Ctrl Pts',(-1.46457145100006,5.2,4.22113607699998));
#301706=CARTESIAN_POINT('Ctrl Pts',(-1.46457145100006,2.2,4.22113607699998));
#301707=CARTESIAN_POINT('Ctrl Pts',(-1.46485495700006,12.2,4.21897491499998));
#301708=CARTESIAN_POINT('Ctrl Pts',(-1.46485495700006,5.2,4.21897491499998));
#301709=CARTESIAN_POINT('Ctrl Pts',(-1.46485495700006,2.2,4.21897491499998));
#301710=CARTESIAN_POINT('Ctrl Pts',(-1.46513560900006,12.2,4.21681728399999));
#301711=CARTESIAN_POINT('Ctrl Pts',(-1.46513560900006,5.2,4.21681728399999));
#301712=CARTESIAN_POINT('Ctrl Pts',(-1.46513560900006,2.2,4.21681728399999));
#301713=CARTESIAN_POINT('Ctrl Pts',(-1.46541341300006,12.2,4.21466318899999));
#301714=CARTESIAN_POINT('Ctrl Pts',(-1.46541341300006,5.2,4.21466318899999));
#301715=CARTESIAN_POINT('Ctrl Pts',(-1.46541341300006,2.2,4.21466318899999));
#301716=CARTESIAN_POINT('Ctrl Pts',(-1.46568837800006,12.2,4.21251264099999));
#301717=CARTESIAN_POINT('Ctrl Pts',(-1.46568837800006,5.2,4.21251264099999));
#301718=CARTESIAN_POINT('Ctrl Pts',(-1.46568837800006,2.2,4.21251264099999));
#301719=CARTESIAN_POINT('Ctrl Pts',(-1.46596050800005,12.2,4.21036564699998));
#301720=CARTESIAN_POINT('Ctrl Pts',(-1.46596050800005,5.2,4.21036564699998));
#301721=CARTESIAN_POINT('Ctrl Pts',(-1.46596050800005,2.2,4.21036564699998));
#301722=CARTESIAN_POINT('Ctrl Pts',(-1.46622981100006,12.2,4.20822221299999));
#301723=CARTESIAN_POINT('Ctrl Pts',(-1.46622981100006,5.2,4.20822221299999));
#301724=CARTESIAN_POINT('Ctrl Pts',(-1.46622981100006,2.2,4.20822221299999));
#301725=CARTESIAN_POINT('Ctrl Pts',(-1.46649629200006,12.2,4.20608234999998));
#301726=CARTESIAN_POINT('Ctrl Pts',(-1.46649629200006,5.2,4.20608234999998));
#301727=CARTESIAN_POINT('Ctrl Pts',(-1.46649629200006,2.2,4.20608234999998));
#301728=CARTESIAN_POINT('Ctrl Pts',(-1.46675996000006,12.2,4.20394606199999));
#301729=CARTESIAN_POINT('Ctrl Pts',(-1.46675996000006,5.2,4.20394606199999));
#301730=CARTESIAN_POINT('Ctrl Pts',(-1.46675996000006,2.2,4.20394606199999));
#301731=CARTESIAN_POINT('Ctrl Pts',(-1.46702082000005,12.2,4.20181335999998));
#301732=CARTESIAN_POINT('Ctrl Pts',(-1.46702082000005,5.2,4.20181335999998));
#301733=CARTESIAN_POINT('Ctrl Pts',(-1.46702082000005,2.2,4.20181335999998));
#301734=CARTESIAN_POINT('Ctrl Pts',(-1.46727887800005,12.2,4.19968425099999));
#301735=CARTESIAN_POINT('Ctrl Pts',(-1.46727887800005,5.2,4.19968425099999));
#301736=CARTESIAN_POINT('Ctrl Pts',(-1.46727887800005,2.2,4.19968425099999));
#301737=CARTESIAN_POINT('Ctrl Pts',(-1.46753414300006,12.2,4.19755874099998));
#301738=CARTESIAN_POINT('Ctrl Pts',(-1.46753414300006,5.2,4.19755874099998));
#301739=CARTESIAN_POINT('Ctrl Pts',(-1.46753414300006,2.2,4.19755874099998));
#301740=CARTESIAN_POINT('Ctrl Pts',(-1.46778662100005,12.2,4.19543684099998));
#301741=CARTESIAN_POINT('Ctrl Pts',(-1.46778662100005,5.2,4.19543684099998));
#301742=CARTESIAN_POINT('Ctrl Pts',(-1.46778662100005,2.2,4.19543684099998));
#301743=CARTESIAN_POINT('Ctrl Pts',(-1.46803631800006,12.2,4.19331855599999));
#301744=CARTESIAN_POINT('Ctrl Pts',(-1.46803631800006,5.2,4.19331855599999));
#301745=CARTESIAN_POINT('Ctrl Pts',(-1.46803631800006,2.2,4.19331855599999));
#301746=CARTESIAN_POINT('Ctrl Pts',(-1.46828324000006,12.2,4.19120389499999));
#301747=CARTESIAN_POINT('Ctrl Pts',(-1.46828324000006,5.2,4.19120389499999));
#301748=CARTESIAN_POINT('Ctrl Pts',(-1.46828324000006,2.2,4.19120389499999));
#301749=CARTESIAN_POINT('Ctrl Pts',(-1.46852739600006,12.2,4.18909286499999));
#301750=CARTESIAN_POINT('Ctrl Pts',(-1.46852739600006,5.2,4.18909286499999));
#301751=CARTESIAN_POINT('Ctrl Pts',(-1.46852739600006,2.2,4.18909286499999));
#301752=CARTESIAN_POINT('Ctrl Pts',(-1.46876879100006,12.2,4.18698547499999));
#301753=CARTESIAN_POINT('Ctrl Pts',(-1.46876879100006,5.2,4.18698547499999));
#301754=CARTESIAN_POINT('Ctrl Pts',(-1.46876879100006,2.2,4.18698547499999));
#301755=CARTESIAN_POINT('Ctrl Pts',(-1.46900743300006,12.2,4.18488173199999));
#301756=CARTESIAN_POINT('Ctrl Pts',(-1.46900743300006,5.2,4.18488173199999));
#301757=CARTESIAN_POINT('Ctrl Pts',(-1.46900743300006,2.2,4.18488173199999));
#301758=CARTESIAN_POINT('Ctrl Pts',(-1.46924332800006,12.2,4.18278164499998));
#301759=CARTESIAN_POINT('Ctrl Pts',(-1.46924332800006,5.2,4.18278164499998));
#301760=CARTESIAN_POINT('Ctrl Pts',(-1.46924332800006,2.2,4.18278164499998));
#301761=CARTESIAN_POINT('Ctrl Pts',(-1.46947648300006,12.2,4.18068521899999));
#301762=CARTESIAN_POINT('Ctrl Pts',(-1.46947648300006,5.2,4.18068521899999));
#301763=CARTESIAN_POINT('Ctrl Pts',(-1.46947648300006,2.2,4.18068521899999));
#301764=CARTESIAN_POINT('Ctrl Pts',(-1.46970690600006,12.2,4.17859246499999));
#301765=CARTESIAN_POINT('Ctrl Pts',(-1.46970690600006,5.2,4.17859246499999));
#301766=CARTESIAN_POINT('Ctrl Pts',(-1.46970690600006,2.2,4.17859246499999));
#301767=CARTESIAN_POINT('Ctrl Pts',(-1.46993460300005,12.2,4.17650338999999));
#301768=CARTESIAN_POINT('Ctrl Pts',(-1.46993460300005,5.2,4.17650338999999));
#301769=CARTESIAN_POINT('Ctrl Pts',(-1.46993460300005,2.2,4.17650338999999));
#301770=CARTESIAN_POINT('Ctrl Pts',(-1.47015957900006,12.2,4.17441800099999));
#301771=CARTESIAN_POINT('Ctrl Pts',(-1.47015957900006,5.2,4.17441800099999));
#301772=CARTESIAN_POINT('Ctrl Pts',(-1.47015957900006,2.2,4.17441800099999));
#301773=CARTESIAN_POINT('Ctrl Pts',(-1.47038184500005,12.2,4.17233630599998));
#301774=CARTESIAN_POINT('Ctrl Pts',(-1.47038184500005,5.2,4.17233630599998));
#301775=CARTESIAN_POINT('Ctrl Pts',(-1.47038184500005,2.2,4.17233630599998));
#301776=CARTESIAN_POINT('Ctrl Pts',(-1.47060140500006,12.2,4.17025831399998));
#301777=CARTESIAN_POINT('Ctrl Pts',(-1.47060140500006,5.2,4.17025831399998));
#301778=CARTESIAN_POINT('Ctrl Pts',(-1.47060140500006,2.2,4.17025831399998));
#301779=CARTESIAN_POINT('Ctrl Pts',(-1.47081826800005,12.2,4.16818403099998));
#301780=CARTESIAN_POINT('Ctrl Pts',(-1.47081826800005,5.2,4.16818403099998));
#301781=CARTESIAN_POINT('Ctrl Pts',(-1.47081826800005,2.2,4.16818403099998));
#301782=CARTESIAN_POINT('Ctrl Pts',(-1.47103243800006,12.2,4.16611346599999));
#301783=CARTESIAN_POINT('Ctrl Pts',(-1.47103243800006,5.2,4.16611346599999));
#301784=CARTESIAN_POINT('Ctrl Pts',(-1.47103243800006,2.2,4.16611346599999));
#301785=CARTESIAN_POINT('Ctrl Pts',(-1.47124392500006,12.2,4.16404662599999));
#301786=CARTESIAN_POINT('Ctrl Pts',(-1.47124392500006,5.2,4.16404662599999));
#301787=CARTESIAN_POINT('Ctrl Pts',(-1.47124392500006,2.2,4.16404662599999));
#301788=CARTESIAN_POINT('Ctrl Pts',(-1.47145273500006,12.2,4.16198351999999));
#301789=CARTESIAN_POINT('Ctrl Pts',(-1.47145273500006,5.2,4.16198351999999));
#301790=CARTESIAN_POINT('Ctrl Pts',(-1.47145273500006,2.2,4.16198351999999));
#301791=CARTESIAN_POINT('Ctrl Pts',(-1.47165887500006,12.2,4.15992415599998));
#301792=CARTESIAN_POINT('Ctrl Pts',(-1.47165887500006,5.2,4.15992415599998));
#301793=CARTESIAN_POINT('Ctrl Pts',(-1.47165887500006,2.2,4.15992415599998));
#301794=CARTESIAN_POINT('Ctrl Pts',(-1.47186235200006,12.2,4.15786854099998));
#301795=CARTESIAN_POINT('Ctrl Pts',(-1.47186235200006,5.2,4.15786854099998));
#301796=CARTESIAN_POINT('Ctrl Pts',(-1.47186235200006,2.2,4.15786854099998));
#301797=CARTESIAN_POINT('Ctrl Pts',(-1.47206317400006,12.2,4.15581668199999));
#301798=CARTESIAN_POINT('Ctrl Pts',(-1.47206317400006,5.2,4.15581668199999));
#301799=CARTESIAN_POINT('Ctrl Pts',(-1.47206317400006,2.2,4.15581668199999));
#301800=CARTESIAN_POINT('Ctrl Pts',(-1.47226134800006,12.2,4.15376858899998));
#301801=CARTESIAN_POINT('Ctrl Pts',(-1.47226134800006,5.2,4.15376858899998));
#301802=CARTESIAN_POINT('Ctrl Pts',(-1.47226134800006,2.2,4.15376858899998));
#301803=CARTESIAN_POINT('Ctrl Pts',(-1.47245687900006,12.2,4.15172426699999));
#301804=CARTESIAN_POINT('Ctrl Pts',(-1.47245687900006,5.2,4.15172426699999));
#301805=CARTESIAN_POINT('Ctrl Pts',(-1.47245687900006,2.2,4.15172426699999));
#301806=CARTESIAN_POINT('Ctrl Pts',(-1.47264977700006,12.2,4.14968372799999));
#301807=CARTESIAN_POINT('Ctrl Pts',(-1.47264977700006,5.2,4.14968372799999));
#301808=CARTESIAN_POINT('Ctrl Pts',(-1.47264977700006,2.2,4.14968372799999));
#301809=CARTESIAN_POINT('Ctrl Pts',(-1.47284004700006,12.2,4.14764697499999));
#301810=CARTESIAN_POINT('Ctrl Pts',(-1.47284004700006,5.2,4.14764697499999));
#301811=CARTESIAN_POINT('Ctrl Pts',(-1.47284004700006,2.2,4.14764697499999));
#301812=CARTESIAN_POINT('Ctrl Pts',(-1.47302769900006,12.2,4.14561402099999));
#301813=CARTESIAN_POINT('Ctrl Pts',(-1.47302769900006,5.2,4.14561402099999));
#301814=CARTESIAN_POINT('Ctrl Pts',(-1.47302769900006,2.2,4.14561402099999));
#301815=CARTESIAN_POINT('Ctrl Pts',(-1.47321273700006,12.2,4.14358486899999));
#301816=CARTESIAN_POINT('Ctrl Pts',(-1.47321273700006,5.2,4.14358486899999));
#301817=CARTESIAN_POINT('Ctrl Pts',(-1.47321273700006,2.2,4.14358486899999));
#301818=CARTESIAN_POINT('Ctrl Pts',(-1.47339517100006,12.2,4.14155952999998));
#301819=CARTESIAN_POINT('Ctrl Pts',(-1.47339517100006,5.2,4.14155952999998));
#301820=CARTESIAN_POINT('Ctrl Pts',(-1.47339517100006,2.2,4.14155952999998));
#301821=CARTESIAN_POINT('Ctrl Pts',(-1.47357500700006,12.2,4.13953801099999));
#301822=CARTESIAN_POINT('Ctrl Pts',(-1.47357500700006,5.2,4.13953801099999));
#301823=CARTESIAN_POINT('Ctrl Pts',(-1.47357500700006,2.2,4.13953801099999));
#301824=CARTESIAN_POINT('Ctrl Pts',(-1.47375225100006,12.2,4.13752031899998));
#301825=CARTESIAN_POINT('Ctrl Pts',(-1.47375225100006,5.2,4.13752031899998));
#301826=CARTESIAN_POINT('Ctrl Pts',(-1.47375225100006,2.2,4.13752031899998));
#301827=CARTESIAN_POINT('Ctrl Pts',(-1.47392691400006,12.2,4.13550646399998));
#301828=CARTESIAN_POINT('Ctrl Pts',(-1.47392691400006,5.2,4.13550646399998));
#301829=CARTESIAN_POINT('Ctrl Pts',(-1.47392691400006,2.2,4.13550646399998));
#301830=CARTESIAN_POINT('Ctrl Pts',(-1.47409900000006,12.2,4.13349645099998));
#301831=CARTESIAN_POINT('Ctrl Pts',(-1.47409900000006,5.2,4.13349645099998));
#301832=CARTESIAN_POINT('Ctrl Pts',(-1.47409900000006,2.2,4.13349645099998));
#301833=CARTESIAN_POINT('Ctrl Pts',(-1.47426851800006,12.2,4.13149029099999));
#301834=CARTESIAN_POINT('Ctrl Pts',(-1.47426851800006,5.2,4.13149029099999));
#301835=CARTESIAN_POINT('Ctrl Pts',(-1.47426851800006,2.2,4.13149029099999));
#301836=CARTESIAN_POINT('Ctrl Pts',(-1.47443547500006,12.2,4.12948798899999));
#301837=CARTESIAN_POINT('Ctrl Pts',(-1.47443547500006,5.2,4.12948798899999));
#301838=CARTESIAN_POINT('Ctrl Pts',(-1.47443547500006,2.2,4.12948798899999));
#301839=CARTESIAN_POINT('Ctrl Pts',(-1.47459987800006,12.2,4.12748955499998));
#301840=CARTESIAN_POINT('Ctrl Pts',(-1.47459987800006,5.2,4.12748955499998));
#301841=CARTESIAN_POINT('Ctrl Pts',(-1.47459987800006,2.2,4.12748955499998));
#301842=CARTESIAN_POINT('Ctrl Pts',(-1.47476173500006,12.2,4.12549499699999));
#301843=CARTESIAN_POINT('Ctrl Pts',(-1.47476173500006,5.2,4.12549499699999));
#301844=CARTESIAN_POINT('Ctrl Pts',(-1.47476173500006,2.2,4.12549499699999));
#301845=CARTESIAN_POINT('Ctrl Pts',(-1.47492105400006,12.2,4.12350432099998));
#301846=CARTESIAN_POINT('Ctrl Pts',(-1.47492105400006,5.2,4.12350432099998));
#301847=CARTESIAN_POINT('Ctrl Pts',(-1.47492105400006,2.2,4.12350432099998));
#301848=CARTESIAN_POINT('Ctrl Pts',(-1.47507784200006,12.2,4.12151753499998));
#301849=CARTESIAN_POINT('Ctrl Pts',(-1.47507784200006,5.2,4.12151753499998));
#301850=CARTESIAN_POINT('Ctrl Pts',(-1.47507784200006,2.2,4.12151753499998));
#301851=CARTESIAN_POINT('Ctrl Pts',(-1.47523210600006,12.2,4.11953464899998));
#301852=CARTESIAN_POINT('Ctrl Pts',(-1.47523210600006,5.2,4.11953464899998));
#301853=CARTESIAN_POINT('Ctrl Pts',(-1.47523210600006,2.2,4.11953464899998));
#301854=CARTESIAN_POINT('Ctrl Pts',(-1.47538385400006,12.2,4.11755566899998));
#301855=CARTESIAN_POINT('Ctrl Pts',(-1.47538385400006,5.2,4.11755566899998));
#301856=CARTESIAN_POINT('Ctrl Pts',(-1.47538385400006,2.2,4.11755566899998));
#301857=CARTESIAN_POINT('Ctrl Pts',(-1.47553309400006,12.2,4.11558060499999));
#301858=CARTESIAN_POINT('Ctrl Pts',(-1.47553309400006,5.2,4.11558060499999));
#301859=CARTESIAN_POINT('Ctrl Pts',(-1.47553309400006,2.2,4.11558060499999));
#301860=CARTESIAN_POINT('Ctrl Pts',(-1.47567983300006,12.2,4.11360946199999));
#301861=CARTESIAN_POINT('Ctrl Pts',(-1.47567983300006,5.2,4.11360946199999));
#301862=CARTESIAN_POINT('Ctrl Pts',(-1.47567983300006,2.2,4.11360946199999));
#301863=CARTESIAN_POINT('Ctrl Pts',(-1.47582407900006,12.2,4.11164225099999));
#301864=CARTESIAN_POINT('Ctrl Pts',(-1.47582407900006,5.2,4.11164225099999));
#301865=CARTESIAN_POINT('Ctrl Pts',(-1.47582407900006,2.2,4.11164225099999));
#301866=CARTESIAN_POINT('Ctrl Pts',(-1.47596583900006,12.2,4.10967897699998));
#301867=CARTESIAN_POINT('Ctrl Pts',(-1.47596583900006,5.2,4.10967897699998));
#301868=CARTESIAN_POINT('Ctrl Pts',(-1.47596583900006,2.2,4.10967897699998));
#301869=CARTESIAN_POINT('Ctrl Pts',(-1.47610512100006,12.2,4.10771964899999));
#301870=CARTESIAN_POINT('Ctrl Pts',(-1.47610512100006,5.2,4.10771964899999));
#301871=CARTESIAN_POINT('Ctrl Pts',(-1.47610512100006,2.2,4.10771964899999));
#301872=CARTESIAN_POINT('Ctrl Pts',(-1.47624193300006,12.2,4.10576427599998));
#301873=CARTESIAN_POINT('Ctrl Pts',(-1.47624193300006,5.2,4.10576427599998));
#301874=CARTESIAN_POINT('Ctrl Pts',(-1.47624193300006,2.2,4.10576427599998));
#301875=CARTESIAN_POINT('Ctrl Pts',(-1.47637628300005,12.2,4.10381286499998));
#301876=CARTESIAN_POINT('Ctrl Pts',(-1.47637628300005,5.2,4.10381286499998));
#301877=CARTESIAN_POINT('Ctrl Pts',(-1.47637628300005,2.2,4.10381286499998));
#301878=CARTESIAN_POINT('Ctrl Pts',(-1.47650817800006,12.2,4.10186542299999));
#301879=CARTESIAN_POINT('Ctrl Pts',(-1.47650817800006,5.2,4.10186542299999));
#301880=CARTESIAN_POINT('Ctrl Pts',(-1.47650817800006,2.2,4.10186542299999));
#301881=CARTESIAN_POINT('Ctrl Pts',(-1.47663762600006,12.2,4.09992195999998));
#301882=CARTESIAN_POINT('Ctrl Pts',(-1.47663762600006,5.2,4.09992195999998));
#301883=CARTESIAN_POINT('Ctrl Pts',(-1.47663762600006,2.2,4.09992195999998));
#301884=CARTESIAN_POINT('Ctrl Pts',(-1.47676463500006,12.2,4.09798248299998));
#301885=CARTESIAN_POINT('Ctrl Pts',(-1.47676463500006,5.2,4.09798248299998));
#301886=CARTESIAN_POINT('Ctrl Pts',(-1.47676463500006,2.2,4.09798248299998));
#301887=CARTESIAN_POINT('Ctrl Pts',(-1.47688921300006,12.2,4.09604699899998));
#301888=CARTESIAN_POINT('Ctrl Pts',(-1.47688921300006,5.2,4.09604699899998));
#301889=CARTESIAN_POINT('Ctrl Pts',(-1.47688921300006,2.2,4.09604699899998));
#301890=CARTESIAN_POINT('Ctrl Pts',(-1.47701136600006,12.2,4.09411551599998));
#301891=CARTESIAN_POINT('Ctrl Pts',(-1.47701136600006,5.2,4.09411551599998));
#301892=CARTESIAN_POINT('Ctrl Pts',(-1.47701136600006,2.2,4.09411551599998));
#301893=CARTESIAN_POINT('Ctrl Pts',(-1.47713110400006,12.2,4.09218804399998));
#301894=CARTESIAN_POINT('Ctrl Pts',(-1.47713110400006,5.2,4.09218804399998));
#301895=CARTESIAN_POINT('Ctrl Pts',(-1.47713110400006,2.2,4.09218804399998));
#301896=CARTESIAN_POINT('Ctrl Pts',(-1.47724843400006,12.2,4.09026458899999));
#301897=CARTESIAN_POINT('Ctrl Pts',(-1.47724843400006,5.2,4.09026458899999));
#301898=CARTESIAN_POINT('Ctrl Pts',(-1.47724843400006,2.2,4.09026458899999));
#301899=CARTESIAN_POINT('Ctrl Pts',(-1.47736336500006,12.2,4.08834515899999));
#301900=CARTESIAN_POINT('Ctrl Pts',(-1.47736336500006,5.2,4.08834515899999));
#301901=CARTESIAN_POINT('Ctrl Pts',(-1.47736336500006,2.2,4.08834515899999));
#301902=CARTESIAN_POINT('Ctrl Pts',(-1.47747590400006,12.2,4.08642976299999));
#301903=CARTESIAN_POINT('Ctrl Pts',(-1.47747590400006,5.2,4.08642976299999));
#301904=CARTESIAN_POINT('Ctrl Pts',(-1.47747590400006,2.2,4.08642976299999));
#301905=CARTESIAN_POINT('Ctrl Pts',(-1.47758605800006,12.2,4.08451840899998));
#301906=CARTESIAN_POINT('Ctrl Pts',(-1.47758605800006,5.2,4.08451840899998));
#301907=CARTESIAN_POINT('Ctrl Pts',(-1.47758605800006,2.2,4.08451840899998));
#301908=CARTESIAN_POINT('Ctrl Pts',(-1.47769383700005,12.2,4.08261110299998));
#301909=CARTESIAN_POINT('Ctrl Pts',(-1.47769383700005,5.2,4.08261110299998));
#301910=CARTESIAN_POINT('Ctrl Pts',(-1.47769383700005,2.2,4.08261110299998));
#301911=CARTESIAN_POINT('Ctrl Pts',(-1.47779924700006,12.2,4.08070785499999));
#301912=CARTESIAN_POINT('Ctrl Pts',(-1.47779924700006,5.2,4.08070785499999));
#301913=CARTESIAN_POINT('Ctrl Pts',(-1.47779924700006,2.2,4.08070785499999));
#301914=CARTESIAN_POINT('Ctrl Pts',(-1.47790229800006,12.2,4.07880867199999));
#301915=CARTESIAN_POINT('Ctrl Pts',(-1.47790229800006,5.2,4.07880867199999));
#301916=CARTESIAN_POINT('Ctrl Pts',(-1.47790229800006,2.2,4.07880867199999));
#301917=CARTESIAN_POINT('Ctrl Pts',(-1.47800299600006,12.2,4.07691356199999));
#301918=CARTESIAN_POINT('Ctrl Pts',(-1.47800299600006,5.2,4.07691356199999));
#301919=CARTESIAN_POINT('Ctrl Pts',(-1.47800299600006,2.2,4.07691356199999));
#301920=CARTESIAN_POINT('Ctrl Pts',(-1.47810135000006,12.2,4.07502253299998));
#301921=CARTESIAN_POINT('Ctrl Pts',(-1.47810135000006,5.2,4.07502253299998));
#301922=CARTESIAN_POINT('Ctrl Pts',(-1.47810135000006,2.2,4.07502253299998));
#301923=CARTESIAN_POINT('Ctrl Pts',(-1.47819737000006,12.2,4.07313559299999));
#301924=CARTESIAN_POINT('Ctrl Pts',(-1.47819737000006,5.2,4.07313559299999));
#301925=CARTESIAN_POINT('Ctrl Pts',(-1.47819737000006,2.2,4.07313559299999));
#301926=CARTESIAN_POINT('Ctrl Pts',(-1.47829106100006,12.2,4.07125274999999));
#301927=CARTESIAN_POINT('Ctrl Pts',(-1.47829106100006,5.2,4.07125274999999));
#301928=CARTESIAN_POINT('Ctrl Pts',(-1.47829106100006,2.2,4.07125274999999));
#301929=CARTESIAN_POINT('Ctrl Pts',(-1.47838243300006,12.2,4.06937401199999));
#301930=CARTESIAN_POINT('Ctrl Pts',(-1.47838243300006,5.2,4.06937401199999));
#301931=CARTESIAN_POINT('Ctrl Pts',(-1.47838243300006,2.2,4.06937401199999));
#301932=CARTESIAN_POINT('Ctrl Pts',(-1.47847149200006,12.2,4.06749938699999));
#301933=CARTESIAN_POINT('Ctrl Pts',(-1.47847149200006,5.2,4.06749938699999));
#301934=CARTESIAN_POINT('Ctrl Pts',(-1.47847149200006,2.2,4.06749938699999));
#301935=CARTESIAN_POINT('Ctrl Pts',(-1.47855825000006,12.2,4.06562888299998));
#301936=CARTESIAN_POINT('Ctrl Pts',(-1.47855825000006,5.2,4.06562888299998));
#301937=CARTESIAN_POINT('Ctrl Pts',(-1.47855825000006,2.2,4.06562888299998));
#301938=CARTESIAN_POINT('Ctrl Pts',(-1.47864271200006,12.2,4.06376250799998));
#301939=CARTESIAN_POINT('Ctrl Pts',(-1.47864271200006,5.2,4.06376250799998));
#301940=CARTESIAN_POINT('Ctrl Pts',(-1.47864271200006,2.2,4.06376250799998));
#301941=CARTESIAN_POINT('Ctrl Pts',(-1.47872488800005,12.2,4.06190026899999));
#301942=CARTESIAN_POINT('Ctrl Pts',(-1.47872488800005,5.2,4.06190026899999));
#301943=CARTESIAN_POINT('Ctrl Pts',(-1.47872488800005,2.2,4.06190026899999));
#301944=CARTESIAN_POINT('Ctrl Pts',(-1.47880478500006,12.2,4.06004217499999));
#301945=CARTESIAN_POINT('Ctrl Pts',(-1.47880478500006,5.2,4.06004217499999));
#301946=CARTESIAN_POINT('Ctrl Pts',(-1.47880478500006,2.2,4.06004217499999));
#301947=CARTESIAN_POINT('Ctrl Pts',(-1.47888241200006,12.2,4.05818823399999));
#301948=CARTESIAN_POINT('Ctrl Pts',(-1.47888241200006,5.2,4.05818823399999));
#301949=CARTESIAN_POINT('Ctrl Pts',(-1.47888241200006,2.2,4.05818823399999));
#301950=CARTESIAN_POINT('Ctrl Pts',(-1.47895777700006,12.2,4.05633845299998));
#301951=CARTESIAN_POINT('Ctrl Pts',(-1.47895777700006,5.2,4.05633845299998));
#301952=CARTESIAN_POINT('Ctrl Pts',(-1.47895777700006,2.2,4.05633845299998));
#301953=CARTESIAN_POINT('Ctrl Pts',(-1.47903088800006,12.2,4.05449284099999));
#301954=CARTESIAN_POINT('Ctrl Pts',(-1.47903088800006,5.2,4.05449284099999));
#301955=CARTESIAN_POINT('Ctrl Pts',(-1.47903088800006,2.2,4.05449284099999));
#301956=CARTESIAN_POINT('Ctrl Pts',(-1.47910175500006,12.2,4.05265140599998));
#301957=CARTESIAN_POINT('Ctrl Pts',(-1.47910175500006,5.2,4.05265140599998));
#301958=CARTESIAN_POINT('Ctrl Pts',(-1.47910175500006,2.2,4.05265140599998));
#301959=CARTESIAN_POINT('Ctrl Pts',(-1.47917038600006,12.2,4.05081415599999));
#301960=CARTESIAN_POINT('Ctrl Pts',(-1.47917038600006,5.2,4.05081415599999));
#301961=CARTESIAN_POINT('Ctrl Pts',(-1.47917038600006,2.2,4.05081415599999));
#301962=CARTESIAN_POINT('Ctrl Pts',(-1.47923678600006,12.2,4.04898109799999));
#301963=CARTESIAN_POINT('Ctrl Pts',(-1.47923678600006,5.2,4.04898109799999));
#301964=CARTESIAN_POINT('Ctrl Pts',(-1.47923678600006,2.2,4.04898109799999));
#301965=CARTESIAN_POINT('Ctrl Pts',(-1.47930096900006,12.2,4.04715224099998));
#301966=CARTESIAN_POINT('Ctrl Pts',(-1.47930096900006,5.2,4.04715224099998));
#301967=CARTESIAN_POINT('Ctrl Pts',(-1.47930096900006,2.2,4.04715224099998));
#301968=CARTESIAN_POINT('Ctrl Pts',(-1.47936293900006,12.2,4.04532759199999));
#301969=CARTESIAN_POINT('Ctrl Pts',(-1.47936293900006,5.2,4.04532759199999));
#301970=CARTESIAN_POINT('Ctrl Pts',(-1.47936293900006,2.2,4.04532759199999));
#301971=CARTESIAN_POINT('Ctrl Pts',(-1.47942270700006,12.2,4.04350715999998));
#301972=CARTESIAN_POINT('Ctrl Pts',(-1.47942270700006,5.2,4.04350715999998));
#301973=CARTESIAN_POINT('Ctrl Pts',(-1.47942270700006,2.2,4.04350715999998));
#301974=CARTESIAN_POINT('Ctrl Pts',(-1.47948028000006,12.2,4.04169095299999));
#301975=CARTESIAN_POINT('Ctrl Pts',(-1.47948028000006,5.2,4.04169095299999));
#301976=CARTESIAN_POINT('Ctrl Pts',(-1.47948028000006,2.2,4.04169095299999));
#301977=CARTESIAN_POINT('Ctrl Pts',(-1.47953566800005,12.2,4.03987897799999));
#301978=CARTESIAN_POINT('Ctrl Pts',(-1.47953566800005,5.2,4.03987897799999));
#301979=CARTESIAN_POINT('Ctrl Pts',(-1.47953566800005,2.2,4.03987897799999));
#301980=CARTESIAN_POINT('Ctrl Pts',(-1.47958887800006,12.2,4.03807124299998));
#301981=CARTESIAN_POINT('Ctrl Pts',(-1.47958887800006,5.2,4.03807124299998));
#301982=CARTESIAN_POINT('Ctrl Pts',(-1.47958887800006,2.2,4.03807124299998));
#301983=CARTESIAN_POINT('Ctrl Pts',(-1.47963992000006,12.2,4.03626775699998));
#301984=CARTESIAN_POINT('Ctrl Pts',(-1.47963992000006,5.2,4.03626775699998));
#301985=CARTESIAN_POINT('Ctrl Pts',(-1.47963992000006,2.2,4.03626775699998));
#301986=CARTESIAN_POINT('Ctrl Pts',(-1.47968880200006,12.2,4.03446852799998));
#301987=CARTESIAN_POINT('Ctrl Pts',(-1.47968880200006,5.2,4.03446852799998));
#301988=CARTESIAN_POINT('Ctrl Pts',(-1.47968880200006,2.2,4.03446852799998));
#301989=CARTESIAN_POINT('Ctrl Pts',(-1.47973553200006,12.2,4.03267356299998));
#301990=CARTESIAN_POINT('Ctrl Pts',(-1.47973553200006,5.2,4.03267356299998));
#301991=CARTESIAN_POINT('Ctrl Pts',(-1.47973553200006,2.2,4.03267356299998));
#301992=CARTESIAN_POINT('Ctrl Pts',(-1.47978012000006,12.2,4.03088287099998));
#301993=CARTESIAN_POINT('Ctrl Pts',(-1.47978012000006,5.2,4.03088287099998));
#301994=CARTESIAN_POINT('Ctrl Pts',(-1.47978012000006,2.2,4.03088287099998));
#301995=CARTESIAN_POINT('Ctrl Pts',(-1.47982257300006,12.2,4.02909645899998));
#301996=CARTESIAN_POINT('Ctrl Pts',(-1.47982257300006,5.2,4.02909645899998));
#301997=CARTESIAN_POINT('Ctrl Pts',(-1.47982257300006,2.2,4.02909645899998));
#301998=CARTESIAN_POINT('Ctrl Pts',(-1.47986290300006,12.2,4.02731433599998));
#301999=CARTESIAN_POINT('Ctrl Pts',(-1.47986290300006,5.2,4.02731433599998));
#302000=CARTESIAN_POINT('Ctrl Pts',(-1.47986290300006,2.2,4.02731433599998));
#302001=CARTESIAN_POINT('Ctrl Pts',(-1.47990111500006,12.2,4.02553650999998));
#302002=CARTESIAN_POINT('Ctrl Pts',(-1.47990111500006,5.2,4.02553650999998));
#302003=CARTESIAN_POINT('Ctrl Pts',(-1.47990111500006,2.2,4.02553650999998));
#302004=CARTESIAN_POINT('Ctrl Pts',(-1.47993722000006,12.2,4.02376298799999));
#302005=CARTESIAN_POINT('Ctrl Pts',(-1.47993722000006,5.2,4.02376298799999));
#302006=CARTESIAN_POINT('Ctrl Pts',(-1.47993722000006,2.2,4.02376298799999));
#302007=CARTESIAN_POINT('Ctrl Pts',(-1.47997122500006,12.2,4.02199377799998));
#302008=CARTESIAN_POINT('Ctrl Pts',(-1.47997122500006,5.2,4.02199377799998));
#302009=CARTESIAN_POINT('Ctrl Pts',(-1.47997122500006,2.2,4.02199377799998));
#302010=CARTESIAN_POINT('Ctrl Pts',(-1.48000314100006,12.2,4.02022888899998));
#302011=CARTESIAN_POINT('Ctrl Pts',(-1.48000314100006,5.2,4.02022888899998));
#302012=CARTESIAN_POINT('Ctrl Pts',(-1.48000314100006,2.2,4.02022888899998));
#302013=CARTESIAN_POINT('Ctrl Pts',(-1.48003297500006,12.2,4.01846832999999));
#302014=CARTESIAN_POINT('Ctrl Pts',(-1.48003297500006,5.2,4.01846832999999));
#302015=CARTESIAN_POINT('Ctrl Pts',(-1.48003297500006,2.2,4.01846832999999));
#302016=CARTESIAN_POINT('Ctrl Pts',(-1.48006073700006,12.2,4.01671210599999));
#302017=CARTESIAN_POINT('Ctrl Pts',(-1.48006073700006,5.2,4.01671210599999));
#302018=CARTESIAN_POINT('Ctrl Pts',(-1.48006073700006,2.2,4.01671210599999));
#302019=CARTESIAN_POINT('Ctrl Pts',(-1.48008643700006,12.2,4.01496022799999));
#302020=CARTESIAN_POINT('Ctrl Pts',(-1.48008643700006,5.2,4.01496022799999));
#302021=CARTESIAN_POINT('Ctrl Pts',(-1.48008643700006,2.2,4.01496022799999));
#302022=CARTESIAN_POINT('Ctrl Pts',(-1.48011008100006,12.2,4.01321270199999));
#302023=CARTESIAN_POINT('Ctrl Pts',(-1.48011008100006,5.2,4.01321270199999));
#302024=CARTESIAN_POINT('Ctrl Pts',(-1.48011008100006,2.2,4.01321270199999));
#302025=CARTESIAN_POINT('Ctrl Pts',(-1.48013168000006,12.2,4.01146953699998));
#302026=CARTESIAN_POINT('Ctrl Pts',(-1.48013168000006,5.2,4.01146953699998));
#302027=CARTESIAN_POINT('Ctrl Pts',(-1.48013168000006,2.2,4.01146953699998));
#302028=CARTESIAN_POINT('Ctrl Pts',(-1.48015124300006,12.2,4.00973074099999));
#302029=CARTESIAN_POINT('Ctrl Pts',(-1.48015124300006,5.2,4.00973074099999));
#302030=CARTESIAN_POINT('Ctrl Pts',(-1.48015124300006,2.2,4.00973074099999));
#302031=CARTESIAN_POINT('Ctrl Pts',(-1.48016877800006,12.2,4.00799632099999));
#302032=CARTESIAN_POINT('Ctrl Pts',(-1.48016877800006,5.2,4.00799632099999));
#302033=CARTESIAN_POINT('Ctrl Pts',(-1.48016877800006,2.2,4.00799632099999));
#302034=CARTESIAN_POINT('Ctrl Pts',(-1.48018429500006,12.2,4.00626628699998));
#302035=CARTESIAN_POINT('Ctrl Pts',(-1.48018429500006,5.2,4.00626628699998));
#302036=CARTESIAN_POINT('Ctrl Pts',(-1.48018429500006,2.2,4.00626628699998));
#302037=CARTESIAN_POINT('Ctrl Pts',(-1.48019780300006,12.2,4.00454064499999));
#302038=CARTESIAN_POINT('Ctrl Pts',(-1.48019780300006,5.2,4.00454064499999));
#302039=CARTESIAN_POINT('Ctrl Pts',(-1.48019780300006,2.2,4.00454064499999));
#302040=CARTESIAN_POINT('Ctrl Pts',(-1.48020931000006,12.2,4.00281940399999));
#302041=CARTESIAN_POINT('Ctrl Pts',(-1.48020931000006,5.2,4.00281940399999));
#302042=CARTESIAN_POINT('Ctrl Pts',(-1.48020931000006,2.2,4.00281940399999));
#302043=CARTESIAN_POINT('Ctrl Pts',(-1.48021882600006,12.2,4.00110257199999));
#302044=CARTESIAN_POINT('Ctrl Pts',(-1.48021882600006,5.2,4.00110257199999));
#302045=CARTESIAN_POINT('Ctrl Pts',(-1.48021882600006,2.2,4.00110257199999));
#302046=CARTESIAN_POINT('Ctrl Pts',(-1.48022636200006,12.2,3.99939015799998));
#302047=CARTESIAN_POINT('Ctrl Pts',(-1.48022636200006,5.2,3.99939015799998));
#302048=CARTESIAN_POINT('Ctrl Pts',(-1.48022636200006,2.2,3.99939015799998));
#302049=CARTESIAN_POINT('Ctrl Pts',(-1.48023192300006,12.2,3.99768216799998));
#302050=CARTESIAN_POINT('Ctrl Pts',(-1.48023192300006,5.2,3.99768216799998));
#302051=CARTESIAN_POINT('Ctrl Pts',(-1.48023192300006,2.2,3.99768216799998));
#302052=CARTESIAN_POINT('Ctrl Pts',(-1.48023552100006,12.2,3.99597861199998));
#302053=CARTESIAN_POINT('Ctrl Pts',(-1.48023552100006,5.2,3.99597861199998));
#302054=CARTESIAN_POINT('Ctrl Pts',(-1.48023552100006,2.2,3.99597861199998));
#302055=CARTESIAN_POINT('Ctrl Pts',(-1.48023716600005,12.2,3.99427949599998));
#302056=CARTESIAN_POINT('Ctrl Pts',(-1.48023716600005,5.2,3.99427949599998));
#302057=CARTESIAN_POINT('Ctrl Pts',(-1.48023716600005,2.2,3.99427949599998));
#302058=CARTESIAN_POINT('Ctrl Pts',(-1.48023686500006,12.2,3.99258482999999));
#302059=CARTESIAN_POINT('Ctrl Pts',(-1.48023686500006,5.2,3.99258482999999));
#302060=CARTESIAN_POINT('Ctrl Pts',(-1.48023686500006,2.2,3.99258482999999));
#302061=CARTESIAN_POINT('Ctrl Pts',(-1.48023462900006,12.2,3.99089462199999));
#302062=CARTESIAN_POINT('Ctrl Pts',(-1.48023462900006,5.2,3.99089462199999));
#302063=CARTESIAN_POINT('Ctrl Pts',(-1.48023462900006,2.2,3.99089462199999));
#302064=CARTESIAN_POINT('Ctrl Pts',(-1.48023046600006,12.2,3.98920887799999));
#302065=CARTESIAN_POINT('Ctrl Pts',(-1.48023046600006,5.2,3.98920887799999));
#302066=CARTESIAN_POINT('Ctrl Pts',(-1.48023046600006,2.2,3.98920887799999));
#302067=CARTESIAN_POINT('Ctrl Pts',(-1.48022438700006,12.2,3.98752760799999));
#302068=CARTESIAN_POINT('Ctrl Pts',(-1.48022438700006,5.2,3.98752760799999));
#302069=CARTESIAN_POINT('Ctrl Pts',(-1.48022438700006,2.2,3.98752760799999));
#302070=CARTESIAN_POINT('Ctrl Pts',(-1.48021639900006,12.2,3.98585081899999));
#302071=CARTESIAN_POINT('Ctrl Pts',(-1.48021639900006,5.2,3.98585081899999));
#302072=CARTESIAN_POINT('Ctrl Pts',(-1.48021639900006,2.2,3.98585081899999));
#302073=CARTESIAN_POINT('Ctrl Pts',(-1.48020651400006,12.2,3.98417852099998));
#302074=CARTESIAN_POINT('Ctrl Pts',(-1.48020651400006,5.2,3.98417852099998));
#302075=CARTESIAN_POINT('Ctrl Pts',(-1.48020651400006,2.2,3.98417852099998));
#302076=CARTESIAN_POINT('Ctrl Pts',(-1.48019474000006,12.2,3.98251071999999));
#302077=CARTESIAN_POINT('Ctrl Pts',(-1.48019474000006,5.2,3.98251071999999));
#302078=CARTESIAN_POINT('Ctrl Pts',(-1.48019474000006,2.2,3.98251071999999));
#302079=CARTESIAN_POINT('Ctrl Pts',(-1.48018108700006,12.2,3.98084742399998));
#302080=CARTESIAN_POINT('Ctrl Pts',(-1.48018108700006,5.2,3.98084742399998));
#302081=CARTESIAN_POINT('Ctrl Pts',(-1.48018108700006,2.2,3.98084742399998));
#302082=CARTESIAN_POINT('Ctrl Pts',(-1.48016556400006,12.2,3.97918864299999));
#302083=CARTESIAN_POINT('Ctrl Pts',(-1.48016556400006,5.2,3.97918864299999));
#302084=CARTESIAN_POINT('Ctrl Pts',(-1.48016556400006,2.2,3.97918864299999));
#302085=CARTESIAN_POINT('Ctrl Pts',(-1.48014818000005,12.2,3.97753438199998));
#302086=CARTESIAN_POINT('Ctrl Pts',(-1.48014818000005,5.2,3.97753438199998));
#302087=CARTESIAN_POINT('Ctrl Pts',(-1.48014818000005,2.2,3.97753438199998));
#302088=CARTESIAN_POINT('Ctrl Pts',(-1.48012894600006,12.2,3.97588465299999));
#302089=CARTESIAN_POINT('Ctrl Pts',(-1.48012894600006,5.2,3.97588465299999));
#302090=CARTESIAN_POINT('Ctrl Pts',(-1.48012894600006,2.2,3.97588465299999));
#302091=CARTESIAN_POINT('Ctrl Pts',(-1.48010787200006,12.2,3.97423945999999));
#302092=CARTESIAN_POINT('Ctrl Pts',(-1.48010787200006,5.2,3.97423945999999));
#302093=CARTESIAN_POINT('Ctrl Pts',(-1.48010787200006,2.2,3.97423945999999));
#302094=CARTESIAN_POINT('Ctrl Pts',(-1.48008496500006,12.2,3.97259881399999));
#302095=CARTESIAN_POINT('Ctrl Pts',(-1.48008496500006,5.2,3.97259881399999));
#302096=CARTESIAN_POINT('Ctrl Pts',(-1.48008496500006,2.2,3.97259881399999));
#302097=CARTESIAN_POINT('Ctrl Pts',(-1.48006023600006,12.2,3.97096272199998));
#302098=CARTESIAN_POINT('Ctrl Pts',(-1.48006023600006,5.2,3.97096272199998));
#302099=CARTESIAN_POINT('Ctrl Pts',(-1.48006023600006,2.2,3.97096272199998));
#302100=CARTESIAN_POINT('Ctrl Pts',(-1.48003369600006,12.2,3.96933119299998));
#302101=CARTESIAN_POINT('Ctrl Pts',(-1.48003369600006,5.2,3.96933119299998));
#302102=CARTESIAN_POINT('Ctrl Pts',(-1.48003369600006,2.2,3.96933119299998));
#302103=CARTESIAN_POINT('Ctrl Pts',(-1.48000535300006,12.2,3.96770423299999));
#302104=CARTESIAN_POINT('Ctrl Pts',(-1.48000535300006,5.2,3.96770423299999));
#302105=CARTESIAN_POINT('Ctrl Pts',(-1.48000535300006,2.2,3.96770423299999));
#302106=CARTESIAN_POINT('Ctrl Pts',(-1.47997521700006,12.2,3.96608185299999));
#302107=CARTESIAN_POINT('Ctrl Pts',(-1.47997521700006,5.2,3.96608185299999));
#302108=CARTESIAN_POINT('Ctrl Pts',(-1.47997521700006,2.2,3.96608185299999));
#302109=CARTESIAN_POINT('Ctrl Pts',(-1.47994329900005,12.2,3.96446405799999));
#302110=CARTESIAN_POINT('Ctrl Pts',(-1.47994329900005,5.2,3.96446405799999));
#302111=CARTESIAN_POINT('Ctrl Pts',(-1.47994329900005,2.2,3.96446405799999));
#302112=CARTESIAN_POINT('Ctrl Pts',(-1.47990960800006,12.2,3.96285085899999));
#302113=CARTESIAN_POINT('Ctrl Pts',(-1.47990960800006,5.2,3.96285085899999));
#302114=CARTESIAN_POINT('Ctrl Pts',(-1.47990960800006,2.2,3.96285085899999));
#302115=CARTESIAN_POINT('Ctrl Pts',(-1.47987415200006,12.2,3.96124226199999));
#302116=CARTESIAN_POINT('Ctrl Pts',(-1.47987415200006,5.2,3.96124226199999));
#302117=CARTESIAN_POINT('Ctrl Pts',(-1.47987415200006,2.2,3.96124226199999));
#302118=CARTESIAN_POINT('Ctrl Pts',(-1.47983694400006,12.2,3.95963827599999));
#302119=CARTESIAN_POINT('Ctrl Pts',(-1.47983694400006,5.2,3.95963827599999));
#302120=CARTESIAN_POINT('Ctrl Pts',(-1.47983694400006,2.2,3.95963827599999));
#302121=CARTESIAN_POINT('Ctrl Pts',(-1.47979799200006,12.2,3.95803890899998));
#302122=CARTESIAN_POINT('Ctrl Pts',(-1.47979799200006,5.2,3.95803890899998));
#302123=CARTESIAN_POINT('Ctrl Pts',(-1.47979799200006,2.2,3.95803890899998));
#302124=CARTESIAN_POINT('Ctrl Pts',(-1.47975730600006,12.2,3.95644416899999));
#302125=CARTESIAN_POINT('Ctrl Pts',(-1.47975730600006,5.2,3.95644416899999));
#302126=CARTESIAN_POINT('Ctrl Pts',(-1.47975730600006,2.2,3.95644416899999));
#302127=CARTESIAN_POINT('Ctrl Pts',(-1.47971489600006,12.2,3.95485406399998));
#302128=CARTESIAN_POINT('Ctrl Pts',(-1.47971489600006,5.2,3.95485406399998));
#302129=CARTESIAN_POINT('Ctrl Pts',(-1.47971489600006,2.2,3.95485406399998));
#302130=CARTESIAN_POINT('Ctrl Pts',(-1.47967077300006,12.2,3.95326860199999));
#302131=CARTESIAN_POINT('Ctrl Pts',(-1.47967077300006,5.2,3.95326860199999));
#302132=CARTESIAN_POINT('Ctrl Pts',(-1.47967077300006,2.2,3.95326860199999));
#302133=CARTESIAN_POINT('Ctrl Pts',(-1.47962494700006,12.2,3.95168779099999));
#302134=CARTESIAN_POINT('Ctrl Pts',(-1.47962494700006,5.2,3.95168779099999));
#302135=CARTESIAN_POINT('Ctrl Pts',(-1.47962494700006,2.2,3.95168779099999));
#302136=CARTESIAN_POINT('Ctrl Pts',(-1.47957742600005,12.2,3.95011164099999));
#302137=CARTESIAN_POINT('Ctrl Pts',(-1.47957742600005,5.2,3.95011164099999));
#302138=CARTESIAN_POINT('Ctrl Pts',(-1.47957742600005,2.2,3.95011164099999));
#302139=CARTESIAN_POINT('Ctrl Pts',(-1.47952822100006,12.2,3.94854015799999));
#302140=CARTESIAN_POINT('Ctrl Pts',(-1.47952822100006,5.2,3.94854015799999));
#302141=CARTESIAN_POINT('Ctrl Pts',(-1.47952822100006,2.2,3.94854015799999));
#302142=CARTESIAN_POINT('Ctrl Pts',(-1.47947734300006,12.2,3.94697334999999));
#302143=CARTESIAN_POINT('Ctrl Pts',(-1.47947734300006,5.2,3.94697334999999));
#302144=CARTESIAN_POINT('Ctrl Pts',(-1.47947734300006,2.2,3.94697334999999));
#302145=CARTESIAN_POINT('Ctrl Pts',(-1.47942480100006,12.2,3.94541122599998));
#302146=CARTESIAN_POINT('Ctrl Pts',(-1.47942480100006,5.2,3.94541122599998));
#302147=CARTESIAN_POINT('Ctrl Pts',(-1.47942480100006,2.2,3.94541122599998));
#302148=CARTESIAN_POINT('Ctrl Pts',(-1.47937060600006,12.2,3.94385379399999));
#302149=CARTESIAN_POINT('Ctrl Pts',(-1.47937060600006,5.2,3.94385379399999));
#302150=CARTESIAN_POINT('Ctrl Pts',(-1.47937060600006,2.2,3.94385379399999));
#302151=CARTESIAN_POINT('Ctrl Pts',(-1.47931476800006,12.2,3.94230106299998));
#302152=CARTESIAN_POINT('Ctrl Pts',(-1.47931476800006,5.2,3.94230106299998));
#302153=CARTESIAN_POINT('Ctrl Pts',(-1.47931476800006,2.2,3.94230106299998));
#302154=CARTESIAN_POINT('Ctrl Pts',(-1.47925729700006,12.2,3.94075303899999));
#302155=CARTESIAN_POINT('Ctrl Pts',(-1.47925729700006,5.2,3.94075303899999));
#302156=CARTESIAN_POINT('Ctrl Pts',(-1.47925729700006,2.2,3.94075303899999));
#302157=CARTESIAN_POINT('Ctrl Pts',(-1.47919820300006,12.2,3.93920973199998));
#302158=CARTESIAN_POINT('Ctrl Pts',(-1.47919820300006,5.2,3.93920973199998));
#302159=CARTESIAN_POINT('Ctrl Pts',(-1.47919820300006,2.2,3.93920973199998));
#302160=CARTESIAN_POINT('Ctrl Pts',(-1.47913749800006,12.2,3.93767114899998));
#302161=CARTESIAN_POINT('Ctrl Pts',(-1.47913749800006,5.2,3.93767114899998));
#302162=CARTESIAN_POINT('Ctrl Pts',(-1.47913749800006,2.2,3.93767114899998));
#302163=CARTESIAN_POINT('Ctrl Pts',(-1.47907519000006,12.2,3.93613729899998));
#302164=CARTESIAN_POINT('Ctrl Pts',(-1.47907519000006,5.2,3.93613729899998));
#302165=CARTESIAN_POINT('Ctrl Pts',(-1.47907519000006,2.2,3.93613729899998));
#302166=CARTESIAN_POINT('Ctrl Pts',(-1.47901129000006,12.2,3.93460818899998));
#302167=CARTESIAN_POINT('Ctrl Pts',(-1.47901129000006,5.2,3.93460818899998));
#302168=CARTESIAN_POINT('Ctrl Pts',(-1.47901129000006,2.2,3.93460818899998));
#302169=CARTESIAN_POINT('Ctrl Pts',(-1.47894580800006,12.2,3.93308382899999));
#302170=CARTESIAN_POINT('Ctrl Pts',(-1.47894580800006,5.2,3.93308382899999));
#302171=CARTESIAN_POINT('Ctrl Pts',(-1.47894580800006,2.2,3.93308382899999));
#302172=CARTESIAN_POINT('Ctrl Pts',(-1.47887875600005,12.2,3.93156422499998));
#302173=CARTESIAN_POINT('Ctrl Pts',(-1.47887875600005,5.2,3.93156422499998));
#302174=CARTESIAN_POINT('Ctrl Pts',(-1.47887875600005,2.2,3.93156422499998));
#302175=CARTESIAN_POINT('Ctrl Pts',(-1.47881014300006,12.2,3.93004938699999));
#302176=CARTESIAN_POINT('Ctrl Pts',(-1.47881014300006,5.2,3.93004938699999));
#302177=CARTESIAN_POINT('Ctrl Pts',(-1.47881014300006,2.2,3.93004938699999));
#302178=CARTESIAN_POINT('Ctrl Pts',(-1.47873998000006,12.2,3.92853932199999));
#302179=CARTESIAN_POINT('Ctrl Pts',(-1.47873998000006,5.2,3.92853932199999));
#302180=CARTESIAN_POINT('Ctrl Pts',(-1.47873998000006,2.2,3.92853932199999));
#302181=CARTESIAN_POINT('Ctrl Pts',(-1.47866827700006,12.2,3.92703403799998));
#302182=CARTESIAN_POINT('Ctrl Pts',(-1.47866827700006,5.2,3.92703403799998));
#302183=CARTESIAN_POINT('Ctrl Pts',(-1.47866827700006,2.2,3.92703403799998));
#302184=CARTESIAN_POINT('Ctrl Pts',(-1.47859504600006,12.2,3.92553354499999));
#302185=CARTESIAN_POINT('Ctrl Pts',(-1.47859504600006,5.2,3.92553354499999));
#302186=CARTESIAN_POINT('Ctrl Pts',(-1.47859504600006,2.2,3.92553354499999));
#302187=CARTESIAN_POINT('Ctrl Pts',(-1.47852029600006,12.2,3.92403784899999));
#302188=CARTESIAN_POINT('Ctrl Pts',(-1.47852029600006,5.2,3.92403784899999));
#302189=CARTESIAN_POINT('Ctrl Pts',(-1.47852029600006,2.2,3.92403784899999));
#302190=CARTESIAN_POINT('Ctrl Pts',(-1.47844403800006,12.2,3.92254695799998));
#302191=CARTESIAN_POINT('Ctrl Pts',(-1.47844403800006,5.2,3.92254695799998));
#302192=CARTESIAN_POINT('Ctrl Pts',(-1.47844403800006,2.2,3.92254695799998));
#302193=CARTESIAN_POINT('Ctrl Pts',(-1.47836628300006,12.2,3.92106088199998));
#302194=CARTESIAN_POINT('Ctrl Pts',(-1.47836628300006,5.2,3.92106088199998));
#302195=CARTESIAN_POINT('Ctrl Pts',(-1.47836628300006,2.2,3.92106088199998));
#302196=CARTESIAN_POINT('Ctrl Pts',(-1.47828704000006,12.2,3.91957962799999));
#302197=CARTESIAN_POINT('Ctrl Pts',(-1.47828704000006,5.2,3.91957962799999));
#302198=CARTESIAN_POINT('Ctrl Pts',(-1.47828704000006,2.2,3.91957962799999));
#302199=CARTESIAN_POINT('Ctrl Pts',(-1.47820632300006,12.2,3.91810320499999));
#302200=CARTESIAN_POINT('Ctrl Pts',(-1.47820632300006,5.2,3.91810320499999));
#302201=CARTESIAN_POINT('Ctrl Pts',(-1.47820632300006,2.2,3.91810320499999));
#302202=CARTESIAN_POINT('Ctrl Pts',(-1.47812414000006,12.2,3.91663161999999));
#302203=CARTESIAN_POINT('Ctrl Pts',(-1.47812414000006,5.2,3.91663161999999));
#302204=CARTESIAN_POINT('Ctrl Pts',(-1.47812414000006,2.2,3.91663161999999));
#302205=CARTESIAN_POINT('Ctrl Pts',(-1.47804050300006,12.2,3.91516488099998));
#302206=CARTESIAN_POINT('Ctrl Pts',(-1.47804050300006,5.2,3.91516488099998));
#302207=CARTESIAN_POINT('Ctrl Pts',(-1.47804050300006,2.2,3.91516488099998));
#302208=CARTESIAN_POINT('Ctrl Pts',(-1.47795542200006,12.2,3.91370299799998));
#302209=CARTESIAN_POINT('Ctrl Pts',(-1.47795542200006,5.2,3.91370299799998));
#302210=CARTESIAN_POINT('Ctrl Pts',(-1.47795542200006,2.2,3.91370299799998));
#302211=CARTESIAN_POINT('Ctrl Pts',(-1.47786890800006,12.2,3.91224597799999));
#302212=CARTESIAN_POINT('Ctrl Pts',(-1.47786890800006,5.2,3.91224597799999));
#302213=CARTESIAN_POINT('Ctrl Pts',(-1.47786890800006,2.2,3.91224597799999));
#302214=CARTESIAN_POINT('Ctrl Pts',(-1.47778097200006,12.2,3.91079382799998));
#302215=CARTESIAN_POINT('Ctrl Pts',(-1.47778097200006,5.2,3.91079382799998));
#302216=CARTESIAN_POINT('Ctrl Pts',(-1.47778097200006,2.2,3.91079382799998));
#302217=CARTESIAN_POINT('Ctrl Pts',(-1.47769162500005,12.2,3.90934655899999));
#302218=CARTESIAN_POINT('Ctrl Pts',(-1.47769162500005,5.2,3.90934655899999));
#302219=CARTESIAN_POINT('Ctrl Pts',(-1.47769162500005,2.2,3.90934655899999));
#302220=CARTESIAN_POINT('Ctrl Pts',(-1.47760087800005,12.2,3.90790417599998));
#302221=CARTESIAN_POINT('Ctrl Pts',(-1.47760087800005,5.2,3.90790417599998));
#302222=CARTESIAN_POINT('Ctrl Pts',(-1.47760087800005,2.2,3.90790417599998));
#302223=CARTESIAN_POINT('Ctrl Pts',(-1.47750874100006,12.2,3.90646668999998));
#302224=CARTESIAN_POINT('Ctrl Pts',(-1.47750874100006,5.2,3.90646668999998));
#302225=CARTESIAN_POINT('Ctrl Pts',(-1.47750874100006,2.2,3.90646668999998));
#302226=CARTESIAN_POINT('Ctrl Pts',(-1.47741522700006,12.2,3.90503410799998));
#302227=CARTESIAN_POINT('Ctrl Pts',(-1.47741522700006,5.2,3.90503410799998));
#302228=CARTESIAN_POINT('Ctrl Pts',(-1.47741522700006,2.2,3.90503410799998));
#302229=CARTESIAN_POINT('Ctrl Pts',(-1.47732034500006,12.2,3.90360643799998));
#302230=CARTESIAN_POINT('Ctrl Pts',(-1.47732034500006,5.2,3.90360643799998));
#302231=CARTESIAN_POINT('Ctrl Pts',(-1.47732034500006,2.2,3.90360643799998));
#302232=CARTESIAN_POINT('Ctrl Pts',(-1.47722410700006,12.2,3.90218368799999));
#302233=CARTESIAN_POINT('Ctrl Pts',(-1.47722410700006,5.2,3.90218368799999));
#302234=CARTESIAN_POINT('Ctrl Pts',(-1.47722410700006,2.2,3.90218368799999));
#302235=CARTESIAN_POINT('Ctrl Pts',(-1.47712652400006,12.2,3.90076586599999));
#302236=CARTESIAN_POINT('Ctrl Pts',(-1.47712652400006,5.2,3.90076586599999));
#302237=CARTESIAN_POINT('Ctrl Pts',(-1.47712652400006,2.2,3.90076586599999));
#302238=CARTESIAN_POINT('Ctrl Pts',(-1.47702760700006,12.2,3.89935298299999));
#302239=CARTESIAN_POINT('Ctrl Pts',(-1.47702760700006,5.2,3.89935298299999));
#302240=CARTESIAN_POINT('Ctrl Pts',(-1.47702760700006,2.2,3.89935298299999));
#302241=CARTESIAN_POINT('Ctrl Pts',(-1.47692736800005,12.2,3.89794504199998));
#302242=CARTESIAN_POINT('Ctrl Pts',(-1.47692736800005,5.2,3.89794504199998));
#302243=CARTESIAN_POINT('Ctrl Pts',(-1.47692736800005,2.2,3.89794504199998));
#302244=CARTESIAN_POINT('Ctrl Pts',(-1.47682581600006,12.2,3.89654205599999));
#302245=CARTESIAN_POINT('Ctrl Pts',(-1.47682581600006,5.2,3.89654205599999));
#302246=CARTESIAN_POINT('Ctrl Pts',(-1.47682581600006,2.2,3.89654205599999));
#302247=CARTESIAN_POINT('Ctrl Pts',(-1.47672296500006,12.2,3.89514403099999));
#302248=CARTESIAN_POINT('Ctrl Pts',(-1.47672296500006,5.2,3.89514403099999));
#302249=CARTESIAN_POINT('Ctrl Pts',(-1.47672296500006,2.2,3.89514403099999));
#302250=CARTESIAN_POINT('Ctrl Pts',(-1.47661882400006,12.2,3.89375097499999));
#302251=CARTESIAN_POINT('Ctrl Pts',(-1.47661882400006,5.2,3.89375097499999));
#302252=CARTESIAN_POINT('Ctrl Pts',(-1.47661882400006,2.2,3.89375097499999));
#302253=CARTESIAN_POINT('Ctrl Pts',(-1.47651340600006,12.2,3.89236289699999));
#302254=CARTESIAN_POINT('Ctrl Pts',(-1.47651340600006,5.2,3.89236289699999));
#302255=CARTESIAN_POINT('Ctrl Pts',(-1.47651340600006,2.2,3.89236289699999));
#302256=CARTESIAN_POINT('Ctrl Pts',(-1.47640672200006,12.2,3.89097980499999));
#302257=CARTESIAN_POINT('Ctrl Pts',(-1.47640672200006,5.2,3.89097980499999));
#302258=CARTESIAN_POINT('Ctrl Pts',(-1.47640672200006,2.2,3.89097980499999));
#302259=CARTESIAN_POINT('Ctrl Pts',(-1.47629878100005,12.2,3.88960170699999));
#302260=CARTESIAN_POINT('Ctrl Pts',(-1.47629878100005,5.2,3.88960170699999));
#302261=CARTESIAN_POINT('Ctrl Pts',(-1.47629878100005,2.2,3.88960170699999));
#302262=CARTESIAN_POINT('Ctrl Pts',(-1.47618959800006,12.2,3.88822861099998));
#302263=CARTESIAN_POINT('Ctrl Pts',(-1.47618959800006,5.2,3.88822861099998));
#302264=CARTESIAN_POINT('Ctrl Pts',(-1.47618959800006,2.2,3.88822861099998));
#302265=CARTESIAN_POINT('Ctrl Pts',(-1.47607918100006,12.2,3.88686052599999));
#302266=CARTESIAN_POINT('Ctrl Pts',(-1.47607918100006,5.2,3.88686052599999));
#302267=CARTESIAN_POINT('Ctrl Pts',(-1.47607918100006,2.2,3.88686052599999));
#302268=CARTESIAN_POINT('Ctrl Pts',(-1.47596754500006,12.2,3.88549745999998));
#302269=CARTESIAN_POINT('Ctrl Pts',(-1.47596754500006,5.2,3.88549745999998));
#302270=CARTESIAN_POINT('Ctrl Pts',(-1.47596754500006,2.2,3.88549745999998));
#302271=CARTESIAN_POINT('Ctrl Pts',(-1.47585469900006,12.2,3.88413941999998));
#302272=CARTESIAN_POINT('Ctrl Pts',(-1.47585469900006,5.2,3.88413941999998));
#302273=CARTESIAN_POINT('Ctrl Pts',(-1.47585469900006,2.2,3.88413941999998));
#302274=CARTESIAN_POINT('Ctrl Pts',(-1.47574065500006,12.2,3.88278641599998));
#302275=CARTESIAN_POINT('Ctrl Pts',(-1.47574065500006,5.2,3.88278641599998));
#302276=CARTESIAN_POINT('Ctrl Pts',(-1.47574065500006,2.2,3.88278641599998));
#302277=CARTESIAN_POINT('Ctrl Pts',(-1.47562542500006,12.2,3.88143845599998));
#302278=CARTESIAN_POINT('Ctrl Pts',(-1.47562542500006,5.2,3.88143845599998));
#302279=CARTESIAN_POINT('Ctrl Pts',(-1.47562542500006,2.2,3.88143845599998));
#302280=CARTESIAN_POINT('Ctrl Pts',(-1.47550902100006,12.2,3.88009554599999));
#302281=CARTESIAN_POINT('Ctrl Pts',(-1.47550902100006,5.2,3.88009554599999));
#302282=CARTESIAN_POINT('Ctrl Pts',(-1.47550902100006,2.2,3.88009554599999));
#302283=CARTESIAN_POINT('Ctrl Pts',(-1.47539145400006,12.2,3.87875769699999));
#302284=CARTESIAN_POINT('Ctrl Pts',(-1.47539145400006,5.2,3.87875769699999));
#302285=CARTESIAN_POINT('Ctrl Pts',(-1.47539145400006,2.2,3.87875769699999));
#302286=CARTESIAN_POINT('Ctrl Pts',(-1.47527273500006,12.2,3.87742491599998));
#302287=CARTESIAN_POINT('Ctrl Pts',(-1.47527273500006,5.2,3.87742491599998));
#302288=CARTESIAN_POINT('Ctrl Pts',(-1.47527273500006,2.2,3.87742491599998));
#302289=CARTESIAN_POINT('Ctrl Pts',(-1.47515287800006,12.2,3.87609721099999));
#302290=CARTESIAN_POINT('Ctrl Pts',(-1.47515287800006,5.2,3.87609721099999));
#302291=CARTESIAN_POINT('Ctrl Pts',(-1.47515287800006,2.2,3.87609721099999));
#302292=CARTESIAN_POINT('Ctrl Pts',(-1.47503189200005,12.2,3.87477459099999));
#302293=CARTESIAN_POINT('Ctrl Pts',(-1.47503189200005,5.2,3.87477459099999));
#302294=CARTESIAN_POINT('Ctrl Pts',(-1.47503189200005,2.2,3.87477459099999));
#302295=CARTESIAN_POINT('Ctrl Pts',(-1.47490979000006,12.2,3.87345706399999));
#302296=CARTESIAN_POINT('Ctrl Pts',(-1.47490979000006,5.2,3.87345706399999));
#302297=CARTESIAN_POINT('Ctrl Pts',(-1.47490979000006,2.2,3.87345706399999));
#302298=CARTESIAN_POINT('Ctrl Pts',(-1.47478658500006,12.2,3.87214463699999));
#302299=CARTESIAN_POINT('Ctrl Pts',(-1.47478658500006,5.2,3.87214463699999));
#302300=CARTESIAN_POINT('Ctrl Pts',(-1.47478658500006,2.2,3.87214463699999));
#302301=CARTESIAN_POINT('Ctrl Pts',(-1.47466228700006,12.2,3.87083732099998));
#302302=CARTESIAN_POINT('Ctrl Pts',(-1.47466228700006,5.2,3.87083732099998));
#302303=CARTESIAN_POINT('Ctrl Pts',(-1.47466228700006,2.2,3.87083732099998));
#302304=CARTESIAN_POINT('Ctrl Pts',(-1.47453690800006,12.2,3.86953512199998));
#302305=CARTESIAN_POINT('Ctrl Pts',(-1.47453690800006,5.2,3.86953512199998));
#302306=CARTESIAN_POINT('Ctrl Pts',(-1.47453690800006,2.2,3.86953512199998));
#302307=CARTESIAN_POINT('Ctrl Pts',(-1.47441046100006,12.2,3.86823804799998));
#302308=CARTESIAN_POINT('Ctrl Pts',(-1.47441046100006,5.2,3.86823804799998));
#302309=CARTESIAN_POINT('Ctrl Pts',(-1.47441046100006,2.2,3.86823804799998));
#302310=CARTESIAN_POINT('Ctrl Pts',(-1.47428295900006,12.2,3.86694610899998));
#302311=CARTESIAN_POINT('Ctrl Pts',(-1.47428295900006,5.2,3.86694610899998));
#302312=CARTESIAN_POINT('Ctrl Pts',(-1.47428295900006,2.2,3.86694610899998));
#302313=CARTESIAN_POINT('Ctrl Pts',(-1.47415441200006,12.2,3.86565931099998));
#302314=CARTESIAN_POINT('Ctrl Pts',(-1.47415441200006,5.2,3.86565931099998));
#302315=CARTESIAN_POINT('Ctrl Pts',(-1.47415441200006,2.2,3.86565931099998));
#302316=CARTESIAN_POINT('Ctrl Pts',(-1.47402483300006,12.2,3.86437766499999));
#302317=CARTESIAN_POINT('Ctrl Pts',(-1.47402483300006,5.2,3.86437766499999));
#302318=CARTESIAN_POINT('Ctrl Pts',(-1.47402483300006,2.2,3.86437766499999));
#302319=CARTESIAN_POINT('Ctrl Pts',(-1.47389423200006,12.2,3.86310117799999));
#302320=CARTESIAN_POINT('Ctrl Pts',(-1.47389423200006,5.2,3.86310117799999));
#302321=CARTESIAN_POINT('Ctrl Pts',(-1.47389423200006,2.2,3.86310117799999));
#302322=CARTESIAN_POINT('Ctrl Pts',(-1.47376262400006,12.2,3.86182985599999));
#302323=CARTESIAN_POINT('Ctrl Pts',(-1.47376262400006,5.2,3.86182985599999));
#302324=CARTESIAN_POINT('Ctrl Pts',(-1.47376262400006,2.2,3.86182985599999));
#302325=CARTESIAN_POINT('Ctrl Pts',(-1.47363002000006,12.2,3.86056371099999));
#302326=CARTESIAN_POINT('Ctrl Pts',(-1.47363002000006,5.2,3.86056371099999));
#302327=CARTESIAN_POINT('Ctrl Pts',(-1.47363002000006,2.2,3.86056371099999));
#302328=CARTESIAN_POINT('Ctrl Pts',(-1.47349643200006,12.2,3.85930274899999));
#302329=CARTESIAN_POINT('Ctrl Pts',(-1.47349643200006,5.2,3.85930274899999));
#302330=CARTESIAN_POINT('Ctrl Pts',(-1.47349643200006,2.2,3.85930274899999));
#302331=CARTESIAN_POINT('Ctrl Pts',(-1.47336187400006,12.2,3.85804697899999));
#302332=CARTESIAN_POINT('Ctrl Pts',(-1.47336187400006,5.2,3.85804697899999));
#302333=CARTESIAN_POINT('Ctrl Pts',(-1.47336187400006,2.2,3.85804697899999));
#302334=CARTESIAN_POINT('Ctrl Pts',(-1.47322635500006,12.2,3.85679640999999));
#302335=CARTESIAN_POINT('Ctrl Pts',(-1.47322635500006,5.2,3.85679640999999));
#302336=CARTESIAN_POINT('Ctrl Pts',(-1.47322635500006,2.2,3.85679640999999));
#302337=CARTESIAN_POINT('Ctrl Pts',(-1.47308989000006,12.2,3.85555104799998));
#302338=CARTESIAN_POINT('Ctrl Pts',(-1.47308989000006,5.2,3.85555104799998));
#302339=CARTESIAN_POINT('Ctrl Pts',(-1.47308989000006,2.2,3.85555104799998));
#302340=CARTESIAN_POINT('Ctrl Pts',(-1.47295249000006,12.2,3.85431090299999));
#302341=CARTESIAN_POINT('Ctrl Pts',(-1.47295249000006,5.2,3.85431090299999));
#302342=CARTESIAN_POINT('Ctrl Pts',(-1.47295249000006,2.2,3.85431090299999));
#302343=CARTESIAN_POINT('Ctrl Pts',(-1.47281416900006,12.2,3.85307598399999));
#302344=CARTESIAN_POINT('Ctrl Pts',(-1.47281416900006,5.2,3.85307598399999));
#302345=CARTESIAN_POINT('Ctrl Pts',(-1.47281416900006,2.2,3.85307598399999));
#302346=CARTESIAN_POINT('Ctrl Pts',(-1.47267493700006,12.2,3.85184629699998));
#302347=CARTESIAN_POINT('Ctrl Pts',(-1.47267493700006,5.2,3.85184629699998));
#302348=CARTESIAN_POINT('Ctrl Pts',(-1.47267493700006,2.2,3.85184629699998));
#302349=CARTESIAN_POINT('Ctrl Pts',(-1.47253480800006,12.2,3.85062185299999));
#302350=CARTESIAN_POINT('Ctrl Pts',(-1.47253480800006,5.2,3.85062185299999));
#302351=CARTESIAN_POINT('Ctrl Pts',(-1.47253480800006,2.2,3.85062185299999));
#302352=CARTESIAN_POINT('Ctrl Pts',(-1.47239379500006,12.2,3.84940265599998));
#302353=CARTESIAN_POINT('Ctrl Pts',(-1.47239379500006,5.2,3.84940265599998));
#302354=CARTESIAN_POINT('Ctrl Pts',(-1.47239379500006,2.2,3.84940265599998));
#302355=CARTESIAN_POINT('Ctrl Pts',(-1.47225191000006,12.2,3.84818871999999));
#302356=CARTESIAN_POINT('Ctrl Pts',(-1.47225191000006,5.2,3.84818871999999));
#302357=CARTESIAN_POINT('Ctrl Pts',(-1.47225191000006,2.2,3.84818871999999));
#302358=CARTESIAN_POINT('Ctrl Pts',(-1.47210916400006,12.2,3.84698004899998));
#302359=CARTESIAN_POINT('Ctrl Pts',(-1.47210916400006,5.2,3.84698004899998));
#302360=CARTESIAN_POINT('Ctrl Pts',(-1.47210916400006,2.2,3.84698004899998));
#302361=CARTESIAN_POINT('Ctrl Pts',(-1.47196557200005,12.2,3.84577665299998));
#302362=CARTESIAN_POINT('Ctrl Pts',(-1.47196557200005,5.2,3.84577665299998));
#302363=CARTESIAN_POINT('Ctrl Pts',(-1.47196557200005,2.2,3.84577665299998));
#302364=CARTESIAN_POINT('Ctrl Pts',(-1.47182114600006,12.2,3.84457853999999));
#302365=CARTESIAN_POINT('Ctrl Pts',(-1.47182114600006,5.2,3.84457853999999));
#302366=CARTESIAN_POINT('Ctrl Pts',(-1.47182114600006,2.2,3.84457853999999));
#302367=CARTESIAN_POINT('Ctrl Pts',(-1.47167589900006,12.2,3.84338571799999));
#302368=CARTESIAN_POINT('Ctrl Pts',(-1.47167589900006,5.2,3.84338571799999));
#302369=CARTESIAN_POINT('Ctrl Pts',(-1.47167589900006,2.2,3.84338571799999));
#302370=CARTESIAN_POINT('Ctrl Pts',(-1.47152984200006,12.2,3.84219819599998));
#302371=CARTESIAN_POINT('Ctrl Pts',(-1.47152984200006,5.2,3.84219819599998));
#302372=CARTESIAN_POINT('Ctrl Pts',(-1.47152984200006,2.2,3.84219819599998));
#302373=CARTESIAN_POINT('Ctrl Pts',(-1.47138298900006,12.2,3.84101598099999));
#302374=CARTESIAN_POINT('Ctrl Pts',(-1.47138298900006,5.2,3.84101598099999));
#302375=CARTESIAN_POINT('Ctrl Pts',(-1.47138298900006,2.2,3.84101598099999));
#302376=CARTESIAN_POINT('Ctrl Pts',(-1.47123535300006,12.2,3.83983908399999));
#302377=CARTESIAN_POINT('Ctrl Pts',(-1.47123535300006,5.2,3.83983908399999));
#302378=CARTESIAN_POINT('Ctrl Pts',(-1.47123535300006,2.2,3.83983908399999));
#302379=CARTESIAN_POINT('Ctrl Pts',(-1.47108694700006,12.2,3.83866750899998));
#302380=CARTESIAN_POINT('Ctrl Pts',(-1.47108694700006,5.2,3.83866750899998));
#302381=CARTESIAN_POINT('Ctrl Pts',(-1.47108694700006,2.2,3.83866750899998));
#302382=CARTESIAN_POINT('Ctrl Pts',(-1.47093778500005,12.2,3.83750126899999));
#302383=CARTESIAN_POINT('Ctrl Pts',(-1.47093778500005,5.2,3.83750126899999));
#302384=CARTESIAN_POINT('Ctrl Pts',(-1.47093778500005,2.2,3.83750126899999));
#302385=CARTESIAN_POINT('Ctrl Pts',(-1.47078787700006,12.2,3.83634036799998));
#302386=CARTESIAN_POINT('Ctrl Pts',(-1.47078787700006,5.2,3.83634036799998));
#302387=CARTESIAN_POINT('Ctrl Pts',(-1.47078787700006,2.2,3.83634036799998));
#302388=CARTESIAN_POINT('Ctrl Pts',(-1.47063723800006,12.2,3.83518481799998));
#302389=CARTESIAN_POINT('Ctrl Pts',(-1.47063723800006,5.2,3.83518481799998));
#302390=CARTESIAN_POINT('Ctrl Pts',(-1.47063723800006,2.2,3.83518481799998));
#302391=CARTESIAN_POINT('Ctrl Pts',(-1.47048588000006,12.2,3.83403462499999));
#302392=CARTESIAN_POINT('Ctrl Pts',(-1.47048588000006,5.2,3.83403462499999));
#302393=CARTESIAN_POINT('Ctrl Pts',(-1.47048588000006,2.2,3.83403462499999));
#302394=CARTESIAN_POINT('Ctrl Pts',(-1.47033381800005,12.2,3.83288979899999));
#302395=CARTESIAN_POINT('Ctrl Pts',(-1.47033381800005,5.2,3.83288979899999));
#302396=CARTESIAN_POINT('Ctrl Pts',(-1.47033381800005,2.2,3.83288979899999));
#302397=CARTESIAN_POINT('Ctrl Pts',(-1.47018106300006,12.2,3.83175034699998));
#302398=CARTESIAN_POINT('Ctrl Pts',(-1.47018106300006,5.2,3.83175034699998));
#302399=CARTESIAN_POINT('Ctrl Pts',(-1.47018106300006,2.2,3.83175034699998));
#302400=CARTESIAN_POINT('Ctrl Pts',(-1.47002762900006,12.2,3.83061627699998));
#302401=CARTESIAN_POINT('Ctrl Pts',(-1.47002762900006,5.2,3.83061627699998));
#302402=CARTESIAN_POINT('Ctrl Pts',(-1.47002762900006,2.2,3.83061627699998));
#302403=CARTESIAN_POINT('Ctrl Pts',(-1.46987352900006,12.2,3.82948759799999));
#302404=CARTESIAN_POINT('Ctrl Pts',(-1.46987352900006,5.2,3.82948759799999));
#302405=CARTESIAN_POINT('Ctrl Pts',(-1.46987352900006,2.2,3.82948759799999));
#302406=CARTESIAN_POINT('Ctrl Pts',(-1.46971877700006,12.2,3.82836431999999));
#302407=CARTESIAN_POINT('Ctrl Pts',(-1.46971877700006,5.2,3.82836431999999));
#302408=CARTESIAN_POINT('Ctrl Pts',(-1.46971877700006,2.2,3.82836431999999));
#302409=CARTESIAN_POINT('Ctrl Pts',(-1.46956338500006,12.2,3.82724644799998));
#302410=CARTESIAN_POINT('Ctrl Pts',(-1.46956338500006,5.2,3.82724644799998));
#302411=CARTESIAN_POINT('Ctrl Pts',(-1.46956338500006,2.2,3.82724644799998));
#302412=CARTESIAN_POINT('Ctrl Pts',(-1.46940736800006,12.2,3.82613399199998));
#302413=CARTESIAN_POINT('Ctrl Pts',(-1.46940736800006,5.2,3.82613399199998));
#302414=CARTESIAN_POINT('Ctrl Pts',(-1.46940736800006,2.2,3.82613399199998));
#302415=CARTESIAN_POINT('Ctrl Pts',(-1.46925073800006,12.2,3.82502696099999));
#302416=CARTESIAN_POINT('Ctrl Pts',(-1.46925073800006,5.2,3.82502696099999));
#302417=CARTESIAN_POINT('Ctrl Pts',(-1.46925073800006,2.2,3.82502696099999));
#302418=CARTESIAN_POINT('Ctrl Pts',(-1.46909350800006,12.2,3.82392536299999));
#302419=CARTESIAN_POINT('Ctrl Pts',(-1.46909350800006,5.2,3.82392536299999));
#302420=CARTESIAN_POINT('Ctrl Pts',(-1.46909350800006,2.2,3.82392536299999));
#302421=CARTESIAN_POINT('Ctrl Pts',(-1.46893569400006,12.2,3.82282920599998));
#302422=CARTESIAN_POINT('Ctrl Pts',(-1.46893569400006,5.2,3.82282920599998));
#302423=CARTESIAN_POINT('Ctrl Pts',(-1.46893569400006,2.2,3.82282920599998));
#302424=CARTESIAN_POINT('Ctrl Pts',(-1.46877730700006,12.2,3.82173849699999));
#302425=CARTESIAN_POINT('Ctrl Pts',(-1.46877730700006,5.2,3.82173849699999));
#302426=CARTESIAN_POINT('Ctrl Pts',(-1.46877730700006,2.2,3.82173849699999));
#302427=CARTESIAN_POINT('Ctrl Pts',(-1.46861836100006,12.2,3.82065324699998));
#302428=CARTESIAN_POINT('Ctrl Pts',(-1.46861836100006,5.2,3.82065324699998));
#302429=CARTESIAN_POINT('Ctrl Pts',(-1.46861836100006,2.2,3.82065324699998));
#302430=CARTESIAN_POINT('Ctrl Pts',(-1.46845887000006,12.2,3.81957346299998));
#302431=CARTESIAN_POINT('Ctrl Pts',(-1.46845887000006,5.2,3.81957346299998));
#302432=CARTESIAN_POINT('Ctrl Pts',(-1.46845887000006,2.2,3.81957346299998));
#302433=CARTESIAN_POINT('Ctrl Pts',(-1.46829884900006,12.2,3.81849915399999));
#302434=CARTESIAN_POINT('Ctrl Pts',(-1.46829884900006,5.2,3.81849915399999));
#302435=CARTESIAN_POINT('Ctrl Pts',(-1.46829884900006,2.2,3.81849915399999));
#302436=CARTESIAN_POINT('Ctrl Pts',(-1.46813830800006,12.2,3.81743032699998));
#302437=CARTESIAN_POINT('Ctrl Pts',(-1.46813830800006,5.2,3.81743032699998));
#302438=CARTESIAN_POINT('Ctrl Pts',(-1.46813830800006,2.2,3.81743032699998));
#302439=CARTESIAN_POINT('Ctrl Pts',(-1.46797726500006,12.2,3.81636699099998));
#302440=CARTESIAN_POINT('Ctrl Pts',(-1.46797726500006,5.2,3.81636699099998));
#302441=CARTESIAN_POINT('Ctrl Pts',(-1.46797726500006,2.2,3.81636699099998));
#302442=CARTESIAN_POINT('Ctrl Pts',(-1.46781573100006,12.2,3.81530915599999));
#302443=CARTESIAN_POINT('Ctrl Pts',(-1.46781573100006,5.2,3.81530915599999));
#302444=CARTESIAN_POINT('Ctrl Pts',(-1.46781573100006,2.2,3.81530915599999));
#302445=CARTESIAN_POINT('Ctrl Pts',(-1.46765372000006,12.2,3.81425682799998));
#302446=CARTESIAN_POINT('Ctrl Pts',(-1.46765372000006,5.2,3.81425682799998));
#302447=CARTESIAN_POINT('Ctrl Pts',(-1.46765372000006,2.2,3.81425682799998));
#302448=CARTESIAN_POINT('Ctrl Pts',(-1.46749124700006,12.2,3.81321001499998));
#302449=CARTESIAN_POINT('Ctrl Pts',(-1.46749124700006,5.2,3.81321001499998));
#302450=CARTESIAN_POINT('Ctrl Pts',(-1.46749124700006,2.2,3.81321001499998));
#302451=CARTESIAN_POINT('Ctrl Pts',(-1.46732832600006,12.2,3.81216872799998));
#302452=CARTESIAN_POINT('Ctrl Pts',(-1.46732832600006,5.2,3.81216872799998));
#302453=CARTESIAN_POINT('Ctrl Pts',(-1.46732832600006,2.2,3.81216872799998));
#302454=CARTESIAN_POINT('Ctrl Pts',(-1.46716496900006,12.2,3.81113297399998));
#302455=CARTESIAN_POINT('Ctrl Pts',(-1.46716496900006,5.2,3.81113297399998));
#302456=CARTESIAN_POINT('Ctrl Pts',(-1.46716496900006,2.2,3.81113297399998));
#302457=CARTESIAN_POINT('Ctrl Pts',(-1.46700119300006,12.2,3.81010276099998));
#302458=CARTESIAN_POINT('Ctrl Pts',(-1.46700119300006,5.2,3.81010276099998));
#302459=CARTESIAN_POINT('Ctrl Pts',(-1.46700119300006,2.2,3.81010276099998));
#302460=CARTESIAN_POINT('Ctrl Pts',(-1.46683700900006,12.2,3.80907809799999));
#302461=CARTESIAN_POINT('Ctrl Pts',(-1.46683700900006,5.2,3.80907809799999));
#302462=CARTESIAN_POINT('Ctrl Pts',(-1.46683700900006,2.2,3.80907809799999));
#302463=CARTESIAN_POINT('Ctrl Pts',(-1.46667243200006,12.2,3.80805899299999));
#302464=CARTESIAN_POINT('Ctrl Pts',(-1.46667243200006,5.2,3.80805899299999));
#302465=CARTESIAN_POINT('Ctrl Pts',(-1.46667243200006,2.2,3.80805899299999));
#302466=CARTESIAN_POINT('Ctrl Pts',(-1.46650747700006,12.2,3.80704545499999));
#302467=CARTESIAN_POINT('Ctrl Pts',(-1.46650747700006,5.2,3.80704545499999));
#302468=CARTESIAN_POINT('Ctrl Pts',(-1.46650747700006,2.2,3.80704545499999));
#302469=CARTESIAN_POINT('Ctrl Pts',(-1.46634215800006,12.2,3.80603749199998));
#302470=CARTESIAN_POINT('Ctrl Pts',(-1.46634215800006,5.2,3.80603749199998));
#302471=CARTESIAN_POINT('Ctrl Pts',(-1.46634215800006,2.2,3.80603749199998));
#302472=CARTESIAN_POINT('Ctrl Pts',(-1.46617648900006,12.2,3.80503511099998));
#302473=CARTESIAN_POINT('Ctrl Pts',(-1.46617648900006,5.2,3.80503511099998));
#302474=CARTESIAN_POINT('Ctrl Pts',(-1.46617648900006,2.2,3.80503511099998));
#302475=CARTESIAN_POINT('Ctrl Pts',(-1.46601048300006,12.2,3.80403832299999));
#302476=CARTESIAN_POINT('Ctrl Pts',(-1.46601048300006,5.2,3.80403832299999));
#302477=CARTESIAN_POINT('Ctrl Pts',(-1.46601048300006,2.2,3.80403832299999));
#302478=CARTESIAN_POINT('Ctrl Pts',(-1.46584415700006,12.2,3.80304713499999));
#302479=CARTESIAN_POINT('Ctrl Pts',(-1.46584415700006,5.2,3.80304713499999));
#302480=CARTESIAN_POINT('Ctrl Pts',(-1.46584415700006,2.2,3.80304713499999));
#302481=CARTESIAN_POINT('Ctrl Pts',(-1.46567752200006,12.2,3.80206155499998));
#302482=CARTESIAN_POINT('Ctrl Pts',(-1.46567752200006,5.2,3.80206155499998));
#302483=CARTESIAN_POINT('Ctrl Pts',(-1.46567752200006,2.2,3.80206155499998));
#302484=CARTESIAN_POINT('Ctrl Pts',(-1.46551059500006,12.2,3.80108159299999));
#302485=CARTESIAN_POINT('Ctrl Pts',(-1.46551059500006,5.2,3.80108159299999));
#302486=CARTESIAN_POINT('Ctrl Pts',(-1.46551059500006,2.2,3.80108159299999));
#302487=CARTESIAN_POINT('Ctrl Pts',(-1.46534339000006,12.2,3.80010725399998));
#302488=CARTESIAN_POINT('Ctrl Pts',(-1.46534339000006,5.2,3.80010725399998));
#302489=CARTESIAN_POINT('Ctrl Pts',(-1.46534339000006,2.2,3.80010725399998));
#302490=CARTESIAN_POINT('Ctrl Pts',(-1.46517592200005,12.2,3.79913855099999));
#302491=CARTESIAN_POINT('Ctrl Pts',(-1.46517592200005,5.2,3.79913855099999));
#302492=CARTESIAN_POINT('Ctrl Pts',(-1.46517592200005,2.2,3.79913855099999));
#302493=CARTESIAN_POINT('Ctrl Pts',(-1.46500820400006,12.2,3.79817548899998));
#302494=CARTESIAN_POINT('Ctrl Pts',(-1.46500820400006,5.2,3.79817548899998));
#302495=CARTESIAN_POINT('Ctrl Pts',(-1.46500820400006,2.2,3.79817548899998));
#302496=CARTESIAN_POINT('Ctrl Pts',(-1.46484025100006,12.2,3.79721807799999));
#302497=CARTESIAN_POINT('Ctrl Pts',(-1.46484025100006,5.2,3.79721807799999));
#302498=CARTESIAN_POINT('Ctrl Pts',(-1.46484025100006,2.2,3.79721807799999));
#302499=CARTESIAN_POINT('Ctrl Pts',(-1.46467207800006,12.2,3.79626632699999));
#302500=CARTESIAN_POINT('Ctrl Pts',(-1.46467207800006,5.2,3.79626632699999));
#302501=CARTESIAN_POINT('Ctrl Pts',(-1.46467207800006,2.2,3.79626632699999));
#302502=CARTESIAN_POINT('Ctrl Pts',(-1.46450369900006,12.2,3.79532024099999));
#302503=CARTESIAN_POINT('Ctrl Pts',(-1.46450369900006,5.2,3.79532024099999));
#302504=CARTESIAN_POINT('Ctrl Pts',(-1.46450369900006,2.2,3.79532024099999));
#302505=CARTESIAN_POINT('Ctrl Pts',(-1.46433513000006,12.2,3.79437983299999));
#302506=CARTESIAN_POINT('Ctrl Pts',(-1.46433513000006,5.2,3.79437983299999));
#302507=CARTESIAN_POINT('Ctrl Pts',(-1.46433513000006,2.2,3.79437983299999));
#302508=CARTESIAN_POINT('Ctrl Pts',(-1.46416638600006,12.2,3.79344510799999));
#302509=CARTESIAN_POINT('Ctrl Pts',(-1.46416638600006,5.2,3.79344510799999));
#302510=CARTESIAN_POINT('Ctrl Pts',(-1.46416638600006,2.2,3.79344510799999));
#302511=CARTESIAN_POINT('Ctrl Pts',(-1.46399748000006,12.2,3.79251607599999));
#302512=CARTESIAN_POINT('Ctrl Pts',(-1.46399748000006,5.2,3.79251607599999));
#302513=CARTESIAN_POINT('Ctrl Pts',(-1.46399748000006,2.2,3.79251607599999));
#302514=CARTESIAN_POINT('Ctrl Pts',(-1.46382842800006,12.2,3.79159274499998));
#302515=CARTESIAN_POINT('Ctrl Pts',(-1.46382842800006,5.2,3.79159274499998));
#302516=CARTESIAN_POINT('Ctrl Pts',(-1.46382842800006,2.2,3.79159274499998));
#302517=CARTESIAN_POINT('Ctrl Pts',(-1.46365924500006,12.2,3.79067512299999));
#302518=CARTESIAN_POINT('Ctrl Pts',(-1.46365924500006,5.2,3.79067512299999));
#302519=CARTESIAN_POINT('Ctrl Pts',(-1.46365924500006,2.2,3.79067512299999));
#302520=CARTESIAN_POINT('Ctrl Pts',(-1.46348994600006,12.2,3.78976321999998));
#302521=CARTESIAN_POINT('Ctrl Pts',(-1.46348994600006,5.2,3.78976321999998));
#302522=CARTESIAN_POINT('Ctrl Pts',(-1.46348994600006,2.2,3.78976321999998));
#302523=CARTESIAN_POINT('Ctrl Pts',(-1.46332054500006,12.2,3.78885704299999));
#302524=CARTESIAN_POINT('Ctrl Pts',(-1.46332054500006,5.2,3.78885704299999));
#302525=CARTESIAN_POINT('Ctrl Pts',(-1.46332054500006,2.2,3.78885704299999));
#302526=CARTESIAN_POINT('Ctrl Pts',(-1.46315105800006,12.2,3.78795660099998));
#302527=CARTESIAN_POINT('Ctrl Pts',(-1.46315105800006,5.2,3.78795660099998));
#302528=CARTESIAN_POINT('Ctrl Pts',(-1.46315105800006,2.2,3.78795660099998));
#302529=CARTESIAN_POINT('Ctrl Pts',(-1.46298150100006,12.2,3.78706190199999));
#302530=CARTESIAN_POINT('Ctrl Pts',(-1.46298150100006,5.2,3.78706190199999));
#302531=CARTESIAN_POINT('Ctrl Pts',(-1.46298150100006,2.2,3.78706190199999));
#302532=CARTESIAN_POINT('Ctrl Pts',(-1.46281188800006,12.2,3.78617295499998));
#302533=CARTESIAN_POINT('Ctrl Pts',(-1.46281188800006,5.2,3.78617295499998));
#302534=CARTESIAN_POINT('Ctrl Pts',(-1.46281188800006,2.2,3.78617295499998));
#302535=CARTESIAN_POINT('Ctrl Pts',(-1.46264223400006,12.2,3.78528976799998));
#302536=CARTESIAN_POINT('Ctrl Pts',(-1.46264223400006,5.2,3.78528976799998));
#302537=CARTESIAN_POINT('Ctrl Pts',(-1.46264223400006,2.2,3.78528976799998));
#302538=CARTESIAN_POINT('Ctrl Pts',(-1.46247255500006,12.2,3.78441234999999));
#302539=CARTESIAN_POINT('Ctrl Pts',(-1.46247255500006,5.2,3.78441234999999));
#302540=CARTESIAN_POINT('Ctrl Pts',(-1.46247255500006,2.2,3.78441234999999));
#302541=CARTESIAN_POINT('Ctrl Pts',(-1.46230286600006,12.2,3.78354070899999));
#302542=CARTESIAN_POINT('Ctrl Pts',(-1.46230286600006,5.2,3.78354070899999));
#302543=CARTESIAN_POINT('Ctrl Pts',(-1.46230286600006,2.2,3.78354070899999));
#302544=CARTESIAN_POINT('Ctrl Pts',(-1.46213318200005,12.2,3.78267485399999));
#302545=CARTESIAN_POINT('Ctrl Pts',(-1.46213318200005,5.2,3.78267485399999));
#302546=CARTESIAN_POINT('Ctrl Pts',(-1.46213318200005,2.2,3.78267485399999));
#302547=CARTESIAN_POINT('Ctrl Pts',(-1.46196352000006,12.2,3.78181479199998));
#302548=CARTESIAN_POINT('Ctrl Pts',(-1.46196352000006,5.2,3.78181479199998));
#302549=CARTESIAN_POINT('Ctrl Pts',(-1.46196352000006,2.2,3.78181479199998));
#302550=CARTESIAN_POINT('Ctrl Pts',(-1.46179389300006,12.2,3.78096053299998));
#302551=CARTESIAN_POINT('Ctrl Pts',(-1.46179389300006,5.2,3.78096053299998));
#302552=CARTESIAN_POINT('Ctrl Pts',(-1.46179389300006,2.2,3.78096053299998));
#302553=CARTESIAN_POINT('Ctrl Pts',(-1.46162431900006,12.2,3.78011208499998));
#302554=CARTESIAN_POINT('Ctrl Pts',(-1.46162431900006,5.2,3.78011208499998));
#302555=CARTESIAN_POINT('Ctrl Pts',(-1.46162431900006,2.2,3.78011208499998));
#302556=CARTESIAN_POINT('Ctrl Pts',(-1.46145481200006,12.2,3.77926945699999));
#302557=CARTESIAN_POINT('Ctrl Pts',(-1.46145481200006,5.2,3.77926945699999));
#302558=CARTESIAN_POINT('Ctrl Pts',(-1.46145481200006,2.2,3.77926945699999));
#302559=CARTESIAN_POINT('Ctrl Pts',(-1.46128538900006,12.2,3.77843265599999));
#302560=CARTESIAN_POINT('Ctrl Pts',(-1.46128538900006,5.2,3.77843265599999));
#302561=CARTESIAN_POINT('Ctrl Pts',(-1.46128538900006,2.2,3.77843265599999));
#302562=CARTESIAN_POINT('Ctrl Pts',(-1.46111606400006,12.2,3.77760169299999));
#302563=CARTESIAN_POINT('Ctrl Pts',(-1.46111606400006,5.2,3.77760169299999));
#302564=CARTESIAN_POINT('Ctrl Pts',(-1.46111606400006,2.2,3.77760169299999));
#302565=CARTESIAN_POINT('Ctrl Pts',(-1.46094685400006,12.2,3.77677657299999));
#302566=CARTESIAN_POINT('Ctrl Pts',(-1.46094685400006,5.2,3.77677657299999));
#302567=CARTESIAN_POINT('Ctrl Pts',(-1.46094685400006,2.2,3.77677657299999));
#302568=CARTESIAN_POINT('Ctrl Pts',(-1.46077777400005,12.2,3.77595730799998));
#302569=CARTESIAN_POINT('Ctrl Pts',(-1.46077777400005,5.2,3.77595730799998));
#302570=CARTESIAN_POINT('Ctrl Pts',(-1.46077777400005,2.2,3.77595730799998));
#302571=CARTESIAN_POINT('Ctrl Pts',(-1.46060884100006,12.2,3.77514390399998));
#302572=CARTESIAN_POINT('Ctrl Pts',(-1.46060884100006,5.2,3.77514390399998));
#302573=CARTESIAN_POINT('Ctrl Pts',(-1.46060884100006,2.2,3.77514390399998));
#302574=CARTESIAN_POINT('Ctrl Pts',(-1.46044006900006,12.2,3.77433637099998));
#302575=CARTESIAN_POINT('Ctrl Pts',(-1.46044006900006,5.2,3.77433637099998));
#302576=CARTESIAN_POINT('Ctrl Pts',(-1.46044006900006,2.2,3.77433637099998));
#302577=CARTESIAN_POINT('Ctrl Pts',(-1.46027147600006,12.2,3.77353471599999));
#302578=CARTESIAN_POINT('Ctrl Pts',(-1.46027147600006,5.2,3.77353471599999));
#302579=CARTESIAN_POINT('Ctrl Pts',(-1.46027147600006,2.2,3.77353471599999));
#302580=CARTESIAN_POINT('Ctrl Pts',(-1.46010307700006,12.2,3.77273894899999));
#302581=CARTESIAN_POINT('Ctrl Pts',(-1.46010307700006,5.2,3.77273894899999));
#302582=CARTESIAN_POINT('Ctrl Pts',(-1.46010307700006,2.2,3.77273894899999));
#302583=CARTESIAN_POINT('Ctrl Pts',(-1.45993488800006,12.2,3.77194907799999));
#302584=CARTESIAN_POINT('Ctrl Pts',(-1.45993488800006,5.2,3.77194907799999));
#302585=CARTESIAN_POINT('Ctrl Pts',(-1.45993488800006,2.2,3.77194907799999));
#302586=CARTESIAN_POINT('Ctrl Pts',(-1.45976692500006,12.2,3.77116511099998));
#302587=CARTESIAN_POINT('Ctrl Pts',(-1.45976692500006,5.2,3.77116511099998));
#302588=CARTESIAN_POINT('Ctrl Pts',(-1.45976692500006,2.2,3.77116511099998));
#302589=CARTESIAN_POINT('Ctrl Pts',(-1.45959920500006,12.2,3.77038705699999));
#302590=CARTESIAN_POINT('Ctrl Pts',(-1.45959920500006,5.2,3.77038705699999));
#302591=CARTESIAN_POINT('Ctrl Pts',(-1.45959920500006,2.2,3.77038705699999));
#302592=CARTESIAN_POINT('Ctrl Pts',(-1.45943174500006,12.2,3.76961492499999));
#302593=CARTESIAN_POINT('Ctrl Pts',(-1.45943174500006,5.2,3.76961492499999));
#302594=CARTESIAN_POINT('Ctrl Pts',(-1.45943174500006,2.2,3.76961492499999));
#302595=CARTESIAN_POINT('Ctrl Pts',(-1.45926455800006,12.2,3.76884872199999));
#302596=CARTESIAN_POINT('Ctrl Pts',(-1.45926455800006,5.2,3.76884872199999));
#302597=CARTESIAN_POINT('Ctrl Pts',(-1.45926455800006,2.2,3.76884872199999));
#302598=CARTESIAN_POINT('Ctrl Pts',(-1.45909766400006,12.2,3.76808845899999));
#302599=CARTESIAN_POINT('Ctrl Pts',(-1.45909766400006,5.2,3.76808845899999));
#302600=CARTESIAN_POINT('Ctrl Pts',(-1.45909766400006,2.2,3.76808845899999));
#302601=CARTESIAN_POINT('Ctrl Pts',(-1.45893107700006,12.2,3.76733414199999));
#302602=CARTESIAN_POINT('Ctrl Pts',(-1.45893107700006,5.2,3.76733414199999));
#302603=CARTESIAN_POINT('Ctrl Pts',(-1.45893107700006,2.2,3.76733414199999));
#302604=CARTESIAN_POINT('Ctrl Pts',(-1.45876481400006,12.2,3.76658578099998));
#302605=CARTESIAN_POINT('Ctrl Pts',(-1.45876481400006,5.2,3.76658578099998));
#302606=CARTESIAN_POINT('Ctrl Pts',(-1.45876481400006,2.2,3.76658578099998));
#302607=CARTESIAN_POINT('Ctrl Pts',(-1.45859889200006,12.2,3.76584338299998));
#302608=CARTESIAN_POINT('Ctrl Pts',(-1.45859889200006,5.2,3.76584338299998));
#302609=CARTESIAN_POINT('Ctrl Pts',(-1.45859889200006,2.2,3.76584338299998));
#302610=CARTESIAN_POINT('Ctrl Pts',(-1.45843332800006,12.2,3.76510695899999));
#302611=CARTESIAN_POINT('Ctrl Pts',(-1.45843332800006,5.2,3.76510695899999));
#302612=CARTESIAN_POINT('Ctrl Pts',(-1.45843332800006,2.2,3.76510695899999));
#302613=CARTESIAN_POINT('Ctrl Pts',(-1.45826813800006,12.2,3.76437651499998));
#302614=CARTESIAN_POINT('Ctrl Pts',(-1.45826813800006,5.2,3.76437651499998));
#302615=CARTESIAN_POINT('Ctrl Pts',(-1.45826813800006,2.2,3.76437651499998));
#302616=CARTESIAN_POINT('Ctrl Pts',(-1.45810333700006,12.2,3.76365206099998));
#302617=CARTESIAN_POINT('Ctrl Pts',(-1.45810333700006,5.2,3.76365206099998));
#302618=CARTESIAN_POINT('Ctrl Pts',(-1.45810333700006,2.2,3.76365206099998));
#302619=CARTESIAN_POINT('Ctrl Pts',(-1.45793894500006,12.2,3.76293360499999));
#302620=CARTESIAN_POINT('Ctrl Pts',(-1.45793894500006,5.2,3.76293360499999));
#302621=CARTESIAN_POINT('Ctrl Pts',(-1.45793894500006,2.2,3.76293360499999));
#302622=CARTESIAN_POINT('Ctrl Pts',(-1.45777497700006,12.2,3.76222115699999));
#302623=CARTESIAN_POINT('Ctrl Pts',(-1.45777497700006,5.2,3.76222115699999));
#302624=CARTESIAN_POINT('Ctrl Pts',(-1.45777497700006,2.2,3.76222115699999));
#302625=CARTESIAN_POINT('Ctrl Pts',(-1.45761145000006,12.2,3.76151472299998));
#302626=CARTESIAN_POINT('Ctrl Pts',(-1.45761145000006,5.2,3.76151472299998));
#302627=CARTESIAN_POINT('Ctrl Pts',(-1.45761145000006,2.2,3.76151472299998));
#302628=CARTESIAN_POINT('Ctrl Pts',(-1.45744838100006,12.2,3.76081431299998));
#302629=CARTESIAN_POINT('Ctrl Pts',(-1.45744838100006,5.2,3.76081431299998));
#302630=CARTESIAN_POINT('Ctrl Pts',(-1.45744838100006,2.2,3.76081431299998));
#302631=CARTESIAN_POINT('Ctrl Pts',(-1.45728578700006,12.2,3.76011993699999));
#302632=CARTESIAN_POINT('Ctrl Pts',(-1.45728578700006,5.2,3.76011993699999));
#302633=CARTESIAN_POINT('Ctrl Pts',(-1.45728578700006,2.2,3.76011993699999));
#302634=CARTESIAN_POINT('Ctrl Pts',(-1.45712368400006,12.2,3.75943159999998));
#302635=CARTESIAN_POINT('Ctrl Pts',(-1.45712368400006,5.2,3.75943159999998));
#302636=CARTESIAN_POINT('Ctrl Pts',(-1.45712368400006,2.2,3.75943159999998));
#302637=CARTESIAN_POINT('Ctrl Pts',(-1.45696209200006,12.2,3.75874931399999));
#302638=CARTESIAN_POINT('Ctrl Pts',(-1.45696209200006,5.2,3.75874931399999));
#302639=CARTESIAN_POINT('Ctrl Pts',(-1.45696209200006,2.2,3.75874931399999));
#302640=CARTESIAN_POINT('Ctrl Pts',(-1.45680102500006,12.2,3.75807308599998));
#302641=CARTESIAN_POINT('Ctrl Pts',(-1.45680102500006,5.2,3.75807308599998));
#302642=CARTESIAN_POINT('Ctrl Pts',(-1.45680102500006,2.2,3.75807308599998));
#302643=CARTESIAN_POINT('Ctrl Pts',(-1.45664050200006,12.2,3.75740292399998));
#302644=CARTESIAN_POINT('Ctrl Pts',(-1.45664050200006,5.2,3.75740292399998));
#302645=CARTESIAN_POINT('Ctrl Pts',(-1.45664050200006,2.2,3.75740292399998));
#302646=CARTESIAN_POINT('Ctrl Pts',(-1.45648053900006,12.2,3.75673883699999));
#302647=CARTESIAN_POINT('Ctrl Pts',(-1.45648053900006,5.2,3.75673883699999));
#302648=CARTESIAN_POINT('Ctrl Pts',(-1.45648053900006,2.2,3.75673883699999));
#302649=CARTESIAN_POINT('Ctrl Pts',(-1.45632115500006,12.2,3.75608083599998));
#302650=CARTESIAN_POINT('Ctrl Pts',(-1.45632115500006,5.2,3.75608083599998));
#302651=CARTESIAN_POINT('Ctrl Pts',(-1.45632115500006,2.2,3.75608083599998));
#302652=CARTESIAN_POINT('Ctrl Pts',(-1.45616236600006,12.2,3.75542892599999));
#302653=CARTESIAN_POINT('Ctrl Pts',(-1.45616236600006,5.2,3.75542892599999));
#302654=CARTESIAN_POINT('Ctrl Pts',(-1.45616236600006,2.2,3.75542892599999));
#302655=CARTESIAN_POINT('Ctrl Pts',(-1.45600419000006,12.2,3.75478311699998));
#302656=CARTESIAN_POINT('Ctrl Pts',(-1.45600419000006,5.2,3.75478311699998));
#302657=CARTESIAN_POINT('Ctrl Pts',(-1.45600419000006,2.2,3.75478311699998));
#302658=CARTESIAN_POINT('Ctrl Pts',(-1.45584664500006,12.2,3.75414341799999));
#302659=CARTESIAN_POINT('Ctrl Pts',(-1.45584664500006,5.2,3.75414341799999));
#302660=CARTESIAN_POINT('Ctrl Pts',(-1.45584664500006,2.2,3.75414341799999));
#302661=CARTESIAN_POINT('Ctrl Pts',(-1.45568974700006,12.2,3.75350983799999));
#302662=CARTESIAN_POINT('Ctrl Pts',(-1.45568974700006,5.2,3.75350983799999));
#302663=CARTESIAN_POINT('Ctrl Pts',(-1.45568974700006,2.2,3.75350983799999));
#302664=CARTESIAN_POINT('Ctrl Pts',(-1.45553351600006,12.2,3.75288238399998));
#302665=CARTESIAN_POINT('Ctrl Pts',(-1.45553351600006,5.2,3.75288238399998));
#302666=CARTESIAN_POINT('Ctrl Pts',(-1.45553351600006,2.2,3.75288238399998));
#302667=CARTESIAN_POINT('Ctrl Pts',(-1.45537796700006,12.2,3.75226106499999));
#302668=CARTESIAN_POINT('Ctrl Pts',(-1.45537796700006,5.2,3.75226106499999));
#302669=CARTESIAN_POINT('Ctrl Pts',(-1.45537796700006,2.2,3.75226106499999));
#302670=CARTESIAN_POINT('Ctrl Pts',(-1.45522312000006,12.2,3.75164589099998));
#302671=CARTESIAN_POINT('Ctrl Pts',(-1.45522312000006,5.2,3.75164589099998));
#302672=CARTESIAN_POINT('Ctrl Pts',(-1.45522312000006,2.2,3.75164589099998));
#302673=CARTESIAN_POINT('Ctrl Pts',(-1.45506899100006,12.2,3.75103686899998));
#302674=CARTESIAN_POINT('Ctrl Pts',(-1.45506899100006,5.2,3.75103686899998));
#302675=CARTESIAN_POINT('Ctrl Pts',(-1.45506899100006,2.2,3.75103686899998));
#302676=CARTESIAN_POINT('Ctrl Pts',(-1.45491559900006,12.2,3.75043400999999));
#302677=CARTESIAN_POINT('Ctrl Pts',(-1.45491559900006,5.2,3.75043400999999));
#302678=CARTESIAN_POINT('Ctrl Pts',(-1.45491559900006,2.2,3.75043400999999));
#302679=CARTESIAN_POINT('Ctrl Pts',(-1.45476296300005,12.2,3.74983731899999));
#302680=CARTESIAN_POINT('Ctrl Pts',(-1.45476296300005,5.2,3.74983731899999));
#302681=CARTESIAN_POINT('Ctrl Pts',(-1.45476296300005,2.2,3.74983731899999));
#302682=CARTESIAN_POINT('Ctrl Pts',(-1.45461109900006,12.2,3.74924680899999));
#302683=CARTESIAN_POINT('Ctrl Pts',(-1.45461109900006,5.2,3.74924680899999));
#302684=CARTESIAN_POINT('Ctrl Pts',(-1.45461109900006,2.2,3.74924680899999));
#302685=CARTESIAN_POINT('Ctrl Pts',(-1.45446002600006,12.2,3.74866248399999));
#302686=CARTESIAN_POINT('Ctrl Pts',(-1.45446002600006,5.2,3.74866248399999));
#302687=CARTESIAN_POINT('Ctrl Pts',(-1.45446002600006,2.2,3.74866248399999));
#302688=CARTESIAN_POINT('Ctrl Pts',(-1.45430976300006,12.2,3.74808435499999));
#302689=CARTESIAN_POINT('Ctrl Pts',(-1.45430976300006,5.2,3.74808435499999));
#302690=CARTESIAN_POINT('Ctrl Pts',(-1.45430976300006,2.2,3.74808435499999));
#302691=CARTESIAN_POINT('Ctrl Pts',(-1.45416032600005,12.2,3.74751243199999));
#302692=CARTESIAN_POINT('Ctrl Pts',(-1.45416032600005,5.2,3.74751243199999));
#302693=CARTESIAN_POINT('Ctrl Pts',(-1.45416032600005,2.2,3.74751243199999));
#302694=CARTESIAN_POINT('Ctrl Pts',(-1.45401173500006,12.2,3.74694672099999));
#302695=CARTESIAN_POINT('Ctrl Pts',(-1.45401173500006,5.2,3.74694672099999));
#302696=CARTESIAN_POINT('Ctrl Pts',(-1.45401173500006,2.2,3.74694672099999));
#302697=CARTESIAN_POINT('Ctrl Pts',(-1.45386400800006,12.2,3.74638723199999));
#302698=CARTESIAN_POINT('Ctrl Pts',(-1.45386400800006,5.2,3.74638723199999));
#302699=CARTESIAN_POINT('Ctrl Pts',(-1.45386400800006,2.2,3.74638723199999));
#302700=CARTESIAN_POINT('Ctrl Pts',(-1.45371716300006,12.2,3.74583397399999));
#302701=CARTESIAN_POINT('Ctrl Pts',(-1.45371716300006,5.2,3.74583397399999));
#302702=CARTESIAN_POINT('Ctrl Pts',(-1.45371716300006,2.2,3.74583397399999));
#302703=CARTESIAN_POINT('Ctrl Pts',(-1.45357121900005,12.2,3.74528695499999));
#302704=CARTESIAN_POINT('Ctrl Pts',(-1.45357121900005,5.2,3.74528695499999));
#302705=CARTESIAN_POINT('Ctrl Pts',(-1.45357121900005,2.2,3.74528695499999));
#302706=CARTESIAN_POINT('Ctrl Pts',(-1.45342619400005,12.2,3.74474618299999));
#302707=CARTESIAN_POINT('Ctrl Pts',(-1.45342619400005,5.2,3.74474618299999));
#302708=CARTESIAN_POINT('Ctrl Pts',(-1.45342619400005,2.2,3.74474618299999));
#302709=CARTESIAN_POINT('Ctrl Pts',(-1.45328210800006,12.2,3.74421166899998));
#302710=CARTESIAN_POINT('Ctrl Pts',(-1.45328210800006,5.2,3.74421166899998));
#302711=CARTESIAN_POINT('Ctrl Pts',(-1.45328210800006,2.2,3.74421166899998));
#302712=CARTESIAN_POINT('Ctrl Pts',(-1.45313897700006,12.2,3.74368341899999));
#302713=CARTESIAN_POINT('Ctrl Pts',(-1.45313897700006,5.2,3.74368341899999));
#302714=CARTESIAN_POINT('Ctrl Pts',(-1.45313897700006,2.2,3.74368341899999));
#302715=CARTESIAN_POINT('Ctrl Pts',(-1.45299682300006,12.2,3.74316144299998));
#302716=CARTESIAN_POINT('Ctrl Pts',(-1.45299682300006,5.2,3.74316144299998));
#302717=CARTESIAN_POINT('Ctrl Pts',(-1.45299682300006,2.2,3.74316144299998));
#302718=CARTESIAN_POINT('Ctrl Pts',(-1.45285566200006,12.2,3.74264574899998));
#302719=CARTESIAN_POINT('Ctrl Pts',(-1.45285566200006,5.2,3.74264574899998));
#302720=CARTESIAN_POINT('Ctrl Pts',(-1.45285566200006,2.2,3.74264574899998));
#302721=CARTESIAN_POINT('Ctrl Pts',(-1.45271551400006,12.2,3.74213634699998));
#302722=CARTESIAN_POINT('Ctrl Pts',(-1.45271551400006,5.2,3.74213634699998));
#302723=CARTESIAN_POINT('Ctrl Pts',(-1.45271551400006,2.2,3.74213634699998));
#302724=CARTESIAN_POINT('Ctrl Pts',(-1.45257639800006,12.2,3.74163324399999));
#302725=CARTESIAN_POINT('Ctrl Pts',(-1.45257639800006,5.2,3.74163324399999));
#302726=CARTESIAN_POINT('Ctrl Pts',(-1.45257639800006,2.2,3.74163324399999));
#302727=CARTESIAN_POINT('Ctrl Pts',(-1.45243833400006,12.2,3.74113645099998));
#302728=CARTESIAN_POINT('Ctrl Pts',(-1.45243833400006,5.2,3.74113645099998));
#302729=CARTESIAN_POINT('Ctrl Pts',(-1.45243833400006,2.2,3.74113645099998));
#302730=CARTESIAN_POINT('Ctrl Pts',(-1.45230133900006,12.2,3.74064597399999));
#302731=CARTESIAN_POINT('Ctrl Pts',(-1.45230133900006,5.2,3.74064597399999));
#302732=CARTESIAN_POINT('Ctrl Pts',(-1.45230133900006,2.2,3.74064597399999));
#302733=CARTESIAN_POINT('Ctrl Pts',(-1.45216543300006,12.2,3.74016182299999));
#302734=CARTESIAN_POINT('Ctrl Pts',(-1.45216543300006,5.2,3.74016182299999));
#302735=CARTESIAN_POINT('Ctrl Pts',(-1.45216543300006,2.2,3.74016182299999));
#302736=CARTESIAN_POINT('Ctrl Pts',(-1.45203063700006,12.2,3.73968400799999));
#302737=CARTESIAN_POINT('Ctrl Pts',(-1.45203063700006,5.2,3.73968400799999));
#302738=CARTESIAN_POINT('Ctrl Pts',(-1.45203063700006,2.2,3.73968400799999));
#302739=CARTESIAN_POINT('Ctrl Pts',(-1.45189696700006,12.2,3.73921253499999));
#302740=CARTESIAN_POINT('Ctrl Pts',(-1.45189696700006,5.2,3.73921253499999));
#302741=CARTESIAN_POINT('Ctrl Pts',(-1.45189696700006,2.2,3.73921253499999));
#302742=CARTESIAN_POINT('Ctrl Pts',(-1.45176444400006,12.2,3.73874741399998));
#302743=CARTESIAN_POINT('Ctrl Pts',(-1.45176444400006,5.2,3.73874741399998));
#302744=CARTESIAN_POINT('Ctrl Pts',(-1.45176444400006,2.2,3.73874741399998));
#302745=CARTESIAN_POINT('Ctrl Pts',(-1.45163308900006,12.2,3.73828865499998));
#302746=CARTESIAN_POINT('Ctrl Pts',(-1.45163308900006,5.2,3.73828865499998));
#302747=CARTESIAN_POINT('Ctrl Pts',(-1.45163308900006,2.2,3.73828865499998));
#302748=CARTESIAN_POINT('Ctrl Pts',(-1.45150291900006,12.2,3.73783626399998));
#302749=CARTESIAN_POINT('Ctrl Pts',(-1.45150291900006,5.2,3.73783626399998));
#302750=CARTESIAN_POINT('Ctrl Pts',(-1.45150291900006,2.2,3.73783626399998));
#302751=CARTESIAN_POINT('Ctrl Pts',(-1.45137395500006,12.2,3.73739025199999));
#302752=CARTESIAN_POINT('Ctrl Pts',(-1.45137395500006,5.2,3.73739025199999));
#302753=CARTESIAN_POINT('Ctrl Pts',(-1.45137395500006,2.2,3.73739025199999));
#302754=CARTESIAN_POINT('Ctrl Pts',(-1.45124621600006,12.2,3.73695062699999));
#302755=CARTESIAN_POINT('Ctrl Pts',(-1.45124621600006,5.2,3.73695062699999));
#302756=CARTESIAN_POINT('Ctrl Pts',(-1.45124621600006,2.2,3.73695062699999));
#302757=CARTESIAN_POINT('Ctrl Pts',(-1.45111972300006,12.2,3.73651739899999));
#302758=CARTESIAN_POINT('Ctrl Pts',(-1.45111972300006,5.2,3.73651739899999));
#302759=CARTESIAN_POINT('Ctrl Pts',(-1.45111972300006,2.2,3.73651739899999));
#302760=CARTESIAN_POINT('Ctrl Pts',(-1.45099449400006,12.2,3.73609057399998));
#302761=CARTESIAN_POINT('Ctrl Pts',(-1.45099449400006,5.2,3.73609057399998));
#302762=CARTESIAN_POINT('Ctrl Pts',(-1.45099449400006,2.2,3.73609057399998));
#302763=CARTESIAN_POINT('Ctrl Pts',(-1.45087055000006,12.2,3.73567016199999));
#302764=CARTESIAN_POINT('Ctrl Pts',(-1.45087055000006,5.2,3.73567016199999));
#302765=CARTESIAN_POINT('Ctrl Pts',(-1.45087055000006,2.2,3.73567016199999));
#302766=CARTESIAN_POINT('Ctrl Pts',(-1.45074791000006,12.2,3.73525617299999));
#302767=CARTESIAN_POINT('Ctrl Pts',(-1.45074791000006,5.2,3.73525617299999));
#302768=CARTESIAN_POINT('Ctrl Pts',(-1.45074791000006,2.2,3.73525617299999));
#302769=CARTESIAN_POINT('Ctrl Pts',(-1.45062659500006,12.2,3.73484861399999));
#302770=CARTESIAN_POINT('Ctrl Pts',(-1.45062659500006,5.2,3.73484861399999));
#302771=CARTESIAN_POINT('Ctrl Pts',(-1.45062659500006,2.2,3.73484861399999));
#302772=CARTESIAN_POINT('Ctrl Pts',(-1.45050662500006,12.2,3.73444749499999));
#302773=CARTESIAN_POINT('Ctrl Pts',(-1.45050662500006,5.2,3.73444749499999));
#302774=CARTESIAN_POINT('Ctrl Pts',(-1.45050662500006,2.2,3.73444749499999));
#302775=CARTESIAN_POINT('Ctrl Pts',(-1.45038802000006,12.2,3.73405282499998));
#302776=CARTESIAN_POINT('Ctrl Pts',(-1.45038802000006,5.2,3.73405282499998));
#302777=CARTESIAN_POINT('Ctrl Pts',(-1.45038802000006,2.2,3.73405282499998));
#302778=CARTESIAN_POINT('Ctrl Pts',(-1.45027080000006,12.2,3.73366461099998));
#302779=CARTESIAN_POINT('Ctrl Pts',(-1.45027080000006,5.2,3.73366461099998));
#302780=CARTESIAN_POINT('Ctrl Pts',(-1.45027080000006,2.2,3.73366461099998));
#302781=CARTESIAN_POINT('Ctrl Pts',(-1.45015498500006,12.2,3.73328286299999));
#302782=CARTESIAN_POINT('Ctrl Pts',(-1.45015498500006,5.2,3.73328286299999));
#302783=CARTESIAN_POINT('Ctrl Pts',(-1.45015498500006,2.2,3.73328286299999));
#302784=CARTESIAN_POINT('Ctrl Pts',(-1.45004059600006,12.2,3.73290758999998));
#302785=CARTESIAN_POINT('Ctrl Pts',(-1.45004059600006,5.2,3.73290758999998));
#302786=CARTESIAN_POINT('Ctrl Pts',(-1.45004059600006,2.2,3.73290758999998));
#302787=CARTESIAN_POINT('Ctrl Pts',(-1.44992765300006,12.2,3.73253880099998));
#302788=CARTESIAN_POINT('Ctrl Pts',(-1.44992765300006,5.2,3.73253880099998));
#302789=CARTESIAN_POINT('Ctrl Pts',(-1.44992765300006,2.2,3.73253880099998));
#302790=CARTESIAN_POINT('Ctrl Pts',(-1.44981617800006,12.2,3.73217650299999));
#302791=CARTESIAN_POINT('Ctrl Pts',(-1.44981617800006,5.2,3.73217650299999));
#302792=CARTESIAN_POINT('Ctrl Pts',(-1.44981617800006,2.2,3.73217650299999));
#302793=CARTESIAN_POINT('Ctrl Pts',(-1.44970619000006,12.2,3.73182070599999));
#302794=CARTESIAN_POINT('Ctrl Pts',(-1.44970619000006,5.2,3.73182070599999));
#302795=CARTESIAN_POINT('Ctrl Pts',(-1.44970619000006,2.2,3.73182070599999));
#302796=CARTESIAN_POINT('Ctrl Pts',(-1.44959771000006,12.2,3.73147141999999));
#302797=CARTESIAN_POINT('Ctrl Pts',(-1.44959771000006,5.2,3.73147141999999));
#302798=CARTESIAN_POINT('Ctrl Pts',(-1.44959771000006,2.2,3.73147141999999));
#302799=CARTESIAN_POINT('Ctrl Pts',(-1.44949075900006,12.2,3.73112865199998));
#302800=CARTESIAN_POINT('Ctrl Pts',(-1.44949075900006,5.2,3.73112865199998));
#302801=CARTESIAN_POINT('Ctrl Pts',(-1.44949075900006,2.2,3.73112865199998));
#302802=CARTESIAN_POINT('Ctrl Pts',(-1.44938535800006,12.2,3.73079241199999));
#302803=CARTESIAN_POINT('Ctrl Pts',(-1.44938535800006,5.2,3.73079241199999));
#302804=CARTESIAN_POINT('Ctrl Pts',(-1.44938535800006,2.2,3.73079241199999));
#302805=CARTESIAN_POINT('Ctrl Pts',(-1.44928152800005,12.2,3.73046270799998));
#302806=CARTESIAN_POINT('Ctrl Pts',(-1.44928152800005,5.2,3.73046270799998));
#302807=CARTESIAN_POINT('Ctrl Pts',(-1.44928152800005,2.2,3.73046270799998));
#302808=CARTESIAN_POINT('Ctrl Pts',(-1.44917928900006,12.2,3.73013954999998));
#302809=CARTESIAN_POINT('Ctrl Pts',(-1.44917928900006,5.2,3.73013954999998));
#302810=CARTESIAN_POINT('Ctrl Pts',(-1.44917928900006,2.2,3.73013954999998));
#302811=CARTESIAN_POINT('Ctrl Pts',(-1.44907866400006,12.2,3.72982294399999));
#302812=CARTESIAN_POINT('Ctrl Pts',(-1.44907866400006,5.2,3.72982294399999));
#302813=CARTESIAN_POINT('Ctrl Pts',(-1.44907866400006,2.2,3.72982294399999));
#302814=CARTESIAN_POINT('Ctrl Pts',(-1.44897967300005,12.2,3.72951290199998));
#302815=CARTESIAN_POINT('Ctrl Pts',(-1.44897967300005,5.2,3.72951290199998));
#302816=CARTESIAN_POINT('Ctrl Pts',(-1.44897967300005,2.2,3.72951290199998));
#302817=CARTESIAN_POINT('Ctrl Pts',(-1.44888233700006,12.2,3.72920943199999));
#302818=CARTESIAN_POINT('Ctrl Pts',(-1.44888233700006,5.2,3.72920943199999));
#302819=CARTESIAN_POINT('Ctrl Pts',(-1.44888233700006,2.2,3.72920943199999));
#302820=CARTESIAN_POINT('Ctrl Pts',(-1.44878667900006,12.2,3.72891254199998));
#302821=CARTESIAN_POINT('Ctrl Pts',(-1.44878667900006,5.2,3.72891254199998));
#302822=CARTESIAN_POINT('Ctrl Pts',(-1.44878667900006,2.2,3.72891254199998));
#302823=CARTESIAN_POINT('Ctrl Pts',(-1.44869271700006,12.2,3.72862224099999));
#302824=CARTESIAN_POINT('Ctrl Pts',(-1.44869271700006,5.2,3.72862224099999));
#302825=CARTESIAN_POINT('Ctrl Pts',(-1.44869271700006,2.2,3.72862224099999));
#302826=CARTESIAN_POINT('Ctrl Pts',(-1.44860047700006,12.2,3.72833853899999));
#302827=CARTESIAN_POINT('Ctrl Pts',(-1.44860047700006,5.2,3.72833853899999));
#302828=CARTESIAN_POINT('Ctrl Pts',(-1.44860047700006,2.2,3.72833853899999));
#302829=CARTESIAN_POINT('Ctrl Pts',(-1.44850997700006,12.2,3.72806144399998));
#302830=CARTESIAN_POINT('Ctrl Pts',(-1.44850997700006,5.2,3.72806144399998));
#302831=CARTESIAN_POINT('Ctrl Pts',(-1.44850997700006,2.2,3.72806144399998));
#302832=CARTESIAN_POINT('Ctrl Pts',(-1.44842123900006,12.2,3.72779096499999));
#302833=CARTESIAN_POINT('Ctrl Pts',(-1.44842123900006,5.2,3.72779096499999));
#302834=CARTESIAN_POINT('Ctrl Pts',(-1.44842123900006,2.2,3.72779096499999));
#302835=CARTESIAN_POINT('Ctrl Pts',(-1.44833428800006,12.2,3.72752711099999));
#302836=CARTESIAN_POINT('Ctrl Pts',(-1.44833428800006,5.2,3.72752711099999));
#302837=CARTESIAN_POINT('Ctrl Pts',(-1.44833428800006,2.2,3.72752711099999));
#302838=CARTESIAN_POINT('Ctrl Pts',(-1.44824914200006,12.2,3.72726989099998));
#302839=CARTESIAN_POINT('Ctrl Pts',(-1.44824914200006,5.2,3.72726989099998));
#302840=CARTESIAN_POINT('Ctrl Pts',(-1.44824914200006,2.2,3.72726989099998));
#302841=CARTESIAN_POINT('Ctrl Pts',(-1.44816582500006,12.2,3.72701931299999));
#302842=CARTESIAN_POINT('Ctrl Pts',(-1.44816582500006,5.2,3.72701931299999));
#302843=CARTESIAN_POINT('Ctrl Pts',(-1.44816582500006,2.2,3.72701931299999));
#302844=CARTESIAN_POINT('Ctrl Pts',(-1.44808435900006,12.2,3.72677538699998));
#302845=CARTESIAN_POINT('Ctrl Pts',(-1.44808435900006,5.2,3.72677538699998));
#302846=CARTESIAN_POINT('Ctrl Pts',(-1.44808435900006,2.2,3.72677538699998));
#302847=CARTESIAN_POINT('Ctrl Pts',(-1.44800476500005,12.2,3.72653812199999));
#302848=CARTESIAN_POINT('Ctrl Pts',(-1.44800476500005,5.2,3.72653812199999));
#302849=CARTESIAN_POINT('Ctrl Pts',(-1.44800476500005,2.2,3.72653812199999));
#302850=CARTESIAN_POINT('Ctrl Pts',(-1.44792706600006,12.2,3.72630752599999));
#302851=CARTESIAN_POINT('Ctrl Pts',(-1.44792706600006,5.2,3.72630752599999));
#302852=CARTESIAN_POINT('Ctrl Pts',(-1.44792706600006,2.2,3.72630752599999));
#302853=CARTESIAN_POINT('Ctrl Pts',(-1.44785128400006,12.2,3.72608360799998));
#302854=CARTESIAN_POINT('Ctrl Pts',(-1.44785128400006,5.2,3.72608360799998));
#302855=CARTESIAN_POINT('Ctrl Pts',(-1.44785128400006,2.2,3.72608360799998));
#302856=CARTESIAN_POINT('Ctrl Pts',(-1.44777744200006,12.2,3.72586637799999));
#302857=CARTESIAN_POINT('Ctrl Pts',(-1.44777744200006,5.2,3.72586637799999));
#302858=CARTESIAN_POINT('Ctrl Pts',(-1.44777744200006,2.2,3.72586637799999));
#302859=CARTESIAN_POINT('Ctrl Pts',(-1.44770556100006,12.2,3.72565584299998));
#302860=CARTESIAN_POINT('Ctrl Pts',(-1.44770556100006,5.2,3.72565584299998));
#302861=CARTESIAN_POINT('Ctrl Pts',(-1.44770556100006,2.2,3.72565584299998));
#302862=CARTESIAN_POINT('Ctrl Pts',(-1.44763566500006,12.2,3.72545201299998));
#302863=CARTESIAN_POINT('Ctrl Pts',(-1.44763566500006,5.2,3.72545201299998));
#302864=CARTESIAN_POINT('Ctrl Pts',(-1.44763566500006,2.2,3.72545201299998));
#302865=CARTESIAN_POINT('Ctrl Pts',(-1.44756777600006,12.2,3.72525489799998));
#302866=CARTESIAN_POINT('Ctrl Pts',(-1.44756777600006,5.2,3.72525489799998));
#302867=CARTESIAN_POINT('Ctrl Pts',(-1.44756777600006,2.2,3.72525489799998));
#302868=CARTESIAN_POINT('Ctrl Pts',(-1.44750191600005,12.2,3.72506450599998));
#302869=CARTESIAN_POINT('Ctrl Pts',(-1.44750191600005,5.2,3.72506450599998));
#302870=CARTESIAN_POINT('Ctrl Pts',(-1.44750191600005,2.2,3.72506450599998));
#302871=CARTESIAN_POINT('Ctrl Pts',(-1.44743811100006,12.2,3.72488084599999));
#302872=CARTESIAN_POINT('Ctrl Pts',(-1.44743811100006,5.2,3.72488084599999));
#302873=CARTESIAN_POINT('Ctrl Pts',(-1.44743811100006,2.2,3.72488084599999));
#302874=CARTESIAN_POINT('Ctrl Pts',(-1.44737638100006,12.2,3.72470392699999));
#302875=CARTESIAN_POINT('Ctrl Pts',(-1.44737638100006,5.2,3.72470392699999));
#302876=CARTESIAN_POINT('Ctrl Pts',(-1.44737638100006,2.2,3.72470392699999));
#302877=CARTESIAN_POINT('Ctrl Pts',(-1.44731675000005,12.2,3.72453375899998));
#302878=CARTESIAN_POINT('Ctrl Pts',(-1.44731675000005,5.2,3.72453375899998));
#302879=CARTESIAN_POINT('Ctrl Pts',(-1.44731675000005,2.2,3.72453375899998));
#302880=CARTESIAN_POINT('Ctrl Pts',(-1.44725923900006,12.2,3.72437034899999));
#302881=CARTESIAN_POINT('Ctrl Pts',(-1.44725923900006,5.2,3.72437034899999));
#302882=CARTESIAN_POINT('Ctrl Pts',(-1.44725923900006,2.2,3.72437034899999));
#302883=CARTESIAN_POINT('Ctrl Pts',(-1.44720387400006,12.2,3.72421370599999));
#302884=CARTESIAN_POINT('Ctrl Pts',(-1.44720387400006,5.2,3.72421370599999));
#302885=CARTESIAN_POINT('Ctrl Pts',(-1.44720387400006,2.2,3.72421370599999));
#302886=CARTESIAN_POINT('Ctrl Pts',(-1.44715067400006,12.2,3.72406384099998));
#302887=CARTESIAN_POINT('Ctrl Pts',(-1.44715067400006,5.2,3.72406384099998));
#302888=CARTESIAN_POINT('Ctrl Pts',(-1.44715067400006,2.2,3.72406384099998));
#302889=CARTESIAN_POINT('Ctrl Pts',(-1.44709966700006,12.2,3.72392076099998));
#302890=CARTESIAN_POINT('Ctrl Pts',(-1.44709966700006,5.2,3.72392076099998));
#302891=CARTESIAN_POINT('Ctrl Pts',(-1.44709966700006,2.2,3.72392076099998));
#302892=CARTESIAN_POINT('Ctrl Pts',(-1.44705087400006,12.2,3.72378447599999));
#302893=CARTESIAN_POINT('Ctrl Pts',(-1.44705087400006,5.2,3.72378447599999));
#302894=CARTESIAN_POINT('Ctrl Pts',(-1.44705087400006,2.2,3.72378447599999));
#302895=CARTESIAN_POINT('Ctrl Pts',(-1.44700432100006,12.2,3.72365499499999));
#302896=CARTESIAN_POINT('Ctrl Pts',(-1.44700432100006,5.2,3.72365499499999));
#302897=CARTESIAN_POINT('Ctrl Pts',(-1.44700432100006,2.2,3.72365499499999));
#302898=CARTESIAN_POINT('Ctrl Pts',(-1.44696003400006,12.2,3.72353232799998));
#302899=CARTESIAN_POINT('Ctrl Pts',(-1.44696003400006,5.2,3.72353232799998));
#302900=CARTESIAN_POINT('Ctrl Pts',(-1.44696003400006,2.2,3.72353232799998));
#302901=CARTESIAN_POINT('Ctrl Pts',(-1.44691803400006,12.2,3.72341648399999));
#302902=CARTESIAN_POINT('Ctrl Pts',(-1.44691803400006,5.2,3.72341648399999));
#302903=CARTESIAN_POINT('Ctrl Pts',(-1.44691803400006,2.2,3.72341648399999));
#302904=CARTESIAN_POINT('Ctrl Pts',(-1.44687834300006,12.2,3.72330747199998));
#302905=CARTESIAN_POINT('Ctrl Pts',(-1.44687834300006,5.2,3.72330747199998));
#302906=CARTESIAN_POINT('Ctrl Pts',(-1.44687834300006,2.2,3.72330747199998));
#302907=CARTESIAN_POINT('Ctrl Pts',(-1.44684098300006,12.2,3.72320529699999));
#302908=CARTESIAN_POINT('Ctrl Pts',(-1.44684098300006,5.2,3.72320529699999));
#302909=CARTESIAN_POINT('Ctrl Pts',(-1.44684098300006,2.2,3.72320529699999));
#302910=CARTESIAN_POINT('Ctrl Pts',(-1.44680597500006,12.2,3.72310996999998));
#302911=CARTESIAN_POINT('Ctrl Pts',(-1.44680597500006,5.2,3.72310996999998));
#302912=CARTESIAN_POINT('Ctrl Pts',(-1.44680597500006,2.2,3.72310996999998));
#302913=CARTESIAN_POINT('Ctrl Pts',(-1.44677334500006,12.2,3.72302149899999));
#302914=CARTESIAN_POINT('Ctrl Pts',(-1.44677334500006,5.2,3.72302149899999));
#302915=CARTESIAN_POINT('Ctrl Pts',(-1.44677334500006,2.2,3.72302149899999));
#302916=CARTESIAN_POINT('Ctrl Pts',(-1.44674311900006,12.2,3.72293989599999));
#302917=CARTESIAN_POINT('Ctrl Pts',(-1.44674311900006,5.2,3.72293989599999));
#302918=CARTESIAN_POINT('Ctrl Pts',(-1.44674311900006,2.2,3.72293989599999));
#302919=CARTESIAN_POINT('Ctrl Pts',(-1.44671532800006,12.2,3.72286516999999));
#302920=CARTESIAN_POINT('Ctrl Pts',(-1.44671532800006,5.2,3.72286516999999));
#302921=CARTESIAN_POINT('Ctrl Pts',(-1.44671532800006,2.2,3.72286516999999));
#302922=CARTESIAN_POINT('Ctrl Pts',(-1.44669000500006,12.2,3.72279733399999));
#302923=CARTESIAN_POINT('Ctrl Pts',(-1.44669000500006,5.2,3.72279733399999));
#302924=CARTESIAN_POINT('Ctrl Pts',(-1.44669000500006,2.2,3.72279733399999));
#302925=CARTESIAN_POINT('Ctrl Pts',(-1.44666717300006,12.2,3.72273639799998));
#302926=CARTESIAN_POINT('Ctrl Pts',(-1.44666717300006,5.2,3.72273639799998));
#302927=CARTESIAN_POINT('Ctrl Pts',(-1.44666717300006,2.2,3.72273639799998));
#302928=CARTESIAN_POINT('Ctrl Pts',(-1.44664685600006,12.2,3.72268236899998));
#302929=CARTESIAN_POINT('Ctrl Pts',(-1.44664685600006,5.2,3.72268236899998));
#302930=CARTESIAN_POINT('Ctrl Pts',(-1.44664685600006,2.2,3.72268236899998));
#302931=CARTESIAN_POINT('Ctrl Pts',(-1.44662715937635,12.2,3.72263020704428));
#302932=CARTESIAN_POINT('Ctrl Pts',(-1.44662715937635,5.2,3.72263020704428));
#302933=CARTESIAN_POINT('Ctrl Pts',(-1.44662715937635,2.2,3.72263020704428));
#302934=CARTESIAN_POINT('Ctrl Pts',(-1.44661362254973,12.2,3.72259457946533));
#302935=CARTESIAN_POINT('Ctrl Pts',(-1.44661362254973,5.2,3.72259457946533));
#302936=CARTESIAN_POINT('Ctrl Pts',(-1.44661362254973,2.2,3.72259457946533));
#302937=CARTESIAN_POINT('Ctrl Pts',(-1.44660465484929,12.2,3.72257112803267));
#302938=CARTESIAN_POINT('Ctrl Pts',(-1.44660465484929,5.2,3.72257112803267));
#302939=CARTESIAN_POINT('Ctrl Pts',(-1.44660465484929,2.2,3.72257112803267));
#302940=CARTESIAN_POINT('Ctrl Pts',(-1.44659903765901,12.2,3.7225565310091));
#302941=CARTESIAN_POINT('Ctrl Pts',(-1.44659903765901,5.2,3.7225565310091));
#302942=CARTESIAN_POINT('Ctrl Pts',(-1.44659903765901,2.2,3.7225565310091));
#302943=CARTESIAN_POINT('Ctrl Pts',(-1.44659557100006,12.2,3.72254751699998));
#302944=CARTESIAN_POINT('Ctrl Pts',(-1.44659557100006,5.2,3.72254751699998));
#302945=CARTESIAN_POINT('Ctrl Pts',(-1.44659557100006,2.2,3.72254751699998));
#302946=CARTESIAN_POINT('',(-1.44659576000006,2.7,3.72254744499998));
#302947=CARTESIAN_POINT('',(-1.44659576000006,12.2,3.72254744499998));
#302948=CARTESIAN_POINT('Ctrl Pts',(-1.39835267900006,2.7,4.53950545599999));
#302949=CARTESIAN_POINT('Ctrl Pts',(-1.46128293091346,2.7,4.3149625643711));
#302950=CARTESIAN_POINT('Ctrl Pts',(-1.48231430522207,2.7,4.12307648969267));
#302951=CARTESIAN_POINT('Ctrl Pts',(-1.47777222782857,2.7,3.81654919462578));
#302952=CARTESIAN_POINT('Ctrl Pts',(-1.4509749893252,2.7,3.73439048105048));
#302953=CARTESIAN_POINT('Ctrl Pts',(-1.44671500473292,2.7,3.72286373140579));
#302954=CARTESIAN_POINT('Ctrl Pts',(-1.44665623704781,2.7,3.72270526090141));
#302955=CARTESIAN_POINT('Ctrl Pts',(-1.44659557100006,2.7,3.72254751699998));
#302956=CARTESIAN_POINT('Origin',(-1.44657717200006,15.2,3.72249961199999));
#302957=CARTESIAN_POINT('',(-1.31303067400006,2.7,3.37884232399999));
#302958=CARTESIAN_POINT('',(-1.31303067400006,2.2,3.37884232399999));
#302959=CARTESIAN_POINT('',(-0.723288586352956,2.7,1.86124980586285));
#302960=CARTESIAN_POINT('Origin',(-5.66300478732629E-14,15.2,-1.77635683940025E-14));
#302961=CARTESIAN_POINT('',(-1.81888661200006,2.7,3.13564610499998));
#302962=CARTESIAN_POINT('',(-1.81888661200006,12.2,3.13564610499999));
#302963=CARTESIAN_POINT('Origin',(-5.66300478732629E-14,2.7,-1.92943768261394E-14));
#302964=CARTESIAN_POINT('Origin',(-5.66300478732629E-14,15.2,-1.77635683940025E-14));
#302965=CARTESIAN_POINT('',(-2.00390017000006,2.7,3.45459784199999));
#302966=CARTESIAN_POINT('',(-2.00390017000006,12.2,3.45459784199999));
#302967=CARTESIAN_POINT('',(-5.6975542132353E-14,2.7,-1.86987664562669E-14));
#302968=CARTESIAN_POINT('Ctrl Pts',(-2.00390028800005,12.2,3.45459777299999));
#302969=CARTESIAN_POINT('Ctrl Pts',(-2.00390028800005,5.2,3.45459777299999));
#302970=CARTESIAN_POINT('Ctrl Pts',(-2.00390028800005,2.2,3.45459777299999));
#302971=CARTESIAN_POINT('Ctrl Pts',(-2.00390374300006,12.2,3.45460367899998));
#302972=CARTESIAN_POINT('Ctrl Pts',(-2.00390374300006,5.2,3.45460367899998));
#302973=CARTESIAN_POINT('Ctrl Pts',(-2.00390374300006,2.2,3.45460367899998));
#302974=CARTESIAN_POINT('Ctrl Pts',(-2.00391042944521,12.2,3.45461510030709));
#302975=CARTESIAN_POINT('Ctrl Pts',(-2.00391042944521,5.2,3.45461510030709));
#302976=CARTESIAN_POINT('Ctrl Pts',(-2.00391042944521,2.2,3.45461510030709));
#302977=CARTESIAN_POINT('Ctrl Pts',(-2.00392033978938,12.2,3.4546320379243));
#302978=CARTESIAN_POINT('Ctrl Pts',(-2.00392033978938,5.2,3.4546320379243));
#302979=CARTESIAN_POINT('Ctrl Pts',(-2.00392033978938,2.2,3.4546320379243));
#302980=CARTESIAN_POINT('Ctrl Pts',(-2.00393346686492,12.2,3.45465453404064));
#302981=CARTESIAN_POINT('Ctrl Pts',(-2.00393346686492,5.2,3.45465453404064));
#302982=CARTESIAN_POINT('Ctrl Pts',(-2.00393346686492,2.2,3.45465453404064));
#302983=CARTESIAN_POINT('Ctrl Pts',(-2.00395653200005,12.2,3.45469348599998));
#302984=CARTESIAN_POINT('Ctrl Pts',(-2.00395653200005,5.2,3.45469348599998));
#302985=CARTESIAN_POINT('Ctrl Pts',(-2.00395653200005,2.2,3.45469348599998));
#302986=CARTESIAN_POINT('Ctrl Pts',(-2.00398222000006,12.2,3.45473680799999));
#302987=CARTESIAN_POINT('Ctrl Pts',(-2.00398222000006,5.2,3.45473680799999));
#302988=CARTESIAN_POINT('Ctrl Pts',(-2.00398222000006,2.2,3.45473680799999));
#302989=CARTESIAN_POINT('Ctrl Pts',(-2.00401172800006,12.2,3.45478641899999));
#302990=CARTESIAN_POINT('Ctrl Pts',(-2.00401172800006,5.2,3.45478641899999));
#302991=CARTESIAN_POINT('Ctrl Pts',(-2.00401172800006,2.2,3.45478641899999));
#302992=CARTESIAN_POINT('Ctrl Pts',(-2.00404506100006,12.2,3.45484230499999));
#302993=CARTESIAN_POINT('Ctrl Pts',(-2.00404506100006,5.2,3.45484230499999));
#302994=CARTESIAN_POINT('Ctrl Pts',(-2.00404506100006,2.2,3.45484230499999));
#302995=CARTESIAN_POINT('Ctrl Pts',(-2.00408222600006,12.2,3.45490444799999));
#302996=CARTESIAN_POINT('Ctrl Pts',(-2.00408222600006,5.2,3.45490444799999));
#302997=CARTESIAN_POINT('Ctrl Pts',(-2.00408222600006,2.2,3.45490444799999));
#302998=CARTESIAN_POINT('Ctrl Pts',(-2.00412323200006,12.2,3.45497281999998));
#302999=CARTESIAN_POINT('Ctrl Pts',(-2.00412323200006,5.2,3.45497281999998));
#303000=CARTESIAN_POINT('Ctrl Pts',(-2.00412323200006,2.2,3.45497281999998));
#303001=CARTESIAN_POINT('Ctrl Pts',(-2.00416808800005,12.2,3.45504738999999));
#303002=CARTESIAN_POINT('Ctrl Pts',(-2.00416808800005,5.2,3.45504738999999));
#303003=CARTESIAN_POINT('Ctrl Pts',(-2.00416808800005,2.2,3.45504738999999));
#303004=CARTESIAN_POINT('Ctrl Pts',(-2.00421680500006,12.2,3.45512812799999));
#303005=CARTESIAN_POINT('Ctrl Pts',(-2.00421680500006,5.2,3.45512812799999));
#303006=CARTESIAN_POINT('Ctrl Pts',(-2.00421680500006,2.2,3.45512812799999));
#303007=CARTESIAN_POINT('Ctrl Pts',(-2.00426939400006,12.2,3.45521500299999));
#303008=CARTESIAN_POINT('Ctrl Pts',(-2.00426939400006,5.2,3.45521500299999));
#303009=CARTESIAN_POINT('Ctrl Pts',(-2.00426939400006,2.2,3.45521500299999));
#303010=CARTESIAN_POINT('Ctrl Pts',(-2.00432586000006,12.2,3.45530799099999));
#303011=CARTESIAN_POINT('Ctrl Pts',(-2.00432586000006,5.2,3.45530799099999));
#303012=CARTESIAN_POINT('Ctrl Pts',(-2.00432586000006,2.2,3.45530799099999));
#303013=CARTESIAN_POINT('Ctrl Pts',(-2.00438621300006,12.2,3.45540706999999));
#303014=CARTESIAN_POINT('Ctrl Pts',(-2.00438621300006,5.2,3.45540706999999));
#303015=CARTESIAN_POINT('Ctrl Pts',(-2.00438621300006,2.2,3.45540706999999));
#303016=CARTESIAN_POINT('Ctrl Pts',(-2.00445045700006,12.2,3.45551221899999));
#303017=CARTESIAN_POINT('Ctrl Pts',(-2.00445045700006,5.2,3.45551221899999));
#303018=CARTESIAN_POINT('Ctrl Pts',(-2.00445045700006,2.2,3.45551221899999));
#303019=CARTESIAN_POINT('Ctrl Pts',(-2.00451860300006,12.2,3.45562341599998));
#303020=CARTESIAN_POINT('Ctrl Pts',(-2.00451860300006,5.2,3.45562341599998));
#303021=CARTESIAN_POINT('Ctrl Pts',(-2.00451860300006,2.2,3.45562341599998));
#303022=CARTESIAN_POINT('Ctrl Pts',(-2.00459065500006,12.2,3.45574063699999));
#303023=CARTESIAN_POINT('Ctrl Pts',(-2.00459065500006,5.2,3.45574063699999));
#303024=CARTESIAN_POINT('Ctrl Pts',(-2.00459065500006,2.2,3.45574063699999));
#303025=CARTESIAN_POINT('Ctrl Pts',(-2.00466662200005,12.2,3.45586385799999));
#303026=CARTESIAN_POINT('Ctrl Pts',(-2.00466662200005,5.2,3.45586385799999));
#303027=CARTESIAN_POINT('Ctrl Pts',(-2.00466662200005,2.2,3.45586385799999));
#303028=CARTESIAN_POINT('Ctrl Pts',(-2.00474651300006,12.2,3.45599305199999));
#303029=CARTESIAN_POINT('Ctrl Pts',(-2.00474651300006,5.2,3.45599305199999));
#303030=CARTESIAN_POINT('Ctrl Pts',(-2.00474651300006,2.2,3.45599305199999));
#303031=CARTESIAN_POINT('Ctrl Pts',(-2.00483033600006,12.2,3.45612819499999));
#303032=CARTESIAN_POINT('Ctrl Pts',(-2.00483033600006,5.2,3.45612819499999));
#303033=CARTESIAN_POINT('Ctrl Pts',(-2.00483033600006,2.2,3.45612819499999));
#303034=CARTESIAN_POINT('Ctrl Pts',(-2.00491809800006,12.2,3.45626926299998));
#303035=CARTESIAN_POINT('Ctrl Pts',(-2.00491809800006,5.2,3.45626926299998));
#303036=CARTESIAN_POINT('Ctrl Pts',(-2.00491809800006,2.2,3.45626926299998));
#303037=CARTESIAN_POINT('Ctrl Pts',(-2.00500980600005,12.2,3.45641623299999));
#303038=CARTESIAN_POINT('Ctrl Pts',(-2.00500980600005,5.2,3.45641623299999));
#303039=CARTESIAN_POINT('Ctrl Pts',(-2.00500980600005,2.2,3.45641623299999));
#303040=CARTESIAN_POINT('Ctrl Pts',(-2.00510546900006,12.2,3.45656907899999));
#303041=CARTESIAN_POINT('Ctrl Pts',(-2.00510546900006,5.2,3.45656907899999));
#303042=CARTESIAN_POINT('Ctrl Pts',(-2.00510546900006,2.2,3.45656907899999));
#303043=CARTESIAN_POINT('Ctrl Pts',(-2.00520509200006,12.2,3.45672777999999));
#303044=CARTESIAN_POINT('Ctrl Pts',(-2.00520509200006,5.2,3.45672777999999));
#303045=CARTESIAN_POINT('Ctrl Pts',(-2.00520509200006,2.2,3.45672777999999));
#303046=CARTESIAN_POINT('Ctrl Pts',(-2.00530868400006,12.2,3.45689231299998));
#303047=CARTESIAN_POINT('Ctrl Pts',(-2.00530868400006,5.2,3.45689231299998));
#303048=CARTESIAN_POINT('Ctrl Pts',(-2.00530868400006,2.2,3.45689231299998));
#303049=CARTESIAN_POINT('Ctrl Pts',(-2.00541625000006,12.2,3.45706265199999));
#303050=CARTESIAN_POINT('Ctrl Pts',(-2.00541625000006,5.2,3.45706265199999));
#303051=CARTESIAN_POINT('Ctrl Pts',(-2.00541625000006,2.2,3.45706265199999));
#303052=CARTESIAN_POINT('Ctrl Pts',(-2.00552780100006,12.2,3.45723877799998));
#303053=CARTESIAN_POINT('Ctrl Pts',(-2.00552780100006,5.2,3.45723877799998));
#303054=CARTESIAN_POINT('Ctrl Pts',(-2.00552780100006,2.2,3.45723877799998));
#303055=CARTESIAN_POINT('Ctrl Pts',(-2.00564334200006,12.2,3.45742066199998));
#303056=CARTESIAN_POINT('Ctrl Pts',(-2.00564334200006,5.2,3.45742066199998));
#303057=CARTESIAN_POINT('Ctrl Pts',(-2.00564334200006,2.2,3.45742066199998));
#303058=CARTESIAN_POINT('Ctrl Pts',(-2.00576288000006,12.2,3.45760828499999));
#303059=CARTESIAN_POINT('Ctrl Pts',(-2.00576288000006,5.2,3.45760828499999));
#303060=CARTESIAN_POINT('Ctrl Pts',(-2.00576288000006,2.2,3.45760828499999));
#303061=CARTESIAN_POINT('Ctrl Pts',(-2.00588642200006,12.2,3.45780162099998));
#303062=CARTESIAN_POINT('Ctrl Pts',(-2.00588642200006,5.2,3.45780162099998));
#303063=CARTESIAN_POINT('Ctrl Pts',(-2.00588642200006,2.2,3.45780162099998));
#303064=CARTESIAN_POINT('Ctrl Pts',(-2.00601397600006,12.2,3.45800064899999));
#303065=CARTESIAN_POINT('Ctrl Pts',(-2.00601397600006,5.2,3.45800064899999));
#303066=CARTESIAN_POINT('Ctrl Pts',(-2.00601397600006,2.2,3.45800064899999));
#303067=CARTESIAN_POINT('Ctrl Pts',(-2.00614554900006,12.2,3.45820534399999));
#303068=CARTESIAN_POINT('Ctrl Pts',(-2.00614554900006,5.2,3.45820534399999));
#303069=CARTESIAN_POINT('Ctrl Pts',(-2.00614554900006,2.2,3.45820534399999));
#303070=CARTESIAN_POINT('Ctrl Pts',(-2.00628114700006,12.2,3.45841568499999));
#303071=CARTESIAN_POINT('Ctrl Pts',(-2.00628114700006,5.2,3.45841568499999));
#303072=CARTESIAN_POINT('Ctrl Pts',(-2.00628114700006,2.2,3.45841568499999));
#303073=CARTESIAN_POINT('Ctrl Pts',(-2.00642077800006,12.2,3.45863164899999));
#303074=CARTESIAN_POINT('Ctrl Pts',(-2.00642077800006,5.2,3.45863164899999));
#303075=CARTESIAN_POINT('Ctrl Pts',(-2.00642077800006,2.2,3.45863164899999));
#303076=CARTESIAN_POINT('Ctrl Pts',(-2.00656444800006,12.2,3.45885321099999));
#303077=CARTESIAN_POINT('Ctrl Pts',(-2.00656444800006,5.2,3.45885321099999));
#303078=CARTESIAN_POINT('Ctrl Pts',(-2.00656444800006,2.2,3.45885321099999));
#303079=CARTESIAN_POINT('Ctrl Pts',(-2.00671216400006,12.2,3.45908034999999));
#303080=CARTESIAN_POINT('Ctrl Pts',(-2.00671216400006,5.2,3.45908034999999));
#303081=CARTESIAN_POINT('Ctrl Pts',(-2.00671216400006,2.2,3.45908034999999));
#303082=CARTESIAN_POINT('Ctrl Pts',(-2.00686393300006,12.2,3.45931304199999));
#303083=CARTESIAN_POINT('Ctrl Pts',(-2.00686393300006,5.2,3.45931304199999));
#303084=CARTESIAN_POINT('Ctrl Pts',(-2.00686393300006,2.2,3.45931304199999));
#303085=CARTESIAN_POINT('Ctrl Pts',(-2.00701976100006,12.2,3.45955126599998));
#303086=CARTESIAN_POINT('Ctrl Pts',(-2.00701976100006,5.2,3.45955126599998));
#303087=CARTESIAN_POINT('Ctrl Pts',(-2.00701976100006,2.2,3.45955126599998));
#303088=CARTESIAN_POINT('Ctrl Pts',(-2.00717965500006,12.2,3.45979499899999));
#303089=CARTESIAN_POINT('Ctrl Pts',(-2.00717965500006,5.2,3.45979499899999));
#303090=CARTESIAN_POINT('Ctrl Pts',(-2.00717965500006,2.2,3.45979499899999));
#303091=CARTESIAN_POINT('Ctrl Pts',(-2.00734362100006,12.2,3.46004421799999));
#303092=CARTESIAN_POINT('Ctrl Pts',(-2.00734362100006,5.2,3.46004421799999));
#303093=CARTESIAN_POINT('Ctrl Pts',(-2.00734362100006,2.2,3.46004421799999));
#303094=CARTESIAN_POINT('Ctrl Pts',(-2.00751166900006,12.2,3.46029890099998));
#303095=CARTESIAN_POINT('Ctrl Pts',(-2.00751166900006,5.2,3.46029890099998));
#303096=CARTESIAN_POINT('Ctrl Pts',(-2.00751166900006,2.2,3.46029890099998));
#303097=CARTESIAN_POINT('Ctrl Pts',(-2.00768380000006,12.2,3.46055902599999));
#303098=CARTESIAN_POINT('Ctrl Pts',(-2.00768380000006,5.2,3.46055902599999));
#303099=CARTESIAN_POINT('Ctrl Pts',(-2.00768380000006,2.2,3.46055902599999));
#303100=CARTESIAN_POINT('Ctrl Pts',(-2.00786002500006,12.2,3.46082456999999));
#303101=CARTESIAN_POINT('Ctrl Pts',(-2.00786002500006,5.2,3.46082456999999));
#303102=CARTESIAN_POINT('Ctrl Pts',(-2.00786002500006,2.2,3.46082456999999));
#303103=CARTESIAN_POINT('Ctrl Pts',(-2.00804034800006,12.2,3.46109550999999));
#303104=CARTESIAN_POINT('Ctrl Pts',(-2.00804034800006,5.2,3.46109550999999));
#303105=CARTESIAN_POINT('Ctrl Pts',(-2.00804034800006,2.2,3.46109550999999));
#303106=CARTESIAN_POINT('Ctrl Pts',(-2.00822477600005,12.2,3.46137182599998));
#303107=CARTESIAN_POINT('Ctrl Pts',(-2.00822477600005,5.2,3.46137182599998));
#303108=CARTESIAN_POINT('Ctrl Pts',(-2.00822477600005,2.2,3.46137182599998));
#303109=CARTESIAN_POINT('Ctrl Pts',(-2.00841331600006,12.2,3.46165349399998));
#303110=CARTESIAN_POINT('Ctrl Pts',(-2.00841331600006,5.2,3.46165349399998));
#303111=CARTESIAN_POINT('Ctrl Pts',(-2.00841331600006,2.2,3.46165349399998));
#303112=CARTESIAN_POINT('Ctrl Pts',(-2.00860597300006,12.2,3.46194049399998));
#303113=CARTESIAN_POINT('Ctrl Pts',(-2.00860597300006,5.2,3.46194049399998));
#303114=CARTESIAN_POINT('Ctrl Pts',(-2.00860597300006,2.2,3.46194049399998));
#303115=CARTESIAN_POINT('Ctrl Pts',(-2.00880275500006,12.2,3.46223280199998));
#303116=CARTESIAN_POINT('Ctrl Pts',(-2.00880275500006,5.2,3.46223280199998));
#303117=CARTESIAN_POINT('Ctrl Pts',(-2.00880275500006,2.2,3.46223280199998));
#303118=CARTESIAN_POINT('Ctrl Pts',(-2.00900366600006,12.2,3.46253039699998));
#303119=CARTESIAN_POINT('Ctrl Pts',(-2.00900366600006,5.2,3.46253039699998));
#303120=CARTESIAN_POINT('Ctrl Pts',(-2.00900366600006,2.2,3.46253039699998));
#303121=CARTESIAN_POINT('Ctrl Pts',(-2.00920871300006,12.2,3.46283325799998));
#303122=CARTESIAN_POINT('Ctrl Pts',(-2.00920871300006,5.2,3.46283325799998));
#303123=CARTESIAN_POINT('Ctrl Pts',(-2.00920871300006,2.2,3.46283325799998));
#303124=CARTESIAN_POINT('Ctrl Pts',(-2.00941790300006,12.2,3.46314136199998));
#303125=CARTESIAN_POINT('Ctrl Pts',(-2.00941790300006,5.2,3.46314136199998));
#303126=CARTESIAN_POINT('Ctrl Pts',(-2.00941790300006,2.2,3.46314136199998));
#303127=CARTESIAN_POINT('Ctrl Pts',(-2.00963124100006,12.2,3.46345468799999));
#303128=CARTESIAN_POINT('Ctrl Pts',(-2.00963124100006,5.2,3.46345468799999));
#303129=CARTESIAN_POINT('Ctrl Pts',(-2.00963124100006,2.2,3.46345468799999));
#303130=CARTESIAN_POINT('Ctrl Pts',(-2.00984873400006,12.2,3.46377321299999));
#303131=CARTESIAN_POINT('Ctrl Pts',(-2.00984873400006,5.2,3.46377321299999));
#303132=CARTESIAN_POINT('Ctrl Pts',(-2.00984873400006,2.2,3.46377321299999));
#303133=CARTESIAN_POINT('Ctrl Pts',(-2.01007038700005,12.2,3.46409691799998));
#303134=CARTESIAN_POINT('Ctrl Pts',(-2.01007038700005,5.2,3.46409691799998));
#303135=CARTESIAN_POINT('Ctrl Pts',(-2.01007038700005,2.2,3.46409691799998));
#303136=CARTESIAN_POINT('Ctrl Pts',(-2.01029620600006,12.2,3.46442577899998));
#303137=CARTESIAN_POINT('Ctrl Pts',(-2.01029620600006,5.2,3.46442577899998));
#303138=CARTESIAN_POINT('Ctrl Pts',(-2.01029620600006,2.2,3.46442577899998));
#303139=CARTESIAN_POINT('Ctrl Pts',(-2.01052619700006,12.2,3.46475977699999));
#303140=CARTESIAN_POINT('Ctrl Pts',(-2.01052619700006,5.2,3.46475977699999));
#303141=CARTESIAN_POINT('Ctrl Pts',(-2.01052619700006,2.2,3.46475977699999));
#303142=CARTESIAN_POINT('Ctrl Pts',(-2.01076036700006,12.2,3.46509888899998));
#303143=CARTESIAN_POINT('Ctrl Pts',(-2.01076036700006,5.2,3.46509888899998));
#303144=CARTESIAN_POINT('Ctrl Pts',(-2.01076036700006,2.2,3.46509888899998));
#303145=CARTESIAN_POINT('Ctrl Pts',(-2.01099872000006,12.2,3.46544309399999));
#303146=CARTESIAN_POINT('Ctrl Pts',(-2.01099872000006,5.2,3.46544309399999));
#303147=CARTESIAN_POINT('Ctrl Pts',(-2.01099872000006,2.2,3.46544309399999));
#303148=CARTESIAN_POINT('Ctrl Pts',(-2.01124126300006,12.2,3.46579237099998));
#303149=CARTESIAN_POINT('Ctrl Pts',(-2.01124126300006,5.2,3.46579237099998));
#303150=CARTESIAN_POINT('Ctrl Pts',(-2.01124126300006,2.2,3.46579237099998));
#303151=CARTESIAN_POINT('Ctrl Pts',(-2.01148800000006,12.2,3.46614669899999));
#303152=CARTESIAN_POINT('Ctrl Pts',(-2.01148800000006,5.2,3.46614669899999));
#303153=CARTESIAN_POINT('Ctrl Pts',(-2.01148800000006,2.2,3.46614669899999));
#303154=CARTESIAN_POINT('Ctrl Pts',(-2.01173893900005,12.2,3.46650605599999));
#303155=CARTESIAN_POINT('Ctrl Pts',(-2.01173893900005,5.2,3.46650605599999));
#303156=CARTESIAN_POINT('Ctrl Pts',(-2.01173893900005,2.2,3.46650605599999));
#303157=CARTESIAN_POINT('Ctrl Pts',(-2.01199408500006,12.2,3.46687042099998));
#303158=CARTESIAN_POINT('Ctrl Pts',(-2.01199408500006,5.2,3.46687042099998));
#303159=CARTESIAN_POINT('Ctrl Pts',(-2.01199408500006,2.2,3.46687042099998));
#303160=CARTESIAN_POINT('Ctrl Pts',(-2.01225344200005,12.2,3.46723977499998));
#303161=CARTESIAN_POINT('Ctrl Pts',(-2.01225344200005,5.2,3.46723977499998));
#303162=CARTESIAN_POINT('Ctrl Pts',(-2.01225344200005,2.2,3.46723977499998));
#303163=CARTESIAN_POINT('Ctrl Pts',(-2.01251701700006,12.2,3.46761409499998));
#303164=CARTESIAN_POINT('Ctrl Pts',(-2.01251701700006,5.2,3.46761409499998));
#303165=CARTESIAN_POINT('Ctrl Pts',(-2.01251701700006,2.2,3.46761409499998));
#303166=CARTESIAN_POINT('Ctrl Pts',(-2.01278481500006,12.2,3.46799336099998));
#303167=CARTESIAN_POINT('Ctrl Pts',(-2.01278481500006,5.2,3.46799336099998));
#303168=CARTESIAN_POINT('Ctrl Pts',(-2.01278481500006,2.2,3.46799336099998));
#303169=CARTESIAN_POINT('Ctrl Pts',(-2.01305684200006,12.2,3.46837755199999));
#303170=CARTESIAN_POINT('Ctrl Pts',(-2.01305684200006,5.2,3.46837755199999));
#303171=CARTESIAN_POINT('Ctrl Pts',(-2.01305684200006,2.2,3.46837755199999));
#303172=CARTESIAN_POINT('Ctrl Pts',(-2.01333310200006,12.2,3.46876664699998));
#303173=CARTESIAN_POINT('Ctrl Pts',(-2.01333310200006,5.2,3.46876664699998));
#303174=CARTESIAN_POINT('Ctrl Pts',(-2.01333310200006,2.2,3.46876664699998));
#303175=CARTESIAN_POINT('Ctrl Pts',(-2.01361360100006,12.2,3.46916062499999));
#303176=CARTESIAN_POINT('Ctrl Pts',(-2.01361360100006,5.2,3.46916062499999));
#303177=CARTESIAN_POINT('Ctrl Pts',(-2.01361360100006,2.2,3.46916062499999));
#303178=CARTESIAN_POINT('Ctrl Pts',(-2.01389834600006,12.2,3.46955946699998));
#303179=CARTESIAN_POINT('Ctrl Pts',(-2.01389834600006,5.2,3.46955946699998));
#303180=CARTESIAN_POINT('Ctrl Pts',(-2.01389834600006,2.2,3.46955946699998));
#303181=CARTESIAN_POINT('Ctrl Pts',(-2.01418734100006,12.2,3.46996315099998));
#303182=CARTESIAN_POINT('Ctrl Pts',(-2.01418734100006,5.2,3.46996315099998));
#303183=CARTESIAN_POINT('Ctrl Pts',(-2.01418734100006,2.2,3.46996315099998));
#303184=CARTESIAN_POINT('Ctrl Pts',(-2.01448059000006,12.2,3.47037165699999));
#303185=CARTESIAN_POINT('Ctrl Pts',(-2.01448059000006,5.2,3.47037165699999));
#303186=CARTESIAN_POINT('Ctrl Pts',(-2.01448059000006,2.2,3.47037165699999));
#303187=CARTESIAN_POINT('Ctrl Pts',(-2.01477810100006,12.2,3.47078496399998));
#303188=CARTESIAN_POINT('Ctrl Pts',(-2.01477810100006,5.2,3.47078496399998));
#303189=CARTESIAN_POINT('Ctrl Pts',(-2.01477810100006,2.2,3.47078496399998));
#303190=CARTESIAN_POINT('Ctrl Pts',(-2.01507987500006,12.2,3.47120305099998));
#303191=CARTESIAN_POINT('Ctrl Pts',(-2.01507987500006,5.2,3.47120305099998));
#303192=CARTESIAN_POINT('Ctrl Pts',(-2.01507987500006,2.2,3.47120305099998));
#303193=CARTESIAN_POINT('Ctrl Pts',(-2.01538592200006,12.2,3.47162589999999));
#303194=CARTESIAN_POINT('Ctrl Pts',(-2.01538592200006,5.2,3.47162589999999));
#303195=CARTESIAN_POINT('Ctrl Pts',(-2.01538592200006,2.2,3.47162589999999));
#303196=CARTESIAN_POINT('Ctrl Pts',(-2.01569624400005,12.2,3.47205348999999));
#303197=CARTESIAN_POINT('Ctrl Pts',(-2.01569624400005,5.2,3.47205348999999));
#303198=CARTESIAN_POINT('Ctrl Pts',(-2.01569624400005,2.2,3.47205348999999));
#303199=CARTESIAN_POINT('Ctrl Pts',(-2.01601084700005,12.2,3.47248579799999));
#303200=CARTESIAN_POINT('Ctrl Pts',(-2.01601084700005,5.2,3.47248579799999));
#303201=CARTESIAN_POINT('Ctrl Pts',(-2.01601084700005,2.2,3.47248579799999));
#303202=CARTESIAN_POINT('Ctrl Pts',(-2.01632973500006,12.2,3.47292280699998));
#303203=CARTESIAN_POINT('Ctrl Pts',(-2.01632973500006,5.2,3.47292280699998));
#303204=CARTESIAN_POINT('Ctrl Pts',(-2.01632973500006,2.2,3.47292280699998));
#303205=CARTESIAN_POINT('Ctrl Pts',(-2.01665291500006,12.2,3.47336449599998));
#303206=CARTESIAN_POINT('Ctrl Pts',(-2.01665291500006,5.2,3.47336449599998));
#303207=CARTESIAN_POINT('Ctrl Pts',(-2.01665291500006,2.2,3.47336449599998));
#303208=CARTESIAN_POINT('Ctrl Pts',(-2.01698039000005,12.2,3.47381084599999));
#303209=CARTESIAN_POINT('Ctrl Pts',(-2.01698039000005,5.2,3.47381084599999));
#303210=CARTESIAN_POINT('Ctrl Pts',(-2.01698039000005,2.2,3.47381084599999));
#303211=CARTESIAN_POINT('Ctrl Pts',(-2.01731216500006,12.2,3.47426183399998));
#303212=CARTESIAN_POINT('Ctrl Pts',(-2.01731216500006,5.2,3.47426183399998));
#303213=CARTESIAN_POINT('Ctrl Pts',(-2.01731216500006,2.2,3.47426183399998));
#303214=CARTESIAN_POINT('Ctrl Pts',(-2.01764824700006,12.2,3.47471744199999));
#303215=CARTESIAN_POINT('Ctrl Pts',(-2.01764824700006,5.2,3.47471744199999));
#303216=CARTESIAN_POINT('Ctrl Pts',(-2.01764824700006,2.2,3.47471744199999));
#303217=CARTESIAN_POINT('Ctrl Pts',(-2.01798863800006,12.2,3.47517765199999));
#303218=CARTESIAN_POINT('Ctrl Pts',(-2.01798863800006,5.2,3.47517765199999));
#303219=CARTESIAN_POINT('Ctrl Pts',(-2.01798863800006,2.2,3.47517765199999));
#303220=CARTESIAN_POINT('Ctrl Pts',(-2.01833334400006,12.2,3.47564244099999));
#303221=CARTESIAN_POINT('Ctrl Pts',(-2.01833334400006,5.2,3.47564244099999));
#303222=CARTESIAN_POINT('Ctrl Pts',(-2.01833334400006,2.2,3.47564244099999));
#303223=CARTESIAN_POINT('Ctrl Pts',(-2.01868237000005,12.2,3.47611178899999));
#303224=CARTESIAN_POINT('Ctrl Pts',(-2.01868237000005,5.2,3.47611178899999));
#303225=CARTESIAN_POINT('Ctrl Pts',(-2.01868237000005,2.2,3.47611178899999));
#303226=CARTESIAN_POINT('Ctrl Pts',(-2.01903572100006,12.2,3.47658567899998));
#303227=CARTESIAN_POINT('Ctrl Pts',(-2.01903572100006,5.2,3.47658567899998));
#303228=CARTESIAN_POINT('Ctrl Pts',(-2.01903572100006,2.2,3.47658567899998));
#303229=CARTESIAN_POINT('Ctrl Pts',(-2.01939340100005,12.2,3.47706408999999));
#303230=CARTESIAN_POINT('Ctrl Pts',(-2.01939340100005,5.2,3.47706408999999));
#303231=CARTESIAN_POINT('Ctrl Pts',(-2.01939340100005,2.2,3.47706408999999));
#303232=CARTESIAN_POINT('Ctrl Pts',(-2.01975541400006,12.2,3.47754700199999));
#303233=CARTESIAN_POINT('Ctrl Pts',(-2.01975541400006,5.2,3.47754700199999));
#303234=CARTESIAN_POINT('Ctrl Pts',(-2.01975541400006,2.2,3.47754700199999));
#303235=CARTESIAN_POINT('Ctrl Pts',(-2.02012176600005,12.2,3.47803439599998));
#303236=CARTESIAN_POINT('Ctrl Pts',(-2.02012176600005,5.2,3.47803439599998));
#303237=CARTESIAN_POINT('Ctrl Pts',(-2.02012176600005,2.2,3.47803439599998));
#303238=CARTESIAN_POINT('Ctrl Pts',(-2.02049246100006,12.2,3.47852625099998));
#303239=CARTESIAN_POINT('Ctrl Pts',(-2.02049246100006,5.2,3.47852625099998));
#303240=CARTESIAN_POINT('Ctrl Pts',(-2.02049246100006,2.2,3.47852625099998));
#303241=CARTESIAN_POINT('Ctrl Pts',(-2.02086750300006,12.2,3.47902254999998));
#303242=CARTESIAN_POINT('Ctrl Pts',(-2.02086750300006,5.2,3.47902254999998));
#303243=CARTESIAN_POINT('Ctrl Pts',(-2.02086750300006,2.2,3.47902254999998));
#303244=CARTESIAN_POINT('Ctrl Pts',(-2.02124689700006,12.2,3.47952327299998));
#303245=CARTESIAN_POINT('Ctrl Pts',(-2.02124689700006,5.2,3.47952327299998));
#303246=CARTESIAN_POINT('Ctrl Pts',(-2.02124689700006,2.2,3.47952327299998));
#303247=CARTESIAN_POINT('Ctrl Pts',(-2.02163064700006,12.2,3.48002839899999));
#303248=CARTESIAN_POINT('Ctrl Pts',(-2.02163064700006,5.2,3.48002839899999));
#303249=CARTESIAN_POINT('Ctrl Pts',(-2.02163064700006,2.2,3.48002839899999));
#303250=CARTESIAN_POINT('Ctrl Pts',(-2.02201875900006,12.2,3.48053790899999));
#303251=CARTESIAN_POINT('Ctrl Pts',(-2.02201875900006,5.2,3.48053790899999));
#303252=CARTESIAN_POINT('Ctrl Pts',(-2.02201875900006,2.2,3.48053790899999));
#303253=CARTESIAN_POINT('Ctrl Pts',(-2.02241123400006,12.2,3.48105178599998));
#303254=CARTESIAN_POINT('Ctrl Pts',(-2.02241123400006,5.2,3.48105178599998));
#303255=CARTESIAN_POINT('Ctrl Pts',(-2.02241123400006,2.2,3.48105178599998));
#303256=CARTESIAN_POINT('Ctrl Pts',(-2.02280808000005,12.2,3.48157000899998));
#303257=CARTESIAN_POINT('Ctrl Pts',(-2.02280808000005,5.2,3.48157000899998));
#303258=CARTESIAN_POINT('Ctrl Pts',(-2.02280808000005,2.2,3.48157000899998));
#303259=CARTESIAN_POINT('Ctrl Pts',(-2.02320930000006,12.2,3.48209255899998));
#303260=CARTESIAN_POINT('Ctrl Pts',(-2.02320930000006,5.2,3.48209255899998));
#303261=CARTESIAN_POINT('Ctrl Pts',(-2.02320930000006,2.2,3.48209255899998));
#303262=CARTESIAN_POINT('Ctrl Pts',(-2.02361489700006,12.2,3.48261941699998));
#303263=CARTESIAN_POINT('Ctrl Pts',(-2.02361489700006,5.2,3.48261941699998));
#303264=CARTESIAN_POINT('Ctrl Pts',(-2.02361489700006,2.2,3.48261941699998));
#303265=CARTESIAN_POINT('Ctrl Pts',(-2.02402487700006,12.2,3.48315056399999));
#303266=CARTESIAN_POINT('Ctrl Pts',(-2.02402487700006,5.2,3.48315056399999));
#303267=CARTESIAN_POINT('Ctrl Pts',(-2.02402487700006,2.2,3.48315056399999));
#303268=CARTESIAN_POINT('Ctrl Pts',(-2.02443924200006,12.2,3.48368597999999));
#303269=CARTESIAN_POINT('Ctrl Pts',(-2.02443924200006,5.2,3.48368597999999));
#303270=CARTESIAN_POINT('Ctrl Pts',(-2.02443924200006,2.2,3.48368597999999));
#303271=CARTESIAN_POINT('Ctrl Pts',(-2.02485799900006,12.2,3.48422564899998));
#303272=CARTESIAN_POINT('Ctrl Pts',(-2.02485799900006,5.2,3.48422564899998));
#303273=CARTESIAN_POINT('Ctrl Pts',(-2.02485799900006,2.2,3.48422564899998));
#303274=CARTESIAN_POINT('Ctrl Pts',(-2.02528115000006,12.2,3.48476954899999));
#303275=CARTESIAN_POINT('Ctrl Pts',(-2.02528115000006,5.2,3.48476954899999));
#303276=CARTESIAN_POINT('Ctrl Pts',(-2.02528115000006,2.2,3.48476954899999));
#303277=CARTESIAN_POINT('Ctrl Pts',(-2.02570870000006,12.2,3.48531766099998));
#303278=CARTESIAN_POINT('Ctrl Pts',(-2.02570870000006,5.2,3.48531766099998));
#303279=CARTESIAN_POINT('Ctrl Pts',(-2.02570870000006,2.2,3.48531766099998));
#303280=CARTESIAN_POINT('Ctrl Pts',(-2.02614065300006,12.2,3.48586996899999));
#303281=CARTESIAN_POINT('Ctrl Pts',(-2.02614065300006,5.2,3.48586996899999));
#303282=CARTESIAN_POINT('Ctrl Pts',(-2.02614065300006,2.2,3.48586996899999));
#303283=CARTESIAN_POINT('Ctrl Pts',(-2.02657701300006,12.2,3.48642645299999));
#303284=CARTESIAN_POINT('Ctrl Pts',(-2.02657701300006,5.2,3.48642645299999));
#303285=CARTESIAN_POINT('Ctrl Pts',(-2.02657701300006,2.2,3.48642645299999));
#303286=CARTESIAN_POINT('Ctrl Pts',(-2.02701778400006,12.2,3.48698709399999));
#303287=CARTESIAN_POINT('Ctrl Pts',(-2.02701778400006,5.2,3.48698709399999));
#303288=CARTESIAN_POINT('Ctrl Pts',(-2.02701778400006,2.2,3.48698709399999));
#303289=CARTESIAN_POINT('Ctrl Pts',(-2.02746296900005,12.2,3.48755187299999));
#303290=CARTESIAN_POINT('Ctrl Pts',(-2.02746296900005,5.2,3.48755187299999));
#303291=CARTESIAN_POINT('Ctrl Pts',(-2.02746296900005,2.2,3.48755187299999));
#303292=CARTESIAN_POINT('Ctrl Pts',(-2.02791257300006,12.2,3.48812077099999));
#303293=CARTESIAN_POINT('Ctrl Pts',(-2.02791257300006,5.2,3.48812077099999));
#303294=CARTESIAN_POINT('Ctrl Pts',(-2.02791257300006,2.2,3.48812077099999));
#303295=CARTESIAN_POINT('Ctrl Pts',(-2.02836659900006,12.2,3.48869377099999));
#303296=CARTESIAN_POINT('Ctrl Pts',(-2.02836659900006,5.2,3.48869377099999));
#303297=CARTESIAN_POINT('Ctrl Pts',(-2.02836659900006,2.2,3.48869377099999));
#303298=CARTESIAN_POINT('Ctrl Pts',(-2.02882505200006,12.2,3.48927085299999));
#303299=CARTESIAN_POINT('Ctrl Pts',(-2.02882505200006,5.2,3.48927085299999));
#303300=CARTESIAN_POINT('Ctrl Pts',(-2.02882505200006,2.2,3.48927085299999));
#303301=CARTESIAN_POINT('Ctrl Pts',(-2.02928793500006,12.2,3.48985199999999));
#303302=CARTESIAN_POINT('Ctrl Pts',(-2.02928793500006,5.2,3.48985199999999));
#303303=CARTESIAN_POINT('Ctrl Pts',(-2.02928793500006,2.2,3.48985199999999));
#303304=CARTESIAN_POINT('Ctrl Pts',(-2.02975525200006,12.2,3.49043719299999));
#303305=CARTESIAN_POINT('Ctrl Pts',(-2.02975525200006,5.2,3.49043719299999));
#303306=CARTESIAN_POINT('Ctrl Pts',(-2.02975525200006,2.2,3.49043719299999));
#303307=CARTESIAN_POINT('Ctrl Pts',(-2.03022700700005,12.2,3.49102641199998));
#303308=CARTESIAN_POINT('Ctrl Pts',(-2.03022700700005,5.2,3.49102641199998));
#303309=CARTESIAN_POINT('Ctrl Pts',(-2.03022700700005,2.2,3.49102641199998));
#303310=CARTESIAN_POINT('Ctrl Pts',(-2.03070320300006,12.2,3.49161964199999));
#303311=CARTESIAN_POINT('Ctrl Pts',(-2.03070320300006,5.2,3.49161964199999));
#303312=CARTESIAN_POINT('Ctrl Pts',(-2.03070320300006,2.2,3.49161964199999));
#303313=CARTESIAN_POINT('Ctrl Pts',(-2.03118384500006,12.2,3.49221686199999));
#303314=CARTESIAN_POINT('Ctrl Pts',(-2.03118384500006,5.2,3.49221686199999));
#303315=CARTESIAN_POINT('Ctrl Pts',(-2.03118384500006,2.2,3.49221686199999));
#303316=CARTESIAN_POINT('Ctrl Pts',(-2.03166893600006,12.2,3.49281805499999));
#303317=CARTESIAN_POINT('Ctrl Pts',(-2.03166893600006,5.2,3.49281805499999));
#303318=CARTESIAN_POINT('Ctrl Pts',(-2.03166893600006,2.2,3.49281805499999));
#303319=CARTESIAN_POINT('Ctrl Pts',(-2.03215847800006,12.2,3.49342320099999));
#303320=CARTESIAN_POINT('Ctrl Pts',(-2.03215847800006,5.2,3.49342320099999));
#303321=CARTESIAN_POINT('Ctrl Pts',(-2.03215847800006,2.2,3.49342320099999));
#303322=CARTESIAN_POINT('Ctrl Pts',(-2.03265247700006,12.2,3.49403228499998));
#303323=CARTESIAN_POINT('Ctrl Pts',(-2.03265247700006,5.2,3.49403228499998));
#303324=CARTESIAN_POINT('Ctrl Pts',(-2.03265247700006,2.2,3.49403228499998));
#303325=CARTESIAN_POINT('Ctrl Pts',(-2.03315093500006,12.2,3.49464528699999));
#303326=CARTESIAN_POINT('Ctrl Pts',(-2.03315093500006,5.2,3.49464528699999));
#303327=CARTESIAN_POINT('Ctrl Pts',(-2.03315093500006,2.2,3.49464528699999));
#303328=CARTESIAN_POINT('Ctrl Pts',(-2.03365385700006,12.2,3.49526218799999));
#303329=CARTESIAN_POINT('Ctrl Pts',(-2.03365385700006,5.2,3.49526218799999));
#303330=CARTESIAN_POINT('Ctrl Pts',(-2.03365385700006,2.2,3.49526218799999));
#303331=CARTESIAN_POINT('Ctrl Pts',(-2.03416124500006,12.2,3.49588297199999));
#303332=CARTESIAN_POINT('Ctrl Pts',(-2.03416124500006,5.2,3.49588297199999));
#303333=CARTESIAN_POINT('Ctrl Pts',(-2.03416124500006,2.2,3.49588297199999));
#303334=CARTESIAN_POINT('Ctrl Pts',(-2.03467310300006,12.2,3.49650761999998));
#303335=CARTESIAN_POINT('Ctrl Pts',(-2.03467310300006,5.2,3.49650761999998));
#303336=CARTESIAN_POINT('Ctrl Pts',(-2.03467310300006,2.2,3.49650761999998));
#303337=CARTESIAN_POINT('Ctrl Pts',(-2.03518943400006,12.2,3.49713611399999));
#303338=CARTESIAN_POINT('Ctrl Pts',(-2.03518943400006,5.2,3.49713611399999));
#303339=CARTESIAN_POINT('Ctrl Pts',(-2.03518943400006,2.2,3.49713611399999));
#303340=CARTESIAN_POINT('Ctrl Pts',(-2.03571024300006,12.2,3.49776843699999));
#303341=CARTESIAN_POINT('Ctrl Pts',(-2.03571024300006,5.2,3.49776843699999));
#303342=CARTESIAN_POINT('Ctrl Pts',(-2.03571024300006,2.2,3.49776843699999));
#303343=CARTESIAN_POINT('Ctrl Pts',(-2.03623553100006,12.2,3.49840457099998));
#303344=CARTESIAN_POINT('Ctrl Pts',(-2.03623553100006,5.2,3.49840457099998));
#303345=CARTESIAN_POINT('Ctrl Pts',(-2.03623553100006,2.2,3.49840457099998));
#303346=CARTESIAN_POINT('Ctrl Pts',(-2.03676530300006,12.2,3.49904449799999));
#303347=CARTESIAN_POINT('Ctrl Pts',(-2.03676530300006,5.2,3.49904449799999));
#303348=CARTESIAN_POINT('Ctrl Pts',(-2.03676530300006,2.2,3.49904449799999));
#303349=CARTESIAN_POINT('Ctrl Pts',(-2.03729956200006,12.2,3.49968819899999));
#303350=CARTESIAN_POINT('Ctrl Pts',(-2.03729956200006,5.2,3.49968819899999));
#303351=CARTESIAN_POINT('Ctrl Pts',(-2.03729956200006,2.2,3.49968819899999));
#303352=CARTESIAN_POINT('Ctrl Pts',(-2.03783831100006,12.2,3.50033565799999));
#303353=CARTESIAN_POINT('Ctrl Pts',(-2.03783831100006,5.2,3.50033565799999));
#303354=CARTESIAN_POINT('Ctrl Pts',(-2.03783831100006,2.2,3.50033565799999));
#303355=CARTESIAN_POINT('Ctrl Pts',(-2.03838155400006,12.2,3.50098685599999));
#303356=CARTESIAN_POINT('Ctrl Pts',(-2.03838155400006,5.2,3.50098685599999));
#303357=CARTESIAN_POINT('Ctrl Pts',(-2.03838155400006,2.2,3.50098685599999));
#303358=CARTESIAN_POINT('Ctrl Pts',(-2.03892929300005,12.2,3.50164177699998));
#303359=CARTESIAN_POINT('Ctrl Pts',(-2.03892929300005,5.2,3.50164177699998));
#303360=CARTESIAN_POINT('Ctrl Pts',(-2.03892929300005,2.2,3.50164177699998));
#303361=CARTESIAN_POINT('Ctrl Pts',(-2.03948153100006,12.2,3.50230040299999));
#303362=CARTESIAN_POINT('Ctrl Pts',(-2.03948153100006,5.2,3.50230040299999));
#303363=CARTESIAN_POINT('Ctrl Pts',(-2.03948153100006,2.2,3.50230040299999));
#303364=CARTESIAN_POINT('Ctrl Pts',(-2.04003827300005,12.2,3.50296271599999));
#303365=CARTESIAN_POINT('Ctrl Pts',(-2.04003827300005,5.2,3.50296271599999));
#303366=CARTESIAN_POINT('Ctrl Pts',(-2.04003827300005,2.2,3.50296271599999));
#303367=CARTESIAN_POINT('Ctrl Pts',(-2.04059952000006,12.2,3.50362869699998));
#303368=CARTESIAN_POINT('Ctrl Pts',(-2.04059952000006,5.2,3.50362869699998));
#303369=CARTESIAN_POINT('Ctrl Pts',(-2.04059952000006,2.2,3.50362869699998));
#303370=CARTESIAN_POINT('Ctrl Pts',(-2.04116527700006,12.2,3.50429833199998));
#303371=CARTESIAN_POINT('Ctrl Pts',(-2.04116527700006,5.2,3.50429833199998));
#303372=CARTESIAN_POINT('Ctrl Pts',(-2.04116527700006,2.2,3.50429833199998));
#303373=CARTESIAN_POINT('Ctrl Pts',(-2.04173554600006,12.2,3.50497160199998));
#303374=CARTESIAN_POINT('Ctrl Pts',(-2.04173554600006,5.2,3.50497160199998));
#303375=CARTESIAN_POINT('Ctrl Pts',(-2.04173554600006,2.2,3.50497160199998));
#303376=CARTESIAN_POINT('Ctrl Pts',(-2.04231033000006,12.2,3.50564848799999));
#303377=CARTESIAN_POINT('Ctrl Pts',(-2.04231033000006,5.2,3.50564848799999));
#303378=CARTESIAN_POINT('Ctrl Pts',(-2.04231033000006,2.2,3.50564848799999));
#303379=CARTESIAN_POINT('Ctrl Pts',(-2.04288963300006,12.2,3.50632897599999));
#303380=CARTESIAN_POINT('Ctrl Pts',(-2.04288963300006,5.2,3.50632897599999));
#303381=CARTESIAN_POINT('Ctrl Pts',(-2.04288963300006,2.2,3.50632897599999));
#303382=CARTESIAN_POINT('Ctrl Pts',(-2.04347345600006,12.2,3.50701304499999));
#303383=CARTESIAN_POINT('Ctrl Pts',(-2.04347345600006,5.2,3.50701304499999));
#303384=CARTESIAN_POINT('Ctrl Pts',(-2.04347345600006,2.2,3.50701304499999));
#303385=CARTESIAN_POINT('Ctrl Pts',(-2.04406180300006,12.2,3.50770068099998));
#303386=CARTESIAN_POINT('Ctrl Pts',(-2.04406180300006,5.2,3.50770068099998));
#303387=CARTESIAN_POINT('Ctrl Pts',(-2.04406180300006,2.2,3.50770068099998));
#303388=CARTESIAN_POINT('Ctrl Pts',(-2.04465467800006,12.2,3.50839186499999));
#303389=CARTESIAN_POINT('Ctrl Pts',(-2.04465467800006,5.2,3.50839186499999));
#303390=CARTESIAN_POINT('Ctrl Pts',(-2.04465467800006,2.2,3.50839186499999));
#303391=CARTESIAN_POINT('Ctrl Pts',(-2.04525208200006,12.2,3.50908657999998));
#303392=CARTESIAN_POINT('Ctrl Pts',(-2.04525208200006,5.2,3.50908657999998));
#303393=CARTESIAN_POINT('Ctrl Pts',(-2.04525208200006,2.2,3.50908657999998));
#303394=CARTESIAN_POINT('Ctrl Pts',(-2.04585401900006,12.2,3.50978480999999));
#303395=CARTESIAN_POINT('Ctrl Pts',(-2.04585401900006,5.2,3.50978480999999));
#303396=CARTESIAN_POINT('Ctrl Pts',(-2.04585401900006,2.2,3.50978480999999));
#303397=CARTESIAN_POINT('Ctrl Pts',(-2.04646049200006,12.2,3.51048653799998));
#303398=CARTESIAN_POINT('Ctrl Pts',(-2.04646049200006,5.2,3.51048653799998));
#303399=CARTESIAN_POINT('Ctrl Pts',(-2.04646049200006,2.2,3.51048653799998));
#303400=CARTESIAN_POINT('Ctrl Pts',(-2.04707150300006,12.2,3.51119174499999));
#303401=CARTESIAN_POINT('Ctrl Pts',(-2.04707150300006,5.2,3.51119174499999));
#303402=CARTESIAN_POINT('Ctrl Pts',(-2.04707150300006,2.2,3.51119174499999));
#303403=CARTESIAN_POINT('Ctrl Pts',(-2.04768705500005,12.2,3.51190041499999));
#303404=CARTESIAN_POINT('Ctrl Pts',(-2.04768705500005,5.2,3.51190041499999));
#303405=CARTESIAN_POINT('Ctrl Pts',(-2.04768705500005,2.2,3.51190041499999));
#303406=CARTESIAN_POINT('Ctrl Pts',(-2.04830715100006,12.2,3.51261253299998));
#303407=CARTESIAN_POINT('Ctrl Pts',(-2.04830715100006,5.2,3.51261253299998));
#303408=CARTESIAN_POINT('Ctrl Pts',(-2.04830715100006,2.2,3.51261253299998));
#303409=CARTESIAN_POINT('Ctrl Pts',(-2.04893179400006,12.2,3.51332807899999));
#303410=CARTESIAN_POINT('Ctrl Pts',(-2.04893179400006,5.2,3.51332807899999));
#303411=CARTESIAN_POINT('Ctrl Pts',(-2.04893179400006,2.2,3.51332807899999));
#303412=CARTESIAN_POINT('Ctrl Pts',(-2.04956098500006,12.2,3.51404703799999));
#303413=CARTESIAN_POINT('Ctrl Pts',(-2.04956098500006,5.2,3.51404703799999));
#303414=CARTESIAN_POINT('Ctrl Pts',(-2.04956098500006,2.2,3.51404703799999));
#303415=CARTESIAN_POINT('Ctrl Pts',(-2.05019473000006,12.2,3.51476939299998));
#303416=CARTESIAN_POINT('Ctrl Pts',(-2.05019473000006,5.2,3.51476939299998));
#303417=CARTESIAN_POINT('Ctrl Pts',(-2.05019473000006,2.2,3.51476939299998));
#303418=CARTESIAN_POINT('Ctrl Pts',(-2.05083302700006,12.2,3.51549512699999));
#303419=CARTESIAN_POINT('Ctrl Pts',(-2.05083302700006,5.2,3.51549512699999));
#303420=CARTESIAN_POINT('Ctrl Pts',(-2.05083302700006,2.2,3.51549512699999));
#303421=CARTESIAN_POINT('Ctrl Pts',(-2.05147588300005,12.2,3.51622422299998));
#303422=CARTESIAN_POINT('Ctrl Pts',(-2.05147588300005,5.2,3.51622422299998));
#303423=CARTESIAN_POINT('Ctrl Pts',(-2.05147588300005,2.2,3.51622422299998));
#303424=CARTESIAN_POINT('Ctrl Pts',(-2.05212329700006,12.2,3.51695666399999));
#303425=CARTESIAN_POINT('Ctrl Pts',(-2.05212329700006,5.2,3.51695666399999));
#303426=CARTESIAN_POINT('Ctrl Pts',(-2.05212329700006,2.2,3.51695666399999));
#303427=CARTESIAN_POINT('Ctrl Pts',(-2.05277527500006,12.2,3.51769243499999));
#303428=CARTESIAN_POINT('Ctrl Pts',(-2.05277527500006,5.2,3.51769243499999));
#303429=CARTESIAN_POINT('Ctrl Pts',(-2.05277527500006,2.2,3.51769243499999));
#303430=CARTESIAN_POINT('Ctrl Pts',(-2.05343181700006,12.2,3.51843151799999));
#303431=CARTESIAN_POINT('Ctrl Pts',(-2.05343181700006,5.2,3.51843151799999));
#303432=CARTESIAN_POINT('Ctrl Pts',(-2.05343181700006,2.2,3.51843151799999));
#303433=CARTESIAN_POINT('Ctrl Pts',(-2.05409292700006,12.2,3.51917389699998));
#303434=CARTESIAN_POINT('Ctrl Pts',(-2.05409292700006,5.2,3.51917389699998));
#303435=CARTESIAN_POINT('Ctrl Pts',(-2.05409292700006,2.2,3.51917389699998));
#303436=CARTESIAN_POINT('Ctrl Pts',(-2.05475860500006,12.2,3.51991955499999));
#303437=CARTESIAN_POINT('Ctrl Pts',(-2.05475860500006,5.2,3.51991955499999));
#303438=CARTESIAN_POINT('Ctrl Pts',(-2.05475860500006,2.2,3.51991955499999));
#303439=CARTESIAN_POINT('Ctrl Pts',(-2.05542885700006,12.2,3.52066847499999));
#303440=CARTESIAN_POINT('Ctrl Pts',(-2.05542885700006,5.2,3.52066847499999));
#303441=CARTESIAN_POINT('Ctrl Pts',(-2.05542885700006,2.2,3.52066847499999));
#303442=CARTESIAN_POINT('Ctrl Pts',(-2.05610368200006,12.2,3.52142064199998));
#303443=CARTESIAN_POINT('Ctrl Pts',(-2.05610368200006,5.2,3.52142064199998));
#303444=CARTESIAN_POINT('Ctrl Pts',(-2.05610368200006,2.2,3.52142064199998));
#303445=CARTESIAN_POINT('Ctrl Pts',(-2.05678308500006,12.2,3.52217603899999));
#303446=CARTESIAN_POINT('Ctrl Pts',(-2.05678308500006,5.2,3.52217603899999));
#303447=CARTESIAN_POINT('Ctrl Pts',(-2.05678308500006,2.2,3.52217603899999));
#303448=CARTESIAN_POINT('Ctrl Pts',(-2.05746706600006,12.2,3.52293464899999));
#303449=CARTESIAN_POINT('Ctrl Pts',(-2.05746706600006,5.2,3.52293464899999));
#303450=CARTESIAN_POINT('Ctrl Pts',(-2.05746706600006,2.2,3.52293464899999));
#303451=CARTESIAN_POINT('Ctrl Pts',(-2.05815563000006,12.2,3.52369645699999));
#303452=CARTESIAN_POINT('Ctrl Pts',(-2.05815563000006,5.2,3.52369645699999));
#303453=CARTESIAN_POINT('Ctrl Pts',(-2.05815563000006,2.2,3.52369645699999));
#303454=CARTESIAN_POINT('Ctrl Pts',(-2.05884877800006,12.2,3.52446144499999));
#303455=CARTESIAN_POINT('Ctrl Pts',(-2.05884877800006,5.2,3.52446144499999));
#303456=CARTESIAN_POINT('Ctrl Pts',(-2.05884877800006,2.2,3.52446144499999));
#303457=CARTESIAN_POINT('Ctrl Pts',(-2.05954651100006,12.2,3.52522959799998));
#303458=CARTESIAN_POINT('Ctrl Pts',(-2.05954651100006,5.2,3.52522959799998));
#303459=CARTESIAN_POINT('Ctrl Pts',(-2.05954651100006,2.2,3.52522959799998));
#303460=CARTESIAN_POINT('Ctrl Pts',(-2.06024883300006,12.2,3.52600089799999));
#303461=CARTESIAN_POINT('Ctrl Pts',(-2.06024883300006,5.2,3.52600089799999));
#303462=CARTESIAN_POINT('Ctrl Pts',(-2.06024883300006,2.2,3.52600089799999));
#303463=CARTESIAN_POINT('Ctrl Pts',(-2.06095574500006,12.2,3.52677533199999));
#303464=CARTESIAN_POINT('Ctrl Pts',(-2.06095574500006,5.2,3.52677533199999));
#303465=CARTESIAN_POINT('Ctrl Pts',(-2.06095574500006,2.2,3.52677533199999));
#303466=CARTESIAN_POINT('Ctrl Pts',(-2.06166725100006,12.2,3.52755288099999));
#303467=CARTESIAN_POINT('Ctrl Pts',(-2.06166725100006,5.2,3.52755288099999));
#303468=CARTESIAN_POINT('Ctrl Pts',(-2.06166725100006,2.2,3.52755288099999));
#303469=CARTESIAN_POINT('Ctrl Pts',(-2.06238335200006,12.2,3.52833352999999));
#303470=CARTESIAN_POINT('Ctrl Pts',(-2.06238335200006,5.2,3.52833352999999));
#303471=CARTESIAN_POINT('Ctrl Pts',(-2.06238335200006,2.2,3.52833352999999));
#303472=CARTESIAN_POINT('Ctrl Pts',(-2.06310404900006,12.2,3.52911726299999));
#303473=CARTESIAN_POINT('Ctrl Pts',(-2.06310404900006,5.2,3.52911726299999));
#303474=CARTESIAN_POINT('Ctrl Pts',(-2.06310404900006,2.2,3.52911726299999));
#303475=CARTESIAN_POINT('Ctrl Pts',(-2.06382934600006,12.2,3.52990406399999));
#303476=CARTESIAN_POINT('Ctrl Pts',(-2.06382934600006,5.2,3.52990406399999));
#303477=CARTESIAN_POINT('Ctrl Pts',(-2.06382934600006,2.2,3.52990406399999));
#303478=CARTESIAN_POINT('Ctrl Pts',(-2.06455924400006,12.2,3.53069391599998));
#303479=CARTESIAN_POINT('Ctrl Pts',(-2.06455924400006,5.2,3.53069391599998));
#303480=CARTESIAN_POINT('Ctrl Pts',(-2.06455924400006,2.2,3.53069391599998));
#303481=CARTESIAN_POINT('Ctrl Pts',(-2.06529374600006,12.2,3.53148680299999));
#303482=CARTESIAN_POINT('Ctrl Pts',(-2.06529374600006,5.2,3.53148680299999));
#303483=CARTESIAN_POINT('Ctrl Pts',(-2.06529374600006,2.2,3.53148680299999));
#303484=CARTESIAN_POINT('Ctrl Pts',(-2.06603285300006,12.2,3.53228271099999));
#303485=CARTESIAN_POINT('Ctrl Pts',(-2.06603285300006,5.2,3.53228271099999));
#303486=CARTESIAN_POINT('Ctrl Pts',(-2.06603285300006,2.2,3.53228271099999));
#303487=CARTESIAN_POINT('Ctrl Pts',(-2.06677656700006,12.2,3.53308162299999));
#303488=CARTESIAN_POINT('Ctrl Pts',(-2.06677656700006,5.2,3.53308162299999));
#303489=CARTESIAN_POINT('Ctrl Pts',(-2.06677656700006,2.2,3.53308162299999));
#303490=CARTESIAN_POINT('Ctrl Pts',(-2.06752489200006,12.2,3.53388352199998));
#303491=CARTESIAN_POINT('Ctrl Pts',(-2.06752489200006,5.2,3.53388352199998));
#303492=CARTESIAN_POINT('Ctrl Pts',(-2.06752489200006,2.2,3.53388352199998));
#303493=CARTESIAN_POINT('Ctrl Pts',(-2.06827782600006,12.2,3.53468839399999));
#303494=CARTESIAN_POINT('Ctrl Pts',(-2.06827782600006,5.2,3.53468839399999));
#303495=CARTESIAN_POINT('Ctrl Pts',(-2.06827782600006,2.2,3.53468839399999));
#303496=CARTESIAN_POINT('Ctrl Pts',(-2.06903537500006,12.2,3.53549622199999));
#303497=CARTESIAN_POINT('Ctrl Pts',(-2.06903537500006,5.2,3.53549622199999));
#303498=CARTESIAN_POINT('Ctrl Pts',(-2.06903537500006,2.2,3.53549622199999));
#303499=CARTESIAN_POINT('Ctrl Pts',(-2.06979753900006,12.2,3.53630699099998));
#303500=CARTESIAN_POINT('Ctrl Pts',(-2.06979753900006,5.2,3.53630699099998));
#303501=CARTESIAN_POINT('Ctrl Pts',(-2.06979753900006,2.2,3.53630699099998));
#303502=CARTESIAN_POINT('Ctrl Pts',(-2.07056432000006,12.2,3.53712068399999));
#303503=CARTESIAN_POINT('Ctrl Pts',(-2.07056432000006,5.2,3.53712068399999));
#303504=CARTESIAN_POINT('Ctrl Pts',(-2.07056432000006,2.2,3.53712068399999));
#303505=CARTESIAN_POINT('Ctrl Pts',(-2.07133572000005,12.2,3.53793728699999));
#303506=CARTESIAN_POINT('Ctrl Pts',(-2.07133572000005,5.2,3.53793728699999));
#303507=CARTESIAN_POINT('Ctrl Pts',(-2.07133572000005,2.2,3.53793728699999));
#303508=CARTESIAN_POINT('Ctrl Pts',(-2.07211174100005,12.2,3.53875678399999));
#303509=CARTESIAN_POINT('Ctrl Pts',(-2.07211174100005,5.2,3.53875678399999));
#303510=CARTESIAN_POINT('Ctrl Pts',(-2.07211174100005,2.2,3.53875678399999));
#303511=CARTESIAN_POINT('Ctrl Pts',(-2.07289238500006,12.2,3.53957915799998));
#303512=CARTESIAN_POINT('Ctrl Pts',(-2.07289238500006,5.2,3.53957915799998));
#303513=CARTESIAN_POINT('Ctrl Pts',(-2.07289238500006,2.2,3.53957915799998));
#303514=CARTESIAN_POINT('Ctrl Pts',(-2.07367765300006,12.2,3.54040439499999));
#303515=CARTESIAN_POINT('Ctrl Pts',(-2.07367765300006,5.2,3.54040439499999));
#303516=CARTESIAN_POINT('Ctrl Pts',(-2.07367765300006,2.2,3.54040439499999));
#303517=CARTESIAN_POINT('Ctrl Pts',(-2.07446754800006,12.2,3.54123247799999));
#303518=CARTESIAN_POINT('Ctrl Pts',(-2.07446754800006,5.2,3.54123247799999));
#303519=CARTESIAN_POINT('Ctrl Pts',(-2.07446754800006,2.2,3.54123247799999));
#303520=CARTESIAN_POINT('Ctrl Pts',(-2.07526207000006,12.2,3.54206339399998));
#303521=CARTESIAN_POINT('Ctrl Pts',(-2.07526207000006,5.2,3.54206339399998));
#303522=CARTESIAN_POINT('Ctrl Pts',(-2.07526207000006,2.2,3.54206339399998));
#303523=CARTESIAN_POINT('Ctrl Pts',(-2.07606122200006,12.2,3.54289712399999));
#303524=CARTESIAN_POINT('Ctrl Pts',(-2.07606122200006,5.2,3.54289712399999));
#303525=CARTESIAN_POINT('Ctrl Pts',(-2.07606122200006,2.2,3.54289712399999));
#303526=CARTESIAN_POINT('Ctrl Pts',(-2.07686500500006,12.2,3.54373365599999));
#303527=CARTESIAN_POINT('Ctrl Pts',(-2.07686500500006,5.2,3.54373365599999));
#303528=CARTESIAN_POINT('Ctrl Pts',(-2.07686500500006,2.2,3.54373365599999));
#303529=CARTESIAN_POINT('Ctrl Pts',(-2.07767342200006,12.2,3.54457297199998));
#303530=CARTESIAN_POINT('Ctrl Pts',(-2.07767342200006,5.2,3.54457297199998));
#303531=CARTESIAN_POINT('Ctrl Pts',(-2.07767342200006,2.2,3.54457297199998));
#303532=CARTESIAN_POINT('Ctrl Pts',(-2.07848647300006,12.2,3.54541505699999));
#303533=CARTESIAN_POINT('Ctrl Pts',(-2.07848647300006,5.2,3.54541505699999));
#303534=CARTESIAN_POINT('Ctrl Pts',(-2.07848647300006,2.2,3.54541505699999));
#303535=CARTESIAN_POINT('Ctrl Pts',(-2.07930416100006,12.2,3.54625989799998));
#303536=CARTESIAN_POINT('Ctrl Pts',(-2.07930416100006,5.2,3.54625989799998));
#303537=CARTESIAN_POINT('Ctrl Pts',(-2.07930416100006,2.2,3.54625989799998));
#303538=CARTESIAN_POINT('Ctrl Pts',(-2.08012648600006,12.2,3.54710747599999));
#303539=CARTESIAN_POINT('Ctrl Pts',(-2.08012648600006,5.2,3.54710747599999));
#303540=CARTESIAN_POINT('Ctrl Pts',(-2.08012648600006,2.2,3.54710747599999));
#303541=CARTESIAN_POINT('Ctrl Pts',(-2.08095345200006,12.2,3.54795777899999));
#303542=CARTESIAN_POINT('Ctrl Pts',(-2.08095345200006,5.2,3.54795777899999));
#303543=CARTESIAN_POINT('Ctrl Pts',(-2.08095345200006,2.2,3.54795777899999));
#303544=CARTESIAN_POINT('Ctrl Pts',(-2.08178505800006,12.2,3.54881078999998));
#303545=CARTESIAN_POINT('Ctrl Pts',(-2.08178505800006,5.2,3.54881078999998));
#303546=CARTESIAN_POINT('Ctrl Pts',(-2.08178505800006,2.2,3.54881078999998));
#303547=CARTESIAN_POINT('Ctrl Pts',(-2.08262130700006,12.2,3.54966649399999));
#303548=CARTESIAN_POINT('Ctrl Pts',(-2.08262130700006,5.2,3.54966649399999));
#303549=CARTESIAN_POINT('Ctrl Pts',(-2.08262130700006,2.2,3.54966649399999));
#303550=CARTESIAN_POINT('Ctrl Pts',(-2.08346219900006,12.2,3.55052487699999));
#303551=CARTESIAN_POINT('Ctrl Pts',(-2.08346219900006,5.2,3.55052487699999));
#303552=CARTESIAN_POINT('Ctrl Pts',(-2.08346219900006,2.2,3.55052487699999));
#303553=CARTESIAN_POINT('Ctrl Pts',(-2.08430773800006,12.2,3.55138592199998));
#303554=CARTESIAN_POINT('Ctrl Pts',(-2.08430773800006,5.2,3.55138592199998));
#303555=CARTESIAN_POINT('Ctrl Pts',(-2.08430773800006,2.2,3.55138592199998));
#303556=CARTESIAN_POINT('Ctrl Pts',(-2.08515792300005,12.2,3.55224961399998));
#303557=CARTESIAN_POINT('Ctrl Pts',(-2.08515792300005,5.2,3.55224961399998));
#303558=CARTESIAN_POINT('Ctrl Pts',(-2.08515792300005,2.2,3.55224961399998));
#303559=CARTESIAN_POINT('Ctrl Pts',(-2.08601275700006,12.2,3.55311593999998));
#303560=CARTESIAN_POINT('Ctrl Pts',(-2.08601275700006,5.2,3.55311593999998));
#303561=CARTESIAN_POINT('Ctrl Pts',(-2.08601275700006,2.2,3.55311593999998));
#303562=CARTESIAN_POINT('Ctrl Pts',(-2.08687224100006,12.2,3.55398488399998));
#303563=CARTESIAN_POINT('Ctrl Pts',(-2.08687224100006,5.2,3.55398488399998));
#303564=CARTESIAN_POINT('Ctrl Pts',(-2.08687224100006,2.2,3.55398488399998));
#303565=CARTESIAN_POINT('Ctrl Pts',(-2.08773637600005,12.2,3.55485642999999));
#303566=CARTESIAN_POINT('Ctrl Pts',(-2.08773637600005,5.2,3.55485642999999));
#303567=CARTESIAN_POINT('Ctrl Pts',(-2.08773637600005,2.2,3.55485642999999));
#303568=CARTESIAN_POINT('Ctrl Pts',(-2.08860516300006,12.2,3.55573056299999));
#303569=CARTESIAN_POINT('Ctrl Pts',(-2.08860516300006,5.2,3.55573056299999));
#303570=CARTESIAN_POINT('Ctrl Pts',(-2.08860516300006,2.2,3.55573056299999));
#303571=CARTESIAN_POINT('Ctrl Pts',(-2.08947860600006,12.2,3.55660726999999));
#303572=CARTESIAN_POINT('Ctrl Pts',(-2.08947860600006,5.2,3.55660726999999));
#303573=CARTESIAN_POINT('Ctrl Pts',(-2.08947860600006,2.2,3.55660726999999));
#303574=CARTESIAN_POINT('Ctrl Pts',(-2.09035670200006,12.2,3.55748653299998));
#303575=CARTESIAN_POINT('Ctrl Pts',(-2.09035670200006,5.2,3.55748653299998));
#303576=CARTESIAN_POINT('Ctrl Pts',(-2.09035670200006,2.2,3.55748653299998));
#303577=CARTESIAN_POINT('Ctrl Pts',(-2.09123945700005,12.2,3.55836833999999));
#303578=CARTESIAN_POINT('Ctrl Pts',(-2.09123945700005,5.2,3.55836833999999));
#303579=CARTESIAN_POINT('Ctrl Pts',(-2.09123945700005,2.2,3.55836833999999));
#303580=CARTESIAN_POINT('Ctrl Pts',(-2.09212686800006,12.2,3.55925267499998));
#303581=CARTESIAN_POINT('Ctrl Pts',(-2.09212686800006,5.2,3.55925267499998));
#303582=CARTESIAN_POINT('Ctrl Pts',(-2.09212686800006,2.2,3.55925267499998));
#303583=CARTESIAN_POINT('Ctrl Pts',(-2.09301893900005,12.2,3.56013952299998));
#303584=CARTESIAN_POINT('Ctrl Pts',(-2.09301893900005,5.2,3.56013952299998));
#303585=CARTESIAN_POINT('Ctrl Pts',(-2.09301893900005,2.2,3.56013952299998));
#303586=CARTESIAN_POINT('Ctrl Pts',(-2.09391567000006,12.2,3.56102886999999));
#303587=CARTESIAN_POINT('Ctrl Pts',(-2.09391567000006,5.2,3.56102886999999));
#303588=CARTESIAN_POINT('Ctrl Pts',(-2.09391567000006,2.2,3.56102886999999));
#303589=CARTESIAN_POINT('Ctrl Pts',(-2.09481706300005,12.2,3.56192070099999));
#303590=CARTESIAN_POINT('Ctrl Pts',(-2.09481706300005,5.2,3.56192070099999));
#303591=CARTESIAN_POINT('Ctrl Pts',(-2.09481706300005,2.2,3.56192070099999));
#303592=CARTESIAN_POINT('Ctrl Pts',(-2.09572311800006,12.2,3.56281500099998));
#303593=CARTESIAN_POINT('Ctrl Pts',(-2.09572311800006,5.2,3.56281500099998));
#303594=CARTESIAN_POINT('Ctrl Pts',(-2.09572311800006,2.2,3.56281500099998));
#303595=CARTESIAN_POINT('Ctrl Pts',(-2.09663383700006,12.2,3.56371175399998));
#303596=CARTESIAN_POINT('Ctrl Pts',(-2.09663383700006,5.2,3.56371175399998));
#303597=CARTESIAN_POINT('Ctrl Pts',(-2.09663383700006,2.2,3.56371175399998));
#303598=CARTESIAN_POINT('Ctrl Pts',(-2.09754922100006,12.2,3.56461094699998));
#303599=CARTESIAN_POINT('Ctrl Pts',(-2.09754922100006,5.2,3.56461094699998));
#303600=CARTESIAN_POINT('Ctrl Pts',(-2.09754922100006,2.2,3.56461094699998));
#303601=CARTESIAN_POINT('Ctrl Pts',(-2.09846927300006,12.2,3.56551256499999));
#303602=CARTESIAN_POINT('Ctrl Pts',(-2.09846927300006,5.2,3.56551256499999));
#303603=CARTESIAN_POINT('Ctrl Pts',(-2.09846927300006,2.2,3.56551256499999));
#303604=CARTESIAN_POINT('Ctrl Pts',(-2.09939399000006,12.2,3.56641659399998));
#303605=CARTESIAN_POINT('Ctrl Pts',(-2.09939399000006,5.2,3.56641659399998));
#303606=CARTESIAN_POINT('Ctrl Pts',(-2.09939399000006,2.2,3.56641659399998));
#303607=CARTESIAN_POINT('Ctrl Pts',(-2.10032337800006,12.2,3.56732301899999));
#303608=CARTESIAN_POINT('Ctrl Pts',(-2.10032337800006,5.2,3.56732301899999));
#303609=CARTESIAN_POINT('Ctrl Pts',(-2.10032337800006,2.2,3.56732301899999));
#303610=CARTESIAN_POINT('Ctrl Pts',(-2.10125743300006,12.2,3.56823182499999));
#303611=CARTESIAN_POINT('Ctrl Pts',(-2.10125743300006,5.2,3.56823182499999));
#303612=CARTESIAN_POINT('Ctrl Pts',(-2.10125743300006,2.2,3.56823182499999));
#303613=CARTESIAN_POINT('Ctrl Pts',(-2.10219615900006,12.2,3.56914299699999));
#303614=CARTESIAN_POINT('Ctrl Pts',(-2.10219615900006,5.2,3.56914299699999));
#303615=CARTESIAN_POINT('Ctrl Pts',(-2.10219615900006,2.2,3.56914299699999));
#303616=CARTESIAN_POINT('Ctrl Pts',(-2.10313955700005,12.2,3.57005652199998));
#303617=CARTESIAN_POINT('Ctrl Pts',(-2.10313955700005,5.2,3.57005652199998));
#303618=CARTESIAN_POINT('Ctrl Pts',(-2.10313955700005,2.2,3.57005652199998));
#303619=CARTESIAN_POINT('Ctrl Pts',(-2.10408762800005,12.2,3.57097238399999));
#303620=CARTESIAN_POINT('Ctrl Pts',(-2.10408762800005,5.2,3.57097238399999));
#303621=CARTESIAN_POINT('Ctrl Pts',(-2.10408762800005,2.2,3.57097238399999));
#303622=CARTESIAN_POINT('Ctrl Pts',(-2.10504037200006,12.2,3.57189057099998));
#303623=CARTESIAN_POINT('Ctrl Pts',(-2.10504037200006,5.2,3.57189057099998));
#303624=CARTESIAN_POINT('Ctrl Pts',(-2.10504037200006,2.2,3.57189057099998));
#303625=CARTESIAN_POINT('Ctrl Pts',(-2.10599779100006,12.2,3.57281106599999));
#303626=CARTESIAN_POINT('Ctrl Pts',(-2.10599779100006,5.2,3.57281106599999));
#303627=CARTESIAN_POINT('Ctrl Pts',(-2.10599779100006,2.2,3.57281106599999));
#303628=CARTESIAN_POINT('Ctrl Pts',(-2.10695988400006,12.2,3.57373385599999));
#303629=CARTESIAN_POINT('Ctrl Pts',(-2.10695988400006,5.2,3.57373385599999));
#303630=CARTESIAN_POINT('Ctrl Pts',(-2.10695988400006,2.2,3.57373385599999));
#303631=CARTESIAN_POINT('Ctrl Pts',(-2.10792665500006,12.2,3.57465892499999));
#303632=CARTESIAN_POINT('Ctrl Pts',(-2.10792665500006,5.2,3.57465892499999));
#303633=CARTESIAN_POINT('Ctrl Pts',(-2.10792665500006,2.2,3.57465892499999));
#303634=CARTESIAN_POINT('Ctrl Pts',(-2.10889810200006,12.2,3.57558626199998));
#303635=CARTESIAN_POINT('Ctrl Pts',(-2.10889810200006,5.2,3.57558626199998));
#303636=CARTESIAN_POINT('Ctrl Pts',(-2.10889810200006,2.2,3.57558626199998));
#303637=CARTESIAN_POINT('Ctrl Pts',(-2.10987422800006,12.2,3.57651584899998));
#303638=CARTESIAN_POINT('Ctrl Pts',(-2.10987422800006,5.2,3.57651584899998));
#303639=CARTESIAN_POINT('Ctrl Pts',(-2.10987422800006,2.2,3.57651584899998));
#303640=CARTESIAN_POINT('Ctrl Pts',(-2.11085503200006,12.2,3.57744767599999));
#303641=CARTESIAN_POINT('Ctrl Pts',(-2.11085503200006,5.2,3.57744767599999));
#303642=CARTESIAN_POINT('Ctrl Pts',(-2.11085503200006,2.2,3.57744767599999));
#303643=CARTESIAN_POINT('Ctrl Pts',(-2.11184051600006,12.2,3.57838172399998));
#303644=CARTESIAN_POINT('Ctrl Pts',(-2.11184051600006,5.2,3.57838172399998));
#303645=CARTESIAN_POINT('Ctrl Pts',(-2.11184051600006,2.2,3.57838172399998));
#303646=CARTESIAN_POINT('Ctrl Pts',(-2.11283068000006,12.2,3.57931798199999));
#303647=CARTESIAN_POINT('Ctrl Pts',(-2.11283068000006,5.2,3.57931798199999));
#303648=CARTESIAN_POINT('Ctrl Pts',(-2.11283068000006,2.2,3.57931798199999));
#303649=CARTESIAN_POINT('Ctrl Pts',(-2.11382552700006,12.2,3.58025643499998));
#303650=CARTESIAN_POINT('Ctrl Pts',(-2.11382552700006,5.2,3.58025643499998));
#303651=CARTESIAN_POINT('Ctrl Pts',(-2.11382552700006,2.2,3.58025643499998));
#303652=CARTESIAN_POINT('Ctrl Pts',(-2.11482505400005,12.2,3.58119706899998));
#303653=CARTESIAN_POINT('Ctrl Pts',(-2.11482505400005,5.2,3.58119706899998));
#303654=CARTESIAN_POINT('Ctrl Pts',(-2.11482505400005,2.2,3.58119706899998));
#303655=CARTESIAN_POINT('Ctrl Pts',(-2.11582926500005,12.2,3.58213986899998));
#303656=CARTESIAN_POINT('Ctrl Pts',(-2.11582926500005,5.2,3.58213986899998));
#303657=CARTESIAN_POINT('Ctrl Pts',(-2.11582926500005,2.2,3.58213986899998));
#303658=CARTESIAN_POINT('Ctrl Pts',(-2.11683815900006,12.2,3.58308482299999));
#303659=CARTESIAN_POINT('Ctrl Pts',(-2.11683815900006,5.2,3.58308482299999));
#303660=CARTESIAN_POINT('Ctrl Pts',(-2.11683815900006,2.2,3.58308482299999));
#303661=CARTESIAN_POINT('Ctrl Pts',(-2.11785173800005,12.2,3.58403191499999));
#303662=CARTESIAN_POINT('Ctrl Pts',(-2.11785173800005,5.2,3.58403191499999));
#303663=CARTESIAN_POINT('Ctrl Pts',(-2.11785173800005,2.2,3.58403191499999));
#303664=CARTESIAN_POINT('Ctrl Pts',(-2.11887000200006,12.2,3.58498113199998));
#303665=CARTESIAN_POINT('Ctrl Pts',(-2.11887000200006,5.2,3.58498113199998));
#303666=CARTESIAN_POINT('Ctrl Pts',(-2.11887000200006,2.2,3.58498113199998));
#303667=CARTESIAN_POINT('Ctrl Pts',(-2.11989295200006,12.2,3.58593245999998));
#303668=CARTESIAN_POINT('Ctrl Pts',(-2.11989295200006,5.2,3.58593245999998));
#303669=CARTESIAN_POINT('Ctrl Pts',(-2.11989295200006,2.2,3.58593245999998));
#303670=CARTESIAN_POINT('Ctrl Pts',(-2.12092058700006,12.2,3.58688588399998));
#303671=CARTESIAN_POINT('Ctrl Pts',(-2.12092058700006,5.2,3.58688588399998));
#303672=CARTESIAN_POINT('Ctrl Pts',(-2.12092058700006,2.2,3.58688588399998));
#303673=CARTESIAN_POINT('Ctrl Pts',(-2.12195291000006,12.2,3.58784139099999));
#303674=CARTESIAN_POINT('Ctrl Pts',(-2.12195291000006,5.2,3.58784139099999));
#303675=CARTESIAN_POINT('Ctrl Pts',(-2.12195291000006,2.2,3.58784139099999));
#303676=CARTESIAN_POINT('Ctrl Pts',(-2.12298992100005,12.2,3.58879896799999));
#303677=CARTESIAN_POINT('Ctrl Pts',(-2.12298992100005,5.2,3.58879896799999));
#303678=CARTESIAN_POINT('Ctrl Pts',(-2.12298992100005,2.2,3.58879896799999));
#303679=CARTESIAN_POINT('Ctrl Pts',(-2.12403161800006,12.2,3.58975859899999));
#303680=CARTESIAN_POINT('Ctrl Pts',(-2.12403161800006,5.2,3.58975859899999));
#303681=CARTESIAN_POINT('Ctrl Pts',(-2.12403161800006,2.2,3.58975859899999));
#303682=CARTESIAN_POINT('Ctrl Pts',(-2.12507800500005,12.2,3.59072027199999));
#303683=CARTESIAN_POINT('Ctrl Pts',(-2.12507800500005,5.2,3.59072027199999));
#303684=CARTESIAN_POINT('Ctrl Pts',(-2.12507800500005,2.2,3.59072027199999));
#303685=CARTESIAN_POINT('Ctrl Pts',(-2.12612908200006,12.2,3.59168397199999));
#303686=CARTESIAN_POINT('Ctrl Pts',(-2.12612908200006,5.2,3.59168397199999));
#303687=CARTESIAN_POINT('Ctrl Pts',(-2.12612908200006,2.2,3.59168397199999));
#303688=CARTESIAN_POINT('Ctrl Pts',(-2.12718484700006,12.2,3.59264968499998));
#303689=CARTESIAN_POINT('Ctrl Pts',(-2.12718484700006,5.2,3.59264968499998));
#303690=CARTESIAN_POINT('Ctrl Pts',(-2.12718484700006,2.2,3.59264968499998));
#303691=CARTESIAN_POINT('Ctrl Pts',(-2.12824530300006,12.2,3.59361739899998));
#303692=CARTESIAN_POINT('Ctrl Pts',(-2.12824530300006,5.2,3.59361739899998));
#303693=CARTESIAN_POINT('Ctrl Pts',(-2.12824530300006,2.2,3.59361739899998));
#303694=CARTESIAN_POINT('Ctrl Pts',(-2.12931045000006,12.2,3.59458709999998));
#303695=CARTESIAN_POINT('Ctrl Pts',(-2.12931045000006,5.2,3.59458709999998));
#303696=CARTESIAN_POINT('Ctrl Pts',(-2.12931045000006,2.2,3.59458709999998));
#303697=CARTESIAN_POINT('Ctrl Pts',(-2.13038028900006,12.2,3.59555877199998));
#303698=CARTESIAN_POINT('Ctrl Pts',(-2.13038028900006,5.2,3.59555877199998));
#303699=CARTESIAN_POINT('Ctrl Pts',(-2.13038028900006,2.2,3.59555877199998));
#303700=CARTESIAN_POINT('Ctrl Pts',(-2.13145481800006,12.2,3.59653240399999));
#303701=CARTESIAN_POINT('Ctrl Pts',(-2.13145481800006,5.2,3.59653240399999));
#303702=CARTESIAN_POINT('Ctrl Pts',(-2.13145481800006,2.2,3.59653240399999));
#303703=CARTESIAN_POINT('Ctrl Pts',(-2.13253404000006,12.2,3.59750797899999));
#303704=CARTESIAN_POINT('Ctrl Pts',(-2.13253404000006,5.2,3.59750797899999));
#303705=CARTESIAN_POINT('Ctrl Pts',(-2.13253404000006,2.2,3.59750797899999));
#303706=CARTESIAN_POINT('Ctrl Pts',(-2.13361795400006,12.2,3.59848548799999));
#303707=CARTESIAN_POINT('Ctrl Pts',(-2.13361795400006,5.2,3.59848548799999));
#303708=CARTESIAN_POINT('Ctrl Pts',(-2.13361795400006,2.2,3.59848548799999));
#303709=CARTESIAN_POINT('Ctrl Pts',(-2.13470656200006,12.2,3.59946491399998));
#303710=CARTESIAN_POINT('Ctrl Pts',(-2.13470656200006,5.2,3.59946491399998));
#303711=CARTESIAN_POINT('Ctrl Pts',(-2.13470656200006,2.2,3.59946491399998));
#303712=CARTESIAN_POINT('Ctrl Pts',(-2.13579986300005,12.2,3.60044624499999));
#303713=CARTESIAN_POINT('Ctrl Pts',(-2.13579986300005,5.2,3.60044624499999));
#303714=CARTESIAN_POINT('Ctrl Pts',(-2.13579986300005,2.2,3.60044624499999));
#303715=CARTESIAN_POINT('Ctrl Pts',(-2.13689785700006,12.2,3.60142946699998));
#303716=CARTESIAN_POINT('Ctrl Pts',(-2.13689785700006,5.2,3.60142946699998));
#303717=CARTESIAN_POINT('Ctrl Pts',(-2.13689785700006,2.2,3.60142946699998));
#303718=CARTESIAN_POINT('Ctrl Pts',(-2.13800054500005,12.2,3.60241456599999));
#303719=CARTESIAN_POINT('Ctrl Pts',(-2.13800054500005,5.2,3.60241456599999));
#303720=CARTESIAN_POINT('Ctrl Pts',(-2.13800054500005,2.2,3.60241456599999));
#303721=CARTESIAN_POINT('Ctrl Pts',(-2.13910792800006,12.2,3.60340152899998));
#303722=CARTESIAN_POINT('Ctrl Pts',(-2.13910792800006,5.2,3.60340152899998));
#303723=CARTESIAN_POINT('Ctrl Pts',(-2.13910792800006,2.2,3.60340152899998));
#303724=CARTESIAN_POINT('Ctrl Pts',(-2.14022000500006,12.2,3.60439034299999));
#303725=CARTESIAN_POINT('Ctrl Pts',(-2.14022000500006,5.2,3.60439034299999));
#303726=CARTESIAN_POINT('Ctrl Pts',(-2.14022000500006,2.2,3.60439034299999));
#303727=CARTESIAN_POINT('Ctrl Pts',(-2.14133677700006,12.2,3.60538099399999));
#303728=CARTESIAN_POINT('Ctrl Pts',(-2.14133677700006,5.2,3.60538099399999));
#303729=CARTESIAN_POINT('Ctrl Pts',(-2.14133677700006,2.2,3.60538099399999));
#303730=CARTESIAN_POINT('Ctrl Pts',(-2.14245824500006,12.2,3.60637346799999));
#303731=CARTESIAN_POINT('Ctrl Pts',(-2.14245824500006,5.2,3.60637346799999));
#303732=CARTESIAN_POINT('Ctrl Pts',(-2.14245824500006,2.2,3.60637346799999));
#303733=CARTESIAN_POINT('Ctrl Pts',(-2.14358440700006,12.2,3.60736775199998));
#303734=CARTESIAN_POINT('Ctrl Pts',(-2.14358440700006,5.2,3.60736775199998));
#303735=CARTESIAN_POINT('Ctrl Pts',(-2.14358440700006,2.2,3.60736775199998));
#303736=CARTESIAN_POINT('Ctrl Pts',(-2.14471526600006,12.2,3.60836383499999));
#303737=CARTESIAN_POINT('Ctrl Pts',(-2.14471526600006,5.2,3.60836383499999));
#303738=CARTESIAN_POINT('Ctrl Pts',(-2.14471526600006,2.2,3.60836383499999));
#303739=CARTESIAN_POINT('Ctrl Pts',(-2.14585082000006,12.2,3.60936169999999));
#303740=CARTESIAN_POINT('Ctrl Pts',(-2.14585082000006,5.2,3.60936169999999));
#303741=CARTESIAN_POINT('Ctrl Pts',(-2.14585082000006,2.2,3.60936169999999));
#303742=CARTESIAN_POINT('Ctrl Pts',(-2.14699107100006,12.2,3.61036133599999));
#303743=CARTESIAN_POINT('Ctrl Pts',(-2.14699107100006,5.2,3.61036133599999));
#303744=CARTESIAN_POINT('Ctrl Pts',(-2.14699107100006,2.2,3.61036133599999));
#303745=CARTESIAN_POINT('Ctrl Pts',(-2.14813601800006,12.2,3.61136272899999));
#303746=CARTESIAN_POINT('Ctrl Pts',(-2.14813601800006,5.2,3.61136272899999));
#303747=CARTESIAN_POINT('Ctrl Pts',(-2.14813601800006,2.2,3.61136272899999));
#303748=CARTESIAN_POINT('Ctrl Pts',(-2.14928566100005,12.2,3.61236586599999));
#303749=CARTESIAN_POINT('Ctrl Pts',(-2.14928566100005,5.2,3.61236586599999));
#303750=CARTESIAN_POINT('Ctrl Pts',(-2.14928566100005,2.2,3.61236586599999));
#303751=CARTESIAN_POINT('Ctrl Pts',(-2.15044000000006,12.2,3.61337073399999));
#303752=CARTESIAN_POINT('Ctrl Pts',(-2.15044000000006,5.2,3.61337073399999));
#303753=CARTESIAN_POINT('Ctrl Pts',(-2.15044000000006,2.2,3.61337073399999));
#303754=CARTESIAN_POINT('Ctrl Pts',(-2.15159903600005,12.2,3.61437731899999));
#303755=CARTESIAN_POINT('Ctrl Pts',(-2.15159903600005,5.2,3.61437731899999));
#303756=CARTESIAN_POINT('Ctrl Pts',(-2.15159903600005,2.2,3.61437731899999));
#303757=CARTESIAN_POINT('Ctrl Pts',(-2.15276276900005,12.2,3.61538560899999));
#303758=CARTESIAN_POINT('Ctrl Pts',(-2.15276276900005,5.2,3.61538560899999));
#303759=CARTESIAN_POINT('Ctrl Pts',(-2.15276276900005,2.2,3.61538560899999));
#303760=CARTESIAN_POINT('Ctrl Pts',(-2.15393119800006,12.2,3.61639558899999));
#303761=CARTESIAN_POINT('Ctrl Pts',(-2.15393119800006,5.2,3.61639558899999));
#303762=CARTESIAN_POINT('Ctrl Pts',(-2.15393119800006,2.2,3.61639558899999));
#303763=CARTESIAN_POINT('Ctrl Pts',(-2.15510432500006,12.2,3.61740724799999));
#303764=CARTESIAN_POINT('Ctrl Pts',(-2.15510432500006,5.2,3.61740724799999));
#303765=CARTESIAN_POINT('Ctrl Pts',(-2.15510432500006,2.2,3.61740724799999));
#303766=CARTESIAN_POINT('Ctrl Pts',(-2.15628214900006,12.2,3.61842057199999));
#303767=CARTESIAN_POINT('Ctrl Pts',(-2.15628214900006,5.2,3.61842057199999));
#303768=CARTESIAN_POINT('Ctrl Pts',(-2.15628214900006,2.2,3.61842057199999));
#303769=CARTESIAN_POINT('Ctrl Pts',(-2.15746466900006,12.2,3.61943554799999));
#303770=CARTESIAN_POINT('Ctrl Pts',(-2.15746466900006,5.2,3.61943554799999));
#303771=CARTESIAN_POINT('Ctrl Pts',(-2.15746466900006,2.2,3.61943554799999));
#303772=CARTESIAN_POINT('Ctrl Pts',(-2.15865188700006,12.2,3.62045216299999));
#303773=CARTESIAN_POINT('Ctrl Pts',(-2.15865188700006,5.2,3.62045216299999));
#303774=CARTESIAN_POINT('Ctrl Pts',(-2.15865188700006,2.2,3.62045216299999));
#303775=CARTESIAN_POINT('Ctrl Pts',(-2.15984380100006,12.2,3.62147040399999));
#303776=CARTESIAN_POINT('Ctrl Pts',(-2.15984380100006,5.2,3.62147040399999));
#303777=CARTESIAN_POINT('Ctrl Pts',(-2.15984380100006,2.2,3.62147040399999));
#303778=CARTESIAN_POINT('Ctrl Pts',(-2.16104041300006,12.2,3.62249025699998));
#303779=CARTESIAN_POINT('Ctrl Pts',(-2.16104041300006,5.2,3.62249025699998));
#303780=CARTESIAN_POINT('Ctrl Pts',(-2.16104041300006,2.2,3.62249025699998));
#303781=CARTESIAN_POINT('Ctrl Pts',(-2.16224172200006,12.2,3.62351171199998));
#303782=CARTESIAN_POINT('Ctrl Pts',(-2.16224172200006,5.2,3.62351171199998));
#303783=CARTESIAN_POINT('Ctrl Pts',(-2.16224172200006,2.2,3.62351171199998));
#303784=CARTESIAN_POINT('Ctrl Pts',(-2.16344772600006,12.2,3.62453475299999));
#303785=CARTESIAN_POINT('Ctrl Pts',(-2.16344772600006,5.2,3.62453475299999));
#303786=CARTESIAN_POINT('Ctrl Pts',(-2.16344772600006,2.2,3.62453475299999));
#303787=CARTESIAN_POINT('Ctrl Pts',(-2.16465842900006,12.2,3.62555936799998));
#303788=CARTESIAN_POINT('Ctrl Pts',(-2.16465842900006,5.2,3.62555936799998));
#303789=CARTESIAN_POINT('Ctrl Pts',(-2.16465842900006,2.2,3.62555936799998));
#303790=CARTESIAN_POINT('Ctrl Pts',(-2.16587382700005,12.2,3.62658554399999));
#303791=CARTESIAN_POINT('Ctrl Pts',(-2.16587382700005,5.2,3.62658554399999));
#303792=CARTESIAN_POINT('Ctrl Pts',(-2.16587382700005,2.2,3.62658554399999));
#303793=CARTESIAN_POINT('Ctrl Pts',(-2.16709392200006,12.2,3.62761326999999));
#303794=CARTESIAN_POINT('Ctrl Pts',(-2.16709392200006,5.2,3.62761326999999));
#303795=CARTESIAN_POINT('Ctrl Pts',(-2.16709392200006,2.2,3.62761326999999));
#303796=CARTESIAN_POINT('Ctrl Pts',(-2.16831871400006,12.2,3.62864252999999));
#303797=CARTESIAN_POINT('Ctrl Pts',(-2.16831871400006,5.2,3.62864252999999));
#303798=CARTESIAN_POINT('Ctrl Pts',(-2.16831871400006,2.2,3.62864252999999));
#303799=CARTESIAN_POINT('Ctrl Pts',(-2.16954820200006,12.2,3.62967331299998));
#303800=CARTESIAN_POINT('Ctrl Pts',(-2.16954820200006,5.2,3.62967331299998));
#303801=CARTESIAN_POINT('Ctrl Pts',(-2.16954820200006,2.2,3.62967331299998));
#303802=CARTESIAN_POINT('Ctrl Pts',(-2.17078238700006,12.2,3.63070560699998));
#303803=CARTESIAN_POINT('Ctrl Pts',(-2.17078238700006,5.2,3.63070560699998));
#303804=CARTESIAN_POINT('Ctrl Pts',(-2.17078238700006,2.2,3.63070560699998));
#303805=CARTESIAN_POINT('Ctrl Pts',(-2.17202126700006,12.2,3.63173939899998));
#303806=CARTESIAN_POINT('Ctrl Pts',(-2.17202126700006,5.2,3.63173939899998));
#303807=CARTESIAN_POINT('Ctrl Pts',(-2.17202126700006,2.2,3.63173939899998));
#303808=CARTESIAN_POINT('Ctrl Pts',(-2.17326484300005,12.2,3.63277467399998));
#303809=CARTESIAN_POINT('Ctrl Pts',(-2.17326484300005,5.2,3.63277467399998));
#303810=CARTESIAN_POINT('Ctrl Pts',(-2.17326484300005,2.2,3.63277467399998));
#303811=CARTESIAN_POINT('Ctrl Pts',(-2.17451311500006,12.2,3.63381142099998));
#303812=CARTESIAN_POINT('Ctrl Pts',(-2.17451311500006,5.2,3.63381142099998));
#303813=CARTESIAN_POINT('Ctrl Pts',(-2.17451311500006,2.2,3.63381142099998));
#303814=CARTESIAN_POINT('Ctrl Pts',(-2.17576608200006,12.2,3.63484962799999));
#303815=CARTESIAN_POINT('Ctrl Pts',(-2.17576608200006,5.2,3.63484962799999));
#303816=CARTESIAN_POINT('Ctrl Pts',(-2.17576608200006,2.2,3.63484962799999));
#303817=CARTESIAN_POINT('Ctrl Pts',(-2.17702374500006,12.2,3.63588928099999));
#303818=CARTESIAN_POINT('Ctrl Pts',(-2.17702374500006,5.2,3.63588928099999));
#303819=CARTESIAN_POINT('Ctrl Pts',(-2.17702374500006,2.2,3.63588928099999));
#303820=CARTESIAN_POINT('Ctrl Pts',(-2.17828610200006,12.2,3.63693036799998));
#303821=CARTESIAN_POINT('Ctrl Pts',(-2.17828610200006,5.2,3.63693036799998));
#303822=CARTESIAN_POINT('Ctrl Pts',(-2.17828610200006,2.2,3.63693036799998));
#303823=CARTESIAN_POINT('Ctrl Pts',(-2.17955315300005,12.2,3.63797287599999));
#303824=CARTESIAN_POINT('Ctrl Pts',(-2.17955315300005,5.2,3.63797287599999));
#303825=CARTESIAN_POINT('Ctrl Pts',(-2.17955315300005,2.2,3.63797287599999));
#303826=CARTESIAN_POINT('Ctrl Pts',(-2.18082490000006,12.2,3.63901679299998));
#303827=CARTESIAN_POINT('Ctrl Pts',(-2.18082490000006,5.2,3.63901679299998));
#303828=CARTESIAN_POINT('Ctrl Pts',(-2.18082490000006,2.2,3.63901679299998));
#303829=CARTESIAN_POINT('Ctrl Pts',(-2.18210134000006,12.2,3.64006210699999));
#303830=CARTESIAN_POINT('Ctrl Pts',(-2.18210134000006,5.2,3.64006210699999));
#303831=CARTESIAN_POINT('Ctrl Pts',(-2.18210134000006,2.2,3.64006210699999));
#303832=CARTESIAN_POINT('Ctrl Pts',(-2.18338247300006,12.2,3.64110880499998));
#303833=CARTESIAN_POINT('Ctrl Pts',(-2.18338247300006,5.2,3.64110880499998));
#303834=CARTESIAN_POINT('Ctrl Pts',(-2.18338247300006,2.2,3.64110880499998));
#303835=CARTESIAN_POINT('Ctrl Pts',(-2.18466830000006,12.2,3.64215687199999));
#303836=CARTESIAN_POINT('Ctrl Pts',(-2.18466830000006,5.2,3.64215687199999));
#303837=CARTESIAN_POINT('Ctrl Pts',(-2.18466830000006,2.2,3.64215687199999));
#303838=CARTESIAN_POINT('Ctrl Pts',(-2.18595882000006,12.2,3.64320629899999));
#303839=CARTESIAN_POINT('Ctrl Pts',(-2.18595882000006,5.2,3.64320629899999));
#303840=CARTESIAN_POINT('Ctrl Pts',(-2.18595882000006,2.2,3.64320629899999));
#303841=CARTESIAN_POINT('Ctrl Pts',(-2.18725403300006,12.2,3.64425707199998));
#303842=CARTESIAN_POINT('Ctrl Pts',(-2.18725403300006,5.2,3.64425707199998));
#303843=CARTESIAN_POINT('Ctrl Pts',(-2.18725403300006,2.2,3.64425707199998));
#303844=CARTESIAN_POINT('Ctrl Pts',(-2.18855393700006,12.2,3.64530917899998));
#303845=CARTESIAN_POINT('Ctrl Pts',(-2.18855393700006,5.2,3.64530917899998));
#303846=CARTESIAN_POINT('Ctrl Pts',(-2.18855393700006,2.2,3.64530917899998));
#303847=CARTESIAN_POINT('Ctrl Pts',(-2.18985853500006,12.2,3.64636260699999));
#303848=CARTESIAN_POINT('Ctrl Pts',(-2.18985853500006,5.2,3.64636260699999));
#303849=CARTESIAN_POINT('Ctrl Pts',(-2.18985853500006,2.2,3.64636260699999));
#303850=CARTESIAN_POINT('Ctrl Pts',(-2.19116782200006,12.2,3.64741734399999));
#303851=CARTESIAN_POINT('Ctrl Pts',(-2.19116782200006,5.2,3.64741734399999));
#303852=CARTESIAN_POINT('Ctrl Pts',(-2.19116782200006,2.2,3.64741734399999));
#303853=CARTESIAN_POINT('Ctrl Pts',(-2.19248180100006,12.2,3.64847337799999));
#303854=CARTESIAN_POINT('Ctrl Pts',(-2.19248180100006,5.2,3.64847337799999));
#303855=CARTESIAN_POINT('Ctrl Pts',(-2.19248180100006,2.2,3.64847337799999));
#303856=CARTESIAN_POINT('Ctrl Pts',(-2.19380047100006,12.2,3.64953069599999));
#303857=CARTESIAN_POINT('Ctrl Pts',(-2.19380047100006,5.2,3.64953069599999));
#303858=CARTESIAN_POINT('Ctrl Pts',(-2.19380047100006,2.2,3.64953069599999));
#303859=CARTESIAN_POINT('Ctrl Pts',(-2.19512383000006,12.2,3.65058928599999));
#303860=CARTESIAN_POINT('Ctrl Pts',(-2.19512383000006,5.2,3.65058928599999));
#303861=CARTESIAN_POINT('Ctrl Pts',(-2.19512383000006,2.2,3.65058928599999));
#303862=CARTESIAN_POINT('Ctrl Pts',(-2.19645187900006,12.2,3.65164913499999));
#303863=CARTESIAN_POINT('Ctrl Pts',(-2.19645187900006,5.2,3.65164913499999));
#303864=CARTESIAN_POINT('Ctrl Pts',(-2.19645187900006,2.2,3.65164913499999));
#303865=CARTESIAN_POINT('Ctrl Pts',(-2.19778461700006,12.2,3.65271023199998));
#303866=CARTESIAN_POINT('Ctrl Pts',(-2.19778461700006,5.2,3.65271023199998));
#303867=CARTESIAN_POINT('Ctrl Pts',(-2.19778461700006,2.2,3.65271023199998));
#303868=CARTESIAN_POINT('Ctrl Pts',(-2.19912204400006,12.2,3.65377256399999));
#303869=CARTESIAN_POINT('Ctrl Pts',(-2.19912204400006,5.2,3.65377256399999));
#303870=CARTESIAN_POINT('Ctrl Pts',(-2.19912204400006,2.2,3.65377256399999));
#303871=CARTESIAN_POINT('Ctrl Pts',(-2.20046415900006,12.2,3.65483611899998));
#303872=CARTESIAN_POINT('Ctrl Pts',(-2.20046415900006,5.2,3.65483611899998));
#303873=CARTESIAN_POINT('Ctrl Pts',(-2.20046415900006,2.2,3.65483611899998));
#303874=CARTESIAN_POINT('Ctrl Pts',(-2.20181096100006,12.2,3.65590088399999));
#303875=CARTESIAN_POINT('Ctrl Pts',(-2.20181096100006,5.2,3.65590088399999));
#303876=CARTESIAN_POINT('Ctrl Pts',(-2.20181096100006,2.2,3.65590088399999));
#303877=CARTESIAN_POINT('Ctrl Pts',(-2.20316245000005,12.2,3.65696684799998));
#303878=CARTESIAN_POINT('Ctrl Pts',(-2.20316245000005,5.2,3.65696684799998));
#303879=CARTESIAN_POINT('Ctrl Pts',(-2.20316245000005,2.2,3.65696684799998));
#303880=CARTESIAN_POINT('Ctrl Pts',(-2.20451862500005,12.2,3.65803399899999));
#303881=CARTESIAN_POINT('Ctrl Pts',(-2.20451862500005,5.2,3.65803399899999));
#303882=CARTESIAN_POINT('Ctrl Pts',(-2.20451862500005,2.2,3.65803399899999));
#303883=CARTESIAN_POINT('Ctrl Pts',(-2.20587948700006,12.2,3.65910232399998));
#303884=CARTESIAN_POINT('Ctrl Pts',(-2.20587948700006,5.2,3.65910232399998));
#303885=CARTESIAN_POINT('Ctrl Pts',(-2.20587948700006,2.2,3.65910232399998));
#303886=CARTESIAN_POINT('Ctrl Pts',(-2.20724503300006,12.2,3.66017180999999));
#303887=CARTESIAN_POINT('Ctrl Pts',(-2.20724503300006,5.2,3.66017180999999));
#303888=CARTESIAN_POINT('Ctrl Pts',(-2.20724503300006,2.2,3.66017180999999));
#303889=CARTESIAN_POINT('Ctrl Pts',(-2.20861526400005,12.2,3.66124244699999));
#303890=CARTESIAN_POINT('Ctrl Pts',(-2.20861526400005,5.2,3.66124244699999));
#303891=CARTESIAN_POINT('Ctrl Pts',(-2.20861526400005,2.2,3.66124244699999));
#303892=CARTESIAN_POINT('Ctrl Pts',(-2.20999017900006,12.2,3.66231422099998));
#303893=CARTESIAN_POINT('Ctrl Pts',(-2.20999017900006,5.2,3.66231422099998));
#303894=CARTESIAN_POINT('Ctrl Pts',(-2.20999017900006,2.2,3.66231422099998));
#303895=CARTESIAN_POINT('Ctrl Pts',(-2.21136977600006,12.2,3.66338712199998));
#303896=CARTESIAN_POINT('Ctrl Pts',(-2.21136977600006,5.2,3.66338712199998));
#303897=CARTESIAN_POINT('Ctrl Pts',(-2.21136977600006,2.2,3.66338712199998));
#303898=CARTESIAN_POINT('Ctrl Pts',(-2.21275405700006,12.2,3.66446113599999));
#303899=CARTESIAN_POINT('Ctrl Pts',(-2.21275405700006,5.2,3.66446113599999));
#303900=CARTESIAN_POINT('Ctrl Pts',(-2.21275405700006,2.2,3.66446113599999));
#303901=CARTESIAN_POINT('Ctrl Pts',(-2.21414301900006,12.2,3.66553625199998));
#303902=CARTESIAN_POINT('Ctrl Pts',(-2.21414301900006,5.2,3.66553625199998));
#303903=CARTESIAN_POINT('Ctrl Pts',(-2.21414301900006,2.2,3.66553625199998));
#303904=CARTESIAN_POINT('Ctrl Pts',(-2.21553666200006,12.2,3.66661245899999));
#303905=CARTESIAN_POINT('Ctrl Pts',(-2.21553666200006,5.2,3.66661245899999));
#303906=CARTESIAN_POINT('Ctrl Pts',(-2.21553666200006,2.2,3.66661245899999));
#303907=CARTESIAN_POINT('Ctrl Pts',(-2.21693498600006,12.2,3.66768974299998));
#303908=CARTESIAN_POINT('Ctrl Pts',(-2.21693498600006,5.2,3.66768974299998));
#303909=CARTESIAN_POINT('Ctrl Pts',(-2.21693498600006,2.2,3.66768974299998));
#303910=CARTESIAN_POINT('Ctrl Pts',(-2.21833799000006,12.2,3.66876809299999));
#303911=CARTESIAN_POINT('Ctrl Pts',(-2.21833799000006,5.2,3.66876809299999));
#303912=CARTESIAN_POINT('Ctrl Pts',(-2.21833799000006,2.2,3.66876809299999));
#303913=CARTESIAN_POINT('Ctrl Pts',(-2.21974567200005,12.2,3.66984749699999));
#303914=CARTESIAN_POINT('Ctrl Pts',(-2.21974567200005,5.2,3.66984749699999));
#303915=CARTESIAN_POINT('Ctrl Pts',(-2.21974567200005,2.2,3.66984749699999));
#303916=CARTESIAN_POINT('Ctrl Pts',(-2.22115803300006,12.2,3.67092794299998));
#303917=CARTESIAN_POINT('Ctrl Pts',(-2.22115803300006,5.2,3.67092794299998));
#303918=CARTESIAN_POINT('Ctrl Pts',(-2.22115803300006,2.2,3.67092794299998));
#303919=CARTESIAN_POINT('Ctrl Pts',(-2.22257507100006,12.2,3.67200941999998));
#303920=CARTESIAN_POINT('Ctrl Pts',(-2.22257507100006,5.2,3.67200941999998));
#303921=CARTESIAN_POINT('Ctrl Pts',(-2.22257507100006,2.2,3.67200941999998));
#303922=CARTESIAN_POINT('Ctrl Pts',(-2.22399678600006,12.2,3.67309191499999));
#303923=CARTESIAN_POINT('Ctrl Pts',(-2.22399678600006,5.2,3.67309191499999));
#303924=CARTESIAN_POINT('Ctrl Pts',(-2.22399678600006,2.2,3.67309191499999));
#303925=CARTESIAN_POINT('Ctrl Pts',(-2.22542317600006,12.2,3.67417541699999));
#303926=CARTESIAN_POINT('Ctrl Pts',(-2.22542317600006,5.2,3.67417541699999));
#303927=CARTESIAN_POINT('Ctrl Pts',(-2.22542317600006,2.2,3.67417541699999));
#303928=CARTESIAN_POINT('Ctrl Pts',(-2.22685424200006,12.2,3.67525991399998));
#303929=CARTESIAN_POINT('Ctrl Pts',(-2.22685424200006,5.2,3.67525991399998));
#303930=CARTESIAN_POINT('Ctrl Pts',(-2.22685424200006,2.2,3.67525991399998));
#303931=CARTESIAN_POINT('Ctrl Pts',(-2.22828998300006,12.2,3.67634539399998));
#303932=CARTESIAN_POINT('Ctrl Pts',(-2.22828998300006,5.2,3.67634539399998));
#303933=CARTESIAN_POINT('Ctrl Pts',(-2.22828998300006,2.2,3.67634539399998));
#303934=CARTESIAN_POINT('Ctrl Pts',(-2.22973039500005,12.2,3.67743184499999));
#303935=CARTESIAN_POINT('Ctrl Pts',(-2.22973039500005,5.2,3.67743184499999));
#303936=CARTESIAN_POINT('Ctrl Pts',(-2.22973039500005,2.2,3.67743184499999));
#303937=CARTESIAN_POINT('Ctrl Pts',(-2.23117548100006,12.2,3.67851925599999));
#303938=CARTESIAN_POINT('Ctrl Pts',(-2.23117548100006,5.2,3.67851925599999));
#303939=CARTESIAN_POINT('Ctrl Pts',(-2.23117548100006,2.2,3.67851925599999));
#303940=CARTESIAN_POINT('Ctrl Pts',(-2.23262523900006,12.2,3.67960761499998));
#303941=CARTESIAN_POINT('Ctrl Pts',(-2.23262523900006,5.2,3.67960761499998));
#303942=CARTESIAN_POINT('Ctrl Pts',(-2.23262523900006,2.2,3.67960761499998));
#303943=CARTESIAN_POINT('Ctrl Pts',(-2.23407966600006,12.2,3.68069690999998));
#303944=CARTESIAN_POINT('Ctrl Pts',(-2.23407966600006,5.2,3.68069690999998));
#303945=CARTESIAN_POINT('Ctrl Pts',(-2.23407966600006,2.2,3.68069690999998));
#303946=CARTESIAN_POINT('Ctrl Pts',(-2.23553876500006,12.2,3.68178712899999));
#303947=CARTESIAN_POINT('Ctrl Pts',(-2.23553876500006,5.2,3.68178712899999));
#303948=CARTESIAN_POINT('Ctrl Pts',(-2.23553876500006,2.2,3.68178712899999));
#303949=CARTESIAN_POINT('Ctrl Pts',(-2.23700253100006,12.2,3.68287826199998));
#303950=CARTESIAN_POINT('Ctrl Pts',(-2.23700253100006,5.2,3.68287826199998));
#303951=CARTESIAN_POINT('Ctrl Pts',(-2.23700253100006,2.2,3.68287826199998));
#303952=CARTESIAN_POINT('Ctrl Pts',(-2.23847096600006,12.2,3.68397029499998));
#303953=CARTESIAN_POINT('Ctrl Pts',(-2.23847096600006,5.2,3.68397029499998));
#303954=CARTESIAN_POINT('Ctrl Pts',(-2.23847096600006,2.2,3.68397029499998));
#303955=CARTESIAN_POINT('Ctrl Pts',(-2.23994406800006,12.2,3.68506321899999));
#303956=CARTESIAN_POINT('Ctrl Pts',(-2.23994406800006,5.2,3.68506321899999));
#303957=CARTESIAN_POINT('Ctrl Pts',(-2.23994406800006,2.2,3.68506321899999));
#303958=CARTESIAN_POINT('Ctrl Pts',(-2.24142183500006,12.2,3.68615701999998));
#303959=CARTESIAN_POINT('Ctrl Pts',(-2.24142183500006,5.2,3.68615701999998));
#303960=CARTESIAN_POINT('Ctrl Pts',(-2.24142183500006,2.2,3.68615701999998));
#303961=CARTESIAN_POINT('Ctrl Pts',(-2.24290426800006,12.2,3.68725168899999));
#303962=CARTESIAN_POINT('Ctrl Pts',(-2.24290426800006,5.2,3.68725168899999));
#303963=CARTESIAN_POINT('Ctrl Pts',(-2.24290426800006,2.2,3.68725168899999));
#303964=CARTESIAN_POINT('Ctrl Pts',(-2.24439136500005,12.2,3.68834721199998));
#303965=CARTESIAN_POINT('Ctrl Pts',(-2.24439136500005,5.2,3.68834721199998));
#303966=CARTESIAN_POINT('Ctrl Pts',(-2.24439136500005,2.2,3.68834721199998));
#303967=CARTESIAN_POINT('Ctrl Pts',(-2.24588312600006,12.2,3.68944357799998));
#303968=CARTESIAN_POINT('Ctrl Pts',(-2.24588312600006,5.2,3.68944357799998));
#303969=CARTESIAN_POINT('Ctrl Pts',(-2.24588312600006,2.2,3.68944357799998));
#303970=CARTESIAN_POINT('Ctrl Pts',(-2.24737954800006,12.2,3.69054077599999));
#303971=CARTESIAN_POINT('Ctrl Pts',(-2.24737954800006,5.2,3.69054077599999));
#303972=CARTESIAN_POINT('Ctrl Pts',(-2.24737954800006,2.2,3.69054077599999));
#303973=CARTESIAN_POINT('Ctrl Pts',(-2.24888063100006,12.2,3.69163879499999));
#303974=CARTESIAN_POINT('Ctrl Pts',(-2.24888063100006,5.2,3.69163879499999));
#303975=CARTESIAN_POINT('Ctrl Pts',(-2.24888063100006,2.2,3.69163879499999));
#303976=CARTESIAN_POINT('Ctrl Pts',(-2.25038637400006,12.2,3.69273762399998));
#303977=CARTESIAN_POINT('Ctrl Pts',(-2.25038637400006,5.2,3.69273762399998));
#303978=CARTESIAN_POINT('Ctrl Pts',(-2.25038637400006,2.2,3.69273762399998));
#303979=CARTESIAN_POINT('Ctrl Pts',(-2.25189677600006,12.2,3.69383724899999));
#303980=CARTESIAN_POINT('Ctrl Pts',(-2.25189677600006,5.2,3.69383724899999));
#303981=CARTESIAN_POINT('Ctrl Pts',(-2.25189677600006,2.2,3.69383724899999));
#303982=CARTESIAN_POINT('Ctrl Pts',(-2.25341183700006,12.2,3.69493766099998));
#303983=CARTESIAN_POINT('Ctrl Pts',(-2.25341183700006,5.2,3.69493766099998));
#303984=CARTESIAN_POINT('Ctrl Pts',(-2.25341183700006,2.2,3.69493766099998));
#303985=CARTESIAN_POINT('Ctrl Pts',(-2.25493155300006,12.2,3.69603884699998));
#303986=CARTESIAN_POINT('Ctrl Pts',(-2.25493155300006,5.2,3.69603884699998));
#303987=CARTESIAN_POINT('Ctrl Pts',(-2.25493155300006,2.2,3.69603884699998));
#303988=CARTESIAN_POINT('Ctrl Pts',(-2.25645592500006,12.2,3.69714079599999));
#303989=CARTESIAN_POINT('Ctrl Pts',(-2.25645592500006,5.2,3.69714079599999));
#303990=CARTESIAN_POINT('Ctrl Pts',(-2.25645592500006,2.2,3.69714079599999));
#303991=CARTESIAN_POINT('Ctrl Pts',(-2.25798495200006,12.2,3.69824349899999));
#303992=CARTESIAN_POINT('Ctrl Pts',(-2.25798495200006,5.2,3.69824349899999));
#303993=CARTESIAN_POINT('Ctrl Pts',(-2.25798495200006,2.2,3.69824349899999));
#303994=CARTESIAN_POINT('Ctrl Pts',(-2.25951863300006,12.2,3.69934694199999));
#303995=CARTESIAN_POINT('Ctrl Pts',(-2.25951863300006,5.2,3.69934694199999));
#303996=CARTESIAN_POINT('Ctrl Pts',(-2.25951863300006,2.2,3.69934694199999));
#303997=CARTESIAN_POINT('Ctrl Pts',(-2.26105696600006,12.2,3.70045111299999));
#303998=CARTESIAN_POINT('Ctrl Pts',(-2.26105696600006,5.2,3.70045111299999));
#303999=CARTESIAN_POINT('Ctrl Pts',(-2.26105696600006,2.2,3.70045111299999));
#304000=CARTESIAN_POINT('Ctrl Pts',(-2.26259995000006,12.2,3.70155600399999));
#304001=CARTESIAN_POINT('Ctrl Pts',(-2.26259995000006,5.2,3.70155600399999));
#304002=CARTESIAN_POINT('Ctrl Pts',(-2.26259995000006,2.2,3.70155600399999));
#304003=CARTESIAN_POINT('Ctrl Pts',(-2.26414758400006,12.2,3.70266159999999));
#304004=CARTESIAN_POINT('Ctrl Pts',(-2.26414758400006,5.2,3.70266159999999));
#304005=CARTESIAN_POINT('Ctrl Pts',(-2.26414758400006,2.2,3.70266159999999));
#304006=CARTESIAN_POINT('Ctrl Pts',(-2.26569986700006,12.2,3.70376789299999));
#304007=CARTESIAN_POINT('Ctrl Pts',(-2.26569986700006,5.2,3.70376789299999));
#304008=CARTESIAN_POINT('Ctrl Pts',(-2.26569986700006,2.2,3.70376789299999));
#304009=CARTESIAN_POINT('Ctrl Pts',(-2.26725679800006,12.2,3.70487486999998));
#304010=CARTESIAN_POINT('Ctrl Pts',(-2.26725679800006,5.2,3.70487486999998));
#304011=CARTESIAN_POINT('Ctrl Pts',(-2.26725679800006,2.2,3.70487486999998));
#304012=CARTESIAN_POINT('Ctrl Pts',(-2.26881837400006,12.2,3.70598251999999));
#304013=CARTESIAN_POINT('Ctrl Pts',(-2.26881837400006,5.2,3.70598251999999));
#304014=CARTESIAN_POINT('Ctrl Pts',(-2.26881837400006,2.2,3.70598251999999));
#304015=CARTESIAN_POINT('Ctrl Pts',(-2.27038459700006,12.2,3.70709083299998));
#304016=CARTESIAN_POINT('Ctrl Pts',(-2.27038459700006,5.2,3.70709083299998));
#304017=CARTESIAN_POINT('Ctrl Pts',(-2.27038459700006,2.2,3.70709083299998));
#304018=CARTESIAN_POINT('Ctrl Pts',(-2.27195546200006,12.2,3.70819979599998));
#304019=CARTESIAN_POINT('Ctrl Pts',(-2.27195546200006,5.2,3.70819979599998));
#304020=CARTESIAN_POINT('Ctrl Pts',(-2.27195546200006,2.2,3.70819979599998));
#304021=CARTESIAN_POINT('Ctrl Pts',(-2.27353097200006,12.2,3.70930939799998));
#304022=CARTESIAN_POINT('Ctrl Pts',(-2.27353097200006,5.2,3.70930939799998));
#304023=CARTESIAN_POINT('Ctrl Pts',(-2.27353097200006,2.2,3.70930939799998));
#304024=CARTESIAN_POINT('Ctrl Pts',(-2.27511112200005,12.2,3.71041962899999));
#304025=CARTESIAN_POINT('Ctrl Pts',(-2.27511112200005,5.2,3.71041962899999));
#304026=CARTESIAN_POINT('Ctrl Pts',(-2.27511112200005,2.2,3.71041962899999));
#304027=CARTESIAN_POINT('Ctrl Pts',(-2.27669591200006,12.2,3.71153047699998));
#304028=CARTESIAN_POINT('Ctrl Pts',(-2.27669591200006,5.2,3.71153047699998));
#304029=CARTESIAN_POINT('Ctrl Pts',(-2.27669591200006,2.2,3.71153047699998));
#304030=CARTESIAN_POINT('Ctrl Pts',(-2.27828534100006,12.2,3.71264193299999));
#304031=CARTESIAN_POINT('Ctrl Pts',(-2.27828534100006,5.2,3.71264193299999));
#304032=CARTESIAN_POINT('Ctrl Pts',(-2.27828534100006,2.2,3.71264193299999));
#304033=CARTESIAN_POINT('Ctrl Pts',(-2.27987940700006,12.2,3.71375398199999));
#304034=CARTESIAN_POINT('Ctrl Pts',(-2.27987940700006,5.2,3.71375398199999));
#304035=CARTESIAN_POINT('Ctrl Pts',(-2.27987940700006,2.2,3.71375398199999));
#304036=CARTESIAN_POINT('Ctrl Pts',(-2.28147811000006,12.2,3.71486661699999));
#304037=CARTESIAN_POINT('Ctrl Pts',(-2.28147811000006,5.2,3.71486661699999));
#304038=CARTESIAN_POINT('Ctrl Pts',(-2.28147811000006,2.2,3.71486661699999));
#304039=CARTESIAN_POINT('Ctrl Pts',(-2.28308144900006,12.2,3.71597982399998));
#304040=CARTESIAN_POINT('Ctrl Pts',(-2.28308144900006,5.2,3.71597982399998));
#304041=CARTESIAN_POINT('Ctrl Pts',(-2.28308144900006,2.2,3.71597982399998));
#304042=CARTESIAN_POINT('Ctrl Pts',(-2.28468942000006,12.2,3.71709359399999));
#304043=CARTESIAN_POINT('Ctrl Pts',(-2.28468942000006,5.2,3.71709359399999));
#304044=CARTESIAN_POINT('Ctrl Pts',(-2.28468942000006,2.2,3.71709359399999));
#304045=CARTESIAN_POINT('Ctrl Pts',(-2.28630202400006,12.2,3.71820791499999));
#304046=CARTESIAN_POINT('Ctrl Pts',(-2.28630202400006,5.2,3.71820791499999));
#304047=CARTESIAN_POINT('Ctrl Pts',(-2.28630202400006,2.2,3.71820791499999));
#304048=CARTESIAN_POINT('Ctrl Pts',(-2.28791925900006,12.2,3.71932277699998));
#304049=CARTESIAN_POINT('Ctrl Pts',(-2.28791925900006,5.2,3.71932277699998));
#304050=CARTESIAN_POINT('Ctrl Pts',(-2.28791925900006,2.2,3.71932277699998));
#304051=CARTESIAN_POINT('Ctrl Pts',(-2.28954112300006,12.2,3.72043816699998));
#304052=CARTESIAN_POINT('Ctrl Pts',(-2.28954112300006,5.2,3.72043816699998));
#304053=CARTESIAN_POINT('Ctrl Pts',(-2.28954112300006,2.2,3.72043816699998));
#304054=CARTESIAN_POINT('Ctrl Pts',(-2.29116761500006,12.2,3.72155407499999));
#304055=CARTESIAN_POINT('Ctrl Pts',(-2.29116761500006,5.2,3.72155407499999));
#304056=CARTESIAN_POINT('Ctrl Pts',(-2.29116761500006,2.2,3.72155407499999));
#304057=CARTESIAN_POINT('Ctrl Pts',(-2.29279873500006,12.2,3.72267049199999));
#304058=CARTESIAN_POINT('Ctrl Pts',(-2.29279873500006,5.2,3.72267049199999));
#304059=CARTESIAN_POINT('Ctrl Pts',(-2.29279873500006,2.2,3.72267049199999));
#304060=CARTESIAN_POINT('Ctrl Pts',(-2.29443447900006,12.2,3.72378740399999));
#304061=CARTESIAN_POINT('Ctrl Pts',(-2.29443447900006,5.2,3.72378740399999));
#304062=CARTESIAN_POINT('Ctrl Pts',(-2.29443447900006,2.2,3.72378740399999));
#304063=CARTESIAN_POINT('Ctrl Pts',(-2.29607484800006,12.2,3.72490480199998));
#304064=CARTESIAN_POINT('Ctrl Pts',(-2.29607484800006,5.2,3.72490480199998));
#304065=CARTESIAN_POINT('Ctrl Pts',(-2.29607484800006,2.2,3.72490480199998));
#304066=CARTESIAN_POINT('Ctrl Pts',(-2.29771983800005,12.2,3.72602267599999));
#304067=CARTESIAN_POINT('Ctrl Pts',(-2.29771983800005,5.2,3.72602267599999));
#304068=CARTESIAN_POINT('Ctrl Pts',(-2.29771983800005,2.2,3.72602267599999));
#304069=CARTESIAN_POINT('Ctrl Pts',(-2.29936945000006,12.2,3.72714101299999));
#304070=CARTESIAN_POINT('Ctrl Pts',(-2.29936945000006,5.2,3.72714101299999));
#304071=CARTESIAN_POINT('Ctrl Pts',(-2.29936945000006,2.2,3.72714101299999));
#304072=CARTESIAN_POINT('Ctrl Pts',(-2.30102368200006,12.2,3.72825980299999));
#304073=CARTESIAN_POINT('Ctrl Pts',(-2.30102368200006,5.2,3.72825980299999));
#304074=CARTESIAN_POINT('Ctrl Pts',(-2.30102368200006,2.2,3.72825980299999));
#304075=CARTESIAN_POINT('Ctrl Pts',(-2.30268253100005,12.2,3.72937903599999));
#304076=CARTESIAN_POINT('Ctrl Pts',(-2.30268253100005,5.2,3.72937903599999));
#304077=CARTESIAN_POINT('Ctrl Pts',(-2.30268253100005,2.2,3.72937903599999));
#304078=CARTESIAN_POINT('Ctrl Pts',(-2.30434599700006,12.2,3.73049869999999));
#304079=CARTESIAN_POINT('Ctrl Pts',(-2.30434599700006,5.2,3.73049869999999));
#304080=CARTESIAN_POINT('Ctrl Pts',(-2.30434599700006,2.2,3.73049869999999));
#304081=CARTESIAN_POINT('Ctrl Pts',(-2.30601407800005,12.2,3.73161878499998));
#304082=CARTESIAN_POINT('Ctrl Pts',(-2.30601407800005,5.2,3.73161878499998));
#304083=CARTESIAN_POINT('Ctrl Pts',(-2.30601407800005,2.2,3.73161878499998));
#304084=CARTESIAN_POINT('Ctrl Pts',(-2.30768677300006,12.2,3.73273928099999));
#304085=CARTESIAN_POINT('Ctrl Pts',(-2.30768677300006,5.2,3.73273928099999));
#304086=CARTESIAN_POINT('Ctrl Pts',(-2.30768677300006,2.2,3.73273928099999));
#304087=CARTESIAN_POINT('Ctrl Pts',(-2.30936408000006,12.2,3.73386017499998));
#304088=CARTESIAN_POINT('Ctrl Pts',(-2.30936408000006,5.2,3.73386017499998));
#304089=CARTESIAN_POINT('Ctrl Pts',(-2.30936408000006,2.2,3.73386017499998));
#304090=CARTESIAN_POINT('Ctrl Pts',(-2.31104599700005,12.2,3.73498145799999));
#304091=CARTESIAN_POINT('Ctrl Pts',(-2.31104599700005,5.2,3.73498145799999));
#304092=CARTESIAN_POINT('Ctrl Pts',(-2.31104599700005,2.2,3.73498145799999));
#304093=CARTESIAN_POINT('Ctrl Pts',(-2.31273252300006,12.2,3.73610311999999));
#304094=CARTESIAN_POINT('Ctrl Pts',(-2.31273252300006,5.2,3.73610311999999));
#304095=CARTESIAN_POINT('Ctrl Pts',(-2.31273252300006,2.2,3.73610311999999));
#304096=CARTESIAN_POINT('Ctrl Pts',(-2.31442365600006,12.2,3.73722514799999));
#304097=CARTESIAN_POINT('Ctrl Pts',(-2.31442365600006,5.2,3.73722514799999));
#304098=CARTESIAN_POINT('Ctrl Pts',(-2.31442365600006,2.2,3.73722514799999));
#304099=CARTESIAN_POINT('Ctrl Pts',(-2.31611939500006,12.2,3.73834753399999));
#304100=CARTESIAN_POINT('Ctrl Pts',(-2.31611939500006,5.2,3.73834753399999));
#304101=CARTESIAN_POINT('Ctrl Pts',(-2.31611939500006,2.2,3.73834753399999));
#304102=CARTESIAN_POINT('Ctrl Pts',(-2.31781973900006,12.2,3.73947026499999));
#304103=CARTESIAN_POINT('Ctrl Pts',(-2.31781973900006,5.2,3.73947026499999));
#304104=CARTESIAN_POINT('Ctrl Pts',(-2.31781973900006,2.2,3.73947026499999));
#304105=CARTESIAN_POINT('Ctrl Pts',(-2.31952468500006,12.2,3.74059333199998));
#304106=CARTESIAN_POINT('Ctrl Pts',(-2.31952468500006,5.2,3.74059333199998));
#304107=CARTESIAN_POINT('Ctrl Pts',(-2.31952468500006,2.2,3.74059333199998));
#304108=CARTESIAN_POINT('Ctrl Pts',(-2.32123423200005,12.2,3.74171672399999));
#304109=CARTESIAN_POINT('Ctrl Pts',(-2.32123423200005,5.2,3.74171672399999));
#304110=CARTESIAN_POINT('Ctrl Pts',(-2.32123423200005,2.2,3.74171672399999));
#304111=CARTESIAN_POINT('Ctrl Pts',(-2.32294837900006,12.2,3.74284042999999));
#304112=CARTESIAN_POINT('Ctrl Pts',(-2.32294837900006,5.2,3.74284042999999));
#304113=CARTESIAN_POINT('Ctrl Pts',(-2.32294837900006,2.2,3.74284042999999));
#304114=CARTESIAN_POINT('Ctrl Pts',(-2.32466712300006,12.2,3.74396443999998));
#304115=CARTESIAN_POINT('Ctrl Pts',(-2.32466712300006,5.2,3.74396443999998));
#304116=CARTESIAN_POINT('Ctrl Pts',(-2.32466712300006,2.2,3.74396443999998));
#304117=CARTESIAN_POINT('Ctrl Pts',(-2.32639046300006,12.2,3.74508874299998));
#304118=CARTESIAN_POINT('Ctrl Pts',(-2.32639046300006,5.2,3.74508874299998));
#304119=CARTESIAN_POINT('Ctrl Pts',(-2.32639046300006,2.2,3.74508874299998));
#304120=CARTESIAN_POINT('Ctrl Pts',(-2.32811839800006,12.2,3.74621332899999));
#304121=CARTESIAN_POINT('Ctrl Pts',(-2.32811839800006,5.2,3.74621332899999));
#304122=CARTESIAN_POINT('Ctrl Pts',(-2.32811839800006,2.2,3.74621332899999));
#304123=CARTESIAN_POINT('Ctrl Pts',(-2.32985092500006,12.2,3.74733818699998));
#304124=CARTESIAN_POINT('Ctrl Pts',(-2.32985092500006,5.2,3.74733818699998));
#304125=CARTESIAN_POINT('Ctrl Pts',(-2.32985092500006,2.2,3.74733818699998));
#304126=CARTESIAN_POINT('Ctrl Pts',(-2.33158804400006,12.2,3.74846330799999));
#304127=CARTESIAN_POINT('Ctrl Pts',(-2.33158804400006,5.2,3.74846330799999));
#304128=CARTESIAN_POINT('Ctrl Pts',(-2.33158804400006,2.2,3.74846330799999));
#304129=CARTESIAN_POINT('Ctrl Pts',(-2.33332975200006,12.2,3.74958867799998));
#304130=CARTESIAN_POINT('Ctrl Pts',(-2.33332975200006,5.2,3.74958867799998));
#304131=CARTESIAN_POINT('Ctrl Pts',(-2.33332975200006,2.2,3.74958867799998));
#304132=CARTESIAN_POINT('Ctrl Pts',(-2.33507604800006,12.2,3.75071429099999));
#304133=CARTESIAN_POINT('Ctrl Pts',(-2.33507604800006,5.2,3.75071429099999));
#304134=CARTESIAN_POINT('Ctrl Pts',(-2.33507604800006,2.2,3.75071429099999));
#304135=CARTESIAN_POINT('Ctrl Pts',(-2.33682693000006,12.2,3.75184013399998));
#304136=CARTESIAN_POINT('Ctrl Pts',(-2.33682693000006,5.2,3.75184013399998));
#304137=CARTESIAN_POINT('Ctrl Pts',(-2.33682693000006,2.2,3.75184013399998));
#304138=CARTESIAN_POINT('Ctrl Pts',(-2.33858239600006,12.2,3.75296619599998));
#304139=CARTESIAN_POINT('Ctrl Pts',(-2.33858239600006,5.2,3.75296619599998));
#304140=CARTESIAN_POINT('Ctrl Pts',(-2.33858239600006,2.2,3.75296619599998));
#304141=CARTESIAN_POINT('Ctrl Pts',(-2.34034244400006,12.2,3.75409246799999));
#304142=CARTESIAN_POINT('Ctrl Pts',(-2.34034244400006,5.2,3.75409246799999));
#304143=CARTESIAN_POINT('Ctrl Pts',(-2.34034244400006,2.2,3.75409246799999));
#304144=CARTESIAN_POINT('Ctrl Pts',(-2.34210707400006,12.2,3.75521893999998));
#304145=CARTESIAN_POINT('Ctrl Pts',(-2.34210707400006,5.2,3.75521893999998));
#304146=CARTESIAN_POINT('Ctrl Pts',(-2.34210707400006,2.2,3.75521893999998));
#304147=CARTESIAN_POINT('Ctrl Pts',(-2.34387628200006,12.2,3.75634560099999));
#304148=CARTESIAN_POINT('Ctrl Pts',(-2.34387628200006,5.2,3.75634560099999));
#304149=CARTESIAN_POINT('Ctrl Pts',(-2.34387628200006,2.2,3.75634560099999));
#304150=CARTESIAN_POINT('Ctrl Pts',(-2.34565006800006,12.2,3.75747243999999));
#304151=CARTESIAN_POINT('Ctrl Pts',(-2.34565006800006,5.2,3.75747243999999));
#304152=CARTESIAN_POINT('Ctrl Pts',(-2.34565006800006,2.2,3.75747243999999));
#304153=CARTESIAN_POINT('Ctrl Pts',(-2.34742842800005,12.2,3.75859944799998));
#304154=CARTESIAN_POINT('Ctrl Pts',(-2.34742842800005,5.2,3.75859944799998));
#304155=CARTESIAN_POINT('Ctrl Pts',(-2.34742842800005,2.2,3.75859944799998));
#304156=CARTESIAN_POINT('Ctrl Pts',(-2.34921136300006,12.2,3.75972661399998));
#304157=CARTESIAN_POINT('Ctrl Pts',(-2.34921136300006,5.2,3.75972661399998));
#304158=CARTESIAN_POINT('Ctrl Pts',(-2.34921136300006,2.2,3.75972661399998));
#304159=CARTESIAN_POINT('Ctrl Pts',(-2.35099887000006,12.2,3.76085392699999));
#304160=CARTESIAN_POINT('Ctrl Pts',(-2.35099887000006,5.2,3.76085392699999));
#304161=CARTESIAN_POINT('Ctrl Pts',(-2.35099887000006,2.2,3.76085392699999));
#304162=CARTESIAN_POINT('Ctrl Pts',(-2.35279094600005,12.2,3.76198137799998));
#304163=CARTESIAN_POINT('Ctrl Pts',(-2.35279094600005,5.2,3.76198137799998));
#304164=CARTESIAN_POINT('Ctrl Pts',(-2.35279094600005,2.2,3.76198137799998));
#304165=CARTESIAN_POINT('Ctrl Pts',(-2.35458759100006,12.2,3.76310895699999));
#304166=CARTESIAN_POINT('Ctrl Pts',(-2.35458759100006,5.2,3.76310895699999));
#304167=CARTESIAN_POINT('Ctrl Pts',(-2.35458759100006,2.2,3.76310895699999));
#304168=CARTESIAN_POINT('Ctrl Pts',(-2.35638880100006,12.2,3.76423665199999));
#304169=CARTESIAN_POINT('Ctrl Pts',(-2.35638880100006,5.2,3.76423665199999));
#304170=CARTESIAN_POINT('Ctrl Pts',(-2.35638880100006,2.2,3.76423665199999));
#304171=CARTESIAN_POINT('Ctrl Pts',(-2.35819457700006,12.2,3.76536445399999));
#304172=CARTESIAN_POINT('Ctrl Pts',(-2.35819457700006,5.2,3.76536445399999));
#304173=CARTESIAN_POINT('Ctrl Pts',(-2.35819457700006,2.2,3.76536445399999));
#304174=CARTESIAN_POINT('Ctrl Pts',(-2.36000491500006,12.2,3.76649235399999));
#304175=CARTESIAN_POINT('Ctrl Pts',(-2.36000491500006,5.2,3.76649235399999));
#304176=CARTESIAN_POINT('Ctrl Pts',(-2.36000491500006,2.2,3.76649235399999));
#304177=CARTESIAN_POINT('Ctrl Pts',(-2.36181981300006,12.2,3.76762033899999));
#304178=CARTESIAN_POINT('Ctrl Pts',(-2.36181981300006,5.2,3.76762033899999));
#304179=CARTESIAN_POINT('Ctrl Pts',(-2.36181981300006,2.2,3.76762033899999));
#304180=CARTESIAN_POINT('Ctrl Pts',(-2.36363927100005,12.2,3.76874840099998));
#304181=CARTESIAN_POINT('Ctrl Pts',(-2.36363927100005,5.2,3.76874840099998));
#304182=CARTESIAN_POINT('Ctrl Pts',(-2.36363927100005,2.2,3.76874840099998));
#304183=CARTESIAN_POINT('Ctrl Pts',(-2.36546328500005,12.2,3.76987652899999));
#304184=CARTESIAN_POINT('Ctrl Pts',(-2.36546328500005,5.2,3.76987652899999));
#304185=CARTESIAN_POINT('Ctrl Pts',(-2.36546328500005,2.2,3.76987652899999));
#304186=CARTESIAN_POINT('Ctrl Pts',(-2.36729185500006,12.2,3.77100471299999));
#304187=CARTESIAN_POINT('Ctrl Pts',(-2.36729185500006,5.2,3.77100471299999));
#304188=CARTESIAN_POINT('Ctrl Pts',(-2.36729185500006,2.2,3.77100471299999));
#304189=CARTESIAN_POINT('Ctrl Pts',(-2.36912497900006,12.2,3.77213294399999));
#304190=CARTESIAN_POINT('Ctrl Pts',(-2.36912497900006,5.2,3.77213294399999));
#304191=CARTESIAN_POINT('Ctrl Pts',(-2.36912497900006,2.2,3.77213294399999));
#304192=CARTESIAN_POINT('Ctrl Pts',(-2.37096265200006,12.2,3.77326120999999));
#304193=CARTESIAN_POINT('Ctrl Pts',(-2.37096265200006,5.2,3.77326120999999));
#304194=CARTESIAN_POINT('Ctrl Pts',(-2.37096265200006,2.2,3.77326120999999));
#304195=CARTESIAN_POINT('Ctrl Pts',(-2.37280487500006,12.2,3.77438950199998));
#304196=CARTESIAN_POINT('Ctrl Pts',(-2.37280487500006,5.2,3.77438950199998));
#304197=CARTESIAN_POINT('Ctrl Pts',(-2.37280487500006,2.2,3.77438950199998));
#304198=CARTESIAN_POINT('Ctrl Pts',(-2.37465164600006,12.2,3.77551780999998));
#304199=CARTESIAN_POINT('Ctrl Pts',(-2.37465164600006,5.2,3.77551780999998));
#304200=CARTESIAN_POINT('Ctrl Pts',(-2.37465164600006,2.2,3.77551780999998));
#304201=CARTESIAN_POINT('Ctrl Pts',(-2.37650296200006,12.2,3.77664612399998));
#304202=CARTESIAN_POINT('Ctrl Pts',(-2.37650296200006,5.2,3.77664612399998));
#304203=CARTESIAN_POINT('Ctrl Pts',(-2.37650296200006,2.2,3.77664612399998));
#304204=CARTESIAN_POINT('Ctrl Pts',(-2.37835882100006,12.2,3.77777443399999));
#304205=CARTESIAN_POINT('Ctrl Pts',(-2.37835882100006,5.2,3.77777443399999));
#304206=CARTESIAN_POINT('Ctrl Pts',(-2.37835882100006,2.2,3.77777443399999));
#304207=CARTESIAN_POINT('Ctrl Pts',(-2.38021922100006,12.2,3.77890272899998));
#304208=CARTESIAN_POINT('Ctrl Pts',(-2.38021922100006,5.2,3.77890272899998));
#304209=CARTESIAN_POINT('Ctrl Pts',(-2.38021922100006,2.2,3.77890272899998));
#304210=CARTESIAN_POINT('Ctrl Pts',(-2.38208416100006,12.2,3.78003099999999));
#304211=CARTESIAN_POINT('Ctrl Pts',(-2.38208416100006,5.2,3.78003099999999));
#304212=CARTESIAN_POINT('Ctrl Pts',(-2.38208416100006,2.2,3.78003099999999));
#304213=CARTESIAN_POINT('Ctrl Pts',(-2.38395363900006,12.2,3.78115923799999));
#304214=CARTESIAN_POINT('Ctrl Pts',(-2.38395363900006,5.2,3.78115923799999));
#304215=CARTESIAN_POINT('Ctrl Pts',(-2.38395363900006,2.2,3.78115923799999));
#304216=CARTESIAN_POINT('Ctrl Pts',(-2.38582765100006,12.2,3.78228743199998));
#304217=CARTESIAN_POINT('Ctrl Pts',(-2.38582765100006,5.2,3.78228743199998));
#304218=CARTESIAN_POINT('Ctrl Pts',(-2.38582765100006,2.2,3.78228743199998));
#304219=CARTESIAN_POINT('Ctrl Pts',(-2.38770619700006,12.2,3.78341556999998));
#304220=CARTESIAN_POINT('Ctrl Pts',(-2.38770619700006,5.2,3.78341556999998));
#304221=CARTESIAN_POINT('Ctrl Pts',(-2.38770619700006,2.2,3.78341556999998));
#304222=CARTESIAN_POINT('Ctrl Pts',(-2.38958927400006,12.2,3.78454364599998));
#304223=CARTESIAN_POINT('Ctrl Pts',(-2.38958927400006,5.2,3.78454364599998));
#304224=CARTESIAN_POINT('Ctrl Pts',(-2.38958927400006,2.2,3.78454364599998));
#304225=CARTESIAN_POINT('Ctrl Pts',(-2.39147688100006,12.2,3.78567164799998));
#304226=CARTESIAN_POINT('Ctrl Pts',(-2.39147688100006,5.2,3.78567164799998));
#304227=CARTESIAN_POINT('Ctrl Pts',(-2.39147688100006,2.2,3.78567164799998));
#304228=CARTESIAN_POINT('Ctrl Pts',(-2.39336901400006,12.2,3.78679956599999));
#304229=CARTESIAN_POINT('Ctrl Pts',(-2.39336901400006,5.2,3.78679956599999));
#304230=CARTESIAN_POINT('Ctrl Pts',(-2.39336901400006,2.2,3.78679956599999));
#304231=CARTESIAN_POINT('Ctrl Pts',(-2.39526567400006,12.2,3.78792739099998));
#304232=CARTESIAN_POINT('Ctrl Pts',(-2.39526567400006,5.2,3.78792739099998));
#304233=CARTESIAN_POINT('Ctrl Pts',(-2.39526567400006,2.2,3.78792739099998));
#304234=CARTESIAN_POINT('Ctrl Pts',(-2.39716685500006,12.2,3.78905511199999));
#304235=CARTESIAN_POINT('Ctrl Pts',(-2.39716685500006,5.2,3.78905511199999));
#304236=CARTESIAN_POINT('Ctrl Pts',(-2.39716685500006,2.2,3.78905511199999));
#304237=CARTESIAN_POINT('Ctrl Pts',(-2.39907255800006,12.2,3.79018271999998));
#304238=CARTESIAN_POINT('Ctrl Pts',(-2.39907255800006,5.2,3.79018271999998));
#304239=CARTESIAN_POINT('Ctrl Pts',(-2.39907255800006,2.2,3.79018271999998));
#304240=CARTESIAN_POINT('Ctrl Pts',(-2.40098277900006,12.2,3.79131020599999));
#304241=CARTESIAN_POINT('Ctrl Pts',(-2.40098277900006,5.2,3.79131020599999));
#304242=CARTESIAN_POINT('Ctrl Pts',(-2.40098277900006,2.2,3.79131020599999));
#304243=CARTESIAN_POINT('Ctrl Pts',(-2.40289751700006,12.2,3.79243755799998));
#304244=CARTESIAN_POINT('Ctrl Pts',(-2.40289751700006,5.2,3.79243755799998));
#304245=CARTESIAN_POINT('Ctrl Pts',(-2.40289751700006,2.2,3.79243755799998));
#304246=CARTESIAN_POINT('Ctrl Pts',(-2.40481677100005,12.2,3.79356476899999));
#304247=CARTESIAN_POINT('Ctrl Pts',(-2.40481677100005,5.2,3.79356476899999));
#304248=CARTESIAN_POINT('Ctrl Pts',(-2.40481677100005,2.2,3.79356476899999));
#304249=CARTESIAN_POINT('Ctrl Pts',(-2.40674053600006,12.2,3.79469182699999));
#304250=CARTESIAN_POINT('Ctrl Pts',(-2.40674053600006,5.2,3.79469182699999));
#304251=CARTESIAN_POINT('Ctrl Pts',(-2.40674053600006,2.2,3.79469182699999));
#304252=CARTESIAN_POINT('Ctrl Pts',(-2.40866881100006,12.2,3.79581872299998));
#304253=CARTESIAN_POINT('Ctrl Pts',(-2.40866881100006,5.2,3.79581872299998));
#304254=CARTESIAN_POINT('Ctrl Pts',(-2.40866881100006,2.2,3.79581872299998));
#304255=CARTESIAN_POINT('Ctrl Pts',(-2.41060159600006,12.2,3.79694544699999));
#304256=CARTESIAN_POINT('Ctrl Pts',(-2.41060159600006,5.2,3.79694544699999));
#304257=CARTESIAN_POINT('Ctrl Pts',(-2.41060159600006,2.2,3.79694544699999));
#304258=CARTESIAN_POINT('Ctrl Pts',(-2.41253888500006,12.2,3.79807198999998));
#304259=CARTESIAN_POINT('Ctrl Pts',(-2.41253888500006,5.2,3.79807198999998));
#304260=CARTESIAN_POINT('Ctrl Pts',(-2.41253888500006,2.2,3.79807198999998));
#304261=CARTESIAN_POINT('Ctrl Pts',(-2.41448067900006,12.2,3.79919834299999));
#304262=CARTESIAN_POINT('Ctrl Pts',(-2.41448067900006,5.2,3.79919834299999));
#304263=CARTESIAN_POINT('Ctrl Pts',(-2.41448067900006,2.2,3.79919834299999));
#304264=CARTESIAN_POINT('Ctrl Pts',(-2.41642697400006,12.2,3.80032449399998));
#304265=CARTESIAN_POINT('Ctrl Pts',(-2.41642697400006,5.2,3.80032449399998));
#304266=CARTESIAN_POINT('Ctrl Pts',(-2.41642697400006,2.2,3.80032449399998));
#304267=CARTESIAN_POINT('Ctrl Pts',(-2.41837776900006,12.2,3.80145043399998));
#304268=CARTESIAN_POINT('Ctrl Pts',(-2.41837776900006,5.2,3.80145043399998));
#304269=CARTESIAN_POINT('Ctrl Pts',(-2.41837776900006,2.2,3.80145043399998));
#304270=CARTESIAN_POINT('Ctrl Pts',(-2.42033306000006,12.2,3.80257615499998));
#304271=CARTESIAN_POINT('Ctrl Pts',(-2.42033306000006,5.2,3.80257615499998));
#304272=CARTESIAN_POINT('Ctrl Pts',(-2.42033306000006,2.2,3.80257615499998));
#304273=CARTESIAN_POINT('Ctrl Pts',(-2.42229284800006,12.2,3.80370164699999));
#304274=CARTESIAN_POINT('Ctrl Pts',(-2.42229284800006,5.2,3.80370164699999));
#304275=CARTESIAN_POINT('Ctrl Pts',(-2.42229284800006,2.2,3.80370164699999));
#304276=CARTESIAN_POINT('Ctrl Pts',(-2.42425712700005,12.2,3.80482689899999));
#304277=CARTESIAN_POINT('Ctrl Pts',(-2.42425712700005,5.2,3.80482689899999));
#304278=CARTESIAN_POINT('Ctrl Pts',(-2.42425712700005,2.2,3.80482689899999));
#304279=CARTESIAN_POINT('Ctrl Pts',(-2.42622589800006,12.2,3.80595190299999));
#304280=CARTESIAN_POINT('Ctrl Pts',(-2.42622589800006,5.2,3.80595190299999));
#304281=CARTESIAN_POINT('Ctrl Pts',(-2.42622589800006,2.2,3.80595190299999));
#304282=CARTESIAN_POINT('Ctrl Pts',(-2.42819915600006,12.2,3.80707664799999));
#304283=CARTESIAN_POINT('Ctrl Pts',(-2.42819915600006,5.2,3.80707664799999));
#304284=CARTESIAN_POINT('Ctrl Pts',(-2.42819915600006,2.2,3.80707664799999));
#304285=CARTESIAN_POINT('Ctrl Pts',(-2.43017690100006,12.2,3.80820112499999));
#304286=CARTESIAN_POINT('Ctrl Pts',(-2.43017690100006,5.2,3.80820112499999));
#304287=CARTESIAN_POINT('Ctrl Pts',(-2.43017690100006,2.2,3.80820112499999));
#304288=CARTESIAN_POINT('Ctrl Pts',(-2.43215912900005,12.2,3.80932532399999));
#304289=CARTESIAN_POINT('Ctrl Pts',(-2.43215912900005,5.2,3.80932532399999));
#304290=CARTESIAN_POINT('Ctrl Pts',(-2.43215912900005,2.2,3.80932532399999));
#304291=CARTESIAN_POINT('Ctrl Pts',(-2.43414584000006,12.2,3.81044923799998));
#304292=CARTESIAN_POINT('Ctrl Pts',(-2.43414584000006,5.2,3.81044923799998));
#304293=CARTESIAN_POINT('Ctrl Pts',(-2.43414584000006,2.2,3.81044923799998));
#304294=CARTESIAN_POINT('Ctrl Pts',(-2.43613703000006,12.2,3.81157285399999));
#304295=CARTESIAN_POINT('Ctrl Pts',(-2.43613703000006,5.2,3.81157285399999));
#304296=CARTESIAN_POINT('Ctrl Pts',(-2.43613703000006,2.2,3.81157285399999));
#304297=CARTESIAN_POINT('Ctrl Pts',(-2.43813269600006,12.2,3.81269616399998));
#304298=CARTESIAN_POINT('Ctrl Pts',(-2.43813269600006,5.2,3.81269616399998));
#304299=CARTESIAN_POINT('Ctrl Pts',(-2.43813269600006,2.2,3.81269616399998));
#304300=CARTESIAN_POINT('Ctrl Pts',(-2.44013283600006,12.2,3.81381915999999));
#304301=CARTESIAN_POINT('Ctrl Pts',(-2.44013283600006,5.2,3.81381915999999));
#304302=CARTESIAN_POINT('Ctrl Pts',(-2.44013283600006,2.2,3.81381915999999));
#304303=CARTESIAN_POINT('Ctrl Pts',(-2.44213745000006,12.2,3.81494182999998));
#304304=CARTESIAN_POINT('Ctrl Pts',(-2.44213745000006,5.2,3.81494182999998));
#304305=CARTESIAN_POINT('Ctrl Pts',(-2.44213745000006,2.2,3.81494182999998));
#304306=CARTESIAN_POINT('Ctrl Pts',(-2.44414653200006,12.2,3.81606416499999));
#304307=CARTESIAN_POINT('Ctrl Pts',(-2.44414653200006,5.2,3.81606416499999));
#304308=CARTESIAN_POINT('Ctrl Pts',(-2.44414653200006,2.2,3.81606416499999));
#304309=CARTESIAN_POINT('Ctrl Pts',(-2.44616008300006,12.2,3.81718615699998));
#304310=CARTESIAN_POINT('Ctrl Pts',(-2.44616008300006,5.2,3.81718615699998));
#304311=CARTESIAN_POINT('Ctrl Pts',(-2.44616008300006,2.2,3.81718615699998));
#304312=CARTESIAN_POINT('Ctrl Pts',(-2.44817810000006,12.2,3.81830779599999));
#304313=CARTESIAN_POINT('Ctrl Pts',(-2.44817810000006,5.2,3.81830779599999));
#304314=CARTESIAN_POINT('Ctrl Pts',(-2.44817810000006,2.2,3.81830779599999));
#304315=CARTESIAN_POINT('Ctrl Pts',(-2.45020057900006,12.2,3.81942907299998));
#304316=CARTESIAN_POINT('Ctrl Pts',(-2.45020057900006,5.2,3.81942907299998));
#304317=CARTESIAN_POINT('Ctrl Pts',(-2.45020057900006,2.2,3.81942907299998));
#304318=CARTESIAN_POINT('Ctrl Pts',(-2.45222751900006,12.2,3.82054997699999));
#304319=CARTESIAN_POINT('Ctrl Pts',(-2.45222751900006,5.2,3.82054997699999));
#304320=CARTESIAN_POINT('Ctrl Pts',(-2.45222751900006,2.2,3.82054997699999));
#304321=CARTESIAN_POINT('Ctrl Pts',(-2.45425891600005,12.2,3.82167049999998));
#304322=CARTESIAN_POINT('Ctrl Pts',(-2.45425891600005,5.2,3.82167049999998));
#304323=CARTESIAN_POINT('Ctrl Pts',(-2.45425891600005,2.2,3.82167049999998));
#304324=CARTESIAN_POINT('Ctrl Pts',(-2.45629477100006,12.2,3.82279063299999));
#304325=CARTESIAN_POINT('Ctrl Pts',(-2.45629477100006,5.2,3.82279063299999));
#304326=CARTESIAN_POINT('Ctrl Pts',(-2.45629477100006,2.2,3.82279063299999));
#304327=CARTESIAN_POINT('Ctrl Pts',(-2.45833507800006,12.2,3.82391036599999));
#304328=CARTESIAN_POINT('Ctrl Pts',(-2.45833507800006,5.2,3.82391036599999));
#304329=CARTESIAN_POINT('Ctrl Pts',(-2.45833507800006,2.2,3.82391036599999));
#304330=CARTESIAN_POINT('Ctrl Pts',(-2.46037983700006,12.2,3.82502968999999));
#304331=CARTESIAN_POINT('Ctrl Pts',(-2.46037983700006,5.2,3.82502968999999));
#304332=CARTESIAN_POINT('Ctrl Pts',(-2.46037983700006,2.2,3.82502968999999));
#304333=CARTESIAN_POINT('Ctrl Pts',(-2.46242904400006,12.2,3.82614859499999));
#304334=CARTESIAN_POINT('Ctrl Pts',(-2.46242904400006,5.2,3.82614859499999));
#304335=CARTESIAN_POINT('Ctrl Pts',(-2.46242904400006,2.2,3.82614859499999));
#304336=CARTESIAN_POINT('Ctrl Pts',(-2.46448269700006,12.2,3.82726707199998));
#304337=CARTESIAN_POINT('Ctrl Pts',(-2.46448269700006,5.2,3.82726707199998));
#304338=CARTESIAN_POINT('Ctrl Pts',(-2.46448269700006,2.2,3.82726707199998));
#304339=CARTESIAN_POINT('Ctrl Pts',(-2.46654079500006,12.2,3.82838511199999));
#304340=CARTESIAN_POINT('Ctrl Pts',(-2.46654079500006,5.2,3.82838511199999));
#304341=CARTESIAN_POINT('Ctrl Pts',(-2.46654079500006,2.2,3.82838511199999));
#304342=CARTESIAN_POINT('Ctrl Pts',(-2.46860333300006,12.2,3.82950270699999));
#304343=CARTESIAN_POINT('Ctrl Pts',(-2.46860333300006,5.2,3.82950270699999));
#304344=CARTESIAN_POINT('Ctrl Pts',(-2.46860333300006,2.2,3.82950270699999));
#304345=CARTESIAN_POINT('Ctrl Pts',(-2.47067031100006,12.2,3.83061984499999));
#304346=CARTESIAN_POINT('Ctrl Pts',(-2.47067031100006,5.2,3.83061984499999));
#304347=CARTESIAN_POINT('Ctrl Pts',(-2.47067031100006,2.2,3.83061984499999));
#304348=CARTESIAN_POINT('Ctrl Pts',(-2.47274172400005,12.2,3.83173651899998));
#304349=CARTESIAN_POINT('Ctrl Pts',(-2.47274172400005,5.2,3.83173651899998));
#304350=CARTESIAN_POINT('Ctrl Pts',(-2.47274172400005,2.2,3.83173651899998));
#304351=CARTESIAN_POINT('Ctrl Pts',(-2.47481757200006,12.2,3.83285271899998));
#304352=CARTESIAN_POINT('Ctrl Pts',(-2.47481757200006,5.2,3.83285271899998));
#304353=CARTESIAN_POINT('Ctrl Pts',(-2.47481757200006,2.2,3.83285271899998));
#304354=CARTESIAN_POINT('Ctrl Pts',(-2.47689785200006,12.2,3.83396843499998));
#304355=CARTESIAN_POINT('Ctrl Pts',(-2.47689785200006,5.2,3.83396843499998));
#304356=CARTESIAN_POINT('Ctrl Pts',(-2.47689785200006,2.2,3.83396843499998));
#304357=CARTESIAN_POINT('Ctrl Pts',(-2.47898256100005,12.2,3.83508365999998));
#304358=CARTESIAN_POINT('Ctrl Pts',(-2.47898256100005,5.2,3.83508365999998));
#304359=CARTESIAN_POINT('Ctrl Pts',(-2.47898256100005,2.2,3.83508365999998));
#304360=CARTESIAN_POINT('Ctrl Pts',(-2.48107169600006,12.2,3.83619838299998));
#304361=CARTESIAN_POINT('Ctrl Pts',(-2.48107169600006,5.2,3.83619838299998));
#304362=CARTESIAN_POINT('Ctrl Pts',(-2.48107169600006,2.2,3.83619838299998));
#304363=CARTESIAN_POINT('Ctrl Pts',(-2.48316525500006,12.2,3.83731259599998));
#304364=CARTESIAN_POINT('Ctrl Pts',(-2.48316525500006,5.2,3.83731259599998));
#304365=CARTESIAN_POINT('Ctrl Pts',(-2.48316525500006,2.2,3.83731259599998));
#304366=CARTESIAN_POINT('Ctrl Pts',(-2.48526323500006,12.2,3.83842628899998));
#304367=CARTESIAN_POINT('Ctrl Pts',(-2.48526323500006,5.2,3.83842628899998));
#304368=CARTESIAN_POINT('Ctrl Pts',(-2.48526323500006,2.2,3.83842628899998));
#304369=CARTESIAN_POINT('Ctrl Pts',(-2.48736563500006,12.2,3.83953945299999));
#304370=CARTESIAN_POINT('Ctrl Pts',(-2.48736563500006,5.2,3.83953945299999));
#304371=CARTESIAN_POINT('Ctrl Pts',(-2.48736563500006,2.2,3.83953945299999));
#304372=CARTESIAN_POINT('Ctrl Pts',(-2.48947245100006,12.2,3.84065207999999));
#304373=CARTESIAN_POINT('Ctrl Pts',(-2.48947245100006,5.2,3.84065207999999));
#304374=CARTESIAN_POINT('Ctrl Pts',(-2.48947245100006,2.2,3.84065207999999));
#304375=CARTESIAN_POINT('Ctrl Pts',(-2.49158368100006,12.2,3.84176415999999));
#304376=CARTESIAN_POINT('Ctrl Pts',(-2.49158368100006,5.2,3.84176415999999));
#304377=CARTESIAN_POINT('Ctrl Pts',(-2.49158368100006,2.2,3.84176415999999));
#304378=CARTESIAN_POINT('Ctrl Pts',(-2.49369932300006,12.2,3.84287568299998));
#304379=CARTESIAN_POINT('Ctrl Pts',(-2.49369932300006,5.2,3.84287568299998));
#304380=CARTESIAN_POINT('Ctrl Pts',(-2.49369932300006,2.2,3.84287568299998));
#304381=CARTESIAN_POINT('Ctrl Pts',(-2.49581937300006,12.2,3.84398664099999));
#304382=CARTESIAN_POINT('Ctrl Pts',(-2.49581937300006,5.2,3.84398664099999));
#304383=CARTESIAN_POINT('Ctrl Pts',(-2.49581937300006,2.2,3.84398664099999));
#304384=CARTESIAN_POINT('Ctrl Pts',(-2.49794383000005,12.2,3.84509702499999));
#304385=CARTESIAN_POINT('Ctrl Pts',(-2.49794383000005,5.2,3.84509702499999));
#304386=CARTESIAN_POINT('Ctrl Pts',(-2.49794383000005,2.2,3.84509702499999));
#304387=CARTESIAN_POINT('Ctrl Pts',(-2.50007269000006,12.2,3.84620682699998));
#304388=CARTESIAN_POINT('Ctrl Pts',(-2.50007269000006,5.2,3.84620682699998));
#304389=CARTESIAN_POINT('Ctrl Pts',(-2.50007269000006,2.2,3.84620682699998));
#304390=CARTESIAN_POINT('Ctrl Pts',(-2.50220595100005,12.2,3.84731603599998));
#304391=CARTESIAN_POINT('Ctrl Pts',(-2.50220595100005,5.2,3.84731603599998));
#304392=CARTESIAN_POINT('Ctrl Pts',(-2.50220595100005,2.2,3.84731603599998));
#304393=CARTESIAN_POINT('Ctrl Pts',(-2.50434361100006,12.2,3.84842464399998));
#304394=CARTESIAN_POINT('Ctrl Pts',(-2.50434361100006,5.2,3.84842464399998));
#304395=CARTESIAN_POINT('Ctrl Pts',(-2.50434361100006,2.2,3.84842464399998));
#304396=CARTESIAN_POINT('Ctrl Pts',(-2.50648566700006,12.2,3.84953264199999));
#304397=CARTESIAN_POINT('Ctrl Pts',(-2.50648566700006,5.2,3.84953264199999));
#304398=CARTESIAN_POINT('Ctrl Pts',(-2.50648566700006,2.2,3.84953264199999));
#304399=CARTESIAN_POINT('Ctrl Pts',(-2.50863211600006,12.2,3.85064002099998));
#304400=CARTESIAN_POINT('Ctrl Pts',(-2.50863211600006,5.2,3.85064002099998));
#304401=CARTESIAN_POINT('Ctrl Pts',(-2.50863211600006,2.2,3.85064002099998));
#304402=CARTESIAN_POINT('Ctrl Pts',(-2.51078295600006,12.2,3.85174677299998));
#304403=CARTESIAN_POINT('Ctrl Pts',(-2.51078295600006,5.2,3.85174677299998));
#304404=CARTESIAN_POINT('Ctrl Pts',(-2.51078295600006,2.2,3.85174677299998));
#304405=CARTESIAN_POINT('Ctrl Pts',(-2.51293818400006,12.2,3.85285288799999));
#304406=CARTESIAN_POINT('Ctrl Pts',(-2.51293818400006,5.2,3.85285288799999));
#304407=CARTESIAN_POINT('Ctrl Pts',(-2.51293818400006,2.2,3.85285288799999));
#304408=CARTESIAN_POINT('Ctrl Pts',(-2.51509779700006,12.2,3.85395835599999));
#304409=CARTESIAN_POINT('Ctrl Pts',(-2.51509779700006,5.2,3.85395835599999));
#304410=CARTESIAN_POINT('Ctrl Pts',(-2.51509779700006,2.2,3.85395835599999));
#304411=CARTESIAN_POINT('Ctrl Pts',(-2.51726179300006,12.2,3.85506317199999));
#304412=CARTESIAN_POINT('Ctrl Pts',(-2.51726179300006,5.2,3.85506317199999));
#304413=CARTESIAN_POINT('Ctrl Pts',(-2.51726179300006,2.2,3.85506317199999));
#304414=CARTESIAN_POINT('Ctrl Pts',(-2.51943016900006,12.2,3.85616732199999));
#304415=CARTESIAN_POINT('Ctrl Pts',(-2.51943016900006,5.2,3.85616732199999));
#304416=CARTESIAN_POINT('Ctrl Pts',(-2.51943016900006,2.2,3.85616732199999));
#304417=CARTESIAN_POINT('Ctrl Pts',(-2.52160292300006,12.2,3.85727079999998));
#304418=CARTESIAN_POINT('Ctrl Pts',(-2.52160292300006,5.2,3.85727079999998));
#304419=CARTESIAN_POINT('Ctrl Pts',(-2.52160292300006,2.2,3.85727079999998));
#304420=CARTESIAN_POINT('Ctrl Pts',(-2.52378005200006,12.2,3.85837359799999));
#304421=CARTESIAN_POINT('Ctrl Pts',(-2.52378005200006,5.2,3.85837359799999));
#304422=CARTESIAN_POINT('Ctrl Pts',(-2.52378005200006,2.2,3.85837359799999));
#304423=CARTESIAN_POINT('Ctrl Pts',(-2.52596155200006,12.2,3.85947570499999));
#304424=CARTESIAN_POINT('Ctrl Pts',(-2.52596155200006,5.2,3.85947570499999));
#304425=CARTESIAN_POINT('Ctrl Pts',(-2.52596155200006,2.2,3.85947570499999));
#304426=CARTESIAN_POINT('Ctrl Pts',(-2.52814742100006,12.2,3.86057711399998));
#304427=CARTESIAN_POINT('Ctrl Pts',(-2.52814742100006,5.2,3.86057711399998));
#304428=CARTESIAN_POINT('Ctrl Pts',(-2.52814742100006,2.2,3.86057711399998));
#304429=CARTESIAN_POINT('Ctrl Pts',(-2.53033765900006,12.2,3.86167781499999));
#304430=CARTESIAN_POINT('Ctrl Pts',(-2.53033765900006,5.2,3.86167781499999));
#304431=CARTESIAN_POINT('Ctrl Pts',(-2.53033765900006,2.2,3.86167781499999));
#304432=CARTESIAN_POINT('Ctrl Pts',(-2.53253225900006,12.2,3.86277779999999));
#304433=CARTESIAN_POINT('Ctrl Pts',(-2.53253225900006,5.2,3.86277779999999));
#304434=CARTESIAN_POINT('Ctrl Pts',(-2.53253225900006,2.2,3.86277779999999));
#304435=CARTESIAN_POINT('Ctrl Pts',(-2.53473122100006,12.2,3.86387705899998));
#304436=CARTESIAN_POINT('Ctrl Pts',(-2.53473122100006,5.2,3.86387705899998));
#304437=CARTESIAN_POINT('Ctrl Pts',(-2.53473122100006,2.2,3.86387705899998));
#304438=CARTESIAN_POINT('Ctrl Pts',(-2.53693454100006,12.2,3.86497558399999));
#304439=CARTESIAN_POINT('Ctrl Pts',(-2.53693454100006,5.2,3.86497558399999));
#304440=CARTESIAN_POINT('Ctrl Pts',(-2.53693454100006,2.2,3.86497558399999));
#304441=CARTESIAN_POINT('Ctrl Pts',(-2.53914221700006,12.2,3.86607336699999));
#304442=CARTESIAN_POINT('Ctrl Pts',(-2.53914221700006,5.2,3.86607336699999));
#304443=CARTESIAN_POINT('Ctrl Pts',(-2.53914221700006,2.2,3.86607336699999));
#304444=CARTESIAN_POINT('Ctrl Pts',(-2.54135424600006,12.2,3.86717039899998));
#304445=CARTESIAN_POINT('Ctrl Pts',(-2.54135424600006,5.2,3.86717039899998));
#304446=CARTESIAN_POINT('Ctrl Pts',(-2.54135424600006,2.2,3.86717039899998));
#304447=CARTESIAN_POINT('Ctrl Pts',(-2.54357062600006,12.2,3.86826666999998));
#304448=CARTESIAN_POINT('Ctrl Pts',(-2.54357062600006,5.2,3.86826666999998));
#304449=CARTESIAN_POINT('Ctrl Pts',(-2.54357062600006,2.2,3.86826666999998));
#304450=CARTESIAN_POINT('Ctrl Pts',(-2.54579135400005,12.2,3.86936217299999));
#304451=CARTESIAN_POINT('Ctrl Pts',(-2.54579135400005,5.2,3.86936217299999));
#304452=CARTESIAN_POINT('Ctrl Pts',(-2.54579135400005,2.2,3.86936217299999));
#304453=CARTESIAN_POINT('Ctrl Pts',(-2.54801642600006,12.2,3.87045689799999));
#304454=CARTESIAN_POINT('Ctrl Pts',(-2.54801642600006,5.2,3.87045689799999));
#304455=CARTESIAN_POINT('Ctrl Pts',(-2.54801642600006,2.2,3.87045689799999));
#304456=CARTESIAN_POINT('Ctrl Pts',(-2.55024583900005,12.2,3.87155083699999));
#304457=CARTESIAN_POINT('Ctrl Pts',(-2.55024583900005,5.2,3.87155083699999));
#304458=CARTESIAN_POINT('Ctrl Pts',(-2.55024583900005,2.2,3.87155083699999));
#304459=CARTESIAN_POINT('Ctrl Pts',(-2.55247959300006,12.2,3.87264398099998));
#304460=CARTESIAN_POINT('Ctrl Pts',(-2.55247959300006,5.2,3.87264398099998));
#304461=CARTESIAN_POINT('Ctrl Pts',(-2.55247959300006,2.2,3.87264398099998));
#304462=CARTESIAN_POINT('Ctrl Pts',(-2.55471768200006,12.2,3.87373632199999));
#304463=CARTESIAN_POINT('Ctrl Pts',(-2.55471768200006,5.2,3.87373632199999));
#304464=CARTESIAN_POINT('Ctrl Pts',(-2.55471768200006,2.2,3.87373632199999));
#304465=CARTESIAN_POINT('Ctrl Pts',(-2.55696010600006,12.2,3.87482785099999));
#304466=CARTESIAN_POINT('Ctrl Pts',(-2.55696010600006,5.2,3.87482785099999));
#304467=CARTESIAN_POINT('Ctrl Pts',(-2.55696010600006,2.2,3.87482785099999));
#304468=CARTESIAN_POINT('Ctrl Pts',(-2.55920686100006,12.2,3.87591855899998));
#304469=CARTESIAN_POINT('Ctrl Pts',(-2.55920686100006,5.2,3.87591855899998));
#304470=CARTESIAN_POINT('Ctrl Pts',(-2.55920686100006,2.2,3.87591855899998));
#304471=CARTESIAN_POINT('Ctrl Pts',(-2.56145794300005,12.2,3.87700843799998));
#304472=CARTESIAN_POINT('Ctrl Pts',(-2.56145794300005,5.2,3.87700843799998));
#304473=CARTESIAN_POINT('Ctrl Pts',(-2.56145794300005,2.2,3.87700843799998));
#304474=CARTESIAN_POINT('Ctrl Pts',(-2.56371335000006,12.2,3.87809747899999));
#304475=CARTESIAN_POINT('Ctrl Pts',(-2.56371335000006,5.2,3.87809747899999));
#304476=CARTESIAN_POINT('Ctrl Pts',(-2.56371335000006,2.2,3.87809747899999));
#304477=CARTESIAN_POINT('Ctrl Pts',(-2.56597308000006,12.2,3.87918567399999));
#304478=CARTESIAN_POINT('Ctrl Pts',(-2.56597308000006,5.2,3.87918567399999));
#304479=CARTESIAN_POINT('Ctrl Pts',(-2.56597308000006,2.2,3.87918567399999));
#304480=CARTESIAN_POINT('Ctrl Pts',(-2.56823713000006,12.2,3.88027301299999));
#304481=CARTESIAN_POINT('Ctrl Pts',(-2.56823713000006,5.2,3.88027301299999));
#304482=CARTESIAN_POINT('Ctrl Pts',(-2.56823713000006,2.2,3.88027301299999));
#304483=CARTESIAN_POINT('Ctrl Pts',(-2.57050549600006,12.2,3.88135948999999));
#304484=CARTESIAN_POINT('Ctrl Pts',(-2.57050549600006,5.2,3.88135948999999));
#304485=CARTESIAN_POINT('Ctrl Pts',(-2.57050549600006,2.2,3.88135948999999));
#304486=CARTESIAN_POINT('Ctrl Pts',(-2.57277817600006,12.2,3.88244509499999));
#304487=CARTESIAN_POINT('Ctrl Pts',(-2.57277817600006,5.2,3.88244509499999));
#304488=CARTESIAN_POINT('Ctrl Pts',(-2.57277817600006,2.2,3.88244509499999));
#304489=CARTESIAN_POINT('Ctrl Pts',(-2.57505516700005,12.2,3.88352981899998));
#304490=CARTESIAN_POINT('Ctrl Pts',(-2.57505516700005,5.2,3.88352981899998));
#304491=CARTESIAN_POINT('Ctrl Pts',(-2.57505516700005,2.2,3.88352981899998));
#304492=CARTESIAN_POINT('Ctrl Pts',(-2.57733646600005,12.2,3.88461365399999));
#304493=CARTESIAN_POINT('Ctrl Pts',(-2.57733646600005,5.2,3.88461365399999));
#304494=CARTESIAN_POINT('Ctrl Pts',(-2.57733646600005,2.2,3.88461365399999));
#304495=CARTESIAN_POINT('Ctrl Pts',(-2.57962207000006,12.2,3.88569659099999));
#304496=CARTESIAN_POINT('Ctrl Pts',(-2.57962207000006,5.2,3.88569659099999));
#304497=CARTESIAN_POINT('Ctrl Pts',(-2.57962207000006,2.2,3.88569659099999));
#304498=CARTESIAN_POINT('Ctrl Pts',(-2.58191197600006,12.2,3.88677862299998));
#304499=CARTESIAN_POINT('Ctrl Pts',(-2.58191197600006,5.2,3.88677862299998));
#304500=CARTESIAN_POINT('Ctrl Pts',(-2.58191197600006,2.2,3.88677862299998));
#304501=CARTESIAN_POINT('Ctrl Pts',(-2.58420618300006,12.2,3.88785973999998));
#304502=CARTESIAN_POINT('Ctrl Pts',(-2.58420618300006,5.2,3.88785973999998));
#304503=CARTESIAN_POINT('Ctrl Pts',(-2.58420618300006,2.2,3.88785973999998));
#304504=CARTESIAN_POINT('Ctrl Pts',(-2.58650468600006,12.2,3.88893993399999));
#304505=CARTESIAN_POINT('Ctrl Pts',(-2.58650468600006,5.2,3.88893993399999));
#304506=CARTESIAN_POINT('Ctrl Pts',(-2.58650468600006,2.2,3.88893993399999));
#304507=CARTESIAN_POINT('Ctrl Pts',(-2.58880748100006,12.2,3.89001919799998));
#304508=CARTESIAN_POINT('Ctrl Pts',(-2.58880748100006,5.2,3.89001919799998));
#304509=CARTESIAN_POINT('Ctrl Pts',(-2.58880748100006,2.2,3.89001919799998));
#304510=CARTESIAN_POINT('Ctrl Pts',(-2.59111456800006,12.2,3.89109752099999));
#304511=CARTESIAN_POINT('Ctrl Pts',(-2.59111456800006,5.2,3.89109752099999));
#304512=CARTESIAN_POINT('Ctrl Pts',(-2.59111456800006,2.2,3.89109752099999));
#304513=CARTESIAN_POINT('Ctrl Pts',(-2.59342594300006,12.2,3.89217489699998));
#304514=CARTESIAN_POINT('Ctrl Pts',(-2.59342594300006,5.2,3.89217489699998));
#304515=CARTESIAN_POINT('Ctrl Pts',(-2.59342594300006,2.2,3.89217489699998));
#304516=CARTESIAN_POINT('Ctrl Pts',(-2.59574160300006,12.2,3.89325131699999));
#304517=CARTESIAN_POINT('Ctrl Pts',(-2.59574160300006,5.2,3.89325131699999));
#304518=CARTESIAN_POINT('Ctrl Pts',(-2.59574160300006,2.2,3.89325131699999));
#304519=CARTESIAN_POINT('Ctrl Pts',(-2.59806154400006,12.2,3.89432677199999));
#304520=CARTESIAN_POINT('Ctrl Pts',(-2.59806154400006,5.2,3.89432677199999));
#304521=CARTESIAN_POINT('Ctrl Pts',(-2.59806154400006,2.2,3.89432677199999));
#304522=CARTESIAN_POINT('Ctrl Pts',(-2.60038576400006,12.2,3.89540125299998));
#304523=CARTESIAN_POINT('Ctrl Pts',(-2.60038576400006,5.2,3.89540125299998));
#304524=CARTESIAN_POINT('Ctrl Pts',(-2.60038576400006,2.2,3.89540125299998));
#304525=CARTESIAN_POINT('Ctrl Pts',(-2.60271426100006,12.2,3.89647475399999));
#304526=CARTESIAN_POINT('Ctrl Pts',(-2.60271426100006,5.2,3.89647475399999));
#304527=CARTESIAN_POINT('Ctrl Pts',(-2.60271426100006,2.2,3.89647475399999));
#304528=CARTESIAN_POINT('Ctrl Pts',(-2.60504703000006,12.2,3.89754726299999));
#304529=CARTESIAN_POINT('Ctrl Pts',(-2.60504703000006,5.2,3.89754726299999));
#304530=CARTESIAN_POINT('Ctrl Pts',(-2.60504703000006,2.2,3.89754726299999));
#304531=CARTESIAN_POINT('Ctrl Pts',(-2.60738406800006,12.2,3.89861877599999));
#304532=CARTESIAN_POINT('Ctrl Pts',(-2.60738406800006,5.2,3.89861877599999));
#304533=CARTESIAN_POINT('Ctrl Pts',(-2.60738406800006,2.2,3.89861877599999));
#304534=CARTESIAN_POINT('Ctrl Pts',(-2.60972537500006,12.2,3.89968928099999));
#304535=CARTESIAN_POINT('Ctrl Pts',(-2.60972537500006,5.2,3.89968928099999));
#304536=CARTESIAN_POINT('Ctrl Pts',(-2.60972537500006,2.2,3.89968928099999));
#304537=CARTESIAN_POINT('Ctrl Pts',(-2.61207094500006,12.2,3.90075877199998));
#304538=CARTESIAN_POINT('Ctrl Pts',(-2.61207094500006,5.2,3.90075877199998));
#304539=CARTESIAN_POINT('Ctrl Pts',(-2.61207094500006,2.2,3.90075877199998));
#304540=CARTESIAN_POINT('Ctrl Pts',(-2.61442077600006,12.2,3.90182724099999));
#304541=CARTESIAN_POINT('Ctrl Pts',(-2.61442077600006,5.2,3.90182724099999));
#304542=CARTESIAN_POINT('Ctrl Pts',(-2.61442077600006,2.2,3.90182724099999));
#304543=CARTESIAN_POINT('Ctrl Pts',(-2.61677486500006,12.2,3.90289467799998));
#304544=CARTESIAN_POINT('Ctrl Pts',(-2.61677486500006,5.2,3.90289467799998));
#304545=CARTESIAN_POINT('Ctrl Pts',(-2.61677486500006,2.2,3.90289467799998));
#304546=CARTESIAN_POINT('Ctrl Pts',(-2.61913321100006,12.2,3.90396107699999));
#304547=CARTESIAN_POINT('Ctrl Pts',(-2.61913321100006,5.2,3.90396107699999));
#304548=CARTESIAN_POINT('Ctrl Pts',(-2.61913321100006,2.2,3.90396107699999));
#304549=CARTESIAN_POINT('Ctrl Pts',(-2.62149580800005,12.2,3.90502642799999));
#304550=CARTESIAN_POINT('Ctrl Pts',(-2.62149580800005,5.2,3.90502642799999));
#304551=CARTESIAN_POINT('Ctrl Pts',(-2.62149580800005,2.2,3.90502642799999));
#304552=CARTESIAN_POINT('Ctrl Pts',(-2.62386265300006,12.2,3.90609072399998));
#304553=CARTESIAN_POINT('Ctrl Pts',(-2.62386265300006,5.2,3.90609072399998));
#304554=CARTESIAN_POINT('Ctrl Pts',(-2.62386265300006,2.2,3.90609072399998));
#304555=CARTESIAN_POINT('Ctrl Pts',(-2.62623374500006,12.2,3.90715395499999));
#304556=CARTESIAN_POINT('Ctrl Pts',(-2.62623374500006,5.2,3.90715395499999));
#304557=CARTESIAN_POINT('Ctrl Pts',(-2.62623374500006,2.2,3.90715395499999));
#304558=CARTESIAN_POINT('Ctrl Pts',(-2.62860907900006,12.2,3.90821611299998));
#304559=CARTESIAN_POINT('Ctrl Pts',(-2.62860907900006,5.2,3.90821611299998));
#304560=CARTESIAN_POINT('Ctrl Pts',(-2.62860907900006,2.2,3.90821611299998));
#304561=CARTESIAN_POINT('Ctrl Pts',(-2.63098865200006,12.2,3.90927718999999));
#304562=CARTESIAN_POINT('Ctrl Pts',(-2.63098865200006,5.2,3.90927718999999));
#304563=CARTESIAN_POINT('Ctrl Pts',(-2.63098865200006,2.2,3.90927718999999));
#304564=CARTESIAN_POINT('Ctrl Pts',(-2.63337246200006,12.2,3.91033717599999));
#304565=CARTESIAN_POINT('Ctrl Pts',(-2.63337246200006,5.2,3.91033717599999));
#304566=CARTESIAN_POINT('Ctrl Pts',(-2.63337246200006,2.2,3.91033717599999));
#304567=CARTESIAN_POINT('Ctrl Pts',(-2.63576050600005,12.2,3.91139606699999));
#304568=CARTESIAN_POINT('Ctrl Pts',(-2.63576050600005,5.2,3.91139606699999));
#304569=CARTESIAN_POINT('Ctrl Pts',(-2.63576050600005,2.2,3.91139606699999));
#304570=CARTESIAN_POINT('Ctrl Pts',(-2.63815278000005,12.2,3.91245385499998));
#304571=CARTESIAN_POINT('Ctrl Pts',(-2.63815278000005,5.2,3.91245385499998));
#304572=CARTESIAN_POINT('Ctrl Pts',(-2.63815278000005,2.2,3.91245385499998));
#304573=CARTESIAN_POINT('Ctrl Pts',(-2.64054928300005,12.2,3.91351052999998));
#304574=CARTESIAN_POINT('Ctrl Pts',(-2.64054928300005,5.2,3.91351052999998));
#304575=CARTESIAN_POINT('Ctrl Pts',(-2.64054928300005,2.2,3.91351052999998));
#304576=CARTESIAN_POINT('Ctrl Pts',(-2.64295001200006,12.2,3.91456608699999));
#304577=CARTESIAN_POINT('Ctrl Pts',(-2.64295001200006,5.2,3.91456608699999));
#304578=CARTESIAN_POINT('Ctrl Pts',(-2.64295001200006,2.2,3.91456608699999));
#304579=CARTESIAN_POINT('Ctrl Pts',(-2.64535496200006,12.2,3.91562051599998));
#304580=CARTESIAN_POINT('Ctrl Pts',(-2.64535496200006,5.2,3.91562051599998));
#304581=CARTESIAN_POINT('Ctrl Pts',(-2.64535496200006,2.2,3.91562051599998));
#304582=CARTESIAN_POINT('Ctrl Pts',(-2.64776413100006,12.2,3.91667381099998));
#304583=CARTESIAN_POINT('Ctrl Pts',(-2.64776413100006,5.2,3.91667381099998));
#304584=CARTESIAN_POINT('Ctrl Pts',(-2.64776413100006,2.2,3.91667381099998));
#304585=CARTESIAN_POINT('Ctrl Pts',(-2.65017751500006,12.2,3.91772595899998));
#304586=CARTESIAN_POINT('Ctrl Pts',(-2.65017751500006,5.2,3.91772595899998));
#304587=CARTESIAN_POINT('Ctrl Pts',(-2.65017751500006,2.2,3.91772595899998));
#304588=CARTESIAN_POINT('Ctrl Pts',(-2.65259511000006,12.2,3.91877695099998));
#304589=CARTESIAN_POINT('Ctrl Pts',(-2.65259511000006,5.2,3.91877695099998));
#304590=CARTESIAN_POINT('Ctrl Pts',(-2.65259511000006,2.2,3.91877695099998));
#304591=CARTESIAN_POINT('Ctrl Pts',(-2.65501691200006,12.2,3.91982677899998));
#304592=CARTESIAN_POINT('Ctrl Pts',(-2.65501691200006,5.2,3.91982677899998));
#304593=CARTESIAN_POINT('Ctrl Pts',(-2.65501691200006,2.2,3.91982677899998));
#304594=CARTESIAN_POINT('Ctrl Pts',(-2.65744291800006,12.2,3.92087542999998));
#304595=CARTESIAN_POINT('Ctrl Pts',(-2.65744291800006,5.2,3.92087542999998));
#304596=CARTESIAN_POINT('Ctrl Pts',(-2.65744291800006,2.2,3.92087542999998));
#304597=CARTESIAN_POINT('Ctrl Pts',(-2.65987312500005,12.2,3.92192289899998));
#304598=CARTESIAN_POINT('Ctrl Pts',(-2.65987312500005,5.2,3.92192289899998));
#304599=CARTESIAN_POINT('Ctrl Pts',(-2.65987312500005,2.2,3.92192289899998));
#304600=CARTESIAN_POINT('Ctrl Pts',(-2.66230753100006,12.2,3.92296918099999));
#304601=CARTESIAN_POINT('Ctrl Pts',(-2.66230753100006,5.2,3.92296918099999));
#304602=CARTESIAN_POINT('Ctrl Pts',(-2.66230753100006,2.2,3.92296918099999));
#304603=CARTESIAN_POINT('Ctrl Pts',(-2.66474613200006,12.2,3.92401427099998));
#304604=CARTESIAN_POINT('Ctrl Pts',(-2.66474613200006,5.2,3.92401427099998));
#304605=CARTESIAN_POINT('Ctrl Pts',(-2.66474613200006,2.2,3.92401427099998));
#304606=CARTESIAN_POINT('Ctrl Pts',(-2.66718893010949,12.2,3.92505816704675));
#304607=CARTESIAN_POINT('Ctrl Pts',(-2.66718893010949,5.2,3.92505816704675));
#304608=CARTESIAN_POINT('Ctrl Pts',(-2.66718893010949,2.2,3.92505816704675));
#304609=CARTESIAN_POINT('Ctrl Pts',(-2.6691465242193,12.2,3.92589232709341));
#304610=CARTESIAN_POINT('Ctrl Pts',(-2.6691465242193,5.2,3.92589232709341));
#304611=CARTESIAN_POINT('Ctrl Pts',(-2.6691465242193,2.2,3.92589232709341));
#304612=CARTESIAN_POINT('Ctrl Pts',(-2.67061660832935,12.2,3.92651741014));
#304613=CARTESIAN_POINT('Ctrl Pts',(-2.67061660832935,5.2,3.92651741014));
#304614=CARTESIAN_POINT('Ctrl Pts',(-2.67061660832935,2.2,3.92651741014));
#304615=CARTESIAN_POINT('Ctrl Pts',(-2.67159750343949,12.2,3.92693389218658));
#304616=CARTESIAN_POINT('Ctrl Pts',(-2.67159750343949,5.2,3.92693389218658));
#304617=CARTESIAN_POINT('Ctrl Pts',(-2.67159750343949,2.2,3.92693389218658));
#304618=CARTESIAN_POINT('Ctrl Pts',(-2.67208816000006,12.2,3.92714207399998));
#304619=CARTESIAN_POINT('Ctrl Pts',(-2.67208816000006,5.2,3.92714207399998));
#304620=CARTESIAN_POINT('Ctrl Pts',(-2.67208816000006,2.2,3.92714207399998));
#304621=CARTESIAN_POINT('',(-2.67208816000006,2.7,3.92714207399998));
#304622=CARTESIAN_POINT('',(-2.67208816000006,12.2,3.92714207399998));
#304623=CARTESIAN_POINT('Ctrl Pts',(-2.00390028800005,2.7,3.45459777299999));
#304624=CARTESIAN_POINT('Ctrl Pts',(-2.00531915316731,2.7,3.4570231905594));
#304625=CARTESIAN_POINT('Ctrl Pts',(-2.01694587943621,2.70000000004265,
3.47600453024496));
#304626=CARTESIAN_POINT('Ctrl Pts',(-2.07286963137762,2.70000000004265,
3.54137416856458));
#304627=CARTESIAN_POINT('Ctrl Pts',(-2.11342407259217,2.7,3.58245428063435));
#304628=CARTESIAN_POINT('Ctrl Pts',(-2.28821013174135,2.7,3.72952114371137));
#304629=CARTESIAN_POINT('Ctrl Pts',(-2.45288578684387,2.7,3.83413618920365));
#304630=CARTESIAN_POINT('Ctrl Pts',(-2.67208816000006,2.7,3.92714207399998));
#304631=CARTESIAN_POINT('Origin',(-5.66300478732629E-14,15.2,-1.77635683940025E-14));
#304632=CARTESIAN_POINT('',(-2.94378355400006,2.7,3.72781952199999));
#304633=CARTESIAN_POINT('',(-2.94378355400006,12.2,3.72781952199999));
#304634=CARTESIAN_POINT('Origin',(-5.66300478732629E-14,2.7,-1.92943768261394E-14));
#304635=CARTESIAN_POINT('Ctrl Pts',(-2.94378355400006,12.2,3.72781952199999));
#304636=CARTESIAN_POINT('Ctrl Pts',(-2.94378355400006,5.2,3.72781952199999));
#304637=CARTESIAN_POINT('Ctrl Pts',(-2.94378355400006,2.2,3.72781952199999));
#304638=CARTESIAN_POINT('Ctrl Pts',(-2.94373227900006,12.2,3.72728899799998));
#304639=CARTESIAN_POINT('Ctrl Pts',(-2.94373227900006,5.2,3.72728899799998));
#304640=CARTESIAN_POINT('Ctrl Pts',(-2.94373227900006,2.2,3.72728899799998));
#304641=CARTESIAN_POINT('Ctrl Pts',(-2.94362949000006,12.2,3.72622831699999));
#304642=CARTESIAN_POINT('Ctrl Pts',(-2.94362949000006,5.2,3.72622831699999));
#304643=CARTESIAN_POINT('Ctrl Pts',(-2.94362949000006,2.2,3.72622831699999));
#304644=CARTESIAN_POINT('Ctrl Pts',(-2.94347458500006,12.2,3.72463838599998));
#304645=CARTESIAN_POINT('Ctrl Pts',(-2.94347458500006,5.2,3.72463838599998));
#304646=CARTESIAN_POINT('Ctrl Pts',(-2.94347458500006,2.2,3.72463838599998));
#304647=CARTESIAN_POINT('Ctrl Pts',(-2.94326660500006,12.2,3.72252066499998));
#304648=CARTESIAN_POINT('Ctrl Pts',(-2.94326660500006,5.2,3.72252066499998));
#304649=CARTESIAN_POINT('Ctrl Pts',(-2.94326660500006,2.2,3.72252066499998));
#304650=CARTESIAN_POINT('Ctrl Pts',(-2.94300422900006,12.2,3.71987715499999));
#304651=CARTESIAN_POINT('Ctrl Pts',(-2.94300422900006,5.2,3.71987715499999));
#304652=CARTESIAN_POINT('Ctrl Pts',(-2.94300422900006,2.2,3.71987715499999));
#304653=CARTESIAN_POINT('Ctrl Pts',(-2.94273945600006,12.2,3.71723729099998));
#304654=CARTESIAN_POINT('Ctrl Pts',(-2.94273945600006,5.2,3.71723729099998));
#304655=CARTESIAN_POINT('Ctrl Pts',(-2.94273945600006,2.2,3.71723729099998));
#304656=CARTESIAN_POINT('Ctrl Pts',(-2.94247228600006,12.2,3.71460107099999));
#304657=CARTESIAN_POINT('Ctrl Pts',(-2.94247228600006,5.2,3.71460107099999));
#304658=CARTESIAN_POINT('Ctrl Pts',(-2.94247228600006,2.2,3.71460107099999));
#304659=CARTESIAN_POINT('Ctrl Pts',(-2.94220272300006,12.2,3.71196849999999));
#304660=CARTESIAN_POINT('Ctrl Pts',(-2.94220272300006,5.2,3.71196849999999));
#304661=CARTESIAN_POINT('Ctrl Pts',(-2.94220272300006,2.2,3.71196849999999));
#304662=CARTESIAN_POINT('Ctrl Pts',(-2.94193076900005,12.2,3.70933957999998));
#304663=CARTESIAN_POINT('Ctrl Pts',(-2.94193076900005,5.2,3.70933957999998));
#304664=CARTESIAN_POINT('Ctrl Pts',(-2.94193076900005,2.2,3.70933957999998));
#304665=CARTESIAN_POINT('Ctrl Pts',(-2.94165643500006,12.2,3.70671431799998));
#304666=CARTESIAN_POINT('Ctrl Pts',(-2.94165643500006,5.2,3.70671431799998));
#304667=CARTESIAN_POINT('Ctrl Pts',(-2.94165643500006,2.2,3.70671431799998));
#304668=CARTESIAN_POINT('Ctrl Pts',(-2.94137972400006,12.2,3.70409271899998));
#304669=CARTESIAN_POINT('Ctrl Pts',(-2.94137972400006,5.2,3.70409271899998));
#304670=CARTESIAN_POINT('Ctrl Pts',(-2.94137972400006,2.2,3.70409271899998));
#304671=CARTESIAN_POINT('Ctrl Pts',(-2.94110064700006,12.2,3.70147478899998));
#304672=CARTESIAN_POINT('Ctrl Pts',(-2.94110064700006,5.2,3.70147478899998));
#304673=CARTESIAN_POINT('Ctrl Pts',(-2.94110064700006,2.2,3.70147478899998));
#304674=CARTESIAN_POINT('Ctrl Pts',(-2.94081921200006,12.2,3.69886053599998));
#304675=CARTESIAN_POINT('Ctrl Pts',(-2.94081921200006,5.2,3.69886053599998));
#304676=CARTESIAN_POINT('Ctrl Pts',(-2.94081921200006,2.2,3.69886053599998));
#304677=CARTESIAN_POINT('Ctrl Pts',(-2.94053542700006,12.2,3.69624996699999));
#304678=CARTESIAN_POINT('Ctrl Pts',(-2.94053542700006,5.2,3.69624996699999));
#304679=CARTESIAN_POINT('Ctrl Pts',(-2.94053542700006,2.2,3.69624996699999));
#304680=CARTESIAN_POINT('Ctrl Pts',(-2.94024929900006,12.2,3.69364308599998));
#304681=CARTESIAN_POINT('Ctrl Pts',(-2.94024929900006,5.2,3.69364308599998));
#304682=CARTESIAN_POINT('Ctrl Pts',(-2.94024929900006,2.2,3.69364308599998));
#304683=CARTESIAN_POINT('Ctrl Pts',(-2.93996083600006,12.2,3.69103989999999));
#304684=CARTESIAN_POINT('Ctrl Pts',(-2.93996083600006,5.2,3.69103989999999));
#304685=CARTESIAN_POINT('Ctrl Pts',(-2.93996083600006,2.2,3.69103989999999));
#304686=CARTESIAN_POINT('Ctrl Pts',(-2.93967004300006,12.2,3.68844041299998));
#304687=CARTESIAN_POINT('Ctrl Pts',(-2.93967004300006,5.2,3.68844041299998));
#304688=CARTESIAN_POINT('Ctrl Pts',(-2.93967004300006,2.2,3.68844041299998));
#304689=CARTESIAN_POINT('Ctrl Pts',(-2.93937692700006,12.2,3.68584463099998));
#304690=CARTESIAN_POINT('Ctrl Pts',(-2.93937692700006,5.2,3.68584463099998));
#304691=CARTESIAN_POINT('Ctrl Pts',(-2.93937692700006,2.2,3.68584463099998));
#304692=CARTESIAN_POINT('Ctrl Pts',(-2.93908149400006,12.2,3.68325255699999));
#304693=CARTESIAN_POINT('Ctrl Pts',(-2.93908149400006,5.2,3.68325255699999));
#304694=CARTESIAN_POINT('Ctrl Pts',(-2.93908149400006,2.2,3.68325255699999));
#304695=CARTESIAN_POINT('Ctrl Pts',(-2.93878375000005,12.2,3.68066419899999));
#304696=CARTESIAN_POINT('Ctrl Pts',(-2.93878375000005,5.2,3.68066419899999));
#304697=CARTESIAN_POINT('Ctrl Pts',(-2.93878375000005,2.2,3.68066419899999));
#304698=CARTESIAN_POINT('Ctrl Pts',(-2.93848370200006,12.2,3.67807955899998));
#304699=CARTESIAN_POINT('Ctrl Pts',(-2.93848370200006,5.2,3.67807955899998));
#304700=CARTESIAN_POINT('Ctrl Pts',(-2.93848370200006,2.2,3.67807955899998));
#304701=CARTESIAN_POINT('Ctrl Pts',(-2.93818135600006,12.2,3.67549864399999));
#304702=CARTESIAN_POINT('Ctrl Pts',(-2.93818135600006,5.2,3.67549864399999));
#304703=CARTESIAN_POINT('Ctrl Pts',(-2.93818135600006,2.2,3.67549864399999));
#304704=CARTESIAN_POINT('Ctrl Pts',(-2.93787672200006,12.2,3.67292145899999));
#304705=CARTESIAN_POINT('Ctrl Pts',(-2.93787672200006,5.2,3.67292145899999));
#304706=CARTESIAN_POINT('Ctrl Pts',(-2.93787672200006,2.2,3.67292145899999));
#304707=CARTESIAN_POINT('Ctrl Pts',(-2.93756980300006,12.2,3.67034801099998));
#304708=CARTESIAN_POINT('Ctrl Pts',(-2.93756980300006,5.2,3.67034801099998));
#304709=CARTESIAN_POINT('Ctrl Pts',(-2.93756980300006,2.2,3.67034801099998));
#304710=CARTESIAN_POINT('Ctrl Pts',(-2.93726060900006,12.2,3.66777830299998));
#304711=CARTESIAN_POINT('Ctrl Pts',(-2.93726060900006,5.2,3.66777830299998));
#304712=CARTESIAN_POINT('Ctrl Pts',(-2.93726060900006,2.2,3.66777830299998));
#304713=CARTESIAN_POINT('Ctrl Pts',(-2.93694914700006,12.2,3.66521234299999));
#304714=CARTESIAN_POINT('Ctrl Pts',(-2.93694914700006,5.2,3.66521234299999));
#304715=CARTESIAN_POINT('Ctrl Pts',(-2.93694914700006,2.2,3.66521234299999));
#304716=CARTESIAN_POINT('Ctrl Pts',(-2.93663542300005,12.2,3.66265013499999));
#304717=CARTESIAN_POINT('Ctrl Pts',(-2.93663542300005,5.2,3.66265013499999));
#304718=CARTESIAN_POINT('Ctrl Pts',(-2.93663542300005,2.2,3.66265013499999));
#304719=CARTESIAN_POINT('Ctrl Pts',(-2.93631944400006,12.2,3.66009168499998));
#304720=CARTESIAN_POINT('Ctrl Pts',(-2.93631944400006,5.2,3.66009168499998));
#304721=CARTESIAN_POINT('Ctrl Pts',(-2.93631944400006,2.2,3.66009168499998));
#304722=CARTESIAN_POINT('Ctrl Pts',(-2.93600121800006,12.2,3.65753699699999));
#304723=CARTESIAN_POINT('Ctrl Pts',(-2.93600121800006,5.2,3.65753699699999));
#304724=CARTESIAN_POINT('Ctrl Pts',(-2.93600121800006,2.2,3.65753699699999));
#304725=CARTESIAN_POINT('Ctrl Pts',(-2.93568075100006,12.2,3.65498607799999));
#304726=CARTESIAN_POINT('Ctrl Pts',(-2.93568075100006,5.2,3.65498607799999));
#304727=CARTESIAN_POINT('Ctrl Pts',(-2.93568075100006,2.2,3.65498607799999));
#304728=CARTESIAN_POINT('Ctrl Pts',(-2.93535804900006,12.2,3.65243893199998));
#304729=CARTESIAN_POINT('Ctrl Pts',(-2.93535804900006,5.2,3.65243893199998));
#304730=CARTESIAN_POINT('Ctrl Pts',(-2.93535804900006,2.2,3.65243893199998));
#304731=CARTESIAN_POINT('Ctrl Pts',(-2.93503312000006,12.2,3.64989556399999));
#304732=CARTESIAN_POINT('Ctrl Pts',(-2.93503312000006,5.2,3.64989556399999));
#304733=CARTESIAN_POINT('Ctrl Pts',(-2.93503312000006,2.2,3.64989556399999));
#304734=CARTESIAN_POINT('Ctrl Pts',(-2.93470597200006,12.2,3.64735597999999));
#304735=CARTESIAN_POINT('Ctrl Pts',(-2.93470597200006,5.2,3.64735597999999));
#304736=CARTESIAN_POINT('Ctrl Pts',(-2.93470597200006,2.2,3.64735597999999));
#304737=CARTESIAN_POINT('Ctrl Pts',(-2.93437661100006,12.2,3.64482018699999));
#304738=CARTESIAN_POINT('Ctrl Pts',(-2.93437661100006,5.2,3.64482018699999));
#304739=CARTESIAN_POINT('Ctrl Pts',(-2.93437661100006,2.2,3.64482018699999));
#304740=CARTESIAN_POINT('Ctrl Pts',(-2.93404504400006,12.2,3.64228818699999));
#304741=CARTESIAN_POINT('Ctrl Pts',(-2.93404504400006,5.2,3.64228818699999));
#304742=CARTESIAN_POINT('Ctrl Pts',(-2.93404504400006,2.2,3.64228818699999));
#304743=CARTESIAN_POINT('Ctrl Pts',(-2.93371127800006,12.2,3.63975998699999));
#304744=CARTESIAN_POINT('Ctrl Pts',(-2.93371127800006,5.2,3.63975998699999));
#304745=CARTESIAN_POINT('Ctrl Pts',(-2.93371127800006,2.2,3.63975998699999));
#304746=CARTESIAN_POINT('Ctrl Pts',(-2.93337532100006,12.2,3.63723559299999));
#304747=CARTESIAN_POINT('Ctrl Pts',(-2.93337532100006,5.2,3.63723559299999));
#304748=CARTESIAN_POINT('Ctrl Pts',(-2.93337532100006,2.2,3.63723559299999));
#304749=CARTESIAN_POINT('Ctrl Pts',(-2.93303717900006,12.2,3.63471500999999));
#304750=CARTESIAN_POINT('Ctrl Pts',(-2.93303717900006,5.2,3.63471500999999));
#304751=CARTESIAN_POINT('Ctrl Pts',(-2.93303717900006,2.2,3.63471500999999));
#304752=CARTESIAN_POINT('Ctrl Pts',(-2.93269686000006,12.2,3.63219824299998));
#304753=CARTESIAN_POINT('Ctrl Pts',(-2.93269686000006,5.2,3.63219824299998));
#304754=CARTESIAN_POINT('Ctrl Pts',(-2.93269686000006,2.2,3.63219824299998));
#304755=CARTESIAN_POINT('Ctrl Pts',(-2.93235437200006,12.2,3.62968529699998));
#304756=CARTESIAN_POINT('Ctrl Pts',(-2.93235437200006,5.2,3.62968529699998));
#304757=CARTESIAN_POINT('Ctrl Pts',(-2.93235437200006,2.2,3.62968529699998));
#304758=CARTESIAN_POINT('Ctrl Pts',(-2.93200972000006,12.2,3.62717617799999));
#304759=CARTESIAN_POINT('Ctrl Pts',(-2.93200972000006,5.2,3.62717617799999));
#304760=CARTESIAN_POINT('Ctrl Pts',(-2.93200972000006,2.2,3.62717617799999));
#304761=CARTESIAN_POINT('Ctrl Pts',(-2.93166291300006,12.2,3.62467089099999));
#304762=CARTESIAN_POINT('Ctrl Pts',(-2.93166291300006,5.2,3.62467089099999));
#304763=CARTESIAN_POINT('Ctrl Pts',(-2.93166291300006,2.2,3.62467089099999));
#304764=CARTESIAN_POINT('Ctrl Pts',(-2.93131395600006,12.2,3.62216943999999));
#304765=CARTESIAN_POINT('Ctrl Pts',(-2.93131395600006,5.2,3.62216943999999));
#304766=CARTESIAN_POINT('Ctrl Pts',(-2.93131395600006,2.2,3.62216943999999));
#304767=CARTESIAN_POINT('Ctrl Pts',(-2.93096285900006,12.2,3.61967183199998));
#304768=CARTESIAN_POINT('Ctrl Pts',(-2.93096285900006,5.2,3.61967183199998));
#304769=CARTESIAN_POINT('Ctrl Pts',(-2.93096285900006,2.2,3.61967183199998));
#304770=CARTESIAN_POINT('Ctrl Pts',(-2.93060962800006,12.2,3.61717807199998));
#304771=CARTESIAN_POINT('Ctrl Pts',(-2.93060962800006,5.2,3.61717807199998));
#304772=CARTESIAN_POINT('Ctrl Pts',(-2.93060962800006,2.2,3.61717807199998));
#304773=CARTESIAN_POINT('Ctrl Pts',(-2.93025426900006,12.2,3.61468816499999));
#304774=CARTESIAN_POINT('Ctrl Pts',(-2.93025426900006,5.2,3.61468816499999));
#304775=CARTESIAN_POINT('Ctrl Pts',(-2.93025426900006,2.2,3.61468816499999));
#304776=CARTESIAN_POINT('Ctrl Pts',(-2.92989679200006,12.2,3.61220211699998));
#304777=CARTESIAN_POINT('Ctrl Pts',(-2.92989679200006,5.2,3.61220211699998));
#304778=CARTESIAN_POINT('Ctrl Pts',(-2.92989679200006,2.2,3.61220211699998));
#304779=CARTESIAN_POINT('Ctrl Pts',(-2.92953720100006,12.2,3.60971993199998));
#304780=CARTESIAN_POINT('Ctrl Pts',(-2.92953720100006,5.2,3.60971993199998));
#304781=CARTESIAN_POINT('Ctrl Pts',(-2.92953720100006,2.2,3.60971993199998));
#304782=CARTESIAN_POINT('Ctrl Pts',(-2.92917550600006,12.2,3.60724161599999));
#304783=CARTESIAN_POINT('Ctrl Pts',(-2.92917550600006,5.2,3.60724161599999));
#304784=CARTESIAN_POINT('Ctrl Pts',(-2.92917550600006,2.2,3.60724161599999));
#304785=CARTESIAN_POINT('Ctrl Pts',(-2.92881171300006,12.2,3.60476717399998));
#304786=CARTESIAN_POINT('Ctrl Pts',(-2.92881171300006,5.2,3.60476717399998));
#304787=CARTESIAN_POINT('Ctrl Pts',(-2.92881171300006,2.2,3.60476717399998));
#304788=CARTESIAN_POINT('Ctrl Pts',(-2.92844583100006,12.2,3.60229661199998));
#304789=CARTESIAN_POINT('Ctrl Pts',(-2.92844583100006,5.2,3.60229661199998));
#304790=CARTESIAN_POINT('Ctrl Pts',(-2.92844583100006,2.2,3.60229661199998));
#304791=CARTESIAN_POINT('Ctrl Pts',(-2.92807786400005,12.2,3.59982993399999));
#304792=CARTESIAN_POINT('Ctrl Pts',(-2.92807786400005,5.2,3.59982993399999));
#304793=CARTESIAN_POINT('Ctrl Pts',(-2.92807786400005,2.2,3.59982993399999));
#304794=CARTESIAN_POINT('Ctrl Pts',(-2.92770782300006,12.2,3.59736714599999));
#304795=CARTESIAN_POINT('Ctrl Pts',(-2.92770782300006,5.2,3.59736714599999));
#304796=CARTESIAN_POINT('Ctrl Pts',(-2.92770782300006,2.2,3.59736714599999));
#304797=CARTESIAN_POINT('Ctrl Pts',(-2.92733571200006,12.2,3.59490825399998));
#304798=CARTESIAN_POINT('Ctrl Pts',(-2.92733571200006,5.2,3.59490825399998));
#304799=CARTESIAN_POINT('Ctrl Pts',(-2.92733571200006,2.2,3.59490825399998));
#304800=CARTESIAN_POINT('Ctrl Pts',(-2.92696154200006,12.2,3.59245326099998));
#304801=CARTESIAN_POINT('Ctrl Pts',(-2.92696154200006,5.2,3.59245326099998));
#304802=CARTESIAN_POINT('Ctrl Pts',(-2.92696154200006,2.2,3.59245326099998));
#304803=CARTESIAN_POINT('Ctrl Pts',(-2.92658531800006,12.2,3.59000217499998));
#304804=CARTESIAN_POINT('Ctrl Pts',(-2.92658531800006,5.2,3.59000217499998));
#304805=CARTESIAN_POINT('Ctrl Pts',(-2.92658531800006,2.2,3.59000217499998));
#304806=CARTESIAN_POINT('Ctrl Pts',(-2.92620704700005,12.2,3.58755499999998));
#304807=CARTESIAN_POINT('Ctrl Pts',(-2.92620704700005,5.2,3.58755499999998));
#304808=CARTESIAN_POINT('Ctrl Pts',(-2.92620704700005,2.2,3.58755499999998));
#304809=CARTESIAN_POINT('Ctrl Pts',(-2.92582673900006,12.2,3.58511173999998));
#304810=CARTESIAN_POINT('Ctrl Pts',(-2.92582673900006,5.2,3.58511173999998));
#304811=CARTESIAN_POINT('Ctrl Pts',(-2.92582673900006,2.2,3.58511173999998));
#304812=CARTESIAN_POINT('Ctrl Pts',(-2.92544440000006,12.2,3.58267240299998));
#304813=CARTESIAN_POINT('Ctrl Pts',(-2.92544440000006,5.2,3.58267240299998));
#304814=CARTESIAN_POINT('Ctrl Pts',(-2.92544440000006,2.2,3.58267240299998));
#304815=CARTESIAN_POINT('Ctrl Pts',(-2.92506003600006,12.2,3.58023699199999));
#304816=CARTESIAN_POINT('Ctrl Pts',(-2.92506003600006,5.2,3.58023699199999));
#304817=CARTESIAN_POINT('Ctrl Pts',(-2.92506003600006,2.2,3.58023699199999));
#304818=CARTESIAN_POINT('Ctrl Pts',(-2.92467365700006,12.2,3.57780551299999));
#304819=CARTESIAN_POINT('Ctrl Pts',(-2.92467365700006,5.2,3.57780551299999));
#304820=CARTESIAN_POINT('Ctrl Pts',(-2.92467365700006,2.2,3.57780551299999));
#304821=CARTESIAN_POINT('Ctrl Pts',(-2.92428526900005,12.2,3.57537797099998));
#304822=CARTESIAN_POINT('Ctrl Pts',(-2.92428526900005,5.2,3.57537797099998));
#304823=CARTESIAN_POINT('Ctrl Pts',(-2.92428526900005,2.2,3.57537797099998));
#304824=CARTESIAN_POINT('Ctrl Pts',(-2.92389488000006,12.2,3.57295437199999));
#304825=CARTESIAN_POINT('Ctrl Pts',(-2.92389488000006,5.2,3.57295437199999));
#304826=CARTESIAN_POINT('Ctrl Pts',(-2.92389488000006,2.2,3.57295437199999));
#304827=CARTESIAN_POINT('Ctrl Pts',(-2.92350249700006,12.2,3.57053471999999));
#304828=CARTESIAN_POINT('Ctrl Pts',(-2.92350249700006,5.2,3.57053471999999));
#304829=CARTESIAN_POINT('Ctrl Pts',(-2.92350249700006,2.2,3.57053471999999));
#304830=CARTESIAN_POINT('Ctrl Pts',(-2.92310812900006,12.2,3.56811902099999));
#304831=CARTESIAN_POINT('Ctrl Pts',(-2.92310812900006,5.2,3.56811902099999));
#304832=CARTESIAN_POINT('Ctrl Pts',(-2.92310812900006,2.2,3.56811902099999));
#304833=CARTESIAN_POINT('Ctrl Pts',(-2.92271178200005,12.2,3.56570727999999));
#304834=CARTESIAN_POINT('Ctrl Pts',(-2.92271178200005,5.2,3.56570727999999));
#304835=CARTESIAN_POINT('Ctrl Pts',(-2.92271178200005,2.2,3.56570727999999));
#304836=CARTESIAN_POINT('Ctrl Pts',(-2.92231346500006,12.2,3.56329950299998));
#304837=CARTESIAN_POINT('Ctrl Pts',(-2.92231346500006,5.2,3.56329950299998));
#304838=CARTESIAN_POINT('Ctrl Pts',(-2.92231346500006,2.2,3.56329950299998));
#304839=CARTESIAN_POINT('Ctrl Pts',(-2.92191318400006,12.2,3.56089569299999));
#304840=CARTESIAN_POINT('Ctrl Pts',(-2.92191318400006,5.2,3.56089569299999));
#304841=CARTESIAN_POINT('Ctrl Pts',(-2.92191318400006,2.2,3.56089569299999));
#304842=CARTESIAN_POINT('Ctrl Pts',(-2.92151094800006,12.2,3.55849585699998));
#304843=CARTESIAN_POINT('Ctrl Pts',(-2.92151094800006,5.2,3.55849585699998));
#304844=CARTESIAN_POINT('Ctrl Pts',(-2.92151094800006,2.2,3.55849585699998));
#304845=CARTESIAN_POINT('Ctrl Pts',(-2.92110676400006,12.2,3.55610000199999));
#304846=CARTESIAN_POINT('Ctrl Pts',(-2.92110676400006,5.2,3.55610000199999));
#304847=CARTESIAN_POINT('Ctrl Pts',(-2.92110676400006,2.2,3.55610000199999));
#304848=CARTESIAN_POINT('Ctrl Pts',(-2.92070064000006,12.2,3.55370812899999));
#304849=CARTESIAN_POINT('Ctrl Pts',(-2.92070064000006,5.2,3.55370812899999));
#304850=CARTESIAN_POINT('Ctrl Pts',(-2.92070064000006,2.2,3.55370812899999));
#304851=CARTESIAN_POINT('Ctrl Pts',(-2.92029258400006,12.2,3.55132024499999));
#304852=CARTESIAN_POINT('Ctrl Pts',(-2.92029258400006,5.2,3.55132024499999));
#304853=CARTESIAN_POINT('Ctrl Pts',(-2.92029258400006,2.2,3.55132024499999));
#304854=CARTESIAN_POINT('Ctrl Pts',(-2.91988260200006,12.2,3.54893635699998));
#304855=CARTESIAN_POINT('Ctrl Pts',(-2.91988260200006,5.2,3.54893635699998));
#304856=CARTESIAN_POINT('Ctrl Pts',(-2.91988260200006,2.2,3.54893635699998));
#304857=CARTESIAN_POINT('Ctrl Pts',(-2.91947070300006,12.2,3.54655646799999));
#304858=CARTESIAN_POINT('Ctrl Pts',(-2.91947070300006,5.2,3.54655646799999));
#304859=CARTESIAN_POINT('Ctrl Pts',(-2.91947070300006,2.2,3.54655646799999));
#304860=CARTESIAN_POINT('Ctrl Pts',(-2.91905689500005,12.2,3.54418058299999));
#304861=CARTESIAN_POINT('Ctrl Pts',(-2.91905689500005,5.2,3.54418058299999));
#304862=CARTESIAN_POINT('Ctrl Pts',(-2.91905689500005,2.2,3.54418058299999));
#304863=CARTESIAN_POINT('Ctrl Pts',(-2.91864118600006,12.2,3.54180870899999));
#304864=CARTESIAN_POINT('Ctrl Pts',(-2.91864118600006,5.2,3.54180870899999));
#304865=CARTESIAN_POINT('Ctrl Pts',(-2.91864118600006,2.2,3.54180870899999));
#304866=CARTESIAN_POINT('Ctrl Pts',(-2.91822358300006,12.2,3.53944084999998));
#304867=CARTESIAN_POINT('Ctrl Pts',(-2.91822358300006,5.2,3.53944084999998));
#304868=CARTESIAN_POINT('Ctrl Pts',(-2.91822358300006,2.2,3.53944084999998));
#304869=CARTESIAN_POINT('Ctrl Pts',(-2.91780409400006,12.2,3.53707701099999));
#304870=CARTESIAN_POINT('Ctrl Pts',(-2.91780409400006,5.2,3.53707701099999));
#304871=CARTESIAN_POINT('Ctrl Pts',(-2.91780409400006,2.2,3.53707701099999));
#304872=CARTESIAN_POINT('Ctrl Pts',(-2.91738272700006,12.2,3.53471719699999));
#304873=CARTESIAN_POINT('Ctrl Pts',(-2.91738272700006,5.2,3.53471719699999));
#304874=CARTESIAN_POINT('Ctrl Pts',(-2.91738272700006,2.2,3.53471719699999));
#304875=CARTESIAN_POINT('Ctrl Pts',(-2.91695948900006,12.2,3.53236141499998));
#304876=CARTESIAN_POINT('Ctrl Pts',(-2.91695948900006,5.2,3.53236141499998));
#304877=CARTESIAN_POINT('Ctrl Pts',(-2.91695948900006,2.2,3.53236141499998));
#304878=CARTESIAN_POINT('Ctrl Pts',(-2.91653438800005,12.2,3.53000966899998));
#304879=CARTESIAN_POINT('Ctrl Pts',(-2.91653438800005,5.2,3.53000966899998));
#304880=CARTESIAN_POINT('Ctrl Pts',(-2.91653438800005,2.2,3.53000966899998));
#304881=CARTESIAN_POINT('Ctrl Pts',(-2.91610743300006,12.2,3.52766196299999));
#304882=CARTESIAN_POINT('Ctrl Pts',(-2.91610743300006,5.2,3.52766196299999));
#304883=CARTESIAN_POINT('Ctrl Pts',(-2.91610743300006,2.2,3.52766196299999));
#304884=CARTESIAN_POINT('Ctrl Pts',(-2.91567863100005,12.2,3.52531830299998));
#304885=CARTESIAN_POINT('Ctrl Pts',(-2.91567863100005,5.2,3.52531830299998));
#304886=CARTESIAN_POINT('Ctrl Pts',(-2.91567863100005,2.2,3.52531830299998));
#304887=CARTESIAN_POINT('Ctrl Pts',(-2.91524799000006,12.2,3.52297869399998));
#304888=CARTESIAN_POINT('Ctrl Pts',(-2.91524799000006,5.2,3.52297869399998));
#304889=CARTESIAN_POINT('Ctrl Pts',(-2.91524799000006,2.2,3.52297869399998));
#304890=CARTESIAN_POINT('Ctrl Pts',(-2.91481551900006,12.2,3.52064314199998));
#304891=CARTESIAN_POINT('Ctrl Pts',(-2.91481551900006,5.2,3.52064314199998));
#304892=CARTESIAN_POINT('Ctrl Pts',(-2.91481551900006,2.2,3.52064314199998));
#304893=CARTESIAN_POINT('Ctrl Pts',(-2.91438122300006,12.2,3.51831165199999));
#304894=CARTESIAN_POINT('Ctrl Pts',(-2.91438122300006,5.2,3.51831165199999));
#304895=CARTESIAN_POINT('Ctrl Pts',(-2.91438122300006,2.2,3.51831165199999));
#304896=CARTESIAN_POINT('Ctrl Pts',(-2.91394511400005,12.2,3.51598422799999));
#304897=CARTESIAN_POINT('Ctrl Pts',(-2.91394511400005,5.2,3.51598422799999));
#304898=CARTESIAN_POINT('Ctrl Pts',(-2.91394511400005,2.2,3.51598422799999));
#304899=CARTESIAN_POINT('Ctrl Pts',(-2.91350719600006,12.2,3.51366087699999));
#304900=CARTESIAN_POINT('Ctrl Pts',(-2.91350719600006,5.2,3.51366087699999));
#304901=CARTESIAN_POINT('Ctrl Pts',(-2.91350719600006,2.2,3.51366087699999));
#304902=CARTESIAN_POINT('Ctrl Pts',(-2.91306748000005,12.2,3.51134160099999));
#304903=CARTESIAN_POINT('Ctrl Pts',(-2.91306748000005,5.2,3.51134160099999));
#304904=CARTESIAN_POINT('Ctrl Pts',(-2.91306748000005,2.2,3.51134160099999));
#304905=CARTESIAN_POINT('Ctrl Pts',(-2.91262597100005,12.2,3.50902640899999));
#304906=CARTESIAN_POINT('Ctrl Pts',(-2.91262597100005,5.2,3.50902640899999));
#304907=CARTESIAN_POINT('Ctrl Pts',(-2.91262597100005,2.2,3.50902640899999));
#304908=CARTESIAN_POINT('Ctrl Pts',(-2.91218268100006,12.2,3.50671530299999));
#304909=CARTESIAN_POINT('Ctrl Pts',(-2.91218268100006,5.2,3.50671530299999));
#304910=CARTESIAN_POINT('Ctrl Pts',(-2.91218268100006,2.2,3.50671530299999));
#304911=CARTESIAN_POINT('Ctrl Pts',(-2.91173761400006,12.2,3.50440828999999));
#304912=CARTESIAN_POINT('Ctrl Pts',(-2.91173761400006,5.2,3.50440828999999));
#304913=CARTESIAN_POINT('Ctrl Pts',(-2.91173761400006,2.2,3.50440828999999));
#304914=CARTESIAN_POINT('Ctrl Pts',(-2.91129078100006,12.2,3.50210537399998));
#304915=CARTESIAN_POINT('Ctrl Pts',(-2.91129078100006,5.2,3.50210537399998));
#304916=CARTESIAN_POINT('Ctrl Pts',(-2.91129078100006,2.2,3.50210537399998));
#304917=CARTESIAN_POINT('Ctrl Pts',(-2.91084218900005,12.2,3.49980655999998));
#304918=CARTESIAN_POINT('Ctrl Pts',(-2.91084218900005,5.2,3.49980655999998));
#304919=CARTESIAN_POINT('Ctrl Pts',(-2.91084218900005,2.2,3.49980655999998));
#304920=CARTESIAN_POINT('Ctrl Pts',(-2.91039184500006,12.2,3.49751185399998));
#304921=CARTESIAN_POINT('Ctrl Pts',(-2.91039184500006,5.2,3.49751185399998));
#304922=CARTESIAN_POINT('Ctrl Pts',(-2.91039184500006,2.2,3.49751185399998));
#304923=CARTESIAN_POINT('Ctrl Pts',(-2.90993975900005,12.2,3.49522126099998));
#304924=CARTESIAN_POINT('Ctrl Pts',(-2.90993975900005,5.2,3.49522126099998));
#304925=CARTESIAN_POINT('Ctrl Pts',(-2.90993975900005,2.2,3.49522126099998));
#304926=CARTESIAN_POINT('Ctrl Pts',(-2.90948593800006,12.2,3.49293478699998));
#304927=CARTESIAN_POINT('Ctrl Pts',(-2.90948593800006,5.2,3.49293478699998));
#304928=CARTESIAN_POINT('Ctrl Pts',(-2.90948593800006,2.2,3.49293478699998));
#304929=CARTESIAN_POINT('Ctrl Pts',(-2.90903039100006,12.2,3.49065243299999));
#304930=CARTESIAN_POINT('Ctrl Pts',(-2.90903039100006,5.2,3.49065243299999));
#304931=CARTESIAN_POINT('Ctrl Pts',(-2.90903039100006,2.2,3.49065243299999));
#304932=CARTESIAN_POINT('Ctrl Pts',(-2.90857312500005,12.2,3.48837420999998));
#304933=CARTESIAN_POINT('Ctrl Pts',(-2.90857312500005,5.2,3.48837420999998));
#304934=CARTESIAN_POINT('Ctrl Pts',(-2.90857312500005,2.2,3.48837420999998));
#304935=CARTESIAN_POINT('Ctrl Pts',(-2.90811414800006,12.2,3.48610011899999));
#304936=CARTESIAN_POINT('Ctrl Pts',(-2.90811414800006,5.2,3.48610011899999));
#304937=CARTESIAN_POINT('Ctrl Pts',(-2.90811414800006,2.2,3.48610011899999));
#304938=CARTESIAN_POINT('Ctrl Pts',(-2.90765347000006,12.2,3.48383016499999));
#304939=CARTESIAN_POINT('Ctrl Pts',(-2.90765347000006,5.2,3.48383016499999));
#304940=CARTESIAN_POINT('Ctrl Pts',(-2.90765347000006,2.2,3.48383016499999));
#304941=CARTESIAN_POINT('Ctrl Pts',(-2.90719109800006,12.2,3.48156435399999));
#304942=CARTESIAN_POINT('Ctrl Pts',(-2.90719109800006,5.2,3.48156435399999));
#304943=CARTESIAN_POINT('Ctrl Pts',(-2.90719109800006,2.2,3.48156435399999));
#304944=CARTESIAN_POINT('Ctrl Pts',(-2.90672704000006,12.2,3.47930269299999));
#304945=CARTESIAN_POINT('Ctrl Pts',(-2.90672704000006,5.2,3.47930269299999));
#304946=CARTESIAN_POINT('Ctrl Pts',(-2.90672704000006,2.2,3.47930269299999));
#304947=CARTESIAN_POINT('Ctrl Pts',(-2.90626130400006,12.2,3.47704518499998));
#304948=CARTESIAN_POINT('Ctrl Pts',(-2.90626130400006,5.2,3.47704518499998));
#304949=CARTESIAN_POINT('Ctrl Pts',(-2.90626130400006,2.2,3.47704518499998));
#304950=CARTESIAN_POINT('Ctrl Pts',(-2.90579390000006,12.2,3.47479183399999));
#304951=CARTESIAN_POINT('Ctrl Pts',(-2.90579390000006,5.2,3.47479183399999));
#304952=CARTESIAN_POINT('Ctrl Pts',(-2.90579390000006,2.2,3.47479183399999));
#304953=CARTESIAN_POINT('Ctrl Pts',(-2.90532483500006,12.2,3.47254264799999));
#304954=CARTESIAN_POINT('Ctrl Pts',(-2.90532483500006,5.2,3.47254264799999));
#304955=CARTESIAN_POINT('Ctrl Pts',(-2.90532483500006,2.2,3.47254264799999));
#304956=CARTESIAN_POINT('Ctrl Pts',(-2.90485411700006,12.2,3.47029762999998));
#304957=CARTESIAN_POINT('Ctrl Pts',(-2.90485411700006,5.2,3.47029762999998));
#304958=CARTESIAN_POINT('Ctrl Pts',(-2.90485411700006,2.2,3.47029762999998));
#304959=CARTESIAN_POINT('Ctrl Pts',(-2.90438175500006,12.2,3.46805678499998));
#304960=CARTESIAN_POINT('Ctrl Pts',(-2.90438175500006,5.2,3.46805678499998));
#304961=CARTESIAN_POINT('Ctrl Pts',(-2.90438175500006,2.2,3.46805678499998));
#304962=CARTESIAN_POINT('Ctrl Pts',(-2.90390775600006,12.2,3.46582011999998));
#304963=CARTESIAN_POINT('Ctrl Pts',(-2.90390775600006,5.2,3.46582011999998));
#304964=CARTESIAN_POINT('Ctrl Pts',(-2.90390775600006,2.2,3.46582011999998));
#304965=CARTESIAN_POINT('Ctrl Pts',(-2.90343213100006,12.2,3.46358763699998));
#304966=CARTESIAN_POINT('Ctrl Pts',(-2.90343213100006,5.2,3.46358763699998));
#304967=CARTESIAN_POINT('Ctrl Pts',(-2.90343213100006,2.2,3.46358763699998));
#304968=CARTESIAN_POINT('Ctrl Pts',(-2.90295488600006,12.2,3.46135934399998));
#304969=CARTESIAN_POINT('Ctrl Pts',(-2.90295488600006,5.2,3.46135934399998));
#304970=CARTESIAN_POINT('Ctrl Pts',(-2.90295488600006,2.2,3.46135934399998));
#304971=CARTESIAN_POINT('Ctrl Pts',(-2.90247603100006,12.2,3.45913524399998));
#304972=CARTESIAN_POINT('Ctrl Pts',(-2.90247603100006,5.2,3.45913524399998));
#304973=CARTESIAN_POINT('Ctrl Pts',(-2.90247603100006,2.2,3.45913524399998));
#304974=CARTESIAN_POINT('Ctrl Pts',(-2.90199557400005,12.2,3.45691534299998));
#304975=CARTESIAN_POINT('Ctrl Pts',(-2.90199557400005,5.2,3.45691534299998));
#304976=CARTESIAN_POINT('Ctrl Pts',(-2.90199557400005,2.2,3.45691534299998));
#304977=CARTESIAN_POINT('Ctrl Pts',(-2.90151352200006,12.2,3.45469964499999));
#304978=CARTESIAN_POINT('Ctrl Pts',(-2.90151352200006,5.2,3.45469964499999));
#304979=CARTESIAN_POINT('Ctrl Pts',(-2.90151352200006,2.2,3.45469964499999));
#304980=CARTESIAN_POINT('Ctrl Pts',(-2.90102988400006,12.2,3.45248815599999));
#304981=CARTESIAN_POINT('Ctrl Pts',(-2.90102988400006,5.2,3.45248815599999));
#304982=CARTESIAN_POINT('Ctrl Pts',(-2.90102988400006,2.2,3.45248815599999));
#304983=CARTESIAN_POINT('Ctrl Pts',(-2.90054467100005,12.2,3.45028088099999));
#304984=CARTESIAN_POINT('Ctrl Pts',(-2.90054467100005,5.2,3.45028088099999));
#304985=CARTESIAN_POINT('Ctrl Pts',(-2.90054467100005,2.2,3.45028088099999));
#304986=CARTESIAN_POINT('Ctrl Pts',(-2.90005788800006,12.2,3.44807782499998));
#304987=CARTESIAN_POINT('Ctrl Pts',(-2.90005788800006,5.2,3.44807782499998));
#304988=CARTESIAN_POINT('Ctrl Pts',(-2.90005788800006,2.2,3.44807782499998));
#304989=CARTESIAN_POINT('Ctrl Pts',(-2.89956954600005,12.2,3.44587899199999));
#304990=CARTESIAN_POINT('Ctrl Pts',(-2.89956954600005,5.2,3.44587899199999));
#304991=CARTESIAN_POINT('Ctrl Pts',(-2.89956954600005,2.2,3.44587899199999));
#304992=CARTESIAN_POINT('Ctrl Pts',(-2.89907965200006,12.2,3.44368438899998));
#304993=CARTESIAN_POINT('Ctrl Pts',(-2.89907965200006,5.2,3.44368438899998));
#304994=CARTESIAN_POINT('Ctrl Pts',(-2.89907965200006,2.2,3.44368438899998));
#304995=CARTESIAN_POINT('Ctrl Pts',(-2.89858821500005,12.2,3.44149401799999));
#304996=CARTESIAN_POINT('Ctrl Pts',(-2.89858821500005,5.2,3.44149401799999));
#304997=CARTESIAN_POINT('Ctrl Pts',(-2.89858821500005,2.2,3.44149401799999));
#304998=CARTESIAN_POINT('Ctrl Pts',(-2.89809524300006,12.2,3.43930788699998));
#304999=CARTESIAN_POINT('Ctrl Pts',(-2.89809524300006,5.2,3.43930788699998));
#305000=CARTESIAN_POINT('Ctrl Pts',(-2.89809524300006,2.2,3.43930788699998));
#305001=CARTESIAN_POINT('Ctrl Pts',(-2.89760074700005,12.2,3.43712599899998));
#305002=CARTESIAN_POINT('Ctrl Pts',(-2.89760074700005,5.2,3.43712599899998));
#305003=CARTESIAN_POINT('Ctrl Pts',(-2.89760074700005,2.2,3.43712599899998));
#305004=CARTESIAN_POINT('Ctrl Pts',(-2.89710473200006,12.2,3.43494835999999));
#305005=CARTESIAN_POINT('Ctrl Pts',(-2.89710473200006,5.2,3.43494835999999));
#305006=CARTESIAN_POINT('Ctrl Pts',(-2.89710473200006,2.2,3.43494835999999));
#305007=CARTESIAN_POINT('Ctrl Pts',(-2.89660720900006,12.2,3.43277497499999));
#305008=CARTESIAN_POINT('Ctrl Pts',(-2.89660720900006,5.2,3.43277497499999));
#305009=CARTESIAN_POINT('Ctrl Pts',(-2.89660720900006,2.2,3.43277497499999));
#305010=CARTESIAN_POINT('Ctrl Pts',(-2.89610818700006,12.2,3.43060584799999));
#305011=CARTESIAN_POINT('Ctrl Pts',(-2.89610818700006,5.2,3.43060584799999));
#305012=CARTESIAN_POINT('Ctrl Pts',(-2.89610818700006,2.2,3.43060584799999));
#305013=CARTESIAN_POINT('Ctrl Pts',(-2.89560767300005,12.2,3.42844098499998));
#305014=CARTESIAN_POINT('Ctrl Pts',(-2.89560767300005,5.2,3.42844098499998));
#305015=CARTESIAN_POINT('Ctrl Pts',(-2.89560767300005,2.2,3.42844098499998));
#305016=CARTESIAN_POINT('Ctrl Pts',(-2.89510567700006,12.2,3.42628038999998));
#305017=CARTESIAN_POINT('Ctrl Pts',(-2.89510567700006,5.2,3.42628038999998));
#305018=CARTESIAN_POINT('Ctrl Pts',(-2.89510567700006,2.2,3.42628038999998));
#305019=CARTESIAN_POINT('Ctrl Pts',(-2.89460220700006,12.2,3.42412406899999));
#305020=CARTESIAN_POINT('Ctrl Pts',(-2.89460220700006,5.2,3.42412406899999));
#305021=CARTESIAN_POINT('Ctrl Pts',(-2.89460220700006,2.2,3.42412406899999));
#305022=CARTESIAN_POINT('Ctrl Pts',(-2.89409727200006,12.2,3.42197202599999));
#305023=CARTESIAN_POINT('Ctrl Pts',(-2.89409727200006,5.2,3.42197202599999));
#305024=CARTESIAN_POINT('Ctrl Pts',(-2.89409727200006,2.2,3.42197202599999));
#305025=CARTESIAN_POINT('Ctrl Pts',(-2.89359087900006,12.2,3.41982426699998));
#305026=CARTESIAN_POINT('Ctrl Pts',(-2.89359087900006,5.2,3.41982426699998));
#305027=CARTESIAN_POINT('Ctrl Pts',(-2.89359087900006,2.2,3.41982426699998));
#305028=CARTESIAN_POINT('Ctrl Pts',(-2.89308304000006,12.2,3.41768079499998));
#305029=CARTESIAN_POINT('Ctrl Pts',(-2.89308304000006,5.2,3.41768079499998));
#305030=CARTESIAN_POINT('Ctrl Pts',(-2.89308304000006,2.2,3.41768079499998));
#305031=CARTESIAN_POINT('Ctrl Pts',(-2.89257376100006,12.2,3.41554161799999));
#305032=CARTESIAN_POINT('Ctrl Pts',(-2.89257376100006,5.2,3.41554161799999));
#305033=CARTESIAN_POINT('Ctrl Pts',(-2.89257376100006,2.2,3.41554161799999));
#305034=CARTESIAN_POINT('Ctrl Pts',(-2.89206305300006,12.2,3.41340673799999));
#305035=CARTESIAN_POINT('Ctrl Pts',(-2.89206305300006,5.2,3.41340673799999));
#305036=CARTESIAN_POINT('Ctrl Pts',(-2.89206305300006,2.2,3.41340673799999));
#305037=CARTESIAN_POINT('Ctrl Pts',(-2.89155092300006,12.2,3.41127616099998));
#305038=CARTESIAN_POINT('Ctrl Pts',(-2.89155092300006,5.2,3.41127616099998));
#305039=CARTESIAN_POINT('Ctrl Pts',(-2.89155092300006,2.2,3.41127616099998));
#305040=CARTESIAN_POINT('Ctrl Pts',(-2.89103738100006,12.2,3.40914989399998));
#305041=CARTESIAN_POINT('Ctrl Pts',(-2.89103738100006,5.2,3.40914989399998));
#305042=CARTESIAN_POINT('Ctrl Pts',(-2.89103738100006,2.2,3.40914989399998));
#305043=CARTESIAN_POINT('Ctrl Pts',(-2.89052243500006,12.2,3.40702793799998));
#305044=CARTESIAN_POINT('Ctrl Pts',(-2.89052243500006,5.2,3.40702793799998));
#305045=CARTESIAN_POINT('Ctrl Pts',(-2.89052243500006,2.2,3.40702793799998));
#305046=CARTESIAN_POINT('Ctrl Pts',(-2.89000609500006,12.2,3.40491029899999));
#305047=CARTESIAN_POINT('Ctrl Pts',(-2.89000609500006,5.2,3.40491029899999));
#305048=CARTESIAN_POINT('Ctrl Pts',(-2.89000609500006,2.2,3.40491029899999));
#305049=CARTESIAN_POINT('Ctrl Pts',(-2.88948836900006,12.2,3.40279698399998));
#305050=CARTESIAN_POINT('Ctrl Pts',(-2.88948836900006,5.2,3.40279698399998));
#305051=CARTESIAN_POINT('Ctrl Pts',(-2.88948836900006,2.2,3.40279698399998));
#305052=CARTESIAN_POINT('Ctrl Pts',(-2.88896926500006,12.2,3.40068799699999));
#305053=CARTESIAN_POINT('Ctrl Pts',(-2.88896926500006,5.2,3.40068799699999));
#305054=CARTESIAN_POINT('Ctrl Pts',(-2.88896926500006,2.2,3.40068799699999));
#305055=CARTESIAN_POINT('Ctrl Pts',(-2.88844879500005,12.2,3.39858334199998));
#305056=CARTESIAN_POINT('Ctrl Pts',(-2.88844879500005,5.2,3.39858334199998));
#305057=CARTESIAN_POINT('Ctrl Pts',(-2.88844879500005,2.2,3.39858334199998));
#305058=CARTESIAN_POINT('Ctrl Pts',(-2.88792696500006,12.2,3.39648302499998));
#305059=CARTESIAN_POINT('Ctrl Pts',(-2.88792696500006,5.2,3.39648302499998));
#305060=CARTESIAN_POINT('Ctrl Pts',(-2.88792696500006,2.2,3.39648302499998));
#305061=CARTESIAN_POINT('Ctrl Pts',(-2.88740378400006,12.2,3.39438704899998));
#305062=CARTESIAN_POINT('Ctrl Pts',(-2.88740378400006,5.2,3.39438704899998));
#305063=CARTESIAN_POINT('Ctrl Pts',(-2.88740378400006,2.2,3.39438704899998));
#305064=CARTESIAN_POINT('Ctrl Pts',(-2.88687926300006,12.2,3.39229542199998));
#305065=CARTESIAN_POINT('Ctrl Pts',(-2.88687926300006,5.2,3.39229542199998));
#305066=CARTESIAN_POINT('Ctrl Pts',(-2.88687926300006,2.2,3.39229542199998));
#305067=CARTESIAN_POINT('Ctrl Pts',(-2.88635341000006,12.2,3.39020814599999));
#305068=CARTESIAN_POINT('Ctrl Pts',(-2.88635341000006,5.2,3.39020814599999));
#305069=CARTESIAN_POINT('Ctrl Pts',(-2.88635341000006,2.2,3.39020814599999));
#305070=CARTESIAN_POINT('Ctrl Pts',(-2.88582623400006,12.2,3.38812522599999));
#305071=CARTESIAN_POINT('Ctrl Pts',(-2.88582623400006,5.2,3.38812522599999));
#305072=CARTESIAN_POINT('Ctrl Pts',(-2.88582623400006,2.2,3.38812522599999));
#305073=CARTESIAN_POINT('Ctrl Pts',(-2.88529774300006,12.2,3.38604666899998));
#305074=CARTESIAN_POINT('Ctrl Pts',(-2.88529774300006,5.2,3.38604666899998));
#305075=CARTESIAN_POINT('Ctrl Pts',(-2.88529774300006,2.2,3.38604666899998));
#305076=CARTESIAN_POINT('Ctrl Pts',(-2.88476794800005,12.2,3.38397247899999));
#305077=CARTESIAN_POINT('Ctrl Pts',(-2.88476794800005,5.2,3.38397247899999));
#305078=CARTESIAN_POINT('Ctrl Pts',(-2.88476794800005,2.2,3.38397247899999));
#305079=CARTESIAN_POINT('Ctrl Pts',(-2.88423685700006,12.2,3.38190265899998));
#305080=CARTESIAN_POINT('Ctrl Pts',(-2.88423685700006,5.2,3.38190265899998));
#305081=CARTESIAN_POINT('Ctrl Pts',(-2.88423685700006,2.2,3.38190265899998));
#305082=CARTESIAN_POINT('Ctrl Pts',(-2.88370448000005,12.2,3.37983721699998));
#305083=CARTESIAN_POINT('Ctrl Pts',(-2.88370448000005,5.2,3.37983721699998));
#305084=CARTESIAN_POINT('Ctrl Pts',(-2.88370448000005,2.2,3.37983721699998));
#305085=CARTESIAN_POINT('Ctrl Pts',(-2.88317082500006,12.2,3.37777615499999));
#305086=CARTESIAN_POINT('Ctrl Pts',(-2.88317082500006,5.2,3.37777615499999));
#305087=CARTESIAN_POINT('Ctrl Pts',(-2.88317082500006,2.2,3.37777615499999));
#305088=CARTESIAN_POINT('Ctrl Pts',(-2.88263590100006,12.2,3.37571947899999));
#305089=CARTESIAN_POINT('Ctrl Pts',(-2.88263590100006,5.2,3.37571947899999));
#305090=CARTESIAN_POINT('Ctrl Pts',(-2.88263590100006,2.2,3.37571947899999));
#305091=CARTESIAN_POINT('Ctrl Pts',(-2.88209971800006,12.2,3.37366719499999));
#305092=CARTESIAN_POINT('Ctrl Pts',(-2.88209971800006,5.2,3.37366719499999));
#305093=CARTESIAN_POINT('Ctrl Pts',(-2.88209971800006,2.2,3.37366719499999));
#305094=CARTESIAN_POINT('Ctrl Pts',(-2.88156228600006,12.2,3.37161930599999));
#305095=CARTESIAN_POINT('Ctrl Pts',(-2.88156228600006,5.2,3.37161930599999));
#305096=CARTESIAN_POINT('Ctrl Pts',(-2.88156228600006,2.2,3.37161930599999));
#305097=CARTESIAN_POINT('Ctrl Pts',(-2.88102361300006,12.2,3.36957581699998));
#305098=CARTESIAN_POINT('Ctrl Pts',(-2.88102361300006,5.2,3.36957581699998));
#305099=CARTESIAN_POINT('Ctrl Pts',(-2.88102361300006,2.2,3.36957581699998));
#305100=CARTESIAN_POINT('Ctrl Pts',(-2.88048370700006,12.2,3.36753673399999));
#305101=CARTESIAN_POINT('Ctrl Pts',(-2.88048370700006,5.2,3.36753673399999));
#305102=CARTESIAN_POINT('Ctrl Pts',(-2.88048370700006,2.2,3.36753673399999));
#305103=CARTESIAN_POINT('Ctrl Pts',(-2.87994257900006,12.2,3.36550206099999));
#305104=CARTESIAN_POINT('Ctrl Pts',(-2.87994257900006,5.2,3.36550206099999));
#305105=CARTESIAN_POINT('Ctrl Pts',(-2.87994257900006,2.2,3.36550206099999));
#305106=CARTESIAN_POINT('Ctrl Pts',(-2.87940023900005,12.2,3.36347180199999));
#305107=CARTESIAN_POINT('Ctrl Pts',(-2.87940023900005,5.2,3.36347180199999));
#305108=CARTESIAN_POINT('Ctrl Pts',(-2.87940023900005,2.2,3.36347180199999));
#305109=CARTESIAN_POINT('Ctrl Pts',(-2.87885669500006,12.2,3.36144596399999));
#305110=CARTESIAN_POINT('Ctrl Pts',(-2.87885669500006,5.2,3.36144596399999));
#305111=CARTESIAN_POINT('Ctrl Pts',(-2.87885669500006,2.2,3.36144596399999));
#305112=CARTESIAN_POINT('Ctrl Pts',(-2.87831195600006,12.2,3.35942454999999));
#305113=CARTESIAN_POINT('Ctrl Pts',(-2.87831195600006,5.2,3.35942454999999));
#305114=CARTESIAN_POINT('Ctrl Pts',(-2.87831195600006,2.2,3.35942454999999));
#305115=CARTESIAN_POINT('Ctrl Pts',(-2.87776603200005,12.2,3.35740756499998));
#305116=CARTESIAN_POINT('Ctrl Pts',(-2.87776603200005,5.2,3.35740756499998));
#305117=CARTESIAN_POINT('Ctrl Pts',(-2.87776603200005,2.2,3.35740756499998));
#305118=CARTESIAN_POINT('Ctrl Pts',(-2.87721893300006,12.2,3.35539501399998));
#305119=CARTESIAN_POINT('Ctrl Pts',(-2.87721893300006,5.2,3.35539501399998));
#305120=CARTESIAN_POINT('Ctrl Pts',(-2.87721893300006,2.2,3.35539501399998));
#305121=CARTESIAN_POINT('Ctrl Pts',(-2.87667066700006,12.2,3.35338690199999));
#305122=CARTESIAN_POINT('Ctrl Pts',(-2.87667066700006,5.2,3.35338690199999));
#305123=CARTESIAN_POINT('Ctrl Pts',(-2.87667066700006,2.2,3.35338690199999));
#305124=CARTESIAN_POINT('Ctrl Pts',(-2.87612124500006,12.2,3.35138323399998));
#305125=CARTESIAN_POINT('Ctrl Pts',(-2.87612124500006,5.2,3.35138323399998));
#305126=CARTESIAN_POINT('Ctrl Pts',(-2.87612124500006,2.2,3.35138323399998));
#305127=CARTESIAN_POINT('Ctrl Pts',(-2.87557067400006,12.2,3.34938401399998));
#305128=CARTESIAN_POINT('Ctrl Pts',(-2.87557067400006,5.2,3.34938401399998));
#305129=CARTESIAN_POINT('Ctrl Pts',(-2.87557067400006,2.2,3.34938401399998));
#305130=CARTESIAN_POINT('Ctrl Pts',(-2.87501896500005,12.2,3.34738924799999));
#305131=CARTESIAN_POINT('Ctrl Pts',(-2.87501896500005,5.2,3.34738924799999));
#305132=CARTESIAN_POINT('Ctrl Pts',(-2.87501896500005,2.2,3.34738924799999));
#305133=CARTESIAN_POINT('Ctrl Pts',(-2.87446612800006,12.2,3.34539893899999));
#305134=CARTESIAN_POINT('Ctrl Pts',(-2.87446612800006,5.2,3.34539893899999));
#305135=CARTESIAN_POINT('Ctrl Pts',(-2.87446612800006,2.2,3.34539893899999));
#305136=CARTESIAN_POINT('Ctrl Pts',(-2.87391217200006,12.2,3.34341309299998));
#305137=CARTESIAN_POINT('Ctrl Pts',(-2.87391217200006,5.2,3.34341309299998));
#305138=CARTESIAN_POINT('Ctrl Pts',(-2.87391217200006,2.2,3.34341309299998));
#305139=CARTESIAN_POINT('Ctrl Pts',(-2.87335710600006,12.2,3.34143171399998));
#305140=CARTESIAN_POINT('Ctrl Pts',(-2.87335710600006,5.2,3.34143171399998));
#305141=CARTESIAN_POINT('Ctrl Pts',(-2.87335710600006,2.2,3.34143171399998));
#305142=CARTESIAN_POINT('Ctrl Pts',(-2.87280094100006,12.2,3.33945480699998));
#305143=CARTESIAN_POINT('Ctrl Pts',(-2.87280094100006,5.2,3.33945480699998));
#305144=CARTESIAN_POINT('Ctrl Pts',(-2.87280094100006,2.2,3.33945480699998));
#305145=CARTESIAN_POINT('Ctrl Pts',(-2.87224368400006,12.2,3.33748237699999));
#305146=CARTESIAN_POINT('Ctrl Pts',(-2.87224368400006,5.2,3.33748237699999));
#305147=CARTESIAN_POINT('Ctrl Pts',(-2.87224368400006,2.2,3.33748237699999));
#305148=CARTESIAN_POINT('Ctrl Pts',(-2.87168534700006,12.2,3.33551442899999));
#305149=CARTESIAN_POINT('Ctrl Pts',(-2.87168534700006,5.2,3.33551442899999));
#305150=CARTESIAN_POINT('Ctrl Pts',(-2.87168534700006,2.2,3.33551442899999));
#305151=CARTESIAN_POINT('Ctrl Pts',(-2.87112593900006,12.2,3.33355096799998));
#305152=CARTESIAN_POINT('Ctrl Pts',(-2.87112593900006,5.2,3.33355096799998));
#305153=CARTESIAN_POINT('Ctrl Pts',(-2.87112593900006,2.2,3.33355096799998));
#305154=CARTESIAN_POINT('Ctrl Pts',(-2.87056546800006,12.2,3.33159199699999));
#305155=CARTESIAN_POINT('Ctrl Pts',(-2.87056546800006,5.2,3.33159199699999));
#305156=CARTESIAN_POINT('Ctrl Pts',(-2.87056546800006,2.2,3.33159199699999));
#305157=CARTESIAN_POINT('Ctrl Pts',(-2.87000394500006,12.2,3.32963752199999));
#305158=CARTESIAN_POINT('Ctrl Pts',(-2.87000394500006,5.2,3.32963752199999));
#305159=CARTESIAN_POINT('Ctrl Pts',(-2.87000394500006,2.2,3.32963752199999));
#305160=CARTESIAN_POINT('Ctrl Pts',(-2.86944138000006,12.2,3.32768754699998));
#305161=CARTESIAN_POINT('Ctrl Pts',(-2.86944138000006,5.2,3.32768754699998));
#305162=CARTESIAN_POINT('Ctrl Pts',(-2.86944138000006,2.2,3.32768754699998));
#305163=CARTESIAN_POINT('Ctrl Pts',(-2.86887778300006,12.2,3.32574207799999));
#305164=CARTESIAN_POINT('Ctrl Pts',(-2.86887778300006,5.2,3.32574207799999));
#305165=CARTESIAN_POINT('Ctrl Pts',(-2.86887778300006,2.2,3.32574207799999));
#305166=CARTESIAN_POINT('Ctrl Pts',(-2.86831316100006,12.2,3.32380111699998));
#305167=CARTESIAN_POINT('Ctrl Pts',(-2.86831316100006,5.2,3.32380111699998));
#305168=CARTESIAN_POINT('Ctrl Pts',(-2.86831316100006,2.2,3.32380111699998));
#305169=CARTESIAN_POINT('Ctrl Pts',(-2.86774752600006,12.2,3.32186467299999));
#305170=CARTESIAN_POINT('Ctrl Pts',(-2.86774752600006,5.2,3.32186467299999));
#305171=CARTESIAN_POINT('Ctrl Pts',(-2.86774752600006,2.2,3.32186467299999));
#305172=CARTESIAN_POINT('Ctrl Pts',(-2.86718088800006,12.2,3.31993274599999));
#305173=CARTESIAN_POINT('Ctrl Pts',(-2.86718088800006,5.2,3.31993274599999));
#305174=CARTESIAN_POINT('Ctrl Pts',(-2.86718088800006,2.2,3.31993274599999));
#305175=CARTESIAN_POINT('Ctrl Pts',(-2.86661325600006,12.2,3.31800534399999));
#305176=CARTESIAN_POINT('Ctrl Pts',(-2.86661325600006,5.2,3.31800534399999));
#305177=CARTESIAN_POINT('Ctrl Pts',(-2.86661325600006,2.2,3.31800534399999));
#305178=CARTESIAN_POINT('Ctrl Pts',(-2.86604464000006,12.2,3.31608247099999));
#305179=CARTESIAN_POINT('Ctrl Pts',(-2.86604464000006,5.2,3.31608247099999));
#305180=CARTESIAN_POINT('Ctrl Pts',(-2.86604464000006,2.2,3.31608247099999));
#305181=CARTESIAN_POINT('Ctrl Pts',(-2.86547505000006,12.2,3.31416412999998));
#305182=CARTESIAN_POINT('Ctrl Pts',(-2.86547505000006,5.2,3.31416412999998));
#305183=CARTESIAN_POINT('Ctrl Pts',(-2.86547505000006,2.2,3.31416412999998));
#305184=CARTESIAN_POINT('Ctrl Pts',(-2.86490449600006,12.2,3.31225032799999));
#305185=CARTESIAN_POINT('Ctrl Pts',(-2.86490449600006,5.2,3.31225032799999));
#305186=CARTESIAN_POINT('Ctrl Pts',(-2.86490449600006,2.2,3.31225032799999));
#305187=CARTESIAN_POINT('Ctrl Pts',(-2.86433298600006,12.2,3.31034106699998));
#305188=CARTESIAN_POINT('Ctrl Pts',(-2.86433298600006,5.2,3.31034106699998));
#305189=CARTESIAN_POINT('Ctrl Pts',(-2.86433298600006,2.2,3.31034106699998));
#305190=CARTESIAN_POINT('Ctrl Pts',(-2.86376053200006,12.2,3.30843635499999));
#305191=CARTESIAN_POINT('Ctrl Pts',(-2.86376053200006,5.2,3.30843635499999));
#305192=CARTESIAN_POINT('Ctrl Pts',(-2.86376053200006,2.2,3.30843635499999));
#305193=CARTESIAN_POINT('Ctrl Pts',(-2.86318714300006,12.2,3.30653619399998));
#305194=CARTESIAN_POINT('Ctrl Pts',(-2.86318714300006,5.2,3.30653619399998));
#305195=CARTESIAN_POINT('Ctrl Pts',(-2.86318714300006,2.2,3.30653619399998));
#305196=CARTESIAN_POINT('Ctrl Pts',(-2.86261282900006,12.2,3.30464058799999));
#305197=CARTESIAN_POINT('Ctrl Pts',(-2.86261282900006,5.2,3.30464058799999));
#305198=CARTESIAN_POINT('Ctrl Pts',(-2.86261282900006,2.2,3.30464058799999));
#305199=CARTESIAN_POINT('Ctrl Pts',(-2.86203760000005,12.2,3.30274954499998));
#305200=CARTESIAN_POINT('Ctrl Pts',(-2.86203760000005,5.2,3.30274954499998));
#305201=CARTESIAN_POINT('Ctrl Pts',(-2.86203760000005,2.2,3.30274954499998));
#305202=CARTESIAN_POINT('Ctrl Pts',(-2.86146146600006,12.2,3.30086306599998));
#305203=CARTESIAN_POINT('Ctrl Pts',(-2.86146146600006,5.2,3.30086306599998));
#305204=CARTESIAN_POINT('Ctrl Pts',(-2.86146146600006,2.2,3.30086306599998));
#305205=CARTESIAN_POINT('Ctrl Pts',(-2.86088443800006,12.2,3.29898115899999));
#305206=CARTESIAN_POINT('Ctrl Pts',(-2.86088443800006,5.2,3.29898115899999));
#305207=CARTESIAN_POINT('Ctrl Pts',(-2.86088443800006,2.2,3.29898115899999));
#305208=CARTESIAN_POINT('Ctrl Pts',(-2.86030652300005,12.2,3.29710382599998));
#305209=CARTESIAN_POINT('Ctrl Pts',(-2.86030652300005,5.2,3.29710382599998));
#305210=CARTESIAN_POINT('Ctrl Pts',(-2.86030652300005,2.2,3.29710382599998));
#305211=CARTESIAN_POINT('Ctrl Pts',(-2.85972773500006,12.2,3.29523107299998));
#305212=CARTESIAN_POINT('Ctrl Pts',(-2.85972773500006,5.2,3.29523107299998));
#305213=CARTESIAN_POINT('Ctrl Pts',(-2.85972773500006,2.2,3.29523107299998));
#305214=CARTESIAN_POINT('Ctrl Pts',(-2.85914808100005,12.2,3.29336290299998));
#305215=CARTESIAN_POINT('Ctrl Pts',(-2.85914808100005,5.2,3.29336290299998));
#305216=CARTESIAN_POINT('Ctrl Pts',(-2.85914808100005,2.2,3.29336290299998));
#305217=CARTESIAN_POINT('Ctrl Pts',(-2.85856757300006,12.2,3.29149932199999));
#305218=CARTESIAN_POINT('Ctrl Pts',(-2.85856757300006,5.2,3.29149932199999));
#305219=CARTESIAN_POINT('Ctrl Pts',(-2.85856757300006,2.2,3.29149932199999));
#305220=CARTESIAN_POINT('Ctrl Pts',(-2.85798621900006,12.2,3.28964033399998));
#305221=CARTESIAN_POINT('Ctrl Pts',(-2.85798621900006,5.2,3.28964033399998));
#305222=CARTESIAN_POINT('Ctrl Pts',(-2.85798621900006,2.2,3.28964033399998));
#305223=CARTESIAN_POINT('Ctrl Pts',(-2.85740403200006,12.2,3.28778594499998));
#305224=CARTESIAN_POINT('Ctrl Pts',(-2.85740403200006,5.2,3.28778594499998));
#305225=CARTESIAN_POINT('Ctrl Pts',(-2.85740403200006,2.2,3.28778594499998));
#305226=CARTESIAN_POINT('Ctrl Pts',(-2.85682101900006,12.2,3.28593615699998));
#305227=CARTESIAN_POINT('Ctrl Pts',(-2.85682101900006,5.2,3.28593615699998));
#305228=CARTESIAN_POINT('Ctrl Pts',(-2.85682101900006,2.2,3.28593615699998));
#305229=CARTESIAN_POINT('Ctrl Pts',(-2.85623719200006,12.2,3.28409097699998));
#305230=CARTESIAN_POINT('Ctrl Pts',(-2.85623719200006,5.2,3.28409097699998));
#305231=CARTESIAN_POINT('Ctrl Pts',(-2.85623719200006,2.2,3.28409097699998));
#305232=CARTESIAN_POINT('Ctrl Pts',(-2.85565256200006,12.2,3.28225040699999));
#305233=CARTESIAN_POINT('Ctrl Pts',(-2.85565256200006,5.2,3.28225040699999));
#305234=CARTESIAN_POINT('Ctrl Pts',(-2.85565256200006,2.2,3.28225040699999));
#305235=CARTESIAN_POINT('Ctrl Pts',(-2.85506713700005,12.2,3.28041445499998));
#305236=CARTESIAN_POINT('Ctrl Pts',(-2.85506713700005,5.2,3.28041445499998));
#305237=CARTESIAN_POINT('Ctrl Pts',(-2.85506713700005,2.2,3.28041445499998));
#305238=CARTESIAN_POINT('Ctrl Pts',(-2.85448092800006,12.2,3.27858312199999));
#305239=CARTESIAN_POINT('Ctrl Pts',(-2.85448092800006,5.2,3.27858312199999));
#305240=CARTESIAN_POINT('Ctrl Pts',(-2.85448092800006,2.2,3.27858312199999));
#305241=CARTESIAN_POINT('Ctrl Pts',(-2.85389394600006,12.2,3.27675641499999));
#305242=CARTESIAN_POINT('Ctrl Pts',(-2.85389394600006,5.2,3.27675641499999));
#305243=CARTESIAN_POINT('Ctrl Pts',(-2.85389394600006,2.2,3.27675641499999));
#305244=CARTESIAN_POINT('Ctrl Pts',(-2.85330620200006,12.2,3.27493433699999));
#305245=CARTESIAN_POINT('Ctrl Pts',(-2.85330620200006,5.2,3.27493433699999));
#305246=CARTESIAN_POINT('Ctrl Pts',(-2.85330620200006,2.2,3.27493433699999));
#305247=CARTESIAN_POINT('Ctrl Pts',(-2.85271770300006,12.2,3.27311689299999));
#305248=CARTESIAN_POINT('Ctrl Pts',(-2.85271770300006,5.2,3.27311689299999));
#305249=CARTESIAN_POINT('Ctrl Pts',(-2.85271770300006,2.2,3.27311689299999));
#305250=CARTESIAN_POINT('Ctrl Pts',(-2.85212846300006,12.2,3.27130408899999));
#305251=CARTESIAN_POINT('Ctrl Pts',(-2.85212846300006,5.2,3.27130408899999));
#305252=CARTESIAN_POINT('Ctrl Pts',(-2.85212846300006,2.2,3.27130408899999));
#305253=CARTESIAN_POINT('Ctrl Pts',(-2.85153849100006,12.2,3.26949592699999));
#305254=CARTESIAN_POINT('Ctrl Pts',(-2.85153849100006,5.2,3.26949592699999));
#305255=CARTESIAN_POINT('Ctrl Pts',(-2.85153849100006,2.2,3.26949592699999));
#305256=CARTESIAN_POINT('Ctrl Pts',(-2.85094779600006,12.2,3.26769241299999));
#305257=CARTESIAN_POINT('Ctrl Pts',(-2.85094779600006,5.2,3.26769241299999));
#305258=CARTESIAN_POINT('Ctrl Pts',(-2.85094779600006,2.2,3.26769241299999));
#305259=CARTESIAN_POINT('Ctrl Pts',(-2.85035639200005,12.2,3.26589355199999));
#305260=CARTESIAN_POINT('Ctrl Pts',(-2.85035639200005,5.2,3.26589355199999));
#305261=CARTESIAN_POINT('Ctrl Pts',(-2.85035639200005,2.2,3.26589355199999));
#305262=CARTESIAN_POINT('Ctrl Pts',(-2.84976428500006,12.2,3.26409934599998));
#305263=CARTESIAN_POINT('Ctrl Pts',(-2.84976428500006,5.2,3.26409934599998));
#305264=CARTESIAN_POINT('Ctrl Pts',(-2.84976428500006,2.2,3.26409934599998));
#305265=CARTESIAN_POINT('Ctrl Pts',(-2.84917148800006,12.2,3.26230980199998));
#305266=CARTESIAN_POINT('Ctrl Pts',(-2.84917148800006,5.2,3.26230980199998));
#305267=CARTESIAN_POINT('Ctrl Pts',(-2.84917148800006,2.2,3.26230980199998));
#305268=CARTESIAN_POINT('Ctrl Pts',(-2.84857801100005,12.2,3.26052492399998));
#305269=CARTESIAN_POINT('Ctrl Pts',(-2.84857801100005,5.2,3.26052492399998));
#305270=CARTESIAN_POINT('Ctrl Pts',(-2.84857801100005,2.2,3.26052492399998));
#305271=CARTESIAN_POINT('Ctrl Pts',(-2.84798386500006,12.2,3.25874471599998));
#305272=CARTESIAN_POINT('Ctrl Pts',(-2.84798386500006,5.2,3.25874471599998));
#305273=CARTESIAN_POINT('Ctrl Pts',(-2.84798386500006,2.2,3.25874471599998));
#305274=CARTESIAN_POINT('Ctrl Pts',(-2.84738906000006,12.2,3.25696918299998));
#305275=CARTESIAN_POINT('Ctrl Pts',(-2.84738906000006,5.2,3.25696918299998));
#305276=CARTESIAN_POINT('Ctrl Pts',(-2.84738906000006,2.2,3.25696918299998));
#305277=CARTESIAN_POINT('Ctrl Pts',(-2.84679360500005,12.2,3.25519832899998));
#305278=CARTESIAN_POINT('Ctrl Pts',(-2.84679360500005,5.2,3.25519832899998));
#305279=CARTESIAN_POINT('Ctrl Pts',(-2.84679360500005,2.2,3.25519832899998));
#305280=CARTESIAN_POINT('Ctrl Pts',(-2.84619751300006,12.2,3.25343215699998));
#305281=CARTESIAN_POINT('Ctrl Pts',(-2.84619751300006,5.2,3.25343215699998));
#305282=CARTESIAN_POINT('Ctrl Pts',(-2.84619751300006,2.2,3.25343215699998));
#305283=CARTESIAN_POINT('Ctrl Pts',(-2.84560079400006,12.2,3.25167067399998));
#305284=CARTESIAN_POINT('Ctrl Pts',(-2.84560079400006,5.2,3.25167067399998));
#305285=CARTESIAN_POINT('Ctrl Pts',(-2.84560079400006,2.2,3.25167067399998));
#305286=CARTESIAN_POINT('Ctrl Pts',(-2.84500345900006,12.2,3.24991388399998));
#305287=CARTESIAN_POINT('Ctrl Pts',(-2.84500345900006,5.2,3.24991388399998));
#305288=CARTESIAN_POINT('Ctrl Pts',(-2.84500345900006,2.2,3.24991388399998));
#305289=CARTESIAN_POINT('Ctrl Pts',(-2.84440551700006,12.2,3.24816178999999));
#305290=CARTESIAN_POINT('Ctrl Pts',(-2.84440551700006,5.2,3.24816178999999));
#305291=CARTESIAN_POINT('Ctrl Pts',(-2.84440551700006,2.2,3.24816178999999));
#305292=CARTESIAN_POINT('Ctrl Pts',(-2.84380697900006,12.2,3.24641439699998));
#305293=CARTESIAN_POINT('Ctrl Pts',(-2.84380697900006,5.2,3.24641439699998));
#305294=CARTESIAN_POINT('Ctrl Pts',(-2.84380697900006,2.2,3.24641439699998));
#305295=CARTESIAN_POINT('Ctrl Pts',(-2.84320785800006,12.2,3.24467170999998));
#305296=CARTESIAN_POINT('Ctrl Pts',(-2.84320785800006,5.2,3.24467170999998));
#305297=CARTESIAN_POINT('Ctrl Pts',(-2.84320785800006,2.2,3.24467170999998));
#305298=CARTESIAN_POINT('Ctrl Pts',(-2.84260816200006,12.2,3.24293373299999));
#305299=CARTESIAN_POINT('Ctrl Pts',(-2.84260816200006,5.2,3.24293373299999));
#305300=CARTESIAN_POINT('Ctrl Pts',(-2.84260816200006,2.2,3.24293373299999));
#305301=CARTESIAN_POINT('Ctrl Pts',(-2.84200790300006,12.2,3.24120046999998));
#305302=CARTESIAN_POINT('Ctrl Pts',(-2.84200790300006,5.2,3.24120046999998));
#305303=CARTESIAN_POINT('Ctrl Pts',(-2.84200790300006,2.2,3.24120046999998));
#305304=CARTESIAN_POINT('Ctrl Pts',(-2.84140709100006,12.2,3.23947192599999));
#305305=CARTESIAN_POINT('Ctrl Pts',(-2.84140709100006,5.2,3.23947192599999));
#305306=CARTESIAN_POINT('Ctrl Pts',(-2.84140709100006,2.2,3.23947192599999));
#305307=CARTESIAN_POINT('Ctrl Pts',(-2.84080573800006,12.2,3.23774810599998));
#305308=CARTESIAN_POINT('Ctrl Pts',(-2.84080573800006,5.2,3.23774810599998));
#305309=CARTESIAN_POINT('Ctrl Pts',(-2.84080573800006,2.2,3.23774810599998));
#305310=CARTESIAN_POINT('Ctrl Pts',(-2.84020385300006,12.2,3.23602901199998));
#305311=CARTESIAN_POINT('Ctrl Pts',(-2.84020385300006,5.2,3.23602901199998));
#305312=CARTESIAN_POINT('Ctrl Pts',(-2.84020385300006,2.2,3.23602901199998));
#305313=CARTESIAN_POINT('Ctrl Pts',(-2.83960144900006,12.2,3.23431465199998));
#305314=CARTESIAN_POINT('Ctrl Pts',(-2.83960144900006,5.2,3.23431465199998));
#305315=CARTESIAN_POINT('Ctrl Pts',(-2.83960144900006,2.2,3.23431465199998));
#305316=CARTESIAN_POINT('Ctrl Pts',(-2.83899853600006,12.2,3.23260502699998));
#305317=CARTESIAN_POINT('Ctrl Pts',(-2.83899853600006,5.2,3.23260502699998));
#305318=CARTESIAN_POINT('Ctrl Pts',(-2.83899853600006,2.2,3.23260502699998));
#305319=CARTESIAN_POINT('Ctrl Pts',(-2.83839512400006,12.2,3.23090014199998));
#305320=CARTESIAN_POINT('Ctrl Pts',(-2.83839512400006,5.2,3.23090014199998));
#305321=CARTESIAN_POINT('Ctrl Pts',(-2.83839512400006,2.2,3.23090014199998));
#305322=CARTESIAN_POINT('Ctrl Pts',(-2.83779122500006,12.2,3.22920000399999));
#305323=CARTESIAN_POINT('Ctrl Pts',(-2.83779122500006,5.2,3.22920000399999));
#305324=CARTESIAN_POINT('Ctrl Pts',(-2.83779122500006,2.2,3.22920000399999));
#305325=CARTESIAN_POINT('Ctrl Pts',(-2.83718684900006,12.2,3.22750461399998));
#305326=CARTESIAN_POINT('Ctrl Pts',(-2.83718684900006,5.2,3.22750461399998));
#305327=CARTESIAN_POINT('Ctrl Pts',(-2.83718684900006,2.2,3.22750461399998));
#305328=CARTESIAN_POINT('Ctrl Pts',(-2.83658200700006,12.2,3.22581397899998));
#305329=CARTESIAN_POINT('Ctrl Pts',(-2.83658200700006,5.2,3.22581397899998));
#305330=CARTESIAN_POINT('Ctrl Pts',(-2.83658200700006,2.2,3.22581397899998));
#305331=CARTESIAN_POINT('Ctrl Pts',(-2.83597671200006,12.2,3.22412810099999));
#305332=CARTESIAN_POINT('Ctrl Pts',(-2.83597671200006,5.2,3.22412810099999));
#305333=CARTESIAN_POINT('Ctrl Pts',(-2.83597671200006,2.2,3.22412810099999));
#305334=CARTESIAN_POINT('Ctrl Pts',(-2.83537097200006,12.2,3.22244698499999));
#305335=CARTESIAN_POINT('Ctrl Pts',(-2.83537097200006,5.2,3.22244698499999));
#305336=CARTESIAN_POINT('Ctrl Pts',(-2.83537097200006,2.2,3.22244698499999));
#305337=CARTESIAN_POINT('Ctrl Pts',(-2.83476480100005,12.2,3.22077063699999));
#305338=CARTESIAN_POINT('Ctrl Pts',(-2.83476480100005,5.2,3.22077063699999));
#305339=CARTESIAN_POINT('Ctrl Pts',(-2.83476480100005,2.2,3.22077063699999));
#305340=CARTESIAN_POINT('Ctrl Pts',(-2.83415820700006,12.2,3.21909905899999));
#305341=CARTESIAN_POINT('Ctrl Pts',(-2.83415820700006,5.2,3.21909905899999));
#305342=CARTESIAN_POINT('Ctrl Pts',(-2.83415820700006,2.2,3.21909905899999));
#305343=CARTESIAN_POINT('Ctrl Pts',(-2.83355120500006,12.2,3.21743225699999));
#305344=CARTESIAN_POINT('Ctrl Pts',(-2.83355120500006,5.2,3.21743225699999));
#305345=CARTESIAN_POINT('Ctrl Pts',(-2.83355120500006,2.2,3.21743225699999));
#305346=CARTESIAN_POINT('Ctrl Pts',(-2.83294380200006,12.2,3.21577023399998));
#305347=CARTESIAN_POINT('Ctrl Pts',(-2.83294380200006,5.2,3.21577023399998));
#305348=CARTESIAN_POINT('Ctrl Pts',(-2.83294380200006,2.2,3.21577023399998));
#305349=CARTESIAN_POINT('Ctrl Pts',(-2.83233601100005,12.2,3.21411299499999));
#305350=CARTESIAN_POINT('Ctrl Pts',(-2.83233601100005,5.2,3.21411299499999));
#305351=CARTESIAN_POINT('Ctrl Pts',(-2.83233601100005,2.2,3.21411299499999));
#305352=CARTESIAN_POINT('Ctrl Pts',(-2.83172784300006,12.2,3.21246054399998));
#305353=CARTESIAN_POINT('Ctrl Pts',(-2.83172784300006,5.2,3.21246054399998));
#305354=CARTESIAN_POINT('Ctrl Pts',(-2.83172784300006,2.2,3.21246054399998));
#305355=CARTESIAN_POINT('Ctrl Pts',(-2.83111930900006,12.2,3.21081288599999));
#305356=CARTESIAN_POINT('Ctrl Pts',(-2.83111930900006,5.2,3.21081288599999));
#305357=CARTESIAN_POINT('Ctrl Pts',(-2.83111930900006,2.2,3.21081288599999));
#305358=CARTESIAN_POINT('Ctrl Pts',(-2.83051042200006,12.2,3.20917002399998));
#305359=CARTESIAN_POINT('Ctrl Pts',(-2.83051042200006,5.2,3.20917002399998));
#305360=CARTESIAN_POINT('Ctrl Pts',(-2.83051042200006,2.2,3.20917002399998));
#305361=CARTESIAN_POINT('Ctrl Pts',(-2.82990119000006,12.2,3.20753196299999));
#305362=CARTESIAN_POINT('Ctrl Pts',(-2.82990119000006,5.2,3.20753196299999));
#305363=CARTESIAN_POINT('Ctrl Pts',(-2.82990119000006,2.2,3.20753196299999));
#305364=CARTESIAN_POINT('Ctrl Pts',(-2.82929162700006,12.2,3.20589870799999));
#305365=CARTESIAN_POINT('Ctrl Pts',(-2.82929162700006,5.2,3.20589870799999));
#305366=CARTESIAN_POINT('Ctrl Pts',(-2.82929162700006,2.2,3.20589870799999));
#305367=CARTESIAN_POINT('Ctrl Pts',(-2.82868174300006,12.2,3.20427026199999));
#305368=CARTESIAN_POINT('Ctrl Pts',(-2.82868174300006,5.2,3.20427026199999));
#305369=CARTESIAN_POINT('Ctrl Pts',(-2.82868174300006,2.2,3.20427026199999));
#305370=CARTESIAN_POINT('Ctrl Pts',(-2.82807155000006,12.2,3.20264662899999));
#305371=CARTESIAN_POINT('Ctrl Pts',(-2.82807155000006,5.2,3.20264662899999));
#305372=CARTESIAN_POINT('Ctrl Pts',(-2.82807155000006,2.2,3.20264662899999));
#305373=CARTESIAN_POINT('Ctrl Pts',(-2.82746105800005,12.2,3.20102781399999));
#305374=CARTESIAN_POINT('Ctrl Pts',(-2.82746105800005,5.2,3.20102781399999));
#305375=CARTESIAN_POINT('Ctrl Pts',(-2.82746105800005,2.2,3.20102781399999));
#305376=CARTESIAN_POINT('Ctrl Pts',(-2.82685028000006,12.2,3.19941382199998));
#305377=CARTESIAN_POINT('Ctrl Pts',(-2.82685028000006,5.2,3.19941382199998));
#305378=CARTESIAN_POINT('Ctrl Pts',(-2.82685028000006,2.2,3.19941382199998));
#305379=CARTESIAN_POINT('Ctrl Pts',(-2.82623922700005,12.2,3.19780465599998));
#305380=CARTESIAN_POINT('Ctrl Pts',(-2.82623922700005,5.2,3.19780465599998));
#305381=CARTESIAN_POINT('Ctrl Pts',(-2.82623922700005,2.2,3.19780465599998));
#305382=CARTESIAN_POINT('Ctrl Pts',(-2.82562791000006,12.2,3.19620032099999));
#305383=CARTESIAN_POINT('Ctrl Pts',(-2.82562791000006,5.2,3.19620032099999));
#305384=CARTESIAN_POINT('Ctrl Pts',(-2.82562791000006,2.2,3.19620032099999));
#305385=CARTESIAN_POINT('Ctrl Pts',(-2.82501634000006,12.2,3.19460081899998));
#305386=CARTESIAN_POINT('Ctrl Pts',(-2.82501634000006,5.2,3.19460081899998));
#305387=CARTESIAN_POINT('Ctrl Pts',(-2.82501634000006,2.2,3.19460081899998));
#305388=CARTESIAN_POINT('Ctrl Pts',(-2.82440452900006,12.2,3.19300615799998));
#305389=CARTESIAN_POINT('Ctrl Pts',(-2.82440452900006,5.2,3.19300615799998));
#305390=CARTESIAN_POINT('Ctrl Pts',(-2.82440452900006,2.2,3.19300615799998));
#305391=CARTESIAN_POINT('Ctrl Pts',(-2.82379248900006,12.2,3.19141633799998));
#305392=CARTESIAN_POINT('Ctrl Pts',(-2.82379248900006,5.2,3.19141633799998));
#305393=CARTESIAN_POINT('Ctrl Pts',(-2.82379248900006,2.2,3.19141633799998));
#305394=CARTESIAN_POINT('Ctrl Pts',(-2.82318023000005,12.2,3.18983136699998));
#305395=CARTESIAN_POINT('Ctrl Pts',(-2.82318023000005,5.2,3.18983136699998));
#305396=CARTESIAN_POINT('Ctrl Pts',(-2.82318023000005,2.2,3.18983136699998));
#305397=CARTESIAN_POINT('Ctrl Pts',(-2.82256776600006,12.2,3.18825124699998));
#305398=CARTESIAN_POINT('Ctrl Pts',(-2.82256776600006,5.2,3.18825124699998));
#305399=CARTESIAN_POINT('Ctrl Pts',(-2.82256776600006,2.2,3.18825124699998));
#305400=CARTESIAN_POINT('Ctrl Pts',(-2.82195510700006,12.2,3.18667598099999));
#305401=CARTESIAN_POINT('Ctrl Pts',(-2.82195510700006,5.2,3.18667598099999));
#305402=CARTESIAN_POINT('Ctrl Pts',(-2.82195510700006,2.2,3.18667598099999));
#305403=CARTESIAN_POINT('Ctrl Pts',(-2.82134226500005,12.2,3.18510557699998));
#305404=CARTESIAN_POINT('Ctrl Pts',(-2.82134226500005,5.2,3.18510557699998));
#305405=CARTESIAN_POINT('Ctrl Pts',(-2.82134226500005,2.2,3.18510557699998));
#305406=CARTESIAN_POINT('Ctrl Pts',(-2.82072925100006,12.2,3.18354003499999));
#305407=CARTESIAN_POINT('Ctrl Pts',(-2.82072925100006,5.2,3.18354003499999));
#305408=CARTESIAN_POINT('Ctrl Pts',(-2.82072925100006,2.2,3.18354003499999));
#305409=CARTESIAN_POINT('Ctrl Pts',(-2.82011607700006,12.2,3.18197936199999));
#305410=CARTESIAN_POINT('Ctrl Pts',(-2.82011607700006,5.2,3.18197936199999));
#305411=CARTESIAN_POINT('Ctrl Pts',(-2.82011607700006,2.2,3.18197936199999));
#305412=CARTESIAN_POINT('Ctrl Pts',(-2.81950275500006,12.2,3.18042356099999));
#305413=CARTESIAN_POINT('Ctrl Pts',(-2.81950275500006,5.2,3.18042356099999));
#305414=CARTESIAN_POINT('Ctrl Pts',(-2.81950275500006,2.2,3.18042356099999));
#305415=CARTESIAN_POINT('Ctrl Pts',(-2.81888929700005,12.2,3.17887263499999));
#305416=CARTESIAN_POINT('Ctrl Pts',(-2.81888929700005,5.2,3.17887263499999));
#305417=CARTESIAN_POINT('Ctrl Pts',(-2.81888929700005,2.2,3.17887263499999));
#305418=CARTESIAN_POINT('Ctrl Pts',(-2.81827571400005,12.2,3.17732658999999));
#305419=CARTESIAN_POINT('Ctrl Pts',(-2.81827571400005,5.2,3.17732658999999));
#305420=CARTESIAN_POINT('Ctrl Pts',(-2.81827571400005,2.2,3.17732658999999));
#305421=CARTESIAN_POINT('Ctrl Pts',(-2.81766201800006,12.2,3.17578542999998));
#305422=CARTESIAN_POINT('Ctrl Pts',(-2.81766201800006,5.2,3.17578542999998));
#305423=CARTESIAN_POINT('Ctrl Pts',(-2.81766201800006,2.2,3.17578542999998));
#305424=CARTESIAN_POINT('Ctrl Pts',(-2.81704822000005,12.2,3.17424915799998));
#305425=CARTESIAN_POINT('Ctrl Pts',(-2.81704822000005,5.2,3.17424915799998));
#305426=CARTESIAN_POINT('Ctrl Pts',(-2.81704822000005,2.2,3.17424915799998));
#305427=CARTESIAN_POINT('Ctrl Pts',(-2.81643433500005,12.2,3.17271777899998));
#305428=CARTESIAN_POINT('Ctrl Pts',(-2.81643433500005,5.2,3.17271777899998));
#305429=CARTESIAN_POINT('Ctrl Pts',(-2.81643433500005,2.2,3.17271777899998));
#305430=CARTESIAN_POINT('Ctrl Pts',(-2.81582037000006,12.2,3.17119129599998));
#305431=CARTESIAN_POINT('Ctrl Pts',(-2.81582037000006,5.2,3.17119129599998));
#305432=CARTESIAN_POINT('Ctrl Pts',(-2.81582037000006,2.2,3.17119129599998));
#305433=CARTESIAN_POINT('Ctrl Pts',(-2.81520634200006,12.2,3.16966971399999));
#305434=CARTESIAN_POINT('Ctrl Pts',(-2.81520634200006,5.2,3.16966971399999));
#305435=CARTESIAN_POINT('Ctrl Pts',(-2.81520634200006,2.2,3.16966971399999));
#305436=CARTESIAN_POINT('Ctrl Pts',(-2.81459225800006,12.2,3.16815303599999));
#305437=CARTESIAN_POINT('Ctrl Pts',(-2.81459225800006,5.2,3.16815303599999));
#305438=CARTESIAN_POINT('Ctrl Pts',(-2.81459225800006,2.2,3.16815303599999));
#305439=CARTESIAN_POINT('Ctrl Pts',(-2.81397813400006,12.2,3.16664126899998));
#305440=CARTESIAN_POINT('Ctrl Pts',(-2.81397813400006,5.2,3.16664126899998));
#305441=CARTESIAN_POINT('Ctrl Pts',(-2.81397813400006,2.2,3.16664126899998));
#305442=CARTESIAN_POINT('Ctrl Pts',(-2.81336398000006,12.2,3.16513441199999));
#305443=CARTESIAN_POINT('Ctrl Pts',(-2.81336398000006,5.2,3.16513441199999));
#305444=CARTESIAN_POINT('Ctrl Pts',(-2.81336398000006,2.2,3.16513441199999));
#305445=CARTESIAN_POINT('Ctrl Pts',(-2.81274980700006,12.2,3.16363247299999));
#305446=CARTESIAN_POINT('Ctrl Pts',(-2.81274980700006,5.2,3.16363247299999));
#305447=CARTESIAN_POINT('Ctrl Pts',(-2.81274980700006,2.2,3.16363247299999));
#305448=CARTESIAN_POINT('Ctrl Pts',(-2.81213563000006,12.2,3.16213545599999));
#305449=CARTESIAN_POINT('Ctrl Pts',(-2.81213563000006,5.2,3.16213545599999));
#305450=CARTESIAN_POINT('Ctrl Pts',(-2.81213563000006,2.2,3.16213545599999));
#305451=CARTESIAN_POINT('Ctrl Pts',(-2.81152145800006,12.2,3.16064336299998));
#305452=CARTESIAN_POINT('Ctrl Pts',(-2.81152145800006,5.2,3.16064336299998));
#305453=CARTESIAN_POINT('Ctrl Pts',(-2.81152145800006,2.2,3.16064336299998));
#305454=CARTESIAN_POINT('Ctrl Pts',(-2.81090730500006,12.2,3.15915619899998));
#305455=CARTESIAN_POINT('Ctrl Pts',(-2.81090730500006,5.2,3.15915619899998));
#305456=CARTESIAN_POINT('Ctrl Pts',(-2.81090730500006,2.2,3.15915619899998));
#305457=CARTESIAN_POINT('Ctrl Pts',(-2.81029318300006,12.2,3.15767396799998));
#305458=CARTESIAN_POINT('Ctrl Pts',(-2.81029318300006,5.2,3.15767396799998));
#305459=CARTESIAN_POINT('Ctrl Pts',(-2.81029318300006,2.2,3.15767396799998));
#305460=CARTESIAN_POINT('Ctrl Pts',(-2.80967910300005,12.2,3.15619667399999));
#305461=CARTESIAN_POINT('Ctrl Pts',(-2.80967910300005,5.2,3.15619667399999));
#305462=CARTESIAN_POINT('Ctrl Pts',(-2.80967910300005,2.2,3.15619667399999));
#305463=CARTESIAN_POINT('Ctrl Pts',(-2.80906507800006,12.2,3.15472431999999));
#305464=CARTESIAN_POINT('Ctrl Pts',(-2.80906507800006,5.2,3.15472431999999));
#305465=CARTESIAN_POINT('Ctrl Pts',(-2.80906507800006,2.2,3.15472431999999));
#305466=CARTESIAN_POINT('Ctrl Pts',(-2.80845112000006,12.2,3.15325691099999));
#305467=CARTESIAN_POINT('Ctrl Pts',(-2.80845112000006,5.2,3.15325691099999));
#305468=CARTESIAN_POINT('Ctrl Pts',(-2.80845112000006,2.2,3.15325691099999));
#305469=CARTESIAN_POINT('Ctrl Pts',(-2.80783724200006,12.2,3.15179445199998));
#305470=CARTESIAN_POINT('Ctrl Pts',(-2.80783724200006,5.2,3.15179445199998));
#305471=CARTESIAN_POINT('Ctrl Pts',(-2.80783724200006,2.2,3.15179445199998));
#305472=CARTESIAN_POINT('Ctrl Pts',(-2.80722345500005,12.2,3.15033694399999));
#305473=CARTESIAN_POINT('Ctrl Pts',(-2.80722345500005,5.2,3.15033694399999));
#305474=CARTESIAN_POINT('Ctrl Pts',(-2.80722345500005,2.2,3.15033694399999));
#305475=CARTESIAN_POINT('Ctrl Pts',(-2.80660977100006,12.2,3.14888439299998));
#305476=CARTESIAN_POINT('Ctrl Pts',(-2.80660977100006,5.2,3.14888439299998));
#305477=CARTESIAN_POINT('Ctrl Pts',(-2.80660977100006,2.2,3.14888439299998));
#305478=CARTESIAN_POINT('Ctrl Pts',(-2.80599620400006,12.2,3.14743680399998));
#305479=CARTESIAN_POINT('Ctrl Pts',(-2.80599620400006,5.2,3.14743680399998));
#305480=CARTESIAN_POINT('Ctrl Pts',(-2.80599620400006,2.2,3.14743680399998));
#305481=CARTESIAN_POINT('Ctrl Pts',(-2.80538276500006,12.2,3.14599417899998));
#305482=CARTESIAN_POINT('Ctrl Pts',(-2.80538276500006,5.2,3.14599417899998));
#305483=CARTESIAN_POINT('Ctrl Pts',(-2.80538276500006,2.2,3.14599417899998));
#305484=CARTESIAN_POINT('Ctrl Pts',(-2.80476946700006,12.2,3.14455652199998));
#305485=CARTESIAN_POINT('Ctrl Pts',(-2.80476946700006,5.2,3.14455652199998));
#305486=CARTESIAN_POINT('Ctrl Pts',(-2.80476946700006,2.2,3.14455652199998));
#305487=CARTESIAN_POINT('Ctrl Pts',(-2.80415632300006,12.2,3.14312383699999));
#305488=CARTESIAN_POINT('Ctrl Pts',(-2.80415632300006,5.2,3.14312383699999));
#305489=CARTESIAN_POINT('Ctrl Pts',(-2.80415632300006,2.2,3.14312383699999));
#305490=CARTESIAN_POINT('Ctrl Pts',(-2.80354334400006,12.2,3.14169612899998));
#305491=CARTESIAN_POINT('Ctrl Pts',(-2.80354334400006,5.2,3.14169612899998));
#305492=CARTESIAN_POINT('Ctrl Pts',(-2.80354334400006,2.2,3.14169612899998));
#305493=CARTESIAN_POINT('Ctrl Pts',(-2.80293054400006,12.2,3.14027340099998));
#305494=CARTESIAN_POINT('Ctrl Pts',(-2.80293054400006,5.2,3.14027340099998));
#305495=CARTESIAN_POINT('Ctrl Pts',(-2.80293054400006,2.2,3.14027340099998));
#305496=CARTESIAN_POINT('Ctrl Pts',(-2.80231793300006,12.2,3.13885565799998));
#305497=CARTESIAN_POINT('Ctrl Pts',(-2.80231793300006,5.2,3.13885565799998));
#305498=CARTESIAN_POINT('Ctrl Pts',(-2.80231793300006,2.2,3.13885565799998));
#305499=CARTESIAN_POINT('Ctrl Pts',(-2.80170552700006,12.2,3.13744290199998));
#305500=CARTESIAN_POINT('Ctrl Pts',(-2.80170552700006,5.2,3.13744290199998));
#305501=CARTESIAN_POINT('Ctrl Pts',(-2.80170552700006,2.2,3.13744290199998));
#305502=CARTESIAN_POINT('Ctrl Pts',(-2.80109333500006,12.2,3.13603513699999));
#305503=CARTESIAN_POINT('Ctrl Pts',(-2.80109333500006,5.2,3.13603513699999));
#305504=CARTESIAN_POINT('Ctrl Pts',(-2.80109333500006,2.2,3.13603513699999));
#305505=CARTESIAN_POINT('Ctrl Pts',(-2.80048137300006,12.2,3.13463236799999));
#305506=CARTESIAN_POINT('Ctrl Pts',(-2.80048137300006,5.2,3.13463236799999));
#305507=CARTESIAN_POINT('Ctrl Pts',(-2.80048137300006,2.2,3.13463236799999));
#305508=CARTESIAN_POINT('Ctrl Pts',(-2.79986965000006,12.2,3.13323459799999));
#305509=CARTESIAN_POINT('Ctrl Pts',(-2.79986965000006,5.2,3.13323459799999));
#305510=CARTESIAN_POINT('Ctrl Pts',(-2.79986965000006,2.2,3.13323459799999));
#305511=CARTESIAN_POINT('Ctrl Pts',(-2.79925818200006,12.2,3.13184183299998));
#305512=CARTESIAN_POINT('Ctrl Pts',(-2.79925818200006,5.2,3.13184183299998));
#305513=CARTESIAN_POINT('Ctrl Pts',(-2.79925818200006,2.2,3.13184183299998));
#305514=CARTESIAN_POINT('Ctrl Pts',(-2.79864698000006,12.2,3.13045407399999));
#305515=CARTESIAN_POINT('Ctrl Pts',(-2.79864698000006,5.2,3.13045407399999));
#305516=CARTESIAN_POINT('Ctrl Pts',(-2.79864698000006,2.2,3.13045407399999));
#305517=CARTESIAN_POINT('Ctrl Pts',(-2.79803605600006,12.2,3.12907132599998));
#305518=CARTESIAN_POINT('Ctrl Pts',(-2.79803605600006,5.2,3.12907132599998));
#305519=CARTESIAN_POINT('Ctrl Pts',(-2.79803605600006,2.2,3.12907132599998));
#305520=CARTESIAN_POINT('Ctrl Pts',(-2.79742542500005,12.2,3.12769359199999));
#305521=CARTESIAN_POINT('Ctrl Pts',(-2.79742542500005,5.2,3.12769359199999));
#305522=CARTESIAN_POINT('Ctrl Pts',(-2.79742542500005,2.2,3.12769359199999));
#305523=CARTESIAN_POINT('Ctrl Pts',(-2.79681509700006,12.2,3.12632087799999));
#305524=CARTESIAN_POINT('Ctrl Pts',(-2.79681509700006,5.2,3.12632087799999));
#305525=CARTESIAN_POINT('Ctrl Pts',(-2.79681509700006,2.2,3.12632087799999));
#305526=CARTESIAN_POINT('Ctrl Pts',(-2.79620508700006,12.2,3.12495318599999));
#305527=CARTESIAN_POINT('Ctrl Pts',(-2.79620508700006,5.2,3.12495318599999));
#305528=CARTESIAN_POINT('Ctrl Pts',(-2.79620508700006,2.2,3.12495318599999));
#305529=CARTESIAN_POINT('Ctrl Pts',(-2.79559540700005,12.2,3.12359051999999));
#305530=CARTESIAN_POINT('Ctrl Pts',(-2.79559540700005,5.2,3.12359051999999));
#305531=CARTESIAN_POINT('Ctrl Pts',(-2.79559540700005,2.2,3.12359051999999));
#305532=CARTESIAN_POINT('Ctrl Pts',(-2.79498607000006,12.2,3.12223288299998));
#305533=CARTESIAN_POINT('Ctrl Pts',(-2.79498607000006,5.2,3.12223288299998));
#305534=CARTESIAN_POINT('Ctrl Pts',(-2.79498607000006,2.2,3.12223288299998));
#305535=CARTESIAN_POINT('Ctrl Pts',(-2.79437708900006,12.2,3.12088028099998));
#305536=CARTESIAN_POINT('Ctrl Pts',(-2.79437708900006,5.2,3.12088028099998));
#305537=CARTESIAN_POINT('Ctrl Pts',(-2.79437708900006,2.2,3.12088028099998));
#305538=CARTESIAN_POINT('Ctrl Pts',(-2.79376847500005,12.2,3.11953271599998));
#305539=CARTESIAN_POINT('Ctrl Pts',(-2.79376847500005,5.2,3.11953271599998));
#305540=CARTESIAN_POINT('Ctrl Pts',(-2.79376847500005,2.2,3.11953271599998));
#305541=CARTESIAN_POINT('Ctrl Pts',(-2.79316024400006,12.2,3.11819019099998));
#305542=CARTESIAN_POINT('Ctrl Pts',(-2.79316024400006,5.2,3.11819019099998));
#305543=CARTESIAN_POINT('Ctrl Pts',(-2.79316024400006,2.2,3.11819019099998));
#305544=CARTESIAN_POINT('Ctrl Pts',(-2.79255240800006,12.2,3.11685271099999));
#305545=CARTESIAN_POINT('Ctrl Pts',(-2.79255240800006,5.2,3.11685271099999));
#305546=CARTESIAN_POINT('Ctrl Pts',(-2.79255240800006,2.2,3.11685271099999));
#305547=CARTESIAN_POINT('Ctrl Pts',(-2.79194497900006,12.2,3.11552028099998));
#305548=CARTESIAN_POINT('Ctrl Pts',(-2.79194497900006,5.2,3.11552028099998));
#305549=CARTESIAN_POINT('Ctrl Pts',(-2.79194497900006,2.2,3.11552028099998));
#305550=CARTESIAN_POINT('Ctrl Pts',(-2.79133797000005,12.2,3.11419290199999));
#305551=CARTESIAN_POINT('Ctrl Pts',(-2.79133797000005,5.2,3.11419290199999));
#305552=CARTESIAN_POINT('Ctrl Pts',(-2.79133797000005,2.2,3.11419290199999));
#305553=CARTESIAN_POINT('Ctrl Pts',(-2.79073139700006,12.2,3.11287057999999));
#305554=CARTESIAN_POINT('Ctrl Pts',(-2.79073139700006,5.2,3.11287057999999));
#305555=CARTESIAN_POINT('Ctrl Pts',(-2.79073139700006,2.2,3.11287057999999));
#305556=CARTESIAN_POINT('Ctrl Pts',(-2.79012526800006,12.2,3.11155331599998));
#305557=CARTESIAN_POINT('Ctrl Pts',(-2.79012526800006,5.2,3.11155331599998));
#305558=CARTESIAN_POINT('Ctrl Pts',(-2.79012526800006,2.2,3.11155331599998));
#305559=CARTESIAN_POINT('Ctrl Pts',(-2.78951960100006,12.2,3.11024111699999));
#305560=CARTESIAN_POINT('Ctrl Pts',(-2.78951960100006,5.2,3.11024111699999));
#305561=CARTESIAN_POINT('Ctrl Pts',(-2.78951960100006,2.2,3.11024111699999));
#305562=CARTESIAN_POINT('Ctrl Pts',(-2.78891440600006,12.2,3.10893398399998));
#305563=CARTESIAN_POINT('Ctrl Pts',(-2.78891440600006,5.2,3.10893398399998));
#305564=CARTESIAN_POINT('Ctrl Pts',(-2.78891440600006,2.2,3.10893398399998));
#305565=CARTESIAN_POINT('Ctrl Pts',(-2.78830969800006,12.2,3.10763192299999));
#305566=CARTESIAN_POINT('Ctrl Pts',(-2.78830969800006,5.2,3.10763192299999));
#305567=CARTESIAN_POINT('Ctrl Pts',(-2.78830969800006,2.2,3.10763192299999));
#305568=CARTESIAN_POINT('Ctrl Pts',(-2.78770549000006,12.2,3.10633493499999));
#305569=CARTESIAN_POINT('Ctrl Pts',(-2.78770549000006,5.2,3.10633493499999));
#305570=CARTESIAN_POINT('Ctrl Pts',(-2.78770549000006,2.2,3.10633493499999));
#305571=CARTESIAN_POINT('Ctrl Pts',(-2.78710179400006,12.2,3.10504302599998));
#305572=CARTESIAN_POINT('Ctrl Pts',(-2.78710179400006,5.2,3.10504302599998));
#305573=CARTESIAN_POINT('Ctrl Pts',(-2.78710179400006,2.2,3.10504302599998));
#305574=CARTESIAN_POINT('Ctrl Pts',(-2.78649862400006,12.2,3.10375619799999));
#305575=CARTESIAN_POINT('Ctrl Pts',(-2.78649862400006,5.2,3.10375619799999));
#305576=CARTESIAN_POINT('Ctrl Pts',(-2.78649862400006,2.2,3.10375619799999));
#305577=CARTESIAN_POINT('Ctrl Pts',(-2.78589599400005,12.2,3.10247445499999));
#305578=CARTESIAN_POINT('Ctrl Pts',(-2.78589599400005,5.2,3.10247445499999));
#305579=CARTESIAN_POINT('Ctrl Pts',(-2.78589599400005,2.2,3.10247445499999));
#305580=CARTESIAN_POINT('Ctrl Pts',(-2.78529391700005,12.2,3.10119780099999));
#305581=CARTESIAN_POINT('Ctrl Pts',(-2.78529391700005,5.2,3.10119780099999));
#305582=CARTESIAN_POINT('Ctrl Pts',(-2.78529391700005,2.2,3.10119780099999));
#305583=CARTESIAN_POINT('Ctrl Pts',(-2.78469240600006,12.2,3.09992623899999));
#305584=CARTESIAN_POINT('Ctrl Pts',(-2.78469240600006,5.2,3.09992623899999));
#305585=CARTESIAN_POINT('Ctrl Pts',(-2.78469240600006,2.2,3.09992623899999));
#305586=CARTESIAN_POINT('Ctrl Pts',(-2.78409147500006,12.2,3.09865977399999));
#305587=CARTESIAN_POINT('Ctrl Pts',(-2.78409147500006,5.2,3.09865977399999));
#305588=CARTESIAN_POINT('Ctrl Pts',(-2.78409147500006,2.2,3.09865977399999));
#305589=CARTESIAN_POINT('Ctrl Pts',(-2.78349113700005,12.2,3.09739840799999));
#305590=CARTESIAN_POINT('Ctrl Pts',(-2.78349113700005,5.2,3.09739840799999));
#305591=CARTESIAN_POINT('Ctrl Pts',(-2.78349113700005,2.2,3.09739840799999));
#305592=CARTESIAN_POINT('Ctrl Pts',(-2.78289140600006,12.2,3.09614214499998));
#305593=CARTESIAN_POINT('Ctrl Pts',(-2.78289140600006,5.2,3.09614214499998));
#305594=CARTESIAN_POINT('Ctrl Pts',(-2.78289140600006,2.2,3.09614214499998));
#305595=CARTESIAN_POINT('Ctrl Pts',(-2.78229229400006,12.2,3.09489098899999));
#305596=CARTESIAN_POINT('Ctrl Pts',(-2.78229229400006,5.2,3.09489098899999));
#305597=CARTESIAN_POINT('Ctrl Pts',(-2.78229229400006,2.2,3.09489098899999));
#305598=CARTESIAN_POINT('Ctrl Pts',(-2.78169381700006,12.2,3.09364494299999));
#305599=CARTESIAN_POINT('Ctrl Pts',(-2.78169381700006,5.2,3.09364494299999));
#305600=CARTESIAN_POINT('Ctrl Pts',(-2.78169381700006,2.2,3.09364494299999));
#305601=CARTESIAN_POINT('Ctrl Pts',(-2.78109598700006,12.2,3.09240401199999));
#305602=CARTESIAN_POINT('Ctrl Pts',(-2.78109598700006,5.2,3.09240401199999));
#305603=CARTESIAN_POINT('Ctrl Pts',(-2.78109598700006,2.2,3.09240401199999));
#305604=CARTESIAN_POINT('Ctrl Pts',(-2.78049881700006,12.2,3.09116819699998));
#305605=CARTESIAN_POINT('Ctrl Pts',(-2.78049881700006,5.2,3.09116819699998));
#305606=CARTESIAN_POINT('Ctrl Pts',(-2.78049881700006,2.2,3.09116819699998));
#305607=CARTESIAN_POINT('Ctrl Pts',(-2.77990232300006,12.2,3.08993750299998));
#305608=CARTESIAN_POINT('Ctrl Pts',(-2.77990232300006,5.2,3.08993750299998));
#305609=CARTESIAN_POINT('Ctrl Pts',(-2.77990232300006,2.2,3.08993750299998));
#305610=CARTESIAN_POINT('Ctrl Pts',(-2.77930651700005,12.2,3.08871193399998));
#305611=CARTESIAN_POINT('Ctrl Pts',(-2.77930651700005,5.2,3.08871193399998));
#305612=CARTESIAN_POINT('Ctrl Pts',(-2.77930651700005,2.2,3.08871193399998));
#305613=CARTESIAN_POINT('Ctrl Pts',(-2.77871141300006,12.2,3.08749149299998));
#305614=CARTESIAN_POINT('Ctrl Pts',(-2.77871141300006,5.2,3.08749149299998));
#305615=CARTESIAN_POINT('Ctrl Pts',(-2.77871141300006,2.2,3.08749149299998));
#305616=CARTESIAN_POINT('Ctrl Pts',(-2.77811702500005,12.2,3.08627618199999));
#305617=CARTESIAN_POINT('Ctrl Pts',(-2.77811702500005,5.2,3.08627618199999));
#305618=CARTESIAN_POINT('Ctrl Pts',(-2.77811702500005,2.2,3.08627618199999));
#305619=CARTESIAN_POINT('Ctrl Pts',(-2.77752336600006,12.2,3.08506600699998));
#305620=CARTESIAN_POINT('Ctrl Pts',(-2.77752336600006,5.2,3.08506600699998));
#305621=CARTESIAN_POINT('Ctrl Pts',(-2.77752336600006,2.2,3.08506600699998));
#305622=CARTESIAN_POINT('Ctrl Pts',(-2.77693045100006,12.2,3.08386097099999));
#305623=CARTESIAN_POINT('Ctrl Pts',(-2.77693045100006,5.2,3.08386097099999));
#305624=CARTESIAN_POINT('Ctrl Pts',(-2.77693045100006,2.2,3.08386097099999));
#305625=CARTESIAN_POINT('Ctrl Pts',(-2.77633829400005,12.2,3.08266107499998));
#305626=CARTESIAN_POINT('Ctrl Pts',(-2.77633829400005,5.2,3.08266107499998));
#305627=CARTESIAN_POINT('Ctrl Pts',(-2.77633829400005,2.2,3.08266107499998));
#305628=CARTESIAN_POINT('Ctrl Pts',(-2.77574690700006,12.2,3.08146632499999));
#305629=CARTESIAN_POINT('Ctrl Pts',(-2.77574690700006,5.2,3.08146632499999));
#305630=CARTESIAN_POINT('Ctrl Pts',(-2.77574690700006,2.2,3.08146632499999));
#305631=CARTESIAN_POINT('Ctrl Pts',(-2.77515630600006,12.2,3.08027672299998));
#305632=CARTESIAN_POINT('Ctrl Pts',(-2.77515630600006,5.2,3.08027672299998));
#305633=CARTESIAN_POINT('Ctrl Pts',(-2.77515630600006,2.2,3.08027672299998));
#305634=CARTESIAN_POINT('Ctrl Pts',(-2.77456650400006,12.2,3.07909227399998));
#305635=CARTESIAN_POINT('Ctrl Pts',(-2.77456650400006,5.2,3.07909227399998));
#305636=CARTESIAN_POINT('Ctrl Pts',(-2.77456650400006,2.2,3.07909227399998));
#305637=CARTESIAN_POINT('Ctrl Pts',(-2.77397751500006,12.2,3.07791298099998));
#305638=CARTESIAN_POINT('Ctrl Pts',(-2.77397751500006,5.2,3.07791298099998));
#305639=CARTESIAN_POINT('Ctrl Pts',(-2.77397751500006,2.2,3.07791298099998));
#305640=CARTESIAN_POINT('Ctrl Pts',(-2.77338935300006,12.2,3.07673884499999));
#305641=CARTESIAN_POINT('Ctrl Pts',(-2.77338935300006,5.2,3.07673884499999));
#305642=CARTESIAN_POINT('Ctrl Pts',(-2.77338935300006,2.2,3.07673884499999));
#305643=CARTESIAN_POINT('Ctrl Pts',(-2.77280203300006,12.2,3.07556987199998));
#305644=CARTESIAN_POINT('Ctrl Pts',(-2.77280203300006,5.2,3.07556987199998));
#305645=CARTESIAN_POINT('Ctrl Pts',(-2.77280203300006,2.2,3.07556987199998));
#305646=CARTESIAN_POINT('Ctrl Pts',(-2.77221556900006,12.2,3.07440606499998));
#305647=CARTESIAN_POINT('Ctrl Pts',(-2.77221556900006,5.2,3.07440606499998));
#305648=CARTESIAN_POINT('Ctrl Pts',(-2.77221556900006,2.2,3.07440606499998));
#305649=CARTESIAN_POINT('Ctrl Pts',(-2.77162997300006,12.2,3.07324742699999));
#305650=CARTESIAN_POINT('Ctrl Pts',(-2.77162997300006,5.2,3.07324742699999));
#305651=CARTESIAN_POINT('Ctrl Pts',(-2.77162997300006,2.2,3.07324742699999));
#305652=CARTESIAN_POINT('Ctrl Pts',(-2.77104526100006,12.2,3.07209396099999));
#305653=CARTESIAN_POINT('Ctrl Pts',(-2.77104526100006,5.2,3.07209396099999));
#305654=CARTESIAN_POINT('Ctrl Pts',(-2.77104526100006,2.2,3.07209396099999));
#305655=CARTESIAN_POINT('Ctrl Pts',(-2.77046144700006,12.2,3.07094566999999));
#305656=CARTESIAN_POINT('Ctrl Pts',(-2.77046144700006,5.2,3.07094566999999));
#305657=CARTESIAN_POINT('Ctrl Pts',(-2.77046144700006,2.2,3.07094566999999));
#305658=CARTESIAN_POINT('Ctrl Pts',(-2.76987854600006,12.2,3.06980255899998));
#305659=CARTESIAN_POINT('Ctrl Pts',(-2.76987854600006,5.2,3.06980255899998));
#305660=CARTESIAN_POINT('Ctrl Pts',(-2.76987854600006,2.2,3.06980255899998));
#305661=CARTESIAN_POINT('Ctrl Pts',(-2.76929657200006,12.2,3.06866462899999));
#305662=CARTESIAN_POINT('Ctrl Pts',(-2.76929657200006,5.2,3.06866462899999));
#305663=CARTESIAN_POINT('Ctrl Pts',(-2.76929657200006,2.2,3.06866462899999));
#305664=CARTESIAN_POINT('Ctrl Pts',(-2.76871553700006,12.2,3.06753188599998));
#305665=CARTESIAN_POINT('Ctrl Pts',(-2.76871553700006,5.2,3.06753188599998));
#305666=CARTESIAN_POINT('Ctrl Pts',(-2.76871553700006,2.2,3.06753188599998));
#305667=CARTESIAN_POINT('Ctrl Pts',(-2.76813545900006,12.2,3.06640433199998));
#305668=CARTESIAN_POINT('Ctrl Pts',(-2.76813545900006,5.2,3.06640433199998));
#305669=CARTESIAN_POINT('Ctrl Pts',(-2.76813545900006,2.2,3.06640433199998));
#305670=CARTESIAN_POINT('Ctrl Pts',(-2.76755635000006,12.2,3.06528196999999));
#305671=CARTESIAN_POINT('Ctrl Pts',(-2.76755635000006,5.2,3.06528196999999));
#305672=CARTESIAN_POINT('Ctrl Pts',(-2.76755635000006,2.2,3.06528196999999));
#305673=CARTESIAN_POINT('Ctrl Pts',(-2.76697822500005,12.2,3.06416480299998));
#305674=CARTESIAN_POINT('Ctrl Pts',(-2.76697822500005,5.2,3.06416480299998));
#305675=CARTESIAN_POINT('Ctrl Pts',(-2.76697822500005,2.2,3.06416480299998));
#305676=CARTESIAN_POINT('Ctrl Pts',(-2.76640109900006,12.2,3.06305283499999));
#305677=CARTESIAN_POINT('Ctrl Pts',(-2.76640109900006,5.2,3.06305283499999));
#305678=CARTESIAN_POINT('Ctrl Pts',(-2.76640109900006,2.2,3.06305283499999));
#305679=CARTESIAN_POINT('Ctrl Pts',(-2.76582498600006,12.2,3.06194606899999));
#305680=CARTESIAN_POINT('Ctrl Pts',(-2.76582498600006,5.2,3.06194606899999));
#305681=CARTESIAN_POINT('Ctrl Pts',(-2.76582498600006,2.2,3.06194606899999));
#305682=CARTESIAN_POINT('Ctrl Pts',(-2.76524990000006,12.2,3.06084450799998));
#305683=CARTESIAN_POINT('Ctrl Pts',(-2.76524990000006,5.2,3.06084450799998));
#305684=CARTESIAN_POINT('Ctrl Pts',(-2.76524990000006,2.2,3.06084450799998));
#305685=CARTESIAN_POINT('Ctrl Pts',(-2.76467585600006,12.2,3.05974815599999));
#305686=CARTESIAN_POINT('Ctrl Pts',(-2.76467585600006,5.2,3.05974815599999));
#305687=CARTESIAN_POINT('Ctrl Pts',(-2.76467585600006,2.2,3.05974815599999));
#305688=CARTESIAN_POINT('Ctrl Pts',(-2.76410287000005,12.2,3.05865701499999));
#305689=CARTESIAN_POINT('Ctrl Pts',(-2.76410287000005,5.2,3.05865701499999));
#305690=CARTESIAN_POINT('Ctrl Pts',(-2.76410287000005,2.2,3.05865701499999));
#305691=CARTESIAN_POINT('Ctrl Pts',(-2.76353095500005,12.2,3.05757108899999));
#305692=CARTESIAN_POINT('Ctrl Pts',(-2.76353095500005,5.2,3.05757108899999));
#305693=CARTESIAN_POINT('Ctrl Pts',(-2.76353095500005,2.2,3.05757108899999));
#305694=CARTESIAN_POINT('Ctrl Pts',(-2.76296012600006,12.2,3.05649038199999));
#305695=CARTESIAN_POINT('Ctrl Pts',(-2.76296012600006,5.2,3.05649038199999));
#305696=CARTESIAN_POINT('Ctrl Pts',(-2.76296012600006,2.2,3.05649038199999));
#305697=CARTESIAN_POINT('Ctrl Pts',(-2.76239039700005,12.2,3.05541489599998));
#305698=CARTESIAN_POINT('Ctrl Pts',(-2.76239039700005,5.2,3.05541489599998));
#305699=CARTESIAN_POINT('Ctrl Pts',(-2.76239039700005,2.2,3.05541489599998));
#305700=CARTESIAN_POINT('Ctrl Pts',(-2.76182178500005,12.2,3.05434463399998));
#305701=CARTESIAN_POINT('Ctrl Pts',(-2.76182178500005,5.2,3.05434463399998));
#305702=CARTESIAN_POINT('Ctrl Pts',(-2.76182178500005,2.2,3.05434463399998));
#305703=CARTESIAN_POINT('Ctrl Pts',(-2.76125430200006,12.2,3.05327959899999));
#305704=CARTESIAN_POINT('Ctrl Pts',(-2.76125430200006,5.2,3.05327959899999));
#305705=CARTESIAN_POINT('Ctrl Pts',(-2.76125430200006,2.2,3.05327959899999));
#305706=CARTESIAN_POINT('Ctrl Pts',(-2.76068796600006,12.2,3.05221979499999));
#305707=CARTESIAN_POINT('Ctrl Pts',(-2.76068796600006,5.2,3.05221979499999));
#305708=CARTESIAN_POINT('Ctrl Pts',(-2.76068796600006,2.2,3.05221979499999));
#305709=CARTESIAN_POINT('Ctrl Pts',(-2.76012279100006,12.2,3.05116522499999));
#305710=CARTESIAN_POINT('Ctrl Pts',(-2.76012279100006,5.2,3.05116522499999));
#305711=CARTESIAN_POINT('Ctrl Pts',(-2.76012279100006,2.2,3.05116522499999));
#305712=CARTESIAN_POINT('Ctrl Pts',(-2.75955878900006,12.2,3.05011589299998));
#305713=CARTESIAN_POINT('Ctrl Pts',(-2.75955878900006,5.2,3.05011589299998));
#305714=CARTESIAN_POINT('Ctrl Pts',(-2.75955878900006,2.2,3.05011589299998));
#305715=CARTESIAN_POINT('Ctrl Pts',(-2.75899597900006,12.2,3.04907179999999));
#305716=CARTESIAN_POINT('Ctrl Pts',(-2.75899597900006,5.2,3.04907179999999));
#305717=CARTESIAN_POINT('Ctrl Pts',(-2.75899597900006,2.2,3.04907179999999));
#305718=CARTESIAN_POINT('Ctrl Pts',(-2.75843437300006,12.2,3.04803295099998));
#305719=CARTESIAN_POINT('Ctrl Pts',(-2.75843437300006,5.2,3.04803295099998));
#305720=CARTESIAN_POINT('Ctrl Pts',(-2.75843437300006,2.2,3.04803295099998));
#305721=CARTESIAN_POINT('Ctrl Pts',(-2.75787398700006,12.2,3.04699934699999));
#305722=CARTESIAN_POINT('Ctrl Pts',(-2.75787398700006,5.2,3.04699934699999));
#305723=CARTESIAN_POINT('Ctrl Pts',(-2.75787398700006,2.2,3.04699934699999));
#305724=CARTESIAN_POINT('Ctrl Pts',(-2.75731483700006,12.2,3.04597099299999));
#305725=CARTESIAN_POINT('Ctrl Pts',(-2.75731483700006,5.2,3.04597099299999));
#305726=CARTESIAN_POINT('Ctrl Pts',(-2.75731483700006,2.2,3.04597099299999));
#305727=CARTESIAN_POINT('Ctrl Pts',(-2.75675693700005,12.2,3.04494789199998));
#305728=CARTESIAN_POINT('Ctrl Pts',(-2.75675693700005,5.2,3.04494789199998));
#305729=CARTESIAN_POINT('Ctrl Pts',(-2.75675693700005,2.2,3.04494789199998));
#305730=CARTESIAN_POINT('Ctrl Pts',(-2.75620030300006,12.2,3.04393004499998));
#305731=CARTESIAN_POINT('Ctrl Pts',(-2.75620030300006,5.2,3.04393004499998));
#305732=CARTESIAN_POINT('Ctrl Pts',(-2.75620030300006,2.2,3.04393004499998));
#305733=CARTESIAN_POINT('Ctrl Pts',(-2.75564495000005,12.2,3.04291745799999));
#305734=CARTESIAN_POINT('Ctrl Pts',(-2.75564495000005,5.2,3.04291745799999));
#305735=CARTESIAN_POINT('Ctrl Pts',(-2.75564495000005,2.2,3.04291745799999));
#305736=CARTESIAN_POINT('Ctrl Pts',(-2.75509089200006,12.2,3.04191013099998));
#305737=CARTESIAN_POINT('Ctrl Pts',(-2.75509089200006,5.2,3.04191013099998));
#305738=CARTESIAN_POINT('Ctrl Pts',(-2.75509089200006,2.2,3.04191013099998));
#305739=CARTESIAN_POINT('Ctrl Pts',(-2.75453814700006,12.2,3.04090806999999));
#305740=CARTESIAN_POINT('Ctrl Pts',(-2.75453814700006,5.2,3.04090806999999));
#305741=CARTESIAN_POINT('Ctrl Pts',(-2.75453814700006,2.2,3.04090806999999));
#305742=CARTESIAN_POINT('Ctrl Pts',(-2.75398672700006,12.2,3.03991127599998));
#305743=CARTESIAN_POINT('Ctrl Pts',(-2.75398672700006,5.2,3.03991127599998));
#305744=CARTESIAN_POINT('Ctrl Pts',(-2.75398672700006,2.2,3.03991127599998));
#305745=CARTESIAN_POINT('Ctrl Pts',(-2.75343665000006,12.2,3.03891975299998));
#305746=CARTESIAN_POINT('Ctrl Pts',(-2.75343665000006,5.2,3.03891975299998));
#305747=CARTESIAN_POINT('Ctrl Pts',(-2.75343665000006,2.2,3.03891975299998));
#305748=CARTESIAN_POINT('Ctrl Pts',(-2.75288792900006,12.2,3.03793350199999));
#305749=CARTESIAN_POINT('Ctrl Pts',(-2.75288792900006,5.2,3.03793350199999));
#305750=CARTESIAN_POINT('Ctrl Pts',(-2.75288792900006,2.2,3.03793350199999));
#305751=CARTESIAN_POINT('Ctrl Pts',(-2.75234058200006,12.2,3.03695252899999));
#305752=CARTESIAN_POINT('Ctrl Pts',(-2.75234058200006,5.2,3.03695252899999));
#305753=CARTESIAN_POINT('Ctrl Pts',(-2.75234058200006,2.2,3.03695252899999));
#305754=CARTESIAN_POINT('Ctrl Pts',(-2.75179462400006,12.2,3.03597683399998));
#305755=CARTESIAN_POINT('Ctrl Pts',(-2.75179462400006,5.2,3.03597683399998));
#305756=CARTESIAN_POINT('Ctrl Pts',(-2.75179462400006,2.2,3.03597683399998));
#305757=CARTESIAN_POINT('Ctrl Pts',(-2.75125006900006,12.2,3.03500642199998));
#305758=CARTESIAN_POINT('Ctrl Pts',(-2.75125006900006,5.2,3.03500642199998));
#305759=CARTESIAN_POINT('Ctrl Pts',(-2.75125006900006,2.2,3.03500642199998));
#305760=CARTESIAN_POINT('Ctrl Pts',(-2.75070693300006,12.2,3.03404129499998));
#305761=CARTESIAN_POINT('Ctrl Pts',(-2.75070693300006,5.2,3.03404129499998));
#305762=CARTESIAN_POINT('Ctrl Pts',(-2.75070693300006,2.2,3.03404129499998));
#305763=CARTESIAN_POINT('Ctrl Pts',(-2.75016523200006,12.2,3.03308145599999));
#305764=CARTESIAN_POINT('Ctrl Pts',(-2.75016523200006,5.2,3.03308145599999));
#305765=CARTESIAN_POINT('Ctrl Pts',(-2.75016523200006,2.2,3.03308145599999));
#305766=CARTESIAN_POINT('Ctrl Pts',(-2.74962498200006,12.2,3.03212690799998));
#305767=CARTESIAN_POINT('Ctrl Pts',(-2.74962498200006,5.2,3.03212690799998));
#305768=CARTESIAN_POINT('Ctrl Pts',(-2.74962498200006,2.2,3.03212690799998));
#305769=CARTESIAN_POINT('Ctrl Pts',(-2.74908619900006,12.2,3.03117765399998));
#305770=CARTESIAN_POINT('Ctrl Pts',(-2.74908619900006,5.2,3.03117765399998));
#305771=CARTESIAN_POINT('Ctrl Pts',(-2.74908619900006,2.2,3.03117765399998));
#305772=CARTESIAN_POINT('Ctrl Pts',(-2.74854889700006,12.2,3.03023369599998));
#305773=CARTESIAN_POINT('Ctrl Pts',(-2.74854889700006,5.2,3.03023369599998));
#305774=CARTESIAN_POINT('Ctrl Pts',(-2.74854889700006,2.2,3.03023369599998));
#305775=CARTESIAN_POINT('Ctrl Pts',(-2.74801309400006,12.2,3.02929503899998));
#305776=CARTESIAN_POINT('Ctrl Pts',(-2.74801309400006,5.2,3.02929503899998));
#305777=CARTESIAN_POINT('Ctrl Pts',(-2.74801309400006,2.2,3.02929503899998));
#305778=CARTESIAN_POINT('Ctrl Pts',(-2.74747880300006,12.2,3.02836168399998));
#305779=CARTESIAN_POINT('Ctrl Pts',(-2.74747880300006,5.2,3.02836168399998));
#305780=CARTESIAN_POINT('Ctrl Pts',(-2.74747880300006,2.2,3.02836168399998));
#305781=CARTESIAN_POINT('Ctrl Pts',(-2.74694604300006,12.2,3.02743363399999));
#305782=CARTESIAN_POINT('Ctrl Pts',(-2.74694604300006,5.2,3.02743363399999));
#305783=CARTESIAN_POINT('Ctrl Pts',(-2.74694604300006,2.2,3.02743363399999));
#305784=CARTESIAN_POINT('Ctrl Pts',(-2.74641482900006,12.2,3.02651089199999));
#305785=CARTESIAN_POINT('Ctrl Pts',(-2.74641482900006,5.2,3.02651089199999));
#305786=CARTESIAN_POINT('Ctrl Pts',(-2.74641482900006,2.2,3.02651089199999));
#305787=CARTESIAN_POINT('Ctrl Pts',(-2.74588517500006,12.2,3.02559346099999));
#305788=CARTESIAN_POINT('Ctrl Pts',(-2.74588517500006,5.2,3.02559346099999));
#305789=CARTESIAN_POINT('Ctrl Pts',(-2.74588517500006,2.2,3.02559346099999));
#305790=CARTESIAN_POINT('Ctrl Pts',(-2.74535709800006,12.2,3.02468134399999));
#305791=CARTESIAN_POINT('Ctrl Pts',(-2.74535709800006,5.2,3.02468134399999));
#305792=CARTESIAN_POINT('Ctrl Pts',(-2.74535709800006,2.2,3.02468134399999));
#305793=CARTESIAN_POINT('Ctrl Pts',(-2.74483061500006,12.2,3.02377454299998));
#305794=CARTESIAN_POINT('Ctrl Pts',(-2.74483061500006,5.2,3.02377454299998));
#305795=CARTESIAN_POINT('Ctrl Pts',(-2.74483061500006,2.2,3.02377454299998));
#305796=CARTESIAN_POINT('Ctrl Pts',(-2.74430574200006,12.2,3.02287306099998));
#305797=CARTESIAN_POINT('Ctrl Pts',(-2.74430574200006,5.2,3.02287306099998));
#305798=CARTESIAN_POINT('Ctrl Pts',(-2.74430574200006,2.2,3.02287306099998));
#305799=CARTESIAN_POINT('Ctrl Pts',(-2.74378249400006,12.2,3.02197690099998));
#305800=CARTESIAN_POINT('Ctrl Pts',(-2.74378249400006,5.2,3.02197690099998));
#305801=CARTESIAN_POINT('Ctrl Pts',(-2.74378249400006,2.2,3.02197690099998));
#305802=CARTESIAN_POINT('Ctrl Pts',(-2.74326088800006,12.2,3.02108606599998));
#305803=CARTESIAN_POINT('Ctrl Pts',(-2.74326088800006,5.2,3.02108606599998));
#305804=CARTESIAN_POINT('Ctrl Pts',(-2.74326088800006,2.2,3.02108606599998));
#305805=CARTESIAN_POINT('Ctrl Pts',(-2.74274094000006,12.2,3.02020055799999));
#305806=CARTESIAN_POINT('Ctrl Pts',(-2.74274094000006,5.2,3.02020055799999));
#305807=CARTESIAN_POINT('Ctrl Pts',(-2.74274094000006,2.2,3.02020055799999));
#305808=CARTESIAN_POINT('Ctrl Pts',(-2.74222266600006,12.2,3.01932038099999));
#305809=CARTESIAN_POINT('Ctrl Pts',(-2.74222266600006,5.2,3.01932038099999));
#305810=CARTESIAN_POINT('Ctrl Pts',(-2.74222266600006,2.2,3.01932038099999));
#305811=CARTESIAN_POINT('Ctrl Pts',(-2.74170608200006,12.2,3.01844553599998));
#305812=CARTESIAN_POINT('Ctrl Pts',(-2.74170608200006,5.2,3.01844553599998));
#305813=CARTESIAN_POINT('Ctrl Pts',(-2.74170608200006,2.2,3.01844553599998));
#305814=CARTESIAN_POINT('Ctrl Pts',(-2.74119120600006,12.2,3.01757602599999));
#305815=CARTESIAN_POINT('Ctrl Pts',(-2.74119120600006,5.2,3.01757602599999));
#305816=CARTESIAN_POINT('Ctrl Pts',(-2.74119120600006,2.2,3.01757602599999));
#305817=CARTESIAN_POINT('Ctrl Pts',(-2.74067805200006,12.2,3.01671185499998));
#305818=CARTESIAN_POINT('Ctrl Pts',(-2.74067805200006,5.2,3.01671185499998));
#305819=CARTESIAN_POINT('Ctrl Pts',(-2.74067805200006,2.2,3.01671185499998));
#305820=CARTESIAN_POINT('Ctrl Pts',(-2.74016663800006,12.2,3.01585302399998));
#305821=CARTESIAN_POINT('Ctrl Pts',(-2.74016663800006,5.2,3.01585302399998));
#305822=CARTESIAN_POINT('Ctrl Pts',(-2.74016663800006,2.2,3.01585302399998));
#305823=CARTESIAN_POINT('Ctrl Pts',(-2.73965698000006,12.2,3.01499953699999));
#305824=CARTESIAN_POINT('Ctrl Pts',(-2.73965698000006,5.2,3.01499953699999));
#305825=CARTESIAN_POINT('Ctrl Pts',(-2.73965698000006,2.2,3.01499953699999));
#305826=CARTESIAN_POINT('Ctrl Pts',(-2.73914909500005,12.2,3.01415139599998));
#305827=CARTESIAN_POINT('Ctrl Pts',(-2.73914909500005,5.2,3.01415139599998));
#305828=CARTESIAN_POINT('Ctrl Pts',(-2.73914909500005,2.2,3.01415139599998));
#305829=CARTESIAN_POINT('Ctrl Pts',(-2.73864299800006,12.2,3.01330860299998));
#305830=CARTESIAN_POINT('Ctrl Pts',(-2.73864299800006,5.2,3.01330860299998));
#305831=CARTESIAN_POINT('Ctrl Pts',(-2.73864299800006,2.2,3.01330860299998));
#305832=CARTESIAN_POINT('Ctrl Pts',(-2.73813870800006,12.2,3.01247116199999));
#305833=CARTESIAN_POINT('Ctrl Pts',(-2.73813870800006,5.2,3.01247116199999));
#305834=CARTESIAN_POINT('Ctrl Pts',(-2.73813870800006,2.2,3.01247116199999));
#305835=CARTESIAN_POINT('Ctrl Pts',(-2.73763624000006,12.2,3.01163907399999));
#305836=CARTESIAN_POINT('Ctrl Pts',(-2.73763624000006,5.2,3.01163907399999));
#305837=CARTESIAN_POINT('Ctrl Pts',(-2.73763624000006,2.2,3.01163907399999));
#305838=CARTESIAN_POINT('Ctrl Pts',(-2.73713561000006,12.2,3.01081234199999));
#305839=CARTESIAN_POINT('Ctrl Pts',(-2.73713561000006,5.2,3.01081234199999));
#305840=CARTESIAN_POINT('Ctrl Pts',(-2.73713561000006,2.2,3.01081234199999));
#305841=CARTESIAN_POINT('Ctrl Pts',(-2.73663683700006,12.2,3.00999096999998));
#305842=CARTESIAN_POINT('Ctrl Pts',(-2.73663683700006,5.2,3.00999096999998));
#305843=CARTESIAN_POINT('Ctrl Pts',(-2.73663683700006,2.2,3.00999096999998));
#305844=CARTESIAN_POINT('Ctrl Pts',(-2.73613993700006,12.2,3.00917495999999));
#305845=CARTESIAN_POINT('Ctrl Pts',(-2.73613993700006,5.2,3.00917495999999));
#305846=CARTESIAN_POINT('Ctrl Pts',(-2.73613993700006,2.2,3.00917495999999));
#305847=CARTESIAN_POINT('Ctrl Pts',(-2.73564492500005,12.2,3.00836431199999));
#305848=CARTESIAN_POINT('Ctrl Pts',(-2.73564492500005,5.2,3.00836431199999));
#305849=CARTESIAN_POINT('Ctrl Pts',(-2.73564492500005,2.2,3.00836431199999));
#305850=CARTESIAN_POINT('Ctrl Pts',(-2.73515182000006,12.2,3.00755903099999));
#305851=CARTESIAN_POINT('Ctrl Pts',(-2.73515182000006,5.2,3.00755903099999));
#305852=CARTESIAN_POINT('Ctrl Pts',(-2.73515182000006,2.2,3.00755903099999));
#305853=CARTESIAN_POINT('Ctrl Pts',(-2.73466063800006,12.2,3.00675911899998));
#305854=CARTESIAN_POINT('Ctrl Pts',(-2.73466063800006,5.2,3.00675911899998));
#305855=CARTESIAN_POINT('Ctrl Pts',(-2.73466063800006,2.2,3.00675911899998));
#305856=CARTESIAN_POINT('Ctrl Pts',(-2.73417139700005,12.2,3.00596457899999));
#305857=CARTESIAN_POINT('Ctrl Pts',(-2.73417139700005,5.2,3.00596457899999));
#305858=CARTESIAN_POINT('Ctrl Pts',(-2.73417139700005,2.2,3.00596457899999));
#305859=CARTESIAN_POINT('Ctrl Pts',(-2.73368411300006,12.2,3.00517541299998));
#305860=CARTESIAN_POINT('Ctrl Pts',(-2.73368411300006,5.2,3.00517541299998));
#305861=CARTESIAN_POINT('Ctrl Pts',(-2.73368411300006,2.2,3.00517541299998));
#305862=CARTESIAN_POINT('Ctrl Pts',(-2.73319880200006,12.2,3.00439162199999));
#305863=CARTESIAN_POINT('Ctrl Pts',(-2.73319880200006,5.2,3.00439162199999));
#305864=CARTESIAN_POINT('Ctrl Pts',(-2.73319880200006,2.2,3.00439162199999));
#305865=CARTESIAN_POINT('Ctrl Pts',(-2.73271548400006,12.2,3.00361320999999));
#305866=CARTESIAN_POINT('Ctrl Pts',(-2.73271548400006,5.2,3.00361320999999));
#305867=CARTESIAN_POINT('Ctrl Pts',(-2.73271548400006,2.2,3.00361320999999));
#305868=CARTESIAN_POINT('Ctrl Pts',(-2.73223417300006,12.2,3.00284017899998));
#305869=CARTESIAN_POINT('Ctrl Pts',(-2.73223417300006,5.2,3.00284017899998));
#305870=CARTESIAN_POINT('Ctrl Pts',(-2.73223417300006,2.2,3.00284017899998));
#305871=CARTESIAN_POINT('Ctrl Pts',(-2.73175488900006,12.2,3.00207253199999));
#305872=CARTESIAN_POINT('Ctrl Pts',(-2.73175488900006,5.2,3.00207253199999));
#305873=CARTESIAN_POINT('Ctrl Pts',(-2.73175488900006,2.2,3.00207253199999));
#305874=CARTESIAN_POINT('Ctrl Pts',(-2.73127764700006,12.2,3.00131027199999));
#305875=CARTESIAN_POINT('Ctrl Pts',(-2.73127764700006,5.2,3.00131027199999));
#305876=CARTESIAN_POINT('Ctrl Pts',(-2.73127764700006,2.2,3.00131027199999));
#305877=CARTESIAN_POINT('Ctrl Pts',(-2.73080246700005,12.2,3.00055339899998));
#305878=CARTESIAN_POINT('Ctrl Pts',(-2.73080246700005,5.2,3.00055339899998));
#305879=CARTESIAN_POINT('Ctrl Pts',(-2.73080246700005,2.2,3.00055339899998));
#305880=CARTESIAN_POINT('Ctrl Pts',(-2.73032936400006,12.2,2.99980191599998));
#305881=CARTESIAN_POINT('Ctrl Pts',(-2.73032936400006,5.2,2.99980191599998));
#305882=CARTESIAN_POINT('Ctrl Pts',(-2.73032936400006,2.2,2.99980191599998));
#305883=CARTESIAN_POINT('Ctrl Pts',(-2.72985835500006,12.2,2.99905582699999));
#305884=CARTESIAN_POINT('Ctrl Pts',(-2.72985835500006,5.2,2.99905582699999));
#305885=CARTESIAN_POINT('Ctrl Pts',(-2.72985835500006,2.2,2.99905582699999));
#305886=CARTESIAN_POINT('Ctrl Pts',(-2.72938946000005,12.2,2.99831513299999));
#305887=CARTESIAN_POINT('Ctrl Pts',(-2.72938946000005,5.2,2.99831513299999));
#305888=CARTESIAN_POINT('Ctrl Pts',(-2.72938946000005,2.2,2.99831513299999));
#305889=CARTESIAN_POINT('Ctrl Pts',(-2.72892269400006,12.2,2.99757983599999));
#305890=CARTESIAN_POINT('Ctrl Pts',(-2.72892269400006,5.2,2.99757983599999));
#305891=CARTESIAN_POINT('Ctrl Pts',(-2.72892269400006,2.2,2.99757983599999));
#305892=CARTESIAN_POINT('Ctrl Pts',(-2.72845807600006,12.2,2.99684993899999));
#305893=CARTESIAN_POINT('Ctrl Pts',(-2.72845807600006,5.2,2.99684993899999));
#305894=CARTESIAN_POINT('Ctrl Pts',(-2.72845807600006,2.2,2.99684993899999));
#305895=CARTESIAN_POINT('Ctrl Pts',(-2.72799562300006,12.2,2.99612544499999));
#305896=CARTESIAN_POINT('Ctrl Pts',(-2.72799562300006,5.2,2.99612544499999));
#305897=CARTESIAN_POINT('Ctrl Pts',(-2.72799562300006,2.2,2.99612544499999));
#305898=CARTESIAN_POINT('Ctrl Pts',(-2.72753535200006,12.2,2.99540635399998));
#305899=CARTESIAN_POINT('Ctrl Pts',(-2.72753535200006,5.2,2.99540635399998));
#305900=CARTESIAN_POINT('Ctrl Pts',(-2.72753535200006,2.2,2.99540635399998));
#305901=CARTESIAN_POINT('Ctrl Pts',(-2.72707728300006,12.2,2.99469267099998));
#305902=CARTESIAN_POINT('Ctrl Pts',(-2.72707728300006,5.2,2.99469267099998));
#305903=CARTESIAN_POINT('Ctrl Pts',(-2.72707728300006,2.2,2.99469267099998));
#305904=CARTESIAN_POINT('Ctrl Pts',(-2.72662143200006,12.2,2.99398439599998));
#305905=CARTESIAN_POINT('Ctrl Pts',(-2.72662143200006,5.2,2.99398439599998));
#305906=CARTESIAN_POINT('Ctrl Pts',(-2.72662143200006,2.2,2.99398439599998));
#305907=CARTESIAN_POINT('Ctrl Pts',(-2.72616781700005,12.2,2.99328153199999));
#305908=CARTESIAN_POINT('Ctrl Pts',(-2.72616781700005,5.2,2.99328153199999));
#305909=CARTESIAN_POINT('Ctrl Pts',(-2.72616781700005,2.2,2.99328153199999));
#305910=CARTESIAN_POINT('Ctrl Pts',(-2.72571645600005,12.2,2.99258408199999));
#305911=CARTESIAN_POINT('Ctrl Pts',(-2.72571645600005,5.2,2.99258408199999));
#305912=CARTESIAN_POINT('Ctrl Pts',(-2.72571645600005,2.2,2.99258408199999));
#305913=CARTESIAN_POINT('Ctrl Pts',(-2.72526736600006,12.2,2.99189204699999));
#305914=CARTESIAN_POINT('Ctrl Pts',(-2.72526736600006,5.2,2.99189204699999));
#305915=CARTESIAN_POINT('Ctrl Pts',(-2.72526736600006,2.2,2.99189204699999));
#305916=CARTESIAN_POINT('Ctrl Pts',(-2.72482056700006,12.2,2.99120542899999));
#305917=CARTESIAN_POINT('Ctrl Pts',(-2.72482056700006,5.2,2.99120542899999));
#305918=CARTESIAN_POINT('Ctrl Pts',(-2.72482056700006,2.2,2.99120542899999));
#305919=CARTESIAN_POINT('Ctrl Pts',(-2.72437607500006,12.2,2.99052423099998));
#305920=CARTESIAN_POINT('Ctrl Pts',(-2.72437607500006,5.2,2.99052423099998));
#305921=CARTESIAN_POINT('Ctrl Pts',(-2.72437607500006,2.2,2.99052423099998));
#305922=CARTESIAN_POINT('Ctrl Pts',(-2.72393390900006,12.2,2.98984845499999));
#305923=CARTESIAN_POINT('Ctrl Pts',(-2.72393390900006,5.2,2.98984845499999));
#305924=CARTESIAN_POINT('Ctrl Pts',(-2.72393390900006,2.2,2.98984845499999));
#305925=CARTESIAN_POINT('Ctrl Pts',(-2.72349408800005,12.2,2.98917810299999));
#305926=CARTESIAN_POINT('Ctrl Pts',(-2.72349408800005,5.2,2.98917810299999));
#305927=CARTESIAN_POINT('Ctrl Pts',(-2.72349408800005,2.2,2.98917810299999));
#305928=CARTESIAN_POINT('Ctrl Pts',(-2.72305662800005,12.2,2.98851317699998));
#305929=CARTESIAN_POINT('Ctrl Pts',(-2.72305662800005,5.2,2.98851317699998));
#305930=CARTESIAN_POINT('Ctrl Pts',(-2.72305662800005,2.2,2.98851317699998));
#305931=CARTESIAN_POINT('Ctrl Pts',(-2.72262154800006,12.2,2.98785367799999));
#305932=CARTESIAN_POINT('Ctrl Pts',(-2.72262154800006,5.2,2.98785367799999));
#305933=CARTESIAN_POINT('Ctrl Pts',(-2.72262154800006,2.2,2.98785367799999));
#305934=CARTESIAN_POINT('Ctrl Pts',(-2.72218886800006,12.2,2.98719960999998));
#305935=CARTESIAN_POINT('Ctrl Pts',(-2.72218886800006,5.2,2.98719960999998));
#305936=CARTESIAN_POINT('Ctrl Pts',(-2.72218886800006,2.2,2.98719960999998));
#305937=CARTESIAN_POINT('Ctrl Pts',(-2.72175860500006,12.2,2.98655097499999));
#305938=CARTESIAN_POINT('Ctrl Pts',(-2.72175860500006,5.2,2.98655097499999));
#305939=CARTESIAN_POINT('Ctrl Pts',(-2.72175860500006,2.2,2.98655097499999));
#305940=CARTESIAN_POINT('Ctrl Pts',(-2.72133077600006,12.2,2.98590777299999));
#305941=CARTESIAN_POINT('Ctrl Pts',(-2.72133077600006,5.2,2.98590777299999));
#305942=CARTESIAN_POINT('Ctrl Pts',(-2.72133077600006,2.2,2.98590777299999));
#305943=CARTESIAN_POINT('Ctrl Pts',(-2.72090540100006,12.2,2.98527000799999));
#305944=CARTESIAN_POINT('Ctrl Pts',(-2.72090540100006,5.2,2.98527000799999));
#305945=CARTESIAN_POINT('Ctrl Pts',(-2.72090540100006,2.2,2.98527000799999));
#305946=CARTESIAN_POINT('Ctrl Pts',(-2.72048249900006,12.2,2.98463768099998));
#305947=CARTESIAN_POINT('Ctrl Pts',(-2.72048249900006,5.2,2.98463768099998));
#305948=CARTESIAN_POINT('Ctrl Pts',(-2.72048249900006,2.2,2.98463768099998));
#305949=CARTESIAN_POINT('Ctrl Pts',(-2.72006208700006,12.2,2.98401079399999));
#305950=CARTESIAN_POINT('Ctrl Pts',(-2.72006208700006,5.2,2.98401079399999));
#305951=CARTESIAN_POINT('Ctrl Pts',(-2.72006208700006,2.2,2.98401079399999));
#305952=CARTESIAN_POINT('Ctrl Pts',(-2.71964418500006,12.2,2.98338934899999));
#305953=CARTESIAN_POINT('Ctrl Pts',(-2.71964418500006,5.2,2.98338934899999));
#305954=CARTESIAN_POINT('Ctrl Pts',(-2.71964418500006,2.2,2.98338934899999));
#305955=CARTESIAN_POINT('Ctrl Pts',(-2.71922881200005,12.2,2.98277334899999));
#305956=CARTESIAN_POINT('Ctrl Pts',(-2.71922881200005,5.2,2.98277334899999));
#305957=CARTESIAN_POINT('Ctrl Pts',(-2.71922881200005,2.2,2.98277334899999));
#305958=CARTESIAN_POINT('Ctrl Pts',(-2.71881598400005,12.2,2.98216279399998));
#305959=CARTESIAN_POINT('Ctrl Pts',(-2.71881598400005,5.2,2.98216279399998));
#305960=CARTESIAN_POINT('Ctrl Pts',(-2.71881598400005,2.2,2.98216279399998));
#305961=CARTESIAN_POINT('Ctrl Pts',(-2.71840572200006,12.2,2.98155768799998));
#305962=CARTESIAN_POINT('Ctrl Pts',(-2.71840572200006,5.2,2.98155768799998));
#305963=CARTESIAN_POINT('Ctrl Pts',(-2.71840572200006,2.2,2.98155768799998));
#305964=CARTESIAN_POINT('Ctrl Pts',(-2.71799804400006,12.2,2.98095803099999));
#305965=CARTESIAN_POINT('Ctrl Pts',(-2.71799804400006,5.2,2.98095803099999));
#305966=CARTESIAN_POINT('Ctrl Pts',(-2.71799804400006,2.2,2.98095803099999));
#305967=CARTESIAN_POINT('Ctrl Pts',(-2.71759297000005,12.2,2.98036382599999));
#305968=CARTESIAN_POINT('Ctrl Pts',(-2.71759297000005,5.2,2.98036382599999));
#305969=CARTESIAN_POINT('Ctrl Pts',(-2.71759297000005,2.2,2.98036382599999));
#305970=CARTESIAN_POINT('Ctrl Pts',(-2.71719051700006,12.2,2.97977507499999));
#305971=CARTESIAN_POINT('Ctrl Pts',(-2.71719051700006,5.2,2.97977507499999));
#305972=CARTESIAN_POINT('Ctrl Pts',(-2.71719051700006,2.2,2.97977507499999));
#305973=CARTESIAN_POINT('Ctrl Pts',(-2.71679070600006,12.2,2.97919177799999));
#305974=CARTESIAN_POINT('Ctrl Pts',(-2.71679070600006,5.2,2.97919177799999));
#305975=CARTESIAN_POINT('Ctrl Pts',(-2.71679070600006,2.2,2.97919177799999));
#305976=CARTESIAN_POINT('Ctrl Pts',(-2.71639355500006,12.2,2.97861393899999));
#305977=CARTESIAN_POINT('Ctrl Pts',(-2.71639355500006,5.2,2.97861393899999));
#305978=CARTESIAN_POINT('Ctrl Pts',(-2.71639355500006,2.2,2.97861393899999));
#305979=CARTESIAN_POINT('Ctrl Pts',(-2.71599908200006,12.2,2.97804155899998));
#305980=CARTESIAN_POINT('Ctrl Pts',(-2.71599908200006,5.2,2.97804155899998));
#305981=CARTESIAN_POINT('Ctrl Pts',(-2.71599908200006,2.2,2.97804155899998));
#305982=CARTESIAN_POINT('Ctrl Pts',(-2.71560730900006,12.2,2.97747463999999));
#305983=CARTESIAN_POINT('Ctrl Pts',(-2.71560730900006,5.2,2.97747463999999));
#305984=CARTESIAN_POINT('Ctrl Pts',(-2.71560730900006,2.2,2.97747463999999));
#305985=CARTESIAN_POINT('Ctrl Pts',(-2.71521825300006,12.2,2.97691318299999));
#305986=CARTESIAN_POINT('Ctrl Pts',(-2.71521825300006,5.2,2.97691318299999));
#305987=CARTESIAN_POINT('Ctrl Pts',(-2.71521825300006,2.2,2.97691318299999));
#305988=CARTESIAN_POINT('Ctrl Pts',(-2.71483193400006,12.2,2.97635718999998));
#305989=CARTESIAN_POINT('Ctrl Pts',(-2.71483193400006,5.2,2.97635718999998));
#305990=CARTESIAN_POINT('Ctrl Pts',(-2.71483193400006,2.2,2.97635718999998));
#305991=CARTESIAN_POINT('Ctrl Pts',(-2.71444837100006,12.2,2.97580666399998));
#305992=CARTESIAN_POINT('Ctrl Pts',(-2.71444837100006,5.2,2.97580666399998));
#305993=CARTESIAN_POINT('Ctrl Pts',(-2.71444837100006,2.2,2.97580666399998));
#305994=CARTESIAN_POINT('Ctrl Pts',(-2.71406758200006,12.2,2.97526160499999));
#305995=CARTESIAN_POINT('Ctrl Pts',(-2.71406758200006,5.2,2.97526160499999));
#305996=CARTESIAN_POINT('Ctrl Pts',(-2.71406758200006,2.2,2.97526160499999));
#305997=CARTESIAN_POINT('Ctrl Pts',(-2.71368959000006,12.2,2.97472201499998));
#305998=CARTESIAN_POINT('Ctrl Pts',(-2.71368959000006,5.2,2.97472201499998));
#305999=CARTESIAN_POINT('Ctrl Pts',(-2.71368959000006,2.2,2.97472201499998));
#306000=CARTESIAN_POINT('Ctrl Pts',(-2.71331441200005,12.2,2.97418789699999));
#306001=CARTESIAN_POINT('Ctrl Pts',(-2.71331441200005,5.2,2.97418789699999));
#306002=CARTESIAN_POINT('Ctrl Pts',(-2.71331441200005,2.2,2.97418789699999));
#306003=CARTESIAN_POINT('Ctrl Pts',(-2.71294206700006,12.2,2.97365925099999));
#306004=CARTESIAN_POINT('Ctrl Pts',(-2.71294206700006,5.2,2.97365925099999));
#306005=CARTESIAN_POINT('Ctrl Pts',(-2.71294206700006,2.2,2.97365925099999));
#306006=CARTESIAN_POINT('Ctrl Pts',(-2.71257257700006,12.2,2.97313607899999));
#306007=CARTESIAN_POINT('Ctrl Pts',(-2.71257257700006,5.2,2.97313607899999));
#306008=CARTESIAN_POINT('Ctrl Pts',(-2.71257257700006,2.2,2.97313607899999));
#306009=CARTESIAN_POINT('Ctrl Pts',(-2.71220595900005,12.2,2.97261838399999));
#306010=CARTESIAN_POINT('Ctrl Pts',(-2.71220595900005,5.2,2.97261838399999));
#306011=CARTESIAN_POINT('Ctrl Pts',(-2.71220595900005,2.2,2.97261838399999));
#306012=CARTESIAN_POINT('Ctrl Pts',(-2.71184223500006,12.2,2.97210616599998));
#306013=CARTESIAN_POINT('Ctrl Pts',(-2.71184223500006,5.2,2.97210616599998));
#306014=CARTESIAN_POINT('Ctrl Pts',(-2.71184223500006,2.2,2.97210616599998));
#306015=CARTESIAN_POINT('Ctrl Pts',(-2.71148142300006,12.2,2.97159942699999));
#306016=CARTESIAN_POINT('Ctrl Pts',(-2.71148142300006,5.2,2.97159942699999));
#306017=CARTESIAN_POINT('Ctrl Pts',(-2.71148142300006,2.2,2.97159942699999));
#306018=CARTESIAN_POINT('Ctrl Pts',(-2.71112354500006,12.2,2.97109816899999));
#306019=CARTESIAN_POINT('Ctrl Pts',(-2.71112354500006,5.2,2.97109816899999));
#306020=CARTESIAN_POINT('Ctrl Pts',(-2.71112354500006,2.2,2.97109816899999));
#306021=CARTESIAN_POINT('Ctrl Pts',(-2.71076861900006,12.2,2.97060239299999));
#306022=CARTESIAN_POINT('Ctrl Pts',(-2.71076861900006,5.2,2.97060239299999));
#306023=CARTESIAN_POINT('Ctrl Pts',(-2.71076861900006,2.2,2.97060239299999));
#306024=CARTESIAN_POINT('Ctrl Pts',(-2.71041666500006,12.2,2.97011210099999));
#306025=CARTESIAN_POINT('Ctrl Pts',(-2.71041666500006,5.2,2.97011210099999));
#306026=CARTESIAN_POINT('Ctrl Pts',(-2.71041666500006,2.2,2.97011210099999));
#306027=CARTESIAN_POINT('Ctrl Pts',(-2.71006770400006,12.2,2.96962729299998));
#306028=CARTESIAN_POINT('Ctrl Pts',(-2.71006770400006,5.2,2.96962729299998));
#306029=CARTESIAN_POINT('Ctrl Pts',(-2.71006770400006,2.2,2.96962729299998));
#306030=CARTESIAN_POINT('Ctrl Pts',(-2.70972175600006,12.2,2.96914797299999));
#306031=CARTESIAN_POINT('Ctrl Pts',(-2.70972175600006,5.2,2.96914797299999));
#306032=CARTESIAN_POINT('Ctrl Pts',(-2.70972175600006,2.2,2.96914797299999));
#306033=CARTESIAN_POINT('Ctrl Pts',(-2.70937884100006,12.2,2.96867414099999));
#306034=CARTESIAN_POINT('Ctrl Pts',(-2.70937884100006,5.2,2.96867414099999));
#306035=CARTESIAN_POINT('Ctrl Pts',(-2.70937884100006,2.2,2.96867414099999));
#306036=CARTESIAN_POINT('Ctrl Pts',(-2.70903897900005,12.2,2.96820579799999));
#306037=CARTESIAN_POINT('Ctrl Pts',(-2.70903897900005,5.2,2.96820579799999));
#306038=CARTESIAN_POINT('Ctrl Pts',(-2.70903897900005,2.2,2.96820579799999));
#306039=CARTESIAN_POINT('Ctrl Pts',(-2.70870219000006,12.2,2.96774294599999));
#306040=CARTESIAN_POINT('Ctrl Pts',(-2.70870219000006,5.2,2.96774294599999));
#306041=CARTESIAN_POINT('Ctrl Pts',(-2.70870219000006,2.2,2.96774294599999));
#306042=CARTESIAN_POINT('Ctrl Pts',(-2.70836849500005,12.2,2.96728558799998));
#306043=CARTESIAN_POINT('Ctrl Pts',(-2.70836849500005,5.2,2.96728558799998));
#306044=CARTESIAN_POINT('Ctrl Pts',(-2.70836849500005,2.2,2.96728558799998));
#306045=CARTESIAN_POINT('Ctrl Pts',(-2.70803791400006,12.2,2.96683372199999));
#306046=CARTESIAN_POINT('Ctrl Pts',(-2.70803791400006,5.2,2.96683372199999));
#306047=CARTESIAN_POINT('Ctrl Pts',(-2.70803791400006,2.2,2.96683372199999));
#306048=CARTESIAN_POINT('Ctrl Pts',(-2.70771046800005,12.2,2.96638735199998));
#306049=CARTESIAN_POINT('Ctrl Pts',(-2.70771046800005,5.2,2.96638735199998));
#306050=CARTESIAN_POINT('Ctrl Pts',(-2.70771046800005,2.2,2.96638735199998));
#306051=CARTESIAN_POINT('Ctrl Pts',(-2.70738617800005,12.2,2.96594647899998));
#306052=CARTESIAN_POINT('Ctrl Pts',(-2.70738617800005,5.2,2.96594647899998));
#306053=CARTESIAN_POINT('Ctrl Pts',(-2.70738617800005,2.2,2.96594647899998));
#306054=CARTESIAN_POINT('Ctrl Pts',(-2.70706506300006,12.2,2.96551110199999));
#306055=CARTESIAN_POINT('Ctrl Pts',(-2.70706506300006,5.2,2.96551110199999));
#306056=CARTESIAN_POINT('Ctrl Pts',(-2.70706506300006,2.2,2.96551110199999));
#306057=CARTESIAN_POINT('Ctrl Pts',(-2.70674714400006,12.2,2.96508122599998));
#306058=CARTESIAN_POINT('Ctrl Pts',(-2.70674714400006,5.2,2.96508122599998));
#306059=CARTESIAN_POINT('Ctrl Pts',(-2.70674714400006,2.2,2.96508122599998));
#306060=CARTESIAN_POINT('Ctrl Pts',(-2.70643244300006,12.2,2.96465684899999));
#306061=CARTESIAN_POINT('Ctrl Pts',(-2.70643244300006,5.2,2.96465684899999));
#306062=CARTESIAN_POINT('Ctrl Pts',(-2.70643244300006,2.2,2.96465684899999));
#306063=CARTESIAN_POINT('Ctrl Pts',(-2.70612098000006,12.2,2.96423797499998));
#306064=CARTESIAN_POINT('Ctrl Pts',(-2.70612098000006,5.2,2.96423797499998));
#306065=CARTESIAN_POINT('Ctrl Pts',(-2.70612098000006,2.2,2.96423797499998));
#306066=CARTESIAN_POINT('Ctrl Pts',(-2.70581277600006,12.2,2.96382460299998));
#306067=CARTESIAN_POINT('Ctrl Pts',(-2.70581277600006,5.2,2.96382460299998));
#306068=CARTESIAN_POINT('Ctrl Pts',(-2.70581277600006,2.2,2.96382460299998));
#306069=CARTESIAN_POINT('Ctrl Pts',(-2.70550785200005,12.2,2.96341673499998));
#306070=CARTESIAN_POINT('Ctrl Pts',(-2.70550785200005,5.2,2.96341673499998));
#306071=CARTESIAN_POINT('Ctrl Pts',(-2.70550785200005,2.2,2.96341673499998));
#306072=CARTESIAN_POINT('Ctrl Pts',(-2.70520622700006,12.2,2.96301437299999));
#306073=CARTESIAN_POINT('Ctrl Pts',(-2.70520622700006,5.2,2.96301437299999));
#306074=CARTESIAN_POINT('Ctrl Pts',(-2.70520622700006,2.2,2.96301437299999));
#306075=CARTESIAN_POINT('Ctrl Pts',(-2.70490792600006,12.2,2.96261751699999));
#306076=CARTESIAN_POINT('Ctrl Pts',(-2.70490792600006,5.2,2.96261751699999));
#306077=CARTESIAN_POINT('Ctrl Pts',(-2.70490792600006,2.2,2.96261751699999));
#306078=CARTESIAN_POINT('Ctrl Pts',(-2.70461296800006,12.2,2.96222616899998));
#306079=CARTESIAN_POINT('Ctrl Pts',(-2.70461296800006,5.2,2.96222616899998));
#306080=CARTESIAN_POINT('Ctrl Pts',(-2.70461296800006,2.2,2.96222616899998));
#306081=CARTESIAN_POINT('Ctrl Pts',(-2.70432137400006,12.2,2.96184032999999));
#306082=CARTESIAN_POINT('Ctrl Pts',(-2.70432137400006,5.2,2.96184032999999));
#306083=CARTESIAN_POINT('Ctrl Pts',(-2.70432137400006,2.2,2.96184032999999));
#306084=CARTESIAN_POINT('Ctrl Pts',(-2.70403316500006,12.2,2.96145999999998));
#306085=CARTESIAN_POINT('Ctrl Pts',(-2.70403316500006,5.2,2.96145999999998));
#306086=CARTESIAN_POINT('Ctrl Pts',(-2.70403316500006,2.2,2.96145999999998));
#306087=CARTESIAN_POINT('Ctrl Pts',(-2.70374836300005,12.2,2.96108518199999));
#306088=CARTESIAN_POINT('Ctrl Pts',(-2.70374836300005,5.2,2.96108518199999));
#306089=CARTESIAN_POINT('Ctrl Pts',(-2.70374836300005,2.2,2.96108518199999));
#306090=CARTESIAN_POINT('Ctrl Pts',(-2.70346699000005,12.2,2.96071587499998));
#306091=CARTESIAN_POINT('Ctrl Pts',(-2.70346699000005,5.2,2.96071587499998));
#306092=CARTESIAN_POINT('Ctrl Pts',(-2.70346699000005,2.2,2.96071587499998));
#306093=CARTESIAN_POINT('Ctrl Pts',(-2.70318906600005,12.2,2.96035208099998));
#306094=CARTESIAN_POINT('Ctrl Pts',(-2.70318906600005,5.2,2.96035208099998));
#306095=CARTESIAN_POINT('Ctrl Pts',(-2.70318906600005,2.2,2.96035208099998));
#306096=CARTESIAN_POINT('Ctrl Pts',(-2.70291461400006,12.2,2.95999380199999));
#306097=CARTESIAN_POINT('Ctrl Pts',(-2.70291461400006,5.2,2.95999380199999));
#306098=CARTESIAN_POINT('Ctrl Pts',(-2.70291461400006,2.2,2.95999380199999));
#306099=CARTESIAN_POINT('Ctrl Pts',(-2.70264365500006,12.2,2.95964103799999));
#306100=CARTESIAN_POINT('Ctrl Pts',(-2.70264365500006,5.2,2.95964103799999));
#306101=CARTESIAN_POINT('Ctrl Pts',(-2.70264365500006,2.2,2.95964103799999));
#306102=CARTESIAN_POINT('Ctrl Pts',(-2.70237621000006,12.2,2.95929378999999));
#306103=CARTESIAN_POINT('Ctrl Pts',(-2.70237621000006,5.2,2.95929378999999));
#306104=CARTESIAN_POINT('Ctrl Pts',(-2.70237621000006,2.2,2.95929378999999));
#306105=CARTESIAN_POINT('Ctrl Pts',(-2.70211230200006,12.2,2.95895205899999));
#306106=CARTESIAN_POINT('Ctrl Pts',(-2.70211230200006,5.2,2.95895205899999));
#306107=CARTESIAN_POINT('Ctrl Pts',(-2.70211230200006,2.2,2.95895205899999));
#306108=CARTESIAN_POINT('Ctrl Pts',(-2.70185195200006,12.2,2.95861584499999));
#306109=CARTESIAN_POINT('Ctrl Pts',(-2.70185195200006,5.2,2.95861584499999));
#306110=CARTESIAN_POINT('Ctrl Pts',(-2.70185195200006,2.2,2.95861584499999));
#306111=CARTESIAN_POINT('Ctrl Pts',(-2.70159518200006,12.2,2.95828515199998));
#306112=CARTESIAN_POINT('Ctrl Pts',(-2.70159518200006,5.2,2.95828515199998));
#306113=CARTESIAN_POINT('Ctrl Pts',(-2.70159518200006,2.2,2.95828515199998));
#306114=CARTESIAN_POINT('Ctrl Pts',(-2.70134201400006,12.2,2.95795997799999));
#306115=CARTESIAN_POINT('Ctrl Pts',(-2.70134201400006,5.2,2.95795997799999));
#306116=CARTESIAN_POINT('Ctrl Pts',(-2.70134201400006,2.2,2.95795997799999));
#306117=CARTESIAN_POINT('Ctrl Pts',(-2.70109247100006,12.2,2.95764032399998));
#306118=CARTESIAN_POINT('Ctrl Pts',(-2.70109247100006,5.2,2.95764032399998));
#306119=CARTESIAN_POINT('Ctrl Pts',(-2.70109247100006,2.2,2.95764032399998));
#306120=CARTESIAN_POINT('Ctrl Pts',(-2.70084657300006,12.2,2.95732619099999));
#306121=CARTESIAN_POINT('Ctrl Pts',(-2.70084657300006,5.2,2.95732619099999));
#306122=CARTESIAN_POINT('Ctrl Pts',(-2.70084657300006,2.2,2.95732619099999));
#306123=CARTESIAN_POINT('Ctrl Pts',(-2.70060434500006,12.2,2.95701758199999));
#306124=CARTESIAN_POINT('Ctrl Pts',(-2.70060434500006,5.2,2.95701758199999));
#306125=CARTESIAN_POINT('Ctrl Pts',(-2.70060434500006,2.2,2.95701758199999));
#306126=CARTESIAN_POINT('Ctrl Pts',(-2.70036580700005,12.2,2.95671449499999));
#306127=CARTESIAN_POINT('Ctrl Pts',(-2.70036580700005,5.2,2.95671449499999));
#306128=CARTESIAN_POINT('Ctrl Pts',(-2.70036580700005,2.2,2.95671449499999));
#306129=CARTESIAN_POINT('Ctrl Pts',(-2.70013098200006,12.2,2.95641693199999));
#306130=CARTESIAN_POINT('Ctrl Pts',(-2.70013098200006,5.2,2.95641693199999));
#306131=CARTESIAN_POINT('Ctrl Pts',(-2.70013098200006,2.2,2.95641693199999));
#306132=CARTESIAN_POINT('Ctrl Pts',(-2.69989989300006,12.2,2.95612489399999));
#306133=CARTESIAN_POINT('Ctrl Pts',(-2.69989989300006,5.2,2.95612489399999));
#306134=CARTESIAN_POINT('Ctrl Pts',(-2.69989989300006,2.2,2.95612489399999));
#306135=CARTESIAN_POINT('Ctrl Pts',(-2.69967256100006,12.2,2.95583838199998));
#306136=CARTESIAN_POINT('Ctrl Pts',(-2.69967256100006,5.2,2.95583838199998));
#306137=CARTESIAN_POINT('Ctrl Pts',(-2.69967256100006,2.2,2.95583838199998));
#306138=CARTESIAN_POINT('Ctrl Pts',(-2.69944901000006,12.2,2.95555739599998));
#306139=CARTESIAN_POINT('Ctrl Pts',(-2.69944901000006,5.2,2.95555739599998));
#306140=CARTESIAN_POINT('Ctrl Pts',(-2.69944901000006,2.2,2.95555739599998));
#306141=CARTESIAN_POINT('Ctrl Pts',(-2.69922926300006,12.2,2.95528193599999));
#306142=CARTESIAN_POINT('Ctrl Pts',(-2.69922926300006,5.2,2.95528193599999));
#306143=CARTESIAN_POINT('Ctrl Pts',(-2.69922926300006,2.2,2.95528193599999));
#306144=CARTESIAN_POINT('Ctrl Pts',(-2.69901334100005,12.2,2.95501200399999));
#306145=CARTESIAN_POINT('Ctrl Pts',(-2.69901334100005,5.2,2.95501200399999));
#306146=CARTESIAN_POINT('Ctrl Pts',(-2.69901334100005,2.2,2.95501200399999));
#306147=CARTESIAN_POINT('Ctrl Pts',(-2.69880126900006,12.2,2.95474759999999));
#306148=CARTESIAN_POINT('Ctrl Pts',(-2.69880126900006,5.2,2.95474759999999));
#306149=CARTESIAN_POINT('Ctrl Pts',(-2.69880126900006,2.2,2.95474759999999));
#306150=CARTESIAN_POINT('Ctrl Pts',(-2.69859306800006,12.2,2.95448872499998));
#306151=CARTESIAN_POINT('Ctrl Pts',(-2.69859306800006,5.2,2.95448872499998));
#306152=CARTESIAN_POINT('Ctrl Pts',(-2.69859306800006,2.2,2.95448872499998));
#306153=CARTESIAN_POINT('Ctrl Pts',(-2.69838876100006,12.2,2.95423537899998));
#306154=CARTESIAN_POINT('Ctrl Pts',(-2.69838876100006,5.2,2.95423537899998));
#306155=CARTESIAN_POINT('Ctrl Pts',(-2.69838876100006,2.2,2.95423537899998));
#306156=CARTESIAN_POINT('Ctrl Pts',(-2.69818837200006,12.2,2.95398756299999));
#306157=CARTESIAN_POINT('Ctrl Pts',(-2.69818837200006,5.2,2.95398756299999));
#306158=CARTESIAN_POINT('Ctrl Pts',(-2.69818837200006,2.2,2.95398756299999));
#306159=CARTESIAN_POINT('Ctrl Pts',(-2.69799192300006,12.2,2.95374527799999));
#306160=CARTESIAN_POINT('Ctrl Pts',(-2.69799192300006,5.2,2.95374527799999));
#306161=CARTESIAN_POINT('Ctrl Pts',(-2.69799192300006,2.2,2.95374527799999));
#306162=CARTESIAN_POINT('Ctrl Pts',(-2.69779943900006,12.2,2.95350852299999));
#306163=CARTESIAN_POINT('Ctrl Pts',(-2.69779943900006,5.2,2.95350852299999));
#306164=CARTESIAN_POINT('Ctrl Pts',(-2.69779943900006,2.2,2.95350852299999));
#306165=CARTESIAN_POINT('Ctrl Pts',(-2.69761094200006,12.2,2.95327730099999));
#306166=CARTESIAN_POINT('Ctrl Pts',(-2.69761094200006,5.2,2.95327730099999));
#306167=CARTESIAN_POINT('Ctrl Pts',(-2.69761094200006,2.2,2.95327730099999));
#306168=CARTESIAN_POINT('Ctrl Pts',(-2.69742645500005,12.2,2.95305160899999));
#306169=CARTESIAN_POINT('Ctrl Pts',(-2.69742645500005,5.2,2.95305160899999));
#306170=CARTESIAN_POINT('Ctrl Pts',(-2.69742645500005,2.2,2.95305160899999));
#306171=CARTESIAN_POINT('Ctrl Pts',(-2.69724600200006,12.2,2.95283144999999));
#306172=CARTESIAN_POINT('Ctrl Pts',(-2.69724600200006,5.2,2.95283144999999));
#306173=CARTESIAN_POINT('Ctrl Pts',(-2.69724600200006,2.2,2.95283144999999));
#306174=CARTESIAN_POINT('Ctrl Pts',(-2.69706960600006,12.2,2.95261682499999));
#306175=CARTESIAN_POINT('Ctrl Pts',(-2.69706960600006,5.2,2.95261682499999));
#306176=CARTESIAN_POINT('Ctrl Pts',(-2.69706960600006,2.2,2.95261682499999));
#306177=CARTESIAN_POINT('Ctrl Pts',(-2.69689729100006,12.2,2.95240773199998));
#306178=CARTESIAN_POINT('Ctrl Pts',(-2.69689729100006,5.2,2.95240773199998));
#306179=CARTESIAN_POINT('Ctrl Pts',(-2.69689729100006,2.2,2.95240773199998));
#306180=CARTESIAN_POINT('Ctrl Pts',(-2.69672908200006,12.2,2.95220417299999));
#306181=CARTESIAN_POINT('Ctrl Pts',(-2.69672908200006,5.2,2.95220417299999));
#306182=CARTESIAN_POINT('Ctrl Pts',(-2.69672908200006,2.2,2.95220417299999));
#306183=CARTESIAN_POINT('Ctrl Pts',(-2.69656500100006,12.2,2.95200614799998));
#306184=CARTESIAN_POINT('Ctrl Pts',(-2.69656500100006,5.2,2.95200614799998));
#306185=CARTESIAN_POINT('Ctrl Pts',(-2.69656500100006,2.2,2.95200614799998));
#306186=CARTESIAN_POINT('Ctrl Pts',(-2.69640507100006,12.2,2.95181365599999));
#306187=CARTESIAN_POINT('Ctrl Pts',(-2.69640507100006,5.2,2.95181365599999));
#306188=CARTESIAN_POINT('Ctrl Pts',(-2.69640507100006,2.2,2.95181365599999));
#306189=CARTESIAN_POINT('Ctrl Pts',(-2.69624931800006,12.2,2.95162669999999));
#306190=CARTESIAN_POINT('Ctrl Pts',(-2.69624931800006,5.2,2.95162669999999));
#306191=CARTESIAN_POINT('Ctrl Pts',(-2.69624931800006,2.2,2.95162669999999));
#306192=CARTESIAN_POINT('Ctrl Pts',(-2.69609776600006,12.2,2.95144527899998));
#306193=CARTESIAN_POINT('Ctrl Pts',(-2.69609776600006,5.2,2.95144527899998));
#306194=CARTESIAN_POINT('Ctrl Pts',(-2.69609776600006,2.2,2.95144527899998));
#306195=CARTESIAN_POINT('Ctrl Pts',(-2.69595043700006,12.2,2.95126939199999));
#306196=CARTESIAN_POINT('Ctrl Pts',(-2.69595043700006,5.2,2.95126939199999));
#306197=CARTESIAN_POINT('Ctrl Pts',(-2.69595043700006,2.2,2.95126939199999));
#306198=CARTESIAN_POINT('Ctrl Pts',(-2.69580735700006,12.2,2.95109904099998));
#306199=CARTESIAN_POINT('Ctrl Pts',(-2.69580735700006,5.2,2.95109904099998));
#306200=CARTESIAN_POINT('Ctrl Pts',(-2.69580735700006,2.2,2.95109904099998));
#306201=CARTESIAN_POINT('Ctrl Pts',(-2.69566854800006,12.2,2.95093422599999));
#306202=CARTESIAN_POINT('Ctrl Pts',(-2.69566854800006,5.2,2.95093422599999));
#306203=CARTESIAN_POINT('Ctrl Pts',(-2.69566854800006,2.2,2.95093422599999));
#306204=CARTESIAN_POINT('Ctrl Pts',(-2.69553403700006,12.2,2.95077494499999));
#306205=CARTESIAN_POINT('Ctrl Pts',(-2.69553403700006,5.2,2.95077494499999));
#306206=CARTESIAN_POINT('Ctrl Pts',(-2.69553403700006,2.2,2.95077494499999));
#306207=CARTESIAN_POINT('Ctrl Pts',(-2.69540384800006,12.2,2.95062120099999));
#306208=CARTESIAN_POINT('Ctrl Pts',(-2.69540384800006,5.2,2.95062120099999));
#306209=CARTESIAN_POINT('Ctrl Pts',(-2.69540384800006,2.2,2.95062120099999));
#306210=CARTESIAN_POINT('Ctrl Pts',(-2.69527800600006,12.2,2.95047299199998));
#306211=CARTESIAN_POINT('Ctrl Pts',(-2.69527800600006,5.2,2.95047299199998));
#306212=CARTESIAN_POINT('Ctrl Pts',(-2.69527800600006,2.2,2.95047299199998));
#306213=CARTESIAN_POINT('Ctrl Pts',(-2.69515653400005,12.2,2.95033031999999));
#306214=CARTESIAN_POINT('Ctrl Pts',(-2.69515653400005,5.2,2.95033031999999));
#306215=CARTESIAN_POINT('Ctrl Pts',(-2.69515653400005,2.2,2.95033031999999));
#306216=CARTESIAN_POINT('Ctrl Pts',(-2.69503945700006,12.2,2.95019318299998));
#306217=CARTESIAN_POINT('Ctrl Pts',(-2.69503945700006,5.2,2.95019318299998));
#306218=CARTESIAN_POINT('Ctrl Pts',(-2.69503945700006,2.2,2.95019318299998));
#306219=CARTESIAN_POINT('Ctrl Pts',(-2.69492680000006,12.2,2.95006158399998));
#306220=CARTESIAN_POINT('Ctrl Pts',(-2.69492680000006,5.2,2.95006158399998));
#306221=CARTESIAN_POINT('Ctrl Pts',(-2.69492680000006,2.2,2.95006158399998));
#306222=CARTESIAN_POINT('Ctrl Pts',(-2.69481858700006,12.2,2.94993551899999));
#306223=CARTESIAN_POINT('Ctrl Pts',(-2.69481858700006,5.2,2.94993551899999));
#306224=CARTESIAN_POINT('Ctrl Pts',(-2.69481858700006,2.2,2.94993551899999));
#306225=CARTESIAN_POINT('Ctrl Pts',(-2.69471484200006,12.2,2.94981499099999));
#306226=CARTESIAN_POINT('Ctrl Pts',(-2.69471484200006,5.2,2.94981499099999));
#306227=CARTESIAN_POINT('Ctrl Pts',(-2.69471484200006,2.2,2.94981499099999));
#306228=CARTESIAN_POINT('Ctrl Pts',(-2.69461559200006,12.2,2.94969999899998));
#306229=CARTESIAN_POINT('Ctrl Pts',(-2.69461559200006,5.2,2.94969999899998));
#306230=CARTESIAN_POINT('Ctrl Pts',(-2.69461559200006,2.2,2.94969999899998));
#306231=CARTESIAN_POINT('Ctrl Pts',(-2.69452086300006,12.2,2.94959054299999));
#306232=CARTESIAN_POINT('Ctrl Pts',(-2.69452086300006,5.2,2.94959054299999));
#306233=CARTESIAN_POINT('Ctrl Pts',(-2.69452086300006,2.2,2.94959054299999));
#306234=CARTESIAN_POINT('Ctrl Pts',(-2.69443068000006,12.2,2.94948662199998));
#306235=CARTESIAN_POINT('Ctrl Pts',(-2.69443068000006,5.2,2.94948662199998));
#306236=CARTESIAN_POINT('Ctrl Pts',(-2.69443068000006,2.2,2.94948662199998));
#306237=CARTESIAN_POINT('Ctrl Pts',(-2.69434507100006,12.2,2.94938823799999));
#306238=CARTESIAN_POINT('Ctrl Pts',(-2.69434507100006,5.2,2.94938823799999));
#306239=CARTESIAN_POINT('Ctrl Pts',(-2.69434507100006,2.2,2.94938823799999));
#306240=CARTESIAN_POINT('Ctrl Pts',(-2.69426406000006,12.2,2.94929538899999));
#306241=CARTESIAN_POINT('Ctrl Pts',(-2.69426406000006,5.2,2.94929538899999));
#306242=CARTESIAN_POINT('Ctrl Pts',(-2.69426406000006,2.2,2.94929538899999));
#306243=CARTESIAN_POINT('Ctrl Pts',(-2.69418766900006,12.2,2.94920807499999));
#306244=CARTESIAN_POINT('Ctrl Pts',(-2.69418766900006,5.2,2.94920807499999));
#306245=CARTESIAN_POINT('Ctrl Pts',(-2.69418766900006,2.2,2.94920807499999));
#306246=CARTESIAN_POINT('Ctrl Pts',(-2.69411592200006,12.2,2.94912629699999));
#306247=CARTESIAN_POINT('Ctrl Pts',(-2.69411592200006,5.2,2.94912629699999));
#306248=CARTESIAN_POINT('Ctrl Pts',(-2.69411592200006,2.2,2.94912629699999));
#306249=CARTESIAN_POINT('Ctrl Pts',(-2.69404884200006,12.2,2.94905005299999));
#306250=CARTESIAN_POINT('Ctrl Pts',(-2.69404884200006,5.2,2.94905005299999));
#306251=CARTESIAN_POINT('Ctrl Pts',(-2.69404884200006,2.2,2.94905005299999));
#306252=CARTESIAN_POINT('Ctrl Pts',(-2.69398645600006,12.2,2.94897934399999));
#306253=CARTESIAN_POINT('Ctrl Pts',(-2.69398645600006,5.2,2.94897934399999));
#306254=CARTESIAN_POINT('Ctrl Pts',(-2.69398645600006,2.2,2.94897934399999));
#306255=CARTESIAN_POINT('Ctrl Pts',(-2.69392879100006,12.2,2.94891416999998));
#306256=CARTESIAN_POINT('Ctrl Pts',(-2.69392879100006,5.2,2.94891416999998));
#306257=CARTESIAN_POINT('Ctrl Pts',(-2.69392879100006,2.2,2.94891416999998));
#306258=CARTESIAN_POINT('Ctrl Pts',(-2.69387588400006,12.2,2.94885452999999));
#306259=CARTESIAN_POINT('Ctrl Pts',(-2.69387588400006,5.2,2.94885452999999));
#306260=CARTESIAN_POINT('Ctrl Pts',(-2.69387588400006,2.2,2.94885452999999));
#306261=CARTESIAN_POINT('Ctrl Pts',(-2.69382776600006,12.2,2.94880042199999));
#306262=CARTESIAN_POINT('Ctrl Pts',(-2.69382776600006,5.2,2.94880042199999));
#306263=CARTESIAN_POINT('Ctrl Pts',(-2.69382776600006,2.2,2.94880042199999));
#306264=CARTESIAN_POINT('Ctrl Pts',(-2.69378446300006,12.2,2.94875184899999));
#306265=CARTESIAN_POINT('Ctrl Pts',(-2.69378446300006,5.2,2.94875184899999));
#306266=CARTESIAN_POINT('Ctrl Pts',(-2.69378446300006,2.2,2.94875184899999));
#306267=CARTESIAN_POINT('Ctrl Pts',(-2.69374600100006,12.2,2.94870880699998));
#306268=CARTESIAN_POINT('Ctrl Pts',(-2.69374600100006,5.2,2.94870880699998));
#306269=CARTESIAN_POINT('Ctrl Pts',(-2.69374600100006,2.2,2.94870880699998));
#306270=CARTESIAN_POINT('Ctrl Pts',(-2.69370879074423,12.2,2.94866728366678));
#306271=CARTESIAN_POINT('Ctrl Pts',(-2.69370879074423,5.2,2.94866728366678));
#306272=CARTESIAN_POINT('Ctrl Pts',(-2.69370879074423,2.2,2.94866728366678));
#306273=CARTESIAN_POINT('Ctrl Pts',(-2.69368329797707,12.2,2.94863895095595));
#306274=CARTESIAN_POINT('Ctrl Pts',(-2.69368329797707,5.2,2.94863895095595));
#306275=CARTESIAN_POINT('Ctrl Pts',(-2.69368329797707,2.2,2.94863895095595));
#306276=CARTESIAN_POINT('Ctrl Pts',(-2.69366646359,12.2,2.94862032138212));
#306277=CARTESIAN_POINT('Ctrl Pts',(-2.69366646359,5.2,2.94862032138212));
#306278=CARTESIAN_POINT('Ctrl Pts',(-2.69366646359,2.2,2.94862032138212));
#306279=CARTESIAN_POINT('Ctrl Pts',(-2.69365595548621,12.2,2.9486087420261));
#306280=CARTESIAN_POINT('Ctrl Pts',(-2.69365595548621,5.2,2.9486087420261));
#306281=CARTESIAN_POINT('Ctrl Pts',(-2.69365595548621,2.2,2.9486087420261));
#306282=CARTESIAN_POINT('Ctrl Pts',(-2.69364946500006,12.2,2.94860158799998));
#306283=CARTESIAN_POINT('Ctrl Pts',(-2.69364946500006,5.2,2.94860158799998));
#306284=CARTESIAN_POINT('Ctrl Pts',(-2.69364946500006,2.2,2.94860158799998));
#306285=CARTESIAN_POINT('',(-2.69364961400006,2.7,2.94860145299998));
#306286=CARTESIAN_POINT('',(-2.69364961400006,12.2,2.94860145299998));
#306287=CARTESIAN_POINT('Ctrl Pts',(-2.94378355400006,2.7,3.72781952199999));
#306288=CARTESIAN_POINT('Ctrl Pts',(-2.919025134039,2.7,3.47165304727227));
#306289=CARTESIAN_POINT('Ctrl Pts',(-2.86296672116152,2.7,3.28773125003828));
#306290=CARTESIAN_POINT('Ctrl Pts',(-2.75669794542552,2.7,3.02504202830561));
#306291=CARTESIAN_POINT('Ctrl Pts',(-2.70202149940583,2.7,2.95807419909088));
#306292=CARTESIAN_POINT('Ctrl Pts',(-2.69387506136249,2.7,2.94885330493632));
#306293=CARTESIAN_POINT('Ctrl Pts',(-2.69376302502467,2.7,2.94872675757333));
#306294=CARTESIAN_POINT('Ctrl Pts',(-2.69364946500006,2.7,2.94860158799998));
#306295=CARTESIAN_POINT('Origin',(-2.69361500300006,15.2,2.94856356499999));
#306296=CARTESIAN_POINT('',(-2.44494327000006,2.7,2.67635524699998));
#306297=CARTESIAN_POINT('',(-2.44494327000006,2.2,2.67635524699998));
#306298=CARTESIAN_POINT('',(-1.34680750196728,2.7,1.47428178207316));
#306299=CARTESIAN_POINT('Origin',(-5.66300478732629E-14,15.2,-1.77635683940025E-14));
#306300=CARTESIAN_POINT('',(-2.82878727700006,2.7,2.26684528399998));
#306301=CARTESIAN_POINT('',(-2.82878727700006,12.2,2.26684528399999));
#306302=CARTESIAN_POINT('Origin',(-5.66300478732629E-14,2.7,-1.92943768261394E-14));
#306303=CARTESIAN_POINT('Origin',(-5.66300478732629E-14,15.2,-1.77635683940025E-14));
#306304=CARTESIAN_POINT('',(-3.11652594000006,2.7,2.49742431399999));
#306305=CARTESIAN_POINT('',(-3.11652594000006,12.2,2.49742431399999));
#306306=CARTESIAN_POINT('',(-5.70184935903678E-14,2.7,-1.89830963177552E-14));
#306307=CARTESIAN_POINT('Ctrl Pts',(-3.11652602400006,12.2,2.49742420799999));
#306308=CARTESIAN_POINT('Ctrl Pts',(-3.11652602400006,5.2,2.49742420799999));
#306309=CARTESIAN_POINT('Ctrl Pts',(-3.11652602400006,2.2,2.49742420799999));
#306310=CARTESIAN_POINT('Ctrl Pts',(-3.11653137956376,12.2,2.49742846665313));
#306311=CARTESIAN_POINT('Ctrl Pts',(-3.11653137956376,5.2,2.49742846665313));
#306312=CARTESIAN_POINT('Ctrl Pts',(-3.11653137956376,2.2,2.49742846665313));
#306313=CARTESIAN_POINT('Ctrl Pts',(-3.11654173911751,12.2,2.49743670245955));
#306314=CARTESIAN_POINT('Ctrl Pts',(-3.11654173911751,5.2,2.49743670245955));
#306315=CARTESIAN_POINT('Ctrl Pts',(-3.11654173911751,2.2,2.49743670245955));
#306316=CARTESIAN_POINT('Ctrl Pts',(-3.1165571021189,12.2,2.49744892153641));
#306317=CARTESIAN_POINT('Ctrl Pts',(-3.1165571021189,5.19999999999999,2.49744892153641));
#306318=CARTESIAN_POINT('Ctrl Pts',(-3.1165571021189,2.2,2.49744892153641));
#306319=CARTESIAN_POINT('Ctrl Pts',(-3.1165774474675,12.2,2.49746508885391));
#306320=CARTESIAN_POINT('Ctrl Pts',(-3.1165774474675,5.2,2.49746508885391));
#306321=CARTESIAN_POINT('Ctrl Pts',(-3.1165774474675,2.2,2.49746508885391));
#306322=CARTESIAN_POINT('Ctrl Pts',(-3.11661304600006,12.2,2.49749314099999));
#306323=CARTESIAN_POINT('Ctrl Pts',(-3.11661304600006,5.2,2.49749314099999));
#306324=CARTESIAN_POINT('Ctrl Pts',(-3.11661304600006,2.2,2.49749314099999));
#306325=CARTESIAN_POINT('Ctrl Pts',(-3.11665264900005,12.2,2.49752425699998));
#306326=CARTESIAN_POINT('Ctrl Pts',(-3.11665264900005,5.2,2.49752425699998));
#306327=CARTESIAN_POINT('Ctrl Pts',(-3.11665264900005,2.2,2.49752425699998));
#306328=CARTESIAN_POINT('Ctrl Pts',(-3.11669808600006,12.2,2.49755985799998));
#306329=CARTESIAN_POINT('Ctrl Pts',(-3.11669808600006,5.2,2.49755985799998));
#306330=CARTESIAN_POINT('Ctrl Pts',(-3.11669808600006,2.2,2.49755985799998));
#306331=CARTESIAN_POINT('Ctrl Pts',(-3.11674935600006,12.2,2.49759992999999));
#306332=CARTESIAN_POINT('Ctrl Pts',(-3.11674935600006,5.2,2.49759992999999));
#306333=CARTESIAN_POINT('Ctrl Pts',(-3.11674935600006,2.2,2.49759992999999));
#306334=CARTESIAN_POINT('Ctrl Pts',(-3.11680646000006,12.2,2.49764445099999));
#306335=CARTESIAN_POINT('Ctrl Pts',(-3.11680646000006,5.2,2.49764445099999));
#306336=CARTESIAN_POINT('Ctrl Pts',(-3.11680646000006,2.2,2.49764445099999));
#306337=CARTESIAN_POINT('Ctrl Pts',(-3.11686939600006,12.2,2.49769339299998));
#306338=CARTESIAN_POINT('Ctrl Pts',(-3.11686939600006,5.2,2.49769339299998));
#306339=CARTESIAN_POINT('Ctrl Pts',(-3.11686939600006,2.2,2.49769339299998));
#306340=CARTESIAN_POINT('Ctrl Pts',(-3.11693816100005,12.2,2.49774672399998));
#306341=CARTESIAN_POINT('Ctrl Pts',(-3.11693816100005,5.2,2.49774672399998));
#306342=CARTESIAN_POINT('Ctrl Pts',(-3.11693816100005,2.2,2.49774672399998));
#306343=CARTESIAN_POINT('Ctrl Pts',(-3.11701275400006,12.2,2.49780440899999));
#306344=CARTESIAN_POINT('Ctrl Pts',(-3.11701275400006,5.2,2.49780440899999));
#306345=CARTESIAN_POINT('Ctrl Pts',(-3.11701275400006,2.2,2.49780440899999));
#306346=CARTESIAN_POINT('Ctrl Pts',(-3.11709317400005,12.2,2.49786642099998));
#306347=CARTESIAN_POINT('Ctrl Pts',(-3.11709317400005,5.2,2.49786642099998));
#306348=CARTESIAN_POINT('Ctrl Pts',(-3.11709317400005,2.2,2.49786642099998));
#306349=CARTESIAN_POINT('Ctrl Pts',(-3.11717941900006,12.2,2.49793273199998));
#306350=CARTESIAN_POINT('Ctrl Pts',(-3.11717941900006,5.2,2.49793273199998));
#306351=CARTESIAN_POINT('Ctrl Pts',(-3.11717941900006,2.2,2.49793273199998));
#306352=CARTESIAN_POINT('Ctrl Pts',(-3.11727148800006,12.2,2.49800331999998));
#306353=CARTESIAN_POINT('Ctrl Pts',(-3.11727148800006,5.2,2.49800331999998));
#306354=CARTESIAN_POINT('Ctrl Pts',(-3.11727148800006,2.2,2.49800331999998));
#306355=CARTESIAN_POINT('Ctrl Pts',(-3.11736937900006,12.2,2.49807816099998));
#306356=CARTESIAN_POINT('Ctrl Pts',(-3.11736937900006,5.2,2.49807816099998));
#306357=CARTESIAN_POINT('Ctrl Pts',(-3.11736937900006,2.2,2.49807816099998));
#306358=CARTESIAN_POINT('Ctrl Pts',(-3.11747309100005,12.2,2.49815723099999));
#306359=CARTESIAN_POINT('Ctrl Pts',(-3.11747309100005,5.2,2.49815723099999));
#306360=CARTESIAN_POINT('Ctrl Pts',(-3.11747309100005,2.2,2.49815723099999));
#306361=CARTESIAN_POINT('Ctrl Pts',(-3.11758262300006,12.2,2.49824050899999));
#306362=CARTESIAN_POINT('Ctrl Pts',(-3.11758262300006,5.2,2.49824050899999));
#306363=CARTESIAN_POINT('Ctrl Pts',(-3.11758262300006,2.2,2.49824050899999));
#306364=CARTESIAN_POINT('Ctrl Pts',(-3.11769797300005,12.2,2.49832796499999));
#306365=CARTESIAN_POINT('Ctrl Pts',(-3.11769797300005,5.2,2.49832796499999));
#306366=CARTESIAN_POINT('Ctrl Pts',(-3.11769797300005,2.2,2.49832796499999));
#306367=CARTESIAN_POINT('Ctrl Pts',(-3.11781913900006,12.2,2.49841957499999));
#306368=CARTESIAN_POINT('Ctrl Pts',(-3.11781913900006,5.2,2.49841957499999));
#306369=CARTESIAN_POINT('Ctrl Pts',(-3.11781913900006,2.2,2.49841957499999));
#306370=CARTESIAN_POINT('Ctrl Pts',(-3.11794612100006,12.2,2.49851531299999));
#306371=CARTESIAN_POINT('Ctrl Pts',(-3.11794612100006,5.2,2.49851531299999));
#306372=CARTESIAN_POINT('Ctrl Pts',(-3.11794612100006,2.2,2.49851531299999));
#306373=CARTESIAN_POINT('Ctrl Pts',(-3.11807891600006,12.2,2.49861515099998));
#306374=CARTESIAN_POINT('Ctrl Pts',(-3.11807891600006,5.2,2.49861515099998));
#306375=CARTESIAN_POINT('Ctrl Pts',(-3.11807891600006,2.2,2.49861515099998));
#306376=CARTESIAN_POINT('Ctrl Pts',(-3.11821752300005,12.2,2.49871906699998));
#306377=CARTESIAN_POINT('Ctrl Pts',(-3.11821752300005,5.2,2.49871906699998));
#306378=CARTESIAN_POINT('Ctrl Pts',(-3.11821752300005,2.2,2.49871906699998));
#306379=CARTESIAN_POINT('Ctrl Pts',(-3.11836194000006,12.2,2.49882703499999));
#306380=CARTESIAN_POINT('Ctrl Pts',(-3.11836194000006,5.2,2.49882703499999));
#306381=CARTESIAN_POINT('Ctrl Pts',(-3.11836194000006,2.2,2.49882703499999));
#306382=CARTESIAN_POINT('Ctrl Pts',(-3.11851216600005,12.2,2.49893903099998));
#306383=CARTESIAN_POINT('Ctrl Pts',(-3.11851216600005,5.2,2.49893903099998));
#306384=CARTESIAN_POINT('Ctrl Pts',(-3.11851216600005,2.2,2.49893903099998));
#306385=CARTESIAN_POINT('Ctrl Pts',(-3.11866819800006,12.2,2.49905503099999));
#306386=CARTESIAN_POINT('Ctrl Pts',(-3.11866819800006,5.2,2.49905503099999));
#306387=CARTESIAN_POINT('Ctrl Pts',(-3.11866819800006,2.2,2.49905503099999));
#306388=CARTESIAN_POINT('Ctrl Pts',(-3.11883003500005,12.2,2.49917501099999));
#306389=CARTESIAN_POINT('Ctrl Pts',(-3.11883003500005,5.2,2.49917501099999));
#306390=CARTESIAN_POINT('Ctrl Pts',(-3.11883003500005,2.2,2.49917501099999));
#306391=CARTESIAN_POINT('Ctrl Pts',(-3.11899767600006,12.2,2.49929894499999));
#306392=CARTESIAN_POINT('Ctrl Pts',(-3.11899767600006,5.2,2.49929894499999));
#306393=CARTESIAN_POINT('Ctrl Pts',(-3.11899767600006,2.2,2.49929894499999));
#306394=CARTESIAN_POINT('Ctrl Pts',(-3.11917111900006,12.2,2.49942681099999));
#306395=CARTESIAN_POINT('Ctrl Pts',(-3.11917111900006,5.2,2.49942681099999));
#306396=CARTESIAN_POINT('Ctrl Pts',(-3.11917111900006,2.2,2.49942681099999));
#306397=CARTESIAN_POINT('Ctrl Pts',(-3.11935036300006,12.2,2.49955858199999));
#306398=CARTESIAN_POINT('Ctrl Pts',(-3.11935036300006,5.2,2.49955858199999));
#306399=CARTESIAN_POINT('Ctrl Pts',(-3.11935036300006,2.2,2.49955858199999));
#306400=CARTESIAN_POINT('Ctrl Pts',(-3.11953540400005,12.2,2.49969423399998));
#306401=CARTESIAN_POINT('Ctrl Pts',(-3.11953540400005,5.2,2.49969423399998));
#306402=CARTESIAN_POINT('Ctrl Pts',(-3.11953540400005,2.2,2.49969423399998));
#306403=CARTESIAN_POINT('Ctrl Pts',(-3.11972624100005,12.2,2.49983374399999));
#306404=CARTESIAN_POINT('Ctrl Pts',(-3.11972624100005,5.2,2.49983374399999));
#306405=CARTESIAN_POINT('Ctrl Pts',(-3.11972624100005,2.2,2.49983374399999));
#306406=CARTESIAN_POINT('Ctrl Pts',(-3.11992287400006,12.2,2.49997708699999));
#306407=CARTESIAN_POINT('Ctrl Pts',(-3.11992287400006,5.2,2.49997708699999));
#306408=CARTESIAN_POINT('Ctrl Pts',(-3.11992287400006,2.2,2.49997708699999));
#306409=CARTESIAN_POINT('Ctrl Pts',(-3.12012529900006,12.2,2.50012423999999));
#306410=CARTESIAN_POINT('Ctrl Pts',(-3.12012529900006,5.2,2.50012423999999));
#306411=CARTESIAN_POINT('Ctrl Pts',(-3.12012529900006,2.2,2.50012423999999));
#306412=CARTESIAN_POINT('Ctrl Pts',(-3.12033351600005,12.2,2.50027517899999));
#306413=CARTESIAN_POINT('Ctrl Pts',(-3.12033351600005,5.2,2.50027517899999));
#306414=CARTESIAN_POINT('Ctrl Pts',(-3.12033351600005,2.2,2.50027517899999));
#306415=CARTESIAN_POINT('Ctrl Pts',(-3.12054752100006,12.2,2.50042987999999));
#306416=CARTESIAN_POINT('Ctrl Pts',(-3.12054752100006,5.2,2.50042987999999));
#306417=CARTESIAN_POINT('Ctrl Pts',(-3.12054752100006,2.2,2.50042987999999));
#306418=CARTESIAN_POINT('Ctrl Pts',(-3.12076731400006,12.2,2.50058831899998));
#306419=CARTESIAN_POINT('Ctrl Pts',(-3.12076731400006,5.2,2.50058831899998));
#306420=CARTESIAN_POINT('Ctrl Pts',(-3.12076731400006,2.2,2.50058831899998));
#306421=CARTESIAN_POINT('Ctrl Pts',(-3.12099289300006,12.2,2.50075047399999));
#306422=CARTESIAN_POINT('Ctrl Pts',(-3.12099289300006,5.2,2.50075047399999));
#306423=CARTESIAN_POINT('Ctrl Pts',(-3.12099289300006,2.2,2.50075047399999));
#306424=CARTESIAN_POINT('Ctrl Pts',(-3.12122425400006,12.2,2.50091631999998));
#306425=CARTESIAN_POINT('Ctrl Pts',(-3.12122425400006,5.2,2.50091631999998));
#306426=CARTESIAN_POINT('Ctrl Pts',(-3.12122425400006,2.2,2.50091631999998));
#306427=CARTESIAN_POINT('Ctrl Pts',(-3.12146139800006,12.2,2.50108583399999));
#306428=CARTESIAN_POINT('Ctrl Pts',(-3.12146139800006,5.2,2.50108583399999));
#306429=CARTESIAN_POINT('Ctrl Pts',(-3.12146139800006,2.2,2.50108583399999));
#306430=CARTESIAN_POINT('Ctrl Pts',(-3.12170432100006,12.2,2.50125899199999));
#306431=CARTESIAN_POINT('Ctrl Pts',(-3.12170432100006,5.2,2.50125899199999));
#306432=CARTESIAN_POINT('Ctrl Pts',(-3.12170432100006,2.2,2.50125899199999));
#306433=CARTESIAN_POINT('Ctrl Pts',(-3.12195302200006,12.2,2.50143577099998));
#306434=CARTESIAN_POINT('Ctrl Pts',(-3.12195302200006,5.2,2.50143577099998));
#306435=CARTESIAN_POINT('Ctrl Pts',(-3.12195302200006,2.2,2.50143577099998));
#306436=CARTESIAN_POINT('Ctrl Pts',(-3.12220749700006,12.2,2.50161614799998));
#306437=CARTESIAN_POINT('Ctrl Pts',(-3.12220749700006,5.2,2.50161614799998));
#306438=CARTESIAN_POINT('Ctrl Pts',(-3.12220749700006,2.2,2.50161614799998));
#306439=CARTESIAN_POINT('Ctrl Pts',(-3.12246774800006,12.2,2.50180010099999));
#306440=CARTESIAN_POINT('Ctrl Pts',(-3.12246774800006,5.2,2.50180010099999));
#306441=CARTESIAN_POINT('Ctrl Pts',(-3.12246774800006,2.2,2.50180010099999));
#306442=CARTESIAN_POINT('Ctrl Pts',(-3.12273376900006,12.2,2.50198760499998));
#306443=CARTESIAN_POINT('Ctrl Pts',(-3.12273376900006,5.2,2.50198760499998));
#306444=CARTESIAN_POINT('Ctrl Pts',(-3.12273376900006,2.2,2.50198760499998));
#306445=CARTESIAN_POINT('Ctrl Pts',(-3.12300556000006,12.2,2.50217863899999));
#306446=CARTESIAN_POINT('Ctrl Pts',(-3.12300556000006,5.2,2.50217863899999));
#306447=CARTESIAN_POINT('Ctrl Pts',(-3.12300556000006,2.2,2.50217863899999));
#306448=CARTESIAN_POINT('Ctrl Pts',(-3.12328311900006,12.2,2.50237317899998));
#306449=CARTESIAN_POINT('Ctrl Pts',(-3.12328311900006,5.2,2.50237317899998));
#306450=CARTESIAN_POINT('Ctrl Pts',(-3.12328311900006,2.2,2.50237317899998));
#306451=CARTESIAN_POINT('Ctrl Pts',(-3.12356644200006,12.2,2.50257120199999));
#306452=CARTESIAN_POINT('Ctrl Pts',(-3.12356644200006,5.2,2.50257120199999));
#306453=CARTESIAN_POINT('Ctrl Pts',(-3.12356644200006,2.2,2.50257120199999));
#306454=CARTESIAN_POINT('Ctrl Pts',(-3.12385552900006,12.2,2.50277268499998));
#306455=CARTESIAN_POINT('Ctrl Pts',(-3.12385552900006,5.2,2.50277268499998));
#306456=CARTESIAN_POINT('Ctrl Pts',(-3.12385552900006,2.2,2.50277268499998));
#306457=CARTESIAN_POINT('Ctrl Pts',(-3.12415037700006,12.2,2.50297760799998));
#306458=CARTESIAN_POINT('Ctrl Pts',(-3.12415037700006,5.2,2.50297760799998));
#306459=CARTESIAN_POINT('Ctrl Pts',(-3.12415037700006,2.2,2.50297760799998));
#306460=CARTESIAN_POINT('Ctrl Pts',(-3.12445098400006,12.2,2.50318594399998));
#306461=CARTESIAN_POINT('Ctrl Pts',(-3.12445098400006,5.2,2.50318594399998));
#306462=CARTESIAN_POINT('Ctrl Pts',(-3.12445098400006,2.2,2.50318594399998));
#306463=CARTESIAN_POINT('Ctrl Pts',(-3.12475734800006,12.2,2.50339767399999));
#306464=CARTESIAN_POINT('Ctrl Pts',(-3.12475734800006,5.2,2.50339767399999));
#306465=CARTESIAN_POINT('Ctrl Pts',(-3.12475734800006,2.2,2.50339767399999));
#306466=CARTESIAN_POINT('Ctrl Pts',(-3.12506946600006,12.2,2.50361277599998));
#306467=CARTESIAN_POINT('Ctrl Pts',(-3.12506946600006,5.2,2.50361277599998));
#306468=CARTESIAN_POINT('Ctrl Pts',(-3.12506946600006,2.2,2.50361277599998));
#306469=CARTESIAN_POINT('Ctrl Pts',(-3.12538733700006,12.2,2.50383122499999));
#306470=CARTESIAN_POINT('Ctrl Pts',(-3.12538733700006,5.2,2.50383122499999));
#306471=CARTESIAN_POINT('Ctrl Pts',(-3.12538733700006,2.2,2.50383122499999));
#306472=CARTESIAN_POINT('Ctrl Pts',(-3.12571095700005,12.2,2.50405299999999));
#306473=CARTESIAN_POINT('Ctrl Pts',(-3.12571095700005,5.2,2.50405299999999));
#306474=CARTESIAN_POINT('Ctrl Pts',(-3.12571095700005,2.2,2.50405299999999));
#306475=CARTESIAN_POINT('Ctrl Pts',(-3.12604032600006,12.2,2.50427807899998));
#306476=CARTESIAN_POINT('Ctrl Pts',(-3.12604032600006,5.2,2.50427807899998));
#306477=CARTESIAN_POINT('Ctrl Pts',(-3.12604032600006,2.2,2.50427807899998));
#306478=CARTESIAN_POINT('Ctrl Pts',(-3.12637544100005,12.2,2.50450643999999));
#306479=CARTESIAN_POINT('Ctrl Pts',(-3.12637544100005,5.2,2.50450643999999));
#306480=CARTESIAN_POINT('Ctrl Pts',(-3.12637544100005,2.2,2.50450643999999));
#306481=CARTESIAN_POINT('Ctrl Pts',(-3.12671629800006,12.2,2.50473806099999));
#306482=CARTESIAN_POINT('Ctrl Pts',(-3.12671629800006,5.2,2.50473806099999));
#306483=CARTESIAN_POINT('Ctrl Pts',(-3.12671629800006,2.2,2.50473806099999));
#306484=CARTESIAN_POINT('Ctrl Pts',(-3.12706289700006,12.2,2.50497291999999));
#306485=CARTESIAN_POINT('Ctrl Pts',(-3.12706289700006,5.2,2.50497291999999));
#306486=CARTESIAN_POINT('Ctrl Pts',(-3.12706289700006,2.2,2.50497291999999));
#306487=CARTESIAN_POINT('Ctrl Pts',(-3.12741523500006,12.2,2.50521099399998));
#306488=CARTESIAN_POINT('Ctrl Pts',(-3.12741523500006,5.2,2.50521099399998));
#306489=CARTESIAN_POINT('Ctrl Pts',(-3.12741523500006,2.2,2.50521099399998));
#306490=CARTESIAN_POINT('Ctrl Pts',(-3.12777330900006,12.2,2.50545226299998));
#306491=CARTESIAN_POINT('Ctrl Pts',(-3.12777330900006,5.2,2.50545226299998));
#306492=CARTESIAN_POINT('Ctrl Pts',(-3.12777330900006,2.2,2.50545226299998));
#306493=CARTESIAN_POINT('Ctrl Pts',(-3.12813711700006,12.2,2.50569670399998));
#306494=CARTESIAN_POINT('Ctrl Pts',(-3.12813711700006,5.2,2.50569670399998));
#306495=CARTESIAN_POINT('Ctrl Pts',(-3.12813711700006,2.2,2.50569670399998));
#306496=CARTESIAN_POINT('Ctrl Pts',(-3.12850665800006,12.2,2.50594429599998));
#306497=CARTESIAN_POINT('Ctrl Pts',(-3.12850665800006,5.2,2.50594429599998));
#306498=CARTESIAN_POINT('Ctrl Pts',(-3.12850665800006,2.2,2.50594429599998));
#306499=CARTESIAN_POINT('Ctrl Pts',(-3.12888192700005,12.2,2.50619501699998));
#306500=CARTESIAN_POINT('Ctrl Pts',(-3.12888192700005,5.2,2.50619501699998));
#306501=CARTESIAN_POINT('Ctrl Pts',(-3.12888192700005,2.2,2.50619501699998));
#306502=CARTESIAN_POINT('Ctrl Pts',(-3.12926292300005,12.2,2.50644884599998));
#306503=CARTESIAN_POINT('Ctrl Pts',(-3.12926292300005,5.2,2.50644884599998));
#306504=CARTESIAN_POINT('Ctrl Pts',(-3.12926292300005,2.2,2.50644884599998));
#306505=CARTESIAN_POINT('Ctrl Pts',(-3.12964964300006,12.2,2.50670576099999));
#306506=CARTESIAN_POINT('Ctrl Pts',(-3.12964964300006,5.2,2.50670576099999));
#306507=CARTESIAN_POINT('Ctrl Pts',(-3.12964964300006,2.2,2.50670576099999));
#306508=CARTESIAN_POINT('Ctrl Pts',(-3.13004208700006,12.2,2.50696574099998));
#306509=CARTESIAN_POINT('Ctrl Pts',(-3.13004208700006,5.2,2.50696574099998));
#306510=CARTESIAN_POINT('Ctrl Pts',(-3.13004208700006,2.2,2.50696574099998));
#306511=CARTESIAN_POINT('Ctrl Pts',(-3.13044025000006,12.2,2.50722876399998));
#306512=CARTESIAN_POINT('Ctrl Pts',(-3.13044025000006,5.2,2.50722876399998));
#306513=CARTESIAN_POINT('Ctrl Pts',(-3.13044025000006,2.2,2.50722876399998));
#306514=CARTESIAN_POINT('Ctrl Pts',(-3.13084413000006,12.2,2.50749480999998));
#306515=CARTESIAN_POINT('Ctrl Pts',(-3.13084413000006,5.2,2.50749480999998));
#306516=CARTESIAN_POINT('Ctrl Pts',(-3.13084413000006,2.2,2.50749480999998));
#306517=CARTESIAN_POINT('Ctrl Pts',(-3.13125372400005,12.2,2.50776385699999));
#306518=CARTESIAN_POINT('Ctrl Pts',(-3.13125372400005,5.2,2.50776385699999));
#306519=CARTESIAN_POINT('Ctrl Pts',(-3.13125372400005,2.2,2.50776385699999));
#306520=CARTESIAN_POINT('Ctrl Pts',(-3.13166903000006,12.2,2.50803588399998));
#306521=CARTESIAN_POINT('Ctrl Pts',(-3.13166903000006,5.2,2.50803588399998));
#306522=CARTESIAN_POINT('Ctrl Pts',(-3.13166903000006,2.2,2.50803588399998));
#306523=CARTESIAN_POINT('Ctrl Pts',(-3.13209004700005,12.2,2.50831087099999));
#306524=CARTESIAN_POINT('Ctrl Pts',(-3.13209004700005,5.2,2.50831087099999));
#306525=CARTESIAN_POINT('Ctrl Pts',(-3.13209004700005,2.2,2.50831087099999));
#306526=CARTESIAN_POINT('Ctrl Pts',(-3.13251677000005,12.2,2.50858879499999));
#306527=CARTESIAN_POINT('Ctrl Pts',(-3.13251677000005,5.2,2.50858879499999));
#306528=CARTESIAN_POINT('Ctrl Pts',(-3.13251677000005,2.2,2.50858879499999));
#306529=CARTESIAN_POINT('Ctrl Pts',(-3.13294919800006,12.2,2.50886963599999));
#306530=CARTESIAN_POINT('Ctrl Pts',(-3.13294919800006,5.2,2.50886963599999));
#306531=CARTESIAN_POINT('Ctrl Pts',(-3.13294919800006,2.2,2.50886963599999));
#306532=CARTESIAN_POINT('Ctrl Pts',(-3.13338732900006,12.2,2.50915337399999));
#306533=CARTESIAN_POINT('Ctrl Pts',(-3.13338732900006,5.2,2.50915337399999));
#306534=CARTESIAN_POINT('Ctrl Pts',(-3.13338732900006,2.2,2.50915337399999));
#306535=CARTESIAN_POINT('Ctrl Pts',(-3.13383115700006,12.2,2.50943998799999));
#306536=CARTESIAN_POINT('Ctrl Pts',(-3.13383115700006,5.2,2.50943998799999));
#306537=CARTESIAN_POINT('Ctrl Pts',(-3.13383115700006,2.2,2.50943998799999));
#306538=CARTESIAN_POINT('Ctrl Pts',(-3.13428068400006,12.2,2.50972945699999));
#306539=CARTESIAN_POINT('Ctrl Pts',(-3.13428068400006,5.2,2.50972945699999));
#306540=CARTESIAN_POINT('Ctrl Pts',(-3.13428068400006,2.2,2.50972945699999));
#306541=CARTESIAN_POINT('Ctrl Pts',(-3.13473590500006,12.2,2.51002175999999));
#306542=CARTESIAN_POINT('Ctrl Pts',(-3.13473590500006,5.2,2.51002175999999));
#306543=CARTESIAN_POINT('Ctrl Pts',(-3.13473590500006,2.2,2.51002175999999));
#306544=CARTESIAN_POINT('Ctrl Pts',(-3.13519681700006,12.2,2.51031687599998));
#306545=CARTESIAN_POINT('Ctrl Pts',(-3.13519681700006,5.2,2.51031687599998));
#306546=CARTESIAN_POINT('Ctrl Pts',(-3.13519681700006,2.2,2.51031687599998));
#306547=CARTESIAN_POINT('Ctrl Pts',(-3.13566341800006,12.2,2.51061478699998));
#306548=CARTESIAN_POINT('Ctrl Pts',(-3.13566341800006,5.2,2.51061478699998));
#306549=CARTESIAN_POINT('Ctrl Pts',(-3.13566341800006,2.2,2.51061478699998));
#306550=CARTESIAN_POINT('Ctrl Pts',(-3.13613570600006,12.2,2.51091546999999));
#306551=CARTESIAN_POINT('Ctrl Pts',(-3.13613570600006,5.2,2.51091546999999));
#306552=CARTESIAN_POINT('Ctrl Pts',(-3.13613570600006,2.2,2.51091546999999));
#306553=CARTESIAN_POINT('Ctrl Pts',(-3.13661367700006,12.2,2.51121890599999));
#306554=CARTESIAN_POINT('Ctrl Pts',(-3.13661367700006,5.2,2.51121890599999));
#306555=CARTESIAN_POINT('Ctrl Pts',(-3.13661367700006,2.2,2.51121890599999));
#306556=CARTESIAN_POINT('Ctrl Pts',(-3.13709732900006,12.2,2.51152507399999));
#306557=CARTESIAN_POINT('Ctrl Pts',(-3.13709732900006,5.2,2.51152507399999));
#306558=CARTESIAN_POINT('Ctrl Pts',(-3.13709732900006,2.2,2.51152507399999));
#306559=CARTESIAN_POINT('Ctrl Pts',(-3.13758665900005,12.2,2.51183395499999));
#306560=CARTESIAN_POINT('Ctrl Pts',(-3.13758665900005,5.2,2.51183395499999));
#306561=CARTESIAN_POINT('Ctrl Pts',(-3.13758665900005,2.2,2.51183395499999));
#306562=CARTESIAN_POINT('Ctrl Pts',(-3.13808166500006,12.2,2.51214552699999));
#306563=CARTESIAN_POINT('Ctrl Pts',(-3.13808166500006,5.2,2.51214552699999));
#306564=CARTESIAN_POINT('Ctrl Pts',(-3.13808166500006,2.2,2.51214552699999));
#306565=CARTESIAN_POINT('Ctrl Pts',(-3.13858234300006,12.2,2.51245977099998));
#306566=CARTESIAN_POINT('Ctrl Pts',(-3.13858234300006,5.2,2.51245977099998));
#306567=CARTESIAN_POINT('Ctrl Pts',(-3.13858234300006,2.2,2.51245977099998));
#306568=CARTESIAN_POINT('Ctrl Pts',(-3.13908869200006,12.2,2.51277666599999));
#306569=CARTESIAN_POINT('Ctrl Pts',(-3.13908869200006,5.2,2.51277666599999));
#306570=CARTESIAN_POINT('Ctrl Pts',(-3.13908869200006,2.2,2.51277666599999));
#306571=CARTESIAN_POINT('Ctrl Pts',(-3.13960070700006,12.2,2.51309619499998));
#306572=CARTESIAN_POINT('Ctrl Pts',(-3.13960070700006,5.2,2.51309619499998));
#306573=CARTESIAN_POINT('Ctrl Pts',(-3.13960070700006,2.2,2.51309619499998));
#306574=CARTESIAN_POINT('Ctrl Pts',(-3.14011838700006,12.2,2.51341833399999));
#306575=CARTESIAN_POINT('Ctrl Pts',(-3.14011838700006,5.2,2.51341833399999));
#306576=CARTESIAN_POINT('Ctrl Pts',(-3.14011838700006,2.2,2.51341833399999));
#306577=CARTESIAN_POINT('Ctrl Pts',(-3.14064172800005,12.2,2.51374306599998));
#306578=CARTESIAN_POINT('Ctrl Pts',(-3.14064172800005,5.2,2.51374306599998));
#306579=CARTESIAN_POINT('Ctrl Pts',(-3.14064172800005,2.2,2.51374306599998));
#306580=CARTESIAN_POINT('Ctrl Pts',(-3.14117072900005,12.2,2.51407036999999));
#306581=CARTESIAN_POINT('Ctrl Pts',(-3.14117072900005,5.2,2.51407036999999));
#306582=CARTESIAN_POINT('Ctrl Pts',(-3.14117072900005,2.2,2.51407036999999));
#306583=CARTESIAN_POINT('Ctrl Pts',(-3.14170538500006,12.2,2.51440022599999));
#306584=CARTESIAN_POINT('Ctrl Pts',(-3.14170538500006,5.2,2.51440022599999));
#306585=CARTESIAN_POINT('Ctrl Pts',(-3.14170538500006,2.2,2.51440022599999));
#306586=CARTESIAN_POINT('Ctrl Pts',(-3.14224569400006,12.2,2.51473261599998));
#306587=CARTESIAN_POINT('Ctrl Pts',(-3.14224569400006,5.2,2.51473261599998));
#306588=CARTESIAN_POINT('Ctrl Pts',(-3.14224569400006,2.2,2.51473261599998));
#306589=CARTESIAN_POINT('Ctrl Pts',(-3.14279165400006,12.2,2.51506751899999));
#306590=CARTESIAN_POINT('Ctrl Pts',(-3.14279165400006,5.2,2.51506751899999));
#306591=CARTESIAN_POINT('Ctrl Pts',(-3.14279165400006,2.2,2.51506751899999));
#306592=CARTESIAN_POINT('Ctrl Pts',(-3.14334326000006,12.2,2.51540491499998));
#306593=CARTESIAN_POINT('Ctrl Pts',(-3.14334326000006,5.2,2.51540491499998));
#306594=CARTESIAN_POINT('Ctrl Pts',(-3.14334326000006,2.2,2.51540491499998));
#306595=CARTESIAN_POINT('Ctrl Pts',(-3.14390051100006,12.2,2.51574478699998));
#306596=CARTESIAN_POINT('Ctrl Pts',(-3.14390051100006,5.2,2.51574478699998));
#306597=CARTESIAN_POINT('Ctrl Pts',(-3.14390051100006,2.2,2.51574478699998));
#306598=CARTESIAN_POINT('Ctrl Pts',(-3.14446340400006,12.2,2.51608711299999));
#306599=CARTESIAN_POINT('Ctrl Pts',(-3.14446340400006,5.2,2.51608711299999));
#306600=CARTESIAN_POINT('Ctrl Pts',(-3.14446340400006,2.2,2.51608711299999));
#306601=CARTESIAN_POINT('Ctrl Pts',(-3.14503193500005,12.2,2.51643187499998));
#306602=CARTESIAN_POINT('Ctrl Pts',(-3.14503193500005,5.2,2.51643187499998));
#306603=CARTESIAN_POINT('Ctrl Pts',(-3.14503193500005,2.2,2.51643187499998));
#306604=CARTESIAN_POINT('Ctrl Pts',(-3.14560610200005,12.2,2.51677905199998));
#306605=CARTESIAN_POINT('Ctrl Pts',(-3.14560610200005,5.2,2.51677905199998));
#306606=CARTESIAN_POINT('Ctrl Pts',(-3.14560610200005,2.2,2.51677905199998));
#306607=CARTESIAN_POINT('Ctrl Pts',(-3.14618590100006,12.2,2.51712862799998));
#306608=CARTESIAN_POINT('Ctrl Pts',(-3.14618590100006,5.2,2.51712862799998));
#306609=CARTESIAN_POINT('Ctrl Pts',(-3.14618590100006,2.2,2.51712862799998));
#306610=CARTESIAN_POINT('Ctrl Pts',(-3.14677133100006,12.2,2.51748058099999));
#306611=CARTESIAN_POINT('Ctrl Pts',(-3.14677133100006,5.2,2.51748058099999));
#306612=CARTESIAN_POINT('Ctrl Pts',(-3.14677133100006,2.2,2.51748058099999));
#306613=CARTESIAN_POINT('Ctrl Pts',(-3.14736238700006,12.2,2.51783489199998));
#306614=CARTESIAN_POINT('Ctrl Pts',(-3.14736238700006,5.2,2.51783489199998));
#306615=CARTESIAN_POINT('Ctrl Pts',(-3.14736238700006,2.2,2.51783489199998));
#306616=CARTESIAN_POINT('Ctrl Pts',(-3.14795906700006,12.2,2.51819154399998));
#306617=CARTESIAN_POINT('Ctrl Pts',(-3.14795906700006,5.2,2.51819154399998));
#306618=CARTESIAN_POINT('Ctrl Pts',(-3.14795906700006,2.2,2.51819154399998));
#306619=CARTESIAN_POINT('Ctrl Pts',(-3.14856136800006,12.2,2.51855051599998));
#306620=CARTESIAN_POINT('Ctrl Pts',(-3.14856136800006,5.2,2.51855051599998));
#306621=CARTESIAN_POINT('Ctrl Pts',(-3.14856136800006,2.2,2.51855051599998));
#306622=CARTESIAN_POINT('Ctrl Pts',(-3.14916928600006,12.2,2.51891178999998));
#306623=CARTESIAN_POINT('Ctrl Pts',(-3.14916928600006,5.2,2.51891178999998));
#306624=CARTESIAN_POINT('Ctrl Pts',(-3.14916928600006,2.2,2.51891178999998));
#306625=CARTESIAN_POINT('Ctrl Pts',(-3.14978281900005,12.2,2.51927534799999));
#306626=CARTESIAN_POINT('Ctrl Pts',(-3.14978281900005,5.2,2.51927534799999));
#306627=CARTESIAN_POINT('Ctrl Pts',(-3.14978281900005,2.2,2.51927534799999));
#306628=CARTESIAN_POINT('Ctrl Pts',(-3.15040196400005,12.2,2.51964116899998));
#306629=CARTESIAN_POINT('Ctrl Pts',(-3.15040196400005,5.2,2.51964116899998));
#306630=CARTESIAN_POINT('Ctrl Pts',(-3.15040196400005,2.2,2.51964116899998));
#306631=CARTESIAN_POINT('Ctrl Pts',(-3.15102671700005,12.2,2.52000923599999));
#306632=CARTESIAN_POINT('Ctrl Pts',(-3.15102671700005,5.2,2.52000923599999));
#306633=CARTESIAN_POINT('Ctrl Pts',(-3.15102671700005,2.2,2.52000923599999));
#306634=CARTESIAN_POINT('Ctrl Pts',(-3.15165707500006,12.2,2.52037952899999));
#306635=CARTESIAN_POINT('Ctrl Pts',(-3.15165707500006,5.2,2.52037952899999));
#306636=CARTESIAN_POINT('Ctrl Pts',(-3.15165707500006,2.2,2.52037952899999));
#306637=CARTESIAN_POINT('Ctrl Pts',(-3.15229303600006,12.2,2.52075202999999));
#306638=CARTESIAN_POINT('Ctrl Pts',(-3.15229303600006,5.2,2.52075202999999));
#306639=CARTESIAN_POINT('Ctrl Pts',(-3.15229303600006,2.2,2.52075202999999));
#306640=CARTESIAN_POINT('Ctrl Pts',(-3.15293459600006,12.2,2.52112671999999));
#306641=CARTESIAN_POINT('Ctrl Pts',(-3.15293459600006,5.2,2.52112671999999));
#306642=CARTESIAN_POINT('Ctrl Pts',(-3.15293459600006,2.2,2.52112671999999));
#306643=CARTESIAN_POINT('Ctrl Pts',(-3.15358175200006,12.2,2.52150358099998));
#306644=CARTESIAN_POINT('Ctrl Pts',(-3.15358175200006,5.2,2.52150358099998));
#306645=CARTESIAN_POINT('Ctrl Pts',(-3.15358175200006,2.2,2.52150358099998));
#306646=CARTESIAN_POINT('Ctrl Pts',(-3.15423450100006,12.2,2.52188259499999));
#306647=CARTESIAN_POINT('Ctrl Pts',(-3.15423450100006,5.2,2.52188259499999));
#306648=CARTESIAN_POINT('Ctrl Pts',(-3.15423450100006,2.2,2.52188259499999));
#306649=CARTESIAN_POINT('Ctrl Pts',(-3.15489284100006,12.2,2.52226374299998));
#306650=CARTESIAN_POINT('Ctrl Pts',(-3.15489284100006,5.2,2.52226374299998));
#306651=CARTESIAN_POINT('Ctrl Pts',(-3.15489284100006,2.2,2.52226374299998));
#306652=CARTESIAN_POINT('Ctrl Pts',(-3.15555676600006,12.2,2.52264700699998));
#306653=CARTESIAN_POINT('Ctrl Pts',(-3.15555676600006,5.2,2.52264700699998));
#306654=CARTESIAN_POINT('Ctrl Pts',(-3.15555676600006,2.2,2.52264700699998));
#306655=CARTESIAN_POINT('Ctrl Pts',(-3.15622627500006,12.2,2.52303236699999));
#306656=CARTESIAN_POINT('Ctrl Pts',(-3.15622627500006,5.2,2.52303236699999));
#306657=CARTESIAN_POINT('Ctrl Pts',(-3.15622627500006,2.2,2.52303236699999));
#306658=CARTESIAN_POINT('Ctrl Pts',(-3.15690136500006,12.2,2.52341980599999));
#306659=CARTESIAN_POINT('Ctrl Pts',(-3.15690136500006,5.2,2.52341980599999));
#306660=CARTESIAN_POINT('Ctrl Pts',(-3.15690136500006,2.2,2.52341980599999));
#306661=CARTESIAN_POINT('Ctrl Pts',(-3.15758203100006,12.2,2.52380930699999));
#306662=CARTESIAN_POINT('Ctrl Pts',(-3.15758203100006,5.2,2.52380930699999));
#306663=CARTESIAN_POINT('Ctrl Pts',(-3.15758203100006,2.2,2.52380930699999));
#306664=CARTESIAN_POINT('Ctrl Pts',(-3.15826827100006,12.2,2.52420084999999));
#306665=CARTESIAN_POINT('Ctrl Pts',(-3.15826827100006,5.2,2.52420084999999));
#306666=CARTESIAN_POINT('Ctrl Pts',(-3.15826827100006,2.2,2.52420084999999));
#306667=CARTESIAN_POINT('Ctrl Pts',(-3.15896008200005,12.2,2.52459441699998));
#306668=CARTESIAN_POINT('Ctrl Pts',(-3.15896008200005,5.2,2.52459441699998));
#306669=CARTESIAN_POINT('Ctrl Pts',(-3.15896008200005,2.2,2.52459441699998));
#306670=CARTESIAN_POINT('Ctrl Pts',(-3.15965746100006,12.2,2.52498999199998));
#306671=CARTESIAN_POINT('Ctrl Pts',(-3.15965746100006,5.2,2.52498999199998));
#306672=CARTESIAN_POINT('Ctrl Pts',(-3.15965746100006,2.2,2.52498999199998));
#306673=CARTESIAN_POINT('Ctrl Pts',(-3.16036040300005,12.2,2.52538755399998));
#306674=CARTESIAN_POINT('Ctrl Pts',(-3.16036040300005,5.2,2.52538755399998));
#306675=CARTESIAN_POINT('Ctrl Pts',(-3.16036040300005,2.2,2.52538755399998));
#306676=CARTESIAN_POINT('Ctrl Pts',(-3.16106890600006,12.2,2.52578708699998));
#306677=CARTESIAN_POINT('Ctrl Pts',(-3.16106890600006,5.2,2.52578708699998));
#306678=CARTESIAN_POINT('Ctrl Pts',(-3.16106890600006,2.2,2.52578708699998));
#306679=CARTESIAN_POINT('Ctrl Pts',(-3.16178296600006,12.2,2.52618857299999));
#306680=CARTESIAN_POINT('Ctrl Pts',(-3.16178296600006,5.2,2.52618857299999));
#306681=CARTESIAN_POINT('Ctrl Pts',(-3.16178296600006,2.2,2.52618857299999));
#306682=CARTESIAN_POINT('Ctrl Pts',(-3.16250258100006,12.2,2.52659199399999));
#306683=CARTESIAN_POINT('Ctrl Pts',(-3.16250258100006,5.2,2.52659199399999));
#306684=CARTESIAN_POINT('Ctrl Pts',(-3.16250258100006,2.2,2.52659199399999));
#306685=CARTESIAN_POINT('Ctrl Pts',(-3.16322774700006,12.2,2.52699733099998));
#306686=CARTESIAN_POINT('Ctrl Pts',(-3.16322774700006,5.2,2.52699733099998));
#306687=CARTESIAN_POINT('Ctrl Pts',(-3.16322774700006,2.2,2.52699733099998));
#306688=CARTESIAN_POINT('Ctrl Pts',(-3.16395846100006,12.2,2.52740456899998));
#306689=CARTESIAN_POINT('Ctrl Pts',(-3.16395846100006,5.2,2.52740456899998));
#306690=CARTESIAN_POINT('Ctrl Pts',(-3.16395846100006,2.2,2.52740456899998));
#306691=CARTESIAN_POINT('Ctrl Pts',(-3.16469471800006,12.2,2.52781368799998));
#306692=CARTESIAN_POINT('Ctrl Pts',(-3.16469471800006,5.2,2.52781368799998));
#306693=CARTESIAN_POINT('Ctrl Pts',(-3.16469471800006,2.2,2.52781368799998));
#306694=CARTESIAN_POINT('Ctrl Pts',(-3.16543651700006,12.2,2.52822466999999));
#306695=CARTESIAN_POINT('Ctrl Pts',(-3.16543651700006,5.2,2.52822466999999));
#306696=CARTESIAN_POINT('Ctrl Pts',(-3.16543651700006,2.2,2.52822466999999));
#306697=CARTESIAN_POINT('Ctrl Pts',(-3.16618385300006,12.2,2.52863749999998));
#306698=CARTESIAN_POINT('Ctrl Pts',(-3.16618385300006,5.2,2.52863749999998));
#306699=CARTESIAN_POINT('Ctrl Pts',(-3.16618385300006,2.2,2.52863749999998));
#306700=CARTESIAN_POINT('Ctrl Pts',(-3.16693672400006,12.2,2.52905215799998));
#306701=CARTESIAN_POINT('Ctrl Pts',(-3.16693672400006,5.2,2.52905215799998));
#306702=CARTESIAN_POINT('Ctrl Pts',(-3.16693672400006,2.2,2.52905215799998));
#306703=CARTESIAN_POINT('Ctrl Pts',(-3.16769512400006,12.2,2.52946862799998));
#306704=CARTESIAN_POINT('Ctrl Pts',(-3.16769512400006,5.2,2.52946862799998));
#306705=CARTESIAN_POINT('Ctrl Pts',(-3.16769512400006,2.2,2.52946862799998));
#306706=CARTESIAN_POINT('Ctrl Pts',(-3.16845905300006,12.2,2.52988689199999));
#306707=CARTESIAN_POINT('Ctrl Pts',(-3.16845905300006,5.2,2.52988689199999));
#306708=CARTESIAN_POINT('Ctrl Pts',(-3.16845905300006,2.2,2.52988689199999));
#306709=CARTESIAN_POINT('Ctrl Pts',(-3.16922850500006,12.2,2.53030693299999));
#306710=CARTESIAN_POINT('Ctrl Pts',(-3.16922850500006,5.2,2.53030693299999));
#306711=CARTESIAN_POINT('Ctrl Pts',(-3.16922850500006,2.2,2.53030693299999));
#306712=CARTESIAN_POINT('Ctrl Pts',(-3.17000347800006,12.2,2.53072873299999));
#306713=CARTESIAN_POINT('Ctrl Pts',(-3.17000347800006,5.2,2.53072873299999));
#306714=CARTESIAN_POINT('Ctrl Pts',(-3.17000347800006,2.2,2.53072873299999));
#306715=CARTESIAN_POINT('Ctrl Pts',(-3.17078396800006,12.2,2.53115227499999));
#306716=CARTESIAN_POINT('Ctrl Pts',(-3.17078396800006,5.2,2.53115227499999));
#306717=CARTESIAN_POINT('Ctrl Pts',(-3.17078396800006,2.2,2.53115227499999));
#306718=CARTESIAN_POINT('Ctrl Pts',(-3.17156997100006,12.2,2.53157754199999));
#306719=CARTESIAN_POINT('Ctrl Pts',(-3.17156997100006,5.2,2.53157754199999));
#306720=CARTESIAN_POINT('Ctrl Pts',(-3.17156997100006,2.2,2.53157754199999));
#306721=CARTESIAN_POINT('Ctrl Pts',(-3.17236148500006,12.2,2.53200451699998));
#306722=CARTESIAN_POINT('Ctrl Pts',(-3.17236148500006,5.2,2.53200451699998));
#306723=CARTESIAN_POINT('Ctrl Pts',(-3.17236148500006,2.2,2.53200451699998));
#306724=CARTESIAN_POINT('Ctrl Pts',(-3.17315850600006,12.2,2.53243318299998));
#306725=CARTESIAN_POINT('Ctrl Pts',(-3.17315850600006,5.2,2.53243318299998));
#306726=CARTESIAN_POINT('Ctrl Pts',(-3.17315850600006,2.2,2.53243318299998));
#306727=CARTESIAN_POINT('Ctrl Pts',(-3.17396102900006,12.2,2.53286352099998));
#306728=CARTESIAN_POINT('Ctrl Pts',(-3.17396102900006,5.2,2.53286352099998));
#306729=CARTESIAN_POINT('Ctrl Pts',(-3.17396102900006,2.2,2.53286352099998));
#306730=CARTESIAN_POINT('Ctrl Pts',(-3.17476905200006,12.2,2.53329551799998));
#306731=CARTESIAN_POINT('Ctrl Pts',(-3.17476905200006,5.2,2.53329551799998));
#306732=CARTESIAN_POINT('Ctrl Pts',(-3.17476905200006,2.2,2.53329551799998));
#306733=CARTESIAN_POINT('Ctrl Pts',(-3.17558257100006,12.2,2.53372915199999));
#306734=CARTESIAN_POINT('Ctrl Pts',(-3.17558257100006,5.2,2.53372915199999));
#306735=CARTESIAN_POINT('Ctrl Pts',(-3.17558257100006,2.2,2.53372915199999));
#306736=CARTESIAN_POINT('Ctrl Pts',(-3.17640158400006,12.2,2.53416441099999));
#306737=CARTESIAN_POINT('Ctrl Pts',(-3.17640158400006,5.2,2.53416441099999));
#306738=CARTESIAN_POINT('Ctrl Pts',(-3.17640158400006,2.2,2.53416441099999));
#306739=CARTESIAN_POINT('Ctrl Pts',(-3.17722608400006,12.2,2.53460127399999));
#306740=CARTESIAN_POINT('Ctrl Pts',(-3.17722608400006,5.2,2.53460127399999));
#306741=CARTESIAN_POINT('Ctrl Pts',(-3.17722608400006,2.2,2.53460127399999));
#306742=CARTESIAN_POINT('Ctrl Pts',(-3.17805607100006,12.2,2.53503972699999));
#306743=CARTESIAN_POINT('Ctrl Pts',(-3.17805607100006,5.2,2.53503972699999));
#306744=CARTESIAN_POINT('Ctrl Pts',(-3.17805607100006,2.2,2.53503972699999));
#306745=CARTESIAN_POINT('Ctrl Pts',(-3.17889154000006,12.2,2.53547975099998));
#306746=CARTESIAN_POINT('Ctrl Pts',(-3.17889154000006,5.2,2.53547975099998));
#306747=CARTESIAN_POINT('Ctrl Pts',(-3.17889154000006,2.2,2.53547975099998));
#306748=CARTESIAN_POINT('Ctrl Pts',(-3.17973248600006,12.2,2.53592133199999));
#306749=CARTESIAN_POINT('Ctrl Pts',(-3.17973248600006,5.2,2.53592133199999));
#306750=CARTESIAN_POINT('Ctrl Pts',(-3.17973248600006,2.2,2.53592133199999));
#306751=CARTESIAN_POINT('Ctrl Pts',(-3.18057890900006,12.2,2.53636445099998));
#306752=CARTESIAN_POINT('Ctrl Pts',(-3.18057890900006,5.2,2.53636445099998));
#306753=CARTESIAN_POINT('Ctrl Pts',(-3.18057890900006,2.2,2.53636445099998));
#306754=CARTESIAN_POINT('Ctrl Pts',(-3.18143080200006,12.2,2.53680909099998));
#306755=CARTESIAN_POINT('Ctrl Pts',(-3.18143080200006,5.2,2.53680909099998));
#306756=CARTESIAN_POINT('Ctrl Pts',(-3.18143080200006,2.2,2.53680909099998));
#306757=CARTESIAN_POINT('Ctrl Pts',(-3.18228816200006,12.2,2.53725523899998));
#306758=CARTESIAN_POINT('Ctrl Pts',(-3.18228816200006,5.2,2.53725523899998));
#306759=CARTESIAN_POINT('Ctrl Pts',(-3.18228816200006,2.2,2.53725523899998));
#306760=CARTESIAN_POINT('Ctrl Pts',(-3.18315098700006,12.2,2.53770287399998));
#306761=CARTESIAN_POINT('Ctrl Pts',(-3.18315098700006,5.2,2.53770287399998));
#306762=CARTESIAN_POINT('Ctrl Pts',(-3.18315098700006,2.2,2.53770287399998));
#306763=CARTESIAN_POINT('Ctrl Pts',(-3.18401927200005,12.2,2.53815198299999));
#306764=CARTESIAN_POINT('Ctrl Pts',(-3.18401927200005,5.2,2.53815198299999));
#306765=CARTESIAN_POINT('Ctrl Pts',(-3.18401927200005,2.2,2.53815198299999));
#306766=CARTESIAN_POINT('Ctrl Pts',(-3.18489301400006,12.2,2.53860254699998));
#306767=CARTESIAN_POINT('Ctrl Pts',(-3.18489301400006,5.2,2.53860254699998));
#306768=CARTESIAN_POINT('Ctrl Pts',(-3.18489301400006,2.2,2.53860254699998));
#306769=CARTESIAN_POINT('Ctrl Pts',(-3.18577220800006,12.2,2.53905455099999));
#306770=CARTESIAN_POINT('Ctrl Pts',(-3.18577220800006,5.2,2.53905455099999));
#306771=CARTESIAN_POINT('Ctrl Pts',(-3.18577220800006,2.2,2.53905455099999));
#306772=CARTESIAN_POINT('Ctrl Pts',(-3.18665685300005,12.2,2.53950797899999));
#306773=CARTESIAN_POINT('Ctrl Pts',(-3.18665685300005,5.2,2.53950797899999));
#306774=CARTESIAN_POINT('Ctrl Pts',(-3.18665685300005,2.2,2.53950797899999));
#306775=CARTESIAN_POINT('Ctrl Pts',(-3.18754694300006,12.2,2.53996281299998));
#306776=CARTESIAN_POINT('Ctrl Pts',(-3.18754694300006,5.2,2.53996281299998));
#306777=CARTESIAN_POINT('Ctrl Pts',(-3.18754694300006,2.2,2.53996281299998));
#306778=CARTESIAN_POINT('Ctrl Pts',(-3.18844247500006,12.2,2.54041903699999));
#306779=CARTESIAN_POINT('Ctrl Pts',(-3.18844247500006,5.2,2.54041903699999));
#306780=CARTESIAN_POINT('Ctrl Pts',(-3.18844247500006,2.2,2.54041903699999));
#306781=CARTESIAN_POINT('Ctrl Pts',(-3.18934344500006,12.2,2.54087663699998));
#306782=CARTESIAN_POINT('Ctrl Pts',(-3.18934344500006,5.2,2.54087663699998));
#306783=CARTESIAN_POINT('Ctrl Pts',(-3.18934344500006,2.2,2.54087663699998));
#306784=CARTESIAN_POINT('Ctrl Pts',(-3.19024985000006,12.2,2.54133559499999));
#306785=CARTESIAN_POINT('Ctrl Pts',(-3.19024985000006,5.2,2.54133559499999));
#306786=CARTESIAN_POINT('Ctrl Pts',(-3.19024985000006,2.2,2.54133559499999));
#306787=CARTESIAN_POINT('Ctrl Pts',(-3.19116168500006,12.2,2.54179589499999));
#306788=CARTESIAN_POINT('Ctrl Pts',(-3.19116168500006,5.2,2.54179589499999));
#306789=CARTESIAN_POINT('Ctrl Pts',(-3.19116168500006,2.2,2.54179589499999));
#306790=CARTESIAN_POINT('Ctrl Pts',(-3.19207894900006,12.2,2.54225752099998));
#306791=CARTESIAN_POINT('Ctrl Pts',(-3.19207894900006,5.2,2.54225752099998));
#306792=CARTESIAN_POINT('Ctrl Pts',(-3.19207894900006,2.2,2.54225752099998));
#306793=CARTESIAN_POINT('Ctrl Pts',(-3.19300163400006,12.2,2.54272045899998));
#306794=CARTESIAN_POINT('Ctrl Pts',(-3.19300163400006,5.2,2.54272045899998));
#306795=CARTESIAN_POINT('Ctrl Pts',(-3.19300163400006,2.2,2.54272045899998));
#306796=CARTESIAN_POINT('Ctrl Pts',(-3.19392974100006,12.2,2.54318468899999));
#306797=CARTESIAN_POINT('Ctrl Pts',(-3.19392974100006,5.2,2.54318468899999));
#306798=CARTESIAN_POINT('Ctrl Pts',(-3.19392974100006,2.2,2.54318468899999));
#306799=CARTESIAN_POINT('Ctrl Pts',(-3.19486326300006,12.2,2.54365019799998));
#306800=CARTESIAN_POINT('Ctrl Pts',(-3.19486326300006,5.2,2.54365019799998));
#306801=CARTESIAN_POINT('Ctrl Pts',(-3.19486326300006,2.2,2.54365019799998));
#306802=CARTESIAN_POINT('Ctrl Pts',(-3.19580219600006,12.2,2.54411696899999));
#306803=CARTESIAN_POINT('Ctrl Pts',(-3.19580219600006,5.2,2.54411696899999));
#306804=CARTESIAN_POINT('Ctrl Pts',(-3.19580219600006,2.2,2.54411696899999));
#306805=CARTESIAN_POINT('Ctrl Pts',(-3.19674653900006,12.2,2.54458498699999));
#306806=CARTESIAN_POINT('Ctrl Pts',(-3.19674653900006,5.2,2.54458498699999));
#306807=CARTESIAN_POINT('Ctrl Pts',(-3.19674653900006,2.2,2.54458498699999));
#306808=CARTESIAN_POINT('Ctrl Pts',(-3.19769628500006,12.2,2.54505423499998));
#306809=CARTESIAN_POINT('Ctrl Pts',(-3.19769628500006,5.2,2.54505423499998));
#306810=CARTESIAN_POINT('Ctrl Pts',(-3.19769628500006,2.2,2.54505423499998));
#306811=CARTESIAN_POINT('Ctrl Pts',(-3.19865143200006,12.2,2.54552469799999));
#306812=CARTESIAN_POINT('Ctrl Pts',(-3.19865143200006,5.2,2.54552469799999));
#306813=CARTESIAN_POINT('Ctrl Pts',(-3.19865143200006,2.2,2.54552469799999));
#306814=CARTESIAN_POINT('Ctrl Pts',(-3.19961197700006,12.2,2.54599635999998));
#306815=CARTESIAN_POINT('Ctrl Pts',(-3.19961197700006,5.2,2.54599635999998));
#306816=CARTESIAN_POINT('Ctrl Pts',(-3.19961197700006,2.2,2.54599635999998));
#306817=CARTESIAN_POINT('Ctrl Pts',(-3.20057791400005,12.2,2.54646920599999));
#306818=CARTESIAN_POINT('Ctrl Pts',(-3.20057791400005,5.2,2.54646920599999));
#306819=CARTESIAN_POINT('Ctrl Pts',(-3.20057791400005,2.2,2.54646920599999));
#306820=CARTESIAN_POINT('Ctrl Pts',(-3.20154924000006,12.2,2.54694321899999));
#306821=CARTESIAN_POINT('Ctrl Pts',(-3.20154924000006,5.2,2.54694321899999));
#306822=CARTESIAN_POINT('Ctrl Pts',(-3.20154924000006,2.2,2.54694321899999));
#306823=CARTESIAN_POINT('Ctrl Pts',(-3.20252595200006,12.2,2.54741838499999));
#306824=CARTESIAN_POINT('Ctrl Pts',(-3.20252595200006,5.2,2.54741838499999));
#306825=CARTESIAN_POINT('Ctrl Pts',(-3.20252595200006,2.2,2.54741838499999));
#306826=CARTESIAN_POINT('Ctrl Pts',(-3.20350804500006,12.2,2.54789468699999));
#306827=CARTESIAN_POINT('Ctrl Pts',(-3.20350804500006,5.2,2.54789468699999));
#306828=CARTESIAN_POINT('Ctrl Pts',(-3.20350804500006,2.2,2.54789468699999));
#306829=CARTESIAN_POINT('Ctrl Pts',(-3.20449551600006,12.2,2.54837210999998));
#306830=CARTESIAN_POINT('Ctrl Pts',(-3.20449551600006,5.2,2.54837210999998));
#306831=CARTESIAN_POINT('Ctrl Pts',(-3.20449551600006,2.2,2.54837210999998));
#306832=CARTESIAN_POINT('Ctrl Pts',(-3.20548836100006,12.2,2.54885063899999));
#306833=CARTESIAN_POINT('Ctrl Pts',(-3.20548836100006,5.2,2.54885063899999));
#306834=CARTESIAN_POINT('Ctrl Pts',(-3.20548836100006,2.2,2.54885063899999));
#306835=CARTESIAN_POINT('Ctrl Pts',(-3.20648657500006,12.2,2.54933025799998));
#306836=CARTESIAN_POINT('Ctrl Pts',(-3.20648657500006,5.2,2.54933025799998));
#306837=CARTESIAN_POINT('Ctrl Pts',(-3.20648657500006,2.2,2.54933025799998));
#306838=CARTESIAN_POINT('Ctrl Pts',(-3.20749015500006,12.2,2.54981095199999));
#306839=CARTESIAN_POINT('Ctrl Pts',(-3.20749015500006,5.2,2.54981095199999));
#306840=CARTESIAN_POINT('Ctrl Pts',(-3.20749015500006,2.2,2.54981095199999));
#306841=CARTESIAN_POINT('Ctrl Pts',(-3.20849909800006,12.2,2.55029270599999));
#306842=CARTESIAN_POINT('Ctrl Pts',(-3.20849909800006,5.2,2.55029270599999));
#306843=CARTESIAN_POINT('Ctrl Pts',(-3.20849909800006,2.2,2.55029270599999));
#306844=CARTESIAN_POINT('Ctrl Pts',(-3.20951339800006,12.2,2.55077550299998));
#306845=CARTESIAN_POINT('Ctrl Pts',(-3.20951339800006,5.2,2.55077550299998));
#306846=CARTESIAN_POINT('Ctrl Pts',(-3.20951339800006,2.2,2.55077550299998));
#306847=CARTESIAN_POINT('Ctrl Pts',(-3.21053305200006,12.2,2.55125932999999));
#306848=CARTESIAN_POINT('Ctrl Pts',(-3.21053305200006,5.2,2.55125932999999));
#306849=CARTESIAN_POINT('Ctrl Pts',(-3.21053305200006,2.2,2.55125932999999));
#306850=CARTESIAN_POINT('Ctrl Pts',(-3.21155805600006,12.2,2.55174416999999));
#306851=CARTESIAN_POINT('Ctrl Pts',(-3.21155805600006,5.2,2.55174416999999));
#306852=CARTESIAN_POINT('Ctrl Pts',(-3.21155805600006,2.2,2.55174416999999));
#306853=CARTESIAN_POINT('Ctrl Pts',(-3.21258840700006,12.2,2.55223000899999));
#306854=CARTESIAN_POINT('Ctrl Pts',(-3.21258840700006,5.2,2.55223000899999));
#306855=CARTESIAN_POINT('Ctrl Pts',(-3.21258840700006,2.2,2.55223000899999));
#306856=CARTESIAN_POINT('Ctrl Pts',(-3.21362410000006,12.2,2.55271683099998));
#306857=CARTESIAN_POINT('Ctrl Pts',(-3.21362410000006,5.2,2.55271683099998));
#306858=CARTESIAN_POINT('Ctrl Pts',(-3.21362410000006,2.2,2.55271683099998));
#306859=CARTESIAN_POINT('Ctrl Pts',(-3.21466513100006,12.2,2.55320462199998));
#306860=CARTESIAN_POINT('Ctrl Pts',(-3.21466513100006,5.2,2.55320462199998));
#306861=CARTESIAN_POINT('Ctrl Pts',(-3.21466513100006,2.2,2.55320462199998));
#306862=CARTESIAN_POINT('Ctrl Pts',(-3.21571149700006,12.2,2.55369336599998));
#306863=CARTESIAN_POINT('Ctrl Pts',(-3.21571149700006,5.2,2.55369336599998));
#306864=CARTESIAN_POINT('Ctrl Pts',(-3.21571149700006,2.2,2.55369336599998));
#306865=CARTESIAN_POINT('Ctrl Pts',(-3.21676319300006,12.2,2.55418304699998));
#306866=CARTESIAN_POINT('Ctrl Pts',(-3.21676319300006,5.2,2.55418304699998));
#306867=CARTESIAN_POINT('Ctrl Pts',(-3.21676319300006,2.2,2.55418304699998));
#306868=CARTESIAN_POINT('Ctrl Pts',(-3.21782021500006,12.2,2.55467365199999));
#306869=CARTESIAN_POINT('Ctrl Pts',(-3.21782021500006,5.2,2.55467365199999));
#306870=CARTESIAN_POINT('Ctrl Pts',(-3.21782021500006,2.2,2.55467365199999));
#306871=CARTESIAN_POINT('Ctrl Pts',(-3.21888255800005,12.2,2.55516516599998));
#306872=CARTESIAN_POINT('Ctrl Pts',(-3.21888255800005,5.2,2.55516516599998));
#306873=CARTESIAN_POINT('Ctrl Pts',(-3.21888255800005,2.2,2.55516516599998));
#306874=CARTESIAN_POINT('Ctrl Pts',(-3.21995022000006,12.2,2.55565757299999));
#306875=CARTESIAN_POINT('Ctrl Pts',(-3.21995022000006,5.2,2.55565757299999));
#306876=CARTESIAN_POINT('Ctrl Pts',(-3.21995022000006,2.2,2.55565757299999));
#306877=CARTESIAN_POINT('Ctrl Pts',(-3.22102319800006,12.2,2.55615085899999));
#306878=CARTESIAN_POINT('Ctrl Pts',(-3.22102319800006,5.2,2.55615085899999));
#306879=CARTESIAN_POINT('Ctrl Pts',(-3.22102319800006,2.2,2.55615085899999));
#306880=CARTESIAN_POINT('Ctrl Pts',(-3.22210148400006,12.2,2.55664500799998));
#306881=CARTESIAN_POINT('Ctrl Pts',(-3.22210148400006,5.2,2.55664500799998));
#306882=CARTESIAN_POINT('Ctrl Pts',(-3.22210148400006,2.2,2.55664500799998));
#306883=CARTESIAN_POINT('Ctrl Pts',(-3.22318507700006,12.2,2.55714000599998));
#306884=CARTESIAN_POINT('Ctrl Pts',(-3.22318507700006,5.2,2.55714000599998));
#306885=CARTESIAN_POINT('Ctrl Pts',(-3.22318507700006,2.2,2.55714000599998));
#306886=CARTESIAN_POINT('Ctrl Pts',(-3.22427397100005,12.2,2.55763583899999));
#306887=CARTESIAN_POINT('Ctrl Pts',(-3.22427397100005,5.2,2.55763583899999));
#306888=CARTESIAN_POINT('Ctrl Pts',(-3.22427397100005,2.2,2.55763583899999));
#306889=CARTESIAN_POINT('Ctrl Pts',(-3.22536816400006,12.2,2.55813249099998));
#306890=CARTESIAN_POINT('Ctrl Pts',(-3.22536816400006,5.2,2.55813249099998));
#306891=CARTESIAN_POINT('Ctrl Pts',(-3.22536816400006,2.2,2.55813249099998));
#306892=CARTESIAN_POINT('Ctrl Pts',(-3.22646765100005,12.2,2.55862994799998));
#306893=CARTESIAN_POINT('Ctrl Pts',(-3.22646765100005,5.2,2.55862994799998));
#306894=CARTESIAN_POINT('Ctrl Pts',(-3.22646765100005,2.2,2.55862994799998));
#306895=CARTESIAN_POINT('Ctrl Pts',(-3.22757242600006,12.2,2.55912819499999));
#306896=CARTESIAN_POINT('Ctrl Pts',(-3.22757242600006,5.2,2.55912819499999));
#306897=CARTESIAN_POINT('Ctrl Pts',(-3.22757242600006,2.2,2.55912819499999));
#306898=CARTESIAN_POINT('Ctrl Pts',(-3.22868248800006,12.2,2.55962721799998));
#306899=CARTESIAN_POINT('Ctrl Pts',(-3.22868248800006,5.2,2.55962721799998));
#306900=CARTESIAN_POINT('Ctrl Pts',(-3.22868248800006,2.2,2.55962721799998));
#306901=CARTESIAN_POINT('Ctrl Pts',(-3.22979783200006,12.2,2.56012700199998));
#306902=CARTESIAN_POINT('Ctrl Pts',(-3.22979783200006,5.2,2.56012700199998));
#306903=CARTESIAN_POINT('Ctrl Pts',(-3.22979783200006,2.2,2.56012700199998));
#306904=CARTESIAN_POINT('Ctrl Pts',(-3.23091845200006,12.2,2.56062753299998));
#306905=CARTESIAN_POINT('Ctrl Pts',(-3.23091845200006,5.2,2.56062753299998));
#306906=CARTESIAN_POINT('Ctrl Pts',(-3.23091845200006,2.2,2.56062753299998));
#306907=CARTESIAN_POINT('Ctrl Pts',(-3.23204434700005,12.2,2.56112879599999));
#306908=CARTESIAN_POINT('Ctrl Pts',(-3.23204434700005,5.2,2.56112879599999));
#306909=CARTESIAN_POINT('Ctrl Pts',(-3.23204434700005,2.2,2.56112879599999));
#306910=CARTESIAN_POINT('Ctrl Pts',(-3.23317551000006,12.2,2.56163077699998));
#306911=CARTESIAN_POINT('Ctrl Pts',(-3.23317551000006,5.2,2.56163077699998));
#306912=CARTESIAN_POINT('Ctrl Pts',(-3.23317551000006,2.2,2.56163077699998));
#306913=CARTESIAN_POINT('Ctrl Pts',(-3.23431193700006,12.2,2.56213345999999));
#306914=CARTESIAN_POINT('Ctrl Pts',(-3.23431193700006,5.2,2.56213345999999));
#306915=CARTESIAN_POINT('Ctrl Pts',(-3.23431193700006,2.2,2.56213345999999));
#306916=CARTESIAN_POINT('Ctrl Pts',(-3.23545362600006,12.2,2.56263683399998));
#306917=CARTESIAN_POINT('Ctrl Pts',(-3.23545362600006,5.2,2.56263683399998));
#306918=CARTESIAN_POINT('Ctrl Pts',(-3.23545362600006,2.2,2.56263683399998));
#306919=CARTESIAN_POINT('Ctrl Pts',(-3.23660057200006,12.2,2.56314088099998));
#306920=CARTESIAN_POINT('Ctrl Pts',(-3.23660057200006,5.2,2.56314088099998));
#306921=CARTESIAN_POINT('Ctrl Pts',(-3.23660057200006,2.2,2.56314088099998));
#306922=CARTESIAN_POINT('Ctrl Pts',(-3.23775276900006,12.2,2.56364558999999));
#306923=CARTESIAN_POINT('Ctrl Pts',(-3.23775276900006,5.2,2.56364558999999));
#306924=CARTESIAN_POINT('Ctrl Pts',(-3.23775276900006,2.2,2.56364558999999));
#306925=CARTESIAN_POINT('Ctrl Pts',(-3.23891021500006,12.2,2.56415094499998));
#306926=CARTESIAN_POINT('Ctrl Pts',(-3.23891021500006,5.2,2.56415094499998));
#306927=CARTESIAN_POINT('Ctrl Pts',(-3.23891021500006,2.2,2.56415094499998));
#306928=CARTESIAN_POINT('Ctrl Pts',(-3.24007290600006,12.2,2.56465693099998));
#306929=CARTESIAN_POINT('Ctrl Pts',(-3.24007290600006,5.2,2.56465693099998));
#306930=CARTESIAN_POINT('Ctrl Pts',(-3.24007290600006,2.2,2.56465693099998));
#306931=CARTESIAN_POINT('Ctrl Pts',(-3.24124083500006,12.2,2.56516353499999));
#306932=CARTESIAN_POINT('Ctrl Pts',(-3.24124083500006,5.2,2.56516353499999));
#306933=CARTESIAN_POINT('Ctrl Pts',(-3.24124083500006,2.2,2.56516353499999));
#306934=CARTESIAN_POINT('Ctrl Pts',(-3.24241400000005,12.2,2.56567074399998));
#306935=CARTESIAN_POINT('Ctrl Pts',(-3.24241400000005,5.2,2.56567074399998));
#306936=CARTESIAN_POINT('Ctrl Pts',(-3.24241400000005,2.2,2.56567074399998));
#306937=CARTESIAN_POINT('Ctrl Pts',(-3.24359239700006,12.2,2.56617854099999));
#306938=CARTESIAN_POINT('Ctrl Pts',(-3.24359239700006,5.2,2.56617854099999));
#306939=CARTESIAN_POINT('Ctrl Pts',(-3.24359239700006,2.2,2.56617854099999));
#306940=CARTESIAN_POINT('Ctrl Pts',(-3.24477602100006,12.2,2.56668691499998));
#306941=CARTESIAN_POINT('Ctrl Pts',(-3.24477602100006,5.2,2.56668691499998));
#306942=CARTESIAN_POINT('Ctrl Pts',(-3.24477602100006,2.2,2.56668691499998));
#306943=CARTESIAN_POINT('Ctrl Pts',(-3.24596486800006,12.2,2.56719584999999));
#306944=CARTESIAN_POINT('Ctrl Pts',(-3.24596486800006,5.2,2.56719584999999));
#306945=CARTESIAN_POINT('Ctrl Pts',(-3.24596486800006,2.2,2.56719584999999));
#306946=CARTESIAN_POINT('Ctrl Pts',(-3.24715893300006,12.2,2.56770533199998));
#306947=CARTESIAN_POINT('Ctrl Pts',(-3.24715893300006,5.2,2.56770533199998));
#306948=CARTESIAN_POINT('Ctrl Pts',(-3.24715893300006,2.2,2.56770533199998));
#306949=CARTESIAN_POINT('Ctrl Pts',(-3.24835821300006,12.2,2.56821534799998));
#306950=CARTESIAN_POINT('Ctrl Pts',(-3.24835821300006,5.2,2.56821534799998));
#306951=CARTESIAN_POINT('Ctrl Pts',(-3.24835821300006,2.2,2.56821534799998));
#306952=CARTESIAN_POINT('Ctrl Pts',(-3.24956270200006,12.2,2.56872588399998));
#306953=CARTESIAN_POINT('Ctrl Pts',(-3.24956270200006,5.2,2.56872588399998));
#306954=CARTESIAN_POINT('Ctrl Pts',(-3.24956270200006,2.2,2.56872588399998));
#306955=CARTESIAN_POINT('Ctrl Pts',(-3.25077239900006,12.2,2.56923692599998));
#306956=CARTESIAN_POINT('Ctrl Pts',(-3.25077239900006,5.2,2.56923692599998));
#306957=CARTESIAN_POINT('Ctrl Pts',(-3.25077239900006,2.2,2.56923692599998));
#306958=CARTESIAN_POINT('Ctrl Pts',(-3.25198729600006,12.2,2.56974845999999));
#306959=CARTESIAN_POINT('Ctrl Pts',(-3.25198729600006,5.2,2.56974845999999));
#306960=CARTESIAN_POINT('Ctrl Pts',(-3.25198729600006,2.2,2.56974845999999));
#306961=CARTESIAN_POINT('Ctrl Pts',(-3.25320739000006,12.2,2.57026047199999));
#306962=CARTESIAN_POINT('Ctrl Pts',(-3.25320739000006,5.2,2.57026047199999));
#306963=CARTESIAN_POINT('Ctrl Pts',(-3.25320739000006,2.2,2.57026047199999));
#306964=CARTESIAN_POINT('Ctrl Pts',(-3.25443267700006,12.2,2.57077294899998));
#306965=CARTESIAN_POINT('Ctrl Pts',(-3.25443267700006,5.2,2.57077294899998));
#306966=CARTESIAN_POINT('Ctrl Pts',(-3.25443267700006,2.2,2.57077294899998));
#306967=CARTESIAN_POINT('Ctrl Pts',(-3.25566315300006,12.2,2.57128587699999));
#306968=CARTESIAN_POINT('Ctrl Pts',(-3.25566315300006,5.2,2.57128587699999));
#306969=CARTESIAN_POINT('Ctrl Pts',(-3.25566315300006,2.2,2.57128587699999));
#306970=CARTESIAN_POINT('Ctrl Pts',(-3.25689881400006,12.2,2.57179923999999));
#306971=CARTESIAN_POINT('Ctrl Pts',(-3.25689881400006,5.2,2.57179923999999));
#306972=CARTESIAN_POINT('Ctrl Pts',(-3.25689881400006,2.2,2.57179923999999));
#306973=CARTESIAN_POINT('Ctrl Pts',(-3.25813965300005,12.2,2.57231302899999));
#306974=CARTESIAN_POINT('Ctrl Pts',(-3.25813965300005,5.2,2.57231302899999));
#306975=CARTESIAN_POINT('Ctrl Pts',(-3.25813965300005,2.2,2.57231302899999));
#306976=CARTESIAN_POINT('Ctrl Pts',(-3.25938567000006,12.2,2.57282722699999));
#306977=CARTESIAN_POINT('Ctrl Pts',(-3.25938567000006,5.2,2.57282722699999));
#306978=CARTESIAN_POINT('Ctrl Pts',(-3.25938567000006,2.2,2.57282722699999));
#306979=CARTESIAN_POINT('Ctrl Pts',(-3.26063685700006,12.2,2.57334181999998));
#306980=CARTESIAN_POINT('Ctrl Pts',(-3.26063685700006,5.2,2.57334181999998));
#306981=CARTESIAN_POINT('Ctrl Pts',(-3.26063685700006,2.2,2.57334181999998));
#306982=CARTESIAN_POINT('Ctrl Pts',(-3.26189321000005,12.2,2.57385679699999));
#306983=CARTESIAN_POINT('Ctrl Pts',(-3.26189321000005,5.2,2.57385679699999));
#306984=CARTESIAN_POINT('Ctrl Pts',(-3.26189321000005,2.2,2.57385679699999));
#306985=CARTESIAN_POINT('Ctrl Pts',(-3.26315472700006,12.2,2.57437214299999));
#306986=CARTESIAN_POINT('Ctrl Pts',(-3.26315472700006,5.2,2.57437214299999));
#306987=CARTESIAN_POINT('Ctrl Pts',(-3.26315472700006,2.2,2.57437214299999));
#306988=CARTESIAN_POINT('Ctrl Pts',(-3.26442140100006,12.2,2.57488784499999));
#306989=CARTESIAN_POINT('Ctrl Pts',(-3.26442140100006,5.2,2.57488784499999));
#306990=CARTESIAN_POINT('Ctrl Pts',(-3.26442140100006,2.2,2.57488784499999));
#306991=CARTESIAN_POINT('Ctrl Pts',(-3.26569322900006,12.2,2.57540388899999));
#306992=CARTESIAN_POINT('Ctrl Pts',(-3.26569322900006,5.2,2.57540388899999));
#306993=CARTESIAN_POINT('Ctrl Pts',(-3.26569322900006,2.2,2.57540388899999));
#306994=CARTESIAN_POINT('Ctrl Pts',(-3.26697020700006,12.2,2.57592026099999));
#306995=CARTESIAN_POINT('Ctrl Pts',(-3.26697020700006,5.2,2.57592026099999));
#306996=CARTESIAN_POINT('Ctrl Pts',(-3.26697020700006,2.2,2.57592026099999));
#306997=CARTESIAN_POINT('Ctrl Pts',(-3.26825232900006,12.2,2.57643694899999));
#306998=CARTESIAN_POINT('Ctrl Pts',(-3.26825232900006,5.2,2.57643694899999));
#306999=CARTESIAN_POINT('Ctrl Pts',(-3.26825232900006,2.2,2.57643694899999));
#307000=CARTESIAN_POINT('Ctrl Pts',(-3.26953959300006,12.2,2.57695393999998));
#307001=CARTESIAN_POINT('Ctrl Pts',(-3.26953959300006,5.2,2.57695393999998));
#307002=CARTESIAN_POINT('Ctrl Pts',(-3.26953959300006,2.2,2.57695393999998));
#307003=CARTESIAN_POINT('Ctrl Pts',(-3.27083199200006,12.2,2.57747121899998));
#307004=CARTESIAN_POINT('Ctrl Pts',(-3.27083199200006,5.2,2.57747121899998));
#307005=CARTESIAN_POINT('Ctrl Pts',(-3.27083199200006,2.2,2.57747121899998));
#307006=CARTESIAN_POINT('Ctrl Pts',(-3.27212952400005,12.2,2.57798877299999));
#307007=CARTESIAN_POINT('Ctrl Pts',(-3.27212952400005,5.2,2.57798877299999));
#307008=CARTESIAN_POINT('Ctrl Pts',(-3.27212952400005,2.2,2.57798877299999));
#307009=CARTESIAN_POINT('Ctrl Pts',(-3.27343218200005,12.2,2.57850658999998));
#307010=CARTESIAN_POINT('Ctrl Pts',(-3.27343218200005,5.2,2.57850658999998));
#307011=CARTESIAN_POINT('Ctrl Pts',(-3.27343218200005,2.2,2.57850658999998));
#307012=CARTESIAN_POINT('Ctrl Pts',(-3.27473996200006,12.2,2.57902465599999));
#307013=CARTESIAN_POINT('Ctrl Pts',(-3.27473996200006,5.2,2.57902465599999));
#307014=CARTESIAN_POINT('Ctrl Pts',(-3.27473996200006,2.2,2.57902465599999));
#307015=CARTESIAN_POINT('Ctrl Pts',(-3.27605286300006,12.2,2.57954295799999));
#307016=CARTESIAN_POINT('Ctrl Pts',(-3.27605286300006,5.2,2.57954295799999));
#307017=CARTESIAN_POINT('Ctrl Pts',(-3.27605286300006,2.2,2.57954295799999));
#307018=CARTESIAN_POINT('Ctrl Pts',(-3.27737087600006,12.2,2.58006148299998));
#307019=CARTESIAN_POINT('Ctrl Pts',(-3.27737087600006,5.2,2.58006148299998));
#307020=CARTESIAN_POINT('Ctrl Pts',(-3.27737087600006,2.2,2.58006148299998));
#307021=CARTESIAN_POINT('Ctrl Pts',(-3.27869399900006,12.2,2.58058021799998));
#307022=CARTESIAN_POINT('Ctrl Pts',(-3.27869399900006,5.2,2.58058021799998));
#307023=CARTESIAN_POINT('Ctrl Pts',(-3.27869399900006,2.2,2.58058021799998));
#307024=CARTESIAN_POINT('Ctrl Pts',(-3.28002222700006,12.2,2.58109914799999));
#307025=CARTESIAN_POINT('Ctrl Pts',(-3.28002222700006,5.2,2.58109914799999));
#307026=CARTESIAN_POINT('Ctrl Pts',(-3.28002222700006,2.2,2.58109914799999));
#307027=CARTESIAN_POINT('Ctrl Pts',(-3.28135555500006,12.2,2.58161826399999));
#307028=CARTESIAN_POINT('Ctrl Pts',(-3.28135555500006,5.2,2.58161826399999));
#307029=CARTESIAN_POINT('Ctrl Pts',(-3.28135555500006,2.2,2.58161826399999));
#307030=CARTESIAN_POINT('Ctrl Pts',(-3.28269397900006,12.2,2.58213754899998));
#307031=CARTESIAN_POINT('Ctrl Pts',(-3.28269397900006,5.2,2.58213754899998));
#307032=CARTESIAN_POINT('Ctrl Pts',(-3.28269397900006,2.2,2.58213754899998));
#307033=CARTESIAN_POINT('Ctrl Pts',(-3.28403749500006,12.2,2.58265699099999));
#307034=CARTESIAN_POINT('Ctrl Pts',(-3.28403749500006,5.2,2.58265699099999));
#307035=CARTESIAN_POINT('Ctrl Pts',(-3.28403749500006,2.2,2.58265699099999));
#307036=CARTESIAN_POINT('Ctrl Pts',(-3.28538609800006,12.2,2.58317657899998));
#307037=CARTESIAN_POINT('Ctrl Pts',(-3.28538609800006,5.2,2.58317657899998));
#307038=CARTESIAN_POINT('Ctrl Pts',(-3.28538609800006,2.2,2.58317657899998));
#307039=CARTESIAN_POINT('Ctrl Pts',(-3.28673978400006,12.2,2.58369629799999));
#307040=CARTESIAN_POINT('Ctrl Pts',(-3.28673978400006,5.2,2.58369629799999));
#307041=CARTESIAN_POINT('Ctrl Pts',(-3.28673978400006,2.2,2.58369629799999));
#307042=CARTESIAN_POINT('Ctrl Pts',(-3.28809854700005,12.2,2.58421613699999));
#307043=CARTESIAN_POINT('Ctrl Pts',(-3.28809854700005,5.2,2.58421613699999));
#307044=CARTESIAN_POINT('Ctrl Pts',(-3.28809854700005,2.2,2.58421613699999));
#307045=CARTESIAN_POINT('Ctrl Pts',(-3.28946238400006,12.2,2.58473607999999));
#307046=CARTESIAN_POINT('Ctrl Pts',(-3.28946238400006,5.2,2.58473607999999));
#307047=CARTESIAN_POINT('Ctrl Pts',(-3.28946238400006,2.2,2.58473607999999));
#307048=CARTESIAN_POINT('Ctrl Pts',(-3.29083129000006,12.2,2.58525611799998));
#307049=CARTESIAN_POINT('Ctrl Pts',(-3.29083129000006,5.2,2.58525611799998));
#307050=CARTESIAN_POINT('Ctrl Pts',(-3.29083129000006,2.2,2.58525611799998));
#307051=CARTESIAN_POINT('Ctrl Pts',(-3.29220526000006,12.2,2.58577623599999));
#307052=CARTESIAN_POINT('Ctrl Pts',(-3.29220526000006,5.2,2.58577623599999));
#307053=CARTESIAN_POINT('Ctrl Pts',(-3.29220526000006,2.2,2.58577623599999));
#307054=CARTESIAN_POINT('Ctrl Pts',(-3.29358429000006,12.2,2.58629642199999));
#307055=CARTESIAN_POINT('Ctrl Pts',(-3.29358429000006,5.2,2.58629642199999));
#307056=CARTESIAN_POINT('Ctrl Pts',(-3.29358429000006,2.2,2.58629642199999));
#307057=CARTESIAN_POINT('Ctrl Pts',(-3.29496837500006,12.2,2.58681666199998));
#307058=CARTESIAN_POINT('Ctrl Pts',(-3.29496837500006,5.2,2.58681666199998));
#307059=CARTESIAN_POINT('Ctrl Pts',(-3.29496837500006,2.2,2.58681666199998));
#307060=CARTESIAN_POINT('Ctrl Pts',(-3.29635751000006,12.2,2.58733694599999));
#307061=CARTESIAN_POINT('Ctrl Pts',(-3.29635751000006,5.2,2.58733694599999));
#307062=CARTESIAN_POINT('Ctrl Pts',(-3.29635751000006,2.2,2.58733694599999));
#307063=CARTESIAN_POINT('Ctrl Pts',(-3.29775169200006,12.2,2.58785725799999));
#307064=CARTESIAN_POINT('Ctrl Pts',(-3.29775169200006,5.2,2.58785725799999));
#307065=CARTESIAN_POINT('Ctrl Pts',(-3.29775169200006,2.2,2.58785725799999));
#307066=CARTESIAN_POINT('Ctrl Pts',(-3.29915091600005,12.2,2.58837758699999));
#307067=CARTESIAN_POINT('Ctrl Pts',(-3.29915091600005,5.2,2.58837758699999));
#307068=CARTESIAN_POINT('Ctrl Pts',(-3.29915091600005,2.2,2.58837758699999));
#307069=CARTESIAN_POINT('Ctrl Pts',(-3.30055517600006,12.2,2.58889792199999));
#307070=CARTESIAN_POINT('Ctrl Pts',(-3.30055517600006,5.2,2.58889792199999));
#307071=CARTESIAN_POINT('Ctrl Pts',(-3.30055517600006,2.2,2.58889792199999));
#307072=CARTESIAN_POINT('Ctrl Pts',(-3.30196446900006,12.2,2.58941824799999));
#307073=CARTESIAN_POINT('Ctrl Pts',(-3.30196446900006,5.2,2.58941824799999));
#307074=CARTESIAN_POINT('Ctrl Pts',(-3.30196446900006,2.2,2.58941824799999));
#307075=CARTESIAN_POINT('Ctrl Pts',(-3.30337878900006,12.2,2.58993855299998));
#307076=CARTESIAN_POINT('Ctrl Pts',(-3.30337878900006,5.2,2.58993855299998));
#307077=CARTESIAN_POINT('Ctrl Pts',(-3.30337878900006,2.2,2.58993855299998));
#307078=CARTESIAN_POINT('Ctrl Pts',(-3.30479813300005,12.2,2.59045882499999));
#307079=CARTESIAN_POINT('Ctrl Pts',(-3.30479813300005,5.2,2.59045882499999));
#307080=CARTESIAN_POINT('Ctrl Pts',(-3.30479813300005,2.2,2.59045882499999));
#307081=CARTESIAN_POINT('Ctrl Pts',(-3.30622249500006,12.2,2.59097905199998));
#307082=CARTESIAN_POINT('Ctrl Pts',(-3.30622249500006,5.2,2.59097905199998));
#307083=CARTESIAN_POINT('Ctrl Pts',(-3.30622249500006,2.2,2.59097905199998));
#307084=CARTESIAN_POINT('Ctrl Pts',(-3.30765187100006,12.2,2.59149922099999));
#307085=CARTESIAN_POINT('Ctrl Pts',(-3.30765187100006,5.2,2.59149922099999));
#307086=CARTESIAN_POINT('Ctrl Pts',(-3.30765187100006,2.2,2.59149922099999));
#307087=CARTESIAN_POINT('Ctrl Pts',(-3.30908625600005,12.2,2.59201931899998));
#307088=CARTESIAN_POINT('Ctrl Pts',(-3.30908625600005,5.2,2.59201931899998));
#307089=CARTESIAN_POINT('Ctrl Pts',(-3.30908625600005,2.2,2.59201931899998));
#307090=CARTESIAN_POINT('Ctrl Pts',(-3.31052564600005,12.2,2.59253933499998));
#307091=CARTESIAN_POINT('Ctrl Pts',(-3.31052564600005,5.2,2.59253933499998));
#307092=CARTESIAN_POINT('Ctrl Pts',(-3.31052564600005,2.2,2.59253933499998));
#307093=CARTESIAN_POINT('Ctrl Pts',(-3.31197003500006,12.2,2.59305925499999));
#307094=CARTESIAN_POINT('Ctrl Pts',(-3.31197003500006,5.2,2.59305925499999));
#307095=CARTESIAN_POINT('Ctrl Pts',(-3.31197003500006,2.2,2.59305925499999));
#307096=CARTESIAN_POINT('Ctrl Pts',(-3.31341941900006,12.2,2.59357906899999));
#307097=CARTESIAN_POINT('Ctrl Pts',(-3.31341941900006,5.2,2.59357906899999));
#307098=CARTESIAN_POINT('Ctrl Pts',(-3.31341941900006,2.2,2.59357906899999));
#307099=CARTESIAN_POINT('Ctrl Pts',(-3.31487379500006,12.2,2.59409876299999));
#307100=CARTESIAN_POINT('Ctrl Pts',(-3.31487379500006,5.2,2.59409876299999));
#307101=CARTESIAN_POINT('Ctrl Pts',(-3.31487379500006,2.2,2.59409876299999));
#307102=CARTESIAN_POINT('Ctrl Pts',(-3.31633315600006,12.2,2.59461832399998));
#307103=CARTESIAN_POINT('Ctrl Pts',(-3.31633315600006,5.2,2.59461832399998));
#307104=CARTESIAN_POINT('Ctrl Pts',(-3.31633315600006,2.2,2.59461832399998));
#307105=CARTESIAN_POINT('Ctrl Pts',(-3.31779749900006,12.2,2.59513774099998));
#307106=CARTESIAN_POINT('Ctrl Pts',(-3.31779749900006,5.2,2.59513774099998));
#307107=CARTESIAN_POINT('Ctrl Pts',(-3.31779749900006,2.2,2.59513774099998));
#307108=CARTESIAN_POINT('Ctrl Pts',(-3.31926681800006,12.2,2.59565700299999));
#307109=CARTESIAN_POINT('Ctrl Pts',(-3.31926681800006,5.2,2.59565700299999));
#307110=CARTESIAN_POINT('Ctrl Pts',(-3.31926681800006,2.2,2.59565700299999));
#307111=CARTESIAN_POINT('Ctrl Pts',(-3.32074110900006,12.2,2.59617609599999));
#307112=CARTESIAN_POINT('Ctrl Pts',(-3.32074110900006,5.2,2.59617609599999));
#307113=CARTESIAN_POINT('Ctrl Pts',(-3.32074110900006,2.2,2.59617609599999));
#307114=CARTESIAN_POINT('Ctrl Pts',(-3.32222036700006,12.2,2.59669500799999));
#307115=CARTESIAN_POINT('Ctrl Pts',(-3.32222036700006,5.2,2.59669500799999));
#307116=CARTESIAN_POINT('Ctrl Pts',(-3.32222036700006,2.2,2.59669500799999));
#307117=CARTESIAN_POINT('Ctrl Pts',(-3.32370458800006,12.2,2.59721372699998));
#307118=CARTESIAN_POINT('Ctrl Pts',(-3.32370458800006,5.2,2.59721372699998));
#307119=CARTESIAN_POINT('Ctrl Pts',(-3.32370458800006,2.2,2.59721372699998));
#307120=CARTESIAN_POINT('Ctrl Pts',(-3.32519376600006,12.2,2.59773224199999));
#307121=CARTESIAN_POINT('Ctrl Pts',(-3.32519376600006,5.2,2.59773224199999));
#307122=CARTESIAN_POINT('Ctrl Pts',(-3.32519376600006,2.2,2.59773224199999));
#307123=CARTESIAN_POINT('Ctrl Pts',(-3.32668789800006,12.2,2.59825053999998));
#307124=CARTESIAN_POINT('Ctrl Pts',(-3.32668789800006,5.2,2.59825053999998));
#307125=CARTESIAN_POINT('Ctrl Pts',(-3.32668789800006,2.2,2.59825053999998));
#307126=CARTESIAN_POINT('Ctrl Pts',(-3.32818697700006,12.2,2.59876860899999));
#307127=CARTESIAN_POINT('Ctrl Pts',(-3.32818697700006,5.2,2.59876860899999));
#307128=CARTESIAN_POINT('Ctrl Pts',(-3.32818697700006,2.2,2.59876860899999));
#307129=CARTESIAN_POINT('Ctrl Pts',(-3.32969100100006,12.2,2.59928643799999));
#307130=CARTESIAN_POINT('Ctrl Pts',(-3.32969100100006,5.2,2.59928643799999));
#307131=CARTESIAN_POINT('Ctrl Pts',(-3.32969100100006,2.2,2.59928643799999));
#307132=CARTESIAN_POINT('Ctrl Pts',(-3.33119996300006,12.2,2.59980401299998));
#307133=CARTESIAN_POINT('Ctrl Pts',(-3.33119996300006,5.2,2.59980401299998));
#307134=CARTESIAN_POINT('Ctrl Pts',(-3.33119996300006,2.2,2.59980401299998));
#307135=CARTESIAN_POINT('Ctrl Pts',(-3.33271385900006,12.2,2.60032132499998));
#307136=CARTESIAN_POINT('Ctrl Pts',(-3.33271385900006,5.2,2.60032132499998));
#307137=CARTESIAN_POINT('Ctrl Pts',(-3.33271385900006,2.2,2.60032132499998));
#307138=CARTESIAN_POINT('Ctrl Pts',(-3.33423268400006,12.2,2.60083835899999));
#307139=CARTESIAN_POINT('Ctrl Pts',(-3.33423268400006,5.2,2.60083835899999));
#307140=CARTESIAN_POINT('Ctrl Pts',(-3.33423268400006,2.2,2.60083835899999));
#307141=CARTESIAN_POINT('Ctrl Pts',(-3.33575643400006,12.2,2.60135510599999));
#307142=CARTESIAN_POINT('Ctrl Pts',(-3.33575643400006,5.2,2.60135510599999));
#307143=CARTESIAN_POINT('Ctrl Pts',(-3.33575643400006,2.2,2.60135510599999));
#307144=CARTESIAN_POINT('Ctrl Pts',(-3.33728510500006,12.2,2.60187155199999));
#307145=CARTESIAN_POINT('Ctrl Pts',(-3.33728510500006,5.2,2.60187155199999));
#307146=CARTESIAN_POINT('Ctrl Pts',(-3.33728510500006,2.2,2.60187155199999));
#307147=CARTESIAN_POINT('Ctrl Pts',(-3.33881868900006,12.2,2.60238768599999));
#307148=CARTESIAN_POINT('Ctrl Pts',(-3.33881868900006,5.2,2.60238768599999));
#307149=CARTESIAN_POINT('Ctrl Pts',(-3.33881868900006,2.2,2.60238768599999));
#307150=CARTESIAN_POINT('Ctrl Pts',(-3.34035718400005,12.2,2.60290349699999));
#307151=CARTESIAN_POINT('Ctrl Pts',(-3.34035718400005,5.2,2.60290349699999));
#307152=CARTESIAN_POINT('Ctrl Pts',(-3.34035718400005,2.2,2.60290349699999));
#307153=CARTESIAN_POINT('Ctrl Pts',(-3.34190058500006,12.2,2.60341897199999));
#307154=CARTESIAN_POINT('Ctrl Pts',(-3.34190058500006,5.2,2.60341897199999));
#307155=CARTESIAN_POINT('Ctrl Pts',(-3.34190058500006,2.2,2.60341897199999));
#307156=CARTESIAN_POINT('Ctrl Pts',(-3.34344888600006,12.2,2.60393409999998));
#307157=CARTESIAN_POINT('Ctrl Pts',(-3.34344888600006,5.2,2.60393409999998));
#307158=CARTESIAN_POINT('Ctrl Pts',(-3.34344888600006,2.2,2.60393409999998));
#307159=CARTESIAN_POINT('Ctrl Pts',(-3.34500208300006,12.2,2.60444886799998));
#307160=CARTESIAN_POINT('Ctrl Pts',(-3.34500208300006,5.2,2.60444886799998));
#307161=CARTESIAN_POINT('Ctrl Pts',(-3.34500208300006,2.2,2.60444886799998));
#307162=CARTESIAN_POINT('Ctrl Pts',(-3.34656017100006,12.2,2.60496326699998));
#307163=CARTESIAN_POINT('Ctrl Pts',(-3.34656017100006,5.2,2.60496326699998));
#307164=CARTESIAN_POINT('Ctrl Pts',(-3.34656017100006,2.2,2.60496326699998));
#307165=CARTESIAN_POINT('Ctrl Pts',(-3.34812314600006,12.2,2.60547728199998));
#307166=CARTESIAN_POINT('Ctrl Pts',(-3.34812314600006,5.2,2.60547728199998));
#307167=CARTESIAN_POINT('Ctrl Pts',(-3.34812314600006,2.2,2.60547728199998));
#307168=CARTESIAN_POINT('Ctrl Pts',(-3.34969100100006,12.2,2.60599090499999));
#307169=CARTESIAN_POINT('Ctrl Pts',(-3.34969100100006,5.2,2.60599090499999));
#307170=CARTESIAN_POINT('Ctrl Pts',(-3.34969100100006,2.2,2.60599090499999));
#307171=CARTESIAN_POINT('Ctrl Pts',(-3.35126373300006,12.2,2.60650412199999));
#307172=CARTESIAN_POINT('Ctrl Pts',(-3.35126373300006,5.2,2.60650412199999));
#307173=CARTESIAN_POINT('Ctrl Pts',(-3.35126373300006,2.2,2.60650412199999));
#307174=CARTESIAN_POINT('Ctrl Pts',(-3.35284133700006,12.2,2.60701692199999));
#307175=CARTESIAN_POINT('Ctrl Pts',(-3.35284133700006,5.2,2.60701692199999));
#307176=CARTESIAN_POINT('Ctrl Pts',(-3.35284133700006,2.2,2.60701692199999));
#307177=CARTESIAN_POINT('Ctrl Pts',(-3.35442380800006,12.2,2.60752929399998));
#307178=CARTESIAN_POINT('Ctrl Pts',(-3.35442380800006,5.2,2.60752929399998));
#307179=CARTESIAN_POINT('Ctrl Pts',(-3.35442380800006,2.2,2.60752929399998));
#307180=CARTESIAN_POINT('Ctrl Pts',(-3.35601114000006,12.2,2.60804122499999));
#307181=CARTESIAN_POINT('Ctrl Pts',(-3.35601114000006,5.2,2.60804122499999));
#307182=CARTESIAN_POINT('Ctrl Pts',(-3.35601114000006,2.2,2.60804122499999));
#307183=CARTESIAN_POINT('Ctrl Pts',(-3.35760333100006,12.2,2.60855270599999));
#307184=CARTESIAN_POINT('Ctrl Pts',(-3.35760333100006,5.2,2.60855270599999));
#307185=CARTESIAN_POINT('Ctrl Pts',(-3.35760333100006,2.2,2.60855270599999));
#307186=CARTESIAN_POINT('Ctrl Pts',(-3.35920037300005,12.2,2.60906372399998));
#307187=CARTESIAN_POINT('Ctrl Pts',(-3.35920037300005,5.2,2.60906372399998));
#307188=CARTESIAN_POINT('Ctrl Pts',(-3.35920037300005,2.2,2.60906372399998));
#307189=CARTESIAN_POINT('Ctrl Pts',(-3.36080226300006,12.2,2.60957426799998));
#307190=CARTESIAN_POINT('Ctrl Pts',(-3.36080226300006,5.2,2.60957426799998));
#307191=CARTESIAN_POINT('Ctrl Pts',(-3.36080226300006,2.2,2.60957426799998));
#307192=CARTESIAN_POINT('Ctrl Pts',(-3.36240899500006,12.2,2.61008432499998));
#307193=CARTESIAN_POINT('Ctrl Pts',(-3.36240899500006,5.2,2.61008432499998));
#307194=CARTESIAN_POINT('Ctrl Pts',(-3.36240899500006,2.2,2.61008432499998));
#307195=CARTESIAN_POINT('Ctrl Pts',(-3.36402056500006,12.2,2.61059388699999));
#307196=CARTESIAN_POINT('Ctrl Pts',(-3.36402056500006,5.2,2.61059388699999));
#307197=CARTESIAN_POINT('Ctrl Pts',(-3.36402056500006,2.2,2.61059388699999));
#307198=CARTESIAN_POINT('Ctrl Pts',(-3.36563696800006,12.2,2.61110293999998));
#307199=CARTESIAN_POINT('Ctrl Pts',(-3.36563696800006,5.2,2.61110293999998));
#307200=CARTESIAN_POINT('Ctrl Pts',(-3.36563696800006,2.2,2.61110293999998));
#307201=CARTESIAN_POINT('Ctrl Pts',(-3.36725819900006,12.2,2.61161147299998));
#307202=CARTESIAN_POINT('Ctrl Pts',(-3.36725819900006,5.2,2.61161147299998));
#307203=CARTESIAN_POINT('Ctrl Pts',(-3.36725819900006,2.2,2.61161147299998));
#307204=CARTESIAN_POINT('Ctrl Pts',(-3.36888425300006,12.2,2.61211947599998));
#307205=CARTESIAN_POINT('Ctrl Pts',(-3.36888425300006,5.2,2.61211947599998));
#307206=CARTESIAN_POINT('Ctrl Pts',(-3.36888425300006,2.2,2.61211947599998));
#307207=CARTESIAN_POINT('Ctrl Pts',(-3.37051512400006,12.2,2.61262693699998));
#307208=CARTESIAN_POINT('Ctrl Pts',(-3.37051512400006,5.2,2.61262693699998));
#307209=CARTESIAN_POINT('Ctrl Pts',(-3.37051512400006,2.2,2.61262693699998));
#307210=CARTESIAN_POINT('Ctrl Pts',(-3.37215081000006,12.2,2.61313384499999));
#307211=CARTESIAN_POINT('Ctrl Pts',(-3.37215081000006,5.2,2.61313384499999));
#307212=CARTESIAN_POINT('Ctrl Pts',(-3.37215081000006,2.2,2.61313384499999));
#307213=CARTESIAN_POINT('Ctrl Pts',(-3.37379130200006,12.2,2.61364018799998));
#307214=CARTESIAN_POINT('Ctrl Pts',(-3.37379130200006,5.2,2.61364018799998));
#307215=CARTESIAN_POINT('Ctrl Pts',(-3.37379130200006,2.2,2.61364018799998));
#307216=CARTESIAN_POINT('Ctrl Pts',(-3.37543659900006,12.2,2.61414595499998));
#307217=CARTESIAN_POINT('Ctrl Pts',(-3.37543659900006,5.2,2.61414595499998));
#307218=CARTESIAN_POINT('Ctrl Pts',(-3.37543659900006,2.2,2.61414595499998));
#307219=CARTESIAN_POINT('Ctrl Pts',(-3.37708669500006,12.2,2.61465113699998));
#307220=CARTESIAN_POINT('Ctrl Pts',(-3.37708669500006,5.2,2.61465113699998));
#307221=CARTESIAN_POINT('Ctrl Pts',(-3.37708669500006,2.2,2.61465113699998));
#307222=CARTESIAN_POINT('Ctrl Pts',(-3.37874158300006,12.2,2.61515571999999));
#307223=CARTESIAN_POINT('Ctrl Pts',(-3.37874158300006,5.2,2.61515571999999));
#307224=CARTESIAN_POINT('Ctrl Pts',(-3.37874158300006,2.2,2.61515571999999));
#307225=CARTESIAN_POINT('Ctrl Pts',(-3.38040126000006,12.2,2.61565969399999));
#307226=CARTESIAN_POINT('Ctrl Pts',(-3.38040126000006,5.2,2.61565969399999));
#307227=CARTESIAN_POINT('Ctrl Pts',(-3.38040126000006,2.2,2.61565969399999));
#307228=CARTESIAN_POINT('Ctrl Pts',(-3.38206572100006,12.2,2.61616304899999));
#307229=CARTESIAN_POINT('Ctrl Pts',(-3.38206572100006,5.2,2.61616304899999));
#307230=CARTESIAN_POINT('Ctrl Pts',(-3.38206572100006,2.2,2.61616304899999));
#307231=CARTESIAN_POINT('Ctrl Pts',(-3.38373496000006,12.2,2.61666577199998));
#307232=CARTESIAN_POINT('Ctrl Pts',(-3.38373496000006,5.2,2.61666577199998));
#307233=CARTESIAN_POINT('Ctrl Pts',(-3.38373496000006,2.2,2.61666577199998));
#307234=CARTESIAN_POINT('Ctrl Pts',(-3.38540897300006,12.2,2.61716785299999));
#307235=CARTESIAN_POINT('Ctrl Pts',(-3.38540897300006,5.2,2.61716785299999));
#307236=CARTESIAN_POINT('Ctrl Pts',(-3.38540897300006,2.2,2.61716785299999));
#307237=CARTESIAN_POINT('Ctrl Pts',(-3.38708775500006,12.2,2.61766928299998));
#307238=CARTESIAN_POINT('Ctrl Pts',(-3.38708775500006,5.2,2.61766928299998));
#307239=CARTESIAN_POINT('Ctrl Pts',(-3.38708775500006,2.2,2.61766928299998));
#307240=CARTESIAN_POINT('Ctrl Pts',(-3.38877130000005,12.2,2.61817004799998));
#307241=CARTESIAN_POINT('Ctrl Pts',(-3.38877130000005,5.2,2.61817004799998));
#307242=CARTESIAN_POINT('Ctrl Pts',(-3.38877130000005,2.2,2.61817004799998));
#307243=CARTESIAN_POINT('Ctrl Pts',(-3.39045960500005,12.2,2.61867013699998));
#307244=CARTESIAN_POINT('Ctrl Pts',(-3.39045960500005,5.2,2.61867013699998));
#307245=CARTESIAN_POINT('Ctrl Pts',(-3.39045960500005,2.2,2.61867013699998));
#307246=CARTESIAN_POINT('Ctrl Pts',(-3.39215266200006,12.2,2.61916954299998));
#307247=CARTESIAN_POINT('Ctrl Pts',(-3.39215266200006,5.2,2.61916954299998));
#307248=CARTESIAN_POINT('Ctrl Pts',(-3.39215266200006,2.2,2.61916954299998));
#307249=CARTESIAN_POINT('Ctrl Pts',(-3.39385047000006,12.2,2.61966825099999));
#307250=CARTESIAN_POINT('Ctrl Pts',(-3.39385047000006,5.2,2.61966825099999));
#307251=CARTESIAN_POINT('Ctrl Pts',(-3.39385047000006,2.2,2.61966825099999));
#307252=CARTESIAN_POINT('Ctrl Pts',(-3.39555302000006,12.2,2.62016625199998));
#307253=CARTESIAN_POINT('Ctrl Pts',(-3.39555302000006,5.2,2.62016625199998));
#307254=CARTESIAN_POINT('Ctrl Pts',(-3.39555302000006,2.2,2.62016625199998));
#307255=CARTESIAN_POINT('Ctrl Pts',(-3.39726030900006,12.2,2.62066353399998));
#307256=CARTESIAN_POINT('Ctrl Pts',(-3.39726030900006,5.2,2.62066353399998));
#307257=CARTESIAN_POINT('Ctrl Pts',(-3.39726030900006,2.2,2.62066353399998));
#307258=CARTESIAN_POINT('Ctrl Pts',(-3.39897233300006,12.2,2.62116008899999));
#307259=CARTESIAN_POINT('Ctrl Pts',(-3.39897233300006,5.2,2.62116008899999));
#307260=CARTESIAN_POINT('Ctrl Pts',(-3.39897233300006,2.2,2.62116008899999));
#307261=CARTESIAN_POINT('Ctrl Pts',(-3.40068908500006,12.2,2.62165590199999));
#307262=CARTESIAN_POINT('Ctrl Pts',(-3.40068908500006,5.2,2.62165590199999));
#307263=CARTESIAN_POINT('Ctrl Pts',(-3.40068908500006,2.2,2.62165590199999));
#307264=CARTESIAN_POINT('Ctrl Pts',(-3.40241056000006,12.2,2.62215096699999));
#307265=CARTESIAN_POINT('Ctrl Pts',(-3.40241056000006,5.2,2.62215096699999));
#307266=CARTESIAN_POINT('Ctrl Pts',(-3.40241056000006,2.2,2.62215096699999));
#307267=CARTESIAN_POINT('Ctrl Pts',(-3.40413675500006,12.2,2.62264526799999));
#307268=CARTESIAN_POINT('Ctrl Pts',(-3.40413675500006,5.2,2.62264526799999));
#307269=CARTESIAN_POINT('Ctrl Pts',(-3.40413675500006,2.2,2.62264526799999));
#307270=CARTESIAN_POINT('Ctrl Pts',(-3.40586766300006,12.2,2.62313879999999));
#307271=CARTESIAN_POINT('Ctrl Pts',(-3.40586766300006,5.2,2.62313879999999));
#307272=CARTESIAN_POINT('Ctrl Pts',(-3.40586766300006,2.2,2.62313879999999));
#307273=CARTESIAN_POINT('Ctrl Pts',(-3.40760327900006,12.2,2.62363154799999));
#307274=CARTESIAN_POINT('Ctrl Pts',(-3.40760327900006,5.2,2.62363154799999));
#307275=CARTESIAN_POINT('Ctrl Pts',(-3.40760327900006,2.2,2.62363154799999));
#307276=CARTESIAN_POINT('Ctrl Pts',(-3.40934360000006,12.2,2.62412350299999));
#307277=CARTESIAN_POINT('Ctrl Pts',(-3.40934360000006,5.2,2.62412350299999));
#307278=CARTESIAN_POINT('Ctrl Pts',(-3.40934360000006,2.2,2.62412350299999));
#307279=CARTESIAN_POINT('Ctrl Pts',(-3.41108862000006,12.2,2.62461465499998));
#307280=CARTESIAN_POINT('Ctrl Pts',(-3.41108862000006,5.2,2.62461465499998));
#307281=CARTESIAN_POINT('Ctrl Pts',(-3.41108862000006,2.2,2.62461465499998));
#307282=CARTESIAN_POINT('Ctrl Pts',(-3.41283833100006,12.2,2.62510499299999));
#307283=CARTESIAN_POINT('Ctrl Pts',(-3.41283833100006,5.2,2.62510499299999));
#307284=CARTESIAN_POINT('Ctrl Pts',(-3.41283833100006,2.2,2.62510499299999));
#307285=CARTESIAN_POINT('Ctrl Pts',(-3.41459273300006,12.2,2.62559450499998));
#307286=CARTESIAN_POINT('Ctrl Pts',(-3.41459273300006,5.2,2.62559450499998));
#307287=CARTESIAN_POINT('Ctrl Pts',(-3.41459273300006,2.2,2.62559450499998));
#307288=CARTESIAN_POINT('Ctrl Pts',(-3.41635181700005,12.2,2.62608318199998));
#307289=CARTESIAN_POINT('Ctrl Pts',(-3.41635181700005,5.2,2.62608318199998));
#307290=CARTESIAN_POINT('Ctrl Pts',(-3.41635181700005,2.2,2.62608318199998));
#307291=CARTESIAN_POINT('Ctrl Pts',(-3.41811558000006,12.2,2.62657101299999));
#307292=CARTESIAN_POINT('Ctrl Pts',(-3.41811558000006,5.2,2.62657101299999));
#307293=CARTESIAN_POINT('Ctrl Pts',(-3.41811558000006,2.2,2.62657101299999));
#307294=CARTESIAN_POINT('Ctrl Pts',(-3.41988401600006,12.2,2.62705798799999));
#307295=CARTESIAN_POINT('Ctrl Pts',(-3.41988401600006,5.2,2.62705798799999));
#307296=CARTESIAN_POINT('Ctrl Pts',(-3.41988401600006,2.2,2.62705798799999));
#307297=CARTESIAN_POINT('Ctrl Pts',(-3.42165712000006,12.2,2.62754409599999));
#307298=CARTESIAN_POINT('Ctrl Pts',(-3.42165712000006,5.2,2.62754409599999));
#307299=CARTESIAN_POINT('Ctrl Pts',(-3.42165712000006,2.2,2.62754409599999));
#307300=CARTESIAN_POINT('Ctrl Pts',(-3.42343488700006,12.2,2.62802932799998));
#307301=CARTESIAN_POINT('Ctrl Pts',(-3.42343488700006,5.2,2.62802932799998));
#307302=CARTESIAN_POINT('Ctrl Pts',(-3.42343488700006,2.2,2.62802932799998));
#307303=CARTESIAN_POINT('Ctrl Pts',(-3.42521731200006,12.2,2.62851367099999));
#307304=CARTESIAN_POINT('Ctrl Pts',(-3.42521731200006,5.2,2.62851367099999));
#307305=CARTESIAN_POINT('Ctrl Pts',(-3.42521731200006,2.2,2.62851367099999));
#307306=CARTESIAN_POINT('Ctrl Pts',(-3.42700439000006,12.2,2.62899711699998));
#307307=CARTESIAN_POINT('Ctrl Pts',(-3.42700439000006,5.2,2.62899711699998));
#307308=CARTESIAN_POINT('Ctrl Pts',(-3.42700439000006,2.2,2.62899711699998));
#307309=CARTESIAN_POINT('Ctrl Pts',(-3.42879611600006,12.2,2.62947965299999));
#307310=CARTESIAN_POINT('Ctrl Pts',(-3.42879611600006,5.2,2.62947965299999));
#307311=CARTESIAN_POINT('Ctrl Pts',(-3.42879611600006,2.2,2.62947965299999));
#307312=CARTESIAN_POINT('Ctrl Pts',(-3.43059248500006,12.2,2.62996127199998));
#307313=CARTESIAN_POINT('Ctrl Pts',(-3.43059248500006,5.2,2.62996127199998));
#307314=CARTESIAN_POINT('Ctrl Pts',(-3.43059248500006,2.2,2.62996127199998));
#307315=CARTESIAN_POINT('Ctrl Pts',(-3.43239349100006,12.2,2.63044195999999));
#307316=CARTESIAN_POINT('Ctrl Pts',(-3.43239349100006,5.2,2.63044195999999));
#307317=CARTESIAN_POINT('Ctrl Pts',(-3.43239349100006,2.2,2.63044195999999));
#307318=CARTESIAN_POINT('Ctrl Pts',(-3.43419913000006,12.2,2.63092171099998));
#307319=CARTESIAN_POINT('Ctrl Pts',(-3.43419913000006,5.2,2.63092171099998));
#307320=CARTESIAN_POINT('Ctrl Pts',(-3.43419913000006,2.2,2.63092171099998));
#307321=CARTESIAN_POINT('Ctrl Pts',(-3.43600939600006,12.2,2.63140051199999));
#307322=CARTESIAN_POINT('Ctrl Pts',(-3.43600939600006,5.2,2.63140051199999));
#307323=CARTESIAN_POINT('Ctrl Pts',(-3.43600939600006,2.2,2.63140051199999));
#307324=CARTESIAN_POINT('Ctrl Pts',(-3.43782428400006,12.2,2.63187835199999));
#307325=CARTESIAN_POINT('Ctrl Pts',(-3.43782428400006,5.2,2.63187835199999));
#307326=CARTESIAN_POINT('Ctrl Pts',(-3.43782428400006,2.2,2.63187835199999));
#307327=CARTESIAN_POINT('Ctrl Pts',(-3.43964378900006,12.2,2.63235522299999));
#307328=CARTESIAN_POINT('Ctrl Pts',(-3.43964378900006,5.2,2.63235522299999));
#307329=CARTESIAN_POINT('Ctrl Pts',(-3.43964378900006,2.2,2.63235522299999));
#307330=CARTESIAN_POINT('Ctrl Pts',(-3.44146790600006,12.2,2.63283111299998));
#307331=CARTESIAN_POINT('Ctrl Pts',(-3.44146790600006,5.2,2.63283111299998));
#307332=CARTESIAN_POINT('Ctrl Pts',(-3.44146790600006,2.2,2.63283111299998));
#307333=CARTESIAN_POINT('Ctrl Pts',(-3.44329663000006,12.2,2.63330601399999));
#307334=CARTESIAN_POINT('Ctrl Pts',(-3.44329663000006,5.2,2.63330601399999));
#307335=CARTESIAN_POINT('Ctrl Pts',(-3.44329663000006,2.2,2.63330601399999));
#307336=CARTESIAN_POINT('Ctrl Pts',(-3.44512995600006,12.2,2.63377991399998));
#307337=CARTESIAN_POINT('Ctrl Pts',(-3.44512995600006,5.2,2.63377991399998));
#307338=CARTESIAN_POINT('Ctrl Pts',(-3.44512995600006,2.2,2.63377991399998));
#307339=CARTESIAN_POINT('Ctrl Pts',(-3.44696787800005,12.2,2.63425280299998));
#307340=CARTESIAN_POINT('Ctrl Pts',(-3.44696787800005,5.2,2.63425280299998));
#307341=CARTESIAN_POINT('Ctrl Pts',(-3.44696787800005,2.2,2.63425280299998));
#307342=CARTESIAN_POINT('Ctrl Pts',(-3.44881039100006,12.2,2.63472467199998));
#307343=CARTESIAN_POINT('Ctrl Pts',(-3.44881039100006,5.2,2.63472467199998));
#307344=CARTESIAN_POINT('Ctrl Pts',(-3.44881039100006,2.2,2.63472467199998));
#307345=CARTESIAN_POINT('Ctrl Pts',(-3.45065749100006,12.2,2.63519550999998));
#307346=CARTESIAN_POINT('Ctrl Pts',(-3.45065749100006,5.2,2.63519550999998));
#307347=CARTESIAN_POINT('Ctrl Pts',(-3.45065749100006,2.2,2.63519550999998));
#307348=CARTESIAN_POINT('Ctrl Pts',(-3.45250917200006,12.2,2.63566530699999));
#307349=CARTESIAN_POINT('Ctrl Pts',(-3.45250917200006,5.2,2.63566530699999));
#307350=CARTESIAN_POINT('Ctrl Pts',(-3.45250917200006,2.2,2.63566530699999));
#307351=CARTESIAN_POINT('Ctrl Pts',(-3.45436542900006,12.2,2.63613405299999));
#307352=CARTESIAN_POINT('Ctrl Pts',(-3.45436542900006,5.2,2.63613405299999));
#307353=CARTESIAN_POINT('Ctrl Pts',(-3.45436542900006,2.2,2.63613405299999));
#307354=CARTESIAN_POINT('Ctrl Pts',(-3.45622625500006,12.2,2.63660173899999));
#307355=CARTESIAN_POINT('Ctrl Pts',(-3.45622625500006,5.2,2.63660173899999));
#307356=CARTESIAN_POINT('Ctrl Pts',(-3.45622625500006,2.2,2.63660173899999));
#307357=CARTESIAN_POINT('Ctrl Pts',(-3.45809164800006,12.2,2.63706835399999));
#307358=CARTESIAN_POINT('Ctrl Pts',(-3.45809164800006,5.2,2.63706835399999));
#307359=CARTESIAN_POINT('Ctrl Pts',(-3.45809164800006,2.2,2.63706835399999));
#307360=CARTESIAN_POINT('Ctrl Pts',(-3.45996160100006,12.2,2.63753388799999));
#307361=CARTESIAN_POINT('Ctrl Pts',(-3.45996160100006,5.2,2.63753388799999));
#307362=CARTESIAN_POINT('Ctrl Pts',(-3.45996160100006,2.2,2.63753388799999));
#307363=CARTESIAN_POINT('Ctrl Pts',(-3.46183610800006,12.2,2.63799833099998));
#307364=CARTESIAN_POINT('Ctrl Pts',(-3.46183610800006,5.2,2.63799833099998));
#307365=CARTESIAN_POINT('Ctrl Pts',(-3.46183610800006,2.2,2.63799833099998));
#307366=CARTESIAN_POINT('Ctrl Pts',(-3.46371516600006,12.2,2.63846167499998));
#307367=CARTESIAN_POINT('Ctrl Pts',(-3.46371516600006,5.2,2.63846167499998));
#307368=CARTESIAN_POINT('Ctrl Pts',(-3.46371516600006,2.2,2.63846167499998));
#307369=CARTESIAN_POINT('Ctrl Pts',(-3.46559876800006,12.2,2.63892390799998));
#307370=CARTESIAN_POINT('Ctrl Pts',(-3.46559876800006,5.2,2.63892390799998));
#307371=CARTESIAN_POINT('Ctrl Pts',(-3.46559876800006,2.2,2.63892390799998));
#307372=CARTESIAN_POINT('Ctrl Pts',(-3.46748691000006,12.2,2.63938501999998));
#307373=CARTESIAN_POINT('Ctrl Pts',(-3.46748691000006,5.2,2.63938501999998));
#307374=CARTESIAN_POINT('Ctrl Pts',(-3.46748691000006,2.2,2.63938501999998));
#307375=CARTESIAN_POINT('Ctrl Pts',(-3.46937958700006,12.2,2.63984500299999));
#307376=CARTESIAN_POINT('Ctrl Pts',(-3.46937958700006,5.2,2.63984500299999));
#307377=CARTESIAN_POINT('Ctrl Pts',(-3.46937958700006,2.2,2.63984500299999));
#307378=CARTESIAN_POINT('Ctrl Pts',(-3.47127679100006,12.2,2.64030384499998));
#307379=CARTESIAN_POINT('Ctrl Pts',(-3.47127679100006,5.2,2.64030384499998));
#307380=CARTESIAN_POINT('Ctrl Pts',(-3.47127679100006,2.2,2.64030384499998));
#307381=CARTESIAN_POINT('Ctrl Pts',(-3.47317852100006,12.2,2.64076153799999));
#307382=CARTESIAN_POINT('Ctrl Pts',(-3.47317852100006,5.2,2.64076153799999));
#307383=CARTESIAN_POINT('Ctrl Pts',(-3.47317852100006,2.2,2.64076153799999));
#307384=CARTESIAN_POINT('Ctrl Pts',(-3.47508476800006,12.2,2.64121807199999));
#307385=CARTESIAN_POINT('Ctrl Pts',(-3.47508476800006,5.2,2.64121807199999));
#307386=CARTESIAN_POINT('Ctrl Pts',(-3.47508476800006,2.2,2.64121807199999));
#307387=CARTESIAN_POINT('Ctrl Pts',(-3.47699552900006,12.2,2.64167343599999));
#307388=CARTESIAN_POINT('Ctrl Pts',(-3.47699552900006,5.2,2.64167343599999));
#307389=CARTESIAN_POINT('Ctrl Pts',(-3.47699552900006,2.2,2.64167343599999));
#307390=CARTESIAN_POINT('Ctrl Pts',(-3.47891079800006,12.2,2.64212762199998));
#307391=CARTESIAN_POINT('Ctrl Pts',(-3.47891079800006,5.2,2.64212762199998));
#307392=CARTESIAN_POINT('Ctrl Pts',(-3.47891079800006,2.2,2.64212762199998));
#307393=CARTESIAN_POINT('Ctrl Pts',(-3.48083056900006,12.2,2.64258061899999));
#307394=CARTESIAN_POINT('Ctrl Pts',(-3.48083056900006,5.2,2.64258061899999));
#307395=CARTESIAN_POINT('Ctrl Pts',(-3.48083056900006,2.2,2.64258061899999));
#307396=CARTESIAN_POINT('Ctrl Pts',(-3.48275483900006,12.2,2.64303241699999));
#307397=CARTESIAN_POINT('Ctrl Pts',(-3.48275483900006,5.2,2.64303241699999));
#307398=CARTESIAN_POINT('Ctrl Pts',(-3.48275483900006,2.2,2.64303241699999));
#307399=CARTESIAN_POINT('Ctrl Pts',(-3.48468360100005,12.2,2.64348300799998));
#307400=CARTESIAN_POINT('Ctrl Pts',(-3.48468360100005,5.2,2.64348300799998));
#307401=CARTESIAN_POINT('Ctrl Pts',(-3.48468360100005,2.2,2.64348300799998));
#307402=CARTESIAN_POINT('Ctrl Pts',(-3.48661684900006,12.2,2.64393238199998));
#307403=CARTESIAN_POINT('Ctrl Pts',(-3.48661684900006,5.2,2.64393238199998));
#307404=CARTESIAN_POINT('Ctrl Pts',(-3.48661684900006,2.2,2.64393238199998));
#307405=CARTESIAN_POINT('Ctrl Pts',(-3.48855458000005,12.2,2.64438052799999));
#307406=CARTESIAN_POINT('Ctrl Pts',(-3.48855458000005,5.2,2.64438052799999));
#307407=CARTESIAN_POINT('Ctrl Pts',(-3.48855458000005,2.2,2.64438052799999));
#307408=CARTESIAN_POINT('Ctrl Pts',(-3.49049678700006,12.2,2.64482743799999));
#307409=CARTESIAN_POINT('Ctrl Pts',(-3.49049678700006,5.2,2.64482743799999));
#307410=CARTESIAN_POINT('Ctrl Pts',(-3.49049678700006,2.2,2.64482743799999));
#307411=CARTESIAN_POINT('Ctrl Pts',(-3.49244346600006,12.2,2.64527310199998));
#307412=CARTESIAN_POINT('Ctrl Pts',(-3.49244346600006,5.2,2.64527310199998));
#307413=CARTESIAN_POINT('Ctrl Pts',(-3.49244346600006,2.2,2.64527310199998));
#307414=CARTESIAN_POINT('Ctrl Pts',(-3.49439461000005,12.2,2.64571750999998));
#307415=CARTESIAN_POINT('Ctrl Pts',(-3.49439461000005,5.2,2.64571750999998));
#307416=CARTESIAN_POINT('Ctrl Pts',(-3.49439461000005,2.2,2.64571750999998));
#307417=CARTESIAN_POINT('Ctrl Pts',(-3.49635021500006,12.2,2.64616065299998));
#307418=CARTESIAN_POINT('Ctrl Pts',(-3.49635021500006,5.2,2.64616065299998));
#307419=CARTESIAN_POINT('Ctrl Pts',(-3.49635021500006,2.2,2.64616065299998));
#307420=CARTESIAN_POINT('Ctrl Pts',(-3.49831027600006,12.2,2.64660251999998));
#307421=CARTESIAN_POINT('Ctrl Pts',(-3.49831027600006,5.2,2.64660251999998));
#307422=CARTESIAN_POINT('Ctrl Pts',(-3.49831027600006,2.2,2.64660251999998));
#307423=CARTESIAN_POINT('Ctrl Pts',(-3.50027478700006,12.2,2.64704310399999));
#307424=CARTESIAN_POINT('Ctrl Pts',(-3.50027478700006,5.2,2.64704310399999));
#307425=CARTESIAN_POINT('Ctrl Pts',(-3.50027478700006,2.2,2.64704310399999));
#307426=CARTESIAN_POINT('Ctrl Pts',(-3.50224374300006,12.2,2.64748239399999));
#307427=CARTESIAN_POINT('Ctrl Pts',(-3.50224374300006,5.2,2.64748239399999));
#307428=CARTESIAN_POINT('Ctrl Pts',(-3.50224374300006,2.2,2.64748239399999));
#307429=CARTESIAN_POINT('Ctrl Pts',(-3.50421713800006,12.2,2.64792038099999));
#307430=CARTESIAN_POINT('Ctrl Pts',(-3.50421713800006,5.2,2.64792038099999));
#307431=CARTESIAN_POINT('Ctrl Pts',(-3.50421713800006,2.2,2.64792038099999));
#307432=CARTESIAN_POINT('Ctrl Pts',(-3.50619496700006,12.2,2.64835705499999));
#307433=CARTESIAN_POINT('Ctrl Pts',(-3.50619496700006,5.2,2.64835705499999));
#307434=CARTESIAN_POINT('Ctrl Pts',(-3.50619496700006,2.2,2.64835705499999));
#307435=CARTESIAN_POINT('Ctrl Pts',(-3.50817722600006,12.2,2.64879240799999));
#307436=CARTESIAN_POINT('Ctrl Pts',(-3.50817722600006,5.2,2.64879240799999));
#307437=CARTESIAN_POINT('Ctrl Pts',(-3.50817722600006,2.2,2.64879240799999));
#307438=CARTESIAN_POINT('Ctrl Pts',(-3.51016390800006,12.2,2.64922642899998));
#307439=CARTESIAN_POINT('Ctrl Pts',(-3.51016390800006,5.2,2.64922642899998));
#307440=CARTESIAN_POINT('Ctrl Pts',(-3.51016390800006,2.2,2.64922642899998));
#307441=CARTESIAN_POINT('Ctrl Pts',(-3.51215500900006,12.2,2.64965911099999));
#307442=CARTESIAN_POINT('Ctrl Pts',(-3.51215500900006,5.2,2.64965911099999));
#307443=CARTESIAN_POINT('Ctrl Pts',(-3.51215500900006,2.2,2.64965911099999));
#307444=CARTESIAN_POINT('Ctrl Pts',(-3.51415052200006,12.2,2.65009044199999));
#307445=CARTESIAN_POINT('Ctrl Pts',(-3.51415052200006,5.2,2.65009044199999));
#307446=CARTESIAN_POINT('Ctrl Pts',(-3.51415052200006,2.2,2.65009044199999));
#307447=CARTESIAN_POINT('Ctrl Pts',(-3.51615044300006,12.2,2.65052041399999));
#307448=CARTESIAN_POINT('Ctrl Pts',(-3.51615044300006,5.2,2.65052041399999));
#307449=CARTESIAN_POINT('Ctrl Pts',(-3.51615044300006,2.2,2.65052041399999));
#307450=CARTESIAN_POINT('Ctrl Pts',(-3.51815476700006,12.2,2.65094901799999));
#307451=CARTESIAN_POINT('Ctrl Pts',(-3.51815476700006,5.2,2.65094901799999));
#307452=CARTESIAN_POINT('Ctrl Pts',(-3.51815476700006,2.2,2.65094901799999));
#307453=CARTESIAN_POINT('Ctrl Pts',(-3.52016348700006,12.2,2.65137624399999));
#307454=CARTESIAN_POINT('Ctrl Pts',(-3.52016348700006,5.2,2.65137624399999));
#307455=CARTESIAN_POINT('Ctrl Pts',(-3.52016348700006,2.2,2.65137624399999));
#307456=CARTESIAN_POINT('Ctrl Pts',(-3.52217659900006,12.2,2.65180208299999));
#307457=CARTESIAN_POINT('Ctrl Pts',(-3.52217659900006,5.2,2.65180208299999));
#307458=CARTESIAN_POINT('Ctrl Pts',(-3.52217659900006,2.2,2.65180208299999));
#307459=CARTESIAN_POINT('Ctrl Pts',(-3.52419409800006,12.2,2.65222652599999));
#307460=CARTESIAN_POINT('Ctrl Pts',(-3.52419409800006,5.2,2.65222652599999));
#307461=CARTESIAN_POINT('Ctrl Pts',(-3.52419409800006,2.2,2.65222652599999));
#307462=CARTESIAN_POINT('Ctrl Pts',(-3.52621597700006,12.2,2.65264956399999));
#307463=CARTESIAN_POINT('Ctrl Pts',(-3.52621597700006,5.2,2.65264956399999));
#307464=CARTESIAN_POINT('Ctrl Pts',(-3.52621597700006,2.2,2.65264956399999));
#307465=CARTESIAN_POINT('Ctrl Pts',(-3.52824223300006,12.2,2.65307118699998));
#307466=CARTESIAN_POINT('Ctrl Pts',(-3.52824223300006,5.2,2.65307118699998));
#307467=CARTESIAN_POINT('Ctrl Pts',(-3.52824223300006,2.2,2.65307118699998));
#307468=CARTESIAN_POINT('Ctrl Pts',(-3.53027285800006,12.2,2.65349138699998));
#307469=CARTESIAN_POINT('Ctrl Pts',(-3.53027285800006,5.2,2.65349138699998));
#307470=CARTESIAN_POINT('Ctrl Pts',(-3.53027285800006,2.2,2.65349138699998));
#307471=CARTESIAN_POINT('Ctrl Pts',(-3.53230784800005,12.2,2.65391015399998));
#307472=CARTESIAN_POINT('Ctrl Pts',(-3.53230784800005,5.2,2.65391015399998));
#307473=CARTESIAN_POINT('Ctrl Pts',(-3.53230784800005,2.2,2.65391015399998));
#307474=CARTESIAN_POINT('Ctrl Pts',(-3.53434719800005,12.2,2.65432747999998));
#307475=CARTESIAN_POINT('Ctrl Pts',(-3.53434719800005,5.2,2.65432747999998));
#307476=CARTESIAN_POINT('Ctrl Pts',(-3.53434719800005,2.2,2.65432747999998));
#307477=CARTESIAN_POINT('Ctrl Pts',(-3.53639090200006,12.2,2.65474335499999));
#307478=CARTESIAN_POINT('Ctrl Pts',(-3.53639090200006,5.2,2.65474335499999));
#307479=CARTESIAN_POINT('Ctrl Pts',(-3.53639090200006,2.2,2.65474335499999));
#307480=CARTESIAN_POINT('Ctrl Pts',(-3.53843895500006,12.2,2.65515776899999));
#307481=CARTESIAN_POINT('Ctrl Pts',(-3.53843895500006,5.2,2.65515776899999));
#307482=CARTESIAN_POINT('Ctrl Pts',(-3.53843895500006,2.2,2.65515776899999));
#307483=CARTESIAN_POINT('Ctrl Pts',(-3.54049135100006,12.2,2.65557071499998));
#307484=CARTESIAN_POINT('Ctrl Pts',(-3.54049135100006,5.2,2.65557071499998));
#307485=CARTESIAN_POINT('Ctrl Pts',(-3.54049135100006,2.2,2.65557071499998));
#307486=CARTESIAN_POINT('Ctrl Pts',(-3.54254808600006,12.2,2.65598218399998));
#307487=CARTESIAN_POINT('Ctrl Pts',(-3.54254808600006,5.2,2.65598218399998));
#307488=CARTESIAN_POINT('Ctrl Pts',(-3.54254808600006,2.2,2.65598218399998));
#307489=CARTESIAN_POINT('Ctrl Pts',(-3.54460915300006,12.2,2.65639216399999));
#307490=CARTESIAN_POINT('Ctrl Pts',(-3.54460915300006,5.2,2.65639216399999));
#307491=CARTESIAN_POINT('Ctrl Pts',(-3.54460915300006,2.2,2.65639216399999));
#307492=CARTESIAN_POINT('Ctrl Pts',(-3.54667454700006,12.2,2.65680064999999));
#307493=CARTESIAN_POINT('Ctrl Pts',(-3.54667454700006,5.2,2.65680064999999));
#307494=CARTESIAN_POINT('Ctrl Pts',(-3.54667454700006,2.2,2.65680064999999));
#307495=CARTESIAN_POINT('Ctrl Pts',(-3.54874426400006,12.2,2.65720763099999));
#307496=CARTESIAN_POINT('Ctrl Pts',(-3.54874426400006,5.2,2.65720763099999));
#307497=CARTESIAN_POINT('Ctrl Pts',(-3.54874426400006,2.2,2.65720763099999));
#307498=CARTESIAN_POINT('Ctrl Pts',(-3.55081829600006,12.2,2.65761309799998));
#307499=CARTESIAN_POINT('Ctrl Pts',(-3.55081829600006,5.2,2.65761309799998));
#307500=CARTESIAN_POINT('Ctrl Pts',(-3.55081829600006,2.2,2.65761309799998));
#307501=CARTESIAN_POINT('Ctrl Pts',(-3.55289663900006,12.2,2.65801704099999));
#307502=CARTESIAN_POINT('Ctrl Pts',(-3.55289663900006,5.2,2.65801704099999));
#307503=CARTESIAN_POINT('Ctrl Pts',(-3.55289663900006,2.2,2.65801704099999));
#307504=CARTESIAN_POINT('Ctrl Pts',(-3.55497929000006,12.2,2.65841945399998));
#307505=CARTESIAN_POINT('Ctrl Pts',(-3.55497929000006,5.2,2.65841945399998));
#307506=CARTESIAN_POINT('Ctrl Pts',(-3.55497929000006,2.2,2.65841945399998));
#307507=CARTESIAN_POINT('Ctrl Pts',(-3.55706623900006,12.2,2.65882032599999));
#307508=CARTESIAN_POINT('Ctrl Pts',(-3.55706623900006,5.2,2.65882032599999));
#307509=CARTESIAN_POINT('Ctrl Pts',(-3.55706623900006,2.2,2.65882032599999));
#307510=CARTESIAN_POINT('Ctrl Pts',(-3.55915748400006,12.2,2.65921964999999));
#307511=CARTESIAN_POINT('Ctrl Pts',(-3.55915748400006,5.2,2.65921964999999));
#307512=CARTESIAN_POINT('Ctrl Pts',(-3.55915748400006,2.2,2.65921964999999));
#307513=CARTESIAN_POINT('Ctrl Pts',(-3.56125301800006,12.2,2.65961741499999));
#307514=CARTESIAN_POINT('Ctrl Pts',(-3.56125301800006,5.2,2.65961741499999));
#307515=CARTESIAN_POINT('Ctrl Pts',(-3.56125301800006,2.2,2.65961741499999));
#307516=CARTESIAN_POINT('Ctrl Pts',(-3.56335283600006,12.2,2.66001361199999));
#307517=CARTESIAN_POINT('Ctrl Pts',(-3.56335283600006,5.2,2.66001361199999));
#307518=CARTESIAN_POINT('Ctrl Pts',(-3.56335283600006,2.2,2.66001361199999));
#307519=CARTESIAN_POINT('Ctrl Pts',(-3.56545693200006,12.2,2.66040823499999));
#307520=CARTESIAN_POINT('Ctrl Pts',(-3.56545693200006,5.2,2.66040823499999));
#307521=CARTESIAN_POINT('Ctrl Pts',(-3.56545693200006,2.2,2.66040823499999));
#307522=CARTESIAN_POINT('Ctrl Pts',(-3.56756530200006,12.2,2.66080127299999));
#307523=CARTESIAN_POINT('Ctrl Pts',(-3.56756530200006,5.2,2.66080127299999));
#307524=CARTESIAN_POINT('Ctrl Pts',(-3.56756530200006,2.2,2.66080127299999));
#307525=CARTESIAN_POINT('Ctrl Pts',(-3.56967794000006,12.2,2.66119271799998));
#307526=CARTESIAN_POINT('Ctrl Pts',(-3.56967794000006,5.2,2.66119271799998));
#307527=CARTESIAN_POINT('Ctrl Pts',(-3.56967794000006,2.2,2.66119271799998));
#307528=CARTESIAN_POINT('Ctrl Pts',(-3.57179484000006,12.2,2.66158256099998));
#307529=CARTESIAN_POINT('Ctrl Pts',(-3.57179484000006,5.2,2.66158256099998));
#307530=CARTESIAN_POINT('Ctrl Pts',(-3.57179484000006,2.2,2.66158256099998));
#307531=CARTESIAN_POINT('Ctrl Pts',(-3.57391599700006,12.2,2.66197079399999));
#307532=CARTESIAN_POINT('Ctrl Pts',(-3.57391599700006,5.2,2.66197079399999));
#307533=CARTESIAN_POINT('Ctrl Pts',(-3.57391599700006,2.2,2.66197079399999));
#307534=CARTESIAN_POINT('Ctrl Pts',(-3.57604140400006,12.2,2.66235740799999));
#307535=CARTESIAN_POINT('Ctrl Pts',(-3.57604140400006,5.2,2.66235740799999));
#307536=CARTESIAN_POINT('Ctrl Pts',(-3.57604140400006,2.2,2.66235740799999));
#307537=CARTESIAN_POINT('Ctrl Pts',(-3.57817105900006,12.2,2.66274239199999));
#307538=CARTESIAN_POINT('Ctrl Pts',(-3.57817105900006,5.2,2.66274239199999));
#307539=CARTESIAN_POINT('Ctrl Pts',(-3.57817105900006,2.2,2.66274239199999));
#307540=CARTESIAN_POINT('Ctrl Pts',(-3.58030495300006,12.2,2.66312574099998));
#307541=CARTESIAN_POINT('Ctrl Pts',(-3.58030495300006,5.2,2.66312574099998));
#307542=CARTESIAN_POINT('Ctrl Pts',(-3.58030495300006,2.2,2.66312574099998));
#307543=CARTESIAN_POINT('Ctrl Pts',(-3.58244308300006,12.2,2.66350744499999));
#307544=CARTESIAN_POINT('Ctrl Pts',(-3.58244308300006,5.2,2.66350744499999));
#307545=CARTESIAN_POINT('Ctrl Pts',(-3.58244308300006,2.2,2.66350744499999));
#307546=CARTESIAN_POINT('Ctrl Pts',(-3.58458544200006,12.2,2.66388749499999));
#307547=CARTESIAN_POINT('Ctrl Pts',(-3.58458544200006,5.2,2.66388749499999));
#307548=CARTESIAN_POINT('Ctrl Pts',(-3.58458544200006,2.2,2.66388749499999));
#307549=CARTESIAN_POINT('Ctrl Pts',(-3.58673202600006,12.2,2.66426588299999));
#307550=CARTESIAN_POINT('Ctrl Pts',(-3.58673202600006,5.2,2.66426588299999));
#307551=CARTESIAN_POINT('Ctrl Pts',(-3.58673202600006,2.2,2.66426588299999));
#307552=CARTESIAN_POINT('Ctrl Pts',(-3.58888282800006,12.2,2.66464259999999));
#307553=CARTESIAN_POINT('Ctrl Pts',(-3.58888282800006,5.2,2.66464259999999));
#307554=CARTESIAN_POINT('Ctrl Pts',(-3.58888282800006,2.2,2.66464259999999));
#307555=CARTESIAN_POINT('Ctrl Pts',(-3.59103784200006,12.2,2.66501763699999));
#307556=CARTESIAN_POINT('Ctrl Pts',(-3.59103784200006,5.2,2.66501763699999));
#307557=CARTESIAN_POINT('Ctrl Pts',(-3.59103784200006,2.2,2.66501763699999));
#307558=CARTESIAN_POINT('Ctrl Pts',(-3.59319706600005,12.2,2.66539098699998));
#307559=CARTESIAN_POINT('Ctrl Pts',(-3.59319706600005,5.2,2.66539098699998));
#307560=CARTESIAN_POINT('Ctrl Pts',(-3.59319706600005,2.2,2.66539098699998));
#307561=CARTESIAN_POINT('Ctrl Pts',(-3.59536049100006,12.2,2.66576263999998));
#307562=CARTESIAN_POINT('Ctrl Pts',(-3.59536049100006,5.2,2.66576263999998));
#307563=CARTESIAN_POINT('Ctrl Pts',(-3.59536049100006,2.2,2.66576263999998));
#307564=CARTESIAN_POINT('Ctrl Pts',(-3.59752811200006,12.2,2.66613258799998));
#307565=CARTESIAN_POINT('Ctrl Pts',(-3.59752811200006,5.2,2.66613258799998));
#307566=CARTESIAN_POINT('Ctrl Pts',(-3.59752811200006,2.2,2.66613258799998));
#307567=CARTESIAN_POINT('Ctrl Pts',(-3.59969992500006,12.2,2.66650082299999));
#307568=CARTESIAN_POINT('Ctrl Pts',(-3.59969992500006,5.2,2.66650082299999));
#307569=CARTESIAN_POINT('Ctrl Pts',(-3.59969992500006,2.2,2.66650082299999));
#307570=CARTESIAN_POINT('Ctrl Pts',(-3.60187592400006,12.2,2.66686733599999));
#307571=CARTESIAN_POINT('Ctrl Pts',(-3.60187592400006,5.2,2.66686733599999));
#307572=CARTESIAN_POINT('Ctrl Pts',(-3.60187592400006,2.2,2.66686733599999));
#307573=CARTESIAN_POINT('Ctrl Pts',(-3.60405610400006,12.2,2.66723211899999));
#307574=CARTESIAN_POINT('Ctrl Pts',(-3.60405610400006,5.2,2.66723211899999));
#307575=CARTESIAN_POINT('Ctrl Pts',(-3.60405610400006,2.2,2.66723211899999));
#307576=CARTESIAN_POINT('Ctrl Pts',(-3.60624045800006,12.2,2.66759516299999));
#307577=CARTESIAN_POINT('Ctrl Pts',(-3.60624045800006,5.2,2.66759516299999));
#307578=CARTESIAN_POINT('Ctrl Pts',(-3.60624045800006,2.2,2.66759516299999));
#307579=CARTESIAN_POINT('Ctrl Pts',(-3.60842898100006,12.2,2.66795645999998));
#307580=CARTESIAN_POINT('Ctrl Pts',(-3.60842898100006,5.2,2.66795645999998));
#307581=CARTESIAN_POINT('Ctrl Pts',(-3.60842898100006,2.2,2.66795645999998));
#307582=CARTESIAN_POINT('Ctrl Pts',(-3.61062166800005,12.2,2.66831600199998));
#307583=CARTESIAN_POINT('Ctrl Pts',(-3.61062166800005,5.2,2.66831600199998));
#307584=CARTESIAN_POINT('Ctrl Pts',(-3.61062166800005,2.2,2.66831600199998));
#307585=CARTESIAN_POINT('Ctrl Pts',(-3.61281851300006,12.2,2.66867377999999));
#307586=CARTESIAN_POINT('Ctrl Pts',(-3.61281851300006,5.2,2.66867377999999));
#307587=CARTESIAN_POINT('Ctrl Pts',(-3.61281851300006,2.2,2.66867377999999));
#307588=CARTESIAN_POINT('Ctrl Pts',(-3.61501951100006,12.2,2.66902978699999));
#307589=CARTESIAN_POINT('Ctrl Pts',(-3.61501951100006,5.2,2.66902978699999));
#307590=CARTESIAN_POINT('Ctrl Pts',(-3.61501951100006,2.2,2.66902978699999));
#307591=CARTESIAN_POINT('Ctrl Pts',(-3.61722465600006,12.2,2.66938401199998));
#307592=CARTESIAN_POINT('Ctrl Pts',(-3.61722465600006,5.2,2.66938401199998));
#307593=CARTESIAN_POINT('Ctrl Pts',(-3.61722465600006,2.2,2.66938401199998));
#307594=CARTESIAN_POINT('Ctrl Pts',(-3.61943394400006,12.2,2.66973644999998));
#307595=CARTESIAN_POINT('Ctrl Pts',(-3.61943394400006,5.2,2.66973644999998));
#307596=CARTESIAN_POINT('Ctrl Pts',(-3.61943394400006,2.2,2.66973644999998));
#307597=CARTESIAN_POINT('Ctrl Pts',(-3.62164736600006,12.2,2.67008708999998));
#307598=CARTESIAN_POINT('Ctrl Pts',(-3.62164736600006,5.2,2.67008708999998));
#307599=CARTESIAN_POINT('Ctrl Pts',(-3.62164736600006,2.2,2.67008708999998));
#307600=CARTESIAN_POINT('Ctrl Pts',(-3.62386492100006,12.2,2.67043592499999));
#307601=CARTESIAN_POINT('Ctrl Pts',(-3.62386492100006,5.2,2.67043592499999));
#307602=CARTESIAN_POINT('Ctrl Pts',(-3.62386492100006,2.2,2.67043592499999));
#307603=CARTESIAN_POINT('Ctrl Pts',(-3.62608660000006,12.2,2.67078294699999));
#307604=CARTESIAN_POINT('Ctrl Pts',(-3.62608660000006,5.2,2.67078294699999));
#307605=CARTESIAN_POINT('Ctrl Pts',(-3.62608660000006,2.2,2.67078294699999));
#307606=CARTESIAN_POINT('Ctrl Pts',(-3.62831239800006,12.2,2.67112814699999));
#307607=CARTESIAN_POINT('Ctrl Pts',(-3.62831239800006,5.2,2.67112814699999));
#307608=CARTESIAN_POINT('Ctrl Pts',(-3.62831239800006,2.2,2.67112814699999));
#307609=CARTESIAN_POINT('Ctrl Pts',(-3.63054231100006,12.2,2.67147151799998));
#307610=CARTESIAN_POINT('Ctrl Pts',(-3.63054231100006,5.2,2.67147151799998));
#307611=CARTESIAN_POINT('Ctrl Pts',(-3.63054231100006,2.2,2.67147151799998));
#307612=CARTESIAN_POINT('Ctrl Pts',(-3.63277633200005,12.2,2.67181304999998));
#307613=CARTESIAN_POINT('Ctrl Pts',(-3.63277633200005,5.2,2.67181304999998));
#307614=CARTESIAN_POINT('Ctrl Pts',(-3.63277633200005,2.2,2.67181304999998));
#307615=CARTESIAN_POINT('Ctrl Pts',(-3.63501445700006,12.2,2.67215273699998));
#307616=CARTESIAN_POINT('Ctrl Pts',(-3.63501445700006,5.2,2.67215273699998));
#307617=CARTESIAN_POINT('Ctrl Pts',(-3.63501445700006,2.2,2.67215273699998));
#307618=CARTESIAN_POINT('Ctrl Pts',(-3.63725667900006,12.2,2.67249056999999));
#307619=CARTESIAN_POINT('Ctrl Pts',(-3.63725667900006,5.2,2.67249056999999));
#307620=CARTESIAN_POINT('Ctrl Pts',(-3.63725667900006,2.2,2.67249056999999));
#307621=CARTESIAN_POINT('Ctrl Pts',(-3.63950299200006,12.2,2.67282653999998));
#307622=CARTESIAN_POINT('Ctrl Pts',(-3.63950299200006,5.2,2.67282653999998));
#307623=CARTESIAN_POINT('Ctrl Pts',(-3.63950299200006,2.2,2.67282653999998));
#307624=CARTESIAN_POINT('Ctrl Pts',(-3.64175339200006,12.2,2.67316064099998));
#307625=CARTESIAN_POINT('Ctrl Pts',(-3.64175339200006,5.2,2.67316064099998));
#307626=CARTESIAN_POINT('Ctrl Pts',(-3.64175339200006,2.2,2.67316064099998));
#307627=CARTESIAN_POINT('Ctrl Pts',(-3.64400787400006,12.2,2.67349286199998));
#307628=CARTESIAN_POINT('Ctrl Pts',(-3.64400787400006,5.2,2.67349286199998));
#307629=CARTESIAN_POINT('Ctrl Pts',(-3.64400787400006,2.2,2.67349286199998));
#307630=CARTESIAN_POINT('Ctrl Pts',(-3.64626642900006,12.2,2.67382319699998));
#307631=CARTESIAN_POINT('Ctrl Pts',(-3.64626642900006,5.2,2.67382319699998));
#307632=CARTESIAN_POINT('Ctrl Pts',(-3.64626642900006,2.2,2.67382319699998));
#307633=CARTESIAN_POINT('Ctrl Pts',(-3.64852905500006,12.2,2.67415163699999));
#307634=CARTESIAN_POINT('Ctrl Pts',(-3.64852905500006,5.2,2.67415163699999));
#307635=CARTESIAN_POINT('Ctrl Pts',(-3.64852905500006,2.2,2.67415163699999));
#307636=CARTESIAN_POINT('Ctrl Pts',(-3.65079574500006,12.2,2.67447817499999));
#307637=CARTESIAN_POINT('Ctrl Pts',(-3.65079574500006,5.2,2.67447817499999));
#307638=CARTESIAN_POINT('Ctrl Pts',(-3.65079574500006,2.2,2.67447817499999));
#307639=CARTESIAN_POINT('Ctrl Pts',(-3.65306649300006,12.2,2.67480280299999));
#307640=CARTESIAN_POINT('Ctrl Pts',(-3.65306649300006,5.2,2.67480280299999));
#307641=CARTESIAN_POINT('Ctrl Pts',(-3.65306649300006,2.2,2.67480280299999));
#307642=CARTESIAN_POINT('Ctrl Pts',(-3.65534129500006,12.2,2.67512551199999));
#307643=CARTESIAN_POINT('Ctrl Pts',(-3.65534129500006,5.2,2.67512551199999));
#307644=CARTESIAN_POINT('Ctrl Pts',(-3.65534129500006,2.2,2.67512551199999));
#307645=CARTESIAN_POINT('Ctrl Pts',(-3.65762014400006,12.2,2.67544629399998));
#307646=CARTESIAN_POINT('Ctrl Pts',(-3.65762014400006,5.2,2.67544629399998));
#307647=CARTESIAN_POINT('Ctrl Pts',(-3.65762014400006,2.2,2.67544629399998));
#307648=CARTESIAN_POINT('Ctrl Pts',(-3.65990303400006,12.2,2.67576514099999));
#307649=CARTESIAN_POINT('Ctrl Pts',(-3.65990303400006,5.2,2.67576514099999));
#307650=CARTESIAN_POINT('Ctrl Pts',(-3.65990303400006,2.2,2.67576514099999));
#307651=CARTESIAN_POINT('Ctrl Pts',(-3.66218996100006,12.2,2.67608204699999));
#307652=CARTESIAN_POINT('Ctrl Pts',(-3.66218996100006,5.2,2.67608204699999));
#307653=CARTESIAN_POINT('Ctrl Pts',(-3.66218996100006,2.2,2.67608204699999));
#307654=CARTESIAN_POINT('Ctrl Pts',(-3.66448091900006,12.2,2.67639700199998));
#307655=CARTESIAN_POINT('Ctrl Pts',(-3.66448091900006,5.2,2.67639700199998));
#307656=CARTESIAN_POINT('Ctrl Pts',(-3.66448091900006,2.2,2.67639700199998));
#307657=CARTESIAN_POINT('Ctrl Pts',(-3.66677590100006,12.2,2.67670999999999));
#307658=CARTESIAN_POINT('Ctrl Pts',(-3.66677590100006,5.2,2.67670999999999));
#307659=CARTESIAN_POINT('Ctrl Pts',(-3.66677590100006,2.2,2.67670999999999));
#307660=CARTESIAN_POINT('Ctrl Pts',(-3.66907490300005,12.2,2.67702103099998));
#307661=CARTESIAN_POINT('Ctrl Pts',(-3.66907490300005,5.2,2.67702103099998));
#307662=CARTESIAN_POINT('Ctrl Pts',(-3.66907490300005,2.2,2.67702103099998));
#307663=CARTESIAN_POINT('Ctrl Pts',(-3.67137791900006,12.2,2.67733008799999));
#307664=CARTESIAN_POINT('Ctrl Pts',(-3.67137791900006,5.2,2.67733008799999));
#307665=CARTESIAN_POINT('Ctrl Pts',(-3.67137791900006,2.2,2.67733008799999));
#307666=CARTESIAN_POINT('Ctrl Pts',(-3.67368494300006,12.2,2.67763716499999));
#307667=CARTESIAN_POINT('Ctrl Pts',(-3.67368494300006,5.2,2.67763716499999));
#307668=CARTESIAN_POINT('Ctrl Pts',(-3.67368494300006,2.2,2.67763716499999));
#307669=CARTESIAN_POINT('Ctrl Pts',(-3.67599597000006,12.2,2.67794225099999));
#307670=CARTESIAN_POINT('Ctrl Pts',(-3.67599597000006,5.2,2.67794225099999));
#307671=CARTESIAN_POINT('Ctrl Pts',(-3.67599597000006,2.2,2.67794225099999));
#307672=CARTESIAN_POINT('Ctrl Pts',(-3.67831099400005,12.2,2.67824533899999));
#307673=CARTESIAN_POINT('Ctrl Pts',(-3.67831099400005,5.2,2.67824533899999));
#307674=CARTESIAN_POINT('Ctrl Pts',(-3.67831099400005,2.2,2.67824533899999));
#307675=CARTESIAN_POINT('Ctrl Pts',(-3.68063001000006,12.2,2.67854642399998));
#307676=CARTESIAN_POINT('Ctrl Pts',(-3.68063001000006,5.2,2.67854642399998));
#307677=CARTESIAN_POINT('Ctrl Pts',(-3.68063001000006,2.2,2.67854642399998));
#307678=CARTESIAN_POINT('Ctrl Pts',(-3.68295301100006,12.2,2.67884549499998));
#307679=CARTESIAN_POINT('Ctrl Pts',(-3.68295301100006,5.2,2.67884549499998));
#307680=CARTESIAN_POINT('Ctrl Pts',(-3.68295301100006,2.2,2.67884549499998));
#307681=CARTESIAN_POINT('Ctrl Pts',(-3.68527999200006,12.2,2.67914254499999));
#307682=CARTESIAN_POINT('Ctrl Pts',(-3.68527999200006,5.2,2.67914254499999));
#307683=CARTESIAN_POINT('Ctrl Pts',(-3.68527999200006,2.2,2.67914254499999));
#307684=CARTESIAN_POINT('Ctrl Pts',(-3.68761094800006,12.2,2.67943756799998));
#307685=CARTESIAN_POINT('Ctrl Pts',(-3.68761094800006,5.2,2.67943756799998));
#307686=CARTESIAN_POINT('Ctrl Pts',(-3.68761094800006,2.2,2.67943756799998));
#307687=CARTESIAN_POINT('Ctrl Pts',(-3.68994587300006,12.2,2.67973055399998));
#307688=CARTESIAN_POINT('Ctrl Pts',(-3.68994587300006,5.2,2.67973055399998));
#307689=CARTESIAN_POINT('Ctrl Pts',(-3.68994587300006,2.2,2.67973055399998));
#307690=CARTESIAN_POINT('Ctrl Pts',(-3.69228476200006,12.2,2.68002149699999));
#307691=CARTESIAN_POINT('Ctrl Pts',(-3.69228476200006,5.2,2.68002149699999));
#307692=CARTESIAN_POINT('Ctrl Pts',(-3.69228476200006,2.2,2.68002149699999));
#307693=CARTESIAN_POINT('Ctrl Pts',(-3.69462760800006,12.2,2.68031038799998));
#307694=CARTESIAN_POINT('Ctrl Pts',(-3.69462760800006,5.2,2.68031038799998));
#307695=CARTESIAN_POINT('Ctrl Pts',(-3.69462760800006,2.2,2.68031038799998));
#307696=CARTESIAN_POINT('Ctrl Pts',(-3.69697440600006,12.2,2.68059721999999));
#307697=CARTESIAN_POINT('Ctrl Pts',(-3.69697440600006,5.2,2.68059721999999));
#307698=CARTESIAN_POINT('Ctrl Pts',(-3.69697440600006,2.2,2.68059721999999));
#307699=CARTESIAN_POINT('Ctrl Pts',(-3.69932515100006,12.2,2.68088198699999));
#307700=CARTESIAN_POINT('Ctrl Pts',(-3.69932515100006,5.2,2.68088198699999));
#307701=CARTESIAN_POINT('Ctrl Pts',(-3.69932515100006,2.2,2.68088198699999));
#307702=CARTESIAN_POINT('Ctrl Pts',(-3.70167983700005,12.2,2.68116467799998));
#307703=CARTESIAN_POINT('Ctrl Pts',(-3.70167983700005,5.2,2.68116467799998));
#307704=CARTESIAN_POINT('Ctrl Pts',(-3.70167983700005,2.2,2.68116467799998));
#307705=CARTESIAN_POINT('Ctrl Pts',(-3.70403845800006,12.2,2.68144528699998));
#307706=CARTESIAN_POINT('Ctrl Pts',(-3.70403845800006,5.2,2.68144528699998));
#307707=CARTESIAN_POINT('Ctrl Pts',(-3.70403845800006,2.2,2.68144528699998));
#307708=CARTESIAN_POINT('Ctrl Pts',(-3.70640100800006,12.2,2.68172380799999));
#307709=CARTESIAN_POINT('Ctrl Pts',(-3.70640100800006,5.2,2.68172380799999));
#307710=CARTESIAN_POINT('Ctrl Pts',(-3.70640100800006,2.2,2.68172380799999));
#307711=CARTESIAN_POINT('Ctrl Pts',(-3.70876748400006,12.2,2.68200023099999));
#307712=CARTESIAN_POINT('Ctrl Pts',(-3.70876748400006,5.2,2.68200023099999));
#307713=CARTESIAN_POINT('Ctrl Pts',(-3.70876748400006,2.2,2.68200023099999));
#307714=CARTESIAN_POINT('Ctrl Pts',(-3.71113787600006,12.2,2.68227454999998));
#307715=CARTESIAN_POINT('Ctrl Pts',(-3.71113787600006,5.2,2.68227454999998));
#307716=CARTESIAN_POINT('Ctrl Pts',(-3.71113787600006,2.2,2.68227454999998));
#307717=CARTESIAN_POINT('Ctrl Pts',(-3.71351218200005,12.2,2.68254675699998));
#307718=CARTESIAN_POINT('Ctrl Pts',(-3.71351218200005,5.2,2.68254675699998));
#307719=CARTESIAN_POINT('Ctrl Pts',(-3.71351218200005,2.2,2.68254675699998));
#307720=CARTESIAN_POINT('Ctrl Pts',(-3.71589039400006,12.2,2.68281684399999));
#307721=CARTESIAN_POINT('Ctrl Pts',(-3.71589039400006,5.2,2.68281684399999));
#307722=CARTESIAN_POINT('Ctrl Pts',(-3.71589039400006,2.2,2.68281684399999));
#307723=CARTESIAN_POINT('Ctrl Pts',(-3.71827250800006,12.2,2.68308480499999));
#307724=CARTESIAN_POINT('Ctrl Pts',(-3.71827250800006,5.2,2.68308480499999));
#307725=CARTESIAN_POINT('Ctrl Pts',(-3.71827250800006,2.2,2.68308480499999));
#307726=CARTESIAN_POINT('Ctrl Pts',(-3.72065851800006,12.2,2.68335063099999));
#307727=CARTESIAN_POINT('Ctrl Pts',(-3.72065851800006,5.2,2.68335063099999));
#307728=CARTESIAN_POINT('Ctrl Pts',(-3.72065851800006,2.2,2.68335063099999));
#307729=CARTESIAN_POINT('Ctrl Pts',(-3.72304841700006,12.2,2.68361431399998));
#307730=CARTESIAN_POINT('Ctrl Pts',(-3.72304841700006,5.2,2.68361431399998));
#307731=CARTESIAN_POINT('Ctrl Pts',(-3.72304841700006,2.2,2.68361431399998));
#307732=CARTESIAN_POINT('Ctrl Pts',(-3.72544220100006,12.2,2.68387584899998));
#307733=CARTESIAN_POINT('Ctrl Pts',(-3.72544220100006,5.2,2.68387584899998));
#307734=CARTESIAN_POINT('Ctrl Pts',(-3.72544220100006,2.2,2.68387584899998));
#307735=CARTESIAN_POINT('Ctrl Pts',(-3.72783986300006,12.2,2.68413522699999));
#307736=CARTESIAN_POINT('Ctrl Pts',(-3.72783986300006,5.2,2.68413522699999));
#307737=CARTESIAN_POINT('Ctrl Pts',(-3.72783986300006,2.2,2.68413522699999));
#307738=CARTESIAN_POINT('Ctrl Pts',(-3.73024140000005,12.2,2.68439243999998));
#307739=CARTESIAN_POINT('Ctrl Pts',(-3.73024140000005,5.2,2.68439243999998));
#307740=CARTESIAN_POINT('Ctrl Pts',(-3.73024140000005,2.2,2.68439243999998));
#307741=CARTESIAN_POINT('Ctrl Pts',(-3.73264680300006,12.2,2.68464748299999));
#307742=CARTESIAN_POINT('Ctrl Pts',(-3.73264680300006,5.2,2.68464748299999));
#307743=CARTESIAN_POINT('Ctrl Pts',(-3.73264680300006,2.2,2.68464748299999));
#307744=CARTESIAN_POINT('Ctrl Pts',(-3.73505606800006,12.2,2.68490034499998));
#307745=CARTESIAN_POINT('Ctrl Pts',(-3.73505606800006,5.2,2.68490034499998));
#307746=CARTESIAN_POINT('Ctrl Pts',(-3.73505606800006,2.2,2.68490034499998));
#307747=CARTESIAN_POINT('Ctrl Pts',(-3.73746918800006,12.2,2.68515102199999));
#307748=CARTESIAN_POINT('Ctrl Pts',(-3.73746918800006,5.2,2.68515102199999));
#307749=CARTESIAN_POINT('Ctrl Pts',(-3.73746918800006,2.2,2.68515102199999));
#307750=CARTESIAN_POINT('Ctrl Pts',(-3.73988616000006,12.2,2.68539950499999));
#307751=CARTESIAN_POINT('Ctrl Pts',(-3.73988616000006,5.2,2.68539950499999));
#307752=CARTESIAN_POINT('Ctrl Pts',(-3.73988616000006,2.2,2.68539950499999));
#307753=CARTESIAN_POINT('Ctrl Pts',(-3.74230697500006,12.2,2.68564578699999));
#307754=CARTESIAN_POINT('Ctrl Pts',(-3.74230697500006,5.2,2.68564578699999));
#307755=CARTESIAN_POINT('Ctrl Pts',(-3.74230697500006,2.2,2.68564578699999));
#307756=CARTESIAN_POINT('Ctrl Pts',(-3.74473163000006,12.2,2.68588986199998));
#307757=CARTESIAN_POINT('Ctrl Pts',(-3.74473163000006,5.2,2.68588986199998));
#307758=CARTESIAN_POINT('Ctrl Pts',(-3.74473163000006,2.2,2.68588986199998));
#307759=CARTESIAN_POINT('Ctrl Pts',(-3.74716011800006,12.2,2.68613171999998));
#307760=CARTESIAN_POINT('Ctrl Pts',(-3.74716011800006,5.2,2.68613171999998));
#307761=CARTESIAN_POINT('Ctrl Pts',(-3.74716011800006,2.2,2.68613171999998));
#307762=CARTESIAN_POINT('Ctrl Pts',(-3.74959243400006,12.2,2.68637135599998));
#307763=CARTESIAN_POINT('Ctrl Pts',(-3.74959243400006,5.2,2.68637135599998));
#307764=CARTESIAN_POINT('Ctrl Pts',(-3.74959243400006,2.2,2.68637135599998));
#307765=CARTESIAN_POINT('Ctrl Pts',(-3.75202857100006,12.2,2.68660876099998));
#307766=CARTESIAN_POINT('Ctrl Pts',(-3.75202857100006,5.2,2.68660876099998));
#307767=CARTESIAN_POINT('Ctrl Pts',(-3.75202857100006,2.2,2.68660876099998));
#307768=CARTESIAN_POINT('Ctrl Pts',(-3.75446852500006,12.2,2.68684392999998));
#307769=CARTESIAN_POINT('Ctrl Pts',(-3.75446852500006,5.2,2.68684392999998));
#307770=CARTESIAN_POINT('Ctrl Pts',(-3.75446852500006,2.2,2.68684392999998));
#307771=CARTESIAN_POINT('Ctrl Pts',(-3.75691229000005,12.2,2.68707685299999));
#307772=CARTESIAN_POINT('Ctrl Pts',(-3.75691229000005,5.2,2.68707685299999));
#307773=CARTESIAN_POINT('Ctrl Pts',(-3.75691229000005,2.2,2.68707685299999));
#307774=CARTESIAN_POINT('Ctrl Pts',(-3.75935985900006,12.2,2.68730752599998));
#307775=CARTESIAN_POINT('Ctrl Pts',(-3.75935985900006,5.2,2.68730752599998));
#307776=CARTESIAN_POINT('Ctrl Pts',(-3.75935985900006,2.2,2.68730752599998));
#307777=CARTESIAN_POINT('Ctrl Pts',(-3.76181122700006,12.2,2.68753593899999));
#307778=CARTESIAN_POINT('Ctrl Pts',(-3.76181122700006,5.2,2.68753593899999));
#307779=CARTESIAN_POINT('Ctrl Pts',(-3.76181122700006,2.2,2.68753593899999));
#307780=CARTESIAN_POINT('Ctrl Pts',(-3.76426638900006,12.2,2.68776208699999));
#307781=CARTESIAN_POINT('Ctrl Pts',(-3.76426638900006,5.2,2.68776208699999));
#307782=CARTESIAN_POINT('Ctrl Pts',(-3.76426638900006,2.2,2.68776208699999));
#307783=CARTESIAN_POINT('Ctrl Pts',(-3.76672533800006,12.2,2.68798596099998));
#307784=CARTESIAN_POINT('Ctrl Pts',(-3.76672533800006,5.2,2.68798596099998));
#307785=CARTESIAN_POINT('Ctrl Pts',(-3.76672533800006,2.2,2.68798596099998));
#307786=CARTESIAN_POINT('Ctrl Pts',(-3.76918807000005,12.2,2.68820755499998));
#307787=CARTESIAN_POINT('Ctrl Pts',(-3.76918807000005,5.2,2.68820755499998));
#307788=CARTESIAN_POINT('Ctrl Pts',(-3.76918807000005,2.2,2.68820755499998));
#307789=CARTESIAN_POINT('Ctrl Pts',(-3.77165457700006,12.2,2.68842686199999));
#307790=CARTESIAN_POINT('Ctrl Pts',(-3.77165457700006,5.2,2.68842686199999));
#307791=CARTESIAN_POINT('Ctrl Pts',(-3.77165457700006,2.2,2.68842686199999));
#307792=CARTESIAN_POINT('Ctrl Pts',(-3.77412485600006,12.2,2.68864387299999));
#307793=CARTESIAN_POINT('Ctrl Pts',(-3.77412485600006,5.2,2.68864387299999));
#307794=CARTESIAN_POINT('Ctrl Pts',(-3.77412485600006,2.2,2.68864387299999));
#307795=CARTESIAN_POINT('Ctrl Pts',(-3.77659889800006,12.2,2.68885858399998));
#307796=CARTESIAN_POINT('Ctrl Pts',(-3.77659889800006,5.2,2.68885858399998));
#307797=CARTESIAN_POINT('Ctrl Pts',(-3.77659889800006,2.2,2.68885858399998));
#307798=CARTESIAN_POINT('Ctrl Pts',(-3.77907670100006,12.2,2.68907098599998));
#307799=CARTESIAN_POINT('Ctrl Pts',(-3.77907670100006,5.2,2.68907098599998));
#307800=CARTESIAN_POINT('Ctrl Pts',(-3.77907670100006,2.2,2.68907098599998));
#307801=CARTESIAN_POINT('Ctrl Pts',(-3.78155825700006,12.2,2.68928107199999));
#307802=CARTESIAN_POINT('Ctrl Pts',(-3.78155825700006,5.2,2.68928107199999));
#307803=CARTESIAN_POINT('Ctrl Pts',(-3.78155825700006,2.2,2.68928107199999));
#307804=CARTESIAN_POINT('Ctrl Pts',(-3.78404356000006,12.2,2.68948883599998));
#307805=CARTESIAN_POINT('Ctrl Pts',(-3.78404356000006,5.2,2.68948883599998));
#307806=CARTESIAN_POINT('Ctrl Pts',(-3.78404356000006,2.2,2.68948883599998));
#307807=CARTESIAN_POINT('Ctrl Pts',(-3.78653260400006,12.2,2.68969426999998));
#307808=CARTESIAN_POINT('Ctrl Pts',(-3.78653260400006,5.2,2.68969426999998));
#307809=CARTESIAN_POINT('Ctrl Pts',(-3.78653260400006,2.2,2.68969426999998));
#307810=CARTESIAN_POINT('Ctrl Pts',(-3.78902538700006,12.2,2.68989736599998));
#307811=CARTESIAN_POINT('Ctrl Pts',(-3.78902538700006,5.2,2.68989736599998));
#307812=CARTESIAN_POINT('Ctrl Pts',(-3.78902538700006,2.2,2.68989736599998));
#307813=CARTESIAN_POINT('Ctrl Pts',(-3.79152189800006,12.2,2.69009811999998));
#307814=CARTESIAN_POINT('Ctrl Pts',(-3.79152189800006,5.2,2.69009811999998));
#307815=CARTESIAN_POINT('Ctrl Pts',(-3.79152189800006,2.2,2.69009811999998));
#307816=CARTESIAN_POINT('Ctrl Pts',(-3.79402213500006,12.2,2.69029652299999));
#307817=CARTESIAN_POINT('Ctrl Pts',(-3.79402213500006,5.2,2.69029652299999));
#307818=CARTESIAN_POINT('Ctrl Pts',(-3.79402213500006,2.2,2.69029652299999));
#307819=CARTESIAN_POINT('Ctrl Pts',(-3.79652609100006,12.2,2.69049256799998));
#307820=CARTESIAN_POINT('Ctrl Pts',(-3.79652609100006,5.2,2.69049256799998));
#307821=CARTESIAN_POINT('Ctrl Pts',(-3.79652609100006,2.2,2.69049256799998));
#307822=CARTESIAN_POINT('Ctrl Pts',(-3.79903376000006,12.2,2.69068624799999));
#307823=CARTESIAN_POINT('Ctrl Pts',(-3.79903376000006,5.2,2.69068624799999));
#307824=CARTESIAN_POINT('Ctrl Pts',(-3.79903376000006,2.2,2.69068624799999));
#307825=CARTESIAN_POINT('Ctrl Pts',(-3.80154513600006,12.2,2.69087755799998));
#307826=CARTESIAN_POINT('Ctrl Pts',(-3.80154513600006,5.2,2.69087755799998));
#307827=CARTESIAN_POINT('Ctrl Pts',(-3.80154513600006,2.2,2.69087755799998));
#307828=CARTESIAN_POINT('Ctrl Pts',(-3.80406021400006,12.2,2.69106648899999));
#307829=CARTESIAN_POINT('Ctrl Pts',(-3.80406021400006,5.2,2.69106648899999));
#307830=CARTESIAN_POINT('Ctrl Pts',(-3.80406021400006,2.2,2.69106648899999));
#307831=CARTESIAN_POINT('Ctrl Pts',(-3.80657898900005,12.2,2.69125303399999));
#307832=CARTESIAN_POINT('Ctrl Pts',(-3.80657898900005,5.2,2.69125303399999));
#307833=CARTESIAN_POINT('Ctrl Pts',(-3.80657898900005,2.2,2.69125303399999));
#307834=CARTESIAN_POINT('Ctrl Pts',(-3.80910145400006,12.2,2.69143718799998));
#307835=CARTESIAN_POINT('Ctrl Pts',(-3.80910145400006,5.2,2.69143718799998));
#307836=CARTESIAN_POINT('Ctrl Pts',(-3.80910145400006,2.2,2.69143718799998));
#307837=CARTESIAN_POINT('Ctrl Pts',(-3.81162760300006,12.2,2.69161894299998));
#307838=CARTESIAN_POINT('Ctrl Pts',(-3.81162760300006,5.2,2.69161894299998));
#307839=CARTESIAN_POINT('Ctrl Pts',(-3.81162760300006,2.2,2.69161894299998));
#307840=CARTESIAN_POINT('Ctrl Pts',(-3.81415743000006,12.2,2.69179829199999));
#307841=CARTESIAN_POINT('Ctrl Pts',(-3.81415743000006,5.2,2.69179829199999));
#307842=CARTESIAN_POINT('Ctrl Pts',(-3.81415743000006,2.2,2.69179829199999));
#307843=CARTESIAN_POINT('Ctrl Pts',(-3.81669093200006,12.2,2.69197522899999));
#307844=CARTESIAN_POINT('Ctrl Pts',(-3.81669093200006,5.2,2.69197522899999));
#307845=CARTESIAN_POINT('Ctrl Pts',(-3.81669093200006,2.2,2.69197522899999));
#307846=CARTESIAN_POINT('Ctrl Pts',(-3.81922810000006,12.2,2.69214974599999));
#307847=CARTESIAN_POINT('Ctrl Pts',(-3.81922810000006,5.2,2.69214974599999));
#307848=CARTESIAN_POINT('Ctrl Pts',(-3.81922810000006,2.2,2.69214974599999));
#307849=CARTESIAN_POINT('Ctrl Pts',(-3.82176893000006,12.2,2.69232183699998));
#307850=CARTESIAN_POINT('Ctrl Pts',(-3.82176893000006,5.2,2.69232183699998));
#307851=CARTESIAN_POINT('Ctrl Pts',(-3.82176893000006,2.2,2.69232183699998));
#307852=CARTESIAN_POINT('Ctrl Pts',(-3.82431341600006,12.2,2.69249149599998));
#307853=CARTESIAN_POINT('Ctrl Pts',(-3.82431341600006,5.2,2.69249149599998));
#307854=CARTESIAN_POINT('Ctrl Pts',(-3.82431341600006,2.2,2.69249149599998));
#307855=CARTESIAN_POINT('Ctrl Pts',(-3.82686155200005,12.2,2.69265871399998));
#307856=CARTESIAN_POINT('Ctrl Pts',(-3.82686155200005,5.2,2.69265871399998));
#307857=CARTESIAN_POINT('Ctrl Pts',(-3.82686155200005,2.2,2.69265871399998));
#307858=CARTESIAN_POINT('Ctrl Pts',(-3.82941333200006,12.2,2.69282348599998));
#307859=CARTESIAN_POINT('Ctrl Pts',(-3.82941333200006,5.2,2.69282348599998));
#307860=CARTESIAN_POINT('Ctrl Pts',(-3.82941333200006,2.2,2.69282348599998));
#307861=CARTESIAN_POINT('Ctrl Pts',(-3.83196874900006,12.2,2.69298580499999));
#307862=CARTESIAN_POINT('Ctrl Pts',(-3.83196874900006,5.2,2.69298580499999));
#307863=CARTESIAN_POINT('Ctrl Pts',(-3.83196874900006,2.2,2.69298580499999));
#307864=CARTESIAN_POINT('Ctrl Pts',(-3.83452780100006,12.2,2.69314566399999));
#307865=CARTESIAN_POINT('Ctrl Pts',(-3.83452780100006,5.2,2.69314566399999));
#307866=CARTESIAN_POINT('Ctrl Pts',(-3.83452780100006,2.2,2.69314566399999));
#307867=CARTESIAN_POINT('Ctrl Pts',(-3.83709047900005,12.2,2.69330305699999));
#307868=CARTESIAN_POINT('Ctrl Pts',(-3.83709047900005,5.2,2.69330305699999));
#307869=CARTESIAN_POINT('Ctrl Pts',(-3.83709047900005,2.2,2.69330305699999));
#307870=CARTESIAN_POINT('Ctrl Pts',(-3.83965677700006,12.2,2.69345797599998));
#307871=CARTESIAN_POINT('Ctrl Pts',(-3.83965677700006,5.2,2.69345797599998));
#307872=CARTESIAN_POINT('Ctrl Pts',(-3.83965677700006,2.2,2.69345797599998));
#307873=CARTESIAN_POINT('Ctrl Pts',(-3.84222669200006,12.2,2.69361041599999));
#307874=CARTESIAN_POINT('Ctrl Pts',(-3.84222669200006,5.2,2.69361041599999));
#307875=CARTESIAN_POINT('Ctrl Pts',(-3.84222669200006,2.2,2.69361041599999));
#307876=CARTESIAN_POINT('Ctrl Pts',(-3.84480021600006,12.2,2.69376036799999));
#307877=CARTESIAN_POINT('Ctrl Pts',(-3.84480021600006,5.2,2.69376036799999));
#307878=CARTESIAN_POINT('Ctrl Pts',(-3.84480021600006,2.2,2.69376036799999));
#307879=CARTESIAN_POINT('Ctrl Pts',(-3.84737734300006,12.2,2.69390782799999));
#307880=CARTESIAN_POINT('Ctrl Pts',(-3.84737734300006,5.2,2.69390782799999));
#307881=CARTESIAN_POINT('Ctrl Pts',(-3.84737734300006,2.2,2.69390782799999));
#307882=CARTESIAN_POINT('Ctrl Pts',(-3.84995807000006,12.2,2.69405278999999));
#307883=CARTESIAN_POINT('Ctrl Pts',(-3.84995807000006,5.2,2.69405278999999));
#307884=CARTESIAN_POINT('Ctrl Pts',(-3.84995807000006,2.2,2.69405278999999));
#307885=CARTESIAN_POINT('Ctrl Pts',(-3.85254238800006,12.2,2.69419524399999));
#307886=CARTESIAN_POINT('Ctrl Pts',(-3.85254238800006,5.2,2.69419524399999));
#307887=CARTESIAN_POINT('Ctrl Pts',(-3.85254238800006,2.2,2.69419524399999));
#307888=CARTESIAN_POINT('Ctrl Pts',(-3.85513029300006,12.2,2.69433518699999));
#307889=CARTESIAN_POINT('Ctrl Pts',(-3.85513029300006,5.2,2.69433518699999));
#307890=CARTESIAN_POINT('Ctrl Pts',(-3.85513029300006,2.2,2.69433518699999));
#307891=CARTESIAN_POINT('Ctrl Pts',(-3.85772177900006,12.2,2.69447260899998));
#307892=CARTESIAN_POINT('Ctrl Pts',(-3.85772177900006,5.2,2.69447260899998));
#307893=CARTESIAN_POINT('Ctrl Pts',(-3.85772177900006,2.2,2.69447260899998));
#307894=CARTESIAN_POINT('Ctrl Pts',(-3.86031684000006,12.2,2.69460750499999));
#307895=CARTESIAN_POINT('Ctrl Pts',(-3.86031684000006,5.2,2.69460750499999));
#307896=CARTESIAN_POINT('Ctrl Pts',(-3.86031684000006,2.2,2.69460750499999));
#307897=CARTESIAN_POINT('Ctrl Pts',(-3.86291546800006,12.2,2.69473986899998));
#307898=CARTESIAN_POINT('Ctrl Pts',(-3.86291546800006,5.2,2.69473986899998));
#307899=CARTESIAN_POINT('Ctrl Pts',(-3.86291546800006,2.2,2.69473986899998));
#307900=CARTESIAN_POINT('Ctrl Pts',(-3.86551766000006,12.2,2.69486969199999));
#307901=CARTESIAN_POINT('Ctrl Pts',(-3.86551766000006,5.2,2.69486969199999));
#307902=CARTESIAN_POINT('Ctrl Pts',(-3.86551766000006,2.2,2.69486969199999));
#307903=CARTESIAN_POINT('Ctrl Pts',(-3.86812340800006,12.2,2.69499696899998));
#307904=CARTESIAN_POINT('Ctrl Pts',(-3.86812340800006,5.2,2.69499696899998));
#307905=CARTESIAN_POINT('Ctrl Pts',(-3.86812340800006,2.2,2.69499696899998));
#307906=CARTESIAN_POINT('Ctrl Pts',(-3.87073270700006,12.2,2.69512169399999));
#307907=CARTESIAN_POINT('Ctrl Pts',(-3.87073270700006,5.2,2.69512169399999));
#307908=CARTESIAN_POINT('Ctrl Pts',(-3.87073270700006,2.2,2.69512169399999));
#307909=CARTESIAN_POINT('Ctrl Pts',(-3.87334555400006,12.2,2.69524386199999));
#307910=CARTESIAN_POINT('Ctrl Pts',(-3.87334555400006,5.2,2.69524386199999));
#307911=CARTESIAN_POINT('Ctrl Pts',(-3.87334555400006,2.2,2.69524386199999));
#307912=CARTESIAN_POINT('Ctrl Pts',(-3.87596194200006,12.2,2.69536346599998));
#307913=CARTESIAN_POINT('Ctrl Pts',(-3.87596194200006,5.2,2.69536346599998));
#307914=CARTESIAN_POINT('Ctrl Pts',(-3.87596194200006,2.2,2.69536346599998));
#307915=CARTESIAN_POINT('Ctrl Pts',(-3.87858186500006,12.2,2.69548049999998));
#307916=CARTESIAN_POINT('Ctrl Pts',(-3.87858186500006,5.2,2.69548049999998));
#307917=CARTESIAN_POINT('Ctrl Pts',(-3.87858186500006,2.2,2.69548049999998));
#307918=CARTESIAN_POINT('Ctrl Pts',(-3.88120531800006,12.2,2.69559495899999));
#307919=CARTESIAN_POINT('Ctrl Pts',(-3.88120531800006,5.2,2.69559495899999));
#307920=CARTESIAN_POINT('Ctrl Pts',(-3.88120531800006,2.2,2.69559495899999));
#307921=CARTESIAN_POINT('Ctrl Pts',(-3.88383229600006,12.2,2.69570683299998));
#307922=CARTESIAN_POINT('Ctrl Pts',(-3.88383229600006,5.2,2.69570683299998));
#307923=CARTESIAN_POINT('Ctrl Pts',(-3.88383229600006,2.2,2.69570683299998));
#307924=CARTESIAN_POINT('Ctrl Pts',(-3.88646278800006,12.2,2.69581611799998));
#307925=CARTESIAN_POINT('Ctrl Pts',(-3.88646278800006,5.2,2.69581611799998));
#307926=CARTESIAN_POINT('Ctrl Pts',(-3.88646278800006,2.2,2.69581611799998));
#307927=CARTESIAN_POINT('Ctrl Pts',(-3.88909679200006,12.2,2.69592280299998));
#307928=CARTESIAN_POINT('Ctrl Pts',(-3.88909679200006,5.2,2.69592280299998));
#307929=CARTESIAN_POINT('Ctrl Pts',(-3.88909679200006,2.2,2.69592280299998));
#307930=CARTESIAN_POINT('Ctrl Pts',(-3.89173429500006,12.2,2.69602688099998));
#307931=CARTESIAN_POINT('Ctrl Pts',(-3.89173429500006,5.2,2.69602688099998));
#307932=CARTESIAN_POINT('Ctrl Pts',(-3.89173429500006,2.2,2.69602688099998));
#307933=CARTESIAN_POINT('Ctrl Pts',(-3.89437529600006,12.2,2.69612834599998));
#307934=CARTESIAN_POINT('Ctrl Pts',(-3.89437529600006,5.2,2.69612834599998));
#307935=CARTESIAN_POINT('Ctrl Pts',(-3.89437529600006,2.2,2.69612834599998));
#307936=CARTESIAN_POINT('Ctrl Pts',(-3.89701978600006,12.2,2.69622718999998));
#307937=CARTESIAN_POINT('Ctrl Pts',(-3.89701978600006,5.2,2.69622718999998));
#307938=CARTESIAN_POINT('Ctrl Pts',(-3.89701978600006,2.2,2.69622718999998));
#307939=CARTESIAN_POINT('Ctrl Pts',(-3.89966776200006,12.2,2.69632340999999));
#307940=CARTESIAN_POINT('Ctrl Pts',(-3.89966776200006,5.2,2.69632340999999));
#307941=CARTESIAN_POINT('Ctrl Pts',(-3.89966776200006,2.2,2.69632340999999));
#307942=CARTESIAN_POINT('Ctrl Pts',(-3.90231922000006,12.2,2.69641700299999));
#307943=CARTESIAN_POINT('Ctrl Pts',(-3.90231922000006,5.2,2.69641700299999));
#307944=CARTESIAN_POINT('Ctrl Pts',(-3.90231922000006,2.2,2.69641700299999));
#307945=CARTESIAN_POINT('Ctrl Pts',(-3.90497416000006,12.2,2.69650796599999));
#307946=CARTESIAN_POINT('Ctrl Pts',(-3.90497416000006,5.2,2.69650796599999));
#307947=CARTESIAN_POINT('Ctrl Pts',(-3.90497416000006,2.2,2.69650796599999));
#307948=CARTESIAN_POINT('Ctrl Pts',(-3.90710089600006,12.2,2.69657863299999));
#307949=CARTESIAN_POINT('Ctrl Pts',(-3.90710089600006,5.2,2.69657863299999));
#307950=CARTESIAN_POINT('Ctrl Pts',(-3.90710089600006,2.2,2.69657863299999));
#307951=CARTESIAN_POINT('Ctrl Pts',(-3.90869751400006,12.2,2.69663044999999));
#307952=CARTESIAN_POINT('Ctrl Pts',(-3.90869751400006,5.2,2.69663044999999));
#307953=CARTESIAN_POINT('Ctrl Pts',(-3.90869751400006,2.2,2.69663044999999));
#307954=CARTESIAN_POINT('Ctrl Pts',(-3.90976262200006,12.2,2.69666446799998));
#307955=CARTESIAN_POINT('Ctrl Pts',(-3.90976262200006,5.2,2.69666446799998));
#307956=CARTESIAN_POINT('Ctrl Pts',(-3.90976262200006,2.2,2.69666446799998));
#307957=CARTESIAN_POINT('Ctrl Pts',(-3.91029535000006,12.2,2.69668134599998));
#307958=CARTESIAN_POINT('Ctrl Pts',(-3.91029535000006,5.2,2.69668134599998));
#307959=CARTESIAN_POINT('Ctrl Pts',(-3.91029535000006,2.2,2.69668134599998));
#307960=CARTESIAN_POINT('',(-3.91029535000006,2.7,2.69668134599998));
#307961=CARTESIAN_POINT('',(-3.91029535000006,12.2,2.69668134599998));
#307962=CARTESIAN_POINT('Ctrl Pts',(-3.11652602400006,2.7,2.49742420799999));
#307963=CARTESIAN_POINT('Ctrl Pts',(-3.1168936600151,2.7,2.49771654590457));
#307964=CARTESIAN_POINT('Ctrl Pts',(-3.11816799097087,2.7,2.49871239564421));
#307965=CARTESIAN_POINT('Ctrl Pts',(-3.12398442812182,2.7,2.502910285736));
#307966=CARTESIAN_POINT('Ctrl Pts',(-3.12772253913452,2.7,2.50544873038177));
#307967=CARTESIAN_POINT('Ctrl Pts',(-3.14431490947368,2.7,2.51632623854521));
#307968=CARTESIAN_POINT('Ctrl Pts',(-3.15872784906809,2.7,2.52467057788753));
#307969=CARTESIAN_POINT('Ctrl Pts',(-3.21189785985966,2.7,2.55327156940896));
#307970=CARTESIAN_POINT('Ctrl Pts',(-3.26446474401564,2.7,2.57695346780209));
#307971=CARTESIAN_POINT('Ctrl Pts',(-3.45446370493968,2.7,2.64200888222062));
#307972=CARTESIAN_POINT('Ctrl Pts',(-3.64593588656003,2.7,2.68830585414583));
#307973=CARTESIAN_POINT('Ctrl Pts',(-3.91029535000006,2.7,2.69668134599998));
#307974=CARTESIAN_POINT('Origin',(-5.66300478732629E-14,15.2,-1.77635683940025E-14));
#307975=CARTESIAN_POINT('',(-4.09164014900006,2.7,2.41267090399998));
#307976=CARTESIAN_POINT('',(-4.09164014900006,12.2,2.41267090399998));
#307977=CARTESIAN_POINT('Origin',(-5.66300478732629E-14,2.7,-1.92943768261394E-14));
#307978=CARTESIAN_POINT('Ctrl Pts',(-4.09164015000006,12.2,2.41267090399998));
#307979=CARTESIAN_POINT('Ctrl Pts',(-4.09164015000006,5.2,2.41267090399998));
#307980=CARTESIAN_POINT('Ctrl Pts',(-4.09164015000006,2.2,2.41267090399998));
#307981=CARTESIAN_POINT('Ctrl Pts',(-4.09140069000006,12.2,2.41219472799998));
#307982=CARTESIAN_POINT('Ctrl Pts',(-4.09140069000006,5.2,2.41219472799998));
#307983=CARTESIAN_POINT('Ctrl Pts',(-4.09140069000006,2.2,2.41219472799998));
#307984=CARTESIAN_POINT('Ctrl Pts',(-4.09092167800006,12.2,2.41124280399998));
#307985=CARTESIAN_POINT('Ctrl Pts',(-4.09092167800006,5.2,2.41124280399998));
#307986=CARTESIAN_POINT('Ctrl Pts',(-4.09092167800006,2.2,2.41124280399998));
#307987=CARTESIAN_POINT('Ctrl Pts',(-4.09020288500006,12.2,2.40981619699999));
#307988=CARTESIAN_POINT('Ctrl Pts',(-4.09020288500006,5.2,2.40981619699999));
#307989=CARTESIAN_POINT('Ctrl Pts',(-4.09020288500006,2.2,2.40981619699999));
#307990=CARTESIAN_POINT('Ctrl Pts',(-4.08924394000006,12.2,2.40791661099998));
#307991=CARTESIAN_POINT('Ctrl Pts',(-4.08924394000006,5.2,2.40791661099998));
#307992=CARTESIAN_POINT('Ctrl Pts',(-4.08924394000006,2.2,2.40791661099998));
#307993=CARTESIAN_POINT('Ctrl Pts',(-4.08804433600006,12.2,2.40554639299998));
#307994=CARTESIAN_POINT('Ctrl Pts',(-4.08804433600006,5.2,2.40554639299998));
#307995=CARTESIAN_POINT('Ctrl Pts',(-4.08804433600006,2.2,2.40554639299998));
#307996=CARTESIAN_POINT('Ctrl Pts',(-4.08684381400006,12.2,2.40318043899999));
#307997=CARTESIAN_POINT('Ctrl Pts',(-4.08684381400006,5.2,2.40318043899999));
#307998=CARTESIAN_POINT('Ctrl Pts',(-4.08684381400006,2.2,2.40318043899999));
#307999=CARTESIAN_POINT('Ctrl Pts',(-4.08564237300006,12.2,2.40081874999999));
#308000=CARTESIAN_POINT('Ctrl Pts',(-4.08564237300006,5.2,2.40081874999999));
#308001=CARTESIAN_POINT('Ctrl Pts',(-4.08564237300006,2.2,2.40081874999999));
#308002=CARTESIAN_POINT('Ctrl Pts',(-4.08444001800006,12.2,2.39846132899999));
#308003=CARTESIAN_POINT('Ctrl Pts',(-4.08444001800006,5.2,2.39846132899999));
#308004=CARTESIAN_POINT('Ctrl Pts',(-4.08444001800006,2.2,2.39846132899999));
#308005=CARTESIAN_POINT('Ctrl Pts',(-4.08323675400006,12.2,2.39610817499998));
#308006=CARTESIAN_POINT('Ctrl Pts',(-4.08323675400006,5.2,2.39610817499998));
#308007=CARTESIAN_POINT('Ctrl Pts',(-4.08323675400006,2.2,2.39610817499998));
#308008=CARTESIAN_POINT('Ctrl Pts',(-4.08203258900006,12.2,2.39375929199999));
#308009=CARTESIAN_POINT('Ctrl Pts',(-4.08203258900006,5.2,2.39375929199999));
#308010=CARTESIAN_POINT('Ctrl Pts',(-4.08203258900006,2.2,2.39375929199999));
#308011=CARTESIAN_POINT('Ctrl Pts',(-4.08082753400006,12.2,2.39141468199998));
#308012=CARTESIAN_POINT('Ctrl Pts',(-4.08082753400006,5.2,2.39141468199998));
#308013=CARTESIAN_POINT('Ctrl Pts',(-4.08082753400006,2.2,2.39141468199998));
#308014=CARTESIAN_POINT('Ctrl Pts',(-4.07962159800006,12.2,2.38907435099998));
#308015=CARTESIAN_POINT('Ctrl Pts',(-4.07962159800006,5.2,2.38907435099998));
#308016=CARTESIAN_POINT('Ctrl Pts',(-4.07962159800006,2.2,2.38907435099998));
#308017=CARTESIAN_POINT('Ctrl Pts',(-4.07841479000006,12.2,2.38673829799998));
#308018=CARTESIAN_POINT('Ctrl Pts',(-4.07841479000006,5.2,2.38673829799998));
#308019=CARTESIAN_POINT('Ctrl Pts',(-4.07841479000006,2.2,2.38673829799998));
#308020=CARTESIAN_POINT('Ctrl Pts',(-4.07720712200006,12.2,2.38440652899998));
#308021=CARTESIAN_POINT('Ctrl Pts',(-4.07720712200006,5.2,2.38440652899998));
#308022=CARTESIAN_POINT('Ctrl Pts',(-4.07720712200006,2.2,2.38440652899998));
#308023=CARTESIAN_POINT('Ctrl Pts',(-4.07599860100006,12.2,2.38207904699999));
#308024=CARTESIAN_POINT('Ctrl Pts',(-4.07599860100006,5.2,2.38207904699999));
#308025=CARTESIAN_POINT('Ctrl Pts',(-4.07599860100006,2.2,2.38207904699999));
#308026=CARTESIAN_POINT('Ctrl Pts',(-4.07478923800006,12.2,2.37975585299999));
#308027=CARTESIAN_POINT('Ctrl Pts',(-4.07478923800006,5.2,2.37975585299999));
#308028=CARTESIAN_POINT('Ctrl Pts',(-4.07478923800006,2.2,2.37975585299999));
#308029=CARTESIAN_POINT('Ctrl Pts',(-4.07357903900006,12.2,2.37743694999998));
#308030=CARTESIAN_POINT('Ctrl Pts',(-4.07357903900006,5.2,2.37743694999998));
#308031=CARTESIAN_POINT('Ctrl Pts',(-4.07357903900006,2.2,2.37743694999998));
#308032=CARTESIAN_POINT('Ctrl Pts',(-4.07236801200006,12.2,2.37512234199999));
#308033=CARTESIAN_POINT('Ctrl Pts',(-4.07236801200006,5.2,2.37512234199999));
#308034=CARTESIAN_POINT('Ctrl Pts',(-4.07236801200006,2.2,2.37512234199999));
#308035=CARTESIAN_POINT('Ctrl Pts',(-4.07115616400006,12.2,2.37281202899998));
#308036=CARTESIAN_POINT('Ctrl Pts',(-4.07115616400006,5.2,2.37281202899998));
#308037=CARTESIAN_POINT('Ctrl Pts',(-4.07115616400006,2.2,2.37281202899998));
#308038=CARTESIAN_POINT('Ctrl Pts',(-4.06994350400006,12.2,2.37050601299998));
#308039=CARTESIAN_POINT('Ctrl Pts',(-4.06994350400006,5.2,2.37050601299998));
#308040=CARTESIAN_POINT('Ctrl Pts',(-4.06994350400006,2.2,2.37050601299998));
#308041=CARTESIAN_POINT('Ctrl Pts',(-4.06873003700006,12.2,2.36820429799998));
#308042=CARTESIAN_POINT('Ctrl Pts',(-4.06873003700006,5.2,2.36820429799998));
#308043=CARTESIAN_POINT('Ctrl Pts',(-4.06873003700006,2.2,2.36820429799998));
#308044=CARTESIAN_POINT('Ctrl Pts',(-4.06751577500006,12.2,2.36590688599998));
#308045=CARTESIAN_POINT('Ctrl Pts',(-4.06751577500006,5.2,2.36590688599998));
#308046=CARTESIAN_POINT('Ctrl Pts',(-4.06751577500006,2.2,2.36590688599998));
#308047=CARTESIAN_POINT('Ctrl Pts',(-4.06630072400006,12.2,2.36361377999999));
#308048=CARTESIAN_POINT('Ctrl Pts',(-4.06630072400006,5.2,2.36361377999999));
#308049=CARTESIAN_POINT('Ctrl Pts',(-4.06630072400006,2.2,2.36361377999999));
#308050=CARTESIAN_POINT('Ctrl Pts',(-4.06508489400006,12.2,2.36132498199999));
#308051=CARTESIAN_POINT('Ctrl Pts',(-4.06508489400006,5.2,2.36132498199999));
#308052=CARTESIAN_POINT('Ctrl Pts',(-4.06508489400006,2.2,2.36132498199999));
#308053=CARTESIAN_POINT('Ctrl Pts',(-4.06386829400006,12.2,2.35904049499998));
#308054=CARTESIAN_POINT('Ctrl Pts',(-4.06386829400006,5.2,2.35904049499998));
#308055=CARTESIAN_POINT('Ctrl Pts',(-4.06386829400006,2.2,2.35904049499998));
#308056=CARTESIAN_POINT('Ctrl Pts',(-4.06265093200005,12.2,2.35676032199999));
#308057=CARTESIAN_POINT('Ctrl Pts',(-4.06265093200005,5.2,2.35676032199999));
#308058=CARTESIAN_POINT('Ctrl Pts',(-4.06265093200005,2.2,2.35676032199999));
#308059=CARTESIAN_POINT('Ctrl Pts',(-4.06143281700006,12.2,2.35448446399998));
#308060=CARTESIAN_POINT('Ctrl Pts',(-4.06143281700006,5.2,2.35448446399998));
#308061=CARTESIAN_POINT('Ctrl Pts',(-4.06143281700006,2.2,2.35448446399998));
#308062=CARTESIAN_POINT('Ctrl Pts',(-4.06021395700006,12.2,2.35221292499999));
#308063=CARTESIAN_POINT('Ctrl Pts',(-4.06021395700006,5.2,2.35221292499999));
#308064=CARTESIAN_POINT('Ctrl Pts',(-4.06021395700006,2.2,2.35221292499999));
#308065=CARTESIAN_POINT('Ctrl Pts',(-4.05899436000006,12.2,2.34994570499998));
#308066=CARTESIAN_POINT('Ctrl Pts',(-4.05899436000006,5.2,2.34994570499998));
#308067=CARTESIAN_POINT('Ctrl Pts',(-4.05899436000006,2.2,2.34994570499998));
#308068=CARTESIAN_POINT('Ctrl Pts',(-4.05777403500006,12.2,2.34768281099999));
#308069=CARTESIAN_POINT('Ctrl Pts',(-4.05777403500006,5.2,2.34768281099999));
#308070=CARTESIAN_POINT('Ctrl Pts',(-4.05777403500006,2.2,2.34768281099999));
#308071=CARTESIAN_POINT('Ctrl Pts',(-4.05655298900006,12.2,2.34542424099998));
#308072=CARTESIAN_POINT('Ctrl Pts',(-4.05655298900006,5.2,2.34542424099998));
#308073=CARTESIAN_POINT('Ctrl Pts',(-4.05655298900006,2.2,2.34542424099998));
#308074=CARTESIAN_POINT('Ctrl Pts',(-4.05533123200006,12.2,2.34316999899999));
#308075=CARTESIAN_POINT('Ctrl Pts',(-4.05533123200006,5.2,2.34316999899999));
#308076=CARTESIAN_POINT('Ctrl Pts',(-4.05533123200006,2.2,2.34316999899999));
#308077=CARTESIAN_POINT('Ctrl Pts',(-4.05410877200006,12.2,2.34092008799998));
#308078=CARTESIAN_POINT('Ctrl Pts',(-4.05410877200006,5.2,2.34092008799998));
#308079=CARTESIAN_POINT('Ctrl Pts',(-4.05410877200006,2.2,2.34092008799998));
#308080=CARTESIAN_POINT('Ctrl Pts',(-4.05288561800006,12.2,2.33867450899998));
#308081=CARTESIAN_POINT('Ctrl Pts',(-4.05288561800006,5.2,2.33867450899998));
#308082=CARTESIAN_POINT('Ctrl Pts',(-4.05288561800006,2.2,2.33867450899998));
#308083=CARTESIAN_POINT('Ctrl Pts',(-4.05166177700006,12.2,2.33643326599998));
#308084=CARTESIAN_POINT('Ctrl Pts',(-4.05166177700006,5.2,2.33643326599998));
#308085=CARTESIAN_POINT('Ctrl Pts',(-4.05166177700006,2.2,2.33643326599998));
#308086=CARTESIAN_POINT('Ctrl Pts',(-4.05043725800006,12.2,2.33419635999998));
#308087=CARTESIAN_POINT('Ctrl Pts',(-4.05043725800006,5.2,2.33419635999998));
#308088=CARTESIAN_POINT('Ctrl Pts',(-4.05043725800006,2.2,2.33419635999998));
#308089=CARTESIAN_POINT('Ctrl Pts',(-4.04921207100006,12.2,2.33196379399998));
#308090=CARTESIAN_POINT('Ctrl Pts',(-4.04921207100006,5.2,2.33196379399998));
#308091=CARTESIAN_POINT('Ctrl Pts',(-4.04921207100006,2.2,2.33196379399998));
#308092=CARTESIAN_POINT('Ctrl Pts',(-4.04798622300006,12.2,2.32973557199998));
#308093=CARTESIAN_POINT('Ctrl Pts',(-4.04798622300006,5.2,2.32973557199998));
#308094=CARTESIAN_POINT('Ctrl Pts',(-4.04798622300006,2.2,2.32973557199998));
#308095=CARTESIAN_POINT('Ctrl Pts',(-4.04675972500006,12.2,2.32751169299998));
#308096=CARTESIAN_POINT('Ctrl Pts',(-4.04675972500006,5.2,2.32751169299998));
#308097=CARTESIAN_POINT('Ctrl Pts',(-4.04675972500006,2.2,2.32751169299998));
#308098=CARTESIAN_POINT('Ctrl Pts',(-4.04553258300006,12.2,2.32529216199998));
#308099=CARTESIAN_POINT('Ctrl Pts',(-4.04553258300006,5.2,2.32529216199998));
#308100=CARTESIAN_POINT('Ctrl Pts',(-4.04553258300006,2.2,2.32529216199998));
#308101=CARTESIAN_POINT('Ctrl Pts',(-4.04430480600006,12.2,2.32307697999998));
#308102=CARTESIAN_POINT('Ctrl Pts',(-4.04430480600006,5.2,2.32307697999998));
#308103=CARTESIAN_POINT('Ctrl Pts',(-4.04430480600006,2.2,2.32307697999998));
#308104=CARTESIAN_POINT('Ctrl Pts',(-4.04307640300006,12.2,2.32086615099998));
#308105=CARTESIAN_POINT('Ctrl Pts',(-4.04307640300006,5.2,2.32086615099998));
#308106=CARTESIAN_POINT('Ctrl Pts',(-4.04307640300006,2.2,2.32086615099998));
#308107=CARTESIAN_POINT('Ctrl Pts',(-4.04184738300006,12.2,2.31865967499999));
#308108=CARTESIAN_POINT('Ctrl Pts',(-4.04184738300006,5.2,2.31865967499999));
#308109=CARTESIAN_POINT('Ctrl Pts',(-4.04184738300006,2.2,2.31865967499999));
#308110=CARTESIAN_POINT('Ctrl Pts',(-4.04061775500006,12.2,2.31645755699999));
#308111=CARTESIAN_POINT('Ctrl Pts',(-4.04061775500006,5.2,2.31645755699999));
#308112=CARTESIAN_POINT('Ctrl Pts',(-4.04061775500006,2.2,2.31645755699999));
#308113=CARTESIAN_POINT('Ctrl Pts',(-4.03938752700006,12.2,2.31425979699999));
#308114=CARTESIAN_POINT('Ctrl Pts',(-4.03938752700006,5.2,2.31425979699999));
#308115=CARTESIAN_POINT('Ctrl Pts',(-4.03938752700006,2.2,2.31425979699999));
#308116=CARTESIAN_POINT('Ctrl Pts',(-4.03815670700006,12.2,2.31206639799999));
#308117=CARTESIAN_POINT('Ctrl Pts',(-4.03815670700006,5.2,2.31206639799999));
#308118=CARTESIAN_POINT('Ctrl Pts',(-4.03815670700006,2.2,2.31206639799999));
#308119=CARTESIAN_POINT('Ctrl Pts',(-4.03692530400006,12.2,2.30987736199999));
#308120=CARTESIAN_POINT('Ctrl Pts',(-4.03692530400006,5.2,2.30987736199999));
#308121=CARTESIAN_POINT('Ctrl Pts',(-4.03692530400006,2.2,2.30987736199999));
#308122=CARTESIAN_POINT('Ctrl Pts',(-4.03569332700005,12.2,2.30769269299998));
#308123=CARTESIAN_POINT('Ctrl Pts',(-4.03569332700005,5.2,2.30769269299998));
#308124=CARTESIAN_POINT('Ctrl Pts',(-4.03569332700005,2.2,2.30769269299998));
#308125=CARTESIAN_POINT('Ctrl Pts',(-4.03446078600005,12.2,2.30551239099999));
#308126=CARTESIAN_POINT('Ctrl Pts',(-4.03446078600005,5.2,2.30551239099999));
#308127=CARTESIAN_POINT('Ctrl Pts',(-4.03446078600005,2.2,2.30551239099999));
#308128=CARTESIAN_POINT('Ctrl Pts',(-4.03322768800006,12.2,2.30333645999998));
#308129=CARTESIAN_POINT('Ctrl Pts',(-4.03322768800006,5.2,2.30333645999998));
#308130=CARTESIAN_POINT('Ctrl Pts',(-4.03322768800006,2.2,2.30333645999998));
#308131=CARTESIAN_POINT('Ctrl Pts',(-4.03199404200006,12.2,2.30116490199999));
#308132=CARTESIAN_POINT('Ctrl Pts',(-4.03199404200006,5.2,2.30116490199999));
#308133=CARTESIAN_POINT('Ctrl Pts',(-4.03199404200006,2.2,2.30116490199999));
#308134=CARTESIAN_POINT('Ctrl Pts',(-4.03075985700006,12.2,2.29899771799999));
#308135=CARTESIAN_POINT('Ctrl Pts',(-4.03075985700006,5.2,2.29899771799999));
#308136=CARTESIAN_POINT('Ctrl Pts',(-4.03075985700006,2.2,2.29899771799999));
#308137=CARTESIAN_POINT('Ctrl Pts',(-4.02952514200006,12.2,2.29683491099999));
#308138=CARTESIAN_POINT('Ctrl Pts',(-4.02952514200006,5.2,2.29683491099999));
#308139=CARTESIAN_POINT('Ctrl Pts',(-4.02952514200006,2.2,2.29683491099999));
#308140=CARTESIAN_POINT('Ctrl Pts',(-4.02828990600006,12.2,2.29467648299998));
#308141=CARTESIAN_POINT('Ctrl Pts',(-4.02828990600006,5.2,2.29467648299998));
#308142=CARTESIAN_POINT('Ctrl Pts',(-4.02828990600006,2.2,2.29467648299998));
#308143=CARTESIAN_POINT('Ctrl Pts',(-4.02705415600006,12.2,2.29252243799999));
#308144=CARTESIAN_POINT('Ctrl Pts',(-4.02705415600006,5.2,2.29252243799999));
#308145=CARTESIAN_POINT('Ctrl Pts',(-4.02705415600006,2.2,2.29252243799999));
#308146=CARTESIAN_POINT('Ctrl Pts',(-4.02581790300006,12.2,2.29037277599998));
#308147=CARTESIAN_POINT('Ctrl Pts',(-4.02581790300006,5.2,2.29037277599998));
#308148=CARTESIAN_POINT('Ctrl Pts',(-4.02581790300006,2.2,2.29037277599998));
#308149=CARTESIAN_POINT('Ctrl Pts',(-4.02458115500006,12.2,2.28822749899999));
#308150=CARTESIAN_POINT('Ctrl Pts',(-4.02458115500006,5.2,2.28822749899999));
#308151=CARTESIAN_POINT('Ctrl Pts',(-4.02458115500006,2.2,2.28822749899999));
#308152=CARTESIAN_POINT('Ctrl Pts',(-4.02334392100006,12.2,2.28608661099999));
#308153=CARTESIAN_POINT('Ctrl Pts',(-4.02334392100006,5.2,2.28608661099999));
#308154=CARTESIAN_POINT('Ctrl Pts',(-4.02334392100006,2.2,2.28608661099999));
#308155=CARTESIAN_POINT('Ctrl Pts',(-4.02210620900005,12.2,2.28395011399999));
#308156=CARTESIAN_POINT('Ctrl Pts',(-4.02210620900005,5.2,2.28395011399999));
#308157=CARTESIAN_POINT('Ctrl Pts',(-4.02210620900005,2.2,2.28395011399999));
#308158=CARTESIAN_POINT('Ctrl Pts',(-4.02086802900006,12.2,2.28181800899999));
#308159=CARTESIAN_POINT('Ctrl Pts',(-4.02086802900006,5.2,2.28181800899999));
#308160=CARTESIAN_POINT('Ctrl Pts',(-4.02086802900006,2.2,2.28181800899999));
#308161=CARTESIAN_POINT('Ctrl Pts',(-4.01962939000006,12.2,2.27969029899999));
#308162=CARTESIAN_POINT('Ctrl Pts',(-4.01962939000006,5.2,2.27969029899999));
#308163=CARTESIAN_POINT('Ctrl Pts',(-4.01962939000006,2.2,2.27969029899999));
#308164=CARTESIAN_POINT('Ctrl Pts',(-4.01839029900006,12.2,2.27756698499999));
#308165=CARTESIAN_POINT('Ctrl Pts',(-4.01839029900006,5.2,2.27756698499999));
#308166=CARTESIAN_POINT('Ctrl Pts',(-4.01839029900006,2.2,2.27756698499999));
#308167=CARTESIAN_POINT('Ctrl Pts',(-4.01715076700006,12.2,2.27544807099999));
#308168=CARTESIAN_POINT('Ctrl Pts',(-4.01715076700006,5.2,2.27544807099999));
#308169=CARTESIAN_POINT('Ctrl Pts',(-4.01715076700006,2.2,2.27544807099999));
#308170=CARTESIAN_POINT('Ctrl Pts',(-4.01591080300006,12.2,2.27333355699999));
#308171=CARTESIAN_POINT('Ctrl Pts',(-4.01591080300006,5.2,2.27333355699999));
#308172=CARTESIAN_POINT('Ctrl Pts',(-4.01591080300006,2.2,2.27333355699999));
#308173=CARTESIAN_POINT('Ctrl Pts',(-4.01467041400006,12.2,2.27122344799998));
#308174=CARTESIAN_POINT('Ctrl Pts',(-4.01467041400006,5.2,2.27122344799998));
#308175=CARTESIAN_POINT('Ctrl Pts',(-4.01467041400006,2.2,2.27122344799998));
#308176=CARTESIAN_POINT('Ctrl Pts',(-4.01342961000006,12.2,2.26911774299999));
#308177=CARTESIAN_POINT('Ctrl Pts',(-4.01342961000006,5.2,2.26911774299999));
#308178=CARTESIAN_POINT('Ctrl Pts',(-4.01342961000006,2.2,2.26911774299999));
#308179=CARTESIAN_POINT('Ctrl Pts',(-4.01218840000006,12.2,2.26701644599999));
#308180=CARTESIAN_POINT('Ctrl Pts',(-4.01218840000006,5.2,2.26701644599999));
#308181=CARTESIAN_POINT('Ctrl Pts',(-4.01218840000006,2.2,2.26701644599999));
#308182=CARTESIAN_POINT('Ctrl Pts',(-4.01094679400006,12.2,2.26491955899998));
#308183=CARTESIAN_POINT('Ctrl Pts',(-4.01094679400006,5.2,2.26491955899998));
#308184=CARTESIAN_POINT('Ctrl Pts',(-4.01094679400006,2.2,2.26491955899998));
#308185=CARTESIAN_POINT('Ctrl Pts',(-4.00970479900006,12.2,2.26282708299999));
#308186=CARTESIAN_POINT('Ctrl Pts',(-4.00970479900006,5.2,2.26282708299999));
#308187=CARTESIAN_POINT('Ctrl Pts',(-4.00970479900006,2.2,2.26282708299999));
#308188=CARTESIAN_POINT('Ctrl Pts',(-4.00846242600006,12.2,2.26073902199999));
#308189=CARTESIAN_POINT('Ctrl Pts',(-4.00846242600006,5.2,2.26073902199999));
#308190=CARTESIAN_POINT('Ctrl Pts',(-4.00846242600006,2.2,2.26073902199999));
#308191=CARTESIAN_POINT('Ctrl Pts',(-4.00721968300005,12.2,2.25865537699999));
#308192=CARTESIAN_POINT('Ctrl Pts',(-4.00721968300005,5.2,2.25865537699999));
#308193=CARTESIAN_POINT('Ctrl Pts',(-4.00721968300005,2.2,2.25865537699999));
#308194=CARTESIAN_POINT('Ctrl Pts',(-4.00597657800006,12.2,2.25657614799998));
#308195=CARTESIAN_POINT('Ctrl Pts',(-4.00597657800006,5.2,2.25657614799998));
#308196=CARTESIAN_POINT('Ctrl Pts',(-4.00597657800006,2.2,2.25657614799998));
#308197=CARTESIAN_POINT('Ctrl Pts',(-4.00473312200006,12.2,2.25450133999999));
#308198=CARTESIAN_POINT('Ctrl Pts',(-4.00473312200006,5.2,2.25450133999999));
#308199=CARTESIAN_POINT('Ctrl Pts',(-4.00473312200006,2.2,2.25450133999999));
#308200=CARTESIAN_POINT('Ctrl Pts',(-4.00348932300005,12.2,2.25243095499998));
#308201=CARTESIAN_POINT('Ctrl Pts',(-4.00348932300005,5.2,2.25243095499998));
#308202=CARTESIAN_POINT('Ctrl Pts',(-4.00348932300005,2.2,2.25243095499998));
#308203=CARTESIAN_POINT('Ctrl Pts',(-4.00224519000006,12.2,2.25036499399998));
#308204=CARTESIAN_POINT('Ctrl Pts',(-4.00224519000006,5.2,2.25036499399998));
#308205=CARTESIAN_POINT('Ctrl Pts',(-4.00224519000006,2.2,2.25036499399998));
#308206=CARTESIAN_POINT('Ctrl Pts',(-4.00100073300006,12.2,2.24830345699999));
#308207=CARTESIAN_POINT('Ctrl Pts',(-4.00100073300006,5.2,2.24830345699999));
#308208=CARTESIAN_POINT('Ctrl Pts',(-4.00100073300006,2.2,2.24830345699999));
#308209=CARTESIAN_POINT('Ctrl Pts',(-3.99975596000006,12.2,2.24624635099998));
#308210=CARTESIAN_POINT('Ctrl Pts',(-3.99975596000006,5.2,2.24624635099998));
#308211=CARTESIAN_POINT('Ctrl Pts',(-3.99975596000006,2.2,2.24624635099998));
#308212=CARTESIAN_POINT('Ctrl Pts',(-3.99851088100006,12.2,2.24419367399999));
#308213=CARTESIAN_POINT('Ctrl Pts',(-3.99851088100006,5.2,2.24419367399999));
#308214=CARTESIAN_POINT('Ctrl Pts',(-3.99851088100006,2.2,2.24419367399999));
#308215=CARTESIAN_POINT('Ctrl Pts',(-3.99726550600006,12.2,2.24214542899999));
#308216=CARTESIAN_POINT('Ctrl Pts',(-3.99726550600006,5.2,2.24214542899999));
#308217=CARTESIAN_POINT('Ctrl Pts',(-3.99726550600006,2.2,2.24214542899999));
#308218=CARTESIAN_POINT('Ctrl Pts',(-3.99601984000006,12.2,2.24010161799999));
#308219=CARTESIAN_POINT('Ctrl Pts',(-3.99601984000006,5.2,2.24010161799999));
#308220=CARTESIAN_POINT('Ctrl Pts',(-3.99601984000006,2.2,2.24010161799999));
#308221=CARTESIAN_POINT('Ctrl Pts',(-3.99477389700006,12.2,2.23806224299999));
#308222=CARTESIAN_POINT('Ctrl Pts',(-3.99477389700006,5.2,2.23806224299999));
#308223=CARTESIAN_POINT('Ctrl Pts',(-3.99477389700006,2.2,2.23806224299999));
#308224=CARTESIAN_POINT('Ctrl Pts',(-3.99352768500005,12.2,2.23602730699998));
#308225=CARTESIAN_POINT('Ctrl Pts',(-3.99352768500005,5.2,2.23602730699998));
#308226=CARTESIAN_POINT('Ctrl Pts',(-3.99352768500005,2.2,2.23602730699998));
#308227=CARTESIAN_POINT('Ctrl Pts',(-3.99228121100006,12.2,2.23399680999998));
#308228=CARTESIAN_POINT('Ctrl Pts',(-3.99228121100006,5.2,2.23399680999998));
#308229=CARTESIAN_POINT('Ctrl Pts',(-3.99228121100006,2.2,2.23399680999998));
#308230=CARTESIAN_POINT('Ctrl Pts',(-3.99103448600005,12.2,2.23197075599999));
#308231=CARTESIAN_POINT('Ctrl Pts',(-3.99103448600005,5.2,2.23197075599999));
#308232=CARTESIAN_POINT('Ctrl Pts',(-3.99103448600005,2.2,2.23197075599999));
#308233=CARTESIAN_POINT('Ctrl Pts',(-3.98978751900006,12.2,2.22994914599999));
#308234=CARTESIAN_POINT('Ctrl Pts',(-3.98978751900006,5.2,2.22994914599999));
#308235=CARTESIAN_POINT('Ctrl Pts',(-3.98978751900006,2.2,2.22994914599999));
#308236=CARTESIAN_POINT('Ctrl Pts',(-3.98854032000005,12.2,2.22793198099998));
#308237=CARTESIAN_POINT('Ctrl Pts',(-3.98854032000005,5.2,2.22793198099998));
#308238=CARTESIAN_POINT('Ctrl Pts',(-3.98854032000005,2.2,2.22793198099998));
#308239=CARTESIAN_POINT('Ctrl Pts',(-3.98729289800006,12.2,2.22591926399998));
#308240=CARTESIAN_POINT('Ctrl Pts',(-3.98729289800006,5.2,2.22591926399998));
#308241=CARTESIAN_POINT('Ctrl Pts',(-3.98729289800006,2.2,2.22591926399998));
#308242=CARTESIAN_POINT('Ctrl Pts',(-3.98604526000006,12.2,2.22391099699998));
#308243=CARTESIAN_POINT('Ctrl Pts',(-3.98604526000006,5.2,2.22391099699998));
#308244=CARTESIAN_POINT('Ctrl Pts',(-3.98604526000006,2.2,2.22391099699998));
#308245=CARTESIAN_POINT('Ctrl Pts',(-3.98479741800006,12.2,2.22190718199998));
#308246=CARTESIAN_POINT('Ctrl Pts',(-3.98479741800006,5.2,2.22190718199998));
#308247=CARTESIAN_POINT('Ctrl Pts',(-3.98479741800006,2.2,2.22190718199998));
#308248=CARTESIAN_POINT('Ctrl Pts',(-3.98354938000006,12.2,2.21990781899999));
#308249=CARTESIAN_POINT('Ctrl Pts',(-3.98354938000006,5.2,2.21990781899999));
#308250=CARTESIAN_POINT('Ctrl Pts',(-3.98354938000006,2.2,2.21990781899999));
#308251=CARTESIAN_POINT('Ctrl Pts',(-3.98230115500006,12.2,2.21791291299999));
#308252=CARTESIAN_POINT('Ctrl Pts',(-3.98230115500006,5.2,2.21791291299999));
#308253=CARTESIAN_POINT('Ctrl Pts',(-3.98230115500006,2.2,2.21791291299999));
#308254=CARTESIAN_POINT('Ctrl Pts',(-3.98105275500006,12.2,2.21592246299998));
#308255=CARTESIAN_POINT('Ctrl Pts',(-3.98105275500006,5.2,2.21592246299998));
#308256=CARTESIAN_POINT('Ctrl Pts',(-3.98105275500006,2.2,2.21592246299998));
#308257=CARTESIAN_POINT('Ctrl Pts',(-3.97980418500006,12.2,2.21393647299998));
#308258=CARTESIAN_POINT('Ctrl Pts',(-3.97980418500006,5.2,2.21393647299998));
#308259=CARTESIAN_POINT('Ctrl Pts',(-3.97980418500006,2.2,2.21393647299998));
#308260=CARTESIAN_POINT('Ctrl Pts',(-3.97855545900006,12.2,2.21195494399999));
#308261=CARTESIAN_POINT('Ctrl Pts',(-3.97855545900006,5.2,2.21195494399999));
#308262=CARTESIAN_POINT('Ctrl Pts',(-3.97855545900006,2.2,2.21195494399999));
#308263=CARTESIAN_POINT('Ctrl Pts',(-3.97730658300006,12.2,2.20997787699998));
#308264=CARTESIAN_POINT('Ctrl Pts',(-3.97730658300006,5.2,2.20997787699998));
#308265=CARTESIAN_POINT('Ctrl Pts',(-3.97730658300006,2.2,2.20997787699998));
#308266=CARTESIAN_POINT('Ctrl Pts',(-3.97605756700006,12.2,2.20800527499998));
#308267=CARTESIAN_POINT('Ctrl Pts',(-3.97605756700006,5.2,2.20800527499998));
#308268=CARTESIAN_POINT('Ctrl Pts',(-3.97605756700006,2.2,2.20800527499998));
#308269=CARTESIAN_POINT('Ctrl Pts',(-3.97480842100006,12.2,2.20603713899999));
#308270=CARTESIAN_POINT('Ctrl Pts',(-3.97480842100006,5.2,2.20603713899999));
#308271=CARTESIAN_POINT('Ctrl Pts',(-3.97480842100006,2.2,2.20603713899999));
#308272=CARTESIAN_POINT('Ctrl Pts',(-3.97355915400006,12.2,2.20407347199998));
#308273=CARTESIAN_POINT('Ctrl Pts',(-3.97355915400006,5.2,2.20407347199998));
#308274=CARTESIAN_POINT('Ctrl Pts',(-3.97355915400006,2.2,2.20407347199998));
#308275=CARTESIAN_POINT('Ctrl Pts',(-3.97230977800006,12.2,2.20211427399999));
#308276=CARTESIAN_POINT('Ctrl Pts',(-3.97230977800006,5.2,2.20211427399999));
#308277=CARTESIAN_POINT('Ctrl Pts',(-3.97230977800006,2.2,2.20211427399999));
#308278=CARTESIAN_POINT('Ctrl Pts',(-3.97106029800006,12.2,2.20015954799999));
#308279=CARTESIAN_POINT('Ctrl Pts',(-3.97106029800006,5.2,2.20015954799999));
#308280=CARTESIAN_POINT('Ctrl Pts',(-3.97106029800006,2.2,2.20015954799999));
#308281=CARTESIAN_POINT('Ctrl Pts',(-3.96981072700005,12.2,2.19820929599999));
#308282=CARTESIAN_POINT('Ctrl Pts',(-3.96981072700005,5.2,2.19820929599999));
#308283=CARTESIAN_POINT('Ctrl Pts',(-3.96981072700005,2.2,2.19820929599999));
#308284=CARTESIAN_POINT('Ctrl Pts',(-3.96856107200006,12.2,2.19626351999999));
#308285=CARTESIAN_POINT('Ctrl Pts',(-3.96856107200006,5.2,2.19626351999999));
#308286=CARTESIAN_POINT('Ctrl Pts',(-3.96856107200006,2.2,2.19626351999999));
#308287=CARTESIAN_POINT('Ctrl Pts',(-3.96731134500006,12.2,2.19432221999998));
#308288=CARTESIAN_POINT('Ctrl Pts',(-3.96731134500006,5.2,2.19432221999998));
#308289=CARTESIAN_POINT('Ctrl Pts',(-3.96731134500006,2.2,2.19432221999998));
#308290=CARTESIAN_POINT('Ctrl Pts',(-3.96606155400006,12.2,2.19238539899999));
#308291=CARTESIAN_POINT('Ctrl Pts',(-3.96606155400006,5.2,2.19238539899999));
#308292=CARTESIAN_POINT('Ctrl Pts',(-3.96606155400006,2.2,2.19238539899999));
#308293=CARTESIAN_POINT('Ctrl Pts',(-3.96481170800006,12.2,2.19045305899999));
#308294=CARTESIAN_POINT('Ctrl Pts',(-3.96481170800006,5.2,2.19045305899999));
#308295=CARTESIAN_POINT('Ctrl Pts',(-3.96481170800006,2.2,2.19045305899999));
#308296=CARTESIAN_POINT('Ctrl Pts',(-3.96356181700006,12.2,2.18852520099999));
#308297=CARTESIAN_POINT('Ctrl Pts',(-3.96356181700006,5.2,2.18852520099999));
#308298=CARTESIAN_POINT('Ctrl Pts',(-3.96356181700006,2.2,2.18852520099999));
#308299=CARTESIAN_POINT('Ctrl Pts',(-3.96231189200006,12.2,2.18660182699999));
#308300=CARTESIAN_POINT('Ctrl Pts',(-3.96231189200006,5.2,2.18660182699999));
#308301=CARTESIAN_POINT('Ctrl Pts',(-3.96231189200006,2.2,2.18660182699999));
#308302=CARTESIAN_POINT('Ctrl Pts',(-3.96106194100006,12.2,2.18468293799999));
#308303=CARTESIAN_POINT('Ctrl Pts',(-3.96106194100006,5.2,2.18468293799999));
#308304=CARTESIAN_POINT('Ctrl Pts',(-3.96106194100006,2.2,2.18468293799999));
#308305=CARTESIAN_POINT('Ctrl Pts',(-3.95981197400006,12.2,2.18276853699999));
#308306=CARTESIAN_POINT('Ctrl Pts',(-3.95981197400006,5.2,2.18276853699999));
#308307=CARTESIAN_POINT('Ctrl Pts',(-3.95981197400006,2.2,2.18276853699999));
#308308=CARTESIAN_POINT('Ctrl Pts',(-3.95856200100006,12.2,2.18085862499999));
#308309=CARTESIAN_POINT('Ctrl Pts',(-3.95856200100006,5.2,2.18085862499999));
#308310=CARTESIAN_POINT('Ctrl Pts',(-3.95856200100006,2.2,2.18085862499999));
#308311=CARTESIAN_POINT('Ctrl Pts',(-3.95731203200006,12.2,2.17895320399998));
#308312=CARTESIAN_POINT('Ctrl Pts',(-3.95731203200006,5.2,2.17895320399998));
#308313=CARTESIAN_POINT('Ctrl Pts',(-3.95731203200006,2.2,2.17895320399998));
#308314=CARTESIAN_POINT('Ctrl Pts',(-3.95606207500006,12.2,2.17705227499998));
#308315=CARTESIAN_POINT('Ctrl Pts',(-3.95606207500006,5.2,2.17705227499998));
#308316=CARTESIAN_POINT('Ctrl Pts',(-3.95606207500006,2.2,2.17705227499998));
#308317=CARTESIAN_POINT('Ctrl Pts',(-3.95481214000006,12.2,2.17515584099999));
#308318=CARTESIAN_POINT('Ctrl Pts',(-3.95481214000006,5.2,2.17515584099999));
#308319=CARTESIAN_POINT('Ctrl Pts',(-3.95481214000006,2.2,2.17515584099999));
#308320=CARTESIAN_POINT('Ctrl Pts',(-3.95356223800006,12.2,2.17326390099998));
#308321=CARTESIAN_POINT('Ctrl Pts',(-3.95356223800006,5.2,2.17326390099998));
#308322=CARTESIAN_POINT('Ctrl Pts',(-3.95356223800006,2.2,2.17326390099998));
#308323=CARTESIAN_POINT('Ctrl Pts',(-3.95231237800005,12.2,2.17137645899999));
#308324=CARTESIAN_POINT('Ctrl Pts',(-3.95231237800005,5.2,2.17137645899999));
#308325=CARTESIAN_POINT('Ctrl Pts',(-3.95231237800005,2.2,2.17137645899999));
#308326=CARTESIAN_POINT('Ctrl Pts',(-3.95106257000006,12.2,2.16949351599999));
#308327=CARTESIAN_POINT('Ctrl Pts',(-3.95106257000006,5.2,2.16949351599999));
#308328=CARTESIAN_POINT('Ctrl Pts',(-3.95106257000006,2.2,2.16949351599999));
#308329=CARTESIAN_POINT('Ctrl Pts',(-3.94981282300006,12.2,2.16761507299998));
#308330=CARTESIAN_POINT('Ctrl Pts',(-3.94981282300006,5.2,2.16761507299998));
#308331=CARTESIAN_POINT('Ctrl Pts',(-3.94981282300006,2.2,2.16761507299998));
#308332=CARTESIAN_POINT('Ctrl Pts',(-3.94856314700006,12.2,2.16574113299998));
#308333=CARTESIAN_POINT('Ctrl Pts',(-3.94856314700006,5.2,2.16574113299998));
#308334=CARTESIAN_POINT('Ctrl Pts',(-3.94856314700006,2.2,2.16574113299998));
#308335=CARTESIAN_POINT('Ctrl Pts',(-3.94731355300006,12.2,2.16387169499999));
#308336=CARTESIAN_POINT('Ctrl Pts',(-3.94731355300006,5.2,2.16387169499999));
#308337=CARTESIAN_POINT('Ctrl Pts',(-3.94731355300006,2.2,2.16387169499999));
#308338=CARTESIAN_POINT('Ctrl Pts',(-3.94606404800006,12.2,2.16200676399998));
#308339=CARTESIAN_POINT('Ctrl Pts',(-3.94606404800006,5.2,2.16200676399998));
#308340=CARTESIAN_POINT('Ctrl Pts',(-3.94606404800006,2.2,2.16200676399998));
#308341=CARTESIAN_POINT('Ctrl Pts',(-3.94481464400006,12.2,2.16014633899999));
#308342=CARTESIAN_POINT('Ctrl Pts',(-3.94481464400006,5.2,2.16014633899999));
#308343=CARTESIAN_POINT('Ctrl Pts',(-3.94481464400006,2.2,2.16014633899999));
#308344=CARTESIAN_POINT('Ctrl Pts',(-3.94356535100005,12.2,2.15829042199998));
#308345=CARTESIAN_POINT('Ctrl Pts',(-3.94356535100005,5.2,2.15829042199998));
#308346=CARTESIAN_POINT('Ctrl Pts',(-3.94356535100005,2.2,2.15829042199998));
#308347=CARTESIAN_POINT('Ctrl Pts',(-3.94231617800005,12.2,2.15643901499998));
#308348=CARTESIAN_POINT('Ctrl Pts',(-3.94231617800005,5.2,2.15643901499998));
#308349=CARTESIAN_POINT('Ctrl Pts',(-3.94231617800005,2.2,2.15643901499998));
#308350=CARTESIAN_POINT('Ctrl Pts',(-3.94106713400006,12.2,2.15459211999999));
#308351=CARTESIAN_POINT('Ctrl Pts',(-3.94106713400006,5.2,2.15459211999999));
#308352=CARTESIAN_POINT('Ctrl Pts',(-3.94106713400006,2.2,2.15459211999999));
#308353=CARTESIAN_POINT('Ctrl Pts',(-3.93981823000006,12.2,2.15274973599998));
#308354=CARTESIAN_POINT('Ctrl Pts',(-3.93981823000006,5.2,2.15274973599998));
#308355=CARTESIAN_POINT('Ctrl Pts',(-3.93981823000006,2.2,2.15274973599998));
#308356=CARTESIAN_POINT('Ctrl Pts',(-3.93856947700006,12.2,2.15091186799999));
#308357=CARTESIAN_POINT('Ctrl Pts',(-3.93856947700006,5.2,2.15091186799999));
#308358=CARTESIAN_POINT('Ctrl Pts',(-3.93856947700006,2.2,2.15091186799999));
#308359=CARTESIAN_POINT('Ctrl Pts',(-3.93732088100006,12.2,2.14907851499999));
#308360=CARTESIAN_POINT('Ctrl Pts',(-3.93732088100006,5.2,2.14907851499999));
#308361=CARTESIAN_POINT('Ctrl Pts',(-3.93732088100006,2.2,2.14907851499999));
#308362=CARTESIAN_POINT('Ctrl Pts',(-3.93607245700006,12.2,2.14724967999999));
#308363=CARTESIAN_POINT('Ctrl Pts',(-3.93607245700006,5.2,2.14724967999999));
#308364=CARTESIAN_POINT('Ctrl Pts',(-3.93607245700006,2.2,2.14724967999999));
#308365=CARTESIAN_POINT('Ctrl Pts',(-3.93482421000006,12.2,2.14542536399998));
#308366=CARTESIAN_POINT('Ctrl Pts',(-3.93482421000006,5.2,2.14542536399998));
#308367=CARTESIAN_POINT('Ctrl Pts',(-3.93482421000006,2.2,2.14542536399998));
#308368=CARTESIAN_POINT('Ctrl Pts',(-3.93357615500006,12.2,2.14360556799999));
#308369=CARTESIAN_POINT('Ctrl Pts',(-3.93357615500006,5.2,2.14360556799999));
#308370=CARTESIAN_POINT('Ctrl Pts',(-3.93357615500006,2.2,2.14360556799999));
#308371=CARTESIAN_POINT('Ctrl Pts',(-3.93232829700006,12.2,2.14179029299999));
#308372=CARTESIAN_POINT('Ctrl Pts',(-3.93232829700006,5.2,2.14179029299999));
#308373=CARTESIAN_POINT('Ctrl Pts',(-3.93232829700006,2.2,2.14179029299999));
#308374=CARTESIAN_POINT('Ctrl Pts',(-3.93108064900006,12.2,2.13997954199999));
#308375=CARTESIAN_POINT('Ctrl Pts',(-3.93108064900006,5.2,2.13997954199999));
#308376=CARTESIAN_POINT('Ctrl Pts',(-3.93108064900006,2.2,2.13997954199999));
#308377=CARTESIAN_POINT('Ctrl Pts',(-3.92983322000005,12.2,2.13817331499999));
#308378=CARTESIAN_POINT('Ctrl Pts',(-3.92983322000005,5.2,2.13817331499999));
#308379=CARTESIAN_POINT('Ctrl Pts',(-3.92983322000005,2.2,2.13817331499999));
#308380=CARTESIAN_POINT('Ctrl Pts',(-3.92858602100006,12.2,2.13637161499999));
#308381=CARTESIAN_POINT('Ctrl Pts',(-3.92858602100006,5.2,2.13637161499999));
#308382=CARTESIAN_POINT('Ctrl Pts',(-3.92858602100006,2.2,2.13637161499999));
#308383=CARTESIAN_POINT('Ctrl Pts',(-3.92733906000006,12.2,2.13457443999999));
#308384=CARTESIAN_POINT('Ctrl Pts',(-3.92733906000006,5.2,2.13457443999999));
#308385=CARTESIAN_POINT('Ctrl Pts',(-3.92733906000006,2.2,2.13457443999999));
#308386=CARTESIAN_POINT('Ctrl Pts',(-3.92609234900006,12.2,2.13278179599998));
#308387=CARTESIAN_POINT('Ctrl Pts',(-3.92609234900006,5.2,2.13278179599998));
#308388=CARTESIAN_POINT('Ctrl Pts',(-3.92609234900006,2.2,2.13278179599998));
#308389=CARTESIAN_POINT('Ctrl Pts',(-3.92484589600006,12.2,2.13099368199998));
#308390=CARTESIAN_POINT('Ctrl Pts',(-3.92484589600006,5.2,2.13099368199998));
#308391=CARTESIAN_POINT('Ctrl Pts',(-3.92484589600006,2.2,2.13099368199998));
#308392=CARTESIAN_POINT('Ctrl Pts',(-3.92359971400006,12.2,2.12921009799999));
#308393=CARTESIAN_POINT('Ctrl Pts',(-3.92359971400006,5.2,2.12921009799999));
#308394=CARTESIAN_POINT('Ctrl Pts',(-3.92359971400006,2.2,2.12921009799999));
#308395=CARTESIAN_POINT('Ctrl Pts',(-3.92235381000006,12.2,2.12743104699999));
#308396=CARTESIAN_POINT('Ctrl Pts',(-3.92235381000006,5.2,2.12743104699999));
#308397=CARTESIAN_POINT('Ctrl Pts',(-3.92235381000006,2.2,2.12743104699999));
#308398=CARTESIAN_POINT('Ctrl Pts',(-3.92110819600005,12.2,2.12565653099999));
#308399=CARTESIAN_POINT('Ctrl Pts',(-3.92110819600005,5.2,2.12565653099999));
#308400=CARTESIAN_POINT('Ctrl Pts',(-3.92110819600005,2.2,2.12565653099999));
#308401=CARTESIAN_POINT('Ctrl Pts',(-3.91986288200005,12.2,2.12388654999998));
#308402=CARTESIAN_POINT('Ctrl Pts',(-3.91986288200005,5.2,2.12388654999998));
#308403=CARTESIAN_POINT('Ctrl Pts',(-3.91986288200005,2.2,2.12388654999998));
#308404=CARTESIAN_POINT('Ctrl Pts',(-3.91861787700006,12.2,2.12212110599999));
#308405=CARTESIAN_POINT('Ctrl Pts',(-3.91861787700006,5.2,2.12212110599999));
#308406=CARTESIAN_POINT('Ctrl Pts',(-3.91861787700006,2.2,2.12212110599999));
#308407=CARTESIAN_POINT('Ctrl Pts',(-3.91737319300006,12.2,2.12036019899998));
#308408=CARTESIAN_POINT('Ctrl Pts',(-3.91737319300006,5.2,2.12036019899998));
#308409=CARTESIAN_POINT('Ctrl Pts',(-3.91737319300006,2.2,2.12036019899998));
#308410=CARTESIAN_POINT('Ctrl Pts',(-3.91612883800006,12.2,2.11860383299999));
#308411=CARTESIAN_POINT('Ctrl Pts',(-3.91612883800006,5.2,2.11860383299999));
#308412=CARTESIAN_POINT('Ctrl Pts',(-3.91612883800006,2.2,2.11860383299999));
#308413=CARTESIAN_POINT('Ctrl Pts',(-3.91488482300006,12.2,2.11685200699999));
#308414=CARTESIAN_POINT('Ctrl Pts',(-3.91488482300006,5.2,2.11685200699999));
#308415=CARTESIAN_POINT('Ctrl Pts',(-3.91488482300006,2.2,2.11685200699999));
#308416=CARTESIAN_POINT('Ctrl Pts',(-3.91364116000006,12.2,2.11510472299999));
#308417=CARTESIAN_POINT('Ctrl Pts',(-3.91364116000006,5.2,2.11510472299999));
#308418=CARTESIAN_POINT('Ctrl Pts',(-3.91364116000006,2.2,2.11510472299999));
#308419=CARTESIAN_POINT('Ctrl Pts',(-3.91239785600006,12.2,2.11336198099998));
#308420=CARTESIAN_POINT('Ctrl Pts',(-3.91239785600006,5.2,2.11336198099998));
#308421=CARTESIAN_POINT('Ctrl Pts',(-3.91239785600006,2.2,2.11336198099998));
#308422=CARTESIAN_POINT('Ctrl Pts',(-3.91115492400006,12.2,2.11162378499999));
#308423=CARTESIAN_POINT('Ctrl Pts',(-3.91115492400006,5.2,2.11162378499999));
#308424=CARTESIAN_POINT('Ctrl Pts',(-3.91115492400006,2.2,2.11162378499999));
#308425=CARTESIAN_POINT('Ctrl Pts',(-3.90991237300006,12.2,2.10989013399999));
#308426=CARTESIAN_POINT('Ctrl Pts',(-3.90991237300006,5.2,2.10989013399999));
#308427=CARTESIAN_POINT('Ctrl Pts',(-3.90991237300006,2.2,2.10989013399999));
#308428=CARTESIAN_POINT('Ctrl Pts',(-3.90867021300005,12.2,2.10816102999999));
#308429=CARTESIAN_POINT('Ctrl Pts',(-3.90867021300005,5.2,2.10816102999999));
#308430=CARTESIAN_POINT('Ctrl Pts',(-3.90867021300005,2.2,2.10816102999999));
#308431=CARTESIAN_POINT('Ctrl Pts',(-3.90742845400006,12.2,2.10643647399999));
#308432=CARTESIAN_POINT('Ctrl Pts',(-3.90742845400006,5.2,2.10643647399999));
#308433=CARTESIAN_POINT('Ctrl Pts',(-3.90742845400006,2.2,2.10643647399999));
#308434=CARTESIAN_POINT('Ctrl Pts',(-3.90618710900006,12.2,2.10471646599999));
#308435=CARTESIAN_POINT('Ctrl Pts',(-3.90618710900006,5.2,2.10471646599999));
#308436=CARTESIAN_POINT('Ctrl Pts',(-3.90618710900006,2.2,2.10471646599999));
#308437=CARTESIAN_POINT('Ctrl Pts',(-3.90494618400006,12.2,2.10300100899998));
#308438=CARTESIAN_POINT('Ctrl Pts',(-3.90494618400006,5.2,2.10300100899998));
#308439=CARTESIAN_POINT('Ctrl Pts',(-3.90494618400006,2.2,2.10300100899998));
#308440=CARTESIAN_POINT('Ctrl Pts',(-3.90370569300006,12.2,2.10129010399998));
#308441=CARTESIAN_POINT('Ctrl Pts',(-3.90370569300006,5.2,2.10129010399998));
#308442=CARTESIAN_POINT('Ctrl Pts',(-3.90370569300006,2.2,2.10129010399998));
#308443=CARTESIAN_POINT('Ctrl Pts',(-3.90246564400006,12.2,2.09958375199998));
#308444=CARTESIAN_POINT('Ctrl Pts',(-3.90246564400006,5.2,2.09958375199998));
#308445=CARTESIAN_POINT('Ctrl Pts',(-3.90246564400006,2.2,2.09958375199998));
#308446=CARTESIAN_POINT('Ctrl Pts',(-3.90122604900006,12.2,2.09788195299998));
#308447=CARTESIAN_POINT('Ctrl Pts',(-3.90122604900006,5.2,2.09788195299998));
#308448=CARTESIAN_POINT('Ctrl Pts',(-3.90122604900006,2.2,2.09788195299998));
#308449=CARTESIAN_POINT('Ctrl Pts',(-3.89998691800006,12.2,2.09618470999999));
#308450=CARTESIAN_POINT('Ctrl Pts',(-3.89998691800006,5.2,2.09618470999999));
#308451=CARTESIAN_POINT('Ctrl Pts',(-3.89998691800006,2.2,2.09618470999999));
#308452=CARTESIAN_POINT('Ctrl Pts',(-3.89874826100006,12.2,2.09449202299998));
#308453=CARTESIAN_POINT('Ctrl Pts',(-3.89874826100006,5.2,2.09449202299998));
#308454=CARTESIAN_POINT('Ctrl Pts',(-3.89874826100006,2.2,2.09449202299998));
#308455=CARTESIAN_POINT('Ctrl Pts',(-3.89751008800006,12.2,2.09280389199999));
#308456=CARTESIAN_POINT('Ctrl Pts',(-3.89751008800006,5.2,2.09280389199999));
#308457=CARTESIAN_POINT('Ctrl Pts',(-3.89751008800006,2.2,2.09280389199999));
#308458=CARTESIAN_POINT('Ctrl Pts',(-3.89627241100006,12.2,2.09112031999998));
#308459=CARTESIAN_POINT('Ctrl Pts',(-3.89627241100006,5.2,2.09112031999998));
#308460=CARTESIAN_POINT('Ctrl Pts',(-3.89627241100006,2.2,2.09112031999998));
#308461=CARTESIAN_POINT('Ctrl Pts',(-3.89503523800006,12.2,2.08944130799999));
#308462=CARTESIAN_POINT('Ctrl Pts',(-3.89503523800006,5.2,2.08944130799999));
#308463=CARTESIAN_POINT('Ctrl Pts',(-3.89503523800006,2.2,2.08944130799999));
#308464=CARTESIAN_POINT('Ctrl Pts',(-3.89379858200006,12.2,2.08776685599998));
#308465=CARTESIAN_POINT('Ctrl Pts',(-3.89379858200006,5.2,2.08776685599998));
#308466=CARTESIAN_POINT('Ctrl Pts',(-3.89379858200006,2.2,2.08776685599998));
#308467=CARTESIAN_POINT('Ctrl Pts',(-3.89256245200006,12.2,2.08609696499999));
#308468=CARTESIAN_POINT('Ctrl Pts',(-3.89256245200006,5.2,2.08609696499999));
#308469=CARTESIAN_POINT('Ctrl Pts',(-3.89256245200006,2.2,2.08609696499999));
#308470=CARTESIAN_POINT('Ctrl Pts',(-3.89132685900006,12.2,2.08443163799998));
#308471=CARTESIAN_POINT('Ctrl Pts',(-3.89132685900006,5.2,2.08443163799998));
#308472=CARTESIAN_POINT('Ctrl Pts',(-3.89132685900006,2.2,2.08443163799998));
#308473=CARTESIAN_POINT('Ctrl Pts',(-3.89009181400006,12.2,2.08277087299999));
#308474=CARTESIAN_POINT('Ctrl Pts',(-3.89009181400006,5.2,2.08277087299999));
#308475=CARTESIAN_POINT('Ctrl Pts',(-3.89009181400006,2.2,2.08277087299999));
#308476=CARTESIAN_POINT('Ctrl Pts',(-3.88885732600006,12.2,2.08111467299998));
#308477=CARTESIAN_POINT('Ctrl Pts',(-3.88885732600006,5.2,2.08111467299998));
#308478=CARTESIAN_POINT('Ctrl Pts',(-3.88885732600006,2.2,2.08111467299998));
#308479=CARTESIAN_POINT('Ctrl Pts',(-3.88762340700006,12.2,2.07946303899998));
#308480=CARTESIAN_POINT('Ctrl Pts',(-3.88762340700006,5.2,2.07946303899998));
#308481=CARTESIAN_POINT('Ctrl Pts',(-3.88762340700006,2.2,2.07946303899998));
#308482=CARTESIAN_POINT('Ctrl Pts',(-3.88639006700005,12.2,2.07781597099999));
#308483=CARTESIAN_POINT('Ctrl Pts',(-3.88639006700005,5.2,2.07781597099999));
#308484=CARTESIAN_POINT('Ctrl Pts',(-3.88639006700005,2.2,2.07781597099999));
#308485=CARTESIAN_POINT('Ctrl Pts',(-3.88515731700006,12.2,2.07617347099998));
#308486=CARTESIAN_POINT('Ctrl Pts',(-3.88515731700006,5.2,2.07617347099998));
#308487=CARTESIAN_POINT('Ctrl Pts',(-3.88515731700006,2.2,2.07617347099998));
#308488=CARTESIAN_POINT('Ctrl Pts',(-3.88392516600006,12.2,2.07453553899999));
#308489=CARTESIAN_POINT('Ctrl Pts',(-3.88392516600006,5.2,2.07453553899999));
#308490=CARTESIAN_POINT('Ctrl Pts',(-3.88392516600006,2.2,2.07453553899999));
#308491=CARTESIAN_POINT('Ctrl Pts',(-3.88269362800005,12.2,2.07290217699999));
#308492=CARTESIAN_POINT('Ctrl Pts',(-3.88269362800005,5.2,2.07290217699999));
#308493=CARTESIAN_POINT('Ctrl Pts',(-3.88269362800005,2.2,2.07290217699999));
#308494=CARTESIAN_POINT('Ctrl Pts',(-3.88146271000006,12.2,2.07127338399999));
#308495=CARTESIAN_POINT('Ctrl Pts',(-3.88146271000006,5.2,2.07127338399999));
#308496=CARTESIAN_POINT('Ctrl Pts',(-3.88146271000006,2.2,2.07127338399999));
#308497=CARTESIAN_POINT('Ctrl Pts',(-3.88023242500006,12.2,2.06964916399999));
#308498=CARTESIAN_POINT('Ctrl Pts',(-3.88023242500006,5.2,2.06964916399999));
#308499=CARTESIAN_POINT('Ctrl Pts',(-3.88023242500006,2.2,2.06964916399999));
#308500=CARTESIAN_POINT('Ctrl Pts',(-3.87900278300005,12.2,2.06802951599999));
#308501=CARTESIAN_POINT('Ctrl Pts',(-3.87900278300005,5.2,2.06802951599999));
#308502=CARTESIAN_POINT('Ctrl Pts',(-3.87900278300005,2.2,2.06802951599999));
#308503=CARTESIAN_POINT('Ctrl Pts',(-3.87777379500006,12.2,2.06641444099999));
#308504=CARTESIAN_POINT('Ctrl Pts',(-3.87777379500006,5.2,2.06641444099999));
#308505=CARTESIAN_POINT('Ctrl Pts',(-3.87777379500006,2.2,2.06641444099999));
#308506=CARTESIAN_POINT('Ctrl Pts',(-3.87654547000006,12.2,2.06480393899998));
#308507=CARTESIAN_POINT('Ctrl Pts',(-3.87654547000006,5.2,2.06480393899998));
#308508=CARTESIAN_POINT('Ctrl Pts',(-3.87654547000006,2.2,2.06480393899998));
#308509=CARTESIAN_POINT('Ctrl Pts',(-3.87531782100006,12.2,2.06319801299998));
#308510=CARTESIAN_POINT('Ctrl Pts',(-3.87531782100006,5.2,2.06319801299998));
#308511=CARTESIAN_POINT('Ctrl Pts',(-3.87531782100006,2.2,2.06319801299998));
#308512=CARTESIAN_POINT('Ctrl Pts',(-3.87409085900006,12.2,2.06159666199999));
#308513=CARTESIAN_POINT('Ctrl Pts',(-3.87409085900006,5.2,2.06159666199999));
#308514=CARTESIAN_POINT('Ctrl Pts',(-3.87409085900006,2.2,2.06159666199999));
#308515=CARTESIAN_POINT('Ctrl Pts',(-3.87286459200006,12.2,2.05999988799999));
#308516=CARTESIAN_POINT('Ctrl Pts',(-3.87286459200006,5.2,2.05999988799999));
#308517=CARTESIAN_POINT('Ctrl Pts',(-3.87286459200006,2.2,2.05999988799999));
#308518=CARTESIAN_POINT('Ctrl Pts',(-3.87163903300006,12.2,2.05840769199999));
#308519=CARTESIAN_POINT('Ctrl Pts',(-3.87163903300006,5.2,2.05840769199999));
#308520=CARTESIAN_POINT('Ctrl Pts',(-3.87163903300006,2.2,2.05840769199999));
#308521=CARTESIAN_POINT('Ctrl Pts',(-3.87041419300005,12.2,2.05682007299998));
#308522=CARTESIAN_POINT('Ctrl Pts',(-3.87041419300005,5.2,2.05682007299998));
#308523=CARTESIAN_POINT('Ctrl Pts',(-3.87041419300005,2.2,2.05682007299998));
#308524=CARTESIAN_POINT('Ctrl Pts',(-3.86919008000006,12.2,2.05523703399999));
#308525=CARTESIAN_POINT('Ctrl Pts',(-3.86919008000006,5.2,2.05523703399999));
#308526=CARTESIAN_POINT('Ctrl Pts',(-3.86919008000006,2.2,2.05523703399999));
#308527=CARTESIAN_POINT('Ctrl Pts',(-3.86796670900006,12.2,2.05365857399999));
#308528=CARTESIAN_POINT('Ctrl Pts',(-3.86796670900006,5.2,2.05365857399999));
#308529=CARTESIAN_POINT('Ctrl Pts',(-3.86796670900006,2.2,2.05365857399999));
#308530=CARTESIAN_POINT('Ctrl Pts',(-3.86674408800006,12.2,2.05208469499999));
#308531=CARTESIAN_POINT('Ctrl Pts',(-3.86674408800006,5.2,2.05208469499999));
#308532=CARTESIAN_POINT('Ctrl Pts',(-3.86674408800006,2.2,2.05208469499999));
#308533=CARTESIAN_POINT('Ctrl Pts',(-3.86552222900006,12.2,2.05051539699999));
#308534=CARTESIAN_POINT('Ctrl Pts',(-3.86552222900006,5.2,2.05051539699999));
#308535=CARTESIAN_POINT('Ctrl Pts',(-3.86552222900006,2.2,2.05051539699999));
#308536=CARTESIAN_POINT('Ctrl Pts',(-3.86430114200006,12.2,2.04895068199999));
#308537=CARTESIAN_POINT('Ctrl Pts',(-3.86430114200006,5.2,2.04895068199999));
#308538=CARTESIAN_POINT('Ctrl Pts',(-3.86430114200006,2.2,2.04895068199999));
#308539=CARTESIAN_POINT('Ctrl Pts',(-3.86308083900006,12.2,2.04739054899999));
#308540=CARTESIAN_POINT('Ctrl Pts',(-3.86308083900006,5.2,2.04739054899999));
#308541=CARTESIAN_POINT('Ctrl Pts',(-3.86308083900006,2.2,2.04739054899999));
#308542=CARTESIAN_POINT('Ctrl Pts',(-3.86186133000006,12.2,2.04583499999998));
#308543=CARTESIAN_POINT('Ctrl Pts',(-3.86186133000006,5.2,2.04583499999998));
#308544=CARTESIAN_POINT('Ctrl Pts',(-3.86186133000006,2.2,2.04583499999998));
#308545=CARTESIAN_POINT('Ctrl Pts',(-3.86064262700006,12.2,2.04428403499998));
#308546=CARTESIAN_POINT('Ctrl Pts',(-3.86064262700006,5.2,2.04428403499998));
#308547=CARTESIAN_POINT('Ctrl Pts',(-3.86064262700006,2.2,2.04428403499998));
#308548=CARTESIAN_POINT('Ctrl Pts',(-3.85942474000006,12.2,2.04273765499998));
#308549=CARTESIAN_POINT('Ctrl Pts',(-3.85942474000006,5.2,2.04273765499998));
#308550=CARTESIAN_POINT('Ctrl Pts',(-3.85942474000006,2.2,2.04273765499998));
#308551=CARTESIAN_POINT('Ctrl Pts',(-3.85820768000006,12.2,2.04119585999999));
#308552=CARTESIAN_POINT('Ctrl Pts',(-3.85820768000006,5.2,2.04119585999999));
#308553=CARTESIAN_POINT('Ctrl Pts',(-3.85820768000006,2.2,2.04119585999999));
#308554=CARTESIAN_POINT('Ctrl Pts',(-3.85699145900006,12.2,2.03965865299998));
#308555=CARTESIAN_POINT('Ctrl Pts',(-3.85699145900006,5.2,2.03965865299998));
#308556=CARTESIAN_POINT('Ctrl Pts',(-3.85699145900006,2.2,2.03965865299998));
#308557=CARTESIAN_POINT('Ctrl Pts',(-3.85577608800006,12.2,2.03812603199998));
#308558=CARTESIAN_POINT('Ctrl Pts',(-3.85577608800006,5.2,2.03812603199998));
#308559=CARTESIAN_POINT('Ctrl Pts',(-3.85577608800006,2.2,2.03812603199998));
#308560=CARTESIAN_POINT('Ctrl Pts',(-3.85456157700006,12.2,2.03659799799999));
#308561=CARTESIAN_POINT('Ctrl Pts',(-3.85456157700006,5.2,2.03659799799999));
#308562=CARTESIAN_POINT('Ctrl Pts',(-3.85456157700006,2.2,2.03659799799999));
#308563=CARTESIAN_POINT('Ctrl Pts',(-3.85334793700006,12.2,2.03507455299999));
#308564=CARTESIAN_POINT('Ctrl Pts',(-3.85334793700006,5.2,2.03507455299999));
#308565=CARTESIAN_POINT('Ctrl Pts',(-3.85334793700006,2.2,2.03507455299999));
#308566=CARTESIAN_POINT('Ctrl Pts',(-3.85213518000006,12.2,2.03355569699998));
#308567=CARTESIAN_POINT('Ctrl Pts',(-3.85213518000006,5.2,2.03355569699998));
#308568=CARTESIAN_POINT('Ctrl Pts',(-3.85213518000006,2.2,2.03355569699998));
#308569=CARTESIAN_POINT('Ctrl Pts',(-3.85092331700006,12.2,2.03204142899999));
#308570=CARTESIAN_POINT('Ctrl Pts',(-3.85092331700006,5.2,2.03204142899999));
#308571=CARTESIAN_POINT('Ctrl Pts',(-3.85092331700006,2.2,2.03204142899999));
#308572=CARTESIAN_POINT('Ctrl Pts',(-3.84971235800006,12.2,2.03053175199999));
#308573=CARTESIAN_POINT('Ctrl Pts',(-3.84971235800006,5.2,2.03053175199999));
#308574=CARTESIAN_POINT('Ctrl Pts',(-3.84971235800006,2.2,2.03053175199999));
#308575=CARTESIAN_POINT('Ctrl Pts',(-3.84850231600006,12.2,2.02902666499998));
#308576=CARTESIAN_POINT('Ctrl Pts',(-3.84850231600006,5.2,2.02902666499998));
#308577=CARTESIAN_POINT('Ctrl Pts',(-3.84850231600006,2.2,2.02902666499998));
#308578=CARTESIAN_POINT('Ctrl Pts',(-3.84729320100006,12.2,2.02752616999998));
#308579=CARTESIAN_POINT('Ctrl Pts',(-3.84729320100006,5.2,2.02752616999998));
#308580=CARTESIAN_POINT('Ctrl Pts',(-3.84729320100006,2.2,2.02752616999998));
#308581=CARTESIAN_POINT('Ctrl Pts',(-3.84608502400006,12.2,2.02603026699999));
#308582=CARTESIAN_POINT('Ctrl Pts',(-3.84608502400006,5.2,2.02603026699999));
#308583=CARTESIAN_POINT('Ctrl Pts',(-3.84608502400006,2.2,2.02603026699999));
#308584=CARTESIAN_POINT('Ctrl Pts',(-3.84487779800006,12.2,2.02453895399998));
#308585=CARTESIAN_POINT('Ctrl Pts',(-3.84487779800006,5.2,2.02453895399998));
#308586=CARTESIAN_POINT('Ctrl Pts',(-3.84487779800006,2.2,2.02453895399998));
#308587=CARTESIAN_POINT('Ctrl Pts',(-3.84367153100006,12.2,2.02305223599998));
#308588=CARTESIAN_POINT('Ctrl Pts',(-3.84367153100006,5.2,2.02305223599998));
#308589=CARTESIAN_POINT('Ctrl Pts',(-3.84367153100006,2.2,2.02305223599998));
#308590=CARTESIAN_POINT('Ctrl Pts',(-3.84246623700006,12.2,2.02157010999999));
#308591=CARTESIAN_POINT('Ctrl Pts',(-3.84246623700006,5.2,2.02157010999999));
#308592=CARTESIAN_POINT('Ctrl Pts',(-3.84246623700006,2.2,2.02157010999999));
#308593=CARTESIAN_POINT('Ctrl Pts',(-3.84126192700006,12.2,2.02009257799999));
#308594=CARTESIAN_POINT('Ctrl Pts',(-3.84126192700006,5.2,2.02009257799999));
#308595=CARTESIAN_POINT('Ctrl Pts',(-3.84126192700006,2.2,2.02009257799999));
#308596=CARTESIAN_POINT('Ctrl Pts',(-3.84005861100006,12.2,2.01861963999999));
#308597=CARTESIAN_POINT('Ctrl Pts',(-3.84005861100006,5.2,2.01861963999999));
#308598=CARTESIAN_POINT('Ctrl Pts',(-3.84005861100006,2.2,2.01861963999999));
#308599=CARTESIAN_POINT('Ctrl Pts',(-3.83885630100006,12.2,2.01715129799998));
#308600=CARTESIAN_POINT('Ctrl Pts',(-3.83885630100006,5.2,2.01715129799998));
#308601=CARTESIAN_POINT('Ctrl Pts',(-3.83885630100006,2.2,2.01715129799998));
#308602=CARTESIAN_POINT('Ctrl Pts',(-3.83765500700005,12.2,2.01568754899998));
#308603=CARTESIAN_POINT('Ctrl Pts',(-3.83765500700005,5.2,2.01568754899998));
#308604=CARTESIAN_POINT('Ctrl Pts',(-3.83765500700005,2.2,2.01568754899998));
#308605=CARTESIAN_POINT('Ctrl Pts',(-3.83645474300006,12.2,2.01422839599998));
#308606=CARTESIAN_POINT('Ctrl Pts',(-3.83645474300006,5.2,2.01422839599998));
#308607=CARTESIAN_POINT('Ctrl Pts',(-3.83645474300006,2.2,2.01422839599998));
#308608=CARTESIAN_POINT('Ctrl Pts',(-3.83525551800005,12.2,2.01277383899999));
#308609=CARTESIAN_POINT('Ctrl Pts',(-3.83525551800005,5.2,2.01277383899999));
#308610=CARTESIAN_POINT('Ctrl Pts',(-3.83525551800005,2.2,2.01277383899999));
#308611=CARTESIAN_POINT('Ctrl Pts',(-3.83405734600006,12.2,2.01132387799999));
#308612=CARTESIAN_POINT('Ctrl Pts',(-3.83405734600006,5.2,2.01132387799999));
#308613=CARTESIAN_POINT('Ctrl Pts',(-3.83405734600006,2.2,2.01132387799999));
#308614=CARTESIAN_POINT('Ctrl Pts',(-3.83286023400006,12.2,2.00987851499999));
#308615=CARTESIAN_POINT('Ctrl Pts',(-3.83286023400006,5.2,2.00987851499999));
#308616=CARTESIAN_POINT('Ctrl Pts',(-3.83286023400006,2.2,2.00987851499999));
#308617=CARTESIAN_POINT('Ctrl Pts',(-3.83166419800006,12.2,2.00843774699999));
#308618=CARTESIAN_POINT('Ctrl Pts',(-3.83166419800006,5.2,2.00843774699999));
#308619=CARTESIAN_POINT('Ctrl Pts',(-3.83166419800006,2.2,2.00843774699999));
#308620=CARTESIAN_POINT('Ctrl Pts',(-3.83046924700006,12.2,2.00700157699998));
#308621=CARTESIAN_POINT('Ctrl Pts',(-3.83046924700006,5.2,2.00700157699998));
#308622=CARTESIAN_POINT('Ctrl Pts',(-3.83046924700006,2.2,2.00700157699998));
#308623=CARTESIAN_POINT('Ctrl Pts',(-3.82927539400006,12.2,2.00557000499999));
#308624=CARTESIAN_POINT('Ctrl Pts',(-3.82927539400006,5.2,2.00557000499999));
#308625=CARTESIAN_POINT('Ctrl Pts',(-3.82927539400006,2.2,2.00557000499999));
#308626=CARTESIAN_POINT('Ctrl Pts',(-3.82808264900006,12.2,2.00414303099999));
#308627=CARTESIAN_POINT('Ctrl Pts',(-3.82808264900006,5.2,2.00414303099999));
#308628=CARTESIAN_POINT('Ctrl Pts',(-3.82808264900006,2.2,2.00414303099999));
#308629=CARTESIAN_POINT('Ctrl Pts',(-3.82689102400006,12.2,2.00272065499998));
#308630=CARTESIAN_POINT('Ctrl Pts',(-3.82689102400006,5.2,2.00272065499998));
#308631=CARTESIAN_POINT('Ctrl Pts',(-3.82689102400006,2.2,2.00272065499998));
#308632=CARTESIAN_POINT('Ctrl Pts',(-3.82570053100006,12.2,2.00130287699999));
#308633=CARTESIAN_POINT('Ctrl Pts',(-3.82570053100006,5.2,2.00130287699999));
#308634=CARTESIAN_POINT('Ctrl Pts',(-3.82570053100006,2.2,2.00130287699999));
#308635=CARTESIAN_POINT('Ctrl Pts',(-3.82451118100006,12.2,1.99988969899998));
#308636=CARTESIAN_POINT('Ctrl Pts',(-3.82451118100006,5.2,1.99988969899998));
#308637=CARTESIAN_POINT('Ctrl Pts',(-3.82451118100006,2.2,1.99988969899998));
#308638=CARTESIAN_POINT('Ctrl Pts',(-3.82332298400006,12.2,1.99848111899998));
#308639=CARTESIAN_POINT('Ctrl Pts',(-3.82332298400006,5.2,1.99848111899998));
#308640=CARTESIAN_POINT('Ctrl Pts',(-3.82332298400006,2.2,1.99848111899998));
#308641=CARTESIAN_POINT('Ctrl Pts',(-3.82213595500006,12.2,1.99707713899999));
#308642=CARTESIAN_POINT('Ctrl Pts',(-3.82213595500006,5.2,1.99707713899999));
#308643=CARTESIAN_POINT('Ctrl Pts',(-3.82213595500006,2.2,1.99707713899999));
#308644=CARTESIAN_POINT('Ctrl Pts',(-3.82095010300006,12.2,1.99567775799999));
#308645=CARTESIAN_POINT('Ctrl Pts',(-3.82095010300006,5.2,1.99567775799999));
#308646=CARTESIAN_POINT('Ctrl Pts',(-3.82095010300006,2.2,1.99567775799999));
#308647=CARTESIAN_POINT('Ctrl Pts',(-3.81976544100006,12.2,1.99428297799999));
#308648=CARTESIAN_POINT('Ctrl Pts',(-3.81976544100006,5.2,1.99428297799999));
#308649=CARTESIAN_POINT('Ctrl Pts',(-3.81976544100006,2.2,1.99428297799999));
#308650=CARTESIAN_POINT('Ctrl Pts',(-3.81858197900006,12.2,1.99289279599999));
#308651=CARTESIAN_POINT('Ctrl Pts',(-3.81858197900006,5.2,1.99289279599999));
#308652=CARTESIAN_POINT('Ctrl Pts',(-3.81858197900006,2.2,1.99289279599999));
#308653=CARTESIAN_POINT('Ctrl Pts',(-3.81739973200006,12.2,1.99150721599999));
#308654=CARTESIAN_POINT('Ctrl Pts',(-3.81739973200006,5.2,1.99150721599999));
#308655=CARTESIAN_POINT('Ctrl Pts',(-3.81739973200006,2.2,1.99150721599999));
#308656=CARTESIAN_POINT('Ctrl Pts',(-3.81621870800006,12.2,1.99012623499998));
#308657=CARTESIAN_POINT('Ctrl Pts',(-3.81621870800006,5.2,1.99012623499998));
#308658=CARTESIAN_POINT('Ctrl Pts',(-3.81621870800006,2.2,1.99012623499998));
#308659=CARTESIAN_POINT('Ctrl Pts',(-3.81503891900006,12.2,1.98874985499998));
#308660=CARTESIAN_POINT('Ctrl Pts',(-3.81503891900006,5.2,1.98874985499998));
#308661=CARTESIAN_POINT('Ctrl Pts',(-3.81503891900006,2.2,1.98874985499998));
#308662=CARTESIAN_POINT('Ctrl Pts',(-3.81386038000006,12.2,1.98737807599999));
#308663=CARTESIAN_POINT('Ctrl Pts',(-3.81386038000006,5.2,1.98737807599999));
#308664=CARTESIAN_POINT('Ctrl Pts',(-3.81386038000006,2.2,1.98737807599999));
#308665=CARTESIAN_POINT('Ctrl Pts',(-3.81268309900006,12.2,1.98601089699999));
#308666=CARTESIAN_POINT('Ctrl Pts',(-3.81268309900006,5.2,1.98601089699999));
#308667=CARTESIAN_POINT('Ctrl Pts',(-3.81268309900006,2.2,1.98601089699999));
#308668=CARTESIAN_POINT('Ctrl Pts',(-3.81150709100006,12.2,1.98464831899999));
#308669=CARTESIAN_POINT('Ctrl Pts',(-3.81150709100006,5.2,1.98464831899999));
#308670=CARTESIAN_POINT('Ctrl Pts',(-3.81150709100006,2.2,1.98464831899999));
#308671=CARTESIAN_POINT('Ctrl Pts',(-3.81033236500006,12.2,1.98329034199999));
#308672=CARTESIAN_POINT('Ctrl Pts',(-3.81033236500006,5.2,1.98329034199999));
#308673=CARTESIAN_POINT('Ctrl Pts',(-3.81033236500006,2.2,1.98329034199999));
#308674=CARTESIAN_POINT('Ctrl Pts',(-3.80915893500006,12.2,1.98193696599999));
#308675=CARTESIAN_POINT('Ctrl Pts',(-3.80915893500006,5.2,1.98193696599999));
#308676=CARTESIAN_POINT('Ctrl Pts',(-3.80915893500006,2.2,1.98193696599999));
#308677=CARTESIAN_POINT('Ctrl Pts',(-3.80798681000006,12.2,1.98058818999999));
#308678=CARTESIAN_POINT('Ctrl Pts',(-3.80798681000006,5.2,1.98058818999999));
#308679=CARTESIAN_POINT('Ctrl Pts',(-3.80798681000006,2.2,1.98058818999999));
#308680=CARTESIAN_POINT('Ctrl Pts',(-3.80681600500006,12.2,1.97924401599999));
#308681=CARTESIAN_POINT('Ctrl Pts',(-3.80681600500006,5.2,1.97924401599999));
#308682=CARTESIAN_POINT('Ctrl Pts',(-3.80681600500006,2.2,1.97924401599999));
#308683=CARTESIAN_POINT('Ctrl Pts',(-3.80564653100006,12.2,1.97790444299998));
#308684=CARTESIAN_POINT('Ctrl Pts',(-3.80564653100006,5.2,1.97790444299998));
#308685=CARTESIAN_POINT('Ctrl Pts',(-3.80564653100006,2.2,1.97790444299998));
#308686=CARTESIAN_POINT('Ctrl Pts',(-3.80447839700006,12.2,1.97656947099999));
#308687=CARTESIAN_POINT('Ctrl Pts',(-3.80447839700006,5.2,1.97656947099999));
#308688=CARTESIAN_POINT('Ctrl Pts',(-3.80447839700006,2.2,1.97656947099999));
#308689=CARTESIAN_POINT('Ctrl Pts',(-3.80331162000005,12.2,1.97523910099999));
#308690=CARTESIAN_POINT('Ctrl Pts',(-3.80331162000005,5.2,1.97523910099999));
#308691=CARTESIAN_POINT('Ctrl Pts',(-3.80331162000005,2.2,1.97523910099999));
#308692=CARTESIAN_POINT('Ctrl Pts',(-3.80214620800006,12.2,1.97391332999999));
#308693=CARTESIAN_POINT('Ctrl Pts',(-3.80214620800006,5.2,1.97391332999999));
#308694=CARTESIAN_POINT('Ctrl Pts',(-3.80214620800006,2.2,1.97391332999999));
#308695=CARTESIAN_POINT('Ctrl Pts',(-3.80098217400006,12.2,1.97259216199999));
#308696=CARTESIAN_POINT('Ctrl Pts',(-3.80098217400006,5.2,1.97259216199999));
#308697=CARTESIAN_POINT('Ctrl Pts',(-3.80098217400006,2.2,1.97259216199999));
#308698=CARTESIAN_POINT('Ctrl Pts',(-3.79981953100006,12.2,1.97127559299998));
#308699=CARTESIAN_POINT('Ctrl Pts',(-3.79981953100006,5.2,1.97127559299998));
#308700=CARTESIAN_POINT('Ctrl Pts',(-3.79981953100006,2.2,1.97127559299998));
#308701=CARTESIAN_POINT('Ctrl Pts',(-3.79865829000006,12.2,1.96996362599998));
#308702=CARTESIAN_POINT('Ctrl Pts',(-3.79865829000006,5.2,1.96996362599998));
#308703=CARTESIAN_POINT('Ctrl Pts',(-3.79865829000006,2.2,1.96996362599998));
#308704=CARTESIAN_POINT('Ctrl Pts',(-3.79749846300006,12.2,1.96865625899999));
#308705=CARTESIAN_POINT('Ctrl Pts',(-3.79749846300006,5.2,1.96865625899999));
#308706=CARTESIAN_POINT('Ctrl Pts',(-3.79749846300006,2.2,1.96865625899999));
#308707=CARTESIAN_POINT('Ctrl Pts',(-3.79634006200006,12.2,1.96735349499999));
#308708=CARTESIAN_POINT('Ctrl Pts',(-3.79634006200006,5.2,1.96735349499999));
#308709=CARTESIAN_POINT('Ctrl Pts',(-3.79634006200006,2.2,1.96735349499999));
#308710=CARTESIAN_POINT('Ctrl Pts',(-3.79518310000006,12.2,1.96605532899999));
#308711=CARTESIAN_POINT('Ctrl Pts',(-3.79518310000006,5.2,1.96605532899999));
#308712=CARTESIAN_POINT('Ctrl Pts',(-3.79518310000006,2.2,1.96605532899999));
#308713=CARTESIAN_POINT('Ctrl Pts',(-3.79402758800006,12.2,1.96476176399999));
#308714=CARTESIAN_POINT('Ctrl Pts',(-3.79402758800006,5.2,1.96476176399999));
#308715=CARTESIAN_POINT('Ctrl Pts',(-3.79402758800006,2.2,1.96476176399999));
#308716=CARTESIAN_POINT('Ctrl Pts',(-3.79287353800006,12.2,1.96347279899999));
#308717=CARTESIAN_POINT('Ctrl Pts',(-3.79287353800006,5.2,1.96347279899999));
#308718=CARTESIAN_POINT('Ctrl Pts',(-3.79287353800006,2.2,1.96347279899999));
#308719=CARTESIAN_POINT('Ctrl Pts',(-3.79172096300006,12.2,1.96218843399999));
#308720=CARTESIAN_POINT('Ctrl Pts',(-3.79172096300006,5.2,1.96218843399999));
#308721=CARTESIAN_POINT('Ctrl Pts',(-3.79172096300006,2.2,1.96218843399999));
#308722=CARTESIAN_POINT('Ctrl Pts',(-3.79056987400006,12.2,1.96090866999999));
#308723=CARTESIAN_POINT('Ctrl Pts',(-3.79056987400006,5.2,1.96090866999999));
#308724=CARTESIAN_POINT('Ctrl Pts',(-3.79056987400006,2.2,1.96090866999999));
#308725=CARTESIAN_POINT('Ctrl Pts',(-3.78942028500005,12.2,1.95963350399999));
#308726=CARTESIAN_POINT('Ctrl Pts',(-3.78942028500005,5.2,1.95963350399999));
#308727=CARTESIAN_POINT('Ctrl Pts',(-3.78942028500005,2.2,1.95963350399999));
#308728=CARTESIAN_POINT('Ctrl Pts',(-3.78827220700006,12.2,1.95836293899998));
#308729=CARTESIAN_POINT('Ctrl Pts',(-3.78827220700006,5.2,1.95836293899998));
#308730=CARTESIAN_POINT('Ctrl Pts',(-3.78827220700006,2.2,1.95836293899998));
#308731=CARTESIAN_POINT('Ctrl Pts',(-3.78712565200006,12.2,1.95709697199999));
#308732=CARTESIAN_POINT('Ctrl Pts',(-3.78712565200006,5.2,1.95709697199999));
#308733=CARTESIAN_POINT('Ctrl Pts',(-3.78712565200006,2.2,1.95709697199999));
#308734=CARTESIAN_POINT('Ctrl Pts',(-3.78598063200006,12.2,1.95583560399998));
#308735=CARTESIAN_POINT('Ctrl Pts',(-3.78598063200006,5.2,1.95583560399998));
#308736=CARTESIAN_POINT('Ctrl Pts',(-3.78598063200006,2.2,1.95583560399998));
#308737=CARTESIAN_POINT('Ctrl Pts',(-3.78483716200006,12.2,1.95457883599999));
#308738=CARTESIAN_POINT('Ctrl Pts',(-3.78483716200006,5.2,1.95457883599999));
#308739=CARTESIAN_POINT('Ctrl Pts',(-3.78483716200006,2.2,1.95457883599999));
#308740=CARTESIAN_POINT('Ctrl Pts',(-3.78369525000006,12.2,1.95332666499999));
#308741=CARTESIAN_POINT('Ctrl Pts',(-3.78369525000006,5.2,1.95332666499999));
#308742=CARTESIAN_POINT('Ctrl Pts',(-3.78369525000006,2.2,1.95332666499999));
#308743=CARTESIAN_POINT('Ctrl Pts',(-3.78255491200005,12.2,1.95207909299999));
#308744=CARTESIAN_POINT('Ctrl Pts',(-3.78255491200005,5.2,1.95207909299999));
#308745=CARTESIAN_POINT('Ctrl Pts',(-3.78255491200005,2.2,1.95207909299999));
#308746=CARTESIAN_POINT('Ctrl Pts',(-3.78141615700006,12.2,1.95083611699999));
#308747=CARTESIAN_POINT('Ctrl Pts',(-3.78141615700006,5.2,1.95083611699999));
#308748=CARTESIAN_POINT('Ctrl Pts',(-3.78141615700006,2.2,1.95083611699999));
#308749=CARTESIAN_POINT('Ctrl Pts',(-3.78027899900006,12.2,1.94959773899999));
#308750=CARTESIAN_POINT('Ctrl Pts',(-3.78027899900006,5.2,1.94959773899999));
#308751=CARTESIAN_POINT('Ctrl Pts',(-3.78027899900006,2.2,1.94959773899999));
#308752=CARTESIAN_POINT('Ctrl Pts',(-3.77914345200006,12.2,1.94836395899999));
#308753=CARTESIAN_POINT('Ctrl Pts',(-3.77914345200006,5.2,1.94836395899999));
#308754=CARTESIAN_POINT('Ctrl Pts',(-3.77914345200006,2.2,1.94836395899999));
#308755=CARTESIAN_POINT('Ctrl Pts',(-3.77800952600006,12.2,1.94713477499999));
#308756=CARTESIAN_POINT('Ctrl Pts',(-3.77800952600006,5.2,1.94713477499999));
#308757=CARTESIAN_POINT('Ctrl Pts',(-3.77800952600006,2.2,1.94713477499999));
#308758=CARTESIAN_POINT('Ctrl Pts',(-3.77687723500006,12.2,1.94591018699999));
#308759=CARTESIAN_POINT('Ctrl Pts',(-3.77687723500006,5.2,1.94591018699999));
#308760=CARTESIAN_POINT('Ctrl Pts',(-3.77687723500006,2.2,1.94591018699999));
#308761=CARTESIAN_POINT('Ctrl Pts',(-3.77574659000006,12.2,1.94469019499998));
#308762=CARTESIAN_POINT('Ctrl Pts',(-3.77574659000006,5.2,1.94469019499998));
#308763=CARTESIAN_POINT('Ctrl Pts',(-3.77574659000006,2.2,1.94469019499998));
#308764=CARTESIAN_POINT('Ctrl Pts',(-3.77461760400006,12.2,1.94347479799998));
#308765=CARTESIAN_POINT('Ctrl Pts',(-3.77461760400006,5.2,1.94347479799998));
#308766=CARTESIAN_POINT('Ctrl Pts',(-3.77461760400006,2.2,1.94347479799998));
#308767=CARTESIAN_POINT('Ctrl Pts',(-3.77349028900006,12.2,1.94226399599998));
#308768=CARTESIAN_POINT('Ctrl Pts',(-3.77349028900006,5.2,1.94226399599998));
#308769=CARTESIAN_POINT('Ctrl Pts',(-3.77349028900006,2.2,1.94226399599998));
#308770=CARTESIAN_POINT('Ctrl Pts',(-3.77236465900006,12.2,1.94105778899999));
#308771=CARTESIAN_POINT('Ctrl Pts',(-3.77236465900006,5.2,1.94105778899999));
#308772=CARTESIAN_POINT('Ctrl Pts',(-3.77236465900006,2.2,1.94105778899999));
#308773=CARTESIAN_POINT('Ctrl Pts',(-3.77124072700005,12.2,1.93985617599999));
#308774=CARTESIAN_POINT('Ctrl Pts',(-3.77124072700005,5.2,1.93985617599999));
#308775=CARTESIAN_POINT('Ctrl Pts',(-3.77124072700005,2.2,1.93985617599999));
#308776=CARTESIAN_POINT('Ctrl Pts',(-3.77011850300006,12.2,1.93865915599998));
#308777=CARTESIAN_POINT('Ctrl Pts',(-3.77011850300006,5.2,1.93865915599998));
#308778=CARTESIAN_POINT('Ctrl Pts',(-3.77011850300006,2.2,1.93865915599998));
#308779=CARTESIAN_POINT('Ctrl Pts',(-3.76899800000006,12.2,1.93746672799998));
#308780=CARTESIAN_POINT('Ctrl Pts',(-3.76899800000006,5.2,1.93746672799998));
#308781=CARTESIAN_POINT('Ctrl Pts',(-3.76899800000006,2.2,1.93746672799998));
#308782=CARTESIAN_POINT('Ctrl Pts',(-3.76787923300006,12.2,1.93627889399998));
#308783=CARTESIAN_POINT('Ctrl Pts',(-3.76787923300006,5.2,1.93627889399998));
#308784=CARTESIAN_POINT('Ctrl Pts',(-3.76787923300006,2.2,1.93627889399998));
#308785=CARTESIAN_POINT('Ctrl Pts',(-3.76676221100006,12.2,1.93509564999998));
#308786=CARTESIAN_POINT('Ctrl Pts',(-3.76676221100006,5.2,1.93509564999998));
#308787=CARTESIAN_POINT('Ctrl Pts',(-3.76676221100006,2.2,1.93509564999998));
#308788=CARTESIAN_POINT('Ctrl Pts',(-3.76564695000006,12.2,1.93391699899998));
#308789=CARTESIAN_POINT('Ctrl Pts',(-3.76564695000006,5.2,1.93391699899998));
#308790=CARTESIAN_POINT('Ctrl Pts',(-3.76564695000006,2.2,1.93391699899998));
#308791=CARTESIAN_POINT('Ctrl Pts',(-3.76453346100006,12.2,1.93274293799998));
#308792=CARTESIAN_POINT('Ctrl Pts',(-3.76453346100006,5.2,1.93274293799998));
#308793=CARTESIAN_POINT('Ctrl Pts',(-3.76453346100006,2.2,1.93274293799998));
#308794=CARTESIAN_POINT('Ctrl Pts',(-3.76342175700006,12.2,1.93157346699998));
#308795=CARTESIAN_POINT('Ctrl Pts',(-3.76342175700006,5.2,1.93157346699998));
#308796=CARTESIAN_POINT('Ctrl Pts',(-3.76342175700006,2.2,1.93157346699998));
#308797=CARTESIAN_POINT('Ctrl Pts',(-3.76231185100006,12.2,1.93040858599999));
#308798=CARTESIAN_POINT('Ctrl Pts',(-3.76231185100006,5.2,1.93040858599999));
#308799=CARTESIAN_POINT('Ctrl Pts',(-3.76231185100006,2.2,1.93040858599999));
#308800=CARTESIAN_POINT('Ctrl Pts',(-3.76120375500006,12.2,1.92924829299999));
#308801=CARTESIAN_POINT('Ctrl Pts',(-3.76120375500006,5.2,1.92924829299999));
#308802=CARTESIAN_POINT('Ctrl Pts',(-3.76120375500006,2.2,1.92924829299999));
#308803=CARTESIAN_POINT('Ctrl Pts',(-3.76009748200006,12.2,1.92809258799999));
#308804=CARTESIAN_POINT('Ctrl Pts',(-3.76009748200006,5.2,1.92809258799999));
#308805=CARTESIAN_POINT('Ctrl Pts',(-3.76009748200006,2.2,1.92809258799999));
#308806=CARTESIAN_POINT('Ctrl Pts',(-3.75899304500006,12.2,1.92694146999999));
#308807=CARTESIAN_POINT('Ctrl Pts',(-3.75899304500006,5.2,1.92694146999999));
#308808=CARTESIAN_POINT('Ctrl Pts',(-3.75899304500006,2.2,1.92694146999999));
#308809=CARTESIAN_POINT('Ctrl Pts',(-3.75789045700006,12.2,1.92579493999999));
#308810=CARTESIAN_POINT('Ctrl Pts',(-3.75789045700006,5.2,1.92579493999999));
#308811=CARTESIAN_POINT('Ctrl Pts',(-3.75789045700006,2.2,1.92579493999999));
#308812=CARTESIAN_POINT('Ctrl Pts',(-3.75678973100006,12.2,1.92465299499998));
#308813=CARTESIAN_POINT('Ctrl Pts',(-3.75678973100006,5.2,1.92465299499998));
#308814=CARTESIAN_POINT('Ctrl Pts',(-3.75678973100006,2.2,1.92465299499998));
#308815=CARTESIAN_POINT('Ctrl Pts',(-3.75569087900006,12.2,1.92351563499999));
#308816=CARTESIAN_POINT('Ctrl Pts',(-3.75569087900006,5.2,1.92351563499999));
#308817=CARTESIAN_POINT('Ctrl Pts',(-3.75569087900006,2.2,1.92351563499999));
#308818=CARTESIAN_POINT('Ctrl Pts',(-3.75459391600006,12.2,1.92238285999998));
#308819=CARTESIAN_POINT('Ctrl Pts',(-3.75459391600006,5.2,1.92238285999998));
#308820=CARTESIAN_POINT('Ctrl Pts',(-3.75459391600006,2.2,1.92238285999998));
#308821=CARTESIAN_POINT('Ctrl Pts',(-3.75349885100006,12.2,1.92125466899999));
#308822=CARTESIAN_POINT('Ctrl Pts',(-3.75349885100006,5.2,1.92125466899999));
#308823=CARTESIAN_POINT('Ctrl Pts',(-3.75349885100006,2.2,1.92125466899999));
#308824=CARTESIAN_POINT('Ctrl Pts',(-3.75240570000006,12.2,1.92013106099999));
#308825=CARTESIAN_POINT('Ctrl Pts',(-3.75240570000006,5.2,1.92013106099999));
#308826=CARTESIAN_POINT('Ctrl Pts',(-3.75240570000006,2.2,1.92013106099999));
#308827=CARTESIAN_POINT('Ctrl Pts',(-3.75131447600006,12.2,1.91901203499999));
#308828=CARTESIAN_POINT('Ctrl Pts',(-3.75131447600006,5.2,1.91901203499999));
#308829=CARTESIAN_POINT('Ctrl Pts',(-3.75131447600006,2.2,1.91901203499999));
#308830=CARTESIAN_POINT('Ctrl Pts',(-3.75022519000006,12.2,1.91789758999999));
#308831=CARTESIAN_POINT('Ctrl Pts',(-3.75022519000006,5.2,1.91789758999999));
#308832=CARTESIAN_POINT('Ctrl Pts',(-3.75022519000006,2.2,1.91789758999999));
#308833=CARTESIAN_POINT('Ctrl Pts',(-3.74913785700006,12.2,1.91678772499999));
#308834=CARTESIAN_POINT('Ctrl Pts',(-3.74913785700006,5.2,1.91678772499999));
#308835=CARTESIAN_POINT('Ctrl Pts',(-3.74913785700006,2.2,1.91678772499999));
#308836=CARTESIAN_POINT('Ctrl Pts',(-3.74805248800006,12.2,1.91568243999999));
#308837=CARTESIAN_POINT('Ctrl Pts',(-3.74805248800006,5.2,1.91568243999999));
#308838=CARTESIAN_POINT('Ctrl Pts',(-3.74805248800006,2.2,1.91568243999999));
#308839=CARTESIAN_POINT('Ctrl Pts',(-3.74696909800006,12.2,1.91458173299999));
#308840=CARTESIAN_POINT('Ctrl Pts',(-3.74696909800006,5.2,1.91458173299999));
#308841=CARTESIAN_POINT('Ctrl Pts',(-3.74696909800006,2.2,1.91458173299999));
#308842=CARTESIAN_POINT('Ctrl Pts',(-3.74588770000006,12.2,1.91348560399998));
#308843=CARTESIAN_POINT('Ctrl Pts',(-3.74588770000006,5.2,1.91348560399998));
#308844=CARTESIAN_POINT('Ctrl Pts',(-3.74588770000006,2.2,1.91348560399998));
#308845=CARTESIAN_POINT('Ctrl Pts',(-3.74480830500006,12.2,1.91239405099998));
#308846=CARTESIAN_POINT('Ctrl Pts',(-3.74480830500006,5.2,1.91239405099998));
#308847=CARTESIAN_POINT('Ctrl Pts',(-3.74480830500006,2.2,1.91239405099998));
#308848=CARTESIAN_POINT('Ctrl Pts',(-3.74373092900006,12.2,1.91130707499998));
#308849=CARTESIAN_POINT('Ctrl Pts',(-3.74373092900006,5.2,1.91130707499998));
#308850=CARTESIAN_POINT('Ctrl Pts',(-3.74373092900006,2.2,1.91130707499998));
#308851=CARTESIAN_POINT('Ctrl Pts',(-3.74265558200006,12.2,1.91022467399999));
#308852=CARTESIAN_POINT('Ctrl Pts',(-3.74265558200006,5.2,1.91022467399999));
#308853=CARTESIAN_POINT('Ctrl Pts',(-3.74265558200006,2.2,1.91022467399999));
#308854=CARTESIAN_POINT('Ctrl Pts',(-3.74158227900006,12.2,1.90914684599999));
#308855=CARTESIAN_POINT('Ctrl Pts',(-3.74158227900006,5.2,1.90914684599999));
#308856=CARTESIAN_POINT('Ctrl Pts',(-3.74158227900006,2.2,1.90914684599999));
#308857=CARTESIAN_POINT('Ctrl Pts',(-3.74051103400006,12.2,1.90807359099999));
#308858=CARTESIAN_POINT('Ctrl Pts',(-3.74051103400006,5.2,1.90807359099999));
#308859=CARTESIAN_POINT('Ctrl Pts',(-3.74051103400006,2.2,1.90807359099999));
#308860=CARTESIAN_POINT('Ctrl Pts',(-3.73944185800006,12.2,1.90700490799999));
#308861=CARTESIAN_POINT('Ctrl Pts',(-3.73944185800006,5.2,1.90700490799999));
#308862=CARTESIAN_POINT('Ctrl Pts',(-3.73944185800006,2.2,1.90700490799999));
#308863=CARTESIAN_POINT('Ctrl Pts',(-3.73837476700006,12.2,1.90594079599999));
#308864=CARTESIAN_POINT('Ctrl Pts',(-3.73837476700006,5.2,1.90594079599999));
#308865=CARTESIAN_POINT('Ctrl Pts',(-3.73837476700006,2.2,1.90594079599999));
#308866=CARTESIAN_POINT('Ctrl Pts',(-3.73730977200006,12.2,1.90488125399999));
#308867=CARTESIAN_POINT('Ctrl Pts',(-3.73730977200006,5.2,1.90488125399999));
#308868=CARTESIAN_POINT('Ctrl Pts',(-3.73730977200006,2.2,1.90488125399999));
#308869=CARTESIAN_POINT('Ctrl Pts',(-3.73624688700006,12.2,1.90382627899998));
#308870=CARTESIAN_POINT('Ctrl Pts',(-3.73624688700006,5.2,1.90382627899998));
#308871=CARTESIAN_POINT('Ctrl Pts',(-3.73624688700006,2.2,1.90382627899998));
#308872=CARTESIAN_POINT('Ctrl Pts',(-3.73518612500006,12.2,1.90277587299999));
#308873=CARTESIAN_POINT('Ctrl Pts',(-3.73518612500006,5.2,1.90277587299999));
#308874=CARTESIAN_POINT('Ctrl Pts',(-3.73518612500006,2.2,1.90277587299999));
#308875=CARTESIAN_POINT('Ctrl Pts',(-3.73412750100006,12.2,1.90173003299998));
#308876=CARTESIAN_POINT('Ctrl Pts',(-3.73412750100006,5.2,1.90173003299998));
#308877=CARTESIAN_POINT('Ctrl Pts',(-3.73412750100006,2.2,1.90173003299998));
#308878=CARTESIAN_POINT('Ctrl Pts',(-3.73307102500006,12.2,1.90068875799998));
#308879=CARTESIAN_POINT('Ctrl Pts',(-3.73307102500006,5.2,1.90068875799998));
#308880=CARTESIAN_POINT('Ctrl Pts',(-3.73307102500006,2.2,1.90068875799998));
#308881=CARTESIAN_POINT('Ctrl Pts',(-3.73201671400006,12.2,1.89965204599998));
#308882=CARTESIAN_POINT('Ctrl Pts',(-3.73201671400006,5.2,1.89965204599998));
#308883=CARTESIAN_POINT('Ctrl Pts',(-3.73201671400006,2.2,1.89965204599998));
#308884=CARTESIAN_POINT('Ctrl Pts',(-3.73096458000005,12.2,1.89861989799998));
#308885=CARTESIAN_POINT('Ctrl Pts',(-3.73096458000005,5.2,1.89861989799998));
#308886=CARTESIAN_POINT('Ctrl Pts',(-3.73096458000005,2.2,1.89861989799998));
#308887=CARTESIAN_POINT('Ctrl Pts',(-3.72991463600005,12.2,1.89759231199998));
#308888=CARTESIAN_POINT('Ctrl Pts',(-3.72991463600005,5.2,1.89759231199998));
#308889=CARTESIAN_POINT('Ctrl Pts',(-3.72991463600005,2.2,1.89759231199998));
#308890=CARTESIAN_POINT('Ctrl Pts',(-3.72886689600006,12.2,1.89656928499998));
#308891=CARTESIAN_POINT('Ctrl Pts',(-3.72886689600006,5.2,1.89656928499998));
#308892=CARTESIAN_POINT('Ctrl Pts',(-3.72886689600006,2.2,1.89656928499998));
#308893=CARTESIAN_POINT('Ctrl Pts',(-3.72782137300006,12.2,1.89555081899998));
#308894=CARTESIAN_POINT('Ctrl Pts',(-3.72782137300006,5.2,1.89555081899998));
#308895=CARTESIAN_POINT('Ctrl Pts',(-3.72782137300006,2.2,1.89555081899998));
#308896=CARTESIAN_POINT('Ctrl Pts',(-3.72677808100006,12.2,1.89453690999999));
#308897=CARTESIAN_POINT('Ctrl Pts',(-3.72677808100006,5.2,1.89453690999999));
#308898=CARTESIAN_POINT('Ctrl Pts',(-3.72677808100006,2.2,1.89453690999999));
#308899=CARTESIAN_POINT('Ctrl Pts',(-3.72573703400006,12.2,1.89352755799999));
#308900=CARTESIAN_POINT('Ctrl Pts',(-3.72573703400006,5.2,1.89352755799999));
#308901=CARTESIAN_POINT('Ctrl Pts',(-3.72573703400006,2.2,1.89352755799999));
#308902=CARTESIAN_POINT('Ctrl Pts',(-3.72469824400006,12.2,1.89252275999999));
#308903=CARTESIAN_POINT('Ctrl Pts',(-3.72469824400006,5.2,1.89252275999999));
#308904=CARTESIAN_POINT('Ctrl Pts',(-3.72469824400006,2.2,1.89252275999999));
#308905=CARTESIAN_POINT('Ctrl Pts',(-3.72366172600006,12.2,1.89152251699999));
#308906=CARTESIAN_POINT('Ctrl Pts',(-3.72366172600006,5.2,1.89152251699999));
#308907=CARTESIAN_POINT('Ctrl Pts',(-3.72366172600006,2.2,1.89152251699999));
#308908=CARTESIAN_POINT('Ctrl Pts',(-3.72262749400006,12.2,1.89052682599999));
#308909=CARTESIAN_POINT('Ctrl Pts',(-3.72262749400006,5.2,1.89052682599999));
#308910=CARTESIAN_POINT('Ctrl Pts',(-3.72262749400006,2.2,1.89052682599999));
#308911=CARTESIAN_POINT('Ctrl Pts',(-3.72159556000006,12.2,1.88953568699999));
#308912=CARTESIAN_POINT('Ctrl Pts',(-3.72159556000006,5.2,1.88953568699999));
#308913=CARTESIAN_POINT('Ctrl Pts',(-3.72159556000006,2.2,1.88953568699999));
#308914=CARTESIAN_POINT('Ctrl Pts',(-3.72056593900006,12.2,1.88854909599999));
#308915=CARTESIAN_POINT('Ctrl Pts',(-3.72056593900006,5.2,1.88854909599999));
#308916=CARTESIAN_POINT('Ctrl Pts',(-3.72056593900006,2.2,1.88854909599999));
#308917=CARTESIAN_POINT('Ctrl Pts',(-3.71953864400006,12.2,1.88756705499999));
#308918=CARTESIAN_POINT('Ctrl Pts',(-3.71953864400006,5.2,1.88756705499999));
#308919=CARTESIAN_POINT('Ctrl Pts',(-3.71953864400006,2.2,1.88756705499999));
#308920=CARTESIAN_POINT('Ctrl Pts',(-3.71851369000006,12.2,1.88658955999998));
#308921=CARTESIAN_POINT('Ctrl Pts',(-3.71851369000006,5.2,1.88658955999998));
#308922=CARTESIAN_POINT('Ctrl Pts',(-3.71851369000006,2.2,1.88658955999998));
#308923=CARTESIAN_POINT('Ctrl Pts',(-3.71749108900006,12.2,1.88561661199998));
#308924=CARTESIAN_POINT('Ctrl Pts',(-3.71749108900006,5.2,1.88561661199998));
#308925=CARTESIAN_POINT('Ctrl Pts',(-3.71749108900006,2.2,1.88561661199998));
#308926=CARTESIAN_POINT('Ctrl Pts',(-3.71647085600006,12.2,1.88464820699998));
#308927=CARTESIAN_POINT('Ctrl Pts',(-3.71647085600006,5.2,1.88464820699998));
#308928=CARTESIAN_POINT('Ctrl Pts',(-3.71647085600006,2.2,1.88464820699998));
#308929=CARTESIAN_POINT('Ctrl Pts',(-3.71545300400006,12.2,1.88368434499999));
#308930=CARTESIAN_POINT('Ctrl Pts',(-3.71545300400006,5.2,1.88368434499999));
#308931=CARTESIAN_POINT('Ctrl Pts',(-3.71545300400006,2.2,1.88368434499999));
#308932=CARTESIAN_POINT('Ctrl Pts',(-3.71443754800006,12.2,1.88272502299998));
#308933=CARTESIAN_POINT('Ctrl Pts',(-3.71443754800006,5.2,1.88272502299998));
#308934=CARTESIAN_POINT('Ctrl Pts',(-3.71443754800006,2.2,1.88272502299998));
#308935=CARTESIAN_POINT('Ctrl Pts',(-3.71342450000006,12.2,1.88177023999998));
#308936=CARTESIAN_POINT('Ctrl Pts',(-3.71342450000006,5.2,1.88177023999998));
#308937=CARTESIAN_POINT('Ctrl Pts',(-3.71342450000006,2.2,1.88177023999998));
#308938=CARTESIAN_POINT('Ctrl Pts',(-3.71241387600006,12.2,1.88081999599999));
#308939=CARTESIAN_POINT('Ctrl Pts',(-3.71241387600006,5.2,1.88081999599999));
#308940=CARTESIAN_POINT('Ctrl Pts',(-3.71241387600006,2.2,1.88081999599999));
#308941=CARTESIAN_POINT('Ctrl Pts',(-3.71140568900006,12.2,1.87987428799998));
#308942=CARTESIAN_POINT('Ctrl Pts',(-3.71140568900006,5.2,1.87987428799998));
#308943=CARTESIAN_POINT('Ctrl Pts',(-3.71140568900006,2.2,1.87987428799998));
#308944=CARTESIAN_POINT('Ctrl Pts',(-3.71039995200006,12.2,1.87893311499999));
#308945=CARTESIAN_POINT('Ctrl Pts',(-3.71039995200006,5.2,1.87893311499999));
#308946=CARTESIAN_POINT('Ctrl Pts',(-3.71039995200006,2.2,1.87893311499999));
#308947=CARTESIAN_POINT('Ctrl Pts',(-3.70939668200006,12.2,1.87799647399999));
#308948=CARTESIAN_POINT('Ctrl Pts',(-3.70939668200006,5.2,1.87799647399999));
#308949=CARTESIAN_POINT('Ctrl Pts',(-3.70939668200006,2.2,1.87799647399999));
#308950=CARTESIAN_POINT('Ctrl Pts',(-3.70839588900005,12.2,1.87706436599999));
#308951=CARTESIAN_POINT('Ctrl Pts',(-3.70839588900005,5.2,1.87706436599999));
#308952=CARTESIAN_POINT('Ctrl Pts',(-3.70839588900005,2.2,1.87706436599999));
#308953=CARTESIAN_POINT('Ctrl Pts',(-3.70739759000006,12.2,1.87613678599998));
#308954=CARTESIAN_POINT('Ctrl Pts',(-3.70739759000006,5.2,1.87613678599998));
#308955=CARTESIAN_POINT('Ctrl Pts',(-3.70739759000006,2.2,1.87613678599998));
#308956=CARTESIAN_POINT('Ctrl Pts',(-3.70640179700006,12.2,1.87521373399999));
#308957=CARTESIAN_POINT('Ctrl Pts',(-3.70640179700006,5.2,1.87521373399999));
#308958=CARTESIAN_POINT('Ctrl Pts',(-3.70640179700006,2.2,1.87521373399999));
#308959=CARTESIAN_POINT('Ctrl Pts',(-3.70540852600006,12.2,1.87429520899999));
#308960=CARTESIAN_POINT('Ctrl Pts',(-3.70540852600006,5.2,1.87429520899999));
#308961=CARTESIAN_POINT('Ctrl Pts',(-3.70540852600006,2.2,1.87429520899999));
#308962=CARTESIAN_POINT('Ctrl Pts',(-3.70441779000005,12.2,1.87338120899998));
#308963=CARTESIAN_POINT('Ctrl Pts',(-3.70441779000005,5.2,1.87338120899998));
#308964=CARTESIAN_POINT('Ctrl Pts',(-3.70441779000005,2.2,1.87338120899998));
#308965=CARTESIAN_POINT('Ctrl Pts',(-3.70342960400006,12.2,1.87247173099998));
#308966=CARTESIAN_POINT('Ctrl Pts',(-3.70342960400006,5.2,1.87247173099998));
#308967=CARTESIAN_POINT('Ctrl Pts',(-3.70342960400006,2.2,1.87247173099998));
#308968=CARTESIAN_POINT('Ctrl Pts',(-3.70244398200006,12.2,1.87156677399999));
#308969=CARTESIAN_POINT('Ctrl Pts',(-3.70244398200006,5.2,1.87156677399999));
#308970=CARTESIAN_POINT('Ctrl Pts',(-3.70244398200006,2.2,1.87156677399999));
#308971=CARTESIAN_POINT('Ctrl Pts',(-3.70146093700006,12.2,1.87066633599999));
#308972=CARTESIAN_POINT('Ctrl Pts',(-3.70146093700006,5.2,1.87066633599999));
#308973=CARTESIAN_POINT('Ctrl Pts',(-3.70146093700006,2.2,1.87066633599999));
#308974=CARTESIAN_POINT('Ctrl Pts',(-3.70048048300006,12.2,1.86977041599999));
#308975=CARTESIAN_POINT('Ctrl Pts',(-3.70048048300006,5.2,1.86977041599999));
#308976=CARTESIAN_POINT('Ctrl Pts',(-3.70048048300006,2.2,1.86977041599999));
#308977=CARTESIAN_POINT('Ctrl Pts',(-3.69950263700006,12.2,1.86887901099999));
#308978=CARTESIAN_POINT('Ctrl Pts',(-3.69950263700006,5.2,1.86887901099999));
#308979=CARTESIAN_POINT('Ctrl Pts',(-3.69950263700006,2.2,1.86887901099999));
#308980=CARTESIAN_POINT('Ctrl Pts',(-3.69852741200006,12.2,1.86799211899999));
#308981=CARTESIAN_POINT('Ctrl Pts',(-3.69852741200006,5.2,1.86799211899999));
#308982=CARTESIAN_POINT('Ctrl Pts',(-3.69852741200006,2.2,1.86799211899999));
#308983=CARTESIAN_POINT('Ctrl Pts',(-3.69755482000006,12.2,1.86710973899999));
#308984=CARTESIAN_POINT('Ctrl Pts',(-3.69755482000006,5.2,1.86710973899999));
#308985=CARTESIAN_POINT('Ctrl Pts',(-3.69755482000006,2.2,1.86710973899999));
#308986=CARTESIAN_POINT('Ctrl Pts',(-3.69658487900006,12.2,1.86623186999999));
#308987=CARTESIAN_POINT('Ctrl Pts',(-3.69658487900006,5.2,1.86623186999999));
#308988=CARTESIAN_POINT('Ctrl Pts',(-3.69658487900006,2.2,1.86623186999999));
#308989=CARTESIAN_POINT('Ctrl Pts',(-3.69561760100006,12.2,1.86535850699999));
#308990=CARTESIAN_POINT('Ctrl Pts',(-3.69561760100006,5.2,1.86535850699999));
#308991=CARTESIAN_POINT('Ctrl Pts',(-3.69561760100006,2.2,1.86535850699999));
#308992=CARTESIAN_POINT('Ctrl Pts',(-3.69465300100006,12.2,1.86448964999999));
#308993=CARTESIAN_POINT('Ctrl Pts',(-3.69465300100006,5.2,1.86448964999999));
#308994=CARTESIAN_POINT('Ctrl Pts',(-3.69465300100006,2.2,1.86448964999999));
#308995=CARTESIAN_POINT('Ctrl Pts',(-3.69369109400006,12.2,1.86362529699998));
#308996=CARTESIAN_POINT('Ctrl Pts',(-3.69369109400006,5.2,1.86362529699998));
#308997=CARTESIAN_POINT('Ctrl Pts',(-3.69369109400006,2.2,1.86362529699998));
#308998=CARTESIAN_POINT('Ctrl Pts',(-3.69273189400006,12.2,1.86276544599998));
#308999=CARTESIAN_POINT('Ctrl Pts',(-3.69273189400006,5.2,1.86276544599998));
#309000=CARTESIAN_POINT('Ctrl Pts',(-3.69273189400006,2.2,1.86276544599998));
#309001=CARTESIAN_POINT('Ctrl Pts',(-3.69177541500005,12.2,1.86191009499999));
#309002=CARTESIAN_POINT('Ctrl Pts',(-3.69177541500005,5.2,1.86191009499999));
#309003=CARTESIAN_POINT('Ctrl Pts',(-3.69177541500005,2.2,1.86191009499999));
#309004=CARTESIAN_POINT('Ctrl Pts',(-3.69082167100006,12.2,1.86105924099999));
#309005=CARTESIAN_POINT('Ctrl Pts',(-3.69082167100006,5.2,1.86105924099999));
#309006=CARTESIAN_POINT('Ctrl Pts',(-3.69082167100006,2.2,1.86105924099999));
#309007=CARTESIAN_POINT('Ctrl Pts',(-3.68987068000005,12.2,1.86021288299999));
#309008=CARTESIAN_POINT('Ctrl Pts',(-3.68987068000005,5.2,1.86021288299999));
#309009=CARTESIAN_POINT('Ctrl Pts',(-3.68987068000005,2.2,1.86021288299999));
#309010=CARTESIAN_POINT('Ctrl Pts',(-3.68892245300006,12.2,1.85937101899999));
#309011=CARTESIAN_POINT('Ctrl Pts',(-3.68892245300006,5.2,1.85937101899999));
#309012=CARTESIAN_POINT('Ctrl Pts',(-3.68892245300006,2.2,1.85937101899999));
#309013=CARTESIAN_POINT('Ctrl Pts',(-3.68797700500005,12.2,1.85853364499998));
#309014=CARTESIAN_POINT('Ctrl Pts',(-3.68797700500005,5.2,1.85853364499998));
#309015=CARTESIAN_POINT('Ctrl Pts',(-3.68797700500005,2.2,1.85853364499998));
#309016=CARTESIAN_POINT('Ctrl Pts',(-3.68703435300006,12.2,1.85770076099999));
#309017=CARTESIAN_POINT('Ctrl Pts',(-3.68703435300006,5.2,1.85770076099999));
#309018=CARTESIAN_POINT('Ctrl Pts',(-3.68703435300006,2.2,1.85770076099999));
#309019=CARTESIAN_POINT('Ctrl Pts',(-3.68609450900006,12.2,1.85687236399998));
#309020=CARTESIAN_POINT('Ctrl Pts',(-3.68609450900006,5.2,1.85687236399998));
#309021=CARTESIAN_POINT('Ctrl Pts',(-3.68609450900006,2.2,1.85687236399998));
#309022=CARTESIAN_POINT('Ctrl Pts',(-3.68515749000006,12.2,1.85604845099999));
#309023=CARTESIAN_POINT('Ctrl Pts',(-3.68515749000006,5.2,1.85604845099999));
#309024=CARTESIAN_POINT('Ctrl Pts',(-3.68515749000006,2.2,1.85604845099999));
#309025=CARTESIAN_POINT('Ctrl Pts',(-3.68422330900006,12.2,1.85522902099999));
#309026=CARTESIAN_POINT('Ctrl Pts',(-3.68422330900006,5.2,1.85522902099999));
#309027=CARTESIAN_POINT('Ctrl Pts',(-3.68422330900006,2.2,1.85522902099999));
#309028=CARTESIAN_POINT('Ctrl Pts',(-3.68329198100006,12.2,1.85441407199999));
#309029=CARTESIAN_POINT('Ctrl Pts',(-3.68329198100006,5.2,1.85441407199999));
#309030=CARTESIAN_POINT('Ctrl Pts',(-3.68329198100006,2.2,1.85441407199999));
#309031=CARTESIAN_POINT('Ctrl Pts',(-3.68236352100006,12.2,1.85360359999999));
#309032=CARTESIAN_POINT('Ctrl Pts',(-3.68236352100006,5.2,1.85360359999999));
#309033=CARTESIAN_POINT('Ctrl Pts',(-3.68236352100006,2.2,1.85360359999999));
#309034=CARTESIAN_POINT('Ctrl Pts',(-3.68143794400006,12.2,1.85279760399998));
#309035=CARTESIAN_POINT('Ctrl Pts',(-3.68143794400006,5.2,1.85279760399998));
#309036=CARTESIAN_POINT('Ctrl Pts',(-3.68143794400006,2.2,1.85279760399998));
#309037=CARTESIAN_POINT('Ctrl Pts',(-3.68051526600006,12.2,1.85199608199999));
#309038=CARTESIAN_POINT('Ctrl Pts',(-3.68051526600006,5.2,1.85199608199999));
#309039=CARTESIAN_POINT('Ctrl Pts',(-3.68051526600006,2.2,1.85199608199999));
#309040=CARTESIAN_POINT('Ctrl Pts',(-3.67959550000006,12.2,1.85119902999999));
#309041=CARTESIAN_POINT('Ctrl Pts',(-3.67959550000006,5.2,1.85119902999999));
#309042=CARTESIAN_POINT('Ctrl Pts',(-3.67959550000006,2.2,1.85119902999999));
#309043=CARTESIAN_POINT('Ctrl Pts',(-3.67867866100006,12.2,1.85040644699999));
#309044=CARTESIAN_POINT('Ctrl Pts',(-3.67867866100006,5.2,1.85040644699999));
#309045=CARTESIAN_POINT('Ctrl Pts',(-3.67867866100006,2.2,1.85040644699999));
#309046=CARTESIAN_POINT('Ctrl Pts',(-3.67776476600006,12.2,1.84961832999999));
#309047=CARTESIAN_POINT('Ctrl Pts',(-3.67776476600006,5.2,1.84961832999999));
#309048=CARTESIAN_POINT('Ctrl Pts',(-3.67776476600006,2.2,1.84961832999999));
#309049=CARTESIAN_POINT('Ctrl Pts',(-3.67685382700006,12.2,1.84883467599999));
#309050=CARTESIAN_POINT('Ctrl Pts',(-3.67685382700006,5.2,1.84883467599999));
#309051=CARTESIAN_POINT('Ctrl Pts',(-3.67685382700006,2.2,1.84883467599999));
#309052=CARTESIAN_POINT('Ctrl Pts',(-3.67594586200005,12.2,1.84805548499998));
#309053=CARTESIAN_POINT('Ctrl Pts',(-3.67594586200005,5.2,1.84805548499998));
#309054=CARTESIAN_POINT('Ctrl Pts',(-3.67594586200005,2.2,1.84805548499998));
#309055=CARTESIAN_POINT('Ctrl Pts',(-3.67504088400006,12.2,1.84728075099999));
#309056=CARTESIAN_POINT('Ctrl Pts',(-3.67504088400006,5.2,1.84728075099999));
#309057=CARTESIAN_POINT('Ctrl Pts',(-3.67504088400006,2.2,1.84728075099999));
#309058=CARTESIAN_POINT('Ctrl Pts',(-3.67413890800006,12.2,1.84651047499999));
#309059=CARTESIAN_POINT('Ctrl Pts',(-3.67413890800006,5.2,1.84651047499999));
#309060=CARTESIAN_POINT('Ctrl Pts',(-3.67413890800006,2.2,1.84651047499999));
#309061=CARTESIAN_POINT('Ctrl Pts',(-3.67323995100006,12.2,1.84574465199999));
#309062=CARTESIAN_POINT('Ctrl Pts',(-3.67323995100006,5.2,1.84574465199999));
#309063=CARTESIAN_POINT('Ctrl Pts',(-3.67323995100006,2.2,1.84574465199999));
#309064=CARTESIAN_POINT('Ctrl Pts',(-3.67234402700006,12.2,1.84498327999998));
#309065=CARTESIAN_POINT('Ctrl Pts',(-3.67234402700006,5.2,1.84498327999998));
#309066=CARTESIAN_POINT('Ctrl Pts',(-3.67234402700006,2.2,1.84498327999998));
#309067=CARTESIAN_POINT('Ctrl Pts',(-3.67145115000006,12.2,1.84422635699999));
#309068=CARTESIAN_POINT('Ctrl Pts',(-3.67145115000006,5.2,1.84422635699999));
#309069=CARTESIAN_POINT('Ctrl Pts',(-3.67145115000006,2.2,1.84422635699999));
#309070=CARTESIAN_POINT('Ctrl Pts',(-3.67056133700006,12.2,1.84347387999999));
#309071=CARTESIAN_POINT('Ctrl Pts',(-3.67056133700006,5.2,1.84347387999999));
#309072=CARTESIAN_POINT('Ctrl Pts',(-3.67056133700006,2.2,1.84347387999999));
#309073=CARTESIAN_POINT('Ctrl Pts',(-3.66967460300006,12.2,1.84272584599999));
#309074=CARTESIAN_POINT('Ctrl Pts',(-3.66967460300006,5.2,1.84272584599999));
#309075=CARTESIAN_POINT('Ctrl Pts',(-3.66967460300006,2.2,1.84272584599999));
#309076=CARTESIAN_POINT('Ctrl Pts',(-3.66879096200006,12.2,1.84198225299999));
#309077=CARTESIAN_POINT('Ctrl Pts',(-3.66879096200006,5.2,1.84198225299999));
#309078=CARTESIAN_POINT('Ctrl Pts',(-3.66879096200006,2.2,1.84198225299999));
#309079=CARTESIAN_POINT('Ctrl Pts',(-3.66791043200006,12.2,1.84124309799999));
#309080=CARTESIAN_POINT('Ctrl Pts',(-3.66791043200006,5.2,1.84124309799999));
#309081=CARTESIAN_POINT('Ctrl Pts',(-3.66791043200006,2.2,1.84124309799999));
#309082=CARTESIAN_POINT('Ctrl Pts',(-3.66703302500006,12.2,1.84050837899999));
#309083=CARTESIAN_POINT('Ctrl Pts',(-3.66703302500006,5.2,1.84050837899999));
#309084=CARTESIAN_POINT('Ctrl Pts',(-3.66703302500006,2.2,1.84050837899999));
#309085=CARTESIAN_POINT('Ctrl Pts',(-3.66615875800006,12.2,1.83977809099999));
#309086=CARTESIAN_POINT('Ctrl Pts',(-3.66615875800006,5.2,1.83977809099999));
#309087=CARTESIAN_POINT('Ctrl Pts',(-3.66615875800006,2.2,1.83977809099999));
#309088=CARTESIAN_POINT('Ctrl Pts',(-3.66528764600006,12.2,1.83905223399998));
#309089=CARTESIAN_POINT('Ctrl Pts',(-3.66528764600006,5.2,1.83905223399998));
#309090=CARTESIAN_POINT('Ctrl Pts',(-3.66528764600006,2.2,1.83905223399998));
#309091=CARTESIAN_POINT('Ctrl Pts',(-3.66441970600006,12.2,1.83833080299999));
#309092=CARTESIAN_POINT('Ctrl Pts',(-3.66441970600006,5.2,1.83833080299999));
#309093=CARTESIAN_POINT('Ctrl Pts',(-3.66441970600006,2.2,1.83833080299999));
#309094=CARTESIAN_POINT('Ctrl Pts',(-3.66355495100006,12.2,1.83761379699999));
#309095=CARTESIAN_POINT('Ctrl Pts',(-3.66355495100006,5.2,1.83761379699999));
#309096=CARTESIAN_POINT('Ctrl Pts',(-3.66355495100006,2.2,1.83761379699999));
#309097=CARTESIAN_POINT('Ctrl Pts',(-3.66269339700006,12.2,1.83690121199998));
#309098=CARTESIAN_POINT('Ctrl Pts',(-3.66269339700006,5.2,1.83690121199998));
#309099=CARTESIAN_POINT('Ctrl Pts',(-3.66269339700006,2.2,1.83690121199998));
#309100=CARTESIAN_POINT('Ctrl Pts',(-3.66183506100006,12.2,1.83619304499999));
#309101=CARTESIAN_POINT('Ctrl Pts',(-3.66183506100006,5.2,1.83619304499999));
#309102=CARTESIAN_POINT('Ctrl Pts',(-3.66183506100006,2.2,1.83619304499999));
#309103=CARTESIAN_POINT('Ctrl Pts',(-3.66097995800006,12.2,1.83548929399999));
#309104=CARTESIAN_POINT('Ctrl Pts',(-3.66097995800006,5.2,1.83548929399999));
#309105=CARTESIAN_POINT('Ctrl Pts',(-3.66097995800006,2.2,1.83548929399999));
#309106=CARTESIAN_POINT('Ctrl Pts',(-3.66012810400006,12.2,1.83478995599998));
#309107=CARTESIAN_POINT('Ctrl Pts',(-3.66012810400006,5.2,1.83478995599998));
#309108=CARTESIAN_POINT('Ctrl Pts',(-3.66012810400006,2.2,1.83478995599998));
#309109=CARTESIAN_POINT('Ctrl Pts',(-3.65927951400006,12.2,1.83409502799998));
#309110=CARTESIAN_POINT('Ctrl Pts',(-3.65927951400006,5.2,1.83409502799998));
#309111=CARTESIAN_POINT('Ctrl Pts',(-3.65927951400006,2.2,1.83409502799998));
#309112=CARTESIAN_POINT('Ctrl Pts',(-3.65843420300005,12.2,1.83340450599998));
#309113=CARTESIAN_POINT('Ctrl Pts',(-3.65843420300005,5.2,1.83340450599998));
#309114=CARTESIAN_POINT('Ctrl Pts',(-3.65843420300005,2.2,1.83340450599998));
#309115=CARTESIAN_POINT('Ctrl Pts',(-3.65759218800005,12.2,1.83271838799998));
#309116=CARTESIAN_POINT('Ctrl Pts',(-3.65759218800005,5.2,1.83271838799998));
#309117=CARTESIAN_POINT('Ctrl Pts',(-3.65759218800005,2.2,1.83271838799998));
#309118=CARTESIAN_POINT('Ctrl Pts',(-3.65675348400006,12.2,1.83203666999999));
#309119=CARTESIAN_POINT('Ctrl Pts',(-3.65675348400006,5.2,1.83203666999999));
#309120=CARTESIAN_POINT('Ctrl Pts',(-3.65675348400006,2.2,1.83203666999999));
#309121=CARTESIAN_POINT('Ctrl Pts',(-3.65591810600006,12.2,1.83135934999999));
#309122=CARTESIAN_POINT('Ctrl Pts',(-3.65591810600006,5.2,1.83135934999999));
#309123=CARTESIAN_POINT('Ctrl Pts',(-3.65591810600006,2.2,1.83135934999999));
#309124=CARTESIAN_POINT('Ctrl Pts',(-3.65508607100006,12.2,1.83068642499999));
#309125=CARTESIAN_POINT('Ctrl Pts',(-3.65508607100006,5.2,1.83068642499999));
#309126=CARTESIAN_POINT('Ctrl Pts',(-3.65508607100006,2.2,1.83068642499999));
#309127=CARTESIAN_POINT('Ctrl Pts',(-3.65425739600005,12.2,1.83001788999999));
#309128=CARTESIAN_POINT('Ctrl Pts',(-3.65425739600005,5.2,1.83001788999999));
#309129=CARTESIAN_POINT('Ctrl Pts',(-3.65425739600005,2.2,1.83001788999999));
#309130=CARTESIAN_POINT('Ctrl Pts',(-3.65343209400006,12.2,1.82935374399999));
#309131=CARTESIAN_POINT('Ctrl Pts',(-3.65343209400006,5.2,1.82935374399999));
#309132=CARTESIAN_POINT('Ctrl Pts',(-3.65343209400006,2.2,1.82935374399999));
#309133=CARTESIAN_POINT('Ctrl Pts',(-3.65261018300005,12.2,1.82869398399998));
#309134=CARTESIAN_POINT('Ctrl Pts',(-3.65261018300005,5.2,1.82869398399998));
#309135=CARTESIAN_POINT('Ctrl Pts',(-3.65261018300005,2.2,1.82869398399998));
#309136=CARTESIAN_POINT('Ctrl Pts',(-3.65179167700005,12.2,1.82803860399999));
#309137=CARTESIAN_POINT('Ctrl Pts',(-3.65179167700005,5.2,1.82803860399999));
#309138=CARTESIAN_POINT('Ctrl Pts',(-3.65179167700005,2.2,1.82803860399999));
#309139=CARTESIAN_POINT('Ctrl Pts',(-3.65097659500006,12.2,1.82738760299999));
#309140=CARTESIAN_POINT('Ctrl Pts',(-3.65097659500006,5.2,1.82738760299999));
#309141=CARTESIAN_POINT('Ctrl Pts',(-3.65097659500006,2.2,1.82738760299999));
#309142=CARTESIAN_POINT('Ctrl Pts',(-3.65016495000006,12.2,1.82674097899998));
#309143=CARTESIAN_POINT('Ctrl Pts',(-3.65016495000006,5.2,1.82674097899998));
#309144=CARTESIAN_POINT('Ctrl Pts',(-3.65016495000006,2.2,1.82674097899998));
#309145=CARTESIAN_POINT('Ctrl Pts',(-3.64935676100006,12.2,1.82609872499999));
#309146=CARTESIAN_POINT('Ctrl Pts',(-3.64935676100006,5.2,1.82609872499999));
#309147=CARTESIAN_POINT('Ctrl Pts',(-3.64935676100006,2.2,1.82609872499999));
#309148=CARTESIAN_POINT('Ctrl Pts',(-3.64855204100006,12.2,1.82546084099998));
#309149=CARTESIAN_POINT('Ctrl Pts',(-3.64855204100006,5.2,1.82546084099998));
#309150=CARTESIAN_POINT('Ctrl Pts',(-3.64855204100006,2.2,1.82546084099998));
#309151=CARTESIAN_POINT('Ctrl Pts',(-3.64775080700006,12.2,1.82482732199999));
#309152=CARTESIAN_POINT('Ctrl Pts',(-3.64775080700006,5.2,1.82482732199999));
#309153=CARTESIAN_POINT('Ctrl Pts',(-3.64775080700006,2.2,1.82482732199999));
#309154=CARTESIAN_POINT('Ctrl Pts',(-3.64695307800006,12.2,1.82419816399999));
#309155=CARTESIAN_POINT('Ctrl Pts',(-3.64695307800006,5.2,1.82419816399999));
#309156=CARTESIAN_POINT('Ctrl Pts',(-3.64695307800006,2.2,1.82419816399999));
#309157=CARTESIAN_POINT('Ctrl Pts',(-3.64615886600006,12.2,1.82357336599999));
#309158=CARTESIAN_POINT('Ctrl Pts',(-3.64615886600006,5.2,1.82357336599999));
#309159=CARTESIAN_POINT('Ctrl Pts',(-3.64615886600006,2.2,1.82357336599999));
#309160=CARTESIAN_POINT('Ctrl Pts',(-3.64536819000006,12.2,1.82295292299999));
#309161=CARTESIAN_POINT('Ctrl Pts',(-3.64536819000006,5.2,1.82295292299999));
#309162=CARTESIAN_POINT('Ctrl Pts',(-3.64536819000006,2.2,1.82295292299999));
#309163=CARTESIAN_POINT('Ctrl Pts',(-3.64458106600006,12.2,1.82233683099998));
#309164=CARTESIAN_POINT('Ctrl Pts',(-3.64458106600006,5.2,1.82233683099998));
#309165=CARTESIAN_POINT('Ctrl Pts',(-3.64458106600006,2.2,1.82233683099998));
#309166=CARTESIAN_POINT('Ctrl Pts',(-3.64379750800006,12.2,1.82172508799999));
#309167=CARTESIAN_POINT('Ctrl Pts',(-3.64379750800006,5.2,1.82172508799999));
#309168=CARTESIAN_POINT('Ctrl Pts',(-3.64379750800006,2.2,1.82172508799999));
#309169=CARTESIAN_POINT('Ctrl Pts',(-3.64301753500006,12.2,1.82111768899999));
#309170=CARTESIAN_POINT('Ctrl Pts',(-3.64301753500006,5.2,1.82111768899999));
#309171=CARTESIAN_POINT('Ctrl Pts',(-3.64301753500006,2.2,1.82111768899999));
#309172=CARTESIAN_POINT('Ctrl Pts',(-3.64224116200006,12.2,1.82051463099999));
#309173=CARTESIAN_POINT('Ctrl Pts',(-3.64224116200006,5.2,1.82051463099999));
#309174=CARTESIAN_POINT('Ctrl Pts',(-3.64224116200006,2.2,1.82051463099999));
#309175=CARTESIAN_POINT('Ctrl Pts',(-3.64146840700006,12.2,1.81991591099999));
#309176=CARTESIAN_POINT('Ctrl Pts',(-3.64146840700006,5.2,1.81991591099999));
#309177=CARTESIAN_POINT('Ctrl Pts',(-3.64146840700006,2.2,1.81991591099999));
#309178=CARTESIAN_POINT('Ctrl Pts',(-3.64069928400006,12.2,1.81932152599999));
#309179=CARTESIAN_POINT('Ctrl Pts',(-3.64069928400006,5.2,1.81932152599999));
#309180=CARTESIAN_POINT('Ctrl Pts',(-3.64069928400006,2.2,1.81932152599999));
#309181=CARTESIAN_POINT('Ctrl Pts',(-3.63993381200006,12.2,1.81873146999999));
#309182=CARTESIAN_POINT('Ctrl Pts',(-3.63993381200006,5.2,1.81873146999999));
#309183=CARTESIAN_POINT('Ctrl Pts',(-3.63993381200006,2.2,1.81873146999999));
#309184=CARTESIAN_POINT('Ctrl Pts',(-3.63917200600006,12.2,1.81814573999999));
#309185=CARTESIAN_POINT('Ctrl Pts',(-3.63917200600006,5.2,1.81814573999999));
#309186=CARTESIAN_POINT('Ctrl Pts',(-3.63917200600006,2.2,1.81814573999999));
#309187=CARTESIAN_POINT('Ctrl Pts',(-3.63841388300005,12.2,1.81756433299999));
#309188=CARTESIAN_POINT('Ctrl Pts',(-3.63841388300005,5.2,1.81756433299999));
#309189=CARTESIAN_POINT('Ctrl Pts',(-3.63841388300005,2.2,1.81756433299999));
#309190=CARTESIAN_POINT('Ctrl Pts',(-3.63765945900006,12.2,1.81698724599999));
#309191=CARTESIAN_POINT('Ctrl Pts',(-3.63765945900006,5.2,1.81698724599999));
#309192=CARTESIAN_POINT('Ctrl Pts',(-3.63765945900006,2.2,1.81698724599999));
#309193=CARTESIAN_POINT('Ctrl Pts',(-3.63690875100006,12.2,1.81641447499999));
#309194=CARTESIAN_POINT('Ctrl Pts',(-3.63690875100006,5.2,1.81641447499999));
#309195=CARTESIAN_POINT('Ctrl Pts',(-3.63690875100006,2.2,1.81641447499999));
#309196=CARTESIAN_POINT('Ctrl Pts',(-3.63616177600006,12.2,1.81584601399999));
#309197=CARTESIAN_POINT('Ctrl Pts',(-3.63616177600006,5.2,1.81584601399999));
#309198=CARTESIAN_POINT('Ctrl Pts',(-3.63616177600006,2.2,1.81584601399999));
#309199=CARTESIAN_POINT('Ctrl Pts',(-3.63541855100006,12.2,1.81528186099999));
#309200=CARTESIAN_POINT('Ctrl Pts',(-3.63541855100006,5.2,1.81528186099999));
#309201=CARTESIAN_POINT('Ctrl Pts',(-3.63541855100006,2.2,1.81528186099999));
#309202=CARTESIAN_POINT('Ctrl Pts',(-3.63467909100006,12.2,1.81472201299998));
#309203=CARTESIAN_POINT('Ctrl Pts',(-3.63467909100006,5.2,1.81472201299998));
#309204=CARTESIAN_POINT('Ctrl Pts',(-3.63467909100006,2.2,1.81472201299998));
#309205=CARTESIAN_POINT('Ctrl Pts',(-3.63394341600006,12.2,1.81416646399999));
#309206=CARTESIAN_POINT('Ctrl Pts',(-3.63394341600006,5.2,1.81416646399999));
#309207=CARTESIAN_POINT('Ctrl Pts',(-3.63394341600006,2.2,1.81416646399999));
#309208=CARTESIAN_POINT('Ctrl Pts',(-3.63321154000006,12.2,1.81361521199999));
#309209=CARTESIAN_POINT('Ctrl Pts',(-3.63321154000006,5.2,1.81361521199999));
#309210=CARTESIAN_POINT('Ctrl Pts',(-3.63321154000006,2.2,1.81361521199999));
#309211=CARTESIAN_POINT('Ctrl Pts',(-3.63248348000006,12.2,1.81306825299998));
#309212=CARTESIAN_POINT('Ctrl Pts',(-3.63248348000006,5.2,1.81306825299998));
#309213=CARTESIAN_POINT('Ctrl Pts',(-3.63248348000006,2.2,1.81306825299998));
#309214=CARTESIAN_POINT('Ctrl Pts',(-3.63175925500006,12.2,1.81252557999999));
#309215=CARTESIAN_POINT('Ctrl Pts',(-3.63175925500006,5.2,1.81252557999999));
#309216=CARTESIAN_POINT('Ctrl Pts',(-3.63175925500006,2.2,1.81252557999999));
#309217=CARTESIAN_POINT('Ctrl Pts',(-3.63103888100006,12.2,1.81198719199998));
#309218=CARTESIAN_POINT('Ctrl Pts',(-3.63103888100006,5.2,1.81198719199998));
#309219=CARTESIAN_POINT('Ctrl Pts',(-3.63103888100006,2.2,1.81198719199998));
#309220=CARTESIAN_POINT('Ctrl Pts',(-3.63032237400006,12.2,1.81145308399998));
#309221=CARTESIAN_POINT('Ctrl Pts',(-3.63032237400006,5.2,1.81145308399998));
#309222=CARTESIAN_POINT('Ctrl Pts',(-3.63032237400006,2.2,1.81145308399998));
#309223=CARTESIAN_POINT('Ctrl Pts',(-3.62960975100005,12.2,1.81092325199999));
#309224=CARTESIAN_POINT('Ctrl Pts',(-3.62960975100005,5.2,1.81092325199999));
#309225=CARTESIAN_POINT('Ctrl Pts',(-3.62960975100005,2.2,1.81092325199999));
#309226=CARTESIAN_POINT('Ctrl Pts',(-3.62890103000006,12.2,1.81039769199999));
#309227=CARTESIAN_POINT('Ctrl Pts',(-3.62890103000006,5.2,1.81039769199999));
#309228=CARTESIAN_POINT('Ctrl Pts',(-3.62890103000006,2.2,1.81039769199999));
#309229=CARTESIAN_POINT('Ctrl Pts',(-3.62819622900005,12.2,1.80987640099998));
#309230=CARTESIAN_POINT('Ctrl Pts',(-3.62819622900005,5.2,1.80987640099998));
#309231=CARTESIAN_POINT('Ctrl Pts',(-3.62819622900005,2.2,1.80987640099998));
#309232=CARTESIAN_POINT('Ctrl Pts',(-3.62749536200006,12.2,1.80935937299999));
#309233=CARTESIAN_POINT('Ctrl Pts',(-3.62749536200006,5.2,1.80935937299999));
#309234=CARTESIAN_POINT('Ctrl Pts',(-3.62749536200006,2.2,1.80935937299999));
#309235=CARTESIAN_POINT('Ctrl Pts',(-3.62679845000006,12.2,1.80884660299999));
#309236=CARTESIAN_POINT('Ctrl Pts',(-3.62679845000006,5.2,1.80884660299999));
#309237=CARTESIAN_POINT('Ctrl Pts',(-3.62679845000006,2.2,1.80884660299999));
#309238=CARTESIAN_POINT('Ctrl Pts',(-3.62610550700006,12.2,1.80833808899999));
#309239=CARTESIAN_POINT('Ctrl Pts',(-3.62610550700006,5.2,1.80833808899999));
#309240=CARTESIAN_POINT('Ctrl Pts',(-3.62610550700006,2.2,1.80833808899999));
#309241=CARTESIAN_POINT('Ctrl Pts',(-3.62541655300006,12.2,1.80783382599999));
#309242=CARTESIAN_POINT('Ctrl Pts',(-3.62541655300006,5.2,1.80783382599999));
#309243=CARTESIAN_POINT('Ctrl Pts',(-3.62541655300006,2.2,1.80783382599999));
#309244=CARTESIAN_POINT('Ctrl Pts',(-3.62473160400006,12.2,1.80733380999999));
#309245=CARTESIAN_POINT('Ctrl Pts',(-3.62473160400006,5.2,1.80733380999999));
#309246=CARTESIAN_POINT('Ctrl Pts',(-3.62473160400006,2.2,1.80733380999999));
#309247=CARTESIAN_POINT('Ctrl Pts',(-3.62405067700006,12.2,1.80683803499999));
#309248=CARTESIAN_POINT('Ctrl Pts',(-3.62405067700006,5.2,1.80683803499999));
#309249=CARTESIAN_POINT('Ctrl Pts',(-3.62405067700006,2.2,1.80683803499999));
#309250=CARTESIAN_POINT('Ctrl Pts',(-3.62337379000006,12.2,1.80634649899998));
#309251=CARTESIAN_POINT('Ctrl Pts',(-3.62337379000006,5.2,1.80634649899998));
#309252=CARTESIAN_POINT('Ctrl Pts',(-3.62337379000006,2.2,1.80634649899998));
#309253=CARTESIAN_POINT('Ctrl Pts',(-3.62270096000006,12.2,1.80585919599999));
#309254=CARTESIAN_POINT('Ctrl Pts',(-3.62270096000006,5.2,1.80585919599999));
#309255=CARTESIAN_POINT('Ctrl Pts',(-3.62270096000006,2.2,1.80585919599999));
#309256=CARTESIAN_POINT('Ctrl Pts',(-3.62203220500006,12.2,1.80537612199998));
#309257=CARTESIAN_POINT('Ctrl Pts',(-3.62203220500006,5.2,1.80537612199998));
#309258=CARTESIAN_POINT('Ctrl Pts',(-3.62203220500006,2.2,1.80537612199998));
#309259=CARTESIAN_POINT('Ctrl Pts',(-3.62136754200006,12.2,1.80489727299999));
#309260=CARTESIAN_POINT('Ctrl Pts',(-3.62136754200006,5.2,1.80489727299999));
#309261=CARTESIAN_POINT('Ctrl Pts',(-3.62136754200006,2.2,1.80489727299999));
#309262=CARTESIAN_POINT('Ctrl Pts',(-3.62070698900006,12.2,1.80442264399999));
#309263=CARTESIAN_POINT('Ctrl Pts',(-3.62070698900006,5.2,1.80442264399999));
#309264=CARTESIAN_POINT('Ctrl Pts',(-3.62070698900006,2.2,1.80442264399999));
#309265=CARTESIAN_POINT('Ctrl Pts',(-3.62005056300006,12.2,1.80395222999998));
#309266=CARTESIAN_POINT('Ctrl Pts',(-3.62005056300006,5.2,1.80395222999998));
#309267=CARTESIAN_POINT('Ctrl Pts',(-3.62005056300006,2.2,1.80395222999998));
#309268=CARTESIAN_POINT('Ctrl Pts',(-3.61939828100006,12.2,1.80348602699999));
#309269=CARTESIAN_POINT('Ctrl Pts',(-3.61939828100006,5.2,1.80348602699999));
#309270=CARTESIAN_POINT('Ctrl Pts',(-3.61939828100006,2.2,1.80348602699999));
#309271=CARTESIAN_POINT('Ctrl Pts',(-3.61875016400006,12.2,1.80302403099999));
#309272=CARTESIAN_POINT('Ctrl Pts',(-3.61875016400006,5.2,1.80302403099999));
#309273=CARTESIAN_POINT('Ctrl Pts',(-3.61875016400006,2.2,1.80302403099999));
#309274=CARTESIAN_POINT('Ctrl Pts',(-3.61810622700006,12.2,1.80256623599998));
#309275=CARTESIAN_POINT('Ctrl Pts',(-3.61810622700006,5.2,1.80256623599998));
#309276=CARTESIAN_POINT('Ctrl Pts',(-3.61810622700006,2.2,1.80256623599998));
#309277=CARTESIAN_POINT('Ctrl Pts',(-3.61746648700006,12.2,1.80211263799999));
#309278=CARTESIAN_POINT('Ctrl Pts',(-3.61746648700006,5.2,1.80211263799999));
#309279=CARTESIAN_POINT('Ctrl Pts',(-3.61746648700006,2.2,1.80211263799999));
#309280=CARTESIAN_POINT('Ctrl Pts',(-3.61683096400006,12.2,1.80166323299999));
#309281=CARTESIAN_POINT('Ctrl Pts',(-3.61683096400006,5.2,1.80166323299999));
#309282=CARTESIAN_POINT('Ctrl Pts',(-3.61683096400006,2.2,1.80166323299999));
#309283=CARTESIAN_POINT('Ctrl Pts',(-3.61619967500006,12.2,1.80121801399999));
#309284=CARTESIAN_POINT('Ctrl Pts',(-3.61619967500006,5.2,1.80121801399999));
#309285=CARTESIAN_POINT('Ctrl Pts',(-3.61619967500006,2.2,1.80121801399999));
#309286=CARTESIAN_POINT('Ctrl Pts',(-3.61557263800006,12.2,1.80077697899999));
#309287=CARTESIAN_POINT('Ctrl Pts',(-3.61557263800006,5.2,1.80077697899999));
#309288=CARTESIAN_POINT('Ctrl Pts',(-3.61557263800006,2.2,1.80077697899999));
#309289=CARTESIAN_POINT('Ctrl Pts',(-3.61494987000006,12.2,1.80034012099998));
#309290=CARTESIAN_POINT('Ctrl Pts',(-3.61494987000006,5.2,1.80034012099998));
#309291=CARTESIAN_POINT('Ctrl Pts',(-3.61494987000006,2.2,1.80034012099998));
#309292=CARTESIAN_POINT('Ctrl Pts',(-3.61433139100006,12.2,1.79990743799999));
#309293=CARTESIAN_POINT('Ctrl Pts',(-3.61433139100006,5.2,1.79990743799999));
#309294=CARTESIAN_POINT('Ctrl Pts',(-3.61433139100006,2.2,1.79990743799999));
#309295=CARTESIAN_POINT('Ctrl Pts',(-3.61371721600006,12.2,1.79947892099999));
#309296=CARTESIAN_POINT('Ctrl Pts',(-3.61371721600006,5.2,1.79947892099999));
#309297=CARTESIAN_POINT('Ctrl Pts',(-3.61371721600006,2.2,1.79947892099999));
#309298=CARTESIAN_POINT('Ctrl Pts',(-3.61310736600006,12.2,1.79905456799998));
#309299=CARTESIAN_POINT('Ctrl Pts',(-3.61310736600006,5.2,1.79905456799998));
#309300=CARTESIAN_POINT('Ctrl Pts',(-3.61310736600006,2.2,1.79905456799998));
#309301=CARTESIAN_POINT('Ctrl Pts',(-3.61250185900006,12.2,1.79863437299999));
#309302=CARTESIAN_POINT('Ctrl Pts',(-3.61250185900006,5.2,1.79863437299999));
#309303=CARTESIAN_POINT('Ctrl Pts',(-3.61250185900006,2.2,1.79863437299999));
#309304=CARTESIAN_POINT('Ctrl Pts',(-3.61190071000006,12.2,1.79821833199998));
#309305=CARTESIAN_POINT('Ctrl Pts',(-3.61190071000006,5.2,1.79821833199998));
#309306=CARTESIAN_POINT('Ctrl Pts',(-3.61190071000006,2.2,1.79821833199998));
#309307=CARTESIAN_POINT('Ctrl Pts',(-3.61130394200006,12.2,1.79780643799999));
#309308=CARTESIAN_POINT('Ctrl Pts',(-3.61130394200006,5.2,1.79780643799999));
#309309=CARTESIAN_POINT('Ctrl Pts',(-3.61130394200006,2.2,1.79780643799999));
#309310=CARTESIAN_POINT('Ctrl Pts',(-3.61071156900006,12.2,1.79739868899999));
#309311=CARTESIAN_POINT('Ctrl Pts',(-3.61071156900006,5.2,1.79739868899999));
#309312=CARTESIAN_POINT('Ctrl Pts',(-3.61071156900006,2.2,1.79739868899999));
#309313=CARTESIAN_POINT('Ctrl Pts',(-3.61012361200006,12.2,1.79699507699999));
#309314=CARTESIAN_POINT('Ctrl Pts',(-3.61012361200006,5.2,1.79699507699999));
#309315=CARTESIAN_POINT('Ctrl Pts',(-3.61012361200006,2.2,1.79699507699999));
#309316=CARTESIAN_POINT('Ctrl Pts',(-3.60954008800006,12.2,1.79659559799999));
#309317=CARTESIAN_POINT('Ctrl Pts',(-3.60954008800006,5.2,1.79659559799999));
#309318=CARTESIAN_POINT('Ctrl Pts',(-3.60954008800006,2.2,1.79659559799999));
#309319=CARTESIAN_POINT('Ctrl Pts',(-3.60896101600006,12.2,1.79620024699998));
#309320=CARTESIAN_POINT('Ctrl Pts',(-3.60896101600006,5.2,1.79620024699998));
#309321=CARTESIAN_POINT('Ctrl Pts',(-3.60896101600006,2.2,1.79620024699998));
#309322=CARTESIAN_POINT('Ctrl Pts',(-3.60838641400006,12.2,1.79580901699998));
#309323=CARTESIAN_POINT('Ctrl Pts',(-3.60838641400006,5.2,1.79580901699998));
#309324=CARTESIAN_POINT('Ctrl Pts',(-3.60838641400006,2.2,1.79580901699998));
#309325=CARTESIAN_POINT('Ctrl Pts',(-3.60781630100006,12.2,1.79542190599999));
#309326=CARTESIAN_POINT('Ctrl Pts',(-3.60781630100006,5.2,1.79542190599999));
#309327=CARTESIAN_POINT('Ctrl Pts',(-3.60781630100006,2.2,1.79542190599999));
#309328=CARTESIAN_POINT('Ctrl Pts',(-3.60725069600006,12.2,1.79503890699999));
#309329=CARTESIAN_POINT('Ctrl Pts',(-3.60725069600006,5.2,1.79503890699999));
#309330=CARTESIAN_POINT('Ctrl Pts',(-3.60725069600006,2.2,1.79503890699999));
#309331=CARTESIAN_POINT('Ctrl Pts',(-3.60668961600005,12.2,1.79466001299998));
#309332=CARTESIAN_POINT('Ctrl Pts',(-3.60668961600005,5.2,1.79466001299998));
#309333=CARTESIAN_POINT('Ctrl Pts',(-3.60668961600005,2.2,1.79466001299998));
#309334=CARTESIAN_POINT('Ctrl Pts',(-3.60613308100006,12.2,1.79428522199998));
#309335=CARTESIAN_POINT('Ctrl Pts',(-3.60613308100006,5.2,1.79428522199998));
#309336=CARTESIAN_POINT('Ctrl Pts',(-3.60613308100006,2.2,1.79428522199998));
#309337=CARTESIAN_POINT('Ctrl Pts',(-3.60558110800006,12.2,1.79391452599999));
#309338=CARTESIAN_POINT('Ctrl Pts',(-3.60558110800006,5.2,1.79391452599999));
#309339=CARTESIAN_POINT('Ctrl Pts',(-3.60558110800006,2.2,1.79391452599999));
#309340=CARTESIAN_POINT('Ctrl Pts',(-3.60503372000006,12.2,1.79354792099998));
#309341=CARTESIAN_POINT('Ctrl Pts',(-3.60503372000006,5.2,1.79354792099998));
#309342=CARTESIAN_POINT('Ctrl Pts',(-3.60503372000006,2.2,1.79354792099998));
#309343=CARTESIAN_POINT('Ctrl Pts',(-3.60449093000006,12.2,1.79318539999999));
#309344=CARTESIAN_POINT('Ctrl Pts',(-3.60449093000006,5.2,1.79318539999999));
#309345=CARTESIAN_POINT('Ctrl Pts',(-3.60449093000006,2.2,1.79318539999999));
#309346=CARTESIAN_POINT('Ctrl Pts',(-3.60395276000006,12.2,1.79282695799999));
#309347=CARTESIAN_POINT('Ctrl Pts',(-3.60395276000006,5.2,1.79282695799999));
#309348=CARTESIAN_POINT('Ctrl Pts',(-3.60395276000006,2.2,1.79282695799999));
#309349=CARTESIAN_POINT('Ctrl Pts',(-3.60341923000006,12.2,1.79247259099999));
#309350=CARTESIAN_POINT('Ctrl Pts',(-3.60341923000006,5.2,1.79247259099999));
#309351=CARTESIAN_POINT('Ctrl Pts',(-3.60341923000006,2.2,1.79247259099999));
#309352=CARTESIAN_POINT('Ctrl Pts',(-3.60289035500006,12.2,1.79212229099999));
#309353=CARTESIAN_POINT('Ctrl Pts',(-3.60289035500006,5.2,1.79212229099999));
#309354=CARTESIAN_POINT('Ctrl Pts',(-3.60289035500006,2.2,1.79212229099999));
#309355=CARTESIAN_POINT('Ctrl Pts',(-3.60236615800006,12.2,1.79177605499998));
#309356=CARTESIAN_POINT('Ctrl Pts',(-3.60236615800006,5.2,1.79177605499998));
#309357=CARTESIAN_POINT('Ctrl Pts',(-3.60236615800006,2.2,1.79177605499998));
#309358=CARTESIAN_POINT('Ctrl Pts',(-3.60184665600006,12.2,1.79143387499999));
#309359=CARTESIAN_POINT('Ctrl Pts',(-3.60184665600006,5.2,1.79143387499999));
#309360=CARTESIAN_POINT('Ctrl Pts',(-3.60184665600006,2.2,1.79143387499999));
#309361=CARTESIAN_POINT('Ctrl Pts',(-3.60133186900006,12.2,1.79109574699998));
#309362=CARTESIAN_POINT('Ctrl Pts',(-3.60133186900006,5.2,1.79109574699998));
#309363=CARTESIAN_POINT('Ctrl Pts',(-3.60133186900006,2.2,1.79109574699998));
#309364=CARTESIAN_POINT('Ctrl Pts',(-3.60082181600006,12.2,1.79076166399998));
#309365=CARTESIAN_POINT('Ctrl Pts',(-3.60082181600006,5.2,1.79076166399998));
#309366=CARTESIAN_POINT('Ctrl Pts',(-3.60082181600006,2.2,1.79076166399998));
#309367=CARTESIAN_POINT('Ctrl Pts',(-3.60031651500006,12.2,1.79043161999999));
#309368=CARTESIAN_POINT('Ctrl Pts',(-3.60031651500006,5.2,1.79043161999999));
#309369=CARTESIAN_POINT('Ctrl Pts',(-3.60031651500006,2.2,1.79043161999999));
#309370=CARTESIAN_POINT('Ctrl Pts',(-3.59981598500006,12.2,1.79010560999998));
#309371=CARTESIAN_POINT('Ctrl Pts',(-3.59981598500006,5.2,1.79010560999998));
#309372=CARTESIAN_POINT('Ctrl Pts',(-3.59981598500006,2.2,1.79010560999998));
#309373=CARTESIAN_POINT('Ctrl Pts',(-3.59932024800006,12.2,1.78978362799999));
#309374=CARTESIAN_POINT('Ctrl Pts',(-3.59932024800006,5.2,1.78978362799999));
#309375=CARTESIAN_POINT('Ctrl Pts',(-3.59932024800006,2.2,1.78978362799999));
#309376=CARTESIAN_POINT('Ctrl Pts',(-3.59882932100006,12.2,1.78946566799999));
#309377=CARTESIAN_POINT('Ctrl Pts',(-3.59882932100006,5.2,1.78946566799999));
#309378=CARTESIAN_POINT('Ctrl Pts',(-3.59882932100006,2.2,1.78946566799999));
#309379=CARTESIAN_POINT('Ctrl Pts',(-3.59834322400006,12.2,1.78915172399998));
#309380=CARTESIAN_POINT('Ctrl Pts',(-3.59834322400006,5.2,1.78915172399998));
#309381=CARTESIAN_POINT('Ctrl Pts',(-3.59834322400006,2.2,1.78915172399998));
#309382=CARTESIAN_POINT('Ctrl Pts',(-3.59786197700006,12.2,1.78884178999999));
#309383=CARTESIAN_POINT('Ctrl Pts',(-3.59786197700006,5.2,1.78884178999999));
#309384=CARTESIAN_POINT('Ctrl Pts',(-3.59786197700006,2.2,1.78884178999999));
#309385=CARTESIAN_POINT('Ctrl Pts',(-3.59738559900006,12.2,1.78853585999999));
#309386=CARTESIAN_POINT('Ctrl Pts',(-3.59738559900006,5.2,1.78853585999999));
#309387=CARTESIAN_POINT('Ctrl Pts',(-3.59738559900006,2.2,1.78853585999999));
#309388=CARTESIAN_POINT('Ctrl Pts',(-3.59691410800006,12.2,1.78823392699998));
#309389=CARTESIAN_POINT('Ctrl Pts',(-3.59691410800006,5.2,1.78823392699998));
#309390=CARTESIAN_POINT('Ctrl Pts',(-3.59691410800006,2.2,1.78823392699998));
#309391=CARTESIAN_POINT('Ctrl Pts',(-3.59644752700006,12.2,1.78793598599999));
#309392=CARTESIAN_POINT('Ctrl Pts',(-3.59644752700006,5.2,1.78793598599999));
#309393=CARTESIAN_POINT('Ctrl Pts',(-3.59644752700006,2.2,1.78793598599999));
#309394=CARTESIAN_POINT('Ctrl Pts',(-3.59598587300006,12.2,1.78764203199998));
#309395=CARTESIAN_POINT('Ctrl Pts',(-3.59598587300006,5.2,1.78764203199998));
#309396=CARTESIAN_POINT('Ctrl Pts',(-3.59598587300006,2.2,1.78764203199998));
#309397=CARTESIAN_POINT('Ctrl Pts',(-3.59552916600006,12.2,1.78735205599999));
#309398=CARTESIAN_POINT('Ctrl Pts',(-3.59552916600006,5.2,1.78735205599999));
#309399=CARTESIAN_POINT('Ctrl Pts',(-3.59552916600006,2.2,1.78735205599999));
#309400=CARTESIAN_POINT('Ctrl Pts',(-3.59507742600006,12.2,1.78706605299999));
#309401=CARTESIAN_POINT('Ctrl Pts',(-3.59507742600006,5.2,1.78706605299999));
#309402=CARTESIAN_POINT('Ctrl Pts',(-3.59507742600006,2.2,1.78706605299999));
#309403=CARTESIAN_POINT('Ctrl Pts',(-3.59463067400006,12.2,1.78678401699999));
#309404=CARTESIAN_POINT('Ctrl Pts',(-3.59463067400006,5.2,1.78678401699999));
#309405=CARTESIAN_POINT('Ctrl Pts',(-3.59463067400006,2.2,1.78678401699999));
#309406=CARTESIAN_POINT('Ctrl Pts',(-3.59418892800006,12.2,1.78650594099999));
#309407=CARTESIAN_POINT('Ctrl Pts',(-3.59418892800006,5.2,1.78650594099999));
#309408=CARTESIAN_POINT('Ctrl Pts',(-3.59418892800006,2.2,1.78650594099999));
#309409=CARTESIAN_POINT('Ctrl Pts',(-3.59375221000006,12.2,1.78623181999999));
#309410=CARTESIAN_POINT('Ctrl Pts',(-3.59375221000006,5.2,1.78623181999999));
#309411=CARTESIAN_POINT('Ctrl Pts',(-3.59375221000006,2.2,1.78623181999999));
#309412=CARTESIAN_POINT('Ctrl Pts',(-3.59332053700006,12.2,1.78596164699998));
#309413=CARTESIAN_POINT('Ctrl Pts',(-3.59332053700006,5.2,1.78596164699998));
#309414=CARTESIAN_POINT('Ctrl Pts',(-3.59332053700006,2.2,1.78596164699998));
#309415=CARTESIAN_POINT('Ctrl Pts',(-3.59289393100005,12.2,1.78569541399999));
#309416=CARTESIAN_POINT('Ctrl Pts',(-3.59289393100005,5.2,1.78569541399999));
#309417=CARTESIAN_POINT('Ctrl Pts',(-3.59289393100005,2.2,1.78569541399999));
#309418=CARTESIAN_POINT('Ctrl Pts',(-3.59247241200006,12.2,1.78543311499999));
#309419=CARTESIAN_POINT('Ctrl Pts',(-3.59247241200006,5.2,1.78543311499999));
#309420=CARTESIAN_POINT('Ctrl Pts',(-3.59247241200006,2.2,1.78543311499999));
#309421=CARTESIAN_POINT('Ctrl Pts',(-3.59205600100006,12.2,1.78517474599999));
#309422=CARTESIAN_POINT('Ctrl Pts',(-3.59205600100006,5.2,1.78517474599999));
#309423=CARTESIAN_POINT('Ctrl Pts',(-3.59205600100006,2.2,1.78517474599999));
#309424=CARTESIAN_POINT('Ctrl Pts',(-3.59164471600006,12.2,1.78492029699999));
#309425=CARTESIAN_POINT('Ctrl Pts',(-3.59164471600006,5.2,1.78492029699999));
#309426=CARTESIAN_POINT('Ctrl Pts',(-3.59164471600006,2.2,1.78492029699999));
#309427=CARTESIAN_POINT('Ctrl Pts',(-3.59123857800006,12.2,1.78466976299998));
#309428=CARTESIAN_POINT('Ctrl Pts',(-3.59123857800006,5.2,1.78466976299998));
#309429=CARTESIAN_POINT('Ctrl Pts',(-3.59123857800006,2.2,1.78466976299998));
#309430=CARTESIAN_POINT('Ctrl Pts',(-3.59083760900006,12.2,1.78442313799998));
#309431=CARTESIAN_POINT('Ctrl Pts',(-3.59083760900006,5.2,1.78442313799998));
#309432=CARTESIAN_POINT('Ctrl Pts',(-3.59083760900006,2.2,1.78442313799998));
#309433=CARTESIAN_POINT('Ctrl Pts',(-3.59044182600006,12.2,1.78418041299999));
#309434=CARTESIAN_POINT('Ctrl Pts',(-3.59044182600006,5.2,1.78418041299999));
#309435=CARTESIAN_POINT('Ctrl Pts',(-3.59044182600006,2.2,1.78418041299999));
#309436=CARTESIAN_POINT('Ctrl Pts',(-3.59005125300006,12.2,1.78394158299998));
#309437=CARTESIAN_POINT('Ctrl Pts',(-3.59005125300006,5.2,1.78394158299998));
#309438=CARTESIAN_POINT('Ctrl Pts',(-3.59005125300006,2.2,1.78394158299998));
#309439=CARTESIAN_POINT('Ctrl Pts',(-3.58966590900006,12.2,1.78370664199999));
#309440=CARTESIAN_POINT('Ctrl Pts',(-3.58966590900006,5.2,1.78370664199999));
#309441=CARTESIAN_POINT('Ctrl Pts',(-3.58966590900006,2.2,1.78370664199999));
#309442=CARTESIAN_POINT('Ctrl Pts',(-3.58928581300006,12.2,1.78347557999999));
#309443=CARTESIAN_POINT('Ctrl Pts',(-3.58928581300006,5.2,1.78347557999999));
#309444=CARTESIAN_POINT('Ctrl Pts',(-3.58928581300006,2.2,1.78347557999999));
#309445=CARTESIAN_POINT('Ctrl Pts',(-3.58891098800005,12.2,1.78324839299998));
#309446=CARTESIAN_POINT('Ctrl Pts',(-3.58891098800005,5.2,1.78324839299998));
#309447=CARTESIAN_POINT('Ctrl Pts',(-3.58891098800005,2.2,1.78324839299998));
#309448=CARTESIAN_POINT('Ctrl Pts',(-3.58854145300006,12.2,1.78302507299998));
#309449=CARTESIAN_POINT('Ctrl Pts',(-3.58854145300006,5.2,1.78302507299998));
#309450=CARTESIAN_POINT('Ctrl Pts',(-3.58854145300006,2.2,1.78302507299998));
#309451=CARTESIAN_POINT('Ctrl Pts',(-3.58817723000006,12.2,1.78280561299998));
#309452=CARTESIAN_POINT('Ctrl Pts',(-3.58817723000006,5.2,1.78280561299998));
#309453=CARTESIAN_POINT('Ctrl Pts',(-3.58817723000006,2.2,1.78280561299998));
#309454=CARTESIAN_POINT('Ctrl Pts',(-3.58781834000006,12.2,1.78259000599999));
#309455=CARTESIAN_POINT('Ctrl Pts',(-3.58781834000006,5.2,1.78259000599999));
#309456=CARTESIAN_POINT('Ctrl Pts',(-3.58781834000006,2.2,1.78259000599999));
#309457=CARTESIAN_POINT('Ctrl Pts',(-3.58746480100006,12.2,1.78237824499998));
#309458=CARTESIAN_POINT('Ctrl Pts',(-3.58746480100006,5.2,1.78237824499998));
#309459=CARTESIAN_POINT('Ctrl Pts',(-3.58746480100006,2.2,1.78237824499998));
#309460=CARTESIAN_POINT('Ctrl Pts',(-3.58711663600006,12.2,1.78217032199999));
#309461=CARTESIAN_POINT('Ctrl Pts',(-3.58711663600006,5.2,1.78217032199999));
#309462=CARTESIAN_POINT('Ctrl Pts',(-3.58711663600006,2.2,1.78217032199999));
#309463=CARTESIAN_POINT('Ctrl Pts',(-3.58677386600006,12.2,1.78196623099999));
#309464=CARTESIAN_POINT('Ctrl Pts',(-3.58677386600006,5.2,1.78196623099999));
#309465=CARTESIAN_POINT('Ctrl Pts',(-3.58677386600006,2.2,1.78196623099999));
#309466=CARTESIAN_POINT('Ctrl Pts',(-3.58643651200006,12.2,1.78176596399998));
#309467=CARTESIAN_POINT('Ctrl Pts',(-3.58643651200006,5.2,1.78176596399998));
#309468=CARTESIAN_POINT('Ctrl Pts',(-3.58643651200006,2.2,1.78176596399998));
#309469=CARTESIAN_POINT('Ctrl Pts',(-3.58610459400006,12.2,1.78156951399998));
#309470=CARTESIAN_POINT('Ctrl Pts',(-3.58610459400006,5.2,1.78156951399998));
#309471=CARTESIAN_POINT('Ctrl Pts',(-3.58610459400006,2.2,1.78156951399998));
#309472=CARTESIAN_POINT('Ctrl Pts',(-3.58577813500006,12.2,1.78137687299999));
#309473=CARTESIAN_POINT('Ctrl Pts',(-3.58577813500006,5.2,1.78137687299999));
#309474=CARTESIAN_POINT('Ctrl Pts',(-3.58577813500006,2.2,1.78137687299999));
#309475=CARTESIAN_POINT('Ctrl Pts',(-3.58545715400005,12.2,1.78118803499999));
#309476=CARTESIAN_POINT('Ctrl Pts',(-3.58545715400005,5.2,1.78118803499999));
#309477=CARTESIAN_POINT('Ctrl Pts',(-3.58545715400005,2.2,1.78118803499999));
#309478=CARTESIAN_POINT('Ctrl Pts',(-3.58514167400006,12.2,1.78100299199999));
#309479=CARTESIAN_POINT('Ctrl Pts',(-3.58514167400006,5.2,1.78100299199999));
#309480=CARTESIAN_POINT('Ctrl Pts',(-3.58514167400006,2.2,1.78100299199999));
#309481=CARTESIAN_POINT('Ctrl Pts',(-3.58483171500006,12.2,1.78082173499998));
#309482=CARTESIAN_POINT('Ctrl Pts',(-3.58483171500006,5.2,1.78082173499998));
#309483=CARTESIAN_POINT('Ctrl Pts',(-3.58483171500006,2.2,1.78082173499998));
#309484=CARTESIAN_POINT('Ctrl Pts',(-3.58452729900006,12.2,1.78064425899999));
#309485=CARTESIAN_POINT('Ctrl Pts',(-3.58452729900006,5.2,1.78064425899999));
#309486=CARTESIAN_POINT('Ctrl Pts',(-3.58452729900006,2.2,1.78064425899999));
#309487=CARTESIAN_POINT('Ctrl Pts',(-3.58422844800006,12.2,1.78047055499999));
#309488=CARTESIAN_POINT('Ctrl Pts',(-3.58422844800006,5.2,1.78047055499999));
#309489=CARTESIAN_POINT('Ctrl Pts',(-3.58422844800006,2.2,1.78047055499999));
#309490=CARTESIAN_POINT('Ctrl Pts',(-3.58393518200006,12.2,1.78030061499999));
#309491=CARTESIAN_POINT('Ctrl Pts',(-3.58393518200006,5.2,1.78030061499999));
#309492=CARTESIAN_POINT('Ctrl Pts',(-3.58393518200006,2.2,1.78030061499999));
#309493=CARTESIAN_POINT('Ctrl Pts',(-3.58364752400006,12.2,1.78013443199998));
#309494=CARTESIAN_POINT('Ctrl Pts',(-3.58364752400006,5.2,1.78013443199998));
#309495=CARTESIAN_POINT('Ctrl Pts',(-3.58364752400006,2.2,1.78013443199998));
#309496=CARTESIAN_POINT('Ctrl Pts',(-3.58336549500006,12.2,1.77997199799998));
#309497=CARTESIAN_POINT('Ctrl Pts',(-3.58336549500006,5.2,1.77997199799998));
#309498=CARTESIAN_POINT('Ctrl Pts',(-3.58336549500006,2.2,1.77997199799998));
#309499=CARTESIAN_POINT('Ctrl Pts',(-3.58308911600006,12.2,1.77981330499998));
#309500=CARTESIAN_POINT('Ctrl Pts',(-3.58308911600006,5.2,1.77981330499998));
#309501=CARTESIAN_POINT('Ctrl Pts',(-3.58308911600006,2.2,1.77981330499998));
#309502=CARTESIAN_POINT('Ctrl Pts',(-3.58281840900006,12.2,1.77965834599998));
#309503=CARTESIAN_POINT('Ctrl Pts',(-3.58281840900006,5.2,1.77965834599998));
#309504=CARTESIAN_POINT('Ctrl Pts',(-3.58281840900006,2.2,1.77965834599998));
#309505=CARTESIAN_POINT('Ctrl Pts',(-3.58255339700006,12.2,1.77950711299999));
#309506=CARTESIAN_POINT('Ctrl Pts',(-3.58255339700006,5.2,1.77950711299999));
#309507=CARTESIAN_POINT('Ctrl Pts',(-3.58255339700006,2.2,1.77950711299999));
#309508=CARTESIAN_POINT('Ctrl Pts',(-3.58229410100006,12.2,1.77935959699999));
#309509=CARTESIAN_POINT('Ctrl Pts',(-3.58229410100006,5.2,1.77935959699999));
#309510=CARTESIAN_POINT('Ctrl Pts',(-3.58229410100006,2.2,1.77935959699999));
#309511=CARTESIAN_POINT('Ctrl Pts',(-3.58204054400006,12.2,1.77921579099999));
#309512=CARTESIAN_POINT('Ctrl Pts',(-3.58204054400006,5.2,1.77921579099999));
#309513=CARTESIAN_POINT('Ctrl Pts',(-3.58204054400006,2.2,1.77921579099999));
#309514=CARTESIAN_POINT('Ctrl Pts',(-3.58179274500006,12.2,1.77907568499998));
#309515=CARTESIAN_POINT('Ctrl Pts',(-3.58179274500006,5.2,1.77907568499998));
#309516=CARTESIAN_POINT('Ctrl Pts',(-3.58179274500006,2.2,1.77907568499998));
#309517=CARTESIAN_POINT('Ctrl Pts',(-3.58155073000006,12.2,1.77893927499999));
#309518=CARTESIAN_POINT('Ctrl Pts',(-3.58155073000006,5.2,1.77893927499999));
#309519=CARTESIAN_POINT('Ctrl Pts',(-3.58155073000006,2.2,1.77893927499999));
#309520=CARTESIAN_POINT('Ctrl Pts',(-3.58131451900006,12.2,1.77880654899999));
#309521=CARTESIAN_POINT('Ctrl Pts',(-3.58131451900006,5.2,1.77880654899999));
#309522=CARTESIAN_POINT('Ctrl Pts',(-3.58131451900006,2.2,1.77880654899999));
#309523=CARTESIAN_POINT('Ctrl Pts',(-3.58108413300006,12.2,1.77867749899999));
#309524=CARTESIAN_POINT('Ctrl Pts',(-3.58108413300006,5.2,1.77867749899999));
#309525=CARTESIAN_POINT('Ctrl Pts',(-3.58108413300006,2.2,1.77867749899999));
#309526=CARTESIAN_POINT('Ctrl Pts',(-3.58085959700006,12.2,1.77855211999999));
#309527=CARTESIAN_POINT('Ctrl Pts',(-3.58085959700006,5.2,1.77855211999999));
#309528=CARTESIAN_POINT('Ctrl Pts',(-3.58085959700006,2.2,1.77855211999999));
#309529=CARTESIAN_POINT('Ctrl Pts',(-3.58064093200006,12.2,1.77843039999999));
#309530=CARTESIAN_POINT('Ctrl Pts',(-3.58064093200006,5.2,1.77843039999999));
#309531=CARTESIAN_POINT('Ctrl Pts',(-3.58064093200006,2.2,1.77843039999999));
#309532=CARTESIAN_POINT('Ctrl Pts',(-3.58042816000006,12.2,1.77831233299999));
#309533=CARTESIAN_POINT('Ctrl Pts',(-3.58042816000006,5.2,1.77831233299999));
#309534=CARTESIAN_POINT('Ctrl Pts',(-3.58042816000006,2.2,1.77831233299999));
#309535=CARTESIAN_POINT('Ctrl Pts',(-3.58022130400006,12.2,1.77819790999999));
#309536=CARTESIAN_POINT('Ctrl Pts',(-3.58022130400006,5.2,1.77819790999999));
#309537=CARTESIAN_POINT('Ctrl Pts',(-3.58022130400006,2.2,1.77819790999999));
#309538=CARTESIAN_POINT('Ctrl Pts',(-3.58002038700006,12.2,1.77808712199999));
#309539=CARTESIAN_POINT('Ctrl Pts',(-3.58002038700006,5.2,1.77808712199999));
#309540=CARTESIAN_POINT('Ctrl Pts',(-3.58002038700006,2.2,1.77808712199999));
#309541=CARTESIAN_POINT('Ctrl Pts',(-3.57982543100006,12.2,1.77797995999999));
#309542=CARTESIAN_POINT('Ctrl Pts',(-3.57982543100006,5.2,1.77797995999999));
#309543=CARTESIAN_POINT('Ctrl Pts',(-3.57982543100006,2.2,1.77797995999999));
#309544=CARTESIAN_POINT('Ctrl Pts',(-3.57963645700006,12.2,1.77787641799998));
#309545=CARTESIAN_POINT('Ctrl Pts',(-3.57963645700006,5.2,1.77787641799998));
#309546=CARTESIAN_POINT('Ctrl Pts',(-3.57963645700006,2.2,1.77787641799998));
#309547=CARTESIAN_POINT('Ctrl Pts',(-3.57945349100006,12.2,1.77777648499998));
#309548=CARTESIAN_POINT('Ctrl Pts',(-3.57945349100006,5.2,1.77777648499998));
#309549=CARTESIAN_POINT('Ctrl Pts',(-3.57945349100006,2.2,1.77777648499998));
#309550=CARTESIAN_POINT('Ctrl Pts',(-3.57927655500006,12.2,1.77768015199999));
#309551=CARTESIAN_POINT('Ctrl Pts',(-3.57927655500006,5.2,1.77768015199999));
#309552=CARTESIAN_POINT('Ctrl Pts',(-3.57927655500006,2.2,1.77768015199999));
#309553=CARTESIAN_POINT('Ctrl Pts',(-3.57910567000006,12.2,1.77758741099999));
#309554=CARTESIAN_POINT('Ctrl Pts',(-3.57910567000006,5.2,1.77758741099999));
#309555=CARTESIAN_POINT('Ctrl Pts',(-3.57910567000006,2.2,1.77758741099999));
#309556=CARTESIAN_POINT('Ctrl Pts',(-3.57894086200006,12.2,1.77749825399999));
#309557=CARTESIAN_POINT('Ctrl Pts',(-3.57894086200006,5.2,1.77749825399999));
#309558=CARTESIAN_POINT('Ctrl Pts',(-3.57894086200006,2.2,1.77749825399999));
#309559=CARTESIAN_POINT('Ctrl Pts',(-3.57878215200006,12.2,1.77741267099998));
#309560=CARTESIAN_POINT('Ctrl Pts',(-3.57878215200006,5.2,1.77741267099998));
#309561=CARTESIAN_POINT('Ctrl Pts',(-3.57878215200006,2.2,1.77741267099998));
#309562=CARTESIAN_POINT('Ctrl Pts',(-3.57862956300006,12.2,1.77733065399998));
#309563=CARTESIAN_POINT('Ctrl Pts',(-3.57862956300006,5.2,1.77733065399998));
#309564=CARTESIAN_POINT('Ctrl Pts',(-3.57862956300006,2.2,1.77733065399998));
#309565=CARTESIAN_POINT('Ctrl Pts',(-3.57848311700006,12.2,1.77725219399999));
#309566=CARTESIAN_POINT('Ctrl Pts',(-3.57848311700006,5.2,1.77725219399999));
#309567=CARTESIAN_POINT('Ctrl Pts',(-3.57848311700006,2.2,1.77725219399999));
#309568=CARTESIAN_POINT('Ctrl Pts',(-3.57834283900006,12.2,1.77717728099998));
#309569=CARTESIAN_POINT('Ctrl Pts',(-3.57834283900006,5.2,1.77717728099998));
#309570=CARTESIAN_POINT('Ctrl Pts',(-3.57834283900006,2.2,1.77717728099998));
#309571=CARTESIAN_POINT('Ctrl Pts',(-3.57820875100006,12.2,1.77710590699999));
#309572=CARTESIAN_POINT('Ctrl Pts',(-3.57820875100006,5.2,1.77710590699999));
#309573=CARTESIAN_POINT('Ctrl Pts',(-3.57820875100006,2.2,1.77710590699999));
#309574=CARTESIAN_POINT('Ctrl Pts',(-3.57808087800006,12.2,1.77703806299998));
#309575=CARTESIAN_POINT('Ctrl Pts',(-3.57808087800006,5.2,1.77703806299998));
#309576=CARTESIAN_POINT('Ctrl Pts',(-3.57808087800006,2.2,1.77703806299998));
#309577=CARTESIAN_POINT('Ctrl Pts',(-3.57795924500006,12.2,1.77697373799999));
#309578=CARTESIAN_POINT('Ctrl Pts',(-3.57795924500006,5.2,1.77697373799999));
#309579=CARTESIAN_POINT('Ctrl Pts',(-3.57795924500006,2.2,1.77697373799999));
#309580=CARTESIAN_POINT('Ctrl Pts',(-3.57784387600006,12.2,1.77691292299999));
#309581=CARTESIAN_POINT('Ctrl Pts',(-3.57784387600006,5.2,1.77691292299999));
#309582=CARTESIAN_POINT('Ctrl Pts',(-3.57784387600006,2.2,1.77691292299999));
#309583=CARTESIAN_POINT('Ctrl Pts',(-3.57773479500006,12.2,1.77685560799999));
#309584=CARTESIAN_POINT('Ctrl Pts',(-3.57773479500006,5.2,1.77685560799999));
#309585=CARTESIAN_POINT('Ctrl Pts',(-3.57773479500006,2.2,1.77685560799999));
#309586=CARTESIAN_POINT('Ctrl Pts',(-3.57763202200006,12.2,1.77680178599998));
#309587=CARTESIAN_POINT('Ctrl Pts',(-3.57763202200006,5.2,1.77680178599998));
#309588=CARTESIAN_POINT('Ctrl Pts',(-3.57763202200006,2.2,1.77680178599998));
#309589=CARTESIAN_POINT('Ctrl Pts',(-3.57753557800006,12.2,1.77675144799998));
#309590=CARTESIAN_POINT('Ctrl Pts',(-3.57753557800006,5.2,1.77675144799998));
#309591=CARTESIAN_POINT('Ctrl Pts',(-3.57753557800006,2.2,1.77675144799998));
#309592=CARTESIAN_POINT('Ctrl Pts',(-3.57744548500006,12.2,1.77670458499998));
#309593=CARTESIAN_POINT('Ctrl Pts',(-3.57744548500006,5.2,1.77670458499998));
#309594=CARTESIAN_POINT('Ctrl Pts',(-3.57744548500006,2.2,1.77670458499998));
#309595=CARTESIAN_POINT('Ctrl Pts',(-3.57736176800006,12.2,1.77666118799999));
#309596=CARTESIAN_POINT('Ctrl Pts',(-3.57736176800006,5.2,1.77666118799999));
#309597=CARTESIAN_POINT('Ctrl Pts',(-3.57736176800006,2.2,1.77666118799999));
#309598=CARTESIAN_POINT('Ctrl Pts',(-3.57728445400006,12.2,1.77662124499999));
#309599=CARTESIAN_POINT('Ctrl Pts',(-3.57728445400006,5.2,1.77662124499999));
#309600=CARTESIAN_POINT('Ctrl Pts',(-3.57728445400006,2.2,1.77662124499999));
#309601=CARTESIAN_POINT('Ctrl Pts',(-3.57721357500006,12.2,1.77658474499998));
#309602=CARTESIAN_POINT('Ctrl Pts',(-3.57721357500006,5.2,1.77658474499998));
#309603=CARTESIAN_POINT('Ctrl Pts',(-3.57721357500006,2.2,1.77658474499998));
#309604=CARTESIAN_POINT('Ctrl Pts',(-3.57714916000006,12.2,1.77655167399998));
#309605=CARTESIAN_POINT('Ctrl Pts',(-3.57714916000006,5.2,1.77655167399998));
#309606=CARTESIAN_POINT('Ctrl Pts',(-3.57714916000006,2.2,1.77655167399998));
#309607=CARTESIAN_POINT('Ctrl Pts',(-3.57709123600006,12.2,1.77652202299999));
#309608=CARTESIAN_POINT('Ctrl Pts',(-3.57709123600006,5.2,1.77652202299999));
#309609=CARTESIAN_POINT('Ctrl Pts',(-3.57709123600006,2.2,1.77652202299999));
#309610=CARTESIAN_POINT('Ctrl Pts',(-3.57703982100006,12.2,1.77649578199999));
#309611=CARTESIAN_POINT('Ctrl Pts',(-3.57703982100006,5.2,1.77649578199999));
#309612=CARTESIAN_POINT('Ctrl Pts',(-3.57703982100006,2.2,1.77649578199999));
#309613=CARTESIAN_POINT('Ctrl Pts',(-3.57699012332173,12.2,1.77647050473256));
#309614=CARTESIAN_POINT('Ctrl Pts',(-3.57699012332173,5.2,1.77647050473256));
#309615=CARTESIAN_POINT('Ctrl Pts',(-3.57699012332173,2.2,1.77647050473256));
#309616=CARTESIAN_POINT('Ctrl Pts',(-3.5769561191391,12.2,1.77645329379262));
#309617=CARTESIAN_POINT('Ctrl Pts',(-3.5769561191391,5.2,1.77645329379262));
#309618=CARTESIAN_POINT('Ctrl Pts',(-3.5769561191391,2.2,1.77645329379262));
#309619=CARTESIAN_POINT('Ctrl Pts',(-3.57693369172082,12.2,1.77644200373862));
#309620=CARTESIAN_POINT('Ctrl Pts',(-3.57693369172082,5.2,1.77644200373862));
#309621=CARTESIAN_POINT('Ctrl Pts',(-3.57693369172082,2.2,1.77644200373862));
#309622=CARTESIAN_POINT('Ctrl Pts',(-3.57691970642208,12.2,1.77643500294693));
#309623=CARTESIAN_POINT('Ctrl Pts',(-3.57691970642208,5.2,1.77643500294693));
#309624=CARTESIAN_POINT('Ctrl Pts',(-3.57691970642208,2.2,1.77643500294693));
#309625=CARTESIAN_POINT('Ctrl Pts',(-3.57691107200006,12.2,1.77643067499998));
#309626=CARTESIAN_POINT('Ctrl Pts',(-3.57691107200006,5.2,1.77643067499998));
#309627=CARTESIAN_POINT('Ctrl Pts',(-3.57691107200006,2.2,1.77643067499998));
#309628=CARTESIAN_POINT('',(-3.57691116300006,2.7,1.77643049499998));
#309629=CARTESIAN_POINT('',(-3.57691116300006,12.2,1.77643049499999));
#309630=CARTESIAN_POINT('Ctrl Pts',(-4.09164015000006,2.7,2.41267090399998));
#309631=CARTESIAN_POINT('Ctrl Pts',(-3.98263969989265,2.7,2.19591905262488));
#309632=CARTESIAN_POINT('Ctrl Pts',(-3.86694481153583,2.6999999999955,2.0417626137312));
#309633=CARTESIAN_POINT('Ctrl Pts',(-3.66335261251423,2.6999999999955,1.82497302201057));
#309634=CARTESIAN_POINT('Ctrl Pts',(-3.58821589879921,2.7,1.78227875956844));
#309635=CARTESIAN_POINT('Ctrl Pts',(-3.57721236596159,2.7,1.77658390024682));
#309636=CARTESIAN_POINT('Ctrl Pts',(-3.57706216165585,2.7,1.77650640769084));
#309637=CARTESIAN_POINT('Ctrl Pts',(-3.57691107226376,2.7,1.77643067513216));
#309638=CARTESIAN_POINT('Origin',(-3.57686520200006,15.2,1.77640766899998));
#309639=CARTESIAN_POINT('',(-3.24665273100006,2.7,1.61241156299999));
#309640=CARTESIAN_POINT('',(-3.24665273100006,2.2,1.61241156299999));
#309641=CARTESIAN_POINT('',(-1.78843260106674,2.7,0.888203834365703));
#309642=CARTESIAN_POINT('Origin',(-5.66300478732629E-14,15.2,-1.77635683940025E-14));
#309643=CARTESIAN_POINT('',(-3.45664454600006,2.7,1.09189444699998));
#309644=CARTESIAN_POINT('',(-3.45664454600006,12.2,1.09189444699998));
#309645=CARTESIAN_POINT('Origin',(-5.66300478732629E-14,2.7,-1.92943768261394E-14));
#309646=CARTESIAN_POINT('Origin',(-5.66300478732629E-14,15.2,-1.77635683940025E-14));
#309647=CARTESIAN_POINT('',(-3.80824761100006,2.7,1.20295979699998));
#309648=CARTESIAN_POINT('',(-3.80824761100006,12.2,1.20295979699999));
#309649=CARTESIAN_POINT('',(-5.68586833118453E-14,2.7,-1.92221548309966E-14));
#309650=CARTESIAN_POINT('Ctrl Pts',(-3.80828031400006,12.2,1.20296984599999));
#309651=CARTESIAN_POINT('Ctrl Pts',(-3.80828031400006,5.2,1.20296984599999));
#309652=CARTESIAN_POINT('Ctrl Pts',(-3.80828031400006,2.2,1.20296984599999));
#309653=CARTESIAN_POINT('Ctrl Pts',(-3.80828641700006,12.2,1.20297174799999));
#309654=CARTESIAN_POINT('Ctrl Pts',(-3.80828641700006,5.2,1.20297174799999));
#309655=CARTESIAN_POINT('Ctrl Pts',(-3.80828641700006,2.2,1.20297174799999));
#309656=CARTESIAN_POINT('Ctrl Pts',(-3.80829932800006,12.2,1.20297575999999));
#309657=CARTESIAN_POINT('Ctrl Pts',(-3.80829932800006,5.2,1.20297575999999));
#309658=CARTESIAN_POINT('Ctrl Pts',(-3.80829932800006,2.2,1.20297575999999));
#309659=CARTESIAN_POINT('Ctrl Pts',(-3.80832081300006,12.2,1.20298240199999));
#309660=CARTESIAN_POINT('Ctrl Pts',(-3.80832081300006,5.2,1.20298240199999));
#309661=CARTESIAN_POINT('Ctrl Pts',(-3.80832081300006,2.2,1.20298240199999));
#309662=CARTESIAN_POINT('Ctrl Pts',(-3.80835369800006,12.2,1.20299250699999));
#309663=CARTESIAN_POINT('Ctrl Pts',(-3.80835369800006,5.2,1.20299250699999));
#309664=CARTESIAN_POINT('Ctrl Pts',(-3.80835369800006,2.2,1.20299250699999));
#309665=CARTESIAN_POINT('Ctrl Pts',(-3.80840186700006,12.2,1.20300721599999));
#309666=CARTESIAN_POINT('Ctrl Pts',(-3.80840186700006,5.2,1.20300721599999));
#309667=CARTESIAN_POINT('Ctrl Pts',(-3.80840186700006,2.2,1.20300721599999));
#309668=CARTESIAN_POINT('Ctrl Pts',(-3.80845709700006,12.2,1.20302399999999));
#309669=CARTESIAN_POINT('Ctrl Pts',(-3.80845709700006,5.2,1.20302399999999));
#309670=CARTESIAN_POINT('Ctrl Pts',(-3.80845709700006,2.2,1.20302399999999));
#309671=CARTESIAN_POINT('Ctrl Pts',(-3.80851938100006,12.2,1.20304284399999));
#309672=CARTESIAN_POINT('Ctrl Pts',(-3.80851938100006,5.2,1.20304284399999));
#309673=CARTESIAN_POINT('Ctrl Pts',(-3.80851938100006,2.2,1.20304284399999));
#309674=CARTESIAN_POINT('Ctrl Pts',(-3.80858871200005,12.2,1.20306372999998));
#309675=CARTESIAN_POINT('Ctrl Pts',(-3.80858871200005,5.2,1.20306372999998));
#309676=CARTESIAN_POINT('Ctrl Pts',(-3.80858871200005,2.2,1.20306372999998));
#309677=CARTESIAN_POINT('Ctrl Pts',(-3.80866507800006,12.2,1.20308663199999));
#309678=CARTESIAN_POINT('Ctrl Pts',(-3.80866507800006,5.2,1.20308663199999));
#309679=CARTESIAN_POINT('Ctrl Pts',(-3.80866507800006,2.2,1.20308663199999));
#309680=CARTESIAN_POINT('Ctrl Pts',(-3.80874846400006,12.2,1.20311152099998));
#309681=CARTESIAN_POINT('Ctrl Pts',(-3.80874846400006,5.2,1.20311152099998));
#309682=CARTESIAN_POINT('Ctrl Pts',(-3.80874846400006,2.2,1.20311152099998));
#309683=CARTESIAN_POINT('Ctrl Pts',(-3.80883885900006,12.2,1.20313836599999));
#309684=CARTESIAN_POINT('Ctrl Pts',(-3.80883885900006,5.2,1.20313836599999));
#309685=CARTESIAN_POINT('Ctrl Pts',(-3.80883885900006,2.2,1.20313836599999));
#309686=CARTESIAN_POINT('Ctrl Pts',(-3.80893624900006,12.2,1.20316713899999));
#309687=CARTESIAN_POINT('Ctrl Pts',(-3.80893624900006,5.2,1.20316713899999));
#309688=CARTESIAN_POINT('Ctrl Pts',(-3.80893624900006,2.2,1.20316713899999));
#309689=CARTESIAN_POINT('Ctrl Pts',(-3.80904062400006,12.2,1.20319781699999));
#309690=CARTESIAN_POINT('Ctrl Pts',(-3.80904062400006,5.2,1.20319781699999));
#309691=CARTESIAN_POINT('Ctrl Pts',(-3.80904062400006,2.2,1.20319781699999));
#309692=CARTESIAN_POINT('Ctrl Pts',(-3.80915197500006,12.2,1.20323037899999));
#309693=CARTESIAN_POINT('Ctrl Pts',(-3.80915197500006,5.2,1.20323037899999));
#309694=CARTESIAN_POINT('Ctrl Pts',(-3.80915197500006,2.2,1.20323037899999));
#309695=CARTESIAN_POINT('Ctrl Pts',(-3.80927029100006,12.2,1.20326480299998));
#309696=CARTESIAN_POINT('Ctrl Pts',(-3.80927029100006,5.2,1.20326480299998));
#309697=CARTESIAN_POINT('Ctrl Pts',(-3.80927029100006,2.2,1.20326480299998));
#309698=CARTESIAN_POINT('Ctrl Pts',(-3.80939556400006,12.2,1.20330106999999));
#309699=CARTESIAN_POINT('Ctrl Pts',(-3.80939556400006,5.2,1.20330106999999));
#309700=CARTESIAN_POINT('Ctrl Pts',(-3.80939556400006,2.2,1.20330106999999));
#309701=CARTESIAN_POINT('Ctrl Pts',(-3.80952778300006,12.2,1.20333915499999));
#309702=CARTESIAN_POINT('Ctrl Pts',(-3.80952778300006,5.2,1.20333915499999));
#309703=CARTESIAN_POINT('Ctrl Pts',(-3.80952778300006,2.2,1.20333915499999));
#309704=CARTESIAN_POINT('Ctrl Pts',(-3.80966693600006,12.2,1.20337903699999));
#309705=CARTESIAN_POINT('Ctrl Pts',(-3.80966693600006,5.2,1.20337903699999));
#309706=CARTESIAN_POINT('Ctrl Pts',(-3.80966693600006,2.2,1.20337903699999));
#309707=CARTESIAN_POINT('Ctrl Pts',(-3.80981301400006,12.2,1.20342068999999));
#309708=CARTESIAN_POINT('Ctrl Pts',(-3.80981301400006,5.2,1.20342068999999));
#309709=CARTESIAN_POINT('Ctrl Pts',(-3.80981301400006,2.2,1.20342068999999));
#309710=CARTESIAN_POINT('Ctrl Pts',(-3.80996600500006,12.2,1.20346409199998));
#309711=CARTESIAN_POINT('Ctrl Pts',(-3.80996600500006,5.2,1.20346409199998));
#309712=CARTESIAN_POINT('Ctrl Pts',(-3.80996600500006,2.2,1.20346409199998));
#309713=CARTESIAN_POINT('Ctrl Pts',(-3.81012589900006,12.2,1.20350921799998));
#309714=CARTESIAN_POINT('Ctrl Pts',(-3.81012589900006,5.2,1.20350921799998));
#309715=CARTESIAN_POINT('Ctrl Pts',(-3.81012589900006,2.2,1.20350921799998));
#309716=CARTESIAN_POINT('Ctrl Pts',(-3.81029268400006,12.2,1.20355604499998));
#309717=CARTESIAN_POINT('Ctrl Pts',(-3.81029268400006,5.2,1.20355604499998));
#309718=CARTESIAN_POINT('Ctrl Pts',(-3.81029268400006,2.2,1.20355604499998));
#309719=CARTESIAN_POINT('Ctrl Pts',(-3.81046635100006,12.2,1.20360455299998));
#309720=CARTESIAN_POINT('Ctrl Pts',(-3.81046635100006,5.2,1.20360455299998));
#309721=CARTESIAN_POINT('Ctrl Pts',(-3.81046635100006,2.2,1.20360455299998));
#309722=CARTESIAN_POINT('Ctrl Pts',(-3.81064689100006,12.2,1.20365471899999));
#309723=CARTESIAN_POINT('Ctrl Pts',(-3.81064689100006,5.2,1.20365471899999));
#309724=CARTESIAN_POINT('Ctrl Pts',(-3.81064689100006,2.2,1.20365471899999));
#309725=CARTESIAN_POINT('Ctrl Pts',(-3.81083429100006,12.2,1.20370652099998));
#309726=CARTESIAN_POINT('Ctrl Pts',(-3.81083429100006,5.2,1.20370652099998));
#309727=CARTESIAN_POINT('Ctrl Pts',(-3.81083429100006,2.2,1.20370652099998));
#309728=CARTESIAN_POINT('Ctrl Pts',(-3.81102854100006,12.2,1.20375993599998));
#309729=CARTESIAN_POINT('Ctrl Pts',(-3.81102854100006,5.2,1.20375993599998));
#309730=CARTESIAN_POINT('Ctrl Pts',(-3.81102854100006,2.2,1.20375993599998));
#309731=CARTESIAN_POINT('Ctrl Pts',(-3.81122963200006,12.2,1.20381494299998));
#309732=CARTESIAN_POINT('Ctrl Pts',(-3.81122963200006,5.2,1.20381494299998));
#309733=CARTESIAN_POINT('Ctrl Pts',(-3.81122963200006,2.2,1.20381494299998));
#309734=CARTESIAN_POINT('Ctrl Pts',(-3.81143755300006,12.2,1.20387151799998));
#309735=CARTESIAN_POINT('Ctrl Pts',(-3.81143755300006,5.2,1.20387151799998));
#309736=CARTESIAN_POINT('Ctrl Pts',(-3.81143755300006,2.2,1.20387151799998));
#309737=CARTESIAN_POINT('Ctrl Pts',(-3.81165229300006,12.2,1.20392964099999));
#309738=CARTESIAN_POINT('Ctrl Pts',(-3.81165229300006,5.2,1.20392964099999));
#309739=CARTESIAN_POINT('Ctrl Pts',(-3.81165229300006,2.2,1.20392964099999));
#309740=CARTESIAN_POINT('Ctrl Pts',(-3.81187384200006,12.2,1.20398928799998));
#309741=CARTESIAN_POINT('Ctrl Pts',(-3.81187384200006,5.2,1.20398928799998));
#309742=CARTESIAN_POINT('Ctrl Pts',(-3.81187384200006,2.2,1.20398928799998));
#309743=CARTESIAN_POINT('Ctrl Pts',(-3.81210219000006,12.2,1.20405043799999));
#309744=CARTESIAN_POINT('Ctrl Pts',(-3.81210219000006,5.2,1.20405043799999));
#309745=CARTESIAN_POINT('Ctrl Pts',(-3.81210219000006,2.2,1.20405043799999));
#309746=CARTESIAN_POINT('Ctrl Pts',(-3.81233732600006,12.2,1.20411306999999));
#309747=CARTESIAN_POINT('Ctrl Pts',(-3.81233732600006,5.2,1.20411306999999));
#309748=CARTESIAN_POINT('Ctrl Pts',(-3.81233732600006,2.2,1.20411306999999));
#309749=CARTESIAN_POINT('Ctrl Pts',(-3.81257924000006,12.2,1.20417716199999));
#309750=CARTESIAN_POINT('Ctrl Pts',(-3.81257924000006,5.2,1.20417716199999));
#309751=CARTESIAN_POINT('Ctrl Pts',(-3.81257924000006,2.2,1.20417716199999));
#309752=CARTESIAN_POINT('Ctrl Pts',(-3.81282792200006,12.2,1.20424269199999));
#309753=CARTESIAN_POINT('Ctrl Pts',(-3.81282792200006,5.2,1.20424269199999));
#309754=CARTESIAN_POINT('Ctrl Pts',(-3.81282792200006,2.2,1.20424269199999));
#309755=CARTESIAN_POINT('Ctrl Pts',(-3.81308336100005,12.2,1.20430963899999));
#309756=CARTESIAN_POINT('Ctrl Pts',(-3.81308336100005,5.2,1.20430963899999));
#309757=CARTESIAN_POINT('Ctrl Pts',(-3.81308336100005,2.2,1.20430963899999));
#309758=CARTESIAN_POINT('Ctrl Pts',(-3.81334554600006,12.2,1.20437798099998));
#309759=CARTESIAN_POINT('Ctrl Pts',(-3.81334554600006,5.2,1.20437798099998));
#309760=CARTESIAN_POINT('Ctrl Pts',(-3.81334554600006,2.2,1.20437798099998));
#309761=CARTESIAN_POINT('Ctrl Pts',(-3.81361446800006,12.2,1.20444769799999));
#309762=CARTESIAN_POINT('Ctrl Pts',(-3.81361446800006,5.2,1.20444769799999));
#309763=CARTESIAN_POINT('Ctrl Pts',(-3.81361446800006,2.2,1.20444769799999));
#309764=CARTESIAN_POINT('Ctrl Pts',(-3.81389011800006,12.2,1.20451876599999));
#309765=CARTESIAN_POINT('Ctrl Pts',(-3.81389011800006,5.2,1.20451876599999));
#309766=CARTESIAN_POINT('Ctrl Pts',(-3.81389011800006,2.2,1.20451876599999));
#309767=CARTESIAN_POINT('Ctrl Pts',(-3.81417248200006,12.2,1.20459116699998));
#309768=CARTESIAN_POINT('Ctrl Pts',(-3.81417248200006,5.2,1.20459116699998));
#309769=CARTESIAN_POINT('Ctrl Pts',(-3.81417248200006,2.2,1.20459116699998));
#309770=CARTESIAN_POINT('Ctrl Pts',(-3.81446155400006,12.2,1.20466487799999));
#309771=CARTESIAN_POINT('Ctrl Pts',(-3.81446155400006,5.2,1.20466487799999));
#309772=CARTESIAN_POINT('Ctrl Pts',(-3.81446155400006,2.2,1.20466487799999));
#309773=CARTESIAN_POINT('Ctrl Pts',(-3.81475731900006,12.2,1.20473987899999));
#309774=CARTESIAN_POINT('Ctrl Pts',(-3.81475731900006,5.2,1.20473987899999));
#309775=CARTESIAN_POINT('Ctrl Pts',(-3.81475731900006,2.2,1.20473987899999));
#309776=CARTESIAN_POINT('Ctrl Pts',(-3.81505977100006,12.2,1.20481614899999));
#309777=CARTESIAN_POINT('Ctrl Pts',(-3.81505977100006,5.2,1.20481614899999));
#309778=CARTESIAN_POINT('Ctrl Pts',(-3.81505977100006,2.2,1.20481614899999));
#309779=CARTESIAN_POINT('Ctrl Pts',(-3.81536889800006,12.2,1.20489366599998));
#309780=CARTESIAN_POINT('Ctrl Pts',(-3.81536889800006,5.2,1.20489366599998));
#309781=CARTESIAN_POINT('Ctrl Pts',(-3.81536889800006,2.2,1.20489366599998));
#309782=CARTESIAN_POINT('Ctrl Pts',(-3.81568469000006,12.2,1.20497241099998));
#309783=CARTESIAN_POINT('Ctrl Pts',(-3.81568469000006,5.2,1.20497241099998));
#309784=CARTESIAN_POINT('Ctrl Pts',(-3.81568469000006,2.2,1.20497241099998));
#309785=CARTESIAN_POINT('Ctrl Pts',(-3.81600713700006,12.2,1.20505236199998));
#309786=CARTESIAN_POINT('Ctrl Pts',(-3.81600713700006,5.2,1.20505236199998));
#309787=CARTESIAN_POINT('Ctrl Pts',(-3.81600713700006,2.2,1.20505236199998));
#309788=CARTESIAN_POINT('Ctrl Pts',(-3.81633622800006,12.2,1.20513349999999));
#309789=CARTESIAN_POINT('Ctrl Pts',(-3.81633622800006,5.2,1.20513349999999));
#309790=CARTESIAN_POINT('Ctrl Pts',(-3.81633622800006,2.2,1.20513349999999));
#309791=CARTESIAN_POINT('Ctrl Pts',(-3.81667195400006,12.2,1.20521580199998));
#309792=CARTESIAN_POINT('Ctrl Pts',(-3.81667195400006,5.2,1.20521580199998));
#309793=CARTESIAN_POINT('Ctrl Pts',(-3.81667195400006,2.2,1.20521580199998));
#309794=CARTESIAN_POINT('Ctrl Pts',(-3.81701430400006,12.2,1.20529924999999));
#309795=CARTESIAN_POINT('Ctrl Pts',(-3.81701430400006,5.2,1.20529924999999));
#309796=CARTESIAN_POINT('Ctrl Pts',(-3.81701430400006,2.2,1.20529924999999));
#309797=CARTESIAN_POINT('Ctrl Pts',(-3.81736326800006,12.2,1.20538382199999));
#309798=CARTESIAN_POINT('Ctrl Pts',(-3.81736326800006,5.2,1.20538382199999));
#309799=CARTESIAN_POINT('Ctrl Pts',(-3.81736326800006,2.2,1.20538382199999));
#309800=CARTESIAN_POINT('Ctrl Pts',(-3.81771883600006,12.2,1.20546949899999));
#309801=CARTESIAN_POINT('Ctrl Pts',(-3.81771883600006,5.2,1.20546949899999));
#309802=CARTESIAN_POINT('Ctrl Pts',(-3.81771883600006,2.2,1.20546949899999));
#309803=CARTESIAN_POINT('Ctrl Pts',(-3.81808099700006,12.2,1.20555625999998));
#309804=CARTESIAN_POINT('Ctrl Pts',(-3.81808099700006,5.2,1.20555625999998));
#309805=CARTESIAN_POINT('Ctrl Pts',(-3.81808099700006,2.2,1.20555625999998));
#309806=CARTESIAN_POINT('Ctrl Pts',(-3.81844974300006,12.2,1.20564408499999));
#309807=CARTESIAN_POINT('Ctrl Pts',(-3.81844974300006,5.2,1.20564408499999));
#309808=CARTESIAN_POINT('Ctrl Pts',(-3.81844974300006,2.2,1.20564408499999));
#309809=CARTESIAN_POINT('Ctrl Pts',(-3.81882506000006,12.2,1.20573295599999));
#309810=CARTESIAN_POINT('Ctrl Pts',(-3.81882506000006,5.2,1.20573295599999));
#309811=CARTESIAN_POINT('Ctrl Pts',(-3.81882506000006,2.2,1.20573295599999));
#309812=CARTESIAN_POINT('Ctrl Pts',(-3.81920694300006,12.2,1.20582284899998));
#309813=CARTESIAN_POINT('Ctrl Pts',(-3.81920694300006,5.2,1.20582284899998));
#309814=CARTESIAN_POINT('Ctrl Pts',(-3.81920694300006,2.2,1.20582284899998));
#309815=CARTESIAN_POINT('Ctrl Pts',(-3.81959537800006,12.2,1.20591374799998));
#309816=CARTESIAN_POINT('Ctrl Pts',(-3.81959537800006,5.2,1.20591374799998));
#309817=CARTESIAN_POINT('Ctrl Pts',(-3.81959537800006,2.2,1.20591374799998));
#309818=CARTESIAN_POINT('Ctrl Pts',(-3.81999035700006,12.2,1.20600563099998));
#309819=CARTESIAN_POINT('Ctrl Pts',(-3.81999035700006,5.2,1.20600563099998));
#309820=CARTESIAN_POINT('Ctrl Pts',(-3.81999035700006,2.2,1.20600563099998));
#309821=CARTESIAN_POINT('Ctrl Pts',(-3.82039186800006,12.2,1.20609847899999));
#309822=CARTESIAN_POINT('Ctrl Pts',(-3.82039186800006,5.2,1.20609847899999));
#309823=CARTESIAN_POINT('Ctrl Pts',(-3.82039186800006,2.2,1.20609847899999));
#309824=CARTESIAN_POINT('Ctrl Pts',(-3.82079990200006,12.2,1.20619227199999));
#309825=CARTESIAN_POINT('Ctrl Pts',(-3.82079990200006,5.2,1.20619227199999));
#309826=CARTESIAN_POINT('Ctrl Pts',(-3.82079990200006,2.2,1.20619227199999));
#309827=CARTESIAN_POINT('Ctrl Pts',(-3.82121445000006,12.2,1.20628698999999));
#309828=CARTESIAN_POINT('Ctrl Pts',(-3.82121445000006,5.2,1.20628698999999));
#309829=CARTESIAN_POINT('Ctrl Pts',(-3.82121445000006,2.2,1.20628698999999));
#309830=CARTESIAN_POINT('Ctrl Pts',(-3.82163550100006,12.2,1.20638261599999));
#309831=CARTESIAN_POINT('Ctrl Pts',(-3.82163550100006,5.2,1.20638261599999));
#309832=CARTESIAN_POINT('Ctrl Pts',(-3.82163550100006,2.2,1.20638261599999));
#309833=CARTESIAN_POINT('Ctrl Pts',(-3.82206304400006,12.2,1.20647912799999));
#309834=CARTESIAN_POINT('Ctrl Pts',(-3.82206304400006,5.2,1.20647912799999));
#309835=CARTESIAN_POINT('Ctrl Pts',(-3.82206304400006,2.2,1.20647912799999));
#309836=CARTESIAN_POINT('Ctrl Pts',(-3.82249707000006,12.2,1.20657650699998));
#309837=CARTESIAN_POINT('Ctrl Pts',(-3.82249707000006,5.2,1.20657650699998));
#309838=CARTESIAN_POINT('Ctrl Pts',(-3.82249707000006,2.2,1.20657650699998));
#309839=CARTESIAN_POINT('Ctrl Pts',(-3.82293757000006,12.2,1.20667473499998));
#309840=CARTESIAN_POINT('Ctrl Pts',(-3.82293757000006,5.2,1.20667473499998));
#309841=CARTESIAN_POINT('Ctrl Pts',(-3.82293757000006,2.2,1.20667473499998));
#309842=CARTESIAN_POINT('Ctrl Pts',(-3.82338453200005,12.2,1.20677379099998));
#309843=CARTESIAN_POINT('Ctrl Pts',(-3.82338453200005,5.2,1.20677379099998));
#309844=CARTESIAN_POINT('Ctrl Pts',(-3.82338453200005,2.2,1.20677379099998));
#309845=CARTESIAN_POINT('Ctrl Pts',(-3.82383794600006,12.2,1.20687365699998));
#309846=CARTESIAN_POINT('Ctrl Pts',(-3.82383794600006,5.2,1.20687365699998));
#309847=CARTESIAN_POINT('Ctrl Pts',(-3.82383794600006,2.2,1.20687365699998));
#309848=CARTESIAN_POINT('Ctrl Pts',(-3.82429780400006,12.2,1.20697431499998));
#309849=CARTESIAN_POINT('Ctrl Pts',(-3.82429780400006,5.2,1.20697431499998));
#309850=CARTESIAN_POINT('Ctrl Pts',(-3.82429780400006,2.2,1.20697431499998));
#309851=CARTESIAN_POINT('Ctrl Pts',(-3.82476409500006,12.2,1.20707574399999));
#309852=CARTESIAN_POINT('Ctrl Pts',(-3.82476409500006,5.2,1.20707574399999));
#309853=CARTESIAN_POINT('Ctrl Pts',(-3.82476409500006,2.2,1.20707574399999));
#309854=CARTESIAN_POINT('Ctrl Pts',(-3.82523680800006,12.2,1.20717792599998));
#309855=CARTESIAN_POINT('Ctrl Pts',(-3.82523680800006,5.2,1.20717792599998));
#309856=CARTESIAN_POINT('Ctrl Pts',(-3.82523680800006,2.2,1.20717792599998));
#309857=CARTESIAN_POINT('Ctrl Pts',(-3.82571593500006,12.2,1.20728084299999));
#309858=CARTESIAN_POINT('Ctrl Pts',(-3.82571593500006,5.2,1.20728084299999));
#309859=CARTESIAN_POINT('Ctrl Pts',(-3.82571593500006,2.2,1.20728084299999));
#309860=CARTESIAN_POINT('Ctrl Pts',(-3.82620146300006,12.2,1.20738447399999));
#309861=CARTESIAN_POINT('Ctrl Pts',(-3.82620146300006,5.2,1.20738447399999));
#309862=CARTESIAN_POINT('Ctrl Pts',(-3.82620146300006,2.2,1.20738447399999));
#309863=CARTESIAN_POINT('Ctrl Pts',(-3.82669338600006,12.2,1.20748880199999));
#309864=CARTESIAN_POINT('Ctrl Pts',(-3.82669338600006,5.2,1.20748880199999));
#309865=CARTESIAN_POINT('Ctrl Pts',(-3.82669338600006,2.2,1.20748880199999));
#309866=CARTESIAN_POINT('Ctrl Pts',(-3.82719169200006,12.2,1.20759380899999));
#309867=CARTESIAN_POINT('Ctrl Pts',(-3.82719169200006,5.2,1.20759380899999));
#309868=CARTESIAN_POINT('Ctrl Pts',(-3.82719169200006,2.2,1.20759380899999));
#309869=CARTESIAN_POINT('Ctrl Pts',(-3.82769637100006,12.2,1.20769947499999));
#309870=CARTESIAN_POINT('Ctrl Pts',(-3.82769637100006,5.2,1.20769947499999));
#309871=CARTESIAN_POINT('Ctrl Pts',(-3.82769637100006,2.2,1.20769947499999));
#309872=CARTESIAN_POINT('Ctrl Pts',(-3.82820741400006,12.2,1.20780578099998));
#309873=CARTESIAN_POINT('Ctrl Pts',(-3.82820741400006,5.2,1.20780578099998));
#309874=CARTESIAN_POINT('Ctrl Pts',(-3.82820741400006,2.2,1.20780578099998));
#309875=CARTESIAN_POINT('Ctrl Pts',(-3.82872480900006,12.2,1.20791271199999));
#309876=CARTESIAN_POINT('Ctrl Pts',(-3.82872480900006,5.2,1.20791271199999));
#309877=CARTESIAN_POINT('Ctrl Pts',(-3.82872480900006,2.2,1.20791271199999));
#309878=CARTESIAN_POINT('Ctrl Pts',(-3.82924854800006,12.2,1.20802024499998));
#309879=CARTESIAN_POINT('Ctrl Pts',(-3.82924854800006,5.2,1.20802024499998));
#309880=CARTESIAN_POINT('Ctrl Pts',(-3.82924854800006,2.2,1.20802024499998));
#309881=CARTESIAN_POINT('Ctrl Pts',(-3.82977862000006,12.2,1.20812836499999));
#309882=CARTESIAN_POINT('Ctrl Pts',(-3.82977862000006,5.2,1.20812836499999));
#309883=CARTESIAN_POINT('Ctrl Pts',(-3.82977862000006,2.2,1.20812836499999));
#309884=CARTESIAN_POINT('Ctrl Pts',(-3.83031501700006,12.2,1.20823705199999));
#309885=CARTESIAN_POINT('Ctrl Pts',(-3.83031501700006,5.2,1.20823705199999));
#309886=CARTESIAN_POINT('Ctrl Pts',(-3.83031501700006,2.2,1.20823705199999));
#309887=CARTESIAN_POINT('Ctrl Pts',(-3.83085772700006,12.2,1.20834629099999));
#309888=CARTESIAN_POINT('Ctrl Pts',(-3.83085772700006,5.2,1.20834629099999));
#309889=CARTESIAN_POINT('Ctrl Pts',(-3.83085772700006,2.2,1.20834629099999));
#309890=CARTESIAN_POINT('Ctrl Pts',(-3.83140674200006,12.2,1.20845605799999));
#309891=CARTESIAN_POINT('Ctrl Pts',(-3.83140674200006,5.2,1.20845605799999));
#309892=CARTESIAN_POINT('Ctrl Pts',(-3.83140674200006,2.2,1.20845605799999));
#309893=CARTESIAN_POINT('Ctrl Pts',(-3.83196205000006,12.2,1.20856634199999));
#309894=CARTESIAN_POINT('Ctrl Pts',(-3.83196205000006,5.2,1.20856634199999));
#309895=CARTESIAN_POINT('Ctrl Pts',(-3.83196205000006,2.2,1.20856634199999));
#309896=CARTESIAN_POINT('Ctrl Pts',(-3.83252364200006,12.2,1.20867711899999));
#309897=CARTESIAN_POINT('Ctrl Pts',(-3.83252364200006,5.2,1.20867711899999));
#309898=CARTESIAN_POINT('Ctrl Pts',(-3.83252364200006,2.2,1.20867711899999));
#309899=CARTESIAN_POINT('Ctrl Pts',(-3.83309151000006,12.2,1.20878837499999));
#309900=CARTESIAN_POINT('Ctrl Pts',(-3.83309151000006,5.2,1.20878837499999));
#309901=CARTESIAN_POINT('Ctrl Pts',(-3.83309151000006,2.2,1.20878837499999));
#309902=CARTESIAN_POINT('Ctrl Pts',(-3.83366564200006,12.2,1.20890009099998));
#309903=CARTESIAN_POINT('Ctrl Pts',(-3.83366564200006,5.2,1.20890009099998));
#309904=CARTESIAN_POINT('Ctrl Pts',(-3.83366564200006,2.2,1.20890009099998));
#309905=CARTESIAN_POINT('Ctrl Pts',(-3.83424602900006,12.2,1.20901224799999));
#309906=CARTESIAN_POINT('Ctrl Pts',(-3.83424602900006,5.2,1.20901224799999));
#309907=CARTESIAN_POINT('Ctrl Pts',(-3.83424602900006,2.2,1.20901224799999));
#309908=CARTESIAN_POINT('Ctrl Pts',(-3.83483266100006,12.2,1.20912483099998));
#309909=CARTESIAN_POINT('Ctrl Pts',(-3.83483266100006,5.2,1.20912483099998));
#309910=CARTESIAN_POINT('Ctrl Pts',(-3.83483266100006,2.2,1.20912483099998));
#309911=CARTESIAN_POINT('Ctrl Pts',(-3.83542552800006,12.2,1.20923782099998));
#309912=CARTESIAN_POINT('Ctrl Pts',(-3.83542552800006,5.2,1.20923782099998));
#309913=CARTESIAN_POINT('Ctrl Pts',(-3.83542552800006,2.2,1.20923782099998));
#309914=CARTESIAN_POINT('Ctrl Pts',(-3.83602461900006,12.2,1.20935119999999));
#309915=CARTESIAN_POINT('Ctrl Pts',(-3.83602461900006,5.2,1.20935119999999));
#309916=CARTESIAN_POINT('Ctrl Pts',(-3.83602461900006,2.2,1.20935119999999));
#309917=CARTESIAN_POINT('Ctrl Pts',(-3.83662992800006,12.2,1.20946494999998));
#309918=CARTESIAN_POINT('Ctrl Pts',(-3.83662992800006,5.2,1.20946494999998));
#309919=CARTESIAN_POINT('Ctrl Pts',(-3.83662992800006,2.2,1.20946494999998));
#309920=CARTESIAN_POINT('Ctrl Pts',(-3.83724144100006,12.2,1.20957905399999));
#309921=CARTESIAN_POINT('Ctrl Pts',(-3.83724144100006,5.2,1.20957905399999));
#309922=CARTESIAN_POINT('Ctrl Pts',(-3.83724144100006,2.2,1.20957905399999));
#309923=CARTESIAN_POINT('Ctrl Pts',(-3.83785915100006,12.2,1.20969349699998));
#309924=CARTESIAN_POINT('Ctrl Pts',(-3.83785915100006,5.2,1.20969349699998));
#309925=CARTESIAN_POINT('Ctrl Pts',(-3.83785915100006,2.2,1.20969349699998));
#309926=CARTESIAN_POINT('Ctrl Pts',(-3.83848304800006,12.2,1.20980825899998));
#309927=CARTESIAN_POINT('Ctrl Pts',(-3.83848304800006,5.2,1.20980825899998));
#309928=CARTESIAN_POINT('Ctrl Pts',(-3.83848304800006,2.2,1.20980825899998));
#309929=CARTESIAN_POINT('Ctrl Pts',(-3.83911312000006,12.2,1.20992332299998));
#309930=CARTESIAN_POINT('Ctrl Pts',(-3.83911312000006,5.2,1.20992332299998));
#309931=CARTESIAN_POINT('Ctrl Pts',(-3.83911312000006,2.2,1.20992332299998));
#309932=CARTESIAN_POINT('Ctrl Pts',(-3.83974936000006,12.2,1.21003867299999));
#309933=CARTESIAN_POINT('Ctrl Pts',(-3.83974936000006,5.2,1.21003867299999));
#309934=CARTESIAN_POINT('Ctrl Pts',(-3.83974936000006,2.2,1.21003867299999));
#309935=CARTESIAN_POINT('Ctrl Pts',(-3.84039175700006,12.2,1.21015429099999));
#309936=CARTESIAN_POINT('Ctrl Pts',(-3.84039175700006,5.2,1.21015429099999));
#309937=CARTESIAN_POINT('Ctrl Pts',(-3.84039175700006,2.2,1.21015429099999));
#309938=CARTESIAN_POINT('Ctrl Pts',(-3.84104030200006,12.2,1.21027015999998));
#309939=CARTESIAN_POINT('Ctrl Pts',(-3.84104030200006,5.2,1.21027015999998));
#309940=CARTESIAN_POINT('Ctrl Pts',(-3.84104030200006,2.2,1.21027015999998));
#309941=CARTESIAN_POINT('Ctrl Pts',(-3.84169498400006,12.2,1.21038626399999));
#309942=CARTESIAN_POINT('Ctrl Pts',(-3.84169498400006,5.2,1.21038626399999));
#309943=CARTESIAN_POINT('Ctrl Pts',(-3.84169498400006,2.2,1.21038626399999));
#309944=CARTESIAN_POINT('Ctrl Pts',(-3.84235579300006,12.2,1.21050258499999));
#309945=CARTESIAN_POINT('Ctrl Pts',(-3.84235579300006,5.2,1.21050258499999));
#309946=CARTESIAN_POINT('Ctrl Pts',(-3.84235579300006,2.2,1.21050258499999));
#309947=CARTESIAN_POINT('Ctrl Pts',(-3.84302272200006,12.2,1.21061910599999));
#309948=CARTESIAN_POINT('Ctrl Pts',(-3.84302272200006,5.2,1.21061910599999));
#309949=CARTESIAN_POINT('Ctrl Pts',(-3.84302272200006,2.2,1.21061910599999));
#309950=CARTESIAN_POINT('Ctrl Pts',(-3.84369575800006,12.2,1.21073581099999));
#309951=CARTESIAN_POINT('Ctrl Pts',(-3.84369575800006,5.2,1.21073581099999));
#309952=CARTESIAN_POINT('Ctrl Pts',(-3.84369575800006,2.2,1.21073581099999));
#309953=CARTESIAN_POINT('Ctrl Pts',(-3.84437489400006,12.2,1.21085268299999));
#309954=CARTESIAN_POINT('Ctrl Pts',(-3.84437489400006,5.2,1.21085268299999));
#309955=CARTESIAN_POINT('Ctrl Pts',(-3.84437489400006,2.2,1.21085268299999));
#309956=CARTESIAN_POINT('Ctrl Pts',(-3.84506011900006,12.2,1.21096970499998));
#309957=CARTESIAN_POINT('Ctrl Pts',(-3.84506011900006,5.2,1.21096970499998));
#309958=CARTESIAN_POINT('Ctrl Pts',(-3.84506011900006,2.2,1.21096970499998));
#309959=CARTESIAN_POINT('Ctrl Pts',(-3.84575142300006,12.2,1.21108685999999));
#309960=CARTESIAN_POINT('Ctrl Pts',(-3.84575142300006,5.2,1.21108685999999));
#309961=CARTESIAN_POINT('Ctrl Pts',(-3.84575142300006,2.2,1.21108685999999));
#309962=CARTESIAN_POINT('Ctrl Pts',(-3.84644879800006,12.2,1.21120413299999));
#309963=CARTESIAN_POINT('Ctrl Pts',(-3.84644879800006,5.2,1.21120413299999));
#309964=CARTESIAN_POINT('Ctrl Pts',(-3.84644879800006,2.2,1.21120413299999));
#309965=CARTESIAN_POINT('Ctrl Pts',(-3.84715223200006,12.2,1.21132150599998));
#309966=CARTESIAN_POINT('Ctrl Pts',(-3.84715223200006,5.2,1.21132150599998));
#309967=CARTESIAN_POINT('Ctrl Pts',(-3.84715223200006,2.2,1.21132150599998));
#309968=CARTESIAN_POINT('Ctrl Pts',(-3.84786171700005,12.2,1.21143896399999));
#309969=CARTESIAN_POINT('Ctrl Pts',(-3.84786171700005,5.2,1.21143896399999));
#309970=CARTESIAN_POINT('Ctrl Pts',(-3.84786171700005,2.2,1.21143896399999));
#309971=CARTESIAN_POINT('Ctrl Pts',(-3.84857724200006,12.2,1.21155648899999));
#309972=CARTESIAN_POINT('Ctrl Pts',(-3.84857724200006,5.2,1.21155648899999));
#309973=CARTESIAN_POINT('Ctrl Pts',(-3.84857724200006,2.2,1.21155648899999));
#309974=CARTESIAN_POINT('Ctrl Pts',(-3.84929880000006,12.2,1.21167406499998));
#309975=CARTESIAN_POINT('Ctrl Pts',(-3.84929880000006,5.2,1.21167406499998));
#309976=CARTESIAN_POINT('Ctrl Pts',(-3.84929880000006,2.2,1.21167406499998));
#309977=CARTESIAN_POINT('Ctrl Pts',(-3.85002637800006,12.2,1.21179167599998));
#309978=CARTESIAN_POINT('Ctrl Pts',(-3.85002637800006,5.2,1.21179167599998));
#309979=CARTESIAN_POINT('Ctrl Pts',(-3.85002637800006,2.2,1.21179167599998));
#309980=CARTESIAN_POINT('Ctrl Pts',(-3.85075996900006,12.2,1.21190930699999));
#309981=CARTESIAN_POINT('Ctrl Pts',(-3.85075996900006,5.2,1.21190930699999));
#309982=CARTESIAN_POINT('Ctrl Pts',(-3.85075996900006,2.2,1.21190930699999));
#309983=CARTESIAN_POINT('Ctrl Pts',(-3.85149956200006,12.2,1.21202693899999));
#309984=CARTESIAN_POINT('Ctrl Pts',(-3.85149956200006,5.2,1.21202693899999));
#309985=CARTESIAN_POINT('Ctrl Pts',(-3.85149956200006,2.2,1.21202693899999));
#309986=CARTESIAN_POINT('Ctrl Pts',(-3.85224514800006,12.2,1.21214455899999));
#309987=CARTESIAN_POINT('Ctrl Pts',(-3.85224514800006,5.2,1.21214455899999));
#309988=CARTESIAN_POINT('Ctrl Pts',(-3.85224514800006,2.2,1.21214455899999));
#309989=CARTESIAN_POINT('Ctrl Pts',(-3.85299671700006,12.2,1.21226214899998));
#309990=CARTESIAN_POINT('Ctrl Pts',(-3.85299671700006,5.2,1.21226214899998));
#309991=CARTESIAN_POINT('Ctrl Pts',(-3.85299671700006,2.2,1.21226214899998));
#309992=CARTESIAN_POINT('Ctrl Pts',(-3.85375426000006,12.2,1.21237969399999));
#309993=CARTESIAN_POINT('Ctrl Pts',(-3.85375426000006,5.2,1.21237969399999));
#309994=CARTESIAN_POINT('Ctrl Pts',(-3.85375426000006,2.2,1.21237969399999));
#309995=CARTESIAN_POINT('Ctrl Pts',(-3.85451776700005,12.2,1.21249717699999));
#309996=CARTESIAN_POINT('Ctrl Pts',(-3.85451776700005,5.2,1.21249717699999));
#309997=CARTESIAN_POINT('Ctrl Pts',(-3.85451776700005,2.2,1.21249717699999));
#309998=CARTESIAN_POINT('Ctrl Pts',(-3.85528722900006,12.2,1.21261458399998));
#309999=CARTESIAN_POINT('Ctrl Pts',(-3.85528722900006,5.2,1.21261458399998));
#310000=CARTESIAN_POINT('Ctrl Pts',(-3.85528722900006,2.2,1.21261458399998));
#310001=CARTESIAN_POINT('Ctrl Pts',(-3.85606263500006,12.2,1.21273189699998));
#310002=CARTESIAN_POINT('Ctrl Pts',(-3.85606263500006,5.2,1.21273189699998));
#310003=CARTESIAN_POINT('Ctrl Pts',(-3.85606263500006,2.2,1.21273189699998));
#310004=CARTESIAN_POINT('Ctrl Pts',(-3.85684397700006,12.2,1.21284910099998));
#310005=CARTESIAN_POINT('Ctrl Pts',(-3.85684397700006,5.2,1.21284910099998));
#310006=CARTESIAN_POINT('Ctrl Pts',(-3.85684397700006,2.2,1.21284910099998));
#310007=CARTESIAN_POINT('Ctrl Pts',(-3.85763124500006,12.2,1.21296618199999));
#310008=CARTESIAN_POINT('Ctrl Pts',(-3.85763124500006,5.2,1.21296618199999));
#310009=CARTESIAN_POINT('Ctrl Pts',(-3.85763124500006,2.2,1.21296618199999));
#310010=CARTESIAN_POINT('Ctrl Pts',(-3.85842442800006,12.2,1.21308312099998));
#310011=CARTESIAN_POINT('Ctrl Pts',(-3.85842442800006,5.2,1.21308312099998));
#310012=CARTESIAN_POINT('Ctrl Pts',(-3.85842442800006,2.2,1.21308312099998));
#310013=CARTESIAN_POINT('Ctrl Pts',(-3.85922351900006,12.2,1.21319990499998));
#310014=CARTESIAN_POINT('Ctrl Pts',(-3.85922351900006,5.2,1.21319990499998));
#310015=CARTESIAN_POINT('Ctrl Pts',(-3.85922351900006,2.2,1.21319990499998));
#310016=CARTESIAN_POINT('Ctrl Pts',(-3.86002850600006,12.2,1.21331651799998));
#310017=CARTESIAN_POINT('Ctrl Pts',(-3.86002850600006,5.2,1.21331651799998));
#310018=CARTESIAN_POINT('Ctrl Pts',(-3.86002850600006,2.2,1.21331651799998));
#310019=CARTESIAN_POINT('Ctrl Pts',(-3.86083938100006,12.2,1.21343294399999));
#310020=CARTESIAN_POINT('Ctrl Pts',(-3.86083938100006,5.2,1.21343294399999));
#310021=CARTESIAN_POINT('Ctrl Pts',(-3.86083938100006,2.2,1.21343294399999));
#310022=CARTESIAN_POINT('Ctrl Pts',(-3.86165613400006,12.2,1.21354916799998));
#310023=CARTESIAN_POINT('Ctrl Pts',(-3.86165613400006,5.2,1.21354916799998));
#310024=CARTESIAN_POINT('Ctrl Pts',(-3.86165613400006,2.2,1.21354916799998));
#310025=CARTESIAN_POINT('Ctrl Pts',(-3.86247875600006,12.2,1.21366517399998));
#310026=CARTESIAN_POINT('Ctrl Pts',(-3.86247875600006,5.2,1.21366517399998));
#310027=CARTESIAN_POINT('Ctrl Pts',(-3.86247875600006,2.2,1.21366517399998));
#310028=CARTESIAN_POINT('Ctrl Pts',(-3.86330723700006,12.2,1.21378094699998));
#310029=CARTESIAN_POINT('Ctrl Pts',(-3.86330723700006,5.2,1.21378094699998));
#310030=CARTESIAN_POINT('Ctrl Pts',(-3.86330723700006,2.2,1.21378094699998));
#310031=CARTESIAN_POINT('Ctrl Pts',(-3.86414156800006,12.2,1.21389647099999));
#310032=CARTESIAN_POINT('Ctrl Pts',(-3.86414156800006,5.2,1.21389647099999));
#310033=CARTESIAN_POINT('Ctrl Pts',(-3.86414156800006,2.2,1.21389647099999));
#310034=CARTESIAN_POINT('Ctrl Pts',(-3.86498173800006,12.2,1.21401173299999));
#310035=CARTESIAN_POINT('Ctrl Pts',(-3.86498173800006,5.2,1.21401173299999));
#310036=CARTESIAN_POINT('Ctrl Pts',(-3.86498173800006,2.2,1.21401173299999));
#310037=CARTESIAN_POINT('Ctrl Pts',(-3.86582774000006,12.2,1.21412671599999));
#310038=CARTESIAN_POINT('Ctrl Pts',(-3.86582774000006,5.2,1.21412671599999));
#310039=CARTESIAN_POINT('Ctrl Pts',(-3.86582774000006,2.2,1.21412671599999));
#310040=CARTESIAN_POINT('Ctrl Pts',(-3.86667956300006,12.2,1.21424140599999));
#310041=CARTESIAN_POINT('Ctrl Pts',(-3.86667956300006,5.2,1.21424140599999));
#310042=CARTESIAN_POINT('Ctrl Pts',(-3.86667956300006,2.2,1.21424140599999));
#310043=CARTESIAN_POINT('Ctrl Pts',(-3.86753719600006,12.2,1.21435578599999));
#310044=CARTESIAN_POINT('Ctrl Pts',(-3.86753719600006,5.2,1.21435578599999));
#310045=CARTESIAN_POINT('Ctrl Pts',(-3.86753719600006,2.2,1.21435578599999));
#310046=CARTESIAN_POINT('Ctrl Pts',(-3.86840063300006,12.2,1.21446984299999));
#310047=CARTESIAN_POINT('Ctrl Pts',(-3.86840063300006,5.2,1.21446984299999));
#310048=CARTESIAN_POINT('Ctrl Pts',(-3.86840063300006,2.2,1.21446984299999));
#310049=CARTESIAN_POINT('Ctrl Pts',(-3.86926986200006,12.2,1.21458356099998));
#310050=CARTESIAN_POINT('Ctrl Pts',(-3.86926986200006,5.2,1.21458356099998));
#310051=CARTESIAN_POINT('Ctrl Pts',(-3.86926986200006,2.2,1.21458356099998));
#310052=CARTESIAN_POINT('Ctrl Pts',(-3.87014487400006,12.2,1.21469692599999));
#310053=CARTESIAN_POINT('Ctrl Pts',(-3.87014487400006,5.2,1.21469692599999));
#310054=CARTESIAN_POINT('Ctrl Pts',(-3.87014487400006,2.2,1.21469692599999));
#310055=CARTESIAN_POINT('Ctrl Pts',(-3.87102566100006,12.2,1.21480992199999));
#310056=CARTESIAN_POINT('Ctrl Pts',(-3.87102566100006,5.2,1.21480992199999));
#310057=CARTESIAN_POINT('Ctrl Pts',(-3.87102566100006,2.2,1.21480992199999));
#310058=CARTESIAN_POINT('Ctrl Pts',(-3.87191221100006,12.2,1.21492253399999));
#310059=CARTESIAN_POINT('Ctrl Pts',(-3.87191221100006,5.2,1.21492253399999));
#310060=CARTESIAN_POINT('Ctrl Pts',(-3.87191221100006,2.2,1.21492253399999));
#310061=CARTESIAN_POINT('Ctrl Pts',(-3.87280451700006,12.2,1.21503474899999));
#310062=CARTESIAN_POINT('Ctrl Pts',(-3.87280451700006,5.2,1.21503474899999));
#310063=CARTESIAN_POINT('Ctrl Pts',(-3.87280451700006,2.2,1.21503474899999));
#310064=CARTESIAN_POINT('Ctrl Pts',(-3.87370256800006,12.2,1.21514654999999));
#310065=CARTESIAN_POINT('Ctrl Pts',(-3.87370256800006,5.2,1.21514654999999));
#310066=CARTESIAN_POINT('Ctrl Pts',(-3.87370256800006,2.2,1.21514654999999));
#310067=CARTESIAN_POINT('Ctrl Pts',(-3.87460635500006,12.2,1.21525792399999));
#310068=CARTESIAN_POINT('Ctrl Pts',(-3.87460635500006,5.2,1.21525792399999));
#310069=CARTESIAN_POINT('Ctrl Pts',(-3.87460635500006,2.2,1.21525792399999));
#310070=CARTESIAN_POINT('Ctrl Pts',(-3.87551586900006,12.2,1.21536885699999));
#310071=CARTESIAN_POINT('Ctrl Pts',(-3.87551586900006,5.2,1.21536885699999));
#310072=CARTESIAN_POINT('Ctrl Pts',(-3.87551586900006,2.2,1.21536885699999));
#310073=CARTESIAN_POINT('Ctrl Pts',(-3.87643110100006,12.2,1.21547933299999));
#310074=CARTESIAN_POINT('Ctrl Pts',(-3.87643110100006,5.2,1.21547933299999));
#310075=CARTESIAN_POINT('Ctrl Pts',(-3.87643110100006,2.2,1.21547933299999));
#310076=CARTESIAN_POINT('Ctrl Pts',(-3.87735204000006,12.2,1.21558933699998));
#310077=CARTESIAN_POINT('Ctrl Pts',(-3.87735204000006,5.2,1.21558933699998));
#310078=CARTESIAN_POINT('Ctrl Pts',(-3.87735204000006,2.2,1.21558933699998));
#310079=CARTESIAN_POINT('Ctrl Pts',(-3.87827867800006,12.2,1.21569885599999));
#310080=CARTESIAN_POINT('Ctrl Pts',(-3.87827867800006,5.2,1.21569885599999));
#310081=CARTESIAN_POINT('Ctrl Pts',(-3.87827867800006,2.2,1.21569885599999));
#310082=CARTESIAN_POINT('Ctrl Pts',(-3.87921100400006,12.2,1.21580787499999));
#310083=CARTESIAN_POINT('Ctrl Pts',(-3.87921100400006,5.2,1.21580787499999));
#310084=CARTESIAN_POINT('Ctrl Pts',(-3.87921100400006,2.2,1.21580787499999));
#310085=CARTESIAN_POINT('Ctrl Pts',(-3.88014901100005,12.2,1.21591637999999));
#310086=CARTESIAN_POINT('Ctrl Pts',(-3.88014901100005,5.2,1.21591637999999));
#310087=CARTESIAN_POINT('Ctrl Pts',(-3.88014901100005,2.2,1.21591637999999));
#310088=CARTESIAN_POINT('Ctrl Pts',(-3.88109268800005,12.2,1.21602435599999));
#310089=CARTESIAN_POINT('Ctrl Pts',(-3.88109268800005,5.2,1.21602435599999));
#310090=CARTESIAN_POINT('Ctrl Pts',(-3.88109268800005,2.2,1.21602435599999));
#310091=CARTESIAN_POINT('Ctrl Pts',(-3.88204202600006,12.2,1.21613178899999));
#310092=CARTESIAN_POINT('Ctrl Pts',(-3.88204202600006,5.2,1.21613178899999));
#310093=CARTESIAN_POINT('Ctrl Pts',(-3.88204202600006,2.2,1.21613178899999));
#310094=CARTESIAN_POINT('Ctrl Pts',(-3.88299701500006,12.2,1.21623866599998));
#310095=CARTESIAN_POINT('Ctrl Pts',(-3.88299701500006,5.2,1.21623866599998));
#310096=CARTESIAN_POINT('Ctrl Pts',(-3.88299701500006,2.2,1.21623866599998));
#310097=CARTESIAN_POINT('Ctrl Pts',(-3.88395764700006,12.2,1.21634497099999));
#310098=CARTESIAN_POINT('Ctrl Pts',(-3.88395764700006,5.2,1.21634497099999));
#310099=CARTESIAN_POINT('Ctrl Pts',(-3.88395764700006,2.2,1.21634497099999));
#310100=CARTESIAN_POINT('Ctrl Pts',(-3.88492391200006,12.2,1.21645068999999));
#310101=CARTESIAN_POINT('Ctrl Pts',(-3.88492391200006,5.2,1.21645068999999));
#310102=CARTESIAN_POINT('Ctrl Pts',(-3.88492391200006,2.2,1.21645068999999));
#310103=CARTESIAN_POINT('Ctrl Pts',(-3.88589580000006,12.2,1.21655580999999));
#310104=CARTESIAN_POINT('Ctrl Pts',(-3.88589580000006,5.2,1.21655580999999));
#310105=CARTESIAN_POINT('Ctrl Pts',(-3.88589580000006,2.2,1.21655580999999));
#310106=CARTESIAN_POINT('Ctrl Pts',(-3.88687330200006,12.2,1.21666031799998));
#310107=CARTESIAN_POINT('Ctrl Pts',(-3.88687330200006,5.2,1.21666031799998));
#310108=CARTESIAN_POINT('Ctrl Pts',(-3.88687330200006,2.2,1.21666031799998));
#310109=CARTESIAN_POINT('Ctrl Pts',(-3.88785641000006,12.2,1.21676419699998));
#310110=CARTESIAN_POINT('Ctrl Pts',(-3.88785641000006,5.2,1.21676419699998));
#310111=CARTESIAN_POINT('Ctrl Pts',(-3.88785641000006,2.2,1.21676419699998));
#310112=CARTESIAN_POINT('Ctrl Pts',(-3.88884511400006,12.2,1.21686743499998));
#310113=CARTESIAN_POINT('Ctrl Pts',(-3.88884511400006,5.2,1.21686743499998));
#310114=CARTESIAN_POINT('Ctrl Pts',(-3.88884511400006,2.2,1.21686743499998));
#310115=CARTESIAN_POINT('Ctrl Pts',(-3.88983940300006,12.2,1.21697001799999));
#310116=CARTESIAN_POINT('Ctrl Pts',(-3.88983940300006,5.2,1.21697001799999));
#310117=CARTESIAN_POINT('Ctrl Pts',(-3.88983940300006,2.2,1.21697001799999));
#310118=CARTESIAN_POINT('Ctrl Pts',(-3.89083926900006,12.2,1.21707193199999));
#310119=CARTESIAN_POINT('Ctrl Pts',(-3.89083926900006,5.2,1.21707193199999));
#310120=CARTESIAN_POINT('Ctrl Pts',(-3.89083926900006,2.2,1.21707193199999));
#310121=CARTESIAN_POINT('Ctrl Pts',(-3.89184470200005,12.2,1.21717316299998));
#310122=CARTESIAN_POINT('Ctrl Pts',(-3.89184470200005,5.2,1.21717316299998));
#310123=CARTESIAN_POINT('Ctrl Pts',(-3.89184470200005,2.2,1.21717316299998));
#310124=CARTESIAN_POINT('Ctrl Pts',(-3.89285569500006,12.2,1.21727369699999));
#310125=CARTESIAN_POINT('Ctrl Pts',(-3.89285569500006,5.2,1.21727369699999));
#310126=CARTESIAN_POINT('Ctrl Pts',(-3.89285569500006,2.2,1.21727369699999));
#310127=CARTESIAN_POINT('Ctrl Pts',(-3.89387223600006,12.2,1.21737352099998));
#310128=CARTESIAN_POINT('Ctrl Pts',(-3.89387223600006,5.2,1.21737352099998));
#310129=CARTESIAN_POINT('Ctrl Pts',(-3.89387223600006,2.2,1.21737352099998));
#310130=CARTESIAN_POINT('Ctrl Pts',(-3.89489431600006,12.2,1.21747262099999));
#310131=CARTESIAN_POINT('Ctrl Pts',(-3.89489431600006,5.2,1.21747262099999));
#310132=CARTESIAN_POINT('Ctrl Pts',(-3.89489431600006,2.2,1.21747262099999));
#310133=CARTESIAN_POINT('Ctrl Pts',(-3.89592192800006,12.2,1.21757098399998));
#310134=CARTESIAN_POINT('Ctrl Pts',(-3.89592192800006,5.2,1.21757098399998));
#310135=CARTESIAN_POINT('Ctrl Pts',(-3.89592192800006,2.2,1.21757098399998));
#310136=CARTESIAN_POINT('Ctrl Pts',(-3.89695506000006,12.2,1.21766859599999));
#310137=CARTESIAN_POINT('Ctrl Pts',(-3.89695506000006,5.2,1.21766859599999));
#310138=CARTESIAN_POINT('Ctrl Pts',(-3.89695506000006,2.2,1.21766859599999));
#310139=CARTESIAN_POINT('Ctrl Pts',(-3.89799370500006,12.2,1.21776544299999));
#310140=CARTESIAN_POINT('Ctrl Pts',(-3.89799370500006,5.2,1.21776544299999));
#310141=CARTESIAN_POINT('Ctrl Pts',(-3.89799370500006,2.2,1.21776544299999));
#310142=CARTESIAN_POINT('Ctrl Pts',(-3.89903785100006,12.2,1.21786151199998));
#310143=CARTESIAN_POINT('Ctrl Pts',(-3.89903785100006,5.2,1.21786151199998));
#310144=CARTESIAN_POINT('Ctrl Pts',(-3.89903785100006,2.2,1.21786151199998));
#310145=CARTESIAN_POINT('Ctrl Pts',(-3.90008749200006,12.2,1.21795678899999));
#310146=CARTESIAN_POINT('Ctrl Pts',(-3.90008749200006,5.2,1.21795678899999));
#310147=CARTESIAN_POINT('Ctrl Pts',(-3.90008749200006,2.2,1.21795678899999));
#310148=CARTESIAN_POINT('Ctrl Pts',(-3.90114261600006,12.2,1.21805126199999));
#310149=CARTESIAN_POINT('Ctrl Pts',(-3.90114261600006,5.2,1.21805126199999));
#310150=CARTESIAN_POINT('Ctrl Pts',(-3.90114261600006,2.2,1.21805126199999));
#310151=CARTESIAN_POINT('Ctrl Pts',(-3.90220321500006,12.2,1.21814491699999));
#310152=CARTESIAN_POINT('Ctrl Pts',(-3.90220321500006,5.2,1.21814491699999));
#310153=CARTESIAN_POINT('Ctrl Pts',(-3.90220321500006,2.2,1.21814491699999));
#310154=CARTESIAN_POINT('Ctrl Pts',(-3.90326928000006,12.2,1.21823773999999));
#310155=CARTESIAN_POINT('Ctrl Pts',(-3.90326928000006,5.2,1.21823773999999));
#310156=CARTESIAN_POINT('Ctrl Pts',(-3.90326928000006,2.2,1.21823773999999));
#310157=CARTESIAN_POINT('Ctrl Pts',(-3.90434080200006,12.2,1.21832971899998));
#310158=CARTESIAN_POINT('Ctrl Pts',(-3.90434080200006,5.2,1.21832971899998));
#310159=CARTESIAN_POINT('Ctrl Pts',(-3.90434080200006,2.2,1.21832971899998));
#310160=CARTESIAN_POINT('Ctrl Pts',(-3.90541777000006,12.2,1.21842083999999));
#310161=CARTESIAN_POINT('Ctrl Pts',(-3.90541777000006,5.2,1.21842083999999));
#310162=CARTESIAN_POINT('Ctrl Pts',(-3.90541777000006,2.2,1.21842083999999));
#310163=CARTESIAN_POINT('Ctrl Pts',(-3.90650017600006,12.2,1.21851108999998));
#310164=CARTESIAN_POINT('Ctrl Pts',(-3.90650017600006,5.2,1.21851108999998));
#310165=CARTESIAN_POINT('Ctrl Pts',(-3.90650017600006,2.2,1.21851108999998));
#310166=CARTESIAN_POINT('Ctrl Pts',(-3.90758801000006,12.2,1.21860045499998));
#310167=CARTESIAN_POINT('Ctrl Pts',(-3.90758801000006,5.2,1.21860045499998));
#310168=CARTESIAN_POINT('Ctrl Pts',(-3.90758801000006,2.2,1.21860045499998));
#310169=CARTESIAN_POINT('Ctrl Pts',(-3.90868126500005,12.2,1.21868892299998));
#310170=CARTESIAN_POINT('Ctrl Pts',(-3.90868126500005,5.2,1.21868892299998));
#310171=CARTESIAN_POINT('Ctrl Pts',(-3.90868126500005,2.2,1.21868892299998));
#310172=CARTESIAN_POINT('Ctrl Pts',(-3.90977993000006,12.2,1.21877648099999));
#310173=CARTESIAN_POINT('Ctrl Pts',(-3.90977993000006,5.2,1.21877648099999));
#310174=CARTESIAN_POINT('Ctrl Pts',(-3.90977993000006,2.2,1.21877648099999));
#310175=CARTESIAN_POINT('Ctrl Pts',(-3.91088399500005,12.2,1.21886311599999));
#310176=CARTESIAN_POINT('Ctrl Pts',(-3.91088399500005,5.2,1.21886311599999));
#310177=CARTESIAN_POINT('Ctrl Pts',(-3.91088399500005,2.2,1.21886311599999));
#310178=CARTESIAN_POINT('Ctrl Pts',(-3.91199345200006,12.2,1.21894881599999));
#310179=CARTESIAN_POINT('Ctrl Pts',(-3.91199345200006,5.2,1.21894881599999));
#310180=CARTESIAN_POINT('Ctrl Pts',(-3.91199345200006,2.2,1.21894881599999));
#310181=CARTESIAN_POINT('Ctrl Pts',(-3.91310829200005,12.2,1.21903356499999));
#310182=CARTESIAN_POINT('Ctrl Pts',(-3.91310829200005,5.2,1.21903356499999));
#310183=CARTESIAN_POINT('Ctrl Pts',(-3.91310829200005,2.2,1.21903356499999));
#310184=CARTESIAN_POINT('Ctrl Pts',(-3.91422850500006,12.2,1.21911735199999));
#310185=CARTESIAN_POINT('Ctrl Pts',(-3.91422850500006,5.2,1.21911735199999));
#310186=CARTESIAN_POINT('Ctrl Pts',(-3.91422850500006,2.2,1.21911735199999));
#310187=CARTESIAN_POINT('Ctrl Pts',(-3.91535408400006,12.2,1.21920016599999));
#310188=CARTESIAN_POINT('Ctrl Pts',(-3.91535408400006,5.2,1.21920016599999));
#310189=CARTESIAN_POINT('Ctrl Pts',(-3.91535408400006,2.2,1.21920016599999));
#310190=CARTESIAN_POINT('Ctrl Pts',(-3.91648501700006,12.2,1.21928199199999));
#310191=CARTESIAN_POINT('Ctrl Pts',(-3.91648501700006,5.2,1.21928199199999));
#310192=CARTESIAN_POINT('Ctrl Pts',(-3.91648501700006,2.2,1.21928199199999));
#310193=CARTESIAN_POINT('Ctrl Pts',(-3.91762129500006,12.2,1.21936281799998));
#310194=CARTESIAN_POINT('Ctrl Pts',(-3.91762129500006,5.2,1.21936281799998));
#310195=CARTESIAN_POINT('Ctrl Pts',(-3.91762129500006,2.2,1.21936281799998));
#310196=CARTESIAN_POINT('Ctrl Pts',(-3.91876291000006,12.2,1.21944262999999));
#310197=CARTESIAN_POINT('Ctrl Pts',(-3.91876291000006,5.2,1.21944262999999));
#310198=CARTESIAN_POINT('Ctrl Pts',(-3.91876291000006,2.2,1.21944262999999));
#310199=CARTESIAN_POINT('Ctrl Pts',(-3.91990985300006,12.2,1.21952141699999));
#310200=CARTESIAN_POINT('Ctrl Pts',(-3.91990985300006,5.2,1.21952141699999));
#310201=CARTESIAN_POINT('Ctrl Pts',(-3.91990985300006,2.2,1.21952141699999));
#310202=CARTESIAN_POINT('Ctrl Pts',(-3.92106211500006,12.2,1.21959916599998));
#310203=CARTESIAN_POINT('Ctrl Pts',(-3.92106211500006,5.2,1.21959916599998));
#310204=CARTESIAN_POINT('Ctrl Pts',(-3.92106211500006,2.2,1.21959916599998));
#310205=CARTESIAN_POINT('Ctrl Pts',(-3.92221968500006,12.2,1.21967586499999));
#310206=CARTESIAN_POINT('Ctrl Pts',(-3.92221968500006,5.2,1.21967586499999));
#310207=CARTESIAN_POINT('Ctrl Pts',(-3.92221968500006,2.2,1.21967586499999));
#310208=CARTESIAN_POINT('Ctrl Pts',(-3.92338255600006,12.2,1.21975150099999));
#310209=CARTESIAN_POINT('Ctrl Pts',(-3.92338255600006,5.2,1.21975150099999));
#310210=CARTESIAN_POINT('Ctrl Pts',(-3.92338255600006,2.2,1.21975150099999));
#310211=CARTESIAN_POINT('Ctrl Pts',(-3.92455071700006,12.2,1.21982605999999));
#310212=CARTESIAN_POINT('Ctrl Pts',(-3.92455071700006,5.2,1.21982605999999));
#310213=CARTESIAN_POINT('Ctrl Pts',(-3.92455071700006,2.2,1.21982605999999));
#310214=CARTESIAN_POINT('Ctrl Pts',(-3.92572416100006,12.2,1.21989953199999));
#310215=CARTESIAN_POINT('Ctrl Pts',(-3.92572416100006,5.2,1.21989953199999));
#310216=CARTESIAN_POINT('Ctrl Pts',(-3.92572416100006,2.2,1.21989953199999));
#310217=CARTESIAN_POINT('Ctrl Pts',(-3.92690287700006,12.2,1.21997190299998));
#310218=CARTESIAN_POINT('Ctrl Pts',(-3.92690287700006,5.2,1.21997190299998));
#310219=CARTESIAN_POINT('Ctrl Pts',(-3.92690287700006,2.2,1.21997190299998));
#310220=CARTESIAN_POINT('Ctrl Pts',(-3.92808685700006,12.2,1.22004316099999));
#310221=CARTESIAN_POINT('Ctrl Pts',(-3.92808685700006,5.2,1.22004316099999));
#310222=CARTESIAN_POINT('Ctrl Pts',(-3.92808685700006,2.2,1.22004316099999));
#310223=CARTESIAN_POINT('Ctrl Pts',(-3.92927609100005,12.2,1.22011329499998));
#310224=CARTESIAN_POINT('Ctrl Pts',(-3.92927609100005,5.2,1.22011329499998));
#310225=CARTESIAN_POINT('Ctrl Pts',(-3.92927609100005,2.2,1.22011329499998));
#310226=CARTESIAN_POINT('Ctrl Pts',(-3.93047057000006,12.2,1.22018229099998));
#310227=CARTESIAN_POINT('Ctrl Pts',(-3.93047057000006,5.2,1.22018229099998));
#310228=CARTESIAN_POINT('Ctrl Pts',(-3.93047057000006,2.2,1.22018229099998));
#310229=CARTESIAN_POINT('Ctrl Pts',(-3.93167028600006,12.2,1.22025013799998));
#310230=CARTESIAN_POINT('Ctrl Pts',(-3.93167028600006,5.2,1.22025013799998));
#310231=CARTESIAN_POINT('Ctrl Pts',(-3.93167028600006,2.2,1.22025013799998));
#310232=CARTESIAN_POINT('Ctrl Pts',(-3.93287522900006,12.2,1.22031682099998));
#310233=CARTESIAN_POINT('Ctrl Pts',(-3.93287522900006,5.2,1.22031682099998));
#310234=CARTESIAN_POINT('Ctrl Pts',(-3.93287522900006,2.2,1.22031682099998));
#310235=CARTESIAN_POINT('Ctrl Pts',(-3.93408539000006,12.2,1.22038233299998));
#310236=CARTESIAN_POINT('Ctrl Pts',(-3.93408539000006,5.2,1.22038233299998));
#310237=CARTESIAN_POINT('Ctrl Pts',(-3.93408539000006,2.2,1.22038233299998));
#310238=CARTESIAN_POINT('Ctrl Pts',(-3.93530076000006,12.2,1.22044665699999));
#310239=CARTESIAN_POINT('Ctrl Pts',(-3.93530076000006,5.2,1.22044665699999));
#310240=CARTESIAN_POINT('Ctrl Pts',(-3.93530076000006,2.2,1.22044665699999));
#310241=CARTESIAN_POINT('Ctrl Pts',(-3.93652132800006,12.2,1.22050978299999));
#310242=CARTESIAN_POINT('Ctrl Pts',(-3.93652132800006,5.2,1.22050978299999));
#310243=CARTESIAN_POINT('Ctrl Pts',(-3.93652132800006,2.2,1.22050978299999));
#310244=CARTESIAN_POINT('Ctrl Pts',(-3.93774708800006,12.2,1.22057169899998));
#310245=CARTESIAN_POINT('Ctrl Pts',(-3.93774708800006,5.2,1.22057169899998));
#310246=CARTESIAN_POINT('Ctrl Pts',(-3.93774708800006,2.2,1.22057169899998));
#310247=CARTESIAN_POINT('Ctrl Pts',(-3.93897803100006,12.2,1.22063239299999));
#310248=CARTESIAN_POINT('Ctrl Pts',(-3.93897803100006,5.2,1.22063239299999));
#310249=CARTESIAN_POINT('Ctrl Pts',(-3.93897803100006,2.2,1.22063239299999));
#310250=CARTESIAN_POINT('Ctrl Pts',(-3.94021414500005,12.2,1.22069185299999));
#310251=CARTESIAN_POINT('Ctrl Pts',(-3.94021414500005,5.2,1.22069185299999));
#310252=CARTESIAN_POINT('Ctrl Pts',(-3.94021414500005,2.2,1.22069185299999));
#310253=CARTESIAN_POINT('Ctrl Pts',(-3.94145542300006,12.2,1.22075006699998));
#310254=CARTESIAN_POINT('Ctrl Pts',(-3.94145542300006,5.2,1.22075006699998));
#310255=CARTESIAN_POINT('Ctrl Pts',(-3.94145542300006,2.2,1.22075006699998));
#310256=CARTESIAN_POINT('Ctrl Pts',(-3.94270185600006,12.2,1.22080702299999));
#310257=CARTESIAN_POINT('Ctrl Pts',(-3.94270185600006,5.2,1.22080702299999));
#310258=CARTESIAN_POINT('Ctrl Pts',(-3.94270185600006,2.2,1.22080702299999));
#310259=CARTESIAN_POINT('Ctrl Pts',(-3.94395343300006,12.2,1.22086270899999));
#310260=CARTESIAN_POINT('Ctrl Pts',(-3.94395343300006,5.2,1.22086270899999));
#310261=CARTESIAN_POINT('Ctrl Pts',(-3.94395343300006,2.2,1.22086270899999));
#310262=CARTESIAN_POINT('Ctrl Pts',(-3.94521014800006,12.2,1.22091711399999));
#310263=CARTESIAN_POINT('Ctrl Pts',(-3.94521014800006,5.2,1.22091711399999));
#310264=CARTESIAN_POINT('Ctrl Pts',(-3.94521014800006,2.2,1.22091711399999));
#310265=CARTESIAN_POINT('Ctrl Pts',(-3.94647198800006,12.2,1.22097022499998));
#310266=CARTESIAN_POINT('Ctrl Pts',(-3.94647198800006,5.2,1.22097022499998));
#310267=CARTESIAN_POINT('Ctrl Pts',(-3.94647198800006,2.2,1.22097022499998));
#310268=CARTESIAN_POINT('Ctrl Pts',(-3.94773894800006,12.2,1.22102203099999));
#310269=CARTESIAN_POINT('Ctrl Pts',(-3.94773894800006,5.2,1.22102203099999));
#310270=CARTESIAN_POINT('Ctrl Pts',(-3.94773894800006,2.2,1.22102203099999));
#310271=CARTESIAN_POINT('Ctrl Pts',(-3.94901101700006,12.2,1.22107252099998));
#310272=CARTESIAN_POINT('Ctrl Pts',(-3.94901101700006,5.2,1.22107252099998));
#310273=CARTESIAN_POINT('Ctrl Pts',(-3.94901101700006,2.2,1.22107252099998));
#310274=CARTESIAN_POINT('Ctrl Pts',(-3.95028818600006,12.2,1.22112168199998));
#310275=CARTESIAN_POINT('Ctrl Pts',(-3.95028818600006,5.2,1.22112168199998));
#310276=CARTESIAN_POINT('Ctrl Pts',(-3.95028818600006,2.2,1.22112168199998));
#310277=CARTESIAN_POINT('Ctrl Pts',(-3.95157044600006,12.2,1.22116950299999));
#310278=CARTESIAN_POINT('Ctrl Pts',(-3.95157044600006,5.2,1.22116950299999));
#310279=CARTESIAN_POINT('Ctrl Pts',(-3.95157044600006,2.2,1.22116950299999));
#310280=CARTESIAN_POINT('Ctrl Pts',(-3.95285778800006,12.2,1.22121597299999));
#310281=CARTESIAN_POINT('Ctrl Pts',(-3.95285778800006,5.2,1.22121597299999));
#310282=CARTESIAN_POINT('Ctrl Pts',(-3.95285778800006,2.2,1.22121597299999));
#310283=CARTESIAN_POINT('Ctrl Pts',(-3.95415020300006,12.2,1.22126108099998));
#310284=CARTESIAN_POINT('Ctrl Pts',(-3.95415020300006,5.2,1.22126108099998));
#310285=CARTESIAN_POINT('Ctrl Pts',(-3.95415020300006,2.2,1.22126108099998));
#310286=CARTESIAN_POINT('Ctrl Pts',(-3.95544768200006,12.2,1.22130481199999));
#310287=CARTESIAN_POINT('Ctrl Pts',(-3.95544768200006,5.2,1.22130481199999));
#310288=CARTESIAN_POINT('Ctrl Pts',(-3.95544768200006,2.2,1.22130481199999));
#310289=CARTESIAN_POINT('Ctrl Pts',(-3.95675021600006,12.2,1.22134715899998));
#310290=CARTESIAN_POINT('Ctrl Pts',(-3.95675021600006,5.2,1.22134715899998));
#310291=CARTESIAN_POINT('Ctrl Pts',(-3.95675021600006,2.2,1.22134715899998));
#310292=CARTESIAN_POINT('Ctrl Pts',(-3.95805779600006,12.2,1.22138810799999));
#310293=CARTESIAN_POINT('Ctrl Pts',(-3.95805779600006,5.2,1.22138810799999));
#310294=CARTESIAN_POINT('Ctrl Pts',(-3.95805779600006,2.2,1.22138810799999));
#310295=CARTESIAN_POINT('Ctrl Pts',(-3.95937041400006,12.2,1.22142764599999));
#310296=CARTESIAN_POINT('Ctrl Pts',(-3.95937041400006,5.2,1.22142764599999));
#310297=CARTESIAN_POINT('Ctrl Pts',(-3.95937041400006,2.2,1.22142764599999));
#310298=CARTESIAN_POINT('Ctrl Pts',(-3.96068805900006,12.2,1.22146576599999));
#310299=CARTESIAN_POINT('Ctrl Pts',(-3.96068805900006,5.2,1.22146576599999));
#310300=CARTESIAN_POINT('Ctrl Pts',(-3.96068805900006,2.2,1.22146576599999));
#310301=CARTESIAN_POINT('Ctrl Pts',(-3.96201072300006,12.2,1.22150245499999));
#310302=CARTESIAN_POINT('Ctrl Pts',(-3.96201072300006,5.2,1.22150245499999));
#310303=CARTESIAN_POINT('Ctrl Pts',(-3.96201072300006,2.2,1.22150245499999));
#310304=CARTESIAN_POINT('Ctrl Pts',(-3.96333839700006,12.2,1.22153769999999));
#310305=CARTESIAN_POINT('Ctrl Pts',(-3.96333839700006,5.2,1.22153769999999));
#310306=CARTESIAN_POINT('Ctrl Pts',(-3.96333839700006,2.2,1.22153769999999));
#310307=CARTESIAN_POINT('Ctrl Pts',(-3.96467107200006,12.2,1.22157149099999));
#310308=CARTESIAN_POINT('Ctrl Pts',(-3.96467107200006,5.2,1.22157149099999));
#310309=CARTESIAN_POINT('Ctrl Pts',(-3.96467107200006,2.2,1.22157149099999));
#310310=CARTESIAN_POINT('Ctrl Pts',(-3.96600874000006,12.2,1.22160381699999));
#310311=CARTESIAN_POINT('Ctrl Pts',(-3.96600874000006,5.2,1.22160381699999));
#310312=CARTESIAN_POINT('Ctrl Pts',(-3.96600874000006,2.2,1.22160381699999));
#310313=CARTESIAN_POINT('Ctrl Pts',(-3.96735139100006,12.2,1.22163466699998));
#310314=CARTESIAN_POINT('Ctrl Pts',(-3.96735139100006,5.2,1.22163466699998));
#310315=CARTESIAN_POINT('Ctrl Pts',(-3.96735139100006,2.2,1.22163466699998));
#310316=CARTESIAN_POINT('Ctrl Pts',(-3.96869901600006,12.2,1.22166402999999));
#310317=CARTESIAN_POINT('Ctrl Pts',(-3.96869901600006,5.2,1.22166402999999));
#310318=CARTESIAN_POINT('Ctrl Pts',(-3.96869901600006,2.2,1.22166402999999));
#310319=CARTESIAN_POINT('Ctrl Pts',(-3.97005160500006,12.2,1.22169189399999));
#310320=CARTESIAN_POINT('Ctrl Pts',(-3.97005160500006,5.2,1.22169189399999));
#310321=CARTESIAN_POINT('Ctrl Pts',(-3.97005160500006,2.2,1.22169189399999));
#310322=CARTESIAN_POINT('Ctrl Pts',(-3.97140915200006,12.2,1.22171824799999));
#310323=CARTESIAN_POINT('Ctrl Pts',(-3.97140915200006,5.2,1.22171824799999));
#310324=CARTESIAN_POINT('Ctrl Pts',(-3.97140915200006,2.2,1.22171824799999));
#310325=CARTESIAN_POINT('Ctrl Pts',(-3.97277164500006,12.2,1.22174308099999));
#310326=CARTESIAN_POINT('Ctrl Pts',(-3.97277164500006,5.2,1.22174308099999));
#310327=CARTESIAN_POINT('Ctrl Pts',(-3.97277164500006,2.2,1.22174308099999));
#310328=CARTESIAN_POINT('Ctrl Pts',(-3.97413907700006,12.2,1.22176638299999));
#310329=CARTESIAN_POINT('Ctrl Pts',(-3.97413907700006,5.2,1.22176638299999));
#310330=CARTESIAN_POINT('Ctrl Pts',(-3.97413907700006,2.2,1.22176638299999));
#310331=CARTESIAN_POINT('Ctrl Pts',(-3.97551143800006,12.2,1.22178814199998));
#310332=CARTESIAN_POINT('Ctrl Pts',(-3.97551143800006,5.2,1.22178814199998));
#310333=CARTESIAN_POINT('Ctrl Pts',(-3.97551143800006,2.2,1.22178814199998));
#310334=CARTESIAN_POINT('Ctrl Pts',(-3.97688871900006,12.2,1.22180834799998));
#310335=CARTESIAN_POINT('Ctrl Pts',(-3.97688871900006,5.2,1.22180834799998));
#310336=CARTESIAN_POINT('Ctrl Pts',(-3.97688871900006,2.2,1.22180834799998));
#310337=CARTESIAN_POINT('Ctrl Pts',(-3.97827091300006,12.2,1.22182698899998));
#310338=CARTESIAN_POINT('Ctrl Pts',(-3.97827091300006,5.2,1.22182698899998));
#310339=CARTESIAN_POINT('Ctrl Pts',(-3.97827091300006,2.2,1.22182698899998));
#310340=CARTESIAN_POINT('Ctrl Pts',(-3.97965800800006,12.2,1.22184405499999));
#310341=CARTESIAN_POINT('Ctrl Pts',(-3.97965800800006,5.2,1.22184405499999));
#310342=CARTESIAN_POINT('Ctrl Pts',(-3.97965800800006,2.2,1.22184405499999));
#310343=CARTESIAN_POINT('Ctrl Pts',(-3.98104999700006,12.2,1.22185953499999));
#310344=CARTESIAN_POINT('Ctrl Pts',(-3.98104999700006,5.2,1.22185953499999));
#310345=CARTESIAN_POINT('Ctrl Pts',(-3.98104999700006,2.2,1.22185953499999));
#310346=CARTESIAN_POINT('Ctrl Pts',(-3.98244687100005,12.2,1.22187341799998));
#310347=CARTESIAN_POINT('Ctrl Pts',(-3.98244687100005,5.2,1.22187341799998));
#310348=CARTESIAN_POINT('Ctrl Pts',(-3.98244687100005,2.2,1.22187341799998));
#310349=CARTESIAN_POINT('Ctrl Pts',(-3.98384862200006,12.2,1.22188569399999));
#310350=CARTESIAN_POINT('Ctrl Pts',(-3.98384862200006,5.2,1.22188569399999));
#310351=CARTESIAN_POINT('Ctrl Pts',(-3.98384862200006,2.2,1.22188569399999));
#310352=CARTESIAN_POINT('Ctrl Pts',(-3.98525523800005,12.2,1.22189634999998));
#310353=CARTESIAN_POINT('Ctrl Pts',(-3.98525523800005,5.2,1.22189634999998));
#310354=CARTESIAN_POINT('Ctrl Pts',(-3.98525523800005,2.2,1.22189634999998));
#310355=CARTESIAN_POINT('Ctrl Pts',(-3.98666671300006,12.2,1.22190537899999));
#310356=CARTESIAN_POINT('Ctrl Pts',(-3.98666671300006,5.2,1.22190537899999));
#310357=CARTESIAN_POINT('Ctrl Pts',(-3.98666671300006,2.2,1.22190537899999));
#310358=CARTESIAN_POINT('Ctrl Pts',(-3.98808303600005,12.2,1.22191276799999));
#310359=CARTESIAN_POINT('Ctrl Pts',(-3.98808303600005,5.2,1.22191276799999));
#310360=CARTESIAN_POINT('Ctrl Pts',(-3.98808303600005,2.2,1.22191276799999));
#310361=CARTESIAN_POINT('Ctrl Pts',(-3.98950420000006,12.2,1.22191850599998));
#310362=CARTESIAN_POINT('Ctrl Pts',(-3.98950420000006,5.2,1.22191850599998));
#310363=CARTESIAN_POINT('Ctrl Pts',(-3.98950420000006,2.2,1.22191850599998));
#310364=CARTESIAN_POINT('Ctrl Pts',(-3.99093019600006,12.2,1.22192258299998));
#310365=CARTESIAN_POINT('Ctrl Pts',(-3.99093019600006,5.2,1.22192258299998));
#310366=CARTESIAN_POINT('Ctrl Pts',(-3.99093019600006,2.2,1.22192258299998));
#310367=CARTESIAN_POINT('Ctrl Pts',(-3.99236101300006,12.2,1.22192498899999));
#310368=CARTESIAN_POINT('Ctrl Pts',(-3.99236101300006,5.2,1.22192498899999));
#310369=CARTESIAN_POINT('Ctrl Pts',(-3.99236101300006,2.2,1.22192498899999));
#310370=CARTESIAN_POINT('Ctrl Pts',(-3.99379664400006,12.2,1.22192571399999));
#310371=CARTESIAN_POINT('Ctrl Pts',(-3.99379664400006,5.2,1.22192571399999));
#310372=CARTESIAN_POINT('Ctrl Pts',(-3.99379664400006,2.2,1.22192571399999));
#310373=CARTESIAN_POINT('Ctrl Pts',(-3.99523707900006,12.2,1.22192474599998));
#310374=CARTESIAN_POINT('Ctrl Pts',(-3.99523707900006,5.2,1.22192474599998));
#310375=CARTESIAN_POINT('Ctrl Pts',(-3.99523707900006,2.2,1.22192474599998));
#310376=CARTESIAN_POINT('Ctrl Pts',(-3.99668231100006,12.2,1.22192207599999));
#310377=CARTESIAN_POINT('Ctrl Pts',(-3.99668231100006,5.2,1.22192207599999));
#310378=CARTESIAN_POINT('Ctrl Pts',(-3.99668231100006,2.2,1.22192207599999));
#310379=CARTESIAN_POINT('Ctrl Pts',(-3.99813233000006,12.2,1.22191769199999));
#310380=CARTESIAN_POINT('Ctrl Pts',(-3.99813233000006,5.2,1.22191769199999));
#310381=CARTESIAN_POINT('Ctrl Pts',(-3.99813233000006,2.2,1.22191769199999));
#310382=CARTESIAN_POINT('Ctrl Pts',(-3.99958712600006,12.2,1.22191158499998));
#310383=CARTESIAN_POINT('Ctrl Pts',(-3.99958712600006,5.2,1.22191158499998));
#310384=CARTESIAN_POINT('Ctrl Pts',(-3.99958712600006,2.2,1.22191158499998));
#310385=CARTESIAN_POINT('Ctrl Pts',(-4.00104669100006,12.2,1.22190374299999));
#310386=CARTESIAN_POINT('Ctrl Pts',(-4.00104669100006,5.2,1.22190374299999));
#310387=CARTESIAN_POINT('Ctrl Pts',(-4.00104669100006,2.2,1.22190374299999));
#310388=CARTESIAN_POINT('Ctrl Pts',(-4.00251101700006,12.2,1.22189415799999));
#310389=CARTESIAN_POINT('Ctrl Pts',(-4.00251101700006,5.2,1.22189415799999));
#310390=CARTESIAN_POINT('Ctrl Pts',(-4.00251101700006,2.2,1.22189415799999));
#310391=CARTESIAN_POINT('Ctrl Pts',(-4.00398009500006,12.2,1.22188281799998));
#310392=CARTESIAN_POINT('Ctrl Pts',(-4.00398009500006,5.2,1.22188281799998));
#310393=CARTESIAN_POINT('Ctrl Pts',(-4.00398009500006,2.2,1.22188281799998));
#310394=CARTESIAN_POINT('Ctrl Pts',(-4.00545391400006,12.2,1.22186971399998));
#310395=CARTESIAN_POINT('Ctrl Pts',(-4.00545391400006,5.2,1.22186971399998));
#310396=CARTESIAN_POINT('Ctrl Pts',(-4.00545391400006,2.2,1.22186971399998));
#310397=CARTESIAN_POINT('Ctrl Pts',(-4.00693246700006,12.2,1.22185483399999));
#310398=CARTESIAN_POINT('Ctrl Pts',(-4.00693246700006,5.2,1.22185483399999));
#310399=CARTESIAN_POINT('Ctrl Pts',(-4.00693246700006,2.2,1.22185483399999));
#310400=CARTESIAN_POINT('Ctrl Pts',(-4.00841574600006,12.2,1.22183816999998));
#310401=CARTESIAN_POINT('Ctrl Pts',(-4.00841574600006,5.2,1.22183816999998));
#310402=CARTESIAN_POINT('Ctrl Pts',(-4.00841574600006,2.2,1.22183816999998));
#310403=CARTESIAN_POINT('Ctrl Pts',(-4.00990374000005,12.2,1.22181970999999));
#310404=CARTESIAN_POINT('Ctrl Pts',(-4.00990374000005,5.2,1.22181970999999));
#310405=CARTESIAN_POINT('Ctrl Pts',(-4.00990374000005,2.2,1.22181970999999));
#310406=CARTESIAN_POINT('Ctrl Pts',(-4.01139644200006,12.2,1.22179944599999));
#310407=CARTESIAN_POINT('Ctrl Pts',(-4.01139644200006,5.2,1.22179944599999));
#310408=CARTESIAN_POINT('Ctrl Pts',(-4.01139644200006,2.2,1.22179944599999));
#310409=CARTESIAN_POINT('Ctrl Pts',(-4.01289384200005,12.2,1.22177736499999));
#310410=CARTESIAN_POINT('Ctrl Pts',(-4.01289384200005,5.2,1.22177736499999));
#310411=CARTESIAN_POINT('Ctrl Pts',(-4.01289384200005,2.2,1.22177736499999));
#310412=CARTESIAN_POINT('Ctrl Pts',(-4.01439593200006,12.2,1.22175345999999));
#310413=CARTESIAN_POINT('Ctrl Pts',(-4.01439593200006,5.2,1.22175345999999));
#310414=CARTESIAN_POINT('Ctrl Pts',(-4.01439593200006,2.2,1.22175345999999));
#310415=CARTESIAN_POINT('Ctrl Pts',(-4.01590270300006,12.2,1.22172771799999));
#310416=CARTESIAN_POINT('Ctrl Pts',(-4.01590270300006,5.2,1.22172771799999));
#310417=CARTESIAN_POINT('Ctrl Pts',(-4.01590270300006,2.2,1.22172771799999));
#310418=CARTESIAN_POINT('Ctrl Pts',(-4.01741414500006,12.2,1.22170013199999));
#310419=CARTESIAN_POINT('Ctrl Pts',(-4.01741414500006,5.2,1.22170013199999));
#310420=CARTESIAN_POINT('Ctrl Pts',(-4.01741414500006,2.2,1.22170013199999));
#310421=CARTESIAN_POINT('Ctrl Pts',(-4.01893025000006,12.2,1.22167069099998));
#310422=CARTESIAN_POINT('Ctrl Pts',(-4.01893025000006,5.2,1.22167069099998));
#310423=CARTESIAN_POINT('Ctrl Pts',(-4.01893025000006,2.2,1.22167069099998));
#310424=CARTESIAN_POINT('Ctrl Pts',(-4.02045101100006,12.2,1.22163938299999));
#310425=CARTESIAN_POINT('Ctrl Pts',(-4.02045101100006,5.2,1.22163938299999));
#310426=CARTESIAN_POINT('Ctrl Pts',(-4.02045101100006,2.2,1.22163938299999));
#310427=CARTESIAN_POINT('Ctrl Pts',(-4.02197641600006,12.2,1.22160620099999));
#310428=CARTESIAN_POINT('Ctrl Pts',(-4.02197641600006,5.2,1.22160620099999));
#310429=CARTESIAN_POINT('Ctrl Pts',(-4.02197641600006,2.2,1.22160620099999));
#310430=CARTESIAN_POINT('Ctrl Pts',(-4.02350645800006,12.2,1.22157113399998));
#310431=CARTESIAN_POINT('Ctrl Pts',(-4.02350645800006,5.2,1.22157113399998));
#310432=CARTESIAN_POINT('Ctrl Pts',(-4.02350645800006,2.2,1.22157113399998));
#310433=CARTESIAN_POINT('Ctrl Pts',(-4.02504112800006,12.2,1.22153417099998));
#310434=CARTESIAN_POINT('Ctrl Pts',(-4.02504112800006,5.2,1.22153417099998));
#310435=CARTESIAN_POINT('Ctrl Pts',(-4.02504112800006,2.2,1.22153417099998));
#310436=CARTESIAN_POINT('Ctrl Pts',(-4.02658041700006,12.2,1.22149530499998));
#310437=CARTESIAN_POINT('Ctrl Pts',(-4.02658041700006,5.2,1.22149530499998));
#310438=CARTESIAN_POINT('Ctrl Pts',(-4.02658041700006,2.2,1.22149530499998));
#310439=CARTESIAN_POINT('Ctrl Pts',(-4.02812431700006,12.2,1.22145452299999));
#310440=CARTESIAN_POINT('Ctrl Pts',(-4.02812431700006,5.2,1.22145452299999));
#310441=CARTESIAN_POINT('Ctrl Pts',(-4.02812431700006,2.2,1.22145452299999));
#310442=CARTESIAN_POINT('Ctrl Pts',(-4.02967281800006,12.2,1.22141181799998));
#310443=CARTESIAN_POINT('Ctrl Pts',(-4.02967281800006,5.2,1.22141181799998));
#310444=CARTESIAN_POINT('Ctrl Pts',(-4.02967281800006,2.2,1.22141181799998));
#310445=CARTESIAN_POINT('Ctrl Pts',(-4.03122591200006,12.2,1.22136717899998));
#310446=CARTESIAN_POINT('Ctrl Pts',(-4.03122591200006,5.2,1.22136717899998));
#310447=CARTESIAN_POINT('Ctrl Pts',(-4.03122591200006,2.2,1.22136717899998));
#310448=CARTESIAN_POINT('Ctrl Pts',(-4.03278359100006,12.2,1.22132059599998));
#310449=CARTESIAN_POINT('Ctrl Pts',(-4.03278359100006,5.2,1.22132059599998));
#310450=CARTESIAN_POINT('Ctrl Pts',(-4.03278359100006,2.2,1.22132059599998));
#310451=CARTESIAN_POINT('Ctrl Pts',(-4.03434584400006,12.2,1.22127206099998));
#310452=CARTESIAN_POINT('Ctrl Pts',(-4.03434584400006,5.2,1.22127206099998));
#310453=CARTESIAN_POINT('Ctrl Pts',(-4.03434584400006,2.2,1.22127206099998));
#310454=CARTESIAN_POINT('Ctrl Pts',(-4.03591266300006,12.2,1.22122156299998));
#310455=CARTESIAN_POINT('Ctrl Pts',(-4.03591266300006,5.2,1.22122156299998));
#310456=CARTESIAN_POINT('Ctrl Pts',(-4.03591266300006,2.2,1.22122156299998));
#310457=CARTESIAN_POINT('Ctrl Pts',(-4.03748404100006,12.2,1.22116909199999));
#310458=CARTESIAN_POINT('Ctrl Pts',(-4.03748404100006,5.2,1.22116909199999));
#310459=CARTESIAN_POINT('Ctrl Pts',(-4.03748404100006,2.2,1.22116909199999));
#310460=CARTESIAN_POINT('Ctrl Pts',(-4.03905996800006,12.2,1.22111463899999));
#310461=CARTESIAN_POINT('Ctrl Pts',(-4.03905996800006,5.2,1.22111463899999));
#310462=CARTESIAN_POINT('Ctrl Pts',(-4.03905996800006,2.2,1.22111463899999));
#310463=CARTESIAN_POINT('Ctrl Pts',(-4.04064043500005,12.2,1.22105819399998));
#310464=CARTESIAN_POINT('Ctrl Pts',(-4.04064043500005,5.2,1.22105819399998));
#310465=CARTESIAN_POINT('Ctrl Pts',(-4.04064043500005,2.2,1.22105819399998));
#310466=CARTESIAN_POINT('Ctrl Pts',(-4.04222543400006,12.2,1.22099974999998));
#310467=CARTESIAN_POINT('Ctrl Pts',(-4.04222543400006,5.2,1.22099974999998));
#310468=CARTESIAN_POINT('Ctrl Pts',(-4.04222543400006,2.2,1.22099974999998));
#310469=CARTESIAN_POINT('Ctrl Pts',(-4.04381495400005,12.2,1.22093929399998));
#310470=CARTESIAN_POINT('Ctrl Pts',(-4.04381495400005,5.2,1.22093929399998));
#310471=CARTESIAN_POINT('Ctrl Pts',(-4.04381495400005,2.2,1.22093929399998));
#310472=CARTESIAN_POINT('Ctrl Pts',(-4.04540899000006,12.2,1.22087681899998));
#310473=CARTESIAN_POINT('Ctrl Pts',(-4.04540899000006,5.2,1.22087681899998));
#310474=CARTESIAN_POINT('Ctrl Pts',(-4.04540899000006,2.2,1.22087681899998));
#310475=CARTESIAN_POINT('Ctrl Pts',(-4.04700753000006,12.2,1.22081231499998));
#310476=CARTESIAN_POINT('Ctrl Pts',(-4.04700753000006,5.2,1.22081231499998));
#310477=CARTESIAN_POINT('Ctrl Pts',(-4.04700753000006,2.2,1.22081231499998));
#310478=CARTESIAN_POINT('Ctrl Pts',(-4.04861056700006,12.2,1.22074577299998));
#310479=CARTESIAN_POINT('Ctrl Pts',(-4.04861056700006,5.2,1.22074577299998));
#310480=CARTESIAN_POINT('Ctrl Pts',(-4.04861056700006,2.2,1.22074577299998));
#310481=CARTESIAN_POINT('Ctrl Pts',(-4.05021809200006,12.2,1.22067718299999));
#310482=CARTESIAN_POINT('Ctrl Pts',(-4.05021809200006,5.2,1.22067718299999));
#310483=CARTESIAN_POINT('Ctrl Pts',(-4.05021809200006,2.2,1.22067718299999));
#310484=CARTESIAN_POINT('Ctrl Pts',(-4.05183009600006,12.2,1.22060653499998));
#310485=CARTESIAN_POINT('Ctrl Pts',(-4.05183009600006,5.2,1.22060653499998));
#310486=CARTESIAN_POINT('Ctrl Pts',(-4.05183009600006,2.2,1.22060653499998));
#310487=CARTESIAN_POINT('Ctrl Pts',(-4.05344657100006,12.2,1.22053382099998));
#310488=CARTESIAN_POINT('Ctrl Pts',(-4.05344657100006,5.2,1.22053382099998));
#310489=CARTESIAN_POINT('Ctrl Pts',(-4.05344657100006,2.2,1.22053382099998));
#310490=CARTESIAN_POINT('Ctrl Pts',(-4.05506750700006,12.2,1.22045903099998));
#310491=CARTESIAN_POINT('Ctrl Pts',(-4.05506750700006,5.2,1.22045903099998));
#310492=CARTESIAN_POINT('Ctrl Pts',(-4.05506750700006,2.2,1.22045903099998));
#310493=CARTESIAN_POINT('Ctrl Pts',(-4.05669289600006,12.2,1.22038215699999));
#310494=CARTESIAN_POINT('Ctrl Pts',(-4.05669289600006,5.2,1.22038215699999));
#310495=CARTESIAN_POINT('Ctrl Pts',(-4.05669289600006,2.2,1.22038215699999));
#310496=CARTESIAN_POINT('Ctrl Pts',(-4.05832272900006,12.2,1.22030318799998));
#310497=CARTESIAN_POINT('Ctrl Pts',(-4.05832272900006,5.2,1.22030318799998));
#310498=CARTESIAN_POINT('Ctrl Pts',(-4.05832272900006,2.2,1.22030318799998));
#310499=CARTESIAN_POINT('Ctrl Pts',(-4.05995699900005,12.2,1.22022211699999));
#310500=CARTESIAN_POINT('Ctrl Pts',(-4.05995699900005,5.2,1.22022211699999));
#310501=CARTESIAN_POINT('Ctrl Pts',(-4.05995699900005,2.2,1.22022211699999));
#310502=CARTESIAN_POINT('Ctrl Pts',(-4.06159569400006,12.2,1.22013893199998));
#310503=CARTESIAN_POINT('Ctrl Pts',(-4.06159569400006,5.2,1.22013893199998));
#310504=CARTESIAN_POINT('Ctrl Pts',(-4.06159569400006,2.2,1.22013893199998));
#310505=CARTESIAN_POINT('Ctrl Pts',(-4.06323880800006,12.2,1.22005362699999));
#310506=CARTESIAN_POINT('Ctrl Pts',(-4.06323880800006,5.2,1.22005362699999));
#310507=CARTESIAN_POINT('Ctrl Pts',(-4.06323880800006,2.2,1.22005362699999));
#310508=CARTESIAN_POINT('Ctrl Pts',(-4.06488633200006,12.2,1.21996618999999));
#310509=CARTESIAN_POINT('Ctrl Pts',(-4.06488633200006,5.2,1.21996618999999));
#310510=CARTESIAN_POINT('Ctrl Pts',(-4.06488633200006,2.2,1.21996618999999));
#310511=CARTESIAN_POINT('Ctrl Pts',(-4.06653825600006,12.2,1.21987661499999));
#310512=CARTESIAN_POINT('Ctrl Pts',(-4.06653825600006,5.2,1.21987661499999));
#310513=CARTESIAN_POINT('Ctrl Pts',(-4.06653825600006,2.2,1.21987661499999));
#310514=CARTESIAN_POINT('Ctrl Pts',(-4.06819457300006,12.2,1.21978488999999));
#310515=CARTESIAN_POINT('Ctrl Pts',(-4.06819457300006,5.2,1.21978488999999));
#310516=CARTESIAN_POINT('Ctrl Pts',(-4.06819457300006,2.2,1.21978488999999));
#310517=CARTESIAN_POINT('Ctrl Pts',(-4.06985527300006,12.2,1.21969100899999));
#310518=CARTESIAN_POINT('Ctrl Pts',(-4.06985527300006,5.2,1.21969100899999));
#310519=CARTESIAN_POINT('Ctrl Pts',(-4.06985527300006,2.2,1.21969100899999));
#310520=CARTESIAN_POINT('Ctrl Pts',(-4.07152034800006,12.2,1.21959495999999));
#310521=CARTESIAN_POINT('Ctrl Pts',(-4.07152034800006,5.2,1.21959495999999));
#310522=CARTESIAN_POINT('Ctrl Pts',(-4.07152034800006,2.2,1.21959495999999));
#310523=CARTESIAN_POINT('Ctrl Pts',(-4.07318978900006,12.2,1.21949673599998));
#310524=CARTESIAN_POINT('Ctrl Pts',(-4.07318978900006,5.2,1.21949673599998));
#310525=CARTESIAN_POINT('Ctrl Pts',(-4.07318978900006,2.2,1.21949673599998));
#310526=CARTESIAN_POINT('Ctrl Pts',(-4.07486358800006,12.2,1.21939632799998));
#310527=CARTESIAN_POINT('Ctrl Pts',(-4.07486358800006,5.2,1.21939632799998));
#310528=CARTESIAN_POINT('Ctrl Pts',(-4.07486358800006,2.2,1.21939632799998));
#310529=CARTESIAN_POINT('Ctrl Pts',(-4.07654173500006,12.2,1.21929372599999));
#310530=CARTESIAN_POINT('Ctrl Pts',(-4.07654173500006,5.2,1.21929372599999));
#310531=CARTESIAN_POINT('Ctrl Pts',(-4.07654173500006,2.2,1.21929372599999));
#310532=CARTESIAN_POINT('Ctrl Pts',(-4.07822422300006,12.2,1.21918892199998));
#310533=CARTESIAN_POINT('Ctrl Pts',(-4.07822422300006,5.2,1.21918892199998));
#310534=CARTESIAN_POINT('Ctrl Pts',(-4.07822422300006,2.2,1.21918892199998));
#310535=CARTESIAN_POINT('Ctrl Pts',(-4.07991104100006,12.2,1.21908190799998));
#310536=CARTESIAN_POINT('Ctrl Pts',(-4.07991104100006,5.2,1.21908190799998));
#310537=CARTESIAN_POINT('Ctrl Pts',(-4.07991104100006,2.2,1.21908190799998));
#310538=CARTESIAN_POINT('Ctrl Pts',(-4.08160218300006,12.2,1.21897267399998));
#310539=CARTESIAN_POINT('Ctrl Pts',(-4.08160218300006,5.2,1.21897267399998));
#310540=CARTESIAN_POINT('Ctrl Pts',(-4.08160218300006,2.2,1.21897267399998));
#310541=CARTESIAN_POINT('Ctrl Pts',(-4.08329763900006,12.2,1.21886121099998));
#310542=CARTESIAN_POINT('Ctrl Pts',(-4.08329763900006,5.2,1.21886121099998));
#310543=CARTESIAN_POINT('Ctrl Pts',(-4.08329763900006,2.2,1.21886121099998));
#310544=CARTESIAN_POINT('Ctrl Pts',(-4.08499740100006,12.2,1.21874751099998));
#310545=CARTESIAN_POINT('Ctrl Pts',(-4.08499740100006,5.2,1.21874751099998));
#310546=CARTESIAN_POINT('Ctrl Pts',(-4.08499740100006,2.2,1.21874751099998));
#310547=CARTESIAN_POINT('Ctrl Pts',(-4.08670146000006,12.2,1.21863156499999));
#310548=CARTESIAN_POINT('Ctrl Pts',(-4.08670146000006,5.2,1.21863156499999));
#310549=CARTESIAN_POINT('Ctrl Pts',(-4.08670146000006,2.2,1.21863156499999));
#310550=CARTESIAN_POINT('Ctrl Pts',(-4.08840980700006,12.2,1.21851336499998));
#310551=CARTESIAN_POINT('Ctrl Pts',(-4.08840980700006,5.2,1.21851336499998));
#310552=CARTESIAN_POINT('Ctrl Pts',(-4.08840980700006,2.2,1.21851336499998));
#310553=CARTESIAN_POINT('Ctrl Pts',(-4.09012243300006,12.2,1.21839290099999));
#310554=CARTESIAN_POINT('Ctrl Pts',(-4.09012243300006,5.2,1.21839290099999));
#310555=CARTESIAN_POINT('Ctrl Pts',(-4.09012243300006,2.2,1.21839290099999));
#310556=CARTESIAN_POINT('Ctrl Pts',(-4.09183933100006,12.2,1.21827016599998));
#310557=CARTESIAN_POINT('Ctrl Pts',(-4.09183933100006,5.2,1.21827016599998));
#310558=CARTESIAN_POINT('Ctrl Pts',(-4.09183933100006,2.2,1.21827016599998));
#310559=CARTESIAN_POINT('Ctrl Pts',(-4.09356049200006,12.2,1.21814514999999));
#310560=CARTESIAN_POINT('Ctrl Pts',(-4.09356049200006,5.2,1.21814514999999));
#310561=CARTESIAN_POINT('Ctrl Pts',(-4.09356049200006,2.2,1.21814514999999));
#310562=CARTESIAN_POINT('Ctrl Pts',(-4.09528590600006,12.2,1.21801784499999));
#310563=CARTESIAN_POINT('Ctrl Pts',(-4.09528590600006,5.2,1.21801784499999));
#310564=CARTESIAN_POINT('Ctrl Pts',(-4.09528590600006,2.2,1.21801784499999));
#310565=CARTESIAN_POINT('Ctrl Pts',(-4.09701556600006,12.2,1.21788824299998));
#310566=CARTESIAN_POINT('Ctrl Pts',(-4.09701556600006,5.2,1.21788824299998));
#310567=CARTESIAN_POINT('Ctrl Pts',(-4.09701556600006,2.2,1.21788824299998));
#310568=CARTESIAN_POINT('Ctrl Pts',(-4.09874946100006,12.2,1.21775633399999));
#310569=CARTESIAN_POINT('Ctrl Pts',(-4.09874946100006,5.2,1.21775633399999));
#310570=CARTESIAN_POINT('Ctrl Pts',(-4.09874946100006,2.2,1.21775633399999));
#310571=CARTESIAN_POINT('Ctrl Pts',(-4.10048758500006,12.2,1.21762211099998));
#310572=CARTESIAN_POINT('Ctrl Pts',(-4.10048758500006,5.2,1.21762211099998));
#310573=CARTESIAN_POINT('Ctrl Pts',(-4.10048758500006,2.2,1.21762211099998));
#310574=CARTESIAN_POINT('Ctrl Pts',(-4.10222992800006,12.2,1.21748556499998));
#310575=CARTESIAN_POINT('Ctrl Pts',(-4.10222992800006,5.2,1.21748556499998));
#310576=CARTESIAN_POINT('Ctrl Pts',(-4.10222992800006,2.2,1.21748556499998));
#310577=CARTESIAN_POINT('Ctrl Pts',(-4.10397648300005,12.2,1.21734668799999));
#310578=CARTESIAN_POINT('Ctrl Pts',(-4.10397648300005,5.2,1.21734668799999));
#310579=CARTESIAN_POINT('Ctrl Pts',(-4.10397648300005,2.2,1.21734668799999));
#310580=CARTESIAN_POINT('Ctrl Pts',(-4.10572724000006,12.2,1.21720546999999));
#310581=CARTESIAN_POINT('Ctrl Pts',(-4.10572724000006,5.2,1.21720546999999));
#310582=CARTESIAN_POINT('Ctrl Pts',(-4.10572724000006,2.2,1.21720546999999));
#310583=CARTESIAN_POINT('Ctrl Pts',(-4.10748219000006,12.2,1.21706190499999));
#310584=CARTESIAN_POINT('Ctrl Pts',(-4.10748219000006,5.2,1.21706190499999));
#310585=CARTESIAN_POINT('Ctrl Pts',(-4.10748219000006,2.2,1.21706190499999));
#310586=CARTESIAN_POINT('Ctrl Pts',(-4.10924132600006,12.2,1.21691598299998));
#310587=CARTESIAN_POINT('Ctrl Pts',(-4.10924132600006,5.2,1.21691598299998));
#310588=CARTESIAN_POINT('Ctrl Pts',(-4.10924132600006,2.2,1.21691598299998));
#310589=CARTESIAN_POINT('Ctrl Pts',(-4.11100463700006,12.2,1.21676769599999));
#310590=CARTESIAN_POINT('Ctrl Pts',(-4.11100463700006,5.2,1.21676769599999));
#310591=CARTESIAN_POINT('Ctrl Pts',(-4.11100463700006,2.2,1.21676769599999));
#310592=CARTESIAN_POINT('Ctrl Pts',(-4.11277211800006,12.2,1.21661703499999));
#310593=CARTESIAN_POINT('Ctrl Pts',(-4.11277211800006,5.2,1.21661703499999));
#310594=CARTESIAN_POINT('Ctrl Pts',(-4.11277211800006,2.2,1.21661703499999));
#310595=CARTESIAN_POINT('Ctrl Pts',(-4.11454375600006,12.2,1.21646399399999));
#310596=CARTESIAN_POINT('Ctrl Pts',(-4.11454375600006,5.2,1.21646399399999));
#310597=CARTESIAN_POINT('Ctrl Pts',(-4.11454375600006,2.2,1.21646399399999));
#310598=CARTESIAN_POINT('Ctrl Pts',(-4.11631954700006,12.2,1.21630856299999));
#310599=CARTESIAN_POINT('Ctrl Pts',(-4.11631954700006,5.2,1.21630856299999));
#310600=CARTESIAN_POINT('Ctrl Pts',(-4.11631954700006,2.2,1.21630856299999));
#310601=CARTESIAN_POINT('Ctrl Pts',(-4.11809947900006,12.2,1.21615073299999));
#310602=CARTESIAN_POINT('Ctrl Pts',(-4.11809947900006,5.2,1.21615073299999));
#310603=CARTESIAN_POINT('Ctrl Pts',(-4.11809947900006,2.2,1.21615073299999));
#310604=CARTESIAN_POINT('Ctrl Pts',(-4.11988354400005,12.2,1.21599049699999));
#310605=CARTESIAN_POINT('Ctrl Pts',(-4.11988354400005,5.2,1.21599049699999));
#310606=CARTESIAN_POINT('Ctrl Pts',(-4.11988354400005,2.2,1.21599049699999));
#310607=CARTESIAN_POINT('Ctrl Pts',(-4.12167173600006,12.2,1.21582784799998));
#310608=CARTESIAN_POINT('Ctrl Pts',(-4.12167173600006,5.2,1.21582784799998));
#310609=CARTESIAN_POINT('Ctrl Pts',(-4.12167173600006,2.2,1.21582784799998));
#310610=CARTESIAN_POINT('Ctrl Pts',(-4.12346404300005,12.2,1.21566277499999));
#310611=CARTESIAN_POINT('Ctrl Pts',(-4.12346404300005,5.2,1.21566277499999));
#310612=CARTESIAN_POINT('Ctrl Pts',(-4.12346404300005,2.2,1.21566277499999));
#310613=CARTESIAN_POINT('Ctrl Pts',(-4.12526045900006,12.2,1.21549527199999));
#310614=CARTESIAN_POINT('Ctrl Pts',(-4.12526045900006,5.2,1.21549527199999));
#310615=CARTESIAN_POINT('Ctrl Pts',(-4.12526045900006,2.2,1.21549527199999));
#310616=CARTESIAN_POINT('Ctrl Pts',(-4.12706097400006,12.2,1.21532533099999));
#310617=CARTESIAN_POINT('Ctrl Pts',(-4.12706097400006,5.2,1.21532533099999));
#310618=CARTESIAN_POINT('Ctrl Pts',(-4.12706097400006,2.2,1.21532533099999));
#310619=CARTESIAN_POINT('Ctrl Pts',(-4.12886558100006,12.2,1.21515294199999));
#310620=CARTESIAN_POINT('Ctrl Pts',(-4.12886558100006,5.2,1.21515294199999));
#310621=CARTESIAN_POINT('Ctrl Pts',(-4.12886558100006,2.2,1.21515294199999));
#310622=CARTESIAN_POINT('Ctrl Pts',(-4.13067426900006,12.2,1.21497809899999));
#310623=CARTESIAN_POINT('Ctrl Pts',(-4.13067426900006,5.2,1.21497809899999));
#310624=CARTESIAN_POINT('Ctrl Pts',(-4.13067426900006,2.2,1.21497809899999));
#310625=CARTESIAN_POINT('Ctrl Pts',(-4.13248703200006,12.2,1.21480079399999));
#310626=CARTESIAN_POINT('Ctrl Pts',(-4.13248703200006,5.2,1.21480079399999));
#310627=CARTESIAN_POINT('Ctrl Pts',(-4.13248703200006,2.2,1.21480079399999));
#310628=CARTESIAN_POINT('Ctrl Pts',(-4.13430386000006,12.2,1.21462101699999));
#310629=CARTESIAN_POINT('Ctrl Pts',(-4.13430386000006,5.2,1.21462101699999));
#310630=CARTESIAN_POINT('Ctrl Pts',(-4.13430386000006,2.2,1.21462101699999));
#310631=CARTESIAN_POINT('Ctrl Pts',(-4.13612474400006,12.2,1.21443876199999));
#310632=CARTESIAN_POINT('Ctrl Pts',(-4.13612474400006,5.2,1.21443876199999));
#310633=CARTESIAN_POINT('Ctrl Pts',(-4.13612474400006,2.2,1.21443876199999));
#310634=CARTESIAN_POINT('Ctrl Pts',(-4.13794967700006,12.2,1.21425401899999));
#310635=CARTESIAN_POINT('Ctrl Pts',(-4.13794967700006,5.2,1.21425401899999));
#310636=CARTESIAN_POINT('Ctrl Pts',(-4.13794967700006,2.2,1.21425401899999));
#310637=CARTESIAN_POINT('Ctrl Pts',(-4.13977865000006,12.2,1.21406678299998));
#310638=CARTESIAN_POINT('Ctrl Pts',(-4.13977865000006,5.2,1.21406678299998));
#310639=CARTESIAN_POINT('Ctrl Pts',(-4.13977865000006,2.2,1.21406678299998));
#310640=CARTESIAN_POINT('Ctrl Pts',(-4.14161165400006,12.2,1.21387704299998));
#310641=CARTESIAN_POINT('Ctrl Pts',(-4.14161165400006,5.2,1.21387704299998));
#310642=CARTESIAN_POINT('Ctrl Pts',(-4.14161165400006,2.2,1.21387704299998));
#310643=CARTESIAN_POINT('Ctrl Pts',(-4.14344868100006,12.2,1.21368479399999));
#310644=CARTESIAN_POINT('Ctrl Pts',(-4.14344868100006,5.2,1.21368479399999));
#310645=CARTESIAN_POINT('Ctrl Pts',(-4.14344868100006,2.2,1.21368479399999));
#310646=CARTESIAN_POINT('Ctrl Pts',(-4.14528972300006,12.2,1.21349002599999));
#310647=CARTESIAN_POINT('Ctrl Pts',(-4.14528972300006,5.2,1.21349002599999));
#310648=CARTESIAN_POINT('Ctrl Pts',(-4.14528972300006,2.2,1.21349002599999));
#310649=CARTESIAN_POINT('Ctrl Pts',(-4.14713477000006,12.2,1.21329273299999));
#310650=CARTESIAN_POINT('Ctrl Pts',(-4.14713477000006,5.2,1.21329273299999));
#310651=CARTESIAN_POINT('Ctrl Pts',(-4.14713477000006,2.2,1.21329273299999));
#310652=CARTESIAN_POINT('Ctrl Pts',(-4.14898381500006,12.2,1.21309290499998));
#310653=CARTESIAN_POINT('Ctrl Pts',(-4.14898381500006,5.2,1.21309290499998));
#310654=CARTESIAN_POINT('Ctrl Pts',(-4.14898381500006,2.2,1.21309290499998));
#310655=CARTESIAN_POINT('Ctrl Pts',(-4.15083684800006,12.2,1.21289053599998));
#310656=CARTESIAN_POINT('Ctrl Pts',(-4.15083684800006,5.2,1.21289053599998));
#310657=CARTESIAN_POINT('Ctrl Pts',(-4.15083684800006,2.2,1.21289053599998));
#310658=CARTESIAN_POINT('Ctrl Pts',(-4.15269386100006,12.2,1.21268561699999));
#310659=CARTESIAN_POINT('Ctrl Pts',(-4.15269386100006,5.2,1.21268561699999));
#310660=CARTESIAN_POINT('Ctrl Pts',(-4.15269386100006,2.2,1.21268561699999));
#310661=CARTESIAN_POINT('Ctrl Pts',(-4.15455484700006,12.2,1.21247814199998));
#310662=CARTESIAN_POINT('Ctrl Pts',(-4.15455484700006,5.2,1.21247814199998));
#310663=CARTESIAN_POINT('Ctrl Pts',(-4.15455484700006,2.2,1.21247814199998));
#310664=CARTESIAN_POINT('Ctrl Pts',(-4.15641979500006,12.2,1.21226810299999));
#310665=CARTESIAN_POINT('Ctrl Pts',(-4.15641979500006,5.2,1.21226810299999));
#310666=CARTESIAN_POINT('Ctrl Pts',(-4.15641979500006,2.2,1.21226810299999));
#310667=CARTESIAN_POINT('Ctrl Pts',(-4.15828869900006,12.2,1.21205548999999));
#310668=CARTESIAN_POINT('Ctrl Pts',(-4.15828869900006,5.2,1.21205548999999));
#310669=CARTESIAN_POINT('Ctrl Pts',(-4.15828869900006,2.2,1.21205548999999));
#310670=CARTESIAN_POINT('Ctrl Pts',(-4.16016154900006,12.2,1.21184029699998));
#310671=CARTESIAN_POINT('Ctrl Pts',(-4.16016154900006,5.2,1.21184029699998));
#310672=CARTESIAN_POINT('Ctrl Pts',(-4.16016154900006,2.2,1.21184029699998));
#310673=CARTESIAN_POINT('Ctrl Pts',(-4.16203833700005,12.2,1.21162251699999));
#310674=CARTESIAN_POINT('Ctrl Pts',(-4.16203833700005,5.2,1.21162251699999));
#310675=CARTESIAN_POINT('Ctrl Pts',(-4.16203833700005,2.2,1.21162251699999));
#310676=CARTESIAN_POINT('Ctrl Pts',(-4.16391905500006,12.2,1.21140214299999));
#310677=CARTESIAN_POINT('Ctrl Pts',(-4.16391905500006,5.2,1.21140214299999));
#310678=CARTESIAN_POINT('Ctrl Pts',(-4.16391905500006,2.2,1.21140214299999));
#310679=CARTESIAN_POINT('Ctrl Pts',(-4.16580369400006,12.2,1.21117916399998));
#310680=CARTESIAN_POINT('Ctrl Pts',(-4.16580369400006,5.2,1.21117916399998));
#310681=CARTESIAN_POINT('Ctrl Pts',(-4.16580369400006,2.2,1.21117916399998));
#310682=CARTESIAN_POINT('Ctrl Pts',(-4.16769224400006,12.2,1.21095357599998));
#310683=CARTESIAN_POINT('Ctrl Pts',(-4.16769224400006,5.2,1.21095357599998));
#310684=CARTESIAN_POINT('Ctrl Pts',(-4.16769224400006,2.2,1.21095357599998));
#310685=CARTESIAN_POINT('Ctrl Pts',(-4.16958470100006,12.2,1.21072537099999));
#310686=CARTESIAN_POINT('Ctrl Pts',(-4.16958470100006,5.2,1.21072537099999));
#310687=CARTESIAN_POINT('Ctrl Pts',(-4.16958470100006,2.2,1.21072537099999));
#310688=CARTESIAN_POINT('Ctrl Pts',(-4.17148105100006,12.2,1.21049453899999));
#310689=CARTESIAN_POINT('Ctrl Pts',(-4.17148105100006,5.2,1.21049453899999));
#310690=CARTESIAN_POINT('Ctrl Pts',(-4.17148105100006,2.2,1.21049453899999));
#310691=CARTESIAN_POINT('Ctrl Pts',(-4.17338129000006,12.2,1.21026107499999));
#310692=CARTESIAN_POINT('Ctrl Pts',(-4.17338129000006,5.2,1.21026107499999));
#310693=CARTESIAN_POINT('Ctrl Pts',(-4.17338129000006,2.2,1.21026107499999));
#310694=CARTESIAN_POINT('Ctrl Pts',(-4.17528540700006,12.2,1.21002497099999));
#310695=CARTESIAN_POINT('Ctrl Pts',(-4.17528540700006,5.2,1.21002497099999));
#310696=CARTESIAN_POINT('Ctrl Pts',(-4.17528540700006,2.2,1.21002497099999));
#310697=CARTESIAN_POINT('Ctrl Pts',(-4.17719339400006,12.2,1.20978621799999));
#310698=CARTESIAN_POINT('Ctrl Pts',(-4.17719339400006,5.2,1.20978621799999));
#310699=CARTESIAN_POINT('Ctrl Pts',(-4.17719339400006,2.2,1.20978621799999));
#310700=CARTESIAN_POINT('Ctrl Pts',(-4.17910524400006,12.2,1.20954481199998));
#310701=CARTESIAN_POINT('Ctrl Pts',(-4.17910524400006,5.2,1.20954481199998));
#310702=CARTESIAN_POINT('Ctrl Pts',(-4.17910524400006,2.2,1.20954481199998));
#310703=CARTESIAN_POINT('Ctrl Pts',(-4.18102094700005,12.2,1.20930074099999));
#310704=CARTESIAN_POINT('Ctrl Pts',(-4.18102094700005,5.2,1.20930074099999));
#310705=CARTESIAN_POINT('Ctrl Pts',(-4.18102094700005,2.2,1.20930074099999));
#310706=CARTESIAN_POINT('Ctrl Pts',(-4.18294049500005,12.2,1.20905400199999));
#310707=CARTESIAN_POINT('Ctrl Pts',(-4.18294049500005,5.2,1.20905400199999));
#310708=CARTESIAN_POINT('Ctrl Pts',(-4.18294049500005,2.2,1.20905400199999));
#310709=CARTESIAN_POINT('Ctrl Pts',(-4.18486388000006,12.2,1.20880458599999));
#310710=CARTESIAN_POINT('Ctrl Pts',(-4.18486388000006,5.2,1.20880458599999));
#310711=CARTESIAN_POINT('Ctrl Pts',(-4.18486388000006,2.2,1.20880458599999));
#310712=CARTESIAN_POINT('Ctrl Pts',(-4.18679109200006,12.2,1.20855248499999));
#310713=CARTESIAN_POINT('Ctrl Pts',(-4.18679109200006,5.2,1.20855248499999));
#310714=CARTESIAN_POINT('Ctrl Pts',(-4.18679109200006,2.2,1.20855248499999));
#310715=CARTESIAN_POINT('Ctrl Pts',(-4.18872212500006,12.2,1.20829769199998));
#310716=CARTESIAN_POINT('Ctrl Pts',(-4.18872212500006,5.2,1.20829769199998));
#310717=CARTESIAN_POINT('Ctrl Pts',(-4.18872212500006,2.2,1.20829769199998));
#310718=CARTESIAN_POINT('Ctrl Pts',(-4.19065696900006,12.2,1.20804020099999));
#310719=CARTESIAN_POINT('Ctrl Pts',(-4.19065696900006,5.2,1.20804020099999));
#310720=CARTESIAN_POINT('Ctrl Pts',(-4.19065696900006,2.2,1.20804020099999));
#310721=CARTESIAN_POINT('Ctrl Pts',(-4.19259561700006,12.2,1.20778000299998));
#310722=CARTESIAN_POINT('Ctrl Pts',(-4.19259561700006,5.2,1.20778000299998));
#310723=CARTESIAN_POINT('Ctrl Pts',(-4.19259561700006,2.2,1.20778000299998));
#310724=CARTESIAN_POINT('Ctrl Pts',(-4.19453805800006,12.2,1.20751709199999));
#310725=CARTESIAN_POINT('Ctrl Pts',(-4.19453805800006,5.2,1.20751709199999));
#310726=CARTESIAN_POINT('Ctrl Pts',(-4.19453805800006,2.2,1.20751709199999));
#310727=CARTESIAN_POINT('Ctrl Pts',(-4.19648428600006,12.2,1.20725145999999));
#310728=CARTESIAN_POINT('Ctrl Pts',(-4.19648428600006,5.2,1.20725145999999));
#310729=CARTESIAN_POINT('Ctrl Pts',(-4.19648428600006,2.2,1.20725145999999));
#310730=CARTESIAN_POINT('Ctrl Pts',(-4.19843429200006,12.2,1.20698310099999));
#310731=CARTESIAN_POINT('Ctrl Pts',(-4.19843429200006,5.2,1.20698310099999));
#310732=CARTESIAN_POINT('Ctrl Pts',(-4.19843429200006,2.2,1.20698310099999));
#310733=CARTESIAN_POINT('Ctrl Pts',(-4.20038806700005,12.2,1.20671200599999));
#310734=CARTESIAN_POINT('Ctrl Pts',(-4.20038806700005,5.2,1.20671200599999));
#310735=CARTESIAN_POINT('Ctrl Pts',(-4.20038806700005,2.2,1.20671200599999));
#310736=CARTESIAN_POINT('Ctrl Pts',(-4.20234560400006,12.2,1.20643816999999));
#310737=CARTESIAN_POINT('Ctrl Pts',(-4.20234560400006,5.2,1.20643816999999));
#310738=CARTESIAN_POINT('Ctrl Pts',(-4.20234560400006,2.2,1.20643816999999));
#310739=CARTESIAN_POINT('Ctrl Pts',(-4.20430689200006,12.2,1.20616158499999));
#310740=CARTESIAN_POINT('Ctrl Pts',(-4.20430689200006,5.2,1.20616158499999));
#310741=CARTESIAN_POINT('Ctrl Pts',(-4.20430689200006,2.2,1.20616158499999));
#310742=CARTESIAN_POINT('Ctrl Pts',(-4.20627192600006,12.2,1.20588224299999));
#310743=CARTESIAN_POINT('Ctrl Pts',(-4.20627192600006,5.2,1.20588224299999));
#310744=CARTESIAN_POINT('Ctrl Pts',(-4.20627192600006,2.2,1.20588224299999));
#310745=CARTESIAN_POINT('Ctrl Pts',(-4.20824069400005,12.2,1.20560013799999));
#310746=CARTESIAN_POINT('Ctrl Pts',(-4.20824069400005,5.2,1.20560013799999));
#310747=CARTESIAN_POINT('Ctrl Pts',(-4.20824069400005,2.2,1.20560013799999));
#310748=CARTESIAN_POINT('Ctrl Pts',(-4.21021319200006,12.2,1.20531526299999));
#310749=CARTESIAN_POINT('Ctrl Pts',(-4.21021319200006,5.2,1.20531526299999));
#310750=CARTESIAN_POINT('Ctrl Pts',(-4.21021319200006,2.2,1.20531526299999));
#310751=CARTESIAN_POINT('Ctrl Pts',(-4.21218940700006,12.2,1.20502761099999));
#310752=CARTESIAN_POINT('Ctrl Pts',(-4.21218940700006,5.2,1.20502761099999));
#310753=CARTESIAN_POINT('Ctrl Pts',(-4.21218940700006,2.2,1.20502761099999));
#310754=CARTESIAN_POINT('Ctrl Pts',(-4.21416933400006,12.2,1.20473717299999));
#310755=CARTESIAN_POINT('Ctrl Pts',(-4.21416933400006,5.2,1.20473717299999));
#310756=CARTESIAN_POINT('Ctrl Pts',(-4.21416933400006,2.2,1.20473717299999));
#310757=CARTESIAN_POINT('Ctrl Pts',(-4.21615296300006,12.2,1.20444394499998));
#310758=CARTESIAN_POINT('Ctrl Pts',(-4.21615296300006,5.2,1.20444394499998));
#310759=CARTESIAN_POINT('Ctrl Pts',(-4.21615296300006,2.2,1.20444394499998));
#310760=CARTESIAN_POINT('Ctrl Pts',(-4.21814028600005,12.2,1.20414791999998));
#310761=CARTESIAN_POINT('Ctrl Pts',(-4.21814028600005,5.2,1.20414791999998));
#310762=CARTESIAN_POINT('Ctrl Pts',(-4.21814028600005,2.2,1.20414791999998));
#310763=CARTESIAN_POINT('Ctrl Pts',(-4.22013129500006,12.2,1.20384908899998));
#310764=CARTESIAN_POINT('Ctrl Pts',(-4.22013129500006,5.2,1.20384908899998));
#310765=CARTESIAN_POINT('Ctrl Pts',(-4.22013129500006,2.2,1.20384908899998));
#310766=CARTESIAN_POINT('Ctrl Pts',(-4.22212598100006,12.2,1.20354744499998));
#310767=CARTESIAN_POINT('Ctrl Pts',(-4.22212598100006,5.2,1.20354744499998));
#310768=CARTESIAN_POINT('Ctrl Pts',(-4.22212598100006,2.2,1.20354744499998));
#310769=CARTESIAN_POINT('Ctrl Pts',(-4.22412433700006,12.2,1.20324298299999));
#310770=CARTESIAN_POINT('Ctrl Pts',(-4.22412433700006,5.2,1.20324298299999));
#310771=CARTESIAN_POINT('Ctrl Pts',(-4.22412433700006,2.2,1.20324298299999));
#310772=CARTESIAN_POINT('Ctrl Pts',(-4.22612635400006,12.2,1.20293569499998));
#310773=CARTESIAN_POINT('Ctrl Pts',(-4.22612635400006,5.2,1.20293569499998));
#310774=CARTESIAN_POINT('Ctrl Pts',(-4.22612635400006,2.2,1.20293569499998));
#310775=CARTESIAN_POINT('Ctrl Pts',(-4.22813202200006,12.2,1.20262557599998));
#310776=CARTESIAN_POINT('Ctrl Pts',(-4.22813202200006,5.2,1.20262557599998));
#310777=CARTESIAN_POINT('Ctrl Pts',(-4.22813202200006,2.2,1.20262557599998));
#310778=CARTESIAN_POINT('Ctrl Pts',(-4.23014133400006,12.2,1.20231261699999));
#310779=CARTESIAN_POINT('Ctrl Pts',(-4.23014133400006,5.2,1.20231261699999));
#310780=CARTESIAN_POINT('Ctrl Pts',(-4.23014133400006,2.2,1.20231261699999));
#310781=CARTESIAN_POINT('Ctrl Pts',(-4.23215428300006,12.2,1.20199681099999));
#310782=CARTESIAN_POINT('Ctrl Pts',(-4.23215428300006,5.2,1.20199681099999));
#310783=CARTESIAN_POINT('Ctrl Pts',(-4.23215428300006,2.2,1.20199681099999));
#310784=CARTESIAN_POINT('Ctrl Pts',(-4.23417085900006,12.2,1.20167815299999));
#310785=CARTESIAN_POINT('Ctrl Pts',(-4.23417085900006,5.2,1.20167815299999));
#310786=CARTESIAN_POINT('Ctrl Pts',(-4.23417085900006,2.2,1.20167815299999));
#310787=CARTESIAN_POINT('Ctrl Pts',(-4.23619105300006,12.2,1.20135663499998));
#310788=CARTESIAN_POINT('Ctrl Pts',(-4.23619105300006,5.2,1.20135663499998));
#310789=CARTESIAN_POINT('Ctrl Pts',(-4.23619105300006,2.2,1.20135663499998));
#310790=CARTESIAN_POINT('Ctrl Pts',(-4.23821485900006,12.2,1.20103224999998));
#310791=CARTESIAN_POINT('Ctrl Pts',(-4.23821485900006,5.2,1.20103224999998));
#310792=CARTESIAN_POINT('Ctrl Pts',(-4.23821485900006,2.2,1.20103224999998));
#310793=CARTESIAN_POINT('Ctrl Pts',(-4.24024226600006,12.2,1.20070499299999));
#310794=CARTESIAN_POINT('Ctrl Pts',(-4.24024226600006,5.2,1.20070499299999));
#310795=CARTESIAN_POINT('Ctrl Pts',(-4.24024226600006,2.2,1.20070499299999));
#310796=CARTESIAN_POINT('Ctrl Pts',(-4.24227326800006,12.2,1.20037485699998));
#310797=CARTESIAN_POINT('Ctrl Pts',(-4.24227326800006,5.2,1.20037485699998));
#310798=CARTESIAN_POINT('Ctrl Pts',(-4.24227326800006,2.2,1.20037485699998));
#310799=CARTESIAN_POINT('Ctrl Pts',(-4.24430785700006,12.2,1.20004183399999));
#310800=CARTESIAN_POINT('Ctrl Pts',(-4.24430785700006,5.2,1.20004183399999));
#310801=CARTESIAN_POINT('Ctrl Pts',(-4.24430785700006,2.2,1.20004183399999));
#310802=CARTESIAN_POINT('Ctrl Pts',(-4.24634602200006,12.2,1.19970591699999));
#310803=CARTESIAN_POINT('Ctrl Pts',(-4.24634602200006,5.2,1.19970591699999));
#310804=CARTESIAN_POINT('Ctrl Pts',(-4.24634602200006,2.2,1.19970591699999));
#310805=CARTESIAN_POINT('Ctrl Pts',(-4.24838775700006,12.2,1.19936710199998));
#310806=CARTESIAN_POINT('Ctrl Pts',(-4.24838775700006,5.2,1.19936710199998));
#310807=CARTESIAN_POINT('Ctrl Pts',(-4.24838775700006,2.2,1.19936710199998));
#310808=CARTESIAN_POINT('Ctrl Pts',(-4.25043305200006,12.2,1.19902537999999));
#310809=CARTESIAN_POINT('Ctrl Pts',(-4.25043305200006,5.2,1.19902537999999));
#310810=CARTESIAN_POINT('Ctrl Pts',(-4.25043305200006,2.2,1.19902537999999));
#310811=CARTESIAN_POINT('Ctrl Pts',(-4.25248190000006,12.2,1.19868074599998));
#310812=CARTESIAN_POINT('Ctrl Pts',(-4.25248190000006,5.2,1.19868074599998));
#310813=CARTESIAN_POINT('Ctrl Pts',(-4.25248190000006,2.2,1.19868074599998));
#310814=CARTESIAN_POINT('Ctrl Pts',(-4.25453429300005,12.2,1.19833319199998));
#310815=CARTESIAN_POINT('Ctrl Pts',(-4.25453429300005,5.2,1.19833319199998));
#310816=CARTESIAN_POINT('Ctrl Pts',(-4.25453429300005,2.2,1.19833319199998));
#310817=CARTESIAN_POINT('Ctrl Pts',(-4.25659022200006,12.2,1.19798271199999));
#310818=CARTESIAN_POINT('Ctrl Pts',(-4.25659022200006,5.2,1.19798271199999));
#310819=CARTESIAN_POINT('Ctrl Pts',(-4.25659022200006,2.2,1.19798271199999));
#310820=CARTESIAN_POINT('Ctrl Pts',(-4.25864967800006,12.2,1.19762930099998));
#310821=CARTESIAN_POINT('Ctrl Pts',(-4.25864967800006,5.2,1.19762930099998));
#310822=CARTESIAN_POINT('Ctrl Pts',(-4.25864967800006,2.2,1.19762930099998));
#310823=CARTESIAN_POINT('Ctrl Pts',(-4.26071265400005,12.2,1.19727295099999));
#310824=CARTESIAN_POINT('Ctrl Pts',(-4.26071265400005,5.2,1.19727295099999));
#310825=CARTESIAN_POINT('Ctrl Pts',(-4.26071265400005,2.2,1.19727295099999));
#310826=CARTESIAN_POINT('Ctrl Pts',(-4.26277914100006,12.2,1.19691365499999));
#310827=CARTESIAN_POINT('Ctrl Pts',(-4.26277914100006,5.2,1.19691365499999));
#310828=CARTESIAN_POINT('Ctrl Pts',(-4.26277914100006,2.2,1.19691365499999));
#310829=CARTESIAN_POINT('Ctrl Pts',(-4.26484913100006,12.2,1.19655140799999));
#310830=CARTESIAN_POINT('Ctrl Pts',(-4.26484913100006,5.2,1.19655140799999));
#310831=CARTESIAN_POINT('Ctrl Pts',(-4.26484913100006,2.2,1.19655140799999));
#310832=CARTESIAN_POINT('Ctrl Pts',(-4.26692261600006,12.2,1.19618620299998));
#310833=CARTESIAN_POINT('Ctrl Pts',(-4.26692261600006,5.2,1.19618620299998));
#310834=CARTESIAN_POINT('Ctrl Pts',(-4.26692261600006,2.2,1.19618620299998));
#310835=CARTESIAN_POINT('Ctrl Pts',(-4.26899958700006,12.2,1.19581803199999));
#310836=CARTESIAN_POINT('Ctrl Pts',(-4.26899958700006,5.2,1.19581803199999));
#310837=CARTESIAN_POINT('Ctrl Pts',(-4.26899958700006,2.2,1.19581803199999));
#310838=CARTESIAN_POINT('Ctrl Pts',(-4.27108003600006,12.2,1.19544689199999));
#310839=CARTESIAN_POINT('Ctrl Pts',(-4.27108003600006,5.2,1.19544689199999));
#310840=CARTESIAN_POINT('Ctrl Pts',(-4.27108003600006,2.2,1.19544689199999));
#310841=CARTESIAN_POINT('Ctrl Pts',(-4.27316395600006,12.2,1.19507277499999));
#310842=CARTESIAN_POINT('Ctrl Pts',(-4.27316395600006,5.2,1.19507277499999));
#310843=CARTESIAN_POINT('Ctrl Pts',(-4.27316395600006,2.2,1.19507277499999));
#310844=CARTESIAN_POINT('Ctrl Pts',(-4.27525133600006,12.2,1.19469567399999));
#310845=CARTESIAN_POINT('Ctrl Pts',(-4.27525133600006,5.2,1.19469567399999));
#310846=CARTESIAN_POINT('Ctrl Pts',(-4.27525133600006,2.2,1.19469567399999));
#310847=CARTESIAN_POINT('Ctrl Pts',(-4.27734217100006,12.2,1.19431558299999));
#310848=CARTESIAN_POINT('Ctrl Pts',(-4.27734217100006,5.2,1.19431558299999));
#310849=CARTESIAN_POINT('Ctrl Pts',(-4.27734217100006,2.2,1.19431558299999));
#310850=CARTESIAN_POINT('Ctrl Pts',(-4.27943645000005,12.2,1.19393249499999));
#310851=CARTESIAN_POINT('Ctrl Pts',(-4.27943645000005,5.2,1.19393249499999));
#310852=CARTESIAN_POINT('Ctrl Pts',(-4.27943645000005,2.2,1.19393249499999));
#310853=CARTESIAN_POINT('Ctrl Pts',(-4.28153416700006,12.2,1.19354640599999));
#310854=CARTESIAN_POINT('Ctrl Pts',(-4.28153416700006,5.2,1.19354640599999));
#310855=CARTESIAN_POINT('Ctrl Pts',(-4.28153416700006,2.2,1.19354640599999));
#310856=CARTESIAN_POINT('Ctrl Pts',(-4.28363531300006,12.2,1.19315730799999));
#310857=CARTESIAN_POINT('Ctrl Pts',(-4.28363531300006,5.2,1.19315730799999));
#310858=CARTESIAN_POINT('Ctrl Pts',(-4.28363531300006,2.2,1.19315730799999));
#310859=CARTESIAN_POINT('Ctrl Pts',(-4.28573987800006,12.2,1.19276519499998));
#310860=CARTESIAN_POINT('Ctrl Pts',(-4.28573987800006,5.2,1.19276519499998));
#310861=CARTESIAN_POINT('Ctrl Pts',(-4.28573987800006,2.2,1.19276519499998));
#310862=CARTESIAN_POINT('Ctrl Pts',(-4.28784785600006,12.2,1.19237006199999));
#310863=CARTESIAN_POINT('Ctrl Pts',(-4.28784785600006,5.2,1.19237006199999));
#310864=CARTESIAN_POINT('Ctrl Pts',(-4.28784785600006,2.2,1.19237006199999));
#310865=CARTESIAN_POINT('Ctrl Pts',(-4.28995923900006,12.2,1.19197189999999));
#310866=CARTESIAN_POINT('Ctrl Pts',(-4.28995923900006,5.2,1.19197189999999));
#310867=CARTESIAN_POINT('Ctrl Pts',(-4.28995923900006,2.2,1.19197189999999));
#310868=CARTESIAN_POINT('Ctrl Pts',(-4.29207401600006,12.2,1.19157070599998));
#310869=CARTESIAN_POINT('Ctrl Pts',(-4.29207401600006,5.2,1.19157070599998));
#310870=CARTESIAN_POINT('Ctrl Pts',(-4.29207401600006,2.2,1.19157070599998));
#310871=CARTESIAN_POINT('Ctrl Pts',(-4.29419218200006,12.2,1.19116647099998));
#310872=CARTESIAN_POINT('Ctrl Pts',(-4.29419218200006,5.2,1.19116647099998));
#310873=CARTESIAN_POINT('Ctrl Pts',(-4.29419218200006,2.2,1.19116647099998));
#310874=CARTESIAN_POINT('Ctrl Pts',(-4.29631372700006,12.2,1.19075919199998));
#310875=CARTESIAN_POINT('Ctrl Pts',(-4.29631372700006,5.2,1.19075919199998));
#310876=CARTESIAN_POINT('Ctrl Pts',(-4.29631372700006,2.2,1.19075919199998));
#310877=CARTESIAN_POINT('Ctrl Pts',(-4.29843864300006,12.2,1.19034885999998));
#310878=CARTESIAN_POINT('Ctrl Pts',(-4.29843864300006,5.2,1.19034885999998));
#310879=CARTESIAN_POINT('Ctrl Pts',(-4.29843864300006,2.2,1.19034885999998));
#310880=CARTESIAN_POINT('Ctrl Pts',(-4.30056692200006,12.2,1.18993547099999));
#310881=CARTESIAN_POINT('Ctrl Pts',(-4.30056692200006,5.2,1.18993547099999));
#310882=CARTESIAN_POINT('Ctrl Pts',(-4.30056692200006,2.2,1.18993547099999));
#310883=CARTESIAN_POINT('Ctrl Pts',(-4.30269855500006,12.2,1.18951901699999));
#310884=CARTESIAN_POINT('Ctrl Pts',(-4.30269855500006,5.2,1.18951901699999));
#310885=CARTESIAN_POINT('Ctrl Pts',(-4.30269855500006,2.2,1.18951901699999));
#310886=CARTESIAN_POINT('Ctrl Pts',(-4.30483353600006,12.2,1.18909949499999));
#310887=CARTESIAN_POINT('Ctrl Pts',(-4.30483353600006,5.2,1.18909949499999));
#310888=CARTESIAN_POINT('Ctrl Pts',(-4.30483353600006,2.2,1.18909949499999));
#310889=CARTESIAN_POINT('Ctrl Pts',(-4.30697185500006,12.2,1.18867689499998));
#310890=CARTESIAN_POINT('Ctrl Pts',(-4.30697185500006,5.2,1.18867689499998));
#310891=CARTESIAN_POINT('Ctrl Pts',(-4.30697185500006,2.2,1.18867689499998));
#310892=CARTESIAN_POINT('Ctrl Pts',(-4.30911350400006,12.2,1.18825121399999));
#310893=CARTESIAN_POINT('Ctrl Pts',(-4.30911350400006,5.2,1.18825121399999));
#310894=CARTESIAN_POINT('Ctrl Pts',(-4.30911350400006,2.2,1.18825121399999));
#310895=CARTESIAN_POINT('Ctrl Pts',(-4.31125847500006,12.2,1.18782244499998));
#310896=CARTESIAN_POINT('Ctrl Pts',(-4.31125847500006,5.2,1.18782244499998));
#310897=CARTESIAN_POINT('Ctrl Pts',(-4.31125847500006,2.2,1.18782244499998));
#310898=CARTESIAN_POINT('Ctrl Pts',(-4.31340675900006,12.2,1.18739058199999));
#310899=CARTESIAN_POINT('Ctrl Pts',(-4.31340675900006,5.2,1.18739058199999));
#310900=CARTESIAN_POINT('Ctrl Pts',(-4.31340675900006,2.2,1.18739058199999));
#310901=CARTESIAN_POINT('Ctrl Pts',(-4.31555834900006,12.2,1.18695561799999));
#310902=CARTESIAN_POINT('Ctrl Pts',(-4.31555834900006,5.2,1.18695561799999));
#310903=CARTESIAN_POINT('Ctrl Pts',(-4.31555834900006,2.2,1.18695561799999));
#310904=CARTESIAN_POINT('Ctrl Pts',(-4.31771323800006,12.2,1.18651754899998));
#310905=CARTESIAN_POINT('Ctrl Pts',(-4.31771323800006,5.2,1.18651754899998));
#310906=CARTESIAN_POINT('Ctrl Pts',(-4.31771323800006,2.2,1.18651754899998));
#310907=CARTESIAN_POINT('Ctrl Pts',(-4.31987141500006,12.2,1.18607636799998));
#310908=CARTESIAN_POINT('Ctrl Pts',(-4.31987141500006,5.2,1.18607636799998));
#310909=CARTESIAN_POINT('Ctrl Pts',(-4.31987141500006,2.2,1.18607636799998));
#310910=CARTESIAN_POINT('Ctrl Pts',(-4.32203287300006,12.2,1.18563207099998));
#310911=CARTESIAN_POINT('Ctrl Pts',(-4.32203287300006,5.2,1.18563207099998));
#310912=CARTESIAN_POINT('Ctrl Pts',(-4.32203287300006,2.2,1.18563207099998));
#310913=CARTESIAN_POINT('Ctrl Pts',(-4.32419760400006,12.2,1.18518464899998));
#310914=CARTESIAN_POINT('Ctrl Pts',(-4.32419760400006,5.2,1.18518464899998));
#310915=CARTESIAN_POINT('Ctrl Pts',(-4.32419760400006,2.2,1.18518464899998));
#310916=CARTESIAN_POINT('Ctrl Pts',(-4.32636560100006,12.2,1.18473409699998));
#310917=CARTESIAN_POINT('Ctrl Pts',(-4.32636560100006,5.2,1.18473409699998));
#310918=CARTESIAN_POINT('Ctrl Pts',(-4.32636560100006,2.2,1.18473409699998));
#310919=CARTESIAN_POINT('Ctrl Pts',(-4.32853685400006,12.2,1.18428041099999));
#310920=CARTESIAN_POINT('Ctrl Pts',(-4.32853685400006,5.2,1.18428041099999));
#310921=CARTESIAN_POINT('Ctrl Pts',(-4.32853685400006,2.2,1.18428041099999));
#310922=CARTESIAN_POINT('Ctrl Pts',(-4.33071135500006,12.2,1.18382358399999));
#310923=CARTESIAN_POINT('Ctrl Pts',(-4.33071135500006,5.2,1.18382358399999));
#310924=CARTESIAN_POINT('Ctrl Pts',(-4.33071135500006,2.2,1.18382358399999));
#310925=CARTESIAN_POINT('Ctrl Pts',(-4.33288909700006,12.2,1.18336361099999));
#310926=CARTESIAN_POINT('Ctrl Pts',(-4.33288909700006,5.2,1.18336361099999));
#310927=CARTESIAN_POINT('Ctrl Pts',(-4.33288909700006,2.2,1.18336361099999));
#310928=CARTESIAN_POINT('Ctrl Pts',(-4.33507007000006,12.2,1.18290048399999));
#310929=CARTESIAN_POINT('Ctrl Pts',(-4.33507007000006,5.2,1.18290048399999));
#310930=CARTESIAN_POINT('Ctrl Pts',(-4.33507007000006,2.2,1.18290048399999));
#310931=CARTESIAN_POINT('Ctrl Pts',(-4.33725426800006,12.2,1.18243419999999));
#310932=CARTESIAN_POINT('Ctrl Pts',(-4.33725426800006,5.2,1.18243419999999));
#310933=CARTESIAN_POINT('Ctrl Pts',(-4.33725426800006,2.2,1.18243419999999));
#310934=CARTESIAN_POINT('Ctrl Pts',(-4.33944168200005,12.2,1.18196475099999));
#310935=CARTESIAN_POINT('Ctrl Pts',(-4.33944168200005,5.2,1.18196475099999));
#310936=CARTESIAN_POINT('Ctrl Pts',(-4.33944168200005,2.2,1.18196475099999));
#310937=CARTESIAN_POINT('Ctrl Pts',(-4.34163230300006,12.2,1.18149213299999));
#310938=CARTESIAN_POINT('Ctrl Pts',(-4.34163230300006,5.2,1.18149213299999));
#310939=CARTESIAN_POINT('Ctrl Pts',(-4.34163230300006,2.2,1.18149213299999));
#310940=CARTESIAN_POINT('Ctrl Pts',(-4.34382612500006,12.2,1.18101633899999));
#310941=CARTESIAN_POINT('Ctrl Pts',(-4.34382612500006,5.2,1.18101633899999));
#310942=CARTESIAN_POINT('Ctrl Pts',(-4.34382612500006,2.2,1.18101633899999));
#310943=CARTESIAN_POINT('Ctrl Pts',(-4.34602313800006,12.2,1.18053736299998));
#310944=CARTESIAN_POINT('Ctrl Pts',(-4.34602313800006,5.2,1.18053736299998));
#310945=CARTESIAN_POINT('Ctrl Pts',(-4.34602313800006,2.2,1.18053736299998));
#310946=CARTESIAN_POINT('Ctrl Pts',(-4.34822333400006,12.2,1.18005520199999));
#310947=CARTESIAN_POINT('Ctrl Pts',(-4.34822333400006,5.2,1.18005520199999));
#310948=CARTESIAN_POINT('Ctrl Pts',(-4.34822333400006,2.2,1.18005520199999));
#310949=CARTESIAN_POINT('Ctrl Pts',(-4.35042670500006,12.2,1.17956984899998));
#310950=CARTESIAN_POINT('Ctrl Pts',(-4.35042670500006,5.2,1.17956984899998));
#310951=CARTESIAN_POINT('Ctrl Pts',(-4.35042670500006,2.2,1.17956984899998));
#310952=CARTESIAN_POINT('Ctrl Pts',(-4.35263324400006,12.2,1.17908129599999));
#310953=CARTESIAN_POINT('Ctrl Pts',(-4.35263324400006,5.2,1.17908129599999));
#310954=CARTESIAN_POINT('Ctrl Pts',(-4.35263324400006,2.2,1.17908129599999));
#310955=CARTESIAN_POINT('Ctrl Pts',(-4.35484294200006,12.2,1.17858954199999));
#310956=CARTESIAN_POINT('Ctrl Pts',(-4.35484294200006,5.2,1.17858954199999));
#310957=CARTESIAN_POINT('Ctrl Pts',(-4.35484294200006,2.2,1.17858954199999));
#310958=CARTESIAN_POINT('Ctrl Pts',(-4.35705579000006,12.2,1.17809457699999));
#310959=CARTESIAN_POINT('Ctrl Pts',(-4.35705579000006,5.2,1.17809457699999));
#310960=CARTESIAN_POINT('Ctrl Pts',(-4.35705579000006,2.2,1.17809457699999));
#310961=CARTESIAN_POINT('Ctrl Pts',(-4.35927178200005,12.2,1.17759639799999));
#310962=CARTESIAN_POINT('Ctrl Pts',(-4.35927178200005,5.2,1.17759639799999));
#310963=CARTESIAN_POINT('Ctrl Pts',(-4.35927178200005,2.2,1.17759639799999));
#310964=CARTESIAN_POINT('Ctrl Pts',(-4.36149090800006,12.2,1.17709499799998));
#310965=CARTESIAN_POINT('Ctrl Pts',(-4.36149090800006,5.2,1.17709499799998));
#310966=CARTESIAN_POINT('Ctrl Pts',(-4.36149090800006,2.2,1.17709499799998));
#310967=CARTESIAN_POINT('Ctrl Pts',(-4.36371316200006,12.2,1.17659037299998));
#310968=CARTESIAN_POINT('Ctrl Pts',(-4.36371316200006,5.2,1.17659037299998));
#310969=CARTESIAN_POINT('Ctrl Pts',(-4.36371316200006,2.2,1.17659037299998));
#310970=CARTESIAN_POINT('Ctrl Pts',(-4.36593853300006,12.2,1.17608251699998));
#310971=CARTESIAN_POINT('Ctrl Pts',(-4.36593853300006,5.2,1.17608251699998));
#310972=CARTESIAN_POINT('Ctrl Pts',(-4.36593853300006,2.2,1.17608251699998));
#310973=CARTESIAN_POINT('Ctrl Pts',(-4.36816701500006,12.2,1.17557142399999));
#310974=CARTESIAN_POINT('Ctrl Pts',(-4.36816701500006,5.2,1.17557142399999));
#310975=CARTESIAN_POINT('Ctrl Pts',(-4.36816701500006,2.2,1.17557142399999));
#310976=CARTESIAN_POINT('Ctrl Pts',(-4.37039860000006,12.2,1.17505708799999));
#310977=CARTESIAN_POINT('Ctrl Pts',(-4.37039860000006,5.2,1.17505708799999));
#310978=CARTESIAN_POINT('Ctrl Pts',(-4.37039860000006,2.2,1.17505708799999));
#310979=CARTESIAN_POINT('Ctrl Pts',(-4.37263327900006,12.2,1.17453950599999));
#310980=CARTESIAN_POINT('Ctrl Pts',(-4.37263327900006,5.2,1.17453950599999));
#310981=CARTESIAN_POINT('Ctrl Pts',(-4.37263327900006,2.2,1.17453950599999));
#310982=CARTESIAN_POINT('Ctrl Pts',(-4.37487104400006,12.2,1.17401866899999));
#310983=CARTESIAN_POINT('Ctrl Pts',(-4.37487104400006,5.2,1.17401866899999));
#310984=CARTESIAN_POINT('Ctrl Pts',(-4.37487104400006,2.2,1.17401866899999));
#310985=CARTESIAN_POINT('Ctrl Pts',(-4.37711188600006,12.2,1.17349457499999));
#310986=CARTESIAN_POINT('Ctrl Pts',(-4.37711188600006,5.2,1.17349457499999));
#310987=CARTESIAN_POINT('Ctrl Pts',(-4.37711188600006,2.2,1.17349457499999));
#310988=CARTESIAN_POINT('Ctrl Pts',(-4.37935580000006,12.2,1.17296721699998));
#310989=CARTESIAN_POINT('Ctrl Pts',(-4.37935580000006,5.2,1.17296721699998));
#310990=CARTESIAN_POINT('Ctrl Pts',(-4.37935580000006,2.2,1.17296721699998));
#310991=CARTESIAN_POINT('Ctrl Pts',(-4.38160277500006,12.2,1.17243658999998));
#310992=CARTESIAN_POINT('Ctrl Pts',(-4.38160277500006,5.2,1.17243658999998));
#310993=CARTESIAN_POINT('Ctrl Pts',(-4.38160277500006,2.2,1.17243658999998));
#310994=CARTESIAN_POINT('Ctrl Pts',(-4.38385280500006,12.2,1.17190268799999));
#310995=CARTESIAN_POINT('Ctrl Pts',(-4.38385280500006,5.2,1.17190268799999));
#310996=CARTESIAN_POINT('Ctrl Pts',(-4.38385280500006,2.2,1.17190268799999));
#310997=CARTESIAN_POINT('Ctrl Pts',(-4.38610588000006,12.2,1.17136550599998));
#310998=CARTESIAN_POINT('Ctrl Pts',(-4.38610588000006,5.2,1.17136550599998));
#310999=CARTESIAN_POINT('Ctrl Pts',(-4.38610588000006,2.2,1.17136550599998));
#311000=CARTESIAN_POINT('Ctrl Pts',(-4.38836199200006,12.2,1.17082503799999));
#311001=CARTESIAN_POINT('Ctrl Pts',(-4.38836199200006,5.2,1.17082503799999));
#311002=CARTESIAN_POINT('Ctrl Pts',(-4.38836199200006,2.2,1.17082503799999));
#311003=CARTESIAN_POINT('Ctrl Pts',(-4.39062113500006,12.2,1.17028128099999));
#311004=CARTESIAN_POINT('Ctrl Pts',(-4.39062113500006,5.2,1.17028128099999));
#311005=CARTESIAN_POINT('Ctrl Pts',(-4.39062113500006,2.2,1.17028128099999));
#311006=CARTESIAN_POINT('Ctrl Pts',(-4.39288330000006,12.2,1.16973422599999));
#311007=CARTESIAN_POINT('Ctrl Pts',(-4.39288330000006,5.2,1.16973422599999));
#311008=CARTESIAN_POINT('Ctrl Pts',(-4.39288330000006,2.2,1.16973422599999));
#311009=CARTESIAN_POINT('Ctrl Pts',(-4.39514847900006,12.2,1.16918387199998));
#311010=CARTESIAN_POINT('Ctrl Pts',(-4.39514847900006,5.2,1.16918387199998));
#311011=CARTESIAN_POINT('Ctrl Pts',(-4.39514847900006,2.2,1.16918387199998));
#311012=CARTESIAN_POINT('Ctrl Pts',(-4.39741666100006,12.2,1.16863021099999));
#311013=CARTESIAN_POINT('Ctrl Pts',(-4.39741666100006,5.2,1.16863021099999));
#311014=CARTESIAN_POINT('Ctrl Pts',(-4.39741666100006,2.2,1.16863021099999));
#311015=CARTESIAN_POINT('Ctrl Pts',(-4.39968784400006,12.2,1.16807323799998));
#311016=CARTESIAN_POINT('Ctrl Pts',(-4.39968784400006,5.2,1.16807323799998));
#311017=CARTESIAN_POINT('Ctrl Pts',(-4.39968784400006,2.2,1.16807323799998));
#311018=CARTESIAN_POINT('Ctrl Pts',(-4.40196201500005,12.2,1.16751294799998));
#311019=CARTESIAN_POINT('Ctrl Pts',(-4.40196201500005,5.2,1.16751294799998));
#311020=CARTESIAN_POINT('Ctrl Pts',(-4.40196201500005,2.2,1.16751294799998));
#311021=CARTESIAN_POINT('Ctrl Pts',(-4.40423916700006,12.2,1.16694933699999));
#311022=CARTESIAN_POINT('Ctrl Pts',(-4.40423916700006,5.2,1.16694933699999));
#311023=CARTESIAN_POINT('Ctrl Pts',(-4.40423916700006,2.2,1.16694933699999));
#311024=CARTESIAN_POINT('Ctrl Pts',(-4.40651929300006,12.2,1.16638239899999));
#311025=CARTESIAN_POINT('Ctrl Pts',(-4.40651929300006,5.2,1.16638239899999));
#311026=CARTESIAN_POINT('Ctrl Pts',(-4.40651929300006,2.2,1.16638239899999));
#311027=CARTESIAN_POINT('Ctrl Pts',(-4.40880238500006,12.2,1.16581212899999));
#311028=CARTESIAN_POINT('Ctrl Pts',(-4.40880238500006,5.2,1.16581212899999));
#311029=CARTESIAN_POINT('Ctrl Pts',(-4.40880238500006,2.2,1.16581212899999));
#311030=CARTESIAN_POINT('Ctrl Pts',(-4.41108843400006,12.2,1.16523851999998));
#311031=CARTESIAN_POINT('Ctrl Pts',(-4.41108843400006,5.2,1.16523851999998));
#311032=CARTESIAN_POINT('Ctrl Pts',(-4.41108843400006,2.2,1.16523851999998));
#311033=CARTESIAN_POINT('Ctrl Pts',(-4.41337743300006,12.2,1.16466156999998));
#311034=CARTESIAN_POINT('Ctrl Pts',(-4.41337743300006,5.2,1.16466156999998));
#311035=CARTESIAN_POINT('Ctrl Pts',(-4.41337743300006,2.2,1.16466156999998));
#311036=CARTESIAN_POINT('Ctrl Pts',(-4.41566937300006,12.2,1.16408127199998));
#311037=CARTESIAN_POINT('Ctrl Pts',(-4.41566937300006,5.2,1.16408127199998));
#311038=CARTESIAN_POINT('Ctrl Pts',(-4.41566937300006,2.2,1.16408127199998));
#311039=CARTESIAN_POINT('Ctrl Pts',(-4.41796424600006,12.2,1.16349762099999));
#311040=CARTESIAN_POINT('Ctrl Pts',(-4.41796424600006,5.2,1.16349762099999));
#311041=CARTESIAN_POINT('Ctrl Pts',(-4.41796424600006,2.2,1.16349762099999));
#311042=CARTESIAN_POINT('Ctrl Pts',(-4.42026204600006,12.2,1.16291061199998));
#311043=CARTESIAN_POINT('Ctrl Pts',(-4.42026204600006,5.2,1.16291061199998));
#311044=CARTESIAN_POINT('Ctrl Pts',(-4.42026204600006,2.2,1.16291061199998));
#311045=CARTESIAN_POINT('Ctrl Pts',(-4.42256276200006,12.2,1.16232024099999));
#311046=CARTESIAN_POINT('Ctrl Pts',(-4.42256276200006,5.2,1.16232024099999));
#311047=CARTESIAN_POINT('Ctrl Pts',(-4.42256276200006,2.2,1.16232024099999));
#311048=CARTESIAN_POINT('Ctrl Pts',(-4.42486638800006,12.2,1.16172650199998));
#311049=CARTESIAN_POINT('Ctrl Pts',(-4.42486638800006,5.2,1.16172650199998));
#311050=CARTESIAN_POINT('Ctrl Pts',(-4.42486638800006,2.2,1.16172650199998));
#311051=CARTESIAN_POINT('Ctrl Pts',(-4.42717291500006,12.2,1.16112938999999));
#311052=CARTESIAN_POINT('Ctrl Pts',(-4.42717291500006,5.2,1.16112938999999));
#311053=CARTESIAN_POINT('Ctrl Pts',(-4.42717291500006,2.2,1.16112938999999));
#311054=CARTESIAN_POINT('Ctrl Pts',(-4.42948233700006,12.2,1.16052889999999));
#311055=CARTESIAN_POINT('Ctrl Pts',(-4.42948233700006,5.2,1.16052889999999));
#311056=CARTESIAN_POINT('Ctrl Pts',(-4.42948233700006,2.2,1.16052889999999));
#311057=CARTESIAN_POINT('Ctrl Pts',(-4.43179464300006,12.2,1.15992502699998));
#311058=CARTESIAN_POINT('Ctrl Pts',(-4.43179464300006,5.2,1.15992502699998));
#311059=CARTESIAN_POINT('Ctrl Pts',(-4.43179464300006,2.2,1.15992502699998));
#311060=CARTESIAN_POINT('Ctrl Pts',(-4.43410982700006,12.2,1.15931776699998));
#311061=CARTESIAN_POINT('Ctrl Pts',(-4.43410982700006,5.2,1.15931776699998));
#311062=CARTESIAN_POINT('Ctrl Pts',(-4.43410982700006,2.2,1.15931776699998));
#311063=CARTESIAN_POINT('Ctrl Pts',(-4.43642788100005,12.2,1.15870711299999));
#311064=CARTESIAN_POINT('Ctrl Pts',(-4.43642788100005,5.2,1.15870711299999));
#311065=CARTESIAN_POINT('Ctrl Pts',(-4.43642788100005,2.2,1.15870711299999));
#311066=CARTESIAN_POINT('Ctrl Pts',(-4.43874879500005,12.2,1.15809306299999));
#311067=CARTESIAN_POINT('Ctrl Pts',(-4.43874879500005,5.2,1.15809306299999));
#311068=CARTESIAN_POINT('Ctrl Pts',(-4.43874879500005,2.2,1.15809306299999));
#311069=CARTESIAN_POINT('Ctrl Pts',(-4.44107256400006,12.2,1.15747560899999));
#311070=CARTESIAN_POINT('Ctrl Pts',(-4.44107256400006,5.2,1.15747560899999));
#311071=CARTESIAN_POINT('Ctrl Pts',(-4.44107256400006,2.2,1.15747560899999));
#311072=CARTESIAN_POINT('Ctrl Pts',(-4.44339917800006,12.2,1.15685474899998));
#311073=CARTESIAN_POINT('Ctrl Pts',(-4.44339917800006,5.2,1.15685474899998));
#311074=CARTESIAN_POINT('Ctrl Pts',(-4.44339917800006,2.2,1.15685474899998));
#311075=CARTESIAN_POINT('Ctrl Pts',(-4.44572863100006,12.2,1.15623047599998));
#311076=CARTESIAN_POINT('Ctrl Pts',(-4.44572863100006,5.2,1.15623047599998));
#311077=CARTESIAN_POINT('Ctrl Pts',(-4.44572863100006,2.2,1.15623047599998));
#311078=CARTESIAN_POINT('Ctrl Pts',(-4.44806091200006,12.2,1.15560278499999));
#311079=CARTESIAN_POINT('Ctrl Pts',(-4.44806091200006,5.2,1.15560278499999));
#311080=CARTESIAN_POINT('Ctrl Pts',(-4.44806091200006,2.2,1.15560278499999));
#311081=CARTESIAN_POINT('Ctrl Pts',(-4.45039601500006,12.2,1.15497167299999));
#311082=CARTESIAN_POINT('Ctrl Pts',(-4.45039601500006,5.2,1.15497167299999));
#311083=CARTESIAN_POINT('Ctrl Pts',(-4.45039601500006,2.2,1.15497167299999));
#311084=CARTESIAN_POINT('Ctrl Pts',(-4.45273393300006,12.2,1.15433713399999));
#311085=CARTESIAN_POINT('Ctrl Pts',(-4.45273393300006,5.2,1.15433713399999));
#311086=CARTESIAN_POINT('Ctrl Pts',(-4.45273393300006,2.2,1.15433713399999));
#311087=CARTESIAN_POINT('Ctrl Pts',(-4.45507465600006,12.2,1.15369916299999));
#311088=CARTESIAN_POINT('Ctrl Pts',(-4.45507465600006,5.2,1.15369916299999));
#311089=CARTESIAN_POINT('Ctrl Pts',(-4.45507465600006,2.2,1.15369916299999));
#311090=CARTESIAN_POINT('Ctrl Pts',(-4.45741817600006,12.2,1.15305775599999));
#311091=CARTESIAN_POINT('Ctrl Pts',(-4.45741817600006,5.2,1.15305775599999));
#311092=CARTESIAN_POINT('Ctrl Pts',(-4.45741817600006,2.2,1.15305775599999));
#311093=CARTESIAN_POINT('Ctrl Pts',(-4.45976448700006,12.2,1.15241290799998));
#311094=CARTESIAN_POINT('Ctrl Pts',(-4.45976448700006,5.2,1.15241290799998));
#311095=CARTESIAN_POINT('Ctrl Pts',(-4.45976448700006,2.2,1.15241290799998));
#311096=CARTESIAN_POINT('Ctrl Pts',(-4.46211358000006,12.2,1.15176461399999));
#311097=CARTESIAN_POINT('Ctrl Pts',(-4.46211358000006,5.2,1.15176461399999));
#311098=CARTESIAN_POINT('Ctrl Pts',(-4.46211358000006,2.2,1.15176461399999));
#311099=CARTESIAN_POINT('Ctrl Pts',(-4.46446544700006,12.2,1.15111286899999));
#311100=CARTESIAN_POINT('Ctrl Pts',(-4.46446544700006,5.2,1.15111286899999));
#311101=CARTESIAN_POINT('Ctrl Pts',(-4.46446544700006,2.2,1.15111286899999));
#311102=CARTESIAN_POINT('Ctrl Pts',(-4.46682008000006,12.2,1.15045766899998));
#311103=CARTESIAN_POINT('Ctrl Pts',(-4.46682008000006,5.2,1.15045766899998));
#311104=CARTESIAN_POINT('Ctrl Pts',(-4.46682008000006,2.2,1.15045766899998));
#311105=CARTESIAN_POINT('Ctrl Pts',(-4.46917747200006,12.2,1.14979900899999));
#311106=CARTESIAN_POINT('Ctrl Pts',(-4.46917747200006,5.2,1.14979900899999));
#311107=CARTESIAN_POINT('Ctrl Pts',(-4.46917747200006,2.2,1.14979900899999));
#311108=CARTESIAN_POINT('Ctrl Pts',(-4.47153761400005,12.2,1.14913688399998));
#311109=CARTESIAN_POINT('Ctrl Pts',(-4.47153761400005,5.2,1.14913688399998));
#311110=CARTESIAN_POINT('Ctrl Pts',(-4.47153761400005,2.2,1.14913688399998));
#311111=CARTESIAN_POINT('Ctrl Pts',(-4.47390049800005,12.2,1.14847128899998));
#311112=CARTESIAN_POINT('Ctrl Pts',(-4.47390049800005,5.2,1.14847128899998));
#311113=CARTESIAN_POINT('Ctrl Pts',(-4.47390049800005,2.2,1.14847128899998));
#311114=CARTESIAN_POINT('Ctrl Pts',(-4.47626611700006,12.2,1.14780221999998));
#311115=CARTESIAN_POINT('Ctrl Pts',(-4.47626611700006,5.2,1.14780221999998));
#311116=CARTESIAN_POINT('Ctrl Pts',(-4.47626611700006,2.2,1.14780221999998));
#311117=CARTESIAN_POINT('Ctrl Pts',(-4.47863446200006,12.2,1.14712967299999));
#311118=CARTESIAN_POINT('Ctrl Pts',(-4.47863446200006,5.2,1.14712967299999));
#311119=CARTESIAN_POINT('Ctrl Pts',(-4.47863446200006,2.2,1.14712967299999));
#311120=CARTESIAN_POINT('Ctrl Pts',(-4.48100552600006,12.2,1.14645364299998));
#311121=CARTESIAN_POINT('Ctrl Pts',(-4.48100552600006,5.2,1.14645364299998));
#311122=CARTESIAN_POINT('Ctrl Pts',(-4.48100552600006,2.2,1.14645364299998));
#311123=CARTESIAN_POINT('Ctrl Pts',(-4.48337930100006,12.2,1.14577412399999));
#311124=CARTESIAN_POINT('Ctrl Pts',(-4.48337930100006,5.2,1.14577412399999));
#311125=CARTESIAN_POINT('Ctrl Pts',(-4.48337930100006,2.2,1.14577412399999));
#311126=CARTESIAN_POINT('Ctrl Pts',(-4.48575577900006,12.2,1.14509111299999));
#311127=CARTESIAN_POINT('Ctrl Pts',(-4.48575577900006,5.2,1.14509111299999));
#311128=CARTESIAN_POINT('Ctrl Pts',(-4.48575577900006,2.2,1.14509111299999));
#311129=CARTESIAN_POINT('Ctrl Pts',(-4.48813495100006,12.2,1.14440460599999));
#311130=CARTESIAN_POINT('Ctrl Pts',(-4.48813495100006,5.2,1.14440460599999));
#311131=CARTESIAN_POINT('Ctrl Pts',(-4.48813495100006,2.2,1.14440460599999));
#311132=CARTESIAN_POINT('Ctrl Pts',(-4.49051681000006,12.2,1.14371459599999));
#311133=CARTESIAN_POINT('Ctrl Pts',(-4.49051681000006,5.2,1.14371459599999));
#311134=CARTESIAN_POINT('Ctrl Pts',(-4.49051681000006,2.2,1.14371459599999));
#311135=CARTESIAN_POINT('Ctrl Pts',(-4.49290134900005,12.2,1.14302107999999));
#311136=CARTESIAN_POINT('Ctrl Pts',(-4.49290134900005,5.2,1.14302107999999));
#311137=CARTESIAN_POINT('Ctrl Pts',(-4.49290134900005,2.2,1.14302107999999));
#311138=CARTESIAN_POINT('Ctrl Pts',(-4.49528855900006,12.2,1.14232405299999));
#311139=CARTESIAN_POINT('Ctrl Pts',(-4.49528855900006,5.2,1.14232405299999));
#311140=CARTESIAN_POINT('Ctrl Pts',(-4.49528855900006,2.2,1.14232405299999));
#311141=CARTESIAN_POINT('Ctrl Pts',(-4.49767843300005,12.2,1.14162351099999));
#311142=CARTESIAN_POINT('Ctrl Pts',(-4.49767843300005,5.2,1.14162351099999));
#311143=CARTESIAN_POINT('Ctrl Pts',(-4.49767843300005,2.2,1.14162351099999));
#311144=CARTESIAN_POINT('Ctrl Pts',(-4.50007096200006,12.2,1.14091944999998));
#311145=CARTESIAN_POINT('Ctrl Pts',(-4.50007096200006,5.2,1.14091944999998));
#311146=CARTESIAN_POINT('Ctrl Pts',(-4.50007096200006,2.2,1.14091944999998));
#311147=CARTESIAN_POINT('Ctrl Pts',(-4.50246613900006,12.2,1.14021186399999));
#311148=CARTESIAN_POINT('Ctrl Pts',(-4.50246613900006,5.2,1.14021186399999));
#311149=CARTESIAN_POINT('Ctrl Pts',(-4.50246613900006,2.2,1.14021186399999));
#311150=CARTESIAN_POINT('Ctrl Pts',(-4.50486395600006,12.2,1.13950074999998));
#311151=CARTESIAN_POINT('Ctrl Pts',(-4.50486395600006,5.2,1.13950074999998));
#311152=CARTESIAN_POINT('Ctrl Pts',(-4.50486395600006,2.2,1.13950074999998));
#311153=CARTESIAN_POINT('Ctrl Pts',(-4.50726440400006,12.2,1.13878610299999));
#311154=CARTESIAN_POINT('Ctrl Pts',(-4.50726440400006,5.2,1.13878610299999));
#311155=CARTESIAN_POINT('Ctrl Pts',(-4.50726440400006,2.2,1.13878610299999));
#311156=CARTESIAN_POINT('Ctrl Pts',(-4.50966747700006,12.2,1.13806791899998));
#311157=CARTESIAN_POINT('Ctrl Pts',(-4.50966747700006,5.2,1.13806791899998));
#311158=CARTESIAN_POINT('Ctrl Pts',(-4.50966747700006,2.2,1.13806791899998));
#311159=CARTESIAN_POINT('Ctrl Pts',(-4.51207316600006,12.2,1.13734619299999));
#311160=CARTESIAN_POINT('Ctrl Pts',(-4.51207316600006,5.2,1.13734619299999));
#311161=CARTESIAN_POINT('Ctrl Pts',(-4.51207316600006,2.2,1.13734619299999));
#311162=CARTESIAN_POINT('Ctrl Pts',(-4.51448146400006,12.2,1.13662091999998));
#311163=CARTESIAN_POINT('Ctrl Pts',(-4.51448146400006,5.2,1.13662091999998));
#311164=CARTESIAN_POINT('Ctrl Pts',(-4.51448146400006,2.2,1.13662091999998));
#311165=CARTESIAN_POINT('Ctrl Pts',(-4.51689236100006,12.2,1.13589209599999));
#311166=CARTESIAN_POINT('Ctrl Pts',(-4.51689236100006,5.2,1.13589209599999));
#311167=CARTESIAN_POINT('Ctrl Pts',(-4.51689236100006,2.2,1.13589209599999));
#311168=CARTESIAN_POINT('Ctrl Pts',(-4.51930585100006,12.2,1.13515971799998));
#311169=CARTESIAN_POINT('Ctrl Pts',(-4.51930585100006,5.2,1.13515971799998));
#311170=CARTESIAN_POINT('Ctrl Pts',(-4.51930585100006,2.2,1.13515971799998));
#311171=CARTESIAN_POINT('Ctrl Pts',(-4.52172192700006,12.2,1.13442378099998));
#311172=CARTESIAN_POINT('Ctrl Pts',(-4.52172192700006,5.2,1.13442378099998));
#311173=CARTESIAN_POINT('Ctrl Pts',(-4.52172192700006,2.2,1.13442378099998));
#311174=CARTESIAN_POINT('Ctrl Pts',(-4.52414057900006,12.2,1.13368427999998));
#311175=CARTESIAN_POINT('Ctrl Pts',(-4.52414057900006,5.2,1.13368427999998));
#311176=CARTESIAN_POINT('Ctrl Pts',(-4.52414057900006,2.2,1.13368427999998));
#311177=CARTESIAN_POINT('Ctrl Pts',(-4.52656180000006,12.2,1.13294121099999));
#311178=CARTESIAN_POINT('Ctrl Pts',(-4.52656180000006,5.2,1.13294121099999));
#311179=CARTESIAN_POINT('Ctrl Pts',(-4.52656180000006,2.2,1.13294121099999));
#311180=CARTESIAN_POINT('Ctrl Pts',(-4.52898558300006,12.2,1.13219456899999));
#311181=CARTESIAN_POINT('Ctrl Pts',(-4.52898558300006,5.2,1.13219456899999));
#311182=CARTESIAN_POINT('Ctrl Pts',(-4.52898558300006,2.2,1.13219456899999));
#311183=CARTESIAN_POINT('Ctrl Pts',(-4.53141191900006,12.2,1.13144435199999));
#311184=CARTESIAN_POINT('Ctrl Pts',(-4.53141191900006,5.2,1.13144435199999));
#311185=CARTESIAN_POINT('Ctrl Pts',(-4.53141191900006,2.2,1.13144435199999));
#311186=CARTESIAN_POINT('Ctrl Pts',(-4.53384080100006,12.2,1.13069055299999));
#311187=CARTESIAN_POINT('Ctrl Pts',(-4.53384080100006,5.2,1.13069055299999));
#311188=CARTESIAN_POINT('Ctrl Pts',(-4.53384080100006,2.2,1.13069055299999));
#311189=CARTESIAN_POINT('Ctrl Pts',(-4.53627222100006,12.2,1.12993316999999));
#311190=CARTESIAN_POINT('Ctrl Pts',(-4.53627222100006,5.2,1.12993316999999));
#311191=CARTESIAN_POINT('Ctrl Pts',(-4.53627222100006,2.2,1.12993316999999));
#311192=CARTESIAN_POINT('Ctrl Pts',(-4.53870617100006,12.2,1.12917219699999));
#311193=CARTESIAN_POINT('Ctrl Pts',(-4.53870617100006,5.2,1.12917219699999));
#311194=CARTESIAN_POINT('Ctrl Pts',(-4.53870617100006,2.2,1.12917219699999));
#311195=CARTESIAN_POINT('Ctrl Pts',(-4.54114264300006,12.2,1.12840763099999));
#311196=CARTESIAN_POINT('Ctrl Pts',(-4.54114264300006,5.2,1.12840763099999));
#311197=CARTESIAN_POINT('Ctrl Pts',(-4.54114264300006,2.2,1.12840763099999));
#311198=CARTESIAN_POINT('Ctrl Pts',(-4.54358163000006,12.2,1.12763946699999));
#311199=CARTESIAN_POINT('Ctrl Pts',(-4.54358163000006,5.2,1.12763946699999));
#311200=CARTESIAN_POINT('Ctrl Pts',(-4.54358163000006,2.2,1.12763946699999));
#311201=CARTESIAN_POINT('Ctrl Pts',(-4.54602312200006,12.2,1.12686770099999));
#311202=CARTESIAN_POINT('Ctrl Pts',(-4.54602312200006,5.2,1.12686770099999));
#311203=CARTESIAN_POINT('Ctrl Pts',(-4.54602312200006,2.2,1.12686770099999));
#311204=CARTESIAN_POINT('Ctrl Pts',(-4.54846711400006,12.2,1.12609232899999));
#311205=CARTESIAN_POINT('Ctrl Pts',(-4.54846711400006,5.2,1.12609232899999));
#311206=CARTESIAN_POINT('Ctrl Pts',(-4.54846711400006,2.2,1.12609232899999));
#311207=CARTESIAN_POINT('Ctrl Pts',(-4.55091359700006,12.2,1.12531334799999));
#311208=CARTESIAN_POINT('Ctrl Pts',(-4.55091359700006,5.2,1.12531334799999));
#311209=CARTESIAN_POINT('Ctrl Pts',(-4.55091359700006,2.2,1.12531334799999));
#311210=CARTESIAN_POINT('Ctrl Pts',(-4.55336256300006,12.2,1.12453075199999));
#311211=CARTESIAN_POINT('Ctrl Pts',(-4.55336256300006,5.2,1.12453075199999));
#311212=CARTESIAN_POINT('Ctrl Pts',(-4.55336256300006,2.2,1.12453075199999));
#311213=CARTESIAN_POINT('Ctrl Pts',(-4.55581400300006,12.2,1.12374453699998));
#311214=CARTESIAN_POINT('Ctrl Pts',(-4.55581400300006,5.2,1.12374453699998));
#311215=CARTESIAN_POINT('Ctrl Pts',(-4.55581400300006,2.2,1.12374453699998));
#311216=CARTESIAN_POINT('Ctrl Pts',(-4.55826791200006,12.2,1.12295469999999));
#311217=CARTESIAN_POINT('Ctrl Pts',(-4.55826791200006,5.2,1.12295469999999));
#311218=CARTESIAN_POINT('Ctrl Pts',(-4.55826791200006,2.2,1.12295469999999));
#311219=CARTESIAN_POINT('Ctrl Pts',(-4.56072428100006,12.2,1.12216123699998));
#311220=CARTESIAN_POINT('Ctrl Pts',(-4.56072428100006,5.2,1.12216123699998));
#311221=CARTESIAN_POINT('Ctrl Pts',(-4.56072428100006,2.2,1.12216123699998));
#311222=CARTESIAN_POINT('Ctrl Pts',(-4.56318310300006,12.2,1.12136414299998));
#311223=CARTESIAN_POINT('Ctrl Pts',(-4.56318310300006,5.2,1.12136414299998));
#311224=CARTESIAN_POINT('Ctrl Pts',(-4.56318310300006,2.2,1.12136414299998));
#311225=CARTESIAN_POINT('Ctrl Pts',(-4.56564436900006,12.2,1.12056341499999));
#311226=CARTESIAN_POINT('Ctrl Pts',(-4.56564436900006,5.2,1.12056341499999));
#311227=CARTESIAN_POINT('Ctrl Pts',(-4.56564436900006,2.2,1.12056341499999));
#311228=CARTESIAN_POINT('Ctrl Pts',(-4.56810807200006,12.2,1.11975904799999));
#311229=CARTESIAN_POINT('Ctrl Pts',(-4.56810807200006,5.2,1.11975904799999));
#311230=CARTESIAN_POINT('Ctrl Pts',(-4.56810807200006,2.2,1.11975904799999));
#311231=CARTESIAN_POINT('Ctrl Pts',(-4.57057420300006,12.2,1.11895103799998));
#311232=CARTESIAN_POINT('Ctrl Pts',(-4.57057420300006,5.2,1.11895103799998));
#311233=CARTESIAN_POINT('Ctrl Pts',(-4.57057420300006,2.2,1.11895103799998));
#311234=CARTESIAN_POINT('Ctrl Pts',(-4.57304275500006,12.2,1.11813938099999));
#311235=CARTESIAN_POINT('Ctrl Pts',(-4.57304275500006,5.2,1.11813938099999));
#311236=CARTESIAN_POINT('Ctrl Pts',(-4.57304275500006,2.2,1.11813938099999));
#311237=CARTESIAN_POINT('Ctrl Pts',(-4.57551371900006,12.2,1.11732407299999));
#311238=CARTESIAN_POINT('Ctrl Pts',(-4.57551371900006,5.2,1.11732407299999));
#311239=CARTESIAN_POINT('Ctrl Pts',(-4.57551371900006,2.2,1.11732407299999));
#311240=CARTESIAN_POINT('Ctrl Pts',(-4.57798708800006,12.2,1.11650510999999));
#311241=CARTESIAN_POINT('Ctrl Pts',(-4.57798708800006,5.2,1.11650510999999));
#311242=CARTESIAN_POINT('Ctrl Pts',(-4.57798708800006,2.2,1.11650510999999));
#311243=CARTESIAN_POINT('Ctrl Pts',(-4.58046285400005,12.2,1.11568248799998));
#311244=CARTESIAN_POINT('Ctrl Pts',(-4.58046285400005,5.2,1.11568248799998));
#311245=CARTESIAN_POINT('Ctrl Pts',(-4.58046285400005,2.2,1.11568248799998));
#311246=CARTESIAN_POINT('Ctrl Pts',(-4.58294100900006,12.2,1.11485620299999));
#311247=CARTESIAN_POINT('Ctrl Pts',(-4.58294100900006,5.2,1.11485620299999));
#311248=CARTESIAN_POINT('Ctrl Pts',(-4.58294100900006,2.2,1.11485620299999));
#311249=CARTESIAN_POINT('Ctrl Pts',(-4.58542154700006,12.2,1.11402625099998));
#311250=CARTESIAN_POINT('Ctrl Pts',(-4.58542154700006,5.2,1.11402625099998));
#311251=CARTESIAN_POINT('Ctrl Pts',(-4.58542154700006,2.2,1.11402625099998));
#311252=CARTESIAN_POINT('Ctrl Pts',(-4.58790446200006,12.2,1.11319262999999));
#311253=CARTESIAN_POINT('Ctrl Pts',(-4.58790446200006,5.2,1.11319262999999));
#311254=CARTESIAN_POINT('Ctrl Pts',(-4.58790446200006,2.2,1.11319262999999));
#311255=CARTESIAN_POINT('Ctrl Pts',(-4.59038974600006,12.2,1.11235533599999));
#311256=CARTESIAN_POINT('Ctrl Pts',(-4.59038974600006,5.2,1.11235533599999));
#311257=CARTESIAN_POINT('Ctrl Pts',(-4.59038974600006,2.2,1.11235533599999));
#311258=CARTESIAN_POINT('Ctrl Pts',(-4.59287739000006,12.2,1.11151436499998));
#311259=CARTESIAN_POINT('Ctrl Pts',(-4.59287739000006,5.2,1.11151436499998));
#311260=CARTESIAN_POINT('Ctrl Pts',(-4.59287739000006,2.2,1.11151436499998));
#311261=CARTESIAN_POINT('Ctrl Pts',(-4.59536738800006,12.2,1.11066971099998));
#311262=CARTESIAN_POINT('Ctrl Pts',(-4.59536738800006,5.2,1.11066971099998));
#311263=CARTESIAN_POINT('Ctrl Pts',(-4.59536738800006,2.2,1.11066971099998));
#311264=CARTESIAN_POINT('Ctrl Pts',(-4.59785972700006,12.2,1.10982137199999));
#311265=CARTESIAN_POINT('Ctrl Pts',(-4.59785972700006,5.2,1.10982137199999));
#311266=CARTESIAN_POINT('Ctrl Pts',(-4.59785972700006,2.2,1.10982137199999));
#311267=CARTESIAN_POINT('Ctrl Pts',(-4.60035440100006,12.2,1.10896934199999));
#311268=CARTESIAN_POINT('Ctrl Pts',(-4.60035440100006,5.2,1.10896934199999));
#311269=CARTESIAN_POINT('Ctrl Pts',(-4.60035440100006,2.2,1.10896934199999));
#311270=CARTESIAN_POINT('Ctrl Pts',(-4.60285139700006,12.2,1.10811361599998));
#311271=CARTESIAN_POINT('Ctrl Pts',(-4.60285139700006,5.2,1.10811361599998));
#311272=CARTESIAN_POINT('Ctrl Pts',(-4.60285139700006,2.2,1.10811361599998));
#311273=CARTESIAN_POINT('Ctrl Pts',(-4.60535071000006,12.2,1.10725418899999));
#311274=CARTESIAN_POINT('Ctrl Pts',(-4.60535071000006,5.2,1.10725418899999));
#311275=CARTESIAN_POINT('Ctrl Pts',(-4.60535071000006,2.2,1.10725418899999));
#311276=CARTESIAN_POINT('Ctrl Pts',(-4.60785233100006,12.2,1.10639105899998));
#311277=CARTESIAN_POINT('Ctrl Pts',(-4.60785233100006,5.2,1.10639105899998));
#311278=CARTESIAN_POINT('Ctrl Pts',(-4.60785233100006,2.2,1.10639105899998));
#311279=CARTESIAN_POINT('Ctrl Pts',(-4.61035625300006,12.2,1.10552422199999));
#311280=CARTESIAN_POINT('Ctrl Pts',(-4.61035625300006,5.2,1.10552422199999));
#311281=CARTESIAN_POINT('Ctrl Pts',(-4.61035625300006,2.2,1.10552422199999));
#311282=CARTESIAN_POINT('Ctrl Pts',(-4.61286247400006,12.2,1.10465367699998));
#311283=CARTESIAN_POINT('Ctrl Pts',(-4.61286247400006,5.2,1.10465367699998));
#311284=CARTESIAN_POINT('Ctrl Pts',(-4.61286247400006,2.2,1.10465367699998));
#311285=CARTESIAN_POINT('Ctrl Pts',(-4.61537099100005,12.2,1.10377942299999));
#311286=CARTESIAN_POINT('Ctrl Pts',(-4.61537099100005,5.2,1.10377942299999));
#311287=CARTESIAN_POINT('Ctrl Pts',(-4.61537099100005,2.2,1.10377942299999));
#311288=CARTESIAN_POINT('Ctrl Pts',(-4.61737964100006,12.2,1.10307705199999));
#311289=CARTESIAN_POINT('Ctrl Pts',(-4.61737964100006,5.2,1.10307705199999));
#311290=CARTESIAN_POINT('Ctrl Pts',(-4.61737964100006,2.2,1.10307705199999));
#311291=CARTESIAN_POINT('Ctrl Pts',(-4.61888716100006,12.2,1.10254860399999));
#311292=CARTESIAN_POINT('Ctrl Pts',(-4.61888716100006,5.2,1.10254860399999));
#311293=CARTESIAN_POINT('Ctrl Pts',(-4.61888716100006,2.2,1.10254860399999));
#311294=CARTESIAN_POINT('Ctrl Pts',(-4.61989263400006,12.2,1.10219556399999));
#311295=CARTESIAN_POINT('Ctrl Pts',(-4.61989263400006,5.2,1.10219556399999));
#311296=CARTESIAN_POINT('Ctrl Pts',(-4.61989263400006,2.2,1.10219556399999));
#311297=CARTESIAN_POINT('Ctrl Pts',(-4.62039548500006,12.2,1.10201885899999));
#311298=CARTESIAN_POINT('Ctrl Pts',(-4.62039548500006,5.2,1.10201885899999));
#311299=CARTESIAN_POINT('Ctrl Pts',(-4.62039548500006,2.2,1.10201885899999));
#311300=CARTESIAN_POINT('',(-4.62039548500006,2.7,1.10201885899999));
#311301=CARTESIAN_POINT('',(-4.62039548500006,12.2,1.10201885899999));
#311302=CARTESIAN_POINT('Ctrl Pts',(-3.80828031400006,2.7,1.20296984599999));
#311303=CARTESIAN_POINT('Ctrl Pts',(-3.80845769136914,2.7,1.20302512565856));
#311304=CARTESIAN_POINT('Ctrl Pts',(-3.81014983883408,2.7,1.20354748054386));
#311305=CARTESIAN_POINT('Ctrl Pts',(-3.81751691756265,2.7,1.20546182228747));
#311306=CARTESIAN_POINT('Ctrl Pts',(-3.82198099636819,2.7,1.20648710942369));
#311307=CARTESIAN_POINT('Ctrl Pts',(-3.84154121060164,2.7,1.21064530016897));
#311308=CARTESIAN_POINT('Ctrl Pts',(-3.85807057032119,2.7,1.21321507966715));
#311309=CARTESIAN_POINT('Ctrl Pts',(-3.91840592137738,2.7,1.22066908254686));
#311310=CARTESIAN_POINT('Ctrl Pts',(-3.97606115021901,2.7,1.22367498425562));
#311311=CARTESIAN_POINT('Ctrl Pts',(-4.17888715549711,2.7,1.21549033946434));
#311312=CARTESIAN_POINT('Ctrl Pts',(-4.3738307801898,2.7,1.1886632450385));
#311313=CARTESIAN_POINT('Ctrl Pts',(-4.62039548500006,2.7,1.10201885899999));
#311314=CARTESIAN_POINT('Origin',(-5.66300478732629E-14,15.2,-1.77635683940025E-14));
#311315=CARTESIAN_POINT('',(-4.68689806900006,2.7,0.771677711999986));
#311316=CARTESIAN_POINT('',(-4.68689806900006,12.2,0.771677711999987));
#311317=CARTESIAN_POINT('Origin',(-5.66300478732629E-14,2.7,-1.92943768261394E-14));
#311318=CARTESIAN_POINT('Ctrl Pts',(-4.68689806900006,12.2,0.771677711999987));
#311319=CARTESIAN_POINT('Ctrl Pts',(-4.68689806900006,5.2,0.771677711999987));
#311320=CARTESIAN_POINT('Ctrl Pts',(-4.68689806900006,2.2,0.771677711999987));
#311321=CARTESIAN_POINT('Ctrl Pts',(-4.68650276500005,12.2,0.771320194999987));
#311322=CARTESIAN_POINT('Ctrl Pts',(-4.68650276500005,5.2,0.771320194999987));
#311323=CARTESIAN_POINT('Ctrl Pts',(-4.68650276500005,2.2,0.771320194999987));
#311324=CARTESIAN_POINT('Ctrl Pts',(-4.68571222500006,12.2,0.770605589999986));
#311325=CARTESIAN_POINT('Ctrl Pts',(-4.68571222500006,5.2,0.770605589999986));
#311326=CARTESIAN_POINT('Ctrl Pts',(-4.68571222500006,2.2,0.770605589999986));
#311327=CARTESIAN_POINT('Ctrl Pts',(-4.68452662000006,12.2,0.769534975999986));
#311328=CARTESIAN_POINT('Ctrl Pts',(-4.68452662000006,5.2,0.769534975999986));
#311329=CARTESIAN_POINT('Ctrl Pts',(-4.68452662000006,2.2,0.769534975999986));
#311330=CARTESIAN_POINT('Ctrl Pts',(-4.68294622100006,12.2,0.768110075999986));
#311331=CARTESIAN_POINT('Ctrl Pts',(-4.68294622100006,5.2,0.768110075999986));
#311332=CARTESIAN_POINT('Ctrl Pts',(-4.68294622100006,2.2,0.768110075999986));
#311333=CARTESIAN_POINT('Ctrl Pts',(-4.68097140300006,12.2,0.766333260999983));
#311334=CARTESIAN_POINT('Ctrl Pts',(-4.68097140300006,5.2,0.766333260999983));
#311335=CARTESIAN_POINT('Ctrl Pts',(-4.68097140300006,2.2,0.766333260999983));
#311336=CARTESIAN_POINT('Ctrl Pts',(-4.67899726800006,12.2,0.764560752999985));
#311337=CARTESIAN_POINT('Ctrl Pts',(-4.67899726800006,5.2,0.764560752999985));
#311338=CARTESIAN_POINT('Ctrl Pts',(-4.67899726800006,2.2,0.764560752999985));
#311339=CARTESIAN_POINT('Ctrl Pts',(-4.67702381800006,12.2,0.762792554999985));
#311340=CARTESIAN_POINT('Ctrl Pts',(-4.67702381800006,5.2,0.762792554999985));
#311341=CARTESIAN_POINT('Ctrl Pts',(-4.67702381800006,2.2,0.762792554999985));
#311342=CARTESIAN_POINT('Ctrl Pts',(-4.67505105600006,12.2,0.761028664999985));
#311343=CARTESIAN_POINT('Ctrl Pts',(-4.67505105600006,5.2,0.761028664999985));
#311344=CARTESIAN_POINT('Ctrl Pts',(-4.67505105600006,2.2,0.761028664999985));
#311345=CARTESIAN_POINT('Ctrl Pts',(-4.67307898900006,12.2,0.759269083999987));
#311346=CARTESIAN_POINT('Ctrl Pts',(-4.67307898900006,5.2,0.759269083999987));
#311347=CARTESIAN_POINT('Ctrl Pts',(-4.67307898900006,2.2,0.759269083999987));
#311348=CARTESIAN_POINT('Ctrl Pts',(-4.67110762500006,12.2,0.757513809999986));
#311349=CARTESIAN_POINT('Ctrl Pts',(-4.67110762500006,5.2,0.757513809999986));
#311350=CARTESIAN_POINT('Ctrl Pts',(-4.67110762500006,2.2,0.757513809999986));
#311351=CARTESIAN_POINT('Ctrl Pts',(-4.66913697300006,12.2,0.755762842999985));
#311352=CARTESIAN_POINT('Ctrl Pts',(-4.66913697300006,5.2,0.755762842999985));
#311353=CARTESIAN_POINT('Ctrl Pts',(-4.66913697300006,2.2,0.755762842999985));
#311354=CARTESIAN_POINT('Ctrl Pts',(-4.66716704600006,12.2,0.754016181999986));
#311355=CARTESIAN_POINT('Ctrl Pts',(-4.66716704600006,5.2,0.754016181999986));
#311356=CARTESIAN_POINT('Ctrl Pts',(-4.66716704600006,2.2,0.754016181999986));
#311357=CARTESIAN_POINT('Ctrl Pts',(-4.66519785100005,12.2,0.752273827999983));
#311358=CARTESIAN_POINT('Ctrl Pts',(-4.66519785100005,5.2,0.752273827999983));
#311359=CARTESIAN_POINT('Ctrl Pts',(-4.66519785100005,2.2,0.752273827999983));
#311360=CARTESIAN_POINT('Ctrl Pts',(-4.66322940300006,12.2,0.750535778999986));
#311361=CARTESIAN_POINT('Ctrl Pts',(-4.66322940300006,5.2,0.750535778999986));
#311362=CARTESIAN_POINT('Ctrl Pts',(-4.66322940300006,2.2,0.750535778999986));
#311363=CARTESIAN_POINT('Ctrl Pts',(-4.66126170700006,12.2,0.748802032999984));
#311364=CARTESIAN_POINT('Ctrl Pts',(-4.66126170700006,5.2,0.748802032999984));
#311365=CARTESIAN_POINT('Ctrl Pts',(-4.66126170700006,2.2,0.748802032999984));
#311366=CARTESIAN_POINT('Ctrl Pts',(-4.65929477500006,12.2,0.747072591999984));
#311367=CARTESIAN_POINT('Ctrl Pts',(-4.65929477500006,5.2,0.747072591999984));
#311368=CARTESIAN_POINT('Ctrl Pts',(-4.65929477500006,2.2,0.747072591999984));
#311369=CARTESIAN_POINT('Ctrl Pts',(-4.65732861400006,12.2,0.745347453999985));
#311370=CARTESIAN_POINT('Ctrl Pts',(-4.65732861400006,5.2,0.745347453999985));
#311371=CARTESIAN_POINT('Ctrl Pts',(-4.65732861400006,2.2,0.745347453999985));
#311372=CARTESIAN_POINT('Ctrl Pts',(-4.65536323200006,12.2,0.743626618999986));
#311373=CARTESIAN_POINT('Ctrl Pts',(-4.65536323200006,5.2,0.743626618999986));
#311374=CARTESIAN_POINT('Ctrl Pts',(-4.65536323200006,2.2,0.743626618999986));
#311375=CARTESIAN_POINT('Ctrl Pts',(-4.65339863500006,12.2,0.741910085999984));
#311376=CARTESIAN_POINT('Ctrl Pts',(-4.65339863500006,5.2,0.741910085999984));
#311377=CARTESIAN_POINT('Ctrl Pts',(-4.65339863500006,2.2,0.741910085999984));
#311378=CARTESIAN_POINT('Ctrl Pts',(-4.65143483400006,12.2,0.740197854999987));
#311379=CARTESIAN_POINT('Ctrl Pts',(-4.65143483400006,5.2,0.740197854999987));
#311380=CARTESIAN_POINT('Ctrl Pts',(-4.65143483400006,2.2,0.740197854999987));
#311381=CARTESIAN_POINT('Ctrl Pts',(-4.64947183500006,12.2,0.738489923999985));
#311382=CARTESIAN_POINT('Ctrl Pts',(-4.64947183500006,5.2,0.738489923999985));
#311383=CARTESIAN_POINT('Ctrl Pts',(-4.64947183500006,2.2,0.738489923999985));
#311384=CARTESIAN_POINT('Ctrl Pts',(-4.64750964800006,12.2,0.736786292999985));
#311385=CARTESIAN_POINT('Ctrl Pts',(-4.64750964800006,5.2,0.736786292999985));
#311386=CARTESIAN_POINT('Ctrl Pts',(-4.64750964800006,2.2,0.736786292999985));
#311387=CARTESIAN_POINT('Ctrl Pts',(-4.64554828100006,12.2,0.735086962999985));
#311388=CARTESIAN_POINT('Ctrl Pts',(-4.64554828100006,5.2,0.735086962999985));
#311389=CARTESIAN_POINT('Ctrl Pts',(-4.64554828100006,2.2,0.735086962999985));
#311390=CARTESIAN_POINT('Ctrl Pts',(-4.64358774500006,12.2,0.733391930999985));
#311391=CARTESIAN_POINT('Ctrl Pts',(-4.64358774500006,5.2,0.733391930999985));
#311392=CARTESIAN_POINT('Ctrl Pts',(-4.64358774500006,2.2,0.733391930999985));
#311393=CARTESIAN_POINT('Ctrl Pts',(-4.64162804700006,12.2,0.731701195999985));
#311394=CARTESIAN_POINT('Ctrl Pts',(-4.64162804700006,5.2,0.731701195999985));
#311395=CARTESIAN_POINT('Ctrl Pts',(-4.64162804700006,2.2,0.731701195999985));
#311396=CARTESIAN_POINT('Ctrl Pts',(-4.63966919700006,12.2,0.730014758999986));
#311397=CARTESIAN_POINT('Ctrl Pts',(-4.63966919700006,5.2,0.730014758999986));
#311398=CARTESIAN_POINT('Ctrl Pts',(-4.63966919700006,2.2,0.730014758999986));
#311399=CARTESIAN_POINT('Ctrl Pts',(-4.63771120400006,12.2,0.728332618999987));
#311400=CARTESIAN_POINT('Ctrl Pts',(-4.63771120400006,5.2,0.728332618999987));
#311401=CARTESIAN_POINT('Ctrl Pts',(-4.63771120400006,2.2,0.728332618999987));
#311402=CARTESIAN_POINT('Ctrl Pts',(-4.63575407600006,12.2,0.726654774999984));
#311403=CARTESIAN_POINT('Ctrl Pts',(-4.63575407600006,5.2,0.726654774999984));
#311404=CARTESIAN_POINT('Ctrl Pts',(-4.63575407600006,2.2,0.726654774999984));
#311405=CARTESIAN_POINT('Ctrl Pts',(-4.63379782200006,12.2,0.724981225999985));
#311406=CARTESIAN_POINT('Ctrl Pts',(-4.63379782200006,5.2,0.724981225999985));
#311407=CARTESIAN_POINT('Ctrl Pts',(-4.63379782200006,2.2,0.724981225999985));
#311408=CARTESIAN_POINT('Ctrl Pts',(-4.63184245000006,12.2,0.723311970999987));
#311409=CARTESIAN_POINT('Ctrl Pts',(-4.63184245000006,5.2,0.723311970999987));
#311410=CARTESIAN_POINT('Ctrl Pts',(-4.63184245000006,2.2,0.723311970999987));
#311411=CARTESIAN_POINT('Ctrl Pts',(-4.62988797000006,12.2,0.721647009999984));
#311412=CARTESIAN_POINT('Ctrl Pts',(-4.62988797000006,5.2,0.721647009999984));
#311413=CARTESIAN_POINT('Ctrl Pts',(-4.62988797000006,2.2,0.721647009999984));
#311414=CARTESIAN_POINT('Ctrl Pts',(-4.62793439000006,12.2,0.719986340999985));
#311415=CARTESIAN_POINT('Ctrl Pts',(-4.62793439000006,5.2,0.719986340999985));
#311416=CARTESIAN_POINT('Ctrl Pts',(-4.62793439000006,2.2,0.719986340999985));
#311417=CARTESIAN_POINT('Ctrl Pts',(-4.62598171700006,12.2,0.718329964999986));
#311418=CARTESIAN_POINT('Ctrl Pts',(-4.62598171700006,5.2,0.718329964999986));
#311419=CARTESIAN_POINT('Ctrl Pts',(-4.62598171700006,2.2,0.718329964999986));
#311420=CARTESIAN_POINT('Ctrl Pts',(-4.62402996300006,12.2,0.716677880999987));
#311421=CARTESIAN_POINT('Ctrl Pts',(-4.62402996300006,5.2,0.716677880999987));
#311422=CARTESIAN_POINT('Ctrl Pts',(-4.62402996300006,2.2,0.716677880999987));
#311423=CARTESIAN_POINT('Ctrl Pts',(-4.62207913600006,12.2,0.715030085999988));
#311424=CARTESIAN_POINT('Ctrl Pts',(-4.62207913600006,5.2,0.715030085999988));
#311425=CARTESIAN_POINT('Ctrl Pts',(-4.62207913600006,2.2,0.715030085999988));
#311426=CARTESIAN_POINT('Ctrl Pts',(-4.62012924300006,12.2,0.713386579999984));
#311427=CARTESIAN_POINT('Ctrl Pts',(-4.62012924300006,5.2,0.713386579999984));
#311428=CARTESIAN_POINT('Ctrl Pts',(-4.62012924300006,2.2,0.713386579999984));
#311429=CARTESIAN_POINT('Ctrl Pts',(-4.61818029300006,12.2,0.711747362999984));
#311430=CARTESIAN_POINT('Ctrl Pts',(-4.61818029300006,5.2,0.711747362999984));
#311431=CARTESIAN_POINT('Ctrl Pts',(-4.61818029300006,2.2,0.711747362999984));
#311432=CARTESIAN_POINT('Ctrl Pts',(-4.61623229800006,12.2,0.710112433999988));
#311433=CARTESIAN_POINT('Ctrl Pts',(-4.61623229800006,5.2,0.710112433999988));
#311434=CARTESIAN_POINT('Ctrl Pts',(-4.61623229800006,2.2,0.710112433999988));
#311435=CARTESIAN_POINT('Ctrl Pts',(-4.61428526400006,12.2,0.708481791999986));
#311436=CARTESIAN_POINT('Ctrl Pts',(-4.61428526400006,5.2,0.708481791999986));
#311437=CARTESIAN_POINT('Ctrl Pts',(-4.61428526400006,2.2,0.708481791999986));
#311438=CARTESIAN_POINT('Ctrl Pts',(-4.61233920200006,12.2,0.706855434999984));
#311439=CARTESIAN_POINT('Ctrl Pts',(-4.61233920200006,5.2,0.706855434999984));
#311440=CARTESIAN_POINT('Ctrl Pts',(-4.61233920200006,2.2,0.706855434999984));
#311441=CARTESIAN_POINT('Ctrl Pts',(-4.61039411800006,12.2,0.705233363999986));
#311442=CARTESIAN_POINT('Ctrl Pts',(-4.61039411800006,5.2,0.705233363999986));
#311443=CARTESIAN_POINT('Ctrl Pts',(-4.61039411800006,2.2,0.705233363999986));
#311444=CARTESIAN_POINT('Ctrl Pts',(-4.60845002300006,12.2,0.703615577999983));
#311445=CARTESIAN_POINT('Ctrl Pts',(-4.60845002300006,5.2,0.703615577999983));
#311446=CARTESIAN_POINT('Ctrl Pts',(-4.60845002300006,2.2,0.703615577999983));
#311447=CARTESIAN_POINT('Ctrl Pts',(-4.60650692500006,12.2,0.702002073999988));
#311448=CARTESIAN_POINT('Ctrl Pts',(-4.60650692500006,5.2,0.702002073999988));
#311449=CARTESIAN_POINT('Ctrl Pts',(-4.60650692500006,2.2,0.702002073999988));
#311450=CARTESIAN_POINT('Ctrl Pts',(-4.60456483400006,12.2,0.700392851999982));
#311451=CARTESIAN_POINT('Ctrl Pts',(-4.60456483400006,5.2,0.700392851999982));
#311452=CARTESIAN_POINT('Ctrl Pts',(-4.60456483400006,2.2,0.700392851999982));
#311453=CARTESIAN_POINT('Ctrl Pts',(-4.60262375700006,12.2,0.698787911999985));
#311454=CARTESIAN_POINT('Ctrl Pts',(-4.60262375700006,5.2,0.698787911999985));
#311455=CARTESIAN_POINT('Ctrl Pts',(-4.60262375700006,2.2,0.698787911999985));
#311456=CARTESIAN_POINT('Ctrl Pts',(-4.60068370500006,12.2,0.697187250999987));
#311457=CARTESIAN_POINT('Ctrl Pts',(-4.60068370500006,5.2,0.697187250999987));
#311458=CARTESIAN_POINT('Ctrl Pts',(-4.60068370500006,2.2,0.697187250999987));
#311459=CARTESIAN_POINT('Ctrl Pts',(-4.59874468500006,12.2,0.695590870999983));
#311460=CARTESIAN_POINT('Ctrl Pts',(-4.59874468500006,5.2,0.695590870999983));
#311461=CARTESIAN_POINT('Ctrl Pts',(-4.59874468500006,2.2,0.695590870999983));
#311462=CARTESIAN_POINT('Ctrl Pts',(-4.59680670800005,12.2,0.693998767999986));
#311463=CARTESIAN_POINT('Ctrl Pts',(-4.59680670800005,5.2,0.693998767999986));
#311464=CARTESIAN_POINT('Ctrl Pts',(-4.59680670800005,2.2,0.693998767999986));
#311465=CARTESIAN_POINT('Ctrl Pts',(-4.59486978100006,12.2,0.692410942999988));
#311466=CARTESIAN_POINT('Ctrl Pts',(-4.59486978100006,5.2,0.692410942999988));
#311467=CARTESIAN_POINT('Ctrl Pts',(-4.59486978100006,2.2,0.692410942999988));
#311468=CARTESIAN_POINT('Ctrl Pts',(-4.59293391500006,12.2,0.690827393999989));
#311469=CARTESIAN_POINT('Ctrl Pts',(-4.59293391500006,5.2,0.690827393999989));
#311470=CARTESIAN_POINT('Ctrl Pts',(-4.59293391500006,2.2,0.690827393999989));
#311471=CARTESIAN_POINT('Ctrl Pts',(-4.59099911700006,12.2,0.689248119999988));
#311472=CARTESIAN_POINT('Ctrl Pts',(-4.59099911700006,5.2,0.689248119999988));
#311473=CARTESIAN_POINT('Ctrl Pts',(-4.59099911700006,2.2,0.689248119999988));
#311474=CARTESIAN_POINT('Ctrl Pts',(-4.58906539600005,12.2,0.687673120999985));
#311475=CARTESIAN_POINT('Ctrl Pts',(-4.58906539600005,5.2,0.687673120999985));
#311476=CARTESIAN_POINT('Ctrl Pts',(-4.58906539600005,2.2,0.687673120999985));
#311477=CARTESIAN_POINT('Ctrl Pts',(-4.58713276200006,12.2,0.686102393999986));
#311478=CARTESIAN_POINT('Ctrl Pts',(-4.58713276200006,5.2,0.686102393999986));
#311479=CARTESIAN_POINT('Ctrl Pts',(-4.58713276200006,2.2,0.686102393999986));
#311480=CARTESIAN_POINT('Ctrl Pts',(-4.58520122500006,12.2,0.684535938999984));
#311481=CARTESIAN_POINT('Ctrl Pts',(-4.58520122500006,5.2,0.684535938999984));
#311482=CARTESIAN_POINT('Ctrl Pts',(-4.58520122500006,2.2,0.684535938999984));
#311483=CARTESIAN_POINT('Ctrl Pts',(-4.58327079200005,12.2,0.682973754999985));
#311484=CARTESIAN_POINT('Ctrl Pts',(-4.58327079200005,5.2,0.682973754999985));
#311485=CARTESIAN_POINT('Ctrl Pts',(-4.58327079200005,2.2,0.682973754999985));
#311486=CARTESIAN_POINT('Ctrl Pts',(-4.58134147300005,12.2,0.681415840999984));
#311487=CARTESIAN_POINT('Ctrl Pts',(-4.58134147300005,5.2,0.681415840999984));
#311488=CARTESIAN_POINT('Ctrl Pts',(-4.58134147300005,2.2,0.681415840999984));
#311489=CARTESIAN_POINT('Ctrl Pts',(-4.57941327700006,12.2,0.679862194999985));
#311490=CARTESIAN_POINT('Ctrl Pts',(-4.57941327700006,5.2,0.679862194999985));
#311491=CARTESIAN_POINT('Ctrl Pts',(-4.57941327700006,2.2,0.679862194999985));
#311492=CARTESIAN_POINT('Ctrl Pts',(-4.57748621200006,12.2,0.678312816999984));
#311493=CARTESIAN_POINT('Ctrl Pts',(-4.57748621200006,5.2,0.678312816999984));
#311494=CARTESIAN_POINT('Ctrl Pts',(-4.57748621200006,2.2,0.678312816999984));
#311495=CARTESIAN_POINT('Ctrl Pts',(-4.57556028800005,12.2,0.676767706999986));
#311496=CARTESIAN_POINT('Ctrl Pts',(-4.57556028800005,5.2,0.676767706999986));
#311497=CARTESIAN_POINT('Ctrl Pts',(-4.57556028800005,2.2,0.676767706999986));
#311498=CARTESIAN_POINT('Ctrl Pts',(-4.57363551500006,12.2,0.675226858999984));
#311499=CARTESIAN_POINT('Ctrl Pts',(-4.57363551500006,5.2,0.675226858999984));
#311500=CARTESIAN_POINT('Ctrl Pts',(-4.57363551500006,2.2,0.675226858999984));
#311501=CARTESIAN_POINT('Ctrl Pts',(-4.57171190000006,12.2,0.673690276999985));
#311502=CARTESIAN_POINT('Ctrl Pts',(-4.57171190000006,5.2,0.673690276999985));
#311503=CARTESIAN_POINT('Ctrl Pts',(-4.57171190000006,2.2,0.673690276999985));
#311504=CARTESIAN_POINT('Ctrl Pts',(-4.56978945400006,12.2,0.672157956999988));
#311505=CARTESIAN_POINT('Ctrl Pts',(-4.56978945400006,5.2,0.672157956999988));
#311506=CARTESIAN_POINT('Ctrl Pts',(-4.56978945400006,2.2,0.672157956999988));
#311507=CARTESIAN_POINT('Ctrl Pts',(-4.56786818400006,12.2,0.670629898999984));
#311508=CARTESIAN_POINT('Ctrl Pts',(-4.56786818400006,5.2,0.670629898999984));
#311509=CARTESIAN_POINT('Ctrl Pts',(-4.56786818400006,2.2,0.670629898999984));
#311510=CARTESIAN_POINT('Ctrl Pts',(-4.56594810100006,12.2,0.669106100999985));
#311511=CARTESIAN_POINT('Ctrl Pts',(-4.56594810100006,5.2,0.669106100999985));
#311512=CARTESIAN_POINT('Ctrl Pts',(-4.56594810100006,2.2,0.669106100999985));
#311513=CARTESIAN_POINT('Ctrl Pts',(-4.56402921300006,12.2,0.667586562999984));
#311514=CARTESIAN_POINT('Ctrl Pts',(-4.56402921300006,5.2,0.667586562999984));
#311515=CARTESIAN_POINT('Ctrl Pts',(-4.56402921300006,2.2,0.667586562999984));
#311516=CARTESIAN_POINT('Ctrl Pts',(-4.56211153000006,12.2,0.666071280999985));
#311517=CARTESIAN_POINT('Ctrl Pts',(-4.56211153000006,5.2,0.666071280999985));
#311518=CARTESIAN_POINT('Ctrl Pts',(-4.56211153000006,2.2,0.666071280999985));
#311519=CARTESIAN_POINT('Ctrl Pts',(-4.56019506100006,12.2,0.664560255999986));
#311520=CARTESIAN_POINT('Ctrl Pts',(-4.56019506100006,5.2,0.664560255999986));
#311521=CARTESIAN_POINT('Ctrl Pts',(-4.56019506100006,2.2,0.664560255999986));
#311522=CARTESIAN_POINT('Ctrl Pts',(-4.55827981400006,12.2,0.663053487999985));
#311523=CARTESIAN_POINT('Ctrl Pts',(-4.55827981400006,5.2,0.663053487999985));
#311524=CARTESIAN_POINT('Ctrl Pts',(-4.55827981400006,2.2,0.663053487999985));
#311525=CARTESIAN_POINT('Ctrl Pts',(-4.55636580000006,12.2,0.661550972999985));
#311526=CARTESIAN_POINT('Ctrl Pts',(-4.55636580000006,5.2,0.661550972999985));
#311527=CARTESIAN_POINT('Ctrl Pts',(-4.55636580000006,2.2,0.661550972999985));
#311528=CARTESIAN_POINT('Ctrl Pts',(-4.55445302600006,12.2,0.660052709999985));
#311529=CARTESIAN_POINT('Ctrl Pts',(-4.55445302600006,5.2,0.660052709999985));
#311530=CARTESIAN_POINT('Ctrl Pts',(-4.55445302600006,2.2,0.660052709999985));
#311531=CARTESIAN_POINT('Ctrl Pts',(-4.55254150300005,12.2,0.658558698999983));
#311532=CARTESIAN_POINT('Ctrl Pts',(-4.55254150300005,5.2,0.658558698999983));
#311533=CARTESIAN_POINT('Ctrl Pts',(-4.55254150300005,2.2,0.658558698999983));
#311534=CARTESIAN_POINT('Ctrl Pts',(-4.55063123800006,12.2,0.657068937999985));
#311535=CARTESIAN_POINT('Ctrl Pts',(-4.55063123800006,5.2,0.657068937999985));
#311536=CARTESIAN_POINT('Ctrl Pts',(-4.55063123800006,2.2,0.657068937999985));
#311537=CARTESIAN_POINT('Ctrl Pts',(-4.54872224300006,12.2,0.655583424999988));
#311538=CARTESIAN_POINT('Ctrl Pts',(-4.54872224300006,5.2,0.655583424999988));
#311539=CARTESIAN_POINT('Ctrl Pts',(-4.54872224300006,2.2,0.655583424999988));
#311540=CARTESIAN_POINT('Ctrl Pts',(-4.54681452600005,12.2,0.654102160999983));
#311541=CARTESIAN_POINT('Ctrl Pts',(-4.54681452600005,5.2,0.654102160999983));
#311542=CARTESIAN_POINT('Ctrl Pts',(-4.54681452600005,2.2,0.654102160999983));
#311543=CARTESIAN_POINT('Ctrl Pts',(-4.54490809500006,12.2,0.652625140999987));
#311544=CARTESIAN_POINT('Ctrl Pts',(-4.54490809500006,5.2,0.652625140999987));
#311545=CARTESIAN_POINT('Ctrl Pts',(-4.54490809500006,2.2,0.652625140999987));
#311546=CARTESIAN_POINT('Ctrl Pts',(-4.54300296100006,12.2,0.651152365999987));
#311547=CARTESIAN_POINT('Ctrl Pts',(-4.54300296100006,5.2,0.651152365999987));
#311548=CARTESIAN_POINT('Ctrl Pts',(-4.54300296100006,2.2,0.651152365999987));
#311549=CARTESIAN_POINT('Ctrl Pts',(-4.54109913200006,12.2,0.649683834999983));
#311550=CARTESIAN_POINT('Ctrl Pts',(-4.54109913200006,5.2,0.649683834999983));
#311551=CARTESIAN_POINT('Ctrl Pts',(-4.54109913200006,2.2,0.649683834999983));
#311552=CARTESIAN_POINT('Ctrl Pts',(-4.53919661700006,12.2,0.648219544999984));
#311553=CARTESIAN_POINT('Ctrl Pts',(-4.53919661700006,5.2,0.648219544999984));
#311554=CARTESIAN_POINT('Ctrl Pts',(-4.53919661700006,2.2,0.648219544999984));
#311555=CARTESIAN_POINT('Ctrl Pts',(-4.53729542700006,12.2,0.646759494999984));
#311556=CARTESIAN_POINT('Ctrl Pts',(-4.53729542700006,5.2,0.646759494999984));
#311557=CARTESIAN_POINT('Ctrl Pts',(-4.53729542700006,2.2,0.646759494999984));
#311558=CARTESIAN_POINT('Ctrl Pts',(-4.53539557000005,12.2,0.645303683999985));
#311559=CARTESIAN_POINT('Ctrl Pts',(-4.53539557000005,5.2,0.645303683999985));
#311560=CARTESIAN_POINT('Ctrl Pts',(-4.53539557000005,2.2,0.645303683999985));
#311561=CARTESIAN_POINT('Ctrl Pts',(-4.53349705600006,12.2,0.643852110999985));
#311562=CARTESIAN_POINT('Ctrl Pts',(-4.53349705600006,5.2,0.643852110999985));
#311563=CARTESIAN_POINT('Ctrl Pts',(-4.53349705600006,2.2,0.643852110999985));
#311564=CARTESIAN_POINT('Ctrl Pts',(-4.53159989300006,12.2,0.642404772999985));
#311565=CARTESIAN_POINT('Ctrl Pts',(-4.53159989300006,5.2,0.642404772999985));
#311566=CARTESIAN_POINT('Ctrl Pts',(-4.53159989300006,2.2,0.642404772999985));
#311567=CARTESIAN_POINT('Ctrl Pts',(-4.52970409100006,12.2,0.640961668999989));
#311568=CARTESIAN_POINT('Ctrl Pts',(-4.52970409100006,5.2,0.640961668999989));
#311569=CARTESIAN_POINT('Ctrl Pts',(-4.52970409100006,2.2,0.640961668999989));
#311570=CARTESIAN_POINT('Ctrl Pts',(-4.52780966000006,12.2,0.639522799999988));
#311571=CARTESIAN_POINT('Ctrl Pts',(-4.52780966000006,5.2,0.639522799999988));
#311572=CARTESIAN_POINT('Ctrl Pts',(-4.52780966000006,2.2,0.639522799999988));
#311573=CARTESIAN_POINT('Ctrl Pts',(-4.52591660800006,12.2,0.638088159999985));
#311574=CARTESIAN_POINT('Ctrl Pts',(-4.52591660800006,5.2,0.638088159999985));
#311575=CARTESIAN_POINT('Ctrl Pts',(-4.52591660800006,2.2,0.638088159999985));
#311576=CARTESIAN_POINT('Ctrl Pts',(-4.52402494500006,12.2,0.636657750999987));
#311577=CARTESIAN_POINT('Ctrl Pts',(-4.52402494500006,5.2,0.636657750999987));
#311578=CARTESIAN_POINT('Ctrl Pts',(-4.52402494500006,2.2,0.636657750999987));
#311579=CARTESIAN_POINT('Ctrl Pts',(-4.52213468100005,12.2,0.635231568999988));
#311580=CARTESIAN_POINT('Ctrl Pts',(-4.52213468100005,5.2,0.635231568999988));
#311581=CARTESIAN_POINT('Ctrl Pts',(-4.52213468100005,2.2,0.635231568999988));
#311582=CARTESIAN_POINT('Ctrl Pts',(-4.52024582400006,12.2,0.633809614999983));
#311583=CARTESIAN_POINT('Ctrl Pts',(-4.52024582400006,5.2,0.633809614999983));
#311584=CARTESIAN_POINT('Ctrl Pts',(-4.52024582400006,2.2,0.633809614999983));
#311585=CARTESIAN_POINT('Ctrl Pts',(-4.51835838500006,12.2,0.632391883999985));
#311586=CARTESIAN_POINT('Ctrl Pts',(-4.51835838500006,5.2,0.632391883999985));
#311587=CARTESIAN_POINT('Ctrl Pts',(-4.51835838500006,2.2,0.632391883999985));
#311588=CARTESIAN_POINT('Ctrl Pts',(-4.51647237000006,12.2,0.630978377999987));
#311589=CARTESIAN_POINT('Ctrl Pts',(-4.51647237000006,5.2,0.630978377999987));
#311590=CARTESIAN_POINT('Ctrl Pts',(-4.51647237000006,2.2,0.630978377999987));
#311591=CARTESIAN_POINT('Ctrl Pts',(-4.51458779300006,12.2,0.629569093999987));
#311592=CARTESIAN_POINT('Ctrl Pts',(-4.51458779300006,5.2,0.629569093999987));
#311593=CARTESIAN_POINT('Ctrl Pts',(-4.51458779300006,2.2,0.629569093999987));
#311594=CARTESIAN_POINT('Ctrl Pts',(-4.51270466000006,12.2,0.628164028999985));
#311595=CARTESIAN_POINT('Ctrl Pts',(-4.51270466000006,5.2,0.628164028999985));
#311596=CARTESIAN_POINT('Ctrl Pts',(-4.51270466000006,2.2,0.628164028999985));
#311597=CARTESIAN_POINT('Ctrl Pts',(-4.51082298200006,12.2,0.626763183999985));
#311598=CARTESIAN_POINT('Ctrl Pts',(-4.51082298200006,5.2,0.626763183999985));
#311599=CARTESIAN_POINT('Ctrl Pts',(-4.51082298200006,2.2,0.626763183999985));
#311600=CARTESIAN_POINT('Ctrl Pts',(-4.50894276700006,12.2,0.625366554999989));
#311601=CARTESIAN_POINT('Ctrl Pts',(-4.50894276700006,5.2,0.625366554999989));
#311602=CARTESIAN_POINT('Ctrl Pts',(-4.50894276700006,2.2,0.625366554999989));
#311603=CARTESIAN_POINT('Ctrl Pts',(-4.50706402700006,12.2,0.623974140999985));
#311604=CARTESIAN_POINT('Ctrl Pts',(-4.50706402700006,5.2,0.623974140999985));
#311605=CARTESIAN_POINT('Ctrl Pts',(-4.50706402700006,2.2,0.623974140999985));
#311606=CARTESIAN_POINT('Ctrl Pts',(-4.50518676800006,12.2,0.622585940999985));
#311607=CARTESIAN_POINT('Ctrl Pts',(-4.50518676800006,5.2,0.622585940999985));
#311608=CARTESIAN_POINT('Ctrl Pts',(-4.50518676800006,2.2,0.622585940999985));
#311609=CARTESIAN_POINT('Ctrl Pts',(-4.50331100200006,12.2,0.621201952999986));
#311610=CARTESIAN_POINT('Ctrl Pts',(-4.50331100200006,5.2,0.621201952999986));
#311611=CARTESIAN_POINT('Ctrl Pts',(-4.50331100200006,2.2,0.621201952999986));
#311612=CARTESIAN_POINT('Ctrl Pts',(-4.50143673700006,12.2,0.619822173999989));
#311613=CARTESIAN_POINT('Ctrl Pts',(-4.50143673700006,5.2,0.619822173999989));
#311614=CARTESIAN_POINT('Ctrl Pts',(-4.50143673700006,2.2,0.619822173999989));
#311615=CARTESIAN_POINT('Ctrl Pts',(-4.49956398400006,12.2,0.618446604999985));
#311616=CARTESIAN_POINT('Ctrl Pts',(-4.49956398400006,5.2,0.618446604999985));
#311617=CARTESIAN_POINT('Ctrl Pts',(-4.49956398400006,2.2,0.618446604999985));
#311618=CARTESIAN_POINT('Ctrl Pts',(-4.49769275100006,12.2,0.617075240999987));
#311619=CARTESIAN_POINT('Ctrl Pts',(-4.49769275100006,5.2,0.617075240999987));
#311620=CARTESIAN_POINT('Ctrl Pts',(-4.49769275100006,2.2,0.617075240999987));
#311621=CARTESIAN_POINT('Ctrl Pts',(-4.49582304800006,12.2,0.615708081999986));
#311622=CARTESIAN_POINT('Ctrl Pts',(-4.49582304800006,5.2,0.615708081999986));
#311623=CARTESIAN_POINT('Ctrl Pts',(-4.49582304800006,2.2,0.615708081999986));
#311624=CARTESIAN_POINT('Ctrl Pts',(-4.49395488400006,12.2,0.614345126999982));
#311625=CARTESIAN_POINT('Ctrl Pts',(-4.49395488400006,5.2,0.614345126999982));
#311626=CARTESIAN_POINT('Ctrl Pts',(-4.49395488400006,2.2,0.614345126999982));
#311627=CARTESIAN_POINT('Ctrl Pts',(-4.49208827000006,12.2,0.612986371999984));
#311628=CARTESIAN_POINT('Ctrl Pts',(-4.49208827000006,5.2,0.612986371999984));
#311629=CARTESIAN_POINT('Ctrl Pts',(-4.49208827000006,2.2,0.612986371999984));
#311630=CARTESIAN_POINT('Ctrl Pts',(-4.49022321300006,12.2,0.611631817999987));
#311631=CARTESIAN_POINT('Ctrl Pts',(-4.49022321300006,5.2,0.611631817999987));
#311632=CARTESIAN_POINT('Ctrl Pts',(-4.49022321300006,2.2,0.611631817999987));
#311633=CARTESIAN_POINT('Ctrl Pts',(-4.48835972600006,12.2,0.610281459999986));
#311634=CARTESIAN_POINT('Ctrl Pts',(-4.48835972600006,5.2,0.610281459999986));
#311635=CARTESIAN_POINT('Ctrl Pts',(-4.48835972600006,2.2,0.610281459999986));
#311636=CARTESIAN_POINT('Ctrl Pts',(-4.48649781400006,12.2,0.608935297999986));
#311637=CARTESIAN_POINT('Ctrl Pts',(-4.48649781400006,5.2,0.608935297999986));
#311638=CARTESIAN_POINT('Ctrl Pts',(-4.48649781400006,2.2,0.608935297999986));
#311639=CARTESIAN_POINT('Ctrl Pts',(-4.48463749100006,12.2,0.607593329999983));
#311640=CARTESIAN_POINT('Ctrl Pts',(-4.48463749100006,5.2,0.607593329999983));
#311641=CARTESIAN_POINT('Ctrl Pts',(-4.48463749100006,2.2,0.607593329999983));
#311642=CARTESIAN_POINT('Ctrl Pts',(-4.48277876400006,12.2,0.606255554999984));
#311643=CARTESIAN_POINT('Ctrl Pts',(-4.48277876400006,5.2,0.606255554999984));
#311644=CARTESIAN_POINT('Ctrl Pts',(-4.48277876400006,2.2,0.606255554999984));
#311645=CARTESIAN_POINT('Ctrl Pts',(-4.48092164300006,12.2,0.604921968999985));
#311646=CARTESIAN_POINT('Ctrl Pts',(-4.48092164300006,5.2,0.604921968999985));
#311647=CARTESIAN_POINT('Ctrl Pts',(-4.48092164300006,2.2,0.604921968999985));
#311648=CARTESIAN_POINT('Ctrl Pts',(-4.47906613800006,12.2,0.603592571999982));
#311649=CARTESIAN_POINT('Ctrl Pts',(-4.47906613800006,5.2,0.603592571999982));
#311650=CARTESIAN_POINT('Ctrl Pts',(-4.47906613800006,2.2,0.603592571999982));
#311651=CARTESIAN_POINT('Ctrl Pts',(-4.47721225800006,12.2,0.602267359999988));
#311652=CARTESIAN_POINT('Ctrl Pts',(-4.47721225800006,5.2,0.602267359999988));
#311653=CARTESIAN_POINT('Ctrl Pts',(-4.47721225800006,2.2,0.602267359999988));
#311654=CARTESIAN_POINT('Ctrl Pts',(-4.47536001400006,12.2,0.600946333999985));
#311655=CARTESIAN_POINT('Ctrl Pts',(-4.47536001400006,5.2,0.600946333999985));
#311656=CARTESIAN_POINT('Ctrl Pts',(-4.47536001400006,2.2,0.600946333999985));
#311657=CARTESIAN_POINT('Ctrl Pts',(-4.47350941300006,12.2,0.599629488999986));
#311658=CARTESIAN_POINT('Ctrl Pts',(-4.47350941300006,5.2,0.599629488999986));
#311659=CARTESIAN_POINT('Ctrl Pts',(-4.47350941300006,2.2,0.599629488999986));
#311660=CARTESIAN_POINT('Ctrl Pts',(-4.47166046700006,12.2,0.598316823999987));
#311661=CARTESIAN_POINT('Ctrl Pts',(-4.47166046700006,5.2,0.598316823999987));
#311662=CARTESIAN_POINT('Ctrl Pts',(-4.47166046700006,2.2,0.598316823999987));
#311663=CARTESIAN_POINT('Ctrl Pts',(-4.46981318400006,12.2,0.597008338999987));
#311664=CARTESIAN_POINT('Ctrl Pts',(-4.46981318400006,5.2,0.597008338999987));
#311665=CARTESIAN_POINT('Ctrl Pts',(-4.46981318400006,2.2,0.597008338999987));
#311666=CARTESIAN_POINT('Ctrl Pts',(-4.46796757600006,12.2,0.595704029999986));
#311667=CARTESIAN_POINT('Ctrl Pts',(-4.46796757600006,5.2,0.595704029999986));
#311668=CARTESIAN_POINT('Ctrl Pts',(-4.46796757600006,2.2,0.595704029999986));
#311669=CARTESIAN_POINT('Ctrl Pts',(-4.46612365000005,12.2,0.594403894999989));
#311670=CARTESIAN_POINT('Ctrl Pts',(-4.46612365000005,5.2,0.594403894999989));
#311671=CARTESIAN_POINT('Ctrl Pts',(-4.46612365000005,2.2,0.594403894999989));
#311672=CARTESIAN_POINT('Ctrl Pts',(-4.46428141600006,12.2,0.593107931999985));
#311673=CARTESIAN_POINT('Ctrl Pts',(-4.46428141600006,5.2,0.593107931999985));
#311674=CARTESIAN_POINT('Ctrl Pts',(-4.46428141600006,2.2,0.593107931999985));
#311675=CARTESIAN_POINT('Ctrl Pts',(-4.46244088500006,12.2,0.591816139999986));
#311676=CARTESIAN_POINT('Ctrl Pts',(-4.46244088500006,5.2,0.591816139999986));
#311677=CARTESIAN_POINT('Ctrl Pts',(-4.46244088500006,2.2,0.591816139999986));
#311678=CARTESIAN_POINT('Ctrl Pts',(-4.46060206600006,12.2,0.590528515999988));
#311679=CARTESIAN_POINT('Ctrl Pts',(-4.46060206600006,5.2,0.590528515999988));
#311680=CARTESIAN_POINT('Ctrl Pts',(-4.46060206600006,2.2,0.590528515999988));
#311681=CARTESIAN_POINT('Ctrl Pts',(-4.45876496900006,12.2,0.589245056999985));
#311682=CARTESIAN_POINT('Ctrl Pts',(-4.45876496900006,5.2,0.589245056999985));
#311683=CARTESIAN_POINT('Ctrl Pts',(-4.45876496900006,2.2,0.589245056999985));
#311684=CARTESIAN_POINT('Ctrl Pts',(-4.45692960200006,12.2,0.587965762999985));
#311685=CARTESIAN_POINT('Ctrl Pts',(-4.45692960200006,5.2,0.587965762999985));
#311686=CARTESIAN_POINT('Ctrl Pts',(-4.45692960200006,2.2,0.587965762999985));
#311687=CARTESIAN_POINT('Ctrl Pts',(-4.45509597700006,12.2,0.586690630999982));
#311688=CARTESIAN_POINT('Ctrl Pts',(-4.45509597700006,5.2,0.586690630999982));
#311689=CARTESIAN_POINT('Ctrl Pts',(-4.45509597700006,2.2,0.586690630999982));
#311690=CARTESIAN_POINT('Ctrl Pts',(-4.45326410400006,12.2,0.585419658999986));
#311691=CARTESIAN_POINT('Ctrl Pts',(-4.45326410400006,5.2,0.585419658999986));
#311692=CARTESIAN_POINT('Ctrl Pts',(-4.45326410400006,2.2,0.585419658999986));
#311693=CARTESIAN_POINT('Ctrl Pts',(-4.45143399000006,12.2,0.584152843999988));
#311694=CARTESIAN_POINT('Ctrl Pts',(-4.45143399000006,5.2,0.584152843999988));
#311695=CARTESIAN_POINT('Ctrl Pts',(-4.45143399000006,2.2,0.584152843999988));
#311696=CARTESIAN_POINT('Ctrl Pts',(-4.44960564700006,12.2,0.582890184999982));
#311697=CARTESIAN_POINT('Ctrl Pts',(-4.44960564700006,5.2,0.582890184999982));
#311698=CARTESIAN_POINT('Ctrl Pts',(-4.44960564700006,2.2,0.582890184999982));
#311699=CARTESIAN_POINT('Ctrl Pts',(-4.44777908400006,12.2,0.581631678999983));
#311700=CARTESIAN_POINT('Ctrl Pts',(-4.44777908400006,5.2,0.581631678999983));
#311701=CARTESIAN_POINT('Ctrl Pts',(-4.44777908400006,2.2,0.581631678999983));
#311702=CARTESIAN_POINT('Ctrl Pts',(-4.44595431100006,12.2,0.580377323999985));
#311703=CARTESIAN_POINT('Ctrl Pts',(-4.44595431100006,5.2,0.580377323999985));
#311704=CARTESIAN_POINT('Ctrl Pts',(-4.44595431100006,2.2,0.580377323999985));
#311705=CARTESIAN_POINT('Ctrl Pts',(-4.44413133800006,12.2,0.579127117999985));
#311706=CARTESIAN_POINT('Ctrl Pts',(-4.44413133800006,5.2,0.579127117999985));
#311707=CARTESIAN_POINT('Ctrl Pts',(-4.44413133800006,2.2,0.579127117999985));
#311708=CARTESIAN_POINT('Ctrl Pts',(-4.44231017300006,12.2,0.577881058999985));
#311709=CARTESIAN_POINT('Ctrl Pts',(-4.44231017300006,5.2,0.577881058999985));
#311710=CARTESIAN_POINT('Ctrl Pts',(-4.44231017300006,2.2,0.577881058999985));
#311711=CARTESIAN_POINT('Ctrl Pts',(-4.44049082800006,12.2,0.576639143999986));
#311712=CARTESIAN_POINT('Ctrl Pts',(-4.44049082800006,5.2,0.576639143999986));
#311713=CARTESIAN_POINT('Ctrl Pts',(-4.44049082800006,2.2,0.576639143999986));
#311714=CARTESIAN_POINT('Ctrl Pts',(-4.43867331200006,12.2,0.575401370999984));
#311715=CARTESIAN_POINT('Ctrl Pts',(-4.43867331200006,5.2,0.575401370999984));
#311716=CARTESIAN_POINT('Ctrl Pts',(-4.43867331200006,2.2,0.575401370999984));
#311717=CARTESIAN_POINT('Ctrl Pts',(-4.43685763500006,12.2,0.574167737999982));
#311718=CARTESIAN_POINT('Ctrl Pts',(-4.43685763500006,5.2,0.574167737999982));
#311719=CARTESIAN_POINT('Ctrl Pts',(-4.43685763500006,2.2,0.574167737999982));
#311720=CARTESIAN_POINT('Ctrl Pts',(-4.43504380600006,12.2,0.572938241999985));
#311721=CARTESIAN_POINT('Ctrl Pts',(-4.43504380600006,5.2,0.572938241999985));
#311722=CARTESIAN_POINT('Ctrl Pts',(-4.43504380600006,2.2,0.572938241999985));
#311723=CARTESIAN_POINT('Ctrl Pts',(-4.43323183600006,12.2,0.571712881999984));
#311724=CARTESIAN_POINT('Ctrl Pts',(-4.43323183600006,5.2,0.571712881999984));
#311725=CARTESIAN_POINT('Ctrl Pts',(-4.43323183600006,2.2,0.571712881999984));
#311726=CARTESIAN_POINT('Ctrl Pts',(-4.43142173400005,12.2,0.570491653999987));
#311727=CARTESIAN_POINT('Ctrl Pts',(-4.43142173400005,5.2,0.570491653999987));
#311728=CARTESIAN_POINT('Ctrl Pts',(-4.43142173400005,2.2,0.570491653999987));
#311729=CARTESIAN_POINT('Ctrl Pts',(-4.42961351100006,12.2,0.569274557999986));
#311730=CARTESIAN_POINT('Ctrl Pts',(-4.42961351100006,5.2,0.569274557999986));
#311731=CARTESIAN_POINT('Ctrl Pts',(-4.42961351100006,2.2,0.569274557999986));
#311732=CARTESIAN_POINT('Ctrl Pts',(-4.42780717600006,12.2,0.568061588999988));
#311733=CARTESIAN_POINT('Ctrl Pts',(-4.42780717600006,5.2,0.568061588999988));
#311734=CARTESIAN_POINT('Ctrl Pts',(-4.42780717600006,2.2,0.568061588999988));
#311735=CARTESIAN_POINT('Ctrl Pts',(-4.42600273800006,12.2,0.566852745999986));
#311736=CARTESIAN_POINT('Ctrl Pts',(-4.42600273800006,5.2,0.566852745999986));
#311737=CARTESIAN_POINT('Ctrl Pts',(-4.42600273800006,2.2,0.566852745999986));
#311738=CARTESIAN_POINT('Ctrl Pts',(-4.42420020900006,12.2,0.565648025999987));
#311739=CARTESIAN_POINT('Ctrl Pts',(-4.42420020900006,5.2,0.565648025999987));
#311740=CARTESIAN_POINT('Ctrl Pts',(-4.42420020900006,2.2,0.565648025999987));
#311741=CARTESIAN_POINT('Ctrl Pts',(-4.42239959700006,12.2,0.564447427999983));
#311742=CARTESIAN_POINT('Ctrl Pts',(-4.42239959700006,5.2,0.564447427999983));
#311743=CARTESIAN_POINT('Ctrl Pts',(-4.42239959700006,2.2,0.564447427999983));
#311744=CARTESIAN_POINT('Ctrl Pts',(-4.42060091200006,12.2,0.563250946999982));
#311745=CARTESIAN_POINT('Ctrl Pts',(-4.42060091200006,5.2,0.563250946999982));
#311746=CARTESIAN_POINT('Ctrl Pts',(-4.42060091200006,2.2,0.563250946999982));
#311747=CARTESIAN_POINT('Ctrl Pts',(-4.41880416600006,12.2,0.562058582999985));
#311748=CARTESIAN_POINT('Ctrl Pts',(-4.41880416600006,5.2,0.562058582999985));
#311749=CARTESIAN_POINT('Ctrl Pts',(-4.41880416600006,2.2,0.562058582999985));
#311750=CARTESIAN_POINT('Ctrl Pts',(-4.41700936600006,12.2,0.560870332999985));
#311751=CARTESIAN_POINT('Ctrl Pts',(-4.41700936600006,5.2,0.560870332999985));
#311752=CARTESIAN_POINT('Ctrl Pts',(-4.41700936600006,2.2,0.560870332999985));
#311753=CARTESIAN_POINT('Ctrl Pts',(-4.41521652500006,12.2,0.559686192999984));
#311754=CARTESIAN_POINT('Ctrl Pts',(-4.41521652500006,5.2,0.559686192999984));
#311755=CARTESIAN_POINT('Ctrl Pts',(-4.41521652500006,2.2,0.559686192999984));
#311756=CARTESIAN_POINT('Ctrl Pts',(-4.41342565100006,12.2,0.558506162999985));
#311757=CARTESIAN_POINT('Ctrl Pts',(-4.41342565100006,5.2,0.558506162999985));
#311758=CARTESIAN_POINT('Ctrl Pts',(-4.41342565100006,2.2,0.558506162999985));
#311759=CARTESIAN_POINT('Ctrl Pts',(-4.41163675500006,12.2,0.557330237999984));
#311760=CARTESIAN_POINT('Ctrl Pts',(-4.41163675500006,5.2,0.557330237999984));
#311761=CARTESIAN_POINT('Ctrl Pts',(-4.41163675500006,2.2,0.557330237999984));
#311762=CARTESIAN_POINT('Ctrl Pts',(-4.40984984500005,12.2,0.556158416999986));
#311763=CARTESIAN_POINT('Ctrl Pts',(-4.40984984500005,5.2,0.556158416999986));
#311764=CARTESIAN_POINT('Ctrl Pts',(-4.40984984500005,2.2,0.556158416999986));
#311765=CARTESIAN_POINT('Ctrl Pts',(-4.40806493400006,12.2,0.554990695999984));
#311766=CARTESIAN_POINT('Ctrl Pts',(-4.40806493400006,5.2,0.554990695999984));
#311767=CARTESIAN_POINT('Ctrl Pts',(-4.40806493400006,2.2,0.554990695999984));
#311768=CARTESIAN_POINT('Ctrl Pts',(-4.40628203000006,12.2,0.553827074999984));
#311769=CARTESIAN_POINT('Ctrl Pts',(-4.40628203000006,5.2,0.553827074999984));
#311770=CARTESIAN_POINT('Ctrl Pts',(-4.40628203000006,2.2,0.553827074999984));
#311771=CARTESIAN_POINT('Ctrl Pts',(-4.40450114300006,12.2,0.552667548999985));
#311772=CARTESIAN_POINT('Ctrl Pts',(-4.40450114300006,5.2,0.552667548999985));
#311773=CARTESIAN_POINT('Ctrl Pts',(-4.40450114300006,2.2,0.552667548999985));
#311774=CARTESIAN_POINT('Ctrl Pts',(-4.40272228400006,12.2,0.551512115999984));
#311775=CARTESIAN_POINT('Ctrl Pts',(-4.40272228400006,5.2,0.551512115999984));
#311776=CARTESIAN_POINT('Ctrl Pts',(-4.40272228400006,2.2,0.551512115999984));
#311777=CARTESIAN_POINT('Ctrl Pts',(-4.40094546300006,12.2,0.550360773999987));
#311778=CARTESIAN_POINT('Ctrl Pts',(-4.40094546300006,5.2,0.550360773999987));
#311779=CARTESIAN_POINT('Ctrl Pts',(-4.40094546300006,2.2,0.550360773999987));
#311780=CARTESIAN_POINT('Ctrl Pts',(-4.39917068900006,12.2,0.549213519999987));
#311781=CARTESIAN_POINT('Ctrl Pts',(-4.39917068900006,5.2,0.549213519999987));
#311782=CARTESIAN_POINT('Ctrl Pts',(-4.39917068900006,2.2,0.549213519999987));
#311783=CARTESIAN_POINT('Ctrl Pts',(-4.39739797300006,12.2,0.548070350999983));
#311784=CARTESIAN_POINT('Ctrl Pts',(-4.39739797300006,5.2,0.548070350999983));
#311785=CARTESIAN_POINT('Ctrl Pts',(-4.39739797300006,2.2,0.548070350999983));
#311786=CARTESIAN_POINT('Ctrl Pts',(-4.39562732400006,12.2,0.546931263999983));
#311787=CARTESIAN_POINT('Ctrl Pts',(-4.39562732400006,5.2,0.546931263999983));
#311788=CARTESIAN_POINT('Ctrl Pts',(-4.39562732400006,2.2,0.546931263999983));
#311789=CARTESIAN_POINT('Ctrl Pts',(-4.39385875300006,12.2,0.545796257999989));
#311790=CARTESIAN_POINT('Ctrl Pts',(-4.39385875300006,5.2,0.545796257999989));
#311791=CARTESIAN_POINT('Ctrl Pts',(-4.39385875300006,2.2,0.545796257999989));
#311792=CARTESIAN_POINT('Ctrl Pts',(-4.39209227100006,12.2,0.544665327999985));
#311793=CARTESIAN_POINT('Ctrl Pts',(-4.39209227100006,5.2,0.544665327999985));
#311794=CARTESIAN_POINT('Ctrl Pts',(-4.39209227100006,2.2,0.544665327999985));
#311795=CARTESIAN_POINT('Ctrl Pts',(-4.39032788600006,12.2,0.543538472999985));
#311796=CARTESIAN_POINT('Ctrl Pts',(-4.39032788600006,5.2,0.543538472999985));
#311797=CARTESIAN_POINT('Ctrl Pts',(-4.39032788600006,2.2,0.543538472999985));
#311798=CARTESIAN_POINT('Ctrl Pts',(-4.38856561000006,12.2,0.542415689999984));
#311799=CARTESIAN_POINT('Ctrl Pts',(-4.38856561000006,5.2,0.542415689999984));
#311800=CARTESIAN_POINT('Ctrl Pts',(-4.38856561000006,2.2,0.542415689999984));
#311801=CARTESIAN_POINT('Ctrl Pts',(-4.38680545200006,12.2,0.541296975999987));
#311802=CARTESIAN_POINT('Ctrl Pts',(-4.38680545200006,5.2,0.541296975999987));
#311803=CARTESIAN_POINT('Ctrl Pts',(-4.38680545200006,2.2,0.541296975999987));
#311804=CARTESIAN_POINT('Ctrl Pts',(-4.38504742300006,12.2,0.540182326999985));
#311805=CARTESIAN_POINT('Ctrl Pts',(-4.38504742300006,5.2,0.540182326999985));
#311806=CARTESIAN_POINT('Ctrl Pts',(-4.38504742300006,2.2,0.540182326999985));
#311807=CARTESIAN_POINT('Ctrl Pts',(-4.38329153100006,12.2,0.539071742999986));
#311808=CARTESIAN_POINT('Ctrl Pts',(-4.38329153100006,5.2,0.539071742999986));
#311809=CARTESIAN_POINT('Ctrl Pts',(-4.38329153100006,2.2,0.539071742999986));
#311810=CARTESIAN_POINT('Ctrl Pts',(-4.38153778900006,12.2,0.537965217999985));
#311811=CARTESIAN_POINT('Ctrl Pts',(-4.38153778900006,5.2,0.537965217999985));
#311812=CARTESIAN_POINT('Ctrl Pts',(-4.38153778900006,2.2,0.537965217999985));
#311813=CARTESIAN_POINT('Ctrl Pts',(-4.37978620700005,12.2,0.536862750999987));
#311814=CARTESIAN_POINT('Ctrl Pts',(-4.37978620700005,5.2,0.536862750999987));
#311815=CARTESIAN_POINT('Ctrl Pts',(-4.37978620700005,2.2,0.536862750999987));
#311816=CARTESIAN_POINT('Ctrl Pts',(-4.37803679200006,12.2,0.535764338999982));
#311817=CARTESIAN_POINT('Ctrl Pts',(-4.37803679200006,5.2,0.535764338999982));
#311818=CARTESIAN_POINT('Ctrl Pts',(-4.37803679200006,2.2,0.535764338999982));
#311819=CARTESIAN_POINT('Ctrl Pts',(-4.37628955800006,12.2,0.534669978999984));
#311820=CARTESIAN_POINT('Ctrl Pts',(-4.37628955800006,5.2,0.534669978999984));
#311821=CARTESIAN_POINT('Ctrl Pts',(-4.37628955800006,2.2,0.534669978999984));
#311822=CARTESIAN_POINT('Ctrl Pts',(-4.37454451300006,12.2,0.533579666999984));
#311823=CARTESIAN_POINT('Ctrl Pts',(-4.37454451300006,5.2,0.533579666999984));
#311824=CARTESIAN_POINT('Ctrl Pts',(-4.37454451300006,2.2,0.533579666999984));
#311825=CARTESIAN_POINT('Ctrl Pts',(-4.37280166800006,12.2,0.532493402999985));
#311826=CARTESIAN_POINT('Ctrl Pts',(-4.37280166800006,5.2,0.532493402999985));
#311827=CARTESIAN_POINT('Ctrl Pts',(-4.37280166800006,2.2,0.532493402999985));
#311828=CARTESIAN_POINT('Ctrl Pts',(-4.37106103400006,12.2,0.531411180999988));
#311829=CARTESIAN_POINT('Ctrl Pts',(-4.37106103400006,5.2,0.531411180999988));
#311830=CARTESIAN_POINT('Ctrl Pts',(-4.37106103400006,2.2,0.531411180999988));
#311831=CARTESIAN_POINT('Ctrl Pts',(-4.36932262000005,12.2,0.530332998999987));
#311832=CARTESIAN_POINT('Ctrl Pts',(-4.36932262000005,5.2,0.530332998999987));
#311833=CARTESIAN_POINT('Ctrl Pts',(-4.36932262000005,2.2,0.530332998999987));
#311834=CARTESIAN_POINT('Ctrl Pts',(-4.36758643600006,12.2,0.529258853999988));
#311835=CARTESIAN_POINT('Ctrl Pts',(-4.36758643600006,5.2,0.529258853999988));
#311836=CARTESIAN_POINT('Ctrl Pts',(-4.36758643600006,2.2,0.529258853999988));
#311837=CARTESIAN_POINT('Ctrl Pts',(-4.36585249300006,12.2,0.528188743999984));
#311838=CARTESIAN_POINT('Ctrl Pts',(-4.36585249300006,5.2,0.528188743999984));
#311839=CARTESIAN_POINT('Ctrl Pts',(-4.36585249300006,2.2,0.528188743999984));
#311840=CARTESIAN_POINT('Ctrl Pts',(-4.36412080200006,12.2,0.527122664999986));
#311841=CARTESIAN_POINT('Ctrl Pts',(-4.36412080200006,5.2,0.527122664999986));
#311842=CARTESIAN_POINT('Ctrl Pts',(-4.36412080200006,2.2,0.527122664999986));
#311843=CARTESIAN_POINT('Ctrl Pts',(-4.36239137100006,12.2,0.526060612999988));
#311844=CARTESIAN_POINT('Ctrl Pts',(-4.36239137100006,5.2,0.526060612999988));
#311845=CARTESIAN_POINT('Ctrl Pts',(-4.36239137100006,2.2,0.526060612999988));
#311846=CARTESIAN_POINT('Ctrl Pts',(-4.36066421300006,12.2,0.525002587999985));
#311847=CARTESIAN_POINT('Ctrl Pts',(-4.36066421300006,5.2,0.525002587999985));
#311848=CARTESIAN_POINT('Ctrl Pts',(-4.36066421300006,2.2,0.525002587999985));
#311849=CARTESIAN_POINT('Ctrl Pts',(-4.35893933600005,12.2,0.523948583999987));
#311850=CARTESIAN_POINT('Ctrl Pts',(-4.35893933600005,5.2,0.523948583999987));
#311851=CARTESIAN_POINT('Ctrl Pts',(-4.35893933600005,2.2,0.523948583999987));
#311852=CARTESIAN_POINT('Ctrl Pts',(-4.35721675300006,12.2,0.522898598999983));
#311853=CARTESIAN_POINT('Ctrl Pts',(-4.35721675300006,5.2,0.522898598999983));
#311854=CARTESIAN_POINT('Ctrl Pts',(-4.35721675300006,2.2,0.522898598999983));
#311855=CARTESIAN_POINT('Ctrl Pts',(-4.35549647200006,12.2,0.521852629999984));
#311856=CARTESIAN_POINT('Ctrl Pts',(-4.35549647200006,5.2,0.521852629999984));
#311857=CARTESIAN_POINT('Ctrl Pts',(-4.35549647200006,2.2,0.521852629999984));
#311858=CARTESIAN_POINT('Ctrl Pts',(-4.35377850500006,12.2,0.520810673999983));
#311859=CARTESIAN_POINT('Ctrl Pts',(-4.35377850500006,5.2,0.520810673999983));
#311860=CARTESIAN_POINT('Ctrl Pts',(-4.35377850500006,2.2,0.520810673999983));
#311861=CARTESIAN_POINT('Ctrl Pts',(-4.35206286100006,12.2,0.519772727999985));
#311862=CARTESIAN_POINT('Ctrl Pts',(-4.35206286100006,5.2,0.519772727999985));
#311863=CARTESIAN_POINT('Ctrl Pts',(-4.35206286100006,2.2,0.519772727999985));
#311864=CARTESIAN_POINT('Ctrl Pts',(-4.35034955100006,12.2,0.518738786999986));
#311865=CARTESIAN_POINT('Ctrl Pts',(-4.35034955100006,5.2,0.518738786999986));
#311866=CARTESIAN_POINT('Ctrl Pts',(-4.35034955100006,2.2,0.518738786999986));
#311867=CARTESIAN_POINT('Ctrl Pts',(-4.34863858500006,12.2,0.517708849999985));
#311868=CARTESIAN_POINT('Ctrl Pts',(-4.34863858500006,5.2,0.517708849999985));
#311869=CARTESIAN_POINT('Ctrl Pts',(-4.34863858500006,2.2,0.517708849999985));
#311870=CARTESIAN_POINT('Ctrl Pts',(-4.34692997500005,12.2,0.516682913999986));
#311871=CARTESIAN_POINT('Ctrl Pts',(-4.34692997500005,5.2,0.516682913999986));
#311872=CARTESIAN_POINT('Ctrl Pts',(-4.34692997500005,2.2,0.516682913999986));
#311873=CARTESIAN_POINT('Ctrl Pts',(-4.34522372900005,12.2,0.515660973999985));
#311874=CARTESIAN_POINT('Ctrl Pts',(-4.34522372900005,5.2,0.515660973999985));
#311875=CARTESIAN_POINT('Ctrl Pts',(-4.34522372900005,2.2,0.515660973999985));
#311876=CARTESIAN_POINT('Ctrl Pts',(-4.34351985900006,12.2,0.514643026999986));
#311877=CARTESIAN_POINT('Ctrl Pts',(-4.34351985900006,5.2,0.514643026999986));
#311878=CARTESIAN_POINT('Ctrl Pts',(-4.34351985900006,2.2,0.514643026999986));
#311879=CARTESIAN_POINT('Ctrl Pts',(-4.34181837600006,12.2,0.513629070999984));
#311880=CARTESIAN_POINT('Ctrl Pts',(-4.34181837600006,5.2,0.513629070999984));
#311881=CARTESIAN_POINT('Ctrl Pts',(-4.34181837600006,2.2,0.513629070999984));
#311882=CARTESIAN_POINT('Ctrl Pts',(-4.34011928900006,12.2,0.512619101999987));
#311883=CARTESIAN_POINT('Ctrl Pts',(-4.34011928900006,5.2,0.512619101999987));
#311884=CARTESIAN_POINT('Ctrl Pts',(-4.34011928900006,2.2,0.512619101999987));
#311885=CARTESIAN_POINT('Ctrl Pts',(-4.33842260800006,12.2,0.511613116999987));
#311886=CARTESIAN_POINT('Ctrl Pts',(-4.33842260800006,5.2,0.511613116999987));
#311887=CARTESIAN_POINT('Ctrl Pts',(-4.33842260800006,2.2,0.511613116999987));
#311888=CARTESIAN_POINT('Ctrl Pts',(-4.33672834600006,12.2,0.510611111999988));
#311889=CARTESIAN_POINT('Ctrl Pts',(-4.33672834600006,5.2,0.510611111999988));
#311890=CARTESIAN_POINT('Ctrl Pts',(-4.33672834600006,2.2,0.510611111999988));
#311891=CARTESIAN_POINT('Ctrl Pts',(-4.33503651100006,12.2,0.509613083999985));
#311892=CARTESIAN_POINT('Ctrl Pts',(-4.33503651100006,5.2,0.509613083999985));
#311893=CARTESIAN_POINT('Ctrl Pts',(-4.33503651100006,2.2,0.509613083999985));
#311894=CARTESIAN_POINT('Ctrl Pts',(-4.33334711500006,12.2,0.508619029999986));
#311895=CARTESIAN_POINT('Ctrl Pts',(-4.33334711500006,5.2,0.508619029999986));
#311896=CARTESIAN_POINT('Ctrl Pts',(-4.33334711500006,2.2,0.508619029999986));
#311897=CARTESIAN_POINT('Ctrl Pts',(-4.33166016800006,12.2,0.507628945999983));
#311898=CARTESIAN_POINT('Ctrl Pts',(-4.33166016800006,5.2,0.507628945999983));
#311899=CARTESIAN_POINT('Ctrl Pts',(-4.33166016800006,2.2,0.507628945999983));
#311900=CARTESIAN_POINT('Ctrl Pts',(-4.32997568100006,12.2,0.506642829999984));
#311901=CARTESIAN_POINT('Ctrl Pts',(-4.32997568100006,5.2,0.506642829999984));
#311902=CARTESIAN_POINT('Ctrl Pts',(-4.32997568100006,2.2,0.506642829999984));
#311903=CARTESIAN_POINT('Ctrl Pts',(-4.32829366300005,12.2,0.505660676999984));
#311904=CARTESIAN_POINT('Ctrl Pts',(-4.32829366300005,5.2,0.505660676999984));
#311905=CARTESIAN_POINT('Ctrl Pts',(-4.32829366300005,2.2,0.505660676999984));
#311906=CARTESIAN_POINT('Ctrl Pts',(-4.32661412700006,12.2,0.504682482999983));
#311907=CARTESIAN_POINT('Ctrl Pts',(-4.32661412700006,5.2,0.504682482999983));
#311908=CARTESIAN_POINT('Ctrl Pts',(-4.32661412700006,2.2,0.504682482999983));
#311909=CARTESIAN_POINT('Ctrl Pts',(-4.32493708300006,12.2,0.503708246999985));
#311910=CARTESIAN_POINT('Ctrl Pts',(-4.32493708300006,5.2,0.503708246999985));
#311911=CARTESIAN_POINT('Ctrl Pts',(-4.32493708300006,2.2,0.503708246999985));
#311912=CARTESIAN_POINT('Ctrl Pts',(-4.32326253900006,12.2,0.502737962999986));
#311913=CARTESIAN_POINT('Ctrl Pts',(-4.32326253900006,5.2,0.502737962999986));
#311914=CARTESIAN_POINT('Ctrl Pts',(-4.32326253900006,2.2,0.502737962999986));
#311915=CARTESIAN_POINT('Ctrl Pts',(-4.32159050800006,12.2,0.501771628999985));
#311916=CARTESIAN_POINT('Ctrl Pts',(-4.32159050800006,5.2,0.501771628999985));
#311917=CARTESIAN_POINT('Ctrl Pts',(-4.32159050800006,2.2,0.501771628999985));
#311918=CARTESIAN_POINT('Ctrl Pts',(-4.31992100100006,12.2,0.500809241999987));
#311919=CARTESIAN_POINT('Ctrl Pts',(-4.31992100100006,5.2,0.500809241999987));
#311920=CARTESIAN_POINT('Ctrl Pts',(-4.31992100100006,2.2,0.500809241999987));
#311921=CARTESIAN_POINT('Ctrl Pts',(-4.31825402600006,12.2,0.499850796999985));
#311922=CARTESIAN_POINT('Ctrl Pts',(-4.31825402600006,5.2,0.499850796999985));
#311923=CARTESIAN_POINT('Ctrl Pts',(-4.31825402600006,2.2,0.499850796999985));
#311924=CARTESIAN_POINT('Ctrl Pts',(-4.31658959700005,12.2,0.498896291999986));
#311925=CARTESIAN_POINT('Ctrl Pts',(-4.31658959700005,5.2,0.498896291999986));
#311926=CARTESIAN_POINT('Ctrl Pts',(-4.31658959700005,2.2,0.498896291999986));
#311927=CARTESIAN_POINT('Ctrl Pts',(-4.31492772200006,12.2,0.497945720999984));
#311928=CARTESIAN_POINT('Ctrl Pts',(-4.31492772200006,5.2,0.497945720999984));
#311929=CARTESIAN_POINT('Ctrl Pts',(-4.31492772200006,2.2,0.497945720999984));
#311930=CARTESIAN_POINT('Ctrl Pts',(-4.31326841300006,12.2,0.496999082999987));
#311931=CARTESIAN_POINT('Ctrl Pts',(-4.31326841300006,5.2,0.496999082999987));
#311932=CARTESIAN_POINT('Ctrl Pts',(-4.31326841300006,2.2,0.496999082999987));
#311933=CARTESIAN_POINT('Ctrl Pts',(-4.31161168100005,12.2,0.496056371999987));
#311934=CARTESIAN_POINT('Ctrl Pts',(-4.31161168100005,5.2,0.496056371999987));
#311935=CARTESIAN_POINT('Ctrl Pts',(-4.31161168100005,2.2,0.496056371999987));
#311936=CARTESIAN_POINT('Ctrl Pts',(-4.30995753500006,12.2,0.495117585999987));
#311937=CARTESIAN_POINT('Ctrl Pts',(-4.30995753500006,5.2,0.495117585999987));
#311938=CARTESIAN_POINT('Ctrl Pts',(-4.30995753500006,2.2,0.495117585999987));
#311939=CARTESIAN_POINT('Ctrl Pts',(-4.30830598800005,12.2,0.494182721999987));
#311940=CARTESIAN_POINT('Ctrl Pts',(-4.30830598800005,5.2,0.494182721999987));
#311941=CARTESIAN_POINT('Ctrl Pts',(-4.30830598800005,2.2,0.494182721999987));
#311942=CARTESIAN_POINT('Ctrl Pts',(-4.30665704900006,12.2,0.493251773999983));
#311943=CARTESIAN_POINT('Ctrl Pts',(-4.30665704900006,5.2,0.493251773999983));
#311944=CARTESIAN_POINT('Ctrl Pts',(-4.30665704900006,2.2,0.493251773999983));
#311945=CARTESIAN_POINT('Ctrl Pts',(-4.30501072900006,12.2,0.492324739999983));
#311946=CARTESIAN_POINT('Ctrl Pts',(-4.30501072900006,5.2,0.492324739999983));
#311947=CARTESIAN_POINT('Ctrl Pts',(-4.30501072900006,2.2,0.492324739999983));
#311948=CARTESIAN_POINT('Ctrl Pts',(-4.30336703900006,12.2,0.491401615999987));
#311949=CARTESIAN_POINT('Ctrl Pts',(-4.30336703900006,5.2,0.491401615999987));
#311950=CARTESIAN_POINT('Ctrl Pts',(-4.30336703900006,2.2,0.491401615999987));
#311951=CARTESIAN_POINT('Ctrl Pts',(-4.30172598900006,12.2,0.490482396999985));
#311952=CARTESIAN_POINT('Ctrl Pts',(-4.30172598900006,5.2,0.490482396999985));
#311953=CARTESIAN_POINT('Ctrl Pts',(-4.30172598900006,2.2,0.490482396999985));
#311954=CARTESIAN_POINT('Ctrl Pts',(-4.30008759200006,12.2,0.489567081999986));
#311955=CARTESIAN_POINT('Ctrl Pts',(-4.30008759200006,5.2,0.489567081999986));
#311956=CARTESIAN_POINT('Ctrl Pts',(-4.30008759200006,2.2,0.489567081999986));
#311957=CARTESIAN_POINT('Ctrl Pts',(-4.29845185500006,12.2,0.488655663999986));
#311958=CARTESIAN_POINT('Ctrl Pts',(-4.29845185500006,5.2,0.488655663999986));
#311959=CARTESIAN_POINT('Ctrl Pts',(-4.29845185500006,2.2,0.488655663999986));
#311960=CARTESIAN_POINT('Ctrl Pts',(-4.29681879300006,12.2,0.487748140999984));
#311961=CARTESIAN_POINT('Ctrl Pts',(-4.29681879300006,5.2,0.487748140999984));
#311962=CARTESIAN_POINT('Ctrl Pts',(-4.29681879300006,2.2,0.487748140999984));
#311963=CARTESIAN_POINT('Ctrl Pts',(-4.29518841400006,12.2,0.486844509999984));
#311964=CARTESIAN_POINT('Ctrl Pts',(-4.29518841400006,5.2,0.486844509999984));
#311965=CARTESIAN_POINT('Ctrl Pts',(-4.29518841400006,2.2,0.486844509999984));
#311966=CARTESIAN_POINT('Ctrl Pts',(-4.29356073000006,12.2,0.485944765999986));
#311967=CARTESIAN_POINT('Ctrl Pts',(-4.29356073000006,5.2,0.485944765999986));
#311968=CARTESIAN_POINT('Ctrl Pts',(-4.29356073000006,2.2,0.485944765999986));
#311969=CARTESIAN_POINT('Ctrl Pts',(-4.29193575100006,12.2,0.485048903999985));
#311970=CARTESIAN_POINT('Ctrl Pts',(-4.29193575100006,5.2,0.485048903999985));
#311971=CARTESIAN_POINT('Ctrl Pts',(-4.29193575100006,2.2,0.485048903999985));
#311972=CARTESIAN_POINT('Ctrl Pts',(-4.29031348800006,12.2,0.484156920999985));
#311973=CARTESIAN_POINT('Ctrl Pts',(-4.29031348800006,5.2,0.484156920999985));
#311974=CARTESIAN_POINT('Ctrl Pts',(-4.29031348800006,2.2,0.484156920999985));
#311975=CARTESIAN_POINT('Ctrl Pts',(-4.28869395300006,12.2,0.483268814999986));
#311976=CARTESIAN_POINT('Ctrl Pts',(-4.28869395300006,5.2,0.483268814999986));
#311977=CARTESIAN_POINT('Ctrl Pts',(-4.28869395300006,2.2,0.483268814999986));
#311978=CARTESIAN_POINT('Ctrl Pts',(-4.28707715600006,12.2,0.482384579999984));
#311979=CARTESIAN_POINT('Ctrl Pts',(-4.28707715600006,5.2,0.482384579999984));
#311980=CARTESIAN_POINT('Ctrl Pts',(-4.28707715600006,2.2,0.482384579999984));
#311981=CARTESIAN_POINT('Ctrl Pts',(-4.28546310800006,12.2,0.481504210999986));
#311982=CARTESIAN_POINT('Ctrl Pts',(-4.28546310800006,5.2,0.481504210999986));
#311983=CARTESIAN_POINT('Ctrl Pts',(-4.28546310800006,2.2,0.481504210999986));
#311984=CARTESIAN_POINT('Ctrl Pts',(-4.28385181900006,12.2,0.480627706999983));
#311985=CARTESIAN_POINT('Ctrl Pts',(-4.28385181900006,5.2,0.480627706999983));
#311986=CARTESIAN_POINT('Ctrl Pts',(-4.28385181900006,2.2,0.480627706999983));
#311987=CARTESIAN_POINT('Ctrl Pts',(-4.28224330200006,12.2,0.479755061999985));
#311988=CARTESIAN_POINT('Ctrl Pts',(-4.28224330200006,5.2,0.479755061999985));
#311989=CARTESIAN_POINT('Ctrl Pts',(-4.28224330200006,2.2,0.479755061999985));
#311990=CARTESIAN_POINT('Ctrl Pts',(-4.28063756600006,12.2,0.478886270999985));
#311991=CARTESIAN_POINT('Ctrl Pts',(-4.28063756600006,5.2,0.478886270999985));
#311992=CARTESIAN_POINT('Ctrl Pts',(-4.28063756600006,2.2,0.478886270999985));
#311993=CARTESIAN_POINT('Ctrl Pts',(-4.27903462300006,12.2,0.478021332999985));
#311994=CARTESIAN_POINT('Ctrl Pts',(-4.27903462300006,5.2,0.478021332999985));
#311995=CARTESIAN_POINT('Ctrl Pts',(-4.27903462300006,2.2,0.478021332999985));
#311996=CARTESIAN_POINT('Ctrl Pts',(-4.27743448300006,12.2,0.477160242999983));
#311997=CARTESIAN_POINT('Ctrl Pts',(-4.27743448300006,5.2,0.477160242999983));
#311998=CARTESIAN_POINT('Ctrl Pts',(-4.27743448300006,2.2,0.477160242999983));
#311999=CARTESIAN_POINT('Ctrl Pts',(-4.27583715800006,12.2,0.476302994999984));
#312000=CARTESIAN_POINT('Ctrl Pts',(-4.27583715800006,5.2,0.476302994999984));
#312001=CARTESIAN_POINT('Ctrl Pts',(-4.27583715800006,2.2,0.476302994999984));
#312002=CARTESIAN_POINT('Ctrl Pts',(-4.27424265900005,12.2,0.475449585999983));
#312003=CARTESIAN_POINT('Ctrl Pts',(-4.27424265900005,5.2,0.475449585999983));
#312004=CARTESIAN_POINT('Ctrl Pts',(-4.27424265900005,2.2,0.475449585999983));
#312005=CARTESIAN_POINT('Ctrl Pts',(-4.27265099500006,12.2,0.474600012999984));
#312006=CARTESIAN_POINT('Ctrl Pts',(-4.27265099500006,5.2,0.474600012999984));
#312007=CARTESIAN_POINT('Ctrl Pts',(-4.27265099500006,2.2,0.474600012999984));
#312008=CARTESIAN_POINT('Ctrl Pts',(-4.27106218000006,12.2,0.473754269999986));
#312009=CARTESIAN_POINT('Ctrl Pts',(-4.27106218000006,5.2,0.473754269999986));
#312010=CARTESIAN_POINT('Ctrl Pts',(-4.27106218000006,2.2,0.473754269999986));
#312011=CARTESIAN_POINT('Ctrl Pts',(-4.26947622300006,12.2,0.472912353999986));
#312012=CARTESIAN_POINT('Ctrl Pts',(-4.26947622300006,5.2,0.472912353999986));
#312013=CARTESIAN_POINT('Ctrl Pts',(-4.26947622300006,2.2,0.472912353999986));
#312014=CARTESIAN_POINT('Ctrl Pts',(-4.26789313500006,12.2,0.472074260999986));
#312015=CARTESIAN_POINT('Ctrl Pts',(-4.26789313500006,5.2,0.472074260999986));
#312016=CARTESIAN_POINT('Ctrl Pts',(-4.26789313500006,2.2,0.472074260999986));
#312017=CARTESIAN_POINT('Ctrl Pts',(-4.26631292800006,12.2,0.471239985999983));
#312018=CARTESIAN_POINT('Ctrl Pts',(-4.26631292800006,5.2,0.471239985999983));
#312019=CARTESIAN_POINT('Ctrl Pts',(-4.26631292800006,2.2,0.471239985999983));
#312020=CARTESIAN_POINT('Ctrl Pts',(-4.26473561400006,12.2,0.470409523999984));
#312021=CARTESIAN_POINT('Ctrl Pts',(-4.26473561400006,5.2,0.470409523999984));
#312022=CARTESIAN_POINT('Ctrl Pts',(-4.26473561400006,2.2,0.470409523999984));
#312023=CARTESIAN_POINT('Ctrl Pts',(-4.26316120000005,12.2,0.469582871999985));
#312024=CARTESIAN_POINT('Ctrl Pts',(-4.26316120000005,5.2,0.469582871999985));
#312025=CARTESIAN_POINT('Ctrl Pts',(-4.26316120000005,2.2,0.469582871999985));
#312026=CARTESIAN_POINT('Ctrl Pts',(-4.26158970300006,12.2,0.468760025999986));
#312027=CARTESIAN_POINT('Ctrl Pts',(-4.26158970300006,5.2,0.468760025999986));
#312028=CARTESIAN_POINT('Ctrl Pts',(-4.26158970300006,2.2,0.468760025999986));
#312029=CARTESIAN_POINT('Ctrl Pts',(-4.26002112900006,12.2,0.467940980999986));
#312030=CARTESIAN_POINT('Ctrl Pts',(-4.26002112900006,5.2,0.467940980999986));
#312031=CARTESIAN_POINT('Ctrl Pts',(-4.26002112900006,2.2,0.467940980999986));
#312032=CARTESIAN_POINT('Ctrl Pts',(-4.25845549100006,12.2,0.467125732999989));
#312033=CARTESIAN_POINT('Ctrl Pts',(-4.25845549100006,5.2,0.467125732999989));
#312034=CARTESIAN_POINT('Ctrl Pts',(-4.25845549100006,2.2,0.467125732999989));
#312035=CARTESIAN_POINT('Ctrl Pts',(-4.25689280100006,12.2,0.466314275999986));
#312036=CARTESIAN_POINT('Ctrl Pts',(-4.25689280100006,5.2,0.466314275999986));
#312037=CARTESIAN_POINT('Ctrl Pts',(-4.25689280100006,2.2,0.466314275999986));
#312038=CARTESIAN_POINT('Ctrl Pts',(-4.25533306900006,12.2,0.465506608999986));
#312039=CARTESIAN_POINT('Ctrl Pts',(-4.25533306900006,5.2,0.465506608999986));
#312040=CARTESIAN_POINT('Ctrl Pts',(-4.25533306900006,2.2,0.465506608999986));
#312041=CARTESIAN_POINT('Ctrl Pts',(-4.25377630600006,12.2,0.464702724999988));
#312042=CARTESIAN_POINT('Ctrl Pts',(-4.25377630600006,5.2,0.464702724999988));
#312043=CARTESIAN_POINT('Ctrl Pts',(-4.25377630600006,2.2,0.464702724999988));
#312044=CARTESIAN_POINT('Ctrl Pts',(-4.25222252500006,12.2,0.463902618999987));
#312045=CARTESIAN_POINT('Ctrl Pts',(-4.25222252500006,5.2,0.463902618999987));
#312046=CARTESIAN_POINT('Ctrl Pts',(-4.25222252500006,2.2,0.463902618999987));
#312047=CARTESIAN_POINT('Ctrl Pts',(-4.25067173600006,12.2,0.463106288999988));
#312048=CARTESIAN_POINT('Ctrl Pts',(-4.25067173600006,5.2,0.463106288999988));
#312049=CARTESIAN_POINT('Ctrl Pts',(-4.25067173600006,2.2,0.463106288999988));
#312050=CARTESIAN_POINT('Ctrl Pts',(-4.24912394800006,12.2,0.462313728999986));
#312051=CARTESIAN_POINT('Ctrl Pts',(-4.24912394800006,5.2,0.462313728999986));
#312052=CARTESIAN_POINT('Ctrl Pts',(-4.24912394800006,2.2,0.462313728999986));
#312053=CARTESIAN_POINT('Ctrl Pts',(-4.24757917600005,12.2,0.461524934999984));
#312054=CARTESIAN_POINT('Ctrl Pts',(-4.24757917600005,5.2,0.461524934999984));
#312055=CARTESIAN_POINT('Ctrl Pts',(-4.24757917600005,2.2,0.461524934999984));
#312056=CARTESIAN_POINT('Ctrl Pts',(-4.24603742900006,12.2,0.460739901999982));
#312057=CARTESIAN_POINT('Ctrl Pts',(-4.24603742900006,5.2,0.460739901999982));
#312058=CARTESIAN_POINT('Ctrl Pts',(-4.24603742900006,2.2,0.460739901999982));
#312059=CARTESIAN_POINT('Ctrl Pts',(-4.24449871900006,12.2,0.459958625999985));
#312060=CARTESIAN_POINT('Ctrl Pts',(-4.24449871900006,5.2,0.459958625999985));
#312061=CARTESIAN_POINT('Ctrl Pts',(-4.24449871900006,2.2,0.459958625999985));
#312062=CARTESIAN_POINT('Ctrl Pts',(-4.24296305600006,12.2,0.459181101999988));
#312063=CARTESIAN_POINT('Ctrl Pts',(-4.24296305600006,5.2,0.459181101999988));
#312064=CARTESIAN_POINT('Ctrl Pts',(-4.24296305600006,2.2,0.459181101999988));
#312065=CARTESIAN_POINT('Ctrl Pts',(-4.24143045400006,12.2,0.458407324999985));
#312066=CARTESIAN_POINT('Ctrl Pts',(-4.24143045400006,5.2,0.458407324999985));
#312067=CARTESIAN_POINT('Ctrl Pts',(-4.24143045400006,2.2,0.458407324999985));
#312068=CARTESIAN_POINT('Ctrl Pts',(-4.23990092200006,12.2,0.457637290999986));
#312069=CARTESIAN_POINT('Ctrl Pts',(-4.23990092200006,5.2,0.457637290999986));
#312070=CARTESIAN_POINT('Ctrl Pts',(-4.23990092200006,2.2,0.457637290999986));
#312071=CARTESIAN_POINT('Ctrl Pts',(-4.23837447100006,12.2,0.456870996999985));
#312072=CARTESIAN_POINT('Ctrl Pts',(-4.23837447100006,5.2,0.456870996999985));
#312073=CARTESIAN_POINT('Ctrl Pts',(-4.23837447100006,2.2,0.456870996999985));
#312074=CARTESIAN_POINT('Ctrl Pts',(-4.23685111400006,12.2,0.456108434999987));
#312075=CARTESIAN_POINT('Ctrl Pts',(-4.23685111400006,5.2,0.456108434999987));
#312076=CARTESIAN_POINT('Ctrl Pts',(-4.23685111400006,2.2,0.456108434999987));
#312077=CARTESIAN_POINT('Ctrl Pts',(-4.23533086100006,12.2,0.455349602999986));
#312078=CARTESIAN_POINT('Ctrl Pts',(-4.23533086100006,5.2,0.455349602999986));
#312079=CARTESIAN_POINT('Ctrl Pts',(-4.23533086100006,2.2,0.455349602999986));
#312080=CARTESIAN_POINT('Ctrl Pts',(-4.23381372400006,12.2,0.454594492999987));
#312081=CARTESIAN_POINT('Ctrl Pts',(-4.23381372400006,5.2,0.454594492999987));
#312082=CARTESIAN_POINT('Ctrl Pts',(-4.23381372400006,2.2,0.454594492999987));
#312083=CARTESIAN_POINT('Ctrl Pts',(-4.23229971500006,12.2,0.453843104999985));
#312084=CARTESIAN_POINT('Ctrl Pts',(-4.23229971500006,5.2,0.453843104999985));
#312085=CARTESIAN_POINT('Ctrl Pts',(-4.23229971500006,2.2,0.453843104999985));
#312086=CARTESIAN_POINT('Ctrl Pts',(-4.23078884300006,12.2,0.453095430999984));
#312087=CARTESIAN_POINT('Ctrl Pts',(-4.23078884300006,5.2,0.453095430999984));
#312088=CARTESIAN_POINT('Ctrl Pts',(-4.23078884300006,2.2,0.453095430999984));
#312089=CARTESIAN_POINT('Ctrl Pts',(-4.22928112300006,12.2,0.452351465999987));
#312090=CARTESIAN_POINT('Ctrl Pts',(-4.22928112300006,5.2,0.452351465999987));
#312091=CARTESIAN_POINT('Ctrl Pts',(-4.22928112300006,2.2,0.452351465999987));
#312092=CARTESIAN_POINT('Ctrl Pts',(-4.22777656200005,12.2,0.451611206999987));
#312093=CARTESIAN_POINT('Ctrl Pts',(-4.22777656200005,5.2,0.451611206999987));
#312094=CARTESIAN_POINT('Ctrl Pts',(-4.22777656200005,2.2,0.451611206999987));
#312095=CARTESIAN_POINT('Ctrl Pts',(-4.22627517600006,12.2,0.450874648999986));
#312096=CARTESIAN_POINT('Ctrl Pts',(-4.22627517600006,5.2,0.450874648999986));
#312097=CARTESIAN_POINT('Ctrl Pts',(-4.22627517600006,2.2,0.450874648999986));
#312098=CARTESIAN_POINT('Ctrl Pts',(-4.22477697300006,12.2,0.450141784999989));
#312099=CARTESIAN_POINT('Ctrl Pts',(-4.22477697300006,5.2,0.450141784999989));
#312100=CARTESIAN_POINT('Ctrl Pts',(-4.22477697300006,2.2,0.450141784999989));
#312101=CARTESIAN_POINT('Ctrl Pts',(-4.22328196600006,12.2,0.449412612999982));
#312102=CARTESIAN_POINT('Ctrl Pts',(-4.22328196600006,5.2,0.449412612999982));
#312103=CARTESIAN_POINT('Ctrl Pts',(-4.22328196600006,2.2,0.449412612999982));
#312104=CARTESIAN_POINT('Ctrl Pts',(-4.22179016600006,12.2,0.448687124999987));
#312105=CARTESIAN_POINT('Ctrl Pts',(-4.22179016600006,5.2,0.448687124999987));
#312106=CARTESIAN_POINT('Ctrl Pts',(-4.22179016600006,2.2,0.448687124999987));
#312107=CARTESIAN_POINT('Ctrl Pts',(-4.22030158500006,12.2,0.447965318999985));
#312108=CARTESIAN_POINT('Ctrl Pts',(-4.22030158500006,5.2,0.447965318999985));
#312109=CARTESIAN_POINT('Ctrl Pts',(-4.22030158500006,2.2,0.447965318999985));
#312110=CARTESIAN_POINT('Ctrl Pts',(-4.21881623400005,12.2,0.447247188999986));
#312111=CARTESIAN_POINT('Ctrl Pts',(-4.21881623400005,5.2,0.447247188999986));
#312112=CARTESIAN_POINT('Ctrl Pts',(-4.21881623400005,2.2,0.447247188999986));
#312113=CARTESIAN_POINT('Ctrl Pts',(-4.21733412400005,12.2,0.446532728999984));
#312114=CARTESIAN_POINT('Ctrl Pts',(-4.21733412400005,5.2,0.446532728999984));
#312115=CARTESIAN_POINT('Ctrl Pts',(-4.21733412400005,2.2,0.446532728999984));
#312116=CARTESIAN_POINT('Ctrl Pts',(-4.21585526900006,12.2,0.445821935999984));
#312117=CARTESIAN_POINT('Ctrl Pts',(-4.21585526900006,5.2,0.445821935999984));
#312118=CARTESIAN_POINT('Ctrl Pts',(-4.21585526900006,2.2,0.445821935999984));
#312119=CARTESIAN_POINT('Ctrl Pts',(-4.21437967700006,12.2,0.445114802999989));
#312120=CARTESIAN_POINT('Ctrl Pts',(-4.21437967700006,5.2,0.445114802999989));
#312121=CARTESIAN_POINT('Ctrl Pts',(-4.21437967700006,2.2,0.445114802999989));
#312122=CARTESIAN_POINT('Ctrl Pts',(-4.21290736100006,12.2,0.444411324999985));
#312123=CARTESIAN_POINT('Ctrl Pts',(-4.21290736100006,5.2,0.444411324999985));
#312124=CARTESIAN_POINT('Ctrl Pts',(-4.21290736100006,2.2,0.444411324999985));
#312125=CARTESIAN_POINT('Ctrl Pts',(-4.21143833400006,12.2,0.443711497999986));
#312126=CARTESIAN_POINT('Ctrl Pts',(-4.21143833400006,5.2,0.443711497999986));
#312127=CARTESIAN_POINT('Ctrl Pts',(-4.21143833400006,2.2,0.443711497999986));
#312128=CARTESIAN_POINT('Ctrl Pts',(-4.20997260600006,12.2,0.443015316999986));
#312129=CARTESIAN_POINT('Ctrl Pts',(-4.20997260600006,5.2,0.443015316999986));
#312130=CARTESIAN_POINT('Ctrl Pts',(-4.20997260600006,2.2,0.443015316999986));
#312131=CARTESIAN_POINT('Ctrl Pts',(-4.20851018800006,12.2,0.442322775999986));
#312132=CARTESIAN_POINT('Ctrl Pts',(-4.20851018800006,5.2,0.442322775999986));
#312133=CARTESIAN_POINT('Ctrl Pts',(-4.20851018800006,2.2,0.442322775999986));
#312134=CARTESIAN_POINT('Ctrl Pts',(-4.20705109400005,12.2,0.441633870999985));
#312135=CARTESIAN_POINT('Ctrl Pts',(-4.20705109400005,5.2,0.441633870999985));
#312136=CARTESIAN_POINT('Ctrl Pts',(-4.20705109400005,2.2,0.441633870999985));
#312137=CARTESIAN_POINT('Ctrl Pts',(-4.20559533300006,12.2,0.440948595999986));
#312138=CARTESIAN_POINT('Ctrl Pts',(-4.20559533300006,5.2,0.440948595999986));
#312139=CARTESIAN_POINT('Ctrl Pts',(-4.20559533300006,2.2,0.440948595999986));
#312140=CARTESIAN_POINT('Ctrl Pts',(-4.20414291800006,12.2,0.440266945999985));
#312141=CARTESIAN_POINT('Ctrl Pts',(-4.20414291800006,5.2,0.440266945999985));
#312142=CARTESIAN_POINT('Ctrl Pts',(-4.20414291800006,2.2,0.440266945999985));
#312143=CARTESIAN_POINT('Ctrl Pts',(-4.20269386100006,12.2,0.439588913999986));
#312144=CARTESIAN_POINT('Ctrl Pts',(-4.20269386100006,5.2,0.439588913999986));
#312145=CARTESIAN_POINT('Ctrl Pts',(-4.20269386100006,2.2,0.439588913999986));
#312146=CARTESIAN_POINT('Ctrl Pts',(-4.20124817300006,12.2,0.438914497999985));
#312147=CARTESIAN_POINT('Ctrl Pts',(-4.20124817300006,5.2,0.438914497999985));
#312148=CARTESIAN_POINT('Ctrl Pts',(-4.20124817300006,2.2,0.438914497999985));
#312149=CARTESIAN_POINT('Ctrl Pts',(-4.19980586600006,12.2,0.438243690999984));
#312150=CARTESIAN_POINT('Ctrl Pts',(-4.19980586600006,5.2,0.438243690999984));
#312151=CARTESIAN_POINT('Ctrl Pts',(-4.19980586600006,2.2,0.438243690999984));
#312152=CARTESIAN_POINT('Ctrl Pts',(-4.19836695100006,12.2,0.437576486999984));
#312153=CARTESIAN_POINT('Ctrl Pts',(-4.19836695100006,5.2,0.437576486999984));
#312154=CARTESIAN_POINT('Ctrl Pts',(-4.19836695100006,2.2,0.437576486999984));
#312155=CARTESIAN_POINT('Ctrl Pts',(-4.19693144100005,12.2,0.436912881999985));
#312156=CARTESIAN_POINT('Ctrl Pts',(-4.19693144100005,5.2,0.436912881999985));
#312157=CARTESIAN_POINT('Ctrl Pts',(-4.19693144100005,2.2,0.436912881999985));
#312158=CARTESIAN_POINT('Ctrl Pts',(-4.19549934600006,12.2,0.436252869999985));
#312159=CARTESIAN_POINT('Ctrl Pts',(-4.19549934600006,5.2,0.436252869999985));
#312160=CARTESIAN_POINT('Ctrl Pts',(-4.19549934600006,2.2,0.436252869999985));
#312161=CARTESIAN_POINT('Ctrl Pts',(-4.19407068000006,12.2,0.435596445999984));
#312162=CARTESIAN_POINT('Ctrl Pts',(-4.19407068000006,5.2,0.435596445999984));
#312163=CARTESIAN_POINT('Ctrl Pts',(-4.19407068000006,2.2,0.435596445999984));
#312164=CARTESIAN_POINT('Ctrl Pts',(-4.19264545300006,12.2,0.434943603999987));
#312165=CARTESIAN_POINT('Ctrl Pts',(-4.19264545300006,5.2,0.434943603999987));
#312166=CARTESIAN_POINT('Ctrl Pts',(-4.19264545300006,2.2,0.434943603999987));
#312167=CARTESIAN_POINT('Ctrl Pts',(-4.19122367800006,12.2,0.434294338999983));
#312168=CARTESIAN_POINT('Ctrl Pts',(-4.19122367800006,5.2,0.434294338999983));
#312169=CARTESIAN_POINT('Ctrl Pts',(-4.19122367800006,2.2,0.434294338999983));
#312170=CARTESIAN_POINT('Ctrl Pts',(-4.18980536500006,12.2,0.433648644999987));
#312171=CARTESIAN_POINT('Ctrl Pts',(-4.18980536500006,5.2,0.433648644999987));
#312172=CARTESIAN_POINT('Ctrl Pts',(-4.18980536500006,2.2,0.433648644999987));
#312173=CARTESIAN_POINT('Ctrl Pts',(-4.18839052700006,12.2,0.433006516999987));
#312174=CARTESIAN_POINT('Ctrl Pts',(-4.18839052700006,5.2,0.433006516999987));
#312175=CARTESIAN_POINT('Ctrl Pts',(-4.18839052700006,2.2,0.433006516999987));
#312176=CARTESIAN_POINT('Ctrl Pts',(-4.18697917600006,12.2,0.432367948999985));
#312177=CARTESIAN_POINT('Ctrl Pts',(-4.18697917600006,5.2,0.432367948999985));
#312178=CARTESIAN_POINT('Ctrl Pts',(-4.18697917600006,2.2,0.432367948999985));
#312179=CARTESIAN_POINT('Ctrl Pts',(-4.18557132400006,12.2,0.431732936999989));
#312180=CARTESIAN_POINT('Ctrl Pts',(-4.18557132400006,5.2,0.431732936999989));
#312181=CARTESIAN_POINT('Ctrl Pts',(-4.18557132400006,2.2,0.431732936999989));
#312182=CARTESIAN_POINT('Ctrl Pts',(-4.18416698300006,12.2,0.431101472999984));
#312183=CARTESIAN_POINT('Ctrl Pts',(-4.18416698300006,5.2,0.431101472999984));
#312184=CARTESIAN_POINT('Ctrl Pts',(-4.18416698300006,2.2,0.431101472999984));
#312185=CARTESIAN_POINT('Ctrl Pts',(-4.18276616300005,12.2,0.430473553999988));
#312186=CARTESIAN_POINT('Ctrl Pts',(-4.18276616300005,5.2,0.430473553999988));
#312187=CARTESIAN_POINT('Ctrl Pts',(-4.18276616300005,2.2,0.430473553999988));
#312188=CARTESIAN_POINT('Ctrl Pts',(-4.18136887800006,12.2,0.429849171999983));
#312189=CARTESIAN_POINT('Ctrl Pts',(-4.18136887800006,5.2,0.429849171999983));
#312190=CARTESIAN_POINT('Ctrl Pts',(-4.18136887800006,2.2,0.429849171999983));
#312191=CARTESIAN_POINT('Ctrl Pts',(-4.17997513800006,12.2,0.429228321999986));
#312192=CARTESIAN_POINT('Ctrl Pts',(-4.17997513800006,5.2,0.429228321999986));
#312193=CARTESIAN_POINT('Ctrl Pts',(-4.17997513800006,2.2,0.429228321999986));
#312194=CARTESIAN_POINT('Ctrl Pts',(-4.17858495700006,12.2,0.428610999999983));
#312195=CARTESIAN_POINT('Ctrl Pts',(-4.17858495700006,5.2,0.428610999999983));
#312196=CARTESIAN_POINT('Ctrl Pts',(-4.17858495700006,2.2,0.428610999999983));
#312197=CARTESIAN_POINT('Ctrl Pts',(-4.17719834700006,12.2,0.427997197999983));
#312198=CARTESIAN_POINT('Ctrl Pts',(-4.17719834700006,5.2,0.427997197999983));
#312199=CARTESIAN_POINT('Ctrl Pts',(-4.17719834700006,2.2,0.427997197999983));
#312200=CARTESIAN_POINT('Ctrl Pts',(-4.17581531700006,12.2,0.427386910999985));
#312201=CARTESIAN_POINT('Ctrl Pts',(-4.17581531700006,5.2,0.427386910999985));
#312202=CARTESIAN_POINT('Ctrl Pts',(-4.17581531700006,2.2,0.427386910999985));
#312203=CARTESIAN_POINT('Ctrl Pts',(-4.17443588200006,12.2,0.426780132999984));
#312204=CARTESIAN_POINT('Ctrl Pts',(-4.17443588200006,5.2,0.426780132999984));
#312205=CARTESIAN_POINT('Ctrl Pts',(-4.17443588200006,2.2,0.426780132999984));
#312206=CARTESIAN_POINT('Ctrl Pts',(-4.17306005300006,12.2,0.426176860999985));
#312207=CARTESIAN_POINT('Ctrl Pts',(-4.17306005300006,5.2,0.426176860999985));
#312208=CARTESIAN_POINT('Ctrl Pts',(-4.17306005300006,2.2,0.426176860999985));
#312209=CARTESIAN_POINT('Ctrl Pts',(-4.17168784100006,12.2,0.425577084999986));
#312210=CARTESIAN_POINT('Ctrl Pts',(-4.17168784100006,5.2,0.425577084999986));
#312211=CARTESIAN_POINT('Ctrl Pts',(-4.17168784100006,2.2,0.425577084999986));
#312212=CARTESIAN_POINT('Ctrl Pts',(-4.17031926000006,12.2,0.424980800999983));
#312213=CARTESIAN_POINT('Ctrl Pts',(-4.17031926000006,5.2,0.424980800999983));
#312214=CARTESIAN_POINT('Ctrl Pts',(-4.17031926000006,2.2,0.424980800999983));
#312215=CARTESIAN_POINT('Ctrl Pts',(-4.16895432100006,12.2,0.424388002999985));
#312216=CARTESIAN_POINT('Ctrl Pts',(-4.16895432100006,5.2,0.424388002999985));
#312217=CARTESIAN_POINT('Ctrl Pts',(-4.16895432100006,2.2,0.424388002999985));
#312218=CARTESIAN_POINT('Ctrl Pts',(-4.16759303600006,12.2,0.423798685999985));
#312219=CARTESIAN_POINT('Ctrl Pts',(-4.16759303600006,5.2,0.423798685999985));
#312220=CARTESIAN_POINT('Ctrl Pts',(-4.16759303600006,2.2,0.423798685999985));
#312221=CARTESIAN_POINT('Ctrl Pts',(-4.16623541600006,12.2,0.423212842999985));
#312222=CARTESIAN_POINT('Ctrl Pts',(-4.16623541600006,5.2,0.423212842999985));
#312223=CARTESIAN_POINT('Ctrl Pts',(-4.16623541600006,2.2,0.423212842999985));
#312224=CARTESIAN_POINT('Ctrl Pts',(-4.16488147500006,12.2,0.422630467999987));
#312225=CARTESIAN_POINT('Ctrl Pts',(-4.16488147500006,5.2,0.422630467999987));
#312226=CARTESIAN_POINT('Ctrl Pts',(-4.16488147500006,2.2,0.422630467999987));
#312227=CARTESIAN_POINT('Ctrl Pts',(-4.16353122500006,12.2,0.422051554999987));
#312228=CARTESIAN_POINT('Ctrl Pts',(-4.16353122500006,5.2,0.422051554999987));
#312229=CARTESIAN_POINT('Ctrl Pts',(-4.16353122500006,2.2,0.422051554999987));
#312230=CARTESIAN_POINT('Ctrl Pts',(-4.16218467700006,12.2,0.421476099999989));
#312231=CARTESIAN_POINT('Ctrl Pts',(-4.16218467700006,5.2,0.421476099999989));
#312232=CARTESIAN_POINT('Ctrl Pts',(-4.16218467700006,2.2,0.421476099999989));
#312233=CARTESIAN_POINT('Ctrl Pts',(-4.16084184200006,12.2,0.420904093999983));
#312234=CARTESIAN_POINT('Ctrl Pts',(-4.16084184200006,5.2,0.420904093999983));
#312235=CARTESIAN_POINT('Ctrl Pts',(-4.16084184200006,2.2,0.420904093999983));
#312236=CARTESIAN_POINT('Ctrl Pts',(-4.15950273600005,12.2,0.420335532999987));
#312237=CARTESIAN_POINT('Ctrl Pts',(-4.15950273600005,5.2,0.420335532999987));
#312238=CARTESIAN_POINT('Ctrl Pts',(-4.15950273600005,2.2,0.420335532999987));
#312239=CARTESIAN_POINT('Ctrl Pts',(-4.15816736800006,12.2,0.419770408999987));
#312240=CARTESIAN_POINT('Ctrl Pts',(-4.15816736800006,5.2,0.419770408999987));
#312241=CARTESIAN_POINT('Ctrl Pts',(-4.15816736800006,2.2,0.419770408999987));
#312242=CARTESIAN_POINT('Ctrl Pts',(-4.15683575100006,12.2,0.419208716999986));
#312243=CARTESIAN_POINT('Ctrl Pts',(-4.15683575100006,5.2,0.419208716999986));
#312244=CARTESIAN_POINT('Ctrl Pts',(-4.15683575100006,2.2,0.419208716999986));
#312245=CARTESIAN_POINT('Ctrl Pts',(-4.15550789700006,12.2,0.418650450999984));
#312246=CARTESIAN_POINT('Ctrl Pts',(-4.15550789700006,5.2,0.418650450999984));
#312247=CARTESIAN_POINT('Ctrl Pts',(-4.15550789700006,2.2,0.418650450999984));
#312248=CARTESIAN_POINT('Ctrl Pts',(-4.15418381900006,12.2,0.418095605999986));
#312249=CARTESIAN_POINT('Ctrl Pts',(-4.15418381900006,5.2,0.418095605999986));
#312250=CARTESIAN_POINT('Ctrl Pts',(-4.15418381900006,2.2,0.418095605999986));
#312251=CARTESIAN_POINT('Ctrl Pts',(-4.15286352900006,12.2,0.417544172999986));
#312252=CARTESIAN_POINT('Ctrl Pts',(-4.15286352900006,5.2,0.417544172999986));
#312253=CARTESIAN_POINT('Ctrl Pts',(-4.15286352900006,2.2,0.417544172999986));
#312254=CARTESIAN_POINT('Ctrl Pts',(-4.15154703900006,12.2,0.416996146999988));
#312255=CARTESIAN_POINT('Ctrl Pts',(-4.15154703900006,5.2,0.416996146999988));
#312256=CARTESIAN_POINT('Ctrl Pts',(-4.15154703900006,2.2,0.416996146999988));
#312257=CARTESIAN_POINT('Ctrl Pts',(-4.15023436000006,12.2,0.416451522999988));
#312258=CARTESIAN_POINT('Ctrl Pts',(-4.15023436000006,5.2,0.416451522999988));
#312259=CARTESIAN_POINT('Ctrl Pts',(-4.15023436000006,2.2,0.416451522999988));
#312260=CARTESIAN_POINT('Ctrl Pts',(-4.14892550700006,12.2,0.415910292999988));
#312261=CARTESIAN_POINT('Ctrl Pts',(-4.14892550700006,5.2,0.415910292999988));
#312262=CARTESIAN_POINT('Ctrl Pts',(-4.14892550700006,2.2,0.415910292999988));
#312263=CARTESIAN_POINT('Ctrl Pts',(-4.14762049000006,12.2,0.415372450999989));
#312264=CARTESIAN_POINT('Ctrl Pts',(-4.14762049000006,5.2,0.415372450999989));
#312265=CARTESIAN_POINT('Ctrl Pts',(-4.14762049000006,2.2,0.415372450999989));
#312266=CARTESIAN_POINT('Ctrl Pts',(-4.14631932300006,12.2,0.414837989999985));
#312267=CARTESIAN_POINT('Ctrl Pts',(-4.14631932300006,5.2,0.414837989999985));
#312268=CARTESIAN_POINT('Ctrl Pts',(-4.14631932300006,2.2,0.414837989999985));
#312269=CARTESIAN_POINT('Ctrl Pts',(-4.14502201700006,12.2,0.414306905999986));
#312270=CARTESIAN_POINT('Ctrl Pts',(-4.14502201700006,5.2,0.414306905999986));
#312271=CARTESIAN_POINT('Ctrl Pts',(-4.14502201700006,2.2,0.414306905999986));
#312272=CARTESIAN_POINT('Ctrl Pts',(-4.14372858500006,12.2,0.413779189999985));
#312273=CARTESIAN_POINT('Ctrl Pts',(-4.14372858500006,5.2,0.413779189999985));
#312274=CARTESIAN_POINT('Ctrl Pts',(-4.14372858500006,2.2,0.413779189999985));
#312275=CARTESIAN_POINT('Ctrl Pts',(-4.14243904000006,12.2,0.413254837999983));
#312276=CARTESIAN_POINT('Ctrl Pts',(-4.14243904000006,5.2,0.413254837999983));
#312277=CARTESIAN_POINT('Ctrl Pts',(-4.14243904000006,2.2,0.413254837999983));
#312278=CARTESIAN_POINT('Ctrl Pts',(-4.14115339200006,12.2,0.412733840999984));
#312279=CARTESIAN_POINT('Ctrl Pts',(-4.14115339200006,5.2,0.412733840999984));
#312280=CARTESIAN_POINT('Ctrl Pts',(-4.14115339200006,2.2,0.412733840999984));
#312281=CARTESIAN_POINT('Ctrl Pts',(-4.13987165700005,12.2,0.412216192999986));
#312282=CARTESIAN_POINT('Ctrl Pts',(-4.13987165700005,5.2,0.412216192999986));
#312283=CARTESIAN_POINT('Ctrl Pts',(-4.13987165700005,2.2,0.412216192999986));
#312284=CARTESIAN_POINT('Ctrl Pts',(-4.13859384500006,12.2,0.411701888999985));
#312285=CARTESIAN_POINT('Ctrl Pts',(-4.13859384500006,5.2,0.411701888999985));
#312286=CARTESIAN_POINT('Ctrl Pts',(-4.13859384500006,2.2,0.411701888999985));
#312287=CARTESIAN_POINT('Ctrl Pts',(-4.13731996800006,12.2,0.411190921999989));
#312288=CARTESIAN_POINT('Ctrl Pts',(-4.13731996800006,5.2,0.411190921999989));
#312289=CARTESIAN_POINT('Ctrl Pts',(-4.13731996800006,2.2,0.411190921999989));
#312290=CARTESIAN_POINT('Ctrl Pts',(-4.13605004100006,12.2,0.410683283999984));
#312291=CARTESIAN_POINT('Ctrl Pts',(-4.13605004100006,5.2,0.410683283999984));
#312292=CARTESIAN_POINT('Ctrl Pts',(-4.13605004100006,2.2,0.410683283999984));
#312293=CARTESIAN_POINT('Ctrl Pts',(-4.13478407400006,12.2,0.410178968999984));
#312294=CARTESIAN_POINT('Ctrl Pts',(-4.13478407400006,5.2,0.410178968999984));
#312295=CARTESIAN_POINT('Ctrl Pts',(-4.13478407400006,2.2,0.410178968999984));
#312296=CARTESIAN_POINT('Ctrl Pts',(-4.13352208100005,12.2,0.409677971999987));
#312297=CARTESIAN_POINT('Ctrl Pts',(-4.13352208100005,5.2,0.409677971999987));
#312298=CARTESIAN_POINT('Ctrl Pts',(-4.13352208100005,2.2,0.409677971999987));
#312299=CARTESIAN_POINT('Ctrl Pts',(-4.13226407400006,12.2,0.409180282999984));
#312300=CARTESIAN_POINT('Ctrl Pts',(-4.13226407400006,5.2,0.409180282999984));
#312301=CARTESIAN_POINT('Ctrl Pts',(-4.13226407400006,2.2,0.409180282999984));
#312302=CARTESIAN_POINT('Ctrl Pts',(-4.13101006500006,12.2,0.408685896999987));
#312303=CARTESIAN_POINT('Ctrl Pts',(-4.13101006500006,5.2,0.408685896999987));
#312304=CARTESIAN_POINT('Ctrl Pts',(-4.13101006500006,2.2,0.408685896999987));
#312305=CARTESIAN_POINT('Ctrl Pts',(-4.12976006700006,12.2,0.408194807999984));
#312306=CARTESIAN_POINT('Ctrl Pts',(-4.12976006700006,5.2,0.408194807999984));
#312307=CARTESIAN_POINT('Ctrl Pts',(-4.12976006700006,2.2,0.408194807999984));
#312308=CARTESIAN_POINT('Ctrl Pts',(-4.12851409300006,12.2,0.407707009999987));
#312309=CARTESIAN_POINT('Ctrl Pts',(-4.12851409300006,5.2,0.407707009999987));
#312310=CARTESIAN_POINT('Ctrl Pts',(-4.12851409300006,2.2,0.407707009999987));
#312311=CARTESIAN_POINT('Ctrl Pts',(-4.12727215600006,12.2,0.407222493999986));
#312312=CARTESIAN_POINT('Ctrl Pts',(-4.12727215600006,5.2,0.407222493999986));
#312313=CARTESIAN_POINT('Ctrl Pts',(-4.12727215600006,2.2,0.407222493999986));
#312314=CARTESIAN_POINT('Ctrl Pts',(-4.12603426700006,12.2,0.406741251999985));
#312315=CARTESIAN_POINT('Ctrl Pts',(-4.12603426700006,5.2,0.406741251999985));
#312316=CARTESIAN_POINT('Ctrl Pts',(-4.12603426700006,2.2,0.406741251999985));
#312317=CARTESIAN_POINT('Ctrl Pts',(-4.12480043900006,12.2,0.406263280999983));
#312318=CARTESIAN_POINT('Ctrl Pts',(-4.12480043900006,5.2,0.406263280999983));
#312319=CARTESIAN_POINT('Ctrl Pts',(-4.12480043900006,2.2,0.406263280999983));
#312320=CARTESIAN_POINT('Ctrl Pts',(-4.12357068700006,12.2,0.405788570999985));
#312321=CARTESIAN_POINT('Ctrl Pts',(-4.12357068700006,5.2,0.405788570999985));
#312322=CARTESIAN_POINT('Ctrl Pts',(-4.12357068700006,2.2,0.405788570999985));
#312323=CARTESIAN_POINT('Ctrl Pts',(-4.12234502000006,12.2,0.405317116999986));
#312324=CARTESIAN_POINT('Ctrl Pts',(-4.12234502000006,5.2,0.405317116999986));
#312325=CARTESIAN_POINT('Ctrl Pts',(-4.12234502000006,2.2,0.405317116999986));
#312326=CARTESIAN_POINT('Ctrl Pts',(-4.12112345300006,12.2,0.404848910999984));
#312327=CARTESIAN_POINT('Ctrl Pts',(-4.12112345300006,5.2,0.404848910999984));
#312328=CARTESIAN_POINT('Ctrl Pts',(-4.12112345300006,2.2,0.404848910999984));
#312329=CARTESIAN_POINT('Ctrl Pts',(-4.11990599800006,12.2,0.404383944999989));
#312330=CARTESIAN_POINT('Ctrl Pts',(-4.11990599800006,5.2,0.404383944999989));
#312331=CARTESIAN_POINT('Ctrl Pts',(-4.11990599800006,2.2,0.404383944999989));
#312332=CARTESIAN_POINT('Ctrl Pts',(-4.11869266800006,12.2,0.403922214999985));
#312333=CARTESIAN_POINT('Ctrl Pts',(-4.11869266800006,5.2,0.403922214999985));
#312334=CARTESIAN_POINT('Ctrl Pts',(-4.11869266800006,2.2,0.403922214999985));
#312335=CARTESIAN_POINT('Ctrl Pts',(-4.11748347700006,12.2,0.403463710999983));
#312336=CARTESIAN_POINT('Ctrl Pts',(-4.11748347700006,5.2,0.403463710999983));
#312337=CARTESIAN_POINT('Ctrl Pts',(-4.11748347700006,2.2,0.403463710999983));
#312338=CARTESIAN_POINT('Ctrl Pts',(-4.11627843400006,12.2,0.403008425999989));
#312339=CARTESIAN_POINT('Ctrl Pts',(-4.11627843400006,5.2,0.403008425999989));
#312340=CARTESIAN_POINT('Ctrl Pts',(-4.11627843400006,2.2,0.403008425999989));
#312341=CARTESIAN_POINT('Ctrl Pts',(-4.11507755600006,12.2,0.402556355999986));
#312342=CARTESIAN_POINT('Ctrl Pts',(-4.11507755600006,5.2,0.402556355999986));
#312343=CARTESIAN_POINT('Ctrl Pts',(-4.11507755600006,2.2,0.402556355999986));
#312344=CARTESIAN_POINT('Ctrl Pts',(-4.11388085400006,12.2,0.402107488999985));
#312345=CARTESIAN_POINT('Ctrl Pts',(-4.11388085400006,5.2,0.402107488999985));
#312346=CARTESIAN_POINT('Ctrl Pts',(-4.11388085400006,2.2,0.402107488999985));
#312347=CARTESIAN_POINT('Ctrl Pts',(-4.11268834000006,12.2,0.401661821999983));
#312348=CARTESIAN_POINT('Ctrl Pts',(-4.11268834000006,5.2,0.401661821999983));
#312349=CARTESIAN_POINT('Ctrl Pts',(-4.11268834000006,2.2,0.401661821999983));
#312350=CARTESIAN_POINT('Ctrl Pts',(-4.11150002900006,12.2,0.401219345999984));
#312351=CARTESIAN_POINT('Ctrl Pts',(-4.11150002900006,5.2,0.401219345999984));
#312352=CARTESIAN_POINT('Ctrl Pts',(-4.11150002900006,2.2,0.401219345999984));
#312353=CARTESIAN_POINT('Ctrl Pts',(-4.11031593100006,12.2,0.400780052999985));
#312354=CARTESIAN_POINT('Ctrl Pts',(-4.11031593100006,5.2,0.400780052999985));
#312355=CARTESIAN_POINT('Ctrl Pts',(-4.11031593100006,2.2,0.400780052999985));
#312356=CARTESIAN_POINT('Ctrl Pts',(-4.10913606200006,12.2,0.400343936999987));
#312357=CARTESIAN_POINT('Ctrl Pts',(-4.10913606200006,5.2,0.400343936999987));
#312358=CARTESIAN_POINT('Ctrl Pts',(-4.10913606200006,2.2,0.400343936999987));
#312359=CARTESIAN_POINT('Ctrl Pts',(-4.10796043200006,12.2,0.399910990999985));
#312360=CARTESIAN_POINT('Ctrl Pts',(-4.10796043200006,5.2,0.399910990999985));
#312361=CARTESIAN_POINT('Ctrl Pts',(-4.10796043200006,2.2,0.399910990999985));
#312362=CARTESIAN_POINT('Ctrl Pts',(-4.10678905500006,12.2,0.399481205999983));
#312363=CARTESIAN_POINT('Ctrl Pts',(-4.10678905500006,5.2,0.399481205999983));
#312364=CARTESIAN_POINT('Ctrl Pts',(-4.10678905500006,2.2,0.399481205999983));
#312365=CARTESIAN_POINT('Ctrl Pts',(-4.10562194600006,12.2,0.399054574999984));
#312366=CARTESIAN_POINT('Ctrl Pts',(-4.10562194600006,5.2,0.399054574999984));
#312367=CARTESIAN_POINT('Ctrl Pts',(-4.10562194600006,2.2,0.399054574999984));
#312368=CARTESIAN_POINT('Ctrl Pts',(-4.10445911400006,12.2,0.398631090999988));
#312369=CARTESIAN_POINT('Ctrl Pts',(-4.10445911400006,5.2,0.398631090999988));
#312370=CARTESIAN_POINT('Ctrl Pts',(-4.10445911400006,2.2,0.398631090999988));
#312371=CARTESIAN_POINT('Ctrl Pts',(-4.10330057500006,12.2,0.398210746999985));
#312372=CARTESIAN_POINT('Ctrl Pts',(-4.10330057500006,5.2,0.398210746999985));
#312373=CARTESIAN_POINT('Ctrl Pts',(-4.10330057500006,2.2,0.398210746999985));
#312374=CARTESIAN_POINT('Ctrl Pts',(-4.10214634100006,12.2,0.397793535999984));
#312375=CARTESIAN_POINT('Ctrl Pts',(-4.10214634100006,5.2,0.397793535999984));
#312376=CARTESIAN_POINT('Ctrl Pts',(-4.10214634100006,2.2,0.397793535999984));
#312377=CARTESIAN_POINT('Ctrl Pts',(-4.10099642600006,12.2,0.397379447999988));
#312378=CARTESIAN_POINT('Ctrl Pts',(-4.10099642600006,5.2,0.397379447999988));
#312379=CARTESIAN_POINT('Ctrl Pts',(-4.10099642600006,2.2,0.397379447999988));
#312380=CARTESIAN_POINT('Ctrl Pts',(-4.09985084100006,12.2,0.396968477999984));
#312381=CARTESIAN_POINT('Ctrl Pts',(-4.09985084100006,5.2,0.396968477999984));
#312382=CARTESIAN_POINT('Ctrl Pts',(-4.09985084100006,2.2,0.396968477999984));
#312383=CARTESIAN_POINT('Ctrl Pts',(-4.09870960100006,12.2,0.396560615999988));
#312384=CARTESIAN_POINT('Ctrl Pts',(-4.09870960100006,5.2,0.396560615999988));
#312385=CARTESIAN_POINT('Ctrl Pts',(-4.09870960100006,2.2,0.396560615999988));
#312386=CARTESIAN_POINT('Ctrl Pts',(-4.09757271700006,12.2,0.396155855999982));
#312387=CARTESIAN_POINT('Ctrl Pts',(-4.09757271700006,5.2,0.396155855999982));
#312388=CARTESIAN_POINT('Ctrl Pts',(-4.09757271700006,2.2,0.396155855999982));
#312389=CARTESIAN_POINT('Ctrl Pts',(-4.09644020500005,12.2,0.395754189999984));
#312390=CARTESIAN_POINT('Ctrl Pts',(-4.09644020500005,5.2,0.395754189999984));
#312391=CARTESIAN_POINT('Ctrl Pts',(-4.09644020500005,2.2,0.395754189999984));
#312392=CARTESIAN_POINT('Ctrl Pts',(-4.09531207500006,12.2,0.395355609999988));
#312393=CARTESIAN_POINT('Ctrl Pts',(-4.09531207500006,5.2,0.395355609999988));
#312394=CARTESIAN_POINT('Ctrl Pts',(-4.09531207500006,2.2,0.395355609999988));
#312395=CARTESIAN_POINT('Ctrl Pts',(-4.09418834200006,12.2,0.394960108999989));
#312396=CARTESIAN_POINT('Ctrl Pts',(-4.09418834200006,5.2,0.394960108999989));
#312397=CARTESIAN_POINT('Ctrl Pts',(-4.09418834200006,2.2,0.394960108999989));
#312398=CARTESIAN_POINT('Ctrl Pts',(-4.09306901900006,12.2,0.394567677999986));
#312399=CARTESIAN_POINT('Ctrl Pts',(-4.09306901900006,5.2,0.394567677999986));
#312400=CARTESIAN_POINT('Ctrl Pts',(-4.09306901900006,2.2,0.394567677999986));
#312401=CARTESIAN_POINT('Ctrl Pts',(-4.09195411900006,12.2,0.394178310999984));
#312402=CARTESIAN_POINT('Ctrl Pts',(-4.09195411900006,5.2,0.394178310999984));
#312403=CARTESIAN_POINT('Ctrl Pts',(-4.09195411900006,2.2,0.394178310999984));
#312404=CARTESIAN_POINT('Ctrl Pts',(-4.09084365500005,12.2,0.393791997999986));
#312405=CARTESIAN_POINT('Ctrl Pts',(-4.09084365500005,5.2,0.393791997999986));
#312406=CARTESIAN_POINT('Ctrl Pts',(-4.09084365500005,2.2,0.393791997999986));
#312407=CARTESIAN_POINT('Ctrl Pts',(-4.08973764100006,12.2,0.393408731999987));
#312408=CARTESIAN_POINT('Ctrl Pts',(-4.08973764100006,5.2,0.393408731999987));
#312409=CARTESIAN_POINT('Ctrl Pts',(-4.08973764100006,2.2,0.393408731999987));
#312410=CARTESIAN_POINT('Ctrl Pts',(-4.08863608900006,12.2,0.393028504999986));
#312411=CARTESIAN_POINT('Ctrl Pts',(-4.08863608900006,5.2,0.393028504999986));
#312412=CARTESIAN_POINT('Ctrl Pts',(-4.08863608900006,2.2,0.393028504999986));
#312413=CARTESIAN_POINT('Ctrl Pts',(-4.08753901300006,12.2,0.392651309999987));
#312414=CARTESIAN_POINT('Ctrl Pts',(-4.08753901300006,5.2,0.392651309999987));
#312415=CARTESIAN_POINT('Ctrl Pts',(-4.08753901300006,2.2,0.392651309999987));
#312416=CARTESIAN_POINT('Ctrl Pts',(-4.08644642600006,12.2,0.392277137999986));
#312417=CARTESIAN_POINT('Ctrl Pts',(-4.08644642600006,5.2,0.392277137999986));
#312418=CARTESIAN_POINT('Ctrl Pts',(-4.08644642600006,2.2,0.392277137999986));
#312419=CARTESIAN_POINT('Ctrl Pts',(-4.08535834100006,12.2,0.391905980999985));
#312420=CARTESIAN_POINT('Ctrl Pts',(-4.08535834100006,5.2,0.391905980999985));
#312421=CARTESIAN_POINT('Ctrl Pts',(-4.08535834100006,2.2,0.391905980999985));
#312422=CARTESIAN_POINT('Ctrl Pts',(-4.08427477300005,12.2,0.391537830999984));
#312423=CARTESIAN_POINT('Ctrl Pts',(-4.08427477300005,5.2,0.391537830999984));
#312424=CARTESIAN_POINT('Ctrl Pts',(-4.08427477300005,2.2,0.391537830999984));
#312425=CARTESIAN_POINT('Ctrl Pts',(-4.08319573300005,12.2,0.391172679999983));
#312426=CARTESIAN_POINT('Ctrl Pts',(-4.08319573300005,5.2,0.391172679999983));
#312427=CARTESIAN_POINT('Ctrl Pts',(-4.08319573300005,2.2,0.391172679999983));
#312428=CARTESIAN_POINT('Ctrl Pts',(-4.08212123500006,12.2,0.390810519999985));
#312429=CARTESIAN_POINT('Ctrl Pts',(-4.08212123500006,5.2,0.390810519999985));
#312430=CARTESIAN_POINT('Ctrl Pts',(-4.08212123500006,2.2,0.390810519999985));
#312431=CARTESIAN_POINT('Ctrl Pts',(-4.08105129400006,12.2,0.390451341999984));
#312432=CARTESIAN_POINT('Ctrl Pts',(-4.08105129400006,5.2,0.390451341999984));
#312433=CARTESIAN_POINT('Ctrl Pts',(-4.08105129400006,2.2,0.390451341999984));
#312434=CARTESIAN_POINT('Ctrl Pts',(-4.07998592200006,12.2,0.390095138999986));
#312435=CARTESIAN_POINT('Ctrl Pts',(-4.07998592200006,5.2,0.390095138999986));
#312436=CARTESIAN_POINT('Ctrl Pts',(-4.07998592200006,2.2,0.390095138999986));
#312437=CARTESIAN_POINT('Ctrl Pts',(-4.07892513200006,12.2,0.389741902999985));
#312438=CARTESIAN_POINT('Ctrl Pts',(-4.07892513200006,5.2,0.389741902999985));
#312439=CARTESIAN_POINT('Ctrl Pts',(-4.07892513200006,2.2,0.389741902999985));
#312440=CARTESIAN_POINT('Ctrl Pts',(-4.07786893900006,12.2,0.389391623999984));
#312441=CARTESIAN_POINT('Ctrl Pts',(-4.07786893900006,5.2,0.389391623999984));
#312442=CARTESIAN_POINT('Ctrl Pts',(-4.07786893900006,2.2,0.389391623999984));
#312443=CARTESIAN_POINT('Ctrl Pts',(-4.07681735500006,12.2,0.389044293999987));
#312444=CARTESIAN_POINT('Ctrl Pts',(-4.07681735500006,5.2,0.389044293999987));
#312445=CARTESIAN_POINT('Ctrl Pts',(-4.07681735500006,2.2,0.389044293999987));
#312446=CARTESIAN_POINT('Ctrl Pts',(-4.07577039500006,12.2,0.388699906999985));
#312447=CARTESIAN_POINT('Ctrl Pts',(-4.07577039500006,5.2,0.388699906999985));
#312448=CARTESIAN_POINT('Ctrl Pts',(-4.07577039500006,2.2,0.388699906999985));
#312449=CARTESIAN_POINT('Ctrl Pts',(-4.07472807000006,12.2,0.388358450999986));
#312450=CARTESIAN_POINT('Ctrl Pts',(-4.07472807000006,5.2,0.388358450999986));
#312451=CARTESIAN_POINT('Ctrl Pts',(-4.07472807000006,2.2,0.388358450999986));
#312452=CARTESIAN_POINT('Ctrl Pts',(-4.07369039600006,12.2,0.388019919999985));
#312453=CARTESIAN_POINT('Ctrl Pts',(-4.07369039600006,5.2,0.388019919999985));
#312454=CARTESIAN_POINT('Ctrl Pts',(-4.07369039600006,2.2,0.388019919999985));
#312455=CARTESIAN_POINT('Ctrl Pts',(-4.07265738500006,12.2,0.387684304999985));
#312456=CARTESIAN_POINT('Ctrl Pts',(-4.07265738500006,5.2,0.387684304999985));
#312457=CARTESIAN_POINT('Ctrl Pts',(-4.07265738500006,2.2,0.387684304999985));
#312458=CARTESIAN_POINT('Ctrl Pts',(-4.07162905200006,12.2,0.387351596999985));
#312459=CARTESIAN_POINT('Ctrl Pts',(-4.07162905200006,5.2,0.387351596999985));
#312460=CARTESIAN_POINT('Ctrl Pts',(-4.07162905200006,2.2,0.387351596999985));
#312461=CARTESIAN_POINT('Ctrl Pts',(-4.07060541000006,12.2,0.387021788999986));
#312462=CARTESIAN_POINT('Ctrl Pts',(-4.07060541000006,5.2,0.387021788999986));
#312463=CARTESIAN_POINT('Ctrl Pts',(-4.07060541000006,2.2,0.387021788999986));
#312464=CARTESIAN_POINT('Ctrl Pts',(-4.06958647200006,12.2,0.386694868999986));
#312465=CARTESIAN_POINT('Ctrl Pts',(-4.06958647200006,5.2,0.386694868999986));
#312466=CARTESIAN_POINT('Ctrl Pts',(-4.06958647200006,2.2,0.386694868999986));
#312467=CARTESIAN_POINT('Ctrl Pts',(-4.06857225200006,12.2,0.386370831999985));
#312468=CARTESIAN_POINT('Ctrl Pts',(-4.06857225200006,5.2,0.386370831999985));
#312469=CARTESIAN_POINT('Ctrl Pts',(-4.06857225200006,2.2,0.386370831999985));
#312470=CARTESIAN_POINT('Ctrl Pts',(-4.06756276400006,12.2,0.386049667999986));
#312471=CARTESIAN_POINT('Ctrl Pts',(-4.06756276400006,5.2,0.386049667999986));
#312472=CARTESIAN_POINT('Ctrl Pts',(-4.06756276400006,2.2,0.386049667999986));
#312473=CARTESIAN_POINT('Ctrl Pts',(-4.06655802200006,12.2,0.385731367999984));
#312474=CARTESIAN_POINT('Ctrl Pts',(-4.06655802200006,5.2,0.385731367999984));
#312475=CARTESIAN_POINT('Ctrl Pts',(-4.06655802200006,2.2,0.385731367999984));
#312476=CARTESIAN_POINT('Ctrl Pts',(-4.06555803900006,12.2,0.385415922999983));
#312477=CARTESIAN_POINT('Ctrl Pts',(-4.06555803900006,5.2,0.385415922999983));
#312478=CARTESIAN_POINT('Ctrl Pts',(-4.06555803900006,2.2,0.385415922999983));
#312479=CARTESIAN_POINT('Ctrl Pts',(-4.06456282700006,12.2,0.385103324999987));
#312480=CARTESIAN_POINT('Ctrl Pts',(-4.06456282700006,5.2,0.385103324999987));
#312481=CARTESIAN_POINT('Ctrl Pts',(-4.06456282700006,2.2,0.385103324999987));
#312482=CARTESIAN_POINT('Ctrl Pts',(-4.06357240400006,12.2,0.384793563999986));
#312483=CARTESIAN_POINT('Ctrl Pts',(-4.06357240400006,5.2,0.384793563999986));
#312484=CARTESIAN_POINT('Ctrl Pts',(-4.06357240400006,2.2,0.384793563999986));
#312485=CARTESIAN_POINT('Ctrl Pts',(-4.06258678100006,12.2,0.384486632999987));
#312486=CARTESIAN_POINT('Ctrl Pts',(-4.06258678100006,5.2,0.384486632999987));
#312487=CARTESIAN_POINT('Ctrl Pts',(-4.06258678100006,2.2,0.384486632999987));
#312488=CARTESIAN_POINT('Ctrl Pts',(-4.06160597200006,12.2,0.384182521999987));
#312489=CARTESIAN_POINT('Ctrl Pts',(-4.06160597200006,5.2,0.384182521999987));
#312490=CARTESIAN_POINT('Ctrl Pts',(-4.06160597200006,2.2,0.384182521999987));
#312491=CARTESIAN_POINT('Ctrl Pts',(-4.06062999000006,12.2,0.383881221999989));
#312492=CARTESIAN_POINT('Ctrl Pts',(-4.06062999000006,5.2,0.383881221999989));
#312493=CARTESIAN_POINT('Ctrl Pts',(-4.06062999000006,2.2,0.383881221999989));
#312494=CARTESIAN_POINT('Ctrl Pts',(-4.05965885100006,12.2,0.383582722999982));
#312495=CARTESIAN_POINT('Ctrl Pts',(-4.05965885100006,5.2,0.383582722999982));
#312496=CARTESIAN_POINT('Ctrl Pts',(-4.05965885100006,2.2,0.383582722999982));
#312497=CARTESIAN_POINT('Ctrl Pts',(-4.05869256800006,12.2,0.383287017999985));
#312498=CARTESIAN_POINT('Ctrl Pts',(-4.05869256800006,5.2,0.383287017999985));
#312499=CARTESIAN_POINT('Ctrl Pts',(-4.05869256800006,2.2,0.383287017999985));
#312500=CARTESIAN_POINT('Ctrl Pts',(-4.05773115500006,12.2,0.382994097999987));
#312501=CARTESIAN_POINT('Ctrl Pts',(-4.05773115500006,5.2,0.382994097999987));
#312502=CARTESIAN_POINT('Ctrl Pts',(-4.05773115500006,2.2,0.382994097999987));
#312503=CARTESIAN_POINT('Ctrl Pts',(-4.05677462400006,12.2,0.382703950999983));
#312504=CARTESIAN_POINT('Ctrl Pts',(-4.05677462400006,5.2,0.382703950999983));
#312505=CARTESIAN_POINT('Ctrl Pts',(-4.05677462400006,2.2,0.382703950999983));
#312506=CARTESIAN_POINT('Ctrl Pts',(-4.05582299200006,12.2,0.382416571999986));
#312507=CARTESIAN_POINT('Ctrl Pts',(-4.05582299200006,5.2,0.382416571999986));
#312508=CARTESIAN_POINT('Ctrl Pts',(-4.05582299200006,2.2,0.382416571999986));
#312509=CARTESIAN_POINT('Ctrl Pts',(-4.05487627100006,12.2,0.382131946999986));
#312510=CARTESIAN_POINT('Ctrl Pts',(-4.05487627100006,5.2,0.382131946999986));
#312511=CARTESIAN_POINT('Ctrl Pts',(-4.05487627100006,2.2,0.382131946999986));
#312512=CARTESIAN_POINT('Ctrl Pts',(-4.05393447600006,12.2,0.381850070999987));
#312513=CARTESIAN_POINT('Ctrl Pts',(-4.05393447600006,5.2,0.381850070999987));
#312514=CARTESIAN_POINT('Ctrl Pts',(-4.05393447600006,2.2,0.381850070999987));
#312515=CARTESIAN_POINT('Ctrl Pts',(-4.05299762000006,12.2,0.381570932999988));
#312516=CARTESIAN_POINT('Ctrl Pts',(-4.05299762000006,5.2,0.381570932999988));
#312517=CARTESIAN_POINT('Ctrl Pts',(-4.05299762000006,2.2,0.381570932999988));
#312518=CARTESIAN_POINT('Ctrl Pts',(-4.05206571700006,12.2,0.381294522999984));
#312519=CARTESIAN_POINT('Ctrl Pts',(-4.05206571700006,5.2,0.381294522999984));
#312520=CARTESIAN_POINT('Ctrl Pts',(-4.05206571700006,2.2,0.381294522999984));
#312521=CARTESIAN_POINT('Ctrl Pts',(-4.05113878300006,12.2,0.381020832999983));
#312522=CARTESIAN_POINT('Ctrl Pts',(-4.05113878300006,5.2,0.381020832999983));
#312523=CARTESIAN_POINT('Ctrl Pts',(-4.05113878300006,2.2,0.381020832999983));
#312524=CARTESIAN_POINT('Ctrl Pts',(-4.05021682900006,12.2,0.380749852999984));
#312525=CARTESIAN_POINT('Ctrl Pts',(-4.05021682900006,5.2,0.380749852999984));
#312526=CARTESIAN_POINT('Ctrl Pts',(-4.05021682900006,2.2,0.380749852999984));
#312527=CARTESIAN_POINT('Ctrl Pts',(-4.04929987300005,12.2,0.380481572999987));
#312528=CARTESIAN_POINT('Ctrl Pts',(-4.04929987300005,5.2,0.380481572999987));
#312529=CARTESIAN_POINT('Ctrl Pts',(-4.04929987300005,2.2,0.380481572999987));
#312530=CARTESIAN_POINT('Ctrl Pts',(-4.04838792500006,12.2,0.380215984999985));
#312531=CARTESIAN_POINT('Ctrl Pts',(-4.04838792500006,5.2,0.380215984999985));
#312532=CARTESIAN_POINT('Ctrl Pts',(-4.04838792500006,2.2,0.380215984999985));
#312533=CARTESIAN_POINT('Ctrl Pts',(-4.04748100300006,12.2,0.379953076999984));
#312534=CARTESIAN_POINT('Ctrl Pts',(-4.04748100300006,5.2,0.379953076999984));
#312535=CARTESIAN_POINT('Ctrl Pts',(-4.04748100300006,2.2,0.379953076999984));
#312536=CARTESIAN_POINT('Ctrl Pts',(-4.04657911800006,12.2,0.379692842999986));
#312537=CARTESIAN_POINT('Ctrl Pts',(-4.04657911800006,5.2,0.379692842999986));
#312538=CARTESIAN_POINT('Ctrl Pts',(-4.04657911800006,2.2,0.379692842999986));
#312539=CARTESIAN_POINT('Ctrl Pts',(-4.04568228500006,12.2,0.379435269999986));
#312540=CARTESIAN_POINT('Ctrl Pts',(-4.04568228500006,5.2,0.379435269999986));
#312541=CARTESIAN_POINT('Ctrl Pts',(-4.04568228500006,2.2,0.379435269999986));
#312542=CARTESIAN_POINT('Ctrl Pts',(-4.04479052000006,12.2,0.379180349999988));
#312543=CARTESIAN_POINT('Ctrl Pts',(-4.04479052000006,5.2,0.379180349999988));
#312544=CARTESIAN_POINT('Ctrl Pts',(-4.04479052000006,2.2,0.379180349999988));
#312545=CARTESIAN_POINT('Ctrl Pts',(-4.04390383500006,12.2,0.378928072999987));
#312546=CARTESIAN_POINT('Ctrl Pts',(-4.04390383500006,5.2,0.378928072999987));
#312547=CARTESIAN_POINT('Ctrl Pts',(-4.04390383500006,2.2,0.378928072999987));
#312548=CARTESIAN_POINT('Ctrl Pts',(-4.04302224600006,12.2,0.378678429999986));
#312549=CARTESIAN_POINT('Ctrl Pts',(-4.04302224600006,5.2,0.378678429999986));
#312550=CARTESIAN_POINT('Ctrl Pts',(-4.04302224600006,2.2,0.378678429999986));
#312551=CARTESIAN_POINT('Ctrl Pts',(-4.04214576600006,12.2,0.378431409999984));
#312552=CARTESIAN_POINT('Ctrl Pts',(-4.04214576600006,5.2,0.378431409999984));
#312553=CARTESIAN_POINT('Ctrl Pts',(-4.04214576600006,2.2,0.378431409999984));
#312554=CARTESIAN_POINT('Ctrl Pts',(-4.04127441000006,12.2,0.378187003999986));
#312555=CARTESIAN_POINT('Ctrl Pts',(-4.04127441000006,5.2,0.378187003999986));
#312556=CARTESIAN_POINT('Ctrl Pts',(-4.04127441000006,2.2,0.378187003999986));
#312557=CARTESIAN_POINT('Ctrl Pts',(-4.04040819200006,12.2,0.377945200999985));
#312558=CARTESIAN_POINT('Ctrl Pts',(-4.04040819200006,5.2,0.377945200999985));
#312559=CARTESIAN_POINT('Ctrl Pts',(-4.04040819200006,2.2,0.377945200999985));
#312560=CARTESIAN_POINT('Ctrl Pts',(-4.03954712700005,12.2,0.377705992999986));
#312561=CARTESIAN_POINT('Ctrl Pts',(-4.03954712700005,5.2,0.377705992999986));
#312562=CARTESIAN_POINT('Ctrl Pts',(-4.03954712700005,2.2,0.377705992999986));
#312563=CARTESIAN_POINT('Ctrl Pts',(-4.03869122900006,12.2,0.377469368999983));
#312564=CARTESIAN_POINT('Ctrl Pts',(-4.03869122900006,5.2,0.377469368999983));
#312565=CARTESIAN_POINT('Ctrl Pts',(-4.03869122900006,2.2,0.377469368999983));
#312566=CARTESIAN_POINT('Ctrl Pts',(-4.03784051300006,12.2,0.377235317999984));
#312567=CARTESIAN_POINT('Ctrl Pts',(-4.03784051300006,5.2,0.377235317999984));
#312568=CARTESIAN_POINT('Ctrl Pts',(-4.03784051300006,2.2,0.377235317999984));
#312569=CARTESIAN_POINT('Ctrl Pts',(-4.03699499200005,12.2,0.377003831999985));
#312570=CARTESIAN_POINT('Ctrl Pts',(-4.03699499200005,5.2,0.377003831999985));
#312571=CARTESIAN_POINT('Ctrl Pts',(-4.03699499200005,2.2,0.377003831999985));
#312572=CARTESIAN_POINT('Ctrl Pts',(-4.03615468200006,12.2,0.376774897999983));
#312573=CARTESIAN_POINT('Ctrl Pts',(-4.03615468200006,5.2,0.376774897999983));
#312574=CARTESIAN_POINT('Ctrl Pts',(-4.03615468200006,2.2,0.376774897999983));
#312575=CARTESIAN_POINT('Ctrl Pts',(-4.03531959600006,12.2,0.376548508999988));
#312576=CARTESIAN_POINT('Ctrl Pts',(-4.03531959600006,5.2,0.376548508999988));
#312577=CARTESIAN_POINT('Ctrl Pts',(-4.03531959600006,2.2,0.376548508999988));
#312578=CARTESIAN_POINT('Ctrl Pts',(-4.03448975200006,12.2,0.376324653999984));
#312579=CARTESIAN_POINT('Ctrl Pts',(-4.03448975200006,5.2,0.376324653999984));
#312580=CARTESIAN_POINT('Ctrl Pts',(-4.03448975200006,2.2,0.376324653999984));
#312581=CARTESIAN_POINT('Ctrl Pts',(-4.03366516000006,12.2,0.376103321999985));
#312582=CARTESIAN_POINT('Ctrl Pts',(-4.03366516000006,5.2,0.376103321999985));
#312583=CARTESIAN_POINT('Ctrl Pts',(-4.03366516000006,2.2,0.376103321999985));
#312584=CARTESIAN_POINT('Ctrl Pts',(-4.03284583700006,12.2,0.375884502999986));
#312585=CARTESIAN_POINT('Ctrl Pts',(-4.03284583700006,5.2,0.375884502999986));
#312586=CARTESIAN_POINT('Ctrl Pts',(-4.03284583700006,2.2,0.375884502999986));
#312587=CARTESIAN_POINT('Ctrl Pts',(-4.03203179700006,12.2,0.375668185999984));
#312588=CARTESIAN_POINT('Ctrl Pts',(-4.03203179700006,5.2,0.375668185999984));
#312589=CARTESIAN_POINT('Ctrl Pts',(-4.03203179700006,2.2,0.375668185999984));
#312590=CARTESIAN_POINT('Ctrl Pts',(-4.03122305500006,12.2,0.375454361999985));
#312591=CARTESIAN_POINT('Ctrl Pts',(-4.03122305500006,5.2,0.375454361999985));
#312592=CARTESIAN_POINT('Ctrl Pts',(-4.03122305500006,2.2,0.375454361999985));
#312593=CARTESIAN_POINT('Ctrl Pts',(-4.03041962500006,12.2,0.375243019999987));
#312594=CARTESIAN_POINT('Ctrl Pts',(-4.03041962500006,5.2,0.375243019999987));
#312595=CARTESIAN_POINT('Ctrl Pts',(-4.03041962500006,2.2,0.375243019999987));
#312596=CARTESIAN_POINT('Ctrl Pts',(-4.02962152400006,12.2,0.375034148999984));
#312597=CARTESIAN_POINT('Ctrl Pts',(-4.02962152400006,5.2,0.375034148999984));
#312598=CARTESIAN_POINT('Ctrl Pts',(-4.02962152400006,2.2,0.375034148999984));
#312599=CARTESIAN_POINT('Ctrl Pts',(-4.02882876300006,12.2,0.374827739999986));
#312600=CARTESIAN_POINT('Ctrl Pts',(-4.02882876300006,5.2,0.374827739999986));
#312601=CARTESIAN_POINT('Ctrl Pts',(-4.02882876300006,2.2,0.374827739999986));
#312602=CARTESIAN_POINT('Ctrl Pts',(-4.02804136000006,12.2,0.374623780999985));
#312603=CARTESIAN_POINT('Ctrl Pts',(-4.02804136000006,5.2,0.374623780999985));
#312604=CARTESIAN_POINT('Ctrl Pts',(-4.02804136000006,2.2,0.374623780999985));
#312605=CARTESIAN_POINT('Ctrl Pts',(-4.02725932800006,12.2,0.374422260999987));
#312606=CARTESIAN_POINT('Ctrl Pts',(-4.02725932800006,5.2,0.374422260999987));
#312607=CARTESIAN_POINT('Ctrl Pts',(-4.02725932800006,2.2,0.374422260999987));
#312608=CARTESIAN_POINT('Ctrl Pts',(-4.02648268300006,12.2,0.374223170999985));
#312609=CARTESIAN_POINT('Ctrl Pts',(-4.02648268300006,5.2,0.374223170999985));
#312610=CARTESIAN_POINT('Ctrl Pts',(-4.02648268300006,2.2,0.374223170999985));
#312611=CARTESIAN_POINT('Ctrl Pts',(-4.02571143800006,12.2,0.374026498999989));
#312612=CARTESIAN_POINT('Ctrl Pts',(-4.02571143800006,5.2,0.374026498999989));
#312613=CARTESIAN_POINT('Ctrl Pts',(-4.02571143800006,2.2,0.374026498999989));
#312614=CARTESIAN_POINT('Ctrl Pts',(-4.02494561000006,12.2,0.373832234999987));
#312615=CARTESIAN_POINT('Ctrl Pts',(-4.02494561000006,5.2,0.373832234999987));
#312616=CARTESIAN_POINT('Ctrl Pts',(-4.02494561000006,2.2,0.373832234999987));
#312617=CARTESIAN_POINT('Ctrl Pts',(-4.02418521200006,12.2,0.373640367999983));
#312618=CARTESIAN_POINT('Ctrl Pts',(-4.02418521200006,5.2,0.373640367999983));
#312619=CARTESIAN_POINT('Ctrl Pts',(-4.02418521200006,2.2,0.373640367999983));
#312620=CARTESIAN_POINT('Ctrl Pts',(-4.02343026100006,12.2,0.373450886999986));
#312621=CARTESIAN_POINT('Ctrl Pts',(-4.02343026100006,5.2,0.373450886999986));
#312622=CARTESIAN_POINT('Ctrl Pts',(-4.02343026100006,2.2,0.373450886999986));
#312623=CARTESIAN_POINT('Ctrl Pts',(-4.02268076900006,12.2,0.373263781999986));
#312624=CARTESIAN_POINT('Ctrl Pts',(-4.02268076900006,5.2,0.373263781999986));
#312625=CARTESIAN_POINT('Ctrl Pts',(-4.02268076900006,2.2,0.373263781999986));
#312626=CARTESIAN_POINT('Ctrl Pts',(-4.02193675400006,12.2,0.373079040999986));
#312627=CARTESIAN_POINT('Ctrl Pts',(-4.02193675400006,5.2,0.373079040999986));
#312628=CARTESIAN_POINT('Ctrl Pts',(-4.02193675400006,2.2,0.373079040999986));
#312629=CARTESIAN_POINT('Ctrl Pts',(-4.02119822900006,12.2,0.372896652999986));
#312630=CARTESIAN_POINT('Ctrl Pts',(-4.02119822900006,5.2,0.372896652999986));
#312631=CARTESIAN_POINT('Ctrl Pts',(-4.02119822900006,2.2,0.372896652999986));
#312632=CARTESIAN_POINT('Ctrl Pts',(-4.02046521100006,12.2,0.372716607999983));
#312633=CARTESIAN_POINT('Ctrl Pts',(-4.02046521100006,5.2,0.372716607999983));
#312634=CARTESIAN_POINT('Ctrl Pts',(-4.02046521100006,2.2,0.372716607999983));
#312635=CARTESIAN_POINT('Ctrl Pts',(-4.01973771200006,12.2,0.372538892999987));
#312636=CARTESIAN_POINT('Ctrl Pts',(-4.01973771200006,5.2,0.372538892999987));
#312637=CARTESIAN_POINT('Ctrl Pts',(-4.01973771200006,2.2,0.372538892999987));
#312638=CARTESIAN_POINT('Ctrl Pts',(-4.01901575000006,12.2,0.372363498999988));
#312639=CARTESIAN_POINT('Ctrl Pts',(-4.01901575000006,5.2,0.372363498999988));
#312640=CARTESIAN_POINT('Ctrl Pts',(-4.01901575000006,2.2,0.372363498999988));
#312641=CARTESIAN_POINT('Ctrl Pts',(-4.01829934000006,12.2,0.372190413999984));
#312642=CARTESIAN_POINT('Ctrl Pts',(-4.01829934000006,5.2,0.372190413999984));
#312643=CARTESIAN_POINT('Ctrl Pts',(-4.01829934000006,2.2,0.372190413999984));
#312644=CARTESIAN_POINT('Ctrl Pts',(-4.01758849500006,12.2,0.372019625999984));
#312645=CARTESIAN_POINT('Ctrl Pts',(-4.01758849500006,5.2,0.372019625999984));
#312646=CARTESIAN_POINT('Ctrl Pts',(-4.01758849500006,2.2,0.372019625999984));
#312647=CARTESIAN_POINT('Ctrl Pts',(-4.01688323100006,12.2,0.371851124999987));
#312648=CARTESIAN_POINT('Ctrl Pts',(-4.01688323100006,5.2,0.371851124999987));
#312649=CARTESIAN_POINT('Ctrl Pts',(-4.01688323100006,2.2,0.371851124999987));
#312650=CARTESIAN_POINT('Ctrl Pts',(-4.01618356400006,12.2,0.371684899999987));
#312651=CARTESIAN_POINT('Ctrl Pts',(-4.01618356400006,5.2,0.371684899999987));
#312652=CARTESIAN_POINT('Ctrl Pts',(-4.01618356400006,2.2,0.371684899999987));
#312653=CARTESIAN_POINT('Ctrl Pts',(-4.01548950900006,12.2,0.371520936999987));
#312654=CARTESIAN_POINT('Ctrl Pts',(-4.01548950900006,5.2,0.371520936999987));
#312655=CARTESIAN_POINT('Ctrl Pts',(-4.01548950900006,2.2,0.371520936999987));
#312656=CARTESIAN_POINT('Ctrl Pts',(-4.01480108000006,12.2,0.371359226999988));
#312657=CARTESIAN_POINT('Ctrl Pts',(-4.01480108000006,5.2,0.371359226999988));
#312658=CARTESIAN_POINT('Ctrl Pts',(-4.01480108000006,2.2,0.371359226999988));
#312659=CARTESIAN_POINT('Ctrl Pts',(-4.01411829500006,12.2,0.371199757999987));
#312660=CARTESIAN_POINT('Ctrl Pts',(-4.01411829500006,5.2,0.371199757999987));
#312661=CARTESIAN_POINT('Ctrl Pts',(-4.01411829500006,2.2,0.371199757999987));
#312662=CARTESIAN_POINT('Ctrl Pts',(-4.01344116600006,12.2,0.371042516999989));
#312663=CARTESIAN_POINT('Ctrl Pts',(-4.01344116600006,5.2,0.371042516999989));
#312664=CARTESIAN_POINT('Ctrl Pts',(-4.01344116600006,2.2,0.371042516999989));
#312665=CARTESIAN_POINT('Ctrl Pts',(-4.01276971100006,12.2,0.370887495999987));
#312666=CARTESIAN_POINT('Ctrl Pts',(-4.01276971100006,5.2,0.370887495999987));
#312667=CARTESIAN_POINT('Ctrl Pts',(-4.01276971100006,2.2,0.370887495999987));
#312668=CARTESIAN_POINT('Ctrl Pts',(-4.01210394400006,12.2,0.370734678999987));
#312669=CARTESIAN_POINT('Ctrl Pts',(-4.01210394400006,5.2,0.370734678999987));
#312670=CARTESIAN_POINT('Ctrl Pts',(-4.01210394400006,2.2,0.370734678999987));
#312671=CARTESIAN_POINT('Ctrl Pts',(-4.01144388100006,12.2,0.370584057999985));
#312672=CARTESIAN_POINT('Ctrl Pts',(-4.01144388100006,5.2,0.370584057999985));
#312673=CARTESIAN_POINT('Ctrl Pts',(-4.01144388100006,2.2,0.370584057999985));
#312674=CARTESIAN_POINT('Ctrl Pts',(-4.01078953700006,12.2,0.370435617999987));
#312675=CARTESIAN_POINT('Ctrl Pts',(-4.01078953700006,5.2,0.370435617999987));
#312676=CARTESIAN_POINT('Ctrl Pts',(-4.01078953700006,2.2,0.370435617999987));
#312677=CARTESIAN_POINT('Ctrl Pts',(-4.01014092700006,12.2,0.370289349999986));
#312678=CARTESIAN_POINT('Ctrl Pts',(-4.01014092700006,5.2,0.370289349999986));
#312679=CARTESIAN_POINT('Ctrl Pts',(-4.01014092700006,2.2,0.370289349999986));
#312680=CARTESIAN_POINT('Ctrl Pts',(-4.00949806800006,12.2,0.370145240999986));
#312681=CARTESIAN_POINT('Ctrl Pts',(-4.00949806800006,5.2,0.370145240999986));
#312682=CARTESIAN_POINT('Ctrl Pts',(-4.00949806800006,2.2,0.370145240999986));
#312683=CARTESIAN_POINT('Ctrl Pts',(-4.00886097400006,12.2,0.370003277999986));
#312684=CARTESIAN_POINT('Ctrl Pts',(-4.00886097400006,5.2,0.370003277999986));
#312685=CARTESIAN_POINT('Ctrl Pts',(-4.00886097400006,2.2,0.370003277999986));
#312686=CARTESIAN_POINT('Ctrl Pts',(-4.00822966300006,12.2,0.369863450999985));
#312687=CARTESIAN_POINT('Ctrl Pts',(-4.00822966300006,5.2,0.369863450999985));
#312688=CARTESIAN_POINT('Ctrl Pts',(-4.00822966300006,2.2,0.369863450999985));
#312689=CARTESIAN_POINT('Ctrl Pts',(-4.00760414700006,12.2,0.369725746999983));
#312690=CARTESIAN_POINT('Ctrl Pts',(-4.00760414700006,5.2,0.369725746999983));
#312691=CARTESIAN_POINT('Ctrl Pts',(-4.00760414700006,2.2,0.369725746999983));
#312692=CARTESIAN_POINT('Ctrl Pts',(-4.00698444500006,12.2,0.369590153999986));
#312693=CARTESIAN_POINT('Ctrl Pts',(-4.00698444500006,5.2,0.369590153999986));
#312694=CARTESIAN_POINT('Ctrl Pts',(-4.00698444500006,2.2,0.369590153999986));
#312695=CARTESIAN_POINT('Ctrl Pts',(-4.00637057000006,12.2,0.369456659999985));
#312696=CARTESIAN_POINT('Ctrl Pts',(-4.00637057000006,5.2,0.369456659999985));
#312697=CARTESIAN_POINT('Ctrl Pts',(-4.00637057000006,2.2,0.369456659999985));
#312698=CARTESIAN_POINT('Ctrl Pts',(-4.00576253900006,12.2,0.369325252999988));
#312699=CARTESIAN_POINT('Ctrl Pts',(-4.00576253900006,5.2,0.369325252999988));
#312700=CARTESIAN_POINT('Ctrl Pts',(-4.00576253900006,2.2,0.369325252999988));
#312701=CARTESIAN_POINT('Ctrl Pts',(-4.00516036900005,12.2,0.369195918999985));
#312702=CARTESIAN_POINT('Ctrl Pts',(-4.00516036900005,5.2,0.369195918999985));
#312703=CARTESIAN_POINT('Ctrl Pts',(-4.00516036900005,2.2,0.369195918999985));
#312704=CARTESIAN_POINT('Ctrl Pts',(-4.00456407300006,12.2,0.369068647999988));
#312705=CARTESIAN_POINT('Ctrl Pts',(-4.00456407300006,5.2,0.369068647999988));
#312706=CARTESIAN_POINT('Ctrl Pts',(-4.00456407300006,2.2,0.369068647999988));
#312707=CARTESIAN_POINT('Ctrl Pts',(-4.00397366800005,12.2,0.368943427999984));
#312708=CARTESIAN_POINT('Ctrl Pts',(-4.00397366800005,5.2,0.368943427999984));
#312709=CARTESIAN_POINT('Ctrl Pts',(-4.00397366800005,2.2,0.368943427999984));
#312710=CARTESIAN_POINT('Ctrl Pts',(-4.00338917100005,12.2,0.368820244999988));
#312711=CARTESIAN_POINT('Ctrl Pts',(-4.00338917100005,5.2,0.368820244999988));
#312712=CARTESIAN_POINT('Ctrl Pts',(-4.00338917100005,2.2,0.368820244999988));
#312713=CARTESIAN_POINT('Ctrl Pts',(-4.00281059600006,12.2,0.368699085999986));
#312714=CARTESIAN_POINT('Ctrl Pts',(-4.00281059600006,5.2,0.368699085999986));
#312715=CARTESIAN_POINT('Ctrl Pts',(-4.00281059600006,2.2,0.368699085999986));
#312716=CARTESIAN_POINT('Ctrl Pts',(-4.00223796000006,12.2,0.368579940999982));
#312717=CARTESIAN_POINT('Ctrl Pts',(-4.00223796000006,5.2,0.368579940999982));
#312718=CARTESIAN_POINT('Ctrl Pts',(-4.00223796000006,2.2,0.368579940999982));
#312719=CARTESIAN_POINT('Ctrl Pts',(-4.00167127800006,12.2,0.368462794999989));
#312720=CARTESIAN_POINT('Ctrl Pts',(-4.00167127800006,5.2,0.368462794999989));
#312721=CARTESIAN_POINT('Ctrl Pts',(-4.00167127800006,2.2,0.368462794999989));
#312722=CARTESIAN_POINT('Ctrl Pts',(-4.00111056800006,12.2,0.368347635999986));
#312723=CARTESIAN_POINT('Ctrl Pts',(-4.00111056800006,5.2,0.368347635999986));
#312724=CARTESIAN_POINT('Ctrl Pts',(-4.00111056800006,2.2,0.368347635999986));
#312725=CARTESIAN_POINT('Ctrl Pts',(-4.00055584300006,12.2,0.368234452999987));
#312726=CARTESIAN_POINT('Ctrl Pts',(-4.00055584300006,5.2,0.368234452999987));
#312727=CARTESIAN_POINT('Ctrl Pts',(-4.00055584300006,2.2,0.368234452999987));
#312728=CARTESIAN_POINT('Ctrl Pts',(-4.00000712200006,12.2,0.368123230999986));
#312729=CARTESIAN_POINT('Ctrl Pts',(-4.00000712200006,5.2,0.368123230999986));
#312730=CARTESIAN_POINT('Ctrl Pts',(-4.00000712200006,2.2,0.368123230999986));
#312731=CARTESIAN_POINT('Ctrl Pts',(-3.99946441800005,12.2,0.368013957999986));
#312732=CARTESIAN_POINT('Ctrl Pts',(-3.99946441800005,5.2,0.368013957999986));
#312733=CARTESIAN_POINT('Ctrl Pts',(-3.99946441800005,2.2,0.368013957999986));
#312734=CARTESIAN_POINT('Ctrl Pts',(-3.99892775000006,12.2,0.367906621999987));
#312735=CARTESIAN_POINT('Ctrl Pts',(-3.99892775000006,5.2,0.367906621999987));
#312736=CARTESIAN_POINT('Ctrl Pts',(-3.99892775000006,2.2,0.367906621999987));
#312737=CARTESIAN_POINT('Ctrl Pts',(-3.99839713200006,12.2,0.367801208999987));
#312738=CARTESIAN_POINT('Ctrl Pts',(-3.99839713200006,5.2,0.367801208999987));
#312739=CARTESIAN_POINT('Ctrl Pts',(-3.99839713200006,2.2,0.367801208999987));
#312740=CARTESIAN_POINT('Ctrl Pts',(-3.99787258100006,12.2,0.367697706999985));
#312741=CARTESIAN_POINT('Ctrl Pts',(-3.99787258100006,5.2,0.367697706999985));
#312742=CARTESIAN_POINT('Ctrl Pts',(-3.99787258100006,2.2,0.367697706999985));
#312743=CARTESIAN_POINT('Ctrl Pts',(-3.99735411400005,12.2,0.367596101999985));
#312744=CARTESIAN_POINT('Ctrl Pts',(-3.99735411400005,5.2,0.367596101999985));
#312745=CARTESIAN_POINT('Ctrl Pts',(-3.99735411400005,2.2,0.367596101999985));
#312746=CARTESIAN_POINT('Ctrl Pts',(-3.99684174600006,12.2,0.367496380999985));
#312747=CARTESIAN_POINT('Ctrl Pts',(-3.99684174600006,5.2,0.367496380999985));
#312748=CARTESIAN_POINT('Ctrl Pts',(-3.99684174600006,2.2,0.367496380999985));
#312749=CARTESIAN_POINT('Ctrl Pts',(-3.99633549400006,12.2,0.367398531999985));
#312750=CARTESIAN_POINT('Ctrl Pts',(-3.99633549400006,5.2,0.367398531999985));
#312751=CARTESIAN_POINT('Ctrl Pts',(-3.99633549400006,2.2,0.367398531999985));
#312752=CARTESIAN_POINT('Ctrl Pts',(-3.99583537300006,12.2,0.367302539999983));
#312753=CARTESIAN_POINT('Ctrl Pts',(-3.99583537300006,5.2,0.367302539999983));
#312754=CARTESIAN_POINT('Ctrl Pts',(-3.99583537300006,2.2,0.367302539999983));
#312755=CARTESIAN_POINT('Ctrl Pts',(-3.99534140000006,12.2,0.367208392999987));
#312756=CARTESIAN_POINT('Ctrl Pts',(-3.99534140000006,5.2,0.367208392999987));
#312757=CARTESIAN_POINT('Ctrl Pts',(-3.99534140000006,2.2,0.367208392999987));
#312758=CARTESIAN_POINT('Ctrl Pts',(-3.99485359300006,12.2,0.367116076999987));
#312759=CARTESIAN_POINT('Ctrl Pts',(-3.99485359300006,5.2,0.367116076999987));
#312760=CARTESIAN_POINT('Ctrl Pts',(-3.99485359300006,2.2,0.367116076999987));
#312761=CARTESIAN_POINT('Ctrl Pts',(-3.99437196600006,12.2,0.367025579999982));
#312762=CARTESIAN_POINT('Ctrl Pts',(-3.99437196600006,5.2,0.367025579999982));
#312763=CARTESIAN_POINT('Ctrl Pts',(-3.99437196600006,2.2,0.367025579999982));
#312764=CARTESIAN_POINT('Ctrl Pts',(-3.99389653800006,12.2,0.366936886999985));
#312765=CARTESIAN_POINT('Ctrl Pts',(-3.99389653800006,5.2,0.366936886999985));
#312766=CARTESIAN_POINT('Ctrl Pts',(-3.99389653800006,2.2,0.366936886999985));
#312767=CARTESIAN_POINT('Ctrl Pts',(-3.99342732200005,12.2,0.366849983999984));
#312768=CARTESIAN_POINT('Ctrl Pts',(-3.99342732200005,5.2,0.366849983999984));
#312769=CARTESIAN_POINT('Ctrl Pts',(-3.99342732200005,2.2,0.366849983999984));
#312770=CARTESIAN_POINT('Ctrl Pts',(-3.99296433800005,12.2,0.366764859999984));
#312771=CARTESIAN_POINT('Ctrl Pts',(-3.99296433800005,5.2,0.366764859999984));
#312772=CARTESIAN_POINT('Ctrl Pts',(-3.99296433800005,2.2,0.366764859999984));
#312773=CARTESIAN_POINT('Ctrl Pts',(-3.99250760000006,12.2,0.366681498999988));
#312774=CARTESIAN_POINT('Ctrl Pts',(-3.99250760000006,5.2,0.366681498999988));
#312775=CARTESIAN_POINT('Ctrl Pts',(-3.99250760000006,2.2,0.366681498999988));
#312776=CARTESIAN_POINT('Ctrl Pts',(-3.99205712500006,12.2,0.366599888999986));
#312777=CARTESIAN_POINT('Ctrl Pts',(-3.99205712500006,5.2,0.366599888999986));
#312778=CARTESIAN_POINT('Ctrl Pts',(-3.99205712500006,2.2,0.366599888999986));
#312779=CARTESIAN_POINT('Ctrl Pts',(-3.99161293200006,12.2,0.366520014999985));
#312780=CARTESIAN_POINT('Ctrl Pts',(-3.99161293200006,5.2,0.366520014999985));
#312781=CARTESIAN_POINT('Ctrl Pts',(-3.99161293200006,2.2,0.366520014999985));
#312782=CARTESIAN_POINT('Ctrl Pts',(-3.99117503500006,12.2,0.366441861999984));
#312783=CARTESIAN_POINT('Ctrl Pts',(-3.99117503500006,5.2,0.366441861999984));
#312784=CARTESIAN_POINT('Ctrl Pts',(-3.99117503500006,2.2,0.366441861999984));
#312785=CARTESIAN_POINT('Ctrl Pts',(-3.99074345100006,12.2,0.366365419999983));
#312786=CARTESIAN_POINT('Ctrl Pts',(-3.99074345100006,5.2,0.366365419999983));
#312787=CARTESIAN_POINT('Ctrl Pts',(-3.99074345100006,2.2,0.366365419999983));
#312788=CARTESIAN_POINT('Ctrl Pts',(-3.99031819800006,12.2,0.366290670999985));
#312789=CARTESIAN_POINT('Ctrl Pts',(-3.99031819800006,5.2,0.366290670999985));
#312790=CARTESIAN_POINT('Ctrl Pts',(-3.99031819800006,2.2,0.366290670999985));
#312791=CARTESIAN_POINT('Ctrl Pts',(-3.98989929200006,12.2,0.366217603999988));
#312792=CARTESIAN_POINT('Ctrl Pts',(-3.98989929200006,5.2,0.366217603999988));
#312793=CARTESIAN_POINT('Ctrl Pts',(-3.98989929200006,2.2,0.366217603999988));
#312794=CARTESIAN_POINT('Ctrl Pts',(-3.98948675000006,12.2,0.366146201999986));
#312795=CARTESIAN_POINT('Ctrl Pts',(-3.98948675000006,5.2,0.366146201999986));
#312796=CARTESIAN_POINT('Ctrl Pts',(-3.98948675000006,2.2,0.366146201999986));
#312797=CARTESIAN_POINT('Ctrl Pts',(-3.98908058800005,12.2,0.366076453999984));
#312798=CARTESIAN_POINT('Ctrl Pts',(-3.98908058800005,5.2,0.366076453999984));
#312799=CARTESIAN_POINT('Ctrl Pts',(-3.98908058800005,2.2,0.366076453999984));
#312800=CARTESIAN_POINT('Ctrl Pts',(-3.98868082400006,12.2,0.366008341999984));
#312801=CARTESIAN_POINT('Ctrl Pts',(-3.98868082400006,5.2,0.366008341999984));
#312802=CARTESIAN_POINT('Ctrl Pts',(-3.98868082400006,2.2,0.366008341999984));
#312803=CARTESIAN_POINT('Ctrl Pts',(-3.98828747400006,12.2,0.365941855999985));
#312804=CARTESIAN_POINT('Ctrl Pts',(-3.98828747400006,5.2,0.365941855999985));
#312805=CARTESIAN_POINT('Ctrl Pts',(-3.98828747400006,2.2,0.365941855999985));
#312806=CARTESIAN_POINT('Ctrl Pts',(-3.98790055600006,12.2,0.365876978999986));
#312807=CARTESIAN_POINT('Ctrl Pts',(-3.98790055600006,5.2,0.365876978999986));
#312808=CARTESIAN_POINT('Ctrl Pts',(-3.98790055600006,2.2,0.365876978999986));
#312809=CARTESIAN_POINT('Ctrl Pts',(-3.98752008600006,12.2,0.365813696999986));
#312810=CARTESIAN_POINT('Ctrl Pts',(-3.98752008600006,5.2,0.365813696999986));
#312811=CARTESIAN_POINT('Ctrl Pts',(-3.98752008600006,2.2,0.365813696999986));
#312812=CARTESIAN_POINT('Ctrl Pts',(-3.98714608100006,12.2,0.365751996999983));
#312813=CARTESIAN_POINT('Ctrl Pts',(-3.98714608100006,5.2,0.365751996999983));
#312814=CARTESIAN_POINT('Ctrl Pts',(-3.98714608100006,2.2,0.365751996999983));
#312815=CARTESIAN_POINT('Ctrl Pts',(-3.98677856000006,12.2,0.365691861999986));
#312816=CARTESIAN_POINT('Ctrl Pts',(-3.98677856000006,5.2,0.365691861999986));
#312817=CARTESIAN_POINT('Ctrl Pts',(-3.98677856000006,2.2,0.365691861999986));
#312818=CARTESIAN_POINT('Ctrl Pts',(-3.98641753800006,12.2,0.365633278999984));
#312819=CARTESIAN_POINT('Ctrl Pts',(-3.98641753800006,5.2,0.365633278999984));
#312820=CARTESIAN_POINT('Ctrl Pts',(-3.98641753800006,2.2,0.365633278999984));
#312821=CARTESIAN_POINT('Ctrl Pts',(-3.98606303200006,12.2,0.365576231999984));
#312822=CARTESIAN_POINT('Ctrl Pts',(-3.98606303200006,5.2,0.365576231999984));
#312823=CARTESIAN_POINT('Ctrl Pts',(-3.98606303200006,2.2,0.365576231999984));
#312824=CARTESIAN_POINT('Ctrl Pts',(-3.98571506200006,12.2,0.365520707999987));
#312825=CARTESIAN_POINT('Ctrl Pts',(-3.98571506200006,5.2,0.365520707999987));
#312826=CARTESIAN_POINT('Ctrl Pts',(-3.98571506200006,2.2,0.365520707999987));
#312827=CARTESIAN_POINT('Ctrl Pts',(-3.98537364100005,12.2,0.365466690999985));
#312828=CARTESIAN_POINT('Ctrl Pts',(-3.98537364100005,5.2,0.365466690999985));
#312829=CARTESIAN_POINT('Ctrl Pts',(-3.98537364100005,2.2,0.365466690999985));
#312830=CARTESIAN_POINT('Ctrl Pts',(-3.98503878900006,12.2,0.365414166999987));
#312831=CARTESIAN_POINT('Ctrl Pts',(-3.98503878900006,5.2,0.365414166999987));
#312832=CARTESIAN_POINT('Ctrl Pts',(-3.98503878900006,2.2,0.365414166999987));
#312833=CARTESIAN_POINT('Ctrl Pts',(-3.98471052400006,12.2,0.365363119999986));
#312834=CARTESIAN_POINT('Ctrl Pts',(-3.98471052400006,5.2,0.365363119999986));
#312835=CARTESIAN_POINT('Ctrl Pts',(-3.98471052400006,2.2,0.365363119999986));
#312836=CARTESIAN_POINT('Ctrl Pts',(-3.98438886200006,12.2,0.365313535999987));
#312837=CARTESIAN_POINT('Ctrl Pts',(-3.98438886200006,5.2,0.365313535999987));
#312838=CARTESIAN_POINT('Ctrl Pts',(-3.98438886200006,2.2,0.365313535999987));
#312839=CARTESIAN_POINT('Ctrl Pts',(-3.98407382000006,12.2,0.365265398999988));
#312840=CARTESIAN_POINT('Ctrl Pts',(-3.98407382000006,5.2,0.365265398999988));
#312841=CARTESIAN_POINT('Ctrl Pts',(-3.98407382000006,2.2,0.365265398999988));
#312842=CARTESIAN_POINT('Ctrl Pts',(-3.98376541600006,12.2,0.365218693999987));
#312843=CARTESIAN_POINT('Ctrl Pts',(-3.98376541600006,5.2,0.365218693999987));
#312844=CARTESIAN_POINT('Ctrl Pts',(-3.98376541600006,2.2,0.365218693999987));
#312845=CARTESIAN_POINT('Ctrl Pts',(-3.98346366800006,12.2,0.365173405999983));
#312846=CARTESIAN_POINT('Ctrl Pts',(-3.98346366800006,5.2,0.365173405999983));
#312847=CARTESIAN_POINT('Ctrl Pts',(-3.98346366800006,2.2,0.365173405999983));
#312848=CARTESIAN_POINT('Ctrl Pts',(-3.98316859300006,12.2,0.365129519999985));
#312849=CARTESIAN_POINT('Ctrl Pts',(-3.98316859300006,5.2,0.365129519999985));
#312850=CARTESIAN_POINT('Ctrl Pts',(-3.98316859300006,2.2,0.365129519999985));
#312851=CARTESIAN_POINT('Ctrl Pts',(-3.98288020800006,12.2,0.365087019999986));
#312852=CARTESIAN_POINT('Ctrl Pts',(-3.98288020800006,5.2,0.365087019999986));
#312853=CARTESIAN_POINT('Ctrl Pts',(-3.98288020800006,2.2,0.365087019999986));
#312854=CARTESIAN_POINT('Ctrl Pts',(-3.98259853200006,12.2,0.365045891999984));
#312855=CARTESIAN_POINT('Ctrl Pts',(-3.98259853200006,5.2,0.365045891999984));
#312856=CARTESIAN_POINT('Ctrl Pts',(-3.98259853200006,2.2,0.365045891999984));
#312857=CARTESIAN_POINT('Ctrl Pts',(-3.98232358100006,12.2,0.365006117999984));
#312858=CARTESIAN_POINT('Ctrl Pts',(-3.98232358100006,5.2,0.365006117999984));
#312859=CARTESIAN_POINT('Ctrl Pts',(-3.98232358100006,2.2,0.365006117999984));
#312860=CARTESIAN_POINT('Ctrl Pts',(-3.98205537400006,12.2,0.364967683999984));
#312861=CARTESIAN_POINT('Ctrl Pts',(-3.98205537400006,5.2,0.364967683999984));
#312862=CARTESIAN_POINT('Ctrl Pts',(-3.98205537400006,2.2,0.364967683999984));
#312863=CARTESIAN_POINT('Ctrl Pts',(-3.98179392900006,12.2,0.364930574999986));
#312864=CARTESIAN_POINT('Ctrl Pts',(-3.98179392900006,5.2,0.364930574999986));
#312865=CARTESIAN_POINT('Ctrl Pts',(-3.98179392900006,2.2,0.364930574999986));
#312866=CARTESIAN_POINT('Ctrl Pts',(-3.98153926300005,12.2,0.364894773999982));
#312867=CARTESIAN_POINT('Ctrl Pts',(-3.98153926300005,5.2,0.364894773999982));
#312868=CARTESIAN_POINT('Ctrl Pts',(-3.98153926300005,2.2,0.364894773999982));
#312869=CARTESIAN_POINT('Ctrl Pts',(-3.98129139400006,12.2,0.364860263999987));
#312870=CARTESIAN_POINT('Ctrl Pts',(-3.98129139400006,5.2,0.364860263999987));
#312871=CARTESIAN_POINT('Ctrl Pts',(-3.98129139400006,2.2,0.364860263999987));
#312872=CARTESIAN_POINT('Ctrl Pts',(-3.98105033900006,12.2,0.364827031999986));
#312873=CARTESIAN_POINT('Ctrl Pts',(-3.98105033900006,5.2,0.364827031999986));
#312874=CARTESIAN_POINT('Ctrl Pts',(-3.98105033900006,2.2,0.364827031999986));
#312875=CARTESIAN_POINT('Ctrl Pts',(-3.98081611700006,12.2,0.364795060999987));
#312876=CARTESIAN_POINT('Ctrl Pts',(-3.98081611700006,5.2,0.364795060999987));
#312877=CARTESIAN_POINT('Ctrl Pts',(-3.98081611700006,2.2,0.364795060999987));
#312878=CARTESIAN_POINT('Ctrl Pts',(-3.98058874600006,12.2,0.364764332999985));
#312879=CARTESIAN_POINT('Ctrl Pts',(-3.98058874600006,5.2,0.364764332999985));
#312880=CARTESIAN_POINT('Ctrl Pts',(-3.98058874600006,2.2,0.364764332999985));
#312881=CARTESIAN_POINT('Ctrl Pts',(-3.98036824300006,12.2,0.364734833999982));
#312882=CARTESIAN_POINT('Ctrl Pts',(-3.98036824300006,5.2,0.364734833999982));
#312883=CARTESIAN_POINT('Ctrl Pts',(-3.98036824300006,2.2,0.364734833999982));
#312884=CARTESIAN_POINT('Ctrl Pts',(-3.98015462700006,12.2,0.364706547999987));
#312885=CARTESIAN_POINT('Ctrl Pts',(-3.98015462700006,5.2,0.364706547999987));
#312886=CARTESIAN_POINT('Ctrl Pts',(-3.98015462700006,2.2,0.364706547999987));
#312887=CARTESIAN_POINT('Ctrl Pts',(-3.97994791600006,12.2,0.364679458999984));
#312888=CARTESIAN_POINT('Ctrl Pts',(-3.97994791600006,5.2,0.364679458999984));
#312889=CARTESIAN_POINT('Ctrl Pts',(-3.97994791600006,2.2,0.364679458999984));
#312890=CARTESIAN_POINT('Ctrl Pts',(-3.97974812800006,12.2,0.364653547999985));
#312891=CARTESIAN_POINT('Ctrl Pts',(-3.97974812800006,5.2,0.364653547999985));
#312892=CARTESIAN_POINT('Ctrl Pts',(-3.97974812800006,2.2,0.364653547999985));
#312893=CARTESIAN_POINT('Ctrl Pts',(-3.97955528200006,12.2,0.364628800999984));
#312894=CARTESIAN_POINT('Ctrl Pts',(-3.97955528200006,5.2,0.364628800999984));
#312895=CARTESIAN_POINT('Ctrl Pts',(-3.97955528200006,2.2,0.364628800999984));
#312896=CARTESIAN_POINT('Ctrl Pts',(-3.97936939600006,12.2,0.364605198999985));
#312897=CARTESIAN_POINT('Ctrl Pts',(-3.97936939600006,5.2,0.364605198999985));
#312898=CARTESIAN_POINT('Ctrl Pts',(-3.97936939600006,2.2,0.364605198999985));
#312899=CARTESIAN_POINT('Ctrl Pts',(-3.97919048700006,12.2,0.364582728999987));
#312900=CARTESIAN_POINT('Ctrl Pts',(-3.97919048700006,5.2,0.364582728999987));
#312901=CARTESIAN_POINT('Ctrl Pts',(-3.97919048700006,2.2,0.364582728999987));
#312902=CARTESIAN_POINT('Ctrl Pts',(-3.97901857400006,12.2,0.364561370999983));
#312903=CARTESIAN_POINT('Ctrl Pts',(-3.97901857400006,5.2,0.364561370999983));
#312904=CARTESIAN_POINT('Ctrl Pts',(-3.97901857400006,2.2,0.364561370999983));
#312905=CARTESIAN_POINT('Ctrl Pts',(-3.97885367500006,12.2,0.364541110999985));
#312906=CARTESIAN_POINT('Ctrl Pts',(-3.97885367500006,5.2,0.364541110999985));
#312907=CARTESIAN_POINT('Ctrl Pts',(-3.97885367500006,2.2,0.364541110999985));
#312908=CARTESIAN_POINT('Ctrl Pts',(-3.97869580700006,12.2,0.364521932999988));
#312909=CARTESIAN_POINT('Ctrl Pts',(-3.97869580700006,5.2,0.364521932999988));
#312910=CARTESIAN_POINT('Ctrl Pts',(-3.97869580700006,2.2,0.364521932999988));
#312911=CARTESIAN_POINT('Ctrl Pts',(-3.97854499000006,12.2,0.364503816999986));
#312912=CARTESIAN_POINT('Ctrl Pts',(-3.97854499000006,5.2,0.364503816999986));
#312913=CARTESIAN_POINT('Ctrl Pts',(-3.97854499000006,2.2,0.364503816999986));
#312914=CARTESIAN_POINT('Ctrl Pts',(-3.97840124500005,12.2,0.364486745999986));
#312915=CARTESIAN_POINT('Ctrl Pts',(-3.97840124500005,5.2,0.364486745999986));
#312916=CARTESIAN_POINT('Ctrl Pts',(-3.97840124500005,2.2,0.364486745999986));
#312917=CARTESIAN_POINT('Ctrl Pts',(-3.97826458900005,12.2,0.364470703999986));
#312918=CARTESIAN_POINT('Ctrl Pts',(-3.97826458900005,5.2,0.364470703999986));
#312919=CARTESIAN_POINT('Ctrl Pts',(-3.97826458900005,2.2,0.364470703999986));
#312920=CARTESIAN_POINT('Ctrl Pts',(-3.97813504000006,12.2,0.364455670999986));
#312921=CARTESIAN_POINT('Ctrl Pts',(-3.97813504000006,5.2,0.364455670999986));
#312922=CARTESIAN_POINT('Ctrl Pts',(-3.97813504000006,2.2,0.364455670999986));
#312923=CARTESIAN_POINT('Ctrl Pts',(-3.97801262100006,12.2,0.364441631999988));
#312924=CARTESIAN_POINT('Ctrl Pts',(-3.97801262100006,5.2,0.364441631999988));
#312925=CARTESIAN_POINT('Ctrl Pts',(-3.97801262100006,2.2,0.364441631999988));
#312926=CARTESIAN_POINT('Ctrl Pts',(-3.97789734500006,12.2,0.364428570999986));
#312927=CARTESIAN_POINT('Ctrl Pts',(-3.97789734500006,5.2,0.364428570999986));
#312928=CARTESIAN_POINT('Ctrl Pts',(-3.97789734500006,2.2,0.364428570999986));
#312929=CARTESIAN_POINT('Ctrl Pts',(-3.97778922900006,12.2,0.364416470999984));
#312930=CARTESIAN_POINT('Ctrl Pts',(-3.97778922900006,5.2,0.364416470999984));
#312931=CARTESIAN_POINT('Ctrl Pts',(-3.97778922900006,2.2,0.364416470999984));
#312932=CARTESIAN_POINT('Ctrl Pts',(-3.97768829100006,12.2,0.364405317999985));
#312933=CARTESIAN_POINT('Ctrl Pts',(-3.97768829100006,5.2,0.364405317999985));
#312934=CARTESIAN_POINT('Ctrl Pts',(-3.97768829100006,2.2,0.364405317999985));
#312935=CARTESIAN_POINT('Ctrl Pts',(-3.97759455100006,12.2,0.364395092999987));
#312936=CARTESIAN_POINT('Ctrl Pts',(-3.97759455100006,5.2,0.364395092999987));
#312937=CARTESIAN_POINT('Ctrl Pts',(-3.97759455100006,2.2,0.364395092999987));
#312938=CARTESIAN_POINT('Ctrl Pts',(-3.97750803000006,12.2,0.364385775999985));
#312939=CARTESIAN_POINT('Ctrl Pts',(-3.97750803000006,5.2,0.364385775999985));
#312940=CARTESIAN_POINT('Ctrl Pts',(-3.97750803000006,2.2,0.364385775999985));
#312941=CARTESIAN_POINT('Ctrl Pts',(-3.97742875100006,12.2,0.364377344999984));
#312942=CARTESIAN_POINT('Ctrl Pts',(-3.97742875100006,5.2,0.364377344999984));
#312943=CARTESIAN_POINT('Ctrl Pts',(-3.97742875100006,2.2,0.364377344999984));
#312944=CARTESIAN_POINT('Ctrl Pts',(-3.97735673900006,12.2,0.364369776999984));
#312945=CARTESIAN_POINT('Ctrl Pts',(-3.97735673900006,5.2,0.364369776999984));
#312946=CARTESIAN_POINT('Ctrl Pts',(-3.97735673900006,2.2,0.364369776999984));
#312947=CARTESIAN_POINT('Ctrl Pts',(-3.97729201500006,12.2,0.364363052999988));
#312948=CARTESIAN_POINT('Ctrl Pts',(-3.97729201500006,5.2,0.364363052999988));
#312949=CARTESIAN_POINT('Ctrl Pts',(-3.97729201500006,2.2,0.364363052999988));
#312950=CARTESIAN_POINT('Ctrl Pts',(-3.97723459300006,12.2,0.364357157999984));
#312951=CARTESIAN_POINT('Ctrl Pts',(-3.97723459300006,5.2,0.364357157999984));
#312952=CARTESIAN_POINT('Ctrl Pts',(-3.97723459300006,2.2,0.364357157999984));
#312953=CARTESIAN_POINT('Ctrl Pts',(-3.97717911977753,12.2,0.364351538608712));
#312954=CARTESIAN_POINT('Ctrl Pts',(-3.97717911977753,5.2,0.364351538608712));
#312955=CARTESIAN_POINT('Ctrl Pts',(-3.97717911977753,2.2,0.364351538608712));
#312956=CARTESIAN_POINT('Ctrl Pts',(-3.97714119412776,12.2,0.364347774899514));
#312957=CARTESIAN_POINT('Ctrl Pts',(-3.97714119412776,5.2,0.364347774899514));
#312958=CARTESIAN_POINT('Ctrl Pts',(-3.97714119412776,2.2,0.364347774899514));
#312959=CARTESIAN_POINT('Ctrl Pts',(-3.97711620336759,12.2,0.364345349293931));
#312960=CARTESIAN_POINT('Ctrl Pts',(-3.97711620336759,5.2,0.364345349293931));
#312961=CARTESIAN_POINT('Ctrl Pts',(-3.97711620336759,2.2,0.364345349293931));
#312962=CARTESIAN_POINT('Ctrl Pts',(-3.97710063292244,12.2,0.364343872857997));
#312963=CARTESIAN_POINT('Ctrl Pts',(-3.97710063292244,5.2,0.364343872857997));
#312964=CARTESIAN_POINT('Ctrl Pts',(-3.97710063292244,2.2,0.364343872857997));
#312965=CARTESIAN_POINT('Ctrl Pts',(-3.97709101900006,12.2,0.364342956999986));
#312966=CARTESIAN_POINT('Ctrl Pts',(-3.97709101900006,5.2,0.364342956999986));
#312967=CARTESIAN_POINT('Ctrl Pts',(-3.97709101900006,2.2,0.364342956999986));
#312968=CARTESIAN_POINT('',(-3.97709103800006,2.7,0.364342755999986));
#312969=CARTESIAN_POINT('',(-3.97709103800006,12.2,0.364342755999987));
#312970=CARTESIAN_POINT('Ctrl Pts',(-4.68689806900006,2.7,0.771677711999987));
#312971=CARTESIAN_POINT('Ctrl Pts',(-4.51665756805539,2.7,0.61771045344485));
#312972=CARTESIAN_POINT('Ctrl Pts',(-4.35724736115071,2.69999999999778,
0.51363188389716));
#312973=CARTESIAN_POINT('Ctrl Pts',(-4.07521173625289,2.69999999999778,
0.378371909046352));
#312974=CARTESIAN_POINT('Ctrl Pts',(-3.98972974571173,2.70000000000228,
0.365710767362733));
#312975=CARTESIAN_POINT('Ctrl Pts',(-3.97742731815954,2.70000000000228,
0.364376993680789));
#312976=CARTESIAN_POINT('Ctrl Pts',(-3.97725926445937,2.7,0.36435898468835));
#312977=CARTESIAN_POINT('Ctrl Pts',(-3.97709101900006,2.7,0.364342956999986));
#312978=CARTESIAN_POINT('Origin',(-3.97703993500006,15.2,0.364338073999986));
#312979=CARTESIAN_POINT('',(-3.60988374900006,2.7,0.330702762999984));
#312980=CARTESIAN_POINT('',(-3.60988374900006,2.2,0.330702762999984));
#312981=CARTESIAN_POINT('',(-1.98851996745301,2.7,0.182169037513505));
#312982=CARTESIAN_POINT('Origin',(-5.66300478732629E-14,15.2,-1.77635683940025E-14));
#312983=CARTESIAN_POINT('',(-3.61766281500006,2.7,-0.230522786000017));
#312984=CARTESIAN_POINT('',(-3.61766281500006,12.2,-0.230522786000016));
#312985=CARTESIAN_POINT('Origin',(-5.66300478732629E-14,2.7,-1.92943768261394E-14));
#312986=CARTESIAN_POINT('Origin',(-5.66300478732629E-14,15.2,-1.77635683940025E-14));
#312987=CARTESIAN_POINT('',(-3.98564434100006,2.7,-0.253971109000016));
#312988=CARTESIAN_POINT('',(-3.98564434100006,12.2,-0.253971109000015));
#312989=CARTESIAN_POINT('',(-5.65795294118429E-14,2.7,-1.92911577155913E-14));
#312990=CARTESIAN_POINT('Ctrl Pts',(-3.98564433100006,12.2,-0.253971246000013));
#312991=CARTESIAN_POINT('Ctrl Pts',(-3.98564433100006,5.2,-0.253971246000013));
#312992=CARTESIAN_POINT('Ctrl Pts',(-3.98564433100006,2.2,-0.253971246000013));
#312993=CARTESIAN_POINT('Ctrl Pts',(-3.98565115826319,12.2,-0.253971706950256));
#312994=CARTESIAN_POINT('Ctrl Pts',(-3.98565115826319,5.2,-0.253971706950256));
#312995=CARTESIAN_POINT('Ctrl Pts',(-3.98565115826319,2.2,-0.253971706950256));
#312996=CARTESIAN_POINT('Ctrl Pts',(-3.9856643630646,12.2,-0.253972598617502));
#312997=CARTESIAN_POINT('Ctrl Pts',(-3.9856643630646,5.2,-0.253972598617502));
#312998=CARTESIAN_POINT('Ctrl Pts',(-3.9856643630646,2.2,-0.253972598617502));
#312999=CARTESIAN_POINT('Ctrl Pts',(-3.98568393993797,12.2,-0.253973926488822));
#313000=CARTESIAN_POINT('Ctrl Pts',(-3.98568393993797,5.2,-0.253973926488822));
#313001=CARTESIAN_POINT('Ctrl Pts',(-3.98568393993797,2.2,-0.253973926488822));
#313002=CARTESIAN_POINT('Ctrl Pts',(-3.98570992390786,12.2,-0.253975634437502));
#313003=CARTESIAN_POINT('Ctrl Pts',(-3.98570992390786,5.2,-0.253975634437502));
#313004=CARTESIAN_POINT('Ctrl Pts',(-3.98570992390786,2.2,-0.253975634437502));
#313005=CARTESIAN_POINT('Ctrl Pts',(-3.98575508100006,12.2,-0.253978930000014));
#313006=CARTESIAN_POINT('Ctrl Pts',(-3.98575508100006,5.2,-0.253978930000014));
#313007=CARTESIAN_POINT('Ctrl Pts',(-3.98575508100006,2.2,-0.253978930000014));
#313008=CARTESIAN_POINT('Ctrl Pts',(-3.98580531100006,12.2,-0.253982615000012));
#313009=CARTESIAN_POINT('Ctrl Pts',(-3.98580531100006,5.2,-0.253982615000012));
#313010=CARTESIAN_POINT('Ctrl Pts',(-3.98580531100006,2.2,-0.253982615000012));
#313011=CARTESIAN_POINT('Ctrl Pts',(-3.98586287300006,12.2,-0.253986916000013));
#313012=CARTESIAN_POINT('Ctrl Pts',(-3.98586287300006,5.2,-0.253986916000013));
#313013=CARTESIAN_POINT('Ctrl Pts',(-3.98586287300006,2.2,-0.253986916000013));
#313014=CARTESIAN_POINT('Ctrl Pts',(-3.98592776000006,12.2,-0.253991845000012));
#313015=CARTESIAN_POINT('Ctrl Pts',(-3.98592776000006,5.2,-0.253991845000012));
#313016=CARTESIAN_POINT('Ctrl Pts',(-3.98592776000006,2.2,-0.253991845000012));
#313017=CARTESIAN_POINT('Ctrl Pts',(-3.98599995300006,12.2,-0.253997413000011));
#313018=CARTESIAN_POINT('Ctrl Pts',(-3.98599995300006,5.2,-0.253997413000011));
#313019=CARTESIAN_POINT('Ctrl Pts',(-3.98599995300006,2.2,-0.253997413000011));
#313020=CARTESIAN_POINT('Ctrl Pts',(-3.98607943500005,12.2,-0.254003644000012));
#313021=CARTESIAN_POINT('Ctrl Pts',(-3.98607943500005,5.2,-0.254003644000012));
#313022=CARTESIAN_POINT('Ctrl Pts',(-3.98607943500005,2.2,-0.254003644000012));
#313023=CARTESIAN_POINT('Ctrl Pts',(-3.98616618200006,12.2,-0.254010559000015));
#313024=CARTESIAN_POINT('Ctrl Pts',(-3.98616618200006,5.2,-0.254010559000015));
#313025=CARTESIAN_POINT('Ctrl Pts',(-3.98616618200006,2.2,-0.254010559000015));
#313026=CARTESIAN_POINT('Ctrl Pts',(-3.98626017000006,12.2,-0.254018182000015));
#313027=CARTESIAN_POINT('Ctrl Pts',(-3.98626017000006,5.2,-0.254018182000015));
#313028=CARTESIAN_POINT('Ctrl Pts',(-3.98626017000006,2.2,-0.254018182000015));
#313029=CARTESIAN_POINT('Ctrl Pts',(-3.98636137800006,12.2,-0.254026533000014));
#313030=CARTESIAN_POINT('Ctrl Pts',(-3.98636137800006,5.2,-0.254026533000014));
#313031=CARTESIAN_POINT('Ctrl Pts',(-3.98636137800006,2.2,-0.254026533000014));
#313032=CARTESIAN_POINT('Ctrl Pts',(-3.98646978700006,12.2,-0.254035631000011));
#313033=CARTESIAN_POINT('Ctrl Pts',(-3.98646978700006,5.2,-0.254035631000011));
#313034=CARTESIAN_POINT('Ctrl Pts',(-3.98646978700006,2.2,-0.254035631000011));
#313035=CARTESIAN_POINT('Ctrl Pts',(-3.98658538200006,12.2,-0.254045493000015));
#313036=CARTESIAN_POINT('Ctrl Pts',(-3.98658538200006,5.2,-0.254045493000015));
#313037=CARTESIAN_POINT('Ctrl Pts',(-3.98658538200006,2.2,-0.254045493000015));
#313038=CARTESIAN_POINT('Ctrl Pts',(-3.98670814400006,12.2,-0.254056134000016));
#313039=CARTESIAN_POINT('Ctrl Pts',(-3.98670814400006,5.2,-0.254056134000016));
#313040=CARTESIAN_POINT('Ctrl Pts',(-3.98670814400006,2.2,-0.254056134000016));
#313041=CARTESIAN_POINT('Ctrl Pts',(-3.98683805700006,12.2,-0.254067570000016));
#313042=CARTESIAN_POINT('Ctrl Pts',(-3.98683805700006,5.2,-0.254067570000016));
#313043=CARTESIAN_POINT('Ctrl Pts',(-3.98683805700006,2.2,-0.254067570000016));
#313044=CARTESIAN_POINT('Ctrl Pts',(-3.98697510600006,12.2,-0.254079819000013));
#313045=CARTESIAN_POINT('Ctrl Pts',(-3.98697510600006,5.2,-0.254079819000013));
#313046=CARTESIAN_POINT('Ctrl Pts',(-3.98697510600006,2.2,-0.254079819000013));
#313047=CARTESIAN_POINT('Ctrl Pts',(-3.98711926900006,12.2,-0.254092898000016));
#313048=CARTESIAN_POINT('Ctrl Pts',(-3.98711926900006,5.2,-0.254092898000016));
#313049=CARTESIAN_POINT('Ctrl Pts',(-3.98711926900006,2.2,-0.254092898000016));
#313050=CARTESIAN_POINT('Ctrl Pts',(-3.98727053100006,12.2,-0.254106827000014));
#313051=CARTESIAN_POINT('Ctrl Pts',(-3.98727053100006,5.2,-0.254106827000014));
#313052=CARTESIAN_POINT('Ctrl Pts',(-3.98727053100006,2.2,-0.254106827000014));
#313053=CARTESIAN_POINT('Ctrl Pts',(-3.98742886900005,12.2,-0.254121623000017));
#313054=CARTESIAN_POINT('Ctrl Pts',(-3.98742886900005,5.2,-0.254121623000017));
#313055=CARTESIAN_POINT('Ctrl Pts',(-3.98742886900005,2.2,-0.254121623000017));
#313056=CARTESIAN_POINT('Ctrl Pts',(-3.98759426600006,12.2,-0.254137305000013));
#313057=CARTESIAN_POINT('Ctrl Pts',(-3.98759426600006,5.2,-0.254137305000013));
#313058=CARTESIAN_POINT('Ctrl Pts',(-3.98759426600006,2.2,-0.254137305000013));
#313059=CARTESIAN_POINT('Ctrl Pts',(-3.98776670600006,12.2,-0.254153889000013));
#313060=CARTESIAN_POINT('Ctrl Pts',(-3.98776670600006,5.2,-0.254153889000013));
#313061=CARTESIAN_POINT('Ctrl Pts',(-3.98776670600006,2.2,-0.254153889000013));
#313062=CARTESIAN_POINT('Ctrl Pts',(-3.98794616800005,12.2,-0.254171392000018));
#313063=CARTESIAN_POINT('Ctrl Pts',(-3.98794616800005,5.2,-0.254171392000018));
#313064=CARTESIAN_POINT('Ctrl Pts',(-3.98794616800005,2.2,-0.254171392000018));
#313065=CARTESIAN_POINT('Ctrl Pts',(-3.98813263700006,12.2,-0.254189832000016));
#313066=CARTESIAN_POINT('Ctrl Pts',(-3.98813263700006,5.2,-0.254189832000016));
#313067=CARTESIAN_POINT('Ctrl Pts',(-3.98813263700006,2.2,-0.254189832000016));
#313068=CARTESIAN_POINT('Ctrl Pts',(-3.98832609600006,12.2,-0.254209226000013));
#313069=CARTESIAN_POINT('Ctrl Pts',(-3.98832609600006,5.2,-0.254209226000013));
#313070=CARTESIAN_POINT('Ctrl Pts',(-3.98832609600006,2.2,-0.254209226000013));
#313071=CARTESIAN_POINT('Ctrl Pts',(-3.98852652500006,12.2,-0.254229589000015));
#313072=CARTESIAN_POINT('Ctrl Pts',(-3.98852652500006,5.2,-0.254229589000015));
#313073=CARTESIAN_POINT('Ctrl Pts',(-3.98852652500006,2.2,-0.254229589000015));
#313074=CARTESIAN_POINT('Ctrl Pts',(-3.98873390800006,12.2,-0.254250939000014));
#313075=CARTESIAN_POINT('Ctrl Pts',(-3.98873390800006,5.2,-0.254250939000014));
#313076=CARTESIAN_POINT('Ctrl Pts',(-3.98873390800006,2.2,-0.254250939000014));
#313077=CARTESIAN_POINT('Ctrl Pts',(-3.98894822500006,12.2,-0.254273293000011));
#313078=CARTESIAN_POINT('Ctrl Pts',(-3.98894822500006,5.2,-0.254273293000011));
#313079=CARTESIAN_POINT('Ctrl Pts',(-3.98894822500006,2.2,-0.254273293000011));
#313080=CARTESIAN_POINT('Ctrl Pts',(-3.98916946100006,12.2,-0.254296669000014));
#313081=CARTESIAN_POINT('Ctrl Pts',(-3.98916946100006,5.2,-0.254296669000014));
#313082=CARTESIAN_POINT('Ctrl Pts',(-3.98916946100006,2.2,-0.254296669000014));
#313083=CARTESIAN_POINT('Ctrl Pts',(-3.98939759700006,12.2,-0.254321082000013));
#313084=CARTESIAN_POINT('Ctrl Pts',(-3.98939759700006,5.2,-0.254321082000013));
#313085=CARTESIAN_POINT('Ctrl Pts',(-3.98939759700006,2.2,-0.254321082000013));
#313086=CARTESIAN_POINT('Ctrl Pts',(-3.98963261500006,12.2,-0.254346550000015));
#313087=CARTESIAN_POINT('Ctrl Pts',(-3.98963261500006,5.2,-0.254346550000015));
#313088=CARTESIAN_POINT('Ctrl Pts',(-3.98963261500006,2.2,-0.254346550000015));
#313089=CARTESIAN_POINT('Ctrl Pts',(-3.98987449700006,12.2,-0.254373088000013));
#313090=CARTESIAN_POINT('Ctrl Pts',(-3.98987449700006,5.2,-0.254373088000013));
#313091=CARTESIAN_POINT('Ctrl Pts',(-3.98987449700006,2.2,-0.254373088000013));
#313092=CARTESIAN_POINT('Ctrl Pts',(-3.99012322800006,12.2,-0.254400714000016));
#313093=CARTESIAN_POINT('Ctrl Pts',(-3.99012322800006,5.2,-0.254400714000016));
#313094=CARTESIAN_POINT('Ctrl Pts',(-3.99012322800006,2.2,-0.254400714000016));
#313095=CARTESIAN_POINT('Ctrl Pts',(-3.99037878800006,12.2,-0.254429444000017));
#313096=CARTESIAN_POINT('Ctrl Pts',(-3.99037878800006,5.2,-0.254429444000017));
#313097=CARTESIAN_POINT('Ctrl Pts',(-3.99037878800006,2.2,-0.254429444000017));
#313098=CARTESIAN_POINT('Ctrl Pts',(-3.99064116200006,12.2,-0.254459292000018));
#313099=CARTESIAN_POINT('Ctrl Pts',(-3.99064116200006,5.2,-0.254459292000018));
#313100=CARTESIAN_POINT('Ctrl Pts',(-3.99064116200006,2.2,-0.254459292000018));
#313101=CARTESIAN_POINT('Ctrl Pts',(-3.99091033200006,12.2,-0.254490278000015));
#313102=CARTESIAN_POINT('Ctrl Pts',(-3.99091033200006,5.2,-0.254490278000015));
#313103=CARTESIAN_POINT('Ctrl Pts',(-3.99091033200006,2.2,-0.254490278000015));
#313104=CARTESIAN_POINT('Ctrl Pts',(-3.99118627800005,12.2,-0.254522415000018));
#313105=CARTESIAN_POINT('Ctrl Pts',(-3.99118627800005,5.2,-0.254522415000018));
#313106=CARTESIAN_POINT('Ctrl Pts',(-3.99118627800005,2.2,-0.254522415000018));
#313107=CARTESIAN_POINT('Ctrl Pts',(-3.99146898700006,12.2,-0.254555721000016));
#313108=CARTESIAN_POINT('Ctrl Pts',(-3.99146898700006,5.2,-0.254555721000016));
#313109=CARTESIAN_POINT('Ctrl Pts',(-3.99146898700006,2.2,-0.254555721000016));
#313110=CARTESIAN_POINT('Ctrl Pts',(-3.99175843800006,12.2,-0.254590211000014));
#313111=CARTESIAN_POINT('Ctrl Pts',(-3.99175843800006,5.2,-0.254590211000014));
#313112=CARTESIAN_POINT('Ctrl Pts',(-3.99175843800006,2.2,-0.254590211000014));
#313113=CARTESIAN_POINT('Ctrl Pts',(-3.99205461600006,12.2,-0.254625902000014));
#313114=CARTESIAN_POINT('Ctrl Pts',(-3.99205461600006,5.2,-0.254625902000014));
#313115=CARTESIAN_POINT('Ctrl Pts',(-3.99205461600006,2.2,-0.254625902000014));
#313116=CARTESIAN_POINT('Ctrl Pts',(-3.99235750300006,12.2,-0.254662810000017));
#313117=CARTESIAN_POINT('Ctrl Pts',(-3.99235750300006,5.2,-0.254662810000017));
#313118=CARTESIAN_POINT('Ctrl Pts',(-3.99235750300006,2.2,-0.254662810000017));
#313119=CARTESIAN_POINT('Ctrl Pts',(-3.99266708400006,12.2,-0.254700949000015));
#313120=CARTESIAN_POINT('Ctrl Pts',(-3.99266708400006,5.2,-0.254700949000015));
#313121=CARTESIAN_POINT('Ctrl Pts',(-3.99266708400006,2.2,-0.254700949000015));
#313122=CARTESIAN_POINT('Ctrl Pts',(-3.99298333800005,12.2,-0.254740335000014));
#313123=CARTESIAN_POINT('Ctrl Pts',(-3.99298333800005,5.2,-0.254740335000014));
#313124=CARTESIAN_POINT('Ctrl Pts',(-3.99298333800005,2.2,-0.254740335000014));
#313125=CARTESIAN_POINT('Ctrl Pts',(-3.99330625200006,12.2,-0.254780985000016));
#313126=CARTESIAN_POINT('Ctrl Pts',(-3.99330625200006,5.2,-0.254780985000016));
#313127=CARTESIAN_POINT('Ctrl Pts',(-3.99330625200006,2.2,-0.254780985000016));
#313128=CARTESIAN_POINT('Ctrl Pts',(-3.99363580700006,12.2,-0.254822914000012));
#313129=CARTESIAN_POINT('Ctrl Pts',(-3.99363580700006,5.2,-0.254822914000012));
#313130=CARTESIAN_POINT('Ctrl Pts',(-3.99363580700006,2.2,-0.254822914000012));
#313131=CARTESIAN_POINT('Ctrl Pts',(-3.99397198400006,12.2,-0.254866137000014));
#313132=CARTESIAN_POINT('Ctrl Pts',(-3.99397198400006,5.2,-0.254866137000014));
#313133=CARTESIAN_POINT('Ctrl Pts',(-3.99397198400006,2.2,-0.254866137000014));
#313134=CARTESIAN_POINT('Ctrl Pts',(-3.99431477100006,12.2,-0.254910670000013));
#313135=CARTESIAN_POINT('Ctrl Pts',(-3.99431477100006,5.2,-0.254910670000013));
#313136=CARTESIAN_POINT('Ctrl Pts',(-3.99431477100006,2.2,-0.254910670000013));
#313137=CARTESIAN_POINT('Ctrl Pts',(-3.99466414700006,12.2,-0.254956529000014));
#313138=CARTESIAN_POINT('Ctrl Pts',(-3.99466414700006,5.2,-0.254956529000014));
#313139=CARTESIAN_POINT('Ctrl Pts',(-3.99466414700006,2.2,-0.254956529000014));
#313140=CARTESIAN_POINT('Ctrl Pts',(-3.99502009800006,12.2,-0.255003727000016));
#313141=CARTESIAN_POINT('Ctrl Pts',(-3.99502009800006,5.2,-0.255003727000016));
#313142=CARTESIAN_POINT('Ctrl Pts',(-3.99502009800006,2.2,-0.255003727000016));
#313143=CARTESIAN_POINT('Ctrl Pts',(-3.99538260500006,12.2,-0.255052282000015));
#313144=CARTESIAN_POINT('Ctrl Pts',(-3.99538260500006,5.2,-0.255052282000015));
#313145=CARTESIAN_POINT('Ctrl Pts',(-3.99538260500006,2.2,-0.255052282000015));
#313146=CARTESIAN_POINT('Ctrl Pts',(-3.99575165200006,12.2,-0.255102208000015));
#313147=CARTESIAN_POINT('Ctrl Pts',(-3.99575165200006,5.2,-0.255102208000015));
#313148=CARTESIAN_POINT('Ctrl Pts',(-3.99575165200006,2.2,-0.255102208000015));
#313149=CARTESIAN_POINT('Ctrl Pts',(-3.99612722300006,12.2,-0.255153519000015));
#313150=CARTESIAN_POINT('Ctrl Pts',(-3.99612722300006,5.2,-0.255153519000015));
#313151=CARTESIAN_POINT('Ctrl Pts',(-3.99612722300006,2.2,-0.255153519000015));
#313152=CARTESIAN_POINT('Ctrl Pts',(-3.99650930000006,12.2,-0.255206231000016));
#313153=CARTESIAN_POINT('Ctrl Pts',(-3.99650930000006,5.2,-0.255206231000016));
#313154=CARTESIAN_POINT('Ctrl Pts',(-3.99650930000006,2.2,-0.255206231000016));
#313155=CARTESIAN_POINT('Ctrl Pts',(-3.99689786800006,12.2,-0.255260358000013));
#313156=CARTESIAN_POINT('Ctrl Pts',(-3.99689786800006,5.2,-0.255260358000013));
#313157=CARTESIAN_POINT('Ctrl Pts',(-3.99689786800006,2.2,-0.255260358000013));
#313158=CARTESIAN_POINT('Ctrl Pts',(-3.99729290900006,12.2,-0.255315917000014));
#313159=CARTESIAN_POINT('Ctrl Pts',(-3.99729290900006,5.2,-0.255315917000014));
#313160=CARTESIAN_POINT('Ctrl Pts',(-3.99729290900006,2.2,-0.255315917000014));
#313161=CARTESIAN_POINT('Ctrl Pts',(-3.99769440800006,12.2,-0.255372921000014));
#313162=CARTESIAN_POINT('Ctrl Pts',(-3.99769440800006,5.2,-0.255372921000014));
#313163=CARTESIAN_POINT('Ctrl Pts',(-3.99769440800006,2.2,-0.255372921000014));
#313164=CARTESIAN_POINT('Ctrl Pts',(-3.99810234600006,12.2,-0.255431386000016));
#313165=CARTESIAN_POINT('Ctrl Pts',(-3.99810234600006,5.2,-0.255431386000016));
#313166=CARTESIAN_POINT('Ctrl Pts',(-3.99810234600006,2.2,-0.255431386000016));
#313167=CARTESIAN_POINT('Ctrl Pts',(-3.99851671000006,12.2,-0.255491326000015));
#313168=CARTESIAN_POINT('Ctrl Pts',(-3.99851671000006,5.2,-0.255491326000015));
#313169=CARTESIAN_POINT('Ctrl Pts',(-3.99851671000006,2.2,-0.255491326000015));
#313170=CARTESIAN_POINT('Ctrl Pts',(-3.99893748000006,12.2,-0.255552756000017));
#313171=CARTESIAN_POINT('Ctrl Pts',(-3.99893748000006,5.2,-0.255552756000017));
#313172=CARTESIAN_POINT('Ctrl Pts',(-3.99893748000006,2.2,-0.255552756000017));
#313173=CARTESIAN_POINT('Ctrl Pts',(-3.99936464200006,12.2,-0.255615689000015));
#313174=CARTESIAN_POINT('Ctrl Pts',(-3.99936464200006,5.2,-0.255615689000015));
#313175=CARTESIAN_POINT('Ctrl Pts',(-3.99936464200006,2.2,-0.255615689000015));
#313176=CARTESIAN_POINT('Ctrl Pts',(-3.99979817700006,12.2,-0.255680141000014));
#313177=CARTESIAN_POINT('Ctrl Pts',(-3.99979817700006,5.2,-0.255680141000014));
#313178=CARTESIAN_POINT('Ctrl Pts',(-3.99979817700006,2.2,-0.255680141000014));
#313179=CARTESIAN_POINT('Ctrl Pts',(-4.00023807300006,12.2,-0.255746125000016));
#313180=CARTESIAN_POINT('Ctrl Pts',(-4.00023807300006,5.2,-0.255746125000016));
#313181=CARTESIAN_POINT('Ctrl Pts',(-4.00023807300006,2.2,-0.255746125000016));
#313182=CARTESIAN_POINT('Ctrl Pts',(-4.00068431000006,12.2,-0.255813658000013));
#313183=CARTESIAN_POINT('Ctrl Pts',(-4.00068431000006,5.2,-0.255813658000013));
#313184=CARTESIAN_POINT('Ctrl Pts',(-4.00068431000006,2.2,-0.255813658000013));
#313185=CARTESIAN_POINT('Ctrl Pts',(-4.00113687200006,12.2,-0.255882751000014));
#313186=CARTESIAN_POINT('Ctrl Pts',(-4.00113687200006,5.2,-0.255882751000014));
#313187=CARTESIAN_POINT('Ctrl Pts',(-4.00113687200006,2.2,-0.255882751000014));
#313188=CARTESIAN_POINT('Ctrl Pts',(-4.00159574500006,12.2,-0.255953421000013));
#313189=CARTESIAN_POINT('Ctrl Pts',(-4.00159574500006,5.2,-0.255953421000013));
#313190=CARTESIAN_POINT('Ctrl Pts',(-4.00159574500006,2.2,-0.255953421000013));
#313191=CARTESIAN_POINT('Ctrl Pts',(-4.00206091100006,12.2,-0.256025681000014));
#313192=CARTESIAN_POINT('Ctrl Pts',(-4.00206091100006,5.2,-0.256025681000014));
#313193=CARTESIAN_POINT('Ctrl Pts',(-4.00206091100006,2.2,-0.256025681000014));
#313194=CARTESIAN_POINT('Ctrl Pts',(-4.00253235500006,12.2,-0.256099545000015));
#313195=CARTESIAN_POINT('Ctrl Pts',(-4.00253235500006,5.2,-0.256099545000015));
#313196=CARTESIAN_POINT('Ctrl Pts',(-4.00253235500006,2.2,-0.256099545000015));
#313197=CARTESIAN_POINT('Ctrl Pts',(-4.00301006000006,12.2,-0.256175026000012));
#313198=CARTESIAN_POINT('Ctrl Pts',(-4.00301006000006,5.2,-0.256175026000012));
#313199=CARTESIAN_POINT('Ctrl Pts',(-4.00301006000006,2.2,-0.256175026000012));
#313200=CARTESIAN_POINT('Ctrl Pts',(-4.00349401000006,12.2,-0.256252140000015));
#313201=CARTESIAN_POINT('Ctrl Pts',(-4.00349401000006,5.2,-0.256252140000015));
#313202=CARTESIAN_POINT('Ctrl Pts',(-4.00349401000006,2.2,-0.256252140000015));
#313203=CARTESIAN_POINT('Ctrl Pts',(-4.00398418900005,12.2,-0.256330899000012));
#313204=CARTESIAN_POINT('Ctrl Pts',(-4.00398418900005,5.2,-0.256330899000012));
#313205=CARTESIAN_POINT('Ctrl Pts',(-4.00398418900005,2.2,-0.256330899000012));
#313206=CARTESIAN_POINT('Ctrl Pts',(-4.00448058000006,12.2,-0.256411319000014));
#313207=CARTESIAN_POINT('Ctrl Pts',(-4.00448058000006,5.2,-0.256411319000014));
#313208=CARTESIAN_POINT('Ctrl Pts',(-4.00448058000006,2.2,-0.256411319000014));
#313209=CARTESIAN_POINT('Ctrl Pts',(-4.00498316900006,12.2,-0.256493413000012));
#313210=CARTESIAN_POINT('Ctrl Pts',(-4.00498316900006,5.2,-0.256493413000012));
#313211=CARTESIAN_POINT('Ctrl Pts',(-4.00498316900006,2.2,-0.256493413000012));
#313212=CARTESIAN_POINT('Ctrl Pts',(-4.00549193900006,12.2,-0.256577193000016));
#313213=CARTESIAN_POINT('Ctrl Pts',(-4.00549193900006,5.2,-0.256577193000016));
#313214=CARTESIAN_POINT('Ctrl Pts',(-4.00549193900006,2.2,-0.256577193000016));
#313215=CARTESIAN_POINT('Ctrl Pts',(-4.00600687400006,12.2,-0.256662674000014));
#313216=CARTESIAN_POINT('Ctrl Pts',(-4.00600687400006,5.2,-0.256662674000014));
#313217=CARTESIAN_POINT('Ctrl Pts',(-4.00600687400006,2.2,-0.256662674000014));
#313218=CARTESIAN_POINT('Ctrl Pts',(-4.00652795900006,12.2,-0.256749870000017));
#313219=CARTESIAN_POINT('Ctrl Pts',(-4.00652795900006,5.2,-0.256749870000017));
#313220=CARTESIAN_POINT('Ctrl Pts',(-4.00652795900006,2.2,-0.256749870000017));
#313221=CARTESIAN_POINT('Ctrl Pts',(-4.00705517700006,12.2,-0.256838795000016));
#313222=CARTESIAN_POINT('Ctrl Pts',(-4.00705517700006,5.2,-0.256838795000016));
#313223=CARTESIAN_POINT('Ctrl Pts',(-4.00705517700006,2.2,-0.256838795000016));
#313224=CARTESIAN_POINT('Ctrl Pts',(-4.00758851200006,12.2,-0.256929460000013));
#313225=CARTESIAN_POINT('Ctrl Pts',(-4.00758851200006,5.2,-0.256929460000013));
#313226=CARTESIAN_POINT('Ctrl Pts',(-4.00758851200006,2.2,-0.256929460000013));
#313227=CARTESIAN_POINT('Ctrl Pts',(-4.00812794900006,12.2,-0.257021880000017));
#313228=CARTESIAN_POINT('Ctrl Pts',(-4.00812794900006,5.2,-0.257021880000017));
#313229=CARTESIAN_POINT('Ctrl Pts',(-4.00812794900006,2.2,-0.257021880000017));
#313230=CARTESIAN_POINT('Ctrl Pts',(-4.00867347200006,12.2,-0.257116069000016));
#313231=CARTESIAN_POINT('Ctrl Pts',(-4.00867347200006,5.2,-0.257116069000016));
#313232=CARTESIAN_POINT('Ctrl Pts',(-4.00867347200006,2.2,-0.257116069000016));
#313233=CARTESIAN_POINT('Ctrl Pts',(-4.00922506700006,12.2,-0.257212040000017));
#313234=CARTESIAN_POINT('Ctrl Pts',(-4.00922506700006,5.2,-0.257212040000017));
#313235=CARTESIAN_POINT('Ctrl Pts',(-4.00922506700006,2.2,-0.257212040000017));
#313236=CARTESIAN_POINT('Ctrl Pts',(-4.00978271400006,12.2,-0.257309805000014));
#313237=CARTESIAN_POINT('Ctrl Pts',(-4.00978271400006,5.2,-0.257309805000014));
#313238=CARTESIAN_POINT('Ctrl Pts',(-4.00978271400006,2.2,-0.257309805000014));
#313239=CARTESIAN_POINT('Ctrl Pts',(-4.01034640200006,12.2,-0.257409379000015));
#313240=CARTESIAN_POINT('Ctrl Pts',(-4.01034640200006,5.2,-0.257409379000015));
#313241=CARTESIAN_POINT('Ctrl Pts',(-4.01034640200006,2.2,-0.257409379000015));
#313242=CARTESIAN_POINT('Ctrl Pts',(-4.01091611300005,12.2,-0.257510773000016));
#313243=CARTESIAN_POINT('Ctrl Pts',(-4.01091611300005,5.2,-0.257510773000016));
#313244=CARTESIAN_POINT('Ctrl Pts',(-4.01091611300005,2.2,-0.257510773000016));
#313245=CARTESIAN_POINT('Ctrl Pts',(-4.01149183100006,12.2,-0.257614001000013));
#313246=CARTESIAN_POINT('Ctrl Pts',(-4.01149183100006,5.2,-0.257614001000013));
#313247=CARTESIAN_POINT('Ctrl Pts',(-4.01149183100006,2.2,-0.257614001000013));
#313248=CARTESIAN_POINT('Ctrl Pts',(-4.01207354100006,12.2,-0.257719076000011));
#313249=CARTESIAN_POINT('Ctrl Pts',(-4.01207354100006,5.2,-0.257719076000011));
#313250=CARTESIAN_POINT('Ctrl Pts',(-4.01207354100006,2.2,-0.257719076000011));
#313251=CARTESIAN_POINT('Ctrl Pts',(-4.01266122900005,12.2,-0.257826012000013));
#313252=CARTESIAN_POINT('Ctrl Pts',(-4.01266122900005,5.2,-0.257826012000013));
#313253=CARTESIAN_POINT('Ctrl Pts',(-4.01266122900005,2.2,-0.257826012000013));
#313254=CARTESIAN_POINT('Ctrl Pts',(-4.01325487700006,12.2,-0.257934821000014));
#313255=CARTESIAN_POINT('Ctrl Pts',(-4.01325487700006,5.2,-0.257934821000014));
#313256=CARTESIAN_POINT('Ctrl Pts',(-4.01325487700006,2.2,-0.257934821000014));
#313257=CARTESIAN_POINT('Ctrl Pts',(-4.01385447100005,12.2,-0.258045516000016));
#313258=CARTESIAN_POINT('Ctrl Pts',(-4.01385447100005,5.2,-0.258045516000016));
#313259=CARTESIAN_POINT('Ctrl Pts',(-4.01385447100005,2.2,-0.258045516000016));
#313260=CARTESIAN_POINT('Ctrl Pts',(-4.01445999600006,12.2,-0.258158110000015));
#313261=CARTESIAN_POINT('Ctrl Pts',(-4.01445999600006,5.2,-0.258158110000015));
#313262=CARTESIAN_POINT('Ctrl Pts',(-4.01445999600006,2.2,-0.258158110000015));
#313263=CARTESIAN_POINT('Ctrl Pts',(-4.01507143400006,12.2,-0.258272613000017));
#313264=CARTESIAN_POINT('Ctrl Pts',(-4.01507143400006,5.2,-0.258272613000017));
#313265=CARTESIAN_POINT('Ctrl Pts',(-4.01507143400006,2.2,-0.258272613000017));
#313266=CARTESIAN_POINT('Ctrl Pts',(-4.01568877300006,12.2,-0.258389042000013));
#313267=CARTESIAN_POINT('Ctrl Pts',(-4.01568877300006,5.2,-0.258389042000013));
#313268=CARTESIAN_POINT('Ctrl Pts',(-4.01568877300006,2.2,-0.258389042000013));
#313269=CARTESIAN_POINT('Ctrl Pts',(-4.01631199600006,12.2,-0.258507407000015));
#313270=CARTESIAN_POINT('Ctrl Pts',(-4.01631199600006,5.2,-0.258507407000015));
#313271=CARTESIAN_POINT('Ctrl Pts',(-4.01631199600006,2.2,-0.258507407000015));
#313272=CARTESIAN_POINT('Ctrl Pts',(-4.01694108800006,12.2,-0.258627721000018));
#313273=CARTESIAN_POINT('Ctrl Pts',(-4.01694108800006,5.2,-0.258627721000018));
#313274=CARTESIAN_POINT('Ctrl Pts',(-4.01694108800006,2.2,-0.258627721000018));
#313275=CARTESIAN_POINT('Ctrl Pts',(-4.01757603300006,12.2,-0.258749997000014));
#313276=CARTESIAN_POINT('Ctrl Pts',(-4.01757603300006,5.2,-0.258749997000014));
#313277=CARTESIAN_POINT('Ctrl Pts',(-4.01757603300006,2.2,-0.258749997000014));
#313278=CARTESIAN_POINT('Ctrl Pts',(-4.01821681600006,12.2,-0.258874247000014));
#313279=CARTESIAN_POINT('Ctrl Pts',(-4.01821681600006,5.2,-0.258874247000014));
#313280=CARTESIAN_POINT('Ctrl Pts',(-4.01821681600006,2.2,-0.258874247000014));
#313281=CARTESIAN_POINT('Ctrl Pts',(-4.01886342200005,12.2,-0.259000484000014));
#313282=CARTESIAN_POINT('Ctrl Pts',(-4.01886342200005,5.2,-0.259000484000014));
#313283=CARTESIAN_POINT('Ctrl Pts',(-4.01886342200005,2.2,-0.259000484000014));
#313284=CARTESIAN_POINT('Ctrl Pts',(-4.01951583600006,12.2,-0.259128719000015));
#313285=CARTESIAN_POINT('Ctrl Pts',(-4.01951583600006,5.2,-0.259128719000015));
#313286=CARTESIAN_POINT('Ctrl Pts',(-4.01951583600006,2.2,-0.259128719000015));
#313287=CARTESIAN_POINT('Ctrl Pts',(-4.02017404300006,12.2,-0.259258965000013));
#313288=CARTESIAN_POINT('Ctrl Pts',(-4.02017404300006,5.2,-0.259258965000013));
#313289=CARTESIAN_POINT('Ctrl Pts',(-4.02017404300006,2.2,-0.259258965000013));
#313290=CARTESIAN_POINT('Ctrl Pts',(-4.02083802800006,12.2,-0.259391235000015));
#313291=CARTESIAN_POINT('Ctrl Pts',(-4.02083802800006,5.2,-0.259391235000015));
#313292=CARTESIAN_POINT('Ctrl Pts',(-4.02083802800006,2.2,-0.259391235000015));
#313293=CARTESIAN_POINT('Ctrl Pts',(-4.02150777400006,12.2,-0.259525539000016));
#313294=CARTESIAN_POINT('Ctrl Pts',(-4.02150777400006,5.2,-0.259525539000016));
#313295=CARTESIAN_POINT('Ctrl Pts',(-4.02150777400006,2.2,-0.259525539000016));
#313296=CARTESIAN_POINT('Ctrl Pts',(-4.02218326800006,12.2,-0.259661892000014));
#313297=CARTESIAN_POINT('Ctrl Pts',(-4.02218326800006,5.2,-0.259661892000014));
#313298=CARTESIAN_POINT('Ctrl Pts',(-4.02218326800006,2.2,-0.259661892000014));
#313299=CARTESIAN_POINT('Ctrl Pts',(-4.02286449500005,12.2,-0.259800303000013));
#313300=CARTESIAN_POINT('Ctrl Pts',(-4.02286449500005,5.2,-0.259800303000013));
#313301=CARTESIAN_POINT('Ctrl Pts',(-4.02286449500005,2.2,-0.259800303000013));
#313302=CARTESIAN_POINT('Ctrl Pts',(-4.02355143800006,12.2,-0.259940787000015));
#313303=CARTESIAN_POINT('Ctrl Pts',(-4.02355143800006,5.2,-0.259940787000015));
#313304=CARTESIAN_POINT('Ctrl Pts',(-4.02355143800006,2.2,-0.259940787000015));
#313305=CARTESIAN_POINT('Ctrl Pts',(-4.02424408400006,12.2,-0.260083353000016));
#313306=CARTESIAN_POINT('Ctrl Pts',(-4.02424408400006,5.2,-0.260083353000016));
#313307=CARTESIAN_POINT('Ctrl Pts',(-4.02424408400006,2.2,-0.260083353000016));
#313308=CARTESIAN_POINT('Ctrl Pts',(-4.02494241700006,12.2,-0.260228017000017));
#313309=CARTESIAN_POINT('Ctrl Pts',(-4.02494241700006,5.2,-0.260228017000017));
#313310=CARTESIAN_POINT('Ctrl Pts',(-4.02494241700006,2.2,-0.260228017000017));
#313311=CARTESIAN_POINT('Ctrl Pts',(-4.02564642300006,12.2,-0.260374786000015));
#313312=CARTESIAN_POINT('Ctrl Pts',(-4.02564642300006,5.2,-0.260374786000015));
#313313=CARTESIAN_POINT('Ctrl Pts',(-4.02564642300006,2.2,-0.260374786000015));
#313314=CARTESIAN_POINT('Ctrl Pts',(-4.02635608600006,12.2,-0.260523675000015));
#313315=CARTESIAN_POINT('Ctrl Pts',(-4.02635608600006,5.2,-0.260523675000015));
#313316=CARTESIAN_POINT('Ctrl Pts',(-4.02635608600006,2.2,-0.260523675000015));
#313317=CARTESIAN_POINT('Ctrl Pts',(-4.02707139100006,12.2,-0.260674696000014));
#313318=CARTESIAN_POINT('Ctrl Pts',(-4.02707139100006,5.2,-0.260674696000014));
#313319=CARTESIAN_POINT('Ctrl Pts',(-4.02707139100006,2.2,-0.260674696000014));
#313320=CARTESIAN_POINT('Ctrl Pts',(-4.02779232400006,12.2,-0.260827857000017));
#313321=CARTESIAN_POINT('Ctrl Pts',(-4.02779232400006,5.2,-0.260827857000017));
#313322=CARTESIAN_POINT('Ctrl Pts',(-4.02779232400006,2.2,-0.260827857000017));
#313323=CARTESIAN_POINT('Ctrl Pts',(-4.02851887100006,12.2,-0.260983174000016));
#313324=CARTESIAN_POINT('Ctrl Pts',(-4.02851887100006,5.2,-0.260983174000016));
#313325=CARTESIAN_POINT('Ctrl Pts',(-4.02851887100006,2.2,-0.260983174000016));
#313326=CARTESIAN_POINT('Ctrl Pts',(-4.02925101400006,12.2,-0.261140657000016));
#313327=CARTESIAN_POINT('Ctrl Pts',(-4.02925101400006,5.2,-0.261140657000016));
#313328=CARTESIAN_POINT('Ctrl Pts',(-4.02925101400006,2.2,-0.261140657000016));
#313329=CARTESIAN_POINT('Ctrl Pts',(-4.02998874200006,12.2,-0.261300316000015));
#313330=CARTESIAN_POINT('Ctrl Pts',(-4.02998874200006,5.2,-0.261300316000015));
#313331=CARTESIAN_POINT('Ctrl Pts',(-4.02998874200006,2.2,-0.261300316000015));
#313332=CARTESIAN_POINT('Ctrl Pts',(-4.03073203800006,12.2,-0.261462165000013));
#313333=CARTESIAN_POINT('Ctrl Pts',(-4.03073203800006,5.2,-0.261462165000013));
#313334=CARTESIAN_POINT('Ctrl Pts',(-4.03073203800006,2.2,-0.261462165000013));
#313335=CARTESIAN_POINT('Ctrl Pts',(-4.03148088800005,12.2,-0.261626214000015));
#313336=CARTESIAN_POINT('Ctrl Pts',(-4.03148088800005,5.2,-0.261626214000015));
#313337=CARTESIAN_POINT('Ctrl Pts',(-4.03148088800005,2.2,-0.261626214000015));
#313338=CARTESIAN_POINT('Ctrl Pts',(-4.03223527700006,12.2,-0.261792474000018));
#313339=CARTESIAN_POINT('Ctrl Pts',(-4.03223527700006,5.2,-0.261792474000018));
#313340=CARTESIAN_POINT('Ctrl Pts',(-4.03223527700006,2.2,-0.261792474000018));
#313341=CARTESIAN_POINT('Ctrl Pts',(-4.03299519000006,12.2,-0.261960957000014));
#313342=CARTESIAN_POINT('Ctrl Pts',(-4.03299519000006,5.2,-0.261960957000014));
#313343=CARTESIAN_POINT('Ctrl Pts',(-4.03299519000006,2.2,-0.261960957000014));
#313344=CARTESIAN_POINT('Ctrl Pts',(-4.03376061300006,12.2,-0.262131675000017));
#313345=CARTESIAN_POINT('Ctrl Pts',(-4.03376061300006,5.2,-0.262131675000017));
#313346=CARTESIAN_POINT('Ctrl Pts',(-4.03376061300006,2.2,-0.262131675000017));
#313347=CARTESIAN_POINT('Ctrl Pts',(-4.03453153200005,12.2,-0.262304639000015));
#313348=CARTESIAN_POINT('Ctrl Pts',(-4.03453153200005,5.2,-0.262304639000015));
#313349=CARTESIAN_POINT('Ctrl Pts',(-4.03453153200005,2.2,-0.262304639000015));
#313350=CARTESIAN_POINT('Ctrl Pts',(-4.03530793100006,12.2,-0.262479859000013));
#313351=CARTESIAN_POINT('Ctrl Pts',(-4.03530793100006,5.2,-0.262479859000013));
#313352=CARTESIAN_POINT('Ctrl Pts',(-4.03530793100006,2.2,-0.262479859000013));
#313353=CARTESIAN_POINT('Ctrl Pts',(-4.03608979700006,12.2,-0.262657346000013));
#313354=CARTESIAN_POINT('Ctrl Pts',(-4.03608979700006,5.2,-0.262657346000013));
#313355=CARTESIAN_POINT('Ctrl Pts',(-4.03608979700006,2.2,-0.262657346000013));
#313356=CARTESIAN_POINT('Ctrl Pts',(-4.03687711300006,12.2,-0.262837114000014));
#313357=CARTESIAN_POINT('Ctrl Pts',(-4.03687711300006,5.2,-0.262837114000014));
#313358=CARTESIAN_POINT('Ctrl Pts',(-4.03687711300006,2.2,-0.262837114000014));
#313359=CARTESIAN_POINT('Ctrl Pts',(-4.03766986700006,12.2,-0.263019170000014));
#313360=CARTESIAN_POINT('Ctrl Pts',(-4.03766986700006,5.2,-0.263019170000014));
#313361=CARTESIAN_POINT('Ctrl Pts',(-4.03766986700006,2.2,-0.263019170000014));
#313362=CARTESIAN_POINT('Ctrl Pts',(-4.03846804300006,12.2,-0.263203529000013));
#313363=CARTESIAN_POINT('Ctrl Pts',(-4.03846804300006,5.2,-0.263203529000013));
#313364=CARTESIAN_POINT('Ctrl Pts',(-4.03846804300006,2.2,-0.263203529000013));
#313365=CARTESIAN_POINT('Ctrl Pts',(-4.03927162800006,12.2,-0.263390198000018));
#313366=CARTESIAN_POINT('Ctrl Pts',(-4.03927162800006,5.2,-0.263390198000018));
#313367=CARTESIAN_POINT('Ctrl Pts',(-4.03927162800006,2.2,-0.263390198000018));
#313368=CARTESIAN_POINT('Ctrl Pts',(-4.04008060700006,12.2,-0.263579191000014));
#313369=CARTESIAN_POINT('Ctrl Pts',(-4.04008060700006,5.2,-0.263579191000014));
#313370=CARTESIAN_POINT('Ctrl Pts',(-4.04008060700006,2.2,-0.263579191000014));
#313371=CARTESIAN_POINT('Ctrl Pts',(-4.04089496400006,12.2,-0.263770518000013));
#313372=CARTESIAN_POINT('Ctrl Pts',(-4.04089496400006,5.2,-0.263770518000013));
#313373=CARTESIAN_POINT('Ctrl Pts',(-4.04089496400006,2.2,-0.263770518000013));
#313374=CARTESIAN_POINT('Ctrl Pts',(-4.04171468700006,12.2,-0.263964188000014));
#313375=CARTESIAN_POINT('Ctrl Pts',(-4.04171468700006,5.2,-0.263964188000014));
#313376=CARTESIAN_POINT('Ctrl Pts',(-4.04171468700006,2.2,-0.263964188000014));
#313377=CARTESIAN_POINT('Ctrl Pts',(-4.04253976000006,12.2,-0.264160215000011));
#313378=CARTESIAN_POINT('Ctrl Pts',(-4.04253976000006,5.2,-0.264160215000011));
#313379=CARTESIAN_POINT('Ctrl Pts',(-4.04253976000006,2.2,-0.264160215000011));
#313380=CARTESIAN_POINT('Ctrl Pts',(-4.04337016900006,12.2,-0.264358608000013));
#313381=CARTESIAN_POINT('Ctrl Pts',(-4.04337016900006,5.2,-0.264358608000013));
#313382=CARTESIAN_POINT('Ctrl Pts',(-4.04337016900006,2.2,-0.264358608000013));
#313383=CARTESIAN_POINT('Ctrl Pts',(-4.04420590100006,12.2,-0.264559377000015));
#313384=CARTESIAN_POINT('Ctrl Pts',(-4.04420590100006,5.2,-0.264559377000015));
#313385=CARTESIAN_POINT('Ctrl Pts',(-4.04420590100006,2.2,-0.264559377000015));
#313386=CARTESIAN_POINT('Ctrl Pts',(-4.04504693900006,12.2,-0.264762533000016));
#313387=CARTESIAN_POINT('Ctrl Pts',(-4.04504693900006,5.2,-0.264762533000016));
#313388=CARTESIAN_POINT('Ctrl Pts',(-4.04504693900006,2.2,-0.264762533000016));
#313389=CARTESIAN_POINT('Ctrl Pts',(-4.04589327100005,12.2,-0.264968088000015));
#313390=CARTESIAN_POINT('Ctrl Pts',(-4.04589327100005,5.2,-0.264968088000015));
#313391=CARTESIAN_POINT('Ctrl Pts',(-4.04589327100005,2.2,-0.264968088000015));
#313392=CARTESIAN_POINT('Ctrl Pts',(-4.04674488400006,12.2,-0.265176050000013));
#313393=CARTESIAN_POINT('Ctrl Pts',(-4.04674488400006,5.2,-0.265176050000013));
#313394=CARTESIAN_POINT('Ctrl Pts',(-4.04674488400006,2.2,-0.265176050000013));
#313395=CARTESIAN_POINT('Ctrl Pts',(-4.04760176000006,12.2,-0.265386433000017));
#313396=CARTESIAN_POINT('Ctrl Pts',(-4.04760176000006,5.2,-0.265386433000017));
#313397=CARTESIAN_POINT('Ctrl Pts',(-4.04760176000006,2.2,-0.265386433000017));
#313398=CARTESIAN_POINT('Ctrl Pts',(-4.04846388700006,12.2,-0.265599244000012));
#313399=CARTESIAN_POINT('Ctrl Pts',(-4.04846388700006,5.2,-0.265599244000012));
#313400=CARTESIAN_POINT('Ctrl Pts',(-4.04846388700006,2.2,-0.265599244000012));
#313401=CARTESIAN_POINT('Ctrl Pts',(-4.04933125200006,12.2,-0.265814494000014));
#313402=CARTESIAN_POINT('Ctrl Pts',(-4.04933125200006,5.2,-0.265814494000014));
#313403=CARTESIAN_POINT('Ctrl Pts',(-4.04933125200006,2.2,-0.265814494000014));
#313404=CARTESIAN_POINT('Ctrl Pts',(-4.05020383900006,12.2,-0.266032196000014));
#313405=CARTESIAN_POINT('Ctrl Pts',(-4.05020383900006,5.2,-0.266032196000014));
#313406=CARTESIAN_POINT('Ctrl Pts',(-4.05020383900006,2.2,-0.266032196000014));
#313407=CARTESIAN_POINT('Ctrl Pts',(-4.05108163400006,12.2,-0.266252357000014));
#313408=CARTESIAN_POINT('Ctrl Pts',(-4.05108163400006,5.2,-0.266252357000014));
#313409=CARTESIAN_POINT('Ctrl Pts',(-4.05108163400006,2.2,-0.266252357000014));
#313410=CARTESIAN_POINT('Ctrl Pts',(-4.05196462400006,12.2,-0.266474989000014));
#313411=CARTESIAN_POINT('Ctrl Pts',(-4.05196462400006,5.2,-0.266474989000014));
#313412=CARTESIAN_POINT('Ctrl Pts',(-4.05196462400006,2.2,-0.266474989000014));
#313413=CARTESIAN_POINT('Ctrl Pts',(-4.05285279300006,12.2,-0.266700102000015));
#313414=CARTESIAN_POINT('Ctrl Pts',(-4.05285279300006,5.2,-0.266700102000015));
#313415=CARTESIAN_POINT('Ctrl Pts',(-4.05285279300006,2.2,-0.266700102000015));
#313416=CARTESIAN_POINT('Ctrl Pts',(-4.05374613000006,12.2,-0.266927706000013));
#313417=CARTESIAN_POINT('Ctrl Pts',(-4.05374613000006,5.2,-0.266927706000013));
#313418=CARTESIAN_POINT('Ctrl Pts',(-4.05374613000006,2.2,-0.266927706000013));
#313419=CARTESIAN_POINT('Ctrl Pts',(-4.05464461800006,12.2,-0.267157813000014));
#313420=CARTESIAN_POINT('Ctrl Pts',(-4.05464461800006,5.2,-0.267157813000014));
#313421=CARTESIAN_POINT('Ctrl Pts',(-4.05464461800006,2.2,-0.267157813000014));
#313422=CARTESIAN_POINT('Ctrl Pts',(-4.05554824500006,12.2,-0.267390429000014));
#313423=CARTESIAN_POINT('Ctrl Pts',(-4.05554824500006,5.2,-0.267390429000014));
#313424=CARTESIAN_POINT('Ctrl Pts',(-4.05554824500006,2.2,-0.267390429000014));
#313425=CARTESIAN_POINT('Ctrl Pts',(-4.05645699600006,12.2,-0.267625566000014));
#313426=CARTESIAN_POINT('Ctrl Pts',(-4.05645699600006,5.2,-0.267625566000014));
#313427=CARTESIAN_POINT('Ctrl Pts',(-4.05645699600006,2.2,-0.267625566000014));
#313428=CARTESIAN_POINT('Ctrl Pts',(-4.05737085800006,12.2,-0.267863236000014));
#313429=CARTESIAN_POINT('Ctrl Pts',(-4.05737085800006,5.2,-0.267863236000014));
#313430=CARTESIAN_POINT('Ctrl Pts',(-4.05737085800006,2.2,-0.267863236000014));
#313431=CARTESIAN_POINT('Ctrl Pts',(-4.05828981600005,12.2,-0.268103446000012));
#313432=CARTESIAN_POINT('Ctrl Pts',(-4.05828981600005,5.2,-0.268103446000012));
#313433=CARTESIAN_POINT('Ctrl Pts',(-4.05828981600005,2.2,-0.268103446000012));
#313434=CARTESIAN_POINT('Ctrl Pts',(-4.05921385700006,12.2,-0.268346208000012));
#313435=CARTESIAN_POINT('Ctrl Pts',(-4.05921385700006,5.2,-0.268346208000012));
#313436=CARTESIAN_POINT('Ctrl Pts',(-4.05921385700006,2.2,-0.268346208000012));
#313437=CARTESIAN_POINT('Ctrl Pts',(-4.06014296600006,12.2,-0.268591531000015));
#313438=CARTESIAN_POINT('Ctrl Pts',(-4.06014296600006,5.2,-0.268591531000015));
#313439=CARTESIAN_POINT('Ctrl Pts',(-4.06014296600006,2.2,-0.268591531000015));
#313440=CARTESIAN_POINT('Ctrl Pts',(-4.06107713000006,12.2,-0.268839425000014));
#313441=CARTESIAN_POINT('Ctrl Pts',(-4.06107713000006,5.2,-0.268839425000014));
#313442=CARTESIAN_POINT('Ctrl Pts',(-4.06107713000006,2.2,-0.268839425000014));
#313443=CARTESIAN_POINT('Ctrl Pts',(-4.06201633600006,12.2,-0.269089899000012));
#313444=CARTESIAN_POINT('Ctrl Pts',(-4.06201633600006,5.2,-0.269089899000012));
#313445=CARTESIAN_POINT('Ctrl Pts',(-4.06201633600006,2.2,-0.269089899000012));
#313446=CARTESIAN_POINT('Ctrl Pts',(-4.06296056800006,12.2,-0.269342965000017));
#313447=CARTESIAN_POINT('Ctrl Pts',(-4.06296056800006,5.2,-0.269342965000017));
#313448=CARTESIAN_POINT('Ctrl Pts',(-4.06296056800006,2.2,-0.269342965000017));
#313449=CARTESIAN_POINT('Ctrl Pts',(-4.06390981400006,12.2,-0.269598630000014));
#313450=CARTESIAN_POINT('Ctrl Pts',(-4.06390981400006,5.2,-0.269598630000014));
#313451=CARTESIAN_POINT('Ctrl Pts',(-4.06390981400006,2.2,-0.269598630000014));
#313452=CARTESIAN_POINT('Ctrl Pts',(-4.06486406100006,12.2,-0.269856904000014));
#313453=CARTESIAN_POINT('Ctrl Pts',(-4.06486406100006,5.2,-0.269856904000014));
#313454=CARTESIAN_POINT('Ctrl Pts',(-4.06486406100006,2.2,-0.269856904000014));
#313455=CARTESIAN_POINT('Ctrl Pts',(-4.06582329200006,12.2,-0.270117798000014));
#313456=CARTESIAN_POINT('Ctrl Pts',(-4.06582329200006,5.2,-0.270117798000014));
#313457=CARTESIAN_POINT('Ctrl Pts',(-4.06582329200006,2.2,-0.270117798000014));
#313458=CARTESIAN_POINT('Ctrl Pts',(-4.06678749700006,12.2,-0.270381321000013));
#313459=CARTESIAN_POINT('Ctrl Pts',(-4.06678749700006,5.2,-0.270381321000013));
#313460=CARTESIAN_POINT('Ctrl Pts',(-4.06678749700006,2.2,-0.270381321000013));
#313461=CARTESIAN_POINT('Ctrl Pts',(-4.06775666000006,12.2,-0.270647483000013));
#313462=CARTESIAN_POINT('Ctrl Pts',(-4.06775666000006,5.2,-0.270647483000013));
#313463=CARTESIAN_POINT('Ctrl Pts',(-4.06775666000006,2.2,-0.270647483000013));
#313464=CARTESIAN_POINT('Ctrl Pts',(-4.06873076700006,12.2,-0.270916292000014));
#313465=CARTESIAN_POINT('Ctrl Pts',(-4.06873076700006,5.2,-0.270916292000014));
#313466=CARTESIAN_POINT('Ctrl Pts',(-4.06873076700006,2.2,-0.270916292000014));
#313467=CARTESIAN_POINT('Ctrl Pts',(-4.06970980600006,12.2,-0.271187759000018));
#313468=CARTESIAN_POINT('Ctrl Pts',(-4.06970980600006,5.2,-0.271187759000018));
#313469=CARTESIAN_POINT('Ctrl Pts',(-4.06970980600006,2.2,-0.271187759000018));
#313470=CARTESIAN_POINT('Ctrl Pts',(-4.07069376400006,12.2,-0.271461893000016));
#313471=CARTESIAN_POINT('Ctrl Pts',(-4.07069376400006,5.2,-0.271461893000016));
#313472=CARTESIAN_POINT('Ctrl Pts',(-4.07069376400006,2.2,-0.271461893000016));
#313473=CARTESIAN_POINT('Ctrl Pts',(-4.07168262500006,12.2,-0.271738703000013));
#313474=CARTESIAN_POINT('Ctrl Pts',(-4.07168262500006,5.2,-0.271738703000013));
#313475=CARTESIAN_POINT('Ctrl Pts',(-4.07168262500006,2.2,-0.271738703000013));
#313476=CARTESIAN_POINT('Ctrl Pts',(-4.07267637700006,12.2,-0.272018198000015));
#313477=CARTESIAN_POINT('Ctrl Pts',(-4.07267637700006,5.2,-0.272018198000015));
#313478=CARTESIAN_POINT('Ctrl Pts',(-4.07267637700006,2.2,-0.272018198000015));
#313479=CARTESIAN_POINT('Ctrl Pts',(-4.07367500500006,12.2,-0.272300389000013));
#313480=CARTESIAN_POINT('Ctrl Pts',(-4.07367500500006,5.2,-0.272300389000013));
#313481=CARTESIAN_POINT('Ctrl Pts',(-4.07367500500006,2.2,-0.272300389000013));
#313482=CARTESIAN_POINT('Ctrl Pts',(-4.07467849800006,12.2,-0.272585283000013));
#313483=CARTESIAN_POINT('Ctrl Pts',(-4.07467849800006,5.2,-0.272585283000013));
#313484=CARTESIAN_POINT('Ctrl Pts',(-4.07467849800006,2.2,-0.272585283000013));
#313485=CARTESIAN_POINT('Ctrl Pts',(-4.07568684000006,12.2,-0.272872891000016));
#313486=CARTESIAN_POINT('Ctrl Pts',(-4.07568684000006,5.2,-0.272872891000016));
#313487=CARTESIAN_POINT('Ctrl Pts',(-4.07568684000006,2.2,-0.272872891000016));
#313488=CARTESIAN_POINT('Ctrl Pts',(-4.07670001800006,12.2,-0.273163221000012));
#313489=CARTESIAN_POINT('Ctrl Pts',(-4.07670001800006,5.2,-0.273163221000012));
#313490=CARTESIAN_POINT('Ctrl Pts',(-4.07670001800006,2.2,-0.273163221000012));
#313491=CARTESIAN_POINT('Ctrl Pts',(-4.07771802000005,12.2,-0.273456282000013));
#313492=CARTESIAN_POINT('Ctrl Pts',(-4.07771802000005,5.2,-0.273456282000013));
#313493=CARTESIAN_POINT('Ctrl Pts',(-4.07771802000005,2.2,-0.273456282000013));
#313494=CARTESIAN_POINT('Ctrl Pts',(-4.07874083200006,12.2,-0.273752085000014));
#313495=CARTESIAN_POINT('Ctrl Pts',(-4.07874083200006,5.2,-0.273752085000014));
#313496=CARTESIAN_POINT('Ctrl Pts',(-4.07874083200006,2.2,-0.273752085000014));
#313497=CARTESIAN_POINT('Ctrl Pts',(-4.07976843800006,12.2,-0.274050636000016));
#313498=CARTESIAN_POINT('Ctrl Pts',(-4.07976843800006,5.2,-0.274050636000016));
#313499=CARTESIAN_POINT('Ctrl Pts',(-4.07976843800006,2.2,-0.274050636000016));
#313500=CARTESIAN_POINT('Ctrl Pts',(-4.08080082900006,12.2,-0.274351947000016));
#313501=CARTESIAN_POINT('Ctrl Pts',(-4.08080082900006,5.2,-0.274351947000016));
#313502=CARTESIAN_POINT('Ctrl Pts',(-4.08080082900006,2.2,-0.274351947000016));
#313503=CARTESIAN_POINT('Ctrl Pts',(-4.08183798800006,12.2,-0.274656025000013));
#313504=CARTESIAN_POINT('Ctrl Pts',(-4.08183798800006,5.2,-0.274656025000013));
#313505=CARTESIAN_POINT('Ctrl Pts',(-4.08183798800006,2.2,-0.274656025000013));
#313506=CARTESIAN_POINT('Ctrl Pts',(-4.08287990400006,12.2,-0.274962880000014));
#313507=CARTESIAN_POINT('Ctrl Pts',(-4.08287990400006,5.2,-0.274962880000014));
#313508=CARTESIAN_POINT('Ctrl Pts',(-4.08287990400006,2.2,-0.274962880000014));
#313509=CARTESIAN_POINT('Ctrl Pts',(-4.08392656300006,12.2,-0.275272521000014));
#313510=CARTESIAN_POINT('Ctrl Pts',(-4.08392656300006,5.2,-0.275272521000014));
#313511=CARTESIAN_POINT('Ctrl Pts',(-4.08392656300006,2.2,-0.275272521000014));
#313512=CARTESIAN_POINT('Ctrl Pts',(-4.08497795100006,12.2,-0.275584955000014));
#313513=CARTESIAN_POINT('Ctrl Pts',(-4.08497795100006,5.2,-0.275584955000014));
#313514=CARTESIAN_POINT('Ctrl Pts',(-4.08497795100006,2.2,-0.275584955000014));
#313515=CARTESIAN_POINT('Ctrl Pts',(-4.08603405500005,12.2,-0.275900193000016));
#313516=CARTESIAN_POINT('Ctrl Pts',(-4.08603405500005,5.2,-0.275900193000016));
#313517=CARTESIAN_POINT('Ctrl Pts',(-4.08603405500005,2.2,-0.275900193000016));
#313518=CARTESIAN_POINT('Ctrl Pts',(-4.08709486100006,12.2,-0.276218243000015));
#313519=CARTESIAN_POINT('Ctrl Pts',(-4.08709486100006,5.2,-0.276218243000015));
#313520=CARTESIAN_POINT('Ctrl Pts',(-4.08709486100006,2.2,-0.276218243000015));
#313521=CARTESIAN_POINT('Ctrl Pts',(-4.08816035700006,12.2,-0.276539114000016));
#313522=CARTESIAN_POINT('Ctrl Pts',(-4.08816035700006,5.2,-0.276539114000016));
#313523=CARTESIAN_POINT('Ctrl Pts',(-4.08816035700006,2.2,-0.276539114000016));
#313524=CARTESIAN_POINT('Ctrl Pts',(-4.08923052900006,12.2,-0.276862813000012));
#313525=CARTESIAN_POINT('Ctrl Pts',(-4.08923052900006,5.2,-0.276862813000012));
#313526=CARTESIAN_POINT('Ctrl Pts',(-4.08923052900006,2.2,-0.276862813000012));
#313527=CARTESIAN_POINT('Ctrl Pts',(-4.09030536500006,12.2,-0.277189351000011));
#313528=CARTESIAN_POINT('Ctrl Pts',(-4.09030536500006,5.2,-0.277189351000011));
#313529=CARTESIAN_POINT('Ctrl Pts',(-4.09030536500006,2.2,-0.277189351000011));
#313530=CARTESIAN_POINT('Ctrl Pts',(-4.09138485100006,12.2,-0.277518736000015));
#313531=CARTESIAN_POINT('Ctrl Pts',(-4.09138485100006,5.2,-0.277518736000015));
#313532=CARTESIAN_POINT('Ctrl Pts',(-4.09138485100006,2.2,-0.277518736000015));
#313533=CARTESIAN_POINT('Ctrl Pts',(-4.09246897300005,12.2,-0.277850975000016));
#313534=CARTESIAN_POINT('Ctrl Pts',(-4.09246897300005,5.2,-0.277850975000016));
#313535=CARTESIAN_POINT('Ctrl Pts',(-4.09246897300005,2.2,-0.277850975000016));
#313536=CARTESIAN_POINT('Ctrl Pts',(-4.09355771900006,12.2,-0.278186080000014));
#313537=CARTESIAN_POINT('Ctrl Pts',(-4.09355771900006,5.2,-0.278186080000014));
#313538=CARTESIAN_POINT('Ctrl Pts',(-4.09355771900006,2.2,-0.278186080000014));
#313539=CARTESIAN_POINT('Ctrl Pts',(-4.09465107500006,12.2,-0.278524055000013));
#313540=CARTESIAN_POINT('Ctrl Pts',(-4.09465107500006,5.2,-0.278524055000013));
#313541=CARTESIAN_POINT('Ctrl Pts',(-4.09465107500006,2.2,-0.278524055000013));
#313542=CARTESIAN_POINT('Ctrl Pts',(-4.09574902900006,12.2,-0.278864911000016));
#313543=CARTESIAN_POINT('Ctrl Pts',(-4.09574902900006,5.2,-0.278864911000016));
#313544=CARTESIAN_POINT('Ctrl Pts',(-4.09574902900006,2.2,-0.278864911000016));
#313545=CARTESIAN_POINT('Ctrl Pts',(-4.09685156700006,12.2,-0.279208658000014));
#313546=CARTESIAN_POINT('Ctrl Pts',(-4.09685156700006,5.2,-0.279208658000014));
#313547=CARTESIAN_POINT('Ctrl Pts',(-4.09685156700006,2.2,-0.279208658000014));
#313548=CARTESIAN_POINT('Ctrl Pts',(-4.09795867600006,12.2,-0.279555301000016));
#313549=CARTESIAN_POINT('Ctrl Pts',(-4.09795867600006,5.2,-0.279555301000016));
#313550=CARTESIAN_POINT('Ctrl Pts',(-4.09795867600006,2.2,-0.279555301000016));
#313551=CARTESIAN_POINT('Ctrl Pts',(-4.09907034300006,12.2,-0.279904851000015));
#313552=CARTESIAN_POINT('Ctrl Pts',(-4.09907034300006,5.2,-0.279904851000015));
#313553=CARTESIAN_POINT('Ctrl Pts',(-4.09907034300006,2.2,-0.279904851000015));
#313554=CARTESIAN_POINT('Ctrl Pts',(-4.10018655600005,12.2,-0.280257314000014));
#313555=CARTESIAN_POINT('Ctrl Pts',(-4.10018655600005,5.2,-0.280257314000014));
#313556=CARTESIAN_POINT('Ctrl Pts',(-4.10018655600005,2.2,-0.280257314000014));
#313557=CARTESIAN_POINT('Ctrl Pts',(-4.10130730000006,12.2,-0.280612701000016));
#313558=CARTESIAN_POINT('Ctrl Pts',(-4.10130730000006,5.2,-0.280612701000016));
#313559=CARTESIAN_POINT('Ctrl Pts',(-4.10130730000006,2.2,-0.280612701000016));
#313560=CARTESIAN_POINT('Ctrl Pts',(-4.10243256400006,12.2,-0.280971018000016));
#313561=CARTESIAN_POINT('Ctrl Pts',(-4.10243256400006,5.2,-0.280971018000016));
#313562=CARTESIAN_POINT('Ctrl Pts',(-4.10243256400006,2.2,-0.280971018000016));
#313563=CARTESIAN_POINT('Ctrl Pts',(-4.10356233300006,12.2,-0.281332274000015));
#313564=CARTESIAN_POINT('Ctrl Pts',(-4.10356233300006,5.2,-0.281332274000015));
#313565=CARTESIAN_POINT('Ctrl Pts',(-4.10356233300006,2.2,-0.281332274000015));
#313566=CARTESIAN_POINT('Ctrl Pts',(-4.10469659600006,12.2,-0.281696478000013));
#313567=CARTESIAN_POINT('Ctrl Pts',(-4.10469659600006,5.2,-0.281696478000013));
#313568=CARTESIAN_POINT('Ctrl Pts',(-4.10469659600006,2.2,-0.281696478000013));
#313569=CARTESIAN_POINT('Ctrl Pts',(-4.10583533900006,12.2,-0.282063637000016));
#313570=CARTESIAN_POINT('Ctrl Pts',(-4.10583533900006,5.2,-0.282063637000016));
#313571=CARTESIAN_POINT('Ctrl Pts',(-4.10583533900006,2.2,-0.282063637000016));
#313572=CARTESIAN_POINT('Ctrl Pts',(-4.10697855000006,12.2,-0.282433760000016));
#313573=CARTESIAN_POINT('Ctrl Pts',(-4.10697855000006,5.2,-0.282433760000016));
#313574=CARTESIAN_POINT('Ctrl Pts',(-4.10697855000006,2.2,-0.282433760000016));
#313575=CARTESIAN_POINT('Ctrl Pts',(-4.10812621400006,12.2,-0.282806853000017));
#313576=CARTESIAN_POINT('Ctrl Pts',(-4.10812621400006,5.2,-0.282806853000017));
#313577=CARTESIAN_POINT('Ctrl Pts',(-4.10812621400006,2.2,-0.282806853000017));
#313578=CARTESIAN_POINT('Ctrl Pts',(-4.10927832100006,12.2,-0.283182927000016));
#313579=CARTESIAN_POINT('Ctrl Pts',(-4.10927832100006,5.2,-0.283182927000016));
#313580=CARTESIAN_POINT('Ctrl Pts',(-4.10927832100006,2.2,-0.283182927000016));
#313581=CARTESIAN_POINT('Ctrl Pts',(-4.11043485600006,12.2,-0.283561988000014));
#313582=CARTESIAN_POINT('Ctrl Pts',(-4.11043485600006,5.2,-0.283561988000014));
#313583=CARTESIAN_POINT('Ctrl Pts',(-4.11043485600006,2.2,-0.283561988000014));
#313584=CARTESIAN_POINT('Ctrl Pts',(-4.11159580800006,12.2,-0.283944045000015));
#313585=CARTESIAN_POINT('Ctrl Pts',(-4.11159580800006,5.2,-0.283944045000015));
#313586=CARTESIAN_POINT('Ctrl Pts',(-4.11159580800006,2.2,-0.283944045000015));
#313587=CARTESIAN_POINT('Ctrl Pts',(-4.11276116200006,12.2,-0.284329106000012));
#313588=CARTESIAN_POINT('Ctrl Pts',(-4.11276116200006,5.2,-0.284329106000012));
#313589=CARTESIAN_POINT('Ctrl Pts',(-4.11276116200006,2.2,-0.284329106000012));
#313590=CARTESIAN_POINT('Ctrl Pts',(-4.11393090500006,12.2,-0.284717178000014));
#313591=CARTESIAN_POINT('Ctrl Pts',(-4.11393090500006,5.2,-0.284717178000014));
#313592=CARTESIAN_POINT('Ctrl Pts',(-4.11393090500006,2.2,-0.284717178000014));
#313593=CARTESIAN_POINT('Ctrl Pts',(-4.11510502700006,12.2,-0.285108269000016));
#313594=CARTESIAN_POINT('Ctrl Pts',(-4.11510502700006,5.2,-0.285108269000016));
#313595=CARTESIAN_POINT('Ctrl Pts',(-4.11510502700006,2.2,-0.285108269000016));
#313596=CARTESIAN_POINT('Ctrl Pts',(-4.11628351300006,12.2,-0.285502388000012));
#313597=CARTESIAN_POINT('Ctrl Pts',(-4.11628351300006,5.2,-0.285502388000012));
#313598=CARTESIAN_POINT('Ctrl Pts',(-4.11628351300006,2.2,-0.285502388000012));
#313599=CARTESIAN_POINT('Ctrl Pts',(-4.11746635200006,12.2,-0.285899541000014));
#313600=CARTESIAN_POINT('Ctrl Pts',(-4.11746635200006,5.2,-0.285899541000014));
#313601=CARTESIAN_POINT('Ctrl Pts',(-4.11746635200006,2.2,-0.285899541000014));
#313602=CARTESIAN_POINT('Ctrl Pts',(-4.11865353000006,12.2,-0.286299737000015));
#313603=CARTESIAN_POINT('Ctrl Pts',(-4.11865353000006,5.2,-0.286299737000015));
#313604=CARTESIAN_POINT('Ctrl Pts',(-4.11865353000006,2.2,-0.286299737000015));
#313605=CARTESIAN_POINT('Ctrl Pts',(-4.11984503400006,12.2,-0.286702984000016));
#313606=CARTESIAN_POINT('Ctrl Pts',(-4.11984503400006,5.2,-0.286702984000016));
#313607=CARTESIAN_POINT('Ctrl Pts',(-4.11984503400006,2.2,-0.286702984000016));
#313608=CARTESIAN_POINT('Ctrl Pts',(-4.12104085200006,12.2,-0.287109289000016));
#313609=CARTESIAN_POINT('Ctrl Pts',(-4.12104085200006,5.2,-0.287109289000016));
#313610=CARTESIAN_POINT('Ctrl Pts',(-4.12104085200006,2.2,-0.287109289000016));
#313611=CARTESIAN_POINT('Ctrl Pts',(-4.12224097100006,12.2,-0.287518659000017));
#313612=CARTESIAN_POINT('Ctrl Pts',(-4.12224097100006,5.2,-0.287518659000017));
#313613=CARTESIAN_POINT('Ctrl Pts',(-4.12224097100006,2.2,-0.287518659000017));
#313614=CARTESIAN_POINT('Ctrl Pts',(-4.12344537900006,12.2,-0.287931103000014));
#313615=CARTESIAN_POINT('Ctrl Pts',(-4.12344537900006,5.2,-0.287931103000014));
#313616=CARTESIAN_POINT('Ctrl Pts',(-4.12344537900006,2.2,-0.287931103000014));
#313617=CARTESIAN_POINT('Ctrl Pts',(-4.12465406200006,12.2,-0.288346629000014));
#313618=CARTESIAN_POINT('Ctrl Pts',(-4.12465406200006,5.2,-0.288346629000014));
#313619=CARTESIAN_POINT('Ctrl Pts',(-4.12465406200006,2.2,-0.288346629000014));
#313620=CARTESIAN_POINT('Ctrl Pts',(-4.12586700900006,12.2,-0.288765242000015));
#313621=CARTESIAN_POINT('Ctrl Pts',(-4.12586700900006,5.2,-0.288765242000015));
#313622=CARTESIAN_POINT('Ctrl Pts',(-4.12586700900006,2.2,-0.288765242000015));
#313623=CARTESIAN_POINT('Ctrl Pts',(-4.12708420700006,12.2,-0.289186952000016));
#313624=CARTESIAN_POINT('Ctrl Pts',(-4.12708420700006,5.2,-0.289186952000016));
#313625=CARTESIAN_POINT('Ctrl Pts',(-4.12708420700006,2.2,-0.289186952000016));
#313626=CARTESIAN_POINT('Ctrl Pts',(-4.12830564200006,12.2,-0.289611766000015));
#313627=CARTESIAN_POINT('Ctrl Pts',(-4.12830564200006,5.2,-0.289611766000015));
#313628=CARTESIAN_POINT('Ctrl Pts',(-4.12830564200006,2.2,-0.289611766000015));
#313629=CARTESIAN_POINT('Ctrl Pts',(-4.12953130400005,12.2,-0.290039691000015));
#313630=CARTESIAN_POINT('Ctrl Pts',(-4.12953130400005,5.2,-0.290039691000015));
#313631=CARTESIAN_POINT('Ctrl Pts',(-4.12953130400005,2.2,-0.290039691000015));
#313632=CARTESIAN_POINT('Ctrl Pts',(-4.13076117800006,12.2,-0.290470733000014));
#313633=CARTESIAN_POINT('Ctrl Pts',(-4.13076117800006,5.2,-0.290470733000014));
#313634=CARTESIAN_POINT('Ctrl Pts',(-4.13076117800006,2.2,-0.290470733000014));
#313635=CARTESIAN_POINT('Ctrl Pts',(-4.13199525200006,12.2,-0.290904902000015));
#313636=CARTESIAN_POINT('Ctrl Pts',(-4.13199525200006,5.2,-0.290904902000015));
#313637=CARTESIAN_POINT('Ctrl Pts',(-4.13199525200006,2.2,-0.290904902000015));
#313638=CARTESIAN_POINT('Ctrl Pts',(-4.13323351500006,12.2,-0.291342204000014));
#313639=CARTESIAN_POINT('Ctrl Pts',(-4.13323351500006,5.2,-0.291342204000014));
#313640=CARTESIAN_POINT('Ctrl Pts',(-4.13323351500006,2.2,-0.291342204000014));
#313641=CARTESIAN_POINT('Ctrl Pts',(-4.13447595200005,12.2,-0.291782647000014));
#313642=CARTESIAN_POINT('Ctrl Pts',(-4.13447595200005,5.2,-0.291782647000014));
#313643=CARTESIAN_POINT('Ctrl Pts',(-4.13447595200005,2.2,-0.291782647000014));
#313644=CARTESIAN_POINT('Ctrl Pts',(-4.13572255400006,12.2,-0.292226238000013));
#313645=CARTESIAN_POINT('Ctrl Pts',(-4.13572255400006,5.2,-0.292226238000013));
#313646=CARTESIAN_POINT('Ctrl Pts',(-4.13572255400006,2.2,-0.292226238000013));
#313647=CARTESIAN_POINT('Ctrl Pts',(-4.13697330500006,12.2,-0.292672984000015));
#313648=CARTESIAN_POINT('Ctrl Pts',(-4.13697330500006,5.2,-0.292672984000015));
#313649=CARTESIAN_POINT('Ctrl Pts',(-4.13697330500006,2.2,-0.292672984000015));
#313650=CARTESIAN_POINT('Ctrl Pts',(-4.13822819500006,12.2,-0.293122892000017));
#313651=CARTESIAN_POINT('Ctrl Pts',(-4.13822819500006,5.2,-0.293122892000017));
#313652=CARTESIAN_POINT('Ctrl Pts',(-4.13822819500006,2.2,-0.293122892000017));
#313653=CARTESIAN_POINT('Ctrl Pts',(-4.13948721100006,12.2,-0.293575970000015));
#313654=CARTESIAN_POINT('Ctrl Pts',(-4.13948721100006,5.2,-0.293575970000015));
#313655=CARTESIAN_POINT('Ctrl Pts',(-4.13948721100006,2.2,-0.293575970000015));
#313656=CARTESIAN_POINT('Ctrl Pts',(-4.14075033900006,12.2,-0.294032225000014));
#313657=CARTESIAN_POINT('Ctrl Pts',(-4.14075033900006,5.2,-0.294032225000014));
#313658=CARTESIAN_POINT('Ctrl Pts',(-4.14075033900006,2.2,-0.294032225000014));
#313659=CARTESIAN_POINT('Ctrl Pts',(-4.14201756800006,12.2,-0.294491663000014));
#313660=CARTESIAN_POINT('Ctrl Pts',(-4.14201756800006,5.2,-0.294491663000014));
#313661=CARTESIAN_POINT('Ctrl Pts',(-4.14201756800006,2.2,-0.294491663000014));
#313662=CARTESIAN_POINT('Ctrl Pts',(-4.14328888700005,12.2,-0.294954293000016));
#313663=CARTESIAN_POINT('Ctrl Pts',(-4.14328888700005,5.2,-0.294954293000016));
#313664=CARTESIAN_POINT('Ctrl Pts',(-4.14328888700005,2.2,-0.294954293000016));
#313665=CARTESIAN_POINT('Ctrl Pts',(-4.14456428100006,12.2,-0.295420121000016));
#313666=CARTESIAN_POINT('Ctrl Pts',(-4.14456428100006,5.2,-0.295420121000016));
#313667=CARTESIAN_POINT('Ctrl Pts',(-4.14456428100006,2.2,-0.295420121000016));
#313668=CARTESIAN_POINT('Ctrl Pts',(-4.14584373900006,12.2,-0.295889154000015));
#313669=CARTESIAN_POINT('Ctrl Pts',(-4.14584373900006,5.2,-0.295889154000015));
#313670=CARTESIAN_POINT('Ctrl Pts',(-4.14584373900006,2.2,-0.295889154000015));
#313671=CARTESIAN_POINT('Ctrl Pts',(-4.14712724900006,12.2,-0.296361399000014));
#313672=CARTESIAN_POINT('Ctrl Pts',(-4.14712724900006,5.2,-0.296361399000014));
#313673=CARTESIAN_POINT('Ctrl Pts',(-4.14712724900006,2.2,-0.296361399000014));
#313674=CARTESIAN_POINT('Ctrl Pts',(-4.14841479800006,12.2,-0.296836863000016));
#313675=CARTESIAN_POINT('Ctrl Pts',(-4.14841479800006,5.2,-0.296836863000016));
#313676=CARTESIAN_POINT('Ctrl Pts',(-4.14841479800006,2.2,-0.296836863000016));
#313677=CARTESIAN_POINT('Ctrl Pts',(-4.14970637400006,12.2,-0.297315553000015));
#313678=CARTESIAN_POINT('Ctrl Pts',(-4.14970637400006,5.2,-0.297315553000015));
#313679=CARTESIAN_POINT('Ctrl Pts',(-4.14970637400006,2.2,-0.297315553000015));
#313680=CARTESIAN_POINT('Ctrl Pts',(-4.15100196400005,12.2,-0.297797477000015));
#313681=CARTESIAN_POINT('Ctrl Pts',(-4.15100196400005,5.2,-0.297797477000015));
#313682=CARTESIAN_POINT('Ctrl Pts',(-4.15100196400005,2.2,-0.297797477000015));
#313683=CARTESIAN_POINT('Ctrl Pts',(-4.15230155800006,12.2,-0.298282640000016));
#313684=CARTESIAN_POINT('Ctrl Pts',(-4.15230155800006,5.2,-0.298282640000016));
#313685=CARTESIAN_POINT('Ctrl Pts',(-4.15230155800006,2.2,-0.298282640000016));
#313686=CARTESIAN_POINT('Ctrl Pts',(-4.15360514100006,12.2,-0.298771050000015));
#313687=CARTESIAN_POINT('Ctrl Pts',(-4.15360514100006,5.2,-0.298771050000015));
#313688=CARTESIAN_POINT('Ctrl Pts',(-4.15360514100006,2.2,-0.298771050000015));
#313689=CARTESIAN_POINT('Ctrl Pts',(-4.15491270200006,12.2,-0.299262713000013));
#313690=CARTESIAN_POINT('Ctrl Pts',(-4.15491270200006,5.2,-0.299262713000013));
#313691=CARTESIAN_POINT('Ctrl Pts',(-4.15491270200006,2.2,-0.299262713000013));
#313692=CARTESIAN_POINT('Ctrl Pts',(-4.15622423000006,12.2,-0.299757637000013));
#313693=CARTESIAN_POINT('Ctrl Pts',(-4.15622423000006,5.2,-0.299757637000013));
#313694=CARTESIAN_POINT('Ctrl Pts',(-4.15622423000006,2.2,-0.299757637000013));
#313695=CARTESIAN_POINT('Ctrl Pts',(-4.15753971000006,12.2,-0.300255828000013));
#313696=CARTESIAN_POINT('Ctrl Pts',(-4.15753971000006,5.2,-0.300255828000013));
#313697=CARTESIAN_POINT('Ctrl Pts',(-4.15753971000006,2.2,-0.300255828000013));
#313698=CARTESIAN_POINT('Ctrl Pts',(-4.15885913200006,12.2,-0.300757293000018));
#313699=CARTESIAN_POINT('Ctrl Pts',(-4.15885913200006,5.2,-0.300757293000018));
#313700=CARTESIAN_POINT('Ctrl Pts',(-4.15885913200006,2.2,-0.300757293000018));
#313701=CARTESIAN_POINT('Ctrl Pts',(-4.16018248400006,12.2,-0.301262039000014));
#313702=CARTESIAN_POINT('Ctrl Pts',(-4.16018248400006,5.2,-0.301262039000014));
#313703=CARTESIAN_POINT('Ctrl Pts',(-4.16018248400006,2.2,-0.301262039000014));
#313704=CARTESIAN_POINT('Ctrl Pts',(-4.16150975300006,12.2,-0.301770072000016));
#313705=CARTESIAN_POINT('Ctrl Pts',(-4.16150975300006,5.2,-0.301770072000016));
#313706=CARTESIAN_POINT('Ctrl Pts',(-4.16150975300006,2.2,-0.301770072000016));
#313707=CARTESIAN_POINT('Ctrl Pts',(-4.16284092600006,12.2,-0.302281398000015));
#313708=CARTESIAN_POINT('Ctrl Pts',(-4.16284092600006,5.2,-0.302281398000015));
#313709=CARTESIAN_POINT('Ctrl Pts',(-4.16284092600006,2.2,-0.302281398000015));
#313710=CARTESIAN_POINT('Ctrl Pts',(-4.16417599400006,12.2,-0.302796026000016));
#313711=CARTESIAN_POINT('Ctrl Pts',(-4.16417599400006,5.2,-0.302796026000016));
#313712=CARTESIAN_POINT('Ctrl Pts',(-4.16417599400006,2.2,-0.302796026000016));
#313713=CARTESIAN_POINT('Ctrl Pts',(-4.16551494100006,12.2,-0.303313960000011));
#313714=CARTESIAN_POINT('Ctrl Pts',(-4.16551494100006,5.2,-0.303313960000011));
#313715=CARTESIAN_POINT('Ctrl Pts',(-4.16551494100006,2.2,-0.303313960000011));
#313716=CARTESIAN_POINT('Ctrl Pts',(-4.16685775800006,12.2,-0.303835207000014));
#313717=CARTESIAN_POINT('Ctrl Pts',(-4.16685775800006,5.2,-0.303835207000014));
#313718=CARTESIAN_POINT('Ctrl Pts',(-4.16685775800006,2.2,-0.303835207000014));
#313719=CARTESIAN_POINT('Ctrl Pts',(-4.16820443100006,12.2,-0.304359775000016));
#313720=CARTESIAN_POINT('Ctrl Pts',(-4.16820443100006,5.2,-0.304359775000016));
#313721=CARTESIAN_POINT('Ctrl Pts',(-4.16820443100006,2.2,-0.304359775000016));
#313722=CARTESIAN_POINT('Ctrl Pts',(-4.16955495000006,12.2,-0.304887670000014));
#313723=CARTESIAN_POINT('Ctrl Pts',(-4.16955495000006,5.2,-0.304887670000014));
#313724=CARTESIAN_POINT('Ctrl Pts',(-4.16955495000006,2.2,-0.304887670000014));
#313725=CARTESIAN_POINT('Ctrl Pts',(-4.17090930000006,12.2,-0.305418899000016));
#313726=CARTESIAN_POINT('Ctrl Pts',(-4.17090930000006,5.2,-0.305418899000016));
#313727=CARTESIAN_POINT('Ctrl Pts',(-4.17090930000006,2.2,-0.305418899000016));
#313728=CARTESIAN_POINT('Ctrl Pts',(-4.17226747200006,12.2,-0.305953466000015));
#313729=CARTESIAN_POINT('Ctrl Pts',(-4.17226747200006,5.2,-0.305953466000015));
#313730=CARTESIAN_POINT('Ctrl Pts',(-4.17226747200006,2.2,-0.305953466000015));
#313731=CARTESIAN_POINT('Ctrl Pts',(-4.17362945300006,12.2,-0.306491379000011));
#313732=CARTESIAN_POINT('Ctrl Pts',(-4.17362945300006,5.2,-0.306491379000011));
#313733=CARTESIAN_POINT('Ctrl Pts',(-4.17362945300006,2.2,-0.306491379000011));
#313734=CARTESIAN_POINT('Ctrl Pts',(-4.17499523000005,12.2,-0.307032645000014));
#313735=CARTESIAN_POINT('Ctrl Pts',(-4.17499523000005,5.2,-0.307032645000014));
#313736=CARTESIAN_POINT('Ctrl Pts',(-4.17499523000005,2.2,-0.307032645000014));
#313737=CARTESIAN_POINT('Ctrl Pts',(-4.17636479300006,12.2,-0.307577269000014));
#313738=CARTESIAN_POINT('Ctrl Pts',(-4.17636479300006,5.2,-0.307577269000014));
#313739=CARTESIAN_POINT('Ctrl Pts',(-4.17636479300006,2.2,-0.307577269000014));
#313740=CARTESIAN_POINT('Ctrl Pts',(-4.17773812700006,12.2,-0.308125259000014));
#313741=CARTESIAN_POINT('Ctrl Pts',(-4.17773812700006,5.2,-0.308125259000014));
#313742=CARTESIAN_POINT('Ctrl Pts',(-4.17773812700006,2.2,-0.308125259000014));
#313743=CARTESIAN_POINT('Ctrl Pts',(-4.17911522400006,12.2,-0.308676620000017));
#313744=CARTESIAN_POINT('Ctrl Pts',(-4.17911522400006,5.2,-0.308676620000017));
#313745=CARTESIAN_POINT('Ctrl Pts',(-4.17911522400006,2.2,-0.308676620000017));
#313746=CARTESIAN_POINT('Ctrl Pts',(-4.18049606900006,12.2,-0.309231359000015));
#313747=CARTESIAN_POINT('Ctrl Pts',(-4.18049606900006,5.2,-0.309231359000015));
#313748=CARTESIAN_POINT('Ctrl Pts',(-4.18049606900006,2.2,-0.309231359000015));
#313749=CARTESIAN_POINT('Ctrl Pts',(-4.18188065100006,12.2,-0.309789482000014));
#313750=CARTESIAN_POINT('Ctrl Pts',(-4.18188065100006,5.2,-0.309789482000014));
#313751=CARTESIAN_POINT('Ctrl Pts',(-4.18188065100006,2.2,-0.309789482000014));
#313752=CARTESIAN_POINT('Ctrl Pts',(-4.18326895900006,12.2,-0.310350994000017));
#313753=CARTESIAN_POINT('Ctrl Pts',(-4.18326895900006,5.2,-0.310350994000017));
#313754=CARTESIAN_POINT('Ctrl Pts',(-4.18326895900006,2.2,-0.310350994000017));
#313755=CARTESIAN_POINT('Ctrl Pts',(-4.18466098000006,12.2,-0.310915903000013));
#313756=CARTESIAN_POINT('Ctrl Pts',(-4.18466098000006,5.2,-0.310915903000013));
#313757=CARTESIAN_POINT('Ctrl Pts',(-4.18466098000006,2.2,-0.310915903000013));
#313758=CARTESIAN_POINT('Ctrl Pts',(-4.18605670300006,12.2,-0.311484214000015));
#313759=CARTESIAN_POINT('Ctrl Pts',(-4.18605670300006,5.2,-0.311484214000015));
#313760=CARTESIAN_POINT('Ctrl Pts',(-4.18605670300006,2.2,-0.311484214000015));
#313761=CARTESIAN_POINT('Ctrl Pts',(-4.18745611600006,12.2,-0.312055933000015));
#313762=CARTESIAN_POINT('Ctrl Pts',(-4.18745611600006,5.2,-0.312055933000015));
#313763=CARTESIAN_POINT('Ctrl Pts',(-4.18745611600006,2.2,-0.312055933000015));
#313764=CARTESIAN_POINT('Ctrl Pts',(-4.18885920600006,12.2,-0.312631068000013));
#313765=CARTESIAN_POINT('Ctrl Pts',(-4.18885920600006,5.2,-0.312631068000013));
#313766=CARTESIAN_POINT('Ctrl Pts',(-4.18885920600006,2.2,-0.312631068000013));
#313767=CARTESIAN_POINT('Ctrl Pts',(-4.19026596400006,12.2,-0.313209622000015));
#313768=CARTESIAN_POINT('Ctrl Pts',(-4.19026596400006,5.2,-0.313209622000015));
#313769=CARTESIAN_POINT('Ctrl Pts',(-4.19026596400006,2.2,-0.313209622000015));
#313770=CARTESIAN_POINT('Ctrl Pts',(-4.19167637400006,12.2,-0.313791604000015));
#313771=CARTESIAN_POINT('Ctrl Pts',(-4.19167637400006,5.2,-0.313791604000015));
#313772=CARTESIAN_POINT('Ctrl Pts',(-4.19167637400006,2.2,-0.313791604000015));
#313773=CARTESIAN_POINT('Ctrl Pts',(-4.19309042900006,12.2,-0.314377018000016));
#313774=CARTESIAN_POINT('Ctrl Pts',(-4.19309042900006,5.2,-0.314377018000016));
#313775=CARTESIAN_POINT('Ctrl Pts',(-4.19309042900006,2.2,-0.314377018000016));
#313776=CARTESIAN_POINT('Ctrl Pts',(-4.19450811400006,12.2,-0.314965871000012));
#313777=CARTESIAN_POINT('Ctrl Pts',(-4.19450811400006,5.2,-0.314965871000012));
#313778=CARTESIAN_POINT('Ctrl Pts',(-4.19450811400006,2.2,-0.314965871000012));
#313779=CARTESIAN_POINT('Ctrl Pts',(-4.19592941800006,12.2,-0.315558168000014));
#313780=CARTESIAN_POINT('Ctrl Pts',(-4.19592941800006,5.2,-0.315558168000014));
#313781=CARTESIAN_POINT('Ctrl Pts',(-4.19592941800006,2.2,-0.315558168000014));
#313782=CARTESIAN_POINT('Ctrl Pts',(-4.19735432900006,12.2,-0.316153917000013));
#313783=CARTESIAN_POINT('Ctrl Pts',(-4.19735432900006,5.2,-0.316153917000013));
#313784=CARTESIAN_POINT('Ctrl Pts',(-4.19735432900006,2.2,-0.316153917000013));
#313785=CARTESIAN_POINT('Ctrl Pts',(-4.19878283700006,12.2,-0.316753122000013));
#313786=CARTESIAN_POINT('Ctrl Pts',(-4.19878283700006,5.2,-0.316753122000013));
#313787=CARTESIAN_POINT('Ctrl Pts',(-4.19878283700006,2.2,-0.316753122000013));
#313788=CARTESIAN_POINT('Ctrl Pts',(-4.20021492800006,12.2,-0.317355788000011));
#313789=CARTESIAN_POINT('Ctrl Pts',(-4.20021492800006,5.2,-0.317355788000011));
#313790=CARTESIAN_POINT('Ctrl Pts',(-4.20021492800006,2.2,-0.317355788000011));
#313791=CARTESIAN_POINT('Ctrl Pts',(-4.20165059300006,12.2,-0.317961924000016));
#313792=CARTESIAN_POINT('Ctrl Pts',(-4.20165059300006,5.2,-0.317961924000016));
#313793=CARTESIAN_POINT('Ctrl Pts',(-4.20165059300006,2.2,-0.317961924000016));
#313794=CARTESIAN_POINT('Ctrl Pts',(-4.20308981700006,12.2,-0.318571533000016));
#313795=CARTESIAN_POINT('Ctrl Pts',(-4.20308981700006,5.2,-0.318571533000016));
#313796=CARTESIAN_POINT('Ctrl Pts',(-4.20308981700006,2.2,-0.318571533000016));
#313797=CARTESIAN_POINT('Ctrl Pts',(-4.20453259100006,12.2,-0.319184622000015));
#313798=CARTESIAN_POINT('Ctrl Pts',(-4.20453259100006,5.2,-0.319184622000015));
#313799=CARTESIAN_POINT('Ctrl Pts',(-4.20453259100006,2.2,-0.319184622000015));
#313800=CARTESIAN_POINT('Ctrl Pts',(-4.20597890300006,12.2,-0.319801197000014));
#313801=CARTESIAN_POINT('Ctrl Pts',(-4.20597890300006,5.2,-0.319801197000014));
#313802=CARTESIAN_POINT('Ctrl Pts',(-4.20597890300006,2.2,-0.319801197000014));
#313803=CARTESIAN_POINT('Ctrl Pts',(-4.20742873900006,12.2,-0.320421263000017));
#313804=CARTESIAN_POINT('Ctrl Pts',(-4.20742873900006,5.2,-0.320421263000017));
#313805=CARTESIAN_POINT('Ctrl Pts',(-4.20742873900006,2.2,-0.320421263000017));
#313806=CARTESIAN_POINT('Ctrl Pts',(-4.20888209100006,12.2,-0.321044826000012));
#313807=CARTESIAN_POINT('Ctrl Pts',(-4.20888209100006,5.2,-0.321044826000012));
#313808=CARTESIAN_POINT('Ctrl Pts',(-4.20888209100006,2.2,-0.321044826000012));
#313809=CARTESIAN_POINT('Ctrl Pts',(-4.21033894600006,12.2,-0.321671892000013));
#313810=CARTESIAN_POINT('Ctrl Pts',(-4.21033894600006,5.2,-0.321671892000013));
#313811=CARTESIAN_POINT('Ctrl Pts',(-4.21033894600006,2.2,-0.321671892000013));
#313812=CARTESIAN_POINT('Ctrl Pts',(-4.21179929100005,12.2,-0.322302466000015));
#313813=CARTESIAN_POINT('Ctrl Pts',(-4.21179929100005,5.2,-0.322302466000015));
#313814=CARTESIAN_POINT('Ctrl Pts',(-4.21179929100005,2.2,-0.322302466000015));
#313815=CARTESIAN_POINT('Ctrl Pts',(-4.21326311600006,12.2,-0.322936554000015));
#313816=CARTESIAN_POINT('Ctrl Pts',(-4.21326311600006,5.2,-0.322936554000015));
#313817=CARTESIAN_POINT('Ctrl Pts',(-4.21326311600006,2.2,-0.322936554000015));
#313818=CARTESIAN_POINT('Ctrl Pts',(-4.21473040900006,12.2,-0.323574162000018));
#313819=CARTESIAN_POINT('Ctrl Pts',(-4.21473040900006,5.2,-0.323574162000018));
#313820=CARTESIAN_POINT('Ctrl Pts',(-4.21473040900006,2.2,-0.323574162000018));
#313821=CARTESIAN_POINT('Ctrl Pts',(-4.21620115900006,12.2,-0.324215295000014));
#313822=CARTESIAN_POINT('Ctrl Pts',(-4.21620115900006,5.2,-0.324215295000014));
#313823=CARTESIAN_POINT('Ctrl Pts',(-4.21620115900006,2.2,-0.324215295000014));
#313824=CARTESIAN_POINT('Ctrl Pts',(-4.21767535400006,12.2,-0.324859958000014));
#313825=CARTESIAN_POINT('Ctrl Pts',(-4.21767535400006,5.2,-0.324859958000014));
#313826=CARTESIAN_POINT('Ctrl Pts',(-4.21767535400006,2.2,-0.324859958000014));
#313827=CARTESIAN_POINT('Ctrl Pts',(-4.21915298100005,12.2,-0.325508158000014));
#313828=CARTESIAN_POINT('Ctrl Pts',(-4.21915298100005,5.2,-0.325508158000014));
#313829=CARTESIAN_POINT('Ctrl Pts',(-4.21915298100005,2.2,-0.325508158000014));
#313830=CARTESIAN_POINT('Ctrl Pts',(-4.22063403100006,12.2,-0.326159900000014));
#313831=CARTESIAN_POINT('Ctrl Pts',(-4.22063403100006,5.2,-0.326159900000014));
#313832=CARTESIAN_POINT('Ctrl Pts',(-4.22063403100006,2.2,-0.326159900000014));
#313833=CARTESIAN_POINT('Ctrl Pts',(-4.22211849200006,12.2,-0.326815189000014));
#313834=CARTESIAN_POINT('Ctrl Pts',(-4.22211849200006,5.2,-0.326815189000014));
#313835=CARTESIAN_POINT('Ctrl Pts',(-4.22211849200006,2.2,-0.326815189000014));
#313836=CARTESIAN_POINT('Ctrl Pts',(-4.22360635200006,12.2,-0.327474030000015));
#313837=CARTESIAN_POINT('Ctrl Pts',(-4.22360635200006,5.2,-0.327474030000015));
#313838=CARTESIAN_POINT('Ctrl Pts',(-4.22360635200006,2.2,-0.327474030000015));
#313839=CARTESIAN_POINT('Ctrl Pts',(-4.22509760000006,12.2,-0.328136431000012));
#313840=CARTESIAN_POINT('Ctrl Pts',(-4.22509760000006,5.2,-0.328136431000012));
#313841=CARTESIAN_POINT('Ctrl Pts',(-4.22509760000006,2.2,-0.328136431000012));
#313842=CARTESIAN_POINT('Ctrl Pts',(-4.22659222400006,12.2,-0.328802394000016));
#313843=CARTESIAN_POINT('Ctrl Pts',(-4.22659222400006,5.2,-0.328802394000016));
#313844=CARTESIAN_POINT('Ctrl Pts',(-4.22659222400006,2.2,-0.328802394000016));
#313845=CARTESIAN_POINT('Ctrl Pts',(-4.22809021300006,12.2,-0.329471925000018));
#313846=CARTESIAN_POINT('Ctrl Pts',(-4.22809021300006,5.2,-0.329471925000018));
#313847=CARTESIAN_POINT('Ctrl Pts',(-4.22809021300006,2.2,-0.329471925000018));
#313848=CARTESIAN_POINT('Ctrl Pts',(-4.22959155500005,12.2,-0.330145032000013));
#313849=CARTESIAN_POINT('Ctrl Pts',(-4.22959155500005,5.2,-0.330145032000013));
#313850=CARTESIAN_POINT('Ctrl Pts',(-4.22959155500005,2.2,-0.330145032000013));
#313851=CARTESIAN_POINT('Ctrl Pts',(-4.23109624000006,12.2,-0.330821718000016));
#313852=CARTESIAN_POINT('Ctrl Pts',(-4.23109624000006,5.2,-0.330821718000016));
#313853=CARTESIAN_POINT('Ctrl Pts',(-4.23109624000006,2.2,-0.330821718000016));
#313854=CARTESIAN_POINT('Ctrl Pts',(-4.23260425500006,12.2,-0.331501989000014));
#313855=CARTESIAN_POINT('Ctrl Pts',(-4.23260425500006,5.2,-0.331501989000014));
#313856=CARTESIAN_POINT('Ctrl Pts',(-4.23260425500006,2.2,-0.331501989000014));
#313857=CARTESIAN_POINT('Ctrl Pts',(-4.23411558900006,12.2,-0.332185850000015));
#313858=CARTESIAN_POINT('Ctrl Pts',(-4.23411558900006,5.2,-0.332185850000015));
#313859=CARTESIAN_POINT('Ctrl Pts',(-4.23411558900006,2.2,-0.332185850000015));
#313860=CARTESIAN_POINT('Ctrl Pts',(-4.23563023200006,12.2,-0.332873306000017));
#313861=CARTESIAN_POINT('Ctrl Pts',(-4.23563023200006,5.2,-0.332873306000017));
#313862=CARTESIAN_POINT('Ctrl Pts',(-4.23563023200006,2.2,-0.332873306000017));
#313863=CARTESIAN_POINT('Ctrl Pts',(-4.23714817100006,12.2,-0.333564363000014));
#313864=CARTESIAN_POINT('Ctrl Pts',(-4.23714817100006,5.2,-0.333564363000014));
#313865=CARTESIAN_POINT('Ctrl Pts',(-4.23714817100006,2.2,-0.333564363000014));
#313866=CARTESIAN_POINT('Ctrl Pts',(-4.23866939600006,12.2,-0.334259026000012));
#313867=CARTESIAN_POINT('Ctrl Pts',(-4.23866939600006,5.2,-0.334259026000012));
#313868=CARTESIAN_POINT('Ctrl Pts',(-4.23866939600006,2.2,-0.334259026000012));
#313869=CARTESIAN_POINT('Ctrl Pts',(-4.24019389600006,12.2,-0.334957299000016));
#313870=CARTESIAN_POINT('Ctrl Pts',(-4.24019389600006,5.2,-0.334957299000016));
#313871=CARTESIAN_POINT('Ctrl Pts',(-4.24019389600006,2.2,-0.334957299000016));
#313872=CARTESIAN_POINT('Ctrl Pts',(-4.24172165700006,12.2,-0.335659190000013));
#313873=CARTESIAN_POINT('Ctrl Pts',(-4.24172165700006,5.2,-0.335659190000013));
#313874=CARTESIAN_POINT('Ctrl Pts',(-4.24172165700006,2.2,-0.335659190000013));
#313875=CARTESIAN_POINT('Ctrl Pts',(-4.24325267100006,12.2,-0.336364701000011));
#313876=CARTESIAN_POINT('Ctrl Pts',(-4.24325267100006,5.2,-0.336364701000011));
#313877=CARTESIAN_POINT('Ctrl Pts',(-4.24325267100006,2.2,-0.336364701000011));
#313878=CARTESIAN_POINT('Ctrl Pts',(-4.24478692500006,12.2,-0.337073838000013));
#313879=CARTESIAN_POINT('Ctrl Pts',(-4.24478692500006,5.2,-0.337073838000013));
#313880=CARTESIAN_POINT('Ctrl Pts',(-4.24478692500006,2.2,-0.337073838000013));
#313881=CARTESIAN_POINT('Ctrl Pts',(-4.24632440700006,12.2,-0.337786607000012));
#313882=CARTESIAN_POINT('Ctrl Pts',(-4.24632440700006,5.2,-0.337786607000012));
#313883=CARTESIAN_POINT('Ctrl Pts',(-4.24632440700006,2.2,-0.337786607000012));
#313884=CARTESIAN_POINT('Ctrl Pts',(-4.24786510800006,12.2,-0.338503012000011));
#313885=CARTESIAN_POINT('Ctrl Pts',(-4.24786510800006,5.2,-0.338503012000011));
#313886=CARTESIAN_POINT('Ctrl Pts',(-4.24786510800006,2.2,-0.338503012000011));
#313887=CARTESIAN_POINT('Ctrl Pts',(-4.24940901600006,12.2,-0.339223059000013));
#313888=CARTESIAN_POINT('Ctrl Pts',(-4.24940901600006,5.2,-0.339223059000013));
#313889=CARTESIAN_POINT('Ctrl Pts',(-4.24940901600006,2.2,-0.339223059000013));
#313890=CARTESIAN_POINT('Ctrl Pts',(-4.25095611900006,12.2,-0.339946752000015));
#313891=CARTESIAN_POINT('Ctrl Pts',(-4.25095611900006,5.2,-0.339946752000015));
#313892=CARTESIAN_POINT('Ctrl Pts',(-4.25095611900006,2.2,-0.339946752000015));
#313893=CARTESIAN_POINT('Ctrl Pts',(-4.25250640600006,12.2,-0.340674097000013));
#313894=CARTESIAN_POINT('Ctrl Pts',(-4.25250640600006,5.2,-0.340674097000013));
#313895=CARTESIAN_POINT('Ctrl Pts',(-4.25250640600006,2.2,-0.340674097000013));
#313896=CARTESIAN_POINT('Ctrl Pts',(-4.25405986600006,12.2,-0.341405097000016));
#313897=CARTESIAN_POINT('Ctrl Pts',(-4.25405986600006,5.2,-0.341405097000016));
#313898=CARTESIAN_POINT('Ctrl Pts',(-4.25405986600006,2.2,-0.341405097000016));
#313899=CARTESIAN_POINT('Ctrl Pts',(-4.25561648900006,12.2,-0.342139760000015));
#313900=CARTESIAN_POINT('Ctrl Pts',(-4.25561648900006,5.2,-0.342139760000015));
#313901=CARTESIAN_POINT('Ctrl Pts',(-4.25561648900006,2.2,-0.342139760000015));
#313902=CARTESIAN_POINT('Ctrl Pts',(-4.25717626100006,12.2,-0.342878088000016));
#313903=CARTESIAN_POINT('Ctrl Pts',(-4.25717626100006,5.2,-0.342878088000016));
#313904=CARTESIAN_POINT('Ctrl Pts',(-4.25717626100006,2.2,-0.342878088000016));
#313905=CARTESIAN_POINT('Ctrl Pts',(-4.25873917500006,12.2,-0.343620088000014));
#313906=CARTESIAN_POINT('Ctrl Pts',(-4.25873917500006,5.2,-0.343620088000014));
#313907=CARTESIAN_POINT('Ctrl Pts',(-4.25873917500006,2.2,-0.343620088000014));
#313908=CARTESIAN_POINT('Ctrl Pts',(-4.26030521600006,12.2,-0.344365764000014));
#313909=CARTESIAN_POINT('Ctrl Pts',(-4.26030521600006,5.2,-0.344365764000014));
#313910=CARTESIAN_POINT('Ctrl Pts',(-4.26030521600006,2.2,-0.344365764000014));
#313911=CARTESIAN_POINT('Ctrl Pts',(-4.26187437500006,12.2,-0.345115121000017));
#313912=CARTESIAN_POINT('Ctrl Pts',(-4.26187437500006,5.2,-0.345115121000017));
#313913=CARTESIAN_POINT('Ctrl Pts',(-4.26187437500006,2.2,-0.345115121000017));
#313914=CARTESIAN_POINT('Ctrl Pts',(-4.26344664100006,12.2,-0.345868163000014));
#313915=CARTESIAN_POINT('Ctrl Pts',(-4.26344664100006,5.2,-0.345868163000014));
#313916=CARTESIAN_POINT('Ctrl Pts',(-4.26344664100006,2.2,-0.345868163000014));
#313917=CARTESIAN_POINT('Ctrl Pts',(-4.26502200200006,12.2,-0.346624895000014));
#313918=CARTESIAN_POINT('Ctrl Pts',(-4.26502200200006,5.2,-0.346624895000014));
#313919=CARTESIAN_POINT('Ctrl Pts',(-4.26502200200006,2.2,-0.346624895000014));
#313920=CARTESIAN_POINT('Ctrl Pts',(-4.26660044600006,12.2,-0.347385322000013));
#313921=CARTESIAN_POINT('Ctrl Pts',(-4.26660044600006,5.2,-0.347385322000013));
#313922=CARTESIAN_POINT('Ctrl Pts',(-4.26660044600006,2.2,-0.347385322000013));
#313923=CARTESIAN_POINT('Ctrl Pts',(-4.26818196500006,12.2,-0.348149450000013));
#313924=CARTESIAN_POINT('Ctrl Pts',(-4.26818196500006,5.2,-0.348149450000013));
#313925=CARTESIAN_POINT('Ctrl Pts',(-4.26818196500006,2.2,-0.348149450000013));
#313926=CARTESIAN_POINT('Ctrl Pts',(-4.26976654500006,12.2,-0.348917282000016));
#313927=CARTESIAN_POINT('Ctrl Pts',(-4.26976654500006,5.2,-0.348917282000016));
#313928=CARTESIAN_POINT('Ctrl Pts',(-4.26976654500006,2.2,-0.348917282000016));
#313929=CARTESIAN_POINT('Ctrl Pts',(-4.27135417700006,12.2,-0.349688824000012));
#313930=CARTESIAN_POINT('Ctrl Pts',(-4.27135417700006,5.2,-0.349688824000012));
#313931=CARTESIAN_POINT('Ctrl Pts',(-4.27135417700006,2.2,-0.349688824000012));
#313932=CARTESIAN_POINT('Ctrl Pts',(-4.27294484900006,12.2,-0.350464078000012));
#313933=CARTESIAN_POINT('Ctrl Pts',(-4.27294484900006,5.2,-0.350464078000012));
#313934=CARTESIAN_POINT('Ctrl Pts',(-4.27294484900006,2.2,-0.350464078000012));
#313935=CARTESIAN_POINT('Ctrl Pts',(-4.27453855000006,12.2,-0.351243052000014));
#313936=CARTESIAN_POINT('Ctrl Pts',(-4.27453855000006,5.2,-0.351243052000014));
#313937=CARTESIAN_POINT('Ctrl Pts',(-4.27453855000006,2.2,-0.351243052000014));
#313938=CARTESIAN_POINT('Ctrl Pts',(-4.27613527000006,12.2,-0.352025750000013));
#313939=CARTESIAN_POINT('Ctrl Pts',(-4.27613527000006,5.2,-0.352025750000013));
#313940=CARTESIAN_POINT('Ctrl Pts',(-4.27613527000006,2.2,-0.352025750000013));
#313941=CARTESIAN_POINT('Ctrl Pts',(-4.27773499600006,12.2,-0.352812175000015));
#313942=CARTESIAN_POINT('Ctrl Pts',(-4.27773499600006,5.2,-0.352812175000015));
#313943=CARTESIAN_POINT('Ctrl Pts',(-4.27773499600006,2.2,-0.352812175000015));
#313944=CARTESIAN_POINT('Ctrl Pts',(-4.27933771900006,12.2,-0.353602331000014));
#313945=CARTESIAN_POINT('Ctrl Pts',(-4.27933771900006,5.2,-0.353602331000014));
#313946=CARTESIAN_POINT('Ctrl Pts',(-4.27933771900006,2.2,-0.353602331000014));
#313947=CARTESIAN_POINT('Ctrl Pts',(-4.28094342700006,12.2,-0.354396226000016));
#313948=CARTESIAN_POINT('Ctrl Pts',(-4.28094342700006,5.2,-0.354396226000016));
#313949=CARTESIAN_POINT('Ctrl Pts',(-4.28094342700006,2.2,-0.354396226000016));
#313950=CARTESIAN_POINT('Ctrl Pts',(-4.28255211000006,12.2,-0.355193862000016));
#313951=CARTESIAN_POINT('Ctrl Pts',(-4.28255211000006,5.2,-0.355193862000016));
#313952=CARTESIAN_POINT('Ctrl Pts',(-4.28255211000006,2.2,-0.355193862000016));
#313953=CARTESIAN_POINT('Ctrl Pts',(-4.28416375600006,12.2,-0.355995244000016));
#313954=CARTESIAN_POINT('Ctrl Pts',(-4.28416375600006,5.2,-0.355995244000016));
#313955=CARTESIAN_POINT('Ctrl Pts',(-4.28416375600006,2.2,-0.355995244000016));
#313956=CARTESIAN_POINT('Ctrl Pts',(-4.28577835400006,12.2,-0.356800375000015));
#313957=CARTESIAN_POINT('Ctrl Pts',(-4.28577835400006,5.2,-0.356800375000015));
#313958=CARTESIAN_POINT('Ctrl Pts',(-4.28577835400006,2.2,-0.356800375000015));
#313959=CARTESIAN_POINT('Ctrl Pts',(-4.28739589500006,12.2,-0.357609262000014));
#313960=CARTESIAN_POINT('Ctrl Pts',(-4.28739589500006,5.2,-0.357609262000014));
#313961=CARTESIAN_POINT('Ctrl Pts',(-4.28739589500006,2.2,-0.357609262000014));
#313962=CARTESIAN_POINT('Ctrl Pts',(-4.28901636600005,12.2,-0.358421908000013));
#313963=CARTESIAN_POINT('Ctrl Pts',(-4.28901636600005,5.2,-0.358421908000013));
#313964=CARTESIAN_POINT('Ctrl Pts',(-4.28901636600005,2.2,-0.358421908000013));
#313965=CARTESIAN_POINT('Ctrl Pts',(-4.29063975800006,12.2,-0.359238318000017));
#313966=CARTESIAN_POINT('Ctrl Pts',(-4.29063975800006,5.2,-0.359238318000017));
#313967=CARTESIAN_POINT('Ctrl Pts',(-4.29063975800006,2.2,-0.359238318000017));
#313968=CARTESIAN_POINT('Ctrl Pts',(-4.29226605800006,12.2,-0.360058496000013));
#313969=CARTESIAN_POINT('Ctrl Pts',(-4.29226605800006,5.2,-0.360058496000013));
#313970=CARTESIAN_POINT('Ctrl Pts',(-4.29226605800006,2.2,-0.360058496000013));
#313971=CARTESIAN_POINT('Ctrl Pts',(-4.29389525600006,12.2,-0.360882447000015));
#313972=CARTESIAN_POINT('Ctrl Pts',(-4.29389525600006,5.2,-0.360882447000015));
#313973=CARTESIAN_POINT('Ctrl Pts',(-4.29389525600006,2.2,-0.360882447000015));
#313974=CARTESIAN_POINT('Ctrl Pts',(-4.29552734300006,12.2,-0.361710175000014));
#313975=CARTESIAN_POINT('Ctrl Pts',(-4.29552734300006,5.2,-0.361710175000014));
#313976=CARTESIAN_POINT('Ctrl Pts',(-4.29552734300006,2.2,-0.361710175000014));
#313977=CARTESIAN_POINT('Ctrl Pts',(-4.29716230600006,12.2,-0.362541683000015));
#313978=CARTESIAN_POINT('Ctrl Pts',(-4.29716230600006,5.2,-0.362541683000015));
#313979=CARTESIAN_POINT('Ctrl Pts',(-4.29716230600006,2.2,-0.362541683000015));
#313980=CARTESIAN_POINT('Ctrl Pts',(-4.29880013500005,12.2,-0.363376978000014));
#313981=CARTESIAN_POINT('Ctrl Pts',(-4.29880013500005,5.2,-0.363376978000014));
#313982=CARTESIAN_POINT('Ctrl Pts',(-4.29880013500005,2.2,-0.363376978000014));
#313983=CARTESIAN_POINT('Ctrl Pts',(-4.30044081900006,12.2,-0.364216062000011));
#313984=CARTESIAN_POINT('Ctrl Pts',(-4.30044081900006,5.2,-0.364216062000011));
#313985=CARTESIAN_POINT('Ctrl Pts',(-4.30044081900006,2.2,-0.364216062000011));
#313986=CARTESIAN_POINT('Ctrl Pts',(-4.30208434600006,12.2,-0.365058939000011));
#313987=CARTESIAN_POINT('Ctrl Pts',(-4.30208434600006,5.2,-0.365058939000011));
#313988=CARTESIAN_POINT('Ctrl Pts',(-4.30208434600006,2.2,-0.365058939000011));
#313989=CARTESIAN_POINT('Ctrl Pts',(-4.30373070900006,12.2,-0.365905616000015));
#313990=CARTESIAN_POINT('Ctrl Pts',(-4.30373070900006,5.2,-0.365905616000015));
#313991=CARTESIAN_POINT('Ctrl Pts',(-4.30373070900006,2.2,-0.365905616000015));
#313992=CARTESIAN_POINT('Ctrl Pts',(-4.30537989300006,12.2,-0.366756094000014));
#313993=CARTESIAN_POINT('Ctrl Pts',(-4.30537989300006,5.2,-0.366756094000014));
#313994=CARTESIAN_POINT('Ctrl Pts',(-4.30537989300006,2.2,-0.366756094000014));
#313995=CARTESIAN_POINT('Ctrl Pts',(-4.30703189000006,12.2,-0.367610380000016));
#313996=CARTESIAN_POINT('Ctrl Pts',(-4.30703189000006,5.2,-0.367610380000016));
#313997=CARTESIAN_POINT('Ctrl Pts',(-4.30703189000006,2.2,-0.367610380000016));
#313998=CARTESIAN_POINT('Ctrl Pts',(-4.30868668700006,12.2,-0.368468477000015));
#313999=CARTESIAN_POINT('Ctrl Pts',(-4.30868668700006,5.2,-0.368468477000015));
#314000=CARTESIAN_POINT('Ctrl Pts',(-4.30868668700006,2.2,-0.368468477000015));
#314001=CARTESIAN_POINT('Ctrl Pts',(-4.31034427600006,12.2,-0.369330388000013));
#314002=CARTESIAN_POINT('Ctrl Pts',(-4.31034427600006,5.2,-0.369330388000013));
#314003=CARTESIAN_POINT('Ctrl Pts',(-4.31034427600006,2.2,-0.369330388000013));
#314004=CARTESIAN_POINT('Ctrl Pts',(-4.31200464500006,12.2,-0.370196119000017));
#314005=CARTESIAN_POINT('Ctrl Pts',(-4.31200464500006,5.2,-0.370196119000017));
#314006=CARTESIAN_POINT('Ctrl Pts',(-4.31200464500006,2.2,-0.370196119000017));
#314007=CARTESIAN_POINT('Ctrl Pts',(-4.31366778300006,12.2,-0.371065672000017));
#314008=CARTESIAN_POINT('Ctrl Pts',(-4.31366778300006,5.2,-0.371065672000017));
#314009=CARTESIAN_POINT('Ctrl Pts',(-4.31366778300006,2.2,-0.371065672000017));
#314010=CARTESIAN_POINT('Ctrl Pts',(-4.31533367800006,12.2,-0.371939053000014));
#314011=CARTESIAN_POINT('Ctrl Pts',(-4.31533367800006,5.2,-0.371939053000014));
#314012=CARTESIAN_POINT('Ctrl Pts',(-4.31533367800006,2.2,-0.371939053000014));
#314013=CARTESIAN_POINT('Ctrl Pts',(-4.31700232300006,12.2,-0.372816266000013));
#314014=CARTESIAN_POINT('Ctrl Pts',(-4.31700232300006,5.2,-0.372816266000013));
#314015=CARTESIAN_POINT('Ctrl Pts',(-4.31700232300006,2.2,-0.372816266000013));
#314016=CARTESIAN_POINT('Ctrl Pts',(-4.31867370400006,12.2,-0.373697313000014));
#314017=CARTESIAN_POINT('Ctrl Pts',(-4.31867370400006,5.2,-0.373697313000014));
#314018=CARTESIAN_POINT('Ctrl Pts',(-4.31867370400006,2.2,-0.373697313000014));
#314019=CARTESIAN_POINT('Ctrl Pts',(-4.32034781300006,12.2,-0.374582201000013));
#314020=CARTESIAN_POINT('Ctrl Pts',(-4.32034781300006,5.2,-0.374582201000013));
#314021=CARTESIAN_POINT('Ctrl Pts',(-4.32034781300006,2.2,-0.374582201000013));
#314022=CARTESIAN_POINT('Ctrl Pts',(-4.32202463700006,12.2,-0.375470931000015));
#314023=CARTESIAN_POINT('Ctrl Pts',(-4.32202463700006,5.2,-0.375470931000015));
#314024=CARTESIAN_POINT('Ctrl Pts',(-4.32202463700006,2.2,-0.375470931000015));
#314025=CARTESIAN_POINT('Ctrl Pts',(-4.32370416700006,12.2,-0.376363509000015));
#314026=CARTESIAN_POINT('Ctrl Pts',(-4.32370416700006,5.2,-0.376363509000015));
#314027=CARTESIAN_POINT('Ctrl Pts',(-4.32370416700006,2.2,-0.376363509000015));
#314028=CARTESIAN_POINT('Ctrl Pts',(-4.32538639100006,12.2,-0.377259939000014));
#314029=CARTESIAN_POINT('Ctrl Pts',(-4.32538639100006,5.2,-0.377259939000014));
#314030=CARTESIAN_POINT('Ctrl Pts',(-4.32538639100006,2.2,-0.377259939000014));
#314031=CARTESIAN_POINT('Ctrl Pts',(-4.32707130000006,12.2,-0.378160224000013));
#314032=CARTESIAN_POINT('Ctrl Pts',(-4.32707130000006,5.2,-0.378160224000013));
#314033=CARTESIAN_POINT('Ctrl Pts',(-4.32707130000006,2.2,-0.378160224000013));
#314034=CARTESIAN_POINT('Ctrl Pts',(-4.32875888300006,12.2,-0.379064368000015));
#314035=CARTESIAN_POINT('Ctrl Pts',(-4.32875888300006,5.2,-0.379064368000015));
#314036=CARTESIAN_POINT('Ctrl Pts',(-4.32875888300006,2.2,-0.379064368000015));
#314037=CARTESIAN_POINT('Ctrl Pts',(-4.33044912900006,12.2,-0.379972375000013));
#314038=CARTESIAN_POINT('Ctrl Pts',(-4.33044912900006,5.2,-0.379972375000013));
#314039=CARTESIAN_POINT('Ctrl Pts',(-4.33044912900006,2.2,-0.379972375000013));
#314040=CARTESIAN_POINT('Ctrl Pts',(-4.33214202700006,12.2,-0.380884249000015));
#314041=CARTESIAN_POINT('Ctrl Pts',(-4.33214202700006,5.2,-0.380884249000015));
#314042=CARTESIAN_POINT('Ctrl Pts',(-4.33214202700006,2.2,-0.380884249000015));
#314043=CARTESIAN_POINT('Ctrl Pts',(-4.33383756700006,12.2,-0.381799994000014));
#314044=CARTESIAN_POINT('Ctrl Pts',(-4.33383756700006,5.2,-0.381799994000014));
#314045=CARTESIAN_POINT('Ctrl Pts',(-4.33383756700006,2.2,-0.381799994000014));
#314046=CARTESIAN_POINT('Ctrl Pts',(-4.33553573900006,12.2,-0.382719614000013));
#314047=CARTESIAN_POINT('Ctrl Pts',(-4.33553573900006,5.2,-0.382719614000013));
#314048=CARTESIAN_POINT('Ctrl Pts',(-4.33553573900006,2.2,-0.382719614000013));
#314049=CARTESIAN_POINT('Ctrl Pts',(-4.33723653100006,12.2,-0.383643113000014));
#314050=CARTESIAN_POINT('Ctrl Pts',(-4.33723653100006,5.2,-0.383643113000014));
#314051=CARTESIAN_POINT('Ctrl Pts',(-4.33723653100006,2.2,-0.383643113000014));
#314052=CARTESIAN_POINT('Ctrl Pts',(-4.33893993400006,12.2,-0.384570493000016));
#314053=CARTESIAN_POINT('Ctrl Pts',(-4.33893993400006,5.2,-0.384570493000016));
#314054=CARTESIAN_POINT('Ctrl Pts',(-4.33893993400006,2.2,-0.384570493000016));
#314055=CARTESIAN_POINT('Ctrl Pts',(-4.34064593700006,12.2,-0.385501760000011));
#314056=CARTESIAN_POINT('Ctrl Pts',(-4.34064593700006,5.2,-0.385501760000011));
#314057=CARTESIAN_POINT('Ctrl Pts',(-4.34064593700006,2.2,-0.385501760000011));
#314058=CARTESIAN_POINT('Ctrl Pts',(-4.34235453000006,12.2,-0.386436917000013));
#314059=CARTESIAN_POINT('Ctrl Pts',(-4.34235453000006,5.2,-0.386436917000013));
#314060=CARTESIAN_POINT('Ctrl Pts',(-4.34235453000006,2.2,-0.386436917000013));
#314061=CARTESIAN_POINT('Ctrl Pts',(-4.34406570100006,12.2,-0.387375967000012));
#314062=CARTESIAN_POINT('Ctrl Pts',(-4.34406570100006,5.2,-0.387375967000012));
#314063=CARTESIAN_POINT('Ctrl Pts',(-4.34406570100006,2.2,-0.387375967000012));
#314064=CARTESIAN_POINT('Ctrl Pts',(-4.34577944200006,12.2,-0.388318914000014));
#314065=CARTESIAN_POINT('Ctrl Pts',(-4.34577944200006,5.2,-0.388318914000014));
#314066=CARTESIAN_POINT('Ctrl Pts',(-4.34577944200006,2.2,-0.388318914000014));
#314067=CARTESIAN_POINT('Ctrl Pts',(-4.34749574100006,12.2,-0.389265762000015));
#314068=CARTESIAN_POINT('Ctrl Pts',(-4.34749574100006,5.2,-0.389265762000015));
#314069=CARTESIAN_POINT('Ctrl Pts',(-4.34749574100006,2.2,-0.389265762000015));
#314070=CARTESIAN_POINT('Ctrl Pts',(-4.34921458700006,12.2,-0.390216515000015));
#314071=CARTESIAN_POINT('Ctrl Pts',(-4.34921458700006,5.2,-0.390216515000015));
#314072=CARTESIAN_POINT('Ctrl Pts',(-4.34921458700006,2.2,-0.390216515000015));
#314073=CARTESIAN_POINT('Ctrl Pts',(-4.35093597100006,12.2,-0.391171176000018));
#314074=CARTESIAN_POINT('Ctrl Pts',(-4.35093597100006,5.2,-0.391171176000018));
#314075=CARTESIAN_POINT('Ctrl Pts',(-4.35093597100006,2.2,-0.391171176000018));
#314076=CARTESIAN_POINT('Ctrl Pts',(-4.35265988100006,12.2,-0.392129749000016));
#314077=CARTESIAN_POINT('Ctrl Pts',(-4.35265988100006,5.2,-0.392129749000016));
#314078=CARTESIAN_POINT('Ctrl Pts',(-4.35265988100006,2.2,-0.392129749000016));
#314079=CARTESIAN_POINT('Ctrl Pts',(-4.35438630800006,12.2,-0.393092237000014));
#314080=CARTESIAN_POINT('Ctrl Pts',(-4.35438630800006,5.2,-0.393092237000014));
#314081=CARTESIAN_POINT('Ctrl Pts',(-4.35438630800006,2.2,-0.393092237000014));
#314082=CARTESIAN_POINT('Ctrl Pts',(-4.35611524200006,12.2,-0.394058645000013));
#314083=CARTESIAN_POINT('Ctrl Pts',(-4.35611524200006,5.2,-0.394058645000013));
#314084=CARTESIAN_POINT('Ctrl Pts',(-4.35611524200006,2.2,-0.394058645000013));
#314085=CARTESIAN_POINT('Ctrl Pts',(-4.35784667100005,12.2,-0.395028976000016));
#314086=CARTESIAN_POINT('Ctrl Pts',(-4.35784667100005,5.2,-0.395028976000016));
#314087=CARTESIAN_POINT('Ctrl Pts',(-4.35784667100005,2.2,-0.395028976000016));
#314088=CARTESIAN_POINT('Ctrl Pts',(-4.35958058500006,12.2,-0.396003232000015));
#314089=CARTESIAN_POINT('Ctrl Pts',(-4.35958058500006,5.2,-0.396003232000015));
#314090=CARTESIAN_POINT('Ctrl Pts',(-4.35958058500006,2.2,-0.396003232000015));
#314091=CARTESIAN_POINT('Ctrl Pts',(-4.36131697400006,12.2,-0.396981418000015));
#314092=CARTESIAN_POINT('Ctrl Pts',(-4.36131697400006,5.2,-0.396981418000015));
#314093=CARTESIAN_POINT('Ctrl Pts',(-4.36131697400006,2.2,-0.396981418000015));
#314094=CARTESIAN_POINT('Ctrl Pts',(-4.36305582900006,12.2,-0.397963538000017));
#314095=CARTESIAN_POINT('Ctrl Pts',(-4.36305582900006,5.2,-0.397963538000017));
#314096=CARTESIAN_POINT('Ctrl Pts',(-4.36305582900006,2.2,-0.397963538000017));
#314097=CARTESIAN_POINT('Ctrl Pts',(-4.36479713800006,12.2,-0.398949594000015));
#314098=CARTESIAN_POINT('Ctrl Pts',(-4.36479713800006,5.2,-0.398949594000015));
#314099=CARTESIAN_POINT('Ctrl Pts',(-4.36479713800006,2.2,-0.398949594000015));
#314100=CARTESIAN_POINT('Ctrl Pts',(-4.36654089000006,12.2,-0.399939590000016));
#314101=CARTESIAN_POINT('Ctrl Pts',(-4.36654089000006,5.2,-0.399939590000016));
#314102=CARTESIAN_POINT('Ctrl Pts',(-4.36654089000006,2.2,-0.399939590000016));
#314103=CARTESIAN_POINT('Ctrl Pts',(-4.36828707800006,12.2,-0.400933530000014));
#314104=CARTESIAN_POINT('Ctrl Pts',(-4.36828707800006,5.2,-0.400933530000014));
#314105=CARTESIAN_POINT('Ctrl Pts',(-4.36828707800006,2.2,-0.400933530000014));
#314106=CARTESIAN_POINT('Ctrl Pts',(-4.37003568800006,12.2,-0.401931417000014));
#314107=CARTESIAN_POINT('Ctrl Pts',(-4.37003568800006,5.2,-0.401931417000014));
#314108=CARTESIAN_POINT('Ctrl Pts',(-4.37003568800006,2.2,-0.401931417000014));
#314109=CARTESIAN_POINT('Ctrl Pts',(-4.37178671200006,12.2,-0.402933255000013));
#314110=CARTESIAN_POINT('Ctrl Pts',(-4.37178671200006,5.2,-0.402933255000013));
#314111=CARTESIAN_POINT('Ctrl Pts',(-4.37178671200006,2.2,-0.402933255000013));
#314112=CARTESIAN_POINT('Ctrl Pts',(-4.37354013800006,12.2,-0.403939047000015));
#314113=CARTESIAN_POINT('Ctrl Pts',(-4.37354013800006,5.2,-0.403939047000015));
#314114=CARTESIAN_POINT('Ctrl Pts',(-4.37354013800006,2.2,-0.403939047000015));
#314115=CARTESIAN_POINT('Ctrl Pts',(-4.37529595700005,12.2,-0.404948796000015));
#314116=CARTESIAN_POINT('Ctrl Pts',(-4.37529595700005,5.2,-0.404948796000015));
#314117=CARTESIAN_POINT('Ctrl Pts',(-4.37529595700005,2.2,-0.404948796000015));
#314118=CARTESIAN_POINT('Ctrl Pts',(-4.37705415900006,12.2,-0.405962504000015));
#314119=CARTESIAN_POINT('Ctrl Pts',(-4.37705415900006,5.2,-0.405962504000015));
#314120=CARTESIAN_POINT('Ctrl Pts',(-4.37705415900006,2.2,-0.405962504000015));
#314121=CARTESIAN_POINT('Ctrl Pts',(-4.37881473400005,12.2,-0.406980178000014));
#314122=CARTESIAN_POINT('Ctrl Pts',(-4.37881473400005,5.2,-0.406980178000014));
#314123=CARTESIAN_POINT('Ctrl Pts',(-4.37881473400005,2.2,-0.406980178000014));
#314124=CARTESIAN_POINT('Ctrl Pts',(-4.38057767000006,12.2,-0.408001819000017));
#314125=CARTESIAN_POINT('Ctrl Pts',(-4.38057767000006,5.2,-0.408001819000017));
#314126=CARTESIAN_POINT('Ctrl Pts',(-4.38057767000006,2.2,-0.408001819000017));
#314127=CARTESIAN_POINT('Ctrl Pts',(-4.38234295900005,12.2,-0.409027430000015));
#314128=CARTESIAN_POINT('Ctrl Pts',(-4.38234295900005,5.2,-0.409027430000015));
#314129=CARTESIAN_POINT('Ctrl Pts',(-4.38234295900005,2.2,-0.409027430000015));
#314130=CARTESIAN_POINT('Ctrl Pts',(-4.38411058800006,12.2,-0.410057015000014));
#314131=CARTESIAN_POINT('Ctrl Pts',(-4.38411058800006,5.2,-0.410057015000014));
#314132=CARTESIAN_POINT('Ctrl Pts',(-4.38411058800006,2.2,-0.410057015000014));
#314133=CARTESIAN_POINT('Ctrl Pts',(-4.38588054900006,12.2,-0.411090577000017));
#314134=CARTESIAN_POINT('Ctrl Pts',(-4.38588054900006,5.2,-0.411090577000017));
#314135=CARTESIAN_POINT('Ctrl Pts',(-4.38588054900006,2.2,-0.411090577000017));
#314136=CARTESIAN_POINT('Ctrl Pts',(-4.38765283200006,12.2,-0.412128119000013));
#314137=CARTESIAN_POINT('Ctrl Pts',(-4.38765283200006,5.2,-0.412128119000013));
#314138=CARTESIAN_POINT('Ctrl Pts',(-4.38765283200006,2.2,-0.412128119000013));
#314139=CARTESIAN_POINT('Ctrl Pts',(-4.38942742600006,12.2,-0.413169645000018));
#314140=CARTESIAN_POINT('Ctrl Pts',(-4.38942742600006,5.2,-0.413169645000018));
#314141=CARTESIAN_POINT('Ctrl Pts',(-4.38942742600006,2.2,-0.413169645000018));
#314142=CARTESIAN_POINT('Ctrl Pts',(-4.39120432000006,12.2,-0.414215158000015));
#314143=CARTESIAN_POINT('Ctrl Pts',(-4.39120432000006,5.2,-0.414215158000015));
#314144=CARTESIAN_POINT('Ctrl Pts',(-4.39120432000006,2.2,-0.414215158000015));
#314145=CARTESIAN_POINT('Ctrl Pts',(-4.39298350700006,12.2,-0.415264660000014));
#314146=CARTESIAN_POINT('Ctrl Pts',(-4.39298350700006,5.2,-0.415264660000014));
#314147=CARTESIAN_POINT('Ctrl Pts',(-4.39298350700006,2.2,-0.415264660000014));
#314148=CARTESIAN_POINT('Ctrl Pts',(-4.39476497300006,12.2,-0.416318157000015));
#314149=CARTESIAN_POINT('Ctrl Pts',(-4.39476497300006,5.2,-0.416318157000015));
#314150=CARTESIAN_POINT('Ctrl Pts',(-4.39476497300006,2.2,-0.416318157000015));
#314151=CARTESIAN_POINT('Ctrl Pts',(-4.39654871000006,12.2,-0.417375648000018));
#314152=CARTESIAN_POINT('Ctrl Pts',(-4.39654871000006,5.2,-0.417375648000018));
#314153=CARTESIAN_POINT('Ctrl Pts',(-4.39654871000006,2.2,-0.417375648000018));
#314154=CARTESIAN_POINT('Ctrl Pts',(-4.39833470800005,12.2,-0.418437140000014));
#314155=CARTESIAN_POINT('Ctrl Pts',(-4.39833470800005,5.2,-0.418437140000014));
#314156=CARTESIAN_POINT('Ctrl Pts',(-4.39833470800005,2.2,-0.418437140000014));
#314157=CARTESIAN_POINT('Ctrl Pts',(-4.40012295600006,12.2,-0.419502633000013));
#314158=CARTESIAN_POINT('Ctrl Pts',(-4.40012295600006,5.2,-0.419502633000013));
#314159=CARTESIAN_POINT('Ctrl Pts',(-4.40012295600006,2.2,-0.419502633000013));
#314160=CARTESIAN_POINT('Ctrl Pts',(-4.40191344400006,12.2,-0.420572133000015));
#314161=CARTESIAN_POINT('Ctrl Pts',(-4.40191344400006,5.2,-0.420572133000015));
#314162=CARTESIAN_POINT('Ctrl Pts',(-4.40191344400006,2.2,-0.420572133000015));
#314163=CARTESIAN_POINT('Ctrl Pts',(-4.40370616300005,12.2,-0.421645641000015));
#314164=CARTESIAN_POINT('Ctrl Pts',(-4.40370616300005,5.2,-0.421645641000015));
#314165=CARTESIAN_POINT('Ctrl Pts',(-4.40370616300005,2.2,-0.421645641000015));
#314166=CARTESIAN_POINT('Ctrl Pts',(-4.40550110300006,12.2,-0.422723161000014));
#314167=CARTESIAN_POINT('Ctrl Pts',(-4.40550110300006,5.2,-0.422723161000014));
#314168=CARTESIAN_POINT('Ctrl Pts',(-4.40550110300006,2.2,-0.422723161000014));
#314169=CARTESIAN_POINT('Ctrl Pts',(-4.40729825200005,12.2,-0.423804695000012));
#314170=CARTESIAN_POINT('Ctrl Pts',(-4.40729825200005,5.2,-0.423804695000012));
#314171=CARTESIAN_POINT('Ctrl Pts',(-4.40729825200005,2.2,-0.423804695000012));
#314172=CARTESIAN_POINT('Ctrl Pts',(-4.40909760100006,12.2,-0.424890247000014));
#314173=CARTESIAN_POINT('Ctrl Pts',(-4.40909760100006,5.2,-0.424890247000014));
#314174=CARTESIAN_POINT('Ctrl Pts',(-4.40909760100006,2.2,-0.424890247000014));
#314175=CARTESIAN_POINT('Ctrl Pts',(-4.41089914100006,12.2,-0.425979821000015));
#314176=CARTESIAN_POINT('Ctrl Pts',(-4.41089914100006,5.2,-0.425979821000015));
#314177=CARTESIAN_POINT('Ctrl Pts',(-4.41089914100006,2.2,-0.425979821000015));
#314178=CARTESIAN_POINT('Ctrl Pts',(-4.41270286100006,12.2,-0.427073417000017));
#314179=CARTESIAN_POINT('Ctrl Pts',(-4.41270286100006,5.2,-0.427073417000017));
#314180=CARTESIAN_POINT('Ctrl Pts',(-4.41270286100006,2.2,-0.427073417000017));
#314181=CARTESIAN_POINT('Ctrl Pts',(-4.41450875100006,12.2,-0.428171040000014));
#314182=CARTESIAN_POINT('Ctrl Pts',(-4.41450875100006,5.2,-0.428171040000014));
#314183=CARTESIAN_POINT('Ctrl Pts',(-4.41450875100006,2.2,-0.428171040000014));
#314184=CARTESIAN_POINT('Ctrl Pts',(-4.41631680000006,12.2,-0.429272693000016));
#314185=CARTESIAN_POINT('Ctrl Pts',(-4.41631680000006,5.2,-0.429272693000016));
#314186=CARTESIAN_POINT('Ctrl Pts',(-4.41631680000006,2.2,-0.429272693000016));
#314187=CARTESIAN_POINT('Ctrl Pts',(-4.41812700100006,12.2,-0.430378378000014));
#314188=CARTESIAN_POINT('Ctrl Pts',(-4.41812700100006,5.2,-0.430378378000014));
#314189=CARTESIAN_POINT('Ctrl Pts',(-4.41812700100006,2.2,-0.430378378000014));
#314190=CARTESIAN_POINT('Ctrl Pts',(-4.41993934100006,12.2,-0.431488099000017));
#314191=CARTESIAN_POINT('Ctrl Pts',(-4.41993934100006,5.2,-0.431488099000017));
#314192=CARTESIAN_POINT('Ctrl Pts',(-4.41993934100006,2.2,-0.431488099000017));
#314193=CARTESIAN_POINT('Ctrl Pts',(-4.42175381100006,12.2,-0.432601858000012));
#314194=CARTESIAN_POINT('Ctrl Pts',(-4.42175381100006,5.2,-0.432601858000012));
#314195=CARTESIAN_POINT('Ctrl Pts',(-4.42175381100006,2.2,-0.432601858000012));
#314196=CARTESIAN_POINT('Ctrl Pts',(-4.42357040200006,12.2,-0.433719658000014));
#314197=CARTESIAN_POINT('Ctrl Pts',(-4.42357040200006,5.2,-0.433719658000014));
#314198=CARTESIAN_POINT('Ctrl Pts',(-4.42357040200006,2.2,-0.433719658000014));
#314199=CARTESIAN_POINT('Ctrl Pts',(-4.42538910400006,12.2,-0.434841503000012));
#314200=CARTESIAN_POINT('Ctrl Pts',(-4.42538910400006,5.2,-0.434841503000012));
#314201=CARTESIAN_POINT('Ctrl Pts',(-4.42538910400006,2.2,-0.434841503000012));
#314202=CARTESIAN_POINT('Ctrl Pts',(-4.42720990500006,12.2,-0.435967394000016));
#314203=CARTESIAN_POINT('Ctrl Pts',(-4.42720990500006,5.2,-0.435967394000016));
#314204=CARTESIAN_POINT('Ctrl Pts',(-4.42720990500006,2.2,-0.435967394000016));
#314205=CARTESIAN_POINT('Ctrl Pts',(-4.42903279800006,12.2,-0.437097334000014));
#314206=CARTESIAN_POINT('Ctrl Pts',(-4.42903279800006,5.2,-0.437097334000014));
#314207=CARTESIAN_POINT('Ctrl Pts',(-4.42903279800006,2.2,-0.437097334000014));
#314208=CARTESIAN_POINT('Ctrl Pts',(-4.43085777000006,12.2,-0.438231328000014));
#314209=CARTESIAN_POINT('Ctrl Pts',(-4.43085777000006,5.2,-0.438231328000014));
#314210=CARTESIAN_POINT('Ctrl Pts',(-4.43085777000006,2.2,-0.438231328000014));
#314211=CARTESIAN_POINT('Ctrl Pts',(-4.43268481400006,12.2,-0.439369377000016));
#314212=CARTESIAN_POINT('Ctrl Pts',(-4.43268481400006,5.2,-0.439369377000016));
#314213=CARTESIAN_POINT('Ctrl Pts',(-4.43268481400006,2.2,-0.439369377000016));
#314214=CARTESIAN_POINT('Ctrl Pts',(-4.43451391800005,12.2,-0.440511483000012));
#314215=CARTESIAN_POINT('Ctrl Pts',(-4.43451391800005,5.2,-0.440511483000012));
#314216=CARTESIAN_POINT('Ctrl Pts',(-4.43451391800005,2.2,-0.440511483000012));
#314217=CARTESIAN_POINT('Ctrl Pts',(-4.43634507400006,12.2,-0.441657651000016));
#314218=CARTESIAN_POINT('Ctrl Pts',(-4.43634507400006,5.2,-0.441657651000016));
#314219=CARTESIAN_POINT('Ctrl Pts',(-4.43634507400006,2.2,-0.441657651000016));
#314220=CARTESIAN_POINT('Ctrl Pts',(-4.43817827000006,12.2,-0.442807882000014));
#314221=CARTESIAN_POINT('Ctrl Pts',(-4.43817827000006,5.2,-0.442807882000014));
#314222=CARTESIAN_POINT('Ctrl Pts',(-4.43817827000006,2.2,-0.442807882000014));
#314223=CARTESIAN_POINT('Ctrl Pts',(-4.44001349800006,12.2,-0.443962179000015));
#314224=CARTESIAN_POINT('Ctrl Pts',(-4.44001349800006,5.2,-0.443962179000015));
#314225=CARTESIAN_POINT('Ctrl Pts',(-4.44001349800006,2.2,-0.443962179000015));
#314226=CARTESIAN_POINT('Ctrl Pts',(-4.44185074700005,12.2,-0.445120545000015));
#314227=CARTESIAN_POINT('Ctrl Pts',(-4.44185074700005,5.2,-0.445120545000015));
#314228=CARTESIAN_POINT('Ctrl Pts',(-4.44185074700005,2.2,-0.445120545000015));
#314229=CARTESIAN_POINT('Ctrl Pts',(-4.44369000700005,12.2,-0.446282983000015));
#314230=CARTESIAN_POINT('Ctrl Pts',(-4.44369000700005,5.2,-0.446282983000015));
#314231=CARTESIAN_POINT('Ctrl Pts',(-4.44369000700005,2.2,-0.446282983000015));
#314232=CARTESIAN_POINT('Ctrl Pts',(-4.44553127000006,12.2,-0.447449495000014));
#314233=CARTESIAN_POINT('Ctrl Pts',(-4.44553127000006,5.2,-0.447449495000014));
#314234=CARTESIAN_POINT('Ctrl Pts',(-4.44553127000006,2.2,-0.447449495000014));
#314235=CARTESIAN_POINT('Ctrl Pts',(-4.44737452400005,12.2,-0.448620083000013));
#314236=CARTESIAN_POINT('Ctrl Pts',(-4.44737452400005,5.2,-0.448620083000013));
#314237=CARTESIAN_POINT('Ctrl Pts',(-4.44737452400005,2.2,-0.448620083000013));
#314238=CARTESIAN_POINT('Ctrl Pts',(-4.44921976000006,12.2,-0.449794752000017));
#314239=CARTESIAN_POINT('Ctrl Pts',(-4.44921976000006,5.2,-0.449794752000017));
#314240=CARTESIAN_POINT('Ctrl Pts',(-4.44921976000006,2.2,-0.449794752000017));
#314241=CARTESIAN_POINT('Ctrl Pts',(-4.45106696900006,12.2,-0.450973502000016));
#314242=CARTESIAN_POINT('Ctrl Pts',(-4.45106696900006,5.2,-0.450973502000016));
#314243=CARTESIAN_POINT('Ctrl Pts',(-4.45106696900006,2.2,-0.450973502000016));
#314244=CARTESIAN_POINT('Ctrl Pts',(-4.45291614100006,12.2,-0.452156337000016));
#314245=CARTESIAN_POINT('Ctrl Pts',(-4.45291614100006,5.2,-0.452156337000016));
#314246=CARTESIAN_POINT('Ctrl Pts',(-4.45291614100006,2.2,-0.452156337000016));
#314247=CARTESIAN_POINT('Ctrl Pts',(-4.45476726500006,12.2,-0.453343260000012));
#314248=CARTESIAN_POINT('Ctrl Pts',(-4.45476726500006,5.2,-0.453343260000012));
#314249=CARTESIAN_POINT('Ctrl Pts',(-4.45476726500006,2.2,-0.453343260000012));
#314250=CARTESIAN_POINT('Ctrl Pts',(-4.45662033300006,12.2,-0.454534272000018));
#314251=CARTESIAN_POINT('Ctrl Pts',(-4.45662033300006,5.2,-0.454534272000018));
#314252=CARTESIAN_POINT('Ctrl Pts',(-4.45662033300006,2.2,-0.454534272000018));
#314253=CARTESIAN_POINT('Ctrl Pts',(-4.45847533300006,12.2,-0.455729376000011));
#314254=CARTESIAN_POINT('Ctrl Pts',(-4.45847533300006,5.2,-0.455729376000011));
#314255=CARTESIAN_POINT('Ctrl Pts',(-4.45847533300006,2.2,-0.455729376000011));
#314256=CARTESIAN_POINT('Ctrl Pts',(-4.46033225800006,12.2,-0.456928576000015));
#314257=CARTESIAN_POINT('Ctrl Pts',(-4.46033225800006,5.2,-0.456928576000015));
#314258=CARTESIAN_POINT('Ctrl Pts',(-4.46033225800006,2.2,-0.456928576000015));
#314259=CARTESIAN_POINT('Ctrl Pts',(-4.46219109600006,12.2,-0.458131872000016));
#314260=CARTESIAN_POINT('Ctrl Pts',(-4.46219109600006,5.2,-0.458131872000016));
#314261=CARTESIAN_POINT('Ctrl Pts',(-4.46219109600006,2.2,-0.458131872000016));
#314262=CARTESIAN_POINT('Ctrl Pts',(-4.46405183800006,12.2,-0.459339270000014));
#314263=CARTESIAN_POINT('Ctrl Pts',(-4.46405183800006,5.2,-0.459339270000014));
#314264=CARTESIAN_POINT('Ctrl Pts',(-4.46405183800006,2.2,-0.459339270000014));
#314265=CARTESIAN_POINT('Ctrl Pts',(-4.46591447600006,12.2,-0.460550769000014));
#314266=CARTESIAN_POINT('Ctrl Pts',(-4.46591447600006,5.2,-0.460550769000014));
#314267=CARTESIAN_POINT('Ctrl Pts',(-4.46591447600006,2.2,-0.460550769000014));
#314268=CARTESIAN_POINT('Ctrl Pts',(-4.46777899700006,12.2,-0.461766372000016));
#314269=CARTESIAN_POINT('Ctrl Pts',(-4.46777899700006,5.2,-0.461766372000016));
#314270=CARTESIAN_POINT('Ctrl Pts',(-4.46777899700006,2.2,-0.461766372000016));
#314271=CARTESIAN_POINT('Ctrl Pts',(-4.46964539400006,12.2,-0.462986083000012));
#314272=CARTESIAN_POINT('Ctrl Pts',(-4.46964539400006,5.2,-0.462986083000012));
#314273=CARTESIAN_POINT('Ctrl Pts',(-4.46964539400006,2.2,-0.462986083000012));
#314274=CARTESIAN_POINT('Ctrl Pts',(-4.47151365700006,12.2,-0.464209904000015));
#314275=CARTESIAN_POINT('Ctrl Pts',(-4.47151365700006,5.2,-0.464209904000015));
#314276=CARTESIAN_POINT('Ctrl Pts',(-4.47151365700006,2.2,-0.464209904000015));
#314277=CARTESIAN_POINT('Ctrl Pts',(-4.47338377500006,12.2,-0.465437837000016));
#314278=CARTESIAN_POINT('Ctrl Pts',(-4.47338377500006,5.2,-0.465437837000016));
#314279=CARTESIAN_POINT('Ctrl Pts',(-4.47338377500006,2.2,-0.465437837000016));
#314280=CARTESIAN_POINT('Ctrl Pts',(-4.47525573900006,12.2,-0.466669885000015));
#314281=CARTESIAN_POINT('Ctrl Pts',(-4.47525573900006,5.2,-0.466669885000015));
#314282=CARTESIAN_POINT('Ctrl Pts',(-4.47525573900006,2.2,-0.466669885000015));
#314283=CARTESIAN_POINT('Ctrl Pts',(-4.47712954000006,12.2,-0.467906048000017));
#314284=CARTESIAN_POINT('Ctrl Pts',(-4.47712954000006,5.2,-0.467906048000017));
#314285=CARTESIAN_POINT('Ctrl Pts',(-4.47712954000006,2.2,-0.467906048000017));
#314286=CARTESIAN_POINT('Ctrl Pts',(-4.47900516900006,12.2,-0.469146332000014));
#314287=CARTESIAN_POINT('Ctrl Pts',(-4.47900516900006,5.2,-0.469146332000014));
#314288=CARTESIAN_POINT('Ctrl Pts',(-4.47900516900006,2.2,-0.469146332000014));
#314289=CARTESIAN_POINT('Ctrl Pts',(-4.48088261400006,12.2,-0.470390737000015));
#314290=CARTESIAN_POINT('Ctrl Pts',(-4.48088261400006,5.2,-0.470390737000015));
#314291=CARTESIAN_POINT('Ctrl Pts',(-4.48088261400006,2.2,-0.470390737000015));
#314292=CARTESIAN_POINT('Ctrl Pts',(-4.48276186600006,12.2,-0.471639264000014));
#314293=CARTESIAN_POINT('Ctrl Pts',(-4.48276186600006,5.2,-0.471639264000014));
#314294=CARTESIAN_POINT('Ctrl Pts',(-4.48276186600006,2.2,-0.471639264000014));
#314295=CARTESIAN_POINT('Ctrl Pts',(-4.48464291700006,12.2,-0.472891920000014));
#314296=CARTESIAN_POINT('Ctrl Pts',(-4.48464291700006,5.2,-0.472891920000014));
#314297=CARTESIAN_POINT('Ctrl Pts',(-4.48464291700006,2.2,-0.472891920000014));
#314298=CARTESIAN_POINT('Ctrl Pts',(-4.48652575600006,12.2,-0.474148702000012));
#314299=CARTESIAN_POINT('Ctrl Pts',(-4.48652575600006,5.2,-0.474148702000012));
#314300=CARTESIAN_POINT('Ctrl Pts',(-4.48652575600006,2.2,-0.474148702000012));
#314301=CARTESIAN_POINT('Ctrl Pts',(-4.48841037500006,12.2,-0.475409616000011));
#314302=CARTESIAN_POINT('Ctrl Pts',(-4.48841037500006,5.2,-0.475409616000011));
#314303=CARTESIAN_POINT('Ctrl Pts',(-4.48841037500006,2.2,-0.475409616000011));
#314304=CARTESIAN_POINT('Ctrl Pts',(-4.49029676200006,12.2,-0.476674663000014));
#314305=CARTESIAN_POINT('Ctrl Pts',(-4.49029676200006,5.2,-0.476674663000014));
#314306=CARTESIAN_POINT('Ctrl Pts',(-4.49029676200006,2.2,-0.476674663000014));
#314307=CARTESIAN_POINT('Ctrl Pts',(-4.49218491000006,12.2,-0.477943845000013));
#314308=CARTESIAN_POINT('Ctrl Pts',(-4.49218491000006,5.2,-0.477943845000013));
#314309=CARTESIAN_POINT('Ctrl Pts',(-4.49218491000006,2.2,-0.477943845000013));
#314310=CARTESIAN_POINT('Ctrl Pts',(-4.49407480700006,12.2,-0.479217165000012));
#314311=CARTESIAN_POINT('Ctrl Pts',(-4.49407480700006,5.2,-0.479217165000012));
#314312=CARTESIAN_POINT('Ctrl Pts',(-4.49407480700006,2.2,-0.479217165000012));
#314313=CARTESIAN_POINT('Ctrl Pts',(-4.49596644600006,12.2,-0.480494623000016));
#314314=CARTESIAN_POINT('Ctrl Pts',(-4.49596644600006,5.2,-0.480494623000016));
#314315=CARTESIAN_POINT('Ctrl Pts',(-4.49596644600006,2.2,-0.480494623000016));
#314316=CARTESIAN_POINT('Ctrl Pts',(-4.49785981500006,12.2,-0.481776225000012));
#314317=CARTESIAN_POINT('Ctrl Pts',(-4.49785981500006,5.2,-0.481776225000012));
#314318=CARTESIAN_POINT('Ctrl Pts',(-4.49785981500006,2.2,-0.481776225000012));
#314319=CARTESIAN_POINT('Ctrl Pts',(-4.49975490600006,12.2,-0.483061969000014));
#314320=CARTESIAN_POINT('Ctrl Pts',(-4.49975490600006,5.2,-0.483061969000014));
#314321=CARTESIAN_POINT('Ctrl Pts',(-4.49975490600006,2.2,-0.483061969000014));
#314322=CARTESIAN_POINT('Ctrl Pts',(-4.50165170900005,12.2,-0.484351860000016));
#314323=CARTESIAN_POINT('Ctrl Pts',(-4.50165170900005,5.2,-0.484351860000016));
#314324=CARTESIAN_POINT('Ctrl Pts',(-4.50165170900005,2.2,-0.484351860000016));
#314325=CARTESIAN_POINT('Ctrl Pts',(-4.50355021600005,12.2,-0.485645898000016));
#314326=CARTESIAN_POINT('Ctrl Pts',(-4.50355021600005,5.2,-0.485645898000016));
#314327=CARTESIAN_POINT('Ctrl Pts',(-4.50355021600005,2.2,-0.485645898000016));
#314328=CARTESIAN_POINT('Ctrl Pts',(-4.50545041500006,12.2,-0.486944088000012));
#314329=CARTESIAN_POINT('Ctrl Pts',(-4.50545041500006,5.2,-0.486944088000012));
#314330=CARTESIAN_POINT('Ctrl Pts',(-4.50545041500006,2.2,-0.486944088000012));
#314331=CARTESIAN_POINT('Ctrl Pts',(-4.50735229700006,12.2,-0.488246430000014));
#314332=CARTESIAN_POINT('Ctrl Pts',(-4.50735229700006,5.2,-0.488246430000014));
#314333=CARTESIAN_POINT('Ctrl Pts',(-4.50735229700006,2.2,-0.488246430000014));
#314334=CARTESIAN_POINT('Ctrl Pts',(-4.50925585500006,12.2,-0.489552926000014));
#314335=CARTESIAN_POINT('Ctrl Pts',(-4.50925585500006,5.2,-0.489552926000014));
#314336=CARTESIAN_POINT('Ctrl Pts',(-4.50925585500006,2.2,-0.489552926000014));
#314337=CARTESIAN_POINT('Ctrl Pts',(-4.51116107700006,12.2,-0.490863580000016));
#314338=CARTESIAN_POINT('Ctrl Pts',(-4.51116107700006,5.2,-0.490863580000016));
#314339=CARTESIAN_POINT('Ctrl Pts',(-4.51116107700006,2.2,-0.490863580000016));
#314340=CARTESIAN_POINT('Ctrl Pts',(-4.51306795400006,12.2,-0.492178392000016));
#314341=CARTESIAN_POINT('Ctrl Pts',(-4.51306795400006,5.2,-0.492178392000016));
#314342=CARTESIAN_POINT('Ctrl Pts',(-4.51306795400006,2.2,-0.492178392000016));
#314343=CARTESIAN_POINT('Ctrl Pts',(-4.51497647800006,12.2,-0.493497364000017));
#314344=CARTESIAN_POINT('Ctrl Pts',(-4.51497647800006,5.2,-0.493497364000017));
#314345=CARTESIAN_POINT('Ctrl Pts',(-4.51497647800006,2.2,-0.493497364000017));
#314346=CARTESIAN_POINT('Ctrl Pts',(-4.51688663800006,12.2,-0.494820500000017));
#314347=CARTESIAN_POINT('Ctrl Pts',(-4.51688663800006,5.2,-0.494820500000017));
#314348=CARTESIAN_POINT('Ctrl Pts',(-4.51688663800006,2.2,-0.494820500000017));
#314349=CARTESIAN_POINT('Ctrl Pts',(-4.51879842500006,12.2,-0.496147800000015));
#314350=CARTESIAN_POINT('Ctrl Pts',(-4.51879842500006,5.2,-0.496147800000015));
#314351=CARTESIAN_POINT('Ctrl Pts',(-4.51879842500006,2.2,-0.496147800000015));
#314352=CARTESIAN_POINT('Ctrl Pts',(-4.52071182900006,12.2,-0.497479267000016));
#314353=CARTESIAN_POINT('Ctrl Pts',(-4.52071182900006,5.2,-0.497479267000016));
#314354=CARTESIAN_POINT('Ctrl Pts',(-4.52071182900006,2.2,-0.497479267000016));
#314355=CARTESIAN_POINT('Ctrl Pts',(-4.52262684200006,12.2,-0.498814904000016));
#314356=CARTESIAN_POINT('Ctrl Pts',(-4.52262684200006,5.2,-0.498814904000016));
#314357=CARTESIAN_POINT('Ctrl Pts',(-4.52262684200006,2.2,-0.498814904000016));
#314358=CARTESIAN_POINT('Ctrl Pts',(-4.52454345500006,12.2,-0.500154710000014));
#314359=CARTESIAN_POINT('Ctrl Pts',(-4.52454345500006,5.2,-0.500154710000014));
#314360=CARTESIAN_POINT('Ctrl Pts',(-4.52454345500006,2.2,-0.500154710000014));
#314361=CARTESIAN_POINT('Ctrl Pts',(-4.52646165600005,12.2,-0.501498690000015));
#314362=CARTESIAN_POINT('Ctrl Pts',(-4.52646165600005,5.2,-0.501498690000015));
#314363=CARTESIAN_POINT('Ctrl Pts',(-4.52646165600005,2.2,-0.501498690000015));
#314364=CARTESIAN_POINT('Ctrl Pts',(-4.52838143800006,12.2,-0.502846844000011));
#314365=CARTESIAN_POINT('Ctrl Pts',(-4.52838143800006,5.2,-0.502846844000011));
#314366=CARTESIAN_POINT('Ctrl Pts',(-4.52838143800006,2.2,-0.502846844000011));
#314367=CARTESIAN_POINT('Ctrl Pts',(-4.53030279000005,12.2,-0.504199175000015));
#314368=CARTESIAN_POINT('Ctrl Pts',(-4.53030279000005,5.2,-0.504199175000015));
#314369=CARTESIAN_POINT('Ctrl Pts',(-4.53030279000005,2.2,-0.504199175000015));
#314370=CARTESIAN_POINT('Ctrl Pts',(-4.53222570400006,12.2,-0.505555685000014));
#314371=CARTESIAN_POINT('Ctrl Pts',(-4.53222570400006,5.2,-0.505555685000014));
#314372=CARTESIAN_POINT('Ctrl Pts',(-4.53222570400006,2.2,-0.505555685000014));
#314373=CARTESIAN_POINT('Ctrl Pts',(-4.53415017100006,12.2,-0.506916375000017));
#314374=CARTESIAN_POINT('Ctrl Pts',(-4.53415017100006,5.2,-0.506916375000017));
#314375=CARTESIAN_POINT('Ctrl Pts',(-4.53415017100006,2.2,-0.506916375000017));
#314376=CARTESIAN_POINT('Ctrl Pts',(-4.53607618000006,12.2,-0.508281247000015));
#314377=CARTESIAN_POINT('Ctrl Pts',(-4.53607618000006,5.2,-0.508281247000015));
#314378=CARTESIAN_POINT('Ctrl Pts',(-4.53607618000006,2.2,-0.508281247000015));
#314379=CARTESIAN_POINT('Ctrl Pts',(-4.53800372300006,12.2,-0.509650302000013));
#314380=CARTESIAN_POINT('Ctrl Pts',(-4.53800372300006,5.2,-0.509650302000013));
#314381=CARTESIAN_POINT('Ctrl Pts',(-4.53800372300006,2.2,-0.509650302000013));
#314382=CARTESIAN_POINT('Ctrl Pts',(-4.53993278900006,12.2,-0.511023545000011));
#314383=CARTESIAN_POINT('Ctrl Pts',(-4.53993278900006,5.2,-0.511023545000011));
#314384=CARTESIAN_POINT('Ctrl Pts',(-4.53993278900006,2.2,-0.511023545000011));
#314385=CARTESIAN_POINT('Ctrl Pts',(-4.54186337200006,12.2,-0.512400975000014));
#314386=CARTESIAN_POINT('Ctrl Pts',(-4.54186337200006,5.2,-0.512400975000014));
#314387=CARTESIAN_POINT('Ctrl Pts',(-4.54186337200006,2.2,-0.512400975000014));
#314388=CARTESIAN_POINT('Ctrl Pts',(-4.54379545900006,12.2,-0.513782595000016));
#314389=CARTESIAN_POINT('Ctrl Pts',(-4.54379545900006,5.2,-0.513782595000016));
#314390=CARTESIAN_POINT('Ctrl Pts',(-4.54379545900006,2.2,-0.513782595000016));
#314391=CARTESIAN_POINT('Ctrl Pts',(-4.54572904300006,12.2,-0.515168406000015));
#314392=CARTESIAN_POINT('Ctrl Pts',(-4.54572904300006,5.2,-0.515168406000015));
#314393=CARTESIAN_POINT('Ctrl Pts',(-4.54572904300006,2.2,-0.515168406000015));
#314394=CARTESIAN_POINT('Ctrl Pts',(-4.54766411400006,12.2,-0.516558410000014));
#314395=CARTESIAN_POINT('Ctrl Pts',(-4.54766411400006,5.2,-0.516558410000014));
#314396=CARTESIAN_POINT('Ctrl Pts',(-4.54766411400006,2.2,-0.516558410000014));
#314397=CARTESIAN_POINT('Ctrl Pts',(-4.54960066300006,12.2,-0.517952609000014));
#314398=CARTESIAN_POINT('Ctrl Pts',(-4.54960066300006,5.2,-0.517952609000014));
#314399=CARTESIAN_POINT('Ctrl Pts',(-4.54960066300006,2.2,-0.517952609000014));
#314400=CARTESIAN_POINT('Ctrl Pts',(-4.55153868000005,12.2,-0.519351005000015));
#314401=CARTESIAN_POINT('Ctrl Pts',(-4.55153868000005,5.2,-0.519351005000015));
#314402=CARTESIAN_POINT('Ctrl Pts',(-4.55153868000005,2.2,-0.519351005000015));
#314403=CARTESIAN_POINT('Ctrl Pts',(-4.55347815700006,12.2,-0.520753599000017));
#314404=CARTESIAN_POINT('Ctrl Pts',(-4.55347815700006,5.2,-0.520753599000017));
#314405=CARTESIAN_POINT('Ctrl Pts',(-4.55347815700006,2.2,-0.520753599000017));
#314406=CARTESIAN_POINT('Ctrl Pts',(-4.55541908500006,12.2,-0.522160394000015));
#314407=CARTESIAN_POINT('Ctrl Pts',(-4.55541908500006,5.2,-0.522160394000015));
#314408=CARTESIAN_POINT('Ctrl Pts',(-4.55541908500006,2.2,-0.522160394000015));
#314409=CARTESIAN_POINT('Ctrl Pts',(-4.55736145300006,12.2,-0.523571390000015));
#314410=CARTESIAN_POINT('Ctrl Pts',(-4.55736145300006,5.2,-0.523571390000015));
#314411=CARTESIAN_POINT('Ctrl Pts',(-4.55736145300006,2.2,-0.523571390000015));
#314412=CARTESIAN_POINT('Ctrl Pts',(-4.55930525300006,12.2,-0.524986591000012));
#314413=CARTESIAN_POINT('Ctrl Pts',(-4.55930525300006,5.2,-0.524986591000012));
#314414=CARTESIAN_POINT('Ctrl Pts',(-4.55930525300006,2.2,-0.524986591000012));
#314415=CARTESIAN_POINT('Ctrl Pts',(-4.56125047500006,12.2,-0.526405996000014));
#314416=CARTESIAN_POINT('Ctrl Pts',(-4.56125047500006,5.2,-0.526405996000014));
#314417=CARTESIAN_POINT('Ctrl Pts',(-4.56125047500006,2.2,-0.526405996000014));
#314418=CARTESIAN_POINT('Ctrl Pts',(-4.56319711000006,12.2,-0.527829609000015));
#314419=CARTESIAN_POINT('Ctrl Pts',(-4.56319711000006,5.2,-0.527829609000015));
#314420=CARTESIAN_POINT('Ctrl Pts',(-4.56319711000006,2.2,-0.527829609000015));
#314421=CARTESIAN_POINT('Ctrl Pts',(-4.56514515100006,12.2,-0.529257430000012));
#314422=CARTESIAN_POINT('Ctrl Pts',(-4.56514515100006,5.2,-0.529257430000012));
#314423=CARTESIAN_POINT('Ctrl Pts',(-4.56514515100006,2.2,-0.529257430000012));
#314424=CARTESIAN_POINT('Ctrl Pts',(-4.56709458600006,12.2,-0.530689461000016));
#314425=CARTESIAN_POINT('Ctrl Pts',(-4.56709458600006,5.2,-0.530689461000016));
#314426=CARTESIAN_POINT('Ctrl Pts',(-4.56709458600006,2.2,-0.530689461000016));
#314427=CARTESIAN_POINT('Ctrl Pts',(-4.56904540700006,12.2,-0.532125704000013));
#314428=CARTESIAN_POINT('Ctrl Pts',(-4.56904540700006,5.2,-0.532125704000013));
#314429=CARTESIAN_POINT('Ctrl Pts',(-4.56904540700006,2.2,-0.532125704000013));
#314430=CARTESIAN_POINT('Ctrl Pts',(-4.57099760400006,12.2,-0.533566161000016));
#314431=CARTESIAN_POINT('Ctrl Pts',(-4.57099760400006,5.2,-0.533566161000016));
#314432=CARTESIAN_POINT('Ctrl Pts',(-4.57099760400006,2.2,-0.533566161000016));
#314433=CARTESIAN_POINT('Ctrl Pts',(-4.57295117000006,12.2,-0.535010832000014));
#314434=CARTESIAN_POINT('Ctrl Pts',(-4.57295117000006,5.2,-0.535010832000014));
#314435=CARTESIAN_POINT('Ctrl Pts',(-4.57295117000006,2.2,-0.535010832000014));
#314436=CARTESIAN_POINT('Ctrl Pts',(-4.57490609300006,12.2,-0.536459721000018));
#314437=CARTESIAN_POINT('Ctrl Pts',(-4.57490609300006,5.2,-0.536459721000018));
#314438=CARTESIAN_POINT('Ctrl Pts',(-4.57490609300006,2.2,-0.536459721000018));
#314439=CARTESIAN_POINT('Ctrl Pts',(-4.57686236600006,12.2,-0.537912827000016));
#314440=CARTESIAN_POINT('Ctrl Pts',(-4.57686236600006,5.2,-0.537912827000016));
#314441=CARTESIAN_POINT('Ctrl Pts',(-4.57686236600006,2.2,-0.537912827000016));
#314442=CARTESIAN_POINT('Ctrl Pts',(-4.57881998000006,12.2,-0.539370154000016));
#314443=CARTESIAN_POINT('Ctrl Pts',(-4.57881998000006,5.2,-0.539370154000016));
#314444=CARTESIAN_POINT('Ctrl Pts',(-4.57881998000006,2.2,-0.539370154000016));
#314445=CARTESIAN_POINT('Ctrl Pts',(-4.58077892400006,12.2,-0.540831701000015));
#314446=CARTESIAN_POINT('Ctrl Pts',(-4.58077892400006,5.2,-0.540831701000015));
#314447=CARTESIAN_POINT('Ctrl Pts',(-4.58077892400006,2.2,-0.540831701000015));
#314448=CARTESIAN_POINT('Ctrl Pts',(-4.58273919000006,12.2,-0.542297472000013));
#314449=CARTESIAN_POINT('Ctrl Pts',(-4.58273919000006,5.2,-0.542297472000013));
#314450=CARTESIAN_POINT('Ctrl Pts',(-4.58273919000006,2.2,-0.542297472000013));
#314451=CARTESIAN_POINT('Ctrl Pts',(-4.58470077000006,12.2,-0.543767466000014));
#314452=CARTESIAN_POINT('Ctrl Pts',(-4.58470077000006,5.2,-0.543767466000014));
#314453=CARTESIAN_POINT('Ctrl Pts',(-4.58470077000006,2.2,-0.543767466000014));
#314454=CARTESIAN_POINT('Ctrl Pts',(-4.58666365300005,12.2,-0.545241687000013));
#314455=CARTESIAN_POINT('Ctrl Pts',(-4.58666365300005,5.2,-0.545241687000013));
#314456=CARTESIAN_POINT('Ctrl Pts',(-4.58666365300005,2.2,-0.545241687000013));
#314457=CARTESIAN_POINT('Ctrl Pts',(-4.58862783200006,12.2,-0.546720135000012));
#314458=CARTESIAN_POINT('Ctrl Pts',(-4.58862783200006,5.2,-0.546720135000012));
#314459=CARTESIAN_POINT('Ctrl Pts',(-4.58862783200006,2.2,-0.546720135000012));
#314460=CARTESIAN_POINT('Ctrl Pts',(-4.59059329600006,12.2,-0.548202811000014));
#314461=CARTESIAN_POINT('Ctrl Pts',(-4.59059329600006,5.2,-0.548202811000014));
#314462=CARTESIAN_POINT('Ctrl Pts',(-4.59059329600006,2.2,-0.548202811000014));
#314463=CARTESIAN_POINT('Ctrl Pts',(-4.59256003700006,12.2,-0.549689718000015));
#314464=CARTESIAN_POINT('Ctrl Pts',(-4.59256003700006,5.2,-0.549689718000015));
#314465=CARTESIAN_POINT('Ctrl Pts',(-4.59256003700006,2.2,-0.549689718000015));
#314466=CARTESIAN_POINT('Ctrl Pts',(-4.59452804600006,12.2,-0.551180856000015));
#314467=CARTESIAN_POINT('Ctrl Pts',(-4.59452804600006,5.2,-0.551180856000015));
#314468=CARTESIAN_POINT('Ctrl Pts',(-4.59452804600006,2.2,-0.551180856000015));
#314469=CARTESIAN_POINT('Ctrl Pts',(-4.59649731300006,12.2,-0.552676228000015));
#314470=CARTESIAN_POINT('Ctrl Pts',(-4.59649731300006,5.2,-0.552676228000015));
#314471=CARTESIAN_POINT('Ctrl Pts',(-4.59649731300006,2.2,-0.552676228000015));
#314472=CARTESIAN_POINT('Ctrl Pts',(-4.59846783000006,12.2,-0.554175834000015));
#314473=CARTESIAN_POINT('Ctrl Pts',(-4.59846783000006,5.2,-0.554175834000015));
#314474=CARTESIAN_POINT('Ctrl Pts',(-4.59846783000006,2.2,-0.554175834000015));
#314475=CARTESIAN_POINT('Ctrl Pts',(-4.60043958800005,12.2,-0.555679676000014));
#314476=CARTESIAN_POINT('Ctrl Pts',(-4.60043958800005,5.2,-0.555679676000014));
#314477=CARTESIAN_POINT('Ctrl Pts',(-4.60043958800005,2.2,-0.555679676000014));
#314478=CARTESIAN_POINT('Ctrl Pts',(-4.60241257700006,12.2,-0.557187755000013));
#314479=CARTESIAN_POINT('Ctrl Pts',(-4.60241257700006,5.2,-0.557187755000013));
#314480=CARTESIAN_POINT('Ctrl Pts',(-4.60241257700006,2.2,-0.557187755000013));
#314481=CARTESIAN_POINT('Ctrl Pts',(-4.60438678900006,12.2,-0.558700072000011));
#314482=CARTESIAN_POINT('Ctrl Pts',(-4.60438678900006,5.2,-0.558700072000011));
#314483=CARTESIAN_POINT('Ctrl Pts',(-4.60438678900006,2.2,-0.558700072000011));
#314484=CARTESIAN_POINT('Ctrl Pts',(-4.60636221500006,12.2,-0.560216630000014));
#314485=CARTESIAN_POINT('Ctrl Pts',(-4.60636221500006,5.2,-0.560216630000014));
#314486=CARTESIAN_POINT('Ctrl Pts',(-4.60636221500006,2.2,-0.560216630000014));
#314487=CARTESIAN_POINT('Ctrl Pts',(-4.60833884500006,12.2,-0.561737429000013));
#314488=CARTESIAN_POINT('Ctrl Pts',(-4.60833884500006,5.2,-0.561737429000013));
#314489=CARTESIAN_POINT('Ctrl Pts',(-4.60833884500006,2.2,-0.561737429000013));
#314490=CARTESIAN_POINT('Ctrl Pts',(-4.61031667200006,12.2,-0.563262470000012));
#314491=CARTESIAN_POINT('Ctrl Pts',(-4.61031667200006,5.2,-0.563262470000012));
#314492=CARTESIAN_POINT('Ctrl Pts',(-4.61031667200006,2.2,-0.563262470000012));
#314493=CARTESIAN_POINT('Ctrl Pts',(-4.61229568600006,12.2,-0.564791756000016));
#314494=CARTESIAN_POINT('Ctrl Pts',(-4.61229568600006,5.2,-0.564791756000016));
#314495=CARTESIAN_POINT('Ctrl Pts',(-4.61229568600006,2.2,-0.564791756000016));
#314496=CARTESIAN_POINT('Ctrl Pts',(-4.61427587700006,12.2,-0.566325286000016));
#314497=CARTESIAN_POINT('Ctrl Pts',(-4.61427587700006,5.2,-0.566325286000016));
#314498=CARTESIAN_POINT('Ctrl Pts',(-4.61427587700006,2.2,-0.566325286000016));
#314499=CARTESIAN_POINT('Ctrl Pts',(-4.61625723700006,12.2,-0.567863064000012));
#314500=CARTESIAN_POINT('Ctrl Pts',(-4.61625723700006,5.2,-0.567863064000012));
#314501=CARTESIAN_POINT('Ctrl Pts',(-4.61625723700006,2.2,-0.567863064000012));
#314502=CARTESIAN_POINT('Ctrl Pts',(-4.61823975700006,12.2,-0.569405089000017));
#314503=CARTESIAN_POINT('Ctrl Pts',(-4.61823975700006,5.2,-0.569405089000017));
#314504=CARTESIAN_POINT('Ctrl Pts',(-4.61823975700006,2.2,-0.569405089000017));
#314505=CARTESIAN_POINT('Ctrl Pts',(-4.62022343000006,12.2,-0.570951362000014));
#314506=CARTESIAN_POINT('Ctrl Pts',(-4.62022343000006,5.2,-0.570951362000014));
#314507=CARTESIAN_POINT('Ctrl Pts',(-4.62022343000006,2.2,-0.570951362000014));
#314508=CARTESIAN_POINT('Ctrl Pts',(-4.62220824300006,12.2,-0.572501887000012));
#314509=CARTESIAN_POINT('Ctrl Pts',(-4.62220824300006,5.2,-0.572501887000012));
#314510=CARTESIAN_POINT('Ctrl Pts',(-4.62220824300006,2.2,-0.572501887000012));
#314511=CARTESIAN_POINT('Ctrl Pts',(-4.62419419100006,12.2,-0.574056662000015));
#314512=CARTESIAN_POINT('Ctrl Pts',(-4.62419419100006,5.2,-0.574056662000015));
#314513=CARTESIAN_POINT('Ctrl Pts',(-4.62419419100006,2.2,-0.574056662000015));
#314514=CARTESIAN_POINT('Ctrl Pts',(-4.62618126300006,12.2,-0.575615691000015));
#314515=CARTESIAN_POINT('Ctrl Pts',(-4.62618126300006,5.2,-0.575615691000015));
#314516=CARTESIAN_POINT('Ctrl Pts',(-4.62618126300006,2.2,-0.575615691000015));
#314517=CARTESIAN_POINT('Ctrl Pts',(-4.62816945000006,12.2,-0.577178973000017));
#314518=CARTESIAN_POINT('Ctrl Pts',(-4.62816945000006,5.2,-0.577178973000017));
#314519=CARTESIAN_POINT('Ctrl Pts',(-4.62816945000006,2.2,-0.577178973000017));
#314520=CARTESIAN_POINT('Ctrl Pts',(-4.63015874400006,12.2,-0.578746510000014));
#314521=CARTESIAN_POINT('Ctrl Pts',(-4.63015874400006,5.2,-0.578746510000014));
#314522=CARTESIAN_POINT('Ctrl Pts',(-4.63015874400006,2.2,-0.578746510000014));
#314523=CARTESIAN_POINT('Ctrl Pts',(-4.63214913600006,12.2,-0.580318304000014));
#314524=CARTESIAN_POINT('Ctrl Pts',(-4.63214913600006,5.2,-0.580318304000014));
#314525=CARTESIAN_POINT('Ctrl Pts',(-4.63214913600006,2.2,-0.580318304000014));
#314526=CARTESIAN_POINT('Ctrl Pts',(-4.63414061700006,12.2,-0.581894355000014));
#314527=CARTESIAN_POINT('Ctrl Pts',(-4.63414061700006,5.2,-0.581894355000014));
#314528=CARTESIAN_POINT('Ctrl Pts',(-4.63414061700006,2.2,-0.581894355000014));
#314529=CARTESIAN_POINT('Ctrl Pts',(-4.63613317800006,12.2,-0.583474665000012));
#314530=CARTESIAN_POINT('Ctrl Pts',(-4.63613317800006,5.2,-0.583474665000012));
#314531=CARTESIAN_POINT('Ctrl Pts',(-4.63613317800006,2.2,-0.583474665000012));
#314532=CARTESIAN_POINT('Ctrl Pts',(-4.63812681200006,12.2,-0.585059233000016));
#314533=CARTESIAN_POINT('Ctrl Pts',(-4.63812681200006,5.2,-0.585059233000016));
#314534=CARTESIAN_POINT('Ctrl Pts',(-4.63812681200006,2.2,-0.585059233000016));
#314535=CARTESIAN_POINT('Ctrl Pts',(-4.64012150800006,12.2,-0.586648064000013));
#314536=CARTESIAN_POINT('Ctrl Pts',(-4.64012150800006,5.2,-0.586648064000013));
#314537=CARTESIAN_POINT('Ctrl Pts',(-4.64012150800006,2.2,-0.586648064000013));
#314538=CARTESIAN_POINT('Ctrl Pts',(-4.64211725700006,12.2,-0.588241155000016));
#314539=CARTESIAN_POINT('Ctrl Pts',(-4.64211725700006,5.2,-0.588241155000016));
#314540=CARTESIAN_POINT('Ctrl Pts',(-4.64211725700006,2.2,-0.588241155000016));
#314541=CARTESIAN_POINT('Ctrl Pts',(-4.64411405100006,12.2,-0.589838511000016));
#314542=CARTESIAN_POINT('Ctrl Pts',(-4.64411405100006,5.2,-0.589838511000016));
#314543=CARTESIAN_POINT('Ctrl Pts',(-4.64411405100006,2.2,-0.589838511000016));
#314544=CARTESIAN_POINT('Ctrl Pts',(-4.64611188200006,12.2,-0.591440130000014));
#314545=CARTESIAN_POINT('Ctrl Pts',(-4.64611188200006,5.2,-0.591440130000014));
#314546=CARTESIAN_POINT('Ctrl Pts',(-4.64611188200006,2.2,-0.591440130000014));
#314547=CARTESIAN_POINT('Ctrl Pts',(-4.64811073900006,12.2,-0.593046014000014));
#314548=CARTESIAN_POINT('Ctrl Pts',(-4.64811073900006,5.2,-0.593046014000014));
#314549=CARTESIAN_POINT('Ctrl Pts',(-4.64811073900006,2.2,-0.593046014000014));
#314550=CARTESIAN_POINT('Ctrl Pts',(-4.65011061600006,12.2,-0.594656164000016));
#314551=CARTESIAN_POINT('Ctrl Pts',(-4.65011061600006,5.2,-0.594656164000016));
#314552=CARTESIAN_POINT('Ctrl Pts',(-4.65011061600006,2.2,-0.594656164000016));
#314553=CARTESIAN_POINT('Ctrl Pts',(-4.65211150200005,12.2,-0.596270581000016));
#314554=CARTESIAN_POINT('Ctrl Pts',(-4.65211150200005,5.2,-0.596270581000016));
#314555=CARTESIAN_POINT('Ctrl Pts',(-4.65211150200005,2.2,-0.596270581000016));
#314556=CARTESIAN_POINT('Ctrl Pts',(-4.65411338900006,12.2,-0.597889268000014));
#314557=CARTESIAN_POINT('Ctrl Pts',(-4.65411338900006,5.2,-0.597889268000014));
#314558=CARTESIAN_POINT('Ctrl Pts',(-4.65411338900006,2.2,-0.597889268000014));
#314559=CARTESIAN_POINT('Ctrl Pts',(-4.65611626900006,12.2,-0.599512222000014));
#314560=CARTESIAN_POINT('Ctrl Pts',(-4.65611626900006,5.2,-0.599512222000014));
#314561=CARTESIAN_POINT('Ctrl Pts',(-4.65611626900006,2.2,-0.599512222000014));
#314562=CARTESIAN_POINT('Ctrl Pts',(-4.65812013300006,12.2,-0.601139448000012));
#314563=CARTESIAN_POINT('Ctrl Pts',(-4.65812013300006,5.2,-0.601139448000012));
#314564=CARTESIAN_POINT('Ctrl Pts',(-4.65812013300006,2.2,-0.601139448000012));
#314565=CARTESIAN_POINT('Ctrl Pts',(-4.66012497200006,12.2,-0.602770944000017));
#314566=CARTESIAN_POINT('Ctrl Pts',(-4.66012497200006,5.2,-0.602770944000017));
#314567=CARTESIAN_POINT('Ctrl Pts',(-4.66012497200006,2.2,-0.602770944000017));
#314568=CARTESIAN_POINT('Ctrl Pts',(-4.66213077800006,12.2,-0.604406713000016));
#314569=CARTESIAN_POINT('Ctrl Pts',(-4.66213077800006,5.2,-0.604406713000016));
#314570=CARTESIAN_POINT('Ctrl Pts',(-4.66213077800006,2.2,-0.604406713000016));
#314571=CARTESIAN_POINT('Ctrl Pts',(-4.66413754100006,12.2,-0.606046755000014));
#314572=CARTESIAN_POINT('Ctrl Pts',(-4.66413754100006,5.2,-0.606046755000014));
#314573=CARTESIAN_POINT('Ctrl Pts',(-4.66413754100006,2.2,-0.606046755000014));
#314574=CARTESIAN_POINT('Ctrl Pts',(-4.66614525400006,12.2,-0.607691072000014));
#314575=CARTESIAN_POINT('Ctrl Pts',(-4.66614525400006,5.2,-0.607691072000014));
#314576=CARTESIAN_POINT('Ctrl Pts',(-4.66614525400006,2.2,-0.607691072000014));
#314577=CARTESIAN_POINT('Ctrl Pts',(-4.66815390600006,12.2,-0.609339663000017));
#314578=CARTESIAN_POINT('Ctrl Pts',(-4.66815390600006,5.2,-0.609339663000017));
#314579=CARTESIAN_POINT('Ctrl Pts',(-4.66815390600006,2.2,-0.609339663000017));
#314580=CARTESIAN_POINT('Ctrl Pts',(-4.67016348800006,12.2,-0.610992530000014));
#314581=CARTESIAN_POINT('Ctrl Pts',(-4.67016348800006,5.2,-0.610992530000014));
#314582=CARTESIAN_POINT('Ctrl Pts',(-4.67016348800006,2.2,-0.610992530000014));
#314583=CARTESIAN_POINT('Ctrl Pts',(-4.67217399200006,12.2,-0.612649674000014));
#314584=CARTESIAN_POINT('Ctrl Pts',(-4.67217399200006,5.2,-0.612649674000014));
#314585=CARTESIAN_POINT('Ctrl Pts',(-4.67217399200006,2.2,-0.612649674000014));
#314586=CARTESIAN_POINT('Ctrl Pts',(-4.67418540900006,12.2,-0.614311096000013));
#314587=CARTESIAN_POINT('Ctrl Pts',(-4.67418540900006,5.2,-0.614311096000013));
#314588=CARTESIAN_POINT('Ctrl Pts',(-4.67418540900006,2.2,-0.614311096000013));
#314589=CARTESIAN_POINT('Ctrl Pts',(-4.67619773200005,12.2,-0.615976798000015));
#314590=CARTESIAN_POINT('Ctrl Pts',(-4.67619773200005,5.2,-0.615976798000015));
#314591=CARTESIAN_POINT('Ctrl Pts',(-4.67619773200005,2.2,-0.615976798000015));
#314592=CARTESIAN_POINT('Ctrl Pts',(-4.67821095300006,12.2,-0.617646778000012));
#314593=CARTESIAN_POINT('Ctrl Pts',(-4.67821095300006,5.2,-0.617646778000012));
#314594=CARTESIAN_POINT('Ctrl Pts',(-4.67821095300006,2.2,-0.617646778000012));
#314595=CARTESIAN_POINT('Ctrl Pts',(-4.68022506300006,12.2,-0.619321038000016));
#314596=CARTESIAN_POINT('Ctrl Pts',(-4.68022506300006,5.2,-0.619321038000016));
#314597=CARTESIAN_POINT('Ctrl Pts',(-4.68022506300006,2.2,-0.619321038000016));
#314598=CARTESIAN_POINT('Ctrl Pts',(-4.68224005500006,12.2,-0.620999580000015));
#314599=CARTESIAN_POINT('Ctrl Pts',(-4.68224005500006,5.2,-0.620999580000015));
#314600=CARTESIAN_POINT('Ctrl Pts',(-4.68224005500006,2.2,-0.620999580000015));
#314601=CARTESIAN_POINT('Ctrl Pts',(-4.68425592000006,12.2,-0.622682404000017));
#314602=CARTESIAN_POINT('Ctrl Pts',(-4.68425592000006,5.2,-0.622682404000017));
#314603=CARTESIAN_POINT('Ctrl Pts',(-4.68425592000006,2.2,-0.622682404000017));
#314604=CARTESIAN_POINT('Ctrl Pts',(-4.68627265000006,12.2,-0.624369510000014));
#314605=CARTESIAN_POINT('Ctrl Pts',(-4.68627265000006,5.2,-0.624369510000014));
#314606=CARTESIAN_POINT('Ctrl Pts',(-4.68627265000006,2.2,-0.624369510000014));
#314607=CARTESIAN_POINT('Ctrl Pts',(-4.68829023200006,12.2,-0.626060900000014));
#314608=CARTESIAN_POINT('Ctrl Pts',(-4.68829023200006,5.2,-0.626060900000014));
#314609=CARTESIAN_POINT('Ctrl Pts',(-4.68829023200006,2.2,-0.626060900000014));
#314610=CARTESIAN_POINT('Ctrl Pts',(-4.69030865600006,12.2,-0.627756574000014));
#314611=CARTESIAN_POINT('Ctrl Pts',(-4.69030865600006,5.2,-0.627756574000014));
#314612=CARTESIAN_POINT('Ctrl Pts',(-4.69030865600006,2.2,-0.627756574000014));
#314613=CARTESIAN_POINT('Ctrl Pts',(-4.69232791400006,12.2,-0.629456535000017));
#314614=CARTESIAN_POINT('Ctrl Pts',(-4.69232791400006,5.2,-0.629456535000017));
#314615=CARTESIAN_POINT('Ctrl Pts',(-4.69232791400006,2.2,-0.629456535000017));
#314616=CARTESIAN_POINT('Ctrl Pts',(-4.69434799200006,12.2,-0.631160781000015));
#314617=CARTESIAN_POINT('Ctrl Pts',(-4.69434799200006,5.2,-0.631160781000015));
#314618=CARTESIAN_POINT('Ctrl Pts',(-4.69434799200006,2.2,-0.631160781000015));
#314619=CARTESIAN_POINT('Ctrl Pts',(-4.69636888500006,12.2,-0.632869317000013));
#314620=CARTESIAN_POINT('Ctrl Pts',(-4.69636888500006,5.2,-0.632869317000013));
#314621=CARTESIAN_POINT('Ctrl Pts',(-4.69636888500006,2.2,-0.632869317000013));
#314622=CARTESIAN_POINT('Ctrl Pts',(-4.69839058500006,12.2,-0.634582138000015));
#314623=CARTESIAN_POINT('Ctrl Pts',(-4.69839058500006,5.2,-0.634582138000015));
#314624=CARTESIAN_POINT('Ctrl Pts',(-4.69839058500006,2.2,-0.634582138000015));
#314625=CARTESIAN_POINT('Ctrl Pts',(-4.70041308900006,12.2,-0.636299249000012));
#314626=CARTESIAN_POINT('Ctrl Pts',(-4.70041308900006,5.2,-0.636299249000012));
#314627=CARTESIAN_POINT('Ctrl Pts',(-4.70041308900006,2.2,-0.636299249000012));
#314628=CARTESIAN_POINT('Ctrl Pts',(-4.70243639600006,12.2,-0.638020648000013));
#314629=CARTESIAN_POINT('Ctrl Pts',(-4.70243639600006,5.2,-0.638020648000013));
#314630=CARTESIAN_POINT('Ctrl Pts',(-4.70243639600006,2.2,-0.638020648000013));
#314631=CARTESIAN_POINT('Ctrl Pts',(-4.70405568100006,12.2,-0.639401197000016));
#314632=CARTESIAN_POINT('Ctrl Pts',(-4.70405568100006,5.2,-0.639401197000016));
#314633=CARTESIAN_POINT('Ctrl Pts',(-4.70405568100006,2.2,-0.639401197000016));
#314634=CARTESIAN_POINT('Ctrl Pts',(-4.70527050400006,12.2,-0.640438538000012));
#314635=CARTESIAN_POINT('Ctrl Pts',(-4.70527050400006,5.2,-0.640438538000012));
#314636=CARTESIAN_POINT('Ctrl Pts',(-4.70527050400006,2.2,-0.640438538000012));
#314637=CARTESIAN_POINT('Ctrl Pts',(-4.70608054600006,12.2,-0.641130957000016));
#314638=CARTESIAN_POINT('Ctrl Pts',(-4.70608054600006,5.2,-0.641130957000016));
#314639=CARTESIAN_POINT('Ctrl Pts',(-4.70608054600006,2.2,-0.641130957000016));
#314640=CARTESIAN_POINT('Ctrl Pts',(-4.70648560700006,12.2,-0.641477381000013));
#314641=CARTESIAN_POINT('Ctrl Pts',(-4.70648560700006,5.2,-0.641477381000013));
#314642=CARTESIAN_POINT('Ctrl Pts',(-4.70648560700006,2.2,-0.641477381000013));
#314643=CARTESIAN_POINT('',(-4.70648560700006,2.7,-0.641477381000014));
#314644=CARTESIAN_POINT('',(-4.70648560700006,12.2,-0.641477381000013));
#314645=CARTESIAN_POINT('Ctrl Pts',(-3.98564433100006,2.7,-0.253971246000013));
#314646=CARTESIAN_POINT('Ctrl Pts',(-3.98580310824698,2.7,-0.25398196602194));
#314647=CARTESIAN_POINT('Ctrl Pts',(-3.98596177671456,2.7000000000014,-0.25399427786866));
#314648=CARTESIAN_POINT('Ctrl Pts',(-3.98645074029173,2.7000000000014,-0.254033260508237));
#314649=CARTESIAN_POINT('Ctrl Pts',(-3.98679793600037,2.70000000000153,
-0.254063570547946));
#314650=CARTESIAN_POINT('Ctrl Pts',(-3.98827065862374,2.70000000000153,
-0.254198213319473));
#314651=CARTESIAN_POINT('Ctrl Pts',(-3.98949352013573,2.70000000000098,
-0.254327938167664));
#314652=CARTESIAN_POINT('Ctrl Pts',(-3.99485063526251,2.70000000000098,
-0.2549415055447));
#314653=CARTESIAN_POINT('Ctrl Pts',(-3.9993227241105,2.7,-0.255583772964764));
#314654=CARTESIAN_POINT('Ctrl Pts',(-4.0189152228829,2.7,-0.258723793406327));
#314655=CARTESIAN_POINT('Ctrl Pts',(-4.03518303527141,2.7,-0.262265975327654));
#314656=CARTESIAN_POINT('Ctrl Pts',(-4.09406179711125,2.7,-0.277029537551965));
#314657=CARTESIAN_POINT('Ctrl Pts',(-4.14889894882159,2.7,-0.295015074741555));
#314658=CARTESIAN_POINT('Ctrl Pts',(-4.34245093015488,2.7,-0.378980348471285));
#314659=CARTESIAN_POINT('Ctrl Pts',(-4.51394467642948,2.7,-0.476808851243891));
#314660=CARTESIAN_POINT('Ctrl Pts',(-4.70648560700006,2.7,-0.641477381000013));
#314661=CARTESIAN_POINT('Origin',(-5.66300478732629E-14,15.2,-1.77635683940025E-14));
#314662=CARTESIAN_POINT('',(-4.64916443400006,2.7,-0.973534832000015));
#314663=CARTESIAN_POINT('',(-4.64916443400006,12.2,-0.973534832000014));
#314664=CARTESIAN_POINT('Origin',(-5.66300478732629E-14,2.7,-1.92943768261394E-14));
#314665=CARTESIAN_POINT('Ctrl Pts',(-4.64916443400006,12.2,-0.973534832000014));
#314666=CARTESIAN_POINT('Ctrl Pts',(-4.64916443400006,5.2,-0.973534832000014));
#314667=CARTESIAN_POINT('Ctrl Pts',(-4.64916443400006,2.2,-0.973534832000014));
#314668=CARTESIAN_POINT('Ctrl Pts',(-4.64866667400006,12.2,-0.973725406000017));
#314669=CARTESIAN_POINT('Ctrl Pts',(-4.64866667400006,5.2,-0.973725406000017));
#314670=CARTESIAN_POINT('Ctrl Pts',(-4.64866667400006,2.2,-0.973725406000017));
#314671=CARTESIAN_POINT('Ctrl Pts',(-4.64767137300006,12.2,-0.974106179000014));
#314672=CARTESIAN_POINT('Ctrl Pts',(-4.64767137300006,5.2,-0.974106179000014));
#314673=CARTESIAN_POINT('Ctrl Pts',(-4.64767137300006,2.2,-0.974106179000014));
#314674=CARTESIAN_POINT('Ctrl Pts',(-4.64617907800006,12.2,-0.974676206000016));
#314675=CARTESIAN_POINT('Ctrl Pts',(-4.64617907800006,5.2,-0.974676206000016));
#314676=CARTESIAN_POINT('Ctrl Pts',(-4.64617907800006,2.2,-0.974676206000016));
#314677=CARTESIAN_POINT('Ctrl Pts',(-4.64419066700006,12.2,-0.975433980000013));
#314678=CARTESIAN_POINT('Ctrl Pts',(-4.64419066700006,5.2,-0.975433980000013));
#314679=CARTESIAN_POINT('Ctrl Pts',(-4.64419066700006,2.2,-0.975433980000013));
#314680=CARTESIAN_POINT('Ctrl Pts',(-4.64170734400006,12.2,-0.976377425000017));
#314681=CARTESIAN_POINT('Ctrl Pts',(-4.64170734400006,5.2,-0.976377425000017));
#314682=CARTESIAN_POINT('Ctrl Pts',(-4.64170734400006,2.2,-0.976377425000017));
#314683=CARTESIAN_POINT('Ctrl Pts',(-4.63922621400005,12.2,-0.977317099000015));
#314684=CARTESIAN_POINT('Ctrl Pts',(-4.63922621400005,5.2,-0.977317099000015));
#314685=CARTESIAN_POINT('Ctrl Pts',(-4.63922621400005,2.2,-0.977317099000015));
#314686=CARTESIAN_POINT('Ctrl Pts',(-4.63674727900006,12.2,-0.978253002000016));
#314687=CARTESIAN_POINT('Ctrl Pts',(-4.63674727900006,5.2,-0.978253002000016));
#314688=CARTESIAN_POINT('Ctrl Pts',(-4.63674727900006,2.2,-0.978253002000016));
#314689=CARTESIAN_POINT('Ctrl Pts',(-4.63427054300006,12.2,-0.979185137000016));
#314690=CARTESIAN_POINT('Ctrl Pts',(-4.63427054300006,5.2,-0.979185137000016));
#314691=CARTESIAN_POINT('Ctrl Pts',(-4.63427054300006,2.2,-0.979185137000016));
#314692=CARTESIAN_POINT('Ctrl Pts',(-4.63179601100006,12.2,-0.980113505000015));
#314693=CARTESIAN_POINT('Ctrl Pts',(-4.63179601100006,5.2,-0.980113505000015));
#314694=CARTESIAN_POINT('Ctrl Pts',(-4.63179601100006,2.2,-0.980113505000015));
#314695=CARTESIAN_POINT('Ctrl Pts',(-4.62932369100006,12.2,-0.981038110000014));
#314696=CARTESIAN_POINT('Ctrl Pts',(-4.62932369100006,5.2,-0.981038110000014));
#314697=CARTESIAN_POINT('Ctrl Pts',(-4.62932369100006,2.2,-0.981038110000014));
#314698=CARTESIAN_POINT('Ctrl Pts',(-4.62685359100006,12.2,-0.981958957000018));
#314699=CARTESIAN_POINT('Ctrl Pts',(-4.62685359100006,5.2,-0.981958957000018));
#314700=CARTESIAN_POINT('Ctrl Pts',(-4.62685359100006,2.2,-0.981958957000018));
#314701=CARTESIAN_POINT('Ctrl Pts',(-4.62438572200006,12.2,-0.982876050000012));
#314702=CARTESIAN_POINT('Ctrl Pts',(-4.62438572200006,5.2,-0.982876050000012));
#314703=CARTESIAN_POINT('Ctrl Pts',(-4.62438572200006,2.2,-0.982876050000012));
#314704=CARTESIAN_POINT('Ctrl Pts',(-4.62192009200006,12.2,-0.983789392000016));
#314705=CARTESIAN_POINT('Ctrl Pts',(-4.62192009200006,5.2,-0.983789392000016));
#314706=CARTESIAN_POINT('Ctrl Pts',(-4.62192009200006,2.2,-0.983789392000016));
#314707=CARTESIAN_POINT('Ctrl Pts',(-4.61945671200006,12.2,-0.984698988000012));
#314708=CARTESIAN_POINT('Ctrl Pts',(-4.61945671200006,5.2,-0.984698988000012));
#314709=CARTESIAN_POINT('Ctrl Pts',(-4.61945671200006,2.2,-0.984698988000012));
#314710=CARTESIAN_POINT('Ctrl Pts',(-4.61699559000006,12.2,-0.985604844000014));
#314711=CARTESIAN_POINT('Ctrl Pts',(-4.61699559000006,5.2,-0.985604844000014));
#314712=CARTESIAN_POINT('Ctrl Pts',(-4.61699559000006,2.2,-0.985604844000014));
#314713=CARTESIAN_POINT('Ctrl Pts',(-4.61453673400006,12.2,-0.986506962000018));
#314714=CARTESIAN_POINT('Ctrl Pts',(-4.61453673400006,5.2,-0.986506962000018));
#314715=CARTESIAN_POINT('Ctrl Pts',(-4.61453673400006,2.2,-0.986506962000018));
#314716=CARTESIAN_POINT('Ctrl Pts',(-4.61208015200006,12.2,-0.987405346000014));
#314717=CARTESIAN_POINT('Ctrl Pts',(-4.61208015200006,5.2,-0.987405346000014));
#314718=CARTESIAN_POINT('Ctrl Pts',(-4.61208015200006,2.2,-0.987405346000014));
#314719=CARTESIAN_POINT('Ctrl Pts',(-4.60962585000006,12.2,-0.988299999000013));
#314720=CARTESIAN_POINT('Ctrl Pts',(-4.60962585000006,5.2,-0.988299999000013));
#314721=CARTESIAN_POINT('Ctrl Pts',(-4.60962585000006,2.2,-0.988299999000013));
#314722=CARTESIAN_POINT('Ctrl Pts',(-4.60717383500006,12.2,-0.989190924000014));
#314723=CARTESIAN_POINT('Ctrl Pts',(-4.60717383500006,5.2,-0.989190924000014));
#314724=CARTESIAN_POINT('Ctrl Pts',(-4.60717383500006,2.2,-0.989190924000014));
#314725=CARTESIAN_POINT('Ctrl Pts',(-4.60472411600006,12.2,-0.990078126000018));
#314726=CARTESIAN_POINT('Ctrl Pts',(-4.60472411600006,5.2,-0.990078126000018));
#314727=CARTESIAN_POINT('Ctrl Pts',(-4.60472411600006,2.2,-0.990078126000018));
#314728=CARTESIAN_POINT('Ctrl Pts',(-4.60227669800005,12.2,-0.990961607000016));
#314729=CARTESIAN_POINT('Ctrl Pts',(-4.60227669800005,5.2,-0.990961607000016));
#314730=CARTESIAN_POINT('Ctrl Pts',(-4.60227669800005,2.2,-0.990961607000016));
#314731=CARTESIAN_POINT('Ctrl Pts',(-4.59983159100006,12.2,-0.991841371000017));
#314732=CARTESIAN_POINT('Ctrl Pts',(-4.59983159100006,5.2,-0.991841371000017));
#314733=CARTESIAN_POINT('Ctrl Pts',(-4.59983159100006,2.2,-0.991841371000017));
#314734=CARTESIAN_POINT('Ctrl Pts',(-4.59738880200006,12.2,-0.992717423000014));
#314735=CARTESIAN_POINT('Ctrl Pts',(-4.59738880200006,5.2,-0.992717423000014));
#314736=CARTESIAN_POINT('Ctrl Pts',(-4.59738880200006,2.2,-0.992717423000014));
#314737=CARTESIAN_POINT('Ctrl Pts',(-4.59494834000005,12.2,-0.993589766000014));
#314738=CARTESIAN_POINT('Ctrl Pts',(-4.59494834000005,5.2,-0.993589766000014));
#314739=CARTESIAN_POINT('Ctrl Pts',(-4.59494834000005,2.2,-0.993589766000014));
#314740=CARTESIAN_POINT('Ctrl Pts',(-4.59251021200005,12.2,-0.994458404000014));
#314741=CARTESIAN_POINT('Ctrl Pts',(-4.59251021200005,5.2,-0.994458404000014));
#314742=CARTESIAN_POINT('Ctrl Pts',(-4.59251021200005,2.2,-0.994458404000014));
#314743=CARTESIAN_POINT('Ctrl Pts',(-4.59007442800006,12.2,-0.995323342000014));
#314744=CARTESIAN_POINT('Ctrl Pts',(-4.59007442800006,5.2,-0.995323342000014));
#314745=CARTESIAN_POINT('Ctrl Pts',(-4.59007442800006,2.2,-0.995323342000014));
#314746=CARTESIAN_POINT('Ctrl Pts',(-4.58764099500006,12.2,-0.996184581000015));
#314747=CARTESIAN_POINT('Ctrl Pts',(-4.58764099500006,5.2,-0.996184581000015));
#314748=CARTESIAN_POINT('Ctrl Pts',(-4.58764099500006,2.2,-0.996184581000015));
#314749=CARTESIAN_POINT('Ctrl Pts',(-4.58520992000006,12.2,-0.997042128000012));
#314750=CARTESIAN_POINT('Ctrl Pts',(-4.58520992000006,5.2,-0.997042128000012));
#314751=CARTESIAN_POINT('Ctrl Pts',(-4.58520992000006,2.2,-0.997042128000012));
#314752=CARTESIAN_POINT('Ctrl Pts',(-4.58278121200006,12.2,-0.997895986000015));
#314753=CARTESIAN_POINT('Ctrl Pts',(-4.58278121200006,5.2,-0.997895986000015));
#314754=CARTESIAN_POINT('Ctrl Pts',(-4.58278121200006,2.2,-0.997895986000015));
#314755=CARTESIAN_POINT('Ctrl Pts',(-4.58035487800006,12.2,-0.998746158000015));
#314756=CARTESIAN_POINT('Ctrl Pts',(-4.58035487800006,5.2,-0.998746158000015));
#314757=CARTESIAN_POINT('Ctrl Pts',(-4.58035487800006,2.2,-0.998746158000015));
#314758=CARTESIAN_POINT('Ctrl Pts',(-4.57793092600006,12.2,-0.999592648000016));
#314759=CARTESIAN_POINT('Ctrl Pts',(-4.57793092600006,5.2,-0.999592648000016));
#314760=CARTESIAN_POINT('Ctrl Pts',(-4.57793092600006,2.2,-0.999592648000016));
#314761=CARTESIAN_POINT('Ctrl Pts',(-4.57550936400006,12.2,-1.00043546100002));
#314762=CARTESIAN_POINT('Ctrl Pts',(-4.57550936400006,5.2,-1.00043546100002));
#314763=CARTESIAN_POINT('Ctrl Pts',(-4.57550936400006,2.2,-1.00043546100002));
#314764=CARTESIAN_POINT('Ctrl Pts',(-4.57309019900006,12.2,-1.00127459900001));
#314765=CARTESIAN_POINT('Ctrl Pts',(-4.57309019900006,5.2,-1.00127459900001));
#314766=CARTESIAN_POINT('Ctrl Pts',(-4.57309019900006,2.2,-1.00127459900001));
#314767=CARTESIAN_POINT('Ctrl Pts',(-4.57067344100006,12.2,-1.00211006800001));
#314768=CARTESIAN_POINT('Ctrl Pts',(-4.57067344100006,5.2,-1.00211006800001));
#314769=CARTESIAN_POINT('Ctrl Pts',(-4.57067344100006,2.2,-1.00211006800001));
#314770=CARTESIAN_POINT('Ctrl Pts',(-4.56825909500005,12.2,-1.00294187100001));
#314771=CARTESIAN_POINT('Ctrl Pts',(-4.56825909500005,5.2,-1.00294187100001));
#314772=CARTESIAN_POINT('Ctrl Pts',(-4.56825909500005,2.2,-1.00294187100001));
#314773=CARTESIAN_POINT('Ctrl Pts',(-4.56584717200006,12.2,-1.00377001100002));
#314774=CARTESIAN_POINT('Ctrl Pts',(-4.56584717200006,5.2,-1.00377001100002));
#314775=CARTESIAN_POINT('Ctrl Pts',(-4.56584717200006,2.2,-1.00377001100002));
#314776=CARTESIAN_POINT('Ctrl Pts',(-4.56343767800006,12.2,-1.00459449300002));
#314777=CARTESIAN_POINT('Ctrl Pts',(-4.56343767800006,5.2,-1.00459449300002));
#314778=CARTESIAN_POINT('Ctrl Pts',(-4.56343767800006,2.2,-1.00459449300002));
#314779=CARTESIAN_POINT('Ctrl Pts',(-4.56103062200006,12.2,-1.00541532300001));
#314780=CARTESIAN_POINT('Ctrl Pts',(-4.56103062200006,5.2,-1.00541532300001));
#314781=CARTESIAN_POINT('Ctrl Pts',(-4.56103062200006,2.2,-1.00541532300001));
#314782=CARTESIAN_POINT('Ctrl Pts',(-4.55862601000006,12.2,-1.00623250100002));
#314783=CARTESIAN_POINT('Ctrl Pts',(-4.55862601000006,5.2,-1.00623250100002));
#314784=CARTESIAN_POINT('Ctrl Pts',(-4.55862601000006,2.2,-1.00623250100002));
#314785=CARTESIAN_POINT('Ctrl Pts',(-4.55622385400006,12.2,-1.00704603400001));
#314786=CARTESIAN_POINT('Ctrl Pts',(-4.55622385400006,5.2,-1.00704603400001));
#314787=CARTESIAN_POINT('Ctrl Pts',(-4.55622385400006,2.2,-1.00704603400001));
#314788=CARTESIAN_POINT('Ctrl Pts',(-4.55382415700006,12.2,-1.00785592500001));
#314789=CARTESIAN_POINT('Ctrl Pts',(-4.55382415700006,5.2,-1.00785592500001));
#314790=CARTESIAN_POINT('Ctrl Pts',(-4.55382415700006,2.2,-1.00785592500001));
#314791=CARTESIAN_POINT('Ctrl Pts',(-4.55142693100006,12.2,-1.00866217800001));
#314792=CARTESIAN_POINT('Ctrl Pts',(-4.55142693100006,5.2,-1.00866217800001));
#314793=CARTESIAN_POINT('Ctrl Pts',(-4.55142693100006,2.2,-1.00866217800001));
#314794=CARTESIAN_POINT('Ctrl Pts',(-4.54903218100006,12.2,-1.00946479800001));
#314795=CARTESIAN_POINT('Ctrl Pts',(-4.54903218100006,5.2,-1.00946479800001));
#314796=CARTESIAN_POINT('Ctrl Pts',(-4.54903218100006,2.2,-1.00946479800001));
#314797=CARTESIAN_POINT('Ctrl Pts',(-4.54663991700006,12.2,-1.01026378800002));
#314798=CARTESIAN_POINT('Ctrl Pts',(-4.54663991700006,5.2,-1.01026378800002));
#314799=CARTESIAN_POINT('Ctrl Pts',(-4.54663991700006,2.2,-1.01026378800002));
#314800=CARTESIAN_POINT('Ctrl Pts',(-4.54425014500006,12.2,-1.01105915300002));
#314801=CARTESIAN_POINT('Ctrl Pts',(-4.54425014500006,5.2,-1.01105915300002));
#314802=CARTESIAN_POINT('Ctrl Pts',(-4.54425014500006,2.2,-1.01105915300002));
#314803=CARTESIAN_POINT('Ctrl Pts',(-4.54186287500006,12.2,-1.01185089600001));
#314804=CARTESIAN_POINT('Ctrl Pts',(-4.54186287500006,5.2,-1.01185089600001));
#314805=CARTESIAN_POINT('Ctrl Pts',(-4.54186287500006,2.2,-1.01185089600001));
#314806=CARTESIAN_POINT('Ctrl Pts',(-4.53947811500006,12.2,-1.01263902200001));
#314807=CARTESIAN_POINT('Ctrl Pts',(-4.53947811500006,5.2,-1.01263902200001));
#314808=CARTESIAN_POINT('Ctrl Pts',(-4.53947811500006,2.2,-1.01263902200001));
#314809=CARTESIAN_POINT('Ctrl Pts',(-4.53709587000006,12.2,-1.01342353600002));
#314810=CARTESIAN_POINT('Ctrl Pts',(-4.53709587000006,5.2,-1.01342353600002));
#314811=CARTESIAN_POINT('Ctrl Pts',(-4.53709587000006,2.2,-1.01342353600002));
#314812=CARTESIAN_POINT('Ctrl Pts',(-4.53471615200006,12.2,-1.01420444000001));
#314813=CARTESIAN_POINT('Ctrl Pts',(-4.53471615200006,5.2,-1.01420444000001));
#314814=CARTESIAN_POINT('Ctrl Pts',(-4.53471615200006,2.2,-1.01420444000001));
#314815=CARTESIAN_POINT('Ctrl Pts',(-4.53233896600006,12.2,-1.01498174000001));
#314816=CARTESIAN_POINT('Ctrl Pts',(-4.53233896600006,5.2,-1.01498174000001));
#314817=CARTESIAN_POINT('Ctrl Pts',(-4.53233896600006,2.2,-1.01498174000001));
#314818=CARTESIAN_POINT('Ctrl Pts',(-4.52996432000006,12.2,-1.01575543900001));
#314819=CARTESIAN_POINT('Ctrl Pts',(-4.52996432000006,5.2,-1.01575543900001));
#314820=CARTESIAN_POINT('Ctrl Pts',(-4.52996432000006,2.2,-1.01575543900001));
#314821=CARTESIAN_POINT('Ctrl Pts',(-4.52759222500006,12.2,-1.01652554200002));
#314822=CARTESIAN_POINT('Ctrl Pts',(-4.52759222500006,5.2,-1.01652554200002));
#314823=CARTESIAN_POINT('Ctrl Pts',(-4.52759222500006,2.2,-1.01652554200002));
#314824=CARTESIAN_POINT('Ctrl Pts',(-4.52522268600006,12.2,-1.01729205400002));
#314825=CARTESIAN_POINT('Ctrl Pts',(-4.52522268600006,5.2,-1.01729205400002));
#314826=CARTESIAN_POINT('Ctrl Pts',(-4.52522268600006,2.2,-1.01729205400002));
#314827=CARTESIAN_POINT('Ctrl Pts',(-4.52285571200005,12.2,-1.01805497700001));
#314828=CARTESIAN_POINT('Ctrl Pts',(-4.52285571200005,5.2,-1.01805497700001));
#314829=CARTESIAN_POINT('Ctrl Pts',(-4.52285571200005,2.2,-1.01805497700001));
#314830=CARTESIAN_POINT('Ctrl Pts',(-4.52049131100006,12.2,-1.01881431700001));
#314831=CARTESIAN_POINT('Ctrl Pts',(-4.52049131100006,5.2,-1.01881431700001));
#314832=CARTESIAN_POINT('Ctrl Pts',(-4.52049131100006,2.2,-1.01881431700001));
#314833=CARTESIAN_POINT('Ctrl Pts',(-4.51812949000006,12.2,-1.01957007800001));
#314834=CARTESIAN_POINT('Ctrl Pts',(-4.51812949000006,5.2,-1.01957007800001));
#314835=CARTESIAN_POINT('Ctrl Pts',(-4.51812949000006,2.2,-1.01957007800001));
#314836=CARTESIAN_POINT('Ctrl Pts',(-4.51577025900006,12.2,-1.02032226500001));
#314837=CARTESIAN_POINT('Ctrl Pts',(-4.51577025900006,5.2,-1.02032226500001));
#314838=CARTESIAN_POINT('Ctrl Pts',(-4.51577025900006,2.2,-1.02032226500001));
#314839=CARTESIAN_POINT('Ctrl Pts',(-4.51341362500006,12.2,-1.02107088000002));
#314840=CARTESIAN_POINT('Ctrl Pts',(-4.51341362500006,5.2,-1.02107088000002));
#314841=CARTESIAN_POINT('Ctrl Pts',(-4.51341362500006,2.2,-1.02107088000002));
#314842=CARTESIAN_POINT('Ctrl Pts',(-4.51105959700006,12.2,-1.02181593000001));
#314843=CARTESIAN_POINT('Ctrl Pts',(-4.51105959700006,5.2,-1.02181593000001));
#314844=CARTESIAN_POINT('Ctrl Pts',(-4.51105959700006,2.2,-1.02181593000001));
#314845=CARTESIAN_POINT('Ctrl Pts',(-4.50870818000006,12.2,-1.02255741900001));
#314846=CARTESIAN_POINT('Ctrl Pts',(-4.50870818000006,5.2,-1.02255741900001));
#314847=CARTESIAN_POINT('Ctrl Pts',(-4.50870818000006,2.2,-1.02255741900001));
#314848=CARTESIAN_POINT('Ctrl Pts',(-4.50635938600006,12.2,-1.02329534900001));
#314849=CARTESIAN_POINT('Ctrl Pts',(-4.50635938600006,5.2,-1.02329534900001));
#314850=CARTESIAN_POINT('Ctrl Pts',(-4.50635938600006,2.2,-1.02329534900001));
#314851=CARTESIAN_POINT('Ctrl Pts',(-4.50401322000006,12.2,-1.02402972800002));
#314852=CARTESIAN_POINT('Ctrl Pts',(-4.50401322000006,5.2,-1.02402972800002));
#314853=CARTESIAN_POINT('Ctrl Pts',(-4.50401322000006,2.2,-1.02402972800002));
#314854=CARTESIAN_POINT('Ctrl Pts',(-4.50166969200006,12.2,-1.02476055700001));
#314855=CARTESIAN_POINT('Ctrl Pts',(-4.50166969200006,5.2,-1.02476055700001));
#314856=CARTESIAN_POINT('Ctrl Pts',(-4.50166969200006,2.2,-1.02476055700001));
#314857=CARTESIAN_POINT('Ctrl Pts',(-4.49932880800006,12.2,-1.02548784200001));
#314858=CARTESIAN_POINT('Ctrl Pts',(-4.49932880800006,5.2,-1.02548784200001));
#314859=CARTESIAN_POINT('Ctrl Pts',(-4.49932880800006,2.2,-1.02548784200001));
#314860=CARTESIAN_POINT('Ctrl Pts',(-4.49699057800006,12.2,-1.02621158800002));
#314861=CARTESIAN_POINT('Ctrl Pts',(-4.49699057800006,5.2,-1.02621158800002));
#314862=CARTESIAN_POINT('Ctrl Pts',(-4.49699057800006,2.2,-1.02621158800002));
#314863=CARTESIAN_POINT('Ctrl Pts',(-4.49465500900006,12.2,-1.02693179800001));
#314864=CARTESIAN_POINT('Ctrl Pts',(-4.49465500900006,5.2,-1.02693179800001));
#314865=CARTESIAN_POINT('Ctrl Pts',(-4.49465500900006,2.2,-1.02693179800001));
#314866=CARTESIAN_POINT('Ctrl Pts',(-4.49232210900006,12.2,-1.02764847800001));
#314867=CARTESIAN_POINT('Ctrl Pts',(-4.49232210900006,5.2,-1.02764847800001));
#314868=CARTESIAN_POINT('Ctrl Pts',(-4.49232210900006,2.2,-1.02764847800001));
#314869=CARTESIAN_POINT('Ctrl Pts',(-4.48999188700006,12.2,-1.02836163100001));
#314870=CARTESIAN_POINT('Ctrl Pts',(-4.48999188700006,5.2,-1.02836163100001));
#314871=CARTESIAN_POINT('Ctrl Pts',(-4.48999188700006,2.2,-1.02836163100001));
#314872=CARTESIAN_POINT('Ctrl Pts',(-4.48766435100006,12.2,-1.02907126300002));
#314873=CARTESIAN_POINT('Ctrl Pts',(-4.48766435100006,5.2,-1.02907126300002));
#314874=CARTESIAN_POINT('Ctrl Pts',(-4.48766435100006,2.2,-1.02907126300002));
#314875=CARTESIAN_POINT('Ctrl Pts',(-4.48533950700006,12.2,-1.02977737800002));
#314876=CARTESIAN_POINT('Ctrl Pts',(-4.48533950700006,5.2,-1.02977737800002));
#314877=CARTESIAN_POINT('Ctrl Pts',(-4.48533950700006,2.2,-1.02977737800002));
#314878=CARTESIAN_POINT('Ctrl Pts',(-4.48301736600006,12.2,-1.03047998000001));
#314879=CARTESIAN_POINT('Ctrl Pts',(-4.48301736600006,5.2,-1.03047998000001));
#314880=CARTESIAN_POINT('Ctrl Pts',(-4.48301736600006,2.2,-1.03047998000001));
#314881=CARTESIAN_POINT('Ctrl Pts',(-4.48069793400006,12.2,-1.03117907400001));
#314882=CARTESIAN_POINT('Ctrl Pts',(-4.48069793400006,5.2,-1.03117907400001));
#314883=CARTESIAN_POINT('Ctrl Pts',(-4.48069793400006,2.2,-1.03117907400001));
#314884=CARTESIAN_POINT('Ctrl Pts',(-4.47838122000006,12.2,-1.03187466400001));
#314885=CARTESIAN_POINT('Ctrl Pts',(-4.47838122000006,5.2,-1.03187466400001));
#314886=CARTESIAN_POINT('Ctrl Pts',(-4.47838122000006,2.2,-1.03187466400001));
#314887=CARTESIAN_POINT('Ctrl Pts',(-4.47606723100006,12.2,-1.03256675500001));
#314888=CARTESIAN_POINT('Ctrl Pts',(-4.47606723100006,5.2,-1.03256675500001));
#314889=CARTESIAN_POINT('Ctrl Pts',(-4.47606723100006,2.2,-1.03256675500001));
#314890=CARTESIAN_POINT('Ctrl Pts',(-4.47375597800006,12.2,-1.03325535300002));
#314891=CARTESIAN_POINT('Ctrl Pts',(-4.47375597800006,5.2,-1.03325535300002));
#314892=CARTESIAN_POINT('Ctrl Pts',(-4.47375597800006,2.2,-1.03325535300002));
#314893=CARTESIAN_POINT('Ctrl Pts',(-4.47144746500006,12.2,-1.03394046000002));
#314894=CARTESIAN_POINT('Ctrl Pts',(-4.47144746500006,5.2,-1.03394046000002));
#314895=CARTESIAN_POINT('Ctrl Pts',(-4.47144746500006,2.2,-1.03394046000002));
#314896=CARTESIAN_POINT('Ctrl Pts',(-4.46914170300006,12.2,-1.03462208200002));
#314897=CARTESIAN_POINT('Ctrl Pts',(-4.46914170300006,5.2,-1.03462208200002));
#314898=CARTESIAN_POINT('Ctrl Pts',(-4.46914170300006,2.2,-1.03462208200002));
#314899=CARTESIAN_POINT('Ctrl Pts',(-4.46683869800006,12.2,-1.03530022500002));
#314900=CARTESIAN_POINT('Ctrl Pts',(-4.46683869800006,5.2,-1.03530022500002));
#314901=CARTESIAN_POINT('Ctrl Pts',(-4.46683869800006,2.2,-1.03530022500002));
#314902=CARTESIAN_POINT('Ctrl Pts',(-4.46453846000006,12.2,-1.03597489100002));
#314903=CARTESIAN_POINT('Ctrl Pts',(-4.46453846000006,5.2,-1.03597489100002));
#314904=CARTESIAN_POINT('Ctrl Pts',(-4.46453846000006,2.2,-1.03597489100002));
#314905=CARTESIAN_POINT('Ctrl Pts',(-4.46224099700006,12.2,-1.03664608700001));
#314906=CARTESIAN_POINT('Ctrl Pts',(-4.46224099700006,5.2,-1.03664608700001));
#314907=CARTESIAN_POINT('Ctrl Pts',(-4.46224099700006,2.2,-1.03664608700001));
#314908=CARTESIAN_POINT('Ctrl Pts',(-4.45994631700006,12.2,-1.03731381700001));
#314909=CARTESIAN_POINT('Ctrl Pts',(-4.45994631700006,5.2,-1.03731381700001));
#314910=CARTESIAN_POINT('Ctrl Pts',(-4.45994631700006,2.2,-1.03731381700001));
#314911=CARTESIAN_POINT('Ctrl Pts',(-4.45765442500006,12.2,-1.03797808500001));
#314912=CARTESIAN_POINT('Ctrl Pts',(-4.45765442500006,5.2,-1.03797808500001));
#314913=CARTESIAN_POINT('Ctrl Pts',(-4.45765442500006,2.2,-1.03797808500001));
#314914=CARTESIAN_POINT('Ctrl Pts',(-4.45536533500006,12.2,-1.03863889700001));
#314915=CARTESIAN_POINT('Ctrl Pts',(-4.45536533500006,5.2,-1.03863889700001));
#314916=CARTESIAN_POINT('Ctrl Pts',(-4.45536533500006,2.2,-1.03863889700001));
#314917=CARTESIAN_POINT('Ctrl Pts',(-4.45307905000006,12.2,-1.03929625600002));
#314918=CARTESIAN_POINT('Ctrl Pts',(-4.45307905000006,5.2,-1.03929625600002));
#314919=CARTESIAN_POINT('Ctrl Pts',(-4.45307905000006,2.2,-1.03929625600002));
#314920=CARTESIAN_POINT('Ctrl Pts',(-4.45079557900006,12.2,-1.03995016800001));
#314921=CARTESIAN_POINT('Ctrl Pts',(-4.45079557900006,5.2,-1.03995016800001));
#314922=CARTESIAN_POINT('Ctrl Pts',(-4.45079557900006,2.2,-1.03995016800001));
#314923=CARTESIAN_POINT('Ctrl Pts',(-4.44851493300006,12.2,-1.04060063700001));
#314924=CARTESIAN_POINT('Ctrl Pts',(-4.44851493300006,5.2,-1.04060063700001));
#314925=CARTESIAN_POINT('Ctrl Pts',(-4.44851493300006,2.2,-1.04060063700001));
#314926=CARTESIAN_POINT('Ctrl Pts',(-4.44623711800006,12.2,-1.04124767000001));
#314927=CARTESIAN_POINT('Ctrl Pts',(-4.44623711800006,5.2,-1.04124767000001));
#314928=CARTESIAN_POINT('Ctrl Pts',(-4.44623711800006,2.2,-1.04124767000001));
#314929=CARTESIAN_POINT('Ctrl Pts',(-4.44396214200006,12.2,-1.04189126900001));
#314930=CARTESIAN_POINT('Ctrl Pts',(-4.44396214200006,5.2,-1.04189126900001));
#314931=CARTESIAN_POINT('Ctrl Pts',(-4.44396214200006,2.2,-1.04189126900001));
#314932=CARTESIAN_POINT('Ctrl Pts',(-4.44169001300006,12.2,-1.04253144000001));
#314933=CARTESIAN_POINT('Ctrl Pts',(-4.44169001300006,5.2,-1.04253144000001));
#314934=CARTESIAN_POINT('Ctrl Pts',(-4.44169001300006,2.2,-1.04253144000001));
#314935=CARTESIAN_POINT('Ctrl Pts',(-4.43942074200006,12.2,-1.04316818900001));
#314936=CARTESIAN_POINT('Ctrl Pts',(-4.43942074200006,5.2,-1.04316818900001));
#314937=CARTESIAN_POINT('Ctrl Pts',(-4.43942074200006,2.2,-1.04316818900001));
#314938=CARTESIAN_POINT('Ctrl Pts',(-4.43715433200006,12.2,-1.04380152000001));
#314939=CARTESIAN_POINT('Ctrl Pts',(-4.43715433200006,5.2,-1.04380152000001));
#314940=CARTESIAN_POINT('Ctrl Pts',(-4.43715433200006,2.2,-1.04380152000001));
#314941=CARTESIAN_POINT('Ctrl Pts',(-4.43489079500006,12.2,-1.04443143700002));
#314942=CARTESIAN_POINT('Ctrl Pts',(-4.43489079500006,5.2,-1.04443143700002));
#314943=CARTESIAN_POINT('Ctrl Pts',(-4.43489079500006,2.2,-1.04443143700002));
#314944=CARTESIAN_POINT('Ctrl Pts',(-4.43263013900006,12.2,-1.04505794700001));
#314945=CARTESIAN_POINT('Ctrl Pts',(-4.43263013900006,5.2,-1.04505794700001));
#314946=CARTESIAN_POINT('Ctrl Pts',(-4.43263013900006,2.2,-1.04505794700001));
#314947=CARTESIAN_POINT('Ctrl Pts',(-4.43037237100006,12.2,-1.04568105300002));
#314948=CARTESIAN_POINT('Ctrl Pts',(-4.43037237100006,5.2,-1.04568105300002));
#314949=CARTESIAN_POINT('Ctrl Pts',(-4.43037237100006,2.2,-1.04568105300002));
#314950=CARTESIAN_POINT('Ctrl Pts',(-4.42811749900006,12.2,-1.04630076000001));
#314951=CARTESIAN_POINT('Ctrl Pts',(-4.42811749900006,5.2,-1.04630076000001));
#314952=CARTESIAN_POINT('Ctrl Pts',(-4.42811749900006,2.2,-1.04630076000001));
#314953=CARTESIAN_POINT('Ctrl Pts',(-4.42586553200006,12.2,-1.04691707400002));
#314954=CARTESIAN_POINT('Ctrl Pts',(-4.42586553200006,5.2,-1.04691707400002));
#314955=CARTESIAN_POINT('Ctrl Pts',(-4.42586553200006,2.2,-1.04691707400002));
#314956=CARTESIAN_POINT('Ctrl Pts',(-4.42361647800006,12.2,-1.04753000000001));
#314957=CARTESIAN_POINT('Ctrl Pts',(-4.42361647800006,5.2,-1.04753000000001));
#314958=CARTESIAN_POINT('Ctrl Pts',(-4.42361647800006,2.2,-1.04753000000001));
#314959=CARTESIAN_POINT('Ctrl Pts',(-4.42137034500006,12.2,-1.04813954200001));
#314960=CARTESIAN_POINT('Ctrl Pts',(-4.42137034500006,5.2,-1.04813954200001));
#314961=CARTESIAN_POINT('Ctrl Pts',(-4.42137034500006,2.2,-1.04813954200001));
#314962=CARTESIAN_POINT('Ctrl Pts',(-4.41912714100006,12.2,-1.04874570700002));
#314963=CARTESIAN_POINT('Ctrl Pts',(-4.41912714100006,5.2,-1.04874570700002));
#314964=CARTESIAN_POINT('Ctrl Pts',(-4.41912714100006,2.2,-1.04874570700002));
#314965=CARTESIAN_POINT('Ctrl Pts',(-4.41688687400006,12.2,-1.04934849700001));
#314966=CARTESIAN_POINT('Ctrl Pts',(-4.41688687400006,5.2,-1.04934849700001));
#314967=CARTESIAN_POINT('Ctrl Pts',(-4.41688687400006,2.2,-1.04934849700001));
#314968=CARTESIAN_POINT('Ctrl Pts',(-4.41464955400006,12.2,-1.04994792000001));
#314969=CARTESIAN_POINT('Ctrl Pts',(-4.41464955400006,5.2,-1.04994792000001));
#314970=CARTESIAN_POINT('Ctrl Pts',(-4.41464955400006,2.2,-1.04994792000001));
#314971=CARTESIAN_POINT('Ctrl Pts',(-4.41241518600005,12.2,-1.05054398000001));
#314972=CARTESIAN_POINT('Ctrl Pts',(-4.41241518600005,5.2,-1.05054398000001));
#314973=CARTESIAN_POINT('Ctrl Pts',(-4.41241518600005,2.2,-1.05054398000001));
#314974=CARTESIAN_POINT('Ctrl Pts',(-4.41018378200006,12.2,-1.05113668200001));
#314975=CARTESIAN_POINT('Ctrl Pts',(-4.41018378200006,5.2,-1.05113668200001));
#314976=CARTESIAN_POINT('Ctrl Pts',(-4.41018378200006,2.2,-1.05113668200001));
#314977=CARTESIAN_POINT('Ctrl Pts',(-4.40795534700006,12.2,-1.05172603100002));
#314978=CARTESIAN_POINT('Ctrl Pts',(-4.40795534700006,5.2,-1.05172603100002));
#314979=CARTESIAN_POINT('Ctrl Pts',(-4.40795534700006,2.2,-1.05172603100002));
#314980=CARTESIAN_POINT('Ctrl Pts',(-4.40572989000006,12.2,-1.05231203200002));
#314981=CARTESIAN_POINT('Ctrl Pts',(-4.40572989000006,5.2,-1.05231203200002));
#314982=CARTESIAN_POINT('Ctrl Pts',(-4.40572989000006,2.2,-1.05231203200002));
#314983=CARTESIAN_POINT('Ctrl Pts',(-4.40350742100006,12.2,-1.05289469000001));
#314984=CARTESIAN_POINT('Ctrl Pts',(-4.40350742100006,5.2,-1.05289469000001));
#314985=CARTESIAN_POINT('Ctrl Pts',(-4.40350742100006,2.2,-1.05289469000001));
#314986=CARTESIAN_POINT('Ctrl Pts',(-4.40128794700006,12.2,-1.05347401200001));
#314987=CARTESIAN_POINT('Ctrl Pts',(-4.40128794700006,5.2,-1.05347401200001));
#314988=CARTESIAN_POINT('Ctrl Pts',(-4.40128794700006,2.2,-1.05347401200001));
#314989=CARTESIAN_POINT('Ctrl Pts',(-4.39907147400006,12.2,-1.05405000100002));
#314990=CARTESIAN_POINT('Ctrl Pts',(-4.39907147400006,5.2,-1.05405000100002));
#314991=CARTESIAN_POINT('Ctrl Pts',(-4.39907147400006,2.2,-1.05405000100002));
#314992=CARTESIAN_POINT('Ctrl Pts',(-4.39685801400006,12.2,-1.05462266400002));
#314993=CARTESIAN_POINT('Ctrl Pts',(-4.39685801400006,5.2,-1.05462266400002));
#314994=CARTESIAN_POINT('Ctrl Pts',(-4.39685801400006,2.2,-1.05462266400002));
#314995=CARTESIAN_POINT('Ctrl Pts',(-4.39464757300006,12.2,-1.05519200400002));
#314996=CARTESIAN_POINT('Ctrl Pts',(-4.39464757300006,5.2,-1.05519200400002));
#314997=CARTESIAN_POINT('Ctrl Pts',(-4.39464757300006,2.2,-1.05519200400002));
#314998=CARTESIAN_POINT('Ctrl Pts',(-4.39244016100006,12.2,-1.05575802800002));
#314999=CARTESIAN_POINT('Ctrl Pts',(-4.39244016100006,5.2,-1.05575802800002));
#315000=CARTESIAN_POINT('Ctrl Pts',(-4.39244016100006,2.2,-1.05575802800002));
#315001=CARTESIAN_POINT('Ctrl Pts',(-4.39023578400006,12.2,-1.05632074100001));
#315002=CARTESIAN_POINT('Ctrl Pts',(-4.39023578400006,5.2,-1.05632074100001));
#315003=CARTESIAN_POINT('Ctrl Pts',(-4.39023578400006,2.2,-1.05632074100001));
#315004=CARTESIAN_POINT('Ctrl Pts',(-4.38803445100006,12.2,-1.05688014700001));
#315005=CARTESIAN_POINT('Ctrl Pts',(-4.38803445100006,5.2,-1.05688014700001));
#315006=CARTESIAN_POINT('Ctrl Pts',(-4.38803445100006,2.2,-1.05688014700001));
#315007=CARTESIAN_POINT('Ctrl Pts',(-4.38583617100006,12.2,-1.05743625500001));
#315008=CARTESIAN_POINT('Ctrl Pts',(-4.38583617100006,5.2,-1.05743625500001));
#315009=CARTESIAN_POINT('Ctrl Pts',(-4.38583617100006,2.2,-1.05743625500001));
#315010=CARTESIAN_POINT('Ctrl Pts',(-4.38364095300006,12.2,-1.05798906500001));
#315011=CARTESIAN_POINT('Ctrl Pts',(-4.38364095300006,5.2,-1.05798906500001));
#315012=CARTESIAN_POINT('Ctrl Pts',(-4.38364095300006,2.2,-1.05798906500001));
#315013=CARTESIAN_POINT('Ctrl Pts',(-4.38144880200006,12.2,-1.05853858700002));
#315014=CARTESIAN_POINT('Ctrl Pts',(-4.38144880200006,5.2,-1.05853858700002));
#315015=CARTESIAN_POINT('Ctrl Pts',(-4.38144880200006,2.2,-1.05853858700002));
#315016=CARTESIAN_POINT('Ctrl Pts',(-4.37925972900006,12.2,-1.05908482400002));
#315017=CARTESIAN_POINT('Ctrl Pts',(-4.37925972900006,5.2,-1.05908482400002));
#315018=CARTESIAN_POINT('Ctrl Pts',(-4.37925972900006,2.2,-1.05908482400002));
#315019=CARTESIAN_POINT('Ctrl Pts',(-4.37707374200006,12.2,-1.05962778200002));
#315020=CARTESIAN_POINT('Ctrl Pts',(-4.37707374200006,5.2,-1.05962778200002));
#315021=CARTESIAN_POINT('Ctrl Pts',(-4.37707374200006,2.2,-1.05962778200002));
#315022=CARTESIAN_POINT('Ctrl Pts',(-4.37489084900006,12.2,-1.06016746500002));
#315023=CARTESIAN_POINT('Ctrl Pts',(-4.37489084900006,5.2,-1.06016746500002));
#315024=CARTESIAN_POINT('Ctrl Pts',(-4.37489084900006,2.2,-1.06016746500002));
#315025=CARTESIAN_POINT('Ctrl Pts',(-4.37271105700006,12.2,-1.06070388100001));
#315026=CARTESIAN_POINT('Ctrl Pts',(-4.37271105700006,5.2,-1.06070388100001));
#315027=CARTESIAN_POINT('Ctrl Pts',(-4.37271105700006,2.2,-1.06070388100001));
#315028=CARTESIAN_POINT('Ctrl Pts',(-4.37053437700006,12.2,-1.06123703400002));
#315029=CARTESIAN_POINT('Ctrl Pts',(-4.37053437700006,5.2,-1.06123703400002));
#315030=CARTESIAN_POINT('Ctrl Pts',(-4.37053437700006,2.2,-1.06123703400002));
#315031=CARTESIAN_POINT('Ctrl Pts',(-4.36836081500006,12.2,-1.06176692900001));
#315032=CARTESIAN_POINT('Ctrl Pts',(-4.36836081500006,5.2,-1.06176692900001));
#315033=CARTESIAN_POINT('Ctrl Pts',(-4.36836081500006,2.2,-1.06176692900001));
#315034=CARTESIAN_POINT('Ctrl Pts',(-4.36619038000006,12.2,-1.06229357300001));
#315035=CARTESIAN_POINT('Ctrl Pts',(-4.36619038000006,5.2,-1.06229357300001));
#315036=CARTESIAN_POINT('Ctrl Pts',(-4.36619038000006,2.2,-1.06229357300001));
#315037=CARTESIAN_POINT('Ctrl Pts',(-4.36402308000006,12.2,-1.06281697000002));
#315038=CARTESIAN_POINT('Ctrl Pts',(-4.36402308000006,5.2,-1.06281697000002));
#315039=CARTESIAN_POINT('Ctrl Pts',(-4.36402308000006,2.2,-1.06281697000002));
#315040=CARTESIAN_POINT('Ctrl Pts',(-4.36185892400006,12.2,-1.06333712600001));
#315041=CARTESIAN_POINT('Ctrl Pts',(-4.36185892400006,5.2,-1.06333712600001));
#315042=CARTESIAN_POINT('Ctrl Pts',(-4.36185892400006,2.2,-1.06333712600001));
#315043=CARTESIAN_POINT('Ctrl Pts',(-4.35969792000006,12.2,-1.06385404700001));
#315044=CARTESIAN_POINT('Ctrl Pts',(-4.35969792000006,5.2,-1.06385404700001));
#315045=CARTESIAN_POINT('Ctrl Pts',(-4.35969792000006,2.2,-1.06385404700001));
#315046=CARTESIAN_POINT('Ctrl Pts',(-4.35754007500006,12.2,-1.06436773800001));
#315047=CARTESIAN_POINT('Ctrl Pts',(-4.35754007500006,5.2,-1.06436773800001));
#315048=CARTESIAN_POINT('Ctrl Pts',(-4.35754007500006,2.2,-1.06436773800001));
#315049=CARTESIAN_POINT('Ctrl Pts',(-4.35538539900006,12.2,-1.06487820600002));
#315050=CARTESIAN_POINT('Ctrl Pts',(-4.35538539900006,5.2,-1.06487820600002));
#315051=CARTESIAN_POINT('Ctrl Pts',(-4.35538539900006,2.2,-1.06487820600002));
#315052=CARTESIAN_POINT('Ctrl Pts',(-4.35323390100006,12.2,-1.06538545400001));
#315053=CARTESIAN_POINT('Ctrl Pts',(-4.35323390100006,5.2,-1.06538545400001));
#315054=CARTESIAN_POINT('Ctrl Pts',(-4.35323390100006,2.2,-1.06538545400001));
#315055=CARTESIAN_POINT('Ctrl Pts',(-4.35108558800006,12.2,-1.06588948900002));
#315056=CARTESIAN_POINT('Ctrl Pts',(-4.35108558800006,5.2,-1.06588948900002));
#315057=CARTESIAN_POINT('Ctrl Pts',(-4.35108558800006,2.2,-1.06588948900002));
#315058=CARTESIAN_POINT('Ctrl Pts',(-4.34894046700006,12.2,-1.06639031800002));
#315059=CARTESIAN_POINT('Ctrl Pts',(-4.34894046700006,5.2,-1.06639031800002));
#315060=CARTESIAN_POINT('Ctrl Pts',(-4.34894046700006,2.2,-1.06639031800002));
#315061=CARTESIAN_POINT('Ctrl Pts',(-4.34679854900006,12.2,-1.06688794400001));
#315062=CARTESIAN_POINT('Ctrl Pts',(-4.34679854900006,5.2,-1.06688794400001));
#315063=CARTESIAN_POINT('Ctrl Pts',(-4.34679854900006,2.2,-1.06688794400001));
#315064=CARTESIAN_POINT('Ctrl Pts',(-4.34465984100005,12.2,-1.06738237400001));
#315065=CARTESIAN_POINT('Ctrl Pts',(-4.34465984100005,5.2,-1.06738237400001));
#315066=CARTESIAN_POINT('Ctrl Pts',(-4.34465984100005,2.2,-1.06738237400001));
#315067=CARTESIAN_POINT('Ctrl Pts',(-4.34252435100006,12.2,-1.06787361500002));
#315068=CARTESIAN_POINT('Ctrl Pts',(-4.34252435100006,5.2,-1.06787361500002));
#315069=CARTESIAN_POINT('Ctrl Pts',(-4.34252435100006,2.2,-1.06787361500002));
#315070=CARTESIAN_POINT('Ctrl Pts',(-4.34039208900006,12.2,-1.06836166900001));
#315071=CARTESIAN_POINT('Ctrl Pts',(-4.34039208900006,5.2,-1.06836166900001));
#315072=CARTESIAN_POINT('Ctrl Pts',(-4.34039208900006,2.2,-1.06836166900001));
#315073=CARTESIAN_POINT('Ctrl Pts',(-4.33826306000006,12.2,-1.06884654600002));
#315074=CARTESIAN_POINT('Ctrl Pts',(-4.33826306000006,5.2,-1.06884654600002));
#315075=CARTESIAN_POINT('Ctrl Pts',(-4.33826306000006,2.2,-1.06884654600002));
#315076=CARTESIAN_POINT('Ctrl Pts',(-4.33613727600005,12.2,-1.06932824900001));
#315077=CARTESIAN_POINT('Ctrl Pts',(-4.33613727600005,5.2,-1.06932824900001));
#315078=CARTESIAN_POINT('Ctrl Pts',(-4.33613727600005,2.2,-1.06932824900001));
#315079=CARTESIAN_POINT('Ctrl Pts',(-4.33401474400006,12.2,-1.06980678600001));
#315080=CARTESIAN_POINT('Ctrl Pts',(-4.33401474400006,5.2,-1.06980678600001));
#315081=CARTESIAN_POINT('Ctrl Pts',(-4.33401474400006,2.2,-1.06980678600001));
#315082=CARTESIAN_POINT('Ctrl Pts',(-4.33189547100006,12.2,-1.07028216000002));
#315083=CARTESIAN_POINT('Ctrl Pts',(-4.33189547100006,5.2,-1.07028216000002));
#315084=CARTESIAN_POINT('Ctrl Pts',(-4.33189547100006,2.2,-1.07028216000002));
#315085=CARTESIAN_POINT('Ctrl Pts',(-4.32977946700006,12.2,-1.07075437900002));
#315086=CARTESIAN_POINT('Ctrl Pts',(-4.32977946700006,5.2,-1.07075437900002));
#315087=CARTESIAN_POINT('Ctrl Pts',(-4.32977946700006,2.2,-1.07075437900002));
#315088=CARTESIAN_POINT('Ctrl Pts',(-4.32766674000006,12.2,-1.07122344700001));
#315089=CARTESIAN_POINT('Ctrl Pts',(-4.32766674000006,5.2,-1.07122344700001));
#315090=CARTESIAN_POINT('Ctrl Pts',(-4.32766674000006,2.2,-1.07122344700001));
#315091=CARTESIAN_POINT('Ctrl Pts',(-4.32555729900006,12.2,-1.07168937200001));
#315092=CARTESIAN_POINT('Ctrl Pts',(-4.32555729900006,5.2,-1.07168937200001));
#315093=CARTESIAN_POINT('Ctrl Pts',(-4.32555729900006,2.2,-1.07168937200001));
#315094=CARTESIAN_POINT('Ctrl Pts',(-4.32345115100006,12.2,-1.07215215900001));
#315095=CARTESIAN_POINT('Ctrl Pts',(-4.32345115100006,5.2,-1.07215215900001));
#315096=CARTESIAN_POINT('Ctrl Pts',(-4.32345115100006,2.2,-1.07215215900001));
#315097=CARTESIAN_POINT('Ctrl Pts',(-4.32134830500006,12.2,-1.07261181400002));
#315098=CARTESIAN_POINT('Ctrl Pts',(-4.32134830500006,5.2,-1.07261181400002));
#315099=CARTESIAN_POINT('Ctrl Pts',(-4.32134830500006,2.2,-1.07261181400002));
#315100=CARTESIAN_POINT('Ctrl Pts',(-4.31924877000006,12.2,-1.07306834100001));
#315101=CARTESIAN_POINT('Ctrl Pts',(-4.31924877000006,5.2,-1.07306834100001));
#315102=CARTESIAN_POINT('Ctrl Pts',(-4.31924877000006,2.2,-1.07306834100001));
#315103=CARTESIAN_POINT('Ctrl Pts',(-4.31715255400006,12.2,-1.07352174900001));
#315104=CARTESIAN_POINT('Ctrl Pts',(-4.31715255400006,5.2,-1.07352174900001));
#315105=CARTESIAN_POINT('Ctrl Pts',(-4.31715255400006,2.2,-1.07352174900001));
#315106=CARTESIAN_POINT('Ctrl Pts',(-4.31505966400006,12.2,-1.07397204200002));
#315107=CARTESIAN_POINT('Ctrl Pts',(-4.31505966400006,5.2,-1.07397204200002));
#315108=CARTESIAN_POINT('Ctrl Pts',(-4.31505966400006,2.2,-1.07397204200002));
#315109=CARTESIAN_POINT('Ctrl Pts',(-4.31297011000006,12.2,-1.07441922700001));
#315110=CARTESIAN_POINT('Ctrl Pts',(-4.31297011000006,5.2,-1.07441922700001));
#315111=CARTESIAN_POINT('Ctrl Pts',(-4.31297011000006,2.2,-1.07441922700001));
#315112=CARTESIAN_POINT('Ctrl Pts',(-4.31088390100006,12.2,-1.07486330900001));
#315113=CARTESIAN_POINT('Ctrl Pts',(-4.31088390100006,5.2,-1.07486330900001));
#315114=CARTESIAN_POINT('Ctrl Pts',(-4.31088390100006,2.2,-1.07486330900001));
#315115=CARTESIAN_POINT('Ctrl Pts',(-4.30880104300006,12.2,-1.07530429500001));
#315116=CARTESIAN_POINT('Ctrl Pts',(-4.30880104300006,5.2,-1.07530429500001));
#315117=CARTESIAN_POINT('Ctrl Pts',(-4.30880104300006,2.2,-1.07530429500001));
#315118=CARTESIAN_POINT('Ctrl Pts',(-4.30672154600006,12.2,-1.07574219000002));
#315119=CARTESIAN_POINT('Ctrl Pts',(-4.30672154600006,5.2,-1.07574219000002));
#315120=CARTESIAN_POINT('Ctrl Pts',(-4.30672154600006,2.2,-1.07574219000002));
#315121=CARTESIAN_POINT('Ctrl Pts',(-4.30464541900006,12.2,-1.07617700100001));
#315122=CARTESIAN_POINT('Ctrl Pts',(-4.30464541900006,5.2,-1.07617700100001));
#315123=CARTESIAN_POINT('Ctrl Pts',(-4.30464541900006,2.2,-1.07617700100001));
#315124=CARTESIAN_POINT('Ctrl Pts',(-4.30257267000006,12.2,-1.07660873400001));
#315125=CARTESIAN_POINT('Ctrl Pts',(-4.30257267000006,5.2,-1.07660873400001));
#315126=CARTESIAN_POINT('Ctrl Pts',(-4.30257267000006,2.2,-1.07660873400001));
#315127=CARTESIAN_POINT('Ctrl Pts',(-4.30050330700006,12.2,-1.07703739400002));
#315128=CARTESIAN_POINT('Ctrl Pts',(-4.30050330700006,5.2,-1.07703739400002));
#315129=CARTESIAN_POINT('Ctrl Pts',(-4.30050330700006,2.2,-1.07703739400002));
#315130=CARTESIAN_POINT('Ctrl Pts',(-4.29843733800006,12.2,-1.07746298900001));
#315131=CARTESIAN_POINT('Ctrl Pts',(-4.29843733800006,5.2,-1.07746298900001));
#315132=CARTESIAN_POINT('Ctrl Pts',(-4.29843733800006,2.2,-1.07746298900001));
#315133=CARTESIAN_POINT('Ctrl Pts',(-4.29637477200006,12.2,-1.07788552300002));
#315134=CARTESIAN_POINT('Ctrl Pts',(-4.29637477200006,5.2,-1.07788552300002));
#315135=CARTESIAN_POINT('Ctrl Pts',(-4.29637477200006,2.2,-1.07788552300002));
#315136=CARTESIAN_POINT('Ctrl Pts',(-4.29431561700006,12.2,-1.07830500400001));
#315137=CARTESIAN_POINT('Ctrl Pts',(-4.29431561700006,5.2,-1.07830500400001));
#315138=CARTESIAN_POINT('Ctrl Pts',(-4.29431561700006,2.2,-1.07830500400001));
#315139=CARTESIAN_POINT('Ctrl Pts',(-4.29225988200006,12.2,-1.07872143700002));
#315140=CARTESIAN_POINT('Ctrl Pts',(-4.29225988200006,5.2,-1.07872143700002));
#315141=CARTESIAN_POINT('Ctrl Pts',(-4.29225988200006,2.2,-1.07872143700002));
#315142=CARTESIAN_POINT('Ctrl Pts',(-4.29020757500005,12.2,-1.07913482900001));
#315143=CARTESIAN_POINT('Ctrl Pts',(-4.29020757500005,5.2,-1.07913482900001));
#315144=CARTESIAN_POINT('Ctrl Pts',(-4.29020757500005,2.2,-1.07913482900001));
#315145=CARTESIAN_POINT('Ctrl Pts',(-4.28815870600006,12.2,-1.07954518600001));
#315146=CARTESIAN_POINT('Ctrl Pts',(-4.28815870600006,5.2,-1.07954518600001));
#315147=CARTESIAN_POINT('Ctrl Pts',(-4.28815870600006,2.2,-1.07954518600001));
#315148=CARTESIAN_POINT('Ctrl Pts',(-4.28611328100006,12.2,-1.07995251300002));
#315149=CARTESIAN_POINT('Ctrl Pts',(-4.28611328100006,5.2,-1.07995251300002));
#315150=CARTESIAN_POINT('Ctrl Pts',(-4.28611328100006,2.2,-1.07995251300002));
#315151=CARTESIAN_POINT('Ctrl Pts',(-4.28407131000006,12.2,-1.08035681800001));
#315152=CARTESIAN_POINT('Ctrl Pts',(-4.28407131000006,5.2,-1.08035681800001));
#315153=CARTESIAN_POINT('Ctrl Pts',(-4.28407131000006,2.2,-1.08035681800001));
#315154=CARTESIAN_POINT('Ctrl Pts',(-4.28203280000006,12.2,-1.08075810700001));
#315155=CARTESIAN_POINT('Ctrl Pts',(-4.28203280000006,5.2,-1.08075810700001));
#315156=CARTESIAN_POINT('Ctrl Pts',(-4.28203280000006,2.2,-1.08075810700001));
#315157=CARTESIAN_POINT('Ctrl Pts',(-4.27999776200005,12.2,-1.08115638600002));
#315158=CARTESIAN_POINT('Ctrl Pts',(-4.27999776200005,5.2,-1.08115638600002));
#315159=CARTESIAN_POINT('Ctrl Pts',(-4.27999776200005,2.2,-1.08115638600002));
#315160=CARTESIAN_POINT('Ctrl Pts',(-4.27796620300006,12.2,-1.08155166100001));
#315161=CARTESIAN_POINT('Ctrl Pts',(-4.27796620300006,5.2,-1.08155166100001));
#315162=CARTESIAN_POINT('Ctrl Pts',(-4.27796620300006,2.2,-1.08155166100001));
#315163=CARTESIAN_POINT('Ctrl Pts',(-4.27593813100006,12.2,-1.08194393800002));
#315164=CARTESIAN_POINT('Ctrl Pts',(-4.27593813100006,5.2,-1.08194393800002));
#315165=CARTESIAN_POINT('Ctrl Pts',(-4.27593813100006,2.2,-1.08194393800002));
#315166=CARTESIAN_POINT('Ctrl Pts',(-4.27391355500006,12.2,-1.08233322400002));
#315167=CARTESIAN_POINT('Ctrl Pts',(-4.27391355500006,5.2,-1.08233322400002));
#315168=CARTESIAN_POINT('Ctrl Pts',(-4.27391355500006,2.2,-1.08233322400002));
#315169=CARTESIAN_POINT('Ctrl Pts',(-4.27189248300006,12.2,-1.08271952700001));
#315170=CARTESIAN_POINT('Ctrl Pts',(-4.27189248300006,5.2,-1.08271952700001));
#315171=CARTESIAN_POINT('Ctrl Pts',(-4.27189248300006,2.2,-1.08271952700001));
#315172=CARTESIAN_POINT('Ctrl Pts',(-4.26987492400006,12.2,-1.08310285000002));
#315173=CARTESIAN_POINT('Ctrl Pts',(-4.26987492400006,5.2,-1.08310285000002));
#315174=CARTESIAN_POINT('Ctrl Pts',(-4.26987492400006,2.2,-1.08310285000002));
#315175=CARTESIAN_POINT('Ctrl Pts',(-4.26786088700006,12.2,-1.08348320200002));
#315176=CARTESIAN_POINT('Ctrl Pts',(-4.26786088700006,5.2,-1.08348320200002));
#315177=CARTESIAN_POINT('Ctrl Pts',(-4.26786088700006,2.2,-1.08348320200002));
#315178=CARTESIAN_POINT('Ctrl Pts',(-4.26585037900006,12.2,-1.08386058900001));
#315179=CARTESIAN_POINT('Ctrl Pts',(-4.26585037900006,5.2,-1.08386058900001));
#315180=CARTESIAN_POINT('Ctrl Pts',(-4.26585037900006,2.2,-1.08386058900001));
#315181=CARTESIAN_POINT('Ctrl Pts',(-4.26384341100006,12.2,-1.08423501800001));
#315182=CARTESIAN_POINT('Ctrl Pts',(-4.26384341100006,5.2,-1.08423501800001));
#315183=CARTESIAN_POINT('Ctrl Pts',(-4.26384341100006,2.2,-1.08423501800001));
#315184=CARTESIAN_POINT('Ctrl Pts',(-4.26183998900005,12.2,-1.08460649400001));
#315185=CARTESIAN_POINT('Ctrl Pts',(-4.26183998900005,5.2,-1.08460649400001));
#315186=CARTESIAN_POINT('Ctrl Pts',(-4.26183998900005,2.2,-1.08460649400001));
#315187=CARTESIAN_POINT('Ctrl Pts',(-4.25984012300006,12.2,-1.08497502300001));
#315188=CARTESIAN_POINT('Ctrl Pts',(-4.25984012300006,5.2,-1.08497502300001));
#315189=CARTESIAN_POINT('Ctrl Pts',(-4.25984012300006,2.2,-1.08497502300001));
#315190=CARTESIAN_POINT('Ctrl Pts',(-4.25784382000006,12.2,-1.08534061400002));
#315191=CARTESIAN_POINT('Ctrl Pts',(-4.25784382000006,5.2,-1.08534061400002));
#315192=CARTESIAN_POINT('Ctrl Pts',(-4.25784382000006,2.2,-1.08534061400002));
#315193=CARTESIAN_POINT('Ctrl Pts',(-4.25585109000005,12.2,-1.08570327200002));
#315194=CARTESIAN_POINT('Ctrl Pts',(-4.25585109000005,5.2,-1.08570327200002));
#315195=CARTESIAN_POINT('Ctrl Pts',(-4.25585109000005,2.2,-1.08570327200002));
#315196=CARTESIAN_POINT('Ctrl Pts',(-4.25386194100006,12.2,-1.08606300500002));
#315197=CARTESIAN_POINT('Ctrl Pts',(-4.25386194100006,5.2,-1.08606300500002));
#315198=CARTESIAN_POINT('Ctrl Pts',(-4.25386194100006,2.2,-1.08606300500002));
#315199=CARTESIAN_POINT('Ctrl Pts',(-4.25187638100006,12.2,-1.08641981700002));
#315200=CARTESIAN_POINT('Ctrl Pts',(-4.25187638100006,5.2,-1.08641981700002));
#315201=CARTESIAN_POINT('Ctrl Pts',(-4.25187638100006,2.2,-1.08641981700002));
#315202=CARTESIAN_POINT('Ctrl Pts',(-4.24989441900006,12.2,-1.08677371700002));
#315203=CARTESIAN_POINT('Ctrl Pts',(-4.24989441900006,5.2,-1.08677371700002));
#315204=CARTESIAN_POINT('Ctrl Pts',(-4.24989441900006,2.2,-1.08677371700002));
#315205=CARTESIAN_POINT('Ctrl Pts',(-4.24791606500006,12.2,-1.08712471100001));
#315206=CARTESIAN_POINT('Ctrl Pts',(-4.24791606500006,5.2,-1.08712471100001));
#315207=CARTESIAN_POINT('Ctrl Pts',(-4.24791606500006,2.2,-1.08712471100001));
#315208=CARTESIAN_POINT('Ctrl Pts',(-4.24594132400006,12.2,-1.08747280500001));
#315209=CARTESIAN_POINT('Ctrl Pts',(-4.24594132400006,5.2,-1.08747280500001));
#315210=CARTESIAN_POINT('Ctrl Pts',(-4.24594132400006,2.2,-1.08747280500001));
#315211=CARTESIAN_POINT('Ctrl Pts',(-4.24397020800006,12.2,-1.08781800600001));
#315212=CARTESIAN_POINT('Ctrl Pts',(-4.24397020800006,5.2,-1.08781800600001));
#315213=CARTESIAN_POINT('Ctrl Pts',(-4.24397020800006,2.2,-1.08781800600001));
#315214=CARTESIAN_POINT('Ctrl Pts',(-4.24200272500006,12.2,-1.08816032300001));
#315215=CARTESIAN_POINT('Ctrl Pts',(-4.24200272500006,5.2,-1.08816032300001));
#315216=CARTESIAN_POINT('Ctrl Pts',(-4.24200272500006,2.2,-1.08816032300001));
#315217=CARTESIAN_POINT('Ctrl Pts',(-4.24003888100006,12.2,-1.08849975800001));
#315218=CARTESIAN_POINT('Ctrl Pts',(-4.24003888100006,5.2,-1.08849975800001));
#315219=CARTESIAN_POINT('Ctrl Pts',(-4.24003888100006,2.2,-1.08849975800001));
#315220=CARTESIAN_POINT('Ctrl Pts',(-4.23807868800006,12.2,-1.08883632200001));
#315221=CARTESIAN_POINT('Ctrl Pts',(-4.23807868800006,5.2,-1.08883632200001));
#315222=CARTESIAN_POINT('Ctrl Pts',(-4.23807868800006,2.2,-1.08883632200001));
#315223=CARTESIAN_POINT('Ctrl Pts',(-4.23612215200006,12.2,-1.08917002000001));
#315224=CARTESIAN_POINT('Ctrl Pts',(-4.23612215200006,5.2,-1.08917002000001));
#315225=CARTESIAN_POINT('Ctrl Pts',(-4.23612215200006,2.2,-1.08917002000001));
#315226=CARTESIAN_POINT('Ctrl Pts',(-4.23416928100006,12.2,-1.08950086000001));
#315227=CARTESIAN_POINT('Ctrl Pts',(-4.23416928100006,5.2,-1.08950086000001));
#315228=CARTESIAN_POINT('Ctrl Pts',(-4.23416928100006,2.2,-1.08950086000001));
#315229=CARTESIAN_POINT('Ctrl Pts',(-4.23222008800006,12.2,-1.08982884600001));
#315230=CARTESIAN_POINT('Ctrl Pts',(-4.23222008800006,5.2,-1.08982884600001));
#315231=CARTESIAN_POINT('Ctrl Pts',(-4.23222008800006,2.2,-1.08982884600001));
#315232=CARTESIAN_POINT('Ctrl Pts',(-4.23027457600006,12.2,-1.09015398800001));
#315233=CARTESIAN_POINT('Ctrl Pts',(-4.23027457600006,5.2,-1.09015398800001));
#315234=CARTESIAN_POINT('Ctrl Pts',(-4.23027457600006,2.2,-1.09015398800001));
#315235=CARTESIAN_POINT('Ctrl Pts',(-4.22833275800006,12.2,-1.09047629200001));
#315236=CARTESIAN_POINT('Ctrl Pts',(-4.22833275800006,5.2,-1.09047629200001));
#315237=CARTESIAN_POINT('Ctrl Pts',(-4.22833275800006,2.2,-1.09047629200001));
#315238=CARTESIAN_POINT('Ctrl Pts',(-4.22639464000006,12.2,-1.09079576400001));
#315239=CARTESIAN_POINT('Ctrl Pts',(-4.22639464000006,5.2,-1.09079576400001));
#315240=CARTESIAN_POINT('Ctrl Pts',(-4.22639464000006,2.2,-1.09079576400001));
#315241=CARTESIAN_POINT('Ctrl Pts',(-4.22446023100005,12.2,-1.09111241100001));
#315242=CARTESIAN_POINT('Ctrl Pts',(-4.22446023100005,5.2,-1.09111241100001));
#315243=CARTESIAN_POINT('Ctrl Pts',(-4.22446023100005,2.2,-1.09111241100001));
#315244=CARTESIAN_POINT('Ctrl Pts',(-4.22252954000006,12.2,-1.09142624100001));
#315245=CARTESIAN_POINT('Ctrl Pts',(-4.22252954000006,5.2,-1.09142624100001));
#315246=CARTESIAN_POINT('Ctrl Pts',(-4.22252954000006,2.2,-1.09142624100001));
#315247=CARTESIAN_POINT('Ctrl Pts',(-4.22060257600006,12.2,-1.09173726000002));
#315248=CARTESIAN_POINT('Ctrl Pts',(-4.22060257600006,5.2,-1.09173726000002));
#315249=CARTESIAN_POINT('Ctrl Pts',(-4.22060257600006,2.2,-1.09173726000002));
#315250=CARTESIAN_POINT('Ctrl Pts',(-4.21867934700006,12.2,-1.09204547600001));
#315251=CARTESIAN_POINT('Ctrl Pts',(-4.21867934700006,5.2,-1.09204547600001));
#315252=CARTESIAN_POINT('Ctrl Pts',(-4.21867934700006,2.2,-1.09204547600001));
#315253=CARTESIAN_POINT('Ctrl Pts',(-4.21675986200006,12.2,-1.09235089600002));
#315254=CARTESIAN_POINT('Ctrl Pts',(-4.21675986200006,5.2,-1.09235089600002));
#315255=CARTESIAN_POINT('Ctrl Pts',(-4.21675986200006,2.2,-1.09235089600002));
#315256=CARTESIAN_POINT('Ctrl Pts',(-4.21484413000006,12.2,-1.09265352600001));
#315257=CARTESIAN_POINT('Ctrl Pts',(-4.21484413000006,5.2,-1.09265352600001));
#315258=CARTESIAN_POINT('Ctrl Pts',(-4.21484413000006,2.2,-1.09265352600001));
#315259=CARTESIAN_POINT('Ctrl Pts',(-4.21293215800006,12.2,-1.09295337400001));
#315260=CARTESIAN_POINT('Ctrl Pts',(-4.21293215800006,5.2,-1.09295337400001));
#315261=CARTESIAN_POINT('Ctrl Pts',(-4.21293215800006,2.2,-1.09295337400001));
#315262=CARTESIAN_POINT('Ctrl Pts',(-4.21102395600006,12.2,-1.09325044600002));
#315263=CARTESIAN_POINT('Ctrl Pts',(-4.21102395600006,5.2,-1.09325044600002));
#315264=CARTESIAN_POINT('Ctrl Pts',(-4.21102395600006,2.2,-1.09325044600002));
#315265=CARTESIAN_POINT('Ctrl Pts',(-4.20911953100005,12.2,-1.09354475000002));
#315266=CARTESIAN_POINT('Ctrl Pts',(-4.20911953100005,5.2,-1.09354475000002));
#315267=CARTESIAN_POINT('Ctrl Pts',(-4.20911953100005,2.2,-1.09354475000002));
#315268=CARTESIAN_POINT('Ctrl Pts',(-4.20721889400006,12.2,-1.09383629300002));
#315269=CARTESIAN_POINT('Ctrl Pts',(-4.20721889400006,5.2,-1.09383629300002));
#315270=CARTESIAN_POINT('Ctrl Pts',(-4.20721889400006,2.2,-1.09383629300002));
#315271=CARTESIAN_POINT('Ctrl Pts',(-4.20532205200006,12.2,-1.09412508200001));
#315272=CARTESIAN_POINT('Ctrl Pts',(-4.20532205200006,5.2,-1.09412508200001));
#315273=CARTESIAN_POINT('Ctrl Pts',(-4.20532205200006,2.2,-1.09412508200001));
#315274=CARTESIAN_POINT('Ctrl Pts',(-4.20342901500006,12.2,-1.09441112300001));
#315275=CARTESIAN_POINT('Ctrl Pts',(-4.20342901500006,5.2,-1.09441112300001));
#315276=CARTESIAN_POINT('Ctrl Pts',(-4.20342901500006,2.2,-1.09441112300001));
#315277=CARTESIAN_POINT('Ctrl Pts',(-4.20153979000006,12.2,-1.09469442700002));
#315278=CARTESIAN_POINT('Ctrl Pts',(-4.20153979000006,5.2,-1.09469442700002));
#315279=CARTESIAN_POINT('Ctrl Pts',(-4.20153979000006,2.2,-1.09469442700002));
#315280=CARTESIAN_POINT('Ctrl Pts',(-4.19965438700006,12.2,-1.09497499600002));
#315281=CARTESIAN_POINT('Ctrl Pts',(-4.19965438700006,5.2,-1.09497499600002));
#315282=CARTESIAN_POINT('Ctrl Pts',(-4.19965438700006,2.2,-1.09497499600002));
#315283=CARTESIAN_POINT('Ctrl Pts',(-4.19777281400005,12.2,-1.09525284200001));
#315284=CARTESIAN_POINT('Ctrl Pts',(-4.19777281400005,5.2,-1.09525284200001));
#315285=CARTESIAN_POINT('Ctrl Pts',(-4.19777281400005,2.2,-1.09525284200001));
#315286=CARTESIAN_POINT('Ctrl Pts',(-4.19589508000006,12.2,-1.09552797000001));
#315287=CARTESIAN_POINT('Ctrl Pts',(-4.19589508000006,5.2,-1.09552797000001));
#315288=CARTESIAN_POINT('Ctrl Pts',(-4.19589508000006,2.2,-1.09552797000001));
#315289=CARTESIAN_POINT('Ctrl Pts',(-4.19402119200006,12.2,-1.09580038700001));
#315290=CARTESIAN_POINT('Ctrl Pts',(-4.19402119200006,5.2,-1.09580038700001));
#315291=CARTESIAN_POINT('Ctrl Pts',(-4.19402119200006,2.2,-1.09580038700001));
#315292=CARTESIAN_POINT('Ctrl Pts',(-4.19215116100006,12.2,-1.09607010100001));
#315293=CARTESIAN_POINT('Ctrl Pts',(-4.19215116100006,5.2,-1.09607010100001));
#315294=CARTESIAN_POINT('Ctrl Pts',(-4.19215116100006,2.2,-1.09607010100001));
#315295=CARTESIAN_POINT('Ctrl Pts',(-4.19028499500006,12.2,-1.09633711900001));
#315296=CARTESIAN_POINT('Ctrl Pts',(-4.19028499500006,5.2,-1.09633711900001));
#315297=CARTESIAN_POINT('Ctrl Pts',(-4.19028499500006,2.2,-1.09633711900001));
#315298=CARTESIAN_POINT('Ctrl Pts',(-4.18842270200006,12.2,-1.09660144900001));
#315299=CARTESIAN_POINT('Ctrl Pts',(-4.18842270200006,5.2,-1.09660144900001));
#315300=CARTESIAN_POINT('Ctrl Pts',(-4.18842270200006,2.2,-1.09660144900001));
#315301=CARTESIAN_POINT('Ctrl Pts',(-4.18656429100006,12.2,-1.09686309800002));
#315302=CARTESIAN_POINT('Ctrl Pts',(-4.18656429100006,5.2,-1.09686309800002));
#315303=CARTESIAN_POINT('Ctrl Pts',(-4.18656429100006,2.2,-1.09686309800002));
#315304=CARTESIAN_POINT('Ctrl Pts',(-4.18470977100006,12.2,-1.09712207300001));
#315305=CARTESIAN_POINT('Ctrl Pts',(-4.18470977100006,5.2,-1.09712207300001));
#315306=CARTESIAN_POINT('Ctrl Pts',(-4.18470977100006,2.2,-1.09712207300001));
#315307=CARTESIAN_POINT('Ctrl Pts',(-4.18285915000006,12.2,-1.09737838300001));
#315308=CARTESIAN_POINT('Ctrl Pts',(-4.18285915000006,5.2,-1.09737838300001));
#315309=CARTESIAN_POINT('Ctrl Pts',(-4.18285915000006,2.2,-1.09737838300001));
#315310=CARTESIAN_POINT('Ctrl Pts',(-4.18101243800006,12.2,-1.09763203300002));
#315311=CARTESIAN_POINT('Ctrl Pts',(-4.18101243800006,5.2,-1.09763203300002));
#315312=CARTESIAN_POINT('Ctrl Pts',(-4.18101243800006,2.2,-1.09763203300002));
#315313=CARTESIAN_POINT('Ctrl Pts',(-4.17916964200006,12.2,-1.09788303300002));
#315314=CARTESIAN_POINT('Ctrl Pts',(-4.17916964200006,5.2,-1.09788303300002));
#315315=CARTESIAN_POINT('Ctrl Pts',(-4.17916964200006,2.2,-1.09788303300002));
#315316=CARTESIAN_POINT('Ctrl Pts',(-4.17733077200006,12.2,-1.09813138900002));
#315317=CARTESIAN_POINT('Ctrl Pts',(-4.17733077200006,5.2,-1.09813138900002));
#315318=CARTESIAN_POINT('Ctrl Pts',(-4.17733077200006,2.2,-1.09813138900002));
#315319=CARTESIAN_POINT('Ctrl Pts',(-4.17549583700006,12.2,-1.09837710900001));
#315320=CARTESIAN_POINT('Ctrl Pts',(-4.17549583700006,5.2,-1.09837710900001));
#315321=CARTESIAN_POINT('Ctrl Pts',(-4.17549583700006,2.2,-1.09837710900001));
#315322=CARTESIAN_POINT('Ctrl Pts',(-4.17366484400006,12.2,-1.09862020100001));
#315323=CARTESIAN_POINT('Ctrl Pts',(-4.17366484400006,5.2,-1.09862020100001));
#315324=CARTESIAN_POINT('Ctrl Pts',(-4.17366484400006,2.2,-1.09862020100001));
#315325=CARTESIAN_POINT('Ctrl Pts',(-4.17183780200006,12.2,-1.09886067100001));
#315326=CARTESIAN_POINT('Ctrl Pts',(-4.17183780200006,5.2,-1.09886067100001));
#315327=CARTESIAN_POINT('Ctrl Pts',(-4.17183780200006,2.2,-1.09886067100001));
#315328=CARTESIAN_POINT('Ctrl Pts',(-4.17001472200006,12.2,-1.09909852800001));
#315329=CARTESIAN_POINT('Ctrl Pts',(-4.17001472200006,5.2,-1.09909852800001));
#315330=CARTESIAN_POINT('Ctrl Pts',(-4.17001472200006,2.2,-1.09909852800001));
#315331=CARTESIAN_POINT('Ctrl Pts',(-4.16819561000006,12.2,-1.09933378000001));
#315332=CARTESIAN_POINT('Ctrl Pts',(-4.16819561000006,5.2,-1.09933378000001));
#315333=CARTESIAN_POINT('Ctrl Pts',(-4.16819561000006,2.2,-1.09933378000001));
#315334=CARTESIAN_POINT('Ctrl Pts',(-4.16638047600006,12.2,-1.09956643300002));
#315335=CARTESIAN_POINT('Ctrl Pts',(-4.16638047600006,5.2,-1.09956643300002));
#315336=CARTESIAN_POINT('Ctrl Pts',(-4.16638047600006,2.2,-1.09956643300002));
#315337=CARTESIAN_POINT('Ctrl Pts',(-4.16456932900005,12.2,-1.09979649700001));
#315338=CARTESIAN_POINT('Ctrl Pts',(-4.16456932900005,5.2,-1.09979649700001));
#315339=CARTESIAN_POINT('Ctrl Pts',(-4.16456932900005,2.2,-1.09979649700001));
#315340=CARTESIAN_POINT('Ctrl Pts',(-4.16276217800006,12.2,-1.10002397800002));
#315341=CARTESIAN_POINT('Ctrl Pts',(-4.16276217800006,5.2,-1.10002397800002));
#315342=CARTESIAN_POINT('Ctrl Pts',(-4.16276217800006,2.2,-1.10002397800002));
#315343=CARTESIAN_POINT('Ctrl Pts',(-4.16095903000006,12.2,-1.10024888400002));
#315344=CARTESIAN_POINT('Ctrl Pts',(-4.16095903000006,5.2,-1.10024888400002));
#315345=CARTESIAN_POINT('Ctrl Pts',(-4.16095903000006,2.2,-1.10024888400002));
#315346=CARTESIAN_POINT('Ctrl Pts',(-4.15915989500006,12.2,-1.10047122300001));
#315347=CARTESIAN_POINT('Ctrl Pts',(-4.15915989500006,5.2,-1.10047122300001));
#315348=CARTESIAN_POINT('Ctrl Pts',(-4.15915989500006,2.2,-1.10047122300001));
#315349=CARTESIAN_POINT('Ctrl Pts',(-4.15736478200006,12.2,-1.10069100400001));
#315350=CARTESIAN_POINT('Ctrl Pts',(-4.15736478200006,5.2,-1.10069100400001));
#315351=CARTESIAN_POINT('Ctrl Pts',(-4.15736478200006,2.2,-1.10069100400001));
#315352=CARTESIAN_POINT('Ctrl Pts',(-4.15557369900006,12.2,-1.10090823200002));
#315353=CARTESIAN_POINT('Ctrl Pts',(-4.15557369900006,5.2,-1.10090823200002));
#315354=CARTESIAN_POINT('Ctrl Pts',(-4.15557369900006,2.2,-1.10090823200002));
#315355=CARTESIAN_POINT('Ctrl Pts',(-4.15378665500006,12.2,-1.10112291800001));
#315356=CARTESIAN_POINT('Ctrl Pts',(-4.15378665500006,5.2,-1.10112291800001));
#315357=CARTESIAN_POINT('Ctrl Pts',(-4.15378665500006,2.2,-1.10112291800001));
#315358=CARTESIAN_POINT('Ctrl Pts',(-4.15200365900006,12.2,-1.10133506700001));
#315359=CARTESIAN_POINT('Ctrl Pts',(-4.15200365900006,5.2,-1.10133506700001));
#315360=CARTESIAN_POINT('Ctrl Pts',(-4.15200365900006,2.2,-1.10133506700001));
#315361=CARTESIAN_POINT('Ctrl Pts',(-4.15022472000006,12.2,-1.10154468900001));
#315362=CARTESIAN_POINT('Ctrl Pts',(-4.15022472000006,5.2,-1.10154468900001));
#315363=CARTESIAN_POINT('Ctrl Pts',(-4.15022472000006,2.2,-1.10154468900001));
#315364=CARTESIAN_POINT('Ctrl Pts',(-4.14844984500006,12.2,-1.10175179100001));
#315365=CARTESIAN_POINT('Ctrl Pts',(-4.14844984500006,5.2,-1.10175179100001));
#315366=CARTESIAN_POINT('Ctrl Pts',(-4.14844984500006,2.2,-1.10175179100001));
#315367=CARTESIAN_POINT('Ctrl Pts',(-4.14667904500006,12.2,-1.10195638100001));
#315368=CARTESIAN_POINT('Ctrl Pts',(-4.14667904500006,5.2,-1.10195638100001));
#315369=CARTESIAN_POINT('Ctrl Pts',(-4.14667904500006,2.2,-1.10195638100001));
#315370=CARTESIAN_POINT('Ctrl Pts',(-4.14491232900006,12.2,-1.10215846800001));
#315371=CARTESIAN_POINT('Ctrl Pts',(-4.14491232900006,5.2,-1.10215846800001));
#315372=CARTESIAN_POINT('Ctrl Pts',(-4.14491232900006,2.2,-1.10215846800001));
#315373=CARTESIAN_POINT('Ctrl Pts',(-4.14314970300006,12.2,-1.10235805800002));
#315374=CARTESIAN_POINT('Ctrl Pts',(-4.14314970300006,5.2,-1.10235805800002));
#315375=CARTESIAN_POINT('Ctrl Pts',(-4.14314970300006,2.2,-1.10235805800002));
#315376=CARTESIAN_POINT('Ctrl Pts',(-4.14139117900006,12.2,-1.10255516000001));
#315377=CARTESIAN_POINT('Ctrl Pts',(-4.14139117900006,5.2,-1.10255516000001));
#315378=CARTESIAN_POINT('Ctrl Pts',(-4.14139117900006,2.2,-1.10255516000001));
#315379=CARTESIAN_POINT('Ctrl Pts',(-4.13963676400006,12.2,-1.10274978300001));
#315380=CARTESIAN_POINT('Ctrl Pts',(-4.13963676400006,5.2,-1.10274978300001));
#315381=CARTESIAN_POINT('Ctrl Pts',(-4.13963676400006,2.2,-1.10274978300001));
#315382=CARTESIAN_POINT('Ctrl Pts',(-4.13788646700006,12.2,-1.10294193400001));
#315383=CARTESIAN_POINT('Ctrl Pts',(-4.13788646700006,5.2,-1.10294193400001));
#315384=CARTESIAN_POINT('Ctrl Pts',(-4.13788646700006,2.2,-1.10294193400001));
#315385=CARTESIAN_POINT('Ctrl Pts',(-4.13614029700006,12.2,-1.10313162300002));
#315386=CARTESIAN_POINT('Ctrl Pts',(-4.13614029700006,5.2,-1.10313162300002));
#315387=CARTESIAN_POINT('Ctrl Pts',(-4.13614029700006,2.2,-1.10313162300002));
#315388=CARTESIAN_POINT('Ctrl Pts',(-4.13439826300006,12.2,-1.10331885500001));
#315389=CARTESIAN_POINT('Ctrl Pts',(-4.13439826300006,5.2,-1.10331885500001));
#315390=CARTESIAN_POINT('Ctrl Pts',(-4.13439826300006,2.2,-1.10331885500001));
#315391=CARTESIAN_POINT('Ctrl Pts',(-4.13266037300006,12.2,-1.10350364000002));
#315392=CARTESIAN_POINT('Ctrl Pts',(-4.13266037300006,5.2,-1.10350364000002));
#315393=CARTESIAN_POINT('Ctrl Pts',(-4.13266037300006,2.2,-1.10350364000002));
#315394=CARTESIAN_POINT('Ctrl Pts',(-4.13092663700006,12.2,-1.10368598600001));
#315395=CARTESIAN_POINT('Ctrl Pts',(-4.13092663700006,5.2,-1.10368598600001));
#315396=CARTESIAN_POINT('Ctrl Pts',(-4.13092663700006,2.2,-1.10368598600001));
#315397=CARTESIAN_POINT('Ctrl Pts',(-4.12919706300006,12.2,-1.10386590200001));
#315398=CARTESIAN_POINT('Ctrl Pts',(-4.12919706300006,5.2,-1.10386590200001));
#315399=CARTESIAN_POINT('Ctrl Pts',(-4.12919706300006,2.2,-1.10386590200001));
#315400=CARTESIAN_POINT('Ctrl Pts',(-4.12747166000006,12.2,-1.10404339400001));
#315401=CARTESIAN_POINT('Ctrl Pts',(-4.12747166000006,5.2,-1.10404339400001));
#315402=CARTESIAN_POINT('Ctrl Pts',(-4.12747166000006,2.2,-1.10404339400001));
#315403=CARTESIAN_POINT('Ctrl Pts',(-4.12575043700006,12.2,-1.10421847200001));
#315404=CARTESIAN_POINT('Ctrl Pts',(-4.12575043700006,5.2,-1.10421847200001));
#315405=CARTESIAN_POINT('Ctrl Pts',(-4.12575043700006,2.2,-1.10421847200001));
#315406=CARTESIAN_POINT('Ctrl Pts',(-4.12403340300005,12.2,-1.10439114400001));
#315407=CARTESIAN_POINT('Ctrl Pts',(-4.12403340300005,5.2,-1.10439114400001));
#315408=CARTESIAN_POINT('Ctrl Pts',(-4.12403340300005,2.2,-1.10439114400001));
#315409=CARTESIAN_POINT('Ctrl Pts',(-4.12232056700006,12.2,-1.10456141800002));
#315410=CARTESIAN_POINT('Ctrl Pts',(-4.12232056700006,5.2,-1.10456141800002));
#315411=CARTESIAN_POINT('Ctrl Pts',(-4.12232056700006,2.2,-1.10456141800002));
#315412=CARTESIAN_POINT('Ctrl Pts',(-4.12061193700006,12.2,-1.10472930400002));
#315413=CARTESIAN_POINT('Ctrl Pts',(-4.12061193700006,5.2,-1.10472930400002));
#315414=CARTESIAN_POINT('Ctrl Pts',(-4.12061193700006,2.2,-1.10472930400002));
#315415=CARTESIAN_POINT('Ctrl Pts',(-4.11890752200006,12.2,-1.10489480800001));
#315416=CARTESIAN_POINT('Ctrl Pts',(-4.11890752200006,5.2,-1.10489480800001));
#315417=CARTESIAN_POINT('Ctrl Pts',(-4.11890752200006,2.2,-1.10489480800001));
#315418=CARTESIAN_POINT('Ctrl Pts',(-4.11720733200006,12.2,-1.10505794000002));
#315419=CARTESIAN_POINT('Ctrl Pts',(-4.11720733200006,5.2,-1.10505794000002));
#315420=CARTESIAN_POINT('Ctrl Pts',(-4.11720733200006,2.2,-1.10505794000002));
#315421=CARTESIAN_POINT('Ctrl Pts',(-4.11551137500005,12.2,-1.10521870600001));
#315422=CARTESIAN_POINT('Ctrl Pts',(-4.11551137500005,5.2,-1.10521870600001));
#315423=CARTESIAN_POINT('Ctrl Pts',(-4.11551137500005,2.2,-1.10521870600001));
#315424=CARTESIAN_POINT('Ctrl Pts',(-4.11381965900006,12.2,-1.10537711800001));
#315425=CARTESIAN_POINT('Ctrl Pts',(-4.11381965900006,5.2,-1.10537711800001));
#315426=CARTESIAN_POINT('Ctrl Pts',(-4.11381965900006,2.2,-1.10537711800001));
#315427=CARTESIAN_POINT('Ctrl Pts',(-4.11213219500006,12.2,-1.10553318300001));
#315428=CARTESIAN_POINT('Ctrl Pts',(-4.11213219500006,5.2,-1.10553318300001));
#315429=CARTESIAN_POINT('Ctrl Pts',(-4.11213219500006,2.2,-1.10553318300001));
#315430=CARTESIAN_POINT('Ctrl Pts',(-4.11044899000006,12.2,-1.10568690900001));
#315431=CARTESIAN_POINT('Ctrl Pts',(-4.11044899000006,5.2,-1.10568690900001));
#315432=CARTESIAN_POINT('Ctrl Pts',(-4.11044899000006,2.2,-1.10568690900001));
#315433=CARTESIAN_POINT('Ctrl Pts',(-4.10877005300006,12.2,-1.10583830500001));
#315434=CARTESIAN_POINT('Ctrl Pts',(-4.10877005300006,5.2,-1.10583830500001));
#315435=CARTESIAN_POINT('Ctrl Pts',(-4.10877005300006,2.2,-1.10583830500001));
#315436=CARTESIAN_POINT('Ctrl Pts',(-4.10709539400006,12.2,-1.10598737900002));
#315437=CARTESIAN_POINT('Ctrl Pts',(-4.10709539400006,5.2,-1.10598737900002));
#315438=CARTESIAN_POINT('Ctrl Pts',(-4.10709539400006,2.2,-1.10598737900002));
#315439=CARTESIAN_POINT('Ctrl Pts',(-4.10542502200006,12.2,-1.10613414000001));
#315440=CARTESIAN_POINT('Ctrl Pts',(-4.10542502200006,5.2,-1.10613414000001));
#315441=CARTESIAN_POINT('Ctrl Pts',(-4.10542502200006,2.2,-1.10613414000001));
#315442=CARTESIAN_POINT('Ctrl Pts',(-4.10375894400006,12.2,-1.10627859800001));
#315443=CARTESIAN_POINT('Ctrl Pts',(-4.10375894400006,5.2,-1.10627859800001));
#315444=CARTESIAN_POINT('Ctrl Pts',(-4.10375894400006,2.2,-1.10627859800001));
#315445=CARTESIAN_POINT('Ctrl Pts',(-4.10209717100006,12.2,-1.10642075900001));
#315446=CARTESIAN_POINT('Ctrl Pts',(-4.10209717100006,5.2,-1.10642075900001));
#315447=CARTESIAN_POINT('Ctrl Pts',(-4.10209717100006,2.2,-1.10642075900001));
#315448=CARTESIAN_POINT('Ctrl Pts',(-4.10043971100006,12.2,-1.10656063300001));
#315449=CARTESIAN_POINT('Ctrl Pts',(-4.10043971100006,5.2,-1.10656063300001));
#315450=CARTESIAN_POINT('Ctrl Pts',(-4.10043971100006,2.2,-1.10656063300001));
#315451=CARTESIAN_POINT('Ctrl Pts',(-4.09878657300006,12.2,-1.10669823000002));
#315452=CARTESIAN_POINT('Ctrl Pts',(-4.09878657300006,5.2,-1.10669823000002));
#315453=CARTESIAN_POINT('Ctrl Pts',(-4.09878657300006,2.2,-1.10669823000002));
#315454=CARTESIAN_POINT('Ctrl Pts',(-4.09713776600006,12.2,-1.10683355700001));
#315455=CARTESIAN_POINT('Ctrl Pts',(-4.09713776600006,5.2,-1.10683355700001));
#315456=CARTESIAN_POINT('Ctrl Pts',(-4.09713776600006,2.2,-1.10683355700001));
#315457=CARTESIAN_POINT('Ctrl Pts',(-4.09549329900006,12.2,-1.10696662200001));
#315458=CARTESIAN_POINT('Ctrl Pts',(-4.09549329900006,5.2,-1.10696662200001));
#315459=CARTESIAN_POINT('Ctrl Pts',(-4.09549329900006,2.2,-1.10696662200001));
#315460=CARTESIAN_POINT('Ctrl Pts',(-4.09385318100006,12.2,-1.10709743600002));
#315461=CARTESIAN_POINT('Ctrl Pts',(-4.09385318100006,5.2,-1.10709743600002));
#315462=CARTESIAN_POINT('Ctrl Pts',(-4.09385318100006,2.2,-1.10709743600002));
#315463=CARTESIAN_POINT('Ctrl Pts',(-4.09221742000006,12.2,-1.10722600800001));
#315464=CARTESIAN_POINT('Ctrl Pts',(-4.09221742000006,5.2,-1.10722600800001));
#315465=CARTESIAN_POINT('Ctrl Pts',(-4.09221742000006,2.2,-1.10722600800001));
#315466=CARTESIAN_POINT('Ctrl Pts',(-4.09058602500005,12.2,-1.10735234400002));
#315467=CARTESIAN_POINT('Ctrl Pts',(-4.09058602500005,5.2,-1.10735234400002));
#315468=CARTESIAN_POINT('Ctrl Pts',(-4.09058602500005,2.2,-1.10735234400002));
#315469=CARTESIAN_POINT('Ctrl Pts',(-4.08895900700006,12.2,-1.10747645600001));
#315470=CARTESIAN_POINT('Ctrl Pts',(-4.08895900700006,5.2,-1.10747645600001));
#315471=CARTESIAN_POINT('Ctrl Pts',(-4.08895900700006,2.2,-1.10747645600001));
#315472=CARTESIAN_POINT('Ctrl Pts',(-4.08733637300006,12.2,-1.10759835000001));
#315473=CARTESIAN_POINT('Ctrl Pts',(-4.08733637300006,5.2,-1.10759835000001));
#315474=CARTESIAN_POINT('Ctrl Pts',(-4.08733637300006,2.2,-1.10759835000001));
#315475=CARTESIAN_POINT('Ctrl Pts',(-4.08571813300005,12.2,-1.10771803800001));
#315476=CARTESIAN_POINT('Ctrl Pts',(-4.08571813300005,5.2,-1.10771803800001));
#315477=CARTESIAN_POINT('Ctrl Pts',(-4.08571813300005,2.2,-1.10771803800001));
#315478=CARTESIAN_POINT('Ctrl Pts',(-4.08410429500006,12.2,-1.10783552700001));
#315479=CARTESIAN_POINT('Ctrl Pts',(-4.08410429500006,5.2,-1.10783552700001));
#315480=CARTESIAN_POINT('Ctrl Pts',(-4.08410429500006,2.2,-1.10783552700001));
#315481=CARTESIAN_POINT('Ctrl Pts',(-4.08249486800006,12.2,-1.10795082600001));
#315482=CARTESIAN_POINT('Ctrl Pts',(-4.08249486800006,5.2,-1.10795082600001));
#315483=CARTESIAN_POINT('Ctrl Pts',(-4.08249486800006,2.2,-1.10795082600001));
#315484=CARTESIAN_POINT('Ctrl Pts',(-4.08088986100006,12.2,-1.10806394500001));
#315485=CARTESIAN_POINT('Ctrl Pts',(-4.08088986100006,5.2,-1.10806394500001));
#315486=CARTESIAN_POINT('Ctrl Pts',(-4.08088986100006,2.2,-1.10806394500001));
#315487=CARTESIAN_POINT('Ctrl Pts',(-4.07928928400006,12.2,-1.10817489300001));
#315488=CARTESIAN_POINT('Ctrl Pts',(-4.07928928400006,5.2,-1.10817489300001));
#315489=CARTESIAN_POINT('Ctrl Pts',(-4.07928928400006,2.2,-1.10817489300001));
#315490=CARTESIAN_POINT('Ctrl Pts',(-4.07769314600006,12.2,-1.10828367800002));
#315491=CARTESIAN_POINT('Ctrl Pts',(-4.07769314600006,5.2,-1.10828367800002));
#315492=CARTESIAN_POINT('Ctrl Pts',(-4.07769314600006,2.2,-1.10828367800002));
#315493=CARTESIAN_POINT('Ctrl Pts',(-4.07610145500006,12.2,-1.10839030900001));
#315494=CARTESIAN_POINT('Ctrl Pts',(-4.07610145500006,5.2,-1.10839030900001));
#315495=CARTESIAN_POINT('Ctrl Pts',(-4.07610145500006,2.2,-1.10839030900001));
#315496=CARTESIAN_POINT('Ctrl Pts',(-4.07451422000006,12.2,-1.10849479700001));
#315497=CARTESIAN_POINT('Ctrl Pts',(-4.07451422000006,5.2,-1.10849479700001));
#315498=CARTESIAN_POINT('Ctrl Pts',(-4.07451422000006,2.2,-1.10849479700001));
#315499=CARTESIAN_POINT('Ctrl Pts',(-4.07293145100006,12.2,-1.10859715000001));
#315500=CARTESIAN_POINT('Ctrl Pts',(-4.07293145100006,5.2,-1.10859715000001));
#315501=CARTESIAN_POINT('Ctrl Pts',(-4.07293145100006,2.2,-1.10859715000001));
#315502=CARTESIAN_POINT('Ctrl Pts',(-4.07135315500006,12.2,-1.10869737700002));
#315503=CARTESIAN_POINT('Ctrl Pts',(-4.07135315500006,5.2,-1.10869737700002));
#315504=CARTESIAN_POINT('Ctrl Pts',(-4.07135315500006,2.2,-1.10869737700002));
#315505=CARTESIAN_POINT('Ctrl Pts',(-4.06977934300006,12.2,-1.10879548800002));
#315506=CARTESIAN_POINT('Ctrl Pts',(-4.06977934300006,5.2,-1.10879548800002));
#315507=CARTESIAN_POINT('Ctrl Pts',(-4.06977934300006,2.2,-1.10879548800002));
#315508=CARTESIAN_POINT('Ctrl Pts',(-4.06821002300005,12.2,-1.10889149100001));
#315509=CARTESIAN_POINT('Ctrl Pts',(-4.06821002300005,5.2,-1.10889149100001));
#315510=CARTESIAN_POINT('Ctrl Pts',(-4.06821002300005,2.2,-1.10889149100001));
#315511=CARTESIAN_POINT('Ctrl Pts',(-4.06664520500006,12.2,-1.10898539700001));
#315512=CARTESIAN_POINT('Ctrl Pts',(-4.06664520500006,5.2,-1.10898539700001));
#315513=CARTESIAN_POINT('Ctrl Pts',(-4.06664520500006,2.2,-1.10898539700001));
#315514=CARTESIAN_POINT('Ctrl Pts',(-4.06508489700006,12.2,-1.10907721400002));
#315515=CARTESIAN_POINT('Ctrl Pts',(-4.06508489700006,5.2,-1.10907721400002));
#315516=CARTESIAN_POINT('Ctrl Pts',(-4.06508489700006,2.2,-1.10907721400002));
#315517=CARTESIAN_POINT('Ctrl Pts',(-4.06352910800006,12.2,-1.10916695200002));
#315518=CARTESIAN_POINT('Ctrl Pts',(-4.06352910800006,5.2,-1.10916695200002));
#315519=CARTESIAN_POINT('Ctrl Pts',(-4.06352910800006,2.2,-1.10916695200002));
#315520=CARTESIAN_POINT('Ctrl Pts',(-4.06197784800006,12.2,-1.10925462000001));
#315521=CARTESIAN_POINT('Ctrl Pts',(-4.06197784800006,5.2,-1.10925462000001));
#315522=CARTESIAN_POINT('Ctrl Pts',(-4.06197784800006,2.2,-1.10925462000001));
#315523=CARTESIAN_POINT('Ctrl Pts',(-4.06043112600006,12.2,-1.10934022800001));
#315524=CARTESIAN_POINT('Ctrl Pts',(-4.06043112600006,5.2,-1.10934022800001));
#315525=CARTESIAN_POINT('Ctrl Pts',(-4.06043112600006,2.2,-1.10934022800001));
#315526=CARTESIAN_POINT('Ctrl Pts',(-4.05888894900006,12.2,-1.10942378500001));
#315527=CARTESIAN_POINT('Ctrl Pts',(-4.05888894900006,5.2,-1.10942378500001));
#315528=CARTESIAN_POINT('Ctrl Pts',(-4.05888894900006,2.2,-1.10942378500001));
#315529=CARTESIAN_POINT('Ctrl Pts',(-4.05735132800006,12.2,-1.10950530000002));
#315530=CARTESIAN_POINT('Ctrl Pts',(-4.05735132800006,5.2,-1.10950530000002));
#315531=CARTESIAN_POINT('Ctrl Pts',(-4.05735132800006,2.2,-1.10950530000002));
#315532=CARTESIAN_POINT('Ctrl Pts',(-4.05581827300006,12.2,-1.10958478400002));
#315533=CARTESIAN_POINT('Ctrl Pts',(-4.05581827300006,5.2,-1.10958478400002));
#315534=CARTESIAN_POINT('Ctrl Pts',(-4.05581827300006,2.2,-1.10958478400002));
#315535=CARTESIAN_POINT('Ctrl Pts',(-4.05428979000006,12.2,-1.10966224400002));
#315536=CARTESIAN_POINT('Ctrl Pts',(-4.05428979000006,5.2,-1.10966224400002));
#315537=CARTESIAN_POINT('Ctrl Pts',(-4.05428979000006,2.2,-1.10966224400002));
#315538=CARTESIAN_POINT('Ctrl Pts',(-4.05276589100006,12.2,-1.10973769300001));
#315539=CARTESIAN_POINT('Ctrl Pts',(-4.05276589100006,5.2,-1.10973769300001));
#315540=CARTESIAN_POINT('Ctrl Pts',(-4.05276589100006,2.2,-1.10973769300001));
#315541=CARTESIAN_POINT('Ctrl Pts',(-4.05124658200006,12.2,-1.10981113800001));
#315542=CARTESIAN_POINT('Ctrl Pts',(-4.05124658200006,5.2,-1.10981113800001));
#315543=CARTESIAN_POINT('Ctrl Pts',(-4.05124658200006,2.2,-1.10981113800001));
#315544=CARTESIAN_POINT('Ctrl Pts',(-4.04973187600006,12.2,-1.10988258900001));
#315545=CARTESIAN_POINT('Ctrl Pts',(-4.04973187600006,5.2,-1.10988258900001));
#315546=CARTESIAN_POINT('Ctrl Pts',(-4.04973187600006,2.2,-1.10988258900001));
#315547=CARTESIAN_POINT('Ctrl Pts',(-4.04822177800006,12.2,-1.10995205700001));
#315548=CARTESIAN_POINT('Ctrl Pts',(-4.04822177800006,5.2,-1.10995205700001));
#315549=CARTESIAN_POINT('Ctrl Pts',(-4.04822177800006,2.2,-1.10995205700001));
#315550=CARTESIAN_POINT('Ctrl Pts',(-4.04671630000006,12.2,-1.11001955000001));
#315551=CARTESIAN_POINT('Ctrl Pts',(-4.04671630000006,5.2,-1.11001955000001));
#315552=CARTESIAN_POINT('Ctrl Pts',(-4.04671630000006,2.2,-1.11001955000001));
#315553=CARTESIAN_POINT('Ctrl Pts',(-4.04521545000006,12.2,-1.11008507900001));
#315554=CARTESIAN_POINT('Ctrl Pts',(-4.04521545000006,5.2,-1.11008507900001));
#315555=CARTESIAN_POINT('Ctrl Pts',(-4.04521545000006,2.2,-1.11008507900001));
#315556=CARTESIAN_POINT('Ctrl Pts',(-4.04371923700006,12.2,-1.11014865300001));
#315557=CARTESIAN_POINT('Ctrl Pts',(-4.04371923700006,5.2,-1.11014865300001));
#315558=CARTESIAN_POINT('Ctrl Pts',(-4.04371923700006,2.2,-1.11014865300001));
#315559=CARTESIAN_POINT('Ctrl Pts',(-4.04222767100006,12.2,-1.11021028300001));
#315560=CARTESIAN_POINT('Ctrl Pts',(-4.04222767100006,5.2,-1.11021028300001));
#315561=CARTESIAN_POINT('Ctrl Pts',(-4.04222767100006,2.2,-1.11021028300001));
#315562=CARTESIAN_POINT('Ctrl Pts',(-4.04074075900006,12.2,-1.11026997800002));
#315563=CARTESIAN_POINT('Ctrl Pts',(-4.04074075900006,5.2,-1.11026997800002));
#315564=CARTESIAN_POINT('Ctrl Pts',(-4.04074075900006,2.2,-1.11026997800002));
#315565=CARTESIAN_POINT('Ctrl Pts',(-4.03925851300006,12.2,-1.11032774700002));
#315566=CARTESIAN_POINT('Ctrl Pts',(-4.03925851300006,5.2,-1.11032774700002));
#315567=CARTESIAN_POINT('Ctrl Pts',(-4.03925851300006,2.2,-1.11032774700002));
#315568=CARTESIAN_POINT('Ctrl Pts',(-4.03778093900006,12.2,-1.11038360000002));
#315569=CARTESIAN_POINT('Ctrl Pts',(-4.03778093900006,5.2,-1.11038360000002));
#315570=CARTESIAN_POINT('Ctrl Pts',(-4.03778093900006,2.2,-1.11038360000002));
#315571=CARTESIAN_POINT('Ctrl Pts',(-4.03630804900006,12.2,-1.11043754800002));
#315572=CARTESIAN_POINT('Ctrl Pts',(-4.03630804900006,5.2,-1.11043754800002));
#315573=CARTESIAN_POINT('Ctrl Pts',(-4.03630804900006,2.2,-1.11043754800002));
#315574=CARTESIAN_POINT('Ctrl Pts',(-4.03483985100006,12.2,-1.11048960100002));
#315575=CARTESIAN_POINT('Ctrl Pts',(-4.03483985100006,5.2,-1.11048960100002));
#315576=CARTESIAN_POINT('Ctrl Pts',(-4.03483985100006,2.2,-1.11048960100002));
#315577=CARTESIAN_POINT('Ctrl Pts',(-4.03337635300006,12.2,-1.11053976900001));
#315578=CARTESIAN_POINT('Ctrl Pts',(-4.03337635300006,5.2,-1.11053976900001));
#315579=CARTESIAN_POINT('Ctrl Pts',(-4.03337635300006,2.2,-1.11053976900001));
#315580=CARTESIAN_POINT('Ctrl Pts',(-4.03191756600005,12.2,-1.11058806100001));
#315581=CARTESIAN_POINT('Ctrl Pts',(-4.03191756600005,5.2,-1.11058806100001));
#315582=CARTESIAN_POINT('Ctrl Pts',(-4.03191756600005,2.2,-1.11058806100001));
#315583=CARTESIAN_POINT('Ctrl Pts',(-4.03046349700006,12.2,-1.11063448800001));
#315584=CARTESIAN_POINT('Ctrl Pts',(-4.03046349700006,5.2,-1.11063448800001));
#315585=CARTESIAN_POINT('Ctrl Pts',(-4.03046349700006,2.2,-1.11063448800001));
#315586=CARTESIAN_POINT('Ctrl Pts',(-4.02901415800006,12.2,-1.11067905900001));
#315587=CARTESIAN_POINT('Ctrl Pts',(-4.02901415800006,5.2,-1.11067905900001));
#315588=CARTESIAN_POINT('Ctrl Pts',(-4.02901415800006,2.2,-1.11067905900001));
#315589=CARTESIAN_POINT('Ctrl Pts',(-4.02756955500006,12.2,-1.11072178500002));
#315590=CARTESIAN_POINT('Ctrl Pts',(-4.02756955500006,5.2,-1.11072178500002));
#315591=CARTESIAN_POINT('Ctrl Pts',(-4.02756955500006,2.2,-1.11072178500002));
#315592=CARTESIAN_POINT('Ctrl Pts',(-4.02612970000006,12.2,-1.11076267600001));
#315593=CARTESIAN_POINT('Ctrl Pts',(-4.02612970000006,5.2,-1.11076267600001));
#315594=CARTESIAN_POINT('Ctrl Pts',(-4.02612970000006,2.2,-1.11076267600001));
#315595=CARTESIAN_POINT('Ctrl Pts',(-4.02469460000006,12.2,-1.11080174300001));
#315596=CARTESIAN_POINT('Ctrl Pts',(-4.02469460000006,5.2,-1.11080174300001));
#315597=CARTESIAN_POINT('Ctrl Pts',(-4.02469460000006,2.2,-1.11080174300001));
#315598=CARTESIAN_POINT('Ctrl Pts',(-4.02326426600006,12.2,-1.11083899500001));
#315599=CARTESIAN_POINT('Ctrl Pts',(-4.02326426600006,5.2,-1.11083899500001));
#315600=CARTESIAN_POINT('Ctrl Pts',(-4.02326426600006,2.2,-1.11083899500001));
#315601=CARTESIAN_POINT('Ctrl Pts',(-4.02183870500005,12.2,-1.11087444200002));
#315602=CARTESIAN_POINT('Ctrl Pts',(-4.02183870500005,5.2,-1.11087444200002));
#315603=CARTESIAN_POINT('Ctrl Pts',(-4.02183870500005,2.2,-1.11087444200002));
#315604=CARTESIAN_POINT('Ctrl Pts',(-4.02041792900006,12.2,-1.11090809600002));
#315605=CARTESIAN_POINT('Ctrl Pts',(-4.02041792900006,5.2,-1.11090809600002));
#315606=CARTESIAN_POINT('Ctrl Pts',(-4.02041792900006,2.2,-1.11090809600002));
#315607=CARTESIAN_POINT('Ctrl Pts',(-4.01900194400006,12.2,-1.11093996500002));
#315608=CARTESIAN_POINT('Ctrl Pts',(-4.01900194400006,5.2,-1.11093996500002));
#315609=CARTESIAN_POINT('Ctrl Pts',(-4.01900194400006,2.2,-1.11093996500002));
#315610=CARTESIAN_POINT('Ctrl Pts',(-4.01759076100006,12.2,-1.11097006100001));
#315611=CARTESIAN_POINT('Ctrl Pts',(-4.01759076100006,5.2,-1.11097006100001));
#315612=CARTESIAN_POINT('Ctrl Pts',(-4.01759076100006,2.2,-1.11097006100001));
#315613=CARTESIAN_POINT('Ctrl Pts',(-4.01618439000006,12.2,-1.11099839500001));
#315614=CARTESIAN_POINT('Ctrl Pts',(-4.01618439000006,5.2,-1.11099839500001));
#315615=CARTESIAN_POINT('Ctrl Pts',(-4.01618439000006,2.2,-1.11099839500001));
#315616=CARTESIAN_POINT('Ctrl Pts',(-4.01478283800006,12.2,-1.11102497500001));
#315617=CARTESIAN_POINT('Ctrl Pts',(-4.01478283800006,5.2,-1.11102497500001));
#315618=CARTESIAN_POINT('Ctrl Pts',(-4.01478283800006,2.2,-1.11102497500001));
#315619=CARTESIAN_POINT('Ctrl Pts',(-4.01338611600006,12.2,-1.11104981400001));
#315620=CARTESIAN_POINT('Ctrl Pts',(-4.01338611600006,5.2,-1.11104981400001));
#315621=CARTESIAN_POINT('Ctrl Pts',(-4.01338611600006,2.2,-1.11104981400001));
#315622=CARTESIAN_POINT('Ctrl Pts',(-4.01199423300006,12.2,-1.11107292100002));
#315623=CARTESIAN_POINT('Ctrl Pts',(-4.01199423300006,5.2,-1.11107292100002));
#315624=CARTESIAN_POINT('Ctrl Pts',(-4.01199423300006,2.2,-1.11107292100002));
#315625=CARTESIAN_POINT('Ctrl Pts',(-4.01060719700006,12.2,-1.11109430700001));
#315626=CARTESIAN_POINT('Ctrl Pts',(-4.01060719700006,5.2,-1.11109430700001));
#315627=CARTESIAN_POINT('Ctrl Pts',(-4.01060719700006,2.2,-1.11109430700001));
#315628=CARTESIAN_POINT('Ctrl Pts',(-4.00922501800006,12.2,-1.11111398200002));
#315629=CARTESIAN_POINT('Ctrl Pts',(-4.00922501800006,5.2,-1.11111398200002));
#315630=CARTESIAN_POINT('Ctrl Pts',(-4.00922501800006,2.2,-1.11111398200002));
#315631=CARTESIAN_POINT('Ctrl Pts',(-4.00784770600006,12.2,-1.11113195800002));
#315632=CARTESIAN_POINT('Ctrl Pts',(-4.00784770600006,5.2,-1.11113195800002));
#315633=CARTESIAN_POINT('Ctrl Pts',(-4.00784770600006,2.2,-1.11113195800002));
#315634=CARTESIAN_POINT('Ctrl Pts',(-4.00647526900006,12.2,-1.11114824400001));
#315635=CARTESIAN_POINT('Ctrl Pts',(-4.00647526900006,5.2,-1.11114824400001));
#315636=CARTESIAN_POINT('Ctrl Pts',(-4.00647526900006,2.2,-1.11114824400001));
#315637=CARTESIAN_POINT('Ctrl Pts',(-4.00510771600006,12.2,-1.11116285100001));
#315638=CARTESIAN_POINT('Ctrl Pts',(-4.00510771600006,5.2,-1.11116285100001));
#315639=CARTESIAN_POINT('Ctrl Pts',(-4.00510771600006,2.2,-1.11116285100001));
#315640=CARTESIAN_POINT('Ctrl Pts',(-4.00374505900006,12.2,-1.11117579000001));
#315641=CARTESIAN_POINT('Ctrl Pts',(-4.00374505900006,5.2,-1.11117579000001));
#315642=CARTESIAN_POINT('Ctrl Pts',(-4.00374505900006,2.2,-1.11117579000001));
#315643=CARTESIAN_POINT('Ctrl Pts',(-4.00238730300006,12.2,-1.11118707300002));
#315644=CARTESIAN_POINT('Ctrl Pts',(-4.00238730300006,5.2,-1.11118707300002));
#315645=CARTESIAN_POINT('Ctrl Pts',(-4.00238730300006,2.2,-1.11118707300002));
#315646=CARTESIAN_POINT('Ctrl Pts',(-4.00103446000006,12.2,-1.11119670800001));
#315647=CARTESIAN_POINT('Ctrl Pts',(-4.00103446000006,5.2,-1.11119670800001));
#315648=CARTESIAN_POINT('Ctrl Pts',(-4.00103446000006,2.2,-1.11119670800001));
#315649=CARTESIAN_POINT('Ctrl Pts',(-3.99968653900006,12.2,-1.11120470900001));
#315650=CARTESIAN_POINT('Ctrl Pts',(-3.99968653900006,5.2,-1.11120470900001));
#315651=CARTESIAN_POINT('Ctrl Pts',(-3.99968653900006,2.2,-1.11120470900001));
#315652=CARTESIAN_POINT('Ctrl Pts',(-3.99834355000006,12.2,-1.11121108400001));
#315653=CARTESIAN_POINT('Ctrl Pts',(-3.99834355000006,5.2,-1.11121108400001));
#315654=CARTESIAN_POINT('Ctrl Pts',(-3.99834355000006,2.2,-1.11121108400001));
#315655=CARTESIAN_POINT('Ctrl Pts',(-3.99700550100006,12.2,-1.11121584600001));
#315656=CARTESIAN_POINT('Ctrl Pts',(-3.99700550100006,5.2,-1.11121584600001));
#315657=CARTESIAN_POINT('Ctrl Pts',(-3.99700550100006,2.2,-1.11121584600001));
#315658=CARTESIAN_POINT('Ctrl Pts',(-3.99567240100006,12.2,-1.11121900500001));
#315659=CARTESIAN_POINT('Ctrl Pts',(-3.99567240100006,5.2,-1.11121900500001));
#315660=CARTESIAN_POINT('Ctrl Pts',(-3.99567240100006,2.2,-1.11121900500001));
#315661=CARTESIAN_POINT('Ctrl Pts',(-3.99434425900006,12.2,-1.11122057100001));
#315662=CARTESIAN_POINT('Ctrl Pts',(-3.99434425900006,5.2,-1.11122057100001));
#315663=CARTESIAN_POINT('Ctrl Pts',(-3.99434425900006,2.2,-1.11122057100001));
#315664=CARTESIAN_POINT('Ctrl Pts',(-3.99302108600006,12.2,-1.11122055600001));
#315665=CARTESIAN_POINT('Ctrl Pts',(-3.99302108600006,5.2,-1.11122055600001));
#315666=CARTESIAN_POINT('Ctrl Pts',(-3.99302108600006,2.2,-1.11122055600001));
#315667=CARTESIAN_POINT('Ctrl Pts',(-3.99170289000006,12.2,-1.11121897100002));
#315668=CARTESIAN_POINT('Ctrl Pts',(-3.99170289000006,5.2,-1.11121897100002));
#315669=CARTESIAN_POINT('Ctrl Pts',(-3.99170289000006,2.2,-1.11121897100002));
#315670=CARTESIAN_POINT('Ctrl Pts',(-3.99038968100006,12.2,-1.11121582800001));
#315671=CARTESIAN_POINT('Ctrl Pts',(-3.99038968100006,5.2,-1.11121582800001));
#315672=CARTESIAN_POINT('Ctrl Pts',(-3.99038968100006,2.2,-1.11121582800001));
#315673=CARTESIAN_POINT('Ctrl Pts',(-3.98908146900006,12.2,-1.11121113600001));
#315674=CARTESIAN_POINT('Ctrl Pts',(-3.98908146900006,5.2,-1.11121113600001));
#315675=CARTESIAN_POINT('Ctrl Pts',(-3.98908146900006,2.2,-1.11121113600001));
#315676=CARTESIAN_POINT('Ctrl Pts',(-3.98777826100006,12.2,-1.11120490800001));
#315677=CARTESIAN_POINT('Ctrl Pts',(-3.98777826100006,5.2,-1.11120490800001));
#315678=CARTESIAN_POINT('Ctrl Pts',(-3.98777826100006,2.2,-1.11120490800001));
#315679=CARTESIAN_POINT('Ctrl Pts',(-3.98648006800006,12.2,-1.11119715400001));
#315680=CARTESIAN_POINT('Ctrl Pts',(-3.98648006800006,5.2,-1.11119715400001));
#315681=CARTESIAN_POINT('Ctrl Pts',(-3.98648006800006,2.2,-1.11119715400001));
#315682=CARTESIAN_POINT('Ctrl Pts',(-3.98518690000006,12.2,-1.11118788500002));
#315683=CARTESIAN_POINT('Ctrl Pts',(-3.98518690000006,5.2,-1.11118788500002));
#315684=CARTESIAN_POINT('Ctrl Pts',(-3.98518690000006,2.2,-1.11118788500002));
#315685=CARTESIAN_POINT('Ctrl Pts',(-3.98389876500006,12.2,-1.11117711500002));
#315686=CARTESIAN_POINT('Ctrl Pts',(-3.98389876500006,5.2,-1.11117711500002));
#315687=CARTESIAN_POINT('Ctrl Pts',(-3.98389876500006,2.2,-1.11117711500002));
#315688=CARTESIAN_POINT('Ctrl Pts',(-3.98261567100006,12.2,-1.11116485000001));
#315689=CARTESIAN_POINT('Ctrl Pts',(-3.98261567100006,5.2,-1.11116485000001));
#315690=CARTESIAN_POINT('Ctrl Pts',(-3.98261567100006,2.2,-1.11116485000001));
#315691=CARTESIAN_POINT('Ctrl Pts',(-3.98133763100006,12.2,-1.11115110700001));
#315692=CARTESIAN_POINT('Ctrl Pts',(-3.98133763100006,5.2,-1.11115110700001));
#315693=CARTESIAN_POINT('Ctrl Pts',(-3.98133763100006,2.2,-1.11115110700001));
#315694=CARTESIAN_POINT('Ctrl Pts',(-3.98006465200006,12.2,-1.11113589400002));
#315695=CARTESIAN_POINT('Ctrl Pts',(-3.98006465200006,5.2,-1.11113589400002));
#315696=CARTESIAN_POINT('Ctrl Pts',(-3.98006465200006,2.2,-1.11113589400002));
#315697=CARTESIAN_POINT('Ctrl Pts',(-3.97879674300006,12.2,-1.11111922300001));
#315698=CARTESIAN_POINT('Ctrl Pts',(-3.97879674300006,5.2,-1.11111922300001));
#315699=CARTESIAN_POINT('Ctrl Pts',(-3.97879674300006,2.2,-1.11111922300001));
#315700=CARTESIAN_POINT('Ctrl Pts',(-3.97753391400006,12.2,-1.11110110600002));
#315701=CARTESIAN_POINT('Ctrl Pts',(-3.97753391400006,5.2,-1.11110110600002));
#315702=CARTESIAN_POINT('Ctrl Pts',(-3.97753391400006,2.2,-1.11110110600002));
#315703=CARTESIAN_POINT('Ctrl Pts',(-3.97627617500006,12.2,-1.11108155300002));
#315704=CARTESIAN_POINT('Ctrl Pts',(-3.97627617500006,5.2,-1.11108155300002));
#315705=CARTESIAN_POINT('Ctrl Pts',(-3.97627617500006,2.2,-1.11108155300002));
#315706=CARTESIAN_POINT('Ctrl Pts',(-3.97502353500006,12.2,-1.11106057800002));
#315707=CARTESIAN_POINT('Ctrl Pts',(-3.97502353500006,5.2,-1.11106057800002));
#315708=CARTESIAN_POINT('Ctrl Pts',(-3.97502353500006,2.2,-1.11106057800002));
#315709=CARTESIAN_POINT('Ctrl Pts',(-3.97377600200006,12.2,-1.11103819100002));
#315710=CARTESIAN_POINT('Ctrl Pts',(-3.97377600200006,5.2,-1.11103819100002));
#315711=CARTESIAN_POINT('Ctrl Pts',(-3.97377600200006,2.2,-1.11103819100002));
#315712=CARTESIAN_POINT('Ctrl Pts',(-3.97253358800006,12.2,-1.11101440300001));
#315713=CARTESIAN_POINT('Ctrl Pts',(-3.97253358800006,5.2,-1.11101440300001));
#315714=CARTESIAN_POINT('Ctrl Pts',(-3.97253358800006,2.2,-1.11101440300001));
#315715=CARTESIAN_POINT('Ctrl Pts',(-3.97129630100006,12.2,-1.11098922600001));
#315716=CARTESIAN_POINT('Ctrl Pts',(-3.97129630100006,5.2,-1.11098922600001));
#315717=CARTESIAN_POINT('Ctrl Pts',(-3.97129630100006,2.2,-1.11098922600001));
#315718=CARTESIAN_POINT('Ctrl Pts',(-3.97006415000006,12.2,-1.11096267300002));
#315719=CARTESIAN_POINT('Ctrl Pts',(-3.97006415000006,5.2,-1.11096267300002));
#315720=CARTESIAN_POINT('Ctrl Pts',(-3.97006415000006,2.2,-1.11096267300002));
#315721=CARTESIAN_POINT('Ctrl Pts',(-3.96883714400006,12.2,-1.11093475400001));
#315722=CARTESIAN_POINT('Ctrl Pts',(-3.96883714400006,5.2,-1.11093475400001));
#315723=CARTESIAN_POINT('Ctrl Pts',(-3.96883714400006,2.2,-1.11093475400001));
#315724=CARTESIAN_POINT('Ctrl Pts',(-3.96761529400006,12.2,-1.11090548200002));
#315725=CARTESIAN_POINT('Ctrl Pts',(-3.96761529400006,5.2,-1.11090548200002));
#315726=CARTESIAN_POINT('Ctrl Pts',(-3.96761529400006,2.2,-1.11090548200002));
#315727=CARTESIAN_POINT('Ctrl Pts',(-3.96639860800006,12.2,-1.11087486800002));
#315728=CARTESIAN_POINT('Ctrl Pts',(-3.96639860800006,5.2,-1.11087486800002));
#315729=CARTESIAN_POINT('Ctrl Pts',(-3.96639860800006,2.2,-1.11087486800002));
#315730=CARTESIAN_POINT('Ctrl Pts',(-3.96518709600006,12.2,-1.11084292400002));
#315731=CARTESIAN_POINT('Ctrl Pts',(-3.96518709600006,5.2,-1.11084292400002));
#315732=CARTESIAN_POINT('Ctrl Pts',(-3.96518709600006,2.2,-1.11084292400002));
#315733=CARTESIAN_POINT('Ctrl Pts',(-3.96398076800006,12.2,-1.11080966100001));
#315734=CARTESIAN_POINT('Ctrl Pts',(-3.96398076800006,5.2,-1.11080966100001));
#315735=CARTESIAN_POINT('Ctrl Pts',(-3.96398076800006,2.2,-1.11080966100001));
#315736=CARTESIAN_POINT('Ctrl Pts',(-3.96277963300006,12.2,-1.11077509300001));
#315737=CARTESIAN_POINT('Ctrl Pts',(-3.96277963300006,5.2,-1.11077509300001));
#315738=CARTESIAN_POINT('Ctrl Pts',(-3.96277963300006,2.2,-1.11077509300001));
#315739=CARTESIAN_POINT('Ctrl Pts',(-3.96158370000006,12.2,-1.11073923000002));
#315740=CARTESIAN_POINT('Ctrl Pts',(-3.96158370000006,5.2,-1.11073923000002));
#315741=CARTESIAN_POINT('Ctrl Pts',(-3.96158370000006,2.2,-1.11073923000002));
#315742=CARTESIAN_POINT('Ctrl Pts',(-3.96039297900006,12.2,-1.11070208500001));
#315743=CARTESIAN_POINT('Ctrl Pts',(-3.96039297900006,5.2,-1.11070208500001));
#315744=CARTESIAN_POINT('Ctrl Pts',(-3.96039297900006,2.2,-1.11070208500001));
#315745=CARTESIAN_POINT('Ctrl Pts',(-3.95920747900006,12.2,-1.11066367000001));
#315746=CARTESIAN_POINT('Ctrl Pts',(-3.95920747900006,5.2,-1.11066367000001));
#315747=CARTESIAN_POINT('Ctrl Pts',(-3.95920747900006,2.2,-1.11066367000001));
#315748=CARTESIAN_POINT('Ctrl Pts',(-3.95802721000006,12.2,-1.11062399600002));
#315749=CARTESIAN_POINT('Ctrl Pts',(-3.95802721000006,5.2,-1.11062399600002));
#315750=CARTESIAN_POINT('Ctrl Pts',(-3.95802721000006,2.2,-1.11062399600002));
#315751=CARTESIAN_POINT('Ctrl Pts',(-3.95685218100006,12.2,-1.11058307600001));
#315752=CARTESIAN_POINT('Ctrl Pts',(-3.95685218100006,5.2,-1.11058307600001));
#315753=CARTESIAN_POINT('Ctrl Pts',(-3.95685218100006,2.2,-1.11058307600001));
#315754=CARTESIAN_POINT('Ctrl Pts',(-3.95568240100006,12.2,-1.11054092200002));
#315755=CARTESIAN_POINT('Ctrl Pts',(-3.95568240100006,5.2,-1.11054092200002));
#315756=CARTESIAN_POINT('Ctrl Pts',(-3.95568240100006,2.2,-1.11054092200002));
#315757=CARTESIAN_POINT('Ctrl Pts',(-3.95451788100006,12.2,-1.11049754700002));
#315758=CARTESIAN_POINT('Ctrl Pts',(-3.95451788100006,5.2,-1.11049754700002));
#315759=CARTESIAN_POINT('Ctrl Pts',(-3.95451788100006,2.2,-1.11049754700002));
#315760=CARTESIAN_POINT('Ctrl Pts',(-3.95335862900006,12.2,-1.11045296100002));
#315761=CARTESIAN_POINT('Ctrl Pts',(-3.95335862900006,5.2,-1.11045296100002));
#315762=CARTESIAN_POINT('Ctrl Pts',(-3.95335862900006,2.2,-1.11045296100002));
#315763=CARTESIAN_POINT('Ctrl Pts',(-3.95220465600006,12.2,-1.11040717800002));
#315764=CARTESIAN_POINT('Ctrl Pts',(-3.95220465600006,5.2,-1.11040717800002));
#315765=CARTESIAN_POINT('Ctrl Pts',(-3.95220465600006,2.2,-1.11040717800002));
#315766=CARTESIAN_POINT('Ctrl Pts',(-3.95105597100006,12.2,-1.11036021000002));
#315767=CARTESIAN_POINT('Ctrl Pts',(-3.95105597100006,5.2,-1.11036021000002));
#315768=CARTESIAN_POINT('Ctrl Pts',(-3.95105597100006,2.2,-1.11036021000002));
#315769=CARTESIAN_POINT('Ctrl Pts',(-3.94991258100006,12.2,-1.11031207000002));
#315770=CARTESIAN_POINT('Ctrl Pts',(-3.94991258100006,5.2,-1.11031207000002));
#315771=CARTESIAN_POINT('Ctrl Pts',(-3.94991258100006,2.2,-1.11031207000002));
#315772=CARTESIAN_POINT('Ctrl Pts',(-3.94877449900005,12.2,-1.11026276800001));
#315773=CARTESIAN_POINT('Ctrl Pts',(-3.94877449900005,5.2,-1.11026276800001));
#315774=CARTESIAN_POINT('Ctrl Pts',(-3.94877449900005,2.2,-1.11026276800001));
#315775=CARTESIAN_POINT('Ctrl Pts',(-3.94764173200006,12.2,-1.11021232000001));
#315776=CARTESIAN_POINT('Ctrl Pts',(-3.94764173200006,5.2,-1.11021232000001));
#315777=CARTESIAN_POINT('Ctrl Pts',(-3.94764173200006,2.2,-1.11021232000001));
#315778=CARTESIAN_POINT('Ctrl Pts',(-3.94651429200006,12.2,-1.11016073500001));
#315779=CARTESIAN_POINT('Ctrl Pts',(-3.94651429200006,5.2,-1.11016073500001));
#315780=CARTESIAN_POINT('Ctrl Pts',(-3.94651429200006,2.2,-1.11016073500001));
#315781=CARTESIAN_POINT('Ctrl Pts',(-3.94539218700006,12.2,-1.11010802800001));
#315782=CARTESIAN_POINT('Ctrl Pts',(-3.94539218700006,5.2,-1.11010802800001));
#315783=CARTESIAN_POINT('Ctrl Pts',(-3.94539218700006,2.2,-1.11010802800001));
#315784=CARTESIAN_POINT('Ctrl Pts',(-3.94427542600006,12.2,-1.11005421000002));
#315785=CARTESIAN_POINT('Ctrl Pts',(-3.94427542600006,5.2,-1.11005421000002));
#315786=CARTESIAN_POINT('Ctrl Pts',(-3.94427542600006,2.2,-1.11005421000002));
#315787=CARTESIAN_POINT('Ctrl Pts',(-3.94316401900006,12.2,-1.10999929400001));
#315788=CARTESIAN_POINT('Ctrl Pts',(-3.94316401900006,5.2,-1.10999929400001));
#315789=CARTESIAN_POINT('Ctrl Pts',(-3.94316401900006,2.2,-1.10999929400001));
#315790=CARTESIAN_POINT('Ctrl Pts',(-3.94205797700006,12.2,-1.10994329300001));
#315791=CARTESIAN_POINT('Ctrl Pts',(-3.94205797700006,5.2,-1.10994329300001));
#315792=CARTESIAN_POINT('Ctrl Pts',(-3.94205797700006,2.2,-1.10994329300001));
#315793=CARTESIAN_POINT('Ctrl Pts',(-3.94095730800006,12.2,-1.10988622000002));
#315794=CARTESIAN_POINT('Ctrl Pts',(-3.94095730800006,5.2,-1.10988622000002));
#315795=CARTESIAN_POINT('Ctrl Pts',(-3.94095730800006,2.2,-1.10988622000002));
#315796=CARTESIAN_POINT('Ctrl Pts',(-3.93986202200006,12.2,-1.10982808600002));
#315797=CARTESIAN_POINT('Ctrl Pts',(-3.93986202200006,5.2,-1.10982808600002));
#315798=CARTESIAN_POINT('Ctrl Pts',(-3.93986202200006,2.2,-1.10982808600002));
#315799=CARTESIAN_POINT('Ctrl Pts',(-3.93877212800006,12.2,-1.10976890700002));
#315800=CARTESIAN_POINT('Ctrl Pts',(-3.93877212800006,5.2,-1.10976890700002));
#315801=CARTESIAN_POINT('Ctrl Pts',(-3.93877212800006,2.2,-1.10976890700002));
#315802=CARTESIAN_POINT('Ctrl Pts',(-3.93768763600006,12.2,-1.10970869100001));
#315803=CARTESIAN_POINT('Ctrl Pts',(-3.93768763600006,5.2,-1.10970869100001));
#315804=CARTESIAN_POINT('Ctrl Pts',(-3.93768763600006,2.2,-1.10970869100001));
#315805=CARTESIAN_POINT('Ctrl Pts',(-3.93660855600006,12.2,-1.10964745600001));
#315806=CARTESIAN_POINT('Ctrl Pts',(-3.93660855600006,5.2,-1.10964745600001));
#315807=CARTESIAN_POINT('Ctrl Pts',(-3.93660855600006,2.2,-1.10964745600001));
#315808=CARTESIAN_POINT('Ctrl Pts',(-3.93553489700006,12.2,-1.10958521100001));
#315809=CARTESIAN_POINT('Ctrl Pts',(-3.93553489700006,5.2,-1.10958521100001));
#315810=CARTESIAN_POINT('Ctrl Pts',(-3.93553489700006,2.2,-1.10958521100001));
#315811=CARTESIAN_POINT('Ctrl Pts',(-3.93446666900005,12.2,-1.10952197100001));
#315812=CARTESIAN_POINT('Ctrl Pts',(-3.93446666900005,5.2,-1.10952197100001));
#315813=CARTESIAN_POINT('Ctrl Pts',(-3.93446666900005,2.2,-1.10952197100001));
#315814=CARTESIAN_POINT('Ctrl Pts',(-3.93340388200006,12.2,-1.10945774800001));
#315815=CARTESIAN_POINT('Ctrl Pts',(-3.93340388200006,5.2,-1.10945774800001));
#315816=CARTESIAN_POINT('Ctrl Pts',(-3.93340388200006,2.2,-1.10945774800001));
#315817=CARTESIAN_POINT('Ctrl Pts',(-3.93234654400006,12.2,-1.10939255600002));
#315818=CARTESIAN_POINT('Ctrl Pts',(-3.93234654400006,5.2,-1.10939255600002));
#315819=CARTESIAN_POINT('Ctrl Pts',(-3.93234654400006,2.2,-1.10939255600002));
#315820=CARTESIAN_POINT('Ctrl Pts',(-3.93129466700006,12.2,-1.10932640700002));
#315821=CARTESIAN_POINT('Ctrl Pts',(-3.93129466700006,5.2,-1.10932640700002));
#315822=CARTESIAN_POINT('Ctrl Pts',(-3.93129466700006,2.2,-1.10932640700002));
#315823=CARTESIAN_POINT('Ctrl Pts',(-3.93024825700006,12.2,-1.10925931500002));
#315824=CARTESIAN_POINT('Ctrl Pts',(-3.93024825700006,5.2,-1.10925931500002));
#315825=CARTESIAN_POINT('Ctrl Pts',(-3.93024825700006,2.2,-1.10925931500002));
#315826=CARTESIAN_POINT('Ctrl Pts',(-3.92920732800006,12.2,-1.10919129200001));
#315827=CARTESIAN_POINT('Ctrl Pts',(-3.92920732800006,5.2,-1.10919129200001));
#315828=CARTESIAN_POINT('Ctrl Pts',(-3.92920732800006,2.2,-1.10919129200001));
#315829=CARTESIAN_POINT('Ctrl Pts',(-3.92817188800006,12.2,-1.10912235300002));
#315830=CARTESIAN_POINT('Ctrl Pts',(-3.92817188800006,5.2,-1.10912235300002));
#315831=CARTESIAN_POINT('Ctrl Pts',(-3.92817188800006,2.2,-1.10912235300002));
#315832=CARTESIAN_POINT('Ctrl Pts',(-3.92714194400006,12.2,-1.10905250900001));
#315833=CARTESIAN_POINT('Ctrl Pts',(-3.92714194400006,5.2,-1.10905250900001));
#315834=CARTESIAN_POINT('Ctrl Pts',(-3.92714194400006,2.2,-1.10905250900001));
#315835=CARTESIAN_POINT('Ctrl Pts',(-3.92611750900006,12.2,-1.10898177600002));
#315836=CARTESIAN_POINT('Ctrl Pts',(-3.92611750900006,5.2,-1.10898177600002));
#315837=CARTESIAN_POINT('Ctrl Pts',(-3.92611750900006,2.2,-1.10898177600002));
#315838=CARTESIAN_POINT('Ctrl Pts',(-3.92509859200006,12.2,-1.10891016400001));
#315839=CARTESIAN_POINT('Ctrl Pts',(-3.92509859200006,5.2,-1.10891016400001));
#315840=CARTESIAN_POINT('Ctrl Pts',(-3.92509859200006,2.2,-1.10891016400001));
#315841=CARTESIAN_POINT('Ctrl Pts',(-3.92408520200005,12.2,-1.10883769000001));
#315842=CARTESIAN_POINT('Ctrl Pts',(-3.92408520200005,5.2,-1.10883769000001));
#315843=CARTESIAN_POINT('Ctrl Pts',(-3.92408520200005,2.2,-1.10883769000001));
#315844=CARTESIAN_POINT('Ctrl Pts',(-3.92307734900006,12.2,-1.10876436500002));
#315845=CARTESIAN_POINT('Ctrl Pts',(-3.92307734900006,5.2,-1.10876436500002));
#315846=CARTESIAN_POINT('Ctrl Pts',(-3.92307734900006,2.2,-1.10876436500002));
#315847=CARTESIAN_POINT('Ctrl Pts',(-3.92207504200006,12.2,-1.10869020300001));
#315848=CARTESIAN_POINT('Ctrl Pts',(-3.92207504200006,5.2,-1.10869020300001));
#315849=CARTESIAN_POINT('Ctrl Pts',(-3.92207504200006,2.2,-1.10869020300001));
#315850=CARTESIAN_POINT('Ctrl Pts',(-3.92107829200006,12.2,-1.10861521800001));
#315851=CARTESIAN_POINT('Ctrl Pts',(-3.92107829200006,5.2,-1.10861521800001));
#315852=CARTESIAN_POINT('Ctrl Pts',(-3.92107829200006,2.2,-1.10861521800001));
#315853=CARTESIAN_POINT('Ctrl Pts',(-3.92008710600006,12.2,-1.10853942300002));
#315854=CARTESIAN_POINT('Ctrl Pts',(-3.92008710600006,5.2,-1.10853942300002));
#315855=CARTESIAN_POINT('Ctrl Pts',(-3.92008710600006,2.2,-1.10853942300002));
#315856=CARTESIAN_POINT('Ctrl Pts',(-3.91910149800006,12.2,-1.10846283100001));
#315857=CARTESIAN_POINT('Ctrl Pts',(-3.91910149800006,5.2,-1.10846283100001));
#315858=CARTESIAN_POINT('Ctrl Pts',(-3.91910149800006,2.2,-1.10846283100001));
#315859=CARTESIAN_POINT('Ctrl Pts',(-3.91812147400006,12.2,-1.10838545800001));
#315860=CARTESIAN_POINT('Ctrl Pts',(-3.91812147400006,5.2,-1.10838545800001));
#315861=CARTESIAN_POINT('Ctrl Pts',(-3.91812147400006,2.2,-1.10838545800001));
#315862=CARTESIAN_POINT('Ctrl Pts',(-3.91714704600005,12.2,-1.10830731500001));
#315863=CARTESIAN_POINT('Ctrl Pts',(-3.91714704600005,5.2,-1.10830731500001));
#315864=CARTESIAN_POINT('Ctrl Pts',(-3.91714704600005,2.2,-1.10830731500001));
#315865=CARTESIAN_POINT('Ctrl Pts',(-3.91617822200006,12.2,-1.10822841700001));
#315866=CARTESIAN_POINT('Ctrl Pts',(-3.91617822200006,5.2,-1.10822841700001));
#315867=CARTESIAN_POINT('Ctrl Pts',(-3.91617822200006,2.2,-1.10822841700001));
#315868=CARTESIAN_POINT('Ctrl Pts',(-3.91521501300006,12.2,-1.10814877800001));
#315869=CARTESIAN_POINT('Ctrl Pts',(-3.91521501300006,5.2,-1.10814877800001));
#315870=CARTESIAN_POINT('Ctrl Pts',(-3.91521501300006,2.2,-1.10814877800001));
#315871=CARTESIAN_POINT('Ctrl Pts',(-3.91425742800006,12.2,-1.10806841200001));
#315872=CARTESIAN_POINT('Ctrl Pts',(-3.91425742800006,5.2,-1.10806841200001));
#315873=CARTESIAN_POINT('Ctrl Pts',(-3.91425742800006,2.2,-1.10806841200001));
#315874=CARTESIAN_POINT('Ctrl Pts',(-3.91330547700006,12.2,-1.10798733200001));
#315875=CARTESIAN_POINT('Ctrl Pts',(-3.91330547700006,5.2,-1.10798733200001));
#315876=CARTESIAN_POINT('Ctrl Pts',(-3.91330547700006,2.2,-1.10798733200001));
#315877=CARTESIAN_POINT('Ctrl Pts',(-3.91235917000006,12.2,-1.10790555300001));
#315878=CARTESIAN_POINT('Ctrl Pts',(-3.91235917000006,5.2,-1.10790555300001));
#315879=CARTESIAN_POINT('Ctrl Pts',(-3.91235917000006,2.2,-1.10790555300001));
#315880=CARTESIAN_POINT('Ctrl Pts',(-3.91141851700006,12.2,-1.10782308700001));
#315881=CARTESIAN_POINT('Ctrl Pts',(-3.91141851700006,5.2,-1.10782308700001));
#315882=CARTESIAN_POINT('Ctrl Pts',(-3.91141851700006,2.2,-1.10782308700001));
#315883=CARTESIAN_POINT('Ctrl Pts',(-3.91048352600006,12.2,-1.10773995100002));
#315884=CARTESIAN_POINT('Ctrl Pts',(-3.91048352600006,5.2,-1.10773995100002));
#315885=CARTESIAN_POINT('Ctrl Pts',(-3.91048352600006,2.2,-1.10773995100002));
#315886=CARTESIAN_POINT('Ctrl Pts',(-3.90955420900006,12.2,-1.10765615700001));
#315887=CARTESIAN_POINT('Ctrl Pts',(-3.90955420900006,5.2,-1.10765615700001));
#315888=CARTESIAN_POINT('Ctrl Pts',(-3.90955420900006,2.2,-1.10765615700001));
#315889=CARTESIAN_POINT('Ctrl Pts',(-3.90863057500006,12.2,-1.10757172000001));
#315890=CARTESIAN_POINT('Ctrl Pts',(-3.90863057500006,5.2,-1.10757172000001));
#315891=CARTESIAN_POINT('Ctrl Pts',(-3.90863057500006,2.2,-1.10757172000001));
#315892=CARTESIAN_POINT('Ctrl Pts',(-3.90771263300006,12.2,-1.10748665400001));
#315893=CARTESIAN_POINT('Ctrl Pts',(-3.90771263300006,5.2,-1.10748665400001));
#315894=CARTESIAN_POINT('Ctrl Pts',(-3.90771263300006,2.2,-1.10748665400001));
#315895=CARTESIAN_POINT('Ctrl Pts',(-3.90680039400006,12.2,-1.10740097200001));
#315896=CARTESIAN_POINT('Ctrl Pts',(-3.90680039400006,5.2,-1.10740097200001));
#315897=CARTESIAN_POINT('Ctrl Pts',(-3.90680039400006,2.2,-1.10740097200001));
#315898=CARTESIAN_POINT('Ctrl Pts',(-3.90589386600006,12.2,-1.10731469100001));
#315899=CARTESIAN_POINT('Ctrl Pts',(-3.90589386600006,5.2,-1.10731469100001));
#315900=CARTESIAN_POINT('Ctrl Pts',(-3.90589386600006,2.2,-1.10731469100001));
#315901=CARTESIAN_POINT('Ctrl Pts',(-3.90499306200006,12.2,-1.10722782200002));
#315902=CARTESIAN_POINT('Ctrl Pts',(-3.90499306200006,5.2,-1.10722782200002));
#315903=CARTESIAN_POINT('Ctrl Pts',(-3.90499306200006,2.2,-1.10722782200002));
#315904=CARTESIAN_POINT('Ctrl Pts',(-3.90409798800006,12.2,-1.10714038300001));
#315905=CARTESIAN_POINT('Ctrl Pts',(-3.90409798800006,5.2,-1.10714038300001));
#315906=CARTESIAN_POINT('Ctrl Pts',(-3.90409798800006,2.2,-1.10714038300001));
#315907=CARTESIAN_POINT('Ctrl Pts',(-3.90320865700006,12.2,-1.10705238500001));
#315908=CARTESIAN_POINT('Ctrl Pts',(-3.90320865700006,5.2,-1.10705238500001));
#315909=CARTESIAN_POINT('Ctrl Pts',(-3.90320865700006,2.2,-1.10705238500001));
#315910=CARTESIAN_POINT('Ctrl Pts',(-3.90232507800006,12.2,-1.10696384600002));
#315911=CARTESIAN_POINT('Ctrl Pts',(-3.90232507800006,5.2,-1.10696384600002));
#315912=CARTESIAN_POINT('Ctrl Pts',(-3.90232507800006,2.2,-1.10696384600002));
#315913=CARTESIAN_POINT('Ctrl Pts',(-3.90144726000006,12.2,-1.10687477600001));
#315914=CARTESIAN_POINT('Ctrl Pts',(-3.90144726000006,5.2,-1.10687477600001));
#315915=CARTESIAN_POINT('Ctrl Pts',(-3.90144726000006,2.2,-1.10687477600001));
#315916=CARTESIAN_POINT('Ctrl Pts',(-3.90057521300006,12.2,-1.10678519400001));
#315917=CARTESIAN_POINT('Ctrl Pts',(-3.90057521300006,5.2,-1.10678519400001));
#315918=CARTESIAN_POINT('Ctrl Pts',(-3.90057521300006,2.2,-1.10678519400001));
#315919=CARTESIAN_POINT('Ctrl Pts',(-3.89970894600006,12.2,-1.10669511200001));
#315920=CARTESIAN_POINT('Ctrl Pts',(-3.89970894600006,5.2,-1.10669511200001));
#315921=CARTESIAN_POINT('Ctrl Pts',(-3.89970894600006,2.2,-1.10669511200001));
#315922=CARTESIAN_POINT('Ctrl Pts',(-3.89884847200006,12.2,-1.10660454700001));
#315923=CARTESIAN_POINT('Ctrl Pts',(-3.89884847200006,5.2,-1.10660454700001));
#315924=CARTESIAN_POINT('Ctrl Pts',(-3.89884847200006,2.2,-1.10660454700001));
#315925=CARTESIAN_POINT('Ctrl Pts',(-3.89799379800006,12.2,-1.10651351100001));
#315926=CARTESIAN_POINT('Ctrl Pts',(-3.89799379800006,5.2,-1.10651351100001));
#315927=CARTESIAN_POINT('Ctrl Pts',(-3.89799379800006,2.2,-1.10651351100001));
#315928=CARTESIAN_POINT('Ctrl Pts',(-3.89714493500006,12.2,-1.10642202000002));
#315929=CARTESIAN_POINT('Ctrl Pts',(-3.89714493500006,5.2,-1.10642202000002));
#315930=CARTESIAN_POINT('Ctrl Pts',(-3.89714493500006,2.2,-1.10642202000002));
#315931=CARTESIAN_POINT('Ctrl Pts',(-3.89630189200005,12.2,-1.10633008900002));
#315932=CARTESIAN_POINT('Ctrl Pts',(-3.89630189200005,5.2,-1.10633008900002));
#315933=CARTESIAN_POINT('Ctrl Pts',(-3.89630189200005,2.2,-1.10633008900002));
#315934=CARTESIAN_POINT('Ctrl Pts',(-3.89546468000006,12.2,-1.10623773300001));
#315935=CARTESIAN_POINT('Ctrl Pts',(-3.89546468000006,5.2,-1.10623773300001));
#315936=CARTESIAN_POINT('Ctrl Pts',(-3.89546468000006,2.2,-1.10623773300001));
#315937=CARTESIAN_POINT('Ctrl Pts',(-3.89463330900006,12.2,-1.10614496700002));
#315938=CARTESIAN_POINT('Ctrl Pts',(-3.89463330900006,5.2,-1.10614496700002));
#315939=CARTESIAN_POINT('Ctrl Pts',(-3.89463330900006,2.2,-1.10614496700002));
#315940=CARTESIAN_POINT('Ctrl Pts',(-3.89380778700006,12.2,-1.10605180600002));
#315941=CARTESIAN_POINT('Ctrl Pts',(-3.89380778700006,5.2,-1.10605180600002));
#315942=CARTESIAN_POINT('Ctrl Pts',(-3.89380778700006,2.2,-1.10605180600002));
#315943=CARTESIAN_POINT('Ctrl Pts',(-3.89298812600006,12.2,-1.10595826400001));
#315944=CARTESIAN_POINT('Ctrl Pts',(-3.89298812600006,5.2,-1.10595826400001));
#315945=CARTESIAN_POINT('Ctrl Pts',(-3.89298812600006,2.2,-1.10595826400001));
#315946=CARTESIAN_POINT('Ctrl Pts',(-3.89217433600006,12.2,-1.10586435700001));
#315947=CARTESIAN_POINT('Ctrl Pts',(-3.89217433600006,5.2,-1.10586435700001));
#315948=CARTESIAN_POINT('Ctrl Pts',(-3.89217433600006,2.2,-1.10586435700001));
#315949=CARTESIAN_POINT('Ctrl Pts',(-3.89136642500006,12.2,-1.10577010100001));
#315950=CARTESIAN_POINT('Ctrl Pts',(-3.89136642500006,5.2,-1.10577010100001));
#315951=CARTESIAN_POINT('Ctrl Pts',(-3.89136642500006,2.2,-1.10577010100001));
#315952=CARTESIAN_POINT('Ctrl Pts',(-3.89056440600006,12.2,-1.10567550900001));
#315953=CARTESIAN_POINT('Ctrl Pts',(-3.89056440600006,5.2,-1.10567550900001));
#315954=CARTESIAN_POINT('Ctrl Pts',(-3.89056440600006,2.2,-1.10567550900001));
#315955=CARTESIAN_POINT('Ctrl Pts',(-3.88976828500006,12.2,-1.10558059800002));
#315956=CARTESIAN_POINT('Ctrl Pts',(-3.88976828500006,5.2,-1.10558059800002));
#315957=CARTESIAN_POINT('Ctrl Pts',(-3.88976828500006,2.2,-1.10558059800002));
#315958=CARTESIAN_POINT('Ctrl Pts',(-3.88897807500006,12.2,-1.10548538300002));
#315959=CARTESIAN_POINT('Ctrl Pts',(-3.88897807500006,5.2,-1.10548538300002));
#315960=CARTESIAN_POINT('Ctrl Pts',(-3.88897807500006,2.2,-1.10548538300002));
#315961=CARTESIAN_POINT('Ctrl Pts',(-3.88819378500005,12.2,-1.10538988000001));
#315962=CARTESIAN_POINT('Ctrl Pts',(-3.88819378500005,5.2,-1.10538988000001));
#315963=CARTESIAN_POINT('Ctrl Pts',(-3.88819378500005,2.2,-1.10538988000001));
#315964=CARTESIAN_POINT('Ctrl Pts',(-3.88741542500005,12.2,-1.10529410400002));
#315965=CARTESIAN_POINT('Ctrl Pts',(-3.88741542500005,5.2,-1.10529410400002));
#315966=CARTESIAN_POINT('Ctrl Pts',(-3.88741542500005,2.2,-1.10529410400002));
#315967=CARTESIAN_POINT('Ctrl Pts',(-3.88664300600006,12.2,-1.10519806900002));
#315968=CARTESIAN_POINT('Ctrl Pts',(-3.88664300600006,5.2,-1.10519806900002));
#315969=CARTESIAN_POINT('Ctrl Pts',(-3.88664300600006,2.2,-1.10519806900002));
#315970=CARTESIAN_POINT('Ctrl Pts',(-3.88587653500006,12.2,-1.10510179300002));
#315971=CARTESIAN_POINT('Ctrl Pts',(-3.88587653500006,5.2,-1.10510179300002));
#315972=CARTESIAN_POINT('Ctrl Pts',(-3.88587653500006,2.2,-1.10510179300002));
#315973=CARTESIAN_POINT('Ctrl Pts',(-3.88511602600006,12.2,-1.10500529000001));
#315974=CARTESIAN_POINT('Ctrl Pts',(-3.88511602600006,5.2,-1.10500529000001));
#315975=CARTESIAN_POINT('Ctrl Pts',(-3.88511602600006,2.2,-1.10500529000001));
#315976=CARTESIAN_POINT('Ctrl Pts',(-3.88436148600006,12.2,-1.10490857500002));
#315977=CARTESIAN_POINT('Ctrl Pts',(-3.88436148600006,5.2,-1.10490857500002));
#315978=CARTESIAN_POINT('Ctrl Pts',(-3.88436148600006,2.2,-1.10490857500002));
#315979=CARTESIAN_POINT('Ctrl Pts',(-3.88361292600006,12.2,-1.10481166500001));
#315980=CARTESIAN_POINT('Ctrl Pts',(-3.88361292600006,5.2,-1.10481166500001));
#315981=CARTESIAN_POINT('Ctrl Pts',(-3.88361292600006,2.2,-1.10481166500001));
#315982=CARTESIAN_POINT('Ctrl Pts',(-3.88287035700006,12.2,-1.10471457700001));
#315983=CARTESIAN_POINT('Ctrl Pts',(-3.88287035700006,5.2,-1.10471457700001));
#315984=CARTESIAN_POINT('Ctrl Pts',(-3.88287035700006,2.2,-1.10471457700001));
#315985=CARTESIAN_POINT('Ctrl Pts',(-3.88213378800006,12.2,-1.10461732400001));
#315986=CARTESIAN_POINT('Ctrl Pts',(-3.88213378800006,5.2,-1.10461732400001));
#315987=CARTESIAN_POINT('Ctrl Pts',(-3.88213378800006,2.2,-1.10461732400001));
#315988=CARTESIAN_POINT('Ctrl Pts',(-3.88140322900006,12.2,-1.10451992400002));
#315989=CARTESIAN_POINT('Ctrl Pts',(-3.88140322900006,5.2,-1.10451992400002));
#315990=CARTESIAN_POINT('Ctrl Pts',(-3.88140322900006,2.2,-1.10451992400002));
#315991=CARTESIAN_POINT('Ctrl Pts',(-3.88067869000006,12.2,-1.10442239100002));
#315992=CARTESIAN_POINT('Ctrl Pts',(-3.88067869000006,5.2,-1.10442239100002));
#315993=CARTESIAN_POINT('Ctrl Pts',(-3.88067869000006,2.2,-1.10442239100002));
#315994=CARTESIAN_POINT('Ctrl Pts',(-3.87996018200006,12.2,-1.10432474300001));
#315995=CARTESIAN_POINT('Ctrl Pts',(-3.87996018200006,5.2,-1.10432474300001));
#315996=CARTESIAN_POINT('Ctrl Pts',(-3.87996018200006,2.2,-1.10432474300001));
#315997=CARTESIAN_POINT('Ctrl Pts',(-3.87924771400006,12.2,-1.10422699600001));
#315998=CARTESIAN_POINT('Ctrl Pts',(-3.87924771400006,5.2,-1.10422699600001));
#315999=CARTESIAN_POINT('Ctrl Pts',(-3.87924771400006,2.2,-1.10422699600001));
#316000=CARTESIAN_POINT('Ctrl Pts',(-3.87854129700006,12.2,-1.10412916400001));
#316001=CARTESIAN_POINT('Ctrl Pts',(-3.87854129700006,5.2,-1.10412916400001));
#316002=CARTESIAN_POINT('Ctrl Pts',(-3.87854129700006,2.2,-1.10412916400001));
#316003=CARTESIAN_POINT('Ctrl Pts',(-3.87784093900006,12.2,-1.10403126600001));
#316004=CARTESIAN_POINT('Ctrl Pts',(-3.87784093900006,5.2,-1.10403126600001));
#316005=CARTESIAN_POINT('Ctrl Pts',(-3.87784093900006,2.2,-1.10403126600001));
#316006=CARTESIAN_POINT('Ctrl Pts',(-3.87714665400006,12.2,-1.10393331500001));
#316007=CARTESIAN_POINT('Ctrl Pts',(-3.87714665400006,5.2,-1.10393331500001));
#316008=CARTESIAN_POINT('Ctrl Pts',(-3.87714665400006,2.2,-1.10393331500001));
#316009=CARTESIAN_POINT('Ctrl Pts',(-3.87645844900006,12.2,-1.10383533000002));
#316010=CARTESIAN_POINT('Ctrl Pts',(-3.87645844900006,5.2,-1.10383533000002));
#316011=CARTESIAN_POINT('Ctrl Pts',(-3.87645844900006,2.2,-1.10383533000002));
#316012=CARTESIAN_POINT('Ctrl Pts',(-3.87577633500006,12.2,-1.10373732700001));
#316013=CARTESIAN_POINT('Ctrl Pts',(-3.87577633500006,5.2,-1.10373732700001));
#316014=CARTESIAN_POINT('Ctrl Pts',(-3.87577633500006,2.2,-1.10373732700001));
#316015=CARTESIAN_POINT('Ctrl Pts',(-3.87510032200006,12.2,-1.10363932000002));
#316016=CARTESIAN_POINT('Ctrl Pts',(-3.87510032200006,5.2,-1.10363932000002));
#316017=CARTESIAN_POINT('Ctrl Pts',(-3.87510032200006,2.2,-1.10363932000002));
#316018=CARTESIAN_POINT('Ctrl Pts',(-3.87443042100006,12.2,-1.10354132900001));
#316019=CARTESIAN_POINT('Ctrl Pts',(-3.87443042100006,5.2,-1.10354132900001));
#316020=CARTESIAN_POINT('Ctrl Pts',(-3.87443042100006,2.2,-1.10354132900001));
#316021=CARTESIAN_POINT('Ctrl Pts',(-3.87376664100006,12.2,-1.10344336800001));
#316022=CARTESIAN_POINT('Ctrl Pts',(-3.87376664100006,5.2,-1.10344336800001));
#316023=CARTESIAN_POINT('Ctrl Pts',(-3.87376664100006,2.2,-1.10344336800001));
#316024=CARTESIAN_POINT('Ctrl Pts',(-3.87310899300005,12.2,-1.10334545400002));
#316025=CARTESIAN_POINT('Ctrl Pts',(-3.87310899300005,5.2,-1.10334545400002));
#316026=CARTESIAN_POINT('Ctrl Pts',(-3.87310899300005,2.2,-1.10334545400002));
#316027=CARTESIAN_POINT('Ctrl Pts',(-3.87245748600006,12.2,-1.10324760500002));
#316028=CARTESIAN_POINT('Ctrl Pts',(-3.87245748600006,5.2,-1.10324760500002));
#316029=CARTESIAN_POINT('Ctrl Pts',(-3.87245748600006,2.2,-1.10324760500002));
#316030=CARTESIAN_POINT('Ctrl Pts',(-3.87181213100006,12.2,-1.10314983600002));
#316031=CARTESIAN_POINT('Ctrl Pts',(-3.87181213100006,5.2,-1.10314983600002));
#316032=CARTESIAN_POINT('Ctrl Pts',(-3.87181213100006,2.2,-1.10314983600002));
#316033=CARTESIAN_POINT('Ctrl Pts',(-3.87117293900006,12.2,-1.10305216500001));
#316034=CARTESIAN_POINT('Ctrl Pts',(-3.87117293900006,5.2,-1.10305216500001));
#316035=CARTESIAN_POINT('Ctrl Pts',(-3.87117293900006,2.2,-1.10305216500001));
#316036=CARTESIAN_POINT('Ctrl Pts',(-3.87053991900006,12.2,-1.10295460800002));
#316037=CARTESIAN_POINT('Ctrl Pts',(-3.87053991900006,5.2,-1.10295460800002));
#316038=CARTESIAN_POINT('Ctrl Pts',(-3.87053991900006,2.2,-1.10295460800002));
#316039=CARTESIAN_POINT('Ctrl Pts',(-3.86991308100006,12.2,-1.10285718300001));
#316040=CARTESIAN_POINT('Ctrl Pts',(-3.86991308100006,5.2,-1.10285718300001));
#316041=CARTESIAN_POINT('Ctrl Pts',(-3.86991308100006,2.2,-1.10285718300001));
#316042=CARTESIAN_POINT('Ctrl Pts',(-3.86929243700005,12.2,-1.10275990500002));
#316043=CARTESIAN_POINT('Ctrl Pts',(-3.86929243700005,5.2,-1.10275990500002));
#316044=CARTESIAN_POINT('Ctrl Pts',(-3.86929243700005,2.2,-1.10275990500002));
#316045=CARTESIAN_POINT('Ctrl Pts',(-3.86867799500005,12.2,-1.10266279300001));
#316046=CARTESIAN_POINT('Ctrl Pts',(-3.86867799500005,5.2,-1.10266279300001));
#316047=CARTESIAN_POINT('Ctrl Pts',(-3.86867799500005,2.2,-1.10266279300001));
#316048=CARTESIAN_POINT('Ctrl Pts',(-3.86806976700006,12.2,-1.10256586300002));
#316049=CARTESIAN_POINT('Ctrl Pts',(-3.86806976700006,5.2,-1.10256586300002));
#316050=CARTESIAN_POINT('Ctrl Pts',(-3.86806976700006,2.2,-1.10256586300002));
#316051=CARTESIAN_POINT('Ctrl Pts',(-3.86746776200006,12.2,-1.10246913200001));
#316052=CARTESIAN_POINT('Ctrl Pts',(-3.86746776200006,5.2,-1.10246913200001));
#316053=CARTESIAN_POINT('Ctrl Pts',(-3.86746776200006,2.2,-1.10246913200001));
#316054=CARTESIAN_POINT('Ctrl Pts',(-3.86687199200006,12.2,-1.10237261900001));
#316055=CARTESIAN_POINT('Ctrl Pts',(-3.86687199200006,5.2,-1.10237261900001));
#316056=CARTESIAN_POINT('Ctrl Pts',(-3.86687199200006,2.2,-1.10237261900001));
#316057=CARTESIAN_POINT('Ctrl Pts',(-3.86628246500006,12.2,-1.10227633800001));
#316058=CARTESIAN_POINT('Ctrl Pts',(-3.86628246500006,5.2,-1.10227633800001));
#316059=CARTESIAN_POINT('Ctrl Pts',(-3.86628246500006,2.2,-1.10227633800001));
#316060=CARTESIAN_POINT('Ctrl Pts',(-3.86569919200006,12.2,-1.10218031000001));
#316061=CARTESIAN_POINT('Ctrl Pts',(-3.86569919200006,5.2,-1.10218031000001));
#316062=CARTESIAN_POINT('Ctrl Pts',(-3.86569919200006,2.2,-1.10218031000001));
#316063=CARTESIAN_POINT('Ctrl Pts',(-3.86512218500005,12.2,-1.10208455000001));
#316064=CARTESIAN_POINT('Ctrl Pts',(-3.86512218500005,5.2,-1.10208455000001));
#316065=CARTESIAN_POINT('Ctrl Pts',(-3.86512218500005,2.2,-1.10208455000001));
#316066=CARTESIAN_POINT('Ctrl Pts',(-3.86455145200006,12.2,-1.10198907600001));
#316067=CARTESIAN_POINT('Ctrl Pts',(-3.86455145200006,5.2,-1.10198907600001));
#316068=CARTESIAN_POINT('Ctrl Pts',(-3.86455145200006,2.2,-1.10198907600001));
#316069=CARTESIAN_POINT('Ctrl Pts',(-3.86398700500005,12.2,-1.10189390600001));
#316070=CARTESIAN_POINT('Ctrl Pts',(-3.86398700500005,5.2,-1.10189390600001));
#316071=CARTESIAN_POINT('Ctrl Pts',(-3.86398700500005,2.2,-1.10189390600001));
#316072=CARTESIAN_POINT('Ctrl Pts',(-3.86342885300006,12.2,-1.10179905700001));
#316073=CARTESIAN_POINT('Ctrl Pts',(-3.86342885300006,5.2,-1.10179905700001));
#316074=CARTESIAN_POINT('Ctrl Pts',(-3.86342885300006,2.2,-1.10179905700001));
#316075=CARTESIAN_POINT('Ctrl Pts',(-3.86287700700006,12.2,-1.10170454700001));
#316076=CARTESIAN_POINT('Ctrl Pts',(-3.86287700700006,5.2,-1.10170454700001));
#316077=CARTESIAN_POINT('Ctrl Pts',(-3.86287700700006,2.2,-1.10170454700001));
#316078=CARTESIAN_POINT('Ctrl Pts',(-3.86233147800006,12.2,-1.10161039400001));
#316079=CARTESIAN_POINT('Ctrl Pts',(-3.86233147800006,5.2,-1.10161039400001));
#316080=CARTESIAN_POINT('Ctrl Pts',(-3.86233147800006,2.2,-1.10161039400001));
#316081=CARTESIAN_POINT('Ctrl Pts',(-3.86179227500006,12.2,-1.10151661500002));
#316082=CARTESIAN_POINT('Ctrl Pts',(-3.86179227500006,5.2,-1.10151661500002));
#316083=CARTESIAN_POINT('Ctrl Pts',(-3.86179227500006,2.2,-1.10151661500002));
#316084=CARTESIAN_POINT('Ctrl Pts',(-3.86125940900006,12.2,-1.10142322800002));
#316085=CARTESIAN_POINT('Ctrl Pts',(-3.86125940900006,5.2,-1.10142322800002));
#316086=CARTESIAN_POINT('Ctrl Pts',(-3.86125940900006,2.2,-1.10142322800002));
#316087=CARTESIAN_POINT('Ctrl Pts',(-3.86073289100006,12.2,-1.10133025100001));
#316088=CARTESIAN_POINT('Ctrl Pts',(-3.86073289100006,5.2,-1.10133025100001));
#316089=CARTESIAN_POINT('Ctrl Pts',(-3.86073289100006,2.2,-1.10133025100001));
#316090=CARTESIAN_POINT('Ctrl Pts',(-3.86021273100006,12.2,-1.10123770400001));
#316091=CARTESIAN_POINT('Ctrl Pts',(-3.86021273100006,5.2,-1.10123770400001));
#316092=CARTESIAN_POINT('Ctrl Pts',(-3.86021273100006,2.2,-1.10123770400001));
#316093=CARTESIAN_POINT('Ctrl Pts',(-3.85969893800006,12.2,-1.10114560200001));
#316094=CARTESIAN_POINT('Ctrl Pts',(-3.85969893800006,5.2,-1.10114560200001));
#316095=CARTESIAN_POINT('Ctrl Pts',(-3.85969893800006,2.2,-1.10114560200001));
#316096=CARTESIAN_POINT('Ctrl Pts',(-3.85919152400006,12.2,-1.10105396400002));
#316097=CARTESIAN_POINT('Ctrl Pts',(-3.85919152400006,5.2,-1.10105396400002));
#316098=CARTESIAN_POINT('Ctrl Pts',(-3.85919152400006,2.2,-1.10105396400002));
#316099=CARTESIAN_POINT('Ctrl Pts',(-3.85869050100006,12.2,-1.10096280900001));
#316100=CARTESIAN_POINT('Ctrl Pts',(-3.85869050100006,5.2,-1.10096280900001));
#316101=CARTESIAN_POINT('Ctrl Pts',(-3.85869050100006,2.2,-1.10096280900001));
#316102=CARTESIAN_POINT('Ctrl Pts',(-3.85819587400006,12.2,-1.10087215500001));
#316103=CARTESIAN_POINT('Ctrl Pts',(-3.85819587400006,5.2,-1.10087215500001));
#316104=CARTESIAN_POINT('Ctrl Pts',(-3.85819587400006,2.2,-1.10087215500001));
#316105=CARTESIAN_POINT('Ctrl Pts',(-3.85770765900006,12.2,-1.10078202100001));
#316106=CARTESIAN_POINT('Ctrl Pts',(-3.85770765900006,5.2,-1.10078202100001));
#316107=CARTESIAN_POINT('Ctrl Pts',(-3.85770765900006,2.2,-1.10078202100001));
#316108=CARTESIAN_POINT('Ctrl Pts',(-3.85722586400005,12.2,-1.10069242400002));
#316109=CARTESIAN_POINT('Ctrl Pts',(-3.85722586400005,5.2,-1.10069242400002));
#316110=CARTESIAN_POINT('Ctrl Pts',(-3.85722586400005,2.2,-1.10069242400002));
#316111=CARTESIAN_POINT('Ctrl Pts',(-3.85675050100006,12.2,-1.10060338200002));
#316112=CARTESIAN_POINT('Ctrl Pts',(-3.85675050100006,5.2,-1.10060338200002));
#316113=CARTESIAN_POINT('Ctrl Pts',(-3.85675050100006,2.2,-1.10060338200002));
#316114=CARTESIAN_POINT('Ctrl Pts',(-3.85628157800006,12.2,-1.10051491600001));
#316115=CARTESIAN_POINT('Ctrl Pts',(-3.85628157800006,5.2,-1.10051491600001));
#316116=CARTESIAN_POINT('Ctrl Pts',(-3.85628157800006,2.2,-1.10051491600001));
#316117=CARTESIAN_POINT('Ctrl Pts',(-3.85581910700005,12.2,-1.10042704300001));
#316118=CARTESIAN_POINT('Ctrl Pts',(-3.85581910700005,5.2,-1.10042704300001));
#316119=CARTESIAN_POINT('Ctrl Pts',(-3.85581910700005,2.2,-1.10042704300001));
#316120=CARTESIAN_POINT('Ctrl Pts',(-3.85536309800006,12.2,-1.10033978300002));
#316121=CARTESIAN_POINT('Ctrl Pts',(-3.85536309800006,5.2,-1.10033978300002));
#316122=CARTESIAN_POINT('Ctrl Pts',(-3.85536309800006,2.2,-1.10033978300002));
#316123=CARTESIAN_POINT('Ctrl Pts',(-3.85491356200006,12.2,-1.10025315200001));
#316124=CARTESIAN_POINT('Ctrl Pts',(-3.85491356200006,5.2,-1.10025315200001));
#316125=CARTESIAN_POINT('Ctrl Pts',(-3.85491356200006,2.2,-1.10025315200001));
#316126=CARTESIAN_POINT('Ctrl Pts',(-3.85447051000006,12.2,-1.10016717100001));
#316127=CARTESIAN_POINT('Ctrl Pts',(-3.85447051000006,5.2,-1.10016717100001));
#316128=CARTESIAN_POINT('Ctrl Pts',(-3.85447051000006,2.2,-1.10016717100001));
#316129=CARTESIAN_POINT('Ctrl Pts',(-3.85403395200006,12.2,-1.10008185900002));
#316130=CARTESIAN_POINT('Ctrl Pts',(-3.85403395200006,5.2,-1.10008185900002));
#316131=CARTESIAN_POINT('Ctrl Pts',(-3.85403395200006,2.2,-1.10008185900002));
#316132=CARTESIAN_POINT('Ctrl Pts',(-3.85360389800006,12.2,-1.09999723400001));
#316133=CARTESIAN_POINT('Ctrl Pts',(-3.85360389800006,5.2,-1.09999723400001));
#316134=CARTESIAN_POINT('Ctrl Pts',(-3.85360389800006,2.2,-1.09999723400001));
#316135=CARTESIAN_POINT('Ctrl Pts',(-3.85318035800006,12.2,-1.09991331500002));
#316136=CARTESIAN_POINT('Ctrl Pts',(-3.85318035800006,5.2,-1.09991331500002));
#316137=CARTESIAN_POINT('Ctrl Pts',(-3.85318035800006,2.2,-1.09991331500002));
#316138=CARTESIAN_POINT('Ctrl Pts',(-3.85276334500006,12.2,-1.09983012300002));
#316139=CARTESIAN_POINT('Ctrl Pts',(-3.85276334500006,5.2,-1.09983012300002));
#316140=CARTESIAN_POINT('Ctrl Pts',(-3.85276334500006,2.2,-1.09983012300002));
#316141=CARTESIAN_POINT('Ctrl Pts',(-3.85235286800006,12.2,-1.09974767600002));
#316142=CARTESIAN_POINT('Ctrl Pts',(-3.85235286800006,5.2,-1.09974767600002));
#316143=CARTESIAN_POINT('Ctrl Pts',(-3.85235286800006,2.2,-1.09974767600002));
#316144=CARTESIAN_POINT('Ctrl Pts',(-3.85194893700006,12.2,-1.09966599100002));
#316145=CARTESIAN_POINT('Ctrl Pts',(-3.85194893700006,5.2,-1.09966599100002));
#316146=CARTESIAN_POINT('Ctrl Pts',(-3.85194893700006,2.2,-1.09966599100002));
#316147=CARTESIAN_POINT('Ctrl Pts',(-3.85155156300006,12.2,-1.09958509100001));
#316148=CARTESIAN_POINT('Ctrl Pts',(-3.85155156300006,5.2,-1.09958509100001));
#316149=CARTESIAN_POINT('Ctrl Pts',(-3.85155156300006,2.2,-1.09958509100001));
#316150=CARTESIAN_POINT('Ctrl Pts',(-3.85116075800005,12.2,-1.09950499300002));
#316151=CARTESIAN_POINT('Ctrl Pts',(-3.85116075800005,5.2,-1.09950499300002));
#316152=CARTESIAN_POINT('Ctrl Pts',(-3.85116075800005,2.2,-1.09950499300002));
#316153=CARTESIAN_POINT('Ctrl Pts',(-3.85077653200006,12.2,-1.09942571900001));
#316154=CARTESIAN_POINT('Ctrl Pts',(-3.85077653200006,5.2,-1.09942571900001));
#316155=CARTESIAN_POINT('Ctrl Pts',(-3.85077653200006,2.2,-1.09942571900001));
#316156=CARTESIAN_POINT('Ctrl Pts',(-3.85039889400006,12.2,-1.09934728600001));
#316157=CARTESIAN_POINT('Ctrl Pts',(-3.85039889400006,5.2,-1.09934728600001));
#316158=CARTESIAN_POINT('Ctrl Pts',(-3.85039889400006,2.2,-1.09934728600001));
#316159=CARTESIAN_POINT('Ctrl Pts',(-3.85002785600006,12.2,-1.09926971400002));
#316160=CARTESIAN_POINT('Ctrl Pts',(-3.85002785600006,5.2,-1.09926971400002));
#316161=CARTESIAN_POINT('Ctrl Pts',(-3.85002785600006,2.2,-1.09926971400002));
#316162=CARTESIAN_POINT('Ctrl Pts',(-3.84966343000006,12.2,-1.09919302400002));
#316163=CARTESIAN_POINT('Ctrl Pts',(-3.84966343000006,5.2,-1.09919302400002));
#316164=CARTESIAN_POINT('Ctrl Pts',(-3.84966343000006,2.2,-1.09919302400002));
#316165=CARTESIAN_POINT('Ctrl Pts',(-3.84930562400006,12.2,-1.09911723500002));
#316166=CARTESIAN_POINT('Ctrl Pts',(-3.84930562400006,5.2,-1.09911723500002));
#316167=CARTESIAN_POINT('Ctrl Pts',(-3.84930562400006,2.2,-1.09911723500002));
#316168=CARTESIAN_POINT('Ctrl Pts',(-3.84895445000006,12.2,-1.09904236700002));
#316169=CARTESIAN_POINT('Ctrl Pts',(-3.84895445000006,5.2,-1.09904236700002));
#316170=CARTESIAN_POINT('Ctrl Pts',(-3.84895445000006,2.2,-1.09904236700002));
#316171=CARTESIAN_POINT('Ctrl Pts',(-3.84860991900006,12.2,-1.09896844000001));
#316172=CARTESIAN_POINT('Ctrl Pts',(-3.84860991900006,5.2,-1.09896844000001));
#316173=CARTESIAN_POINT('Ctrl Pts',(-3.84860991900006,2.2,-1.09896844000001));
#316174=CARTESIAN_POINT('Ctrl Pts',(-3.84827204100006,12.2,-1.09889547500002));
#316175=CARTESIAN_POINT('Ctrl Pts',(-3.84827204100006,5.2,-1.09889547500002));
#316176=CARTESIAN_POINT('Ctrl Pts',(-3.84827204100006,2.2,-1.09889547500002));
#316177=CARTESIAN_POINT('Ctrl Pts',(-3.84794082700005,12.2,-1.09882349000001));
#316178=CARTESIAN_POINT('Ctrl Pts',(-3.84794082700005,5.2,-1.09882349000001));
#316179=CARTESIAN_POINT('Ctrl Pts',(-3.84794082700005,2.2,-1.09882349000001));
#316180=CARTESIAN_POINT('Ctrl Pts',(-3.84761628800006,12.2,-1.09875250600002));
#316181=CARTESIAN_POINT('Ctrl Pts',(-3.84761628800006,5.2,-1.09875250600002));
#316182=CARTESIAN_POINT('Ctrl Pts',(-3.84761628800006,2.2,-1.09875250600002));
#316183=CARTESIAN_POINT('Ctrl Pts',(-3.84729843500006,12.2,-1.09868254300002));
#316184=CARTESIAN_POINT('Ctrl Pts',(-3.84729843500006,5.2,-1.09868254300002));
#316185=CARTESIAN_POINT('Ctrl Pts',(-3.84729843500006,2.2,-1.09868254300002));
#316186=CARTESIAN_POINT('Ctrl Pts',(-3.84698727800005,12.2,-1.09861362400002));
#316187=CARTESIAN_POINT('Ctrl Pts',(-3.84698727800005,5.2,-1.09861362400002));
#316188=CARTESIAN_POINT('Ctrl Pts',(-3.84698727800005,2.2,-1.09861362400002));
#316189=CARTESIAN_POINT('Ctrl Pts',(-3.84668282800006,12.2,-1.09854576700001));
#316190=CARTESIAN_POINT('Ctrl Pts',(-3.84668282800006,5.2,-1.09854576700001));
#316191=CARTESIAN_POINT('Ctrl Pts',(-3.84668282800006,2.2,-1.09854576700001));
#316192=CARTESIAN_POINT('Ctrl Pts',(-3.84638509700006,12.2,-1.09847899200001));
#316193=CARTESIAN_POINT('Ctrl Pts',(-3.84638509700006,5.2,-1.09847899200001));
#316194=CARTESIAN_POINT('Ctrl Pts',(-3.84638509700006,2.2,-1.09847899200001));
#316195=CARTESIAN_POINT('Ctrl Pts',(-3.84609409400006,12.2,-1.09841332200002));
#316196=CARTESIAN_POINT('Ctrl Pts',(-3.84609409400006,5.2,-1.09841332200002));
#316197=CARTESIAN_POINT('Ctrl Pts',(-3.84609409400006,2.2,-1.09841332200002));
#316198=CARTESIAN_POINT('Ctrl Pts',(-3.84580983000006,12.2,-1.09834877500001));
#316199=CARTESIAN_POINT('Ctrl Pts',(-3.84580983000006,5.2,-1.09834877500001));
#316200=CARTESIAN_POINT('Ctrl Pts',(-3.84580983000006,2.2,-1.09834877500001));
#316201=CARTESIAN_POINT('Ctrl Pts',(-3.84553231800006,12.2,-1.09828537300002));
#316202=CARTESIAN_POINT('Ctrl Pts',(-3.84553231800006,5.2,-1.09828537300002));
#316203=CARTESIAN_POINT('Ctrl Pts',(-3.84553231800006,2.2,-1.09828537300002));
#316204=CARTESIAN_POINT('Ctrl Pts',(-3.84526156700006,12.2,-1.09822313700001));
#316205=CARTESIAN_POINT('Ctrl Pts',(-3.84526156700006,5.2,-1.09822313700001));
#316206=CARTESIAN_POINT('Ctrl Pts',(-3.84526156700006,2.2,-1.09822313700001));
#316207=CARTESIAN_POINT('Ctrl Pts',(-3.84499758700006,12.2,-1.09816208800002));
#316208=CARTESIAN_POINT('Ctrl Pts',(-3.84499758700006,5.2,-1.09816208800002));
#316209=CARTESIAN_POINT('Ctrl Pts',(-3.84499758700006,2.2,-1.09816208800002));
#316210=CARTESIAN_POINT('Ctrl Pts',(-3.84474039100006,12.2,-1.09810224700002));
#316211=CARTESIAN_POINT('Ctrl Pts',(-3.84474039100006,5.2,-1.09810224700002));
#316212=CARTESIAN_POINT('Ctrl Pts',(-3.84474039100006,2.2,-1.09810224700002));
#316213=CARTESIAN_POINT('Ctrl Pts',(-3.84448998900006,12.2,-1.09804363400002));
#316214=CARTESIAN_POINT('Ctrl Pts',(-3.84448998900006,5.2,-1.09804363400002));
#316215=CARTESIAN_POINT('Ctrl Pts',(-3.84448998900006,2.2,-1.09804363400002));
#316216=CARTESIAN_POINT('Ctrl Pts',(-3.84424639200006,12.2,-1.09798627300002));
#316217=CARTESIAN_POINT('Ctrl Pts',(-3.84424639200006,5.2,-1.09798627300002));
#316218=CARTESIAN_POINT('Ctrl Pts',(-3.84424639200006,2.2,-1.09798627300002));
#316219=CARTESIAN_POINT('Ctrl Pts',(-3.84400961000006,12.2,-1.09793018200001));
#316220=CARTESIAN_POINT('Ctrl Pts',(-3.84400961000006,5.2,-1.09793018200001));
#316221=CARTESIAN_POINT('Ctrl Pts',(-3.84400961000006,2.2,-1.09793018200001));
#316222=CARTESIAN_POINT('Ctrl Pts',(-3.84377965500006,12.2,-1.09787538400001));
#316223=CARTESIAN_POINT('Ctrl Pts',(-3.84377965500006,5.2,-1.09787538400001));
#316224=CARTESIAN_POINT('Ctrl Pts',(-3.84377965500006,2.2,-1.09787538400001));
#316225=CARTESIAN_POINT('Ctrl Pts',(-3.84355653800006,12.2,-1.09782190000002));
#316226=CARTESIAN_POINT('Ctrl Pts',(-3.84355653800006,5.2,-1.09782190000002));
#316227=CARTESIAN_POINT('Ctrl Pts',(-3.84355653800006,2.2,-1.09782190000002));
#316228=CARTESIAN_POINT('Ctrl Pts',(-3.84334026900006,12.2,-1.09776975200001));
#316229=CARTESIAN_POINT('Ctrl Pts',(-3.84334026900006,5.2,-1.09776975200001));
#316230=CARTESIAN_POINT('Ctrl Pts',(-3.84334026900006,2.2,-1.09776975200001));
#316231=CARTESIAN_POINT('Ctrl Pts',(-3.84313086000006,12.2,-1.09771896100002));
#316232=CARTESIAN_POINT('Ctrl Pts',(-3.84313086000006,5.2,-1.09771896100002));
#316233=CARTESIAN_POINT('Ctrl Pts',(-3.84313086000006,2.2,-1.09771896100002));
#316234=CARTESIAN_POINT('Ctrl Pts',(-3.84292832100006,12.2,-1.09766954900001));
#316235=CARTESIAN_POINT('Ctrl Pts',(-3.84292832100006,5.2,-1.09766954900001));
#316236=CARTESIAN_POINT('Ctrl Pts',(-3.84292832100006,2.2,-1.09766954900001));
#316237=CARTESIAN_POINT('Ctrl Pts',(-3.84273266500006,12.2,-1.09762153800002));
#316238=CARTESIAN_POINT('Ctrl Pts',(-3.84273266500006,5.2,-1.09762153800002));
#316239=CARTESIAN_POINT('Ctrl Pts',(-3.84273266500006,2.2,-1.09762153800002));
#316240=CARTESIAN_POINT('Ctrl Pts',(-3.84254390100006,12.2,-1.09757495000002));
#316241=CARTESIAN_POINT('Ctrl Pts',(-3.84254390100006,5.2,-1.09757495000002));
#316242=CARTESIAN_POINT('Ctrl Pts',(-3.84254390100006,2.2,-1.09757495000002));
#316243=CARTESIAN_POINT('Ctrl Pts',(-3.84236204200006,12.2,-1.09752980700002));
#316244=CARTESIAN_POINT('Ctrl Pts',(-3.84236204200006,5.2,-1.09752980700002));
#316245=CARTESIAN_POINT('Ctrl Pts',(-3.84236204200006,2.2,-1.09752980700002));
#316246=CARTESIAN_POINT('Ctrl Pts',(-3.84218709600006,12.2,-1.09748613100002));
#316247=CARTESIAN_POINT('Ctrl Pts',(-3.84218709600006,5.2,-1.09748613100002));
#316248=CARTESIAN_POINT('Ctrl Pts',(-3.84218709600006,2.2,-1.09748613100002));
#316249=CARTESIAN_POINT('Ctrl Pts',(-3.84201907700006,12.2,-1.09744394400002));
#316250=CARTESIAN_POINT('Ctrl Pts',(-3.84201907700006,5.2,-1.09744394400002));
#316251=CARTESIAN_POINT('Ctrl Pts',(-3.84201907700006,2.2,-1.09744394400002));
#316252=CARTESIAN_POINT('Ctrl Pts',(-3.84185799400006,12.2,-1.09740326700001));
#316253=CARTESIAN_POINT('Ctrl Pts',(-3.84185799400006,5.2,-1.09740326700001));
#316254=CARTESIAN_POINT('Ctrl Pts',(-3.84185799400006,2.2,-1.09740326700001));
#316255=CARTESIAN_POINT('Ctrl Pts',(-3.84170386000006,12.2,-1.09736412400002));
#316256=CARTESIAN_POINT('Ctrl Pts',(-3.84170386000006,5.2,-1.09736412400002));
#316257=CARTESIAN_POINT('Ctrl Pts',(-3.84170386000006,2.2,-1.09736412400002));
#316258=CARTESIAN_POINT('Ctrl Pts',(-3.84155668300005,12.2,-1.09732653400001));
#316259=CARTESIAN_POINT('Ctrl Pts',(-3.84155668300005,5.2,-1.09732653400001));
#316260=CARTESIAN_POINT('Ctrl Pts',(-3.84155668300005,2.2,-1.09732653400001));
#316261=CARTESIAN_POINT('Ctrl Pts',(-3.84141647700006,12.2,-1.09729052600001));
#316262=CARTESIAN_POINT('Ctrl Pts',(-3.84141647700006,5.2,-1.09729052600001));
#316263=CARTESIAN_POINT('Ctrl Pts',(-3.84141647700006,2.2,-1.09729052600001));
#316264=CARTESIAN_POINT('Ctrl Pts',(-3.84128325400006,12.2,-1.09725611800001));
#316265=CARTESIAN_POINT('Ctrl Pts',(-3.84128325400006,5.2,-1.09725611800001));
#316266=CARTESIAN_POINT('Ctrl Pts',(-3.84128325400006,2.2,-1.09725611800001));
#316267=CARTESIAN_POINT('Ctrl Pts',(-3.84115702400006,12.2,-1.09722333700002));
#316268=CARTESIAN_POINT('Ctrl Pts',(-3.84115702400006,5.2,-1.09722333700002));
#316269=CARTESIAN_POINT('Ctrl Pts',(-3.84115702400006,2.2,-1.09722333700002));
#316270=CARTESIAN_POINT('Ctrl Pts',(-3.84103780000006,12.2,-1.09719220600001));
#316271=CARTESIAN_POINT('Ctrl Pts',(-3.84103780000006,5.2,-1.09719220600001));
#316272=CARTESIAN_POINT('Ctrl Pts',(-3.84103780000006,2.2,-1.09719220600001));
#316273=CARTESIAN_POINT('Ctrl Pts',(-3.84092559000006,12.2,-1.09716274300002));
#316274=CARTESIAN_POINT('Ctrl Pts',(-3.84092559000006,5.2,-1.09716274300002));
#316275=CARTESIAN_POINT('Ctrl Pts',(-3.84092559000006,2.2,-1.09716274300002));
#316276=CARTESIAN_POINT('Ctrl Pts',(-3.84082040400005,12.2,-1.09713496900001));
#316277=CARTESIAN_POINT('Ctrl Pts',(-3.84082040400005,5.2,-1.09713496900001));
#316278=CARTESIAN_POINT('Ctrl Pts',(-3.84082040400005,2.2,-1.09713496900001));
#316279=CARTESIAN_POINT('Ctrl Pts',(-3.84072225300006,12.2,-1.09710890700002));
#316280=CARTESIAN_POINT('Ctrl Pts',(-3.84072225300006,5.2,-1.09710890700002));
#316281=CARTESIAN_POINT('Ctrl Pts',(-3.84072225300006,2.2,-1.09710890700002));
#316282=CARTESIAN_POINT('Ctrl Pts',(-3.84063114900006,12.2,-1.09708457800001));
#316283=CARTESIAN_POINT('Ctrl Pts',(-3.84063114900006,5.2,-1.09708457800001));
#316284=CARTESIAN_POINT('Ctrl Pts',(-3.84063114900006,2.2,-1.09708457800001));
#316285=CARTESIAN_POINT('Ctrl Pts',(-3.84054710500005,12.2,-1.09706201000002));
#316286=CARTESIAN_POINT('Ctrl Pts',(-3.84054710500005,5.2,-1.09706201000002));
#316287=CARTESIAN_POINT('Ctrl Pts',(-3.84054710500005,2.2,-1.09706201000002));
#316288=CARTESIAN_POINT('Ctrl Pts',(-3.84047013400005,12.2,-1.09704123400002));
#316289=CARTESIAN_POINT('Ctrl Pts',(-3.84047013400005,5.2,-1.09704123400002));
#316290=CARTESIAN_POINT('Ctrl Pts',(-3.84047013400005,2.2,-1.09704123400002));
#316291=CARTESIAN_POINT('Ctrl Pts',(-3.84040025100005,12.2,-1.09702227600001));
#316292=CARTESIAN_POINT('Ctrl Pts',(-3.84040025100005,5.2,-1.09702227600001));
#316293=CARTESIAN_POINT('Ctrl Pts',(-3.84040025100005,2.2,-1.09702227600001));
#316294=CARTESIAN_POINT('Ctrl Pts',(-3.84033746800006,12.2,-1.09700516500002));
#316295=CARTESIAN_POINT('Ctrl Pts',(-3.84033746800006,5.2,-1.09700516500002));
#316296=CARTESIAN_POINT('Ctrl Pts',(-3.84033746800006,2.2,-1.09700516500002));
#316297=CARTESIAN_POINT('Ctrl Pts',(-3.84028179500006,12.2,-1.09698992100002));
#316298=CARTESIAN_POINT('Ctrl Pts',(-3.84028179500006,5.2,-1.09698992100002));
#316299=CARTESIAN_POINT('Ctrl Pts',(-3.84028179500006,2.2,-1.09698992100002));
#316300=CARTESIAN_POINT('Ctrl Pts',(-3.84022803879258,12.2,-1.09697511972126));
#316301=CARTESIAN_POINT('Ctrl Pts',(-3.84022803879258,5.2,-1.09697511972126));
#316302=CARTESIAN_POINT('Ctrl Pts',(-3.84022803879258,2.2,-1.09697511972126));
#316303=CARTESIAN_POINT('Ctrl Pts',(-3.84019131325105,12.2,-1.09696492845847));
#316304=CARTESIAN_POINT('Ctrl Pts',(-3.84019131325105,5.2,-1.09696492845847));
#316305=CARTESIAN_POINT('Ctrl Pts',(-3.84019131325105,2.2,-1.09696492845847));
#316306=CARTESIAN_POINT('Ctrl Pts',(-3.84016713475081,12.2,-1.0969581629428));
#316307=CARTESIAN_POINT('Ctrl Pts',(-3.84016713475081,5.2,-1.0969581629428));
#316308=CARTESIAN_POINT('Ctrl Pts',(-3.84016713475081,2.2,-1.0969581629428));
#316309=CARTESIAN_POINT('Ctrl Pts',(-3.84015208032585,12.2,-1.09695391765456));
#316310=CARTESIAN_POINT('Ctrl Pts',(-3.84015208032585,5.2,-1.09695391765456));
#316311=CARTESIAN_POINT('Ctrl Pts',(-3.84015208032585,2.2,-1.09695391765456));
#316312=CARTESIAN_POINT('Ctrl Pts',(-3.84014278600006,12.2,-1.09695129700001));
#316313=CARTESIAN_POINT('Ctrl Pts',(-3.84014278600006,5.2,-1.09695129700001));
#316314=CARTESIAN_POINT('Ctrl Pts',(-3.84014278600006,2.2,-1.09695129700001));
#316315=CARTESIAN_POINT('',(-3.84014273100005,2.7,-1.09695149100002));
#316316=CARTESIAN_POINT('',(-3.84014273100005,12.2,-1.09695149100002));
#316317=CARTESIAN_POINT('Ctrl Pts',(-4.64916443400006,2.7,-0.973534832000014));
#316318=CARTESIAN_POINT('Ctrl Pts',(-4.39305820566497,2.7,-1.07158848910283));
#316319=CARTESIAN_POINT('Ctrl Pts',(-4.20747959129484,2.70000000001822,
-1.09719287120144));
#316320=CARTESIAN_POINT('Ctrl Pts',(-3.96057902756421,2.70000000001822,
-1.1188234958715));
#316321=CARTESIAN_POINT('Ctrl Pts',(-3.87277126955167,2.70000000001823,
-1.10458234514971));
#316322=CARTESIAN_POINT('Ctrl Pts',(-3.84199433897037,2.70000000001823,
-1.09746781128816));
#316323=CARTESIAN_POINT('Ctrl Pts',(-3.84047363749101,2.7,-1.09704458482765));
#316324=CARTESIAN_POINT('Ctrl Pts',(-3.84014278600006,2.7,-1.09695129700001));
#316325=CARTESIAN_POINT('Origin',(-3.84009338800006,15.2,-1.09693739600001));
#316326=CARTESIAN_POINT('',(-3.48557996500006,2.7,-0.995669277000015));
#316327=CARTESIAN_POINT('',(-3.48557996500006,2.2,-0.995669277000015));
#316328=CARTESIAN_POINT('',(-1.92004669396261,2.7,-0.548468698131102));
#316329=CARTESIAN_POINT('Origin',(-5.66300478732629E-14,15.2,-1.77635683940025E-14));
#316330=CARTESIAN_POINT('',(-3.29009567500006,2.7,-1.52180664000001));
#316331=CARTESIAN_POINT('',(-3.29009567500006,12.2,-1.52180664000001));
#316332=CARTESIAN_POINT('Origin',(-5.66300478732629E-14,2.7,-1.92943768261394E-14));
#316333=CARTESIAN_POINT('Origin',(-5.66300478732629E-14,15.2,-1.77635683940025E-14));
#316334=CARTESIAN_POINT('',(-3.62475771700006,2.7,-1.67660181100001));
#316335=CARTESIAN_POINT('',(-3.62475771700006,12.2,-1.67660181100001));
#316336=CARTESIAN_POINT('',(-5.63267452475378E-14,2.7,-1.91540866959583E-14));
#316337=CARTESIAN_POINT('Ctrl Pts',(-3.62475766000006,12.2,-1.67660193200001));
#316338=CARTESIAN_POINT('Ctrl Pts',(-3.62475766000006,5.2,-1.67660193200001));
#316339=CARTESIAN_POINT('Ctrl Pts',(-3.62475766000006,2.2,-1.67660193200001));
#316340=CARTESIAN_POINT('Ctrl Pts',(-3.62476385949508,12.2,-1.67660482976411));
#316341=CARTESIAN_POINT('Ctrl Pts',(-3.62476385949508,5.2,-1.67660482976411));
#316342=CARTESIAN_POINT('Ctrl Pts',(-3.62476385949508,2.2,-1.67660482976411));
#316343=CARTESIAN_POINT('Ctrl Pts',(-3.62477584957619,12.2,-1.67661043119582));
#316344=CARTESIAN_POINT('Ctrl Pts',(-3.62477584957619,5.2,-1.67661043119582));
#316345=CARTESIAN_POINT('Ctrl Pts',(-3.62477584957619,2.2,-1.67661043119582));
#316346=CARTESIAN_POINT('Ctrl Pts',(-3.62479362506676,12.2,-1.67661873245304));
#316347=CARTESIAN_POINT('Ctrl Pts',(-3.62479362506676,5.2,-1.67661873245304));
#316348=CARTESIAN_POINT('Ctrl Pts',(-3.62479362506676,2.2,-1.67661873245304));
#316349=CARTESIAN_POINT('Ctrl Pts',(-3.62481722099134,12.2,-1.67662978965931));
#316350=CARTESIAN_POINT('Ctrl Pts',(-3.62481722099134,5.2,-1.67662978965931));
#316351=CARTESIAN_POINT('Ctrl Pts',(-3.62481722099134,2.2,-1.67662978965931));
#316352=CARTESIAN_POINT('Ctrl Pts',(-3.62485815500006,12.2,-1.67664910700001));
#316353=CARTESIAN_POINT('Ctrl Pts',(-3.62485815500006,5.2,-1.67664910700001));
#316354=CARTESIAN_POINT('Ctrl Pts',(-3.62485815500006,2.2,-1.67664910700001));
#316355=CARTESIAN_POINT('Ctrl Pts',(-3.62490366200006,12.2,-1.67667068700001));
#316356=CARTESIAN_POINT('Ctrl Pts',(-3.62490366200006,5.2,-1.67667068700001));
#316357=CARTESIAN_POINT('Ctrl Pts',(-3.62490366200006,2.2,-1.67667068700001));
#316358=CARTESIAN_POINT('Ctrl Pts',(-3.62495578300006,12.2,-1.67669549200001));
#316359=CARTESIAN_POINT('Ctrl Pts',(-3.62495578300006,5.2,-1.67669549200001));
#316360=CARTESIAN_POINT('Ctrl Pts',(-3.62495578300006,2.2,-1.67669549200001));
#316361=CARTESIAN_POINT('Ctrl Pts',(-3.62501450700006,12.2,-1.67672352600002));
#316362=CARTESIAN_POINT('Ctrl Pts',(-3.62501450700006,5.2,-1.67672352600002));
#316363=CARTESIAN_POINT('Ctrl Pts',(-3.62501450700006,2.2,-1.67672352600002));
#316364=CARTESIAN_POINT('Ctrl Pts',(-3.62507981500006,12.2,-1.67675479900002));
#316365=CARTESIAN_POINT('Ctrl Pts',(-3.62507981500006,5.2,-1.67675479900002));
#316366=CARTESIAN_POINT('Ctrl Pts',(-3.62507981500006,2.2,-1.67675479900002));
#316367=CARTESIAN_POINT('Ctrl Pts',(-3.62515167800006,12.2,-1.67678932100001));
#316368=CARTESIAN_POINT('Ctrl Pts',(-3.62515167800006,5.2,-1.67678932100001));
#316369=CARTESIAN_POINT('Ctrl Pts',(-3.62515167800006,2.2,-1.67678932100001));
#316370=CARTESIAN_POINT('Ctrl Pts',(-3.62523006900005,12.2,-1.67682710500001));
#316371=CARTESIAN_POINT('Ctrl Pts',(-3.62523006900005,5.2,-1.67682710500001));
#316372=CARTESIAN_POINT('Ctrl Pts',(-3.62523006900005,2.2,-1.67682710500001));
#316373=CARTESIAN_POINT('Ctrl Pts',(-3.62531495600006,12.2,-1.67686816600002));
#316374=CARTESIAN_POINT('Ctrl Pts',(-3.62531495600006,5.2,-1.67686816600002));
#316375=CARTESIAN_POINT('Ctrl Pts',(-3.62531495600006,2.2,-1.67686816600002));
#316376=CARTESIAN_POINT('Ctrl Pts',(-3.62540631300006,12.2,-1.67691251300001));
#316377=CARTESIAN_POINT('Ctrl Pts',(-3.62540631300006,5.2,-1.67691251300001));
#316378=CARTESIAN_POINT('Ctrl Pts',(-3.62540631300006,2.2,-1.67691251300001));
#316379=CARTESIAN_POINT('Ctrl Pts',(-3.62550411600005,12.2,-1.67696015900002));
#316380=CARTESIAN_POINT('Ctrl Pts',(-3.62550411600005,5.2,-1.67696015900002));
#316381=CARTESIAN_POINT('Ctrl Pts',(-3.62550411600005,2.2,-1.67696015900002));
#316382=CARTESIAN_POINT('Ctrl Pts',(-3.62560834100006,12.2,-1.67701111200001));
#316383=CARTESIAN_POINT('Ctrl Pts',(-3.62560834100006,5.2,-1.67701111200001));
#316384=CARTESIAN_POINT('Ctrl Pts',(-3.62560834100006,2.2,-1.67701111200001));
#316385=CARTESIAN_POINT('Ctrl Pts',(-3.62571897000006,12.2,-1.67706538100001));
#316386=CARTESIAN_POINT('Ctrl Pts',(-3.62571897000006,5.2,-1.67706538100001));
#316387=CARTESIAN_POINT('Ctrl Pts',(-3.62571897000006,2.2,-1.67706538100001));
#316388=CARTESIAN_POINT('Ctrl Pts',(-3.62583598000006,12.2,-1.67712297500001));
#316389=CARTESIAN_POINT('Ctrl Pts',(-3.62583598000006,5.2,-1.67712297500001));
#316390=CARTESIAN_POINT('Ctrl Pts',(-3.62583598000006,2.2,-1.67712297500001));
#316391=CARTESIAN_POINT('Ctrl Pts',(-3.62595934900006,12.2,-1.67718390600001));
#316392=CARTESIAN_POINT('Ctrl Pts',(-3.62595934900006,5.2,-1.67718390600001));
#316393=CARTESIAN_POINT('Ctrl Pts',(-3.62595934900006,2.2,-1.67718390600001));
#316394=CARTESIAN_POINT('Ctrl Pts',(-3.62608905300006,12.2,-1.67724817900002));
#316395=CARTESIAN_POINT('Ctrl Pts',(-3.62608905300006,5.2,-1.67724817900002));
#316396=CARTESIAN_POINT('Ctrl Pts',(-3.62608905300006,2.2,-1.67724817900002));
#316397=CARTESIAN_POINT('Ctrl Pts',(-3.62622506700006,12.2,-1.67731580900002));
#316398=CARTESIAN_POINT('Ctrl Pts',(-3.62622506700006,5.2,-1.67731580900002));
#316399=CARTESIAN_POINT('Ctrl Pts',(-3.62622506700006,2.2,-1.67731580900002));
#316400=CARTESIAN_POINT('Ctrl Pts',(-3.62636736800006,12.2,-1.67738680500001));
#316401=CARTESIAN_POINT('Ctrl Pts',(-3.62636736800006,5.2,-1.67738680500001));
#316402=CARTESIAN_POINT('Ctrl Pts',(-3.62636736800006,2.2,-1.67738680500001));
#316403=CARTESIAN_POINT('Ctrl Pts',(-3.62651593200006,12.2,-1.67746117600001));
#316404=CARTESIAN_POINT('Ctrl Pts',(-3.62651593200006,5.2,-1.67746117600001));
#316405=CARTESIAN_POINT('Ctrl Pts',(-3.62651593200006,2.2,-1.67746117600001));
#316406=CARTESIAN_POINT('Ctrl Pts',(-3.62667073600006,12.2,-1.67753893200001));
#316407=CARTESIAN_POINT('Ctrl Pts',(-3.62667073600006,5.2,-1.67753893200001));
#316408=CARTESIAN_POINT('Ctrl Pts',(-3.62667073600006,2.2,-1.67753893200001));
#316409=CARTESIAN_POINT('Ctrl Pts',(-3.62683175700006,12.2,-1.67762008300001));
#316410=CARTESIAN_POINT('Ctrl Pts',(-3.62683175700006,5.2,-1.67762008300001));
#316411=CARTESIAN_POINT('Ctrl Pts',(-3.62683175700006,2.2,-1.67762008300001));
#316412=CARTESIAN_POINT('Ctrl Pts',(-3.62699897200006,12.2,-1.67770463900001));
#316413=CARTESIAN_POINT('Ctrl Pts',(-3.62699897200006,5.2,-1.67770463900001));
#316414=CARTESIAN_POINT('Ctrl Pts',(-3.62699897200006,2.2,-1.67770463900001));
#316415=CARTESIAN_POINT('Ctrl Pts',(-3.62717236200006,12.2,-1.67779260800001));
#316416=CARTESIAN_POINT('Ctrl Pts',(-3.62717236200006,5.2,-1.67779260800001));
#316417=CARTESIAN_POINT('Ctrl Pts',(-3.62717236200006,2.2,-1.67779260800001));
#316418=CARTESIAN_POINT('Ctrl Pts',(-3.62735190100006,12.2,-1.67788399900001));
#316419=CARTESIAN_POINT('Ctrl Pts',(-3.62735190100006,5.2,-1.67788399900001));
#316420=CARTESIAN_POINT('Ctrl Pts',(-3.62735190100006,2.2,-1.67788399900001));
#316421=CARTESIAN_POINT('Ctrl Pts',(-3.62753756600006,12.2,-1.67797882200002));
#316422=CARTESIAN_POINT('Ctrl Pts',(-3.62753756600006,5.2,-1.67797882200002));
#316423=CARTESIAN_POINT('Ctrl Pts',(-3.62753756600006,2.2,-1.67797882200002));
#316424=CARTESIAN_POINT('Ctrl Pts',(-3.62772933700006,12.2,-1.67807708800002));
#316425=CARTESIAN_POINT('Ctrl Pts',(-3.62772933700006,5.2,-1.67807708800002));
#316426=CARTESIAN_POINT('Ctrl Pts',(-3.62772933700006,2.2,-1.67807708800002));
#316427=CARTESIAN_POINT('Ctrl Pts',(-3.62792718900006,12.2,-1.67817880400001));
#316428=CARTESIAN_POINT('Ctrl Pts',(-3.62792718900006,5.2,-1.67817880400001));
#316429=CARTESIAN_POINT('Ctrl Pts',(-3.62792718900006,2.2,-1.67817880400001));
#316430=CARTESIAN_POINT('Ctrl Pts',(-3.62813109900006,12.2,-1.67828398200002));
#316431=CARTESIAN_POINT('Ctrl Pts',(-3.62813109900006,5.2,-1.67828398200002));
#316432=CARTESIAN_POINT('Ctrl Pts',(-3.62813109900006,2.2,-1.67828398200002));
#316433=CARTESIAN_POINT('Ctrl Pts',(-3.62834104700006,12.2,-1.67839262700001));
#316434=CARTESIAN_POINT('Ctrl Pts',(-3.62834104700006,5.2,-1.67839262700001));
#316435=CARTESIAN_POINT('Ctrl Pts',(-3.62834104700006,2.2,-1.67839262700001));
#316436=CARTESIAN_POINT('Ctrl Pts',(-3.62855700900006,12.2,-1.67850475100002));
#316437=CARTESIAN_POINT('Ctrl Pts',(-3.62855700900006,5.2,-1.67850475100002));
#316438=CARTESIAN_POINT('Ctrl Pts',(-3.62855700900006,2.2,-1.67850475100002));
#316439=CARTESIAN_POINT('Ctrl Pts',(-3.62877896400006,12.2,-1.67862036400001));
#316440=CARTESIAN_POINT('Ctrl Pts',(-3.62877896400006,5.2,-1.67862036400001));
#316441=CARTESIAN_POINT('Ctrl Pts',(-3.62877896400006,2.2,-1.67862036400001));
#316442=CARTESIAN_POINT('Ctrl Pts',(-3.62900688900006,12.2,-1.67873947200002));
#316443=CARTESIAN_POINT('Ctrl Pts',(-3.62900688900006,5.2,-1.67873947200002));
#316444=CARTESIAN_POINT('Ctrl Pts',(-3.62900688900006,2.2,-1.67873947200002));
#316445=CARTESIAN_POINT('Ctrl Pts',(-3.62924076300006,12.2,-1.67886208600001));
#316446=CARTESIAN_POINT('Ctrl Pts',(-3.62924076300006,5.2,-1.67886208600001));
#316447=CARTESIAN_POINT('Ctrl Pts',(-3.62924076300006,2.2,-1.67886208600001));
#316448=CARTESIAN_POINT('Ctrl Pts',(-3.62948056200006,12.2,-1.67898821400001));
#316449=CARTESIAN_POINT('Ctrl Pts',(-3.62948056200006,5.2,-1.67898821400001));
#316450=CARTESIAN_POINT('Ctrl Pts',(-3.62948056200006,2.2,-1.67898821400001));
#316451=CARTESIAN_POINT('Ctrl Pts',(-3.62972626600006,12.2,-1.67911786500001));
#316452=CARTESIAN_POINT('Ctrl Pts',(-3.62972626600006,5.2,-1.67911786500001));
#316453=CARTESIAN_POINT('Ctrl Pts',(-3.62972626600006,2.2,-1.67911786500001));
#316454=CARTESIAN_POINT('Ctrl Pts',(-3.62997785200006,12.2,-1.67925104800001));
#316455=CARTESIAN_POINT('Ctrl Pts',(-3.62997785200006,5.2,-1.67925104800001));
#316456=CARTESIAN_POINT('Ctrl Pts',(-3.62997785200006,2.2,-1.67925104800001));
#316457=CARTESIAN_POINT('Ctrl Pts',(-3.63023529700006,12.2,-1.67938777100002));
#316458=CARTESIAN_POINT('Ctrl Pts',(-3.63023529700006,5.2,-1.67938777100002));
#316459=CARTESIAN_POINT('Ctrl Pts',(-3.63023529700006,2.2,-1.67938777100002));
#316460=CARTESIAN_POINT('Ctrl Pts',(-3.63049858300006,12.2,-1.67952804400001));
#316461=CARTESIAN_POINT('Ctrl Pts',(-3.63049858300006,5.2,-1.67952804400001));
#316462=CARTESIAN_POINT('Ctrl Pts',(-3.63049858300006,2.2,-1.67952804400001));
#316463=CARTESIAN_POINT('Ctrl Pts',(-3.63076768500005,12.2,-1.67967187400002));
#316464=CARTESIAN_POINT('Ctrl Pts',(-3.63076768500005,5.2,-1.67967187400002));
#316465=CARTESIAN_POINT('Ctrl Pts',(-3.63076768500005,2.2,-1.67967187400002));
#316466=CARTESIAN_POINT('Ctrl Pts',(-3.63104258200006,12.2,-1.67981927100001));
#316467=CARTESIAN_POINT('Ctrl Pts',(-3.63104258200006,5.2,-1.67981927100001));
#316468=CARTESIAN_POINT('Ctrl Pts',(-3.63104258200006,2.2,-1.67981927100001));
#316469=CARTESIAN_POINT('Ctrl Pts',(-3.63132325200006,12.2,-1.67997024200002));
#316470=CARTESIAN_POINT('Ctrl Pts',(-3.63132325200006,5.2,-1.67997024200002));
#316471=CARTESIAN_POINT('Ctrl Pts',(-3.63132325200006,2.2,-1.67997024200002));
#316472=CARTESIAN_POINT('Ctrl Pts',(-3.63160967600006,12.2,-1.68012479700002));
#316473=CARTESIAN_POINT('Ctrl Pts',(-3.63160967600006,5.2,-1.68012479700002));
#316474=CARTESIAN_POINT('Ctrl Pts',(-3.63160967600006,2.2,-1.68012479700002));
#316475=CARTESIAN_POINT('Ctrl Pts',(-3.63190183000006,12.2,-1.68028294400001));
#316476=CARTESIAN_POINT('Ctrl Pts',(-3.63190183000006,5.2,-1.68028294400001));
#316477=CARTESIAN_POINT('Ctrl Pts',(-3.63190183000006,2.2,-1.68028294400001));
#316478=CARTESIAN_POINT('Ctrl Pts',(-3.63219969300006,12.2,-1.68044468900002));
#316479=CARTESIAN_POINT('Ctrl Pts',(-3.63219969300006,5.2,-1.68044468900002));
#316480=CARTESIAN_POINT('Ctrl Pts',(-3.63219969300006,2.2,-1.68044468900002));
#316481=CARTESIAN_POINT('Ctrl Pts',(-3.63250324400005,12.2,-1.68061004400001));
#316482=CARTESIAN_POINT('Ctrl Pts',(-3.63250324400005,5.2,-1.68061004400001));
#316483=CARTESIAN_POINT('Ctrl Pts',(-3.63250324400005,2.2,-1.68061004400001));
#316484=CARTESIAN_POINT('Ctrl Pts',(-3.63281246200006,12.2,-1.68077901500002));
#316485=CARTESIAN_POINT('Ctrl Pts',(-3.63281246200006,5.2,-1.68077901500002));
#316486=CARTESIAN_POINT('Ctrl Pts',(-3.63281246200006,2.2,-1.68077901500002));
#316487=CARTESIAN_POINT('Ctrl Pts',(-3.63312732600006,12.2,-1.68095161000001));
#316488=CARTESIAN_POINT('Ctrl Pts',(-3.63312732600006,5.2,-1.68095161000001));
#316489=CARTESIAN_POINT('Ctrl Pts',(-3.63312732600006,2.2,-1.68095161000001));
#316490=CARTESIAN_POINT('Ctrl Pts',(-3.63344781300006,12.2,-1.68112783800002));
#316491=CARTESIAN_POINT('Ctrl Pts',(-3.63344781300006,5.2,-1.68112783800002));
#316492=CARTESIAN_POINT('Ctrl Pts',(-3.63344781300006,2.2,-1.68112783800002));
#316493=CARTESIAN_POINT('Ctrl Pts',(-3.63377390500006,12.2,-1.68130770800001));
#316494=CARTESIAN_POINT('Ctrl Pts',(-3.63377390500006,5.2,-1.68130770800001));
#316495=CARTESIAN_POINT('Ctrl Pts',(-3.63377390500006,2.2,-1.68130770800001));
#316496=CARTESIAN_POINT('Ctrl Pts',(-3.63410557800006,12.2,-1.68149122600001));
#316497=CARTESIAN_POINT('Ctrl Pts',(-3.63410557800006,5.2,-1.68149122600001));
#316498=CARTESIAN_POINT('Ctrl Pts',(-3.63410557800006,2.2,-1.68149122600001));
#316499=CARTESIAN_POINT('Ctrl Pts',(-3.63444281300006,12.2,-1.68167840100002));
#316500=CARTESIAN_POINT('Ctrl Pts',(-3.63444281300006,5.2,-1.68167840100002));
#316501=CARTESIAN_POINT('Ctrl Pts',(-3.63444281300006,2.2,-1.68167840100002));
#316502=CARTESIAN_POINT('Ctrl Pts',(-3.63478558800006,12.2,-1.68186924100001));
#316503=CARTESIAN_POINT('Ctrl Pts',(-3.63478558800006,5.2,-1.68186924100001));
#316504=CARTESIAN_POINT('Ctrl Pts',(-3.63478558800006,2.2,-1.68186924100001));
#316505=CARTESIAN_POINT('Ctrl Pts',(-3.63513388200006,12.2,-1.68206375400001));
#316506=CARTESIAN_POINT('Ctrl Pts',(-3.63513388200006,5.2,-1.68206375400001));
#316507=CARTESIAN_POINT('Ctrl Pts',(-3.63513388200006,2.2,-1.68206375400001));
#316508=CARTESIAN_POINT('Ctrl Pts',(-3.63548767700006,12.2,-1.68226194600001));
#316509=CARTESIAN_POINT('Ctrl Pts',(-3.63548767700006,5.2,-1.68226194600001));
#316510=CARTESIAN_POINT('Ctrl Pts',(-3.63548767700006,2.2,-1.68226194600001));
#316511=CARTESIAN_POINT('Ctrl Pts',(-3.63584694800006,12.2,-1.68246382700001));
#316512=CARTESIAN_POINT('Ctrl Pts',(-3.63584694800006,5.2,-1.68246382700001));
#316513=CARTESIAN_POINT('Ctrl Pts',(-3.63584694800006,2.2,-1.68246382700001));
#316514=CARTESIAN_POINT('Ctrl Pts',(-3.63621167800006,12.2,-1.68266940500001));
#316515=CARTESIAN_POINT('Ctrl Pts',(-3.63621167800006,5.2,-1.68266940500001));
#316516=CARTESIAN_POINT('Ctrl Pts',(-3.63621167800006,2.2,-1.68266940500001));
#316517=CARTESIAN_POINT('Ctrl Pts',(-3.63658184400006,12.2,-1.68287868500002));
#316518=CARTESIAN_POINT('Ctrl Pts',(-3.63658184400006,5.2,-1.68287868500002));
#316519=CARTESIAN_POINT('Ctrl Pts',(-3.63658184400006,2.2,-1.68287868500002));
#316520=CARTESIAN_POINT('Ctrl Pts',(-3.63695742600005,12.2,-1.68309167800002));
#316521=CARTESIAN_POINT('Ctrl Pts',(-3.63695742600005,5.2,-1.68309167800002));
#316522=CARTESIAN_POINT('Ctrl Pts',(-3.63695742600005,2.2,-1.68309167800002));
#316523=CARTESIAN_POINT('Ctrl Pts',(-3.63733840400006,12.2,-1.68330838800001));
#316524=CARTESIAN_POINT('Ctrl Pts',(-3.63733840400006,5.2,-1.68330838800001));
#316525=CARTESIAN_POINT('Ctrl Pts',(-3.63733840400006,2.2,-1.68330838800001));
#316526=CARTESIAN_POINT('Ctrl Pts',(-3.63772475700006,12.2,-1.68352882600002));
#316527=CARTESIAN_POINT('Ctrl Pts',(-3.63772475700006,5.2,-1.68352882600002));
#316528=CARTESIAN_POINT('Ctrl Pts',(-3.63772475700006,2.2,-1.68352882600002));
#316529=CARTESIAN_POINT('Ctrl Pts',(-3.63811646600006,12.2,-1.68375299700001));
#316530=CARTESIAN_POINT('Ctrl Pts',(-3.63811646600006,5.2,-1.68375299700001));
#316531=CARTESIAN_POINT('Ctrl Pts',(-3.63811646600006,2.2,-1.68375299700001));
#316532=CARTESIAN_POINT('Ctrl Pts',(-3.63851350900006,12.2,-1.68398091000002));
#316533=CARTESIAN_POINT('Ctrl Pts',(-3.63851350900006,5.2,-1.68398091000002));
#316534=CARTESIAN_POINT('Ctrl Pts',(-3.63851350900006,2.2,-1.68398091000002));
#316535=CARTESIAN_POINT('Ctrl Pts',(-3.63891586600006,12.2,-1.68421257200002));
#316536=CARTESIAN_POINT('Ctrl Pts',(-3.63891586600006,5.2,-1.68421257200002));
#316537=CARTESIAN_POINT('Ctrl Pts',(-3.63891586600006,2.2,-1.68421257200002));
#316538=CARTESIAN_POINT('Ctrl Pts',(-3.63932351700006,12.2,-1.68444798900001));
#316539=CARTESIAN_POINT('Ctrl Pts',(-3.63932351700006,5.2,-1.68444798900001));
#316540=CARTESIAN_POINT('Ctrl Pts',(-3.63932351700006,2.2,-1.68444798900001));
#316541=CARTESIAN_POINT('Ctrl Pts',(-3.63973644200006,12.2,-1.68468717000001));
#316542=CARTESIAN_POINT('Ctrl Pts',(-3.63973644200006,5.2,-1.68468717000001));
#316543=CARTESIAN_POINT('Ctrl Pts',(-3.63973644200006,2.2,-1.68468717000001));
#316544=CARTESIAN_POINT('Ctrl Pts',(-3.64015462100006,12.2,-1.68493012200001));
#316545=CARTESIAN_POINT('Ctrl Pts',(-3.64015462100006,5.2,-1.68493012200001));
#316546=CARTESIAN_POINT('Ctrl Pts',(-3.64015462100006,2.2,-1.68493012200001));
#316547=CARTESIAN_POINT('Ctrl Pts',(-3.64057803400006,12.2,-1.68517685100001));
#316548=CARTESIAN_POINT('Ctrl Pts',(-3.64057803400006,5.2,-1.68517685100001));
#316549=CARTESIAN_POINT('Ctrl Pts',(-3.64057803400006,2.2,-1.68517685100001));
#316550=CARTESIAN_POINT('Ctrl Pts',(-3.64100666200006,12.2,-1.68542736500001));
#316551=CARTESIAN_POINT('Ctrl Pts',(-3.64100666200006,5.2,-1.68542736500001));
#316552=CARTESIAN_POINT('Ctrl Pts',(-3.64100666200006,2.2,-1.68542736500001));
#316553=CARTESIAN_POINT('Ctrl Pts',(-3.64144048200005,12.2,-1.68568167200001));
#316554=CARTESIAN_POINT('Ctrl Pts',(-3.64144048200005,5.2,-1.68568167200001));
#316555=CARTESIAN_POINT('Ctrl Pts',(-3.64144048200005,2.2,-1.68568167200001));
#316556=CARTESIAN_POINT('Ctrl Pts',(-3.64187947600006,12.2,-1.68593977800001));
#316557=CARTESIAN_POINT('Ctrl Pts',(-3.64187947600006,5.2,-1.68593977800001));
#316558=CARTESIAN_POINT('Ctrl Pts',(-3.64187947600006,2.2,-1.68593977800001));
#316559=CARTESIAN_POINT('Ctrl Pts',(-3.64232362600006,12.2,-1.68620168900001));
#316560=CARTESIAN_POINT('Ctrl Pts',(-3.64232362600006,5.2,-1.68620168900001));
#316561=CARTESIAN_POINT('Ctrl Pts',(-3.64232362600006,2.2,-1.68620168900001));
#316562=CARTESIAN_POINT('Ctrl Pts',(-3.64277290900006,12.2,-1.68646741400002));
#316563=CARTESIAN_POINT('Ctrl Pts',(-3.64277290900006,5.2,-1.68646741400002));
#316564=CARTESIAN_POINT('Ctrl Pts',(-3.64277290900006,2.2,-1.68646741400002));
#316565=CARTESIAN_POINT('Ctrl Pts',(-3.64322730700006,12.2,-1.68673696000001));
#316566=CARTESIAN_POINT('Ctrl Pts',(-3.64322730700006,5.2,-1.68673696000001));
#316567=CARTESIAN_POINT('Ctrl Pts',(-3.64322730700006,2.2,-1.68673696000001));
#316568=CARTESIAN_POINT('Ctrl Pts',(-3.64368680000006,12.2,-1.68701033200001));
#316569=CARTESIAN_POINT('Ctrl Pts',(-3.64368680000006,5.2,-1.68701033200001));
#316570=CARTESIAN_POINT('Ctrl Pts',(-3.64368680000006,2.2,-1.68701033200001));
#316571=CARTESIAN_POINT('Ctrl Pts',(-3.64415136800006,12.2,-1.68728753800002));
#316572=CARTESIAN_POINT('Ctrl Pts',(-3.64415136800006,5.2,-1.68728753800002));
#316573=CARTESIAN_POINT('Ctrl Pts',(-3.64415136800006,2.2,-1.68728753800002));
#316574=CARTESIAN_POINT('Ctrl Pts',(-3.64462099200006,12.2,-1.68756858400001));
#316575=CARTESIAN_POINT('Ctrl Pts',(-3.64462099200006,5.2,-1.68756858400001));
#316576=CARTESIAN_POINT('Ctrl Pts',(-3.64462099200006,2.2,-1.68756858400001));
#316577=CARTESIAN_POINT('Ctrl Pts',(-3.64509565300006,12.2,-1.68785347900001));
#316578=CARTESIAN_POINT('Ctrl Pts',(-3.64509565300006,5.2,-1.68785347900001));
#316579=CARTESIAN_POINT('Ctrl Pts',(-3.64509565300006,2.2,-1.68785347900001));
#316580=CARTESIAN_POINT('Ctrl Pts',(-3.64557533000006,12.2,-1.68814222700002));
#316581=CARTESIAN_POINT('Ctrl Pts',(-3.64557533000006,5.2,-1.68814222700002));
#316582=CARTESIAN_POINT('Ctrl Pts',(-3.64557533000006,2.2,-1.68814222700002));
#316583=CARTESIAN_POINT('Ctrl Pts',(-3.64606000500006,12.2,-1.68843483600002));
#316584=CARTESIAN_POINT('Ctrl Pts',(-3.64606000500006,5.2,-1.68843483600002));
#316585=CARTESIAN_POINT('Ctrl Pts',(-3.64606000500006,2.2,-1.68843483600002));
#316586=CARTESIAN_POINT('Ctrl Pts',(-3.64654965700006,12.2,-1.68873131300002));
#316587=CARTESIAN_POINT('Ctrl Pts',(-3.64654965700006,5.2,-1.68873131300002));
#316588=CARTESIAN_POINT('Ctrl Pts',(-3.64654965700006,2.2,-1.68873131300002));
#316589=CARTESIAN_POINT('Ctrl Pts',(-3.64704426900006,12.2,-1.68903166300002));
#316590=CARTESIAN_POINT('Ctrl Pts',(-3.64704426900006,5.2,-1.68903166300002));
#316591=CARTESIAN_POINT('Ctrl Pts',(-3.64704426900006,2.2,-1.68903166300002));
#316592=CARTESIAN_POINT('Ctrl Pts',(-3.64754381900006,12.2,-1.68933589500002));
#316593=CARTESIAN_POINT('Ctrl Pts',(-3.64754381900006,5.2,-1.68933589500002));
#316594=CARTESIAN_POINT('Ctrl Pts',(-3.64754381900006,2.2,-1.68933589500002));
#316595=CARTESIAN_POINT('Ctrl Pts',(-3.64804829100006,12.2,-1.68964401300002));
#316596=CARTESIAN_POINT('Ctrl Pts',(-3.64804829100006,5.2,-1.68964401300002));
#316597=CARTESIAN_POINT('Ctrl Pts',(-3.64804829100006,2.2,-1.68964401300002));
#316598=CARTESIAN_POINT('Ctrl Pts',(-3.64855766400006,12.2,-1.68995602500001));
#316599=CARTESIAN_POINT('Ctrl Pts',(-3.64855766400006,5.2,-1.68995602500001));
#316600=CARTESIAN_POINT('Ctrl Pts',(-3.64855766400006,2.2,-1.68995602500001));
#316601=CARTESIAN_POINT('Ctrl Pts',(-3.64907191800006,12.2,-1.69027193700002));
#316602=CARTESIAN_POINT('Ctrl Pts',(-3.64907191800006,5.2,-1.69027193700002));
#316603=CARTESIAN_POINT('Ctrl Pts',(-3.64907191800006,2.2,-1.69027193700002));
#316604=CARTESIAN_POINT('Ctrl Pts',(-3.64959103500006,12.2,-1.69059175500001));
#316605=CARTESIAN_POINT('Ctrl Pts',(-3.64959103500006,5.2,-1.69059175500001));
#316606=CARTESIAN_POINT('Ctrl Pts',(-3.64959103500006,2.2,-1.69059175500001));
#316607=CARTESIAN_POINT('Ctrl Pts',(-3.65011499700006,12.2,-1.69091548500001));
#316608=CARTESIAN_POINT('Ctrl Pts',(-3.65011499700006,5.2,-1.69091548500001));
#316609=CARTESIAN_POINT('Ctrl Pts',(-3.65011499700006,2.2,-1.69091548500001));
#316610=CARTESIAN_POINT('Ctrl Pts',(-3.65064378300006,12.2,-1.69124313400001));
#316611=CARTESIAN_POINT('Ctrl Pts',(-3.65064378300006,5.2,-1.69124313400001));
#316612=CARTESIAN_POINT('Ctrl Pts',(-3.65064378300006,2.2,-1.69124313400001));
#316613=CARTESIAN_POINT('Ctrl Pts',(-3.65117737500006,12.2,-1.69157470900001));
#316614=CARTESIAN_POINT('Ctrl Pts',(-3.65117737500006,5.2,-1.69157470900001));
#316615=CARTESIAN_POINT('Ctrl Pts',(-3.65117737500006,2.2,-1.69157470900001));
#316616=CARTESIAN_POINT('Ctrl Pts',(-3.65171575500006,12.2,-1.69191021500001));
#316617=CARTESIAN_POINT('Ctrl Pts',(-3.65171575500006,5.2,-1.69191021500001));
#316618=CARTESIAN_POINT('Ctrl Pts',(-3.65171575500006,2.2,-1.69191021500001));
#316619=CARTESIAN_POINT('Ctrl Pts',(-3.65225890200006,12.2,-1.69224966000002));
#316620=CARTESIAN_POINT('Ctrl Pts',(-3.65225890200006,5.2,-1.69224966000002));
#316621=CARTESIAN_POINT('Ctrl Pts',(-3.65225890200006,2.2,-1.69224966000002));
#316622=CARTESIAN_POINT('Ctrl Pts',(-3.65280680000006,12.2,-1.69259304600001));
#316623=CARTESIAN_POINT('Ctrl Pts',(-3.65280680000006,5.2,-1.69259304600001));
#316624=CARTESIAN_POINT('Ctrl Pts',(-3.65280680000006,2.2,-1.69259304600001));
#316625=CARTESIAN_POINT('Ctrl Pts',(-3.65335942900006,12.2,-1.69294038500002));
#316626=CARTESIAN_POINT('Ctrl Pts',(-3.65335942900006,5.2,-1.69294038500002));
#316627=CARTESIAN_POINT('Ctrl Pts',(-3.65335942900006,2.2,-1.69294038500002));
#316628=CARTESIAN_POINT('Ctrl Pts',(-3.65391676900006,12.2,-1.69329167700001));
#316629=CARTESIAN_POINT('Ctrl Pts',(-3.65391676900006,5.2,-1.69329167700001));
#316630=CARTESIAN_POINT('Ctrl Pts',(-3.65391676900006,2.2,-1.69329167700001));
#316631=CARTESIAN_POINT('Ctrl Pts',(-3.65447880300006,12.2,-1.69364693300002));
#316632=CARTESIAN_POINT('Ctrl Pts',(-3.65447880300006,5.2,-1.69364693300002));
#316633=CARTESIAN_POINT('Ctrl Pts',(-3.65447880300006,2.2,-1.69364693300002));
#316634=CARTESIAN_POINT('Ctrl Pts',(-3.65504551200006,12.2,-1.69400615400002));
#316635=CARTESIAN_POINT('Ctrl Pts',(-3.65504551200006,5.2,-1.69400615400002));
#316636=CARTESIAN_POINT('Ctrl Pts',(-3.65504551200006,2.2,-1.69400615400002));
#316637=CARTESIAN_POINT('Ctrl Pts',(-3.65561687800006,12.2,-1.69436935100002));
#316638=CARTESIAN_POINT('Ctrl Pts',(-3.65561687800006,5.2,-1.69436935100002));
#316639=CARTESIAN_POINT('Ctrl Pts',(-3.65561687800006,2.2,-1.69436935100002));
#316640=CARTESIAN_POINT('Ctrl Pts',(-3.65619288200006,12.2,-1.69473652600002));
#316641=CARTESIAN_POINT('Ctrl Pts',(-3.65619288200006,5.2,-1.69473652600002));
#316642=CARTESIAN_POINT('Ctrl Pts',(-3.65619288200006,2.2,-1.69473652600002));
#316643=CARTESIAN_POINT('Ctrl Pts',(-3.65677350500006,12.2,-1.69510768800002));
#316644=CARTESIAN_POINT('Ctrl Pts',(-3.65677350500006,5.2,-1.69510768800002));
#316645=CARTESIAN_POINT('Ctrl Pts',(-3.65677350500006,2.2,-1.69510768800002));
#316646=CARTESIAN_POINT('Ctrl Pts',(-3.65735873000006,12.2,-1.69548284100001));
#316647=CARTESIAN_POINT('Ctrl Pts',(-3.65735873000006,5.2,-1.69548284100001));
#316648=CARTESIAN_POINT('Ctrl Pts',(-3.65735873000006,2.2,-1.69548284100001));
#316649=CARTESIAN_POINT('Ctrl Pts',(-3.65794853700006,12.2,-1.69586199000001));
#316650=CARTESIAN_POINT('Ctrl Pts',(-3.65794853700006,5.2,-1.69586199000001));
#316651=CARTESIAN_POINT('Ctrl Pts',(-3.65794853700006,2.2,-1.69586199000001));
#316652=CARTESIAN_POINT('Ctrl Pts',(-3.65854290900006,12.2,-1.69624514300001));
#316653=CARTESIAN_POINT('Ctrl Pts',(-3.65854290900006,5.2,-1.69624514300001));
#316654=CARTESIAN_POINT('Ctrl Pts',(-3.65854290900006,2.2,-1.69624514300001));
#316655=CARTESIAN_POINT('Ctrl Pts',(-3.65914182700006,12.2,-1.69663230300001));
#316656=CARTESIAN_POINT('Ctrl Pts',(-3.65914182700006,5.2,-1.69663230300001));
#316657=CARTESIAN_POINT('Ctrl Pts',(-3.65914182700006,2.2,-1.69663230300001));
#316658=CARTESIAN_POINT('Ctrl Pts',(-3.65974527300006,12.2,-1.69702347900001));
#316659=CARTESIAN_POINT('Ctrl Pts',(-3.65974527300006,5.2,-1.69702347900001));
#316660=CARTESIAN_POINT('Ctrl Pts',(-3.65974527300006,2.2,-1.69702347900001));
#316661=CARTESIAN_POINT('Ctrl Pts',(-3.66035322900006,12.2,-1.69741867300001));
#316662=CARTESIAN_POINT('Ctrl Pts',(-3.66035322900006,5.2,-1.69741867300001));
#316663=CARTESIAN_POINT('Ctrl Pts',(-3.66035322900006,2.2,-1.69741867300001));
#316664=CARTESIAN_POINT('Ctrl Pts',(-3.66096567700006,12.2,-1.69781789400002));
#316665=CARTESIAN_POINT('Ctrl Pts',(-3.66096567700006,5.2,-1.69781789400002));
#316666=CARTESIAN_POINT('Ctrl Pts',(-3.66096567700006,2.2,-1.69781789400002));
#316667=CARTESIAN_POINT('Ctrl Pts',(-3.66158259800006,12.2,-1.69822114400001));
#316668=CARTESIAN_POINT('Ctrl Pts',(-3.66158259800006,5.2,-1.69822114400001));
#316669=CARTESIAN_POINT('Ctrl Pts',(-3.66158259800006,2.2,-1.69822114400001));
#316670=CARTESIAN_POINT('Ctrl Pts',(-3.66220397600006,12.2,-1.69862843100002));
#316671=CARTESIAN_POINT('Ctrl Pts',(-3.66220397600006,5.2,-1.69862843100002));
#316672=CARTESIAN_POINT('Ctrl Pts',(-3.66220397600006,2.2,-1.69862843100002));
#316673=CARTESIAN_POINT('Ctrl Pts',(-3.66282979000006,12.2,-1.69903976000001));
#316674=CARTESIAN_POINT('Ctrl Pts',(-3.66282979000006,5.2,-1.69903976000001));
#316675=CARTESIAN_POINT('Ctrl Pts',(-3.66282979000006,2.2,-1.69903976000001));
#316676=CARTESIAN_POINT('Ctrl Pts',(-3.66346002500006,12.2,-1.69945513700001));
#316677=CARTESIAN_POINT('Ctrl Pts',(-3.66346002500006,5.2,-1.69945513700001));
#316678=CARTESIAN_POINT('Ctrl Pts',(-3.66346002500006,2.2,-1.69945513700001));
#316679=CARTESIAN_POINT('Ctrl Pts',(-3.66409466100006,12.2,-1.69987456500001));
#316680=CARTESIAN_POINT('Ctrl Pts',(-3.66409466100006,5.2,-1.69987456500001));
#316681=CARTESIAN_POINT('Ctrl Pts',(-3.66409466100006,2.2,-1.69987456500001));
#316682=CARTESIAN_POINT('Ctrl Pts',(-3.66473368100006,12.2,-1.70029805200001));
#316683=CARTESIAN_POINT('Ctrl Pts',(-3.66473368100006,5.2,-1.70029805200001));
#316684=CARTESIAN_POINT('Ctrl Pts',(-3.66473368100006,2.2,-1.70029805200001));
#316685=CARTESIAN_POINT('Ctrl Pts',(-3.66537706800006,12.2,-1.70072560100001));
#316686=CARTESIAN_POINT('Ctrl Pts',(-3.66537706800006,5.2,-1.70072560100001));
#316687=CARTESIAN_POINT('Ctrl Pts',(-3.66537706800006,2.2,-1.70072560100001));
#316688=CARTESIAN_POINT('Ctrl Pts',(-3.66602480300006,12.2,-1.70115722000002));
#316689=CARTESIAN_POINT('Ctrl Pts',(-3.66602480300006,5.2,-1.70115722000002));
#316690=CARTESIAN_POINT('Ctrl Pts',(-3.66602480300006,2.2,-1.70115722000002));
#316691=CARTESIAN_POINT('Ctrl Pts',(-3.66667686900006,12.2,-1.70159291300001));
#316692=CARTESIAN_POINT('Ctrl Pts',(-3.66667686900006,5.2,-1.70159291300001));
#316693=CARTESIAN_POINT('Ctrl Pts',(-3.66667686900006,2.2,-1.70159291300001));
#316694=CARTESIAN_POINT('Ctrl Pts',(-3.66733324700006,12.2,-1.70203268400002));
#316695=CARTESIAN_POINT('Ctrl Pts',(-3.66733324700006,5.2,-1.70203268400002));
#316696=CARTESIAN_POINT('Ctrl Pts',(-3.66733324700006,2.2,-1.70203268400002));
#316697=CARTESIAN_POINT('Ctrl Pts',(-3.66799392100006,12.2,-1.70247654000002));
#316698=CARTESIAN_POINT('Ctrl Pts',(-3.66799392100006,5.2,-1.70247654000002));
#316699=CARTESIAN_POINT('Ctrl Pts',(-3.66799392100006,2.2,-1.70247654000002));
#316700=CARTESIAN_POINT('Ctrl Pts',(-3.66865887300006,12.2,-1.70292448500001));
#316701=CARTESIAN_POINT('Ctrl Pts',(-3.66865887300006,5.2,-1.70292448500001));
#316702=CARTESIAN_POINT('Ctrl Pts',(-3.66865887300006,2.2,-1.70292448500001));
#316703=CARTESIAN_POINT('Ctrl Pts',(-3.66932808400006,12.2,-1.70337652400002));
#316704=CARTESIAN_POINT('Ctrl Pts',(-3.66932808400006,5.2,-1.70337652400002));
#316705=CARTESIAN_POINT('Ctrl Pts',(-3.66932808400006,2.2,-1.70337652400002));
#316706=CARTESIAN_POINT('Ctrl Pts',(-3.67000153900006,12.2,-1.70383266200002));
#316707=CARTESIAN_POINT('Ctrl Pts',(-3.67000153900006,5.2,-1.70383266200002));
#316708=CARTESIAN_POINT('Ctrl Pts',(-3.67000153900006,2.2,-1.70383266200002));
#316709=CARTESIAN_POINT('Ctrl Pts',(-3.67067921900006,12.2,-1.70429290600001));
#316710=CARTESIAN_POINT('Ctrl Pts',(-3.67067921900006,5.2,-1.70429290600001));
#316711=CARTESIAN_POINT('Ctrl Pts',(-3.67067921900006,2.2,-1.70429290600001));
#316712=CARTESIAN_POINT('Ctrl Pts',(-3.67136110600006,12.2,-1.70475725900001));
#316713=CARTESIAN_POINT('Ctrl Pts',(-3.67136110600006,5.2,-1.70475725900001));
#316714=CARTESIAN_POINT('Ctrl Pts',(-3.67136110600006,2.2,-1.70475725900001));
#316715=CARTESIAN_POINT('Ctrl Pts',(-3.67204718400005,12.2,-1.70522572600001));
#316716=CARTESIAN_POINT('Ctrl Pts',(-3.67204718400005,5.2,-1.70522572600001));
#316717=CARTESIAN_POINT('Ctrl Pts',(-3.67204718400005,2.2,-1.70522572600001));
#316718=CARTESIAN_POINT('Ctrl Pts',(-3.67273743400006,12.2,-1.70569831200002));
#316719=CARTESIAN_POINT('Ctrl Pts',(-3.67273743400006,5.2,-1.70569831200002));
#316720=CARTESIAN_POINT('Ctrl Pts',(-3.67273743400006,2.2,-1.70569831200002));
#316721=CARTESIAN_POINT('Ctrl Pts',(-3.67343184100006,12.2,-1.70617502300002));
#316722=CARTESIAN_POINT('Ctrl Pts',(-3.67343184100006,5.2,-1.70617502300002));
#316723=CARTESIAN_POINT('Ctrl Pts',(-3.67343184100006,2.2,-1.70617502300002));
#316724=CARTESIAN_POINT('Ctrl Pts',(-3.67413038600006,12.2,-1.70665586300002));
#316725=CARTESIAN_POINT('Ctrl Pts',(-3.67413038600006,5.2,-1.70665586300002));
#316726=CARTESIAN_POINT('Ctrl Pts',(-3.67413038600006,2.2,-1.70665586300002));
#316727=CARTESIAN_POINT('Ctrl Pts',(-3.67483305200006,12.2,-1.70714083700001));
#316728=CARTESIAN_POINT('Ctrl Pts',(-3.67483305200006,5.2,-1.70714083700001));
#316729=CARTESIAN_POINT('Ctrl Pts',(-3.67483305200006,2.2,-1.70714083700001));
#316730=CARTESIAN_POINT('Ctrl Pts',(-3.67553982200006,12.2,-1.70762995000001));
#316731=CARTESIAN_POINT('Ctrl Pts',(-3.67553982200006,5.2,-1.70762995000001));
#316732=CARTESIAN_POINT('Ctrl Pts',(-3.67553982200006,2.2,-1.70762995000001));
#316733=CARTESIAN_POINT('Ctrl Pts',(-3.67625067900006,12.2,-1.70812320600001));
#316734=CARTESIAN_POINT('Ctrl Pts',(-3.67625067900006,5.2,-1.70812320600001));
#316735=CARTESIAN_POINT('Ctrl Pts',(-3.67625067900006,2.2,-1.70812320600001));
#316736=CARTESIAN_POINT('Ctrl Pts',(-3.67696560600006,12.2,-1.70862061000001));
#316737=CARTESIAN_POINT('Ctrl Pts',(-3.67696560600006,5.2,-1.70862061000001));
#316738=CARTESIAN_POINT('Ctrl Pts',(-3.67696560600006,2.2,-1.70862061000001));
#316739=CARTESIAN_POINT('Ctrl Pts',(-3.67768458500006,12.2,-1.70912216700001));
#316740=CARTESIAN_POINT('Ctrl Pts',(-3.67768458500006,5.2,-1.70912216700001));
#316741=CARTESIAN_POINT('Ctrl Pts',(-3.67768458500006,2.2,-1.70912216700001));
#316742=CARTESIAN_POINT('Ctrl Pts',(-3.67840760000006,12.2,-1.70962788200002));
#316743=CARTESIAN_POINT('Ctrl Pts',(-3.67840760000006,5.2,-1.70962788200002));
#316744=CARTESIAN_POINT('Ctrl Pts',(-3.67840760000006,2.2,-1.70962788200002));
#316745=CARTESIAN_POINT('Ctrl Pts',(-3.67913463400006,12.2,-1.71013775900001));
#316746=CARTESIAN_POINT('Ctrl Pts',(-3.67913463400006,5.2,-1.71013775900001));
#316747=CARTESIAN_POINT('Ctrl Pts',(-3.67913463400006,2.2,-1.71013775900001));
#316748=CARTESIAN_POINT('Ctrl Pts',(-3.67986567000006,12.2,-1.71065180300001));
#316749=CARTESIAN_POINT('Ctrl Pts',(-3.67986567000006,5.2,-1.71065180300001));
#316750=CARTESIAN_POINT('Ctrl Pts',(-3.67986567000006,2.2,-1.71065180300001));
#316751=CARTESIAN_POINT('Ctrl Pts',(-3.68060069000006,12.2,-1.71117001800001));
#316752=CARTESIAN_POINT('Ctrl Pts',(-3.68060069000006,5.2,-1.71117001800001));
#316753=CARTESIAN_POINT('Ctrl Pts',(-3.68060069000006,2.2,-1.71117001800001));
#316754=CARTESIAN_POINT('Ctrl Pts',(-3.68133967700006,12.2,-1.71169240800001));
#316755=CARTESIAN_POINT('Ctrl Pts',(-3.68133967700006,5.2,-1.71169240800001));
#316756=CARTESIAN_POINT('Ctrl Pts',(-3.68133967700006,2.2,-1.71169240800001));
#316757=CARTESIAN_POINT('Ctrl Pts',(-3.68208261700006,12.2,-1.71221897900002));
#316758=CARTESIAN_POINT('Ctrl Pts',(-3.68208261700006,5.2,-1.71221897900002));
#316759=CARTESIAN_POINT('Ctrl Pts',(-3.68208261700006,2.2,-1.71221897900002));
#316760=CARTESIAN_POINT('Ctrl Pts',(-3.68282949100006,12.2,-1.71274973600001));
#316761=CARTESIAN_POINT('Ctrl Pts',(-3.68282949100006,5.2,-1.71274973600001));
#316762=CARTESIAN_POINT('Ctrl Pts',(-3.68282949100006,2.2,-1.71274973600001));
#316763=CARTESIAN_POINT('Ctrl Pts',(-3.68358028100006,12.2,-1.71328468000001));
#316764=CARTESIAN_POINT('Ctrl Pts',(-3.68358028100006,5.2,-1.71328468000001));
#316765=CARTESIAN_POINT('Ctrl Pts',(-3.68358028100006,2.2,-1.71328468000001));
#316766=CARTESIAN_POINT('Ctrl Pts',(-3.68433497400006,12.2,-1.71382381800001));
#316767=CARTESIAN_POINT('Ctrl Pts',(-3.68433497400006,5.2,-1.71382381800001));
#316768=CARTESIAN_POINT('Ctrl Pts',(-3.68433497400006,2.2,-1.71382381800001));
#316769=CARTESIAN_POINT('Ctrl Pts',(-3.68509354900006,12.2,-1.71436715500001));
#316770=CARTESIAN_POINT('Ctrl Pts',(-3.68509354900006,5.2,-1.71436715500001));
#316771=CARTESIAN_POINT('Ctrl Pts',(-3.68509354900006,2.2,-1.71436715500001));
#316772=CARTESIAN_POINT('Ctrl Pts',(-3.68585599300006,12.2,-1.71491469300001));
#316773=CARTESIAN_POINT('Ctrl Pts',(-3.68585599300006,5.2,-1.71491469300001));
#316774=CARTESIAN_POINT('Ctrl Pts',(-3.68585599300006,2.2,-1.71491469300001));
#316775=CARTESIAN_POINT('Ctrl Pts',(-3.68662228700006,12.2,-1.71546643800002));
#316776=CARTESIAN_POINT('Ctrl Pts',(-3.68662228700006,5.2,-1.71546643800002));
#316777=CARTESIAN_POINT('Ctrl Pts',(-3.68662228700006,2.2,-1.71546643800002));
#316778=CARTESIAN_POINT('Ctrl Pts',(-3.68739241600006,12.2,-1.71602239300002));
#316779=CARTESIAN_POINT('Ctrl Pts',(-3.68739241600006,5.2,-1.71602239300002));
#316780=CARTESIAN_POINT('Ctrl Pts',(-3.68739241600006,2.2,-1.71602239300002));
#316781=CARTESIAN_POINT('Ctrl Pts',(-3.68816636300005,12.2,-1.71658256400002));
#316782=CARTESIAN_POINT('Ctrl Pts',(-3.68816636300005,5.2,-1.71658256400002));
#316783=CARTESIAN_POINT('Ctrl Pts',(-3.68816636300005,2.2,-1.71658256400002));
#316784=CARTESIAN_POINT('Ctrl Pts',(-3.68894411100006,12.2,-1.71714695400001));
#316785=CARTESIAN_POINT('Ctrl Pts',(-3.68894411100006,5.2,-1.71714695400001));
#316786=CARTESIAN_POINT('Ctrl Pts',(-3.68894411100006,2.2,-1.71714695400001));
#316787=CARTESIAN_POINT('Ctrl Pts',(-3.68972564300006,12.2,-1.71771556700001));
#316788=CARTESIAN_POINT('Ctrl Pts',(-3.68972564300006,5.2,-1.71771556700001));
#316789=CARTESIAN_POINT('Ctrl Pts',(-3.68972564300006,2.2,-1.71771556700001));
#316790=CARTESIAN_POINT('Ctrl Pts',(-3.69051094500006,12.2,-1.71828840700002));
#316791=CARTESIAN_POINT('Ctrl Pts',(-3.69051094500006,5.2,-1.71828840700002));
#316792=CARTESIAN_POINT('Ctrl Pts',(-3.69051094500006,2.2,-1.71828840700002));
#316793=CARTESIAN_POINT('Ctrl Pts',(-3.69129999800006,12.2,-1.71886548000002));
#316794=CARTESIAN_POINT('Ctrl Pts',(-3.69129999800006,5.2,-1.71886548000002));
#316795=CARTESIAN_POINT('Ctrl Pts',(-3.69129999800006,2.2,-1.71886548000002));
#316796=CARTESIAN_POINT('Ctrl Pts',(-3.69209278600006,12.2,-1.71944678700001));
#316797=CARTESIAN_POINT('Ctrl Pts',(-3.69209278600006,5.2,-1.71944678700001));
#316798=CARTESIAN_POINT('Ctrl Pts',(-3.69209278600006,2.2,-1.71944678700001));
#316799=CARTESIAN_POINT('Ctrl Pts',(-3.69288929500006,12.2,-1.72003233500002));
#316800=CARTESIAN_POINT('Ctrl Pts',(-3.69288929500006,5.2,-1.72003233500002));
#316801=CARTESIAN_POINT('Ctrl Pts',(-3.69288929500006,2.2,-1.72003233500002));
#316802=CARTESIAN_POINT('Ctrl Pts',(-3.69368950600006,12.2,-1.72062212600002));
#316803=CARTESIAN_POINT('Ctrl Pts',(-3.69368950600006,5.2,-1.72062212600002));
#316804=CARTESIAN_POINT('Ctrl Pts',(-3.69368950600006,2.2,-1.72062212600002));
#316805=CARTESIAN_POINT('Ctrl Pts',(-3.69449340500006,12.2,-1.72121616400001));
#316806=CARTESIAN_POINT('Ctrl Pts',(-3.69449340500006,5.2,-1.72121616400001));
#316807=CARTESIAN_POINT('Ctrl Pts',(-3.69449340500006,2.2,-1.72121616400001));
#316808=CARTESIAN_POINT('Ctrl Pts',(-3.69530097400006,12.2,-1.72181445400001));
#316809=CARTESIAN_POINT('Ctrl Pts',(-3.69530097400006,5.2,-1.72181445400001));
#316810=CARTESIAN_POINT('Ctrl Pts',(-3.69530097400006,2.2,-1.72181445400001));
#316811=CARTESIAN_POINT('Ctrl Pts',(-3.69611219600006,12.2,-1.72241700100002));
#316812=CARTESIAN_POINT('Ctrl Pts',(-3.69611219600006,5.2,-1.72241700100002));
#316813=CARTESIAN_POINT('Ctrl Pts',(-3.69611219600006,2.2,-1.72241700100002));
#316814=CARTESIAN_POINT('Ctrl Pts',(-3.69692705800006,12.2,-1.72302380600001));
#316815=CARTESIAN_POINT('Ctrl Pts',(-3.69692705800006,5.2,-1.72302380600001));
#316816=CARTESIAN_POINT('Ctrl Pts',(-3.69692705800006,2.2,-1.72302380600001));
#316817=CARTESIAN_POINT('Ctrl Pts',(-3.69774554200006,12.2,-1.72363487400002));
#316818=CARTESIAN_POINT('Ctrl Pts',(-3.69774554200006,5.2,-1.72363487400002));
#316819=CARTESIAN_POINT('Ctrl Pts',(-3.69774554200006,2.2,-1.72363487400002));
#316820=CARTESIAN_POINT('Ctrl Pts',(-3.69856763300006,12.2,-1.72425021000001));
#316821=CARTESIAN_POINT('Ctrl Pts',(-3.69856763300006,5.2,-1.72425021000001));
#316822=CARTESIAN_POINT('Ctrl Pts',(-3.69856763300006,2.2,-1.72425021000001));
#316823=CARTESIAN_POINT('Ctrl Pts',(-3.69939331300006,12.2,-1.72486981600001));
#316824=CARTESIAN_POINT('Ctrl Pts',(-3.69939331300006,5.2,-1.72486981600001));
#316825=CARTESIAN_POINT('Ctrl Pts',(-3.69939331300006,2.2,-1.72486981600001));
#316826=CARTESIAN_POINT('Ctrl Pts',(-3.70022256800006,12.2,-1.72549369700001));
#316827=CARTESIAN_POINT('Ctrl Pts',(-3.70022256800006,5.2,-1.72549369700001));
#316828=CARTESIAN_POINT('Ctrl Pts',(-3.70022256800006,2.2,-1.72549369700001));
#316829=CARTESIAN_POINT('Ctrl Pts',(-3.70105538100006,12.2,-1.72612185600002));
#316830=CARTESIAN_POINT('Ctrl Pts',(-3.70105538100006,5.2,-1.72612185600002));
#316831=CARTESIAN_POINT('Ctrl Pts',(-3.70105538100006,2.2,-1.72612185600002));
#316832=CARTESIAN_POINT('Ctrl Pts',(-3.70189173600005,12.2,-1.72675429800002));
#316833=CARTESIAN_POINT('Ctrl Pts',(-3.70189173600005,5.2,-1.72675429800002));
#316834=CARTESIAN_POINT('Ctrl Pts',(-3.70189173600005,2.2,-1.72675429800002));
#316835=CARTESIAN_POINT('Ctrl Pts',(-3.70273161800006,12.2,-1.72739102500001));
#316836=CARTESIAN_POINT('Ctrl Pts',(-3.70273161800006,5.2,-1.72739102500001));
#316837=CARTESIAN_POINT('Ctrl Pts',(-3.70273161800006,2.2,-1.72739102500001));
#316838=CARTESIAN_POINT('Ctrl Pts',(-3.70357501000006,12.2,-1.72803204100001));
#316839=CARTESIAN_POINT('Ctrl Pts',(-3.70357501000006,5.2,-1.72803204100001));
#316840=CARTESIAN_POINT('Ctrl Pts',(-3.70357501000006,2.2,-1.72803204100001));
#316841=CARTESIAN_POINT('Ctrl Pts',(-3.70442189700006,12.2,-1.72867735000001));
#316842=CARTESIAN_POINT('Ctrl Pts',(-3.70442189700006,5.2,-1.72867735000001));
#316843=CARTESIAN_POINT('Ctrl Pts',(-3.70442189700006,2.2,-1.72867735000001));
#316844=CARTESIAN_POINT('Ctrl Pts',(-3.70527226300006,12.2,-1.72932695700001));
#316845=CARTESIAN_POINT('Ctrl Pts',(-3.70527226300006,5.2,-1.72932695700001));
#316846=CARTESIAN_POINT('Ctrl Pts',(-3.70527226300006,2.2,-1.72932695700001));
#316847=CARTESIAN_POINT('Ctrl Pts',(-3.70612609200006,12.2,-1.72998086300002));
#316848=CARTESIAN_POINT('Ctrl Pts',(-3.70612609200006,5.2,-1.72998086300002));
#316849=CARTESIAN_POINT('Ctrl Pts',(-3.70612609200006,2.2,-1.72998086300002));
#316850=CARTESIAN_POINT('Ctrl Pts',(-3.70698336900006,12.2,-1.73063907300001));
#316851=CARTESIAN_POINT('Ctrl Pts',(-3.70698336900006,5.2,-1.73063907300001));
#316852=CARTESIAN_POINT('Ctrl Pts',(-3.70698336900006,2.2,-1.73063907300001));
#316853=CARTESIAN_POINT('Ctrl Pts',(-3.70784407800006,12.2,-1.73130159000001));
#316854=CARTESIAN_POINT('Ctrl Pts',(-3.70784407800006,5.2,-1.73130159000001));
#316855=CARTESIAN_POINT('Ctrl Pts',(-3.70784407800006,2.2,-1.73130159000001));
#316856=CARTESIAN_POINT('Ctrl Pts',(-3.70870820300006,12.2,-1.73196841700001));
#316857=CARTESIAN_POINT('Ctrl Pts',(-3.70870820300006,5.2,-1.73196841700001));
#316858=CARTESIAN_POINT('Ctrl Pts',(-3.70870820300006,2.2,-1.73196841700001));
#316859=CARTESIAN_POINT('Ctrl Pts',(-3.70957572800005,12.2,-1.73263955900001));
#316860=CARTESIAN_POINT('Ctrl Pts',(-3.70957572800005,5.2,-1.73263955900001));
#316861=CARTESIAN_POINT('Ctrl Pts',(-3.70957572800005,2.2,-1.73263955900001));
#316862=CARTESIAN_POINT('Ctrl Pts',(-3.71044663900006,12.2,-1.73331501800002));
#316863=CARTESIAN_POINT('Ctrl Pts',(-3.71044663900006,5.2,-1.73331501800002));
#316864=CARTESIAN_POINT('Ctrl Pts',(-3.71044663900006,2.2,-1.73331501800002));
#316865=CARTESIAN_POINT('Ctrl Pts',(-3.71132091800006,12.2,-1.73399479900001));
#316866=CARTESIAN_POINT('Ctrl Pts',(-3.71132091800006,5.2,-1.73399479900001));
#316867=CARTESIAN_POINT('Ctrl Pts',(-3.71132091800006,2.2,-1.73399479900001));
#316868=CARTESIAN_POINT('Ctrl Pts',(-3.71219855200006,12.2,-1.73467890300001));
#316869=CARTESIAN_POINT('Ctrl Pts',(-3.71219855200006,5.2,-1.73467890300001));
#316870=CARTESIAN_POINT('Ctrl Pts',(-3.71219855200006,2.2,-1.73467890300001));
#316871=CARTESIAN_POINT('Ctrl Pts',(-3.71307952400006,12.2,-1.73536733500002));
#316872=CARTESIAN_POINT('Ctrl Pts',(-3.71307952400006,5.2,-1.73536733500002));
#316873=CARTESIAN_POINT('Ctrl Pts',(-3.71307952400006,2.2,-1.73536733500002));
#316874=CARTESIAN_POINT('Ctrl Pts',(-3.71396382000006,12.2,-1.73606009800002));
#316875=CARTESIAN_POINT('Ctrl Pts',(-3.71396382000006,5.2,-1.73606009800002));
#316876=CARTESIAN_POINT('Ctrl Pts',(-3.71396382000006,2.2,-1.73606009800002));
#316877=CARTESIAN_POINT('Ctrl Pts',(-3.71485142300005,12.2,-1.73675719400002));
#316878=CARTESIAN_POINT('Ctrl Pts',(-3.71485142300005,5.2,-1.73675719400002));
#316879=CARTESIAN_POINT('Ctrl Pts',(-3.71485142300005,2.2,-1.73675719400002));
#316880=CARTESIAN_POINT('Ctrl Pts',(-3.71574231800006,12.2,-1.73745862900001));
#316881=CARTESIAN_POINT('Ctrl Pts',(-3.71574231800006,5.2,-1.73745862900001));
#316882=CARTESIAN_POINT('Ctrl Pts',(-3.71574231800006,2.2,-1.73745862900001));
#316883=CARTESIAN_POINT('Ctrl Pts',(-3.71663649000006,12.2,-1.73816440400001));
#316884=CARTESIAN_POINT('Ctrl Pts',(-3.71663649000006,5.2,-1.73816440400001));
#316885=CARTESIAN_POINT('Ctrl Pts',(-3.71663649000006,2.2,-1.73816440400001));
#316886=CARTESIAN_POINT('Ctrl Pts',(-3.71753392300006,12.2,-1.73887452300002));
#316887=CARTESIAN_POINT('Ctrl Pts',(-3.71753392300006,5.2,-1.73887452300002));
#316888=CARTESIAN_POINT('Ctrl Pts',(-3.71753392300006,2.2,-1.73887452300002));
#316889=CARTESIAN_POINT('Ctrl Pts',(-3.71843460200005,12.2,-1.73958898900001));
#316890=CARTESIAN_POINT('Ctrl Pts',(-3.71843460200005,5.2,-1.73958898900001));
#316891=CARTESIAN_POINT('Ctrl Pts',(-3.71843460200005,2.2,-1.73958898900001));
#316892=CARTESIAN_POINT('Ctrl Pts',(-3.71933851300006,12.2,-1.74030780600001));
#316893=CARTESIAN_POINT('Ctrl Pts',(-3.71933851300006,5.2,-1.74030780600001));
#316894=CARTESIAN_POINT('Ctrl Pts',(-3.71933851300006,2.2,-1.74030780600001));
#316895=CARTESIAN_POINT('Ctrl Pts',(-3.72024564000006,12.2,-1.74103097500002));
#316896=CARTESIAN_POINT('Ctrl Pts',(-3.72024564000006,5.2,-1.74103097500002));
#316897=CARTESIAN_POINT('Ctrl Pts',(-3.72024564000006,2.2,-1.74103097500002));
#316898=CARTESIAN_POINT('Ctrl Pts',(-3.72115596700006,12.2,-1.74175850000001));
#316899=CARTESIAN_POINT('Ctrl Pts',(-3.72115596700006,5.2,-1.74175850000001));
#316900=CARTESIAN_POINT('Ctrl Pts',(-3.72115596700006,2.2,-1.74175850000001));
#316901=CARTESIAN_POINT('Ctrl Pts',(-3.72206947900006,12.2,-1.74249038600002));
#316902=CARTESIAN_POINT('Ctrl Pts',(-3.72206947900006,5.2,-1.74249038600002));
#316903=CARTESIAN_POINT('Ctrl Pts',(-3.72206947900006,2.2,-1.74249038600002));
#316904=CARTESIAN_POINT('Ctrl Pts',(-3.72298616200006,12.2,-1.74322663300002));
#316905=CARTESIAN_POINT('Ctrl Pts',(-3.72298616200006,5.2,-1.74322663300002));
#316906=CARTESIAN_POINT('Ctrl Pts',(-3.72298616200006,2.2,-1.74322663300002));
#316907=CARTESIAN_POINT('Ctrl Pts',(-3.72390600000006,12.2,-1.74396724600001));
#316908=CARTESIAN_POINT('Ctrl Pts',(-3.72390600000006,5.2,-1.74396724600001));
#316909=CARTESIAN_POINT('Ctrl Pts',(-3.72390600000006,2.2,-1.74396724600001));
#316910=CARTESIAN_POINT('Ctrl Pts',(-3.72482897800006,12.2,-1.74471222700001));
#316911=CARTESIAN_POINT('Ctrl Pts',(-3.72482897800006,5.2,-1.74471222700001));
#316912=CARTESIAN_POINT('Ctrl Pts',(-3.72482897800006,2.2,-1.74471222700001));
#316913=CARTESIAN_POINT('Ctrl Pts',(-3.72575508100006,12.2,-1.74546158000001));
#316914=CARTESIAN_POINT('Ctrl Pts',(-3.72575508100006,5.2,-1.74546158000001));
#316915=CARTESIAN_POINT('Ctrl Pts',(-3.72575508100006,2.2,-1.74546158000001));
#316916=CARTESIAN_POINT('Ctrl Pts',(-3.72668429500006,12.2,-1.74621530700001));
#316917=CARTESIAN_POINT('Ctrl Pts',(-3.72668429500006,5.2,-1.74621530700001));
#316918=CARTESIAN_POINT('Ctrl Pts',(-3.72668429500006,2.2,-1.74621530700001));
#316919=CARTESIAN_POINT('Ctrl Pts',(-3.72761660300006,12.2,-1.74697341100002));
#316920=CARTESIAN_POINT('Ctrl Pts',(-3.72761660300006,5.2,-1.74697341100002));
#316921=CARTESIAN_POINT('Ctrl Pts',(-3.72761660300006,2.2,-1.74697341100002));
#316922=CARTESIAN_POINT('Ctrl Pts',(-3.72855199100006,12.2,-1.74773589500001));
#316923=CARTESIAN_POINT('Ctrl Pts',(-3.72855199100006,5.2,-1.74773589500001));
#316924=CARTESIAN_POINT('Ctrl Pts',(-3.72855199100006,2.2,-1.74773589500001));
#316925=CARTESIAN_POINT('Ctrl Pts',(-3.72949044500006,12.2,-1.74850276200001));
#316926=CARTESIAN_POINT('Ctrl Pts',(-3.72949044500006,5.2,-1.74850276200001));
#316927=CARTESIAN_POINT('Ctrl Pts',(-3.72949044500006,2.2,-1.74850276200001));
#316928=CARTESIAN_POINT('Ctrl Pts',(-3.73043194900006,12.2,-1.74927401600002));
#316929=CARTESIAN_POINT('Ctrl Pts',(-3.73043194900006,5.2,-1.74927401600002));
#316930=CARTESIAN_POINT('Ctrl Pts',(-3.73043194900006,2.2,-1.74927401600002));
#316931=CARTESIAN_POINT('Ctrl Pts',(-3.73137648800006,12.2,-1.75004965700001));
#316932=CARTESIAN_POINT('Ctrl Pts',(-3.73137648800006,5.2,-1.75004965700001));
#316933=CARTESIAN_POINT('Ctrl Pts',(-3.73137648800006,2.2,-1.75004965700001));
#316934=CARTESIAN_POINT('Ctrl Pts',(-3.73232404900006,12.2,-1.75082969000002));
#316935=CARTESIAN_POINT('Ctrl Pts',(-3.73232404900006,5.2,-1.75082969000002));
#316936=CARTESIAN_POINT('Ctrl Pts',(-3.73232404900006,2.2,-1.75082969000002));
#316937=CARTESIAN_POINT('Ctrl Pts',(-3.73327461500006,12.2,-1.75161411600001));
#316938=CARTESIAN_POINT('Ctrl Pts',(-3.73327461500006,5.2,-1.75161411600001));
#316939=CARTESIAN_POINT('Ctrl Pts',(-3.73327461500006,2.2,-1.75161411600001));
#316940=CARTESIAN_POINT('Ctrl Pts',(-3.73422817300006,12.2,-1.75240294000002));
#316941=CARTESIAN_POINT('Ctrl Pts',(-3.73422817300006,5.2,-1.75240294000002));
#316942=CARTESIAN_POINT('Ctrl Pts',(-3.73422817300006,2.2,-1.75240294000002));
#316943=CARTESIAN_POINT('Ctrl Pts',(-3.73518470700006,12.2,-1.75319616300001));
#316944=CARTESIAN_POINT('Ctrl Pts',(-3.73518470700006,5.2,-1.75319616300001));
#316945=CARTESIAN_POINT('Ctrl Pts',(-3.73518470700006,2.2,-1.75319616300001));
#316946=CARTESIAN_POINT('Ctrl Pts',(-3.73614420300005,12.2,-1.75399378800002));
#316947=CARTESIAN_POINT('Ctrl Pts',(-3.73614420300005,5.2,-1.75399378800002));
#316948=CARTESIAN_POINT('Ctrl Pts',(-3.73614420300005,2.2,-1.75399378800002));
#316949=CARTESIAN_POINT('Ctrl Pts',(-3.73710664500006,12.2,-1.75479581800001));
#316950=CARTESIAN_POINT('Ctrl Pts',(-3.73710664500006,5.2,-1.75479581800001));
#316951=CARTESIAN_POINT('Ctrl Pts',(-3.73710664500006,2.2,-1.75479581800001));
#316952=CARTESIAN_POINT('Ctrl Pts',(-3.73807202000005,12.2,-1.75560225600002));
#316953=CARTESIAN_POINT('Ctrl Pts',(-3.73807202000005,5.2,-1.75560225600002));
#316954=CARTESIAN_POINT('Ctrl Pts',(-3.73807202000005,2.2,-1.75560225600002));
#316955=CARTESIAN_POINT('Ctrl Pts',(-3.73904031300006,12.2,-1.75641310200001));
#316956=CARTESIAN_POINT('Ctrl Pts',(-3.73904031300006,5.2,-1.75641310200001));
#316957=CARTESIAN_POINT('Ctrl Pts',(-3.73904031300006,2.2,-1.75641310200001));
#316958=CARTESIAN_POINT('Ctrl Pts',(-3.74001150900006,12.2,-1.75722836200002));
#316959=CARTESIAN_POINT('Ctrl Pts',(-3.74001150900006,5.2,-1.75722836200002));
#316960=CARTESIAN_POINT('Ctrl Pts',(-3.74001150900006,2.2,-1.75722836200002));
#316961=CARTESIAN_POINT('Ctrl Pts',(-3.74098559300006,12.2,-1.75804803700002));
#316962=CARTESIAN_POINT('Ctrl Pts',(-3.74098559300006,5.2,-1.75804803700002));
#316963=CARTESIAN_POINT('Ctrl Pts',(-3.74098559300006,2.2,-1.75804803700002));
#316964=CARTESIAN_POINT('Ctrl Pts',(-3.74196255300006,12.2,-1.75887213000001));
#316965=CARTESIAN_POINT('Ctrl Pts',(-3.74196255300006,5.2,-1.75887213000001));
#316966=CARTESIAN_POINT('Ctrl Pts',(-3.74196255300006,2.2,-1.75887213000001));
#316967=CARTESIAN_POINT('Ctrl Pts',(-3.74294237100006,12.2,-1.75970064200001));
#316968=CARTESIAN_POINT('Ctrl Pts',(-3.74294237100006,5.2,-1.75970064200001));
#316969=CARTESIAN_POINT('Ctrl Pts',(-3.74294237100006,2.2,-1.75970064200001));
#316970=CARTESIAN_POINT('Ctrl Pts',(-3.74392503400006,12.2,-1.76053357700001));
#316971=CARTESIAN_POINT('Ctrl Pts',(-3.74392503400006,5.2,-1.76053357700001));
#316972=CARTESIAN_POINT('Ctrl Pts',(-3.74392503400006,2.2,-1.76053357700001));
#316973=CARTESIAN_POINT('Ctrl Pts',(-3.74491052900006,12.2,-1.76137093700001));
#316974=CARTESIAN_POINT('Ctrl Pts',(-3.74491052900006,5.2,-1.76137093700001));
#316975=CARTESIAN_POINT('Ctrl Pts',(-3.74491052900006,2.2,-1.76137093700001));
#316976=CARTESIAN_POINT('Ctrl Pts',(-3.74589884000006,12.2,-1.76221272500001));
#316977=CARTESIAN_POINT('Ctrl Pts',(-3.74589884000006,5.2,-1.76221272500001));
#316978=CARTESIAN_POINT('Ctrl Pts',(-3.74589884000006,2.2,-1.76221272500001));
#316979=CARTESIAN_POINT('Ctrl Pts',(-3.74688995300006,12.2,-1.76305894300001));
#316980=CARTESIAN_POINT('Ctrl Pts',(-3.74688995300006,5.2,-1.76305894300001));
#316981=CARTESIAN_POINT('Ctrl Pts',(-3.74688995300006,2.2,-1.76305894300001));
#316982=CARTESIAN_POINT('Ctrl Pts',(-3.74788385300006,12.2,-1.76390959200001));
#316983=CARTESIAN_POINT('Ctrl Pts',(-3.74788385300006,5.2,-1.76390959200001));
#316984=CARTESIAN_POINT('Ctrl Pts',(-3.74788385300006,2.2,-1.76390959200001));
#316985=CARTESIAN_POINT('Ctrl Pts',(-3.74888052700006,12.2,-1.76476467600001));
#316986=CARTESIAN_POINT('Ctrl Pts',(-3.74888052700006,5.2,-1.76476467600001));
#316987=CARTESIAN_POINT('Ctrl Pts',(-3.74888052700006,2.2,-1.76476467600001));
#316988=CARTESIAN_POINT('Ctrl Pts',(-3.74987996000006,12.2,-1.76562419800002));
#316989=CARTESIAN_POINT('Ctrl Pts',(-3.74987996000006,5.2,-1.76562419800002));
#316990=CARTESIAN_POINT('Ctrl Pts',(-3.74987996000006,2.2,-1.76562419800002));
#316991=CARTESIAN_POINT('Ctrl Pts',(-3.75088213700006,12.2,-1.76648815800001));
#316992=CARTESIAN_POINT('Ctrl Pts',(-3.75088213700006,5.2,-1.76648815800001));
#316993=CARTESIAN_POINT('Ctrl Pts',(-3.75088213700006,2.2,-1.76648815800001));
#316994=CARTESIAN_POINT('Ctrl Pts',(-3.75188704500006,12.2,-1.76735656000002));
#316995=CARTESIAN_POINT('Ctrl Pts',(-3.75188704500006,5.2,-1.76735656000002));
#316996=CARTESIAN_POINT('Ctrl Pts',(-3.75188704500006,2.2,-1.76735656000002));
#316997=CARTESIAN_POINT('Ctrl Pts',(-3.75289466900006,12.2,-1.76822940400001));
#316998=CARTESIAN_POINT('Ctrl Pts',(-3.75289466900006,5.2,-1.76822940400001));
#316999=CARTESIAN_POINT('Ctrl Pts',(-3.75289466900006,2.2,-1.76822940400001));
#317000=CARTESIAN_POINT('Ctrl Pts',(-3.75390499500006,12.2,-1.76910669600002));
#317001=CARTESIAN_POINT('Ctrl Pts',(-3.75390499500006,5.2,-1.76910669600002));
#317002=CARTESIAN_POINT('Ctrl Pts',(-3.75390499500006,2.2,-1.76910669600002));
#317003=CARTESIAN_POINT('Ctrl Pts',(-3.75491800900006,12.2,-1.76998843600002));
#317004=CARTESIAN_POINT('Ctrl Pts',(-3.75491800900006,5.2,-1.76998843600002));
#317005=CARTESIAN_POINT('Ctrl Pts',(-3.75491800900006,2.2,-1.76998843600002));
#317006=CARTESIAN_POINT('Ctrl Pts',(-3.75593369800006,12.2,-1.77087462600001));
#317007=CARTESIAN_POINT('Ctrl Pts',(-3.75593369800006,5.2,-1.77087462600001));
#317008=CARTESIAN_POINT('Ctrl Pts',(-3.75593369800006,2.2,-1.77087462600001));
#317009=CARTESIAN_POINT('Ctrl Pts',(-3.75695204500006,12.2,-1.77176526800002));
#317010=CARTESIAN_POINT('Ctrl Pts',(-3.75695204500006,5.2,-1.77176526800002));
#317011=CARTESIAN_POINT('Ctrl Pts',(-3.75695204500006,2.2,-1.77176526800002));
#317012=CARTESIAN_POINT('Ctrl Pts',(-3.75797303800006,12.2,-1.77266036500002));
#317013=CARTESIAN_POINT('Ctrl Pts',(-3.75797303800006,5.2,-1.77266036500002));
#317014=CARTESIAN_POINT('Ctrl Pts',(-3.75797303800006,2.2,-1.77266036500002));
#317015=CARTESIAN_POINT('Ctrl Pts',(-3.75899666400006,12.2,-1.77355991900002));
#317016=CARTESIAN_POINT('Ctrl Pts',(-3.75899666400006,5.2,-1.77355991900002));
#317017=CARTESIAN_POINT('Ctrl Pts',(-3.75899666400006,2.2,-1.77355991900002));
#317018=CARTESIAN_POINT('Ctrl Pts',(-3.76002290600006,12.2,-1.77446393100002));
#317019=CARTESIAN_POINT('Ctrl Pts',(-3.76002290600006,5.2,-1.77446393100002));
#317020=CARTESIAN_POINT('Ctrl Pts',(-3.76002290600006,2.2,-1.77446393100002));
#317021=CARTESIAN_POINT('Ctrl Pts',(-3.76105175200006,12.2,-1.77537240500001));
#317022=CARTESIAN_POINT('Ctrl Pts',(-3.76105175200006,5.2,-1.77537240500001));
#317023=CARTESIAN_POINT('Ctrl Pts',(-3.76105175200006,2.2,-1.77537240500001));
#317024=CARTESIAN_POINT('Ctrl Pts',(-3.76208318700006,12.2,-1.77628534100001));
#317025=CARTESIAN_POINT('Ctrl Pts',(-3.76208318700006,5.2,-1.77628534100001));
#317026=CARTESIAN_POINT('Ctrl Pts',(-3.76208318700006,2.2,-1.77628534100001));
#317027=CARTESIAN_POINT('Ctrl Pts',(-3.76311719900006,12.2,-1.77720274300002));
#317028=CARTESIAN_POINT('Ctrl Pts',(-3.76311719900006,5.2,-1.77720274300002));
#317029=CARTESIAN_POINT('Ctrl Pts',(-3.76311719900006,2.2,-1.77720274300002));
#317030=CARTESIAN_POINT('Ctrl Pts',(-3.76415377300006,12.2,-1.77812461100002));
#317031=CARTESIAN_POINT('Ctrl Pts',(-3.76415377300006,5.2,-1.77812461100002));
#317032=CARTESIAN_POINT('Ctrl Pts',(-3.76415377300006,2.2,-1.77812461100002));
#317033=CARTESIAN_POINT('Ctrl Pts',(-3.76519289400005,12.2,-1.77905094800002));
#317034=CARTESIAN_POINT('Ctrl Pts',(-3.76519289400005,5.2,-1.77905094800002));
#317035=CARTESIAN_POINT('Ctrl Pts',(-3.76519289400005,2.2,-1.77905094800002));
#317036=CARTESIAN_POINT('Ctrl Pts',(-3.76623455000006,12.2,-1.77998175700001));
#317037=CARTESIAN_POINT('Ctrl Pts',(-3.76623455000006,5.2,-1.77998175700001));
#317038=CARTESIAN_POINT('Ctrl Pts',(-3.76623455000006,2.2,-1.77998175700001));
#317039=CARTESIAN_POINT('Ctrl Pts',(-3.76727872400005,12.2,-1.78091703800002));
#317040=CARTESIAN_POINT('Ctrl Pts',(-3.76727872400005,5.2,-1.78091703800002));
#317041=CARTESIAN_POINT('Ctrl Pts',(-3.76727872400005,2.2,-1.78091703800002));
#317042=CARTESIAN_POINT('Ctrl Pts',(-3.76832540600006,12.2,-1.78185679400002));
#317043=CARTESIAN_POINT('Ctrl Pts',(-3.76832540600006,5.2,-1.78185679400002));
#317044=CARTESIAN_POINT('Ctrl Pts',(-3.76832540600006,2.2,-1.78185679400002));
#317045=CARTESIAN_POINT('Ctrl Pts',(-3.76937458100006,12.2,-1.78280102600001));
#317046=CARTESIAN_POINT('Ctrl Pts',(-3.76937458100006,5.2,-1.78280102600001));
#317047=CARTESIAN_POINT('Ctrl Pts',(-3.76937458100006,2.2,-1.78280102600001));
#317048=CARTESIAN_POINT('Ctrl Pts',(-3.77042623500006,12.2,-1.78374973700001));
#317049=CARTESIAN_POINT('Ctrl Pts',(-3.77042623500006,5.2,-1.78374973700001));
#317050=CARTESIAN_POINT('Ctrl Pts',(-3.77042623500006,2.2,-1.78374973700001));
#317051=CARTESIAN_POINT('Ctrl Pts',(-3.77148035400006,12.2,-1.78470292800001));
#317052=CARTESIAN_POINT('Ctrl Pts',(-3.77148035400006,5.2,-1.78470292800001));
#317053=CARTESIAN_POINT('Ctrl Pts',(-3.77148035400006,2.2,-1.78470292800001));
#317054=CARTESIAN_POINT('Ctrl Pts',(-3.77253692400005,12.2,-1.78566060100001));
#317055=CARTESIAN_POINT('Ctrl Pts',(-3.77253692400005,5.2,-1.78566060100001));
#317056=CARTESIAN_POINT('Ctrl Pts',(-3.77253692400005,2.2,-1.78566060100001));
#317057=CARTESIAN_POINT('Ctrl Pts',(-3.77359593200006,12.2,-1.78662275800002));
#317058=CARTESIAN_POINT('Ctrl Pts',(-3.77359593200006,5.2,-1.78662275800002));
#317059=CARTESIAN_POINT('Ctrl Pts',(-3.77359593200006,2.2,-1.78662275800002));
#317060=CARTESIAN_POINT('Ctrl Pts',(-3.77465736400006,12.2,-1.78758940200002));
#317061=CARTESIAN_POINT('Ctrl Pts',(-3.77465736400006,5.2,-1.78758940200002));
#317062=CARTESIAN_POINT('Ctrl Pts',(-3.77465736400006,2.2,-1.78758940200002));
#317063=CARTESIAN_POINT('Ctrl Pts',(-3.77572120600006,12.2,-1.78856053200001));
#317064=CARTESIAN_POINT('Ctrl Pts',(-3.77572120600006,5.2,-1.78856053200001));
#317065=CARTESIAN_POINT('Ctrl Pts',(-3.77572120600006,2.2,-1.78856053200001));
#317066=CARTESIAN_POINT('Ctrl Pts',(-3.77678744700006,12.2,-1.78953615200002));
#317067=CARTESIAN_POINT('Ctrl Pts',(-3.77678744700006,5.2,-1.78953615200002));
#317068=CARTESIAN_POINT('Ctrl Pts',(-3.77678744700006,2.2,-1.78953615200002));
#317069=CARTESIAN_POINT('Ctrl Pts',(-3.77785607000006,12.2,-1.79051626300001));
#317070=CARTESIAN_POINT('Ctrl Pts',(-3.77785607000006,5.2,-1.79051626300001));
#317071=CARTESIAN_POINT('Ctrl Pts',(-3.77785607000006,2.2,-1.79051626300001));
#317072=CARTESIAN_POINT('Ctrl Pts',(-3.77892706200006,12.2,-1.79150086600002));
#317073=CARTESIAN_POINT('Ctrl Pts',(-3.77892706200006,5.2,-1.79150086600002));
#317074=CARTESIAN_POINT('Ctrl Pts',(-3.77892706200006,2.2,-1.79150086600002));
#317075=CARTESIAN_POINT('Ctrl Pts',(-3.78000041200006,12.2,-1.79248996300001));
#317076=CARTESIAN_POINT('Ctrl Pts',(-3.78000041200006,5.2,-1.79248996300001));
#317077=CARTESIAN_POINT('Ctrl Pts',(-3.78000041200006,2.2,-1.79248996300001));
#317078=CARTESIAN_POINT('Ctrl Pts',(-3.78107610400006,12.2,-1.79348355800002));
#317079=CARTESIAN_POINT('Ctrl Pts',(-3.78107610400006,5.2,-1.79348355800002));
#317080=CARTESIAN_POINT('Ctrl Pts',(-3.78107610400006,2.2,-1.79348355800002));
#317081=CARTESIAN_POINT('Ctrl Pts',(-3.78215412600006,12.2,-1.79448164800001));
#317082=CARTESIAN_POINT('Ctrl Pts',(-3.78215412600006,5.2,-1.79448164800001));
#317083=CARTESIAN_POINT('Ctrl Pts',(-3.78215412600006,2.2,-1.79448164800001));
#317084=CARTESIAN_POINT('Ctrl Pts',(-3.78323446300006,12.2,-1.79548423900001));
#317085=CARTESIAN_POINT('Ctrl Pts',(-3.78323446300006,5.2,-1.79548423900001));
#317086=CARTESIAN_POINT('Ctrl Pts',(-3.78323446300006,2.2,-1.79548423900001));
#317087=CARTESIAN_POINT('Ctrl Pts',(-3.78431710400006,12.2,-1.79649133000002));
#317088=CARTESIAN_POINT('Ctrl Pts',(-3.78431710400006,5.2,-1.79649133000002));
#317089=CARTESIAN_POINT('Ctrl Pts',(-3.78431710400006,2.2,-1.79649133000002));
#317090=CARTESIAN_POINT('Ctrl Pts',(-3.78540203300005,12.2,-1.79750292300001));
#317091=CARTESIAN_POINT('Ctrl Pts',(-3.78540203300005,5.2,-1.79750292300001));
#317092=CARTESIAN_POINT('Ctrl Pts',(-3.78540203300005,2.2,-1.79750292300001));
#317093=CARTESIAN_POINT('Ctrl Pts',(-3.78648923700006,12.2,-1.79851902000001));
#317094=CARTESIAN_POINT('Ctrl Pts',(-3.78648923700006,5.2,-1.79851902000001));
#317095=CARTESIAN_POINT('Ctrl Pts',(-3.78648923700006,2.2,-1.79851902000001));
#317096=CARTESIAN_POINT('Ctrl Pts',(-3.78757870600006,12.2,-1.79953962300001));
#317097=CARTESIAN_POINT('Ctrl Pts',(-3.78757870600006,5.2,-1.79953962300001));
#317098=CARTESIAN_POINT('Ctrl Pts',(-3.78757870600006,2.2,-1.79953962300001));
#317099=CARTESIAN_POINT('Ctrl Pts',(-3.78867042200006,12.2,-1.80056473100001));
#317100=CARTESIAN_POINT('Ctrl Pts',(-3.78867042200006,5.2,-1.80056473100001));
#317101=CARTESIAN_POINT('Ctrl Pts',(-3.78867042200006,2.2,-1.80056473100001));
#317102=CARTESIAN_POINT('Ctrl Pts',(-3.78976437500006,12.2,-1.80159435000002));
#317103=CARTESIAN_POINT('Ctrl Pts',(-3.78976437500006,5.2,-1.80159435000002));
#317104=CARTESIAN_POINT('Ctrl Pts',(-3.78976437500006,2.2,-1.80159435000002));
#317105=CARTESIAN_POINT('Ctrl Pts',(-3.79086055000006,12.2,-1.80262847700002));
#317106=CARTESIAN_POINT('Ctrl Pts',(-3.79086055000006,5.2,-1.80262847700002));
#317107=CARTESIAN_POINT('Ctrl Pts',(-3.79086055000006,2.2,-1.80262847700002));
#317108=CARTESIAN_POINT('Ctrl Pts',(-3.79195893400006,12.2,-1.80366711600001));
#317109=CARTESIAN_POINT('Ctrl Pts',(-3.79195893400006,5.2,-1.80366711600001));
#317110=CARTESIAN_POINT('Ctrl Pts',(-3.79195893400006,2.2,-1.80366711600001));
#317111=CARTESIAN_POINT('Ctrl Pts',(-3.79305951500006,12.2,-1.80471026800001));
#317112=CARTESIAN_POINT('Ctrl Pts',(-3.79305951500006,5.2,-1.80471026800001));
#317113=CARTESIAN_POINT('Ctrl Pts',(-3.79305951500006,2.2,-1.80471026800001));
#317114=CARTESIAN_POINT('Ctrl Pts',(-3.79416227800006,12.2,-1.80575793300001));
#317115=CARTESIAN_POINT('Ctrl Pts',(-3.79416227800006,5.2,-1.80575793300001));
#317116=CARTESIAN_POINT('Ctrl Pts',(-3.79416227800006,2.2,-1.80575793300001));
#317117=CARTESIAN_POINT('Ctrl Pts',(-3.79526721200006,12.2,-1.80681011400001));
#317118=CARTESIAN_POINT('Ctrl Pts',(-3.79526721200006,5.2,-1.80681011400001));
#317119=CARTESIAN_POINT('Ctrl Pts',(-3.79526721200006,2.2,-1.80681011400001));
#317120=CARTESIAN_POINT('Ctrl Pts',(-3.79637430300006,12.2,-1.80786681200001));
#317121=CARTESIAN_POINT('Ctrl Pts',(-3.79637430300006,5.2,-1.80786681200001));
#317122=CARTESIAN_POINT('Ctrl Pts',(-3.79637430300006,2.2,-1.80786681200001));
#317123=CARTESIAN_POINT('Ctrl Pts',(-3.79748353500006,12.2,-1.80892802800001));
#317124=CARTESIAN_POINT('Ctrl Pts',(-3.79748353500006,5.2,-1.80892802800001));
#317125=CARTESIAN_POINT('Ctrl Pts',(-3.79748353500006,2.2,-1.80892802800001));
#317126=CARTESIAN_POINT('Ctrl Pts',(-3.79859490000006,12.2,-1.80999376300001));
#317127=CARTESIAN_POINT('Ctrl Pts',(-3.79859490000006,5.2,-1.80999376300001));
#317128=CARTESIAN_POINT('Ctrl Pts',(-3.79859490000006,2.2,-1.80999376300001));
#317129=CARTESIAN_POINT('Ctrl Pts',(-3.79970838200006,12.2,-1.81106401900001));
#317130=CARTESIAN_POINT('Ctrl Pts',(-3.79970838200006,5.2,-1.81106401900001));
#317131=CARTESIAN_POINT('Ctrl Pts',(-3.79970838200006,2.2,-1.81106401900001));
#317132=CARTESIAN_POINT('Ctrl Pts',(-3.80082396700006,12.2,-1.81213879700001));
#317133=CARTESIAN_POINT('Ctrl Pts',(-3.80082396700006,5.2,-1.81213879700001));
#317134=CARTESIAN_POINT('Ctrl Pts',(-3.80082396700006,2.2,-1.81213879700001));
#317135=CARTESIAN_POINT('Ctrl Pts',(-3.80194164400006,12.2,-1.81321809900002));
#317136=CARTESIAN_POINT('Ctrl Pts',(-3.80194164400006,5.2,-1.81321809900002));
#317137=CARTESIAN_POINT('Ctrl Pts',(-3.80194164400006,2.2,-1.81321809900002));
#317138=CARTESIAN_POINT('Ctrl Pts',(-3.80306140000005,12.2,-1.81430192500001));
#317139=CARTESIAN_POINT('Ctrl Pts',(-3.80306140000005,5.2,-1.81430192500001));
#317140=CARTESIAN_POINT('Ctrl Pts',(-3.80306140000005,2.2,-1.81430192500001));
#317141=CARTESIAN_POINT('Ctrl Pts',(-3.80418322100006,12.2,-1.81539027700001));
#317142=CARTESIAN_POINT('Ctrl Pts',(-3.80418322100006,5.2,-1.81539027700001));
#317143=CARTESIAN_POINT('Ctrl Pts',(-3.80418322100006,2.2,-1.81539027700001));
#317144=CARTESIAN_POINT('Ctrl Pts',(-3.80530709400006,12.2,-1.81648315500002));
#317145=CARTESIAN_POINT('Ctrl Pts',(-3.80530709400006,5.2,-1.81648315500002));
#317146=CARTESIAN_POINT('Ctrl Pts',(-3.80530709400006,2.2,-1.81648315500002));
#317147=CARTESIAN_POINT('Ctrl Pts',(-3.80643300700005,12.2,-1.81758056100001));
#317148=CARTESIAN_POINT('Ctrl Pts',(-3.80643300700005,5.2,-1.81758056100001));
#317149=CARTESIAN_POINT('Ctrl Pts',(-3.80643300700005,2.2,-1.81758056100001));
#317150=CARTESIAN_POINT('Ctrl Pts',(-3.80756094600006,12.2,-1.81868249800001));
#317151=CARTESIAN_POINT('Ctrl Pts',(-3.80756094600006,5.2,-1.81868249800001));
#317152=CARTESIAN_POINT('Ctrl Pts',(-3.80756094600006,2.2,-1.81868249800001));
#317153=CARTESIAN_POINT('Ctrl Pts',(-3.80869089900005,12.2,-1.81978896400001));
#317154=CARTESIAN_POINT('Ctrl Pts',(-3.80869089900005,5.2,-1.81978896400001));
#317155=CARTESIAN_POINT('Ctrl Pts',(-3.80869089900005,2.2,-1.81978896400001));
#317156=CARTESIAN_POINT('Ctrl Pts',(-3.80982285300006,12.2,-1.82089996100002));
#317157=CARTESIAN_POINT('Ctrl Pts',(-3.80982285300006,5.2,-1.82089996100002));
#317158=CARTESIAN_POINT('Ctrl Pts',(-3.80982285300006,2.2,-1.82089996100002));
#317159=CARTESIAN_POINT('Ctrl Pts',(-3.81095679500006,12.2,-1.82201549200002));
#317160=CARTESIAN_POINT('Ctrl Pts',(-3.81095679500006,5.2,-1.82201549200002));
#317161=CARTESIAN_POINT('Ctrl Pts',(-3.81095679500006,2.2,-1.82201549200002));
#317162=CARTESIAN_POINT('Ctrl Pts',(-3.81209271100006,12.2,-1.82313555600001));
#317163=CARTESIAN_POINT('Ctrl Pts',(-3.81209271100006,5.2,-1.82313555600001));
#317164=CARTESIAN_POINT('Ctrl Pts',(-3.81209271100006,2.2,-1.82313555600001));
#317165=CARTESIAN_POINT('Ctrl Pts',(-3.81323059200006,12.2,-1.82426015500001));
#317166=CARTESIAN_POINT('Ctrl Pts',(-3.81323059200006,5.2,-1.82426015500001));
#317167=CARTESIAN_POINT('Ctrl Pts',(-3.81323059200006,2.2,-1.82426015500001));
#317168=CARTESIAN_POINT('Ctrl Pts',(-3.81437042100006,12.2,-1.82538929000001));
#317169=CARTESIAN_POINT('Ctrl Pts',(-3.81437042100006,5.2,-1.82538929000001));
#317170=CARTESIAN_POINT('Ctrl Pts',(-3.81437042100006,2.2,-1.82538929000001));
#317171=CARTESIAN_POINT('Ctrl Pts',(-3.81551218700006,12.2,-1.82652296200001));
#317172=CARTESIAN_POINT('Ctrl Pts',(-3.81551218700006,5.2,-1.82652296200001));
#317173=CARTESIAN_POINT('Ctrl Pts',(-3.81551218700006,2.2,-1.82652296200001));
#317174=CARTESIAN_POINT('Ctrl Pts',(-3.81665587800006,12.2,-1.82766117100002));
#317175=CARTESIAN_POINT('Ctrl Pts',(-3.81665587800006,5.2,-1.82766117100002));
#317176=CARTESIAN_POINT('Ctrl Pts',(-3.81665587800006,2.2,-1.82766117100002));
#317177=CARTESIAN_POINT('Ctrl Pts',(-3.81780147900006,12.2,-1.82880391900001));
#317178=CARTESIAN_POINT('Ctrl Pts',(-3.81780147900006,5.2,-1.82880391900001));
#317179=CARTESIAN_POINT('Ctrl Pts',(-3.81780147900006,2.2,-1.82880391900001));
#317180=CARTESIAN_POINT('Ctrl Pts',(-3.81894898000006,12.2,-1.82995120700001));
#317181=CARTESIAN_POINT('Ctrl Pts',(-3.81894898000006,5.2,-1.82995120700001));
#317182=CARTESIAN_POINT('Ctrl Pts',(-3.81894898000006,2.2,-1.82995120700001));
#317183=CARTESIAN_POINT('Ctrl Pts',(-3.82009836800006,12.2,-1.83110303500001));
#317184=CARTESIAN_POINT('Ctrl Pts',(-3.82009836800006,5.2,-1.83110303500001));
#317185=CARTESIAN_POINT('Ctrl Pts',(-3.82009836800006,2.2,-1.83110303500001));
#317186=CARTESIAN_POINT('Ctrl Pts',(-3.82124962800006,12.2,-1.83225940600002));
#317187=CARTESIAN_POINT('Ctrl Pts',(-3.82124962800006,5.2,-1.83225940600002));
#317188=CARTESIAN_POINT('Ctrl Pts',(-3.82124962800006,2.2,-1.83225940600002));
#317189=CARTESIAN_POINT('Ctrl Pts',(-3.82240274900006,12.2,-1.83342031800001));
#317190=CARTESIAN_POINT('Ctrl Pts',(-3.82240274900006,5.2,-1.83342031800001));
#317191=CARTESIAN_POINT('Ctrl Pts',(-3.82240274900006,2.2,-1.83342031800001));
#317192=CARTESIAN_POINT('Ctrl Pts',(-3.82355772000006,12.2,-1.83458577400001));
#317193=CARTESIAN_POINT('Ctrl Pts',(-3.82355772000006,5.2,-1.83458577400001));
#317194=CARTESIAN_POINT('Ctrl Pts',(-3.82355772000006,2.2,-1.83458577400001));
#317195=CARTESIAN_POINT('Ctrl Pts',(-3.82471452500006,12.2,-1.83575577400001));
#317196=CARTESIAN_POINT('Ctrl Pts',(-3.82471452500006,5.2,-1.83575577400001));
#317197=CARTESIAN_POINT('Ctrl Pts',(-3.82471452500006,2.2,-1.83575577400001));
#317198=CARTESIAN_POINT('Ctrl Pts',(-3.82587315500006,12.2,-1.83693032100001));
#317199=CARTESIAN_POINT('Ctrl Pts',(-3.82587315500006,5.2,-1.83693032100001));
#317200=CARTESIAN_POINT('Ctrl Pts',(-3.82587315500006,2.2,-1.83693032100001));
#317201=CARTESIAN_POINT('Ctrl Pts',(-3.82703359500006,12.2,-1.83810941200001));
#317202=CARTESIAN_POINT('Ctrl Pts',(-3.82703359500006,5.2,-1.83810941200001));
#317203=CARTESIAN_POINT('Ctrl Pts',(-3.82703359500006,2.2,-1.83810941200001));
#317204=CARTESIAN_POINT('Ctrl Pts',(-3.82819583300006,12.2,-1.83929305100001));
#317205=CARTESIAN_POINT('Ctrl Pts',(-3.82819583300006,5.2,-1.83929305100001));
#317206=CARTESIAN_POINT('Ctrl Pts',(-3.82819583300006,2.2,-1.83929305100001));
#317207=CARTESIAN_POINT('Ctrl Pts',(-3.82935985800006,12.2,-1.84048123600002));
#317208=CARTESIAN_POINT('Ctrl Pts',(-3.82935985800006,5.2,-1.84048123600002));
#317209=CARTESIAN_POINT('Ctrl Pts',(-3.82935985800006,2.2,-1.84048123600002));
#317210=CARTESIAN_POINT('Ctrl Pts',(-3.83052565500006,12.2,-1.84167397100001));
#317211=CARTESIAN_POINT('Ctrl Pts',(-3.83052565500006,5.2,-1.84167397100001));
#317212=CARTESIAN_POINT('Ctrl Pts',(-3.83052565500006,2.2,-1.84167397100001));
#317213=CARTESIAN_POINT('Ctrl Pts',(-3.83169321400006,12.2,-1.84287125400001));
#317214=CARTESIAN_POINT('Ctrl Pts',(-3.83169321400006,5.2,-1.84287125400001));
#317215=CARTESIAN_POINT('Ctrl Pts',(-3.83169321400006,2.2,-1.84287125400001));
#317216=CARTESIAN_POINT('Ctrl Pts',(-3.83286252200006,12.2,-1.84407308800001));
#317217=CARTESIAN_POINT('Ctrl Pts',(-3.83286252200006,5.2,-1.84407308800001));
#317218=CARTESIAN_POINT('Ctrl Pts',(-3.83286252200006,2.2,-1.84407308800001));
#317219=CARTESIAN_POINT('Ctrl Pts',(-3.83403356500006,12.2,-1.84527947200001));
#317220=CARTESIAN_POINT('Ctrl Pts',(-3.83403356500006,5.2,-1.84527947200001));
#317221=CARTESIAN_POINT('Ctrl Pts',(-3.83403356500006,2.2,-1.84527947200001));
#317222=CARTESIAN_POINT('Ctrl Pts',(-3.83520633300006,12.2,-1.84649040700001));
#317223=CARTESIAN_POINT('Ctrl Pts',(-3.83520633300006,5.2,-1.84649040700001));
#317224=CARTESIAN_POINT('Ctrl Pts',(-3.83520633300006,2.2,-1.84649040700001));
#317225=CARTESIAN_POINT('Ctrl Pts',(-3.83638081200006,12.2,-1.84770589500001));
#317226=CARTESIAN_POINT('Ctrl Pts',(-3.83638081200006,5.2,-1.84770589500001));
#317227=CARTESIAN_POINT('Ctrl Pts',(-3.83638081200006,2.2,-1.84770589500001));
#317228=CARTESIAN_POINT('Ctrl Pts',(-3.83755699000006,12.2,-1.84892593400001));
#317229=CARTESIAN_POINT('Ctrl Pts',(-3.83755699000006,5.2,-1.84892593400001));
#317230=CARTESIAN_POINT('Ctrl Pts',(-3.83755699000006,2.2,-1.84892593400001));
#317231=CARTESIAN_POINT('Ctrl Pts',(-3.83873485500006,12.2,-1.85015052700002));
#317232=CARTESIAN_POINT('Ctrl Pts',(-3.83873485500006,5.2,-1.85015052700002));
#317233=CARTESIAN_POINT('Ctrl Pts',(-3.83873485500006,2.2,-1.85015052700002));
#317234=CARTESIAN_POINT('Ctrl Pts',(-3.83991439500006,12.2,-1.85137967400001));
#317235=CARTESIAN_POINT('Ctrl Pts',(-3.83991439500006,5.2,-1.85137967400001));
#317236=CARTESIAN_POINT('Ctrl Pts',(-3.83991439500006,2.2,-1.85137967400001));
#317237=CARTESIAN_POINT('Ctrl Pts',(-3.84109559700006,12.2,-1.85261337700001));
#317238=CARTESIAN_POINT('Ctrl Pts',(-3.84109559700006,5.2,-1.85261337700001));
#317239=CARTESIAN_POINT('Ctrl Pts',(-3.84109559700006,2.2,-1.85261337700001));
#317240=CARTESIAN_POINT('Ctrl Pts',(-3.84227845000006,12.2,-1.85385163300001));
#317241=CARTESIAN_POINT('Ctrl Pts',(-3.84227845000006,5.2,-1.85385163300001));
#317242=CARTESIAN_POINT('Ctrl Pts',(-3.84227845000006,2.2,-1.85385163300001));
#317243=CARTESIAN_POINT('Ctrl Pts',(-3.84346294100006,12.2,-1.85509444700001));
#317244=CARTESIAN_POINT('Ctrl Pts',(-3.84346294100006,5.2,-1.85509444700001));
#317245=CARTESIAN_POINT('Ctrl Pts',(-3.84346294100006,2.2,-1.85509444700001));
#317246=CARTESIAN_POINT('Ctrl Pts',(-3.84464905800006,12.2,-1.85634181600001));
#317247=CARTESIAN_POINT('Ctrl Pts',(-3.84464905800006,5.2,-1.85634181600001));
#317248=CARTESIAN_POINT('Ctrl Pts',(-3.84464905800006,2.2,-1.85634181600001));
#317249=CARTESIAN_POINT('Ctrl Pts',(-3.84583678800006,12.2,-1.85759374200002));
#317250=CARTESIAN_POINT('Ctrl Pts',(-3.84583678800006,5.2,-1.85759374200002));
#317251=CARTESIAN_POINT('Ctrl Pts',(-3.84583678800006,2.2,-1.85759374200002));
#317252=CARTESIAN_POINT('Ctrl Pts',(-3.84702612000006,12.2,-1.85885022500001));
#317253=CARTESIAN_POINT('Ctrl Pts',(-3.84702612000006,5.2,-1.85885022500001));
#317254=CARTESIAN_POINT('Ctrl Pts',(-3.84702612000006,2.2,-1.85885022500001));
#317255=CARTESIAN_POINT('Ctrl Pts',(-3.84821704000006,12.2,-1.86011126700001));
#317256=CARTESIAN_POINT('Ctrl Pts',(-3.84821704000006,5.2,-1.86011126700001));
#317257=CARTESIAN_POINT('Ctrl Pts',(-3.84821704000006,2.2,-1.86011126700001));
#317258=CARTESIAN_POINT('Ctrl Pts',(-3.84940953900006,12.2,-1.86137686600001));
#317259=CARTESIAN_POINT('Ctrl Pts',(-3.84940953900006,5.2,-1.86137686600001));
#317260=CARTESIAN_POINT('Ctrl Pts',(-3.84940953900006,2.2,-1.86137686600001));
#317261=CARTESIAN_POINT('Ctrl Pts',(-3.85060360200006,12.2,-1.86264702500001));
#317262=CARTESIAN_POINT('Ctrl Pts',(-3.85060360200006,5.2,-1.86264702500001));
#317263=CARTESIAN_POINT('Ctrl Pts',(-3.85060360200006,2.2,-1.86264702500001));
#317264=CARTESIAN_POINT('Ctrl Pts',(-3.85179922000006,12.2,-1.86392174300002));
#317265=CARTESIAN_POINT('Ctrl Pts',(-3.85179922000006,5.2,-1.86392174300002));
#317266=CARTESIAN_POINT('Ctrl Pts',(-3.85179922000006,2.2,-1.86392174300002));
#317267=CARTESIAN_POINT('Ctrl Pts',(-3.85299637800006,12.2,-1.86520102000001));
#317268=CARTESIAN_POINT('Ctrl Pts',(-3.85299637800006,5.2,-1.86520102000001));
#317269=CARTESIAN_POINT('Ctrl Pts',(-3.85299637800006,2.2,-1.86520102000001));
#317270=CARTESIAN_POINT('Ctrl Pts',(-3.85419506500006,12.2,-1.86648485800001));
#317271=CARTESIAN_POINT('Ctrl Pts',(-3.85419506500006,5.2,-1.86648485800001));
#317272=CARTESIAN_POINT('Ctrl Pts',(-3.85419506500006,2.2,-1.86648485800001));
#317273=CARTESIAN_POINT('Ctrl Pts',(-3.85539526900006,12.2,-1.86777325700001));
#317274=CARTESIAN_POINT('Ctrl Pts',(-3.85539526900006,5.2,-1.86777325700001));
#317275=CARTESIAN_POINT('Ctrl Pts',(-3.85539526900006,2.2,-1.86777325700001));
#317276=CARTESIAN_POINT('Ctrl Pts',(-3.85659697900006,12.2,-1.86906621600002));
#317277=CARTESIAN_POINT('Ctrl Pts',(-3.85659697900006,5.2,-1.86906621600002));
#317278=CARTESIAN_POINT('Ctrl Pts',(-3.85659697900006,2.2,-1.86906621600002));
#317279=CARTESIAN_POINT('Ctrl Pts',(-3.85780018200006,12.2,-1.87036373800002));
#317280=CARTESIAN_POINT('Ctrl Pts',(-3.85780018200006,5.2,-1.87036373800002));
#317281=CARTESIAN_POINT('Ctrl Pts',(-3.85780018200006,2.2,-1.87036373800002));
#317282=CARTESIAN_POINT('Ctrl Pts',(-3.85900486600006,12.2,-1.87166582000001));
#317283=CARTESIAN_POINT('Ctrl Pts',(-3.85900486600006,5.2,-1.87166582000001));
#317284=CARTESIAN_POINT('Ctrl Pts',(-3.85900486600006,2.2,-1.87166582000001));
#317285=CARTESIAN_POINT('Ctrl Pts',(-3.86021102000006,12.2,-1.87297246600002));
#317286=CARTESIAN_POINT('Ctrl Pts',(-3.86021102000006,5.2,-1.87297246600002));
#317287=CARTESIAN_POINT('Ctrl Pts',(-3.86021102000006,2.2,-1.87297246600002));
#317288=CARTESIAN_POINT('Ctrl Pts',(-3.86141863100006,12.2,-1.87428367200001));
#317289=CARTESIAN_POINT('Ctrl Pts',(-3.86141863100006,5.2,-1.87428367200001));
#317290=CARTESIAN_POINT('Ctrl Pts',(-3.86141863100006,2.2,-1.87428367200001));
#317291=CARTESIAN_POINT('Ctrl Pts',(-3.86262768800006,12.2,-1.87559944300002));
#317292=CARTESIAN_POINT('Ctrl Pts',(-3.86262768800006,5.2,-1.87559944300002));
#317293=CARTESIAN_POINT('Ctrl Pts',(-3.86262768800006,2.2,-1.87559944300002));
#317294=CARTESIAN_POINT('Ctrl Pts',(-3.86383817800006,12.2,-1.87691977600001));
#317295=CARTESIAN_POINT('Ctrl Pts',(-3.86383817800006,5.2,-1.87691977600001));
#317296=CARTESIAN_POINT('Ctrl Pts',(-3.86383817800006,2.2,-1.87691977600001));
#317297=CARTESIAN_POINT('Ctrl Pts',(-3.86505009100006,12.2,-1.87824467100001));
#317298=CARTESIAN_POINT('Ctrl Pts',(-3.86505009100006,5.2,-1.87824467100001));
#317299=CARTESIAN_POINT('Ctrl Pts',(-3.86505009100006,2.2,-1.87824467100001));
#317300=CARTESIAN_POINT('Ctrl Pts',(-3.86626341400006,12.2,-1.87957413100001));
#317301=CARTESIAN_POINT('Ctrl Pts',(-3.86626341400006,5.2,-1.87957413100001));
#317302=CARTESIAN_POINT('Ctrl Pts',(-3.86626341400006,2.2,-1.87957413100001));
#317303=CARTESIAN_POINT('Ctrl Pts',(-3.86747813500006,12.2,-1.88090815500002));
#317304=CARTESIAN_POINT('Ctrl Pts',(-3.86747813500006,5.2,-1.88090815500002));
#317305=CARTESIAN_POINT('Ctrl Pts',(-3.86747813500006,2.2,-1.88090815500002));
#317306=CARTESIAN_POINT('Ctrl Pts',(-3.86869424300006,12.2,-1.88224674200002));
#317307=CARTESIAN_POINT('Ctrl Pts',(-3.86869424300006,5.2,-1.88224674200002));
#317308=CARTESIAN_POINT('Ctrl Pts',(-3.86869424300006,2.2,-1.88224674200002));
#317309=CARTESIAN_POINT('Ctrl Pts',(-3.86991172500006,12.2,-1.88358989500002));
#317310=CARTESIAN_POINT('Ctrl Pts',(-3.86991172500006,5.2,-1.88358989500002));
#317311=CARTESIAN_POINT('Ctrl Pts',(-3.86991172500006,2.2,-1.88358989500002));
#317312=CARTESIAN_POINT('Ctrl Pts',(-3.87113057200006,12.2,-1.88493761100001));
#317313=CARTESIAN_POINT('Ctrl Pts',(-3.87113057200006,5.2,-1.88493761100001));
#317314=CARTESIAN_POINT('Ctrl Pts',(-3.87113057200006,2.2,-1.88493761100001));
#317315=CARTESIAN_POINT('Ctrl Pts',(-3.87235076900006,12.2,-1.88628989100001));
#317316=CARTESIAN_POINT('Ctrl Pts',(-3.87235076900006,5.2,-1.88628989100001));
#317317=CARTESIAN_POINT('Ctrl Pts',(-3.87235076900006,2.2,-1.88628989100001));
#317318=CARTESIAN_POINT('Ctrl Pts',(-3.87357230700006,12.2,-1.88764673700001));
#317319=CARTESIAN_POINT('Ctrl Pts',(-3.87357230700006,5.2,-1.88764673700001));
#317320=CARTESIAN_POINT('Ctrl Pts',(-3.87357230700006,2.2,-1.88764673700001));
#317321=CARTESIAN_POINT('Ctrl Pts',(-3.87479517200005,12.2,-1.88900814700002));
#317322=CARTESIAN_POINT('Ctrl Pts',(-3.87479517200005,5.2,-1.88900814700002));
#317323=CARTESIAN_POINT('Ctrl Pts',(-3.87479517200005,2.2,-1.88900814700002));
#317324=CARTESIAN_POINT('Ctrl Pts',(-3.87601935400006,12.2,-1.89037412300001));
#317325=CARTESIAN_POINT('Ctrl Pts',(-3.87601935400006,5.2,-1.89037412300001));
#317326=CARTESIAN_POINT('Ctrl Pts',(-3.87601935400006,2.2,-1.89037412300001));
#317327=CARTESIAN_POINT('Ctrl Pts',(-3.87724484000006,12.2,-1.89174466300001));
#317328=CARTESIAN_POINT('Ctrl Pts',(-3.87724484000006,5.2,-1.89174466300001));
#317329=CARTESIAN_POINT('Ctrl Pts',(-3.87724484000006,2.2,-1.89174466300001));
#317330=CARTESIAN_POINT('Ctrl Pts',(-3.87847162000006,12.2,-1.89311977000001));
#317331=CARTESIAN_POINT('Ctrl Pts',(-3.87847162000006,5.2,-1.89311977000001));
#317332=CARTESIAN_POINT('Ctrl Pts',(-3.87847162000006,2.2,-1.89311977000001));
#317333=CARTESIAN_POINT('Ctrl Pts',(-3.87969968200006,12.2,-1.89449944100001));
#317334=CARTESIAN_POINT('Ctrl Pts',(-3.87969968200006,5.2,-1.89449944100001));
#317335=CARTESIAN_POINT('Ctrl Pts',(-3.87969968200006,2.2,-1.89449944100001));
#317336=CARTESIAN_POINT('Ctrl Pts',(-3.88092901400006,12.2,-1.89588367700001));
#317337=CARTESIAN_POINT('Ctrl Pts',(-3.88092901400006,5.2,-1.89588367700001));
#317338=CARTESIAN_POINT('Ctrl Pts',(-3.88092901400006,2.2,-1.89588367700001));
#317339=CARTESIAN_POINT('Ctrl Pts',(-3.88215960400006,12.2,-1.89727248000001));
#317340=CARTESIAN_POINT('Ctrl Pts',(-3.88215960400006,5.2,-1.89727248000001));
#317341=CARTESIAN_POINT('Ctrl Pts',(-3.88215960400006,2.2,-1.89727248000001));
#317342=CARTESIAN_POINT('Ctrl Pts',(-3.88339144100006,12.2,-1.89866584700002));
#317343=CARTESIAN_POINT('Ctrl Pts',(-3.88339144100006,5.2,-1.89866584700002));
#317344=CARTESIAN_POINT('Ctrl Pts',(-3.88339144100006,2.2,-1.89866584700002));
#317345=CARTESIAN_POINT('Ctrl Pts',(-3.88462451500006,12.2,-1.90006378000001));
#317346=CARTESIAN_POINT('Ctrl Pts',(-3.88462451500006,5.2,-1.90006378000001));
#317347=CARTESIAN_POINT('Ctrl Pts',(-3.88462451500006,2.2,-1.90006378000001));
#317348=CARTESIAN_POINT('Ctrl Pts',(-3.88585881200005,12.2,-1.90146627800001));
#317349=CARTESIAN_POINT('Ctrl Pts',(-3.88585881200005,5.2,-1.90146627800001));
#317350=CARTESIAN_POINT('Ctrl Pts',(-3.88585881200005,2.2,-1.90146627800001));
#317351=CARTESIAN_POINT('Ctrl Pts',(-3.88709432100006,12.2,-1.90287334200002));
#317352=CARTESIAN_POINT('Ctrl Pts',(-3.88709432100006,5.2,-1.90287334200002));
#317353=CARTESIAN_POINT('Ctrl Pts',(-3.88709432100006,2.2,-1.90287334200002));
#317354=CARTESIAN_POINT('Ctrl Pts',(-3.88833103200006,12.2,-1.90428497100001));
#317355=CARTESIAN_POINT('Ctrl Pts',(-3.88833103200006,5.2,-1.90428497100001));
#317356=CARTESIAN_POINT('Ctrl Pts',(-3.88833103200006,2.2,-1.90428497100001));
#317357=CARTESIAN_POINT('Ctrl Pts',(-3.88956893300006,12.2,-1.90570116600002));
#317358=CARTESIAN_POINT('Ctrl Pts',(-3.88956893300006,5.2,-1.90570116600002));
#317359=CARTESIAN_POINT('Ctrl Pts',(-3.88956893300006,2.2,-1.90570116600002));
#317360=CARTESIAN_POINT('Ctrl Pts',(-3.89080801200006,12.2,-1.90712192700001));
#317361=CARTESIAN_POINT('Ctrl Pts',(-3.89080801200006,5.2,-1.90712192700001));
#317362=CARTESIAN_POINT('Ctrl Pts',(-3.89080801200006,2.2,-1.90712192700001));
#317363=CARTESIAN_POINT('Ctrl Pts',(-3.89204825700006,12.2,-1.90854725100001));
#317364=CARTESIAN_POINT('Ctrl Pts',(-3.89204825700006,5.2,-1.90854725100001));
#317365=CARTESIAN_POINT('Ctrl Pts',(-3.89204825700006,2.2,-1.90854725100001));
#317366=CARTESIAN_POINT('Ctrl Pts',(-3.89328965800006,12.2,-1.90997714200002));
#317367=CARTESIAN_POINT('Ctrl Pts',(-3.89328965800006,5.2,-1.90997714200002));
#317368=CARTESIAN_POINT('Ctrl Pts',(-3.89328965800006,2.2,-1.90997714200002));
#317369=CARTESIAN_POINT('Ctrl Pts',(-3.89453220400005,12.2,-1.91141159700001));
#317370=CARTESIAN_POINT('Ctrl Pts',(-3.89453220400005,5.2,-1.91141159700001));
#317371=CARTESIAN_POINT('Ctrl Pts',(-3.89453220400005,2.2,-1.91141159700001));
#317372=CARTESIAN_POINT('Ctrl Pts',(-3.89577588200006,12.2,-1.91285061800002));
#317373=CARTESIAN_POINT('Ctrl Pts',(-3.89577588200006,5.2,-1.91285061800002));
#317374=CARTESIAN_POINT('Ctrl Pts',(-3.89577588200006,2.2,-1.91285061800002));
#317375=CARTESIAN_POINT('Ctrl Pts',(-3.89702068200006,12.2,-1.91429420300001));
#317376=CARTESIAN_POINT('Ctrl Pts',(-3.89702068200006,5.2,-1.91429420300001));
#317377=CARTESIAN_POINT('Ctrl Pts',(-3.89702068200006,2.2,-1.91429420300001));
#317378=CARTESIAN_POINT('Ctrl Pts',(-3.89826659300006,12.2,-1.91574235300001));
#317379=CARTESIAN_POINT('Ctrl Pts',(-3.89826659300006,5.2,-1.91574235300001));
#317380=CARTESIAN_POINT('Ctrl Pts',(-3.89826659300006,2.2,-1.91574235300001));
#317381=CARTESIAN_POINT('Ctrl Pts',(-3.89951360200006,12.2,-1.91719506800001));
#317382=CARTESIAN_POINT('Ctrl Pts',(-3.89951360200006,5.2,-1.91719506800001));
#317383=CARTESIAN_POINT('Ctrl Pts',(-3.89951360200006,2.2,-1.91719506800001));
#317384=CARTESIAN_POINT('Ctrl Pts',(-3.90076169900006,12.2,-1.91865234600002));
#317385=CARTESIAN_POINT('Ctrl Pts',(-3.90076169900006,5.2,-1.91865234600002));
#317386=CARTESIAN_POINT('Ctrl Pts',(-3.90076169900006,2.2,-1.91865234600002));
#317387=CARTESIAN_POINT('Ctrl Pts',(-3.90201087200006,12.2,-1.92011418900002));
#317388=CARTESIAN_POINT('Ctrl Pts',(-3.90201087200006,5.2,-1.92011418900002));
#317389=CARTESIAN_POINT('Ctrl Pts',(-3.90201087200006,2.2,-1.92011418900002));
#317390=CARTESIAN_POINT('Ctrl Pts',(-3.90326111100006,12.2,-1.92158059600001));
#317391=CARTESIAN_POINT('Ctrl Pts',(-3.90326111100006,5.2,-1.92158059600001));
#317392=CARTESIAN_POINT('Ctrl Pts',(-3.90326111100006,2.2,-1.92158059600001));
#317393=CARTESIAN_POINT('Ctrl Pts',(-3.90451240400005,12.2,-1.92305156600002));
#317394=CARTESIAN_POINT('Ctrl Pts',(-3.90451240400005,5.2,-1.92305156600002));
#317395=CARTESIAN_POINT('Ctrl Pts',(-3.90451240400005,2.2,-1.92305156600002));
#317396=CARTESIAN_POINT('Ctrl Pts',(-3.90576474000006,12.2,-1.92452709900001));
#317397=CARTESIAN_POINT('Ctrl Pts',(-3.90576474000006,5.2,-1.92452709900001));
#317398=CARTESIAN_POINT('Ctrl Pts',(-3.90576474000006,2.2,-1.92452709900001));
#317399=CARTESIAN_POINT('Ctrl Pts',(-3.90701810700006,12.2,-1.92600719600001));
#317400=CARTESIAN_POINT('Ctrl Pts',(-3.90701810700006,5.2,-1.92600719600001));
#317401=CARTESIAN_POINT('Ctrl Pts',(-3.90701810700006,2.2,-1.92600719600001));
#317402=CARTESIAN_POINT('Ctrl Pts',(-3.90827249600005,12.2,-1.92749185600002));
#317403=CARTESIAN_POINT('Ctrl Pts',(-3.90827249600005,5.2,-1.92749185600002));
#317404=CARTESIAN_POINT('Ctrl Pts',(-3.90827249600005,2.2,-1.92749185600002));
#317405=CARTESIAN_POINT('Ctrl Pts',(-3.90952789300006,12.2,-1.92898107800001));
#317406=CARTESIAN_POINT('Ctrl Pts',(-3.90952789300006,5.2,-1.92898107800001));
#317407=CARTESIAN_POINT('Ctrl Pts',(-3.90952789300006,2.2,-1.92898107800001));
#317408=CARTESIAN_POINT('Ctrl Pts',(-3.91078429000006,12.2,-1.93047486300001));
#317409=CARTESIAN_POINT('Ctrl Pts',(-3.91078429000006,5.2,-1.93047486300001));
#317410=CARTESIAN_POINT('Ctrl Pts',(-3.91078429000006,2.2,-1.93047486300001));
#317411=CARTESIAN_POINT('Ctrl Pts',(-3.91204167400006,12.2,-1.93197320900001));
#317412=CARTESIAN_POINT('Ctrl Pts',(-3.91204167400006,5.2,-1.93197320900001));
#317413=CARTESIAN_POINT('Ctrl Pts',(-3.91204167400006,2.2,-1.93197320900001));
#317414=CARTESIAN_POINT('Ctrl Pts',(-3.91330003300006,12.2,-1.93347611800001));
#317415=CARTESIAN_POINT('Ctrl Pts',(-3.91330003300006,5.2,-1.93347611800001));
#317416=CARTESIAN_POINT('Ctrl Pts',(-3.91330003300006,2.2,-1.93347611800001));
#317417=CARTESIAN_POINT('Ctrl Pts',(-3.91455935800006,12.2,-1.93498358700001));
#317418=CARTESIAN_POINT('Ctrl Pts',(-3.91455935800006,5.2,-1.93498358700001));
#317419=CARTESIAN_POINT('Ctrl Pts',(-3.91455935800006,2.2,-1.93498358700001));
#317420=CARTESIAN_POINT('Ctrl Pts',(-3.91581963700006,12.2,-1.93649561800001));
#317421=CARTESIAN_POINT('Ctrl Pts',(-3.91581963700006,5.2,-1.93649561800001));
#317422=CARTESIAN_POINT('Ctrl Pts',(-3.91581963700006,2.2,-1.93649561800001));
#317423=CARTESIAN_POINT('Ctrl Pts',(-3.91708085900006,12.2,-1.93801220900002));
#317424=CARTESIAN_POINT('Ctrl Pts',(-3.91708085900006,5.2,-1.93801220900002));
#317425=CARTESIAN_POINT('Ctrl Pts',(-3.91708085900006,2.2,-1.93801220900002));
#317426=CARTESIAN_POINT('Ctrl Pts',(-3.91834301300006,12.2,-1.93953336000002));
#317427=CARTESIAN_POINT('Ctrl Pts',(-3.91834301300006,5.2,-1.93953336000002));
#317428=CARTESIAN_POINT('Ctrl Pts',(-3.91834301300006,2.2,-1.93953336000002));
#317429=CARTESIAN_POINT('Ctrl Pts',(-3.91960608900006,12.2,-1.94105907100001));
#317430=CARTESIAN_POINT('Ctrl Pts',(-3.91960608900006,5.2,-1.94105907100001));
#317431=CARTESIAN_POINT('Ctrl Pts',(-3.91960608900006,2.2,-1.94105907100001));
#317432=CARTESIAN_POINT('Ctrl Pts',(-3.92087007500006,12.2,-1.94258934100001));
#317433=CARTESIAN_POINT('Ctrl Pts',(-3.92087007500006,5.2,-1.94258934100001));
#317434=CARTESIAN_POINT('Ctrl Pts',(-3.92087007500006,2.2,-1.94258934100001));
#317435=CARTESIAN_POINT('Ctrl Pts',(-3.92213496000006,12.2,-1.94412417000001));
#317436=CARTESIAN_POINT('Ctrl Pts',(-3.92213496000006,5.2,-1.94412417000001));
#317437=CARTESIAN_POINT('Ctrl Pts',(-3.92213496000006,2.2,-1.94412417000001));
#317438=CARTESIAN_POINT('Ctrl Pts',(-3.92340073400006,12.2,-1.94566355900001));
#317439=CARTESIAN_POINT('Ctrl Pts',(-3.92340073400006,5.2,-1.94566355900001));
#317440=CARTESIAN_POINT('Ctrl Pts',(-3.92340073400006,2.2,-1.94566355900001));
#317441=CARTESIAN_POINT('Ctrl Pts',(-3.92466738500006,12.2,-1.94720750400001));
#317442=CARTESIAN_POINT('Ctrl Pts',(-3.92466738500006,5.2,-1.94720750400001));
#317443=CARTESIAN_POINT('Ctrl Pts',(-3.92466738500006,2.2,-1.94720750400001));
#317444=CARTESIAN_POINT('Ctrl Pts',(-3.92593490200006,12.2,-1.94875600800001));
#317445=CARTESIAN_POINT('Ctrl Pts',(-3.92593490200006,5.2,-1.94875600800001));
#317446=CARTESIAN_POINT('Ctrl Pts',(-3.92593490200006,2.2,-1.94875600800001));
#317447=CARTESIAN_POINT('Ctrl Pts',(-3.92720327500006,12.2,-1.95030906800001));
#317448=CARTESIAN_POINT('Ctrl Pts',(-3.92720327500006,5.2,-1.95030906800001));
#317449=CARTESIAN_POINT('Ctrl Pts',(-3.92720327500006,2.2,-1.95030906800001));
#317450=CARTESIAN_POINT('Ctrl Pts',(-3.92847249300006,12.2,-1.95186668500002));
#317451=CARTESIAN_POINT('Ctrl Pts',(-3.92847249300006,5.2,-1.95186668500002));
#317452=CARTESIAN_POINT('Ctrl Pts',(-3.92847249300006,2.2,-1.95186668500002));
#317453=CARTESIAN_POINT('Ctrl Pts',(-3.92974254600006,12.2,-1.95342885800001));
#317454=CARTESIAN_POINT('Ctrl Pts',(-3.92974254600006,5.2,-1.95342885800001));
#317455=CARTESIAN_POINT('Ctrl Pts',(-3.92974254600006,2.2,-1.95342885800001));
#317456=CARTESIAN_POINT('Ctrl Pts',(-3.93101342100006,12.2,-1.95499558700002));
#317457=CARTESIAN_POINT('Ctrl Pts',(-3.93101342100006,5.2,-1.95499558700002));
#317458=CARTESIAN_POINT('Ctrl Pts',(-3.93101342100006,2.2,-1.95499558700002));
#317459=CARTESIAN_POINT('Ctrl Pts',(-3.93228510900006,12.2,-1.95656686900001));
#317460=CARTESIAN_POINT('Ctrl Pts',(-3.93228510900006,5.2,-1.95656686900001));
#317461=CARTESIAN_POINT('Ctrl Pts',(-3.93228510900006,2.2,-1.95656686900001));
#317462=CARTESIAN_POINT('Ctrl Pts',(-3.93355759800006,12.2,-1.95814270800001));
#317463=CARTESIAN_POINT('Ctrl Pts',(-3.93355759800006,5.2,-1.95814270800001));
#317464=CARTESIAN_POINT('Ctrl Pts',(-3.93355759800006,2.2,-1.95814270800001));
#317465=CARTESIAN_POINT('Ctrl Pts',(-3.93483087900006,12.2,-1.95972309900001));
#317466=CARTESIAN_POINT('Ctrl Pts',(-3.93483087900006,5.2,-1.95972309900001));
#317467=CARTESIAN_POINT('Ctrl Pts',(-3.93483087900006,2.2,-1.95972309900001));
#317468=CARTESIAN_POINT('Ctrl Pts',(-3.93610493900006,12.2,-1.96130804400001));
#317469=CARTESIAN_POINT('Ctrl Pts',(-3.93610493900006,5.2,-1.96130804400001));
#317470=CARTESIAN_POINT('Ctrl Pts',(-3.93610493900006,2.2,-1.96130804400001));
#317471=CARTESIAN_POINT('Ctrl Pts',(-3.93737976900006,12.2,-1.96289754200001));
#317472=CARTESIAN_POINT('Ctrl Pts',(-3.93737976900006,5.2,-1.96289754200001));
#317473=CARTESIAN_POINT('Ctrl Pts',(-3.93737976900006,2.2,-1.96289754200001));
#317474=CARTESIAN_POINT('Ctrl Pts',(-3.93865535800006,12.2,-1.96449159100001));
#317475=CARTESIAN_POINT('Ctrl Pts',(-3.93865535800006,5.2,-1.96449159100001));
#317476=CARTESIAN_POINT('Ctrl Pts',(-3.93865535800006,2.2,-1.96449159100001));
#317477=CARTESIAN_POINT('Ctrl Pts',(-3.93993169500006,12.2,-1.96609019200002));
#317478=CARTESIAN_POINT('Ctrl Pts',(-3.93993169500006,5.2,-1.96609019200002));
#317479=CARTESIAN_POINT('Ctrl Pts',(-3.93993169500006,2.2,-1.96609019200002));
#317480=CARTESIAN_POINT('Ctrl Pts',(-3.94120876900006,12.2,-1.96769334400001));
#317481=CARTESIAN_POINT('Ctrl Pts',(-3.94120876900006,5.2,-1.96769334400001));
#317482=CARTESIAN_POINT('Ctrl Pts',(-3.94120876900006,2.2,-1.96769334400001));
#317483=CARTESIAN_POINT('Ctrl Pts',(-3.94248657000006,12.2,-1.96930104600002));
#317484=CARTESIAN_POINT('Ctrl Pts',(-3.94248657000006,5.2,-1.96930104600002));
#317485=CARTESIAN_POINT('Ctrl Pts',(-3.94248657000006,2.2,-1.96930104600002));
#317486=CARTESIAN_POINT('Ctrl Pts',(-3.94376508600006,12.2,-1.97091329700001));
#317487=CARTESIAN_POINT('Ctrl Pts',(-3.94376508600006,5.2,-1.97091329700001));
#317488=CARTESIAN_POINT('Ctrl Pts',(-3.94376508600006,2.2,-1.97091329700001));
#317489=CARTESIAN_POINT('Ctrl Pts',(-3.94504430900006,12.2,-1.97253009700002));
#317490=CARTESIAN_POINT('Ctrl Pts',(-3.94504430900006,5.2,-1.97253009700002));
#317491=CARTESIAN_POINT('Ctrl Pts',(-3.94504430900006,2.2,-1.97253009700002));
#317492=CARTESIAN_POINT('Ctrl Pts',(-3.94632422700006,12.2,-1.97415144500001));
#317493=CARTESIAN_POINT('Ctrl Pts',(-3.94632422700006,5.2,-1.97415144500001));
#317494=CARTESIAN_POINT('Ctrl Pts',(-3.94632422700006,2.2,-1.97415144500001));
#317495=CARTESIAN_POINT('Ctrl Pts',(-3.94760482800006,12.2,-1.97577734100001));
#317496=CARTESIAN_POINT('Ctrl Pts',(-3.94760482800006,5.2,-1.97577734100001));
#317497=CARTESIAN_POINT('Ctrl Pts',(-3.94760482800006,2.2,-1.97577734100001));
#317498=CARTESIAN_POINT('Ctrl Pts',(-3.94888610300006,12.2,-1.97740778200002));
#317499=CARTESIAN_POINT('Ctrl Pts',(-3.94888610300006,5.2,-1.97740778200002));
#317500=CARTESIAN_POINT('Ctrl Pts',(-3.94888610300006,2.2,-1.97740778200002));
#317501=CARTESIAN_POINT('Ctrl Pts',(-3.95016804100006,12.2,-1.97904277100001));
#317502=CARTESIAN_POINT('Ctrl Pts',(-3.95016804100006,5.2,-1.97904277100001));
#317503=CARTESIAN_POINT('Ctrl Pts',(-3.95016804100006,2.2,-1.97904277100001));
#317504=CARTESIAN_POINT('Ctrl Pts',(-3.95145063200006,12.2,-1.98068230400001));
#317505=CARTESIAN_POINT('Ctrl Pts',(-3.95145063200006,5.2,-1.98068230400001));
#317506=CARTESIAN_POINT('Ctrl Pts',(-3.95145063200006,2.2,-1.98068230400001));
#317507=CARTESIAN_POINT('Ctrl Pts',(-3.95273386500006,12.2,-1.98232638100002));
#317508=CARTESIAN_POINT('Ctrl Pts',(-3.95273386500006,5.2,-1.98232638100002));
#317509=CARTESIAN_POINT('Ctrl Pts',(-3.95273386500006,2.2,-1.98232638100002));
#317510=CARTESIAN_POINT('Ctrl Pts',(-3.95401773000006,12.2,-1.98397500200001));
#317511=CARTESIAN_POINT('Ctrl Pts',(-3.95401773000006,5.2,-1.98397500200001));
#317512=CARTESIAN_POINT('Ctrl Pts',(-3.95401773000006,2.2,-1.98397500200001));
#317513=CARTESIAN_POINT('Ctrl Pts',(-3.95530221600006,12.2,-1.98562816600001));
#317514=CARTESIAN_POINT('Ctrl Pts',(-3.95530221600006,5.2,-1.98562816600001));
#317515=CARTESIAN_POINT('Ctrl Pts',(-3.95530221600006,2.2,-1.98562816600001));
#317516=CARTESIAN_POINT('Ctrl Pts',(-3.95658731200006,12.2,-1.98728587300002));
#317517=CARTESIAN_POINT('Ctrl Pts',(-3.95658731200006,5.2,-1.98728587300002));
#317518=CARTESIAN_POINT('Ctrl Pts',(-3.95658731200006,2.2,-1.98728587300002));
#317519=CARTESIAN_POINT('Ctrl Pts',(-3.95787300900006,12.2,-1.98894812000002));
#317520=CARTESIAN_POINT('Ctrl Pts',(-3.95787300900006,5.2,-1.98894812000002));
#317521=CARTESIAN_POINT('Ctrl Pts',(-3.95787300900006,2.2,-1.98894812000002));
#317522=CARTESIAN_POINT('Ctrl Pts',(-3.95915929600006,12.2,-1.99061490800001));
#317523=CARTESIAN_POINT('Ctrl Pts',(-3.95915929600006,5.2,-1.99061490800001));
#317524=CARTESIAN_POINT('Ctrl Pts',(-3.95915929600006,2.2,-1.99061490800001));
#317525=CARTESIAN_POINT('Ctrl Pts',(-3.96044616200006,12.2,-1.99228623500002));
#317526=CARTESIAN_POINT('Ctrl Pts',(-3.96044616200006,5.2,-1.99228623500002));
#317527=CARTESIAN_POINT('Ctrl Pts',(-3.96044616200006,2.2,-1.99228623500002));
#317528=CARTESIAN_POINT('Ctrl Pts',(-3.96173359600006,12.2,-1.99396210000002));
#317529=CARTESIAN_POINT('Ctrl Pts',(-3.96173359600006,5.2,-1.99396210000002));
#317530=CARTESIAN_POINT('Ctrl Pts',(-3.96173359600006,2.2,-1.99396210000002));
#317531=CARTESIAN_POINT('Ctrl Pts',(-3.96302159000006,12.2,-1.99564250400002));
#317532=CARTESIAN_POINT('Ctrl Pts',(-3.96302159000006,5.2,-1.99564250400002));
#317533=CARTESIAN_POINT('Ctrl Pts',(-3.96302159000006,2.2,-1.99564250400002));
#317534=CARTESIAN_POINT('Ctrl Pts',(-3.96431013200006,12.2,-1.99732744500002));
#317535=CARTESIAN_POINT('Ctrl Pts',(-3.96431013200006,5.2,-1.99732744500002));
#317536=CARTESIAN_POINT('Ctrl Pts',(-3.96431013200006,2.2,-1.99732744500002));
#317537=CARTESIAN_POINT('Ctrl Pts',(-3.96559921100006,12.2,-1.99901692200001));
#317538=CARTESIAN_POINT('Ctrl Pts',(-3.96559921100006,5.2,-1.99901692200001));
#317539=CARTESIAN_POINT('Ctrl Pts',(-3.96559921100006,2.2,-1.99901692200001));
#317540=CARTESIAN_POINT('Ctrl Pts',(-3.96688881800006,12.2,-2.00071093300001));
#317541=CARTESIAN_POINT('Ctrl Pts',(-3.96688881800006,5.2,-2.00071093300001));
#317542=CARTESIAN_POINT('Ctrl Pts',(-3.96688881800006,2.2,-2.00071093300001));
#317543=CARTESIAN_POINT('Ctrl Pts',(-3.96817894300006,12.2,-2.00240947900001));
#317544=CARTESIAN_POINT('Ctrl Pts',(-3.96817894300006,5.2,-2.00240947900001));
#317545=CARTESIAN_POINT('Ctrl Pts',(-3.96817894300006,2.2,-2.00240947900001));
#317546=CARTESIAN_POINT('Ctrl Pts',(-3.96946957500006,12.2,-2.00411255800002));
#317547=CARTESIAN_POINT('Ctrl Pts',(-3.96946957500006,5.2,-2.00411255800002));
#317548=CARTESIAN_POINT('Ctrl Pts',(-3.96946957500006,2.2,-2.00411255800002));
#317549=CARTESIAN_POINT('Ctrl Pts',(-3.97076070300006,12.2,-2.00582017000002));
#317550=CARTESIAN_POINT('Ctrl Pts',(-3.97076070300006,5.2,-2.00582017000002));
#317551=CARTESIAN_POINT('Ctrl Pts',(-3.97076070300006,2.2,-2.00582017000002));
#317552=CARTESIAN_POINT('Ctrl Pts',(-3.97205231700006,12.2,-2.00753231300002));
#317553=CARTESIAN_POINT('Ctrl Pts',(-3.97205231700006,5.2,-2.00753231300002));
#317554=CARTESIAN_POINT('Ctrl Pts',(-3.97205231700006,2.2,-2.00753231300002));
#317555=CARTESIAN_POINT('Ctrl Pts',(-3.97334440800006,12.2,-2.00924898700002));
#317556=CARTESIAN_POINT('Ctrl Pts',(-3.97334440800006,5.2,-2.00924898700002));
#317557=CARTESIAN_POINT('Ctrl Pts',(-3.97334440800006,2.2,-2.00924898700002));
#317558=CARTESIAN_POINT('Ctrl Pts',(-3.97463696500005,12.2,-2.01097019000001));
#317559=CARTESIAN_POINT('Ctrl Pts',(-3.97463696500005,5.2,-2.01097019000001));
#317560=CARTESIAN_POINT('Ctrl Pts',(-3.97463696500005,2.2,-2.01097019000001));
#317561=CARTESIAN_POINT('Ctrl Pts',(-3.97592997700006,12.2,-2.01269592100001));
#317562=CARTESIAN_POINT('Ctrl Pts',(-3.97592997700006,5.2,-2.01269592100001));
#317563=CARTESIAN_POINT('Ctrl Pts',(-3.97592997700006,2.2,-2.01269592100001));
#317564=CARTESIAN_POINT('Ctrl Pts',(-3.97722343500006,12.2,-2.01442618000002));
#317565=CARTESIAN_POINT('Ctrl Pts',(-3.97722343500006,5.2,-2.01442618000002));
#317566=CARTESIAN_POINT('Ctrl Pts',(-3.97722343500006,2.2,-2.01442618000002));
#317567=CARTESIAN_POINT('Ctrl Pts',(-3.97851732900006,12.2,-2.01616096600001));
#317568=CARTESIAN_POINT('Ctrl Pts',(-3.97851732900006,5.2,-2.01616096600001));
#317569=CARTESIAN_POINT('Ctrl Pts',(-3.97851732900006,2.2,-2.01616096600001));
#317570=CARTESIAN_POINT('Ctrl Pts',(-3.97981164700006,12.2,-2.01790027700001));
#317571=CARTESIAN_POINT('Ctrl Pts',(-3.97981164700006,5.2,-2.01790027700001));
#317572=CARTESIAN_POINT('Ctrl Pts',(-3.97981164700006,2.2,-2.01790027700001));
#317573=CARTESIAN_POINT('Ctrl Pts',(-3.98110638100006,12.2,-2.01964411200001));
#317574=CARTESIAN_POINT('Ctrl Pts',(-3.98110638100006,5.2,-2.01964411200001));
#317575=CARTESIAN_POINT('Ctrl Pts',(-3.98110638100006,2.2,-2.01964411200001));
#317576=CARTESIAN_POINT('Ctrl Pts',(-3.98240151900006,12.2,-2.02139247000002));
#317577=CARTESIAN_POINT('Ctrl Pts',(-3.98240151900006,5.2,-2.02139247000002));
#317578=CARTESIAN_POINT('Ctrl Pts',(-3.98240151900006,2.2,-2.02139247000002));
#317579=CARTESIAN_POINT('Ctrl Pts',(-3.98369705200006,12.2,-2.02314535000002));
#317580=CARTESIAN_POINT('Ctrl Pts',(-3.98369705200006,5.2,-2.02314535000002));
#317581=CARTESIAN_POINT('Ctrl Pts',(-3.98369705200006,2.2,-2.02314535000002));
#317582=CARTESIAN_POINT('Ctrl Pts',(-3.98499297100006,12.2,-2.02490275300002));
#317583=CARTESIAN_POINT('Ctrl Pts',(-3.98499297100006,5.2,-2.02490275300002));
#317584=CARTESIAN_POINT('Ctrl Pts',(-3.98499297100006,2.2,-2.02490275300002));
#317585=CARTESIAN_POINT('Ctrl Pts',(-3.98628926300006,12.2,-2.02666467500002));
#317586=CARTESIAN_POINT('Ctrl Pts',(-3.98628926300006,5.2,-2.02666467500002));
#317587=CARTESIAN_POINT('Ctrl Pts',(-3.98628926300006,2.2,-2.02666467500002));
#317588=CARTESIAN_POINT('Ctrl Pts',(-3.98758592100006,12.2,-2.02843111500002));
#317589=CARTESIAN_POINT('Ctrl Pts',(-3.98758592100006,5.2,-2.02843111500002));
#317590=CARTESIAN_POINT('Ctrl Pts',(-3.98758592100006,2.2,-2.02843111500002));
#317591=CARTESIAN_POINT('Ctrl Pts',(-3.98888293200006,12.2,-2.03020207400002));
#317592=CARTESIAN_POINT('Ctrl Pts',(-3.98888293200006,5.2,-2.03020207400002));
#317593=CARTESIAN_POINT('Ctrl Pts',(-3.98888293200006,2.2,-2.03020207400002));
#317594=CARTESIAN_POINT('Ctrl Pts',(-3.99018028800006,12.2,-2.03197754900001));
#317595=CARTESIAN_POINT('Ctrl Pts',(-3.99018028800006,5.2,-2.03197754900001));
#317596=CARTESIAN_POINT('Ctrl Pts',(-3.99018028800006,2.2,-2.03197754900001));
#317597=CARTESIAN_POINT('Ctrl Pts',(-3.99147798000006,12.2,-2.03375754000001));
#317598=CARTESIAN_POINT('Ctrl Pts',(-3.99147798000006,5.2,-2.03375754000001));
#317599=CARTESIAN_POINT('Ctrl Pts',(-3.99147798000006,2.2,-2.03375754000001));
#317600=CARTESIAN_POINT('Ctrl Pts',(-3.99277599500006,12.2,-2.03554204600001));
#317601=CARTESIAN_POINT('Ctrl Pts',(-3.99277599500006,5.2,-2.03554204600001));
#317602=CARTESIAN_POINT('Ctrl Pts',(-3.99277599500006,2.2,-2.03554204600001));
#317603=CARTESIAN_POINT('Ctrl Pts',(-3.99407432400006,12.2,-2.03733106400001));
#317604=CARTESIAN_POINT('Ctrl Pts',(-3.99407432400006,5.2,-2.03733106400001));
#317605=CARTESIAN_POINT('Ctrl Pts',(-3.99407432400006,2.2,-2.03733106400001));
#317606=CARTESIAN_POINT('Ctrl Pts',(-3.99537295900006,12.2,-2.03912459600001));
#317607=CARTESIAN_POINT('Ctrl Pts',(-3.99537295900006,5.2,-2.03912459600001));
#317608=CARTESIAN_POINT('Ctrl Pts',(-3.99537295900006,2.2,-2.03912459600001));
#317609=CARTESIAN_POINT('Ctrl Pts',(-3.99667188700006,12.2,-2.04092263700002));
#317610=CARTESIAN_POINT('Ctrl Pts',(-3.99667188700006,5.2,-2.04092263700002));
#317611=CARTESIAN_POINT('Ctrl Pts',(-3.99667188700006,2.2,-2.04092263700002));
#317612=CARTESIAN_POINT('Ctrl Pts',(-3.99797110100006,12.2,-2.04272518800002));
#317613=CARTESIAN_POINT('Ctrl Pts',(-3.99797110100006,5.2,-2.04272518800002));
#317614=CARTESIAN_POINT('Ctrl Pts',(-3.99797110100006,2.2,-2.04272518800002));
#317615=CARTESIAN_POINT('Ctrl Pts',(-3.99927058900006,12.2,-2.04453224800002));
#317616=CARTESIAN_POINT('Ctrl Pts',(-3.99927058900006,5.2,-2.04453224800002));
#317617=CARTESIAN_POINT('Ctrl Pts',(-3.99927058900006,2.2,-2.04453224800002));
#317618=CARTESIAN_POINT('Ctrl Pts',(-4.00057034200006,12.2,-2.04634381500002));
#317619=CARTESIAN_POINT('Ctrl Pts',(-4.00057034200006,5.2,-2.04634381500002));
#317620=CARTESIAN_POINT('Ctrl Pts',(-4.00057034200006,2.2,-2.04634381500002));
#317621=CARTESIAN_POINT('Ctrl Pts',(-4.00187034900005,12.2,-2.04815988800001));
#317622=CARTESIAN_POINT('Ctrl Pts',(-4.00187034900005,5.2,-2.04815988800001));
#317623=CARTESIAN_POINT('Ctrl Pts',(-4.00187034900005,2.2,-2.04815988800001));
#317624=CARTESIAN_POINT('Ctrl Pts',(-4.00317060200006,12.2,-2.04998046600001));
#317625=CARTESIAN_POINT('Ctrl Pts',(-4.00317060200006,5.2,-2.04998046600001));
#317626=CARTESIAN_POINT('Ctrl Pts',(-4.00317060200006,2.2,-2.04998046600001));
#317627=CARTESIAN_POINT('Ctrl Pts',(-4.00447109000006,12.2,-2.05180554700001));
#317628=CARTESIAN_POINT('Ctrl Pts',(-4.00447109000006,5.2,-2.05180554700001));
#317629=CARTESIAN_POINT('Ctrl Pts',(-4.00447109000006,2.2,-2.05180554700001));
#317630=CARTESIAN_POINT('Ctrl Pts',(-4.00577180300006,12.2,-2.05363513100002));
#317631=CARTESIAN_POINT('Ctrl Pts',(-4.00577180300006,5.2,-2.05363513100002));
#317632=CARTESIAN_POINT('Ctrl Pts',(-4.00577180300006,2.2,-2.05363513100002));
#317633=CARTESIAN_POINT('Ctrl Pts',(-4.00707273200006,12.2,-2.05546921500002));
#317634=CARTESIAN_POINT('Ctrl Pts',(-4.00707273200006,5.2,-2.05546921500002));
#317635=CARTESIAN_POINT('Ctrl Pts',(-4.00707273200006,2.2,-2.05546921500002));
#317636=CARTESIAN_POINT('Ctrl Pts',(-4.00837386700006,12.2,-2.05730780000001));
#317637=CARTESIAN_POINT('Ctrl Pts',(-4.00837386700006,5.2,-2.05730780000001));
#317638=CARTESIAN_POINT('Ctrl Pts',(-4.00837386700006,2.2,-2.05730780000001));
#317639=CARTESIAN_POINT('Ctrl Pts',(-4.00967519800006,12.2,-2.05915088300001));
#317640=CARTESIAN_POINT('Ctrl Pts',(-4.00967519800006,5.2,-2.05915088300001));
#317641=CARTESIAN_POINT('Ctrl Pts',(-4.00967519800006,2.2,-2.05915088300001));
#317642=CARTESIAN_POINT('Ctrl Pts',(-4.01097671400006,12.2,-2.06099846200001));
#317643=CARTESIAN_POINT('Ctrl Pts',(-4.01097671400006,5.2,-2.06099846200001));
#317644=CARTESIAN_POINT('Ctrl Pts',(-4.01097671400006,2.2,-2.06099846200001));
#317645=CARTESIAN_POINT('Ctrl Pts',(-4.01227840700006,12.2,-2.06285053800002));
#317646=CARTESIAN_POINT('Ctrl Pts',(-4.01227840700006,5.2,-2.06285053800002));
#317647=CARTESIAN_POINT('Ctrl Pts',(-4.01227840700006,2.2,-2.06285053800002));
#317648=CARTESIAN_POINT('Ctrl Pts',(-4.01358026700006,12.2,-2.06470710700001));
#317649=CARTESIAN_POINT('Ctrl Pts',(-4.01358026700006,5.2,-2.06470710700001));
#317650=CARTESIAN_POINT('Ctrl Pts',(-4.01358026700006,2.2,-2.06470710700001));
#317651=CARTESIAN_POINT('Ctrl Pts',(-4.01488228300006,12.2,-2.06656817000002));
#317652=CARTESIAN_POINT('Ctrl Pts',(-4.01488228300006,5.2,-2.06656817000002));
#317653=CARTESIAN_POINT('Ctrl Pts',(-4.01488228300006,2.2,-2.06656817000002));
#317654=CARTESIAN_POINT('Ctrl Pts',(-4.01618444700006,12.2,-2.06843372500002));
#317655=CARTESIAN_POINT('Ctrl Pts',(-4.01618444700006,5.2,-2.06843372500002));
#317656=CARTESIAN_POINT('Ctrl Pts',(-4.01618444700006,2.2,-2.06843372500002));
#317657=CARTESIAN_POINT('Ctrl Pts',(-4.01748674700006,12.2,-2.07030376900001));
#317658=CARTESIAN_POINT('Ctrl Pts',(-4.01748674700006,5.2,-2.07030376900001));
#317659=CARTESIAN_POINT('Ctrl Pts',(-4.01748674700006,2.2,-2.07030376900001));
#317660=CARTESIAN_POINT('Ctrl Pts',(-4.01878917600006,12.2,-2.07217830200001));
#317661=CARTESIAN_POINT('Ctrl Pts',(-4.01878917600006,5.2,-2.07217830200001));
#317662=CARTESIAN_POINT('Ctrl Pts',(-4.01878917600006,2.2,-2.07217830200001));
#317663=CARTESIAN_POINT('Ctrl Pts',(-4.02009172300006,12.2,-2.07405732300002));
#317664=CARTESIAN_POINT('Ctrl Pts',(-4.02009172300006,5.2,-2.07405732300002));
#317665=CARTESIAN_POINT('Ctrl Pts',(-4.02009172300006,2.2,-2.07405732300002));
#317666=CARTESIAN_POINT('Ctrl Pts',(-4.02139437900006,12.2,-2.07594083000001));
#317667=CARTESIAN_POINT('Ctrl Pts',(-4.02139437900006,5.2,-2.07594083000001));
#317668=CARTESIAN_POINT('Ctrl Pts',(-4.02139437900006,2.2,-2.07594083000001));
#317669=CARTESIAN_POINT('Ctrl Pts',(-4.02269713300006,12.2,-2.07782882200001));
#317670=CARTESIAN_POINT('Ctrl Pts',(-4.02269713300006,5.2,-2.07782882200001));
#317671=CARTESIAN_POINT('Ctrl Pts',(-4.02269713300006,2.2,-2.07782882200001));
#317672=CARTESIAN_POINT('Ctrl Pts',(-4.02399997600006,12.2,-2.07972129700002));
#317673=CARTESIAN_POINT('Ctrl Pts',(-4.02399997600006,5.2,-2.07972129700002));
#317674=CARTESIAN_POINT('Ctrl Pts',(-4.02399997600006,2.2,-2.07972129700002));
#317675=CARTESIAN_POINT('Ctrl Pts',(-4.02530289900006,12.2,-2.08161825400001));
#317676=CARTESIAN_POINT('Ctrl Pts',(-4.02530289900006,5.2,-2.08161825400001));
#317677=CARTESIAN_POINT('Ctrl Pts',(-4.02530289900006,2.2,-2.08161825400001));
#317678=CARTESIAN_POINT('Ctrl Pts',(-4.02660589200006,12.2,-2.08351969100002));
#317679=CARTESIAN_POINT('Ctrl Pts',(-4.02660589200006,5.2,-2.08351969100002));
#317680=CARTESIAN_POINT('Ctrl Pts',(-4.02660589200006,2.2,-2.08351969100002));
#317681=CARTESIAN_POINT('Ctrl Pts',(-4.02790894500006,12.2,-2.08542560700002));
#317682=CARTESIAN_POINT('Ctrl Pts',(-4.02790894500006,5.2,-2.08542560700002));
#317683=CARTESIAN_POINT('Ctrl Pts',(-4.02790894500006,2.2,-2.08542560700002));
#317684=CARTESIAN_POINT('Ctrl Pts',(-4.02921204900006,12.2,-2.08733600100001));
#317685=CARTESIAN_POINT('Ctrl Pts',(-4.02921204900006,5.2,-2.08733600100001));
#317686=CARTESIAN_POINT('Ctrl Pts',(-4.02921204900006,2.2,-2.08733600100001));
#317687=CARTESIAN_POINT('Ctrl Pts',(-4.03051519400006,12.2,-2.08925087000001));
#317688=CARTESIAN_POINT('Ctrl Pts',(-4.03051519400006,5.2,-2.08925087000001));
#317689=CARTESIAN_POINT('Ctrl Pts',(-4.03051519400006,2.2,-2.08925087000001));
#317690=CARTESIAN_POINT('Ctrl Pts',(-4.03181837200006,12.2,-2.09117021300001));
#317691=CARTESIAN_POINT('Ctrl Pts',(-4.03181837200006,5.2,-2.09117021300001));
#317692=CARTESIAN_POINT('Ctrl Pts',(-4.03181837200006,2.2,-2.09117021300001));
#317693=CARTESIAN_POINT('Ctrl Pts',(-4.03312157100006,12.2,-2.09309403000002));
#317694=CARTESIAN_POINT('Ctrl Pts',(-4.03312157100006,5.2,-2.09309403000002));
#317695=CARTESIAN_POINT('Ctrl Pts',(-4.03312157100006,2.2,-2.09309403000002));
#317696=CARTESIAN_POINT('Ctrl Pts',(-4.03442478300006,12.2,-2.09502231700001));
#317697=CARTESIAN_POINT('Ctrl Pts',(-4.03442478300006,5.2,-2.09502231700001));
#317698=CARTESIAN_POINT('Ctrl Pts',(-4.03442478300006,2.2,-2.09502231700001));
#317699=CARTESIAN_POINT('Ctrl Pts',(-4.03572799900005,12.2,-2.09695507500001));
#317700=CARTESIAN_POINT('Ctrl Pts',(-4.03572799900005,5.2,-2.09695507500001));
#317701=CARTESIAN_POINT('Ctrl Pts',(-4.03572799900005,2.2,-2.09695507500001));
#317702=CARTESIAN_POINT('Ctrl Pts',(-4.03703120800006,12.2,-2.09889230200002));
#317703=CARTESIAN_POINT('Ctrl Pts',(-4.03703120800006,5.2,-2.09889230200002));
#317704=CARTESIAN_POINT('Ctrl Pts',(-4.03703120800006,2.2,-2.09889230200002));
#317705=CARTESIAN_POINT('Ctrl Pts',(-4.03833440100006,12.2,-2.10083399500002));
#317706=CARTESIAN_POINT('Ctrl Pts',(-4.03833440100006,5.2,-2.10083399500002));
#317707=CARTESIAN_POINT('Ctrl Pts',(-4.03833440100006,2.2,-2.10083399500002));
#317708=CARTESIAN_POINT('Ctrl Pts',(-4.03963757000006,12.2,-2.10278015200001));
#317709=CARTESIAN_POINT('Ctrl Pts',(-4.03963757000006,5.2,-2.10278015200001));
#317710=CARTESIAN_POINT('Ctrl Pts',(-4.03963757000006,2.2,-2.10278015200001));
#317711=CARTESIAN_POINT('Ctrl Pts',(-4.04094070300006,12.2,-2.10473077400001));
#317712=CARTESIAN_POINT('Ctrl Pts',(-4.04094070300006,5.2,-2.10473077400001));
#317713=CARTESIAN_POINT('Ctrl Pts',(-4.04094070300006,2.2,-2.10473077400001));
#317714=CARTESIAN_POINT('Ctrl Pts',(-4.04224379200006,12.2,-2.10668585800001));
#317715=CARTESIAN_POINT('Ctrl Pts',(-4.04224379200006,5.2,-2.10668585800001));
#317716=CARTESIAN_POINT('Ctrl Pts',(-4.04224379200006,2.2,-2.10668585800001));
#317717=CARTESIAN_POINT('Ctrl Pts',(-4.04354682900006,12.2,-2.10864540100001));
#317718=CARTESIAN_POINT('Ctrl Pts',(-4.04354682900006,5.2,-2.10864540100001));
#317719=CARTESIAN_POINT('Ctrl Pts',(-4.04354682900006,2.2,-2.10864540100001));
#317720=CARTESIAN_POINT('Ctrl Pts',(-4.04484980300006,12.2,-2.11060940500001));
#317721=CARTESIAN_POINT('Ctrl Pts',(-4.04484980300006,5.2,-2.11060940500001));
#317722=CARTESIAN_POINT('Ctrl Pts',(-4.04484980300006,2.2,-2.11060940500001));
#317723=CARTESIAN_POINT('Ctrl Pts',(-4.04615270400006,12.2,-2.11257786500001));
#317724=CARTESIAN_POINT('Ctrl Pts',(-4.04615270400006,5.2,-2.11257786500001));
#317725=CARTESIAN_POINT('Ctrl Pts',(-4.04615270400006,2.2,-2.11257786500001));
#317726=CARTESIAN_POINT('Ctrl Pts',(-4.04745552300006,12.2,-2.11455078000002));
#317727=CARTESIAN_POINT('Ctrl Pts',(-4.04745552300006,5.2,-2.11455078000002));
#317728=CARTESIAN_POINT('Ctrl Pts',(-4.04745552300006,2.2,-2.11455078000002));
#317729=CARTESIAN_POINT('Ctrl Pts',(-4.04875825300006,12.2,-2.11652814900001));
#317730=CARTESIAN_POINT('Ctrl Pts',(-4.04875825300006,5.2,-2.11652814900001));
#317731=CARTESIAN_POINT('Ctrl Pts',(-4.04875825300006,2.2,-2.11652814900001));
#317732=CARTESIAN_POINT('Ctrl Pts',(-4.05006088200006,12.2,-2.11850997100001));
#317733=CARTESIAN_POINT('Ctrl Pts',(-4.05006088200006,5.2,-2.11850997100001));
#317734=CARTESIAN_POINT('Ctrl Pts',(-4.05006088200006,2.2,-2.11850997100001));
#317735=CARTESIAN_POINT('Ctrl Pts',(-4.05136340100006,12.2,-2.12049624400001));
#317736=CARTESIAN_POINT('Ctrl Pts',(-4.05136340100006,5.2,-2.12049624400001));
#317737=CARTESIAN_POINT('Ctrl Pts',(-4.05136340100006,2.2,-2.12049624400001));
#317738=CARTESIAN_POINT('Ctrl Pts',(-4.05266580100006,12.2,-2.12248696500001));
#317739=CARTESIAN_POINT('Ctrl Pts',(-4.05266580100006,5.2,-2.12248696500001));
#317740=CARTESIAN_POINT('Ctrl Pts',(-4.05266580100006,2.2,-2.12248696500001));
#317741=CARTESIAN_POINT('Ctrl Pts',(-4.05396807400006,12.2,-2.12448213400001));
#317742=CARTESIAN_POINT('Ctrl Pts',(-4.05396807400006,5.2,-2.12448213400001));
#317743=CARTESIAN_POINT('Ctrl Pts',(-4.05396807400006,2.2,-2.12448213400001));
#317744=CARTESIAN_POINT('Ctrl Pts',(-4.05527020900006,12.2,-2.12648174800002));
#317745=CARTESIAN_POINT('Ctrl Pts',(-4.05527020900006,5.2,-2.12648174800002));
#317746=CARTESIAN_POINT('Ctrl Pts',(-4.05527020900006,2.2,-2.12648174800002));
#317747=CARTESIAN_POINT('Ctrl Pts',(-4.05657219900006,12.2,-2.12848580600001));
#317748=CARTESIAN_POINT('Ctrl Pts',(-4.05657219900006,5.2,-2.12848580600001));
#317749=CARTESIAN_POINT('Ctrl Pts',(-4.05657219900006,2.2,-2.12848580600001));
#317750=CARTESIAN_POINT('Ctrl Pts',(-4.05787403100006,12.2,-2.13049430600002));
#317751=CARTESIAN_POINT('Ctrl Pts',(-4.05787403100006,5.2,-2.13049430600002));
#317752=CARTESIAN_POINT('Ctrl Pts',(-4.05787403100006,2.2,-2.13049430600002));
#317753=CARTESIAN_POINT('Ctrl Pts',(-4.05917569900006,12.2,-2.13250724700002));
#317754=CARTESIAN_POINT('Ctrl Pts',(-4.05917569900006,5.2,-2.13250724700002));
#317755=CARTESIAN_POINT('Ctrl Pts',(-4.05917569900006,2.2,-2.13250724700002));
#317756=CARTESIAN_POINT('Ctrl Pts',(-4.06047719200005,12.2,-2.13452462600001));
#317757=CARTESIAN_POINT('Ctrl Pts',(-4.06047719200005,5.2,-2.13452462600001));
#317758=CARTESIAN_POINT('Ctrl Pts',(-4.06047719200005,2.2,-2.13452462600001));
#317759=CARTESIAN_POINT('Ctrl Pts',(-4.06177850300006,12.2,-2.13654644300002));
#317760=CARTESIAN_POINT('Ctrl Pts',(-4.06177850300006,5.2,-2.13654644300002));
#317761=CARTESIAN_POINT('Ctrl Pts',(-4.06177850300006,2.2,-2.13654644300002));
#317762=CARTESIAN_POINT('Ctrl Pts',(-4.06307962000006,12.2,-2.13857269400001));
#317763=CARTESIAN_POINT('Ctrl Pts',(-4.06307962000006,5.2,-2.13857269400001));
#317764=CARTESIAN_POINT('Ctrl Pts',(-4.06307962000006,2.2,-2.13857269400001));
#317765=CARTESIAN_POINT('Ctrl Pts',(-4.06438053600006,12.2,-2.14060338000001));
#317766=CARTESIAN_POINT('Ctrl Pts',(-4.06438053600006,5.2,-2.14060338000001));
#317767=CARTESIAN_POINT('Ctrl Pts',(-4.06438053600006,2.2,-2.14060338000001));
#317768=CARTESIAN_POINT('Ctrl Pts',(-4.06568124100006,12.2,-2.14263849600002));
#317769=CARTESIAN_POINT('Ctrl Pts',(-4.06568124100006,5.2,-2.14263849600002));
#317770=CARTESIAN_POINT('Ctrl Pts',(-4.06568124100006,2.2,-2.14263849600002));
#317771=CARTESIAN_POINT('Ctrl Pts',(-4.06698172500006,12.2,-2.14467804200002));
#317772=CARTESIAN_POINT('Ctrl Pts',(-4.06698172500006,5.2,-2.14467804200002));
#317773=CARTESIAN_POINT('Ctrl Pts',(-4.06698172500006,2.2,-2.14467804200002));
#317774=CARTESIAN_POINT('Ctrl Pts',(-4.06828198000006,12.2,-2.14672201700001));
#317775=CARTESIAN_POINT('Ctrl Pts',(-4.06828198000006,5.2,-2.14672201700001));
#317776=CARTESIAN_POINT('Ctrl Pts',(-4.06828198000006,2.2,-2.14672201700001));
#317777=CARTESIAN_POINT('Ctrl Pts',(-4.06958199700005,12.2,-2.14877041800001));
#317778=CARTESIAN_POINT('Ctrl Pts',(-4.06958199700005,5.2,-2.14877041800001));
#317779=CARTESIAN_POINT('Ctrl Pts',(-4.06958199700005,2.2,-2.14877041800001));
#317780=CARTESIAN_POINT('Ctrl Pts',(-4.07088176800006,12.2,-2.15082324300001));
#317781=CARTESIAN_POINT('Ctrl Pts',(-4.07088176800006,5.2,-2.15082324300001));
#317782=CARTESIAN_POINT('Ctrl Pts',(-4.07088176800006,2.2,-2.15082324300001));
#317783=CARTESIAN_POINT('Ctrl Pts',(-4.07218128100006,12.2,-2.15288049100002));
#317784=CARTESIAN_POINT('Ctrl Pts',(-4.07218128100006,5.2,-2.15288049100002));
#317785=CARTESIAN_POINT('Ctrl Pts',(-4.07218128100006,2.2,-2.15288049100002));
#317786=CARTESIAN_POINT('Ctrl Pts',(-4.07348052800006,12.2,-2.15494216100002));
#317787=CARTESIAN_POINT('Ctrl Pts',(-4.07348052800006,5.2,-2.15494216100002));
#317788=CARTESIAN_POINT('Ctrl Pts',(-4.07348052800006,2.2,-2.15494216100002));
#317789=CARTESIAN_POINT('Ctrl Pts',(-4.07477950200006,12.2,-2.15700824800001));
#317790=CARTESIAN_POINT('Ctrl Pts',(-4.07477950200006,5.2,-2.15700824800001));
#317791=CARTESIAN_POINT('Ctrl Pts',(-4.07477950200006,2.2,-2.15700824800001));
#317792=CARTESIAN_POINT('Ctrl Pts',(-4.07607819100006,12.2,-2.15907875300001));
#317793=CARTESIAN_POINT('Ctrl Pts',(-4.07607819100006,5.2,-2.15907875300001));
#317794=CARTESIAN_POINT('Ctrl Pts',(-4.07607819100006,2.2,-2.15907875300001));
#317795=CARTESIAN_POINT('Ctrl Pts',(-4.07737658800006,12.2,-2.16115367400001));
#317796=CARTESIAN_POINT('Ctrl Pts',(-4.07737658800006,5.2,-2.16115367400001));
#317797=CARTESIAN_POINT('Ctrl Pts',(-4.07737658800006,2.2,-2.16115367400001));
#317798=CARTESIAN_POINT('Ctrl Pts',(-4.07867468300006,12.2,-2.16323300600001));
#317799=CARTESIAN_POINT('Ctrl Pts',(-4.07867468300006,5.2,-2.16323300600001));
#317800=CARTESIAN_POINT('Ctrl Pts',(-4.07867468300006,2.2,-2.16323300600001));
#317801=CARTESIAN_POINT('Ctrl Pts',(-4.07997246700006,12.2,-2.16531675200001));
#317802=CARTESIAN_POINT('Ctrl Pts',(-4.07997246700006,5.2,-2.16531675200001));
#317803=CARTESIAN_POINT('Ctrl Pts',(-4.07997246700006,2.2,-2.16531675200001));
#317804=CARTESIAN_POINT('Ctrl Pts',(-4.08126993200006,12.2,-2.16740490600001));
#317805=CARTESIAN_POINT('Ctrl Pts',(-4.08126993200006,5.2,-2.16740490600001));
#317806=CARTESIAN_POINT('Ctrl Pts',(-4.08126993200006,2.2,-2.16740490600001));
#317807=CARTESIAN_POINT('Ctrl Pts',(-4.08256706800006,12.2,-2.16949746900001));
#317808=CARTESIAN_POINT('Ctrl Pts',(-4.08256706800006,5.2,-2.16949746900001));
#317809=CARTESIAN_POINT('Ctrl Pts',(-4.08256706800006,2.2,-2.16949746900001));
#317810=CARTESIAN_POINT('Ctrl Pts',(-4.08386386600006,12.2,-2.17159443700002));
#317811=CARTESIAN_POINT('Ctrl Pts',(-4.08386386600006,5.2,-2.17159443700002));
#317812=CARTESIAN_POINT('Ctrl Pts',(-4.08386386600006,2.2,-2.17159443700002));
#317813=CARTESIAN_POINT('Ctrl Pts',(-4.08516031900006,12.2,-2.17369580900002));
#317814=CARTESIAN_POINT('Ctrl Pts',(-4.08516031900006,5.2,-2.17369580900002));
#317815=CARTESIAN_POINT('Ctrl Pts',(-4.08516031900006,2.2,-2.17369580900002));
#317816=CARTESIAN_POINT('Ctrl Pts',(-4.08645641600006,12.2,-2.17580158300001));
#317817=CARTESIAN_POINT('Ctrl Pts',(-4.08645641600006,5.2,-2.17580158300001));
#317818=CARTESIAN_POINT('Ctrl Pts',(-4.08645641600006,2.2,-2.17580158300001));
#317819=CARTESIAN_POINT('Ctrl Pts',(-4.08775214800006,12.2,-2.17791175600001));
#317820=CARTESIAN_POINT('Ctrl Pts',(-4.08775214800006,5.2,-2.17791175600001));
#317821=CARTESIAN_POINT('Ctrl Pts',(-4.08775214800006,2.2,-2.17791175600001));
#317822=CARTESIAN_POINT('Ctrl Pts',(-4.08904750600006,12.2,-2.18002632800002));
#317823=CARTESIAN_POINT('Ctrl Pts',(-4.08904750600006,5.2,-2.18002632800002));
#317824=CARTESIAN_POINT('Ctrl Pts',(-4.08904750600006,2.2,-2.18002632800002));
#317825=CARTESIAN_POINT('Ctrl Pts',(-4.09034248300006,12.2,-2.18214529600001));
#317826=CARTESIAN_POINT('Ctrl Pts',(-4.09034248300006,5.2,-2.18214529600001));
#317827=CARTESIAN_POINT('Ctrl Pts',(-4.09034248300006,2.2,-2.18214529600001));
#317828=CARTESIAN_POINT('Ctrl Pts',(-4.09163706900006,12.2,-2.18426865800001));
#317829=CARTESIAN_POINT('Ctrl Pts',(-4.09163706900006,5.2,-2.18426865800001));
#317830=CARTESIAN_POINT('Ctrl Pts',(-4.09163706900006,2.2,-2.18426865800001));
#317831=CARTESIAN_POINT('Ctrl Pts',(-4.09293125500006,12.2,-2.18639641200001));
#317832=CARTESIAN_POINT('Ctrl Pts',(-4.09293125500006,5.2,-2.18639641200001));
#317833=CARTESIAN_POINT('Ctrl Pts',(-4.09293125500006,2.2,-2.18639641200001));
#317834=CARTESIAN_POINT('Ctrl Pts',(-4.09422503200005,12.2,-2.18852855500002));
#317835=CARTESIAN_POINT('Ctrl Pts',(-4.09422503200005,5.2,-2.18852855500002));
#317836=CARTESIAN_POINT('Ctrl Pts',(-4.09422503200005,2.2,-2.18852855500002));
#317837=CARTESIAN_POINT('Ctrl Pts',(-4.09551839200006,12.2,-2.19066508800001));
#317838=CARTESIAN_POINT('Ctrl Pts',(-4.09551839200006,5.2,-2.19066508800001));
#317839=CARTESIAN_POINT('Ctrl Pts',(-4.09551839200006,2.2,-2.19066508800001));
#317840=CARTESIAN_POINT('Ctrl Pts',(-4.09681132600006,12.2,-2.19280600600001));
#317841=CARTESIAN_POINT('Ctrl Pts',(-4.09681132600006,5.2,-2.19280600600001));
#317842=CARTESIAN_POINT('Ctrl Pts',(-4.09681132600006,2.2,-2.19280600600001));
#317843=CARTESIAN_POINT('Ctrl Pts',(-4.09810382400006,12.2,-2.19495130900001));
#317844=CARTESIAN_POINT('Ctrl Pts',(-4.09810382400006,5.2,-2.19495130900001));
#317845=CARTESIAN_POINT('Ctrl Pts',(-4.09810382400006,2.2,-2.19495130900001));
#317846=CARTESIAN_POINT('Ctrl Pts',(-4.09939587800006,12.2,-2.19710099300002));
#317847=CARTESIAN_POINT('Ctrl Pts',(-4.09939587800006,5.2,-2.19710099300002));
#317848=CARTESIAN_POINT('Ctrl Pts',(-4.09939587800006,2.2,-2.19710099300002));
#317849=CARTESIAN_POINT('Ctrl Pts',(-4.10068748000006,12.2,-2.19925505700001));
#317850=CARTESIAN_POINT('Ctrl Pts',(-4.10068748000006,5.2,-2.19925505700001));
#317851=CARTESIAN_POINT('Ctrl Pts',(-4.10068748000006,2.2,-2.19925505700001));
#317852=CARTESIAN_POINT('Ctrl Pts',(-4.10197862000006,12.2,-2.20141350000001));
#317853=CARTESIAN_POINT('Ctrl Pts',(-4.10197862000006,5.2,-2.20141350000001));
#317854=CARTESIAN_POINT('Ctrl Pts',(-4.10197862000006,2.2,-2.20141350000001));
#317855=CARTESIAN_POINT('Ctrl Pts',(-4.10326929000006,12.2,-2.20357631800002));
#317856=CARTESIAN_POINT('Ctrl Pts',(-4.10326929000006,5.2,-2.20357631800002));
#317857=CARTESIAN_POINT('Ctrl Pts',(-4.10326929000006,2.2,-2.20357631800002));
#317858=CARTESIAN_POINT('Ctrl Pts',(-4.10455948100005,12.2,-2.20574351000002));
#317859=CARTESIAN_POINT('Ctrl Pts',(-4.10455948100005,5.2,-2.20574351000002));
#317860=CARTESIAN_POINT('Ctrl Pts',(-4.10455948100005,2.2,-2.20574351000002));
#317861=CARTESIAN_POINT('Ctrl Pts',(-4.10584918400006,12.2,-2.20791507400001));
#317862=CARTESIAN_POINT('Ctrl Pts',(-4.10584918400006,5.2,-2.20791507400001));
#317863=CARTESIAN_POINT('Ctrl Pts',(-4.10584918400006,2.2,-2.20791507400001));
#317864=CARTESIAN_POINT('Ctrl Pts',(-4.10713839100006,12.2,-2.21009100700002));
#317865=CARTESIAN_POINT('Ctrl Pts',(-4.10713839100006,5.2,-2.21009100700002));
#317866=CARTESIAN_POINT('Ctrl Pts',(-4.10713839100006,2.2,-2.21009100700002));
#317867=CARTESIAN_POINT('Ctrl Pts',(-4.10842709300006,12.2,-2.21227130800001));
#317868=CARTESIAN_POINT('Ctrl Pts',(-4.10842709300006,5.2,-2.21227130800001));
#317869=CARTESIAN_POINT('Ctrl Pts',(-4.10842709300006,2.2,-2.21227130800001));
#317870=CARTESIAN_POINT('Ctrl Pts',(-4.10971528100006,12.2,-2.21445597400002));
#317871=CARTESIAN_POINT('Ctrl Pts',(-4.10971528100006,5.2,-2.21445597400002));
#317872=CARTESIAN_POINT('Ctrl Pts',(-4.10971528100006,2.2,-2.21445597400002));
#317873=CARTESIAN_POINT('Ctrl Pts',(-4.11100294700006,12.2,-2.21664500400002));
#317874=CARTESIAN_POINT('Ctrl Pts',(-4.11100294700006,5.2,-2.21664500400002));
#317875=CARTESIAN_POINT('Ctrl Pts',(-4.11100294700006,2.2,-2.21664500400002));
#317876=CARTESIAN_POINT('Ctrl Pts',(-4.11229008200006,12.2,-2.21883839500002));
#317877=CARTESIAN_POINT('Ctrl Pts',(-4.11229008200006,5.2,-2.21883839500002));
#317878=CARTESIAN_POINT('Ctrl Pts',(-4.11229008200006,2.2,-2.21883839500002));
#317879=CARTESIAN_POINT('Ctrl Pts',(-4.11357667600006,12.2,-2.22103614500002));
#317880=CARTESIAN_POINT('Ctrl Pts',(-4.11357667600006,5.2,-2.22103614500002));
#317881=CARTESIAN_POINT('Ctrl Pts',(-4.11357667600006,2.2,-2.22103614500002));
#317882=CARTESIAN_POINT('Ctrl Pts',(-4.11486272300006,12.2,-2.22323825200001));
#317883=CARTESIAN_POINT('Ctrl Pts',(-4.11486272300006,5.2,-2.22323825200001));
#317884=CARTESIAN_POINT('Ctrl Pts',(-4.11486272300006,2.2,-2.22323825200001));
#317885=CARTESIAN_POINT('Ctrl Pts',(-4.11614821300006,12.2,-2.22544471500001));
#317886=CARTESIAN_POINT('Ctrl Pts',(-4.11614821300006,5.2,-2.22544471500001));
#317887=CARTESIAN_POINT('Ctrl Pts',(-4.11614821300006,2.2,-2.22544471500001));
#317888=CARTESIAN_POINT('Ctrl Pts',(-4.11743313600006,12.2,-2.22765552900002));
#317889=CARTESIAN_POINT('Ctrl Pts',(-4.11743313600006,5.2,-2.22765552900002));
#317890=CARTESIAN_POINT('Ctrl Pts',(-4.11743313600006,2.2,-2.22765552900002));
#317891=CARTESIAN_POINT('Ctrl Pts',(-4.11871748700006,12.2,-2.22987069300002));
#317892=CARTESIAN_POINT('Ctrl Pts',(-4.11871748700006,5.2,-2.22987069300002));
#317893=CARTESIAN_POINT('Ctrl Pts',(-4.11871748700006,2.2,-2.22987069300002));
#317894=CARTESIAN_POINT('Ctrl Pts',(-4.12000125400006,12.2,-2.23209020600001));
#317895=CARTESIAN_POINT('Ctrl Pts',(-4.12000125400006,5.2,-2.23209020600001));
#317896=CARTESIAN_POINT('Ctrl Pts',(-4.12000125400006,2.2,-2.23209020600001));
#317897=CARTESIAN_POINT('Ctrl Pts',(-4.12128443000006,12.2,-2.23431406600001));
#317898=CARTESIAN_POINT('Ctrl Pts',(-4.12128443000006,5.2,-2.23431406600001));
#317899=CARTESIAN_POINT('Ctrl Pts',(-4.12128443000006,2.2,-2.23431406600001));
#317900=CARTESIAN_POINT('Ctrl Pts',(-4.12256700600006,12.2,-2.23654226800001));
#317901=CARTESIAN_POINT('Ctrl Pts',(-4.12256700600006,5.2,-2.23654226800001));
#317902=CARTESIAN_POINT('Ctrl Pts',(-4.12256700600006,2.2,-2.23654226800001));
#317903=CARTESIAN_POINT('Ctrl Pts',(-4.12384897300006,12.2,-2.23877481400002));
#317904=CARTESIAN_POINT('Ctrl Pts',(-4.12384897300006,5.2,-2.23877481400002));
#317905=CARTESIAN_POINT('Ctrl Pts',(-4.12384897300006,2.2,-2.23877481400002));
#317906=CARTESIAN_POINT('Ctrl Pts',(-4.12513032400006,12.2,-2.24101169700001));
#317907=CARTESIAN_POINT('Ctrl Pts',(-4.12513032400006,5.2,-2.24101169700001));
#317908=CARTESIAN_POINT('Ctrl Pts',(-4.12513032400006,2.2,-2.24101169700001));
#317909=CARTESIAN_POINT('Ctrl Pts',(-4.12641104900006,12.2,-2.24325291900001));
#317910=CARTESIAN_POINT('Ctrl Pts',(-4.12641104900006,5.2,-2.24325291900001));
#317911=CARTESIAN_POINT('Ctrl Pts',(-4.12641104900006,2.2,-2.24325291900001));
#317912=CARTESIAN_POINT('Ctrl Pts',(-4.12769114100006,12.2,-2.24549847600001));
#317913=CARTESIAN_POINT('Ctrl Pts',(-4.12769114100006,5.2,-2.24549847600001));
#317914=CARTESIAN_POINT('Ctrl Pts',(-4.12769114100006,2.2,-2.24549847600001));
#317915=CARTESIAN_POINT('Ctrl Pts',(-4.12897059200006,12.2,-2.24774836500002));
#317916=CARTESIAN_POINT('Ctrl Pts',(-4.12897059200006,5.2,-2.24774836500002));
#317917=CARTESIAN_POINT('Ctrl Pts',(-4.12897059200006,2.2,-2.24774836500002));
#317918=CARTESIAN_POINT('Ctrl Pts',(-4.13024939300006,12.2,-2.25000258600002));
#317919=CARTESIAN_POINT('Ctrl Pts',(-4.13024939300006,5.2,-2.25000258600002));
#317920=CARTESIAN_POINT('Ctrl Pts',(-4.13024939300006,2.2,-2.25000258600002));
#317921=CARTESIAN_POINT('Ctrl Pts',(-4.13152753300006,12.2,-2.25226113500002));
#317922=CARTESIAN_POINT('Ctrl Pts',(-4.13152753300006,5.2,-2.25226113500002));
#317923=CARTESIAN_POINT('Ctrl Pts',(-4.13152753300006,2.2,-2.25226113500002));
#317924=CARTESIAN_POINT('Ctrl Pts',(-4.13280500400006,12.2,-2.25452400900001));
#317925=CARTESIAN_POINT('Ctrl Pts',(-4.13280500400006,5.2,-2.25452400900001));
#317926=CARTESIAN_POINT('Ctrl Pts',(-4.13280500400006,2.2,-2.25452400900001));
#317927=CARTESIAN_POINT('Ctrl Pts',(-4.13408180000006,12.2,-2.25679120600002));
#317928=CARTESIAN_POINT('Ctrl Pts',(-4.13408180000006,5.2,-2.25679120600002));
#317929=CARTESIAN_POINT('Ctrl Pts',(-4.13408180000006,2.2,-2.25679120600002));
#317930=CARTESIAN_POINT('Ctrl Pts',(-4.13535791000006,12.2,-2.25906272500001));
#317931=CARTESIAN_POINT('Ctrl Pts',(-4.13535791000006,5.2,-2.25906272500001));
#317932=CARTESIAN_POINT('Ctrl Pts',(-4.13535791000006,2.2,-2.25906272500001));
#317933=CARTESIAN_POINT('Ctrl Pts',(-4.13663332500006,12.2,-2.26133856300001));
#317934=CARTESIAN_POINT('Ctrl Pts',(-4.13663332500006,5.2,-2.26133856300001));
#317935=CARTESIAN_POINT('Ctrl Pts',(-4.13663332500006,2.2,-2.26133856300001));
#317936=CARTESIAN_POINT('Ctrl Pts',(-4.13790803900006,12.2,-2.26361871800002));
#317937=CARTESIAN_POINT('Ctrl Pts',(-4.13790803900006,5.2,-2.26361871800002));
#317938=CARTESIAN_POINT('Ctrl Pts',(-4.13790803900006,2.2,-2.26361871800002));
#317939=CARTESIAN_POINT('Ctrl Pts',(-4.13918204600006,12.2,-2.26590318700001));
#317940=CARTESIAN_POINT('Ctrl Pts',(-4.13918204600006,5.2,-2.26590318700001));
#317941=CARTESIAN_POINT('Ctrl Pts',(-4.13918204600006,2.2,-2.26590318700001));
#317942=CARTESIAN_POINT('Ctrl Pts',(-4.14045533500006,12.2,-2.26819196900002));
#317943=CARTESIAN_POINT('Ctrl Pts',(-4.14045533500006,5.2,-2.26819196900002));
#317944=CARTESIAN_POINT('Ctrl Pts',(-4.14045533500006,2.2,-2.26819196900002));
#317945=CARTESIAN_POINT('Ctrl Pts',(-4.14172790000006,12.2,-2.27048506200001));
#317946=CARTESIAN_POINT('Ctrl Pts',(-4.14172790000006,5.2,-2.27048506200001));
#317947=CARTESIAN_POINT('Ctrl Pts',(-4.14172790000006,2.2,-2.27048506200001));
#317948=CARTESIAN_POINT('Ctrl Pts',(-4.14299973200006,12.2,-2.27278246300001));
#317949=CARTESIAN_POINT('Ctrl Pts',(-4.14299973200006,5.2,-2.27278246300001));
#317950=CARTESIAN_POINT('Ctrl Pts',(-4.14299973200006,2.2,-2.27278246300001));
#317951=CARTESIAN_POINT('Ctrl Pts',(-4.14427082400006,12.2,-2.27508416800001));
#317952=CARTESIAN_POINT('Ctrl Pts',(-4.14427082400006,5.2,-2.27508416800001));
#317953=CARTESIAN_POINT('Ctrl Pts',(-4.14427082400006,2.2,-2.27508416800001));
#317954=CARTESIAN_POINT('Ctrl Pts',(-4.14554116200006,12.2,-2.27739017700001));
#317955=CARTESIAN_POINT('Ctrl Pts',(-4.14554116200006,5.2,-2.27739017700001));
#317956=CARTESIAN_POINT('Ctrl Pts',(-4.14554116200006,2.2,-2.27739017700001));
#317957=CARTESIAN_POINT('Ctrl Pts',(-4.14681073900006,12.2,-2.27970048600001));
#317958=CARTESIAN_POINT('Ctrl Pts',(-4.14681073900006,5.2,-2.27970048600001));
#317959=CARTESIAN_POINT('Ctrl Pts',(-4.14681073900006,2.2,-2.27970048600001));
#317960=CARTESIAN_POINT('Ctrl Pts',(-4.14807954300006,12.2,-2.28201509200002));
#317961=CARTESIAN_POINT('Ctrl Pts',(-4.14807954300006,5.2,-2.28201509200002));
#317962=CARTESIAN_POINT('Ctrl Pts',(-4.14807954300006,2.2,-2.28201509200002));
#317963=CARTESIAN_POINT('Ctrl Pts',(-4.14934756500006,12.2,-2.28433399200001));
#317964=CARTESIAN_POINT('Ctrl Pts',(-4.14934756500006,5.2,-2.28433399200001));
#317965=CARTESIAN_POINT('Ctrl Pts',(-4.14934756500006,2.2,-2.28433399200001));
#317966=CARTESIAN_POINT('Ctrl Pts',(-4.15061479800006,12.2,-2.28665718400002));
#317967=CARTESIAN_POINT('Ctrl Pts',(-4.15061479800006,5.2,-2.28665718400002));
#317968=CARTESIAN_POINT('Ctrl Pts',(-4.15061479800006,2.2,-2.28665718400002));
#317969=CARTESIAN_POINT('Ctrl Pts',(-4.15188123500006,12.2,-2.28898466500001));
#317970=CARTESIAN_POINT('Ctrl Pts',(-4.15188123500006,5.2,-2.28898466500001));
#317971=CARTESIAN_POINT('Ctrl Pts',(-4.15188123500006,2.2,-2.28898466500001));
#317972=CARTESIAN_POINT('Ctrl Pts',(-4.15314687200006,12.2,-2.29131643500001));
#317973=CARTESIAN_POINT('Ctrl Pts',(-4.15314687200006,5.2,-2.29131643500001));
#317974=CARTESIAN_POINT('Ctrl Pts',(-4.15314687200006,2.2,-2.29131643500001));
#317975=CARTESIAN_POINT('Ctrl Pts',(-4.15441170800006,12.2,-2.29365249400002));
#317976=CARTESIAN_POINT('Ctrl Pts',(-4.15441170800006,5.2,-2.29365249400002));
#317977=CARTESIAN_POINT('Ctrl Pts',(-4.15441170800006,2.2,-2.29365249400002));
#317978=CARTESIAN_POINT('Ctrl Pts',(-4.15542293400006,12.2,-2.29552477100002));
#317979=CARTESIAN_POINT('Ctrl Pts',(-4.15542293400006,5.2,-2.29552477100002));
#317980=CARTESIAN_POINT('Ctrl Pts',(-4.15542293400006,2.2,-2.29552477100002));
#317981=CARTESIAN_POINT('Ctrl Pts',(-4.15618099200006,12.2,-2.29693090800001));
#317982=CARTESIAN_POINT('Ctrl Pts',(-4.15618099200006,5.2,-2.29693090800001));
#317983=CARTESIAN_POINT('Ctrl Pts',(-4.15618099200006,2.2,-2.29693090800001));
#317984=CARTESIAN_POINT('Ctrl Pts',(-4.15668620300006,12.2,-2.29786919000002));
#317985=CARTESIAN_POINT('Ctrl Pts',(-4.15668620300006,5.2,-2.29786919000002));
#317986=CARTESIAN_POINT('Ctrl Pts',(-4.15668620300006,2.2,-2.29786919000002));
#317987=CARTESIAN_POINT('Ctrl Pts',(-4.15693876900006,12.2,-2.29833854600002));
#317988=CARTESIAN_POINT('Ctrl Pts',(-4.15693876900006,5.2,-2.29833854600002));
#317989=CARTESIAN_POINT('Ctrl Pts',(-4.15693876900006,2.2,-2.29833854600002));
#317990=CARTESIAN_POINT('',(-4.15693876900006,2.7,-2.29833854600002));
#317991=CARTESIAN_POINT('',(-4.15693876900006,12.2,-2.29833854600002));
#317992=CARTESIAN_POINT('Ctrl Pts',(-3.62475766000006,2.7,-1.67660193200001));
#317993=CARTESIAN_POINT('Ctrl Pts',(-3.62490182724496,2.7,-1.67666931856351));
#317994=CARTESIAN_POINT('Ctrl Pts',(-3.62504534863998,2.69999999999987,
-1.67673808461024));
#317995=CARTESIAN_POINT('Ctrl Pts',(-3.62548714022601,2.69999999999987,
-1.67695103313952));
#317996=CARTESIAN_POINT('Ctrl Pts',(-3.62580033592221,2.7,-1.67710491378894));
#317997=CARTESIAN_POINT('Ctrl Pts',(-3.62712381957932,2.7,-1.67776190097245));
#317998=CARTESIAN_POINT('Ctrl Pts',(-3.62821615035642,2.7,-1.67832401661082));
#317999=CARTESIAN_POINT('Ctrl Pts',(-3.63299368465797,2.7,-1.68083337629142));
#318000=CARTESIAN_POINT('Ctrl Pts',(-3.63693276565636,2.7,-1.68304846860218));
#318001=CARTESIAN_POINT('Ctrl Pts',(-3.65406401132597,2.7,-1.69305178840937));
#318002=CARTESIAN_POINT('Ctrl Pts',(-3.66795497508814,2.7,-1.70223215619653));
#318003=CARTESIAN_POINT('Ctrl Pts',(-3.71732841422647,2.7,-1.73712959869733));
#318004=CARTESIAN_POINT('Ctrl Pts',(-3.76195508351362,2.7,-1.77364496801825));
#318005=CARTESIAN_POINT('Ctrl Pts',(-3.90832243976127,2.7,-1.91812530395877));
#318006=CARTESIAN_POINT('Ctrl Pts',(-4.03404336095063,2.7,-2.06995587715245));
#318007=CARTESIAN_POINT('Ctrl Pts',(-4.15693876900006,2.7,-2.29833854600002));
#318008=CARTESIAN_POINT('Origin',(-5.66300478732629E-14,15.2,-1.77635683940025E-14));
#318009=CARTESIAN_POINT('',(-3.98353538000006,2.7,-2.58726610100002));
#318010=CARTESIAN_POINT('',(-3.98353538000006,12.2,-2.58726610100001));
#318011=CARTESIAN_POINT('Origin',(-5.66300478732629E-14,2.7,-1.92943768261394E-14));
#318012=CARTESIAN_POINT('Ctrl Pts',(-3.98353538000006,12.2,-2.58726610100001));
#318013=CARTESIAN_POINT('Ctrl Pts',(-3.98353538000006,5.2,-2.58726610100001));
#318014=CARTESIAN_POINT('Ctrl Pts',(-3.98353538000006,2.2,-2.58726610100001));
#318015=CARTESIAN_POINT('Ctrl Pts',(-3.98300238900006,12.2,-2.58726399500001));
#318016=CARTESIAN_POINT('Ctrl Pts',(-3.98300238900006,5.2,-2.58726399500001));
#318017=CARTESIAN_POINT('Ctrl Pts',(-3.98300238900006,2.2,-2.58726399500001));
#318018=CARTESIAN_POINT('Ctrl Pts',(-3.98193674700006,12.2,-2.58725951100002));
#318019=CARTESIAN_POINT('Ctrl Pts',(-3.98193674700006,5.2,-2.58725951100002));
#318020=CARTESIAN_POINT('Ctrl Pts',(-3.98193674700006,2.2,-2.58725951100002));
#318021=CARTESIAN_POINT('Ctrl Pts',(-3.98033930600006,12.2,-2.58725196700002));
#318022=CARTESIAN_POINT('Ctrl Pts',(-3.98033930600006,5.2,-2.58725196700002));
#318023=CARTESIAN_POINT('Ctrl Pts',(-3.98033930600006,2.2,-2.58725196700002));
#318024=CARTESIAN_POINT('Ctrl Pts',(-3.97821142800006,12.2,-2.58724027300001));
#318025=CARTESIAN_POINT('Ctrl Pts',(-3.97821142800006,5.2,-2.58724027300001));
#318026=CARTESIAN_POINT('Ctrl Pts',(-3.97821142800006,2.2,-2.58724027300001));
#318027=CARTESIAN_POINT('Ctrl Pts',(-3.97555498800005,12.2,-2.58722293000002));
#318028=CARTESIAN_POINT('Ctrl Pts',(-3.97555498800005,5.2,-2.58722293000002));
#318029=CARTESIAN_POINT('Ctrl Pts',(-3.97555498800005,2.2,-2.58722293000002));
#318030=CARTESIAN_POINT('Ctrl Pts',(-3.97290195400006,12.2,-2.58720286100001));
#318031=CARTESIAN_POINT('Ctrl Pts',(-3.97290195400006,5.2,-2.58720286100001));
#318032=CARTESIAN_POINT('Ctrl Pts',(-3.97290195400006,2.2,-2.58720286100001));
#318033=CARTESIAN_POINT('Ctrl Pts',(-3.97025232800006,12.2,-2.58718007100001));
#318034=CARTESIAN_POINT('Ctrl Pts',(-3.97025232800006,5.2,-2.58718007100001));
#318035=CARTESIAN_POINT('Ctrl Pts',(-3.97025232800006,2.2,-2.58718007100001));
#318036=CARTESIAN_POINT('Ctrl Pts',(-3.96760611500006,12.2,-2.58715456000001));
#318037=CARTESIAN_POINT('Ctrl Pts',(-3.96760611500006,5.2,-2.58715456000001));
#318038=CARTESIAN_POINT('Ctrl Pts',(-3.96760611500006,2.2,-2.58715456000001));
#318039=CARTESIAN_POINT('Ctrl Pts',(-3.96496331700006,12.2,-2.58712633300001));
#318040=CARTESIAN_POINT('Ctrl Pts',(-3.96496331700006,5.2,-2.58712633300001));
#318041=CARTESIAN_POINT('Ctrl Pts',(-3.96496331700006,2.2,-2.58712633300001));
#318042=CARTESIAN_POINT('Ctrl Pts',(-3.96232394100006,12.2,-2.58709539700002));
#318043=CARTESIAN_POINT('Ctrl Pts',(-3.96232394100006,5.2,-2.58709539700002));
#318044=CARTESIAN_POINT('Ctrl Pts',(-3.96232394100006,2.2,-2.58709539700002));
#318045=CARTESIAN_POINT('Ctrl Pts',(-3.95968799400006,12.2,-2.58706175800001));
#318046=CARTESIAN_POINT('Ctrl Pts',(-3.95968799400006,5.2,-2.58706175800001));
#318047=CARTESIAN_POINT('Ctrl Pts',(-3.95968799400006,2.2,-2.58706175800001));
#318048=CARTESIAN_POINT('Ctrl Pts',(-3.95705548200006,12.2,-2.58702542400002));
#318049=CARTESIAN_POINT('Ctrl Pts',(-3.95705548200006,5.2,-2.58702542400002));
#318050=CARTESIAN_POINT('Ctrl Pts',(-3.95705548200006,2.2,-2.58702542400002));
#318051=CARTESIAN_POINT('Ctrl Pts',(-3.95442641300006,12.2,-2.58698640200001));
#318052=CARTESIAN_POINT('Ctrl Pts',(-3.95442641300006,5.2,-2.58698640200001));
#318053=CARTESIAN_POINT('Ctrl Pts',(-3.95442641300006,2.2,-2.58698640200001));
#318054=CARTESIAN_POINT('Ctrl Pts',(-3.95180079600006,12.2,-2.58694470000002));
#318055=CARTESIAN_POINT('Ctrl Pts',(-3.95180079600006,5.2,-2.58694470000002));
#318056=CARTESIAN_POINT('Ctrl Pts',(-3.95180079600006,2.2,-2.58694470000002));
#318057=CARTESIAN_POINT('Ctrl Pts',(-3.94917863600006,12.2,-2.58690032500001));
#318058=CARTESIAN_POINT('Ctrl Pts',(-3.94917863600006,5.2,-2.58690032500001));
#318059=CARTESIAN_POINT('Ctrl Pts',(-3.94917863600006,2.2,-2.58690032500001));
#318060=CARTESIAN_POINT('Ctrl Pts',(-3.94655993800006,12.2,-2.58685328400002));
#318061=CARTESIAN_POINT('Ctrl Pts',(-3.94655993800006,5.2,-2.58685328400002));
#318062=CARTESIAN_POINT('Ctrl Pts',(-3.94655993800006,2.2,-2.58685328400002));
#318063=CARTESIAN_POINT('Ctrl Pts',(-3.94394470900005,12.2,-2.58680358300001));
#318064=CARTESIAN_POINT('Ctrl Pts',(-3.94394470900005,5.2,-2.58680358300001));
#318065=CARTESIAN_POINT('Ctrl Pts',(-3.94394470900005,2.2,-2.58680358300001));
#318066=CARTESIAN_POINT('Ctrl Pts',(-3.94133295400006,12.2,-2.58675122600001));
#318067=CARTESIAN_POINT('Ctrl Pts',(-3.94133295400006,5.2,-2.58675122600001));
#318068=CARTESIAN_POINT('Ctrl Pts',(-3.94133295400006,2.2,-2.58675122600001));
#318069=CARTESIAN_POINT('Ctrl Pts',(-3.93872467900006,12.2,-2.58669621900002));
#318070=CARTESIAN_POINT('Ctrl Pts',(-3.93872467900006,5.2,-2.58669621900002));
#318071=CARTESIAN_POINT('Ctrl Pts',(-3.93872467900006,2.2,-2.58669621900002));
#318072=CARTESIAN_POINT('Ctrl Pts',(-3.93611989000005,12.2,-2.58663856900001));
#318073=CARTESIAN_POINT('Ctrl Pts',(-3.93611989000005,5.2,-2.58663856900001));
#318074=CARTESIAN_POINT('Ctrl Pts',(-3.93611989000005,2.2,-2.58663856900001));
#318075=CARTESIAN_POINT('Ctrl Pts',(-3.93351859100005,12.2,-2.58657828100001));
#318076=CARTESIAN_POINT('Ctrl Pts',(-3.93351859100005,5.2,-2.58657828100001));
#318077=CARTESIAN_POINT('Ctrl Pts',(-3.93351859100005,2.2,-2.58657828100001));
#318078=CARTESIAN_POINT('Ctrl Pts',(-3.93092078900006,12.2,-2.58651536300002));
#318079=CARTESIAN_POINT('Ctrl Pts',(-3.93092078900006,5.2,-2.58651536300002));
#318080=CARTESIAN_POINT('Ctrl Pts',(-3.93092078900006,2.2,-2.58651536300002));
#318081=CARTESIAN_POINT('Ctrl Pts',(-3.92832648900006,12.2,-2.58644982000002));
#318082=CARTESIAN_POINT('Ctrl Pts',(-3.92832648900006,5.2,-2.58644982000002));
#318083=CARTESIAN_POINT('Ctrl Pts',(-3.92832648900006,2.2,-2.58644982000002));
#318084=CARTESIAN_POINT('Ctrl Pts',(-3.92573570000006,12.2,-2.58638165900001));
#318085=CARTESIAN_POINT('Ctrl Pts',(-3.92573570000006,5.2,-2.58638165900001));
#318086=CARTESIAN_POINT('Ctrl Pts',(-3.92573570000006,2.2,-2.58638165900001));
#318087=CARTESIAN_POINT('Ctrl Pts',(-3.92314842600006,12.2,-2.58631088600001));
#318088=CARTESIAN_POINT('Ctrl Pts',(-3.92314842600006,5.2,-2.58631088600001));
#318089=CARTESIAN_POINT('Ctrl Pts',(-3.92314842600006,2.2,-2.58631088600001));
#318090=CARTESIAN_POINT('Ctrl Pts',(-3.92056467300006,12.2,-2.58623750900002));
#318091=CARTESIAN_POINT('Ctrl Pts',(-3.92056467300006,5.2,-2.58623750900002));
#318092=CARTESIAN_POINT('Ctrl Pts',(-3.92056467300006,2.2,-2.58623750900002));
#318093=CARTESIAN_POINT('Ctrl Pts',(-3.91798444800005,12.2,-2.58616153400002));
#318094=CARTESIAN_POINT('Ctrl Pts',(-3.91798444800005,5.2,-2.58616153400002));
#318095=CARTESIAN_POINT('Ctrl Pts',(-3.91798444800005,2.2,-2.58616153400002));
#318096=CARTESIAN_POINT('Ctrl Pts',(-3.91540775700006,12.2,-2.58608296800002));
#318097=CARTESIAN_POINT('Ctrl Pts',(-3.91540775700006,5.2,-2.58608296800002));
#318098=CARTESIAN_POINT('Ctrl Pts',(-3.91540775700006,2.2,-2.58608296800002));
#318099=CARTESIAN_POINT('Ctrl Pts',(-3.91283460500006,12.2,-2.58600181500002));
#318100=CARTESIAN_POINT('Ctrl Pts',(-3.91283460500006,5.2,-2.58600181500002));
#318101=CARTESIAN_POINT('Ctrl Pts',(-3.91283460500006,2.2,-2.58600181500002));
#318102=CARTESIAN_POINT('Ctrl Pts',(-3.91026499800006,12.2,-2.58591808400002));
#318103=CARTESIAN_POINT('Ctrl Pts',(-3.91026499800006,5.2,-2.58591808400002));
#318104=CARTESIAN_POINT('Ctrl Pts',(-3.91026499800006,2.2,-2.58591808400002));
#318105=CARTESIAN_POINT('Ctrl Pts',(-3.90769894300006,12.2,-2.58583178100002));
#318106=CARTESIAN_POINT('Ctrl Pts',(-3.90769894300006,5.2,-2.58583178100002));
#318107=CARTESIAN_POINT('Ctrl Pts',(-3.90769894300006,2.2,-2.58583178100002));
#318108=CARTESIAN_POINT('Ctrl Pts',(-3.90513644400006,12.2,-2.58574291000001));
#318109=CARTESIAN_POINT('Ctrl Pts',(-3.90513644400006,5.2,-2.58574291000001));
#318110=CARTESIAN_POINT('Ctrl Pts',(-3.90513644400006,2.2,-2.58574291000001));
#318111=CARTESIAN_POINT('Ctrl Pts',(-3.90257750900005,12.2,-2.58565148100002));
#318112=CARTESIAN_POINT('Ctrl Pts',(-3.90257750900005,5.2,-2.58565148100002));
#318113=CARTESIAN_POINT('Ctrl Pts',(-3.90257750900005,2.2,-2.58565148100002));
#318114=CARTESIAN_POINT('Ctrl Pts',(-3.90002214200006,12.2,-2.58555749800002));
#318115=CARTESIAN_POINT('Ctrl Pts',(-3.90002214200006,5.2,-2.58555749800002));
#318116=CARTESIAN_POINT('Ctrl Pts',(-3.90002214200006,2.2,-2.58555749800002));
#318117=CARTESIAN_POINT('Ctrl Pts',(-3.89747035000005,12.2,-2.58546096800002));
#318118=CARTESIAN_POINT('Ctrl Pts',(-3.89747035000005,5.2,-2.58546096800002));
#318119=CARTESIAN_POINT('Ctrl Pts',(-3.89747035000005,2.2,-2.58546096800002));
#318120=CARTESIAN_POINT('Ctrl Pts',(-3.89492214000006,12.2,-2.58536190000001));
#318121=CARTESIAN_POINT('Ctrl Pts',(-3.89492214000006,5.2,-2.58536190000001));
#318122=CARTESIAN_POINT('Ctrl Pts',(-3.89492214000006,2.2,-2.58536190000001));
#318123=CARTESIAN_POINT('Ctrl Pts',(-3.89237751600006,12.2,-2.58526029800001));
#318124=CARTESIAN_POINT('Ctrl Pts',(-3.89237751600006,5.2,-2.58526029800001));
#318125=CARTESIAN_POINT('Ctrl Pts',(-3.89237751600006,2.2,-2.58526029800001));
#318126=CARTESIAN_POINT('Ctrl Pts',(-3.88983648600006,12.2,-2.58515616800001));
#318127=CARTESIAN_POINT('Ctrl Pts',(-3.88983648600006,5.2,-2.58515616800001));
#318128=CARTESIAN_POINT('Ctrl Pts',(-3.88983648600006,2.2,-2.58515616800001));
#318129=CARTESIAN_POINT('Ctrl Pts',(-3.88729905400006,12.2,-2.58504951900001));
#318130=CARTESIAN_POINT('Ctrl Pts',(-3.88729905400006,5.2,-2.58504951900001));
#318131=CARTESIAN_POINT('Ctrl Pts',(-3.88729905400006,2.2,-2.58504951900001));
#318132=CARTESIAN_POINT('Ctrl Pts',(-3.88476522700006,12.2,-2.58494035600001));
#318133=CARTESIAN_POINT('Ctrl Pts',(-3.88476522700006,5.2,-2.58494035600001));
#318134=CARTESIAN_POINT('Ctrl Pts',(-3.88476522700006,2.2,-2.58494035600001));
#318135=CARTESIAN_POINT('Ctrl Pts',(-3.88223501100006,12.2,-2.58482868700002));
#318136=CARTESIAN_POINT('Ctrl Pts',(-3.88223501100006,5.2,-2.58482868700002));
#318137=CARTESIAN_POINT('Ctrl Pts',(-3.88223501100006,2.2,-2.58482868700002));
#318138=CARTESIAN_POINT('Ctrl Pts',(-3.87970841200006,12.2,-2.58471451800002));
#318139=CARTESIAN_POINT('Ctrl Pts',(-3.87970841200006,5.2,-2.58471451800002));
#318140=CARTESIAN_POINT('Ctrl Pts',(-3.87970841200006,2.2,-2.58471451800002));
#318141=CARTESIAN_POINT('Ctrl Pts',(-3.87718543400006,12.2,-2.58459785500001));
#318142=CARTESIAN_POINT('Ctrl Pts',(-3.87718543400006,5.2,-2.58459785500001));
#318143=CARTESIAN_POINT('Ctrl Pts',(-3.87718543400006,2.2,-2.58459785500001));
#318144=CARTESIAN_POINT('Ctrl Pts',(-3.87466608600006,12.2,-2.58447870600001));
#318145=CARTESIAN_POINT('Ctrl Pts',(-3.87466608600006,5.2,-2.58447870600001));
#318146=CARTESIAN_POINT('Ctrl Pts',(-3.87466608600006,2.2,-2.58447870600001));
#318147=CARTESIAN_POINT('Ctrl Pts',(-3.87215037100006,12.2,-2.58435707700002));
#318148=CARTESIAN_POINT('Ctrl Pts',(-3.87215037100006,5.2,-2.58435707700002));
#318149=CARTESIAN_POINT('Ctrl Pts',(-3.87215037100006,2.2,-2.58435707700002));
#318150=CARTESIAN_POINT('Ctrl Pts',(-3.86963829700006,12.2,-2.58423297400002));
#318151=CARTESIAN_POINT('Ctrl Pts',(-3.86963829700006,5.2,-2.58423297400002));
#318152=CARTESIAN_POINT('Ctrl Pts',(-3.86963829700006,2.2,-2.58423297400002));
#318153=CARTESIAN_POINT('Ctrl Pts',(-3.86712987000006,12.2,-2.58410640500002));
#318154=CARTESIAN_POINT('Ctrl Pts',(-3.86712987000006,5.2,-2.58410640500002));
#318155=CARTESIAN_POINT('Ctrl Pts',(-3.86712987000006,2.2,-2.58410640500002));
#318156=CARTESIAN_POINT('Ctrl Pts',(-3.86462509500006,12.2,-2.58397737600002));
#318157=CARTESIAN_POINT('Ctrl Pts',(-3.86462509500006,5.2,-2.58397737600002));
#318158=CARTESIAN_POINT('Ctrl Pts',(-3.86462509500006,2.2,-2.58397737600002));
#318159=CARTESIAN_POINT('Ctrl Pts',(-3.86212397800006,12.2,-2.58384589300002));
#318160=CARTESIAN_POINT('Ctrl Pts',(-3.86212397800006,5.2,-2.58384589300002));
#318161=CARTESIAN_POINT('Ctrl Pts',(-3.86212397800006,2.2,-2.58384589300002));
#318162=CARTESIAN_POINT('Ctrl Pts',(-3.85962652500006,12.2,-2.58371196500002));
#318163=CARTESIAN_POINT('Ctrl Pts',(-3.85962652500006,5.2,-2.58371196500002));
#318164=CARTESIAN_POINT('Ctrl Pts',(-3.85962652500006,2.2,-2.58371196500002));
#318165=CARTESIAN_POINT('Ctrl Pts',(-3.85713274200006,12.2,-2.58357559700002));
#318166=CARTESIAN_POINT('Ctrl Pts',(-3.85713274200006,5.2,-2.58357559700002));
#318167=CARTESIAN_POINT('Ctrl Pts',(-3.85713274200006,2.2,-2.58357559700002));
#318168=CARTESIAN_POINT('Ctrl Pts',(-3.85464263400006,12.2,-2.58343679700001));
#318169=CARTESIAN_POINT('Ctrl Pts',(-3.85464263400006,5.2,-2.58343679700001));
#318170=CARTESIAN_POINT('Ctrl Pts',(-3.85464263400006,2.2,-2.58343679700001));
#318171=CARTESIAN_POINT('Ctrl Pts',(-3.85215621000006,12.2,-2.58329557100001));
#318172=CARTESIAN_POINT('Ctrl Pts',(-3.85215621000006,5.2,-2.58329557100001));
#318173=CARTESIAN_POINT('Ctrl Pts',(-3.85215621000006,2.2,-2.58329557100001));
#318174=CARTESIAN_POINT('Ctrl Pts',(-3.84967347300006,12.2,-2.58315192700001));
#318175=CARTESIAN_POINT('Ctrl Pts',(-3.84967347300006,5.2,-2.58315192700001));
#318176=CARTESIAN_POINT('Ctrl Pts',(-3.84967347300006,2.2,-2.58315192700001));
#318177=CARTESIAN_POINT('Ctrl Pts',(-3.84719442900006,12.2,-2.58300587100001));
#318178=CARTESIAN_POINT('Ctrl Pts',(-3.84719442900006,5.2,-2.58300587100001));
#318179=CARTESIAN_POINT('Ctrl Pts',(-3.84719442900006,2.2,-2.58300587100001));
#318180=CARTESIAN_POINT('Ctrl Pts',(-3.84471908500006,12.2,-2.58285740900002));
#318181=CARTESIAN_POINT('Ctrl Pts',(-3.84471908500006,5.2,-2.58285740900002));
#318182=CARTESIAN_POINT('Ctrl Pts',(-3.84471908500006,2.2,-2.58285740900002));
#318183=CARTESIAN_POINT('Ctrl Pts',(-3.84224744700006,12.2,-2.58270654900001));
#318184=CARTESIAN_POINT('Ctrl Pts',(-3.84224744700006,5.2,-2.58270654900001));
#318185=CARTESIAN_POINT('Ctrl Pts',(-3.84224744700006,2.2,-2.58270654900001));
#318186=CARTESIAN_POINT('Ctrl Pts',(-3.83977951900006,12.2,-2.58255329800001));
#318187=CARTESIAN_POINT('Ctrl Pts',(-3.83977951900006,5.2,-2.58255329800001));
#318188=CARTESIAN_POINT('Ctrl Pts',(-3.83977951900006,2.2,-2.58255329800001));
#318189=CARTESIAN_POINT('Ctrl Pts',(-3.83731530900006,12.2,-2.58239766400001));
#318190=CARTESIAN_POINT('Ctrl Pts',(-3.83731530900006,5.2,-2.58239766400001));
#318191=CARTESIAN_POINT('Ctrl Pts',(-3.83731530900006,2.2,-2.58239766400001));
#318192=CARTESIAN_POINT('Ctrl Pts',(-3.83485482300006,12.2,-2.58223965200001));
#318193=CARTESIAN_POINT('Ctrl Pts',(-3.83485482300006,5.2,-2.58223965200001));
#318194=CARTESIAN_POINT('Ctrl Pts',(-3.83485482300006,2.2,-2.58223965200001));
#318195=CARTESIAN_POINT('Ctrl Pts',(-3.83239806600006,12.2,-2.58207926900001));
#318196=CARTESIAN_POINT('Ctrl Pts',(-3.83239806600006,5.2,-2.58207926900001));
#318197=CARTESIAN_POINT('Ctrl Pts',(-3.83239806600006,2.2,-2.58207926900001));
#318198=CARTESIAN_POINT('Ctrl Pts',(-3.82994504400005,12.2,-2.58191652300002));
#318199=CARTESIAN_POINT('Ctrl Pts',(-3.82994504400005,5.2,-2.58191652300002));
#318200=CARTESIAN_POINT('Ctrl Pts',(-3.82994504400005,2.2,-2.58191652300002));
#318201=CARTESIAN_POINT('Ctrl Pts',(-3.82749576200006,12.2,-2.58175142100002));
#318202=CARTESIAN_POINT('Ctrl Pts',(-3.82749576200006,5.2,-2.58175142100002));
#318203=CARTESIAN_POINT('Ctrl Pts',(-3.82749576200006,2.2,-2.58175142100002));
#318204=CARTESIAN_POINT('Ctrl Pts',(-3.82505022800006,12.2,-2.58158396900001));
#318205=CARTESIAN_POINT('Ctrl Pts',(-3.82505022800006,5.2,-2.58158396900001));
#318206=CARTESIAN_POINT('Ctrl Pts',(-3.82505022800006,2.2,-2.58158396900001));
#318207=CARTESIAN_POINT('Ctrl Pts',(-3.82260844600006,12.2,-2.58141417600001));
#318208=CARTESIAN_POINT('Ctrl Pts',(-3.82260844600006,5.2,-2.58141417600001));
#318209=CARTESIAN_POINT('Ctrl Pts',(-3.82260844600006,2.2,-2.58141417600001));
#318210=CARTESIAN_POINT('Ctrl Pts',(-3.82017042300006,12.2,-2.58124204700001));
#318211=CARTESIAN_POINT('Ctrl Pts',(-3.82017042300006,5.2,-2.58124204700001));
#318212=CARTESIAN_POINT('Ctrl Pts',(-3.82017042300006,2.2,-2.58124204700001));
#318213=CARTESIAN_POINT('Ctrl Pts',(-3.81773616400006,12.2,-2.58106759100002));
#318214=CARTESIAN_POINT('Ctrl Pts',(-3.81773616400006,5.2,-2.58106759100002));
#318215=CARTESIAN_POINT('Ctrl Pts',(-3.81773616400006,2.2,-2.58106759100002));
#318216=CARTESIAN_POINT('Ctrl Pts',(-3.81530567700006,12.2,-2.58089081300001));
#318217=CARTESIAN_POINT('Ctrl Pts',(-3.81530567700006,5.2,-2.58089081300001));
#318218=CARTESIAN_POINT('Ctrl Pts',(-3.81530567700006,2.2,-2.58089081300001));
#318219=CARTESIAN_POINT('Ctrl Pts',(-3.81287896500006,12.2,-2.58071172200002));
#318220=CARTESIAN_POINT('Ctrl Pts',(-3.81287896500006,5.2,-2.58071172200002));
#318221=CARTESIAN_POINT('Ctrl Pts',(-3.81287896500006,2.2,-2.58071172200002));
#318222=CARTESIAN_POINT('Ctrl Pts',(-3.81045603500006,12.2,-2.58053032400001));
#318223=CARTESIAN_POINT('Ctrl Pts',(-3.81045603500006,5.2,-2.58053032400001));
#318224=CARTESIAN_POINT('Ctrl Pts',(-3.81045603500006,2.2,-2.58053032400001));
#318225=CARTESIAN_POINT('Ctrl Pts',(-3.80803689300006,12.2,-2.58034662600001));
#318226=CARTESIAN_POINT('Ctrl Pts',(-3.80803689300006,5.2,-2.58034662600001));
#318227=CARTESIAN_POINT('Ctrl Pts',(-3.80803689300006,2.2,-2.58034662600001));
#318228=CARTESIAN_POINT('Ctrl Pts',(-3.80562154500006,12.2,-2.58016063700001));
#318229=CARTESIAN_POINT('Ctrl Pts',(-3.80562154500006,5.2,-2.58016063700001));
#318230=CARTESIAN_POINT('Ctrl Pts',(-3.80562154500006,2.2,-2.58016063700001));
#318231=CARTESIAN_POINT('Ctrl Pts',(-3.80320999800006,12.2,-2.57997236200001));
#318232=CARTESIAN_POINT('Ctrl Pts',(-3.80320999800006,5.2,-2.57997236200001));
#318233=CARTESIAN_POINT('Ctrl Pts',(-3.80320999800006,2.2,-2.57997236200001));
#318234=CARTESIAN_POINT('Ctrl Pts',(-3.80080225500006,12.2,-2.57978180800002));
#318235=CARTESIAN_POINT('Ctrl Pts',(-3.80080225500006,5.2,-2.57978180800002));
#318236=CARTESIAN_POINT('Ctrl Pts',(-3.80080225500006,2.2,-2.57978180800002));
#318237=CARTESIAN_POINT('Ctrl Pts',(-3.79839832500006,12.2,-2.57958898500001));
#318238=CARTESIAN_POINT('Ctrl Pts',(-3.79839832500006,5.2,-2.57958898500001));
#318239=CARTESIAN_POINT('Ctrl Pts',(-3.79839832500006,2.2,-2.57958898500001));
#318240=CARTESIAN_POINT('Ctrl Pts',(-3.79599821200006,12.2,-2.57939389800002));
#318241=CARTESIAN_POINT('Ctrl Pts',(-3.79599821200006,5.2,-2.57939389800002));
#318242=CARTESIAN_POINT('Ctrl Pts',(-3.79599821200006,2.2,-2.57939389800002));
#318243=CARTESIAN_POINT('Ctrl Pts',(-3.79360192100005,12.2,-2.57919655500002));
#318244=CARTESIAN_POINT('Ctrl Pts',(-3.79360192100005,5.2,-2.57919655500002));
#318245=CARTESIAN_POINT('Ctrl Pts',(-3.79360192100005,2.2,-2.57919655500002));
#318246=CARTESIAN_POINT('Ctrl Pts',(-3.79120946100006,12.2,-2.57899696300001));
#318247=CARTESIAN_POINT('Ctrl Pts',(-3.79120946100006,5.2,-2.57899696300001));
#318248=CARTESIAN_POINT('Ctrl Pts',(-3.79120946100006,2.2,-2.57899696300001));
#318249=CARTESIAN_POINT('Ctrl Pts',(-3.78882083600006,12.2,-2.57879512800002));
#318250=CARTESIAN_POINT('Ctrl Pts',(-3.78882083600006,5.2,-2.57879512800002));
#318251=CARTESIAN_POINT('Ctrl Pts',(-3.78882083600006,2.2,-2.57879512800002));
#318252=CARTESIAN_POINT('Ctrl Pts',(-3.78643605100006,12.2,-2.57859106000002));
#318253=CARTESIAN_POINT('Ctrl Pts',(-3.78643605100006,5.2,-2.57859106000002));
#318254=CARTESIAN_POINT('Ctrl Pts',(-3.78643605100006,2.2,-2.57859106000002));
#318255=CARTESIAN_POINT('Ctrl Pts',(-3.78405511300006,12.2,-2.57838476500002));
#318256=CARTESIAN_POINT('Ctrl Pts',(-3.78405511300006,5.2,-2.57838476500002));
#318257=CARTESIAN_POINT('Ctrl Pts',(-3.78405511300006,2.2,-2.57838476500002));
#318258=CARTESIAN_POINT('Ctrl Pts',(-3.78167802700006,12.2,-2.57817625000001));
#318259=CARTESIAN_POINT('Ctrl Pts',(-3.78167802700006,5.2,-2.57817625000001));
#318260=CARTESIAN_POINT('Ctrl Pts',(-3.78167802700006,2.2,-2.57817625000001));
#318261=CARTESIAN_POINT('Ctrl Pts',(-3.77930480100006,12.2,-2.57796552400002));
#318262=CARTESIAN_POINT('Ctrl Pts',(-3.77930480100006,5.2,-2.57796552400002));
#318263=CARTESIAN_POINT('Ctrl Pts',(-3.77930480100006,2.2,-2.57796552400002));
#318264=CARTESIAN_POINT('Ctrl Pts',(-3.77693543800006,12.2,-2.57775259100002));
#318265=CARTESIAN_POINT('Ctrl Pts',(-3.77693543800006,5.2,-2.57775259100002));
#318266=CARTESIAN_POINT('Ctrl Pts',(-3.77693543800006,2.2,-2.57775259100002));
#318267=CARTESIAN_POINT('Ctrl Pts',(-3.77456994600006,12.2,-2.57753746300001));
#318268=CARTESIAN_POINT('Ctrl Pts',(-3.77456994600006,5.2,-2.57753746300001));
#318269=CARTESIAN_POINT('Ctrl Pts',(-3.77456994600006,2.2,-2.57753746300001));
#318270=CARTESIAN_POINT('Ctrl Pts',(-3.77220833000006,12.2,-2.57732014200001));
#318271=CARTESIAN_POINT('Ctrl Pts',(-3.77220833000006,5.2,-2.57732014200001));
#318272=CARTESIAN_POINT('Ctrl Pts',(-3.77220833000006,2.2,-2.57732014200001));
#318273=CARTESIAN_POINT('Ctrl Pts',(-3.76985059500006,12.2,-2.57710064000001));
#318274=CARTESIAN_POINT('Ctrl Pts',(-3.76985059500006,5.2,-2.57710064000001));
#318275=CARTESIAN_POINT('Ctrl Pts',(-3.76985059500006,2.2,-2.57710064000001));
#318276=CARTESIAN_POINT('Ctrl Pts',(-3.76749674800006,12.2,-2.57687896300002));
#318277=CARTESIAN_POINT('Ctrl Pts',(-3.76749674800006,5.2,-2.57687896300002));
#318278=CARTESIAN_POINT('Ctrl Pts',(-3.76749674800006,2.2,-2.57687896300002));
#318279=CARTESIAN_POINT('Ctrl Pts',(-3.76514679500006,12.2,-2.57665511800001));
#318280=CARTESIAN_POINT('Ctrl Pts',(-3.76514679500006,5.2,-2.57665511800001));
#318281=CARTESIAN_POINT('Ctrl Pts',(-3.76514679500006,2.2,-2.57665511800001));
#318282=CARTESIAN_POINT('Ctrl Pts',(-3.76280074100006,12.2,-2.57642911300001));
#318283=CARTESIAN_POINT('Ctrl Pts',(-3.76280074100006,5.2,-2.57642911300001));
#318284=CARTESIAN_POINT('Ctrl Pts',(-3.76280074100006,2.2,-2.57642911300001));
#318285=CARTESIAN_POINT('Ctrl Pts',(-3.76045859300006,12.2,-2.57620095400001));
#318286=CARTESIAN_POINT('Ctrl Pts',(-3.76045859300006,5.2,-2.57620095400001));
#318287=CARTESIAN_POINT('Ctrl Pts',(-3.76045859300006,2.2,-2.57620095400001));
#318288=CARTESIAN_POINT('Ctrl Pts',(-3.75812035500006,12.2,-2.57597065100001));
#318289=CARTESIAN_POINT('Ctrl Pts',(-3.75812035500006,5.2,-2.57597065100001));
#318290=CARTESIAN_POINT('Ctrl Pts',(-3.75812035500006,2.2,-2.57597065100001));
#318291=CARTESIAN_POINT('Ctrl Pts',(-3.75578603400006,12.2,-2.57573821000001));
#318292=CARTESIAN_POINT('Ctrl Pts',(-3.75578603400006,5.2,-2.57573821000001));
#318293=CARTESIAN_POINT('Ctrl Pts',(-3.75578603400006,2.2,-2.57573821000001));
#318294=CARTESIAN_POINT('Ctrl Pts',(-3.75345563600006,12.2,-2.57550363900001));
#318295=CARTESIAN_POINT('Ctrl Pts',(-3.75345563600006,5.2,-2.57550363900001));
#318296=CARTESIAN_POINT('Ctrl Pts',(-3.75345563600006,2.2,-2.57550363900001));
#318297=CARTESIAN_POINT('Ctrl Pts',(-3.75112916600005,12.2,-2.57526694600001));
#318298=CARTESIAN_POINT('Ctrl Pts',(-3.75112916600005,5.2,-2.57526694600001));
#318299=CARTESIAN_POINT('Ctrl Pts',(-3.75112916600005,2.2,-2.57526694600001));
#318300=CARTESIAN_POINT('Ctrl Pts',(-3.74880663200006,12.2,-2.57502813700001));
#318301=CARTESIAN_POINT('Ctrl Pts',(-3.74880663200006,5.2,-2.57502813700001));
#318302=CARTESIAN_POINT('Ctrl Pts',(-3.74880663200006,2.2,-2.57502813700001));
#318303=CARTESIAN_POINT('Ctrl Pts',(-3.74648803600006,12.2,-2.57478722100001));
#318304=CARTESIAN_POINT('Ctrl Pts',(-3.74648803600006,5.2,-2.57478722100001));
#318305=CARTESIAN_POINT('Ctrl Pts',(-3.74648803600006,2.2,-2.57478722100001));
#318306=CARTESIAN_POINT('Ctrl Pts',(-3.74417338800006,12.2,-2.57454420600002));
#318307=CARTESIAN_POINT('Ctrl Pts',(-3.74417338800006,5.2,-2.57454420600002));
#318308=CARTESIAN_POINT('Ctrl Pts',(-3.74417338800006,2.2,-2.57454420600002));
#318309=CARTESIAN_POINT('Ctrl Pts',(-3.74186269100006,12.2,-2.57429909800001));
#318310=CARTESIAN_POINT('Ctrl Pts',(-3.74186269100006,5.2,-2.57429909800001));
#318311=CARTESIAN_POINT('Ctrl Pts',(-3.74186269100006,2.2,-2.57429909800001));
#318312=CARTESIAN_POINT('Ctrl Pts',(-3.73955595100006,12.2,-2.57405190600001));
#318313=CARTESIAN_POINT('Ctrl Pts',(-3.73955595100006,5.2,-2.57405190600001));
#318314=CARTESIAN_POINT('Ctrl Pts',(-3.73955595100006,2.2,-2.57405190600001));
#318315=CARTESIAN_POINT('Ctrl Pts',(-3.73725317500006,12.2,-2.57380263800002));
#318316=CARTESIAN_POINT('Ctrl Pts',(-3.73725317500006,5.2,-2.57380263800002));
#318317=CARTESIAN_POINT('Ctrl Pts',(-3.73725317500006,2.2,-2.57380263800002));
#318318=CARTESIAN_POINT('Ctrl Pts',(-3.73495436900006,12.2,-2.57355130100001));
#318319=CARTESIAN_POINT('Ctrl Pts',(-3.73495436900006,5.2,-2.57355130100001));
#318320=CARTESIAN_POINT('Ctrl Pts',(-3.73495436900006,2.2,-2.57355130100001));
#318321=CARTESIAN_POINT('Ctrl Pts',(-3.73265953700006,12.2,-2.57329790300002));
#318322=CARTESIAN_POINT('Ctrl Pts',(-3.73265953700006,5.2,-2.57329790300002));
#318323=CARTESIAN_POINT('Ctrl Pts',(-3.73265953700006,2.2,-2.57329790300002));
#318324=CARTESIAN_POINT('Ctrl Pts',(-3.73036868600006,12.2,-2.57304245100002));
#318325=CARTESIAN_POINT('Ctrl Pts',(-3.73036868600006,5.2,-2.57304245100002));
#318326=CARTESIAN_POINT('Ctrl Pts',(-3.73036868600006,2.2,-2.57304245100002));
#318327=CARTESIAN_POINT('Ctrl Pts',(-3.72808182200006,12.2,-2.57278495300001));
#318328=CARTESIAN_POINT('Ctrl Pts',(-3.72808182200006,5.2,-2.57278495300001));
#318329=CARTESIAN_POINT('Ctrl Pts',(-3.72808182200006,2.2,-2.57278495300001));
#318330=CARTESIAN_POINT('Ctrl Pts',(-3.72579894900006,12.2,-2.57252541700002));
#318331=CARTESIAN_POINT('Ctrl Pts',(-3.72579894900006,5.2,-2.57252541700002));
#318332=CARTESIAN_POINT('Ctrl Pts',(-3.72579894900006,2.2,-2.57252541700002));
#318333=CARTESIAN_POINT('Ctrl Pts',(-3.72352007600006,12.2,-2.57226385100001));
#318334=CARTESIAN_POINT('Ctrl Pts',(-3.72352007600006,5.2,-2.57226385100001));
#318335=CARTESIAN_POINT('Ctrl Pts',(-3.72352007600006,2.2,-2.57226385100001));
#318336=CARTESIAN_POINT('Ctrl Pts',(-3.72124520700006,12.2,-2.57200026400001));
#318337=CARTESIAN_POINT('Ctrl Pts',(-3.72124520700006,5.2,-2.57200026400001));
#318338=CARTESIAN_POINT('Ctrl Pts',(-3.72124520700006,2.2,-2.57200026400001));
#318339=CARTESIAN_POINT('Ctrl Pts',(-3.71897434700006,12.2,-2.57173466100001));
#318340=CARTESIAN_POINT('Ctrl Pts',(-3.71897434700006,5.2,-2.57173466100001));
#318341=CARTESIAN_POINT('Ctrl Pts',(-3.71897434700006,2.2,-2.57173466100001));
#318342=CARTESIAN_POINT('Ctrl Pts',(-3.71670750300006,12.2,-2.57146705200002));
#318343=CARTESIAN_POINT('Ctrl Pts',(-3.71670750300006,5.2,-2.57146705200002));
#318344=CARTESIAN_POINT('Ctrl Pts',(-3.71670750300006,2.2,-2.57146705200002));
#318345=CARTESIAN_POINT('Ctrl Pts',(-3.71444468100006,12.2,-2.57119744400002));
#318346=CARTESIAN_POINT('Ctrl Pts',(-3.71444468100006,5.2,-2.57119744400002));
#318347=CARTESIAN_POINT('Ctrl Pts',(-3.71444468100006,2.2,-2.57119744400002));
#318348=CARTESIAN_POINT('Ctrl Pts',(-3.71218588500006,12.2,-2.57092584600001));
#318349=CARTESIAN_POINT('Ctrl Pts',(-3.71218588500006,5.2,-2.57092584600001));
#318350=CARTESIAN_POINT('Ctrl Pts',(-3.71218588500006,2.2,-2.57092584600001));
#318351=CARTESIAN_POINT('Ctrl Pts',(-3.70993112200006,12.2,-2.57065226500002));
#318352=CARTESIAN_POINT('Ctrl Pts',(-3.70993112200006,5.2,-2.57065226500002));
#318353=CARTESIAN_POINT('Ctrl Pts',(-3.70993112200006,2.2,-2.57065226500002));
#318354=CARTESIAN_POINT('Ctrl Pts',(-3.70768039800006,12.2,-2.57037670700001));
#318355=CARTESIAN_POINT('Ctrl Pts',(-3.70768039800006,5.2,-2.57037670700001));
#318356=CARTESIAN_POINT('Ctrl Pts',(-3.70768039800006,2.2,-2.57037670700001));
#318357=CARTESIAN_POINT('Ctrl Pts',(-3.70543371900006,12.2,-2.57009918400001));
#318358=CARTESIAN_POINT('Ctrl Pts',(-3.70543371900006,5.2,-2.57009918400001));
#318359=CARTESIAN_POINT('Ctrl Pts',(-3.70543371900006,2.2,-2.57009918400001));
#318360=CARTESIAN_POINT('Ctrl Pts',(-3.70319109000006,12.2,-2.56981970100002));
#318361=CARTESIAN_POINT('Ctrl Pts',(-3.70319109000006,5.2,-2.56981970100002));
#318362=CARTESIAN_POINT('Ctrl Pts',(-3.70319109000006,2.2,-2.56981970100002));
#318363=CARTESIAN_POINT('Ctrl Pts',(-3.70095251600006,12.2,-2.56953826700002));
#318364=CARTESIAN_POINT('Ctrl Pts',(-3.70095251600006,5.2,-2.56953826700002));
#318365=CARTESIAN_POINT('Ctrl Pts',(-3.70095251600006,2.2,-2.56953826700002));
#318366=CARTESIAN_POINT('Ctrl Pts',(-3.69871800500006,12.2,-2.56925489100002));
#318367=CARTESIAN_POINT('Ctrl Pts',(-3.69871800500006,5.2,-2.56925489100002));
#318368=CARTESIAN_POINT('Ctrl Pts',(-3.69871800500006,2.2,-2.56925489100002));
#318369=CARTESIAN_POINT('Ctrl Pts',(-3.69648756100006,12.2,-2.56896958000001));
#318370=CARTESIAN_POINT('Ctrl Pts',(-3.69648756100006,5.2,-2.56896958000001));
#318371=CARTESIAN_POINT('Ctrl Pts',(-3.69648756100006,2.2,-2.56896958000001));
#318372=CARTESIAN_POINT('Ctrl Pts',(-3.69426119100006,12.2,-2.56868234100001));
#318373=CARTESIAN_POINT('Ctrl Pts',(-3.69426119100006,5.2,-2.56868234100001));
#318374=CARTESIAN_POINT('Ctrl Pts',(-3.69426119100006,2.2,-2.56868234100001));
#318375=CARTESIAN_POINT('Ctrl Pts',(-3.69203889900006,12.2,-2.56839318400001));
#318376=CARTESIAN_POINT('Ctrl Pts',(-3.69203889900006,5.2,-2.56839318400001));
#318377=CARTESIAN_POINT('Ctrl Pts',(-3.69203889900006,2.2,-2.56839318400001));
#318378=CARTESIAN_POINT('Ctrl Pts',(-3.68982069300006,12.2,-2.56810211500001));
#318379=CARTESIAN_POINT('Ctrl Pts',(-3.68982069300006,5.2,-2.56810211500001));
#318380=CARTESIAN_POINT('Ctrl Pts',(-3.68982069300006,2.2,-2.56810211500001));
#318381=CARTESIAN_POINT('Ctrl Pts',(-3.68760657700006,12.2,-2.56780914400002));
#318382=CARTESIAN_POINT('Ctrl Pts',(-3.68760657700006,5.2,-2.56780914400002));
#318383=CARTESIAN_POINT('Ctrl Pts',(-3.68760657700006,2.2,-2.56780914400002));
#318384=CARTESIAN_POINT('Ctrl Pts',(-3.68539655700006,12.2,-2.56751427900001));
#318385=CARTESIAN_POINT('Ctrl Pts',(-3.68539655700006,5.2,-2.56751427900001));
#318386=CARTESIAN_POINT('Ctrl Pts',(-3.68539655700006,2.2,-2.56751427900001));
#318387=CARTESIAN_POINT('Ctrl Pts',(-3.68319064000006,12.2,-2.56721752600002));
#318388=CARTESIAN_POINT('Ctrl Pts',(-3.68319064000006,5.2,-2.56721752600002));
#318389=CARTESIAN_POINT('Ctrl Pts',(-3.68319064000006,2.2,-2.56721752600002));
#318390=CARTESIAN_POINT('Ctrl Pts',(-3.68098883000005,12.2,-2.56691889600001));
#318391=CARTESIAN_POINT('Ctrl Pts',(-3.68098883000005,5.2,-2.56691889600001));
#318392=CARTESIAN_POINT('Ctrl Pts',(-3.68098883000005,2.2,-2.56691889600001));
#318393=CARTESIAN_POINT('Ctrl Pts',(-3.67879113400006,12.2,-2.56661839500001));
#318394=CARTESIAN_POINT('Ctrl Pts',(-3.67879113400006,5.2,-2.56661839500001));
#318395=CARTESIAN_POINT('Ctrl Pts',(-3.67879113400006,2.2,-2.56661839500001));
#318396=CARTESIAN_POINT('Ctrl Pts',(-3.67659755700006,12.2,-2.56631603300002));
#318397=CARTESIAN_POINT('Ctrl Pts',(-3.67659755700006,5.2,-2.56631603300002));
#318398=CARTESIAN_POINT('Ctrl Pts',(-3.67659755700006,2.2,-2.56631603300002));
#318399=CARTESIAN_POINT('Ctrl Pts',(-3.67440810500006,12.2,-2.56601181700002));
#318400=CARTESIAN_POINT('Ctrl Pts',(-3.67440810500006,5.2,-2.56601181700002));
#318401=CARTESIAN_POINT('Ctrl Pts',(-3.67440810500006,2.2,-2.56601181700002));
#318402=CARTESIAN_POINT('Ctrl Pts',(-3.67222278300006,12.2,-2.56570575600001));
#318403=CARTESIAN_POINT('Ctrl Pts',(-3.67222278300006,5.2,-2.56570575600001));
#318404=CARTESIAN_POINT('Ctrl Pts',(-3.67222278300006,2.2,-2.56570575600001));
#318405=CARTESIAN_POINT('Ctrl Pts',(-3.67004159800006,12.2,-2.56539785700001));
#318406=CARTESIAN_POINT('Ctrl Pts',(-3.67004159800006,5.2,-2.56539785700001));
#318407=CARTESIAN_POINT('Ctrl Pts',(-3.67004159800006,2.2,-2.56539785700001));
#318408=CARTESIAN_POINT('Ctrl Pts',(-3.66786455500006,12.2,-2.56508813000002));
#318409=CARTESIAN_POINT('Ctrl Pts',(-3.66786455500006,5.2,-2.56508813000002));
#318410=CARTESIAN_POINT('Ctrl Pts',(-3.66786455500006,2.2,-2.56508813000002));
#318411=CARTESIAN_POINT('Ctrl Pts',(-3.66569166000006,12.2,-2.56477658100001));
#318412=CARTESIAN_POINT('Ctrl Pts',(-3.66569166000006,5.2,-2.56477658100001));
#318413=CARTESIAN_POINT('Ctrl Pts',(-3.66569166000006,2.2,-2.56477658100001));
#318414=CARTESIAN_POINT('Ctrl Pts',(-3.66352291900006,12.2,-2.56446322200001));
#318415=CARTESIAN_POINT('Ctrl Pts',(-3.66352291900006,5.2,-2.56446322200001));
#318416=CARTESIAN_POINT('Ctrl Pts',(-3.66352291900006,2.2,-2.56446322200001));
#318417=CARTESIAN_POINT('Ctrl Pts',(-3.66135833700006,12.2,-2.56414805700001));
#318418=CARTESIAN_POINT('Ctrl Pts',(-3.66135833700006,5.2,-2.56414805700001));
#318419=CARTESIAN_POINT('Ctrl Pts',(-3.66135833700006,2.2,-2.56414805700001));
#318420=CARTESIAN_POINT('Ctrl Pts',(-3.65919792000006,12.2,-2.56383109800002));
#318421=CARTESIAN_POINT('Ctrl Pts',(-3.65919792000006,5.2,-2.56383109800002));
#318422=CARTESIAN_POINT('Ctrl Pts',(-3.65919792000006,2.2,-2.56383109800002));
#318423=CARTESIAN_POINT('Ctrl Pts',(-3.65704167500006,12.2,-2.56351235100002));
#318424=CARTESIAN_POINT('Ctrl Pts',(-3.65704167500006,5.2,-2.56351235100002));
#318425=CARTESIAN_POINT('Ctrl Pts',(-3.65704167500006,2.2,-2.56351235100002));
#318426=CARTESIAN_POINT('Ctrl Pts',(-3.65488960400006,12.2,-2.56319182500001));
#318427=CARTESIAN_POINT('Ctrl Pts',(-3.65488960400006,5.2,-2.56319182500001));
#318428=CARTESIAN_POINT('Ctrl Pts',(-3.65488960400006,2.2,-2.56319182500001));
#318429=CARTESIAN_POINT('Ctrl Pts',(-3.65274171600006,12.2,-2.56286952900001));
#318430=CARTESIAN_POINT('Ctrl Pts',(-3.65274171600006,5.2,-2.56286952900001));
#318431=CARTESIAN_POINT('Ctrl Pts',(-3.65274171600006,2.2,-2.56286952900001));
#318432=CARTESIAN_POINT('Ctrl Pts',(-3.65059801700006,12.2,-2.56254547100002));
#318433=CARTESIAN_POINT('Ctrl Pts',(-3.65059801700006,5.2,-2.56254547100002));
#318434=CARTESIAN_POINT('Ctrl Pts',(-3.65059801700006,2.2,-2.56254547100002));
#318435=CARTESIAN_POINT('Ctrl Pts',(-3.64845851100006,12.2,-2.56221966000002));
#318436=CARTESIAN_POINT('Ctrl Pts',(-3.64845851100006,5.2,-2.56221966000002));
#318437=CARTESIAN_POINT('Ctrl Pts',(-3.64845851100006,2.2,-2.56221966000002));
#318438=CARTESIAN_POINT('Ctrl Pts',(-3.64632320400006,12.2,-2.56189210400001));
#318439=CARTESIAN_POINT('Ctrl Pts',(-3.64632320400006,5.2,-2.56189210400001));
#318440=CARTESIAN_POINT('Ctrl Pts',(-3.64632320400006,2.2,-2.56189210400001));
#318441=CARTESIAN_POINT('Ctrl Pts',(-3.64419210100006,12.2,-2.56156281100001));
#318442=CARTESIAN_POINT('Ctrl Pts',(-3.64419210100006,5.2,-2.56156281100001));
#318443=CARTESIAN_POINT('Ctrl Pts',(-3.64419210100006,2.2,-2.56156281100001));
#318444=CARTESIAN_POINT('Ctrl Pts',(-3.64206521000006,12.2,-2.56123179000001));
#318445=CARTESIAN_POINT('Ctrl Pts',(-3.64206521000006,5.2,-2.56123179000001));
#318446=CARTESIAN_POINT('Ctrl Pts',(-3.64206521000006,2.2,-2.56123179000001));
#318447=CARTESIAN_POINT('Ctrl Pts',(-3.63994253400006,12.2,-2.56089905100001));
#318448=CARTESIAN_POINT('Ctrl Pts',(-3.63994253400006,5.2,-2.56089905100001));
#318449=CARTESIAN_POINT('Ctrl Pts',(-3.63994253400006,2.2,-2.56089905100001));
#318450=CARTESIAN_POINT('Ctrl Pts',(-3.63782408100006,12.2,-2.56056460000002));
#318451=CARTESIAN_POINT('Ctrl Pts',(-3.63782408100006,5.2,-2.56056460000002));
#318452=CARTESIAN_POINT('Ctrl Pts',(-3.63782408100006,2.2,-2.56056460000002));
#318453=CARTESIAN_POINT('Ctrl Pts',(-3.63570985500006,12.2,-2.56022844700002));
#318454=CARTESIAN_POINT('Ctrl Pts',(-3.63570985500006,5.2,-2.56022844700002));
#318455=CARTESIAN_POINT('Ctrl Pts',(-3.63570985500006,2.2,-2.56022844700002));
#318456=CARTESIAN_POINT('Ctrl Pts',(-3.63359986300006,12.2,-2.55989060100001));
#318457=CARTESIAN_POINT('Ctrl Pts',(-3.63359986300006,5.2,-2.55989060100001));
#318458=CARTESIAN_POINT('Ctrl Pts',(-3.63359986300006,2.2,-2.55989060100001));
#318459=CARTESIAN_POINT('Ctrl Pts',(-3.63149410900006,12.2,-2.55955106900001));
#318460=CARTESIAN_POINT('Ctrl Pts',(-3.63149410900006,5.2,-2.55955106900001));
#318461=CARTESIAN_POINT('Ctrl Pts',(-3.63149410900006,2.2,-2.55955106900001));
#318462=CARTESIAN_POINT('Ctrl Pts',(-3.62939259900006,12.2,-2.55920986100001));
#318463=CARTESIAN_POINT('Ctrl Pts',(-3.62939259900006,5.2,-2.55920986100001));
#318464=CARTESIAN_POINT('Ctrl Pts',(-3.62939259900006,2.2,-2.55920986100001));
#318465=CARTESIAN_POINT('Ctrl Pts',(-3.62729534200006,12.2,-2.55886698600001));
#318466=CARTESIAN_POINT('Ctrl Pts',(-3.62729534200006,5.2,-2.55886698600001));
#318467=CARTESIAN_POINT('Ctrl Pts',(-3.62729534200006,2.2,-2.55886698600001));
#318468=CARTESIAN_POINT('Ctrl Pts',(-3.62520233900006,12.2,-2.55852245200002));
#318469=CARTESIAN_POINT('Ctrl Pts',(-3.62520233900006,5.2,-2.55852245200002));
#318470=CARTESIAN_POINT('Ctrl Pts',(-3.62520233900006,2.2,-2.55852245200002));
#318471=CARTESIAN_POINT('Ctrl Pts',(-3.62311359700006,12.2,-2.55817626700001));
#318472=CARTESIAN_POINT('Ctrl Pts',(-3.62311359700006,5.2,-2.55817626700001));
#318473=CARTESIAN_POINT('Ctrl Pts',(-3.62311359700006,2.2,-2.55817626700001));
#318474=CARTESIAN_POINT('Ctrl Pts',(-3.62102912300006,12.2,-2.55782844000001));
#318475=CARTESIAN_POINT('Ctrl Pts',(-3.62102912300006,5.2,-2.55782844000001));
#318476=CARTESIAN_POINT('Ctrl Pts',(-3.62102912300006,2.2,-2.55782844000001));
#318477=CARTESIAN_POINT('Ctrl Pts',(-3.61894892200006,12.2,-2.55747898100001));
#318478=CARTESIAN_POINT('Ctrl Pts',(-3.61894892200006,5.2,-2.55747898100001));
#318479=CARTESIAN_POINT('Ctrl Pts',(-3.61894892200006,2.2,-2.55747898100001));
#318480=CARTESIAN_POINT('Ctrl Pts',(-3.61687299900006,12.2,-2.55712789800001));
#318481=CARTESIAN_POINT('Ctrl Pts',(-3.61687299900006,5.2,-2.55712789800001));
#318482=CARTESIAN_POINT('Ctrl Pts',(-3.61687299900006,2.2,-2.55712789800001));
#318483=CARTESIAN_POINT('Ctrl Pts',(-3.61480136100006,12.2,-2.55677520000001));
#318484=CARTESIAN_POINT('Ctrl Pts',(-3.61480136100006,5.2,-2.55677520000001));
#318485=CARTESIAN_POINT('Ctrl Pts',(-3.61480136100006,2.2,-2.55677520000001));
#318486=CARTESIAN_POINT('Ctrl Pts',(-3.61273401200005,12.2,-2.55642089500002));
#318487=CARTESIAN_POINT('Ctrl Pts',(-3.61273401200005,5.2,-2.55642089500002));
#318488=CARTESIAN_POINT('Ctrl Pts',(-3.61273401200005,2.2,-2.55642089500002));
#318489=CARTESIAN_POINT('Ctrl Pts',(-3.61067095900006,12.2,-2.55606499200002));
#318490=CARTESIAN_POINT('Ctrl Pts',(-3.61067095900006,5.2,-2.55606499200002));
#318491=CARTESIAN_POINT('Ctrl Pts',(-3.61067095900006,2.2,-2.55606499200002));
#318492=CARTESIAN_POINT('Ctrl Pts',(-3.60861220700006,12.2,-2.55570750100001));
#318493=CARTESIAN_POINT('Ctrl Pts',(-3.60861220700006,5.2,-2.55570750100001));
#318494=CARTESIAN_POINT('Ctrl Pts',(-3.60861220700006,2.2,-2.55570750100001));
#318495=CARTESIAN_POINT('Ctrl Pts',(-3.60655776100006,12.2,-2.55534843100001));
#318496=CARTESIAN_POINT('Ctrl Pts',(-3.60655776100006,5.2,-2.55534843100001));
#318497=CARTESIAN_POINT('Ctrl Pts',(-3.60655776100006,2.2,-2.55534843100001));
#318498=CARTESIAN_POINT('Ctrl Pts',(-3.60450762800006,12.2,-2.55498778800002));
#318499=CARTESIAN_POINT('Ctrl Pts',(-3.60450762800006,5.2,-2.55498778800002));
#318500=CARTESIAN_POINT('Ctrl Pts',(-3.60450762800006,2.2,-2.55498778800002));
#318501=CARTESIAN_POINT('Ctrl Pts',(-3.60246181300006,12.2,-2.55462558500001));
#318502=CARTESIAN_POINT('Ctrl Pts',(-3.60246181300006,5.2,-2.55462558500001));
#318503=CARTESIAN_POINT('Ctrl Pts',(-3.60246181300006,2.2,-2.55462558500001));
#318504=CARTESIAN_POINT('Ctrl Pts',(-3.60042032100006,12.2,-2.55426182800001));
#318505=CARTESIAN_POINT('Ctrl Pts',(-3.60042032100006,5.2,-2.55426182800001));
#318506=CARTESIAN_POINT('Ctrl Pts',(-3.60042032100006,2.2,-2.55426182800001));
#318507=CARTESIAN_POINT('Ctrl Pts',(-3.59838315900006,12.2,-2.55389652700002));
#318508=CARTESIAN_POINT('Ctrl Pts',(-3.59838315900006,5.2,-2.55389652700002));
#318509=CARTESIAN_POINT('Ctrl Pts',(-3.59838315900006,2.2,-2.55389652700002));
#318510=CARTESIAN_POINT('Ctrl Pts',(-3.59635033100006,12.2,-2.55352969000001));
#318511=CARTESIAN_POINT('Ctrl Pts',(-3.59635033100006,5.2,-2.55352969000001));
#318512=CARTESIAN_POINT('Ctrl Pts',(-3.59635033100006,2.2,-2.55352969000001));
#318513=CARTESIAN_POINT('Ctrl Pts',(-3.59432184300006,12.2,-2.55316132800001));
#318514=CARTESIAN_POINT('Ctrl Pts',(-3.59432184300006,5.2,-2.55316132800001));
#318515=CARTESIAN_POINT('Ctrl Pts',(-3.59432184300006,2.2,-2.55316132800001));
#318516=CARTESIAN_POINT('Ctrl Pts',(-3.59229770100006,12.2,-2.55279144900001));
#318517=CARTESIAN_POINT('Ctrl Pts',(-3.59229770100006,5.2,-2.55279144900001));
#318518=CARTESIAN_POINT('Ctrl Pts',(-3.59229770100006,2.2,-2.55279144900001));
#318519=CARTESIAN_POINT('Ctrl Pts',(-3.59027791200006,12.2,-2.55242006200001));
#318520=CARTESIAN_POINT('Ctrl Pts',(-3.59027791200006,5.2,-2.55242006200001));
#318521=CARTESIAN_POINT('Ctrl Pts',(-3.59027791200006,2.2,-2.55242006200001));
#318522=CARTESIAN_POINT('Ctrl Pts',(-3.58826247900006,12.2,-2.55204717600002));
#318523=CARTESIAN_POINT('Ctrl Pts',(-3.58826247900006,5.2,-2.55204717600002));
#318524=CARTESIAN_POINT('Ctrl Pts',(-3.58826247900006,2.2,-2.55204717600002));
#318525=CARTESIAN_POINT('Ctrl Pts',(-3.58625140900006,12.2,-2.55167279900002));
#318526=CARTESIAN_POINT('Ctrl Pts',(-3.58625140900006,5.2,-2.55167279900002));
#318527=CARTESIAN_POINT('Ctrl Pts',(-3.58625140900006,2.2,-2.55167279900002));
#318528=CARTESIAN_POINT('Ctrl Pts',(-3.58424470700006,12.2,-2.55129694200001));
#318529=CARTESIAN_POINT('Ctrl Pts',(-3.58424470700006,5.2,-2.55129694200001));
#318530=CARTESIAN_POINT('Ctrl Pts',(-3.58424470700006,2.2,-2.55129694200001));
#318531=CARTESIAN_POINT('Ctrl Pts',(-3.58224237900005,12.2,-2.55091961300002));
#318532=CARTESIAN_POINT('Ctrl Pts',(-3.58224237900005,5.2,-2.55091961300002));
#318533=CARTESIAN_POINT('Ctrl Pts',(-3.58224237900005,2.2,-2.55091961300002));
#318534=CARTESIAN_POINT('Ctrl Pts',(-3.58024443100006,12.2,-2.55054082300001));
#318535=CARTESIAN_POINT('Ctrl Pts',(-3.58024443100006,5.2,-2.55054082300001));
#318536=CARTESIAN_POINT('Ctrl Pts',(-3.58024443100006,2.2,-2.55054082300001));
#318537=CARTESIAN_POINT('Ctrl Pts',(-3.57825086800006,12.2,-2.55016057800002));
#318538=CARTESIAN_POINT('Ctrl Pts',(-3.57825086800006,5.2,-2.55016057800002));
#318539=CARTESIAN_POINT('Ctrl Pts',(-3.57825086800006,2.2,-2.55016057800002));
#318540=CARTESIAN_POINT('Ctrl Pts',(-3.57626169500006,12.2,-2.54977888900001));
#318541=CARTESIAN_POINT('Ctrl Pts',(-3.57626169500006,5.2,-2.54977888900001));
#318542=CARTESIAN_POINT('Ctrl Pts',(-3.57626169500006,2.2,-2.54977888900001));
#318543=CARTESIAN_POINT('Ctrl Pts',(-3.57427691800006,12.2,-2.54939576600002));
#318544=CARTESIAN_POINT('Ctrl Pts',(-3.57427691800006,5.2,-2.54939576600002));
#318545=CARTESIAN_POINT('Ctrl Pts',(-3.57427691800006,2.2,-2.54939576600002));
#318546=CARTESIAN_POINT('Ctrl Pts',(-3.57229654300006,12.2,-2.54901121700001));
#318547=CARTESIAN_POINT('Ctrl Pts',(-3.57229654300006,5.2,-2.54901121700001));
#318548=CARTESIAN_POINT('Ctrl Pts',(-3.57229654300006,2.2,-2.54901121700001));
#318549=CARTESIAN_POINT('Ctrl Pts',(-3.57032057600006,12.2,-2.54862525200001));
#318550=CARTESIAN_POINT('Ctrl Pts',(-3.57032057600006,5.2,-2.54862525200001));
#318551=CARTESIAN_POINT('Ctrl Pts',(-3.57032057600006,2.2,-2.54862525200001));
#318552=CARTESIAN_POINT('Ctrl Pts',(-3.56834902100006,12.2,-2.54823787900001));
#318553=CARTESIAN_POINT('Ctrl Pts',(-3.56834902100006,5.2,-2.54823787900001));
#318554=CARTESIAN_POINT('Ctrl Pts',(-3.56834902100006,2.2,-2.54823787900001));
#318555=CARTESIAN_POINT('Ctrl Pts',(-3.56638188500006,12.2,-2.54784911000002));
#318556=CARTESIAN_POINT('Ctrl Pts',(-3.56638188500006,5.2,-2.54784911000002));
#318557=CARTESIAN_POINT('Ctrl Pts',(-3.56638188500006,2.2,-2.54784911000002));
#318558=CARTESIAN_POINT('Ctrl Pts',(-3.56441917200006,12.2,-2.54745895100001));
#318559=CARTESIAN_POINT('Ctrl Pts',(-3.56441917200006,5.2,-2.54745895100001));
#318560=CARTESIAN_POINT('Ctrl Pts',(-3.56441917200006,2.2,-2.54745895100001));
#318561=CARTESIAN_POINT('Ctrl Pts',(-3.56246089000006,12.2,-2.54706741300001));
#318562=CARTESIAN_POINT('Ctrl Pts',(-3.56246089000006,5.2,-2.54706741300001));
#318563=CARTESIAN_POINT('Ctrl Pts',(-3.56246089000006,2.2,-2.54706741300001));
#318564=CARTESIAN_POINT('Ctrl Pts',(-3.56050704200006,12.2,-2.54667450600001));
#318565=CARTESIAN_POINT('Ctrl Pts',(-3.56050704200006,5.2,-2.54667450600001));
#318566=CARTESIAN_POINT('Ctrl Pts',(-3.56050704200006,2.2,-2.54667450600001));
#318567=CARTESIAN_POINT('Ctrl Pts',(-3.55855763500006,12.2,-2.54628023900001));
#318568=CARTESIAN_POINT('Ctrl Pts',(-3.55855763500006,5.2,-2.54628023900001));
#318569=CARTESIAN_POINT('Ctrl Pts',(-3.55855763500006,2.2,-2.54628023900001));
#318570=CARTESIAN_POINT('Ctrl Pts',(-3.55661267300006,12.2,-2.54588462100001));
#318571=CARTESIAN_POINT('Ctrl Pts',(-3.55661267300006,5.2,-2.54588462100001));
#318572=CARTESIAN_POINT('Ctrl Pts',(-3.55661267300006,2.2,-2.54588462100001));
#318573=CARTESIAN_POINT('Ctrl Pts',(-3.55467216400006,12.2,-2.54548766100001));
#318574=CARTESIAN_POINT('Ctrl Pts',(-3.55467216400006,5.2,-2.54548766100001));
#318575=CARTESIAN_POINT('Ctrl Pts',(-3.55467216400006,2.2,-2.54548766100001));
#318576=CARTESIAN_POINT('Ctrl Pts',(-3.55273611200006,12.2,-2.54508937000002));
#318577=CARTESIAN_POINT('Ctrl Pts',(-3.55273611200006,5.2,-2.54508937000002));
#318578=CARTESIAN_POINT('Ctrl Pts',(-3.55273611200006,2.2,-2.54508937000002));
#318579=CARTESIAN_POINT('Ctrl Pts',(-3.55080452200006,12.2,-2.54468975600001));
#318580=CARTESIAN_POINT('Ctrl Pts',(-3.55080452200006,5.2,-2.54468975600001));
#318581=CARTESIAN_POINT('Ctrl Pts',(-3.55080452200006,2.2,-2.54468975600001));
#318582=CARTESIAN_POINT('Ctrl Pts',(-3.54887740000006,12.2,-2.54428882900001));
#318583=CARTESIAN_POINT('Ctrl Pts',(-3.54887740000006,5.2,-2.54428882900001));
#318584=CARTESIAN_POINT('Ctrl Pts',(-3.54887740000006,2.2,-2.54428882900001));
#318585=CARTESIAN_POINT('Ctrl Pts',(-3.54695475300006,12.2,-2.54388659900001));
#318586=CARTESIAN_POINT('Ctrl Pts',(-3.54695475300006,5.2,-2.54388659900001));
#318587=CARTESIAN_POINT('Ctrl Pts',(-3.54695475300006,2.2,-2.54388659900001));
#318588=CARTESIAN_POINT('Ctrl Pts',(-3.54503658400006,12.2,-2.54348307500001));
#318589=CARTESIAN_POINT('Ctrl Pts',(-3.54503658400006,5.2,-2.54348307500001));
#318590=CARTESIAN_POINT('Ctrl Pts',(-3.54503658400006,2.2,-2.54348307500001));
#318591=CARTESIAN_POINT('Ctrl Pts',(-3.54312290000006,12.2,-2.54307826700002));
#318592=CARTESIAN_POINT('Ctrl Pts',(-3.54312290000006,5.2,-2.54307826700002));
#318593=CARTESIAN_POINT('Ctrl Pts',(-3.54312290000006,2.2,-2.54307826700002));
#318594=CARTESIAN_POINT('Ctrl Pts',(-3.54121370600006,12.2,-2.54267218400001));
#318595=CARTESIAN_POINT('Ctrl Pts',(-3.54121370600006,5.2,-2.54267218400001));
#318596=CARTESIAN_POINT('Ctrl Pts',(-3.54121370600006,2.2,-2.54267218400001));
#318597=CARTESIAN_POINT('Ctrl Pts',(-3.53930900900005,12.2,-2.54226483700001));
#318598=CARTESIAN_POINT('Ctrl Pts',(-3.53930900900005,5.2,-2.54226483700001));
#318599=CARTESIAN_POINT('Ctrl Pts',(-3.53930900900005,2.2,-2.54226483700001));
#318600=CARTESIAN_POINT('Ctrl Pts',(-3.53740881100006,12.2,-2.54185623400002));
#318601=CARTESIAN_POINT('Ctrl Pts',(-3.53740881100006,5.2,-2.54185623400002));
#318602=CARTESIAN_POINT('Ctrl Pts',(-3.53740881100006,2.2,-2.54185623400002));
#318603=CARTESIAN_POINT('Ctrl Pts',(-3.53551312200006,12.2,-2.54144638500001));
#318604=CARTESIAN_POINT('Ctrl Pts',(-3.53551312200006,5.2,-2.54144638500001));
#318605=CARTESIAN_POINT('Ctrl Pts',(-3.53551312200006,2.2,-2.54144638500001));
#318606=CARTESIAN_POINT('Ctrl Pts',(-3.53362194400006,12.2,-2.54103530100001));
#318607=CARTESIAN_POINT('Ctrl Pts',(-3.53362194400006,5.2,-2.54103530100001));
#318608=CARTESIAN_POINT('Ctrl Pts',(-3.53362194400006,2.2,-2.54103530100001));
#318609=CARTESIAN_POINT('Ctrl Pts',(-3.53173528300006,12.2,-2.54062299000001));
#318610=CARTESIAN_POINT('Ctrl Pts',(-3.53173528300006,5.2,-2.54062299000001));
#318611=CARTESIAN_POINT('Ctrl Pts',(-3.53173528300006,2.2,-2.54062299000001));
#318612=CARTESIAN_POINT('Ctrl Pts',(-3.52985314600006,12.2,-2.54020946300002));
#318613=CARTESIAN_POINT('Ctrl Pts',(-3.52985314600006,5.2,-2.54020946300002));
#318614=CARTESIAN_POINT('Ctrl Pts',(-3.52985314600006,2.2,-2.54020946300002));
#318615=CARTESIAN_POINT('Ctrl Pts',(-3.52797553700006,12.2,-2.53979472900001));
#318616=CARTESIAN_POINT('Ctrl Pts',(-3.52797553700006,5.2,-2.53979472900001));
#318617=CARTESIAN_POINT('Ctrl Pts',(-3.52797553700006,2.2,-2.53979472900001));
#318618=CARTESIAN_POINT('Ctrl Pts',(-3.52610246200006,12.2,-2.53937879900001));
#318619=CARTESIAN_POINT('Ctrl Pts',(-3.52610246200006,5.2,-2.53937879900001));
#318620=CARTESIAN_POINT('Ctrl Pts',(-3.52610246200006,2.2,-2.53937879900001));
#318621=CARTESIAN_POINT('Ctrl Pts',(-3.52423392700006,12.2,-2.53896168100002));
#318622=CARTESIAN_POINT('Ctrl Pts',(-3.52423392700006,5.2,-2.53896168100002));
#318623=CARTESIAN_POINT('Ctrl Pts',(-3.52423392700006,2.2,-2.53896168100002));
#318624=CARTESIAN_POINT('Ctrl Pts',(-3.52236993700005,12.2,-2.53854338700001));
#318625=CARTESIAN_POINT('Ctrl Pts',(-3.52236993700005,5.2,-2.53854338700001));
#318626=CARTESIAN_POINT('Ctrl Pts',(-3.52236993700005,2.2,-2.53854338700001));
#318627=CARTESIAN_POINT('Ctrl Pts',(-3.52051049600006,12.2,-2.53812392400001));
#318628=CARTESIAN_POINT('Ctrl Pts',(-3.52051049600006,5.2,-2.53812392400001));
#318629=CARTESIAN_POINT('Ctrl Pts',(-3.52051049600006,2.2,-2.53812392400001));
#318630=CARTESIAN_POINT('Ctrl Pts',(-3.51865561200006,12.2,-2.53770330500001));
#318631=CARTESIAN_POINT('Ctrl Pts',(-3.51865561200006,5.2,-2.53770330500001));
#318632=CARTESIAN_POINT('Ctrl Pts',(-3.51865561200006,2.2,-2.53770330500001));
#318633=CARTESIAN_POINT('Ctrl Pts',(-3.51680529000006,12.2,-2.53728153800001));
#318634=CARTESIAN_POINT('Ctrl Pts',(-3.51680529000006,5.2,-2.53728153800001));
#318635=CARTESIAN_POINT('Ctrl Pts',(-3.51680529000006,2.2,-2.53728153800001));
#318636=CARTESIAN_POINT('Ctrl Pts',(-3.51495953300006,12.2,-2.53685863300001));
#318637=CARTESIAN_POINT('Ctrl Pts',(-3.51495953300006,5.2,-2.53685863300001));
#318638=CARTESIAN_POINT('Ctrl Pts',(-3.51495953300006,2.2,-2.53685863300001));
#318639=CARTESIAN_POINT('Ctrl Pts',(-3.51311835000006,12.2,-2.53643460000001));
#318640=CARTESIAN_POINT('Ctrl Pts',(-3.51311835000006,5.2,-2.53643460000001));
#318641=CARTESIAN_POINT('Ctrl Pts',(-3.51311835000006,2.2,-2.53643460000001));
#318642=CARTESIAN_POINT('Ctrl Pts',(-3.51128174300006,12.2,-2.53600945100001));
#318643=CARTESIAN_POINT('Ctrl Pts',(-3.51128174300006,5.2,-2.53600945100001));
#318644=CARTESIAN_POINT('Ctrl Pts',(-3.51128174300006,2.2,-2.53600945100001));
#318645=CARTESIAN_POINT('Ctrl Pts',(-3.50944972000006,12.2,-2.53558319400002));
#318646=CARTESIAN_POINT('Ctrl Pts',(-3.50944972000006,5.2,-2.53558319400002));
#318647=CARTESIAN_POINT('Ctrl Pts',(-3.50944972000006,2.2,-2.53558319400002));
#318648=CARTESIAN_POINT('Ctrl Pts',(-3.50762228500006,12.2,-2.53515583900001));
#318649=CARTESIAN_POINT('Ctrl Pts',(-3.50762228500006,5.2,-2.53515583900001));
#318650=CARTESIAN_POINT('Ctrl Pts',(-3.50762228500006,2.2,-2.53515583900001));
#318651=CARTESIAN_POINT('Ctrl Pts',(-3.50579944300006,12.2,-2.53472739600001));
#318652=CARTESIAN_POINT('Ctrl Pts',(-3.50579944300006,5.2,-2.53472739600001));
#318653=CARTESIAN_POINT('Ctrl Pts',(-3.50579944300006,2.2,-2.53472739600001));
#318654=CARTESIAN_POINT('Ctrl Pts',(-3.50398120200006,12.2,-2.53429787500002));
#318655=CARTESIAN_POINT('Ctrl Pts',(-3.50398120200006,5.2,-2.53429787500002));
#318656=CARTESIAN_POINT('Ctrl Pts',(-3.50398120200006,2.2,-2.53429787500002));
#318657=CARTESIAN_POINT('Ctrl Pts',(-3.50216756400005,12.2,-2.53386728800002));
#318658=CARTESIAN_POINT('Ctrl Pts',(-3.50216756400005,5.2,-2.53386728800002));
#318659=CARTESIAN_POINT('Ctrl Pts',(-3.50216756400005,2.2,-2.53386728800002));
#318660=CARTESIAN_POINT('Ctrl Pts',(-3.50035853800006,12.2,-2.53343564400001));
#318661=CARTESIAN_POINT('Ctrl Pts',(-3.50035853800006,5.2,-2.53343564400001));
#318662=CARTESIAN_POINT('Ctrl Pts',(-3.50035853800006,2.2,-2.53343564400001));
#318663=CARTESIAN_POINT('Ctrl Pts',(-3.49855412600005,12.2,-2.53300295300001));
#318664=CARTESIAN_POINT('Ctrl Pts',(-3.49855412600005,5.2,-2.53300295300001));
#318665=CARTESIAN_POINT('Ctrl Pts',(-3.49855412600005,2.2,-2.53300295300001));
#318666=CARTESIAN_POINT('Ctrl Pts',(-3.49675433400006,12.2,-2.53256922500002));
#318667=CARTESIAN_POINT('Ctrl Pts',(-3.49675433400006,5.2,-2.53256922500002));
#318668=CARTESIAN_POINT('Ctrl Pts',(-3.49675433400006,2.2,-2.53256922500002));
#318669=CARTESIAN_POINT('Ctrl Pts',(-3.49495917000006,12.2,-2.53213446900002));
#318670=CARTESIAN_POINT('Ctrl Pts',(-3.49495917000006,5.2,-2.53213446900002));
#318671=CARTESIAN_POINT('Ctrl Pts',(-3.49495917000006,2.2,-2.53213446900002));
#318672=CARTESIAN_POINT('Ctrl Pts',(-3.49316863700006,12.2,-2.53169869800002));
#318673=CARTESIAN_POINT('Ctrl Pts',(-3.49316863700006,5.2,-2.53169869800002));
#318674=CARTESIAN_POINT('Ctrl Pts',(-3.49316863700006,2.2,-2.53169869800002));
#318675=CARTESIAN_POINT('Ctrl Pts',(-3.49138274100006,12.2,-2.53126192100002));
#318676=CARTESIAN_POINT('Ctrl Pts',(-3.49138274100006,5.2,-2.53126192100002));
#318677=CARTESIAN_POINT('Ctrl Pts',(-3.49138274100006,2.2,-2.53126192100002));
#318678=CARTESIAN_POINT('Ctrl Pts',(-3.48960148600006,12.2,-2.53082414800001));
#318679=CARTESIAN_POINT('Ctrl Pts',(-3.48960148600006,5.2,-2.53082414800001));
#318680=CARTESIAN_POINT('Ctrl Pts',(-3.48960148600006,2.2,-2.53082414800001));
#318681=CARTESIAN_POINT('Ctrl Pts',(-3.48782488200006,12.2,-2.53038538900002));
#318682=CARTESIAN_POINT('Ctrl Pts',(-3.48782488200006,5.2,-2.53038538900002));
#318683=CARTESIAN_POINT('Ctrl Pts',(-3.48782488200006,2.2,-2.53038538900002));
#318684=CARTESIAN_POINT('Ctrl Pts',(-3.48605292900006,12.2,-2.52994565500002));
#318685=CARTESIAN_POINT('Ctrl Pts',(-3.48605292900006,5.2,-2.52994565500002));
#318686=CARTESIAN_POINT('Ctrl Pts',(-3.48605292900006,2.2,-2.52994565500002));
#318687=CARTESIAN_POINT('Ctrl Pts',(-3.48428563300006,12.2,-2.52950495600002));
#318688=CARTESIAN_POINT('Ctrl Pts',(-3.48428563300006,5.2,-2.52950495600002));
#318689=CARTESIAN_POINT('Ctrl Pts',(-3.48428563300006,2.2,-2.52950495600002));
#318690=CARTESIAN_POINT('Ctrl Pts',(-3.48252300300006,12.2,-2.52906330300001));
#318691=CARTESIAN_POINT('Ctrl Pts',(-3.48252300300006,5.2,-2.52906330300001));
#318692=CARTESIAN_POINT('Ctrl Pts',(-3.48252300300006,2.2,-2.52906330300001));
#318693=CARTESIAN_POINT('Ctrl Pts',(-3.48076504100006,12.2,-2.52862070600001));
#318694=CARTESIAN_POINT('Ctrl Pts',(-3.48076504100006,5.2,-2.52862070600001));
#318695=CARTESIAN_POINT('Ctrl Pts',(-3.48076504100006,2.2,-2.52862070600001));
#318696=CARTESIAN_POINT('Ctrl Pts',(-3.47901175400006,12.2,-2.52817717500001));
#318697=CARTESIAN_POINT('Ctrl Pts',(-3.47901175400006,5.2,-2.52817717500001));
#318698=CARTESIAN_POINT('Ctrl Pts',(-3.47901175400006,2.2,-2.52817717500001));
#318699=CARTESIAN_POINT('Ctrl Pts',(-3.47726314700005,12.2,-2.52773272000002));
#318700=CARTESIAN_POINT('Ctrl Pts',(-3.47726314700005,5.2,-2.52773272000002));
#318701=CARTESIAN_POINT('Ctrl Pts',(-3.47726314700005,2.2,-2.52773272000002));
#318702=CARTESIAN_POINT('Ctrl Pts',(-3.47551922500006,12.2,-2.52728735400002));
#318703=CARTESIAN_POINT('Ctrl Pts',(-3.47551922500006,5.2,-2.52728735400002));
#318704=CARTESIAN_POINT('Ctrl Pts',(-3.47551922500006,2.2,-2.52728735400002));
#318705=CARTESIAN_POINT('Ctrl Pts',(-3.47377999300006,12.2,-2.52684108500001));
#318706=CARTESIAN_POINT('Ctrl Pts',(-3.47377999300006,5.2,-2.52684108500001));
#318707=CARTESIAN_POINT('Ctrl Pts',(-3.47377999300006,2.2,-2.52684108500001));
#318708=CARTESIAN_POINT('Ctrl Pts',(-3.47204545800006,12.2,-2.52639392400001));
#318709=CARTESIAN_POINT('Ctrl Pts',(-3.47204545800006,5.2,-2.52639392400001));
#318710=CARTESIAN_POINT('Ctrl Pts',(-3.47204545800006,2.2,-2.52639392400001));
#318711=CARTESIAN_POINT('Ctrl Pts',(-3.47031562400006,12.2,-2.52594588300001));
#318712=CARTESIAN_POINT('Ctrl Pts',(-3.47031562400006,5.2,-2.52594588300001));
#318713=CARTESIAN_POINT('Ctrl Pts',(-3.47031562400006,2.2,-2.52594588300001));
#318714=CARTESIAN_POINT('Ctrl Pts',(-3.46859049400006,12.2,-2.52549697100001));
#318715=CARTESIAN_POINT('Ctrl Pts',(-3.46859049400006,5.2,-2.52549697100001));
#318716=CARTESIAN_POINT('Ctrl Pts',(-3.46859049400006,2.2,-2.52549697100001));
#318717=CARTESIAN_POINT('Ctrl Pts',(-3.46687007900006,12.2,-2.52504719900001));
#318718=CARTESIAN_POINT('Ctrl Pts',(-3.46687007900006,5.2,-2.52504719900001));
#318719=CARTESIAN_POINT('Ctrl Pts',(-3.46687007900006,2.2,-2.52504719900001));
#318720=CARTESIAN_POINT('Ctrl Pts',(-3.46515437900006,12.2,-2.52459657800001));
#318721=CARTESIAN_POINT('Ctrl Pts',(-3.46515437900006,5.2,-2.52459657800001));
#318722=CARTESIAN_POINT('Ctrl Pts',(-3.46515437900006,2.2,-2.52459657800001));
#318723=CARTESIAN_POINT('Ctrl Pts',(-3.46344340300006,12.2,-2.52414511800001));
#318724=CARTESIAN_POINT('Ctrl Pts',(-3.46344340300006,5.2,-2.52414511800001));
#318725=CARTESIAN_POINT('Ctrl Pts',(-3.46344340300006,2.2,-2.52414511800001));
#318726=CARTESIAN_POINT('Ctrl Pts',(-3.46173715200006,12.2,-2.52369283100002));
#318727=CARTESIAN_POINT('Ctrl Pts',(-3.46173715200006,5.2,-2.52369283100002));
#318728=CARTESIAN_POINT('Ctrl Pts',(-3.46173715200006,2.2,-2.52369283100002));
#318729=CARTESIAN_POINT('Ctrl Pts',(-3.46003563600005,12.2,-2.52323972700002));
#318730=CARTESIAN_POINT('Ctrl Pts',(-3.46003563600005,5.2,-2.52323972700002));
#318731=CARTESIAN_POINT('Ctrl Pts',(-3.46003563600005,2.2,-2.52323972700002));
#318732=CARTESIAN_POINT('Ctrl Pts',(-3.45833885900006,12.2,-2.52278581600001));
#318733=CARTESIAN_POINT('Ctrl Pts',(-3.45833885900006,5.2,-2.52278581600001));
#318734=CARTESIAN_POINT('Ctrl Pts',(-3.45833885900006,2.2,-2.52278581600001));
#318735=CARTESIAN_POINT('Ctrl Pts',(-3.45664682400006,12.2,-2.52233111000002));
#318736=CARTESIAN_POINT('Ctrl Pts',(-3.45664682400006,5.2,-2.52233111000002));
#318737=CARTESIAN_POINT('Ctrl Pts',(-3.45664682400006,2.2,-2.52233111000002));
#318738=CARTESIAN_POINT('Ctrl Pts',(-3.45495953800006,12.2,-2.52187561800001));
#318739=CARTESIAN_POINT('Ctrl Pts',(-3.45495953800006,5.2,-2.52187561800001));
#318740=CARTESIAN_POINT('Ctrl Pts',(-3.45495953800006,2.2,-2.52187561800001));
#318741=CARTESIAN_POINT('Ctrl Pts',(-3.45327700600006,12.2,-2.52141935300001));
#318742=CARTESIAN_POINT('Ctrl Pts',(-3.45327700600006,5.2,-2.52141935300001));
#318743=CARTESIAN_POINT('Ctrl Pts',(-3.45327700600006,2.2,-2.52141935300001));
#318744=CARTESIAN_POINT('Ctrl Pts',(-3.45159923300006,12.2,-2.52096232500001));
#318745=CARTESIAN_POINT('Ctrl Pts',(-3.45159923300006,5.2,-2.52096232500001));
#318746=CARTESIAN_POINT('Ctrl Pts',(-3.45159923300006,2.2,-2.52096232500001));
#318747=CARTESIAN_POINT('Ctrl Pts',(-3.44992622600006,12.2,-2.52050454400001));
#318748=CARTESIAN_POINT('Ctrl Pts',(-3.44992622600006,5.2,-2.52050454400001));
#318749=CARTESIAN_POINT('Ctrl Pts',(-3.44992622600006,2.2,-2.52050454400001));
#318750=CARTESIAN_POINT('Ctrl Pts',(-3.44825798800006,12.2,-2.52004602200001));
#318751=CARTESIAN_POINT('Ctrl Pts',(-3.44825798800006,5.2,-2.52004602200001));
#318752=CARTESIAN_POINT('Ctrl Pts',(-3.44825798800006,2.2,-2.52004602200001));
#318753=CARTESIAN_POINT('Ctrl Pts',(-3.44659452500006,12.2,-2.51958677000002));
#318754=CARTESIAN_POINT('Ctrl Pts',(-3.44659452500006,5.2,-2.51958677000002));
#318755=CARTESIAN_POINT('Ctrl Pts',(-3.44659452500006,2.2,-2.51958677000002));
#318756=CARTESIAN_POINT('Ctrl Pts',(-3.44493584300006,12.2,-2.51912679800002));
#318757=CARTESIAN_POINT('Ctrl Pts',(-3.44493584300006,5.2,-2.51912679800002));
#318758=CARTESIAN_POINT('Ctrl Pts',(-3.44493584300006,2.2,-2.51912679800002));
#318759=CARTESIAN_POINT('Ctrl Pts',(-3.44328194500005,12.2,-2.51866611900001));
#318760=CARTESIAN_POINT('Ctrl Pts',(-3.44328194500005,5.2,-2.51866611900001));
#318761=CARTESIAN_POINT('Ctrl Pts',(-3.44328194500005,2.2,-2.51866611900001));
#318762=CARTESIAN_POINT('Ctrl Pts',(-3.44163283900006,12.2,-2.51820474000001));
#318763=CARTESIAN_POINT('Ctrl Pts',(-3.44163283900006,5.2,-2.51820474000001));
#318764=CARTESIAN_POINT('Ctrl Pts',(-3.44163283900006,2.2,-2.51820474000001));
#318765=CARTESIAN_POINT('Ctrl Pts',(-3.43998852900006,12.2,-2.51774267700001));
#318766=CARTESIAN_POINT('Ctrl Pts',(-3.43998852900006,5.2,-2.51774267700001));
#318767=CARTESIAN_POINT('Ctrl Pts',(-3.43998852900006,2.2,-2.51774267700001));
#318768=CARTESIAN_POINT('Ctrl Pts',(-3.43834901900005,12.2,-2.51727993800001));
#318769=CARTESIAN_POINT('Ctrl Pts',(-3.43834901900005,5.2,-2.51727993800001));
#318770=CARTESIAN_POINT('Ctrl Pts',(-3.43834901900005,2.2,-2.51727993800001));
#318771=CARTESIAN_POINT('Ctrl Pts',(-3.43671431700006,12.2,-2.51681653400002));
#318772=CARTESIAN_POINT('Ctrl Pts',(-3.43671431700006,5.2,-2.51681653400002));
#318773=CARTESIAN_POINT('Ctrl Pts',(-3.43671431700006,2.2,-2.51681653400002));
#318774=CARTESIAN_POINT('Ctrl Pts',(-3.43508442600006,12.2,-2.51635247700001));
#318775=CARTESIAN_POINT('Ctrl Pts',(-3.43508442600006,5.2,-2.51635247700001));
#318776=CARTESIAN_POINT('Ctrl Pts',(-3.43508442600006,2.2,-2.51635247700001));
#318777=CARTESIAN_POINT('Ctrl Pts',(-3.43345935200006,12.2,-2.51588777800002));
#318778=CARTESIAN_POINT('Ctrl Pts',(-3.43345935200006,5.2,-2.51588777800002));
#318779=CARTESIAN_POINT('Ctrl Pts',(-3.43345935200006,2.2,-2.51588777800002));
#318780=CARTESIAN_POINT('Ctrl Pts',(-3.43183910100006,12.2,-2.51542244900001));
#318781=CARTESIAN_POINT('Ctrl Pts',(-3.43183910100006,5.2,-2.51542244900001));
#318782=CARTESIAN_POINT('Ctrl Pts',(-3.43183910100006,2.2,-2.51542244900001));
#318783=CARTESIAN_POINT('Ctrl Pts',(-3.43022367500006,12.2,-2.51495650100001));
#318784=CARTESIAN_POINT('Ctrl Pts',(-3.43022367500006,5.2,-2.51495650100001));
#318785=CARTESIAN_POINT('Ctrl Pts',(-3.43022367500006,2.2,-2.51495650100001));
#318786=CARTESIAN_POINT('Ctrl Pts',(-3.42861308300006,12.2,-2.51448994300001));
#318787=CARTESIAN_POINT('Ctrl Pts',(-3.42861308300006,5.2,-2.51448994300001));
#318788=CARTESIAN_POINT('Ctrl Pts',(-3.42861308300006,2.2,-2.51448994300001));
#318789=CARTESIAN_POINT('Ctrl Pts',(-3.42700732800005,12.2,-2.51402278900001));
#318790=CARTESIAN_POINT('Ctrl Pts',(-3.42700732800005,5.2,-2.51402278900001));
#318791=CARTESIAN_POINT('Ctrl Pts',(-3.42700732800005,2.2,-2.51402278900001));
#318792=CARTESIAN_POINT('Ctrl Pts',(-3.42540641600006,12.2,-2.51355504800001));
#318793=CARTESIAN_POINT('Ctrl Pts',(-3.42540641600006,5.2,-2.51355504800001));
#318794=CARTESIAN_POINT('Ctrl Pts',(-3.42540641600006,2.2,-2.51355504800001));
#318795=CARTESIAN_POINT('Ctrl Pts',(-3.42381035200006,12.2,-2.51308673500001));
#318796=CARTESIAN_POINT('Ctrl Pts',(-3.42381035200006,5.2,-2.51308673500001));
#318797=CARTESIAN_POINT('Ctrl Pts',(-3.42381035200006,2.2,-2.51308673500001));
#318798=CARTESIAN_POINT('Ctrl Pts',(-3.42221914100006,12.2,-2.51261785700001));
#318799=CARTESIAN_POINT('Ctrl Pts',(-3.42221914100006,5.2,-2.51261785700001));
#318800=CARTESIAN_POINT('Ctrl Pts',(-3.42221914100006,2.2,-2.51261785700001));
#318801=CARTESIAN_POINT('Ctrl Pts',(-3.42063278900006,12.2,-2.51214842700001));
#318802=CARTESIAN_POINT('Ctrl Pts',(-3.42063278900006,5.2,-2.51214842700001));
#318803=CARTESIAN_POINT('Ctrl Pts',(-3.42063278900006,2.2,-2.51214842700001));
#318804=CARTESIAN_POINT('Ctrl Pts',(-3.41905130000006,12.2,-2.51167845800001));
#318805=CARTESIAN_POINT('Ctrl Pts',(-3.41905130000006,5.2,-2.51167845800001));
#318806=CARTESIAN_POINT('Ctrl Pts',(-3.41905130000006,2.2,-2.51167845800001));
#318807=CARTESIAN_POINT('Ctrl Pts',(-3.41747467900006,12.2,-2.51120795900002));
#318808=CARTESIAN_POINT('Ctrl Pts',(-3.41747467900006,5.2,-2.51120795900002));
#318809=CARTESIAN_POINT('Ctrl Pts',(-3.41747467900006,2.2,-2.51120795900002));
#318810=CARTESIAN_POINT('Ctrl Pts',(-3.41590293200006,12.2,-2.51073694300001));
#318811=CARTESIAN_POINT('Ctrl Pts',(-3.41590293200006,5.2,-2.51073694300001));
#318812=CARTESIAN_POINT('Ctrl Pts',(-3.41590293200006,2.2,-2.51073694300001));
#318813=CARTESIAN_POINT('Ctrl Pts',(-3.41433606500006,12.2,-2.51026542000002));
#318814=CARTESIAN_POINT('Ctrl Pts',(-3.41433606500006,5.2,-2.51026542000002));
#318815=CARTESIAN_POINT('Ctrl Pts',(-3.41433606500006,2.2,-2.51026542000002));
#318816=CARTESIAN_POINT('Ctrl Pts',(-3.41277408100006,12.2,-2.50979340400002));
#318817=CARTESIAN_POINT('Ctrl Pts',(-3.41277408100006,5.2,-2.50979340400002));
#318818=CARTESIAN_POINT('Ctrl Pts',(-3.41277408100006,2.2,-2.50979340400002));
#318819=CARTESIAN_POINT('Ctrl Pts',(-3.41121698600006,12.2,-2.50932090400001));
#318820=CARTESIAN_POINT('Ctrl Pts',(-3.41121698600006,5.2,-2.50932090400001));
#318821=CARTESIAN_POINT('Ctrl Pts',(-3.41121698600006,2.2,-2.50932090400001));
#318822=CARTESIAN_POINT('Ctrl Pts',(-3.40966478600006,12.2,-2.50884793400001));
#318823=CARTESIAN_POINT('Ctrl Pts',(-3.40966478600006,5.2,-2.50884793400001));
#318824=CARTESIAN_POINT('Ctrl Pts',(-3.40966478600006,2.2,-2.50884793400001));
#318825=CARTESIAN_POINT('Ctrl Pts',(-3.40811748400006,12.2,-2.50837450300001));
#318826=CARTESIAN_POINT('Ctrl Pts',(-3.40811748400006,5.2,-2.50837450300001));
#318827=CARTESIAN_POINT('Ctrl Pts',(-3.40811748400006,2.2,-2.50837450300001));
#318828=CARTESIAN_POINT('Ctrl Pts',(-3.40657508900006,12.2,-2.50790062500001));
#318829=CARTESIAN_POINT('Ctrl Pts',(-3.40657508900006,5.2,-2.50790062500001));
#318830=CARTESIAN_POINT('Ctrl Pts',(-3.40657508900006,2.2,-2.50790062500001));
#318831=CARTESIAN_POINT('Ctrl Pts',(-3.40503760100006,12.2,-2.50742631000001));
#318832=CARTESIAN_POINT('Ctrl Pts',(-3.40503760100006,5.2,-2.50742631000001));
#318833=CARTESIAN_POINT('Ctrl Pts',(-3.40503760100006,2.2,-2.50742631000001));
#318834=CARTESIAN_POINT('Ctrl Pts',(-3.40350502900006,12.2,-2.50695157000001));
#318835=CARTESIAN_POINT('Ctrl Pts',(-3.40350502900006,5.2,-2.50695157000001));
#318836=CARTESIAN_POINT('Ctrl Pts',(-3.40350502900006,2.2,-2.50695157000001));
#318837=CARTESIAN_POINT('Ctrl Pts',(-3.40197737600006,12.2,-2.50647641700001));
#318838=CARTESIAN_POINT('Ctrl Pts',(-3.40197737600006,5.2,-2.50647641700001));
#318839=CARTESIAN_POINT('Ctrl Pts',(-3.40197737600006,2.2,-2.50647641700001));
#318840=CARTESIAN_POINT('Ctrl Pts',(-3.40045464900005,12.2,-2.50600086300001));
#318841=CARTESIAN_POINT('Ctrl Pts',(-3.40045464900005,5.2,-2.50600086300001));
#318842=CARTESIAN_POINT('Ctrl Pts',(-3.40045464900005,2.2,-2.50600086300001));
#318843=CARTESIAN_POINT('Ctrl Pts',(-3.39893685000006,12.2,-2.50552492000002));
#318844=CARTESIAN_POINT('Ctrl Pts',(-3.39893685000006,5.2,-2.50552492000002));
#318845=CARTESIAN_POINT('Ctrl Pts',(-3.39893685000006,2.2,-2.50552492000002));
#318846=CARTESIAN_POINT('Ctrl Pts',(-3.39742398800006,12.2,-2.50504859900001));
#318847=CARTESIAN_POINT('Ctrl Pts',(-3.39742398800006,5.2,-2.50504859900001));
#318848=CARTESIAN_POINT('Ctrl Pts',(-3.39742398800006,2.2,-2.50504859900001));
#318849=CARTESIAN_POINT('Ctrl Pts',(-3.39591606600006,12.2,-2.50457191200002));
#318850=CARTESIAN_POINT('Ctrl Pts',(-3.39591606600006,5.2,-2.50457191200002));
#318851=CARTESIAN_POINT('Ctrl Pts',(-3.39591606600006,2.2,-2.50457191200002));
#318852=CARTESIAN_POINT('Ctrl Pts',(-3.39441308800006,12.2,-2.50409487100002));
#318853=CARTESIAN_POINT('Ctrl Pts',(-3.39441308800006,5.2,-2.50409487100002));
#318854=CARTESIAN_POINT('Ctrl Pts',(-3.39441308800006,2.2,-2.50409487100002));
#318855=CARTESIAN_POINT('Ctrl Pts',(-3.39291506000006,12.2,-2.50361748800001));
#318856=CARTESIAN_POINT('Ctrl Pts',(-3.39291506000006,5.2,-2.50361748800001));
#318857=CARTESIAN_POINT('Ctrl Pts',(-3.39291506000006,2.2,-2.50361748800001));
#318858=CARTESIAN_POINT('Ctrl Pts',(-3.39142198700006,12.2,-2.50313977500001));
#318859=CARTESIAN_POINT('Ctrl Pts',(-3.39142198700006,5.2,-2.50313977500001));
#318860=CARTESIAN_POINT('Ctrl Pts',(-3.39142198700006,2.2,-2.50313977500001));
#318861=CARTESIAN_POINT('Ctrl Pts',(-3.38993387600006,12.2,-2.50266174300001));
#318862=CARTESIAN_POINT('Ctrl Pts',(-3.38993387600006,5.2,-2.50266174300001));
#318863=CARTESIAN_POINT('Ctrl Pts',(-3.38993387600006,2.2,-2.50266174300001));
#318864=CARTESIAN_POINT('Ctrl Pts',(-3.38845072900006,12.2,-2.50218340600001));
#318865=CARTESIAN_POINT('Ctrl Pts',(-3.38845072900006,5.2,-2.50218340600001));
#318866=CARTESIAN_POINT('Ctrl Pts',(-3.38845072900006,2.2,-2.50218340600001));
#318867=CARTESIAN_POINT('Ctrl Pts',(-3.38697255200006,12.2,-2.50170477500001));
#318868=CARTESIAN_POINT('Ctrl Pts',(-3.38697255200006,5.2,-2.50170477500001));
#318869=CARTESIAN_POINT('Ctrl Pts',(-3.38697255200006,2.2,-2.50170477500001));
#318870=CARTESIAN_POINT('Ctrl Pts',(-3.38549935200006,12.2,-2.50122586100002));
#318871=CARTESIAN_POINT('Ctrl Pts',(-3.38549935200006,5.2,-2.50122586100002));
#318872=CARTESIAN_POINT('Ctrl Pts',(-3.38549935200006,2.2,-2.50122586100002));
#318873=CARTESIAN_POINT('Ctrl Pts',(-3.38403113100005,12.2,-2.50074667700002));
#318874=CARTESIAN_POINT('Ctrl Pts',(-3.38403113100005,5.2,-2.50074667700002));
#318875=CARTESIAN_POINT('Ctrl Pts',(-3.38403113100005,2.2,-2.50074667700002));
#318876=CARTESIAN_POINT('Ctrl Pts',(-3.38256789600006,12.2,-2.50026723500001));
#318877=CARTESIAN_POINT('Ctrl Pts',(-3.38256789600006,5.2,-2.50026723500001));
#318878=CARTESIAN_POINT('Ctrl Pts',(-3.38256789600006,2.2,-2.50026723500001));
#318879=CARTESIAN_POINT('Ctrl Pts',(-3.38110965100006,12.2,-2.49978754700001));
#318880=CARTESIAN_POINT('Ctrl Pts',(-3.38110965100006,5.2,-2.49978754700001));
#318881=CARTESIAN_POINT('Ctrl Pts',(-3.38110965100006,2.2,-2.49978754700001));
#318882=CARTESIAN_POINT('Ctrl Pts',(-3.37965640100006,12.2,-2.49930762600002));
#318883=CARTESIAN_POINT('Ctrl Pts',(-3.37965640100006,5.2,-2.49930762600002));
#318884=CARTESIAN_POINT('Ctrl Pts',(-3.37965640100006,2.2,-2.49930762600002));
#318885=CARTESIAN_POINT('Ctrl Pts',(-3.37820815200006,12.2,-2.49882748400001));
#318886=CARTESIAN_POINT('Ctrl Pts',(-3.37820815200006,5.2,-2.49882748400001));
#318887=CARTESIAN_POINT('Ctrl Pts',(-3.37820815200006,2.2,-2.49882748400001));
#318888=CARTESIAN_POINT('Ctrl Pts',(-3.37676490800006,12.2,-2.49834713200002));
#318889=CARTESIAN_POINT('Ctrl Pts',(-3.37676490800006,5.2,-2.49834713200002));
#318890=CARTESIAN_POINT('Ctrl Pts',(-3.37676490800006,2.2,-2.49834713200002));
#318891=CARTESIAN_POINT('Ctrl Pts',(-3.37532667400006,12.2,-2.49786658300001));
#318892=CARTESIAN_POINT('Ctrl Pts',(-3.37532667400006,5.2,-2.49786658300001));
#318893=CARTESIAN_POINT('Ctrl Pts',(-3.37532667400006,2.2,-2.49786658300001));
#318894=CARTESIAN_POINT('Ctrl Pts',(-3.37389345600006,12.2,-2.49738584900001));
#318895=CARTESIAN_POINT('Ctrl Pts',(-3.37389345600006,5.2,-2.49738584900001));
#318896=CARTESIAN_POINT('Ctrl Pts',(-3.37389345600006,2.2,-2.49738584900001));
#318897=CARTESIAN_POINT('Ctrl Pts',(-3.37246525800006,12.2,-2.49690494400001));
#318898=CARTESIAN_POINT('Ctrl Pts',(-3.37246525800006,5.2,-2.49690494400001));
#318899=CARTESIAN_POINT('Ctrl Pts',(-3.37246525800006,2.2,-2.49690494400001));
#318900=CARTESIAN_POINT('Ctrl Pts',(-3.37104208500006,12.2,-2.49642387800002));
#318901=CARTESIAN_POINT('Ctrl Pts',(-3.37104208500006,5.2,-2.49642387800002));
#318902=CARTESIAN_POINT('Ctrl Pts',(-3.37104208500006,2.2,-2.49642387800002));
#318903=CARTESIAN_POINT('Ctrl Pts',(-3.36962394300006,12.2,-2.49594266500001));
#318904=CARTESIAN_POINT('Ctrl Pts',(-3.36962394300006,5.2,-2.49594266500001));
#318905=CARTESIAN_POINT('Ctrl Pts',(-3.36962394300006,2.2,-2.49594266500001));
#318906=CARTESIAN_POINT('Ctrl Pts',(-3.36821083500006,12.2,-2.49546131700002));
#318907=CARTESIAN_POINT('Ctrl Pts',(-3.36821083500006,5.2,-2.49546131700002));
#318908=CARTESIAN_POINT('Ctrl Pts',(-3.36821083500006,2.2,-2.49546131700002));
#318909=CARTESIAN_POINT('Ctrl Pts',(-3.36680276800006,12.2,-2.49497984500001));
#318910=CARTESIAN_POINT('Ctrl Pts',(-3.36680276800006,5.2,-2.49497984500001));
#318911=CARTESIAN_POINT('Ctrl Pts',(-3.36680276800006,2.2,-2.49497984500001));
#318912=CARTESIAN_POINT('Ctrl Pts',(-3.36539974500006,12.2,-2.49449826400001));
#318913=CARTESIAN_POINT('Ctrl Pts',(-3.36539974500006,5.2,-2.49449826400001));
#318914=CARTESIAN_POINT('Ctrl Pts',(-3.36539974500006,2.2,-2.49449826400001));
#318915=CARTESIAN_POINT('Ctrl Pts',(-3.36400177300006,12.2,-2.49401658500001));
#318916=CARTESIAN_POINT('Ctrl Pts',(-3.36400177300006,5.2,-2.49401658500001));
#318917=CARTESIAN_POINT('Ctrl Pts',(-3.36400177300006,2.2,-2.49401658500001));
#318918=CARTESIAN_POINT('Ctrl Pts',(-3.36260885500006,12.2,-2.49353482100001));
#318919=CARTESIAN_POINT('Ctrl Pts',(-3.36260885500006,5.2,-2.49353482100001));
#318920=CARTESIAN_POINT('Ctrl Pts',(-3.36260885500006,2.2,-2.49353482100001));
#318921=CARTESIAN_POINT('Ctrl Pts',(-3.36122099700006,12.2,-2.49305298500001));
#318922=CARTESIAN_POINT('Ctrl Pts',(-3.36122099700006,5.2,-2.49305298500001));
#318923=CARTESIAN_POINT('Ctrl Pts',(-3.36122099700006,2.2,-2.49305298500001));
#318924=CARTESIAN_POINT('Ctrl Pts',(-3.35983820300005,12.2,-2.49257108800002));
#318925=CARTESIAN_POINT('Ctrl Pts',(-3.35983820300005,5.2,-2.49257108800002));
#318926=CARTESIAN_POINT('Ctrl Pts',(-3.35983820300005,2.2,-2.49257108800002));
#318927=CARTESIAN_POINT('Ctrl Pts',(-3.35846048000006,12.2,-2.49208914400001));
#318928=CARTESIAN_POINT('Ctrl Pts',(-3.35846048000006,5.2,-2.49208914400001));
#318929=CARTESIAN_POINT('Ctrl Pts',(-3.35846048000006,2.2,-2.49208914400001));
#318930=CARTESIAN_POINT('Ctrl Pts',(-3.35708783000006,12.2,-2.49160716600001));
#318931=CARTESIAN_POINT('Ctrl Pts',(-3.35708783000006,5.2,-2.49160716600001));
#318932=CARTESIAN_POINT('Ctrl Pts',(-3.35708783000006,2.2,-2.49160716600001));
#318933=CARTESIAN_POINT('Ctrl Pts',(-3.35572026000006,12.2,-2.49112516600002));
#318934=CARTESIAN_POINT('Ctrl Pts',(-3.35572026000006,5.2,-2.49112516600002));
#318935=CARTESIAN_POINT('Ctrl Pts',(-3.35572026000006,2.2,-2.49112516600002));
#318936=CARTESIAN_POINT('Ctrl Pts',(-3.35435777400006,12.2,-2.49064315600001));
#318937=CARTESIAN_POINT('Ctrl Pts',(-3.35435777400006,5.2,-2.49064315600001));
#318938=CARTESIAN_POINT('Ctrl Pts',(-3.35435777400006,2.2,-2.49064315600001));
#318939=CARTESIAN_POINT('Ctrl Pts',(-3.35300037700006,12.2,-2.49016115000002));
#318940=CARTESIAN_POINT('Ctrl Pts',(-3.35300037700006,5.2,-2.49016115000002));
#318941=CARTESIAN_POINT('Ctrl Pts',(-3.35300037700006,2.2,-2.49016115000002));
#318942=CARTESIAN_POINT('Ctrl Pts',(-3.35164807400006,12.2,-2.48967916000002));
#318943=CARTESIAN_POINT('Ctrl Pts',(-3.35164807400006,5.2,-2.48967916000002));
#318944=CARTESIAN_POINT('Ctrl Pts',(-3.35164807400006,2.2,-2.48967916000002));
#318945=CARTESIAN_POINT('Ctrl Pts',(-3.35030087000006,12.2,-2.48919720100002));
#318946=CARTESIAN_POINT('Ctrl Pts',(-3.35030087000006,5.2,-2.48919720100002));
#318947=CARTESIAN_POINT('Ctrl Pts',(-3.35030087000006,2.2,-2.48919720100002));
#318948=CARTESIAN_POINT('Ctrl Pts',(-3.34895877000006,12.2,-2.48871528200001));
#318949=CARTESIAN_POINT('Ctrl Pts',(-3.34895877000006,5.2,-2.48871528200001));
#318950=CARTESIAN_POINT('Ctrl Pts',(-3.34895877000006,2.2,-2.48871528200001));
#318951=CARTESIAN_POINT('Ctrl Pts',(-3.34762177700005,12.2,-2.48823341900001));
#318952=CARTESIAN_POINT('Ctrl Pts',(-3.34762177700005,5.2,-2.48823341900001));
#318953=CARTESIAN_POINT('Ctrl Pts',(-3.34762177700005,2.2,-2.48823341900001));
#318954=CARTESIAN_POINT('Ctrl Pts',(-3.34628989900006,12.2,-2.48775162500001));
#318955=CARTESIAN_POINT('Ctrl Pts',(-3.34628989900006,5.2,-2.48775162500001));
#318956=CARTESIAN_POINT('Ctrl Pts',(-3.34628989900006,2.2,-2.48775162500001));
#318957=CARTESIAN_POINT('Ctrl Pts',(-3.34496313800006,12.2,-2.48726991000002));
#318958=CARTESIAN_POINT('Ctrl Pts',(-3.34496313800006,5.2,-2.48726991000002));
#318959=CARTESIAN_POINT('Ctrl Pts',(-3.34496313800006,2.2,-2.48726991000002));
#318960=CARTESIAN_POINT('Ctrl Pts',(-3.34364150100006,12.2,-2.48678829000001));
#318961=CARTESIAN_POINT('Ctrl Pts',(-3.34364150100006,5.2,-2.48678829000001));
#318962=CARTESIAN_POINT('Ctrl Pts',(-3.34364150100006,2.2,-2.48678829000001));
#318963=CARTESIAN_POINT('Ctrl Pts',(-3.34232499000006,12.2,-2.48630677700001));
#318964=CARTESIAN_POINT('Ctrl Pts',(-3.34232499000006,5.2,-2.48630677700001));
#318965=CARTESIAN_POINT('Ctrl Pts',(-3.34232499000006,2.2,-2.48630677700001));
#318966=CARTESIAN_POINT('Ctrl Pts',(-3.34101361300006,12.2,-2.48582538400001));
#318967=CARTESIAN_POINT('Ctrl Pts',(-3.34101361300006,5.2,-2.48582538400001));
#318968=CARTESIAN_POINT('Ctrl Pts',(-3.34101361300006,2.2,-2.48582538400001));
#318969=CARTESIAN_POINT('Ctrl Pts',(-3.33970737300006,12.2,-2.48534412500002));
#318970=CARTESIAN_POINT('Ctrl Pts',(-3.33970737300006,5.2,-2.48534412500002));
#318971=CARTESIAN_POINT('Ctrl Pts',(-3.33970737300006,2.2,-2.48534412500002));
#318972=CARTESIAN_POINT('Ctrl Pts',(-3.33840627500006,12.2,-2.48486301100002));
#318973=CARTESIAN_POINT('Ctrl Pts',(-3.33840627500006,5.2,-2.48486301100002));
#318974=CARTESIAN_POINT('Ctrl Pts',(-3.33840627500006,2.2,-2.48486301100002));
#318975=CARTESIAN_POINT('Ctrl Pts',(-3.33711032500006,12.2,-2.48438205700001));
#318976=CARTESIAN_POINT('Ctrl Pts',(-3.33711032500006,5.2,-2.48438205700001));
#318977=CARTESIAN_POINT('Ctrl Pts',(-3.33711032500006,2.2,-2.48438205700001));
#318978=CARTESIAN_POINT('Ctrl Pts',(-3.33581952600006,12.2,-2.48390127600001));
#318979=CARTESIAN_POINT('Ctrl Pts',(-3.33581952600006,5.2,-2.48390127600001));
#318980=CARTESIAN_POINT('Ctrl Pts',(-3.33581952600006,2.2,-2.48390127600001));
#318981=CARTESIAN_POINT('Ctrl Pts',(-3.33453388300006,12.2,-2.48342068100001));
#318982=CARTESIAN_POINT('Ctrl Pts',(-3.33453388300006,5.2,-2.48342068100001));
#318983=CARTESIAN_POINT('Ctrl Pts',(-3.33453388300006,2.2,-2.48342068100001));
#318984=CARTESIAN_POINT('Ctrl Pts',(-3.33325340200005,12.2,-2.48294028500001));
#318985=CARTESIAN_POINT('Ctrl Pts',(-3.33325340200005,5.2,-2.48294028500001));
#318986=CARTESIAN_POINT('Ctrl Pts',(-3.33325340200005,2.2,-2.48294028500001));
#318987=CARTESIAN_POINT('Ctrl Pts',(-3.33197808600006,12.2,-2.48246010200001));
#318988=CARTESIAN_POINT('Ctrl Pts',(-3.33197808600006,5.2,-2.48246010200001));
#318989=CARTESIAN_POINT('Ctrl Pts',(-3.33197808600006,2.2,-2.48246010200001));
#318990=CARTESIAN_POINT('Ctrl Pts',(-3.33070794200006,12.2,-2.48198014500002));
#318991=CARTESIAN_POINT('Ctrl Pts',(-3.33070794200006,5.2,-2.48198014500002));
#318992=CARTESIAN_POINT('Ctrl Pts',(-3.33070794200006,2.2,-2.48198014500002));
#318993=CARTESIAN_POINT('Ctrl Pts',(-3.32944297300005,12.2,-2.48150042700002));
#318994=CARTESIAN_POINT('Ctrl Pts',(-3.32944297300005,5.2,-2.48150042700002));
#318995=CARTESIAN_POINT('Ctrl Pts',(-3.32944297300005,2.2,-2.48150042700002));
#318996=CARTESIAN_POINT('Ctrl Pts',(-3.32818318400005,12.2,-2.48102096200002));
#318997=CARTESIAN_POINT('Ctrl Pts',(-3.32818318400005,5.2,-2.48102096200002));
#318998=CARTESIAN_POINT('Ctrl Pts',(-3.32818318400005,2.2,-2.48102096200002));
#318999=CARTESIAN_POINT('Ctrl Pts',(-3.32692858000006,12.2,-2.48054176300001));
#319000=CARTESIAN_POINT('Ctrl Pts',(-3.32692858000006,5.2,-2.48054176300001));
#319001=CARTESIAN_POINT('Ctrl Pts',(-3.32692858000006,2.2,-2.48054176300001));
#319002=CARTESIAN_POINT('Ctrl Pts',(-3.32567916700006,12.2,-2.48006284300001));
#319003=CARTESIAN_POINT('Ctrl Pts',(-3.32567916700006,5.2,-2.48006284300001));
#319004=CARTESIAN_POINT('Ctrl Pts',(-3.32567916700006,2.2,-2.48006284300001));
#319005=CARTESIAN_POINT('Ctrl Pts',(-3.32443494700006,12.2,-2.47958421700002));
#319006=CARTESIAN_POINT('Ctrl Pts',(-3.32443494700006,5.2,-2.47958421700002));
#319007=CARTESIAN_POINT('Ctrl Pts',(-3.32443494700006,2.2,-2.47958421700002));
#319008=CARTESIAN_POINT('Ctrl Pts',(-3.32319592500005,12.2,-2.47910589800002));
#319009=CARTESIAN_POINT('Ctrl Pts',(-3.32319592500005,5.2,-2.47910589800002));
#319010=CARTESIAN_POINT('Ctrl Pts',(-3.32319592500005,2.2,-2.47910589800002));
#319011=CARTESIAN_POINT('Ctrl Pts',(-3.32196210900006,12.2,-2.47862789900001));
#319012=CARTESIAN_POINT('Ctrl Pts',(-3.32196210900006,5.2,-2.47862789900001));
#319013=CARTESIAN_POINT('Ctrl Pts',(-3.32196210900006,2.2,-2.47862789900001));
#319014=CARTESIAN_POINT('Ctrl Pts',(-3.32073350000006,12.2,-2.47815023400001));
#319015=CARTESIAN_POINT('Ctrl Pts',(-3.32073350000006,5.2,-2.47815023400001));
#319016=CARTESIAN_POINT('Ctrl Pts',(-3.32073350000006,2.2,-2.47815023400001));
#319017=CARTESIAN_POINT('Ctrl Pts',(-3.31951010500006,12.2,-2.47767291800002));
#319018=CARTESIAN_POINT('Ctrl Pts',(-3.31951010500006,5.2,-2.47767291800002));
#319019=CARTESIAN_POINT('Ctrl Pts',(-3.31951010500006,2.2,-2.47767291800002));
#319020=CARTESIAN_POINT('Ctrl Pts',(-3.31829192800006,12.2,-2.47719596200001));
#319021=CARTESIAN_POINT('Ctrl Pts',(-3.31829192800006,5.2,-2.47719596200001));
#319022=CARTESIAN_POINT('Ctrl Pts',(-3.31829192800006,2.2,-2.47719596200001));
#319023=CARTESIAN_POINT('Ctrl Pts',(-3.31707897300006,12.2,-2.47671938100002));
#319024=CARTESIAN_POINT('Ctrl Pts',(-3.31707897300006,5.2,-2.47671938100002));
#319025=CARTESIAN_POINT('Ctrl Pts',(-3.31707897300006,2.2,-2.47671938100002));
#319026=CARTESIAN_POINT('Ctrl Pts',(-3.31587124500006,12.2,-2.47624318900002));
#319027=CARTESIAN_POINT('Ctrl Pts',(-3.31587124500006,5.2,-2.47624318900002));
#319028=CARTESIAN_POINT('Ctrl Pts',(-3.31587124500006,2.2,-2.47624318900002));
#319029=CARTESIAN_POINT('Ctrl Pts',(-3.31466875000006,12.2,-2.47576740100001));
#319030=CARTESIAN_POINT('Ctrl Pts',(-3.31466875000006,5.2,-2.47576740100001));
#319031=CARTESIAN_POINT('Ctrl Pts',(-3.31466875000006,2.2,-2.47576740100001));
#319032=CARTESIAN_POINT('Ctrl Pts',(-3.31347149000006,12.2,-2.47529202900001));
#319033=CARTESIAN_POINT('Ctrl Pts',(-3.31347149000006,5.2,-2.47529202900001));
#319034=CARTESIAN_POINT('Ctrl Pts',(-3.31347149000006,2.2,-2.47529202900001));
#319035=CARTESIAN_POINT('Ctrl Pts',(-3.31227947200006,12.2,-2.47481708700001));
#319036=CARTESIAN_POINT('Ctrl Pts',(-3.31227947200006,5.2,-2.47481708700001));
#319037=CARTESIAN_POINT('Ctrl Pts',(-3.31227947200006,2.2,-2.47481708700001));
#319038=CARTESIAN_POINT('Ctrl Pts',(-3.31109269900006,12.2,-2.47434258900002));
#319039=CARTESIAN_POINT('Ctrl Pts',(-3.31109269900006,5.2,-2.47434258900002));
#319040=CARTESIAN_POINT('Ctrl Pts',(-3.31109269900006,2.2,-2.47434258900002));
#319041=CARTESIAN_POINT('Ctrl Pts',(-3.30991117600006,12.2,-2.47386855000002));
#319042=CARTESIAN_POINT('Ctrl Pts',(-3.30991117600006,5.2,-2.47386855000002));
#319043=CARTESIAN_POINT('Ctrl Pts',(-3.30991117600006,2.2,-2.47386855000002));
#319044=CARTESIAN_POINT('Ctrl Pts',(-3.30873490900006,12.2,-2.47339498400001));
#319045=CARTESIAN_POINT('Ctrl Pts',(-3.30873490900006,5.2,-2.47339498400001));
#319046=CARTESIAN_POINT('Ctrl Pts',(-3.30873490900006,2.2,-2.47339498400001));
#319047=CARTESIAN_POINT('Ctrl Pts',(-3.30756390200006,12.2,-2.47292190300001));
#319048=CARTESIAN_POINT('Ctrl Pts',(-3.30756390200006,5.2,-2.47292190300001));
#319049=CARTESIAN_POINT('Ctrl Pts',(-3.30756390200006,2.2,-2.47292190300001));
#319050=CARTESIAN_POINT('Ctrl Pts',(-3.30639815800006,12.2,-2.47244932300001));
#319051=CARTESIAN_POINT('Ctrl Pts',(-3.30639815800006,5.2,-2.47244932300001));
#319052=CARTESIAN_POINT('Ctrl Pts',(-3.30639815800006,2.2,-2.47244932300001));
#319053=CARTESIAN_POINT('Ctrl Pts',(-3.30523768300006,12.2,-2.47197725900001));
#319054=CARTESIAN_POINT('Ctrl Pts',(-3.30523768300006,5.2,-2.47197725900001));
#319055=CARTESIAN_POINT('Ctrl Pts',(-3.30523768300006,2.2,-2.47197725900001));
#319056=CARTESIAN_POINT('Ctrl Pts',(-3.30408248100006,12.2,-2.47150572200002));
#319057=CARTESIAN_POINT('Ctrl Pts',(-3.30408248100006,5.2,-2.47150572200002));
#319058=CARTESIAN_POINT('Ctrl Pts',(-3.30408248100006,2.2,-2.47150572200002));
#319059=CARTESIAN_POINT('Ctrl Pts',(-3.30293255700005,12.2,-2.47103473000001));
#319060=CARTESIAN_POINT('Ctrl Pts',(-3.30293255700005,5.2,-2.47103473000001));
#319061=CARTESIAN_POINT('Ctrl Pts',(-3.30293255700005,2.2,-2.47103473000001));
#319062=CARTESIAN_POINT('Ctrl Pts',(-3.30178791500006,12.2,-2.47056429300001));
#319063=CARTESIAN_POINT('Ctrl Pts',(-3.30178791500006,5.2,-2.47056429300001));
#319064=CARTESIAN_POINT('Ctrl Pts',(-3.30178791500006,2.2,-2.47056429300001));
#319065=CARTESIAN_POINT('Ctrl Pts',(-3.30064856100006,12.2,-2.47009442900001));
#319066=CARTESIAN_POINT('Ctrl Pts',(-3.30064856100006,5.2,-2.47009442900001));
#319067=CARTESIAN_POINT('Ctrl Pts',(-3.30064856100006,2.2,-2.47009442900001));
#319068=CARTESIAN_POINT('Ctrl Pts',(-3.29951449800005,12.2,-2.46962514900002));
#319069=CARTESIAN_POINT('Ctrl Pts',(-3.29951449800005,5.2,-2.46962514900002));
#319070=CARTESIAN_POINT('Ctrl Pts',(-3.29951449800005,2.2,-2.46962514900002));
#319071=CARTESIAN_POINT('Ctrl Pts',(-3.29838573100006,12.2,-2.46915647100002));
#319072=CARTESIAN_POINT('Ctrl Pts',(-3.29838573100006,5.2,-2.46915647100002));
#319073=CARTESIAN_POINT('Ctrl Pts',(-3.29838573100006,2.2,-2.46915647100002));
#319074=CARTESIAN_POINT('Ctrl Pts',(-3.29726226400005,12.2,-2.46868840700001));
#319075=CARTESIAN_POINT('Ctrl Pts',(-3.29726226400005,5.2,-2.46868840700001));
#319076=CARTESIAN_POINT('Ctrl Pts',(-3.29726226400005,2.2,-2.46868840700001));
#319077=CARTESIAN_POINT('Ctrl Pts',(-3.29614410300006,12.2,-2.46822097100001));
#319078=CARTESIAN_POINT('Ctrl Pts',(-3.29614410300006,5.2,-2.46822097100001));
#319079=CARTESIAN_POINT('Ctrl Pts',(-3.29614410300006,2.2,-2.46822097100001));
#319080=CARTESIAN_POINT('Ctrl Pts',(-3.29503125100006,12.2,-2.46775417800002));
#319081=CARTESIAN_POINT('Ctrl Pts',(-3.29503125100006,5.2,-2.46775417800002));
#319082=CARTESIAN_POINT('Ctrl Pts',(-3.29503125100006,2.2,-2.46775417800002));
#319083=CARTESIAN_POINT('Ctrl Pts',(-3.29392371400006,12.2,-2.46728804500002));
#319084=CARTESIAN_POINT('Ctrl Pts',(-3.29392371400006,5.2,-2.46728804500002));
#319085=CARTESIAN_POINT('Ctrl Pts',(-3.29392371400006,2.2,-2.46728804500002));
#319086=CARTESIAN_POINT('Ctrl Pts',(-3.29282149400006,12.2,-2.46682258300002));
#319087=CARTESIAN_POINT('Ctrl Pts',(-3.29282149400006,5.2,-2.46682258300002));
#319088=CARTESIAN_POINT('Ctrl Pts',(-3.29282149400006,2.2,-2.46682258300002));
#319089=CARTESIAN_POINT('Ctrl Pts',(-3.29172459900006,12.2,-2.46635780800001));
#319090=CARTESIAN_POINT('Ctrl Pts',(-3.29172459900006,5.2,-2.46635780800001));
#319091=CARTESIAN_POINT('Ctrl Pts',(-3.29172459900006,2.2,-2.46635780800001));
#319092=CARTESIAN_POINT('Ctrl Pts',(-3.29063303000006,12.2,-2.46589373500001));
#319093=CARTESIAN_POINT('Ctrl Pts',(-3.29063303000006,5.2,-2.46589373500001));
#319094=CARTESIAN_POINT('Ctrl Pts',(-3.29063303000006,2.2,-2.46589373500001));
#319095=CARTESIAN_POINT('Ctrl Pts',(-3.28954679400006,12.2,-2.46543037800001));
#319096=CARTESIAN_POINT('Ctrl Pts',(-3.28954679400006,5.2,-2.46543037800001));
#319097=CARTESIAN_POINT('Ctrl Pts',(-3.28954679400006,2.2,-2.46543037800001));
#319098=CARTESIAN_POINT('Ctrl Pts',(-3.28846589400006,12.2,-2.46496775200002));
#319099=CARTESIAN_POINT('Ctrl Pts',(-3.28846589400006,5.2,-2.46496775200002));
#319100=CARTESIAN_POINT('Ctrl Pts',(-3.28846589400006,2.2,-2.46496775200002));
#319101=CARTESIAN_POINT('Ctrl Pts',(-3.28739033400006,12.2,-2.46450587100002));
#319102=CARTESIAN_POINT('Ctrl Pts',(-3.28739033400006,5.2,-2.46450587100002));
#319103=CARTESIAN_POINT('Ctrl Pts',(-3.28739033400006,2.2,-2.46450587100002));
#319104=CARTESIAN_POINT('Ctrl Pts',(-3.28632012100006,12.2,-2.46404475100002));
#319105=CARTESIAN_POINT('Ctrl Pts',(-3.28632012100006,5.2,-2.46404475100002));
#319106=CARTESIAN_POINT('Ctrl Pts',(-3.28632012100006,2.2,-2.46404475100002));
#319107=CARTESIAN_POINT('Ctrl Pts',(-3.28525525700006,12.2,-2.46358440600002));
#319108=CARTESIAN_POINT('Ctrl Pts',(-3.28525525700006,5.2,-2.46358440600002));
#319109=CARTESIAN_POINT('Ctrl Pts',(-3.28525525700006,2.2,-2.46358440600002));
#319110=CARTESIAN_POINT('Ctrl Pts',(-3.28419574700006,12.2,-2.46312485200002));
#319111=CARTESIAN_POINT('Ctrl Pts',(-3.28419574700006,5.2,-2.46312485200002));
#319112=CARTESIAN_POINT('Ctrl Pts',(-3.28419574700006,2.2,-2.46312485200002));
#319113=CARTESIAN_POINT('Ctrl Pts',(-3.28314159600006,12.2,-2.46266610200002));
#319114=CARTESIAN_POINT('Ctrl Pts',(-3.28314159600006,5.2,-2.46266610200002));
#319115=CARTESIAN_POINT('Ctrl Pts',(-3.28314159600006,2.2,-2.46266610200002));
#319116=CARTESIAN_POINT('Ctrl Pts',(-3.28209280800006,12.2,-2.46220817300001));
#319117=CARTESIAN_POINT('Ctrl Pts',(-3.28209280800006,5.2,-2.46220817300001));
#319118=CARTESIAN_POINT('Ctrl Pts',(-3.28209280800006,2.2,-2.46220817300001));
#319119=CARTESIAN_POINT('Ctrl Pts',(-3.28104938800006,12.2,-2.46175107800001));
#319120=CARTESIAN_POINT('Ctrl Pts',(-3.28104938800006,5.2,-2.46175107800001));
#319121=CARTESIAN_POINT('Ctrl Pts',(-3.28104938800006,2.2,-2.46175107800001));
#319122=CARTESIAN_POINT('Ctrl Pts',(-3.28001133900006,12.2,-2.46129483400002));
#319123=CARTESIAN_POINT('Ctrl Pts',(-3.28001133900006,5.2,-2.46129483400002));
#319124=CARTESIAN_POINT('Ctrl Pts',(-3.28001133900006,2.2,-2.46129483400002));
#319125=CARTESIAN_POINT('Ctrl Pts',(-3.27897866600006,12.2,-2.46083945400001));
#319126=CARTESIAN_POINT('Ctrl Pts',(-3.27897866600006,5.2,-2.46083945400001));
#319127=CARTESIAN_POINT('Ctrl Pts',(-3.27897866600006,2.2,-2.46083945400001));
#319128=CARTESIAN_POINT('Ctrl Pts',(-3.27795137500006,12.2,-2.46038495500001));
#319129=CARTESIAN_POINT('Ctrl Pts',(-3.27795137500006,5.2,-2.46038495500001));
#319130=CARTESIAN_POINT('Ctrl Pts',(-3.27795137500006,2.2,-2.46038495500001));
#319131=CARTESIAN_POINT('Ctrl Pts',(-3.27692946800005,12.2,-2.45993135100001));
#319132=CARTESIAN_POINT('Ctrl Pts',(-3.27692946800005,5.2,-2.45993135100001));
#319133=CARTESIAN_POINT('Ctrl Pts',(-3.27692946800005,2.2,-2.45993135100001));
#319134=CARTESIAN_POINT('Ctrl Pts',(-3.27591295000006,12.2,-2.45947865700002));
#319135=CARTESIAN_POINT('Ctrl Pts',(-3.27591295000006,5.2,-2.45947865700002));
#319136=CARTESIAN_POINT('Ctrl Pts',(-3.27591295000006,2.2,-2.45947865700002));
#319137=CARTESIAN_POINT('Ctrl Pts',(-3.27490182500005,12.2,-2.45902688900001));
#319138=CARTESIAN_POINT('Ctrl Pts',(-3.27490182500005,5.2,-2.45902688900001));
#319139=CARTESIAN_POINT('Ctrl Pts',(-3.27490182500005,2.2,-2.45902688900001));
#319140=CARTESIAN_POINT('Ctrl Pts',(-3.27389610000006,12.2,-2.45857606200001));
#319141=CARTESIAN_POINT('Ctrl Pts',(-3.27389610000006,5.2,-2.45857606200001));
#319142=CARTESIAN_POINT('Ctrl Pts',(-3.27389610000006,2.2,-2.45857606200001));
#319143=CARTESIAN_POINT('Ctrl Pts',(-3.27289577600005,12.2,-2.45812619100001));
#319144=CARTESIAN_POINT('Ctrl Pts',(-3.27289577600005,5.2,-2.45812619100001));
#319145=CARTESIAN_POINT('Ctrl Pts',(-3.27289577600005,2.2,-2.45812619100001));
#319146=CARTESIAN_POINT('Ctrl Pts',(-3.27190085800006,12.2,-2.45767729200002));
#319147=CARTESIAN_POINT('Ctrl Pts',(-3.27190085800006,5.2,-2.45767729200002));
#319148=CARTESIAN_POINT('Ctrl Pts',(-3.27190085800006,2.2,-2.45767729200002));
#319149=CARTESIAN_POINT('Ctrl Pts',(-3.27091135200006,12.2,-2.45722938000001));
#319150=CARTESIAN_POINT('Ctrl Pts',(-3.27091135200006,5.2,-2.45722938000001));
#319151=CARTESIAN_POINT('Ctrl Pts',(-3.27091135200006,2.2,-2.45722938000001));
#319152=CARTESIAN_POINT('Ctrl Pts',(-3.26992726100006,12.2,-2.45678247000002));
#319153=CARTESIAN_POINT('Ctrl Pts',(-3.26992726100006,5.2,-2.45678247000002));
#319154=CARTESIAN_POINT('Ctrl Pts',(-3.26992726100006,2.2,-2.45678247000002));
#319155=CARTESIAN_POINT('Ctrl Pts',(-3.26894858800005,12.2,-2.45633657900001));
#319156=CARTESIAN_POINT('Ctrl Pts',(-3.26894858800005,5.2,-2.45633657900001));
#319157=CARTESIAN_POINT('Ctrl Pts',(-3.26894858800005,2.2,-2.45633657900001));
#319158=CARTESIAN_POINT('Ctrl Pts',(-3.26797534100006,12.2,-2.45589172000001));
#319159=CARTESIAN_POINT('Ctrl Pts',(-3.26797534100006,5.2,-2.45589172000001));
#319160=CARTESIAN_POINT('Ctrl Pts',(-3.26797534100006,2.2,-2.45589172000001));
#319161=CARTESIAN_POINT('Ctrl Pts',(-3.26700752100006,12.2,-2.45544791100002));
#319162=CARTESIAN_POINT('Ctrl Pts',(-3.26700752100006,5.2,-2.45544791100002));
#319163=CARTESIAN_POINT('Ctrl Pts',(-3.26700752100006,2.2,-2.45544791100002));
#319164=CARTESIAN_POINT('Ctrl Pts',(-3.26604513300006,12.2,-2.45500516800002));
#319165=CARTESIAN_POINT('Ctrl Pts',(-3.26604513300006,5.2,-2.45500516800002));
#319166=CARTESIAN_POINT('Ctrl Pts',(-3.26604513300006,2.2,-2.45500516800002));
#319167=CARTESIAN_POINT('Ctrl Pts',(-3.26508818200006,12.2,-2.45456350400001));
#319168=CARTESIAN_POINT('Ctrl Pts',(-3.26508818200006,5.2,-2.45456350400001));
#319169=CARTESIAN_POINT('Ctrl Pts',(-3.26508818200006,2.2,-2.45456350400001));
#319170=CARTESIAN_POINT('Ctrl Pts',(-3.26413667200006,12.2,-2.45412293500001));
#319171=CARTESIAN_POINT('Ctrl Pts',(-3.26413667200006,5.2,-2.45412293500001));
#319172=CARTESIAN_POINT('Ctrl Pts',(-3.26413667200006,2.2,-2.45412293500001));
#319173=CARTESIAN_POINT('Ctrl Pts',(-3.26319060600006,12.2,-2.45368347900001));
#319174=CARTESIAN_POINT('Ctrl Pts',(-3.26319060600006,5.2,-2.45368347900001));
#319175=CARTESIAN_POINT('Ctrl Pts',(-3.26319060600006,2.2,-2.45368347900001));
#319176=CARTESIAN_POINT('Ctrl Pts',(-3.26224999000006,12.2,-2.45324515000001));
#319177=CARTESIAN_POINT('Ctrl Pts',(-3.26224999000006,5.2,-2.45324515000001));
#319178=CARTESIAN_POINT('Ctrl Pts',(-3.26224999000006,2.2,-2.45324515000001));
#319179=CARTESIAN_POINT('Ctrl Pts',(-3.26131482700006,12.2,-2.45280796500001));
#319180=CARTESIAN_POINT('Ctrl Pts',(-3.26131482700006,5.2,-2.45280796500001));
#319181=CARTESIAN_POINT('Ctrl Pts',(-3.26131482700006,2.2,-2.45280796500001));
#319182=CARTESIAN_POINT('Ctrl Pts',(-3.26038512300005,12.2,-2.45237194000001));
#319183=CARTESIAN_POINT('Ctrl Pts',(-3.26038512300005,5.2,-2.45237194000001));
#319184=CARTESIAN_POINT('Ctrl Pts',(-3.26038512300005,2.2,-2.45237194000001));
#319185=CARTESIAN_POINT('Ctrl Pts',(-3.25946087900005,12.2,-2.45193708800001));
#319186=CARTESIAN_POINT('Ctrl Pts',(-3.25946087900005,5.2,-2.45193708800001));
#319187=CARTESIAN_POINT('Ctrl Pts',(-3.25946087900005,2.2,-2.45193708800001));
#319188=CARTESIAN_POINT('Ctrl Pts',(-3.25854210200006,12.2,-2.45150342900001));
#319189=CARTESIAN_POINT('Ctrl Pts',(-3.25854210200006,5.2,-2.45150342900001));
#319190=CARTESIAN_POINT('Ctrl Pts',(-3.25854210200006,2.2,-2.45150342900001));
#319191=CARTESIAN_POINT('Ctrl Pts',(-3.25762879500005,12.2,-2.45107097800001));
#319192=CARTESIAN_POINT('Ctrl Pts',(-3.25762879500005,5.2,-2.45107097800001));
#319193=CARTESIAN_POINT('Ctrl Pts',(-3.25762879500005,2.2,-2.45107097800001));
#319194=CARTESIAN_POINT('Ctrl Pts',(-3.25672096200006,12.2,-2.45063974800001));
#319195=CARTESIAN_POINT('Ctrl Pts',(-3.25672096200006,5.2,-2.45063974800001));
#319196=CARTESIAN_POINT('Ctrl Pts',(-3.25672096200006,2.2,-2.45063974800001));
#319197=CARTESIAN_POINT('Ctrl Pts',(-3.25581860800006,12.2,-2.45020975800001));
#319198=CARTESIAN_POINT('Ctrl Pts',(-3.25581860800006,5.2,-2.45020975800001));
#319199=CARTESIAN_POINT('Ctrl Pts',(-3.25581860800006,2.2,-2.45020975800001));
#319200=CARTESIAN_POINT('Ctrl Pts',(-3.25492173600006,12.2,-2.44978102500002));
#319201=CARTESIAN_POINT('Ctrl Pts',(-3.25492173600006,5.2,-2.44978102500002));
#319202=CARTESIAN_POINT('Ctrl Pts',(-3.25492173600006,2.2,-2.44978102500002));
#319203=CARTESIAN_POINT('Ctrl Pts',(-3.25403035100006,12.2,-2.44935356300001));
#319204=CARTESIAN_POINT('Ctrl Pts',(-3.25403035100006,5.2,-2.44935356300001));
#319205=CARTESIAN_POINT('Ctrl Pts',(-3.25403035100006,2.2,-2.44935356300001));
#319206=CARTESIAN_POINT('Ctrl Pts',(-3.25314445700006,12.2,-2.44892738900001));
#319207=CARTESIAN_POINT('Ctrl Pts',(-3.25314445700006,5.2,-2.44892738900001));
#319208=CARTESIAN_POINT('Ctrl Pts',(-3.25314445700006,2.2,-2.44892738900001));
#319209=CARTESIAN_POINT('Ctrl Pts',(-3.25226405800006,12.2,-2.44850251900001));
#319210=CARTESIAN_POINT('Ctrl Pts',(-3.25226405800006,5.2,-2.44850251900001));
#319211=CARTESIAN_POINT('Ctrl Pts',(-3.25226405800006,2.2,-2.44850251900001));
#319212=CARTESIAN_POINT('Ctrl Pts',(-3.25138915700005,12.2,-2.44807896900001));
#319213=CARTESIAN_POINT('Ctrl Pts',(-3.25138915700005,5.2,-2.44807896900001));
#319214=CARTESIAN_POINT('Ctrl Pts',(-3.25138915700005,2.2,-2.44807896900001));
#319215=CARTESIAN_POINT('Ctrl Pts',(-3.25051976000006,12.2,-2.44765675600001));
#319216=CARTESIAN_POINT('Ctrl Pts',(-3.25051976000006,5.2,-2.44765675600001));
#319217=CARTESIAN_POINT('Ctrl Pts',(-3.25051976000006,2.2,-2.44765675600001));
#319218=CARTESIAN_POINT('Ctrl Pts',(-3.24965587200006,12.2,-2.44723589800001));
#319219=CARTESIAN_POINT('Ctrl Pts',(-3.24965587200006,5.2,-2.44723589800001));
#319220=CARTESIAN_POINT('Ctrl Pts',(-3.24965587200006,2.2,-2.44723589800001));
#319221=CARTESIAN_POINT('Ctrl Pts',(-3.24879749300006,12.2,-2.44681640900001));
#319222=CARTESIAN_POINT('Ctrl Pts',(-3.24879749300006,5.2,-2.44681640900001));
#319223=CARTESIAN_POINT('Ctrl Pts',(-3.24879749300006,2.2,-2.44681640900001));
#319224=CARTESIAN_POINT('Ctrl Pts',(-3.24794462900006,12.2,-2.44639830600001));
#319225=CARTESIAN_POINT('Ctrl Pts',(-3.24794462900006,5.2,-2.44639830600001));
#319226=CARTESIAN_POINT('Ctrl Pts',(-3.24794462900006,2.2,-2.44639830600001));
#319227=CARTESIAN_POINT('Ctrl Pts',(-3.24709728600005,12.2,-2.44598160600002));
#319228=CARTESIAN_POINT('Ctrl Pts',(-3.24709728600005,5.2,-2.44598160600002));
#319229=CARTESIAN_POINT('Ctrl Pts',(-3.24709728600005,2.2,-2.44598160600002));
#319230=CARTESIAN_POINT('Ctrl Pts',(-3.24625546600006,12.2,-2.44556632600001));
#319231=CARTESIAN_POINT('Ctrl Pts',(-3.24625546600006,5.2,-2.44556632600001));
#319232=CARTESIAN_POINT('Ctrl Pts',(-3.24625546600006,2.2,-2.44556632600001));
#319233=CARTESIAN_POINT('Ctrl Pts',(-3.24541917300006,12.2,-2.44515248200001));
#319234=CARTESIAN_POINT('Ctrl Pts',(-3.24541917300006,5.2,-2.44515248200001));
#319235=CARTESIAN_POINT('Ctrl Pts',(-3.24541917300006,2.2,-2.44515248200001));
#319236=CARTESIAN_POINT('Ctrl Pts',(-3.24458841200005,12.2,-2.44474009200002));
#319237=CARTESIAN_POINT('Ctrl Pts',(-3.24458841200005,5.2,-2.44474009200002));
#319238=CARTESIAN_POINT('Ctrl Pts',(-3.24458841200005,2.2,-2.44474009200002));
#319239=CARTESIAN_POINT('Ctrl Pts',(-3.24376318700006,12.2,-2.44432917200001));
#319240=CARTESIAN_POINT('Ctrl Pts',(-3.24376318700006,5.2,-2.44432917200001));
#319241=CARTESIAN_POINT('Ctrl Pts',(-3.24376318700006,2.2,-2.44432917200001));
#319242=CARTESIAN_POINT('Ctrl Pts',(-3.24294350100006,12.2,-2.44391973700001));
#319243=CARTESIAN_POINT('Ctrl Pts',(-3.24294350100006,5.2,-2.44391973700001));
#319244=CARTESIAN_POINT('Ctrl Pts',(-3.24294350100006,2.2,-2.44391973700001));
#319245=CARTESIAN_POINT('Ctrl Pts',(-3.24212935800006,12.2,-2.44351180700002));
#319246=CARTESIAN_POINT('Ctrl Pts',(-3.24212935800006,5.2,-2.44351180700002));
#319247=CARTESIAN_POINT('Ctrl Pts',(-3.24212935800006,2.2,-2.44351180700002));
#319248=CARTESIAN_POINT('Ctrl Pts',(-3.24132076300006,12.2,-2.44310539600002));
#319249=CARTESIAN_POINT('Ctrl Pts',(-3.24132076300006,5.2,-2.44310539600002));
#319250=CARTESIAN_POINT('Ctrl Pts',(-3.24132076300006,2.2,-2.44310539600002));
#319251=CARTESIAN_POINT('Ctrl Pts',(-3.24051771900006,12.2,-2.44270052300001));
#319252=CARTESIAN_POINT('Ctrl Pts',(-3.24051771900006,5.2,-2.44270052300001));
#319253=CARTESIAN_POINT('Ctrl Pts',(-3.24051771900006,2.2,-2.44270052300001));
#319254=CARTESIAN_POINT('Ctrl Pts',(-3.23972023100006,12.2,-2.44229720500002));
#319255=CARTESIAN_POINT('Ctrl Pts',(-3.23972023100006,5.2,-2.44229720500002));
#319256=CARTESIAN_POINT('Ctrl Pts',(-3.23972023100006,2.2,-2.44229720500002));
#319257=CARTESIAN_POINT('Ctrl Pts',(-3.23892830200006,12.2,-2.44189545800001));
#319258=CARTESIAN_POINT('Ctrl Pts',(-3.23892830200006,5.2,-2.44189545800001));
#319259=CARTESIAN_POINT('Ctrl Pts',(-3.23892830200006,2.2,-2.44189545800001));
#319260=CARTESIAN_POINT('Ctrl Pts',(-3.23814193600006,12.2,-2.44149529900001));
#319261=CARTESIAN_POINT('Ctrl Pts',(-3.23814193600006,5.2,-2.44149529900001));
#319262=CARTESIAN_POINT('Ctrl Pts',(-3.23814193600006,2.2,-2.44149529900001));
#319263=CARTESIAN_POINT('Ctrl Pts',(-3.23736113700006,12.2,-2.44109674600002));
#319264=CARTESIAN_POINT('Ctrl Pts',(-3.23736113700006,5.2,-2.44109674600002));
#319265=CARTESIAN_POINT('Ctrl Pts',(-3.23736113700006,2.2,-2.44109674600002));
#319266=CARTESIAN_POINT('Ctrl Pts',(-3.23658590900005,12.2,-2.44069981600001));
#319267=CARTESIAN_POINT('Ctrl Pts',(-3.23658590900005,5.2,-2.44069981600001));
#319268=CARTESIAN_POINT('Ctrl Pts',(-3.23658590900005,2.2,-2.44069981600001));
#319269=CARTESIAN_POINT('Ctrl Pts',(-3.23581625600006,12.2,-2.44030452700001));
#319270=CARTESIAN_POINT('Ctrl Pts',(-3.23581625600006,5.2,-2.44030452700001));
#319271=CARTESIAN_POINT('Ctrl Pts',(-3.23581625600006,2.2,-2.44030452700001));
#319272=CARTESIAN_POINT('Ctrl Pts',(-3.23505218300005,12.2,-2.43991089400001));
#319273=CARTESIAN_POINT('Ctrl Pts',(-3.23505218300005,5.2,-2.43991089400001));
#319274=CARTESIAN_POINT('Ctrl Pts',(-3.23505218300005,2.2,-2.43991089400001));
#319275=CARTESIAN_POINT('Ctrl Pts',(-3.23429369200006,12.2,-2.43951893700002));
#319276=CARTESIAN_POINT('Ctrl Pts',(-3.23429369200006,5.2,-2.43951893700002));
#319277=CARTESIAN_POINT('Ctrl Pts',(-3.23429369200006,2.2,-2.43951893700002));
#319278=CARTESIAN_POINT('Ctrl Pts',(-3.23354078700006,12.2,-2.43912867200001));
#319279=CARTESIAN_POINT('Ctrl Pts',(-3.23354078700006,5.2,-2.43912867200001));
#319280=CARTESIAN_POINT('Ctrl Pts',(-3.23354078700006,2.2,-2.43912867200001));
#319281=CARTESIAN_POINT('Ctrl Pts',(-3.23279347300006,12.2,-2.43874011600001));
#319282=CARTESIAN_POINT('Ctrl Pts',(-3.23279347300006,5.2,-2.43874011600001));
#319283=CARTESIAN_POINT('Ctrl Pts',(-3.23279347300006,2.2,-2.43874011600001));
#319284=CARTESIAN_POINT('Ctrl Pts',(-3.23205175300005,12.2,-2.43835328900001));
#319285=CARTESIAN_POINT('Ctrl Pts',(-3.23205175300005,5.2,-2.43835328900001));
#319286=CARTESIAN_POINT('Ctrl Pts',(-3.23205175300005,2.2,-2.43835328900001));
#319287=CARTESIAN_POINT('Ctrl Pts',(-3.23131563100006,12.2,-2.43796820600001));
#319288=CARTESIAN_POINT('Ctrl Pts',(-3.23131563100006,5.2,-2.43796820600001));
#319289=CARTESIAN_POINT('Ctrl Pts',(-3.23131563100006,2.2,-2.43796820600001));
#319290=CARTESIAN_POINT('Ctrl Pts',(-3.23058511200006,12.2,-2.43758488500001));
#319291=CARTESIAN_POINT('Ctrl Pts',(-3.23058511200006,5.2,-2.43758488500001));
#319292=CARTESIAN_POINT('Ctrl Pts',(-3.23058511200006,2.2,-2.43758488500001));
#319293=CARTESIAN_POINT('Ctrl Pts',(-3.22986019800005,12.2,-2.43720334500001));
#319294=CARTESIAN_POINT('Ctrl Pts',(-3.22986019800005,5.2,-2.43720334500001));
#319295=CARTESIAN_POINT('Ctrl Pts',(-3.22986019800005,2.2,-2.43720334500001));
#319296=CARTESIAN_POINT('Ctrl Pts',(-3.22914089300005,12.2,-2.43682360200001));
#319297=CARTESIAN_POINT('Ctrl Pts',(-3.22914089300005,5.2,-2.43682360200001));
#319298=CARTESIAN_POINT('Ctrl Pts',(-3.22914089300005,2.2,-2.43682360200001));
#319299=CARTESIAN_POINT('Ctrl Pts',(-3.22842720200006,12.2,-2.43644567500001));
#319300=CARTESIAN_POINT('Ctrl Pts',(-3.22842720200006,5.2,-2.43644567500001));
#319301=CARTESIAN_POINT('Ctrl Pts',(-3.22842720200006,2.2,-2.43644567500001));
#319302=CARTESIAN_POINT('Ctrl Pts',(-3.22771912700006,12.2,-2.43606958200001));
#319303=CARTESIAN_POINT('Ctrl Pts',(-3.22771912700006,5.2,-2.43606958200001));
#319304=CARTESIAN_POINT('Ctrl Pts',(-3.22771912700006,2.2,-2.43606958200001));
#319305=CARTESIAN_POINT('Ctrl Pts',(-3.22701667400006,12.2,-2.43569534000001));
#319306=CARTESIAN_POINT('Ctrl Pts',(-3.22701667400006,5.2,-2.43569534000001));
#319307=CARTESIAN_POINT('Ctrl Pts',(-3.22701667400006,2.2,-2.43569534000001));
#319308=CARTESIAN_POINT('Ctrl Pts',(-3.22631984500005,12.2,-2.43532296700002));
#319309=CARTESIAN_POINT('Ctrl Pts',(-3.22631984500005,5.2,-2.43532296700002));
#319310=CARTESIAN_POINT('Ctrl Pts',(-3.22631984500005,2.2,-2.43532296700002));
#319311=CARTESIAN_POINT('Ctrl Pts',(-3.22562864500005,12.2,-2.43495248300002));
#319312=CARTESIAN_POINT('Ctrl Pts',(-3.22562864500005,5.2,-2.43495248300002));
#319313=CARTESIAN_POINT('Ctrl Pts',(-3.22562864500005,2.2,-2.43495248300002));
#319314=CARTESIAN_POINT('Ctrl Pts',(-3.22494307600006,12.2,-2.43458390200002));
#319315=CARTESIAN_POINT('Ctrl Pts',(-3.22494307600006,5.2,-2.43458390200002));
#319316=CARTESIAN_POINT('Ctrl Pts',(-3.22494307600006,2.2,-2.43458390200002));
#319317=CARTESIAN_POINT('Ctrl Pts',(-3.22426314400006,12.2,-2.43421724700001));
#319318=CARTESIAN_POINT('Ctrl Pts',(-3.22426314400006,5.2,-2.43421724700001));
#319319=CARTESIAN_POINT('Ctrl Pts',(-3.22426314400006,2.2,-2.43421724700001));
#319320=CARTESIAN_POINT('Ctrl Pts',(-3.22358885100006,12.2,-2.43385253200001));
#319321=CARTESIAN_POINT('Ctrl Pts',(-3.22358885100006,5.2,-2.43385253200001));
#319322=CARTESIAN_POINT('Ctrl Pts',(-3.22358885100006,2.2,-2.43385253200001));
#319323=CARTESIAN_POINT('Ctrl Pts',(-3.22292020000006,12.2,-2.43348977700002));
#319324=CARTESIAN_POINT('Ctrl Pts',(-3.22292020000006,5.2,-2.43348977700002));
#319325=CARTESIAN_POINT('Ctrl Pts',(-3.22292020000006,2.2,-2.43348977700002));
#319326=CARTESIAN_POINT('Ctrl Pts',(-3.22225719700006,12.2,-2.43312900100001));
#319327=CARTESIAN_POINT('Ctrl Pts',(-3.22225719700006,5.2,-2.43312900100001));
#319328=CARTESIAN_POINT('Ctrl Pts',(-3.22225719700006,2.2,-2.43312900100001));
#319329=CARTESIAN_POINT('Ctrl Pts',(-3.22159984400006,12.2,-2.43277022100001));
#319330=CARTESIAN_POINT('Ctrl Pts',(-3.22159984400006,5.2,-2.43277022100001));
#319331=CARTESIAN_POINT('Ctrl Pts',(-3.22159984400006,2.2,-2.43277022100001));
#319332=CARTESIAN_POINT('Ctrl Pts',(-3.22094814500006,12.2,-2.43241345700001));
#319333=CARTESIAN_POINT('Ctrl Pts',(-3.22094814500006,5.2,-2.43241345700001));
#319334=CARTESIAN_POINT('Ctrl Pts',(-3.22094814500006,2.2,-2.43241345700001));
#319335=CARTESIAN_POINT('Ctrl Pts',(-3.22030210500006,12.2,-2.43205872500001));
#319336=CARTESIAN_POINT('Ctrl Pts',(-3.22030210500006,5.2,-2.43205872500001));
#319337=CARTESIAN_POINT('Ctrl Pts',(-3.22030210500006,2.2,-2.43205872500001));
#319338=CARTESIAN_POINT('Ctrl Pts',(-3.21966172400006,12.2,-2.43170604600001));
#319339=CARTESIAN_POINT('Ctrl Pts',(-3.21966172400006,5.2,-2.43170604600001));
#319340=CARTESIAN_POINT('Ctrl Pts',(-3.21966172400006,2.2,-2.43170604600001));
#319341=CARTESIAN_POINT('Ctrl Pts',(-3.21902701000006,12.2,-2.43135543600001));
#319342=CARTESIAN_POINT('Ctrl Pts',(-3.21902701000006,5.2,-2.43135543600001));
#319343=CARTESIAN_POINT('Ctrl Pts',(-3.21902701000006,2.2,-2.43135543600001));
#319344=CARTESIAN_POINT('Ctrl Pts',(-3.21839796500006,12.2,-2.43100691700001));
#319345=CARTESIAN_POINT('Ctrl Pts',(-3.21839796500006,5.2,-2.43100691700001));
#319346=CARTESIAN_POINT('Ctrl Pts',(-3.21839796500006,2.2,-2.43100691700001));
#319347=CARTESIAN_POINT('Ctrl Pts',(-3.21777459100006,12.2,-2.43066050400001));
#319348=CARTESIAN_POINT('Ctrl Pts',(-3.21777459100006,5.2,-2.43066050400001));
#319349=CARTESIAN_POINT('Ctrl Pts',(-3.21777459100006,2.2,-2.43066050400001));
#319350=CARTESIAN_POINT('Ctrl Pts',(-3.21715689300006,12.2,-2.43031621800001));
#319351=CARTESIAN_POINT('Ctrl Pts',(-3.21715689300006,5.2,-2.43031621800001));
#319352=CARTESIAN_POINT('Ctrl Pts',(-3.21715689300006,2.2,-2.43031621800001));
#319353=CARTESIAN_POINT('Ctrl Pts',(-3.21654487500005,12.2,-2.42997407700001));
#319354=CARTESIAN_POINT('Ctrl Pts',(-3.21654487500005,5.2,-2.42997407700001));
#319355=CARTESIAN_POINT('Ctrl Pts',(-3.21654487500005,2.2,-2.42997407700001));
#319356=CARTESIAN_POINT('Ctrl Pts',(-3.21593853800006,12.2,-2.42963410000002));
#319357=CARTESIAN_POINT('Ctrl Pts',(-3.21593853800006,5.2,-2.42963410000002));
#319358=CARTESIAN_POINT('Ctrl Pts',(-3.21593853800006,2.2,-2.42963410000002));
#319359=CARTESIAN_POINT('Ctrl Pts',(-3.21533788800005,12.2,-2.42929630700001));
#319360=CARTESIAN_POINT('Ctrl Pts',(-3.21533788800005,5.2,-2.42929630700001));
#319361=CARTESIAN_POINT('Ctrl Pts',(-3.21533788800005,2.2,-2.42929630700001));
#319362=CARTESIAN_POINT('Ctrl Pts',(-3.21474292900006,12.2,-2.42896071500001));
#319363=CARTESIAN_POINT('Ctrl Pts',(-3.21474292900006,5.2,-2.42896071500001));
#319364=CARTESIAN_POINT('Ctrl Pts',(-3.21474292900006,2.2,-2.42896071500001));
#319365=CARTESIAN_POINT('Ctrl Pts',(-3.21415366400006,12.2,-2.42862734300001));
#319366=CARTESIAN_POINT('Ctrl Pts',(-3.21415366400006,5.2,-2.42862734300001));
#319367=CARTESIAN_POINT('Ctrl Pts',(-3.21415366400006,2.2,-2.42862734300001));
#319368=CARTESIAN_POINT('Ctrl Pts',(-3.21357009500006,12.2,-2.42829621200002));
#319369=CARTESIAN_POINT('Ctrl Pts',(-3.21357009500006,5.2,-2.42829621200002));
#319370=CARTESIAN_POINT('Ctrl Pts',(-3.21357009500006,2.2,-2.42829621200002));
#319371=CARTESIAN_POINT('Ctrl Pts',(-3.21299222700006,12.2,-2.42796734200001));
#319372=CARTESIAN_POINT('Ctrl Pts',(-3.21299222700006,5.2,-2.42796734200001));
#319373=CARTESIAN_POINT('Ctrl Pts',(-3.21299222700006,2.2,-2.42796734200001));
#319374=CARTESIAN_POINT('Ctrl Pts',(-3.21242006200006,12.2,-2.42764074800002));
#319375=CARTESIAN_POINT('Ctrl Pts',(-3.21242006200006,5.2,-2.42764074800002));
#319376=CARTESIAN_POINT('Ctrl Pts',(-3.21242006200006,2.2,-2.42764074800002));
#319377=CARTESIAN_POINT('Ctrl Pts',(-3.21185360400006,12.2,-2.42731645200001));
#319378=CARTESIAN_POINT('Ctrl Pts',(-3.21185360400006,5.2,-2.42731645200001));
#319379=CARTESIAN_POINT('Ctrl Pts',(-3.21185360400006,2.2,-2.42731645200001));
#319380=CARTESIAN_POINT('Ctrl Pts',(-3.21129285900006,12.2,-2.42699447300001));
#319381=CARTESIAN_POINT('Ctrl Pts',(-3.21129285900006,5.2,-2.42699447300001));
#319382=CARTESIAN_POINT('Ctrl Pts',(-3.21129285900006,2.2,-2.42699447300001));
#319383=CARTESIAN_POINT('Ctrl Pts',(-3.21073782700006,12.2,-2.42667483200002));
#319384=CARTESIAN_POINT('Ctrl Pts',(-3.21073782700006,5.2,-2.42667483200002));
#319385=CARTESIAN_POINT('Ctrl Pts',(-3.21073782700006,2.2,-2.42667483200002));
#319386=CARTESIAN_POINT('Ctrl Pts',(-3.21018851300006,12.2,-2.42635754500002));
#319387=CARTESIAN_POINT('Ctrl Pts',(-3.21018851300006,5.2,-2.42635754500002));
#319388=CARTESIAN_POINT('Ctrl Pts',(-3.21018851300006,2.2,-2.42635754500002));
#319389=CARTESIAN_POINT('Ctrl Pts',(-3.20964491900006,12.2,-2.42604263400001));
#319390=CARTESIAN_POINT('Ctrl Pts',(-3.20964491900006,5.2,-2.42604263400001));
#319391=CARTESIAN_POINT('Ctrl Pts',(-3.20964491900006,2.2,-2.42604263400001));
#319392=CARTESIAN_POINT('Ctrl Pts',(-3.20910705000006,12.2,-2.42573011800001));
#319393=CARTESIAN_POINT('Ctrl Pts',(-3.20910705000006,5.2,-2.42573011800001));
#319394=CARTESIAN_POINT('Ctrl Pts',(-3.20910705000006,2.2,-2.42573011800001));
#319395=CARTESIAN_POINT('Ctrl Pts',(-3.20857491000006,12.2,-2.42542001600001));
#319396=CARTESIAN_POINT('Ctrl Pts',(-3.20857491000006,5.2,-2.42542001600001));
#319397=CARTESIAN_POINT('Ctrl Pts',(-3.20857491000006,2.2,-2.42542001600001));
#319398=CARTESIAN_POINT('Ctrl Pts',(-3.20804850000005,12.2,-2.42511234900002));
#319399=CARTESIAN_POINT('Ctrl Pts',(-3.20804850000005,5.2,-2.42511234900002));
#319400=CARTESIAN_POINT('Ctrl Pts',(-3.20804850000005,2.2,-2.42511234900002));
#319401=CARTESIAN_POINT('Ctrl Pts',(-3.20752782500006,12.2,-2.42480713400001));
#319402=CARTESIAN_POINT('Ctrl Pts',(-3.20752782500006,5.2,-2.42480713400001));
#319403=CARTESIAN_POINT('Ctrl Pts',(-3.20752782500006,2.2,-2.42480713400001));
#319404=CARTESIAN_POINT('Ctrl Pts',(-3.20701288800006,12.2,-2.42450439400002));
#319405=CARTESIAN_POINT('Ctrl Pts',(-3.20701288800006,5.2,-2.42450439400002));
#319406=CARTESIAN_POINT('Ctrl Pts',(-3.20701288800006,2.2,-2.42450439400002));
#319407=CARTESIAN_POINT('Ctrl Pts',(-3.20650369300005,12.2,-2.42420414800002));
#319408=CARTESIAN_POINT('Ctrl Pts',(-3.20650369300005,5.2,-2.42420414800002));
#319409=CARTESIAN_POINT('Ctrl Pts',(-3.20650369300005,2.2,-2.42420414800002));
#319410=CARTESIAN_POINT('Ctrl Pts',(-3.20600024200006,12.2,-2.42390641500001));
#319411=CARTESIAN_POINT('Ctrl Pts',(-3.20600024200006,5.2,-2.42390641500001));
#319412=CARTESIAN_POINT('Ctrl Pts',(-3.20600024200006,2.2,-2.42390641500001));
#319413=CARTESIAN_POINT('Ctrl Pts',(-3.20550253900006,12.2,-2.42361121600001));
#319414=CARTESIAN_POINT('Ctrl Pts',(-3.20550253900006,5.2,-2.42361121600001));
#319415=CARTESIAN_POINT('Ctrl Pts',(-3.20550253900006,2.2,-2.42361121600001));
#319416=CARTESIAN_POINT('Ctrl Pts',(-3.20501058600006,12.2,-2.42331857100002));
#319417=CARTESIAN_POINT('Ctrl Pts',(-3.20501058600006,5.2,-2.42331857100002));
#319418=CARTESIAN_POINT('Ctrl Pts',(-3.20501058600006,2.2,-2.42331857100002));
#319419=CARTESIAN_POINT('Ctrl Pts',(-3.20452438900006,12.2,-2.42302849900002));
#319420=CARTESIAN_POINT('Ctrl Pts',(-3.20452438900006,5.2,-2.42302849900002));
#319421=CARTESIAN_POINT('Ctrl Pts',(-3.20452438900006,2.2,-2.42302849900002));
#319422=CARTESIAN_POINT('Ctrl Pts',(-3.20404394900006,12.2,-2.42274102200001));
#319423=CARTESIAN_POINT('Ctrl Pts',(-3.20404394900006,5.2,-2.42274102200001));
#319424=CARTESIAN_POINT('Ctrl Pts',(-3.20404394900006,2.2,-2.42274102200001));
#319425=CARTESIAN_POINT('Ctrl Pts',(-3.20356926900006,12.2,-2.42245615800002));
#319426=CARTESIAN_POINT('Ctrl Pts',(-3.20356926900006,5.2,-2.42245615800002));
#319427=CARTESIAN_POINT('Ctrl Pts',(-3.20356926900006,2.2,-2.42245615800002));
#319428=CARTESIAN_POINT('Ctrl Pts',(-3.20310035500006,12.2,-2.42217393000002));
#319429=CARTESIAN_POINT('Ctrl Pts',(-3.20310035500006,5.2,-2.42217393000002));
#319430=CARTESIAN_POINT('Ctrl Pts',(-3.20310035500006,2.2,-2.42217393000002));
#319431=CARTESIAN_POINT('Ctrl Pts',(-3.20263720800006,12.2,-2.42189435600002));
#319432=CARTESIAN_POINT('Ctrl Pts',(-3.20263720800006,5.2,-2.42189435600002));
#319433=CARTESIAN_POINT('Ctrl Pts',(-3.20263720800006,2.2,-2.42189435600002));
#319434=CARTESIAN_POINT('Ctrl Pts',(-3.20217983100005,12.2,-2.42161745700002));
#319435=CARTESIAN_POINT('Ctrl Pts',(-3.20217983100005,5.2,-2.42161745700002));
#319436=CARTESIAN_POINT('Ctrl Pts',(-3.20217983100005,2.2,-2.42161745700002));
#319437=CARTESIAN_POINT('Ctrl Pts',(-3.20172822800005,12.2,-2.42134325500002));
#319438=CARTESIAN_POINT('Ctrl Pts',(-3.20172822800005,5.2,-2.42134325500002));
#319439=CARTESIAN_POINT('Ctrl Pts',(-3.20172822800005,2.2,-2.42134325500002));
#319440=CARTESIAN_POINT('Ctrl Pts',(-3.20128240200006,12.2,-2.42107177000001));
#319441=CARTESIAN_POINT('Ctrl Pts',(-3.20128240200006,5.2,-2.42107177000001));
#319442=CARTESIAN_POINT('Ctrl Pts',(-3.20128240200006,2.2,-2.42107177000001));
#319443=CARTESIAN_POINT('Ctrl Pts',(-3.20084235600006,12.2,-2.42080302100002));
#319444=CARTESIAN_POINT('Ctrl Pts',(-3.20084235600006,5.2,-2.42080302100002));
#319445=CARTESIAN_POINT('Ctrl Pts',(-3.20084235600006,2.2,-2.42080302100002));
#319446=CARTESIAN_POINT('Ctrl Pts',(-3.20040809300006,12.2,-2.42053703100002));
#319447=CARTESIAN_POINT('Ctrl Pts',(-3.20040809300006,5.2,-2.42053703100002));
#319448=CARTESIAN_POINT('Ctrl Pts',(-3.20040809300006,2.2,-2.42053703100002));
#319449=CARTESIAN_POINT('Ctrl Pts',(-3.19997961700006,12.2,-2.42027381900002));
#319450=CARTESIAN_POINT('Ctrl Pts',(-3.19997961700006,5.2,-2.42027381900002));
#319451=CARTESIAN_POINT('Ctrl Pts',(-3.19997961700006,2.2,-2.42027381900002));
#319452=CARTESIAN_POINT('Ctrl Pts',(-3.19955693100006,12.2,-2.42001340800002));
#319453=CARTESIAN_POINT('Ctrl Pts',(-3.19955693100006,5.2,-2.42001340800002));
#319454=CARTESIAN_POINT('Ctrl Pts',(-3.19955693100006,2.2,-2.42001340800002));
#319455=CARTESIAN_POINT('Ctrl Pts',(-3.19914003600006,12.2,-2.41975581600002));
#319456=CARTESIAN_POINT('Ctrl Pts',(-3.19914003600006,5.2,-2.41975581600002));
#319457=CARTESIAN_POINT('Ctrl Pts',(-3.19914003600006,2.2,-2.41975581600002));
#319458=CARTESIAN_POINT('Ctrl Pts',(-3.19872893800006,12.2,-2.41950106700001));
#319459=CARTESIAN_POINT('Ctrl Pts',(-3.19872893800006,5.2,-2.41950106700001));
#319460=CARTESIAN_POINT('Ctrl Pts',(-3.19872893800006,2.2,-2.41950106700001));
#319461=CARTESIAN_POINT('Ctrl Pts',(-3.19832363800006,12.2,-2.41924917900001));
#319462=CARTESIAN_POINT('Ctrl Pts',(-3.19832363800006,5.2,-2.41924917900001));
#319463=CARTESIAN_POINT('Ctrl Pts',(-3.19832363800006,2.2,-2.41924917900001));
#319464=CARTESIAN_POINT('Ctrl Pts',(-3.19792414100006,12.2,-2.41900017700001));
#319465=CARTESIAN_POINT('Ctrl Pts',(-3.19792414100006,5.2,-2.41900017700001));
#319466=CARTESIAN_POINT('Ctrl Pts',(-3.19792414100006,2.2,-2.41900017700001));
#319467=CARTESIAN_POINT('Ctrl Pts',(-3.19753044800006,12.2,-2.41875407900002));
#319468=CARTESIAN_POINT('Ctrl Pts',(-3.19753044800006,5.2,-2.41875407900002));
#319469=CARTESIAN_POINT('Ctrl Pts',(-3.19753044800006,2.2,-2.41875407900002));
#319470=CARTESIAN_POINT('Ctrl Pts',(-3.19714256200006,12.2,-2.41851090700001));
#319471=CARTESIAN_POINT('Ctrl Pts',(-3.19714256200006,5.2,-2.41851090700001));
#319472=CARTESIAN_POINT('Ctrl Pts',(-3.19714256200006,2.2,-2.41851090700001));
#319473=CARTESIAN_POINT('Ctrl Pts',(-3.19676048800006,12.2,-2.41827068400001));
#319474=CARTESIAN_POINT('Ctrl Pts',(-3.19676048800006,5.2,-2.41827068400001));
#319475=CARTESIAN_POINT('Ctrl Pts',(-3.19676048800006,2.2,-2.41827068400001));
#319476=CARTESIAN_POINT('Ctrl Pts',(-3.19638422800006,12.2,-2.41803342900001));
#319477=CARTESIAN_POINT('Ctrl Pts',(-3.19638422800006,5.2,-2.41803342900001));
#319478=CARTESIAN_POINT('Ctrl Pts',(-3.19638422800006,2.2,-2.41803342900001));
#319479=CARTESIAN_POINT('Ctrl Pts',(-3.19601378400006,12.2,-2.41779916600001));
#319480=CARTESIAN_POINT('Ctrl Pts',(-3.19601378400006,5.2,-2.41779916600001));
#319481=CARTESIAN_POINT('Ctrl Pts',(-3.19601378400006,2.2,-2.41779916600001));
#319482=CARTESIAN_POINT('Ctrl Pts',(-3.19564916000005,12.2,-2.41756791400002));
#319483=CARTESIAN_POINT('Ctrl Pts',(-3.19564916000005,5.2,-2.41756791400002));
#319484=CARTESIAN_POINT('Ctrl Pts',(-3.19564916000005,2.2,-2.41756791400002));
#319485=CARTESIAN_POINT('Ctrl Pts',(-3.19529036000006,12.2,-2.41733969700002));
#319486=CARTESIAN_POINT('Ctrl Pts',(-3.19529036000006,5.2,-2.41733969700002));
#319487=CARTESIAN_POINT('Ctrl Pts',(-3.19529036000006,2.2,-2.41733969700002));
#319488=CARTESIAN_POINT('Ctrl Pts',(-3.19493738400006,12.2,-2.41711453400002));
#319489=CARTESIAN_POINT('Ctrl Pts',(-3.19493738400006,5.2,-2.41711453400002));
#319490=CARTESIAN_POINT('Ctrl Pts',(-3.19493738400006,2.2,-2.41711453400002));
#319491=CARTESIAN_POINT('Ctrl Pts',(-3.19459023800006,12.2,-2.41689245000002));
#319492=CARTESIAN_POINT('Ctrl Pts',(-3.19459023800006,5.2,-2.41689245000002));
#319493=CARTESIAN_POINT('Ctrl Pts',(-3.19459023800006,2.2,-2.41689245000002));
#319494=CARTESIAN_POINT('Ctrl Pts',(-3.19424892300006,12.2,-2.41667346500002));
#319495=CARTESIAN_POINT('Ctrl Pts',(-3.19424892300006,5.2,-2.41667346500002));
#319496=CARTESIAN_POINT('Ctrl Pts',(-3.19424892300006,2.2,-2.41667346500002));
#319497=CARTESIAN_POINT('Ctrl Pts',(-3.19391344200006,12.2,-2.41645760200001));
#319498=CARTESIAN_POINT('Ctrl Pts',(-3.19391344200006,5.2,-2.41645760200001));
#319499=CARTESIAN_POINT('Ctrl Pts',(-3.19391344200006,2.2,-2.41645760200001));
#319500=CARTESIAN_POINT('Ctrl Pts',(-3.19358379900006,12.2,-2.41624488100001));
#319501=CARTESIAN_POINT('Ctrl Pts',(-3.19358379900006,5.2,-2.41624488100001));
#319502=CARTESIAN_POINT('Ctrl Pts',(-3.19358379900006,2.2,-2.41624488100001));
#319503=CARTESIAN_POINT('Ctrl Pts',(-3.19325999500006,12.2,-2.41603532600001));
#319504=CARTESIAN_POINT('Ctrl Pts',(-3.19325999500006,5.2,-2.41603532600001));
#319505=CARTESIAN_POINT('Ctrl Pts',(-3.19325999500006,2.2,-2.41603532600001));
#319506=CARTESIAN_POINT('Ctrl Pts',(-3.19294203600006,12.2,-2.41582895800001));
#319507=CARTESIAN_POINT('Ctrl Pts',(-3.19294203600006,5.2,-2.41582895800001));
#319508=CARTESIAN_POINT('Ctrl Pts',(-3.19294203600006,2.2,-2.41582895800001));
#319509=CARTESIAN_POINT('Ctrl Pts',(-3.19262992100006,12.2,-2.41562580100001));
#319510=CARTESIAN_POINT('Ctrl Pts',(-3.19262992100006,5.2,-2.41562580100001));
#319511=CARTESIAN_POINT('Ctrl Pts',(-3.19262992100006,2.2,-2.41562580100001));
#319512=CARTESIAN_POINT('Ctrl Pts',(-3.19232365500006,12.2,-2.41542587600001));
#319513=CARTESIAN_POINT('Ctrl Pts',(-3.19232365500006,5.2,-2.41542587600001));
#319514=CARTESIAN_POINT('Ctrl Pts',(-3.19232365500006,2.2,-2.41542587600001));
#319515=CARTESIAN_POINT('Ctrl Pts',(-3.19202324000006,12.2,-2.41522920400001));
#319516=CARTESIAN_POINT('Ctrl Pts',(-3.19202324000006,5.2,-2.41522920400001));
#319517=CARTESIAN_POINT('Ctrl Pts',(-3.19202324000006,2.2,-2.41522920400001));
#319518=CARTESIAN_POINT('Ctrl Pts',(-3.19172868100006,12.2,-2.41503581100002));
#319519=CARTESIAN_POINT('Ctrl Pts',(-3.19172868100006,5.2,-2.41503581100002));
#319520=CARTESIAN_POINT('Ctrl Pts',(-3.19172868100006,2.2,-2.41503581100002));
#319521=CARTESIAN_POINT('Ctrl Pts',(-3.19143997700006,12.2,-2.41484571600001));
#319522=CARTESIAN_POINT('Ctrl Pts',(-3.19143997700006,5.2,-2.41484571600001));
#319523=CARTESIAN_POINT('Ctrl Pts',(-3.19143997700006,2.2,-2.41484571600001));
#319524=CARTESIAN_POINT('Ctrl Pts',(-3.19115713300006,12.2,-2.41465894400001));
#319525=CARTESIAN_POINT('Ctrl Pts',(-3.19115713300006,5.2,-2.41465894400001));
#319526=CARTESIAN_POINT('Ctrl Pts',(-3.19115713300006,2.2,-2.41465894400001));
#319527=CARTESIAN_POINT('Ctrl Pts',(-3.19088015200006,12.2,-2.41447551700002));
#319528=CARTESIAN_POINT('Ctrl Pts',(-3.19088015200006,5.2,-2.41447551700002));
#319529=CARTESIAN_POINT('Ctrl Pts',(-3.19088015200006,2.2,-2.41447551700002));
#319530=CARTESIAN_POINT('Ctrl Pts',(-3.19060903600006,12.2,-2.41429545800001));
#319531=CARTESIAN_POINT('Ctrl Pts',(-3.19060903600006,5.2,-2.41429545800001));
#319532=CARTESIAN_POINT('Ctrl Pts',(-3.19060903600006,2.2,-2.41429545800001));
#319533=CARTESIAN_POINT('Ctrl Pts',(-3.19034378700006,12.2,-2.41411878900001));
#319534=CARTESIAN_POINT('Ctrl Pts',(-3.19034378700006,5.2,-2.41411878900001));
#319535=CARTESIAN_POINT('Ctrl Pts',(-3.19034378700006,2.2,-2.41411878900001));
#319536=CARTESIAN_POINT('Ctrl Pts',(-3.19008441000005,12.2,-2.41394553400001));
#319537=CARTESIAN_POINT('Ctrl Pts',(-3.19008441000005,5.2,-2.41394553400001));
#319538=CARTESIAN_POINT('Ctrl Pts',(-3.19008441000005,2.2,-2.41394553400001));
#319539=CARTESIAN_POINT('Ctrl Pts',(-3.18983090500006,12.2,-2.41377571600002));
#319540=CARTESIAN_POINT('Ctrl Pts',(-3.18983090500006,5.2,-2.41377571600002));
#319541=CARTESIAN_POINT('Ctrl Pts',(-3.18983090500006,2.2,-2.41377571600002));
#319542=CARTESIAN_POINT('Ctrl Pts',(-3.18958327600006,12.2,-2.41360935700001));
#319543=CARTESIAN_POINT('Ctrl Pts',(-3.18958327600006,5.2,-2.41360935700001));
#319544=CARTESIAN_POINT('Ctrl Pts',(-3.18958327600006,2.2,-2.41360935700001));
#319545=CARTESIAN_POINT('Ctrl Pts',(-3.18934152500006,12.2,-2.41344648100001));
#319546=CARTESIAN_POINT('Ctrl Pts',(-3.18934152500006,5.2,-2.41344648100001));
#319547=CARTESIAN_POINT('Ctrl Pts',(-3.18934152500006,2.2,-2.41344648100001));
#319548=CARTESIAN_POINT('Ctrl Pts',(-3.18910565500006,12.2,-2.41328711200001));
#319549=CARTESIAN_POINT('Ctrl Pts',(-3.18910565500006,5.2,-2.41328711200001));
#319550=CARTESIAN_POINT('Ctrl Pts',(-3.18910565500006,2.2,-2.41328711200001));
#319551=CARTESIAN_POINT('Ctrl Pts',(-3.18887567000006,12.2,-2.41313127200002));
#319552=CARTESIAN_POINT('Ctrl Pts',(-3.18887567000006,5.2,-2.41313127200002));
#319553=CARTESIAN_POINT('Ctrl Pts',(-3.18887567000006,2.2,-2.41313127200002));
#319554=CARTESIAN_POINT('Ctrl Pts',(-3.18865157000006,12.2,-2.41297898500001));
#319555=CARTESIAN_POINT('Ctrl Pts',(-3.18865157000006,5.2,-2.41297898500001));
#319556=CARTESIAN_POINT('Ctrl Pts',(-3.18865157000006,2.2,-2.41297898500001));
#319557=CARTESIAN_POINT('Ctrl Pts',(-3.18843335800006,12.2,-2.41283027500002));
#319558=CARTESIAN_POINT('Ctrl Pts',(-3.18843335800006,5.2,-2.41283027500002));
#319559=CARTESIAN_POINT('Ctrl Pts',(-3.18843335800006,2.2,-2.41283027500002));
#319560=CARTESIAN_POINT('Ctrl Pts',(-3.18822103800006,12.2,-2.41268516500002));
#319561=CARTESIAN_POINT('Ctrl Pts',(-3.18822103800006,5.2,-2.41268516500002));
#319562=CARTESIAN_POINT('Ctrl Pts',(-3.18822103800006,2.2,-2.41268516500002));
#319563=CARTESIAN_POINT('Ctrl Pts',(-3.18801461200006,12.2,-2.41254367900002));
#319564=CARTESIAN_POINT('Ctrl Pts',(-3.18801461200006,5.2,-2.41254367900002));
#319565=CARTESIAN_POINT('Ctrl Pts',(-3.18801461200006,2.2,-2.41254367900002));
#319566=CARTESIAN_POINT('Ctrl Pts',(-3.18781408200006,12.2,-2.41240584100002));
#319567=CARTESIAN_POINT('Ctrl Pts',(-3.18781408200006,5.2,-2.41240584100002));
#319568=CARTESIAN_POINT('Ctrl Pts',(-3.18781408200006,2.2,-2.41240584100002));
#319569=CARTESIAN_POINT('Ctrl Pts',(-3.18761945100006,12.2,-2.41227167400002));
#319570=CARTESIAN_POINT('Ctrl Pts',(-3.18761945100006,5.2,-2.41227167400002));
#319571=CARTESIAN_POINT('Ctrl Pts',(-3.18761945100006,2.2,-2.41227167400002));
#319572=CARTESIAN_POINT('Ctrl Pts',(-3.18743072200005,12.2,-2.41214120200001));
#319573=CARTESIAN_POINT('Ctrl Pts',(-3.18743072200005,5.2,-2.41214120200001));
#319574=CARTESIAN_POINT('Ctrl Pts',(-3.18743072200005,2.2,-2.41214120200001));
#319575=CARTESIAN_POINT('Ctrl Pts',(-3.18724789400005,12.2,-2.41201445000002));
#319576=CARTESIAN_POINT('Ctrl Pts',(-3.18724789400005,5.2,-2.41201445000002));
#319577=CARTESIAN_POINT('Ctrl Pts',(-3.18724789400005,2.2,-2.41201445000002));
#319578=CARTESIAN_POINT('Ctrl Pts',(-3.18707097400006,12.2,-2.41189144200002));
#319579=CARTESIAN_POINT('Ctrl Pts',(-3.18707097400006,5.2,-2.41189144200002));
#319580=CARTESIAN_POINT('Ctrl Pts',(-3.18707097400006,2.2,-2.41189144200002));
#319581=CARTESIAN_POINT('Ctrl Pts',(-3.18689996300006,12.2,-2.41177220100001));
#319582=CARTESIAN_POINT('Ctrl Pts',(-3.18689996300006,5.2,-2.41177220100001));
#319583=CARTESIAN_POINT('Ctrl Pts',(-3.18689996300006,2.2,-2.41177220100001));
#319584=CARTESIAN_POINT('Ctrl Pts',(-3.18673486200006,12.2,-2.41165675300001));
#319585=CARTESIAN_POINT('Ctrl Pts',(-3.18673486200006,5.2,-2.41165675300001));
#319586=CARTESIAN_POINT('Ctrl Pts',(-3.18673486200006,2.2,-2.41165675300001));
#319587=CARTESIAN_POINT('Ctrl Pts',(-3.18657567500006,12.2,-2.41154512200001));
#319588=CARTESIAN_POINT('Ctrl Pts',(-3.18657567500006,5.2,-2.41154512200001));
#319589=CARTESIAN_POINT('Ctrl Pts',(-3.18657567500006,2.2,-2.41154512200001));
#319590=CARTESIAN_POINT('Ctrl Pts',(-3.18642240300006,12.2,-2.41143733200001));
#319591=CARTESIAN_POINT('Ctrl Pts',(-3.18642240300006,5.2,-2.41143733200001));
#319592=CARTESIAN_POINT('Ctrl Pts',(-3.18642240300006,2.2,-2.41143733200001));
#319593=CARTESIAN_POINT('Ctrl Pts',(-3.18627504900005,12.2,-2.41133340900001));
#319594=CARTESIAN_POINT('Ctrl Pts',(-3.18627504900005,5.2,-2.41133340900001));
#319595=CARTESIAN_POINT('Ctrl Pts',(-3.18627504900005,2.2,-2.41133340900001));
#319596=CARTESIAN_POINT('Ctrl Pts',(-3.18613361600006,12.2,-2.41123337500001));
#319597=CARTESIAN_POINT('Ctrl Pts',(-3.18613361600006,5.2,-2.41123337500001));
#319598=CARTESIAN_POINT('Ctrl Pts',(-3.18613361600006,2.2,-2.41123337500001));
#319599=CARTESIAN_POINT('Ctrl Pts',(-3.18599810500006,12.2,-2.41113725500002));
#319600=CARTESIAN_POINT('Ctrl Pts',(-3.18599810500006,5.2,-2.41113725500002));
#319601=CARTESIAN_POINT('Ctrl Pts',(-3.18599810500006,2.2,-2.41113725500002));
#319602=CARTESIAN_POINT('Ctrl Pts',(-3.18586851800006,12.2,-2.41104507300001));
#319603=CARTESIAN_POINT('Ctrl Pts',(-3.18586851800006,5.2,-2.41104507300001));
#319604=CARTESIAN_POINT('Ctrl Pts',(-3.18586851800006,2.2,-2.41104507300001));
#319605=CARTESIAN_POINT('Ctrl Pts',(-3.18574485900006,12.2,-2.41095685700001));
#319606=CARTESIAN_POINT('Ctrl Pts',(-3.18574485900006,5.2,-2.41095685700001));
#319607=CARTESIAN_POINT('Ctrl Pts',(-3.18574485900006,2.2,-2.41095685700001));
#319608=CARTESIAN_POINT('Ctrl Pts',(-3.18562713000006,12.2,-2.41087263100002));
#319609=CARTESIAN_POINT('Ctrl Pts',(-3.18562713000006,5.2,-2.41087263100002));
#319610=CARTESIAN_POINT('Ctrl Pts',(-3.18562713000006,2.2,-2.41087263100002));
#319611=CARTESIAN_POINT('Ctrl Pts',(-3.18551533200006,12.2,-2.41079242200001));
#319612=CARTESIAN_POINT('Ctrl Pts',(-3.18551533200006,5.2,-2.41079242200001));
#319613=CARTESIAN_POINT('Ctrl Pts',(-3.18551533200006,2.2,-2.41079242200001));
#319614=CARTESIAN_POINT('Ctrl Pts',(-3.18540946800006,12.2,-2.41071625600001));
#319615=CARTESIAN_POINT('Ctrl Pts',(-3.18540946800006,5.2,-2.41071625600001));
#319616=CARTESIAN_POINT('Ctrl Pts',(-3.18540946800006,2.2,-2.41071625600001));
#319617=CARTESIAN_POINT('Ctrl Pts',(-3.18530953900006,12.2,-2.41064415700002));
#319618=CARTESIAN_POINT('Ctrl Pts',(-3.18530953900006,5.2,-2.41064415700002));
#319619=CARTESIAN_POINT('Ctrl Pts',(-3.18530953900006,2.2,-2.41064415700002));
#319620=CARTESIAN_POINT('Ctrl Pts',(-3.18521554900005,12.2,-2.41057614800001));
#319621=CARTESIAN_POINT('Ctrl Pts',(-3.18521554900005,5.2,-2.41057614800001));
#319622=CARTESIAN_POINT('Ctrl Pts',(-3.18521554900005,2.2,-2.41057614800001));
#319623=CARTESIAN_POINT('Ctrl Pts',(-3.18512750000005,12.2,-2.41051225300001));
#319624=CARTESIAN_POINT('Ctrl Pts',(-3.18512750000005,5.2,-2.41051225300001));
#319625=CARTESIAN_POINT('Ctrl Pts',(-3.18512750000005,2.2,-2.41051225300001));
#319626=CARTESIAN_POINT('Ctrl Pts',(-3.18504539300006,12.2,-2.41045249400001));
#319627=CARTESIAN_POINT('Ctrl Pts',(-3.18504539300006,5.2,-2.41045249400001));
#319628=CARTESIAN_POINT('Ctrl Pts',(-3.18504539300006,2.2,-2.41045249400001));
#319629=CARTESIAN_POINT('Ctrl Pts',(-3.18496922900006,12.2,-2.41039689700001));
#319630=CARTESIAN_POINT('Ctrl Pts',(-3.18496922900006,5.2,-2.41039689700001));
#319631=CARTESIAN_POINT('Ctrl Pts',(-3.18496922900006,2.2,-2.41039689700001));
#319632=CARTESIAN_POINT('Ctrl Pts',(-3.18489901200006,12.2,-2.41034549400001));
#319633=CARTESIAN_POINT('Ctrl Pts',(-3.18489901200006,5.2,-2.41034549400001));
#319634=CARTESIAN_POINT('Ctrl Pts',(-3.18489901200006,2.2,-2.41034549400001));
#319635=CARTESIAN_POINT('Ctrl Pts',(-3.18483474500006,12.2,-2.41029831500001));
#319636=CARTESIAN_POINT('Ctrl Pts',(-3.18483474500006,5.2,-2.41029831500001));
#319637=CARTESIAN_POINT('Ctrl Pts',(-3.18483474500006,2.2,-2.41029831500001));
#319638=CARTESIAN_POINT('Ctrl Pts',(-3.18477642900006,12.2,-2.41025539300002));
#319639=CARTESIAN_POINT('Ctrl Pts',(-3.18477642900006,5.2,-2.41025539300002));
#319640=CARTESIAN_POINT('Ctrl Pts',(-3.18477642900006,2.2,-2.41025539300002));
#319641=CARTESIAN_POINT('Ctrl Pts',(-3.18472406700006,12.2,-2.41021675800001));
#319642=CARTESIAN_POINT('Ctrl Pts',(-3.18472406700006,5.2,-2.41021675800001));
#319643=CARTESIAN_POINT('Ctrl Pts',(-3.18472406700006,2.2,-2.41021675800001));
#319644=CARTESIAN_POINT('Ctrl Pts',(-3.18467766000006,12.2,-2.41018243000001));
#319645=CARTESIAN_POINT('Ctrl Pts',(-3.18467766000006,5.2,-2.41018243000001));
#319646=CARTESIAN_POINT('Ctrl Pts',(-3.18467766000006,2.2,-2.41018243000001));
#319647=CARTESIAN_POINT('Ctrl Pts',(-3.18463288082923,12.2,-2.41014921067249));
#319648=CARTESIAN_POINT('Ctrl Pts',(-3.18463288082923,5.2,-2.41014921067249));
#319649=CARTESIAN_POINT('Ctrl Pts',(-3.18463288082923,2.2,-2.41014921067249));
#319650=CARTESIAN_POINT('Ctrl Pts',(-3.18460231601978,12.2,-2.41012644147867));
#319651=CARTESIAN_POINT('Ctrl Pts',(-3.18460231601978,5.2,-2.41012644147867));
#319652=CARTESIAN_POINT('Ctrl Pts',(-3.18460231601978,2.2,-2.41012644147867));
#319653=CARTESIAN_POINT('Ctrl Pts',(-3.18458221430919,12.2,-2.41011139784499));
#319654=CARTESIAN_POINT('Ctrl Pts',(-3.18458221430919,5.2,-2.41011139784499));
#319655=CARTESIAN_POINT('Ctrl Pts',(-3.18458221430919,2.2,-2.41011139784499));
#319656=CARTESIAN_POINT('Ctrl Pts',(-3.18456971176712,12.2,-2.41010199879104));
#319657=CARTESIAN_POINT('Ctrl Pts',(-3.18456971176712,5.2,-2.41010199879104));
#319658=CARTESIAN_POINT('Ctrl Pts',(-3.18456971176712,2.2,-2.41010199879104));
#319659=CARTESIAN_POINT('Ctrl Pts',(-3.18456199000006,12.2,-2.41009620000002));
#319660=CARTESIAN_POINT('Ctrl Pts',(-3.18456199000006,5.2,-2.41009620000002));
#319661=CARTESIAN_POINT('Ctrl Pts',(-3.18456199000006,2.2,-2.41009620000002));
#319662=CARTESIAN_POINT('',(-3.18456186900006,2.7,-2.41009636100001));
#319663=CARTESIAN_POINT('',(-3.18456186900006,12.2,-2.41009636100001));
#319664=CARTESIAN_POINT('Ctrl Pts',(-3.98353538000006,2.7,-2.58726610100001));
#319665=CARTESIAN_POINT('Ctrl Pts',(-3.72873002607504,2.7,-2.58625929211275));
#319666=CARTESIAN_POINT('Ctrl Pts',(-3.54026174963293,2.69999999999094,
-2.54811998493994));
#319667=CARTESIAN_POINT('Ctrl Pts',(-3.26663347427495,2.69999999999094,
-2.46586464912604));
#319668=CARTESIAN_POINT('Ctrl Pts',(-3.19489970037899,2.69999999999544,
-2.41765563987494));
#319669=CARTESIAN_POINT('Ctrl Pts',(-3.18483344867918,2.69999999999544,
-2.4102976087089));
#319670=CARTESIAN_POINT('Ctrl Pts',(-3.18469713278844,2.7,-2.41019768775304));
#319671=CARTESIAN_POINT('Ctrl Pts',(-3.18456199000006,2.7,-2.41009620000002));
#319672=CARTESIAN_POINT('Origin',(-3.18452095000006,15.2,-2.41006539300002));
#319673=CARTESIAN_POINT('',(-2.89052929200006,2.7,-2.18757066500002));
#319674=CARTESIAN_POINT('',(-2.89052929200006,2.2,-2.18757066500002));
#319675=CARTESIAN_POINT('',(-1.59226047414512,2.7,-1.20503269762968));
#319676=CARTESIAN_POINT('Origin',(-5.66300478732629E-14,15.2,-1.77635683940025E-14));
#319677=CARTESIAN_POINT('',(-2.51818288300006,2.7,-2.60756207400001));
#319678=CARTESIAN_POINT('',(-2.51818288300006,12.2,-2.60756207400001));
#319679=CARTESIAN_POINT('Origin',(-5.66300478732629E-14,2.7,-1.92943768261394E-14));
#319680=CARTESIAN_POINT('Origin',(-5.66300478732629E-14,15.2,-1.77635683940025E-14));
#319681=CARTESIAN_POINT('',(-2.77432748000006,2.7,-2.87279814400002));
#319682=CARTESIAN_POINT('',(-2.77432748000006,12.2,-2.87279814400001));
#319683=CARTESIAN_POINT('',(-5.6232279645039E-14,2.7,-1.88824904010619E-14));
#319684=CARTESIAN_POINT('Ctrl Pts',(-2.77432738100006,12.2,-2.87279823800001));
#319685=CARTESIAN_POINT('Ctrl Pts',(-2.77432738100006,5.2,-2.87279823800001));
#319686=CARTESIAN_POINT('Ctrl Pts',(-2.77432738100006,2.2,-2.87279823800001));
#319687=CARTESIAN_POINT('Ctrl Pts',(-2.77433211472047,12.2,-2.87280317870827));
#319688=CARTESIAN_POINT('Ctrl Pts',(-2.77433211472047,5.2,-2.87280317870827));
#319689=CARTESIAN_POINT('Ctrl Pts',(-2.77433211472047,2.2,-2.87280317870827));
#319690=CARTESIAN_POINT('Ctrl Pts',(-2.77434127117772,12.2,-2.87281273360882));
#319691=CARTESIAN_POINT('Ctrl Pts',(-2.77434127117772,5.2,-2.87281273360882));
#319692=CARTESIAN_POINT('Ctrl Pts',(-2.77434127117772,2.2,-2.87281273360882));
#319693=CARTESIAN_POINT('Ctrl Pts',(-2.77435485557306,12.2,-2.87282690333949));
#319694=CARTESIAN_POINT('Ctrl Pts',(-2.77435485557306,5.2,-2.87282690333949));
#319695=CARTESIAN_POINT('Ctrl Pts',(-2.77435485557306,2.2,-2.87282690333949));
#319696=CARTESIAN_POINT('Ctrl Pts',(-2.77437283287678,12.2,-2.8728456878981));
#319697=CARTESIAN_POINT('Ctrl Pts',(-2.77437283287678,5.2,-2.8728456878981));
#319698=CARTESIAN_POINT('Ctrl Pts',(-2.77437283287678,2.2,-2.8728456878981));
#319699=CARTESIAN_POINT('Ctrl Pts',(-2.77440404800006,12.2,-2.87287852900001));
#319700=CARTESIAN_POINT('Ctrl Pts',(-2.77440404800006,5.2,-2.87287852900001));
#319701=CARTESIAN_POINT('Ctrl Pts',(-2.77440404800006,2.2,-2.87287852900001));
#319702=CARTESIAN_POINT('Ctrl Pts',(-2.77443868700006,12.2,-2.87291509200001));
#319703=CARTESIAN_POINT('Ctrl Pts',(-2.77443868700006,5.2,-2.87291509200001));
#319704=CARTESIAN_POINT('Ctrl Pts',(-2.77443868700006,2.2,-2.87291509200001));
#319705=CARTESIAN_POINT('Ctrl Pts',(-2.77447832800005,12.2,-2.87295705000002));
#319706=CARTESIAN_POINT('Ctrl Pts',(-2.77447832800005,5.2,-2.87295705000002));
#319707=CARTESIAN_POINT('Ctrl Pts',(-2.77447832800005,2.2,-2.87295705000002));
#319708=CARTESIAN_POINT('Ctrl Pts',(-2.77452295900006,12.2,-2.87300440500001));
#319709=CARTESIAN_POINT('Ctrl Pts',(-2.77452295900006,5.2,-2.87300440500001));
#319710=CARTESIAN_POINT('Ctrl Pts',(-2.77452295900006,2.2,-2.87300440500001));
#319711=CARTESIAN_POINT('Ctrl Pts',(-2.77457255900006,12.2,-2.87305715700001));
#319712=CARTESIAN_POINT('Ctrl Pts',(-2.77457255900006,5.2,-2.87305715700001));
#319713=CARTESIAN_POINT('Ctrl Pts',(-2.77457255900006,2.2,-2.87305715700001));
#319714=CARTESIAN_POINT('Ctrl Pts',(-2.77462709900006,12.2,-2.87311530900002));
#319715=CARTESIAN_POINT('Ctrl Pts',(-2.77462709900006,5.2,-2.87311530900002));
#319716=CARTESIAN_POINT('Ctrl Pts',(-2.77462709900006,2.2,-2.87311530900002));
#319717=CARTESIAN_POINT('Ctrl Pts',(-2.77468654700006,12.2,-2.87317886000002));
#319718=CARTESIAN_POINT('Ctrl Pts',(-2.77468654700006,5.2,-2.87317886000002));
#319719=CARTESIAN_POINT('Ctrl Pts',(-2.77468654700006,2.2,-2.87317886000002));
#319720=CARTESIAN_POINT('Ctrl Pts',(-2.77475087000006,12.2,-2.87324781200001));
#319721=CARTESIAN_POINT('Ctrl Pts',(-2.77475087000006,5.2,-2.87324781200001));
#319722=CARTESIAN_POINT('Ctrl Pts',(-2.77475087000006,2.2,-2.87324781200001));
#319723=CARTESIAN_POINT('Ctrl Pts',(-2.77482003700006,12.2,-2.87332216700001));
#319724=CARTESIAN_POINT('Ctrl Pts',(-2.77482003700006,5.2,-2.87332216700001));
#319725=CARTESIAN_POINT('Ctrl Pts',(-2.77482003700006,2.2,-2.87332216700001));
#319726=CARTESIAN_POINT('Ctrl Pts',(-2.77489402300006,12.2,-2.87340192500002));
#319727=CARTESIAN_POINT('Ctrl Pts',(-2.77489402300006,5.2,-2.87340192500002));
#319728=CARTESIAN_POINT('Ctrl Pts',(-2.77489402300006,2.2,-2.87340192500002));
#319729=CARTESIAN_POINT('Ctrl Pts',(-2.77497280400006,12.2,-2.87348708800002));
#319730=CARTESIAN_POINT('Ctrl Pts',(-2.77497280400006,5.2,-2.87348708800002));
#319731=CARTESIAN_POINT('Ctrl Pts',(-2.77497280400006,2.2,-2.87348708800002));
#319732=CARTESIAN_POINT('Ctrl Pts',(-2.77505635800006,12.2,-2.87357765600001));
#319733=CARTESIAN_POINT('Ctrl Pts',(-2.77505635800006,5.2,-2.87357765600001));
#319734=CARTESIAN_POINT('Ctrl Pts',(-2.77505635800006,2.2,-2.87357765600001));
#319735=CARTESIAN_POINT('Ctrl Pts',(-2.77514466100006,12.2,-2.87367363100001));
#319736=CARTESIAN_POINT('Ctrl Pts',(-2.77514466100006,5.2,-2.87367363100001));
#319737=CARTESIAN_POINT('Ctrl Pts',(-2.77514466100006,2.2,-2.87367363100001));
#319738=CARTESIAN_POINT('Ctrl Pts',(-2.77523769000006,12.2,-2.87377501100002));
#319739=CARTESIAN_POINT('Ctrl Pts',(-2.77523769000006,5.2,-2.87377501100002));
#319740=CARTESIAN_POINT('Ctrl Pts',(-2.77523769000006,2.2,-2.87377501100002));
#319741=CARTESIAN_POINT('Ctrl Pts',(-2.77533541600006,12.2,-2.87388180000002));
#319742=CARTESIAN_POINT('Ctrl Pts',(-2.77533541600006,5.2,-2.87388180000002));
#319743=CARTESIAN_POINT('Ctrl Pts',(-2.77533541600006,2.2,-2.87388180000002));
#319744=CARTESIAN_POINT('Ctrl Pts',(-2.77543781500006,12.2,-2.87399399700002));
#319745=CARTESIAN_POINT('Ctrl Pts',(-2.77543781500006,5.2,-2.87399399700002));
#319746=CARTESIAN_POINT('Ctrl Pts',(-2.77543781500006,2.2,-2.87399399700002));
#319747=CARTESIAN_POINT('Ctrl Pts',(-2.77554486000006,12.2,-2.87411160400001));
#319748=CARTESIAN_POINT('Ctrl Pts',(-2.77554486000006,5.2,-2.87411160400001));
#319749=CARTESIAN_POINT('Ctrl Pts',(-2.77554486000006,2.2,-2.87411160400001));
#319750=CARTESIAN_POINT('Ctrl Pts',(-2.77565652600006,12.2,-2.87423462000001));
#319751=CARTESIAN_POINT('Ctrl Pts',(-2.77565652600006,5.2,-2.87423462000001));
#319752=CARTESIAN_POINT('Ctrl Pts',(-2.77565652600006,2.2,-2.87423462000001));
#319753=CARTESIAN_POINT('Ctrl Pts',(-2.77577278800006,12.2,-2.87436304800002));
#319754=CARTESIAN_POINT('Ctrl Pts',(-2.77577278800006,5.2,-2.87436304800002));
#319755=CARTESIAN_POINT('Ctrl Pts',(-2.77577278800006,2.2,-2.87436304800002));
#319756=CARTESIAN_POINT('Ctrl Pts',(-2.77589362000006,12.2,-2.87449688600002));
#319757=CARTESIAN_POINT('Ctrl Pts',(-2.77589362000006,5.2,-2.87449688600002));
#319758=CARTESIAN_POINT('Ctrl Pts',(-2.77589362000006,2.2,-2.87449688600002));
#319759=CARTESIAN_POINT('Ctrl Pts',(-2.77601899900006,12.2,-2.87463613700002));
#319760=CARTESIAN_POINT('Ctrl Pts',(-2.77601899900006,5.2,-2.87463613700002));
#319761=CARTESIAN_POINT('Ctrl Pts',(-2.77601899900006,2.2,-2.87463613700002));
#319762=CARTESIAN_POINT('Ctrl Pts',(-2.77614890100006,12.2,-2.87478080100001));
#319763=CARTESIAN_POINT('Ctrl Pts',(-2.77614890100006,5.2,-2.87478080100001));
#319764=CARTESIAN_POINT('Ctrl Pts',(-2.77614890100006,2.2,-2.87478080100001));
#319765=CARTESIAN_POINT('Ctrl Pts',(-2.77628330200006,12.2,-2.87493087700001));
#319766=CARTESIAN_POINT('Ctrl Pts',(-2.77628330200006,5.2,-2.87493087700001));
#319767=CARTESIAN_POINT('Ctrl Pts',(-2.77628330200006,2.2,-2.87493087700001));
#319768=CARTESIAN_POINT('Ctrl Pts',(-2.77642217600006,12.2,-2.87508636800001));
#319769=CARTESIAN_POINT('Ctrl Pts',(-2.77642217600006,5.2,-2.87508636800001));
#319770=CARTESIAN_POINT('Ctrl Pts',(-2.77642217600006,2.2,-2.87508636800001));
#319771=CARTESIAN_POINT('Ctrl Pts',(-2.77656549900006,12.2,-2.87524727300001));
#319772=CARTESIAN_POINT('Ctrl Pts',(-2.77656549900006,5.2,-2.87524727300001));
#319773=CARTESIAN_POINT('Ctrl Pts',(-2.77656549900006,2.2,-2.87524727300001));
#319774=CARTESIAN_POINT('Ctrl Pts',(-2.77671324600006,12.2,-2.87541359300001));
#319775=CARTESIAN_POINT('Ctrl Pts',(-2.77671324600006,5.2,-2.87541359300001));
#319776=CARTESIAN_POINT('Ctrl Pts',(-2.77671324600006,2.2,-2.87541359300001));
#319777=CARTESIAN_POINT('Ctrl Pts',(-2.77686539300006,12.2,-2.87558532900002));
#319778=CARTESIAN_POINT('Ctrl Pts',(-2.77686539300006,5.2,-2.87558532900002));
#319779=CARTESIAN_POINT('Ctrl Pts',(-2.77686539300006,2.2,-2.87558532900002));
#319780=CARTESIAN_POINT('Ctrl Pts',(-2.77702191600006,12.2,-2.87576248100001));
#319781=CARTESIAN_POINT('Ctrl Pts',(-2.77702191600006,5.2,-2.87576248100001));
#319782=CARTESIAN_POINT('Ctrl Pts',(-2.77702191600006,2.2,-2.87576248100001));
#319783=CARTESIAN_POINT('Ctrl Pts',(-2.77718279000006,12.2,-2.87594504800001));
#319784=CARTESIAN_POINT('Ctrl Pts',(-2.77718279000006,5.2,-2.87594504800001));
#319785=CARTESIAN_POINT('Ctrl Pts',(-2.77718279000006,2.2,-2.87594504800001));
#319786=CARTESIAN_POINT('Ctrl Pts',(-2.77734799400006,12.2,-2.87613303200001));
#319787=CARTESIAN_POINT('Ctrl Pts',(-2.77734799400006,5.2,-2.87613303200001));
#319788=CARTESIAN_POINT('Ctrl Pts',(-2.77734799400006,2.2,-2.87613303200001));
#319789=CARTESIAN_POINT('Ctrl Pts',(-2.77751750000006,12.2,-2.87632643300002));
#319790=CARTESIAN_POINT('Ctrl Pts',(-2.77751750000006,5.2,-2.87632643300002));
#319791=CARTESIAN_POINT('Ctrl Pts',(-2.77751750000006,2.2,-2.87632643300002));
#319792=CARTESIAN_POINT('Ctrl Pts',(-2.77769128800006,12.2,-2.87652525200001));
#319793=CARTESIAN_POINT('Ctrl Pts',(-2.77769128800006,5.2,-2.87652525200001));
#319794=CARTESIAN_POINT('Ctrl Pts',(-2.77769128800006,2.2,-2.87652525200001));
#319795=CARTESIAN_POINT('Ctrl Pts',(-2.77786933100006,12.2,-2.87672948900001));
#319796=CARTESIAN_POINT('Ctrl Pts',(-2.77786933100006,5.2,-2.87672948900001));
#319797=CARTESIAN_POINT('Ctrl Pts',(-2.77786933100006,2.2,-2.87672948900001));
#319798=CARTESIAN_POINT('Ctrl Pts',(-2.77805160800006,12.2,-2.87693914300001));
#319799=CARTESIAN_POINT('Ctrl Pts',(-2.77805160800006,5.2,-2.87693914300001));
#319800=CARTESIAN_POINT('Ctrl Pts',(-2.77805160800006,2.2,-2.87693914300001));
#319801=CARTESIAN_POINT('Ctrl Pts',(-2.77823809300005,12.2,-2.87715421600002));
#319802=CARTESIAN_POINT('Ctrl Pts',(-2.77823809300005,5.2,-2.87715421600002));
#319803=CARTESIAN_POINT('Ctrl Pts',(-2.77823809300005,2.2,-2.87715421600002));
#319804=CARTESIAN_POINT('Ctrl Pts',(-2.77842876500006,12.2,-2.87737470600002));
#319805=CARTESIAN_POINT('Ctrl Pts',(-2.77842876500006,5.2,-2.87737470600002));
#319806=CARTESIAN_POINT('Ctrl Pts',(-2.77842876500006,2.2,-2.87737470600002));
#319807=CARTESIAN_POINT('Ctrl Pts',(-2.77862359800006,12.2,-2.87760061600002));
#319808=CARTESIAN_POINT('Ctrl Pts',(-2.77862359800006,5.2,-2.87760061600002));
#319809=CARTESIAN_POINT('Ctrl Pts',(-2.77862359800006,2.2,-2.87760061600002));
#319810=CARTESIAN_POINT('Ctrl Pts',(-2.77882257000006,12.2,-2.87783194500001));
#319811=CARTESIAN_POINT('Ctrl Pts',(-2.77882257000006,5.2,-2.87783194500001));
#319812=CARTESIAN_POINT('Ctrl Pts',(-2.77882257000006,2.2,-2.87783194500001));
#319813=CARTESIAN_POINT('Ctrl Pts',(-2.77902565900006,12.2,-2.87806869300002));
#319814=CARTESIAN_POINT('Ctrl Pts',(-2.77902565900006,5.2,-2.87806869300002));
#319815=CARTESIAN_POINT('Ctrl Pts',(-2.77902565900006,2.2,-2.87806869300002));
#319816=CARTESIAN_POINT('Ctrl Pts',(-2.77923283900006,12.2,-2.87831085900002));
#319817=CARTESIAN_POINT('Ctrl Pts',(-2.77923283900006,5.2,-2.87831085900002));
#319818=CARTESIAN_POINT('Ctrl Pts',(-2.77923283900006,2.2,-2.87831085900002));
#319819=CARTESIAN_POINT('Ctrl Pts',(-2.77944409000006,12.2,-2.87855844500001));
#319820=CARTESIAN_POINT('Ctrl Pts',(-2.77944409000006,5.2,-2.87855844500001));
#319821=CARTESIAN_POINT('Ctrl Pts',(-2.77944409000006,2.2,-2.87855844500001));
#319822=CARTESIAN_POINT('Ctrl Pts',(-2.77965938600006,12.2,-2.87881145000001));
#319823=CARTESIAN_POINT('Ctrl Pts',(-2.77965938600006,5.2,-2.87881145000001));
#319824=CARTESIAN_POINT('Ctrl Pts',(-2.77965938600006,2.2,-2.87881145000001));
#319825=CARTESIAN_POINT('Ctrl Pts',(-2.77987870500006,12.2,-2.87906987400001));
#319826=CARTESIAN_POINT('Ctrl Pts',(-2.77987870500006,5.2,-2.87906987400001));
#319827=CARTESIAN_POINT('Ctrl Pts',(-2.77987870500006,2.2,-2.87906987400001));
#319828=CARTESIAN_POINT('Ctrl Pts',(-2.78010202600006,12.2,-2.87933371800001));
#319829=CARTESIAN_POINT('Ctrl Pts',(-2.78010202600006,5.2,-2.87933371800001));
#319830=CARTESIAN_POINT('Ctrl Pts',(-2.78010202600006,2.2,-2.87933371800001));
#319831=CARTESIAN_POINT('Ctrl Pts',(-2.78032932400006,12.2,-2.87960298100002));
#319832=CARTESIAN_POINT('Ctrl Pts',(-2.78032932400006,5.2,-2.87960298100002));
#319833=CARTESIAN_POINT('Ctrl Pts',(-2.78032932400006,2.2,-2.87960298100002));
#319834=CARTESIAN_POINT('Ctrl Pts',(-2.78056057600006,12.2,-2.87987766400001));
#319835=CARTESIAN_POINT('Ctrl Pts',(-2.78056057600006,5.2,-2.87987766400001));
#319836=CARTESIAN_POINT('Ctrl Pts',(-2.78056057600006,2.2,-2.87987766400001));
#319837=CARTESIAN_POINT('Ctrl Pts',(-2.78079576200006,12.2,-2.88015776600002));
#319838=CARTESIAN_POINT('Ctrl Pts',(-2.78079576200006,5.2,-2.88015776600002));
#319839=CARTESIAN_POINT('Ctrl Pts',(-2.78079576200006,2.2,-2.88015776600002));
#319840=CARTESIAN_POINT('Ctrl Pts',(-2.78103485600006,12.2,-2.88044328600002));
#319841=CARTESIAN_POINT('Ctrl Pts',(-2.78103485600006,5.2,-2.88044328600002));
#319842=CARTESIAN_POINT('Ctrl Pts',(-2.78103485600006,2.2,-2.88044328600002));
#319843=CARTESIAN_POINT('Ctrl Pts',(-2.78127783800006,12.2,-2.88073422700001));
#319844=CARTESIAN_POINT('Ctrl Pts',(-2.78127783800006,5.2,-2.88073422700001));
#319845=CARTESIAN_POINT('Ctrl Pts',(-2.78127783800006,2.2,-2.88073422700001));
#319846=CARTESIAN_POINT('Ctrl Pts',(-2.78152468400005,12.2,-2.88103058500001));
#319847=CARTESIAN_POINT('Ctrl Pts',(-2.78152468400005,5.2,-2.88103058500001));
#319848=CARTESIAN_POINT('Ctrl Pts',(-2.78152468400005,2.2,-2.88103058500001));
#319849=CARTESIAN_POINT('Ctrl Pts',(-2.78177537400006,12.2,-2.88133236300002));
#319850=CARTESIAN_POINT('Ctrl Pts',(-2.78177537400006,5.2,-2.88133236300002));
#319851=CARTESIAN_POINT('Ctrl Pts',(-2.78177537400006,2.2,-2.88133236300002));
#319852=CARTESIAN_POINT('Ctrl Pts',(-2.78202988300006,12.2,-2.88163955900002));
#319853=CARTESIAN_POINT('Ctrl Pts',(-2.78202988300006,5.2,-2.88163955900002));
#319854=CARTESIAN_POINT('Ctrl Pts',(-2.78202988300006,2.2,-2.88163955900002));
#319855=CARTESIAN_POINT('Ctrl Pts',(-2.78228819100006,12.2,-2.88195217300002));
#319856=CARTESIAN_POINT('Ctrl Pts',(-2.78228819100006,5.2,-2.88195217300002));
#319857=CARTESIAN_POINT('Ctrl Pts',(-2.78228819100006,2.2,-2.88195217300002));
#319858=CARTESIAN_POINT('Ctrl Pts',(-2.78255027400005,12.2,-2.88227020500001));
#319859=CARTESIAN_POINT('Ctrl Pts',(-2.78255027400005,5.2,-2.88227020500001));
#319860=CARTESIAN_POINT('Ctrl Pts',(-2.78255027400005,2.2,-2.88227020500001));
#319861=CARTESIAN_POINT('Ctrl Pts',(-2.78281611000006,12.2,-2.88259365600001));
#319862=CARTESIAN_POINT('Ctrl Pts',(-2.78281611000006,5.2,-2.88259365600001));
#319863=CARTESIAN_POINT('Ctrl Pts',(-2.78281611000006,2.2,-2.88259365600001));
#319864=CARTESIAN_POINT('Ctrl Pts',(-2.78308567900006,12.2,-2.88292252400002));
#319865=CARTESIAN_POINT('Ctrl Pts',(-2.78308567900006,5.2,-2.88292252400002));
#319866=CARTESIAN_POINT('Ctrl Pts',(-2.78308567900006,2.2,-2.88292252400002));
#319867=CARTESIAN_POINT('Ctrl Pts',(-2.78335895700006,12.2,-2.88325680900002));
#319868=CARTESIAN_POINT('Ctrl Pts',(-2.78335895700006,5.2,-2.88325680900002));
#319869=CARTESIAN_POINT('Ctrl Pts',(-2.78335895700006,2.2,-2.88325680900002));
#319870=CARTESIAN_POINT('Ctrl Pts',(-2.78363592400006,12.2,-2.88359651200001));
#319871=CARTESIAN_POINT('Ctrl Pts',(-2.78363592400006,5.2,-2.88359651200001));
#319872=CARTESIAN_POINT('Ctrl Pts',(-2.78363592400006,2.2,-2.88359651200001));
#319873=CARTESIAN_POINT('Ctrl Pts',(-2.78391655600006,12.2,-2.88394163000001));
#319874=CARTESIAN_POINT('Ctrl Pts',(-2.78391655600006,5.2,-2.88394163000001));
#319875=CARTESIAN_POINT('Ctrl Pts',(-2.78391655600006,2.2,-2.88394163000001));
#319876=CARTESIAN_POINT('Ctrl Pts',(-2.78420083300006,12.2,-2.88429216500001));
#319877=CARTESIAN_POINT('Ctrl Pts',(-2.78420083300006,5.2,-2.88429216500001));
#319878=CARTESIAN_POINT('Ctrl Pts',(-2.78420083300006,2.2,-2.88429216500001));
#319879=CARTESIAN_POINT('Ctrl Pts',(-2.78448873300006,12.2,-2.88464811600001));
#319880=CARTESIAN_POINT('Ctrl Pts',(-2.78448873300006,5.2,-2.88464811600001));
#319881=CARTESIAN_POINT('Ctrl Pts',(-2.78448873300006,2.2,-2.88464811600001));
#319882=CARTESIAN_POINT('Ctrl Pts',(-2.78478023400006,12.2,-2.88500948100001));
#319883=CARTESIAN_POINT('Ctrl Pts',(-2.78478023400006,5.2,-2.88500948100001));
#319884=CARTESIAN_POINT('Ctrl Pts',(-2.78478023400006,2.2,-2.88500948100001));
#319885=CARTESIAN_POINT('Ctrl Pts',(-2.78507531500006,12.2,-2.88537626300001));
#319886=CARTESIAN_POINT('Ctrl Pts',(-2.78507531500006,5.2,-2.88537626300001));
#319887=CARTESIAN_POINT('Ctrl Pts',(-2.78507531500006,2.2,-2.88537626300001));
#319888=CARTESIAN_POINT('Ctrl Pts',(-2.78537395400006,12.2,-2.88574845800001));
#319889=CARTESIAN_POINT('Ctrl Pts',(-2.78537395400006,5.2,-2.88574845800001));
#319890=CARTESIAN_POINT('Ctrl Pts',(-2.78537395400006,2.2,-2.88574845800001));
#319891=CARTESIAN_POINT('Ctrl Pts',(-2.78567613100006,12.2,-2.88612606700001));
#319892=CARTESIAN_POINT('Ctrl Pts',(-2.78567613100006,5.2,-2.88612606700001));
#319893=CARTESIAN_POINT('Ctrl Pts',(-2.78567613100006,2.2,-2.88612606700001));
#319894=CARTESIAN_POINT('Ctrl Pts',(-2.78598182300006,12.2,-2.88650909000001));
#319895=CARTESIAN_POINT('Ctrl Pts',(-2.78598182300006,5.2,-2.88650909000001));
#319896=CARTESIAN_POINT('Ctrl Pts',(-2.78598182300006,2.2,-2.88650909000001));
#319897=CARTESIAN_POINT('Ctrl Pts',(-2.78629100900006,12.2,-2.88689752600002));
#319898=CARTESIAN_POINT('Ctrl Pts',(-2.78629100900006,5.2,-2.88689752600002));
#319899=CARTESIAN_POINT('Ctrl Pts',(-2.78629100900006,2.2,-2.88689752600002));
#319900=CARTESIAN_POINT('Ctrl Pts',(-2.78660366900006,12.2,-2.88729137400002));
#319901=CARTESIAN_POINT('Ctrl Pts',(-2.78660366900006,5.2,-2.88729137400002));
#319902=CARTESIAN_POINT('Ctrl Pts',(-2.78660366900006,2.2,-2.88729137400002));
#319903=CARTESIAN_POINT('Ctrl Pts',(-2.78691978100006,12.2,-2.88769063300002));
#319904=CARTESIAN_POINT('Ctrl Pts',(-2.78691978100006,5.2,-2.88769063300002));
#319905=CARTESIAN_POINT('Ctrl Pts',(-2.78691978100006,2.2,-2.88769063300002));
#319906=CARTESIAN_POINT('Ctrl Pts',(-2.78723932300006,12.2,-2.88809530300002));
#319907=CARTESIAN_POINT('Ctrl Pts',(-2.78723932300006,5.2,-2.88809530300002));
#319908=CARTESIAN_POINT('Ctrl Pts',(-2.78723932300006,2.2,-2.88809530300002));
#319909=CARTESIAN_POINT('Ctrl Pts',(-2.78756227700006,12.2,-2.88850538500002));
#319910=CARTESIAN_POINT('Ctrl Pts',(-2.78756227700006,5.2,-2.88850538500002));
#319911=CARTESIAN_POINT('Ctrl Pts',(-2.78756227700006,2.2,-2.88850538500002));
#319912=CARTESIAN_POINT('Ctrl Pts',(-2.78788861900006,12.2,-2.88892087500002));
#319913=CARTESIAN_POINT('Ctrl Pts',(-2.78788861900006,5.2,-2.88892087500002));
#319914=CARTESIAN_POINT('Ctrl Pts',(-2.78788861900006,2.2,-2.88892087500002));
#319915=CARTESIAN_POINT('Ctrl Pts',(-2.78821833000006,12.2,-2.88934177600002));
#319916=CARTESIAN_POINT('Ctrl Pts',(-2.78821833000006,5.2,-2.88934177600002));
#319917=CARTESIAN_POINT('Ctrl Pts',(-2.78821833000006,2.2,-2.88934177600002));
#319918=CARTESIAN_POINT('Ctrl Pts',(-2.78855138900005,12.2,-2.88976808400002));
#319919=CARTESIAN_POINT('Ctrl Pts',(-2.78855138900005,5.2,-2.88976808400002));
#319920=CARTESIAN_POINT('Ctrl Pts',(-2.78855138900005,2.2,-2.88976808400002));
#319921=CARTESIAN_POINT('Ctrl Pts',(-2.78888777500006,12.2,-2.89019980000001));
#319922=CARTESIAN_POINT('Ctrl Pts',(-2.78888777500006,5.2,-2.89019980000001));
#319923=CARTESIAN_POINT('Ctrl Pts',(-2.78888777500006,2.2,-2.89019980000001));
#319924=CARTESIAN_POINT('Ctrl Pts',(-2.78922746700006,12.2,-2.89063692400001));
#319925=CARTESIAN_POINT('Ctrl Pts',(-2.78922746700006,5.2,-2.89063692400001));
#319926=CARTESIAN_POINT('Ctrl Pts',(-2.78922746700006,2.2,-2.89063692400001));
#319927=CARTESIAN_POINT('Ctrl Pts',(-2.78957044400005,12.2,-2.89107945200001));
#319928=CARTESIAN_POINT('Ctrl Pts',(-2.78957044400005,5.2,-2.89107945200001));
#319929=CARTESIAN_POINT('Ctrl Pts',(-2.78957044400005,2.2,-2.89107945200001));
#319930=CARTESIAN_POINT('Ctrl Pts',(-2.78991668800006,12.2,-2.89152738600002));
#319931=CARTESIAN_POINT('Ctrl Pts',(-2.78991668800006,5.2,-2.89152738600002));
#319932=CARTESIAN_POINT('Ctrl Pts',(-2.78991668800006,2.2,-2.89152738600002));
#319933=CARTESIAN_POINT('Ctrl Pts',(-2.79026617500006,12.2,-2.89198072600001));
#319934=CARTESIAN_POINT('Ctrl Pts',(-2.79026617500006,5.2,-2.89198072600001));
#319935=CARTESIAN_POINT('Ctrl Pts',(-2.79026617500006,2.2,-2.89198072600001));
#319936=CARTESIAN_POINT('Ctrl Pts',(-2.79061888800006,12.2,-2.89243946900001));
#319937=CARTESIAN_POINT('Ctrl Pts',(-2.79061888800006,5.2,-2.89243946900001));
#319938=CARTESIAN_POINT('Ctrl Pts',(-2.79061888800006,2.2,-2.89243946900001));
#319939=CARTESIAN_POINT('Ctrl Pts',(-2.79097480400006,12.2,-2.89290361400001));
#319940=CARTESIAN_POINT('Ctrl Pts',(-2.79097480400006,5.2,-2.89290361400001));
#319941=CARTESIAN_POINT('Ctrl Pts',(-2.79097480400006,2.2,-2.89290361400001));
#319942=CARTESIAN_POINT('Ctrl Pts',(-2.79133390500005,12.2,-2.89337316200001));
#319943=CARTESIAN_POINT('Ctrl Pts',(-2.79133390500005,5.2,-2.89337316200001));
#319944=CARTESIAN_POINT('Ctrl Pts',(-2.79133390500005,2.2,-2.89337316200001));
#319945=CARTESIAN_POINT('Ctrl Pts',(-2.79169616900006,12.2,-2.89384811200001));
#319946=CARTESIAN_POINT('Ctrl Pts',(-2.79169616900006,5.2,-2.89384811200001));
#319947=CARTESIAN_POINT('Ctrl Pts',(-2.79169616900006,2.2,-2.89384811200001));
#319948=CARTESIAN_POINT('Ctrl Pts',(-2.79206157600006,12.2,-2.89432846000001));
#319949=CARTESIAN_POINT('Ctrl Pts',(-2.79206157600006,5.2,-2.89432846000001));
#319950=CARTESIAN_POINT('Ctrl Pts',(-2.79206157600006,2.2,-2.89432846000001));
#319951=CARTESIAN_POINT('Ctrl Pts',(-2.79243010700006,12.2,-2.89481420900001));
#319952=CARTESIAN_POINT('Ctrl Pts',(-2.79243010700006,5.2,-2.89481420900001));
#319953=CARTESIAN_POINT('Ctrl Pts',(-2.79243010700006,2.2,-2.89481420900001));
#319954=CARTESIAN_POINT('Ctrl Pts',(-2.79280174100006,12.2,-2.89530535500001));
#319955=CARTESIAN_POINT('Ctrl Pts',(-2.79280174100006,5.2,-2.89530535500001));
#319956=CARTESIAN_POINT('Ctrl Pts',(-2.79280174100006,2.2,-2.89530535500001));
#319957=CARTESIAN_POINT('Ctrl Pts',(-2.79317645900006,12.2,-2.89580189800001));
#319958=CARTESIAN_POINT('Ctrl Pts',(-2.79317645900006,5.2,-2.89580189800001));
#319959=CARTESIAN_POINT('Ctrl Pts',(-2.79317645900006,2.2,-2.89580189800001));
#319960=CARTESIAN_POINT('Ctrl Pts',(-2.79355424000005,12.2,-2.89630383900001));
#319961=CARTESIAN_POINT('Ctrl Pts',(-2.79355424000005,5.2,-2.89630383900001));
#319962=CARTESIAN_POINT('Ctrl Pts',(-2.79355424000005,2.2,-2.89630383900001));
#319963=CARTESIAN_POINT('Ctrl Pts',(-2.79393506600006,12.2,-2.89681117400002));
#319964=CARTESIAN_POINT('Ctrl Pts',(-2.79393506600006,5.2,-2.89681117400002));
#319965=CARTESIAN_POINT('Ctrl Pts',(-2.79393506600006,2.2,-2.89681117400002));
#319966=CARTESIAN_POINT('Ctrl Pts',(-2.79431891500006,12.2,-2.89732390400002));
#319967=CARTESIAN_POINT('Ctrl Pts',(-2.79431891500006,5.2,-2.89732390400002));
#319968=CARTESIAN_POINT('Ctrl Pts',(-2.79431891500006,2.2,-2.89732390400002));
#319969=CARTESIAN_POINT('Ctrl Pts',(-2.79470576700006,12.2,-2.89784202700002));
#319970=CARTESIAN_POINT('Ctrl Pts',(-2.79470576700006,5.2,-2.89784202700002));
#319971=CARTESIAN_POINT('Ctrl Pts',(-2.79470576700006,2.2,-2.89784202700002));
#319972=CARTESIAN_POINT('Ctrl Pts',(-2.79509560600005,12.2,-2.89836554100001));
#319973=CARTESIAN_POINT('Ctrl Pts',(-2.79509560600005,5.2,-2.89836554100001));
#319974=CARTESIAN_POINT('Ctrl Pts',(-2.79509560600005,2.2,-2.89836554100001));
#319975=CARTESIAN_POINT('Ctrl Pts',(-2.79548840900006,12.2,-2.89889444600002));
#319976=CARTESIAN_POINT('Ctrl Pts',(-2.79548840900006,5.2,-2.89889444600002));
#319977=CARTESIAN_POINT('Ctrl Pts',(-2.79548840900006,2.2,-2.89889444600002));
#319978=CARTESIAN_POINT('Ctrl Pts',(-2.79588415700006,12.2,-2.89942874200001));
#319979=CARTESIAN_POINT('Ctrl Pts',(-2.79588415700006,5.2,-2.89942874200001));
#319980=CARTESIAN_POINT('Ctrl Pts',(-2.79588415700006,2.2,-2.89942874200001));
#319981=CARTESIAN_POINT('Ctrl Pts',(-2.79628283100006,12.2,-2.89996842600001));
#319982=CARTESIAN_POINT('Ctrl Pts',(-2.79628283100006,5.2,-2.89996842600001));
#319983=CARTESIAN_POINT('Ctrl Pts',(-2.79628283100006,2.2,-2.89996842600001));
#319984=CARTESIAN_POINT('Ctrl Pts',(-2.79668441300006,12.2,-2.90051349800001));
#319985=CARTESIAN_POINT('Ctrl Pts',(-2.79668441300006,5.2,-2.90051349800001));
#319986=CARTESIAN_POINT('Ctrl Pts',(-2.79668441300006,2.2,-2.90051349800001));
#319987=CARTESIAN_POINT('Ctrl Pts',(-2.79708888100005,12.2,-2.90106395600001));
#319988=CARTESIAN_POINT('Ctrl Pts',(-2.79708888100005,5.2,-2.90106395600001));
#319989=CARTESIAN_POINT('Ctrl Pts',(-2.79708888100005,2.2,-2.90106395600001));
#319990=CARTESIAN_POINT('Ctrl Pts',(-2.79749621700006,12.2,-2.90161979900001));
#319991=CARTESIAN_POINT('Ctrl Pts',(-2.79749621700006,5.2,-2.90161979900001));
#319992=CARTESIAN_POINT('Ctrl Pts',(-2.79749621700006,2.2,-2.90161979900001));
#319993=CARTESIAN_POINT('Ctrl Pts',(-2.79790640200006,12.2,-2.90218102600001));
#319994=CARTESIAN_POINT('Ctrl Pts',(-2.79790640200006,5.2,-2.90218102600001));
#319995=CARTESIAN_POINT('Ctrl Pts',(-2.79790640200006,2.2,-2.90218102600001));
#319996=CARTESIAN_POINT('Ctrl Pts',(-2.79831941600006,12.2,-2.90274763500001));
#319997=CARTESIAN_POINT('Ctrl Pts',(-2.79831941600006,5.2,-2.90274763500001));
#319998=CARTESIAN_POINT('Ctrl Pts',(-2.79831941600006,2.2,-2.90274763500001));
#319999=CARTESIAN_POINT('Ctrl Pts',(-2.79873524100006,12.2,-2.90331962600002));
#320000=CARTESIAN_POINT('Ctrl Pts',(-2.79873524100006,5.2,-2.90331962600002));
#320001=CARTESIAN_POINT('Ctrl Pts',(-2.79873524100006,2.2,-2.90331962600002));
#320002=CARTESIAN_POINT('Ctrl Pts',(-2.79915385700006,12.2,-2.90389699700001));
#320003=CARTESIAN_POINT('Ctrl Pts',(-2.79915385700006,5.2,-2.90389699700001));
#320004=CARTESIAN_POINT('Ctrl Pts',(-2.79915385700006,2.2,-2.90389699700001));
#320005=CARTESIAN_POINT('Ctrl Pts',(-2.79957524500006,12.2,-2.90447974700001));
#320006=CARTESIAN_POINT('Ctrl Pts',(-2.79957524500006,5.2,-2.90447974700001));
#320007=CARTESIAN_POINT('Ctrl Pts',(-2.79957524500006,2.2,-2.90447974700001));
#320008=CARTESIAN_POINT('Ctrl Pts',(-2.79999938600006,12.2,-2.90506787400002));
#320009=CARTESIAN_POINT('Ctrl Pts',(-2.79999938600006,5.2,-2.90506787400002));
#320010=CARTESIAN_POINT('Ctrl Pts',(-2.79999938600006,2.2,-2.90506787400002));
#320011=CARTESIAN_POINT('Ctrl Pts',(-2.80042626200005,12.2,-2.90566137700001));
#320012=CARTESIAN_POINT('Ctrl Pts',(-2.80042626200005,5.2,-2.90566137700001));
#320013=CARTESIAN_POINT('Ctrl Pts',(-2.80042626200005,2.2,-2.90566137700001));
#320014=CARTESIAN_POINT('Ctrl Pts',(-2.80085585300006,12.2,-2.90626025500002));
#320015=CARTESIAN_POINT('Ctrl Pts',(-2.80085585300006,5.2,-2.90626025500002));
#320016=CARTESIAN_POINT('Ctrl Pts',(-2.80085585300006,2.2,-2.90626025500002));
#320017=CARTESIAN_POINT('Ctrl Pts',(-2.80128814100005,12.2,-2.90686450600001));
#320018=CARTESIAN_POINT('Ctrl Pts',(-2.80128814100005,5.2,-2.90686450600001));
#320019=CARTESIAN_POINT('Ctrl Pts',(-2.80128814100005,2.2,-2.90686450600001));
#320020=CARTESIAN_POINT('Ctrl Pts',(-2.80172310700006,12.2,-2.90747412900001));
#320021=CARTESIAN_POINT('Ctrl Pts',(-2.80172310700006,5.2,-2.90747412900001));
#320022=CARTESIAN_POINT('Ctrl Pts',(-2.80172310700006,2.2,-2.90747412900001));
#320023=CARTESIAN_POINT('Ctrl Pts',(-2.80216073100005,12.2,-2.90808912300001));
#320024=CARTESIAN_POINT('Ctrl Pts',(-2.80216073100005,5.2,-2.90808912300001));
#320025=CARTESIAN_POINT('Ctrl Pts',(-2.80216073100005,2.2,-2.90808912300001));
#320026=CARTESIAN_POINT('Ctrl Pts',(-2.80260099700006,12.2,-2.90870948500002));
#320027=CARTESIAN_POINT('Ctrl Pts',(-2.80260099700006,5.2,-2.90870948500002));
#320028=CARTESIAN_POINT('Ctrl Pts',(-2.80260099700006,2.2,-2.90870948500002));
#320029=CARTESIAN_POINT('Ctrl Pts',(-2.80304388500006,12.2,-2.90933521600001));
#320030=CARTESIAN_POINT('Ctrl Pts',(-2.80304388500006,5.2,-2.90933521600001));
#320031=CARTESIAN_POINT('Ctrl Pts',(-2.80304388500006,2.2,-2.90933521600001));
#320032=CARTESIAN_POINT('Ctrl Pts',(-2.80348937700006,12.2,-2.90996631300001));
#320033=CARTESIAN_POINT('Ctrl Pts',(-2.80348937700006,5.2,-2.90996631300001));
#320034=CARTESIAN_POINT('Ctrl Pts',(-2.80348937700006,2.2,-2.90996631300001));
#320035=CARTESIAN_POINT('Ctrl Pts',(-2.80393745200006,12.2,-2.91060277400002));
#320036=CARTESIAN_POINT('Ctrl Pts',(-2.80393745200006,5.2,-2.91060277400002));
#320037=CARTESIAN_POINT('Ctrl Pts',(-2.80393745200006,2.2,-2.91060277400002));
#320038=CARTESIAN_POINT('Ctrl Pts',(-2.80438809600006,12.2,-2.91124459800002));
#320039=CARTESIAN_POINT('Ctrl Pts',(-2.80438809600006,5.2,-2.91124459800002));
#320040=CARTESIAN_POINT('Ctrl Pts',(-2.80438809600006,2.2,-2.91124459800002));
#320041=CARTESIAN_POINT('Ctrl Pts',(-2.80484128600006,12.2,-2.91189178400002));
#320042=CARTESIAN_POINT('Ctrl Pts',(-2.80484128600006,5.2,-2.91189178400002));
#320043=CARTESIAN_POINT('Ctrl Pts',(-2.80484128600006,2.2,-2.91189178400002));
#320044=CARTESIAN_POINT('Ctrl Pts',(-2.80529700700006,12.2,-2.91254432900002));
#320045=CARTESIAN_POINT('Ctrl Pts',(-2.80529700700006,5.2,-2.91254432900002));
#320046=CARTESIAN_POINT('Ctrl Pts',(-2.80529700700006,2.2,-2.91254432900002));
#320047=CARTESIAN_POINT('Ctrl Pts',(-2.80575524000006,12.2,-2.91320223400001));
#320048=CARTESIAN_POINT('Ctrl Pts',(-2.80575524000006,5.2,-2.91320223400001));
#320049=CARTESIAN_POINT('Ctrl Pts',(-2.80575524000006,2.2,-2.91320223400001));
#320050=CARTESIAN_POINT('Ctrl Pts',(-2.80621596600006,12.2,-2.91386549600002));
#320051=CARTESIAN_POINT('Ctrl Pts',(-2.80621596600006,5.2,-2.91386549600002));
#320052=CARTESIAN_POINT('Ctrl Pts',(-2.80621596600006,2.2,-2.91386549600002));
#320053=CARTESIAN_POINT('Ctrl Pts',(-2.80667916700006,12.2,-2.91453411200001));
#320054=CARTESIAN_POINT('Ctrl Pts',(-2.80667916700006,5.2,-2.91453411200001));
#320055=CARTESIAN_POINT('Ctrl Pts',(-2.80667916700006,2.2,-2.91453411200001));
#320056=CARTESIAN_POINT('Ctrl Pts',(-2.80714482500006,12.2,-2.91520808200001));
#320057=CARTESIAN_POINT('Ctrl Pts',(-2.80714482500006,5.2,-2.91520808200001));
#320058=CARTESIAN_POINT('Ctrl Pts',(-2.80714482500006,2.2,-2.91520808200001));
#320059=CARTESIAN_POINT('Ctrl Pts',(-2.80761292300005,12.2,-2.91588740400002));
#320060=CARTESIAN_POINT('Ctrl Pts',(-2.80761292300005,5.2,-2.91588740400002));
#320061=CARTESIAN_POINT('Ctrl Pts',(-2.80761292300005,2.2,-2.91588740400002));
#320062=CARTESIAN_POINT('Ctrl Pts',(-2.80808344100006,12.2,-2.91657207700001));
#320063=CARTESIAN_POINT('Ctrl Pts',(-2.80808344100006,5.2,-2.91657207700001));
#320064=CARTESIAN_POINT('Ctrl Pts',(-2.80808344100006,2.2,-2.91657207700001));
#320065=CARTESIAN_POINT('Ctrl Pts',(-2.80855636300006,12.2,-2.91726209800002));
#320066=CARTESIAN_POINT('Ctrl Pts',(-2.80855636300006,5.2,-2.91726209800002));
#320067=CARTESIAN_POINT('Ctrl Pts',(-2.80855636300006,2.2,-2.91726209800002));
#320068=CARTESIAN_POINT('Ctrl Pts',(-2.80903167000006,12.2,-2.91795746600001));
#320069=CARTESIAN_POINT('Ctrl Pts',(-2.80903167000006,5.2,-2.91795746600001));
#320070=CARTESIAN_POINT('Ctrl Pts',(-2.80903167000006,2.2,-2.91795746600001));
#320071=CARTESIAN_POINT('Ctrl Pts',(-2.80950934500006,12.2,-2.91865818000002));
#320072=CARTESIAN_POINT('Ctrl Pts',(-2.80950934500006,5.2,-2.91865818000002));
#320073=CARTESIAN_POINT('Ctrl Pts',(-2.80950934500006,2.2,-2.91865818000002));
#320074=CARTESIAN_POINT('Ctrl Pts',(-2.80998936800006,12.2,-2.91936423700002));
#320075=CARTESIAN_POINT('Ctrl Pts',(-2.80998936800006,5.2,-2.91936423700002));
#320076=CARTESIAN_POINT('Ctrl Pts',(-2.80998936800006,2.2,-2.91936423700002));
#320077=CARTESIAN_POINT('Ctrl Pts',(-2.81047172400006,12.2,-2.92007563600002));
#320078=CARTESIAN_POINT('Ctrl Pts',(-2.81047172400006,5.2,-2.92007563600002));
#320079=CARTESIAN_POINT('Ctrl Pts',(-2.81047172400006,2.2,-2.92007563600002));
#320080=CARTESIAN_POINT('Ctrl Pts',(-2.81095639400006,12.2,-2.92079237500001));
#320081=CARTESIAN_POINT('Ctrl Pts',(-2.81095639400006,5.2,-2.92079237500001));
#320082=CARTESIAN_POINT('Ctrl Pts',(-2.81095639400006,2.2,-2.92079237500001));
#320083=CARTESIAN_POINT('Ctrl Pts',(-2.81144336000006,12.2,-2.92151445100002));
#320084=CARTESIAN_POINT('Ctrl Pts',(-2.81144336000006,5.2,-2.92151445100002));
#320085=CARTESIAN_POINT('Ctrl Pts',(-2.81144336000006,2.2,-2.92151445100002));
#320086=CARTESIAN_POINT('Ctrl Pts',(-2.81193260400005,12.2,-2.92224186500002));
#320087=CARTESIAN_POINT('Ctrl Pts',(-2.81193260400005,5.2,-2.92224186500002));
#320088=CARTESIAN_POINT('Ctrl Pts',(-2.81193260400005,2.2,-2.92224186500002));
#320089=CARTESIAN_POINT('Ctrl Pts',(-2.81242411000005,12.2,-2.92297461300001));
#320090=CARTESIAN_POINT('Ctrl Pts',(-2.81242411000005,5.2,-2.92297461300001));
#320091=CARTESIAN_POINT('Ctrl Pts',(-2.81242411000005,2.2,-2.92297461300001));
#320092=CARTESIAN_POINT('Ctrl Pts',(-2.81291786100006,12.2,-2.92371269400002));
#320093=CARTESIAN_POINT('Ctrl Pts',(-2.81291786100006,5.2,-2.92371269400002));
#320094=CARTESIAN_POINT('Ctrl Pts',(-2.81291786100006,2.2,-2.92371269400002));
#320095=CARTESIAN_POINT('Ctrl Pts',(-2.81341383700005,12.2,-2.92445610600002));
#320096=CARTESIAN_POINT('Ctrl Pts',(-2.81341383700005,5.2,-2.92445610600002));
#320097=CARTESIAN_POINT('Ctrl Pts',(-2.81341383700005,2.2,-2.92445610600002));
#320098=CARTESIAN_POINT('Ctrl Pts',(-2.81391202300005,12.2,-2.92520484700002));
#320099=CARTESIAN_POINT('Ctrl Pts',(-2.81391202300005,5.2,-2.92520484700002));
#320100=CARTESIAN_POINT('Ctrl Pts',(-2.81391202300005,2.2,-2.92520484700002));
#320101=CARTESIAN_POINT('Ctrl Pts',(-2.81441239800006,12.2,-2.92595891500001));
#320102=CARTESIAN_POINT('Ctrl Pts',(-2.81441239800006,5.2,-2.92595891500001));
#320103=CARTESIAN_POINT('Ctrl Pts',(-2.81441239800006,2.2,-2.92595891500001));
#320104=CARTESIAN_POINT('Ctrl Pts',(-2.81491495000005,12.2,-2.92671830800002));
#320105=CARTESIAN_POINT('Ctrl Pts',(-2.81491495000005,5.2,-2.92671830800002));
#320106=CARTESIAN_POINT('Ctrl Pts',(-2.81491495000005,2.2,-2.92671830800002));
#320107=CARTESIAN_POINT('Ctrl Pts',(-2.81541965700006,12.2,-2.92748302500002));
#320108=CARTESIAN_POINT('Ctrl Pts',(-2.81541965700006,5.2,-2.92748302500002));
#320109=CARTESIAN_POINT('Ctrl Pts',(-2.81541965700006,2.2,-2.92748302500002));
#320110=CARTESIAN_POINT('Ctrl Pts',(-2.81592650500006,12.2,-2.92825306300001));
#320111=CARTESIAN_POINT('Ctrl Pts',(-2.81592650500006,5.2,-2.92825306300001));
#320112=CARTESIAN_POINT('Ctrl Pts',(-2.81592650500006,2.2,-2.92825306300001));
#320113=CARTESIAN_POINT('Ctrl Pts',(-2.81643547500006,12.2,-2.92902842100002));
#320114=CARTESIAN_POINT('Ctrl Pts',(-2.81643547500006,5.2,-2.92902842100002));
#320115=CARTESIAN_POINT('Ctrl Pts',(-2.81643547500006,2.2,-2.92902842100002));
#320116=CARTESIAN_POINT('Ctrl Pts',(-2.81694655000006,12.2,-2.92980909600002));
#320117=CARTESIAN_POINT('Ctrl Pts',(-2.81694655000006,5.2,-2.92980909600002));
#320118=CARTESIAN_POINT('Ctrl Pts',(-2.81694655000006,2.2,-2.92980909600002));
#320119=CARTESIAN_POINT('Ctrl Pts',(-2.81745971400006,12.2,-2.93059508700001));
#320120=CARTESIAN_POINT('Ctrl Pts',(-2.81745971400006,5.2,-2.93059508700001));
#320121=CARTESIAN_POINT('Ctrl Pts',(-2.81745971400006,2.2,-2.93059508700001));
#320122=CARTESIAN_POINT('Ctrl Pts',(-2.81797494900006,12.2,-2.93138639100002));
#320123=CARTESIAN_POINT('Ctrl Pts',(-2.81797494900006,5.2,-2.93138639100002));
#320124=CARTESIAN_POINT('Ctrl Pts',(-2.81797494900006,2.2,-2.93138639100002));
#320125=CARTESIAN_POINT('Ctrl Pts',(-2.81849223900006,12.2,-2.93218300800001));
#320126=CARTESIAN_POINT('Ctrl Pts',(-2.81849223900006,5.2,-2.93218300800001));
#320127=CARTESIAN_POINT('Ctrl Pts',(-2.81849223900006,2.2,-2.93218300800001));
#320128=CARTESIAN_POINT('Ctrl Pts',(-2.81901156500005,12.2,-2.93298493300002));
#320129=CARTESIAN_POINT('Ctrl Pts',(-2.81901156500005,5.2,-2.93298493300002));
#320130=CARTESIAN_POINT('Ctrl Pts',(-2.81901156500005,2.2,-2.93298493300002));
#320131=CARTESIAN_POINT('Ctrl Pts',(-2.81953291300006,12.2,-2.93379216500002));
#320132=CARTESIAN_POINT('Ctrl Pts',(-2.81953291300006,5.2,-2.93379216500002));
#320133=CARTESIAN_POINT('Ctrl Pts',(-2.81953291300006,2.2,-2.93379216500002));
#320134=CARTESIAN_POINT('Ctrl Pts',(-2.82005626300006,12.2,-2.93460470400001));
#320135=CARTESIAN_POINT('Ctrl Pts',(-2.82005626300006,5.2,-2.93460470400001));
#320136=CARTESIAN_POINT('Ctrl Pts',(-2.82005626300006,2.2,-2.93460470400001));
#320137=CARTESIAN_POINT('Ctrl Pts',(-2.82058160100005,12.2,-2.93542254400001));
#320138=CARTESIAN_POINT('Ctrl Pts',(-2.82058160100005,5.2,-2.93542254400001));
#320139=CARTESIAN_POINT('Ctrl Pts',(-2.82058160100005,2.2,-2.93542254400001));
#320140=CARTESIAN_POINT('Ctrl Pts',(-2.82110890800006,12.2,-2.93624568700002));
#320141=CARTESIAN_POINT('Ctrl Pts',(-2.82110890800006,5.2,-2.93624568700002));
#320142=CARTESIAN_POINT('Ctrl Pts',(-2.82110890800006,2.2,-2.93624568700002));
#320143=CARTESIAN_POINT('Ctrl Pts',(-2.82163817000006,12.2,-2.93707412900002));
#320144=CARTESIAN_POINT('Ctrl Pts',(-2.82163817000006,5.2,-2.93707412900002));
#320145=CARTESIAN_POINT('Ctrl Pts',(-2.82163817000006,2.2,-2.93707412900002));
#320146=CARTESIAN_POINT('Ctrl Pts',(-2.82216936700005,12.2,-2.93790786800002));
#320147=CARTESIAN_POINT('Ctrl Pts',(-2.82216936700005,5.2,-2.93790786800002));
#320148=CARTESIAN_POINT('Ctrl Pts',(-2.82216936700005,2.2,-2.93790786800002));
#320149=CARTESIAN_POINT('Ctrl Pts',(-2.82270248500006,12.2,-2.93874690100001));
#320150=CARTESIAN_POINT('Ctrl Pts',(-2.82270248500006,5.2,-2.93874690100001));
#320151=CARTESIAN_POINT('Ctrl Pts',(-2.82270248500006,2.2,-2.93874690100001));
#320152=CARTESIAN_POINT('Ctrl Pts',(-2.82323750600006,12.2,-2.93959122700001));
#320153=CARTESIAN_POINT('Ctrl Pts',(-2.82323750600006,5.2,-2.93959122700001));
#320154=CARTESIAN_POINT('Ctrl Pts',(-2.82323750600006,2.2,-2.93959122700001));
#320155=CARTESIAN_POINT('Ctrl Pts',(-2.82377441500006,12.2,-2.94044084400001));
#320156=CARTESIAN_POINT('Ctrl Pts',(-2.82377441500006,5.2,-2.94044084400001));
#320157=CARTESIAN_POINT('Ctrl Pts',(-2.82377441500006,2.2,-2.94044084400001));
#320158=CARTESIAN_POINT('Ctrl Pts',(-2.82431319300006,12.2,-2.94129574900001));
#320159=CARTESIAN_POINT('Ctrl Pts',(-2.82431319300006,5.2,-2.94129574900001));
#320160=CARTESIAN_POINT('Ctrl Pts',(-2.82431319300006,2.2,-2.94129574900001));
#320161=CARTESIAN_POINT('Ctrl Pts',(-2.82485382600006,12.2,-2.94215594000002));
#320162=CARTESIAN_POINT('Ctrl Pts',(-2.82485382600006,5.2,-2.94215594000002));
#320163=CARTESIAN_POINT('Ctrl Pts',(-2.82485382600006,2.2,-2.94215594000002));
#320164=CARTESIAN_POINT('Ctrl Pts',(-2.82539629600006,12.2,-2.94302141400001));
#320165=CARTESIAN_POINT('Ctrl Pts',(-2.82539629600006,5.2,-2.94302141400001));
#320166=CARTESIAN_POINT('Ctrl Pts',(-2.82539629600006,2.2,-2.94302141400001));
#320167=CARTESIAN_POINT('Ctrl Pts',(-2.82594058800006,12.2,-2.94389217100001));
#320168=CARTESIAN_POINT('Ctrl Pts',(-2.82594058800006,5.2,-2.94389217100001));
#320169=CARTESIAN_POINT('Ctrl Pts',(-2.82594058800006,2.2,-2.94389217100001));
#320170=CARTESIAN_POINT('Ctrl Pts',(-2.82648668400005,12.2,-2.94476820700002));
#320171=CARTESIAN_POINT('Ctrl Pts',(-2.82648668400005,5.2,-2.94476820700002));
#320172=CARTESIAN_POINT('Ctrl Pts',(-2.82648668400005,2.2,-2.94476820700002));
#320173=CARTESIAN_POINT('Ctrl Pts',(-2.82703456900005,12.2,-2.94564952000002));
#320174=CARTESIAN_POINT('Ctrl Pts',(-2.82703456900005,5.2,-2.94564952000002));
#320175=CARTESIAN_POINT('Ctrl Pts',(-2.82703456900005,2.2,-2.94564952000002));
#320176=CARTESIAN_POINT('Ctrl Pts',(-2.82758422700006,12.2,-2.94653610700002));
#320177=CARTESIAN_POINT('Ctrl Pts',(-2.82758422700006,5.2,-2.94653610700002));
#320178=CARTESIAN_POINT('Ctrl Pts',(-2.82758422700006,2.2,-2.94653610700002));
#320179=CARTESIAN_POINT('Ctrl Pts',(-2.82813564100006,12.2,-2.94742796800001));
#320180=CARTESIAN_POINT('Ctrl Pts',(-2.82813564100006,5.2,-2.94742796800001));
#320181=CARTESIAN_POINT('Ctrl Pts',(-2.82813564100006,2.2,-2.94742796800001));
#320182=CARTESIAN_POINT('Ctrl Pts',(-2.82868879500006,12.2,-2.94832509800001));
#320183=CARTESIAN_POINT('Ctrl Pts',(-2.82868879500006,5.2,-2.94832509800001));
#320184=CARTESIAN_POINT('Ctrl Pts',(-2.82868879500006,2.2,-2.94832509800001));
#320185=CARTESIAN_POINT('Ctrl Pts',(-2.82924367300006,12.2,-2.94922749700001));
#320186=CARTESIAN_POINT('Ctrl Pts',(-2.82924367300006,5.2,-2.94922749700001));
#320187=CARTESIAN_POINT('Ctrl Pts',(-2.82924367300006,2.2,-2.94922749700001));
#320188=CARTESIAN_POINT('Ctrl Pts',(-2.82980025900006,12.2,-2.95013516100001));
#320189=CARTESIAN_POINT('Ctrl Pts',(-2.82980025900006,5.2,-2.95013516100001));
#320190=CARTESIAN_POINT('Ctrl Pts',(-2.82980025900006,2.2,-2.95013516100001));
#320191=CARTESIAN_POINT('Ctrl Pts',(-2.83035853700006,12.2,-2.95104808800001));
#320192=CARTESIAN_POINT('Ctrl Pts',(-2.83035853700006,5.2,-2.95104808800001));
#320193=CARTESIAN_POINT('Ctrl Pts',(-2.83035853700006,2.2,-2.95104808800001));
#320194=CARTESIAN_POINT('Ctrl Pts',(-2.83091849000006,12.2,-2.95196627600002));
#320195=CARTESIAN_POINT('Ctrl Pts',(-2.83091849000006,5.2,-2.95196627600002));
#320196=CARTESIAN_POINT('Ctrl Pts',(-2.83091849000006,2.2,-2.95196627600002));
#320197=CARTESIAN_POINT('Ctrl Pts',(-2.83148010400006,12.2,-2.95288972300002));
#320198=CARTESIAN_POINT('Ctrl Pts',(-2.83148010400006,5.2,-2.95288972300002));
#320199=CARTESIAN_POINT('Ctrl Pts',(-2.83148010400006,2.2,-2.95288972300002));
#320200=CARTESIAN_POINT('Ctrl Pts',(-2.83204336300006,12.2,-2.95381842500001));
#320201=CARTESIAN_POINT('Ctrl Pts',(-2.83204336300006,5.2,-2.95381842500001));
#320202=CARTESIAN_POINT('Ctrl Pts',(-2.83204336300006,2.2,-2.95381842500001));
#320203=CARTESIAN_POINT('Ctrl Pts',(-2.83260824900006,12.2,-2.95475238100002));
#320204=CARTESIAN_POINT('Ctrl Pts',(-2.83260824900006,5.2,-2.95475238100002));
#320205=CARTESIAN_POINT('Ctrl Pts',(-2.83260824900006,2.2,-2.95475238100002));
#320206=CARTESIAN_POINT('Ctrl Pts',(-2.83317474800006,12.2,-2.95569158900001));
#320207=CARTESIAN_POINT('Ctrl Pts',(-2.83317474800006,5.2,-2.95569158900001));
#320208=CARTESIAN_POINT('Ctrl Pts',(-2.83317474800006,2.2,-2.95569158900001));
#320209=CARTESIAN_POINT('Ctrl Pts',(-2.83374284300006,12.2,-2.95663604500001));
#320210=CARTESIAN_POINT('Ctrl Pts',(-2.83374284300006,5.2,-2.95663604500001));
#320211=CARTESIAN_POINT('Ctrl Pts',(-2.83374284300006,2.2,-2.95663604500001));
#320212=CARTESIAN_POINT('Ctrl Pts',(-2.83431252100006,12.2,-2.95758574700002));
#320213=CARTESIAN_POINT('Ctrl Pts',(-2.83431252100006,5.2,-2.95758574700002));
#320214=CARTESIAN_POINT('Ctrl Pts',(-2.83431252100006,2.2,-2.95758574700002));
#320215=CARTESIAN_POINT('Ctrl Pts',(-2.83488376300005,12.2,-2.95854069400002));
#320216=CARTESIAN_POINT('Ctrl Pts',(-2.83488376300005,5.2,-2.95854069400002));
#320217=CARTESIAN_POINT('Ctrl Pts',(-2.83488376300005,2.2,-2.95854069400002));
#320218=CARTESIAN_POINT('Ctrl Pts',(-2.83545655400005,12.2,-2.95950088100001));
#320219=CARTESIAN_POINT('Ctrl Pts',(-2.83545655400005,5.2,-2.95950088100001));
#320220=CARTESIAN_POINT('Ctrl Pts',(-2.83545655400005,2.2,-2.95950088100001));
#320221=CARTESIAN_POINT('Ctrl Pts',(-2.83603088100006,12.2,-2.96046630800001));
#320222=CARTESIAN_POINT('Ctrl Pts',(-2.83603088100006,5.2,-2.96046630800001));
#320223=CARTESIAN_POINT('Ctrl Pts',(-2.83603088100006,2.2,-2.96046630800001));
#320224=CARTESIAN_POINT('Ctrl Pts',(-2.83660672500006,12.2,-2.96143697100002));
#320225=CARTESIAN_POINT('Ctrl Pts',(-2.83660672500006,5.2,-2.96143697100002));
#320226=CARTESIAN_POINT('Ctrl Pts',(-2.83660672500006,2.2,-2.96143697100002));
#320227=CARTESIAN_POINT('Ctrl Pts',(-2.83718407300006,12.2,-2.96241286700001));
#320228=CARTESIAN_POINT('Ctrl Pts',(-2.83718407300006,5.2,-2.96241286700001));
#320229=CARTESIAN_POINT('Ctrl Pts',(-2.83718407300006,2.2,-2.96241286700001));
#320230=CARTESIAN_POINT('Ctrl Pts',(-2.83776290800006,12.2,-2.96339399500001));
#320231=CARTESIAN_POINT('Ctrl Pts',(-2.83776290800006,5.2,-2.96339399500001));
#320232=CARTESIAN_POINT('Ctrl Pts',(-2.83776290800006,2.2,-2.96339399500001));
#320233=CARTESIAN_POINT('Ctrl Pts',(-2.83834321500006,12.2,-2.96438035200001));
#320234=CARTESIAN_POINT('Ctrl Pts',(-2.83834321500006,5.2,-2.96438035200001));
#320235=CARTESIAN_POINT('Ctrl Pts',(-2.83834321500006,2.2,-2.96438035200001));
#320236=CARTESIAN_POINT('Ctrl Pts',(-2.83892497800006,12.2,-2.96537193400002));
#320237=CARTESIAN_POINT('Ctrl Pts',(-2.83892497800006,5.2,-2.96537193400002));
#320238=CARTESIAN_POINT('Ctrl Pts',(-2.83892497800006,2.2,-2.96537193400002));
#320239=CARTESIAN_POINT('Ctrl Pts',(-2.83950818400006,12.2,-2.96636874000002));
#320240=CARTESIAN_POINT('Ctrl Pts',(-2.83950818400006,5.2,-2.96636874000002));
#320241=CARTESIAN_POINT('Ctrl Pts',(-2.83950818400006,2.2,-2.96636874000002));
#320242=CARTESIAN_POINT('Ctrl Pts',(-2.84009281500006,12.2,-2.96737076700001));
#320243=CARTESIAN_POINT('Ctrl Pts',(-2.84009281500006,5.2,-2.96737076700001));
#320244=CARTESIAN_POINT('Ctrl Pts',(-2.84009281500006,2.2,-2.96737076700001));
#320245=CARTESIAN_POINT('Ctrl Pts',(-2.84067885800006,12.2,-2.96837801300001));
#320246=CARTESIAN_POINT('Ctrl Pts',(-2.84067885800006,5.2,-2.96837801300001));
#320247=CARTESIAN_POINT('Ctrl Pts',(-2.84067885800006,2.2,-2.96837801300001));
#320248=CARTESIAN_POINT('Ctrl Pts',(-2.84126629500005,12.2,-2.96939047400001));
#320249=CARTESIAN_POINT('Ctrl Pts',(-2.84126629500005,5.2,-2.96939047400001));
#320250=CARTESIAN_POINT('Ctrl Pts',(-2.84126629500005,2.2,-2.96939047400001));
#320251=CARTESIAN_POINT('Ctrl Pts',(-2.84185511300006,12.2,-2.97040814900001));
#320252=CARTESIAN_POINT('Ctrl Pts',(-2.84185511300006,5.2,-2.97040814900001));
#320253=CARTESIAN_POINT('Ctrl Pts',(-2.84185511300006,2.2,-2.97040814900001));
#320254=CARTESIAN_POINT('Ctrl Pts',(-2.84244529600006,12.2,-2.97143103400002));
#320255=CARTESIAN_POINT('Ctrl Pts',(-2.84244529600006,5.2,-2.97143103400002));
#320256=CARTESIAN_POINT('Ctrl Pts',(-2.84244529600006,2.2,-2.97143103400002));
#320257=CARTESIAN_POINT('Ctrl Pts',(-2.84303682900005,12.2,-2.97245912600001));
#320258=CARTESIAN_POINT('Ctrl Pts',(-2.84303682900005,5.2,-2.97245912600001));
#320259=CARTESIAN_POINT('Ctrl Pts',(-2.84303682900005,2.2,-2.97245912600001));
#320260=CARTESIAN_POINT('Ctrl Pts',(-2.84362969700005,12.2,-2.97349242400001));
#320261=CARTESIAN_POINT('Ctrl Pts',(-2.84362969700005,5.2,-2.97349242400001));
#320262=CARTESIAN_POINT('Ctrl Pts',(-2.84362969700005,2.2,-2.97349242400001));
#320263=CARTESIAN_POINT('Ctrl Pts',(-2.84422388600006,12.2,-2.97453092400001));
#320264=CARTESIAN_POINT('Ctrl Pts',(-2.84422388600006,5.2,-2.97453092400001));
#320265=CARTESIAN_POINT('Ctrl Pts',(-2.84422388600006,2.2,-2.97453092400001));
#320266=CARTESIAN_POINT('Ctrl Pts',(-2.84481937800006,12.2,-2.97557462400002));
#320267=CARTESIAN_POINT('Ctrl Pts',(-2.84481937800006,5.2,-2.97557462400002));
#320268=CARTESIAN_POINT('Ctrl Pts',(-2.84481937800006,2.2,-2.97557462400002));
#320269=CARTESIAN_POINT('Ctrl Pts',(-2.84541616100006,12.2,-2.97662352000001));
#320270=CARTESIAN_POINT('Ctrl Pts',(-2.84541616100006,5.2,-2.97662352000001));
#320271=CARTESIAN_POINT('Ctrl Pts',(-2.84541616100006,2.2,-2.97662352000001));
#320272=CARTESIAN_POINT('Ctrl Pts',(-2.84601421800006,12.2,-2.97767761100001));
#320273=CARTESIAN_POINT('Ctrl Pts',(-2.84601421800006,5.2,-2.97767761100001));
#320274=CARTESIAN_POINT('Ctrl Pts',(-2.84601421800006,2.2,-2.97767761100001));
#320275=CARTESIAN_POINT('Ctrl Pts',(-2.84661353600006,12.2,-2.97873689300001));
#320276=CARTESIAN_POINT('Ctrl Pts',(-2.84661353600006,5.2,-2.97873689300001));
#320277=CARTESIAN_POINT('Ctrl Pts',(-2.84661353600006,2.2,-2.97873689300001));
#320278=CARTESIAN_POINT('Ctrl Pts',(-2.84721410000006,12.2,-2.97980136500001));
#320279=CARTESIAN_POINT('Ctrl Pts',(-2.84721410000006,5.2,-2.97980136500001));
#320280=CARTESIAN_POINT('Ctrl Pts',(-2.84721410000006,2.2,-2.97980136500001));
#320281=CARTESIAN_POINT('Ctrl Pts',(-2.84781589300006,12.2,-2.98087102200002));
#320282=CARTESIAN_POINT('Ctrl Pts',(-2.84781589300006,5.2,-2.98087102200002));
#320283=CARTESIAN_POINT('Ctrl Pts',(-2.84781589300006,2.2,-2.98087102200002));
#320284=CARTESIAN_POINT('Ctrl Pts',(-2.84841890200005,12.2,-2.98194586200001));
#320285=CARTESIAN_POINT('Ctrl Pts',(-2.84841890200005,5.2,-2.98194586200001));
#320286=CARTESIAN_POINT('Ctrl Pts',(-2.84841890200005,2.2,-2.98194586200001));
#320287=CARTESIAN_POINT('Ctrl Pts',(-2.84902311100006,12.2,-2.98302588300002));
#320288=CARTESIAN_POINT('Ctrl Pts',(-2.84902311100006,5.2,-2.98302588300002));
#320289=CARTESIAN_POINT('Ctrl Pts',(-2.84902311100006,2.2,-2.98302588300002));
#320290=CARTESIAN_POINT('Ctrl Pts',(-2.84962850700006,12.2,-2.98411108200002));
#320291=CARTESIAN_POINT('Ctrl Pts',(-2.84962850700006,5.2,-2.98411108200002));
#320292=CARTESIAN_POINT('Ctrl Pts',(-2.84962850700006,2.2,-2.98411108200002));
#320293=CARTESIAN_POINT('Ctrl Pts',(-2.85023507500005,12.2,-2.98520145500001));
#320294=CARTESIAN_POINT('Ctrl Pts',(-2.85023507500005,5.2,-2.98520145500001));
#320295=CARTESIAN_POINT('Ctrl Pts',(-2.85023507500005,2.2,-2.98520145500001));
#320296=CARTESIAN_POINT('Ctrl Pts',(-2.85084280000006,12.2,-2.98629699900001));
#320297=CARTESIAN_POINT('Ctrl Pts',(-2.85084280000006,5.2,-2.98629699900001));
#320298=CARTESIAN_POINT('Ctrl Pts',(-2.85084280000006,2.2,-2.98629699900001));
#320299=CARTESIAN_POINT('Ctrl Pts',(-2.85145166600006,12.2,-2.98739771400002));
#320300=CARTESIAN_POINT('Ctrl Pts',(-2.85145166600006,5.2,-2.98739771400002));
#320301=CARTESIAN_POINT('Ctrl Pts',(-2.85145166600006,2.2,-2.98739771400002));
#320302=CARTESIAN_POINT('Ctrl Pts',(-2.85206166100005,12.2,-2.98850359400001));
#320303=CARTESIAN_POINT('Ctrl Pts',(-2.85206166100005,5.2,-2.98850359400001));
#320304=CARTESIAN_POINT('Ctrl Pts',(-2.85206166100005,2.2,-2.98850359400001));
#320305=CARTESIAN_POINT('Ctrl Pts',(-2.85267276900006,12.2,-2.98961463700001));
#320306=CARTESIAN_POINT('Ctrl Pts',(-2.85267276900006,5.2,-2.98961463700001));
#320307=CARTESIAN_POINT('Ctrl Pts',(-2.85267276900006,2.2,-2.98961463700001));
#320308=CARTESIAN_POINT('Ctrl Pts',(-2.85328497500006,12.2,-2.99073084200002));
#320309=CARTESIAN_POINT('Ctrl Pts',(-2.85328497500006,5.2,-2.99073084200002));
#320310=CARTESIAN_POINT('Ctrl Pts',(-2.85328497500006,2.2,-2.99073084200002));
#320311=CARTESIAN_POINT('Ctrl Pts',(-2.85389826500006,12.2,-2.99185220200001));
#320312=CARTESIAN_POINT('Ctrl Pts',(-2.85389826500006,5.2,-2.99185220200001));
#320313=CARTESIAN_POINT('Ctrl Pts',(-2.85389826500006,2.2,-2.99185220200001));
#320314=CARTESIAN_POINT('Ctrl Pts',(-2.85451262500006,12.2,-2.99297871900002));
#320315=CARTESIAN_POINT('Ctrl Pts',(-2.85451262500006,5.2,-2.99297871900002));
#320316=CARTESIAN_POINT('Ctrl Pts',(-2.85451262500006,2.2,-2.99297871900002));
#320317=CARTESIAN_POINT('Ctrl Pts',(-2.85512804100006,12.2,-2.99411038700002));
#320318=CARTESIAN_POINT('Ctrl Pts',(-2.85512804100006,5.2,-2.99411038700002));
#320319=CARTESIAN_POINT('Ctrl Pts',(-2.85512804100006,2.2,-2.99411038700002));
#320320=CARTESIAN_POINT('Ctrl Pts',(-2.85574449800006,12.2,-2.99524720400001));
#320321=CARTESIAN_POINT('Ctrl Pts',(-2.85574449800006,5.2,-2.99524720400001));
#320322=CARTESIAN_POINT('Ctrl Pts',(-2.85574449800006,2.2,-2.99524720400001));
#320323=CARTESIAN_POINT('Ctrl Pts',(-2.85636198200006,12.2,-2.99638916700002));
#320324=CARTESIAN_POINT('Ctrl Pts',(-2.85636198200006,5.2,-2.99638916700002));
#320325=CARTESIAN_POINT('Ctrl Pts',(-2.85636198200006,2.2,-2.99638916700002));
#320326=CARTESIAN_POINT('Ctrl Pts',(-2.85698047800006,12.2,-2.99753627200001));
#320327=CARTESIAN_POINT('Ctrl Pts',(-2.85698047800006,5.2,-2.99753627200001));
#320328=CARTESIAN_POINT('Ctrl Pts',(-2.85698047800006,2.2,-2.99753627200001));
#320329=CARTESIAN_POINT('Ctrl Pts',(-2.85759997200006,12.2,-2.99868851700001));
#320330=CARTESIAN_POINT('Ctrl Pts',(-2.85759997200006,5.2,-2.99868851700001));
#320331=CARTESIAN_POINT('Ctrl Pts',(-2.85759997200006,2.2,-2.99868851700001));
#320332=CARTESIAN_POINT('Ctrl Pts',(-2.85822045100006,12.2,-2.99984590000001));
#320333=CARTESIAN_POINT('Ctrl Pts',(-2.85822045100006,5.2,-2.99984590000001));
#320334=CARTESIAN_POINT('Ctrl Pts',(-2.85822045100006,2.2,-2.99984590000001));
#320335=CARTESIAN_POINT('Ctrl Pts',(-2.85884189900006,12.2,-3.00100841600001));
#320336=CARTESIAN_POINT('Ctrl Pts',(-2.85884189900006,5.2,-3.00100841600001));
#320337=CARTESIAN_POINT('Ctrl Pts',(-2.85884189900006,2.2,-3.00100841600001));
#320338=CARTESIAN_POINT('Ctrl Pts',(-2.85946430300006,12.2,-3.00217606300002));
#320339=CARTESIAN_POINT('Ctrl Pts',(-2.85946430300006,5.2,-3.00217606300002));
#320340=CARTESIAN_POINT('Ctrl Pts',(-2.85946430300006,2.2,-3.00217606300002));
#320341=CARTESIAN_POINT('Ctrl Pts',(-2.86008764900005,12.2,-3.00334883900002));
#320342=CARTESIAN_POINT('Ctrl Pts',(-2.86008764900005,5.2,-3.00334883900002));
#320343=CARTESIAN_POINT('Ctrl Pts',(-2.86008764900005,2.2,-3.00334883900002));
#320344=CARTESIAN_POINT('Ctrl Pts',(-2.86071192200006,12.2,-3.00452673900002));
#320345=CARTESIAN_POINT('Ctrl Pts',(-2.86071192200006,5.2,-3.00452673900002));
#320346=CARTESIAN_POINT('Ctrl Pts',(-2.86071192200006,2.2,-3.00452673900002));
#320347=CARTESIAN_POINT('Ctrl Pts',(-2.86133710900006,12.2,-3.00570976000001));
#320348=CARTESIAN_POINT('Ctrl Pts',(-2.86133710900006,5.2,-3.00570976000001));
#320349=CARTESIAN_POINT('Ctrl Pts',(-2.86133710900006,2.2,-3.00570976000001));
#320350=CARTESIAN_POINT('Ctrl Pts',(-2.86196319600006,12.2,-3.00689790100002));
#320351=CARTESIAN_POINT('Ctrl Pts',(-2.86196319600006,5.2,-3.00689790100002));
#320352=CARTESIAN_POINT('Ctrl Pts',(-2.86196319600006,2.2,-3.00689790100002));
#320353=CARTESIAN_POINT('Ctrl Pts',(-2.86259016800006,12.2,-3.00809115700002));
#320354=CARTESIAN_POINT('Ctrl Pts',(-2.86259016800006,5.2,-3.00809115700002));
#320355=CARTESIAN_POINT('Ctrl Pts',(-2.86259016800006,2.2,-3.00809115700002));
#320356=CARTESIAN_POINT('Ctrl Pts',(-2.86321801200006,12.2,-3.00928952600001));
#320357=CARTESIAN_POINT('Ctrl Pts',(-2.86321801200006,5.2,-3.00928952600001));
#320358=CARTESIAN_POINT('Ctrl Pts',(-2.86321801200006,2.2,-3.00928952600001));
#320359=CARTESIAN_POINT('Ctrl Pts',(-2.86384671300006,12.2,-3.01049300400001));
#320360=CARTESIAN_POINT('Ctrl Pts',(-2.86384671300006,5.2,-3.01049300400001));
#320361=CARTESIAN_POINT('Ctrl Pts',(-2.86384671300006,2.2,-3.01049300400001));
#320362=CARTESIAN_POINT('Ctrl Pts',(-2.86447625900006,12.2,-3.01170158900002));
#320363=CARTESIAN_POINT('Ctrl Pts',(-2.86447625900006,5.2,-3.01170158900002));
#320364=CARTESIAN_POINT('Ctrl Pts',(-2.86447625900006,2.2,-3.01170158900002));
#320365=CARTESIAN_POINT('Ctrl Pts',(-2.86510663400006,12.2,-3.01291527700001));
#320366=CARTESIAN_POINT('Ctrl Pts',(-2.86510663400006,5.2,-3.01291527700001));
#320367=CARTESIAN_POINT('Ctrl Pts',(-2.86510663400006,2.2,-3.01291527700001));
#320368=CARTESIAN_POINT('Ctrl Pts',(-2.86573782700006,12.2,-3.01413406600001));
#320369=CARTESIAN_POINT('Ctrl Pts',(-2.86573782700006,5.2,-3.01413406600001));
#320370=CARTESIAN_POINT('Ctrl Pts',(-2.86573782700006,2.2,-3.01413406600001));
#320371=CARTESIAN_POINT('Ctrl Pts',(-2.86636982100006,12.2,-3.01535795100001));
#320372=CARTESIAN_POINT('Ctrl Pts',(-2.86636982100006,5.2,-3.01535795100001));
#320373=CARTESIAN_POINT('Ctrl Pts',(-2.86636982100006,2.2,-3.01535795100001));
#320374=CARTESIAN_POINT('Ctrl Pts',(-2.86700260500006,12.2,-3.01658693000002));
#320375=CARTESIAN_POINT('Ctrl Pts',(-2.86700260500006,5.2,-3.01658693000002));
#320376=CARTESIAN_POINT('Ctrl Pts',(-2.86700260500006,2.2,-3.01658693000002));
#320377=CARTESIAN_POINT('Ctrl Pts',(-2.86763616300005,12.2,-3.01782100100001));
#320378=CARTESIAN_POINT('Ctrl Pts',(-2.86763616300005,5.2,-3.01782100100001));
#320379=CARTESIAN_POINT('Ctrl Pts',(-2.86763616300005,2.2,-3.01782100100001));
#320380=CARTESIAN_POINT('Ctrl Pts',(-2.86827048300006,12.2,-3.01906015800002));
#320381=CARTESIAN_POINT('Ctrl Pts',(-2.86827048300006,5.2,-3.01906015800002));
#320382=CARTESIAN_POINT('Ctrl Pts',(-2.86827048300006,2.2,-3.01906015800002));
#320383=CARTESIAN_POINT('Ctrl Pts',(-2.86890555100006,12.2,-3.02030440000001));
#320384=CARTESIAN_POINT('Ctrl Pts',(-2.86890555100006,5.2,-3.02030440000001));
#320385=CARTESIAN_POINT('Ctrl Pts',(-2.86890555100006,2.2,-3.02030440000001));
#320386=CARTESIAN_POINT('Ctrl Pts',(-2.86954135300005,12.2,-3.02155372400001));
#320387=CARTESIAN_POINT('Ctrl Pts',(-2.86954135300005,5.2,-3.02155372400001));
#320388=CARTESIAN_POINT('Ctrl Pts',(-2.86954135300005,2.2,-3.02155372400001));
#320389=CARTESIAN_POINT('Ctrl Pts',(-2.87017787600006,12.2,-3.02280812500001));
#320390=CARTESIAN_POINT('Ctrl Pts',(-2.87017787600006,5.2,-3.02280812500001));
#320391=CARTESIAN_POINT('Ctrl Pts',(-2.87017787600006,2.2,-3.02280812500001));
#320392=CARTESIAN_POINT('Ctrl Pts',(-2.87081510600005,12.2,-3.02406760100002));
#320393=CARTESIAN_POINT('Ctrl Pts',(-2.87081510600005,5.2,-3.02406760100002));
#320394=CARTESIAN_POINT('Ctrl Pts',(-2.87081510600005,2.2,-3.02406760100002));
#320395=CARTESIAN_POINT('Ctrl Pts',(-2.87145303000006,12.2,-3.02533214800001));
#320396=CARTESIAN_POINT('Ctrl Pts',(-2.87145303000006,5.2,-3.02533214800001));
#320397=CARTESIAN_POINT('Ctrl Pts',(-2.87145303000006,2.2,-3.02533214800001));
#320398=CARTESIAN_POINT('Ctrl Pts',(-2.87209163400005,12.2,-3.02660176500002));
#320399=CARTESIAN_POINT('Ctrl Pts',(-2.87209163400005,5.2,-3.02660176500002));
#320400=CARTESIAN_POINT('Ctrl Pts',(-2.87209163400005,2.2,-3.02660176500002));
#320401=CARTESIAN_POINT('Ctrl Pts',(-2.87273090500006,12.2,-3.02787644600001));
#320402=CARTESIAN_POINT('Ctrl Pts',(-2.87273090500006,5.2,-3.02787644600001));
#320403=CARTESIAN_POINT('Ctrl Pts',(-2.87273090500006,2.2,-3.02787644600001));
#320404=CARTESIAN_POINT('Ctrl Pts',(-2.87337083000006,12.2,-3.02915618800002));
#320405=CARTESIAN_POINT('Ctrl Pts',(-2.87337083000006,5.2,-3.02915618800002));
#320406=CARTESIAN_POINT('Ctrl Pts',(-2.87337083000006,2.2,-3.02915618800002));
#320407=CARTESIAN_POINT('Ctrl Pts',(-2.87401139300006,12.2,-3.03044099000001));
#320408=CARTESIAN_POINT('Ctrl Pts',(-2.87401139300006,5.2,-3.03044099000001));
#320409=CARTESIAN_POINT('Ctrl Pts',(-2.87401139300006,2.2,-3.03044099000001));
#320410=CARTESIAN_POINT('Ctrl Pts',(-2.87465258400006,12.2,-3.03173084600001));
#320411=CARTESIAN_POINT('Ctrl Pts',(-2.87465258400006,5.2,-3.03173084600001));
#320412=CARTESIAN_POINT('Ctrl Pts',(-2.87465258400006,2.2,-3.03173084600001));
#320413=CARTESIAN_POINT('Ctrl Pts',(-2.87529438900005,12.2,-3.03302575500001));
#320414=CARTESIAN_POINT('Ctrl Pts',(-2.87529438900005,5.2,-3.03302575500001));
#320415=CARTESIAN_POINT('Ctrl Pts',(-2.87529438900005,2.2,-3.03302575500001));
#320416=CARTESIAN_POINT('Ctrl Pts',(-2.87593679400006,12.2,-3.03432571200001));
#320417=CARTESIAN_POINT('Ctrl Pts',(-2.87593679400006,5.2,-3.03432571200001));
#320418=CARTESIAN_POINT('Ctrl Pts',(-2.87593679400006,2.2,-3.03432571200001));
#320419=CARTESIAN_POINT('Ctrl Pts',(-2.87657978500006,12.2,-3.03563071500002));
#320420=CARTESIAN_POINT('Ctrl Pts',(-2.87657978500006,5.2,-3.03563071500002));
#320421=CARTESIAN_POINT('Ctrl Pts',(-2.87657978500006,2.2,-3.03563071500002));
#320422=CARTESIAN_POINT('Ctrl Pts',(-2.87722335000006,12.2,-3.03694075900002));
#320423=CARTESIAN_POINT('Ctrl Pts',(-2.87722335000006,5.2,-3.03694075900002));
#320424=CARTESIAN_POINT('Ctrl Pts',(-2.87722335000006,2.2,-3.03694075900002));
#320425=CARTESIAN_POINT('Ctrl Pts',(-2.87786747600005,12.2,-3.03825584200001));
#320426=CARTESIAN_POINT('Ctrl Pts',(-2.87786747600005,5.2,-3.03825584200001));
#320427=CARTESIAN_POINT('Ctrl Pts',(-2.87786747600005,2.2,-3.03825584200001));
#320428=CARTESIAN_POINT('Ctrl Pts',(-2.87851214900006,12.2,-3.03957596100001));
#320429=CARTESIAN_POINT('Ctrl Pts',(-2.87851214900006,5.2,-3.03957596100001));
#320430=CARTESIAN_POINT('Ctrl Pts',(-2.87851214900006,2.2,-3.03957596100001));
#320431=CARTESIAN_POINT('Ctrl Pts',(-2.87915735600006,12.2,-3.04090111200002));
#320432=CARTESIAN_POINT('Ctrl Pts',(-2.87915735600006,5.2,-3.04090111200002));
#320433=CARTESIAN_POINT('Ctrl Pts',(-2.87915735600006,2.2,-3.04090111200002));
#320434=CARTESIAN_POINT('Ctrl Pts',(-2.87980308500006,12.2,-3.04223129000002));
#320435=CARTESIAN_POINT('Ctrl Pts',(-2.87980308500006,5.2,-3.04223129000002));
#320436=CARTESIAN_POINT('Ctrl Pts',(-2.87980308500006,2.2,-3.04223129000002));
#320437=CARTESIAN_POINT('Ctrl Pts',(-2.88044932200005,12.2,-3.04356649500001));
#320438=CARTESIAN_POINT('Ctrl Pts',(-2.88044932200005,5.2,-3.04356649500001));
#320439=CARTESIAN_POINT('Ctrl Pts',(-2.88044932200005,2.2,-3.04356649500001));
#320440=CARTESIAN_POINT('Ctrl Pts',(-2.88109605400006,12.2,-3.04490672100002));
#320441=CARTESIAN_POINT('Ctrl Pts',(-2.88109605400006,5.2,-3.04490672100002));
#320442=CARTESIAN_POINT('Ctrl Pts',(-2.88109605400006,2.2,-3.04490672100002));
#320443=CARTESIAN_POINT('Ctrl Pts',(-2.88174326800006,12.2,-3.04625196600002));
#320444=CARTESIAN_POINT('Ctrl Pts',(-2.88174326800006,5.2,-3.04625196600002));
#320445=CARTESIAN_POINT('Ctrl Pts',(-2.88174326800006,2.2,-3.04625196600002));
#320446=CARTESIAN_POINT('Ctrl Pts',(-2.88239095100006,12.2,-3.04760222600001));
#320447=CARTESIAN_POINT('Ctrl Pts',(-2.88239095100006,5.2,-3.04760222600001));
#320448=CARTESIAN_POINT('Ctrl Pts',(-2.88239095100006,2.2,-3.04760222600001));
#320449=CARTESIAN_POINT('Ctrl Pts',(-2.88303909100006,12.2,-3.04895749700002));
#320450=CARTESIAN_POINT('Ctrl Pts',(-2.88303909100006,5.2,-3.04895749700002));
#320451=CARTESIAN_POINT('Ctrl Pts',(-2.88303909100006,2.2,-3.04895749700002));
#320452=CARTESIAN_POINT('Ctrl Pts',(-2.88368767300006,12.2,-3.05031777600002));
#320453=CARTESIAN_POINT('Ctrl Pts',(-2.88368767300006,5.2,-3.05031777600002));
#320454=CARTESIAN_POINT('Ctrl Pts',(-2.88368767300006,2.2,-3.05031777600002));
#320455=CARTESIAN_POINT('Ctrl Pts',(-2.88433668700006,12.2,-3.05168306000001));
#320456=CARTESIAN_POINT('Ctrl Pts',(-2.88433668700006,5.2,-3.05168306000001));
#320457=CARTESIAN_POINT('Ctrl Pts',(-2.88433668700006,2.2,-3.05168306000001));
#320458=CARTESIAN_POINT('Ctrl Pts',(-2.88498611800006,12.2,-3.05305334600002));
#320459=CARTESIAN_POINT('Ctrl Pts',(-2.88498611800006,5.2,-3.05305334600002));
#320460=CARTESIAN_POINT('Ctrl Pts',(-2.88498611800006,2.2,-3.05305334600002));
#320461=CARTESIAN_POINT('Ctrl Pts',(-2.88563595400006,12.2,-3.05442862900001));
#320462=CARTESIAN_POINT('Ctrl Pts',(-2.88563595400006,5.2,-3.05442862900001));
#320463=CARTESIAN_POINT('Ctrl Pts',(-2.88563595400006,2.2,-3.05442862900001));
#320464=CARTESIAN_POINT('Ctrl Pts',(-2.88628618200006,12.2,-3.05580890700002));
#320465=CARTESIAN_POINT('Ctrl Pts',(-2.88628618200006,5.2,-3.05580890700002));
#320466=CARTESIAN_POINT('Ctrl Pts',(-2.88628618200006,2.2,-3.05580890700002));
#320467=CARTESIAN_POINT('Ctrl Pts',(-2.88693679000006,12.2,-3.05719417500002));
#320468=CARTESIAN_POINT('Ctrl Pts',(-2.88693679000006,5.2,-3.05719417500002));
#320469=CARTESIAN_POINT('Ctrl Pts',(-2.88693679000006,2.2,-3.05719417500002));
#320470=CARTESIAN_POINT('Ctrl Pts',(-2.88758776400006,12.2,-3.05858443100002));
#320471=CARTESIAN_POINT('Ctrl Pts',(-2.88758776400006,5.2,-3.05858443100002));
#320472=CARTESIAN_POINT('Ctrl Pts',(-2.88758776400006,2.2,-3.05858443100002));
#320473=CARTESIAN_POINT('Ctrl Pts',(-2.88823909200006,12.2,-3.05997967000001));
#320474=CARTESIAN_POINT('Ctrl Pts',(-2.88823909200006,5.2,-3.05997967000001));
#320475=CARTESIAN_POINT('Ctrl Pts',(-2.88823909200006,2.2,-3.05997967000001));
#320476=CARTESIAN_POINT('Ctrl Pts',(-2.88889076200006,12.2,-3.06137989000002));
#320477=CARTESIAN_POINT('Ctrl Pts',(-2.88889076200006,5.2,-3.06137989000002));
#320478=CARTESIAN_POINT('Ctrl Pts',(-2.88889076200006,2.2,-3.06137989000002));
#320479=CARTESIAN_POINT('Ctrl Pts',(-2.88954276000006,12.2,-3.06278508700002));
#320480=CARTESIAN_POINT('Ctrl Pts',(-2.88954276000006,5.2,-3.06278508700002));
#320481=CARTESIAN_POINT('Ctrl Pts',(-2.88954276000006,2.2,-3.06278508700002));
#320482=CARTESIAN_POINT('Ctrl Pts',(-2.89019507400006,12.2,-3.06419525700001));
#320483=CARTESIAN_POINT('Ctrl Pts',(-2.89019507400006,5.2,-3.06419525700001));
#320484=CARTESIAN_POINT('Ctrl Pts',(-2.89019507400006,2.2,-3.06419525700001));
#320485=CARTESIAN_POINT('Ctrl Pts',(-2.89084769200006,12.2,-3.06561039700001));
#320486=CARTESIAN_POINT('Ctrl Pts',(-2.89084769200006,5.2,-3.06561039700001));
#320487=CARTESIAN_POINT('Ctrl Pts',(-2.89084769200006,2.2,-3.06561039700001));
#320488=CARTESIAN_POINT('Ctrl Pts',(-2.89150060100006,12.2,-3.06703050300001));
#320489=CARTESIAN_POINT('Ctrl Pts',(-2.89150060100006,5.2,-3.06703050300001));
#320490=CARTESIAN_POINT('Ctrl Pts',(-2.89150060100006,2.2,-3.06703050300001));
#320491=CARTESIAN_POINT('Ctrl Pts',(-2.89215378800006,12.2,-3.06845557200001));
#320492=CARTESIAN_POINT('Ctrl Pts',(-2.89215378800006,5.2,-3.06845557200001));
#320493=CARTESIAN_POINT('Ctrl Pts',(-2.89215378800006,2.2,-3.06845557200001));
#320494=CARTESIAN_POINT('Ctrl Pts',(-2.89280724100006,12.2,-3.06988560000002));
#320495=CARTESIAN_POINT('Ctrl Pts',(-2.89280724100006,5.2,-3.06988560000002));
#320496=CARTESIAN_POINT('Ctrl Pts',(-2.89280724100006,2.2,-3.06988560000002));
#320497=CARTESIAN_POINT('Ctrl Pts',(-2.89346094900006,12.2,-3.07132058300001));
#320498=CARTESIAN_POINT('Ctrl Pts',(-2.89346094900006,5.2,-3.07132058300001));
#320499=CARTESIAN_POINT('Ctrl Pts',(-2.89346094900006,2.2,-3.07132058300001));
#320500=CARTESIAN_POINT('Ctrl Pts',(-2.89411489600006,12.2,-3.07276051900002));
#320501=CARTESIAN_POINT('Ctrl Pts',(-2.89411489600006,5.2,-3.07276051900002));
#320502=CARTESIAN_POINT('Ctrl Pts',(-2.89411489600006,2.2,-3.07276051900002));
#320503=CARTESIAN_POINT('Ctrl Pts',(-2.89476907300006,12.2,-3.07420540200001));
#320504=CARTESIAN_POINT('Ctrl Pts',(-2.89476907300006,5.2,-3.07420540200001));
#320505=CARTESIAN_POINT('Ctrl Pts',(-2.89476907300006,2.2,-3.07420540200001));
#320506=CARTESIAN_POINT('Ctrl Pts',(-2.89542346700005,12.2,-3.07565523000001));
#320507=CARTESIAN_POINT('Ctrl Pts',(-2.89542346700005,5.2,-3.07565523000001));
#320508=CARTESIAN_POINT('Ctrl Pts',(-2.89542346700005,2.2,-3.07565523000001));
#320509=CARTESIAN_POINT('Ctrl Pts',(-2.89607806400006,12.2,-3.07711000000001));
#320510=CARTESIAN_POINT('Ctrl Pts',(-2.89607806400006,5.2,-3.07711000000001));
#320511=CARTESIAN_POINT('Ctrl Pts',(-2.89607806400006,2.2,-3.07711000000001));
#320512=CARTESIAN_POINT('Ctrl Pts',(-2.89673285300006,12.2,-3.07856970600001));
#320513=CARTESIAN_POINT('Ctrl Pts',(-2.89673285300006,5.2,-3.07856970600001));
#320514=CARTESIAN_POINT('Ctrl Pts',(-2.89673285300006,2.2,-3.07856970600001));
#320515=CARTESIAN_POINT('Ctrl Pts',(-2.89738782100006,12.2,-3.08003434700002));
#320516=CARTESIAN_POINT('Ctrl Pts',(-2.89738782100006,5.2,-3.08003434700002));
#320517=CARTESIAN_POINT('Ctrl Pts',(-2.89738782100006,2.2,-3.08003434700002));
#320518=CARTESIAN_POINT('Ctrl Pts',(-2.89804295700006,12.2,-3.08150391700002));
#320519=CARTESIAN_POINT('Ctrl Pts',(-2.89804295700006,5.2,-3.08150391700002));
#320520=CARTESIAN_POINT('Ctrl Pts',(-2.89804295700006,2.2,-3.08150391700002));
#320521=CARTESIAN_POINT('Ctrl Pts',(-2.89869824800005,12.2,-3.08297841400002));
#320522=CARTESIAN_POINT('Ctrl Pts',(-2.89869824800005,5.2,-3.08297841400002));
#320523=CARTESIAN_POINT('Ctrl Pts',(-2.89869824800005,2.2,-3.08297841400002));
#320524=CARTESIAN_POINT('Ctrl Pts',(-2.89935368200006,12.2,-3.08445783500002));
#320525=CARTESIAN_POINT('Ctrl Pts',(-2.89935368200006,5.2,-3.08445783500002));
#320526=CARTESIAN_POINT('Ctrl Pts',(-2.89935368200006,2.2,-3.08445783500002));
#320527=CARTESIAN_POINT('Ctrl Pts',(-2.90000924700006,12.2,-3.08594217400001));
#320528=CARTESIAN_POINT('Ctrl Pts',(-2.90000924700006,5.2,-3.08594217400001));
#320529=CARTESIAN_POINT('Ctrl Pts',(-2.90000924700006,2.2,-3.08594217400001));
#320530=CARTESIAN_POINT('Ctrl Pts',(-2.90066492900006,12.2,-3.08743142800001));
#320531=CARTESIAN_POINT('Ctrl Pts',(-2.90066492900006,5.2,-3.08743142800001));
#320532=CARTESIAN_POINT('Ctrl Pts',(-2.90066492900006,2.2,-3.08743142800001));
#320533=CARTESIAN_POINT('Ctrl Pts',(-2.90132071900006,12.2,-3.08892559500002));
#320534=CARTESIAN_POINT('Ctrl Pts',(-2.90132071900006,5.2,-3.08892559500002));
#320535=CARTESIAN_POINT('Ctrl Pts',(-2.90132071900006,2.2,-3.08892559500002));
#320536=CARTESIAN_POINT('Ctrl Pts',(-2.90197660300006,12.2,-3.09042467000001));
#320537=CARTESIAN_POINT('Ctrl Pts',(-2.90197660300006,5.2,-3.09042467000001));
#320538=CARTESIAN_POINT('Ctrl Pts',(-2.90197660300006,2.2,-3.09042467000001));
#320539=CARTESIAN_POINT('Ctrl Pts',(-2.90263256900006,12.2,-3.09192864800002));
#320540=CARTESIAN_POINT('Ctrl Pts',(-2.90263256900006,5.2,-3.09192864800002));
#320541=CARTESIAN_POINT('Ctrl Pts',(-2.90263256900006,2.2,-3.09192864800002));
#320542=CARTESIAN_POINT('Ctrl Pts',(-2.90328860500006,12.2,-3.09343752800002));
#320543=CARTESIAN_POINT('Ctrl Pts',(-2.90328860500006,5.2,-3.09343752800002));
#320544=CARTESIAN_POINT('Ctrl Pts',(-2.90328860500006,2.2,-3.09343752800002));
#320545=CARTESIAN_POINT('Ctrl Pts',(-2.90394470100006,12.2,-3.09495130400002));
#320546=CARTESIAN_POINT('Ctrl Pts',(-2.90394470100006,5.2,-3.09495130400002));
#320547=CARTESIAN_POINT('Ctrl Pts',(-2.90394470100006,2.2,-3.09495130400002));
#320548=CARTESIAN_POINT('Ctrl Pts',(-2.90460084100005,12.2,-3.09646997400002));
#320549=CARTESIAN_POINT('Ctrl Pts',(-2.90460084100005,5.2,-3.09646997400002));
#320550=CARTESIAN_POINT('Ctrl Pts',(-2.90460084100005,2.2,-3.09646997400002));
#320551=CARTESIAN_POINT('Ctrl Pts',(-2.90525701700005,12.2,-3.09799353300001));
#320552=CARTESIAN_POINT('Ctrl Pts',(-2.90525701700005,5.2,-3.09799353300001));
#320553=CARTESIAN_POINT('Ctrl Pts',(-2.90525701700005,2.2,-3.09799353300001));
#320554=CARTESIAN_POINT('Ctrl Pts',(-2.90591321500006,12.2,-3.09952197700001));
#320555=CARTESIAN_POINT('Ctrl Pts',(-2.90591321500006,5.2,-3.09952197700001));
#320556=CARTESIAN_POINT('Ctrl Pts',(-2.90591321500006,2.2,-3.09952197700001));
#320557=CARTESIAN_POINT('Ctrl Pts',(-2.90656942400005,12.2,-3.10105530400001));
#320558=CARTESIAN_POINT('Ctrl Pts',(-2.90656942400005,5.2,-3.10105530400001));
#320559=CARTESIAN_POINT('Ctrl Pts',(-2.90656942400005,2.2,-3.10105530400001));
#320560=CARTESIAN_POINT('Ctrl Pts',(-2.90722563100006,12.2,-3.10259350800001));
#320561=CARTESIAN_POINT('Ctrl Pts',(-2.90722563100006,5.2,-3.10259350800001));
#320562=CARTESIAN_POINT('Ctrl Pts',(-2.90722563100006,2.2,-3.10259350800001));
#320563=CARTESIAN_POINT('Ctrl Pts',(-2.90788182600005,12.2,-3.10413658700002));
#320564=CARTESIAN_POINT('Ctrl Pts',(-2.90788182600005,5.2,-3.10413658700002));
#320565=CARTESIAN_POINT('Ctrl Pts',(-2.90788182600005,2.2,-3.10413658700002));
#320566=CARTESIAN_POINT('Ctrl Pts',(-2.90853799500006,12.2,-3.10568453500002));
#320567=CARTESIAN_POINT('Ctrl Pts',(-2.90853799500006,5.2,-3.10568453500002));
#320568=CARTESIAN_POINT('Ctrl Pts',(-2.90853799500006,2.2,-3.10568453500002));
#320569=CARTESIAN_POINT('Ctrl Pts',(-2.90919412800006,12.2,-3.10723735200002));
#320570=CARTESIAN_POINT('Ctrl Pts',(-2.90919412800006,5.2,-3.10723735200002));
#320571=CARTESIAN_POINT('Ctrl Pts',(-2.90919412800006,2.2,-3.10723735200002));
#320572=CARTESIAN_POINT('Ctrl Pts',(-2.90985021200005,12.2,-3.10879503100002));
#320573=CARTESIAN_POINT('Ctrl Pts',(-2.90985021200005,5.2,-3.10879503100002));
#320574=CARTESIAN_POINT('Ctrl Pts',(-2.90985021200005,2.2,-3.10879503100002));
#320575=CARTESIAN_POINT('Ctrl Pts',(-2.91050623700006,12.2,-3.11035756900001));
#320576=CARTESIAN_POINT('Ctrl Pts',(-2.91050623700006,5.2,-3.11035756900001));
#320577=CARTESIAN_POINT('Ctrl Pts',(-2.91050623700006,2.2,-3.11035756900001));
#320578=CARTESIAN_POINT('Ctrl Pts',(-2.91116218900005,12.2,-3.11192496300002));
#320579=CARTESIAN_POINT('Ctrl Pts',(-2.91116218900005,5.2,-3.11192496300002));
#320580=CARTESIAN_POINT('Ctrl Pts',(-2.91116218900005,2.2,-3.11192496300002));
#320581=CARTESIAN_POINT('Ctrl Pts',(-2.91181805800006,12.2,-3.11349720700001));
#320582=CARTESIAN_POINT('Ctrl Pts',(-2.91181805800006,5.2,-3.11349720700001));
#320583=CARTESIAN_POINT('Ctrl Pts',(-2.91181805800006,2.2,-3.11349720700001));
#320584=CARTESIAN_POINT('Ctrl Pts',(-2.91247383300006,12.2,-3.11507429900002));
#320585=CARTESIAN_POINT('Ctrl Pts',(-2.91247383300006,5.2,-3.11507429900002));
#320586=CARTESIAN_POINT('Ctrl Pts',(-2.91247383300006,2.2,-3.11507429900002));
#320587=CARTESIAN_POINT('Ctrl Pts',(-2.91312949900006,12.2,-3.11665623500001));
#320588=CARTESIAN_POINT('Ctrl Pts',(-2.91312949900006,5.2,-3.11665623500001));
#320589=CARTESIAN_POINT('Ctrl Pts',(-2.91312949900006,2.2,-3.11665623500001));
#320590=CARTESIAN_POINT('Ctrl Pts',(-2.91378504800006,12.2,-3.11824301100001));
#320591=CARTESIAN_POINT('Ctrl Pts',(-2.91378504800006,5.2,-3.11824301100001));
#320592=CARTESIAN_POINT('Ctrl Pts',(-2.91378504800006,2.2,-3.11824301100001));
#320593=CARTESIAN_POINT('Ctrl Pts',(-2.91444046800006,12.2,-3.11983462300002));
#320594=CARTESIAN_POINT('Ctrl Pts',(-2.91444046800006,5.2,-3.11983462300002));
#320595=CARTESIAN_POINT('Ctrl Pts',(-2.91444046800006,2.2,-3.11983462300002));
#320596=CARTESIAN_POINT('Ctrl Pts',(-2.91509574500005,12.2,-3.12143106700002));
#320597=CARTESIAN_POINT('Ctrl Pts',(-2.91509574500005,5.2,-3.12143106700002));
#320598=CARTESIAN_POINT('Ctrl Pts',(-2.91509574500005,2.2,-3.12143106700002));
#320599=CARTESIAN_POINT('Ctrl Pts',(-2.91575086900006,12.2,-3.12303233800002));
#320600=CARTESIAN_POINT('Ctrl Pts',(-2.91575086900006,5.2,-3.12303233800002));
#320601=CARTESIAN_POINT('Ctrl Pts',(-2.91575086900006,2.2,-3.12303233800002));
#320602=CARTESIAN_POINT('Ctrl Pts',(-2.91640583000006,12.2,-3.12463843500002));
#320603=CARTESIAN_POINT('Ctrl Pts',(-2.91640583000006,5.2,-3.12463843500002));
#320604=CARTESIAN_POINT('Ctrl Pts',(-2.91640583000006,2.2,-3.12463843500002));
#320605=CARTESIAN_POINT('Ctrl Pts',(-2.91706061400005,12.2,-3.12624935200001));
#320606=CARTESIAN_POINT('Ctrl Pts',(-2.91706061400005,5.2,-3.12624935200001));
#320607=CARTESIAN_POINT('Ctrl Pts',(-2.91706061400005,2.2,-3.12624935200001));
#320608=CARTESIAN_POINT('Ctrl Pts',(-2.91771521100006,12.2,-3.12786508500002));
#320609=CARTESIAN_POINT('Ctrl Pts',(-2.91771521100006,5.2,-3.12786508500002));
#320610=CARTESIAN_POINT('Ctrl Pts',(-2.91771521100006,2.2,-3.12786508500002));
#320611=CARTESIAN_POINT('Ctrl Pts',(-2.91836961000006,12.2,-3.12948563000001));
#320612=CARTESIAN_POINT('Ctrl Pts',(-2.91836961000006,5.2,-3.12948563000001));
#320613=CARTESIAN_POINT('Ctrl Pts',(-2.91836961000006,2.2,-3.12948563000001));
#320614=CARTESIAN_POINT('Ctrl Pts',(-2.91902379700006,12.2,-3.13111098500002));
#320615=CARTESIAN_POINT('Ctrl Pts',(-2.91902379700006,5.2,-3.13111098500002));
#320616=CARTESIAN_POINT('Ctrl Pts',(-2.91902379700006,2.2,-3.13111098500002));
#320617=CARTESIAN_POINT('Ctrl Pts',(-2.91967776400006,12.2,-3.13274114400001));
#320618=CARTESIAN_POINT('Ctrl Pts',(-2.91967776400006,5.2,-3.13274114400001));
#320619=CARTESIAN_POINT('Ctrl Pts',(-2.91967776400006,2.2,-3.13274114400001));
#320620=CARTESIAN_POINT('Ctrl Pts',(-2.92033149900006,12.2,-3.13437610400001));
#320621=CARTESIAN_POINT('Ctrl Pts',(-2.92033149900006,5.2,-3.13437610400001));
#320622=CARTESIAN_POINT('Ctrl Pts',(-2.92033149900006,2.2,-3.13437610400001));
#320623=CARTESIAN_POINT('Ctrl Pts',(-2.92098498800006,12.2,-3.13601586100001));
#320624=CARTESIAN_POINT('Ctrl Pts',(-2.92098498800006,5.2,-3.13601586100001));
#320625=CARTESIAN_POINT('Ctrl Pts',(-2.92098498800006,2.2,-3.13601586100001));
#320626=CARTESIAN_POINT('Ctrl Pts',(-2.92163822300005,12.2,-3.13766041000001));
#320627=CARTESIAN_POINT('Ctrl Pts',(-2.92163822300005,5.2,-3.13766041000001));
#320628=CARTESIAN_POINT('Ctrl Pts',(-2.92163822300005,2.2,-3.13766041000001));
#320629=CARTESIAN_POINT('Ctrl Pts',(-2.92229119100006,12.2,-3.13930974800002));
#320630=CARTESIAN_POINT('Ctrl Pts',(-2.92229119100006,5.2,-3.13930974800002));
#320631=CARTESIAN_POINT('Ctrl Pts',(-2.92229119100006,2.2,-3.13930974800002));
#320632=CARTESIAN_POINT('Ctrl Pts',(-2.92294388100005,12.2,-3.14096387100002));
#320633=CARTESIAN_POINT('Ctrl Pts',(-2.92294388100005,5.2,-3.14096387100002));
#320634=CARTESIAN_POINT('Ctrl Pts',(-2.92294388100005,2.2,-3.14096387100002));
#320635=CARTESIAN_POINT('Ctrl Pts',(-2.92359628300006,12.2,-3.14262277500001));
#320636=CARTESIAN_POINT('Ctrl Pts',(-2.92359628300006,5.2,-3.14262277500001));
#320637=CARTESIAN_POINT('Ctrl Pts',(-2.92359628300006,2.2,-3.14262277500001));
#320638=CARTESIAN_POINT('Ctrl Pts',(-2.92424838300006,12.2,-3.14428645500001));
#320639=CARTESIAN_POINT('Ctrl Pts',(-2.92424838300006,5.2,-3.14428645500001));
#320640=CARTESIAN_POINT('Ctrl Pts',(-2.92424838300006,2.2,-3.14428645500001));
#320641=CARTESIAN_POINT('Ctrl Pts',(-2.92490017300006,12.2,-3.14595490900002));
#320642=CARTESIAN_POINT('Ctrl Pts',(-2.92490017300006,5.2,-3.14595490900002));
#320643=CARTESIAN_POINT('Ctrl Pts',(-2.92490017300006,2.2,-3.14595490900002));
#320644=CARTESIAN_POINT('Ctrl Pts',(-2.92555164100006,12.2,-3.14762813100002));
#320645=CARTESIAN_POINT('Ctrl Pts',(-2.92555164100006,5.2,-3.14762813100002));
#320646=CARTESIAN_POINT('Ctrl Pts',(-2.92555164100006,2.2,-3.14762813100002));
#320647=CARTESIAN_POINT('Ctrl Pts',(-2.92620277400006,12.2,-3.14930611800001));
#320648=CARTESIAN_POINT('Ctrl Pts',(-2.92620277400006,5.2,-3.14930611800001));
#320649=CARTESIAN_POINT('Ctrl Pts',(-2.92620277400006,2.2,-3.14930611800001));
#320650=CARTESIAN_POINT('Ctrl Pts',(-2.92685356300006,12.2,-3.15098886600001));
#320651=CARTESIAN_POINT('Ctrl Pts',(-2.92685356300006,5.2,-3.15098886600001));
#320652=CARTESIAN_POINT('Ctrl Pts',(-2.92685356300006,2.2,-3.15098886600001));
#320653=CARTESIAN_POINT('Ctrl Pts',(-2.92750399600005,12.2,-3.15267637000002));
#320654=CARTESIAN_POINT('Ctrl Pts',(-2.92750399600005,5.2,-3.15267637000002));
#320655=CARTESIAN_POINT('Ctrl Pts',(-2.92750399600005,2.2,-3.15267637000002));
#320656=CARTESIAN_POINT('Ctrl Pts',(-2.92815406200006,12.2,-3.15436862800002));
#320657=CARTESIAN_POINT('Ctrl Pts',(-2.92815406200006,5.2,-3.15436862800002));
#320658=CARTESIAN_POINT('Ctrl Pts',(-2.92815406200006,2.2,-3.15436862800002));
#320659=CARTESIAN_POINT('Ctrl Pts',(-2.92880375100005,12.2,-3.15606563300001));
#320660=CARTESIAN_POINT('Ctrl Pts',(-2.92880375100005,5.2,-3.15606563300001));
#320661=CARTESIAN_POINT('Ctrl Pts',(-2.92880375100005,2.2,-3.15606563300001));
#320662=CARTESIAN_POINT('Ctrl Pts',(-2.92945305200006,12.2,-3.15776738400002));
#320663=CARTESIAN_POINT('Ctrl Pts',(-2.92945305200006,5.2,-3.15776738400002));
#320664=CARTESIAN_POINT('Ctrl Pts',(-2.92945305200006,2.2,-3.15776738400002));
#320665=CARTESIAN_POINT('Ctrl Pts',(-2.93010195200006,12.2,-3.15947387500001));
#320666=CARTESIAN_POINT('Ctrl Pts',(-2.93010195200006,5.2,-3.15947387500001));
#320667=CARTESIAN_POINT('Ctrl Pts',(-2.93010195200006,2.2,-3.15947387500001));
#320668=CARTESIAN_POINT('Ctrl Pts',(-2.93075044200005,12.2,-3.16118510200001));
#320669=CARTESIAN_POINT('Ctrl Pts',(-2.93075044200005,5.2,-3.16118510200001));
#320670=CARTESIAN_POINT('Ctrl Pts',(-2.93075044200005,2.2,-3.16118510200001));
#320671=CARTESIAN_POINT('Ctrl Pts',(-2.93139851000006,12.2,-3.16290106200002));
#320672=CARTESIAN_POINT('Ctrl Pts',(-2.93139851000006,5.2,-3.16290106200002));
#320673=CARTESIAN_POINT('Ctrl Pts',(-2.93139851000006,2.2,-3.16290106200002));
#320674=CARTESIAN_POINT('Ctrl Pts',(-2.93204614600006,12.2,-3.16462175100002));
#320675=CARTESIAN_POINT('Ctrl Pts',(-2.93204614600006,5.2,-3.16462175100002));
#320676=CARTESIAN_POINT('Ctrl Pts',(-2.93204614600006,2.2,-3.16462175100002));
#320677=CARTESIAN_POINT('Ctrl Pts',(-2.93269333900006,12.2,-3.16634716300001));
#320678=CARTESIAN_POINT('Ctrl Pts',(-2.93269333900006,5.2,-3.16634716300001));
#320679=CARTESIAN_POINT('Ctrl Pts',(-2.93269333900006,2.2,-3.16634716300001));
#320680=CARTESIAN_POINT('Ctrl Pts',(-2.93334007700006,12.2,-3.16807729400002));
#320681=CARTESIAN_POINT('Ctrl Pts',(-2.93334007700006,5.2,-3.16807729400002));
#320682=CARTESIAN_POINT('Ctrl Pts',(-2.93334007700006,2.2,-3.16807729400002));
#320683=CARTESIAN_POINT('Ctrl Pts',(-2.93398635100006,12.2,-3.16981214300001));
#320684=CARTESIAN_POINT('Ctrl Pts',(-2.93398635100006,5.2,-3.16981214300001));
#320685=CARTESIAN_POINT('Ctrl Pts',(-2.93398635100006,2.2,-3.16981214300001));
#320686=CARTESIAN_POINT('Ctrl Pts',(-2.93463214900005,12.2,-3.17155170200001));
#320687=CARTESIAN_POINT('Ctrl Pts',(-2.93463214900005,5.2,-3.17155170200001));
#320688=CARTESIAN_POINT('Ctrl Pts',(-2.93463214900005,2.2,-3.17155170200001));
#320689=CARTESIAN_POINT('Ctrl Pts',(-2.93527746200006,12.2,-3.17329597000001));
#320690=CARTESIAN_POINT('Ctrl Pts',(-2.93527746200006,5.2,-3.17329597000001));
#320691=CARTESIAN_POINT('Ctrl Pts',(-2.93527746200006,2.2,-3.17329597000001));
#320692=CARTESIAN_POINT('Ctrl Pts',(-2.93592227600006,12.2,-3.17504494100001));
#320693=CARTESIAN_POINT('Ctrl Pts',(-2.93592227600006,5.2,-3.17504494100001));
#320694=CARTESIAN_POINT('Ctrl Pts',(-2.93592227600006,2.2,-3.17504494100001));
#320695=CARTESIAN_POINT('Ctrl Pts',(-2.93656658300006,12.2,-3.17679861200002));
#320696=CARTESIAN_POINT('Ctrl Pts',(-2.93656658300006,5.2,-3.17679861200002));
#320697=CARTESIAN_POINT('Ctrl Pts',(-2.93656658300006,2.2,-3.17679861200002));
#320698=CARTESIAN_POINT('Ctrl Pts',(-2.93721037100005,12.2,-3.17855697700002));
#320699=CARTESIAN_POINT('Ctrl Pts',(-2.93721037100005,5.2,-3.17855697700002));
#320700=CARTESIAN_POINT('Ctrl Pts',(-2.93721037100005,2.2,-3.17855697700002));
#320701=CARTESIAN_POINT('Ctrl Pts',(-2.93785363000006,12.2,-3.18032003400001));
#320702=CARTESIAN_POINT('Ctrl Pts',(-2.93785363000006,5.2,-3.18032003400001));
#320703=CARTESIAN_POINT('Ctrl Pts',(-2.93785363000006,2.2,-3.18032003400001));
#320704=CARTESIAN_POINT('Ctrl Pts',(-2.93849634900006,12.2,-3.18208777600002));
#320705=CARTESIAN_POINT('Ctrl Pts',(-2.93849634900006,5.2,-3.18208777600002));
#320706=CARTESIAN_POINT('Ctrl Pts',(-2.93849634900006,2.2,-3.18208777600002));
#320707=CARTESIAN_POINT('Ctrl Pts',(-2.93913851800006,12.2,-3.18386020300002));
#320708=CARTESIAN_POINT('Ctrl Pts',(-2.93913851800006,5.2,-3.18386020300002));
#320709=CARTESIAN_POINT('Ctrl Pts',(-2.93913851800006,2.2,-3.18386020300002));
#320710=CARTESIAN_POINT('Ctrl Pts',(-2.93978012600005,12.2,-3.18563730800001));
#320711=CARTESIAN_POINT('Ctrl Pts',(-2.93978012600005,5.2,-3.18563730800001));
#320712=CARTESIAN_POINT('Ctrl Pts',(-2.93978012600005,2.2,-3.18563730800001));
#320713=CARTESIAN_POINT('Ctrl Pts',(-2.94042116200006,12.2,-3.18741908600002));
#320714=CARTESIAN_POINT('Ctrl Pts',(-2.94042116200006,5.2,-3.18741908600002));
#320715=CARTESIAN_POINT('Ctrl Pts',(-2.94042116200006,2.2,-3.18741908600002));
#320716=CARTESIAN_POINT('Ctrl Pts',(-2.94106161700005,12.2,-3.18920553600002));
#320717=CARTESIAN_POINT('Ctrl Pts',(-2.94106161700005,5.2,-3.18920553600002));
#320718=CARTESIAN_POINT('Ctrl Pts',(-2.94106161700005,2.2,-3.18920553600002));
#320719=CARTESIAN_POINT('Ctrl Pts',(-2.94170147800005,12.2,-3.19099665100001));
#320720=CARTESIAN_POINT('Ctrl Pts',(-2.94170147800005,5.2,-3.19099665100001));
#320721=CARTESIAN_POINT('Ctrl Pts',(-2.94170147800005,2.2,-3.19099665100001));
#320722=CARTESIAN_POINT('Ctrl Pts',(-2.94234073600005,12.2,-3.19279242700001));
#320723=CARTESIAN_POINT('Ctrl Pts',(-2.94234073600005,5.2,-3.19279242700001));
#320724=CARTESIAN_POINT('Ctrl Pts',(-2.94234073600005,2.2,-3.19279242700001));
#320725=CARTESIAN_POINT('Ctrl Pts',(-2.94297938100006,12.2,-3.19459286200001));
#320726=CARTESIAN_POINT('Ctrl Pts',(-2.94297938100006,5.2,-3.19459286200001));
#320727=CARTESIAN_POINT('Ctrl Pts',(-2.94297938100006,2.2,-3.19459286200001));
#320728=CARTESIAN_POINT('Ctrl Pts',(-2.94361740100006,12.2,-3.19639794900001));
#320729=CARTESIAN_POINT('Ctrl Pts',(-2.94361740100006,5.2,-3.19639794900001));
#320730=CARTESIAN_POINT('Ctrl Pts',(-2.94361740100006,2.2,-3.19639794900001));
#320731=CARTESIAN_POINT('Ctrl Pts',(-2.94425478800005,12.2,-3.19820768600001));
#320732=CARTESIAN_POINT('Ctrl Pts',(-2.94425478800005,5.2,-3.19820768600001));
#320733=CARTESIAN_POINT('Ctrl Pts',(-2.94425478800005,2.2,-3.19820768600001));
#320734=CARTESIAN_POINT('Ctrl Pts',(-2.94489152800006,12.2,-3.20002206700002));
#320735=CARTESIAN_POINT('Ctrl Pts',(-2.94489152800006,5.2,-3.20002206700002));
#320736=CARTESIAN_POINT('Ctrl Pts',(-2.94489152800006,2.2,-3.20002206700002));
#320737=CARTESIAN_POINT('Ctrl Pts',(-2.94552761500006,12.2,-3.20184108900001));
#320738=CARTESIAN_POINT('Ctrl Pts',(-2.94552761500006,5.2,-3.20184108900001));
#320739=CARTESIAN_POINT('Ctrl Pts',(-2.94552761500006,2.2,-3.20184108900001));
#320740=CARTESIAN_POINT('Ctrl Pts',(-2.94616303400006,12.2,-3.20366474800001));
#320741=CARTESIAN_POINT('Ctrl Pts',(-2.94616303400006,5.2,-3.20366474800001));
#320742=CARTESIAN_POINT('Ctrl Pts',(-2.94616303400006,2.2,-3.20366474800001));
#320743=CARTESIAN_POINT('Ctrl Pts',(-2.94679777900006,12.2,-3.20549303700002));
#320744=CARTESIAN_POINT('Ctrl Pts',(-2.94679777900006,5.2,-3.20549303700002));
#320745=CARTESIAN_POINT('Ctrl Pts',(-2.94679777900006,2.2,-3.20549303700002));
#320746=CARTESIAN_POINT('Ctrl Pts',(-2.94743183700006,12.2,-3.20732595500001));
#320747=CARTESIAN_POINT('Ctrl Pts',(-2.94743183700006,5.2,-3.20732595500001));
#320748=CARTESIAN_POINT('Ctrl Pts',(-2.94743183700006,2.2,-3.20732595500001));
#320749=CARTESIAN_POINT('Ctrl Pts',(-2.94806519800006,12.2,-3.20916349600001));
#320750=CARTESIAN_POINT('Ctrl Pts',(-2.94806519800006,5.2,-3.20916349600001));
#320751=CARTESIAN_POINT('Ctrl Pts',(-2.94806519800006,2.2,-3.20916349600001));
#320752=CARTESIAN_POINT('Ctrl Pts',(-2.94869785300006,12.2,-3.21100565700001));
#320753=CARTESIAN_POINT('Ctrl Pts',(-2.94869785300006,5.2,-3.21100565700001));
#320754=CARTESIAN_POINT('Ctrl Pts',(-2.94869785300006,2.2,-3.21100565700001));
#320755=CARTESIAN_POINT('Ctrl Pts',(-2.94932979000006,12.2,-3.21285243200002));
#320756=CARTESIAN_POINT('Ctrl Pts',(-2.94932979000006,5.2,-3.21285243200002));
#320757=CARTESIAN_POINT('Ctrl Pts',(-2.94932979000006,2.2,-3.21285243200002));
#320758=CARTESIAN_POINT('Ctrl Pts',(-2.94996099900006,12.2,-3.21470381800002));
#320759=CARTESIAN_POINT('Ctrl Pts',(-2.94996099900006,5.2,-3.21470381800002));
#320760=CARTESIAN_POINT('Ctrl Pts',(-2.94996099900006,2.2,-3.21470381800002));
#320761=CARTESIAN_POINT('Ctrl Pts',(-2.95059147200006,12.2,-3.21655981000001));
#320762=CARTESIAN_POINT('Ctrl Pts',(-2.95059147200006,5.2,-3.21655981000001));
#320763=CARTESIAN_POINT('Ctrl Pts',(-2.95059147200006,2.2,-3.21655981000001));
#320764=CARTESIAN_POINT('Ctrl Pts',(-2.95122119700005,12.2,-3.21842040400002));
#320765=CARTESIAN_POINT('Ctrl Pts',(-2.95122119700005,5.2,-3.21842040400002));
#320766=CARTESIAN_POINT('Ctrl Pts',(-2.95122119700005,2.2,-3.21842040400002));
#320767=CARTESIAN_POINT('Ctrl Pts',(-2.95185016300006,12.2,-3.22028559600001));
#320768=CARTESIAN_POINT('Ctrl Pts',(-2.95185016300006,5.2,-3.22028559600001));
#320769=CARTESIAN_POINT('Ctrl Pts',(-2.95185016300006,2.2,-3.22028559600001));
#320770=CARTESIAN_POINT('Ctrl Pts',(-2.95247836200006,12.2,-3.22215538200001));
#320771=CARTESIAN_POINT('Ctrl Pts',(-2.95247836200006,5.2,-3.22215538200001));
#320772=CARTESIAN_POINT('Ctrl Pts',(-2.95247836200006,2.2,-3.22215538200001));
#320773=CARTESIAN_POINT('Ctrl Pts',(-2.95310578300006,12.2,-3.22402975500002));
#320774=CARTESIAN_POINT('Ctrl Pts',(-2.95310578300006,5.2,-3.22402975500002));
#320775=CARTESIAN_POINT('Ctrl Pts',(-2.95310578300006,2.2,-3.22402975500002));
#320776=CARTESIAN_POINT('Ctrl Pts',(-2.95373241500006,12.2,-3.22590871400001));
#320777=CARTESIAN_POINT('Ctrl Pts',(-2.95373241500006,5.2,-3.22590871400001));
#320778=CARTESIAN_POINT('Ctrl Pts',(-2.95373241500006,2.2,-3.22590871400001));
#320779=CARTESIAN_POINT('Ctrl Pts',(-2.95435824900005,12.2,-3.22779225300001));
#320780=CARTESIAN_POINT('Ctrl Pts',(-2.95435824900005,5.2,-3.22779225300001));
#320781=CARTESIAN_POINT('Ctrl Pts',(-2.95435824900005,2.2,-3.22779225300001));
#320782=CARTESIAN_POINT('Ctrl Pts',(-2.95498327600006,12.2,-3.22968036800001));
#320783=CARTESIAN_POINT('Ctrl Pts',(-2.95498327600006,5.2,-3.22968036800001));
#320784=CARTESIAN_POINT('Ctrl Pts',(-2.95498327600006,2.2,-3.22968036800001));
#320785=CARTESIAN_POINT('Ctrl Pts',(-2.95560748300006,12.2,-3.23157305400001));
#320786=CARTESIAN_POINT('Ctrl Pts',(-2.95560748300006,5.2,-3.23157305400001));
#320787=CARTESIAN_POINT('Ctrl Pts',(-2.95560748300006,2.2,-3.23157305400001));
#320788=CARTESIAN_POINT('Ctrl Pts',(-2.95623086300006,12.2,-3.23347030800001));
#320789=CARTESIAN_POINT('Ctrl Pts',(-2.95623086300006,5.2,-3.23347030800001));
#320790=CARTESIAN_POINT('Ctrl Pts',(-2.95623086300006,2.2,-3.23347030800001));
#320791=CARTESIAN_POINT('Ctrl Pts',(-2.95685340400006,12.2,-3.23537212400002));
#320792=CARTESIAN_POINT('Ctrl Pts',(-2.95685340400006,5.2,-3.23537212400002));
#320793=CARTESIAN_POINT('Ctrl Pts',(-2.95685340400006,2.2,-3.23537212400002));
#320794=CARTESIAN_POINT('Ctrl Pts',(-2.95747509600006,12.2,-3.23727849900001));
#320795=CARTESIAN_POINT('Ctrl Pts',(-2.95747509600006,5.2,-3.23727849900001));
#320796=CARTESIAN_POINT('Ctrl Pts',(-2.95747509600006,2.2,-3.23727849900001));
#320797=CARTESIAN_POINT('Ctrl Pts',(-2.95809593100006,12.2,-3.23918942800002));
#320798=CARTESIAN_POINT('Ctrl Pts',(-2.95809593100006,5.2,-3.23918942800002));
#320799=CARTESIAN_POINT('Ctrl Pts',(-2.95809593100006,2.2,-3.23918942800002));
#320800=CARTESIAN_POINT('Ctrl Pts',(-2.95871589700006,12.2,-3.24110490600001));
#320801=CARTESIAN_POINT('Ctrl Pts',(-2.95871589700006,5.2,-3.24110490600001));
#320802=CARTESIAN_POINT('Ctrl Pts',(-2.95871589700006,2.2,-3.24110490600001));
#320803=CARTESIAN_POINT('Ctrl Pts',(-2.95933498600006,12.2,-3.24302493100001));
#320804=CARTESIAN_POINT('Ctrl Pts',(-2.95933498600006,5.2,-3.24302493100001));
#320805=CARTESIAN_POINT('Ctrl Pts',(-2.95933498600006,2.2,-3.24302493100001));
#320806=CARTESIAN_POINT('Ctrl Pts',(-2.95995318600006,12.2,-3.24494949500002));
#320807=CARTESIAN_POINT('Ctrl Pts',(-2.95995318600006,5.2,-3.24494949500002));
#320808=CARTESIAN_POINT('Ctrl Pts',(-2.95995318600006,2.2,-3.24494949500002));
#320809=CARTESIAN_POINT('Ctrl Pts',(-2.96057048900006,12.2,-3.24687859600001));
#320810=CARTESIAN_POINT('Ctrl Pts',(-2.96057048900006,5.2,-3.24687859600001));
#320811=CARTESIAN_POINT('Ctrl Pts',(-2.96057048900006,2.2,-3.24687859600001));
#320812=CARTESIAN_POINT('Ctrl Pts',(-2.96118688400006,12.2,-3.24881223000002));
#320813=CARTESIAN_POINT('Ctrl Pts',(-2.96118688400006,5.2,-3.24881223000002));
#320814=CARTESIAN_POINT('Ctrl Pts',(-2.96118688400006,2.2,-3.24881223000002));
#320815=CARTESIAN_POINT('Ctrl Pts',(-2.96180236200006,12.2,-3.25075039000001));
#320816=CARTESIAN_POINT('Ctrl Pts',(-2.96180236200006,5.2,-3.25075039000001));
#320817=CARTESIAN_POINT('Ctrl Pts',(-2.96180236200006,2.2,-3.25075039000001));
#320818=CARTESIAN_POINT('Ctrl Pts',(-2.96241691300006,12.2,-3.25269307400001));
#320819=CARTESIAN_POINT('Ctrl Pts',(-2.96241691300006,5.2,-3.25269307400001));
#320820=CARTESIAN_POINT('Ctrl Pts',(-2.96241691300006,2.2,-3.25269307400001));
#320821=CARTESIAN_POINT('Ctrl Pts',(-2.96303052700006,12.2,-3.25464027700002));
#320822=CARTESIAN_POINT('Ctrl Pts',(-2.96303052700006,5.2,-3.25464027700002));
#320823=CARTESIAN_POINT('Ctrl Pts',(-2.96303052700006,2.2,-3.25464027700002));
#320824=CARTESIAN_POINT('Ctrl Pts',(-2.96364319400006,12.2,-3.25659199500001));
#320825=CARTESIAN_POINT('Ctrl Pts',(-2.96364319400006,5.2,-3.25659199500001));
#320826=CARTESIAN_POINT('Ctrl Pts',(-2.96364319400006,2.2,-3.25659199500001));
#320827=CARTESIAN_POINT('Ctrl Pts',(-2.96425490500006,12.2,-3.25854822100001));
#320828=CARTESIAN_POINT('Ctrl Pts',(-2.96425490500006,5.2,-3.25854822100001));
#320829=CARTESIAN_POINT('Ctrl Pts',(-2.96425490500006,2.2,-3.25854822100001));
#320830=CARTESIAN_POINT('Ctrl Pts',(-2.96486565000006,12.2,-3.26050895400002));
#320831=CARTESIAN_POINT('Ctrl Pts',(-2.96486565000006,5.2,-3.26050895400002));
#320832=CARTESIAN_POINT('Ctrl Pts',(-2.96486565000006,2.2,-3.26050895400002));
#320833=CARTESIAN_POINT('Ctrl Pts',(-2.96547541900006,12.2,-3.26247418600001));
#320834=CARTESIAN_POINT('Ctrl Pts',(-2.96547541900006,5.2,-3.26247418600001));
#320835=CARTESIAN_POINT('Ctrl Pts',(-2.96547541900006,2.2,-3.26247418600001));
#320836=CARTESIAN_POINT('Ctrl Pts',(-2.96608420300006,12.2,-3.26444391600001));
#320837=CARTESIAN_POINT('Ctrl Pts',(-2.96608420300006,5.2,-3.26444391600001));
#320838=CARTESIAN_POINT('Ctrl Pts',(-2.96608420300006,2.2,-3.26444391600001));
#320839=CARTESIAN_POINT('Ctrl Pts',(-2.96669199100006,12.2,-3.26641813800002));
#320840=CARTESIAN_POINT('Ctrl Pts',(-2.96669199100006,5.2,-3.26641813800002));
#320841=CARTESIAN_POINT('Ctrl Pts',(-2.96669199100006,2.2,-3.26641813800002));
#320842=CARTESIAN_POINT('Ctrl Pts',(-2.96729877500006,12.2,-3.26839684700001));
#320843=CARTESIAN_POINT('Ctrl Pts',(-2.96729877500006,5.2,-3.26839684700001));
#320844=CARTESIAN_POINT('Ctrl Pts',(-2.96729877500006,2.2,-3.26839684700001));
#320845=CARTESIAN_POINT('Ctrl Pts',(-2.96790454500006,12.2,-3.27038003900002));
#320846=CARTESIAN_POINT('Ctrl Pts',(-2.96790454500006,5.2,-3.27038003900002));
#320847=CARTESIAN_POINT('Ctrl Pts',(-2.96790454500006,2.2,-3.27038003900002));
#320848=CARTESIAN_POINT('Ctrl Pts',(-2.96850929200006,12.2,-3.27236770900001));
#320849=CARTESIAN_POINT('Ctrl Pts',(-2.96850929200006,5.2,-3.27236770900001));
#320850=CARTESIAN_POINT('Ctrl Pts',(-2.96850929200006,2.2,-3.27236770900001));
#320851=CARTESIAN_POINT('Ctrl Pts',(-2.96911300500006,12.2,-3.27435985300002));
#320852=CARTESIAN_POINT('Ctrl Pts',(-2.96911300500006,5.2,-3.27435985300002));
#320853=CARTESIAN_POINT('Ctrl Pts',(-2.96911300500006,2.2,-3.27435985300002));
#320854=CARTESIAN_POINT('Ctrl Pts',(-2.96971567500006,12.2,-3.27635646800001));
#320855=CARTESIAN_POINT('Ctrl Pts',(-2.96971567500006,5.2,-3.27635646800001));
#320856=CARTESIAN_POINT('Ctrl Pts',(-2.96971567500006,2.2,-3.27635646800001));
#320857=CARTESIAN_POINT('Ctrl Pts',(-2.97031729300006,12.2,-3.27835754600001));
#320858=CARTESIAN_POINT('Ctrl Pts',(-2.97031729300006,5.2,-3.27835754600001));
#320859=CARTESIAN_POINT('Ctrl Pts',(-2.97031729300006,2.2,-3.27835754600001));
#320860=CARTESIAN_POINT('Ctrl Pts',(-2.97091784700006,12.2,-3.28036308600002));
#320861=CARTESIAN_POINT('Ctrl Pts',(-2.97091784700006,5.2,-3.28036308600002));
#320862=CARTESIAN_POINT('Ctrl Pts',(-2.97091784700006,2.2,-3.28036308600002));
#320863=CARTESIAN_POINT('Ctrl Pts',(-2.97151733200006,12.2,-3.28237308100002));
#320864=CARTESIAN_POINT('Ctrl Pts',(-2.97151733200006,5.2,-3.28237308100002));
#320865=CARTESIAN_POINT('Ctrl Pts',(-2.97151733200006,2.2,-3.28237308100002));
#320866=CARTESIAN_POINT('Ctrl Pts',(-2.97211573600006,12.2,-3.28438752800002));
#320867=CARTESIAN_POINT('Ctrl Pts',(-2.97211573600006,5.2,-3.28438752800002));
#320868=CARTESIAN_POINT('Ctrl Pts',(-2.97211573600006,2.2,-3.28438752800002));
#320869=CARTESIAN_POINT('Ctrl Pts',(-2.97271304900006,12.2,-3.28640642100002));
#320870=CARTESIAN_POINT('Ctrl Pts',(-2.97271304900006,5.2,-3.28640642100002));
#320871=CARTESIAN_POINT('Ctrl Pts',(-2.97271304900006,2.2,-3.28640642100002));
#320872=CARTESIAN_POINT('Ctrl Pts',(-2.97330926200006,12.2,-3.28842975700002));
#320873=CARTESIAN_POINT('Ctrl Pts',(-2.97330926200006,5.2,-3.28842975700002));
#320874=CARTESIAN_POINT('Ctrl Pts',(-2.97330926200006,2.2,-3.28842975700002));
#320875=CARTESIAN_POINT('Ctrl Pts',(-2.97390436700006,12.2,-3.29045753100001));
#320876=CARTESIAN_POINT('Ctrl Pts',(-2.97390436700006,5.2,-3.29045753100001));
#320877=CARTESIAN_POINT('Ctrl Pts',(-2.97390436700006,2.2,-3.29045753100001));
#320878=CARTESIAN_POINT('Ctrl Pts',(-2.97449835400006,12.2,-3.29248973700001));
#320879=CARTESIAN_POINT('Ctrl Pts',(-2.97449835400006,5.2,-3.29248973700001));
#320880=CARTESIAN_POINT('Ctrl Pts',(-2.97449835400006,2.2,-3.29248973700001));
#320881=CARTESIAN_POINT('Ctrl Pts',(-2.97509121300005,12.2,-3.29452637300002));
#320882=CARTESIAN_POINT('Ctrl Pts',(-2.97509121300005,5.2,-3.29452637300002));
#320883=CARTESIAN_POINT('Ctrl Pts',(-2.97509121300005,2.2,-3.29452637300002));
#320884=CARTESIAN_POINT('Ctrl Pts',(-2.97568293500006,12.2,-3.29656743200001));
#320885=CARTESIAN_POINT('Ctrl Pts',(-2.97568293500006,5.2,-3.29656743200001));
#320886=CARTESIAN_POINT('Ctrl Pts',(-2.97568293500006,2.2,-3.29656743200001));
#320887=CARTESIAN_POINT('Ctrl Pts',(-2.97627351000005,12.2,-3.29861291100002));
#320888=CARTESIAN_POINT('Ctrl Pts',(-2.97627351000005,5.2,-3.29861291100002));
#320889=CARTESIAN_POINT('Ctrl Pts',(-2.97627351000005,2.2,-3.29861291100002));
#320890=CARTESIAN_POINT('Ctrl Pts',(-2.97686292900006,12.2,-3.30066280500001));
#320891=CARTESIAN_POINT('Ctrl Pts',(-2.97686292900006,5.2,-3.30066280500001));
#320892=CARTESIAN_POINT('Ctrl Pts',(-2.97686292900006,2.2,-3.30066280500001));
#320893=CARTESIAN_POINT('Ctrl Pts',(-2.97745118400006,12.2,-3.30271710800002));
#320894=CARTESIAN_POINT('Ctrl Pts',(-2.97745118400006,5.2,-3.30271710800002));
#320895=CARTESIAN_POINT('Ctrl Pts',(-2.97745118400006,2.2,-3.30271710800002));
#320896=CARTESIAN_POINT('Ctrl Pts',(-2.97803826500005,12.2,-3.30477581800002));
#320897=CARTESIAN_POINT('Ctrl Pts',(-2.97803826500005,5.2,-3.30477581800002));
#320898=CARTESIAN_POINT('Ctrl Pts',(-2.97803826500005,2.2,-3.30477581800002));
#320899=CARTESIAN_POINT('Ctrl Pts',(-2.97862416200006,12.2,-3.30683892800002));
#320900=CARTESIAN_POINT('Ctrl Pts',(-2.97862416200006,5.2,-3.30683892800002));
#320901=CARTESIAN_POINT('Ctrl Pts',(-2.97862416200006,2.2,-3.30683892800002));
#320902=CARTESIAN_POINT('Ctrl Pts',(-2.97920886600005,12.2,-3.30890643600001));
#320903=CARTESIAN_POINT('Ctrl Pts',(-2.97920886600005,5.2,-3.30890643600001));
#320904=CARTESIAN_POINT('Ctrl Pts',(-2.97920886600005,2.2,-3.30890643600001));
#320905=CARTESIAN_POINT('Ctrl Pts',(-2.97979236900006,12.2,-3.31097833600001));
#320906=CARTESIAN_POINT('Ctrl Pts',(-2.97979236900006,5.2,-3.31097833600001));
#320907=CARTESIAN_POINT('Ctrl Pts',(-2.97979236900006,2.2,-3.31097833600001));
#320908=CARTESIAN_POINT('Ctrl Pts',(-2.98037466100005,12.2,-3.31305462200001));
#320909=CARTESIAN_POINT('Ctrl Pts',(-2.98037466100005,5.2,-3.31305462200001));
#320910=CARTESIAN_POINT('Ctrl Pts',(-2.98037466100005,2.2,-3.31305462200001));
#320911=CARTESIAN_POINT('Ctrl Pts',(-2.98095573300006,12.2,-3.31513529200001));
#320912=CARTESIAN_POINT('Ctrl Pts',(-2.98095573300006,5.2,-3.31513529200001));
#320913=CARTESIAN_POINT('Ctrl Pts',(-2.98095573300006,2.2,-3.31513529200001));
#320914=CARTESIAN_POINT('Ctrl Pts',(-2.98153557700005,12.2,-3.31722033900002));
#320915=CARTESIAN_POINT('Ctrl Pts',(-2.98153557700005,5.2,-3.31722033900002));
#320916=CARTESIAN_POINT('Ctrl Pts',(-2.98153557700005,2.2,-3.31722033900002));
#320917=CARTESIAN_POINT('Ctrl Pts',(-2.98211418100006,12.2,-3.31930976000002));
#320918=CARTESIAN_POINT('Ctrl Pts',(-2.98211418100006,5.2,-3.31930976000002));
#320919=CARTESIAN_POINT('Ctrl Pts',(-2.98211418100006,2.2,-3.31930976000002));
#320920=CARTESIAN_POINT('Ctrl Pts',(-2.98269153900006,12.2,-3.32140354900002));
#320921=CARTESIAN_POINT('Ctrl Pts',(-2.98269153900006,5.2,-3.32140354900002));
#320922=CARTESIAN_POINT('Ctrl Pts',(-2.98269153900006,2.2,-3.32140354900002));
#320923=CARTESIAN_POINT('Ctrl Pts',(-2.98326763900006,12.2,-3.32350170300002));
#320924=CARTESIAN_POINT('Ctrl Pts',(-2.98326763900006,5.2,-3.32350170300002));
#320925=CARTESIAN_POINT('Ctrl Pts',(-2.98326763900006,2.2,-3.32350170300002));
#320926=CARTESIAN_POINT('Ctrl Pts',(-2.98384247500006,12.2,-3.32560421600002));
#320927=CARTESIAN_POINT('Ctrl Pts',(-2.98384247500006,5.2,-3.32560421600002));
#320928=CARTESIAN_POINT('Ctrl Pts',(-2.98384247500006,2.2,-3.32560421600002));
#320929=CARTESIAN_POINT('Ctrl Pts',(-2.98441603600006,12.2,-3.32771108400001));
#320930=CARTESIAN_POINT('Ctrl Pts',(-2.98441603600006,5.2,-3.32771108400001));
#320931=CARTESIAN_POINT('Ctrl Pts',(-2.98441603600006,2.2,-3.32771108400001));
#320932=CARTESIAN_POINT('Ctrl Pts',(-2.98498831300006,12.2,-3.32982230300002));
#320933=CARTESIAN_POINT('Ctrl Pts',(-2.98498831300006,5.2,-3.32982230300002));
#320934=CARTESIAN_POINT('Ctrl Pts',(-2.98498831300006,2.2,-3.32982230300002));
#320935=CARTESIAN_POINT('Ctrl Pts',(-2.98555929700006,12.2,-3.33193786600001));
#320936=CARTESIAN_POINT('Ctrl Pts',(-2.98555929700006,5.2,-3.33193786600001));
#320937=CARTESIAN_POINT('Ctrl Pts',(-2.98555929700006,2.2,-3.33193786600001));
#320938=CARTESIAN_POINT('Ctrl Pts',(-2.98612898100005,12.2,-3.33405777100001));
#320939=CARTESIAN_POINT('Ctrl Pts',(-2.98612898100005,5.2,-3.33405777100001));
#320940=CARTESIAN_POINT('Ctrl Pts',(-2.98612898100005,2.2,-3.33405777100001));
#320941=CARTESIAN_POINT('Ctrl Pts',(-2.98669735400006,12.2,-3.33618201100002));
#320942=CARTESIAN_POINT('Ctrl Pts',(-2.98669735400006,5.2,-3.33618201100002));
#320943=CARTESIAN_POINT('Ctrl Pts',(-2.98669735400006,2.2,-3.33618201100002));
#320944=CARTESIAN_POINT('Ctrl Pts',(-2.98726440700006,12.2,-3.33831058400001));
#320945=CARTESIAN_POINT('Ctrl Pts',(-2.98726440700006,5.2,-3.33831058400001));
#320946=CARTESIAN_POINT('Ctrl Pts',(-2.98726440700006,2.2,-3.33831058400001));
#320947=CARTESIAN_POINT('Ctrl Pts',(-2.98783013300006,12.2,-3.34044348300001));
#320948=CARTESIAN_POINT('Ctrl Pts',(-2.98783013300006,5.2,-3.34044348300001));
#320949=CARTESIAN_POINT('Ctrl Pts',(-2.98783013300006,2.2,-3.34044348300001));
#320950=CARTESIAN_POINT('Ctrl Pts',(-2.98839452200005,12.2,-3.34258070300002));
#320951=CARTESIAN_POINT('Ctrl Pts',(-2.98839452200005,5.2,-3.34258070300002));
#320952=CARTESIAN_POINT('Ctrl Pts',(-2.98839452200005,2.2,-3.34258070300002));
#320953=CARTESIAN_POINT('Ctrl Pts',(-2.98895756400006,12.2,-3.34472224200002));
#320954=CARTESIAN_POINT('Ctrl Pts',(-2.98895756400006,5.2,-3.34472224200002));
#320955=CARTESIAN_POINT('Ctrl Pts',(-2.98895756400006,2.2,-3.34472224200002));
#320956=CARTESIAN_POINT('Ctrl Pts',(-2.98951925100006,12.2,-3.34686809300001));
#320957=CARTESIAN_POINT('Ctrl Pts',(-2.98951925100006,5.2,-3.34686809300001));
#320958=CARTESIAN_POINT('Ctrl Pts',(-2.98951925100006,2.2,-3.34686809300001));
#320959=CARTESIAN_POINT('Ctrl Pts',(-2.99007957400006,12.2,-3.34901825200001));
#320960=CARTESIAN_POINT('Ctrl Pts',(-2.99007957400006,5.2,-3.34901825200001));
#320961=CARTESIAN_POINT('Ctrl Pts',(-2.99007957400006,2.2,-3.34901825200001));
#320962=CARTESIAN_POINT('Ctrl Pts',(-2.99063852600006,12.2,-3.35117271400001));
#320963=CARTESIAN_POINT('Ctrl Pts',(-2.99063852600006,5.2,-3.35117271400001));
#320964=CARTESIAN_POINT('Ctrl Pts',(-2.99063852600006,2.2,-3.35117271400001));
#320965=CARTESIAN_POINT('Ctrl Pts',(-2.99119609600006,12.2,-3.35333147500001));
#320966=CARTESIAN_POINT('Ctrl Pts',(-2.99119609600006,5.2,-3.35333147500001));
#320967=CARTESIAN_POINT('Ctrl Pts',(-2.99119609600006,2.2,-3.35333147500001));
#320968=CARTESIAN_POINT('Ctrl Pts',(-2.99175227600006,12.2,-3.35549453000001));
#320969=CARTESIAN_POINT('Ctrl Pts',(-2.99175227600006,5.2,-3.35549453000001));
#320970=CARTESIAN_POINT('Ctrl Pts',(-2.99175227600006,2.2,-3.35549453000001));
#320971=CARTESIAN_POINT('Ctrl Pts',(-2.99230705700006,12.2,-3.35766187400001));
#320972=CARTESIAN_POINT('Ctrl Pts',(-2.99230705700006,5.2,-3.35766187400001));
#320973=CARTESIAN_POINT('Ctrl Pts',(-2.99230705700006,2.2,-3.35766187400001));
#320974=CARTESIAN_POINT('Ctrl Pts',(-2.99286043000006,12.2,-3.35983350200001));
#320975=CARTESIAN_POINT('Ctrl Pts',(-2.99286043000006,5.2,-3.35983350200001));
#320976=CARTESIAN_POINT('Ctrl Pts',(-2.99286043000006,2.2,-3.35983350200001));
#320977=CARTESIAN_POINT('Ctrl Pts',(-2.99341238800006,12.2,-3.36200941000001));
#320978=CARTESIAN_POINT('Ctrl Pts',(-2.99341238800006,5.2,-3.36200941000001));
#320979=CARTESIAN_POINT('Ctrl Pts',(-2.99341238800006,2.2,-3.36200941000001));
#320980=CARTESIAN_POINT('Ctrl Pts',(-2.99396292000006,12.2,-3.36418959200001));
#320981=CARTESIAN_POINT('Ctrl Pts',(-2.99396292000006,5.2,-3.36418959200001));
#320982=CARTESIAN_POINT('Ctrl Pts',(-2.99396292000006,2.2,-3.36418959200001));
#320983=CARTESIAN_POINT('Ctrl Pts',(-2.99451201800006,12.2,-3.36637404500001));
#320984=CARTESIAN_POINT('Ctrl Pts',(-2.99451201800006,5.2,-3.36637404500001));
#320985=CARTESIAN_POINT('Ctrl Pts',(-2.99451201800006,2.2,-3.36637404500001));
#320986=CARTESIAN_POINT('Ctrl Pts',(-2.99505967500005,12.2,-3.36856276300002));
#320987=CARTESIAN_POINT('Ctrl Pts',(-2.99505967500005,5.2,-3.36856276300002));
#320988=CARTESIAN_POINT('Ctrl Pts',(-2.99505967500005,2.2,-3.36856276300002));
#320989=CARTESIAN_POINT('Ctrl Pts',(-2.99560588000006,12.2,-3.37075574200002));
#320990=CARTESIAN_POINT('Ctrl Pts',(-2.99560588000006,5.2,-3.37075574200002));
#320991=CARTESIAN_POINT('Ctrl Pts',(-2.99560588000006,2.2,-3.37075574200002));
#320992=CARTESIAN_POINT('Ctrl Pts',(-2.99615062600005,12.2,-3.37295297600001));
#320993=CARTESIAN_POINT('Ctrl Pts',(-2.99615062600005,5.2,-3.37295297600001));
#320994=CARTESIAN_POINT('Ctrl Pts',(-2.99615062600005,2.2,-3.37295297600001));
#320995=CARTESIAN_POINT('Ctrl Pts',(-2.99669390300005,12.2,-3.37515446200001));
#320996=CARTESIAN_POINT('Ctrl Pts',(-2.99669390300005,5.2,-3.37515446200001));
#320997=CARTESIAN_POINT('Ctrl Pts',(-2.99669390300005,2.2,-3.37515446200001));
#320998=CARTESIAN_POINT('Ctrl Pts',(-2.99723570400006,12.2,-3.37736019300001));
#320999=CARTESIAN_POINT('Ctrl Pts',(-2.99723570400006,5.2,-3.37736019300001));
#321000=CARTESIAN_POINT('Ctrl Pts',(-2.99723570400006,2.2,-3.37736019300001));
#321001=CARTESIAN_POINT('Ctrl Pts',(-2.99777601900006,12.2,-3.37957016700001));
#321002=CARTESIAN_POINT('Ctrl Pts',(-2.99777601900006,5.2,-3.37957016700001));
#321003=CARTESIAN_POINT('Ctrl Pts',(-2.99777601900006,2.2,-3.37957016700001));
#321004=CARTESIAN_POINT('Ctrl Pts',(-2.99831484100006,12.2,-3.38178437700002));
#321005=CARTESIAN_POINT('Ctrl Pts',(-2.99831484100006,5.2,-3.38178437700002));
#321006=CARTESIAN_POINT('Ctrl Pts',(-2.99831484100006,2.2,-3.38178437700002));
#321007=CARTESIAN_POINT('Ctrl Pts',(-2.99885216000006,12.2,-3.38400281900002));
#321008=CARTESIAN_POINT('Ctrl Pts',(-2.99885216000006,5.2,-3.38400281900002));
#321009=CARTESIAN_POINT('Ctrl Pts',(-2.99885216000006,2.2,-3.38400281900002));
#321010=CARTESIAN_POINT('Ctrl Pts',(-2.99938796800005,12.2,-3.38622548900001));
#321011=CARTESIAN_POINT('Ctrl Pts',(-2.99938796800005,5.2,-3.38622548900001));
#321012=CARTESIAN_POINT('Ctrl Pts',(-2.99938796800005,2.2,-3.38622548900001));
#321013=CARTESIAN_POINT('Ctrl Pts',(-2.99992225700006,12.2,-3.38845237900002));
#321014=CARTESIAN_POINT('Ctrl Pts',(-2.99992225700006,5.2,-3.38845237900002));
#321015=CARTESIAN_POINT('Ctrl Pts',(-2.99992225700006,2.2,-3.38845237900002));
#321016=CARTESIAN_POINT('Ctrl Pts',(-3.00045501800006,12.2,-3.39068348900001));
#321017=CARTESIAN_POINT('Ctrl Pts',(-3.00045501800006,5.2,-3.39068348900001));
#321018=CARTESIAN_POINT('Ctrl Pts',(-3.00045501800006,2.2,-3.39068348900001));
#321019=CARTESIAN_POINT('Ctrl Pts',(-3.00098624200006,12.2,-3.39291881100001));
#321020=CARTESIAN_POINT('Ctrl Pts',(-3.00098624200006,5.2,-3.39291881100001));
#321021=CARTESIAN_POINT('Ctrl Pts',(-3.00098624200006,2.2,-3.39291881100001));
#321022=CARTESIAN_POINT('Ctrl Pts',(-3.00151592200006,12.2,-3.39515834000002));
#321023=CARTESIAN_POINT('Ctrl Pts',(-3.00151592200006,5.2,-3.39515834000002));
#321024=CARTESIAN_POINT('Ctrl Pts',(-3.00151592200006,2.2,-3.39515834000002));
#321025=CARTESIAN_POINT('Ctrl Pts',(-3.00204404800006,12.2,-3.39740207200002));
#321026=CARTESIAN_POINT('Ctrl Pts',(-3.00204404800006,5.2,-3.39740207200002));
#321027=CARTESIAN_POINT('Ctrl Pts',(-3.00204404800006,2.2,-3.39740207200002));
#321028=CARTESIAN_POINT('Ctrl Pts',(-3.00257061300006,12.2,-3.39965000400001));
#321029=CARTESIAN_POINT('Ctrl Pts',(-3.00257061300006,5.2,-3.39965000400001));
#321030=CARTESIAN_POINT('Ctrl Pts',(-3.00257061300006,2.2,-3.39965000400001));
#321031=CARTESIAN_POINT('Ctrl Pts',(-3.00309560800006,12.2,-3.40190212700001));
#321032=CARTESIAN_POINT('Ctrl Pts',(-3.00309560800006,5.2,-3.40190212700001));
#321033=CARTESIAN_POINT('Ctrl Pts',(-3.00309560800006,2.2,-3.40190212700001));
#321034=CARTESIAN_POINT('Ctrl Pts',(-3.00361902400006,12.2,-3.40415844100002));
#321035=CARTESIAN_POINT('Ctrl Pts',(-3.00361902400006,5.2,-3.40415844100002));
#321036=CARTESIAN_POINT('Ctrl Pts',(-3.00361902400006,2.2,-3.40415844100002));
#321037=CARTESIAN_POINT('Ctrl Pts',(-3.00414085400006,12.2,-3.40641893700001));
#321038=CARTESIAN_POINT('Ctrl Pts',(-3.00414085400006,5.2,-3.40641893700001));
#321039=CARTESIAN_POINT('Ctrl Pts',(-3.00414085400006,2.2,-3.40641893700001));
#321040=CARTESIAN_POINT('Ctrl Pts',(-3.00466108800005,12.2,-3.40868361300001));
#321041=CARTESIAN_POINT('Ctrl Pts',(-3.00466108800005,5.2,-3.40868361300001));
#321042=CARTESIAN_POINT('Ctrl Pts',(-3.00466108800005,2.2,-3.40868361300001));
#321043=CARTESIAN_POINT('Ctrl Pts',(-3.00517971900006,12.2,-3.41095246200001));
#321044=CARTESIAN_POINT('Ctrl Pts',(-3.00517971900006,5.2,-3.41095246200001));
#321045=CARTESIAN_POINT('Ctrl Pts',(-3.00517971900006,2.2,-3.41095246200001));
#321046=CARTESIAN_POINT('Ctrl Pts',(-3.00569673900006,12.2,-3.41322548000001));
#321047=CARTESIAN_POINT('Ctrl Pts',(-3.00569673900006,5.2,-3.41322548000001));
#321048=CARTESIAN_POINT('Ctrl Pts',(-3.00569673900006,2.2,-3.41322548000001));
#321049=CARTESIAN_POINT('Ctrl Pts',(-3.00621213800006,12.2,-3.41550266300001));
#321050=CARTESIAN_POINT('Ctrl Pts',(-3.00621213800006,5.2,-3.41550266300001));
#321051=CARTESIAN_POINT('Ctrl Pts',(-3.00621213800006,2.2,-3.41550266300001));
#321052=CARTESIAN_POINT('Ctrl Pts',(-3.00672591000006,12.2,-3.41778400600001));
#321053=CARTESIAN_POINT('Ctrl Pts',(-3.00672591000006,5.2,-3.41778400600001));
#321054=CARTESIAN_POINT('Ctrl Pts',(-3.00672591000006,2.2,-3.41778400600001));
#321055=CARTESIAN_POINT('Ctrl Pts',(-3.00723804500006,12.2,-3.42006950300001));
#321056=CARTESIAN_POINT('Ctrl Pts',(-3.00723804500006,5.2,-3.42006950300001));
#321057=CARTESIAN_POINT('Ctrl Pts',(-3.00723804500006,2.2,-3.42006950300001));
#321058=CARTESIAN_POINT('Ctrl Pts',(-3.00774853500006,12.2,-3.42235915000002));
#321059=CARTESIAN_POINT('Ctrl Pts',(-3.00774853500006,5.2,-3.42235915000002));
#321060=CARTESIAN_POINT('Ctrl Pts',(-3.00774853500006,2.2,-3.42235915000002));
#321061=CARTESIAN_POINT('Ctrl Pts',(-3.00825737200006,12.2,-3.42465294000001));
#321062=CARTESIAN_POINT('Ctrl Pts',(-3.00825737200006,5.2,-3.42465294000001));
#321063=CARTESIAN_POINT('Ctrl Pts',(-3.00825737200006,2.2,-3.42465294000001));
#321064=CARTESIAN_POINT('Ctrl Pts',(-3.00876454800005,12.2,-3.42695087200001));
#321065=CARTESIAN_POINT('Ctrl Pts',(-3.00876454800005,5.2,-3.42695087200001));
#321066=CARTESIAN_POINT('Ctrl Pts',(-3.00876454800005,2.2,-3.42695087200001));
#321067=CARTESIAN_POINT('Ctrl Pts',(-3.00927005500006,12.2,-3.42925293800001));
#321068=CARTESIAN_POINT('Ctrl Pts',(-3.00927005500006,5.2,-3.42925293800001));
#321069=CARTESIAN_POINT('Ctrl Pts',(-3.00927005500006,2.2,-3.42925293800001));
#321070=CARTESIAN_POINT('Ctrl Pts',(-3.00977388500006,12.2,-3.43155913500001));
#321071=CARTESIAN_POINT('Ctrl Pts',(-3.00977388500006,5.2,-3.43155913500001));
#321072=CARTESIAN_POINT('Ctrl Pts',(-3.00977388500006,2.2,-3.43155913500001));
#321073=CARTESIAN_POINT('Ctrl Pts',(-3.01027602900006,12.2,-3.43386945700002));
#321074=CARTESIAN_POINT('Ctrl Pts',(-3.01027602900006,5.2,-3.43386945700002));
#321075=CARTESIAN_POINT('Ctrl Pts',(-3.01027602900006,2.2,-3.43386945700002));
#321076=CARTESIAN_POINT('Ctrl Pts',(-3.01077647900006,12.2,-3.43618389900001));
#321077=CARTESIAN_POINT('Ctrl Pts',(-3.01077647900006,5.2,-3.43618389900001));
#321078=CARTESIAN_POINT('Ctrl Pts',(-3.01077647900006,2.2,-3.43618389900001));
#321079=CARTESIAN_POINT('Ctrl Pts',(-3.01127522800006,12.2,-3.43850245700001));
#321080=CARTESIAN_POINT('Ctrl Pts',(-3.01127522800006,5.2,-3.43850245700001));
#321081=CARTESIAN_POINT('Ctrl Pts',(-3.01127522800006,2.2,-3.43850245700001));
#321082=CARTESIAN_POINT('Ctrl Pts',(-3.01177226700006,12.2,-3.44082512600002));
#321083=CARTESIAN_POINT('Ctrl Pts',(-3.01177226700006,5.2,-3.44082512600002));
#321084=CARTESIAN_POINT('Ctrl Pts',(-3.01177226700006,2.2,-3.44082512600002));
#321085=CARTESIAN_POINT('Ctrl Pts',(-3.01226758800006,12.2,-3.44315189900001));
#321086=CARTESIAN_POINT('Ctrl Pts',(-3.01226758800006,5.2,-3.44315189900001));
#321087=CARTESIAN_POINT('Ctrl Pts',(-3.01226758800006,2.2,-3.44315189900001));
#321088=CARTESIAN_POINT('Ctrl Pts',(-3.01276118200006,12.2,-3.44548277300001));
#321089=CARTESIAN_POINT('Ctrl Pts',(-3.01276118200006,5.2,-3.44548277300001));
#321090=CARTESIAN_POINT('Ctrl Pts',(-3.01276118200006,2.2,-3.44548277300001));
#321091=CARTESIAN_POINT('Ctrl Pts',(-3.01325304300006,12.2,-3.44781774300001));
#321092=CARTESIAN_POINT('Ctrl Pts',(-3.01325304300006,5.2,-3.44781774300001));
#321093=CARTESIAN_POINT('Ctrl Pts',(-3.01325304300006,2.2,-3.44781774300001));
#321094=CARTESIAN_POINT('Ctrl Pts',(-3.01374316200006,12.2,-3.45015680500001));
#321095=CARTESIAN_POINT('Ctrl Pts',(-3.01374316200006,5.2,-3.45015680500001));
#321096=CARTESIAN_POINT('Ctrl Pts',(-3.01374316200006,2.2,-3.45015680500001));
#321097=CARTESIAN_POINT('Ctrl Pts',(-3.01423153200005,12.2,-3.45249995200001));
#321098=CARTESIAN_POINT('Ctrl Pts',(-3.01423153200005,5.2,-3.45249995200001));
#321099=CARTESIAN_POINT('Ctrl Pts',(-3.01423153200005,2.2,-3.45249995200001));
#321100=CARTESIAN_POINT('Ctrl Pts',(-3.01471814300006,12.2,-3.45484718000002));
#321101=CARTESIAN_POINT('Ctrl Pts',(-3.01471814300006,5.2,-3.45484718000002));
#321102=CARTESIAN_POINT('Ctrl Pts',(-3.01471814300006,2.2,-3.45484718000002));
#321103=CARTESIAN_POINT('Ctrl Pts',(-3.01520298700006,12.2,-3.45719848300002));
#321104=CARTESIAN_POINT('Ctrl Pts',(-3.01520298700006,5.2,-3.45719848300002));
#321105=CARTESIAN_POINT('Ctrl Pts',(-3.01520298700006,2.2,-3.45719848300002));
#321106=CARTESIAN_POINT('Ctrl Pts',(-3.01568605800006,12.2,-3.45955385800002));
#321107=CARTESIAN_POINT('Ctrl Pts',(-3.01568605800006,5.2,-3.45955385800002));
#321108=CARTESIAN_POINT('Ctrl Pts',(-3.01568605800006,2.2,-3.45955385800002));
#321109=CARTESIAN_POINT('Ctrl Pts',(-3.01616734800006,12.2,-3.46191329900002));
#321110=CARTESIAN_POINT('Ctrl Pts',(-3.01616734800006,5.2,-3.46191329900002));
#321111=CARTESIAN_POINT('Ctrl Pts',(-3.01616734800006,2.2,-3.46191329900002));
#321112=CARTESIAN_POINT('Ctrl Pts',(-3.01664684800006,12.2,-3.46427680200001));
#321113=CARTESIAN_POINT('Ctrl Pts',(-3.01664684800006,5.2,-3.46427680200001));
#321114=CARTESIAN_POINT('Ctrl Pts',(-3.01664684800006,2.2,-3.46427680200001));
#321115=CARTESIAN_POINT('Ctrl Pts',(-3.01712455000006,12.2,-3.46664436100002));
#321116=CARTESIAN_POINT('Ctrl Pts',(-3.01712455000006,5.2,-3.46664436100002));
#321117=CARTESIAN_POINT('Ctrl Pts',(-3.01712455000006,2.2,-3.46664436100002));
#321118=CARTESIAN_POINT('Ctrl Pts',(-3.01760044700006,12.2,-3.46901597100001));
#321119=CARTESIAN_POINT('Ctrl Pts',(-3.01760044700006,5.2,-3.46901597100001));
#321120=CARTESIAN_POINT('Ctrl Pts',(-3.01760044700006,2.2,-3.46901597100001));
#321121=CARTESIAN_POINT('Ctrl Pts',(-3.01807453000006,12.2,-3.47139162600001));
#321122=CARTESIAN_POINT('Ctrl Pts',(-3.01807453000006,5.2,-3.47139162600001));
#321123=CARTESIAN_POINT('Ctrl Pts',(-3.01807453000006,2.2,-3.47139162600001));
#321124=CARTESIAN_POINT('Ctrl Pts',(-3.01854679200006,12.2,-3.47377132400001));
#321125=CARTESIAN_POINT('Ctrl Pts',(-3.01854679200006,5.2,-3.47377132400001));
#321126=CARTESIAN_POINT('Ctrl Pts',(-3.01854679200006,2.2,-3.47377132400001));
#321127=CARTESIAN_POINT('Ctrl Pts',(-3.01901722500005,12.2,-3.47615505700002));
#321128=CARTESIAN_POINT('Ctrl Pts',(-3.01901722500005,5.2,-3.47615505700002));
#321129=CARTESIAN_POINT('Ctrl Pts',(-3.01901722500005,2.2,-3.47615505700002));
#321130=CARTESIAN_POINT('Ctrl Pts',(-3.01948582200006,12.2,-3.47854282200001));
#321131=CARTESIAN_POINT('Ctrl Pts',(-3.01948582200006,5.2,-3.47854282200001));
#321132=CARTESIAN_POINT('Ctrl Pts',(-3.01948582200006,2.2,-3.47854282200001));
#321133=CARTESIAN_POINT('Ctrl Pts',(-3.01995257400006,12.2,-3.48093461300001));
#321134=CARTESIAN_POINT('Ctrl Pts',(-3.01995257400006,5.2,-3.48093461300001));
#321135=CARTESIAN_POINT('Ctrl Pts',(-3.01995257400006,2.2,-3.48093461300001));
#321136=CARTESIAN_POINT('Ctrl Pts',(-3.02041747200006,12.2,-3.48333042600002));
#321137=CARTESIAN_POINT('Ctrl Pts',(-3.02041747200006,5.2,-3.48333042600002));
#321138=CARTESIAN_POINT('Ctrl Pts',(-3.02041747200006,2.2,-3.48333042600002));
#321139=CARTESIAN_POINT('Ctrl Pts',(-3.02088051200006,12.2,-3.48573025600002));
#321140=CARTESIAN_POINT('Ctrl Pts',(-3.02088051200006,5.2,-3.48573025600002));
#321141=CARTESIAN_POINT('Ctrl Pts',(-3.02088051200006,2.2,-3.48573025600002));
#321142=CARTESIAN_POINT('Ctrl Pts',(-3.02134168300006,12.2,-3.48813409600002));
#321143=CARTESIAN_POINT('Ctrl Pts',(-3.02134168300006,5.2,-3.48813409600002));
#321144=CARTESIAN_POINT('Ctrl Pts',(-3.02134168300006,2.2,-3.48813409600002));
#321145=CARTESIAN_POINT('Ctrl Pts',(-3.02180097900006,12.2,-3.49054194300002));
#321146=CARTESIAN_POINT('Ctrl Pts',(-3.02180097900006,5.2,-3.49054194300002));
#321147=CARTESIAN_POINT('Ctrl Pts',(-3.02180097900006,2.2,-3.49054194300002));
#321148=CARTESIAN_POINT('Ctrl Pts',(-3.02225839100006,12.2,-3.49295379000001));
#321149=CARTESIAN_POINT('Ctrl Pts',(-3.02225839100006,5.2,-3.49295379000001));
#321150=CARTESIAN_POINT('Ctrl Pts',(-3.02225839100006,2.2,-3.49295379000001));
#321151=CARTESIAN_POINT('Ctrl Pts',(-3.02271391300006,12.2,-3.49536963500002));
#321152=CARTESIAN_POINT('Ctrl Pts',(-3.02271391300006,5.2,-3.49536963500002));
#321153=CARTESIAN_POINT('Ctrl Pts',(-3.02271391300006,2.2,-3.49536963500002));
#321154=CARTESIAN_POINT('Ctrl Pts',(-3.02316753600006,12.2,-3.49778947100001));
#321155=CARTESIAN_POINT('Ctrl Pts',(-3.02316753600006,5.2,-3.49778947100001));
#321156=CARTESIAN_POINT('Ctrl Pts',(-3.02316753600006,2.2,-3.49778947100001));
#321157=CARTESIAN_POINT('Ctrl Pts',(-3.02361925200006,12.2,-3.50021329300001));
#321158=CARTESIAN_POINT('Ctrl Pts',(-3.02361925200006,5.2,-3.50021329300001));
#321159=CARTESIAN_POINT('Ctrl Pts',(-3.02361925200006,2.2,-3.50021329300001));
#321160=CARTESIAN_POINT('Ctrl Pts',(-3.02406905400006,12.2,-3.50264109700001));
#321161=CARTESIAN_POINT('Ctrl Pts',(-3.02406905400006,5.2,-3.50264109700001));
#321162=CARTESIAN_POINT('Ctrl Pts',(-3.02406905400006,2.2,-3.50264109700001));
#321163=CARTESIAN_POINT('Ctrl Pts',(-3.02451693500006,12.2,-3.50507287600001));
#321164=CARTESIAN_POINT('Ctrl Pts',(-3.02451693500006,5.2,-3.50507287600001));
#321165=CARTESIAN_POINT('Ctrl Pts',(-3.02451693500006,2.2,-3.50507287600001));
#321166=CARTESIAN_POINT('Ctrl Pts',(-3.02496288600006,12.2,-3.50750862700002));
#321167=CARTESIAN_POINT('Ctrl Pts',(-3.02496288600006,5.2,-3.50750862700002));
#321168=CARTESIAN_POINT('Ctrl Pts',(-3.02496288600006,2.2,-3.50750862700002));
#321169=CARTESIAN_POINT('Ctrl Pts',(-3.02540690200006,12.2,-3.50994834400002));
#321170=CARTESIAN_POINT('Ctrl Pts',(-3.02540690200006,5.2,-3.50994834400002));
#321171=CARTESIAN_POINT('Ctrl Pts',(-3.02540690200006,2.2,-3.50994834400002));
#321172=CARTESIAN_POINT('Ctrl Pts',(-3.02584897300005,12.2,-3.51239202200002));
#321173=CARTESIAN_POINT('Ctrl Pts',(-3.02584897300005,5.2,-3.51239202200002));
#321174=CARTESIAN_POINT('Ctrl Pts',(-3.02584897300005,2.2,-3.51239202200002));
#321175=CARTESIAN_POINT('Ctrl Pts',(-3.02628909100005,12.2,-3.51483965700002));
#321176=CARTESIAN_POINT('Ctrl Pts',(-3.02628909100005,5.2,-3.51483965700002));
#321177=CARTESIAN_POINT('Ctrl Pts',(-3.02628909100005,2.2,-3.51483965700002));
#321178=CARTESIAN_POINT('Ctrl Pts',(-3.02672725000006,12.2,-3.51729124200002));
#321179=CARTESIAN_POINT('Ctrl Pts',(-3.02672725000006,5.2,-3.51729124200002));
#321180=CARTESIAN_POINT('Ctrl Pts',(-3.02672725000006,2.2,-3.51729124200002));
#321181=CARTESIAN_POINT('Ctrl Pts',(-3.02716344200006,12.2,-3.51974677400001));
#321182=CARTESIAN_POINT('Ctrl Pts',(-3.02716344200006,5.2,-3.51974677400001));
#321183=CARTESIAN_POINT('Ctrl Pts',(-3.02716344200006,2.2,-3.51974677400001));
#321184=CARTESIAN_POINT('Ctrl Pts',(-3.02759765900006,12.2,-3.52220624600001));
#321185=CARTESIAN_POINT('Ctrl Pts',(-3.02759765900006,5.2,-3.52220624600001));
#321186=CARTESIAN_POINT('Ctrl Pts',(-3.02759765900006,2.2,-3.52220624600001));
#321187=CARTESIAN_POINT('Ctrl Pts',(-3.02802989500006,12.2,-3.52466965500001));
#321188=CARTESIAN_POINT('Ctrl Pts',(-3.02802989500006,5.2,-3.52466965500001));
#321189=CARTESIAN_POINT('Ctrl Pts',(-3.02802989500006,2.2,-3.52466965500001));
#321190=CARTESIAN_POINT('Ctrl Pts',(-3.02846014100006,12.2,-3.52713699300002));
#321191=CARTESIAN_POINT('Ctrl Pts',(-3.02846014100006,5.2,-3.52713699300002));
#321192=CARTESIAN_POINT('Ctrl Pts',(-3.02846014100006,2.2,-3.52713699300002));
#321193=CARTESIAN_POINT('Ctrl Pts',(-3.02888839000006,12.2,-3.52960825900002));
#321194=CARTESIAN_POINT('Ctrl Pts',(-3.02888839000006,5.2,-3.52960825900002));
#321195=CARTESIAN_POINT('Ctrl Pts',(-3.02888839000006,2.2,-3.52960825900002));
#321196=CARTESIAN_POINT('Ctrl Pts',(-3.02931463500005,12.2,-3.53208344400001));
#321197=CARTESIAN_POINT('Ctrl Pts',(-3.02931463500005,5.2,-3.53208344400001));
#321198=CARTESIAN_POINT('Ctrl Pts',(-3.02931463500005,2.2,-3.53208344400001));
#321199=CARTESIAN_POINT('Ctrl Pts',(-3.02973886900006,12.2,-3.53456254500002));
#321200=CARTESIAN_POINT('Ctrl Pts',(-3.02973886900006,5.2,-3.53456254500002));
#321201=CARTESIAN_POINT('Ctrl Pts',(-3.02973886900006,2.2,-3.53456254500002));
#321202=CARTESIAN_POINT('Ctrl Pts',(-3.03016108200006,12.2,-3.53704555700002));
#321203=CARTESIAN_POINT('Ctrl Pts',(-3.03016108200006,5.2,-3.53704555700002));
#321204=CARTESIAN_POINT('Ctrl Pts',(-3.03016108200006,2.2,-3.53704555700002));
#321205=CARTESIAN_POINT('Ctrl Pts',(-3.03058126900006,12.2,-3.53953247400002));
#321206=CARTESIAN_POINT('Ctrl Pts',(-3.03058126900006,5.2,-3.53953247400002));
#321207=CARTESIAN_POINT('Ctrl Pts',(-3.03058126900006,2.2,-3.53953247400002));
#321208=CARTESIAN_POINT('Ctrl Pts',(-3.03099942300005,12.2,-3.54202329100001));
#321209=CARTESIAN_POINT('Ctrl Pts',(-3.03099942300005,5.2,-3.54202329100001));
#321210=CARTESIAN_POINT('Ctrl Pts',(-3.03099942300005,2.2,-3.54202329100001));
#321211=CARTESIAN_POINT('Ctrl Pts',(-3.03141553400006,12.2,-3.54451800500001));
#321212=CARTESIAN_POINT('Ctrl Pts',(-3.03141553400006,5.2,-3.54451800500001));
#321213=CARTESIAN_POINT('Ctrl Pts',(-3.03141553400006,2.2,-3.54451800500001));
#321214=CARTESIAN_POINT('Ctrl Pts',(-3.03182959700006,12.2,-3.54701660600002));
#321215=CARTESIAN_POINT('Ctrl Pts',(-3.03182959700006,5.2,-3.54701660600002));
#321216=CARTESIAN_POINT('Ctrl Pts',(-3.03182959700006,2.2,-3.54701660600002));
#321217=CARTESIAN_POINT('Ctrl Pts',(-3.03224160400006,12.2,-3.54951909500001));
#321218=CARTESIAN_POINT('Ctrl Pts',(-3.03224160400006,5.2,-3.54951909500001));
#321219=CARTESIAN_POINT('Ctrl Pts',(-3.03224160400006,2.2,-3.54951909500001));
#321220=CARTESIAN_POINT('Ctrl Pts',(-3.03265154800005,12.2,-3.55202546300001));
#321221=CARTESIAN_POINT('Ctrl Pts',(-3.03265154800005,5.2,-3.55202546300001));
#321222=CARTESIAN_POINT('Ctrl Pts',(-3.03265154800005,2.2,-3.55202546300001));
#321223=CARTESIAN_POINT('Ctrl Pts',(-3.03305942100006,12.2,-3.55453570500002));
#321224=CARTESIAN_POINT('Ctrl Pts',(-3.03305942100006,5.2,-3.55453570500002));
#321225=CARTESIAN_POINT('Ctrl Pts',(-3.03305942100006,2.2,-3.55453570500002));
#321226=CARTESIAN_POINT('Ctrl Pts',(-3.03346521700006,12.2,-3.55704981800002));
#321227=CARTESIAN_POINT('Ctrl Pts',(-3.03346521700006,5.2,-3.55704981800002));
#321228=CARTESIAN_POINT('Ctrl Pts',(-3.03346521700006,2.2,-3.55704981800002));
#321229=CARTESIAN_POINT('Ctrl Pts',(-3.03386892600006,12.2,-3.55956779500001));
#321230=CARTESIAN_POINT('Ctrl Pts',(-3.03386892600006,5.2,-3.55956779500001));
#321231=CARTESIAN_POINT('Ctrl Pts',(-3.03386892600006,2.2,-3.55956779500001));
#321232=CARTESIAN_POINT('Ctrl Pts',(-3.03427054400006,12.2,-3.56208963200002));
#321233=CARTESIAN_POINT('Ctrl Pts',(-3.03427054400006,5.2,-3.56208963200002));
#321234=CARTESIAN_POINT('Ctrl Pts',(-3.03427054400006,2.2,-3.56208963200002));
#321235=CARTESIAN_POINT('Ctrl Pts',(-3.03467006100006,12.2,-3.56461532400001));
#321236=CARTESIAN_POINT('Ctrl Pts',(-3.03467006100006,5.2,-3.56461532400001));
#321237=CARTESIAN_POINT('Ctrl Pts',(-3.03467006100006,2.2,-3.56461532400001));
#321238=CARTESIAN_POINT('Ctrl Pts',(-3.03506747200006,12.2,-3.56714486400001));
#321239=CARTESIAN_POINT('Ctrl Pts',(-3.03506747200006,5.2,-3.56714486400001));
#321240=CARTESIAN_POINT('Ctrl Pts',(-3.03506747200006,2.2,-3.56714486400001));
#321241=CARTESIAN_POINT('Ctrl Pts',(-3.03546276900006,12.2,-3.56967824900002));
#321242=CARTESIAN_POINT('Ctrl Pts',(-3.03546276900006,5.2,-3.56967824900002));
#321243=CARTESIAN_POINT('Ctrl Pts',(-3.03546276900006,2.2,-3.56967824900002));
#321244=CARTESIAN_POINT('Ctrl Pts',(-3.03585594400006,12.2,-3.57221547200002));
#321245=CARTESIAN_POINT('Ctrl Pts',(-3.03585594400006,5.2,-3.57221547200002));
#321246=CARTESIAN_POINT('Ctrl Pts',(-3.03585594400006,2.2,-3.57221547200002));
#321247=CARTESIAN_POINT('Ctrl Pts',(-3.03624699100005,12.2,-3.57475652900002));
#321248=CARTESIAN_POINT('Ctrl Pts',(-3.03624699100005,5.2,-3.57475652900002));
#321249=CARTESIAN_POINT('Ctrl Pts',(-3.03624699100005,2.2,-3.57475652900002));
#321250=CARTESIAN_POINT('Ctrl Pts',(-3.03663590200005,12.2,-3.57730141600001));
#321251=CARTESIAN_POINT('Ctrl Pts',(-3.03663590200005,5.2,-3.57730141600001));
#321252=CARTESIAN_POINT('Ctrl Pts',(-3.03663590200005,2.2,-3.57730141600001));
#321253=CARTESIAN_POINT('Ctrl Pts',(-3.03702267000005,12.2,-3.57985012500002));
#321254=CARTESIAN_POINT('Ctrl Pts',(-3.03702267000005,5.2,-3.57985012500002));
#321255=CARTESIAN_POINT('Ctrl Pts',(-3.03702267000005,2.2,-3.57985012500002));
#321256=CARTESIAN_POINT('Ctrl Pts',(-3.03740728800005,12.2,-3.58240265400001));
#321257=CARTESIAN_POINT('Ctrl Pts',(-3.03740728800005,5.2,-3.58240265400001));
#321258=CARTESIAN_POINT('Ctrl Pts',(-3.03740728800005,2.2,-3.58240265400001));
#321259=CARTESIAN_POINT('Ctrl Pts',(-3.03778975000006,12.2,-3.58495899600001));
#321260=CARTESIAN_POINT('Ctrl Pts',(-3.03778975000006,5.2,-3.58495899600001));
#321261=CARTESIAN_POINT('Ctrl Pts',(-3.03778975000006,2.2,-3.58495899600001));
#321262=CARTESIAN_POINT('Ctrl Pts',(-3.03817004900006,12.2,-3.58751914600001));
#321263=CARTESIAN_POINT('Ctrl Pts',(-3.03817004900006,5.2,-3.58751914600001));
#321264=CARTESIAN_POINT('Ctrl Pts',(-3.03817004900006,2.2,-3.58751914600001));
#321265=CARTESIAN_POINT('Ctrl Pts',(-3.03854817600006,12.2,-3.59008310000001));
#321266=CARTESIAN_POINT('Ctrl Pts',(-3.03854817600006,5.2,-3.59008310000001));
#321267=CARTESIAN_POINT('Ctrl Pts',(-3.03854817600006,2.2,-3.59008310000001));
#321268=CARTESIAN_POINT('Ctrl Pts',(-3.03892412400006,12.2,-3.59265085000001));
#321269=CARTESIAN_POINT('Ctrl Pts',(-3.03892412400006,5.2,-3.59265085000001));
#321270=CARTESIAN_POINT('Ctrl Pts',(-3.03892412400006,2.2,-3.59265085000001));
#321271=CARTESIAN_POINT('Ctrl Pts',(-3.03929788700006,12.2,-3.59522239500001));
#321272=CARTESIAN_POINT('Ctrl Pts',(-3.03929788700006,5.2,-3.59522239500001));
#321273=CARTESIAN_POINT('Ctrl Pts',(-3.03929788700006,2.2,-3.59522239500001));
#321274=CARTESIAN_POINT('Ctrl Pts',(-3.03966945600005,12.2,-3.59779772400001));
#321275=CARTESIAN_POINT('Ctrl Pts',(-3.03966945600005,5.2,-3.59779772400001));
#321276=CARTESIAN_POINT('Ctrl Pts',(-3.03966945600005,2.2,-3.59779772400001));
#321277=CARTESIAN_POINT('Ctrl Pts',(-3.04003882600006,12.2,-3.60037683700002));
#321278=CARTESIAN_POINT('Ctrl Pts',(-3.04003882600006,5.2,-3.60037683700002));
#321279=CARTESIAN_POINT('Ctrl Pts',(-3.04003882600006,2.2,-3.60037683700002));
#321280=CARTESIAN_POINT('Ctrl Pts',(-3.04040598800006,12.2,-3.60295972600001));
#321281=CARTESIAN_POINT('Ctrl Pts',(-3.04040598800006,5.2,-3.60295972600001));
#321282=CARTESIAN_POINT('Ctrl Pts',(-3.04040598800006,2.2,-3.60295972600001));
#321283=CARTESIAN_POINT('Ctrl Pts',(-3.04077093700006,12.2,-3.60554638700001));
#321284=CARTESIAN_POINT('Ctrl Pts',(-3.04077093700006,5.2,-3.60554638700001));
#321285=CARTESIAN_POINT('Ctrl Pts',(-3.04077093700006,2.2,-3.60554638700001));
#321286=CARTESIAN_POINT('Ctrl Pts',(-3.04113366700005,12.2,-3.60813681500002));
#321287=CARTESIAN_POINT('Ctrl Pts',(-3.04113366700005,5.2,-3.60813681500002));
#321288=CARTESIAN_POINT('Ctrl Pts',(-3.04113366700005,2.2,-3.60813681500002));
#321289=CARTESIAN_POINT('Ctrl Pts',(-3.04149417000006,12.2,-3.61073100600001));
#321290=CARTESIAN_POINT('Ctrl Pts',(-3.04149417000006,5.2,-3.61073100600001));
#321291=CARTESIAN_POINT('Ctrl Pts',(-3.04149417000006,2.2,-3.61073100600001));
#321292=CARTESIAN_POINT('Ctrl Pts',(-3.04185244200006,12.2,-3.61332895400002));
#321293=CARTESIAN_POINT('Ctrl Pts',(-3.04185244200006,5.2,-3.61332895400002));
#321294=CARTESIAN_POINT('Ctrl Pts',(-3.04185244200006,2.2,-3.61332895400002));
#321295=CARTESIAN_POINT('Ctrl Pts',(-3.04220847300006,12.2,-3.61593065600001));
#321296=CARTESIAN_POINT('Ctrl Pts',(-3.04220847300006,5.2,-3.61593065600001));
#321297=CARTESIAN_POINT('Ctrl Pts',(-3.04220847300006,2.2,-3.61593065600001));
#321298=CARTESIAN_POINT('Ctrl Pts',(-3.04256225800006,12.2,-3.61853610400001));
#321299=CARTESIAN_POINT('Ctrl Pts',(-3.04256225800006,5.2,-3.61853610400001));
#321300=CARTESIAN_POINT('Ctrl Pts',(-3.04256225800006,2.2,-3.61853610400001));
#321301=CARTESIAN_POINT('Ctrl Pts',(-3.04291378800006,12.2,-3.62114529300001));
#321302=CARTESIAN_POINT('Ctrl Pts',(-3.04291378800006,5.2,-3.62114529300001));
#321303=CARTESIAN_POINT('Ctrl Pts',(-3.04291378800006,2.2,-3.62114529300001));
#321304=CARTESIAN_POINT('Ctrl Pts',(-3.04326305300005,12.2,-3.62375821500001));
#321305=CARTESIAN_POINT('Ctrl Pts',(-3.04326305300005,5.2,-3.62375821500001));
#321306=CARTESIAN_POINT('Ctrl Pts',(-3.04326305300005,2.2,-3.62375821500001));
#321307=CARTESIAN_POINT('Ctrl Pts',(-3.04361004500006,12.2,-3.62637486600002));
#321308=CARTESIAN_POINT('Ctrl Pts',(-3.04361004500006,5.2,-3.62637486600002));
#321309=CARTESIAN_POINT('Ctrl Pts',(-3.04361004500006,2.2,-3.62637486600002));
#321310=CARTESIAN_POINT('Ctrl Pts',(-3.04395475800006,12.2,-3.62899523800001));
#321311=CARTESIAN_POINT('Ctrl Pts',(-3.04395475800006,5.2,-3.62899523800001));
#321312=CARTESIAN_POINT('Ctrl Pts',(-3.04395475800006,2.2,-3.62899523800001));
#321313=CARTESIAN_POINT('Ctrl Pts',(-3.04429718300006,12.2,-3.63161932600002));
#321314=CARTESIAN_POINT('Ctrl Pts',(-3.04429718300006,5.2,-3.63161932600002));
#321315=CARTESIAN_POINT('Ctrl Pts',(-3.04429718300006,2.2,-3.63161932600002));
#321316=CARTESIAN_POINT('Ctrl Pts',(-3.04463731600006,12.2,-3.63424712900001));
#321317=CARTESIAN_POINT('Ctrl Pts',(-3.04463731600006,5.2,-3.63424712900001));
#321318=CARTESIAN_POINT('Ctrl Pts',(-3.04463731600006,2.2,-3.63424712900001));
#321319=CARTESIAN_POINT('Ctrl Pts',(-3.04497515600006,12.2,-3.63687864000001));
#321320=CARTESIAN_POINT('Ctrl Pts',(-3.04497515600006,5.2,-3.63687864000001));
#321321=CARTESIAN_POINT('Ctrl Pts',(-3.04497515600006,2.2,-3.63687864000001));
#321322=CARTESIAN_POINT('Ctrl Pts',(-3.04531069900006,12.2,-3.63951386200001));
#321323=CARTESIAN_POINT('Ctrl Pts',(-3.04531069900006,5.2,-3.63951386200001));
#321324=CARTESIAN_POINT('Ctrl Pts',(-3.04531069900006,2.2,-3.63951386200001));
#321325=CARTESIAN_POINT('Ctrl Pts',(-3.04557729400006,12.2,-3.64162500500001));
#321326=CARTESIAN_POINT('Ctrl Pts',(-3.04557729400006,5.2,-3.64162500500001));
#321327=CARTESIAN_POINT('Ctrl Pts',(-3.04557729400006,2.2,-3.64162500500001));
#321328=CARTESIAN_POINT('Ctrl Pts',(-3.04577620700006,12.2,-3.64321003100001));
#321329=CARTESIAN_POINT('Ctrl Pts',(-3.04577620700006,5.2,-3.64321003100001));
#321330=CARTESIAN_POINT('Ctrl Pts',(-3.04577620700006,2.2,-3.64321003100001));
#321331=CARTESIAN_POINT('Ctrl Pts',(-3.04590835500006,12.2,-3.64426745700001));
#321332=CARTESIAN_POINT('Ctrl Pts',(-3.04590835500006,5.2,-3.64426745700001));
#321333=CARTESIAN_POINT('Ctrl Pts',(-3.04590835500006,2.2,-3.64426745700001));
#321334=CARTESIAN_POINT('Ctrl Pts',(-3.04597431500006,12.2,-3.64479635500001));
#321335=CARTESIAN_POINT('Ctrl Pts',(-3.04597431500006,5.2,-3.64479635500001));
#321336=CARTESIAN_POINT('Ctrl Pts',(-3.04597431500006,2.2,-3.64479635500001));
#321337=CARTESIAN_POINT('',(-3.04597431500006,2.7,-3.64479635500001));
#321338=CARTESIAN_POINT('',(-3.04597431500006,12.2,-3.64479635500001));
#321339=CARTESIAN_POINT('Ctrl Pts',(-2.77432738100006,2.7,-2.87279823800001));
#321340=CARTESIAN_POINT('Ctrl Pts',(-2.7744374764468,2.7,-2.87291314750764));
#321341=CARTESIAN_POINT('Ctrl Pts',(-2.77454645880482,2.69999999999987,
-2.87302912203624));
#321342=CARTESIAN_POINT('Ctrl Pts',(-2.77488192258474,2.69999999999987,
-2.8733877460855));
#321343=CARTESIAN_POINT('Ctrl Pts',(-2.77511779315,2.7,-2.87364373929698));
#321344=CARTESIAN_POINT('Ctrl Pts',(-2.77611559716086,2.7,-2.87473558902309));
#321345=CARTESIAN_POINT('Ctrl Pts',(-2.77693139030848,2.7,-2.87565470358675));
#321346=CARTESIAN_POINT('Ctrl Pts',(-2.7804778170359,2.7,-2.87971816338106));
#321347=CARTESIAN_POINT('Ctrl Pts',(-2.78335042552836,2.7,-2.88320615918335));
#321348=CARTESIAN_POINT('Ctrl Pts',(-2.79571151680306,2.7,-2.89872292454845));
#321349=CARTESIAN_POINT('Ctrl Pts',(-2.80534829486808,2.7,-2.91230134672957));
#321350=CARTESIAN_POINT('Ctrl Pts',(-2.83882810873472,2.7,-2.96274864644993));
#321351=CARTESIAN_POINT('Ctrl Pts',(-2.86724824082749,2.7,-3.01294763423819));
#321352=CARTESIAN_POINT('Ctrl Pts',(-2.9494517880223,2.7,-3.19589938056903));
#321353=CARTESIAN_POINT('Ctrl Pts',(-3.01313420540364,2.7,-3.38146906140652));
#321354=CARTESIAN_POINT('Ctrl Pts',(-3.04597431500006,2.7,-3.64479635500001));
#321355=CARTESIAN_POINT('Origin',(-5.66300478732629E-14,15.2,-1.77635683940025E-14));
#321356=CARTESIAN_POINT('',(-2.77990780000006,2.7,-3.85157274700001));
#321357=CARTESIAN_POINT('',(-2.77990780000006,12.2,-3.85157274700001));
#321358=CARTESIAN_POINT('Origin',(-5.66300478732629E-14,2.7,-1.92943768261394E-14));
#321359=CARTESIAN_POINT('Ctrl Pts',(-2.77990780000006,12.2,-3.85157274700001));
#321360=CARTESIAN_POINT('Ctrl Pts',(-2.77990780000006,5.2,-3.85157274700001));
#321361=CARTESIAN_POINT('Ctrl Pts',(-2.77990780000006,2.2,-3.85157274700001));
#321362=CARTESIAN_POINT('Ctrl Pts',(-2.77941156100006,12.2,-3.85137824500001));
#321363=CARTESIAN_POINT('Ctrl Pts',(-2.77941156100006,5.2,-3.85137824500001));
#321364=CARTESIAN_POINT('Ctrl Pts',(-2.77941156100006,2.2,-3.85137824500001));
#321365=CARTESIAN_POINT('Ctrl Pts',(-2.77841949900006,12.2,-3.85098910900001));
#321366=CARTESIAN_POINT('Ctrl Pts',(-2.77841949900006,5.2,-3.85098910900001));
#321367=CARTESIAN_POINT('Ctrl Pts',(-2.77841949900006,2.2,-3.85098910900001));
#321368=CARTESIAN_POINT('Ctrl Pts',(-2.77693265500006,12.2,-3.85040501300002));
#321369=CARTESIAN_POINT('Ctrl Pts',(-2.77693265500006,5.2,-3.85040501300002));
#321370=CARTESIAN_POINT('Ctrl Pts',(-2.77693265500006,2.2,-3.85040501300002));
#321371=CARTESIAN_POINT('Ctrl Pts',(-2.77495269300006,12.2,-3.84962543000002));
#321372=CARTESIAN_POINT('Ctrl Pts',(-2.77495269300006,5.2,-3.84962543000002));
#321373=CARTESIAN_POINT('Ctrl Pts',(-2.77495269300006,2.2,-3.84962543000002));
#321374=CARTESIAN_POINT('Ctrl Pts',(-2.77248190100006,12.2,-3.84864964100001));
#321375=CARTESIAN_POINT('Ctrl Pts',(-2.77248190100006,5.2,-3.84864964100001));
#321376=CARTESIAN_POINT('Ctrl Pts',(-2.77248190100006,2.2,-3.84864964100001));
#321377=CARTESIAN_POINT('Ctrl Pts',(-2.77001526900006,12.2,-3.84767254100002));
#321378=CARTESIAN_POINT('Ctrl Pts',(-2.77001526900006,5.2,-3.84767254100002));
#321379=CARTESIAN_POINT('Ctrl Pts',(-2.77001526900006,2.2,-3.84767254100002));
#321380=CARTESIAN_POINT('Ctrl Pts',(-2.76755280100006,12.2,-3.84669413500002));
#321381=CARTESIAN_POINT('Ctrl Pts',(-2.76755280100006,5.2,-3.84669413500002));
#321382=CARTESIAN_POINT('Ctrl Pts',(-2.76755280100006,2.2,-3.84669413500002));
#321383=CARTESIAN_POINT('Ctrl Pts',(-2.76509449600006,12.2,-3.84571442400001));
#321384=CARTESIAN_POINT('Ctrl Pts',(-2.76509449600006,5.2,-3.84571442400001));
#321385=CARTESIAN_POINT('Ctrl Pts',(-2.76509449600006,2.2,-3.84571442400001));
#321386=CARTESIAN_POINT('Ctrl Pts',(-2.76264035700006,12.2,-3.84473341500001));
#321387=CARTESIAN_POINT('Ctrl Pts',(-2.76264035700006,5.2,-3.84473341500001));
#321388=CARTESIAN_POINT('Ctrl Pts',(-2.76264035700006,2.2,-3.84473341500001));
#321389=CARTESIAN_POINT('Ctrl Pts',(-2.76019038700006,12.2,-3.84375111500002));
#321390=CARTESIAN_POINT('Ctrl Pts',(-2.76019038700006,5.2,-3.84375111500002));
#321391=CARTESIAN_POINT('Ctrl Pts',(-2.76019038700006,2.2,-3.84375111500002));
#321392=CARTESIAN_POINT('Ctrl Pts',(-2.75774459100006,12.2,-3.84276753400002));
#321393=CARTESIAN_POINT('Ctrl Pts',(-2.75774459100006,5.2,-3.84276753400002));
#321394=CARTESIAN_POINT('Ctrl Pts',(-2.75774459100006,2.2,-3.84276753400002));
#321395=CARTESIAN_POINT('Ctrl Pts',(-2.75530297200006,12.2,-3.84178268000001));
#321396=CARTESIAN_POINT('Ctrl Pts',(-2.75530297200006,5.2,-3.84178268000001));
#321397=CARTESIAN_POINT('Ctrl Pts',(-2.75530297200006,2.2,-3.84178268000001));
#321398=CARTESIAN_POINT('Ctrl Pts',(-2.75286553500006,12.2,-3.84079656400001));
#321399=CARTESIAN_POINT('Ctrl Pts',(-2.75286553500006,5.2,-3.84079656400001));
#321400=CARTESIAN_POINT('Ctrl Pts',(-2.75286553500006,2.2,-3.84079656400001));
#321401=CARTESIAN_POINT('Ctrl Pts',(-2.75043228400006,12.2,-3.83980919600001));
#321402=CARTESIAN_POINT('Ctrl Pts',(-2.75043228400006,5.2,-3.83980919600001));
#321403=CARTESIAN_POINT('Ctrl Pts',(-2.75043228400006,2.2,-3.83980919600001));
#321404=CARTESIAN_POINT('Ctrl Pts',(-2.74800322200006,12.2,-3.83882058400001));
#321405=CARTESIAN_POINT('Ctrl Pts',(-2.74800322200006,5.2,-3.83882058400001));
#321406=CARTESIAN_POINT('Ctrl Pts',(-2.74800322200006,2.2,-3.83882058400001));
#321407=CARTESIAN_POINT('Ctrl Pts',(-2.74557835200006,12.2,-3.83783073700001));
#321408=CARTESIAN_POINT('Ctrl Pts',(-2.74557835200006,5.2,-3.83783073700001));
#321409=CARTESIAN_POINT('Ctrl Pts',(-2.74557835200006,2.2,-3.83783073700001));
#321410=CARTESIAN_POINT('Ctrl Pts',(-2.74315767900006,12.2,-3.83683966200001));
#321411=CARTESIAN_POINT('Ctrl Pts',(-2.74315767900006,5.2,-3.83683966200001));
#321412=CARTESIAN_POINT('Ctrl Pts',(-2.74315767900006,2.2,-3.83683966200001));
#321413=CARTESIAN_POINT('Ctrl Pts',(-2.74074120400006,12.2,-3.83584736600001));
#321414=CARTESIAN_POINT('Ctrl Pts',(-2.74074120400006,5.2,-3.83584736600001));
#321415=CARTESIAN_POINT('Ctrl Pts',(-2.74074120400006,2.2,-3.83584736600001));
#321416=CARTESIAN_POINT('Ctrl Pts',(-2.73832893100006,12.2,-3.83485385600002));
#321417=CARTESIAN_POINT('Ctrl Pts',(-2.73832893100006,5.2,-3.83485385600002));
#321418=CARTESIAN_POINT('Ctrl Pts',(-2.73832893100006,2.2,-3.83485385600002));
#321419=CARTESIAN_POINT('Ctrl Pts',(-2.73592086200006,12.2,-3.83385914000002));
#321420=CARTESIAN_POINT('Ctrl Pts',(-2.73592086200006,5.2,-3.83385914000002));
#321421=CARTESIAN_POINT('Ctrl Pts',(-2.73592086200006,2.2,-3.83385914000002));
#321422=CARTESIAN_POINT('Ctrl Pts',(-2.73351700100006,12.2,-3.83286322600001));
#321423=CARTESIAN_POINT('Ctrl Pts',(-2.73351700100006,5.2,-3.83286322600001));
#321424=CARTESIAN_POINT('Ctrl Pts',(-2.73351700100006,2.2,-3.83286322600001));
#321425=CARTESIAN_POINT('Ctrl Pts',(-2.73111735300006,12.2,-3.83186612200001));
#321426=CARTESIAN_POINT('Ctrl Pts',(-2.73111735300006,5.2,-3.83186612200001));
#321427=CARTESIAN_POINT('Ctrl Pts',(-2.73111735300006,2.2,-3.83186612200001));
#321428=CARTESIAN_POINT('Ctrl Pts',(-2.72872191700006,12.2,-3.83086783600001));
#321429=CARTESIAN_POINT('Ctrl Pts',(-2.72872191700006,5.2,-3.83086783600001));
#321430=CARTESIAN_POINT('Ctrl Pts',(-2.72872191700006,2.2,-3.83086783600001));
#321431=CARTESIAN_POINT('Ctrl Pts',(-2.72633070100006,12.2,-3.82986837600002));
#321432=CARTESIAN_POINT('Ctrl Pts',(-2.72633070100006,5.2,-3.82986837600002));
#321433=CARTESIAN_POINT('Ctrl Pts',(-2.72633070100006,2.2,-3.82986837600002));
#321434=CARTESIAN_POINT('Ctrl Pts',(-2.72394370500006,12.2,-3.82886775100001));
#321435=CARTESIAN_POINT('Ctrl Pts',(-2.72394370500006,5.2,-3.82886775100001));
#321436=CARTESIAN_POINT('Ctrl Pts',(-2.72394370500006,2.2,-3.82886775100001));
#321437=CARTESIAN_POINT('Ctrl Pts',(-2.72156093400006,12.2,-3.82786597100001));
#321438=CARTESIAN_POINT('Ctrl Pts',(-2.72156093400006,5.2,-3.82786597100001));
#321439=CARTESIAN_POINT('Ctrl Pts',(-2.72156093400006,2.2,-3.82786597100001));
#321440=CARTESIAN_POINT('Ctrl Pts',(-2.71918239200006,12.2,-3.82686304200002));
#321441=CARTESIAN_POINT('Ctrl Pts',(-2.71918239200006,5.2,-3.82686304200002));
#321442=CARTESIAN_POINT('Ctrl Pts',(-2.71918239200006,2.2,-3.82686304200002));
#321443=CARTESIAN_POINT('Ctrl Pts',(-2.71680808000006,12.2,-3.82585897200002));
#321444=CARTESIAN_POINT('Ctrl Pts',(-2.71680808000006,5.2,-3.82585897200002));
#321445=CARTESIAN_POINT('Ctrl Pts',(-2.71680808000006,2.2,-3.82585897200002));
#321446=CARTESIAN_POINT('Ctrl Pts',(-2.71443800200006,12.2,-3.82485377000001));
#321447=CARTESIAN_POINT('Ctrl Pts',(-2.71443800200006,5.2,-3.82485377000001));
#321448=CARTESIAN_POINT('Ctrl Pts',(-2.71443800200006,2.2,-3.82485377000001));
#321449=CARTESIAN_POINT('Ctrl Pts',(-2.71207216300006,12.2,-3.82384744400001));
#321450=CARTESIAN_POINT('Ctrl Pts',(-2.71207216300006,5.2,-3.82384744400001));
#321451=CARTESIAN_POINT('Ctrl Pts',(-2.71207216300006,2.2,-3.82384744400001));
#321452=CARTESIAN_POINT('Ctrl Pts',(-2.70971056400006,12.2,-3.82284000200002));
#321453=CARTESIAN_POINT('Ctrl Pts',(-2.70971056400006,5.2,-3.82284000200002));
#321454=CARTESIAN_POINT('Ctrl Pts',(-2.70971056400006,2.2,-3.82284000200002));
#321455=CARTESIAN_POINT('Ctrl Pts',(-2.70735320900005,12.2,-3.82183145200001));
#321456=CARTESIAN_POINT('Ctrl Pts',(-2.70735320900005,5.2,-3.82183145200001));
#321457=CARTESIAN_POINT('Ctrl Pts',(-2.70735320900005,2.2,-3.82183145200001));
#321458=CARTESIAN_POINT('Ctrl Pts',(-2.70500010100006,12.2,-3.82082180200001));
#321459=CARTESIAN_POINT('Ctrl Pts',(-2.70500010100006,5.2,-3.82082180200001));
#321460=CARTESIAN_POINT('Ctrl Pts',(-2.70500010100006,2.2,-3.82082180200001));
#321461=CARTESIAN_POINT('Ctrl Pts',(-2.70265124300006,12.2,-3.81981106100001));
#321462=CARTESIAN_POINT('Ctrl Pts',(-2.70265124300006,5.2,-3.81981106100001));
#321463=CARTESIAN_POINT('Ctrl Pts',(-2.70265124300006,2.2,-3.81981106100001));
#321464=CARTESIAN_POINT('Ctrl Pts',(-2.70030663800005,12.2,-3.81879923700001));
#321465=CARTESIAN_POINT('Ctrl Pts',(-2.70030663800005,5.2,-3.81879923700001));
#321466=CARTESIAN_POINT('Ctrl Pts',(-2.70030663800005,2.2,-3.81879923700001));
#321467=CARTESIAN_POINT('Ctrl Pts',(-2.69796629100005,12.2,-3.81778633700002));
#321468=CARTESIAN_POINT('Ctrl Pts',(-2.69796629100005,5.2,-3.81778633700002));
#321469=CARTESIAN_POINT('Ctrl Pts',(-2.69796629100005,2.2,-3.81778633700002));
#321470=CARTESIAN_POINT('Ctrl Pts',(-2.69563020300006,12.2,-3.81677237200002));
#321471=CARTESIAN_POINT('Ctrl Pts',(-2.69563020300006,5.2,-3.81677237200002));
#321472=CARTESIAN_POINT('Ctrl Pts',(-2.69563020300006,2.2,-3.81677237200002));
#321473=CARTESIAN_POINT('Ctrl Pts',(-2.69329837900006,12.2,-3.81575734800002));
#321474=CARTESIAN_POINT('Ctrl Pts',(-2.69329837900006,5.2,-3.81575734800002));
#321475=CARTESIAN_POINT('Ctrl Pts',(-2.69329837900006,2.2,-3.81575734800002));
#321476=CARTESIAN_POINT('Ctrl Pts',(-2.69097082000005,12.2,-3.81474127600002));
#321477=CARTESIAN_POINT('Ctrl Pts',(-2.69097082000005,5.2,-3.81474127600002));
#321478=CARTESIAN_POINT('Ctrl Pts',(-2.69097082000005,2.2,-3.81474127600002));
#321479=CARTESIAN_POINT('Ctrl Pts',(-2.68864753000006,12.2,-3.81372416000001));
#321480=CARTESIAN_POINT('Ctrl Pts',(-2.68864753000006,5.2,-3.81372416000001));
#321481=CARTESIAN_POINT('Ctrl Pts',(-2.68864753000006,2.2,-3.81372416000001));
#321482=CARTESIAN_POINT('Ctrl Pts',(-2.68632851300006,12.2,-3.81270601300002));
#321483=CARTESIAN_POINT('Ctrl Pts',(-2.68632851300006,5.2,-3.81270601300002));
#321484=CARTESIAN_POINT('Ctrl Pts',(-2.68632851300006,2.2,-3.81270601300002));
#321485=CARTESIAN_POINT('Ctrl Pts',(-2.68401377200005,12.2,-3.81168684000002));
#321486=CARTESIAN_POINT('Ctrl Pts',(-2.68401377200005,5.2,-3.81168684000002));
#321487=CARTESIAN_POINT('Ctrl Pts',(-2.68401377200005,2.2,-3.81168684000002));
#321488=CARTESIAN_POINT('Ctrl Pts',(-2.68170330900006,12.2,-3.81066665100001));
#321489=CARTESIAN_POINT('Ctrl Pts',(-2.68170330900006,5.2,-3.81066665100001));
#321490=CARTESIAN_POINT('Ctrl Pts',(-2.68170330900006,2.2,-3.81066665100001));
#321491=CARTESIAN_POINT('Ctrl Pts',(-2.67939712900006,12.2,-3.80964545400001));
#321492=CARTESIAN_POINT('Ctrl Pts',(-2.67939712900006,5.2,-3.80964545400001));
#321493=CARTESIAN_POINT('Ctrl Pts',(-2.67939712900006,2.2,-3.80964545400001));
#321494=CARTESIAN_POINT('Ctrl Pts',(-2.67709523200006,12.2,-3.80862325700001));
#321495=CARTESIAN_POINT('Ctrl Pts',(-2.67709523200006,5.2,-3.80862325700001));
#321496=CARTESIAN_POINT('Ctrl Pts',(-2.67709523200006,2.2,-3.80862325700001));
#321497=CARTESIAN_POINT('Ctrl Pts',(-2.67479762500006,12.2,-3.80760006800001));
#321498=CARTESIAN_POINT('Ctrl Pts',(-2.67479762500006,5.2,-3.80760006800001));
#321499=CARTESIAN_POINT('Ctrl Pts',(-2.67479762500006,2.2,-3.80760006800001));
#321500=CARTESIAN_POINT('Ctrl Pts',(-2.67250430800006,12.2,-3.80657589700002));
#321501=CARTESIAN_POINT('Ctrl Pts',(-2.67250430800006,5.2,-3.80657589700002));
#321502=CARTESIAN_POINT('Ctrl Pts',(-2.67250430800006,2.2,-3.80657589700002));
#321503=CARTESIAN_POINT('Ctrl Pts',(-2.67021528500006,12.2,-3.80555075200002));
#321504=CARTESIAN_POINT('Ctrl Pts',(-2.67021528500006,5.2,-3.80555075200002));
#321505=CARTESIAN_POINT('Ctrl Pts',(-2.67021528500006,2.2,-3.80555075200002));
#321506=CARTESIAN_POINT('Ctrl Pts',(-2.66793056000005,12.2,-3.80452464100001));
#321507=CARTESIAN_POINT('Ctrl Pts',(-2.66793056000005,5.2,-3.80452464100001));
#321508=CARTESIAN_POINT('Ctrl Pts',(-2.66793056000005,2.2,-3.80452464100001));
#321509=CARTESIAN_POINT('Ctrl Pts',(-2.66565013400006,12.2,-3.80349757300001));
#321510=CARTESIAN_POINT('Ctrl Pts',(-2.66565013400006,5.2,-3.80349757300001));
#321511=CARTESIAN_POINT('Ctrl Pts',(-2.66565013400006,2.2,-3.80349757300001));
#321512=CARTESIAN_POINT('Ctrl Pts',(-2.66337401300006,12.2,-3.80246955600001));
#321513=CARTESIAN_POINT('Ctrl Pts',(-2.66337401300006,5.2,-3.80246955600001));
#321514=CARTESIAN_POINT('Ctrl Pts',(-2.66337401300006,2.2,-3.80246955600001));
#321515=CARTESIAN_POINT('Ctrl Pts',(-2.66110219800006,12.2,-3.80144059800001));
#321516=CARTESIAN_POINT('Ctrl Pts',(-2.66110219800006,5.2,-3.80144059800001));
#321517=CARTESIAN_POINT('Ctrl Pts',(-2.66110219800006,2.2,-3.80144059800001));
#321518=CARTESIAN_POINT('Ctrl Pts',(-2.65883469300006,12.2,-3.80041070900001));
#321519=CARTESIAN_POINT('Ctrl Pts',(-2.65883469300006,5.2,-3.80041070900001));
#321520=CARTESIAN_POINT('Ctrl Pts',(-2.65883469300006,2.2,-3.80041070900001));
#321521=CARTESIAN_POINT('Ctrl Pts',(-2.65657149900006,12.2,-3.79937989600001));
#321522=CARTESIAN_POINT('Ctrl Pts',(-2.65657149900006,5.2,-3.79937989600001));
#321523=CARTESIAN_POINT('Ctrl Pts',(-2.65657149900006,2.2,-3.79937989600001));
#321524=CARTESIAN_POINT('Ctrl Pts',(-2.65431262200006,12.2,-3.79834816800001));
#321525=CARTESIAN_POINT('Ctrl Pts',(-2.65431262200006,5.2,-3.79834816800001));
#321526=CARTESIAN_POINT('Ctrl Pts',(-2.65431262200006,2.2,-3.79834816800001));
#321527=CARTESIAN_POINT('Ctrl Pts',(-2.65205806300005,12.2,-3.79731553500001));
#321528=CARTESIAN_POINT('Ctrl Pts',(-2.65205806300005,5.2,-3.79731553500001));
#321529=CARTESIAN_POINT('Ctrl Pts',(-2.65205806300005,2.2,-3.79731553500001));
#321530=CARTESIAN_POINT('Ctrl Pts',(-2.64980782600006,12.2,-3.79628200300001));
#321531=CARTESIAN_POINT('Ctrl Pts',(-2.64980782600006,5.2,-3.79628200300001));
#321532=CARTESIAN_POINT('Ctrl Pts',(-2.64980782600006,2.2,-3.79628200300001));
#321533=CARTESIAN_POINT('Ctrl Pts',(-2.64756191200005,12.2,-3.79524758300001));
#321534=CARTESIAN_POINT('Ctrl Pts',(-2.64756191200005,5.2,-3.79524758300001));
#321535=CARTESIAN_POINT('Ctrl Pts',(-2.64756191200005,2.2,-3.79524758300001));
#321536=CARTESIAN_POINT('Ctrl Pts',(-2.64532032700005,12.2,-3.79421228300002));
#321537=CARTESIAN_POINT('Ctrl Pts',(-2.64532032700005,5.2,-3.79421228300002));
#321538=CARTESIAN_POINT('Ctrl Pts',(-2.64532032700005,2.2,-3.79421228300002));
#321539=CARTESIAN_POINT('Ctrl Pts',(-2.64308307200006,12.2,-3.79317611000001));
#321540=CARTESIAN_POINT('Ctrl Pts',(-2.64308307200006,5.2,-3.79317611000001));
#321541=CARTESIAN_POINT('Ctrl Pts',(-2.64308307200006,2.2,-3.79317611000001));
#321542=CARTESIAN_POINT('Ctrl Pts',(-2.64085015200005,12.2,-3.79213907500001));
#321543=CARTESIAN_POINT('Ctrl Pts',(-2.64085015200005,5.2,-3.79213907500001));
#321544=CARTESIAN_POINT('Ctrl Pts',(-2.64085015200005,2.2,-3.79213907500001));
#321545=CARTESIAN_POINT('Ctrl Pts',(-2.63862156700006,12.2,-3.79110118500002));
#321546=CARTESIAN_POINT('Ctrl Pts',(-2.63862156700006,5.2,-3.79110118500002));
#321547=CARTESIAN_POINT('Ctrl Pts',(-2.63862156700006,2.2,-3.79110118500002));
#321548=CARTESIAN_POINT('Ctrl Pts',(-2.63639732200006,12.2,-3.79006245000001));
#321549=CARTESIAN_POINT('Ctrl Pts',(-2.63639732200006,5.2,-3.79006245000001));
#321550=CARTESIAN_POINT('Ctrl Pts',(-2.63639732200006,2.2,-3.79006245000001));
#321551=CARTESIAN_POINT('Ctrl Pts',(-2.63417741900006,12.2,-3.78902287700001));
#321552=CARTESIAN_POINT('Ctrl Pts',(-2.63417741900006,5.2,-3.78902287700001));
#321553=CARTESIAN_POINT('Ctrl Pts',(-2.63417741900006,2.2,-3.78902287700001));
#321554=CARTESIAN_POINT('Ctrl Pts',(-2.63196186200005,12.2,-3.78798247500002));
#321555=CARTESIAN_POINT('Ctrl Pts',(-2.63196186200005,5.2,-3.78798247500002));
#321556=CARTESIAN_POINT('Ctrl Pts',(-2.63196186200005,2.2,-3.78798247500002));
#321557=CARTESIAN_POINT('Ctrl Pts',(-2.62975065300005,12.2,-3.78694125500001));
#321558=CARTESIAN_POINT('Ctrl Pts',(-2.62975065300005,5.2,-3.78694125500001));
#321559=CARTESIAN_POINT('Ctrl Pts',(-2.62975065300005,2.2,-3.78694125500001));
#321560=CARTESIAN_POINT('Ctrl Pts',(-2.62754379500006,12.2,-3.78589922300002));
#321561=CARTESIAN_POINT('Ctrl Pts',(-2.62754379500006,5.2,-3.78589922300002));
#321562=CARTESIAN_POINT('Ctrl Pts',(-2.62754379500006,2.2,-3.78589922300002));
#321563=CARTESIAN_POINT('Ctrl Pts',(-2.62534129200006,12.2,-3.78485639000001));
#321564=CARTESIAN_POINT('Ctrl Pts',(-2.62534129200006,5.2,-3.78485639000001));
#321565=CARTESIAN_POINT('Ctrl Pts',(-2.62534129200006,2.2,-3.78485639000001));
#321566=CARTESIAN_POINT('Ctrl Pts',(-2.62314314600005,12.2,-3.78381276300002));
#321567=CARTESIAN_POINT('Ctrl Pts',(-2.62314314600005,5.2,-3.78381276300002));
#321568=CARTESIAN_POINT('Ctrl Pts',(-2.62314314600005,2.2,-3.78381276300002));
#321569=CARTESIAN_POINT('Ctrl Pts',(-2.62094936000006,12.2,-3.78276835100001));
#321570=CARTESIAN_POINT('Ctrl Pts',(-2.62094936000006,5.2,-3.78276835100001));
#321571=CARTESIAN_POINT('Ctrl Pts',(-2.62094936000006,2.2,-3.78276835100001));
#321572=CARTESIAN_POINT('Ctrl Pts',(-2.61875993600006,12.2,-3.78172316300001));
#321573=CARTESIAN_POINT('Ctrl Pts',(-2.61875993600006,5.2,-3.78172316300001));
#321574=CARTESIAN_POINT('Ctrl Pts',(-2.61875993600006,2.2,-3.78172316300001));
#321575=CARTESIAN_POINT('Ctrl Pts',(-2.61657488000006,12.2,-3.78067720900002));
#321576=CARTESIAN_POINT('Ctrl Pts',(-2.61657488000006,5.2,-3.78067720900002));
#321577=CARTESIAN_POINT('Ctrl Pts',(-2.61657488000006,2.2,-3.78067720900002));
#321578=CARTESIAN_POINT('Ctrl Pts',(-2.61439419100005,12.2,-3.77963049600002));
#321579=CARTESIAN_POINT('Ctrl Pts',(-2.61439419100005,5.2,-3.77963049600002));
#321580=CARTESIAN_POINT('Ctrl Pts',(-2.61439419100005,2.2,-3.77963049600002));
#321581=CARTESIAN_POINT('Ctrl Pts',(-2.61221787400005,12.2,-3.77858303400001));
#321582=CARTESIAN_POINT('Ctrl Pts',(-2.61221787400005,5.2,-3.77858303400001));
#321583=CARTESIAN_POINT('Ctrl Pts',(-2.61221787400005,2.2,-3.77858303400001));
#321584=CARTESIAN_POINT('Ctrl Pts',(-2.61004593100005,12.2,-3.77753483200001));
#321585=CARTESIAN_POINT('Ctrl Pts',(-2.61004593100005,5.2,-3.77753483200001));
#321586=CARTESIAN_POINT('Ctrl Pts',(-2.61004593100005,2.2,-3.77753483200001));
#321587=CARTESIAN_POINT('Ctrl Pts',(-2.60787836600006,12.2,-3.77648589700001));
#321588=CARTESIAN_POINT('Ctrl Pts',(-2.60787836600006,5.2,-3.77648589700001));
#321589=CARTESIAN_POINT('Ctrl Pts',(-2.60787836600006,2.2,-3.77648589700001));
#321590=CARTESIAN_POINT('Ctrl Pts',(-2.60571518100006,12.2,-3.77543624000001));
#321591=CARTESIAN_POINT('Ctrl Pts',(-2.60571518100006,5.2,-3.77543624000001));
#321592=CARTESIAN_POINT('Ctrl Pts',(-2.60571518100006,2.2,-3.77543624000001));
#321593=CARTESIAN_POINT('Ctrl Pts',(-2.60355637900005,12.2,-3.77438587000002));
#321594=CARTESIAN_POINT('Ctrl Pts',(-2.60355637900005,5.2,-3.77438587000002));
#321595=CARTESIAN_POINT('Ctrl Pts',(-2.60355637900005,2.2,-3.77438587000002));
#321596=CARTESIAN_POINT('Ctrl Pts',(-2.60140196200005,12.2,-3.77333479500002));
#321597=CARTESIAN_POINT('Ctrl Pts',(-2.60140196200005,5.2,-3.77333479500002));
#321598=CARTESIAN_POINT('Ctrl Pts',(-2.60140196200005,2.2,-3.77333479500002));
#321599=CARTESIAN_POINT('Ctrl Pts',(-2.59925193500006,12.2,-3.77228302300002));
#321600=CARTESIAN_POINT('Ctrl Pts',(-2.59925193500006,5.2,-3.77228302300002));
#321601=CARTESIAN_POINT('Ctrl Pts',(-2.59925193500006,2.2,-3.77228302300002));
#321602=CARTESIAN_POINT('Ctrl Pts',(-2.59710629800006,12.2,-3.77123056500002));
#321603=CARTESIAN_POINT('Ctrl Pts',(-2.59710629800006,5.2,-3.77123056500002));
#321604=CARTESIAN_POINT('Ctrl Pts',(-2.59710629800006,2.2,-3.77123056500002));
#321605=CARTESIAN_POINT('Ctrl Pts',(-2.59496505700006,12.2,-3.77017742800001));
#321606=CARTESIAN_POINT('Ctrl Pts',(-2.59496505700006,5.2,-3.77017742800001));
#321607=CARTESIAN_POINT('Ctrl Pts',(-2.59496505700006,2.2,-3.77017742800001));
#321608=CARTESIAN_POINT('Ctrl Pts',(-2.59282821200005,12.2,-3.76912362300001));
#321609=CARTESIAN_POINT('Ctrl Pts',(-2.59282821200005,5.2,-3.76912362300001));
#321610=CARTESIAN_POINT('Ctrl Pts',(-2.59282821200005,2.2,-3.76912362300001));
#321611=CARTESIAN_POINT('Ctrl Pts',(-2.59069576700006,12.2,-3.76806915700001));
#321612=CARTESIAN_POINT('Ctrl Pts',(-2.59069576700006,5.2,-3.76806915700001));
#321613=CARTESIAN_POINT('Ctrl Pts',(-2.59069576700006,2.2,-3.76806915700001));
#321614=CARTESIAN_POINT('Ctrl Pts',(-2.58856772500006,12.2,-3.76701404000002));
#321615=CARTESIAN_POINT('Ctrl Pts',(-2.58856772500006,5.2,-3.76701404000002));
#321616=CARTESIAN_POINT('Ctrl Pts',(-2.58856772500006,2.2,-3.76701404000002));
#321617=CARTESIAN_POINT('Ctrl Pts',(-2.58644408800006,12.2,-3.76595828200001));
#321618=CARTESIAN_POINT('Ctrl Pts',(-2.58644408800006,5.2,-3.76595828200001));
#321619=CARTESIAN_POINT('Ctrl Pts',(-2.58644408800006,2.2,-3.76595828200001));
#321620=CARTESIAN_POINT('Ctrl Pts',(-2.58432486000005,12.2,-3.76490188900001));
#321621=CARTESIAN_POINT('Ctrl Pts',(-2.58432486000005,5.2,-3.76490188900001));
#321622=CARTESIAN_POINT('Ctrl Pts',(-2.58432486000005,2.2,-3.76490188900001));
#321623=CARTESIAN_POINT('Ctrl Pts',(-2.58221004200006,12.2,-3.76384487400002));
#321624=CARTESIAN_POINT('Ctrl Pts',(-2.58221004200006,5.2,-3.76384487400002));
#321625=CARTESIAN_POINT('Ctrl Pts',(-2.58221004200006,2.2,-3.76384487400002));
#321626=CARTESIAN_POINT('Ctrl Pts',(-2.58009963800006,12.2,-3.76278724400001));
#321627=CARTESIAN_POINT('Ctrl Pts',(-2.58009963800006,5.2,-3.76278724400001));
#321628=CARTESIAN_POINT('Ctrl Pts',(-2.58009963800006,2.2,-3.76278724400001));
#321629=CARTESIAN_POINT('Ctrl Pts',(-2.57799365100006,12.2,-3.76172900700002));
#321630=CARTESIAN_POINT('Ctrl Pts',(-2.57799365100006,5.2,-3.76172900700002));
#321631=CARTESIAN_POINT('Ctrl Pts',(-2.57799365100006,2.2,-3.76172900700002));
#321632=CARTESIAN_POINT('Ctrl Pts',(-2.57589208100006,12.2,-3.76067017500001));
#321633=CARTESIAN_POINT('Ctrl Pts',(-2.57589208100006,5.2,-3.76067017500001));
#321634=CARTESIAN_POINT('Ctrl Pts',(-2.57589208100006,2.2,-3.76067017500001));
#321635=CARTESIAN_POINT('Ctrl Pts',(-2.57379493500005,12.2,-3.75961075500001));
#321636=CARTESIAN_POINT('Ctrl Pts',(-2.57379493500005,5.2,-3.75961075500001));
#321637=CARTESIAN_POINT('Ctrl Pts',(-2.57379493500005,2.2,-3.75961075500001));
#321638=CARTESIAN_POINT('Ctrl Pts',(-2.57170221300006,12.2,-3.75855075600001));
#321639=CARTESIAN_POINT('Ctrl Pts',(-2.57170221300006,5.2,-3.75855075600001));
#321640=CARTESIAN_POINT('Ctrl Pts',(-2.57170221300006,2.2,-3.75855075600001));
#321641=CARTESIAN_POINT('Ctrl Pts',(-2.56961391900006,12.2,-3.75749018800001));
#321642=CARTESIAN_POINT('Ctrl Pts',(-2.56961391900006,5.2,-3.75749018800001));
#321643=CARTESIAN_POINT('Ctrl Pts',(-2.56961391900006,2.2,-3.75749018800001));
#321644=CARTESIAN_POINT('Ctrl Pts',(-2.56753005400005,12.2,-3.75642906000001));
#321645=CARTESIAN_POINT('Ctrl Pts',(-2.56753005400005,5.2,-3.75642906000001));
#321646=CARTESIAN_POINT('Ctrl Pts',(-2.56753005400005,2.2,-3.75642906000001));
#321647=CARTESIAN_POINT('Ctrl Pts',(-2.56545062200006,12.2,-3.75536738200001));
#321648=CARTESIAN_POINT('Ctrl Pts',(-2.56545062200006,5.2,-3.75536738200001));
#321649=CARTESIAN_POINT('Ctrl Pts',(-2.56545062200006,2.2,-3.75536738200001));
#321650=CARTESIAN_POINT('Ctrl Pts',(-2.56337562600006,12.2,-3.75430516100002));
#321651=CARTESIAN_POINT('Ctrl Pts',(-2.56337562600006,5.2,-3.75430516100002));
#321652=CARTESIAN_POINT('Ctrl Pts',(-2.56337562600006,2.2,-3.75430516100002));
#321653=CARTESIAN_POINT('Ctrl Pts',(-2.56130506800006,12.2,-3.75324240800001));
#321654=CARTESIAN_POINT('Ctrl Pts',(-2.56130506800006,5.2,-3.75324240800001));
#321655=CARTESIAN_POINT('Ctrl Pts',(-2.56130506800006,2.2,-3.75324240800001));
#321656=CARTESIAN_POINT('Ctrl Pts',(-2.55923894900006,12.2,-3.75217913300002));
#321657=CARTESIAN_POINT('Ctrl Pts',(-2.55923894900006,5.2,-3.75217913300002));
#321658=CARTESIAN_POINT('Ctrl Pts',(-2.55923894900006,2.2,-3.75217913300002));
#321659=CARTESIAN_POINT('Ctrl Pts',(-2.55717727500006,12.2,-3.75111534300002));
#321660=CARTESIAN_POINT('Ctrl Pts',(-2.55717727500006,5.2,-3.75111534300002));
#321661=CARTESIAN_POINT('Ctrl Pts',(-2.55717727500006,2.2,-3.75111534300002));
#321662=CARTESIAN_POINT('Ctrl Pts',(-2.55512004700006,12.2,-3.75005104800001));
#321663=CARTESIAN_POINT('Ctrl Pts',(-2.55512004700006,5.2,-3.75005104800001));
#321664=CARTESIAN_POINT('Ctrl Pts',(-2.55512004700006,2.2,-3.75005104800001));
#321665=CARTESIAN_POINT('Ctrl Pts',(-2.55306726700006,12.2,-3.74898625800002));
#321666=CARTESIAN_POINT('Ctrl Pts',(-2.55306726700006,5.2,-3.74898625800002));
#321667=CARTESIAN_POINT('Ctrl Pts',(-2.55306726700006,2.2,-3.74898625800002));
#321668=CARTESIAN_POINT('Ctrl Pts',(-2.55101893800005,12.2,-3.74792098200002));
#321669=CARTESIAN_POINT('Ctrl Pts',(-2.55101893800005,5.2,-3.74792098200002));
#321670=CARTESIAN_POINT('Ctrl Pts',(-2.55101893800005,2.2,-3.74792098200002));
#321671=CARTESIAN_POINT('Ctrl Pts',(-2.54897506300006,12.2,-3.74685523000001));
#321672=CARTESIAN_POINT('Ctrl Pts',(-2.54897506300006,5.2,-3.74685523000001));
#321673=CARTESIAN_POINT('Ctrl Pts',(-2.54897506300006,2.2,-3.74685523000001));
#321674=CARTESIAN_POINT('Ctrl Pts',(-2.54693564500006,12.2,-3.74578901000001));
#321675=CARTESIAN_POINT('Ctrl Pts',(-2.54693564500006,5.2,-3.74578901000001));
#321676=CARTESIAN_POINT('Ctrl Pts',(-2.54693564500006,2.2,-3.74578901000001));
#321677=CARTESIAN_POINT('Ctrl Pts',(-2.54490068500006,12.2,-3.74472233100001));
#321678=CARTESIAN_POINT('Ctrl Pts',(-2.54490068500006,5.2,-3.74472233100001));
#321679=CARTESIAN_POINT('Ctrl Pts',(-2.54490068500006,2.2,-3.74472233100001));
#321680=CARTESIAN_POINT('Ctrl Pts',(-2.54287018700006,12.2,-3.74365520400001));
#321681=CARTESIAN_POINT('Ctrl Pts',(-2.54287018700006,5.2,-3.74365520400001));
#321682=CARTESIAN_POINT('Ctrl Pts',(-2.54287018700006,2.2,-3.74365520400001));
#321683=CARTESIAN_POINT('Ctrl Pts',(-2.54084415400006,12.2,-3.74258763800002));
#321684=CARTESIAN_POINT('Ctrl Pts',(-2.54084415400006,5.2,-3.74258763800002));
#321685=CARTESIAN_POINT('Ctrl Pts',(-2.54084415400006,2.2,-3.74258763800002));
#321686=CARTESIAN_POINT('Ctrl Pts',(-2.53882258600005,12.2,-3.74151964200002));
#321687=CARTESIAN_POINT('Ctrl Pts',(-2.53882258600005,5.2,-3.74151964200002));
#321688=CARTESIAN_POINT('Ctrl Pts',(-2.53882258600005,2.2,-3.74151964200002));
#321689=CARTESIAN_POINT('Ctrl Pts',(-2.53680548900005,12.2,-3.74045122600001));
#321690=CARTESIAN_POINT('Ctrl Pts',(-2.53680548900005,5.2,-3.74045122600001));
#321691=CARTESIAN_POINT('Ctrl Pts',(-2.53680548900005,2.2,-3.74045122600001));
#321692=CARTESIAN_POINT('Ctrl Pts',(-2.53479286300006,12.2,-3.73938239800002));
#321693=CARTESIAN_POINT('Ctrl Pts',(-2.53479286300006,5.2,-3.73938239800002));
#321694=CARTESIAN_POINT('Ctrl Pts',(-2.53479286300006,2.2,-3.73938239800002));
#321695=CARTESIAN_POINT('Ctrl Pts',(-2.53278471100006,12.2,-3.73831316800001));
#321696=CARTESIAN_POINT('Ctrl Pts',(-2.53278471100006,5.2,-3.73831316800001));
#321697=CARTESIAN_POINT('Ctrl Pts',(-2.53278471100006,2.2,-3.73831316800001));
#321698=CARTESIAN_POINT('Ctrl Pts',(-2.53078103700005,12.2,-3.73724354700002));
#321699=CARTESIAN_POINT('Ctrl Pts',(-2.53078103700005,5.2,-3.73724354700002));
#321700=CARTESIAN_POINT('Ctrl Pts',(-2.53078103700005,2.2,-3.73724354700002));
#321701=CARTESIAN_POINT('Ctrl Pts',(-2.52878184200005,12.2,-3.73617354300002));
#321702=CARTESIAN_POINT('Ctrl Pts',(-2.52878184200005,5.2,-3.73617354300002));
#321703=CARTESIAN_POINT('Ctrl Pts',(-2.52878184200005,2.2,-3.73617354300002));
#321704=CARTESIAN_POINT('Ctrl Pts',(-2.52678712900006,12.2,-3.73510316700001));
#321705=CARTESIAN_POINT('Ctrl Pts',(-2.52678712900006,5.2,-3.73510316700001));
#321706=CARTESIAN_POINT('Ctrl Pts',(-2.52678712900006,2.2,-3.73510316700001));
#321707=CARTESIAN_POINT('Ctrl Pts',(-2.52479690100006,12.2,-3.73403242600002));
#321708=CARTESIAN_POINT('Ctrl Pts',(-2.52479690100006,5.2,-3.73403242600002));
#321709=CARTESIAN_POINT('Ctrl Pts',(-2.52479690100006,2.2,-3.73403242600002));
#321710=CARTESIAN_POINT('Ctrl Pts',(-2.52281115900006,12.2,-3.73296133000002));
#321711=CARTESIAN_POINT('Ctrl Pts',(-2.52281115900006,5.2,-3.73296133000002));
#321712=CARTESIAN_POINT('Ctrl Pts',(-2.52281115900006,2.2,-3.73296133000002));
#321713=CARTESIAN_POINT('Ctrl Pts',(-2.52082990700006,12.2,-3.73188989100001));
#321714=CARTESIAN_POINT('Ctrl Pts',(-2.52082990700006,5.2,-3.73188989100001));
#321715=CARTESIAN_POINT('Ctrl Pts',(-2.52082990700006,2.2,-3.73188989100001));
#321716=CARTESIAN_POINT('Ctrl Pts',(-2.51885314600006,12.2,-3.73081811600001));
#321717=CARTESIAN_POINT('Ctrl Pts',(-2.51885314600006,5.2,-3.73081811600001));
#321718=CARTESIAN_POINT('Ctrl Pts',(-2.51885314600006,2.2,-3.73081811600001));
#321719=CARTESIAN_POINT('Ctrl Pts',(-2.51688088000006,12.2,-3.72974601700002));
#321720=CARTESIAN_POINT('Ctrl Pts',(-2.51688088000006,5.2,-3.72974601700002));
#321721=CARTESIAN_POINT('Ctrl Pts',(-2.51688088000006,2.2,-3.72974601700002));
#321722=CARTESIAN_POINT('Ctrl Pts',(-2.51491311100006,12.2,-3.72867360100001));
#321723=CARTESIAN_POINT('Ctrl Pts',(-2.51491311100006,5.2,-3.72867360100001));
#321724=CARTESIAN_POINT('Ctrl Pts',(-2.51491311100006,2.2,-3.72867360100001));
#321725=CARTESIAN_POINT('Ctrl Pts',(-2.51294984100006,12.2,-3.72760087900001));
#321726=CARTESIAN_POINT('Ctrl Pts',(-2.51294984100006,5.2,-3.72760087900001));
#321727=CARTESIAN_POINT('Ctrl Pts',(-2.51294984100006,2.2,-3.72760087900001));
#321728=CARTESIAN_POINT('Ctrl Pts',(-2.51099107300006,12.2,-3.72652786100002));
#321729=CARTESIAN_POINT('Ctrl Pts',(-2.51099107300006,5.2,-3.72652786100002));
#321730=CARTESIAN_POINT('Ctrl Pts',(-2.51099107300006,2.2,-3.72652786100002));
#321731=CARTESIAN_POINT('Ctrl Pts',(-2.50903680800006,12.2,-3.72545455600001));
#321732=CARTESIAN_POINT('Ctrl Pts',(-2.50903680800006,5.2,-3.72545455600001));
#321733=CARTESIAN_POINT('Ctrl Pts',(-2.50903680800006,2.2,-3.72545455600001));
#321734=CARTESIAN_POINT('Ctrl Pts',(-2.50708705000006,12.2,-3.72438097300002));
#321735=CARTESIAN_POINT('Ctrl Pts',(-2.50708705000006,5.2,-3.72438097300002));
#321736=CARTESIAN_POINT('Ctrl Pts',(-2.50708705000006,2.2,-3.72438097300002));
#321737=CARTESIAN_POINT('Ctrl Pts',(-2.50514180200006,12.2,-3.72330712300001));
#321738=CARTESIAN_POINT('Ctrl Pts',(-2.50514180200006,5.2,-3.72330712300001));
#321739=CARTESIAN_POINT('Ctrl Pts',(-2.50514180200006,2.2,-3.72330712300001));
#321740=CARTESIAN_POINT('Ctrl Pts',(-2.50320106400005,12.2,-3.72223301500001));
#321741=CARTESIAN_POINT('Ctrl Pts',(-2.50320106400005,5.2,-3.72223301500001));
#321742=CARTESIAN_POINT('Ctrl Pts',(-2.50320106400005,2.2,-3.72223301500001));
#321743=CARTESIAN_POINT('Ctrl Pts',(-2.50126484000006,12.2,-3.72115866000001));
#321744=CARTESIAN_POINT('Ctrl Pts',(-2.50126484000006,5.2,-3.72115866000001));
#321745=CARTESIAN_POINT('Ctrl Pts',(-2.50126484000006,2.2,-3.72115866000001));
#321746=CARTESIAN_POINT('Ctrl Pts',(-2.49933313300006,12.2,-3.72008406500001));
#321747=CARTESIAN_POINT('Ctrl Pts',(-2.49933313300006,5.2,-3.72008406500001));
#321748=CARTESIAN_POINT('Ctrl Pts',(-2.49933313300006,2.2,-3.72008406500001));
#321749=CARTESIAN_POINT('Ctrl Pts',(-2.49740594300006,12.2,-3.71900924300002));
#321750=CARTESIAN_POINT('Ctrl Pts',(-2.49740594300006,5.2,-3.71900924300002));
#321751=CARTESIAN_POINT('Ctrl Pts',(-2.49740594300006,2.2,-3.71900924300002));
#321752=CARTESIAN_POINT('Ctrl Pts',(-2.49548327500006,12.2,-3.71793420100001));
#321753=CARTESIAN_POINT('Ctrl Pts',(-2.49548327500006,5.2,-3.71793420100001));
#321754=CARTESIAN_POINT('Ctrl Pts',(-2.49548327500006,2.2,-3.71793420100001));
#321755=CARTESIAN_POINT('Ctrl Pts',(-2.49356512900006,12.2,-3.71685895000001));
#321756=CARTESIAN_POINT('Ctrl Pts',(-2.49356512900006,5.2,-3.71685895000001));
#321757=CARTESIAN_POINT('Ctrl Pts',(-2.49356512900006,2.2,-3.71685895000001));
#321758=CARTESIAN_POINT('Ctrl Pts',(-2.49165150900006,12.2,-3.71578350000001));
#321759=CARTESIAN_POINT('Ctrl Pts',(-2.49165150900006,5.2,-3.71578350000001));
#321760=CARTESIAN_POINT('Ctrl Pts',(-2.49165150900006,2.2,-3.71578350000001));
#321761=CARTESIAN_POINT('Ctrl Pts',(-2.48974241700005,12.2,-3.71470786100002));
#321762=CARTESIAN_POINT('Ctrl Pts',(-2.48974241700005,5.2,-3.71470786100002));
#321763=CARTESIAN_POINT('Ctrl Pts',(-2.48974241700005,2.2,-3.71470786100002));
#321764=CARTESIAN_POINT('Ctrl Pts',(-2.48783785500006,12.2,-3.71363204200001));
#321765=CARTESIAN_POINT('Ctrl Pts',(-2.48783785500006,5.2,-3.71363204200001));
#321766=CARTESIAN_POINT('Ctrl Pts',(-2.48783785500006,2.2,-3.71363204200001));
#321767=CARTESIAN_POINT('Ctrl Pts',(-2.48593782500006,12.2,-3.71255605200002));
#321768=CARTESIAN_POINT('Ctrl Pts',(-2.48593782500006,5.2,-3.71255605200002));
#321769=CARTESIAN_POINT('Ctrl Pts',(-2.48593782500006,2.2,-3.71255605200002));
#321770=CARTESIAN_POINT('Ctrl Pts',(-2.48404233000006,12.2,-3.71147990400001));
#321771=CARTESIAN_POINT('Ctrl Pts',(-2.48404233000006,5.2,-3.71147990400001));
#321772=CARTESIAN_POINT('Ctrl Pts',(-2.48404233000006,2.2,-3.71147990400001));
#321773=CARTESIAN_POINT('Ctrl Pts',(-2.48215137200006,12.2,-3.71040360600002));
#321774=CARTESIAN_POINT('Ctrl Pts',(-2.48215137200006,5.2,-3.71040360600002));
#321775=CARTESIAN_POINT('Ctrl Pts',(-2.48215137200006,2.2,-3.71040360600002));
#321776=CARTESIAN_POINT('Ctrl Pts',(-2.48026495300006,12.2,-3.70932716700001));
#321777=CARTESIAN_POINT('Ctrl Pts',(-2.48026495300006,5.2,-3.70932716700001));
#321778=CARTESIAN_POINT('Ctrl Pts',(-2.48026495300006,2.2,-3.70932716700001));
#321779=CARTESIAN_POINT('Ctrl Pts',(-2.47838307600006,12.2,-3.70825059800001));
#321780=CARTESIAN_POINT('Ctrl Pts',(-2.47838307600006,5.2,-3.70825059800001));
#321781=CARTESIAN_POINT('Ctrl Pts',(-2.47838307600006,2.2,-3.70825059800001));
#321782=CARTESIAN_POINT('Ctrl Pts',(-2.47650574200006,12.2,-3.70717391000001));
#321783=CARTESIAN_POINT('Ctrl Pts',(-2.47650574200006,5.2,-3.70717391000001));
#321784=CARTESIAN_POINT('Ctrl Pts',(-2.47650574200006,2.2,-3.70717391000001));
#321785=CARTESIAN_POINT('Ctrl Pts',(-2.47463295400005,12.2,-3.70609711100002));
#321786=CARTESIAN_POINT('Ctrl Pts',(-2.47463295400005,5.2,-3.70609711100002));
#321787=CARTESIAN_POINT('Ctrl Pts',(-2.47463295400005,2.2,-3.70609711100002));
#321788=CARTESIAN_POINT('Ctrl Pts',(-2.47276471500005,12.2,-3.70502021200001));
#321789=CARTESIAN_POINT('Ctrl Pts',(-2.47276471500005,5.2,-3.70502021200001));
#321790=CARTESIAN_POINT('Ctrl Pts',(-2.47276471500005,2.2,-3.70502021200001));
#321791=CARTESIAN_POINT('Ctrl Pts',(-2.47090102700006,12.2,-3.70394322200001));
#321792=CARTESIAN_POINT('Ctrl Pts',(-2.47090102700006,5.2,-3.70394322200001));
#321793=CARTESIAN_POINT('Ctrl Pts',(-2.47090102700006,2.2,-3.70394322200001));
#321794=CARTESIAN_POINT('Ctrl Pts',(-2.46904188900006,12.2,-3.70286615300001));
#321795=CARTESIAN_POINT('Ctrl Pts',(-2.46904188900006,5.2,-3.70286615300001));
#321796=CARTESIAN_POINT('Ctrl Pts',(-2.46904188900006,2.2,-3.70286615300001));
#321797=CARTESIAN_POINT('Ctrl Pts',(-2.46718730800006,12.2,-3.70178901300001));
#321798=CARTESIAN_POINT('Ctrl Pts',(-2.46718730800006,5.2,-3.70178901300001));
#321799=CARTESIAN_POINT('Ctrl Pts',(-2.46718730800006,2.2,-3.70178901300001));
#321800=CARTESIAN_POINT('Ctrl Pts',(-2.46533728400005,12.2,-3.70071181300001));
#321801=CARTESIAN_POINT('Ctrl Pts',(-2.46533728400005,5.2,-3.70071181300001));
#321802=CARTESIAN_POINT('Ctrl Pts',(-2.46533728400005,2.2,-3.70071181300001));
#321803=CARTESIAN_POINT('Ctrl Pts',(-2.46349181900006,12.2,-3.69963456400002));
#321804=CARTESIAN_POINT('Ctrl Pts',(-2.46349181900006,5.2,-3.69963456400002));
#321805=CARTESIAN_POINT('Ctrl Pts',(-2.46349181900006,2.2,-3.69963456400002));
#321806=CARTESIAN_POINT('Ctrl Pts',(-2.46165091500006,12.2,-3.69855727400001));
#321807=CARTESIAN_POINT('Ctrl Pts',(-2.46165091500006,5.2,-3.69855727400001));
#321808=CARTESIAN_POINT('Ctrl Pts',(-2.46165091500006,2.2,-3.69855727400001));
#321809=CARTESIAN_POINT('Ctrl Pts',(-2.45981457400006,12.2,-3.69747995500001));
#321810=CARTESIAN_POINT('Ctrl Pts',(-2.45981457400006,5.2,-3.69747995500001));
#321811=CARTESIAN_POINT('Ctrl Pts',(-2.45981457400006,2.2,-3.69747995500001));
#321812=CARTESIAN_POINT('Ctrl Pts',(-2.45798280000006,12.2,-3.69640261500002));
#321813=CARTESIAN_POINT('Ctrl Pts',(-2.45798280000006,5.2,-3.69640261500002));
#321814=CARTESIAN_POINT('Ctrl Pts',(-2.45798280000006,2.2,-3.69640261500002));
#321815=CARTESIAN_POINT('Ctrl Pts',(-2.45615559300006,12.2,-3.69532526700001));
#321816=CARTESIAN_POINT('Ctrl Pts',(-2.45615559300006,5.2,-3.69532526700001));
#321817=CARTESIAN_POINT('Ctrl Pts',(-2.45615559300006,2.2,-3.69532526700001));
#321818=CARTESIAN_POINT('Ctrl Pts',(-2.45433295700006,12.2,-3.69424791900002));
#321819=CARTESIAN_POINT('Ctrl Pts',(-2.45433295700006,5.2,-3.69424791900002));
#321820=CARTESIAN_POINT('Ctrl Pts',(-2.45433295700006,2.2,-3.69424791900002));
#321821=CARTESIAN_POINT('Ctrl Pts',(-2.45251489200006,12.2,-3.69317058200001));
#321822=CARTESIAN_POINT('Ctrl Pts',(-2.45251489200006,5.2,-3.69317058200001));
#321823=CARTESIAN_POINT('Ctrl Pts',(-2.45251489200006,2.2,-3.69317058200001));
#321824=CARTESIAN_POINT('Ctrl Pts',(-2.45070140100006,12.2,-3.69209326600001));
#321825=CARTESIAN_POINT('Ctrl Pts',(-2.45070140100006,5.2,-3.69209326600001));
#321826=CARTESIAN_POINT('Ctrl Pts',(-2.45070140100006,2.2,-3.69209326600001));
#321827=CARTESIAN_POINT('Ctrl Pts',(-2.44889248600006,12.2,-3.69101598000002));
#321828=CARTESIAN_POINT('Ctrl Pts',(-2.44889248600006,5.2,-3.69101598000002));
#321829=CARTESIAN_POINT('Ctrl Pts',(-2.44889248600006,2.2,-3.69101598000002));
#321830=CARTESIAN_POINT('Ctrl Pts',(-2.44708815000005,12.2,-3.68993873700001));
#321831=CARTESIAN_POINT('Ctrl Pts',(-2.44708815000005,5.2,-3.68993873700001));
#321832=CARTESIAN_POINT('Ctrl Pts',(-2.44708815000005,2.2,-3.68993873700001));
#321833=CARTESIAN_POINT('Ctrl Pts',(-2.44528839500005,12.2,-3.68886154500002));
#321834=CARTESIAN_POINT('Ctrl Pts',(-2.44528839500005,5.2,-3.68886154500002));
#321835=CARTESIAN_POINT('Ctrl Pts',(-2.44528839500005,2.2,-3.68886154500002));
#321836=CARTESIAN_POINT('Ctrl Pts',(-2.44349322200006,12.2,-3.68778441500002));
#321837=CARTESIAN_POINT('Ctrl Pts',(-2.44349322200006,5.2,-3.68778441500002));
#321838=CARTESIAN_POINT('Ctrl Pts',(-2.44349322200006,2.2,-3.68778441500002));
#321839=CARTESIAN_POINT('Ctrl Pts',(-2.44170263400005,12.2,-3.68670735800002));
#321840=CARTESIAN_POINT('Ctrl Pts',(-2.44170263400005,5.2,-3.68670735800002));
#321841=CARTESIAN_POINT('Ctrl Pts',(-2.44170263400005,2.2,-3.68670735800002));
#321842=CARTESIAN_POINT('Ctrl Pts',(-2.43991663200006,12.2,-3.68563038300001));
#321843=CARTESIAN_POINT('Ctrl Pts',(-2.43991663200006,5.2,-3.68563038300001));
#321844=CARTESIAN_POINT('Ctrl Pts',(-2.43991663200006,2.2,-3.68563038300001));
#321845=CARTESIAN_POINT('Ctrl Pts',(-2.43813521800006,12.2,-3.68455350000001));
#321846=CARTESIAN_POINT('Ctrl Pts',(-2.43813521800006,5.2,-3.68455350000001));
#321847=CARTESIAN_POINT('Ctrl Pts',(-2.43813521800006,2.2,-3.68455350000001));
#321848=CARTESIAN_POINT('Ctrl Pts',(-2.43635839500006,12.2,-3.68347672200001));
#321849=CARTESIAN_POINT('Ctrl Pts',(-2.43635839500006,5.2,-3.68347672200001));
#321850=CARTESIAN_POINT('Ctrl Pts',(-2.43635839500006,2.2,-3.68347672200001));
#321851=CARTESIAN_POINT('Ctrl Pts',(-2.43458616500006,12.2,-3.68240005700001));
#321852=CARTESIAN_POINT('Ctrl Pts',(-2.43458616500006,5.2,-3.68240005700001));
#321853=CARTESIAN_POINT('Ctrl Pts',(-2.43458616500006,2.2,-3.68240005700001));
#321854=CARTESIAN_POINT('Ctrl Pts',(-2.43281852900005,12.2,-3.68132351600002));
#321855=CARTESIAN_POINT('Ctrl Pts',(-2.43281852900005,5.2,-3.68132351600002));
#321856=CARTESIAN_POINT('Ctrl Pts',(-2.43281852900005,2.2,-3.68132351600002));
#321857=CARTESIAN_POINT('Ctrl Pts',(-2.43105549100005,12.2,-3.68024710900002));
#321858=CARTESIAN_POINT('Ctrl Pts',(-2.43105549100005,5.2,-3.68024710900002));
#321859=CARTESIAN_POINT('Ctrl Pts',(-2.43105549100005,2.2,-3.68024710900002));
#321860=CARTESIAN_POINT('Ctrl Pts',(-2.42929705000006,12.2,-3.67917084700002));
#321861=CARTESIAN_POINT('Ctrl Pts',(-2.42929705000006,5.2,-3.67917084700002));
#321862=CARTESIAN_POINT('Ctrl Pts',(-2.42929705000006,2.2,-3.67917084700002));
#321863=CARTESIAN_POINT('Ctrl Pts',(-2.42754321100006,12.2,-3.67809474100001));
#321864=CARTESIAN_POINT('Ctrl Pts',(-2.42754321100006,5.2,-3.67809474100001));
#321865=CARTESIAN_POINT('Ctrl Pts',(-2.42754321100006,2.2,-3.67809474100001));
#321866=CARTESIAN_POINT('Ctrl Pts',(-2.42579397300006,12.2,-3.67701880000002));
#321867=CARTESIAN_POINT('Ctrl Pts',(-2.42579397300006,5.2,-3.67701880000002));
#321868=CARTESIAN_POINT('Ctrl Pts',(-2.42579397300006,2.2,-3.67701880000002));
#321869=CARTESIAN_POINT('Ctrl Pts',(-2.42404934000006,12.2,-3.67594303600002));
#321870=CARTESIAN_POINT('Ctrl Pts',(-2.42404934000006,5.2,-3.67594303600002));
#321871=CARTESIAN_POINT('Ctrl Pts',(-2.42404934000006,2.2,-3.67594303600002));
#321872=CARTESIAN_POINT('Ctrl Pts',(-2.42230931300006,12.2,-3.67486745700001));
#321873=CARTESIAN_POINT('Ctrl Pts',(-2.42230931300006,5.2,-3.67486745700001));
#321874=CARTESIAN_POINT('Ctrl Pts',(-2.42230931300006,2.2,-3.67486745700001));
#321875=CARTESIAN_POINT('Ctrl Pts',(-2.42057389400005,12.2,-3.67379207700001));
#321876=CARTESIAN_POINT('Ctrl Pts',(-2.42057389400005,5.2,-3.67379207700001));
#321877=CARTESIAN_POINT('Ctrl Pts',(-2.42057389400005,2.2,-3.67379207700001));
#321878=CARTESIAN_POINT('Ctrl Pts',(-2.41884308600006,12.2,-3.67271690500001));
#321879=CARTESIAN_POINT('Ctrl Pts',(-2.41884308600006,5.2,-3.67271690500001));
#321880=CARTESIAN_POINT('Ctrl Pts',(-2.41884308600006,2.2,-3.67271690500001));
#321881=CARTESIAN_POINT('Ctrl Pts',(-2.41711689000006,12.2,-3.67164195000001));
#321882=CARTESIAN_POINT('Ctrl Pts',(-2.41711689000006,5.2,-3.67164195000001));
#321883=CARTESIAN_POINT('Ctrl Pts',(-2.41711689000006,2.2,-3.67164195000001));
#321884=CARTESIAN_POINT('Ctrl Pts',(-2.41539530800006,12.2,-3.67056722400001));
#321885=CARTESIAN_POINT('Ctrl Pts',(-2.41539530800006,5.2,-3.67056722400001));
#321886=CARTESIAN_POINT('Ctrl Pts',(-2.41539530800006,2.2,-3.67056722400001));
#321887=CARTESIAN_POINT('Ctrl Pts',(-2.41367834100005,12.2,-3.66949273900001));
#321888=CARTESIAN_POINT('Ctrl Pts',(-2.41367834100005,5.2,-3.66949273900001));
#321889=CARTESIAN_POINT('Ctrl Pts',(-2.41367834100005,2.2,-3.66949273900001));
#321890=CARTESIAN_POINT('Ctrl Pts',(-2.41196599200005,12.2,-3.66841850200001));
#321891=CARTESIAN_POINT('Ctrl Pts',(-2.41196599200005,5.2,-3.66841850200001));
#321892=CARTESIAN_POINT('Ctrl Pts',(-2.41196599200005,2.2,-3.66841850200001));
#321893=CARTESIAN_POINT('Ctrl Pts',(-2.41025826200006,12.2,-3.66734452800001));
#321894=CARTESIAN_POINT('Ctrl Pts',(-2.41025826200006,5.2,-3.66734452800001));
#321895=CARTESIAN_POINT('Ctrl Pts',(-2.41025826200006,2.2,-3.66734452800001));
#321896=CARTESIAN_POINT('Ctrl Pts',(-2.40855515500006,12.2,-3.66627082400001));
#321897=CARTESIAN_POINT('Ctrl Pts',(-2.40855515500006,5.2,-3.66627082400001));
#321898=CARTESIAN_POINT('Ctrl Pts',(-2.40855515500006,2.2,-3.66627082400001));
#321899=CARTESIAN_POINT('Ctrl Pts',(-2.40685666900006,12.2,-3.66519740200001));
#321900=CARTESIAN_POINT('Ctrl Pts',(-2.40685666900006,5.2,-3.66519740200001));
#321901=CARTESIAN_POINT('Ctrl Pts',(-2.40685666900006,2.2,-3.66519740200001));
#321902=CARTESIAN_POINT('Ctrl Pts',(-2.40516281000006,12.2,-3.66412427300002));
#321903=CARTESIAN_POINT('Ctrl Pts',(-2.40516281000006,5.2,-3.66412427300002));
#321904=CARTESIAN_POINT('Ctrl Pts',(-2.40516281000006,2.2,-3.66412427300002));
#321905=CARTESIAN_POINT('Ctrl Pts',(-2.40347357600006,12.2,-3.66305144800001));
#321906=CARTESIAN_POINT('Ctrl Pts',(-2.40347357600006,5.2,-3.66305144800001));
#321907=CARTESIAN_POINT('Ctrl Pts',(-2.40347357600006,2.2,-3.66305144800001));
#321908=CARTESIAN_POINT('Ctrl Pts',(-2.40178897100006,12.2,-3.66197893700001));
#321909=CARTESIAN_POINT('Ctrl Pts',(-2.40178897100006,5.2,-3.66197893700001));
#321910=CARTESIAN_POINT('Ctrl Pts',(-2.40178897100006,2.2,-3.66197893700001));
#321911=CARTESIAN_POINT('Ctrl Pts',(-2.40010899700006,12.2,-3.66090675000001));
#321912=CARTESIAN_POINT('Ctrl Pts',(-2.40010899700006,5.2,-3.66090675000001));
#321913=CARTESIAN_POINT('Ctrl Pts',(-2.40010899700006,2.2,-3.66090675000001));
#321914=CARTESIAN_POINT('Ctrl Pts',(-2.39843365500006,12.2,-3.65983490000001));
#321915=CARTESIAN_POINT('Ctrl Pts',(-2.39843365500006,5.2,-3.65983490000001));
#321916=CARTESIAN_POINT('Ctrl Pts',(-2.39843365500006,2.2,-3.65983490000001));
#321917=CARTESIAN_POINT('Ctrl Pts',(-2.39676294700006,12.2,-3.65876339700002));
#321918=CARTESIAN_POINT('Ctrl Pts',(-2.39676294700006,5.2,-3.65876339700002));
#321919=CARTESIAN_POINT('Ctrl Pts',(-2.39676294700006,2.2,-3.65876339700002));
#321920=CARTESIAN_POINT('Ctrl Pts',(-2.39509687400006,12.2,-3.65769224900002));
#321921=CARTESIAN_POINT('Ctrl Pts',(-2.39509687400006,5.2,-3.65769224900002));
#321922=CARTESIAN_POINT('Ctrl Pts',(-2.39509687400006,2.2,-3.65769224900002));
#321923=CARTESIAN_POINT('Ctrl Pts',(-2.39343543800006,12.2,-3.65662147100001));
#321924=CARTESIAN_POINT('Ctrl Pts',(-2.39343543800006,5.2,-3.65662147100001));
#321925=CARTESIAN_POINT('Ctrl Pts',(-2.39343543800006,2.2,-3.65662147100001));
#321926=CARTESIAN_POINT('Ctrl Pts',(-2.39177864100005,12.2,-3.65555107100001));
#321927=CARTESIAN_POINT('Ctrl Pts',(-2.39177864100005,5.2,-3.65555107100001));
#321928=CARTESIAN_POINT('Ctrl Pts',(-2.39177864100005,2.2,-3.65555107100001));
#321929=CARTESIAN_POINT('Ctrl Pts',(-2.39012648600006,12.2,-3.65448106200001));
#321930=CARTESIAN_POINT('Ctrl Pts',(-2.39012648600006,5.2,-3.65448106200001));
#321931=CARTESIAN_POINT('Ctrl Pts',(-2.39012648600006,2.2,-3.65448106200001));
#321932=CARTESIAN_POINT('Ctrl Pts',(-2.38847897200006,12.2,-3.65341145300001));
#321933=CARTESIAN_POINT('Ctrl Pts',(-2.38847897200006,5.2,-3.65341145300001));
#321934=CARTESIAN_POINT('Ctrl Pts',(-2.38847897200006,2.2,-3.65341145300001));
#321935=CARTESIAN_POINT('Ctrl Pts',(-2.38683610300006,12.2,-3.65234225600001));
#321936=CARTESIAN_POINT('Ctrl Pts',(-2.38683610300006,5.2,-3.65234225600001));
#321937=CARTESIAN_POINT('Ctrl Pts',(-2.38683610300006,2.2,-3.65234225600001));
#321938=CARTESIAN_POINT('Ctrl Pts',(-2.38519788000006,12.2,-3.65127348100001));
#321939=CARTESIAN_POINT('Ctrl Pts',(-2.38519788000006,5.2,-3.65127348100001));
#321940=CARTESIAN_POINT('Ctrl Pts',(-2.38519788000006,2.2,-3.65127348100001));
#321941=CARTESIAN_POINT('Ctrl Pts',(-2.38356430300006,12.2,-3.65020514000001));
#321942=CARTESIAN_POINT('Ctrl Pts',(-2.38356430300006,5.2,-3.65020514000001));
#321943=CARTESIAN_POINT('Ctrl Pts',(-2.38356430300006,2.2,-3.65020514000001));
#321944=CARTESIAN_POINT('Ctrl Pts',(-2.38193537600006,12.2,-3.64913724300001));
#321945=CARTESIAN_POINT('Ctrl Pts',(-2.38193537600006,5.2,-3.64913724300001));
#321946=CARTESIAN_POINT('Ctrl Pts',(-2.38193537600006,2.2,-3.64913724300001));
#321947=CARTESIAN_POINT('Ctrl Pts',(-2.38031110000006,12.2,-3.64806980200001));
#321948=CARTESIAN_POINT('Ctrl Pts',(-2.38031110000006,5.2,-3.64806980200001));
#321949=CARTESIAN_POINT('Ctrl Pts',(-2.38031110000006,2.2,-3.64806980200001));
#321950=CARTESIAN_POINT('Ctrl Pts',(-2.37869147600006,12.2,-3.64700282800001));
#321951=CARTESIAN_POINT('Ctrl Pts',(-2.37869147600006,5.2,-3.64700282800001));
#321952=CARTESIAN_POINT('Ctrl Pts',(-2.37869147600006,2.2,-3.64700282800001));
#321953=CARTESIAN_POINT('Ctrl Pts',(-2.37707650600006,12.2,-3.64593633100001));
#321954=CARTESIAN_POINT('Ctrl Pts',(-2.37707650600006,5.2,-3.64593633100001));
#321955=CARTESIAN_POINT('Ctrl Pts',(-2.37707650600006,2.2,-3.64593633100001));
#321956=CARTESIAN_POINT('Ctrl Pts',(-2.37546619100006,12.2,-3.64487032100001));
#321957=CARTESIAN_POINT('Ctrl Pts',(-2.37546619100006,5.2,-3.64487032100001));
#321958=CARTESIAN_POINT('Ctrl Pts',(-2.37546619100006,2.2,-3.64487032100001));
#321959=CARTESIAN_POINT('Ctrl Pts',(-2.37386053300006,12.2,-3.64380481300001));
#321960=CARTESIAN_POINT('Ctrl Pts',(-2.37386053300006,5.2,-3.64380481300001));
#321961=CARTESIAN_POINT('Ctrl Pts',(-2.37386053300006,2.2,-3.64380481300001));
#321962=CARTESIAN_POINT('Ctrl Pts',(-2.37225953400006,12.2,-3.64273981500002));
#321963=CARTESIAN_POINT('Ctrl Pts',(-2.37225953400006,5.2,-3.64273981500002));
#321964=CARTESIAN_POINT('Ctrl Pts',(-2.37225953400006,2.2,-3.64273981500002));
#321965=CARTESIAN_POINT('Ctrl Pts',(-2.37066319500005,12.2,-3.64167533800002));
#321966=CARTESIAN_POINT('Ctrl Pts',(-2.37066319500005,5.2,-3.64167533800002));
#321967=CARTESIAN_POINT('Ctrl Pts',(-2.37066319500005,2.2,-3.64167533800002));
#321968=CARTESIAN_POINT('Ctrl Pts',(-2.36907151800006,12.2,-3.64061139500001));
#321969=CARTESIAN_POINT('Ctrl Pts',(-2.36907151800006,5.2,-3.64061139500001));
#321970=CARTESIAN_POINT('Ctrl Pts',(-2.36907151800006,2.2,-3.64061139500001));
#321971=CARTESIAN_POINT('Ctrl Pts',(-2.36748450500006,12.2,-3.63954799500001));
#321972=CARTESIAN_POINT('Ctrl Pts',(-2.36748450500006,5.2,-3.63954799500001));
#321973=CARTESIAN_POINT('Ctrl Pts',(-2.36748450500006,2.2,-3.63954799500001));
#321974=CARTESIAN_POINT('Ctrl Pts',(-2.36590215600006,12.2,-3.63848515200001));
#321975=CARTESIAN_POINT('Ctrl Pts',(-2.36590215600006,5.2,-3.63848515200001));
#321976=CARTESIAN_POINT('Ctrl Pts',(-2.36590215600006,2.2,-3.63848515200001));
#321977=CARTESIAN_POINT('Ctrl Pts',(-2.36432447400006,12.2,-3.63742287500001));
#321978=CARTESIAN_POINT('Ctrl Pts',(-2.36432447400006,5.2,-3.63742287500001));
#321979=CARTESIAN_POINT('Ctrl Pts',(-2.36432447400006,2.2,-3.63742287500001));
#321980=CARTESIAN_POINT('Ctrl Pts',(-2.36275145800006,12.2,-3.63636117400001));
#321981=CARTESIAN_POINT('Ctrl Pts',(-2.36275145800006,5.2,-3.63636117400001));
#321982=CARTESIAN_POINT('Ctrl Pts',(-2.36275145800006,2.2,-3.63636117400001));
#321983=CARTESIAN_POINT('Ctrl Pts',(-2.36118311300006,12.2,-3.63530006400001));
#321984=CARTESIAN_POINT('Ctrl Pts',(-2.36118311300006,5.2,-3.63530006400001));
#321985=CARTESIAN_POINT('Ctrl Pts',(-2.36118311300006,2.2,-3.63530006400001));
#321986=CARTESIAN_POINT('Ctrl Pts',(-2.35961943900006,12.2,-3.63423955300001));
#321987=CARTESIAN_POINT('Ctrl Pts',(-2.35961943900006,5.2,-3.63423955300001));
#321988=CARTESIAN_POINT('Ctrl Pts',(-2.35961943900006,2.2,-3.63423955300001));
#321989=CARTESIAN_POINT('Ctrl Pts',(-2.35806043600005,12.2,-3.63317965400002));
#321990=CARTESIAN_POINT('Ctrl Pts',(-2.35806043600005,5.2,-3.63317965400002));
#321991=CARTESIAN_POINT('Ctrl Pts',(-2.35806043600005,2.2,-3.63317965400002));
#321992=CARTESIAN_POINT('Ctrl Pts',(-2.35650610600006,12.2,-3.63212037800002));
#321993=CARTESIAN_POINT('Ctrl Pts',(-2.35650610600006,5.2,-3.63212037800002));
#321994=CARTESIAN_POINT('Ctrl Pts',(-2.35650610600006,2.2,-3.63212037800002));
#321995=CARTESIAN_POINT('Ctrl Pts',(-2.35495645300006,12.2,-3.63106173500002));
#321996=CARTESIAN_POINT('Ctrl Pts',(-2.35495645300006,5.2,-3.63106173500002));
#321997=CARTESIAN_POINT('Ctrl Pts',(-2.35495645300006,2.2,-3.63106173500002));
#321998=CARTESIAN_POINT('Ctrl Pts',(-2.35341147600006,12.2,-3.63000373800002));
#321999=CARTESIAN_POINT('Ctrl Pts',(-2.35341147600006,5.2,-3.63000373800002));
#322000=CARTESIAN_POINT('Ctrl Pts',(-2.35341147600006,2.2,-3.63000373800002));
#322001=CARTESIAN_POINT('Ctrl Pts',(-2.35187117600006,12.2,-3.62894639800002));
#322002=CARTESIAN_POINT('Ctrl Pts',(-2.35187117600006,5.2,-3.62894639800002));
#322003=CARTESIAN_POINT('Ctrl Pts',(-2.35187117600006,2.2,-3.62894639800002));
#322004=CARTESIAN_POINT('Ctrl Pts',(-2.35033555600006,12.2,-3.62788972600002));
#322005=CARTESIAN_POINT('Ctrl Pts',(-2.35033555600006,5.2,-3.62788972600002));
#322006=CARTESIAN_POINT('Ctrl Pts',(-2.35033555600006,2.2,-3.62788972600002));
#322007=CARTESIAN_POINT('Ctrl Pts',(-2.34880461600006,12.2,-3.62683373300001));
#322008=CARTESIAN_POINT('Ctrl Pts',(-2.34880461600006,5.2,-3.62683373300001));
#322009=CARTESIAN_POINT('Ctrl Pts',(-2.34880461600006,2.2,-3.62683373300001));
#322010=CARTESIAN_POINT('Ctrl Pts',(-2.34727835800005,12.2,-3.62577843200001));
#322011=CARTESIAN_POINT('Ctrl Pts',(-2.34727835800005,5.2,-3.62577843200001));
#322012=CARTESIAN_POINT('Ctrl Pts',(-2.34727835800005,2.2,-3.62577843200001));
#322013=CARTESIAN_POINT('Ctrl Pts',(-2.34575678400006,12.2,-3.62472383300001));
#322014=CARTESIAN_POINT('Ctrl Pts',(-2.34575678400006,5.2,-3.62472383300001));
#322015=CARTESIAN_POINT('Ctrl Pts',(-2.34575678400006,2.2,-3.62472383300001));
#322016=CARTESIAN_POINT('Ctrl Pts',(-2.34423989400006,12.2,-3.62366994800002));
#322017=CARTESIAN_POINT('Ctrl Pts',(-2.34423989400006,5.2,-3.62366994800002));
#322018=CARTESIAN_POINT('Ctrl Pts',(-2.34423989400006,2.2,-3.62366994800002));
#322019=CARTESIAN_POINT('Ctrl Pts',(-2.34272769000006,12.2,-3.62261678700001));
#322020=CARTESIAN_POINT('Ctrl Pts',(-2.34272769000006,5.2,-3.62261678700001));
#322021=CARTESIAN_POINT('Ctrl Pts',(-2.34272769000006,2.2,-3.62261678700001));
#322022=CARTESIAN_POINT('Ctrl Pts',(-2.34122017400006,12.2,-3.62156436400001));
#322023=CARTESIAN_POINT('Ctrl Pts',(-2.34122017400006,5.2,-3.62156436400001));
#322024=CARTESIAN_POINT('Ctrl Pts',(-2.34122017400006,2.2,-3.62156436400001));
#322025=CARTESIAN_POINT('Ctrl Pts',(-2.33971734600006,12.2,-3.62051269000002));
#322026=CARTESIAN_POINT('Ctrl Pts',(-2.33971734600006,5.2,-3.62051269000002));
#322027=CARTESIAN_POINT('Ctrl Pts',(-2.33971734600006,2.2,-3.62051269000002));
#322028=CARTESIAN_POINT('Ctrl Pts',(-2.33821920800006,12.2,-3.61946177600001));
#322029=CARTESIAN_POINT('Ctrl Pts',(-2.33821920800006,5.2,-3.61946177600001));
#322030=CARTESIAN_POINT('Ctrl Pts',(-2.33821920800006,2.2,-3.61946177600001));
#322031=CARTESIAN_POINT('Ctrl Pts',(-2.33672576200005,12.2,-3.61841163300001));
#322032=CARTESIAN_POINT('Ctrl Pts',(-2.33672576200005,5.2,-3.61841163300001));
#322033=CARTESIAN_POINT('Ctrl Pts',(-2.33672576200005,2.2,-3.61841163300001));
#322034=CARTESIAN_POINT('Ctrl Pts',(-2.33523700800006,12.2,-3.61736227300002));
#322035=CARTESIAN_POINT('Ctrl Pts',(-2.33523700800006,5.2,-3.61736227300002));
#322036=CARTESIAN_POINT('Ctrl Pts',(-2.33523700800006,2.2,-3.61736227300002));
#322037=CARTESIAN_POINT('Ctrl Pts',(-2.33375294700005,12.2,-3.61631370800001));
#322038=CARTESIAN_POINT('Ctrl Pts',(-2.33375294700005,5.2,-3.61631370800001));
#322039=CARTESIAN_POINT('Ctrl Pts',(-2.33375294700005,2.2,-3.61631370800001));
#322040=CARTESIAN_POINT('Ctrl Pts',(-2.33227358100006,12.2,-3.61526595000001));
#322041=CARTESIAN_POINT('Ctrl Pts',(-2.33227358100006,5.2,-3.61526595000001));
#322042=CARTESIAN_POINT('Ctrl Pts',(-2.33227358100006,2.2,-3.61526595000001));
#322043=CARTESIAN_POINT('Ctrl Pts',(-2.33079891200005,12.2,-3.61421900900002));
#322044=CARTESIAN_POINT('Ctrl Pts',(-2.33079891200005,5.2,-3.61421900900002));
#322045=CARTESIAN_POINT('Ctrl Pts',(-2.33079891200005,2.2,-3.61421900900002));
#322046=CARTESIAN_POINT('Ctrl Pts',(-2.32932893900006,12.2,-3.61317289800001));
#322047=CARTESIAN_POINT('Ctrl Pts',(-2.32932893900006,5.2,-3.61317289800001));
#322048=CARTESIAN_POINT('Ctrl Pts',(-2.32932893900006,2.2,-3.61317289800001));
#322049=CARTESIAN_POINT('Ctrl Pts',(-2.32786366600005,12.2,-3.61212762900001));
#322050=CARTESIAN_POINT('Ctrl Pts',(-2.32786366600005,5.2,-3.61212762900001));
#322051=CARTESIAN_POINT('Ctrl Pts',(-2.32786366600005,2.2,-3.61212762900001));
#322052=CARTESIAN_POINT('Ctrl Pts',(-2.32640309200006,12.2,-3.61108321200001));
#322053=CARTESIAN_POINT('Ctrl Pts',(-2.32640309200006,5.2,-3.61108321200001));
#322054=CARTESIAN_POINT('Ctrl Pts',(-2.32640309200006,2.2,-3.61108321200001));
#322055=CARTESIAN_POINT('Ctrl Pts',(-2.32494721700006,12.2,-3.61003966100002));
#322056=CARTESIAN_POINT('Ctrl Pts',(-2.32494721700006,5.2,-3.61003966100002));
#322057=CARTESIAN_POINT('Ctrl Pts',(-2.32494721700006,2.2,-3.61003966100002));
#322058=CARTESIAN_POINT('Ctrl Pts',(-2.32349604700006,12.2,-3.60899698600001));
#322059=CARTESIAN_POINT('Ctrl Pts',(-2.32349604700006,5.2,-3.60899698600001));
#322060=CARTESIAN_POINT('Ctrl Pts',(-2.32349604700006,2.2,-3.60899698600001));
#322061=CARTESIAN_POINT('Ctrl Pts',(-2.32204957800006,12.2,-3.60795520000002));
#322062=CARTESIAN_POINT('Ctrl Pts',(-2.32204957800006,5.2,-3.60795520000002));
#322063=CARTESIAN_POINT('Ctrl Pts',(-2.32204957800006,2.2,-3.60795520000002));
#322064=CARTESIAN_POINT('Ctrl Pts',(-2.32060781400006,12.2,-3.60691431500001));
#322065=CARTESIAN_POINT('Ctrl Pts',(-2.32060781400006,5.2,-3.60691431500001));
#322066=CARTESIAN_POINT('Ctrl Pts',(-2.32060781400006,2.2,-3.60691431500001));
#322067=CARTESIAN_POINT('Ctrl Pts',(-2.31917075400006,12.2,-3.60587434100001));
#322068=CARTESIAN_POINT('Ctrl Pts',(-2.31917075400006,5.2,-3.60587434100001));
#322069=CARTESIAN_POINT('Ctrl Pts',(-2.31917075400006,2.2,-3.60587434100001));
#322070=CARTESIAN_POINT('Ctrl Pts',(-2.31773840300006,12.2,-3.60483529100001));
#322071=CARTESIAN_POINT('Ctrl Pts',(-2.31773840300006,5.2,-3.60483529100001));
#322072=CARTESIAN_POINT('Ctrl Pts',(-2.31773840300006,2.2,-3.60483529100001));
#322073=CARTESIAN_POINT('Ctrl Pts',(-2.31631075700005,12.2,-3.60379717800001));
#322074=CARTESIAN_POINT('Ctrl Pts',(-2.31631075700005,5.2,-3.60379717800001));
#322075=CARTESIAN_POINT('Ctrl Pts',(-2.31631075700005,2.2,-3.60379717800001));
#322076=CARTESIAN_POINT('Ctrl Pts',(-2.31488782100006,12.2,-3.60276001200001));
#322077=CARTESIAN_POINT('Ctrl Pts',(-2.31488782100006,5.2,-3.60276001200001));
#322078=CARTESIAN_POINT('Ctrl Pts',(-2.31488782100006,2.2,-3.60276001200001));
#322079=CARTESIAN_POINT('Ctrl Pts',(-2.31346959400006,12.2,-3.60172380500002));
#322080=CARTESIAN_POINT('Ctrl Pts',(-2.31346959400006,5.2,-3.60172380500002));
#322081=CARTESIAN_POINT('Ctrl Pts',(-2.31346959400006,2.2,-3.60172380500002));
#322082=CARTESIAN_POINT('Ctrl Pts',(-2.31205607800006,12.2,-3.60068857100002));
#322083=CARTESIAN_POINT('Ctrl Pts',(-2.31205607800006,5.2,-3.60068857100002));
#322084=CARTESIAN_POINT('Ctrl Pts',(-2.31205607800006,2.2,-3.60068857100002));
#322085=CARTESIAN_POINT('Ctrl Pts',(-2.31064727300006,12.2,-3.59965432000001));
#322086=CARTESIAN_POINT('Ctrl Pts',(-2.31064727300006,5.2,-3.59965432000001));
#322087=CARTESIAN_POINT('Ctrl Pts',(-2.31064727300006,2.2,-3.59965432000001));
#322088=CARTESIAN_POINT('Ctrl Pts',(-2.30924318100006,12.2,-3.59862106400001));
#322089=CARTESIAN_POINT('Ctrl Pts',(-2.30924318100006,5.2,-3.59862106400001));
#322090=CARTESIAN_POINT('Ctrl Pts',(-2.30924318100006,2.2,-3.59862106400001));
#322091=CARTESIAN_POINT('Ctrl Pts',(-2.30784380200005,12.2,-3.59758881800001));
#322092=CARTESIAN_POINT('Ctrl Pts',(-2.30784380200005,5.2,-3.59758881800001));
#322093=CARTESIAN_POINT('Ctrl Pts',(-2.30784380200005,2.2,-3.59758881800001));
#322094=CARTESIAN_POINT('Ctrl Pts',(-2.30644913800006,12.2,-3.59655759000002));
#322095=CARTESIAN_POINT('Ctrl Pts',(-2.30644913800006,5.2,-3.59655759000002));
#322096=CARTESIAN_POINT('Ctrl Pts',(-2.30644913800006,2.2,-3.59655759000002));
#322097=CARTESIAN_POINT('Ctrl Pts',(-2.30505918900006,12.2,-3.59552739400002));
#322098=CARTESIAN_POINT('Ctrl Pts',(-2.30505918900006,5.2,-3.59552739400002));
#322099=CARTESIAN_POINT('Ctrl Pts',(-2.30505918900006,2.2,-3.59552739400002));
#322100=CARTESIAN_POINT('Ctrl Pts',(-2.30367395700006,12.2,-3.59449824100002));
#322101=CARTESIAN_POINT('Ctrl Pts',(-2.30367395700006,5.2,-3.59449824100002));
#322102=CARTESIAN_POINT('Ctrl Pts',(-2.30367395700006,2.2,-3.59449824100002));
#322103=CARTESIAN_POINT('Ctrl Pts',(-2.30229344300006,12.2,-3.59347014600001));
#322104=CARTESIAN_POINT('Ctrl Pts',(-2.30229344300006,5.2,-3.59347014600001));
#322105=CARTESIAN_POINT('Ctrl Pts',(-2.30229344300006,2.2,-3.59347014600001));
#322106=CARTESIAN_POINT('Ctrl Pts',(-2.30091764700005,12.2,-3.59244311700001));
#322107=CARTESIAN_POINT('Ctrl Pts',(-2.30091764700005,5.2,-3.59244311700001));
#322108=CARTESIAN_POINT('Ctrl Pts',(-2.30091764700005,2.2,-3.59244311700001));
#322109=CARTESIAN_POINT('Ctrl Pts',(-2.29954657000006,12.2,-3.59141717000002));
#322110=CARTESIAN_POINT('Ctrl Pts',(-2.29954657000006,5.2,-3.59141717000002));
#322111=CARTESIAN_POINT('Ctrl Pts',(-2.29954657000006,2.2,-3.59141717000002));
#322112=CARTESIAN_POINT('Ctrl Pts',(-2.29818021300006,12.2,-3.59039231400001));
#322113=CARTESIAN_POINT('Ctrl Pts',(-2.29818021300006,5.2,-3.59039231400001));
#322114=CARTESIAN_POINT('Ctrl Pts',(-2.29818021300006,2.2,-3.59039231400001));
#322115=CARTESIAN_POINT('Ctrl Pts',(-2.29681857700006,12.2,-3.58936856400002));
#322116=CARTESIAN_POINT('Ctrl Pts',(-2.29681857700006,5.2,-3.58936856400002));
#322117=CARTESIAN_POINT('Ctrl Pts',(-2.29681857700006,2.2,-3.58936856400002));
#322118=CARTESIAN_POINT('Ctrl Pts',(-2.29546166300006,12.2,-3.58834593000001));
#322119=CARTESIAN_POINT('Ctrl Pts',(-2.29546166300006,5.2,-3.58834593000001));
#322120=CARTESIAN_POINT('Ctrl Pts',(-2.29546166300006,2.2,-3.58834593000001));
#322121=CARTESIAN_POINT('Ctrl Pts',(-2.29410947100006,12.2,-3.58732442600001));
#322122=CARTESIAN_POINT('Ctrl Pts',(-2.29410947100006,5.2,-3.58732442600001));
#322123=CARTESIAN_POINT('Ctrl Pts',(-2.29410947100006,2.2,-3.58732442600001));
#322124=CARTESIAN_POINT('Ctrl Pts',(-2.29276200300006,12.2,-3.58630406300001));
#322125=CARTESIAN_POINT('Ctrl Pts',(-2.29276200300006,5.2,-3.58630406300001));
#322126=CARTESIAN_POINT('Ctrl Pts',(-2.29276200300006,2.2,-3.58630406300001));
#322127=CARTESIAN_POINT('Ctrl Pts',(-2.29141926000006,12.2,-3.58528485300001));
#322128=CARTESIAN_POINT('Ctrl Pts',(-2.29141926000006,5.2,-3.58528485300001));
#322129=CARTESIAN_POINT('Ctrl Pts',(-2.29141926000006,2.2,-3.58528485300001));
#322130=CARTESIAN_POINT('Ctrl Pts',(-2.29008124100006,12.2,-3.58426681000001));
#322131=CARTESIAN_POINT('Ctrl Pts',(-2.29008124100006,5.2,-3.58426681000001));
#322132=CARTESIAN_POINT('Ctrl Pts',(-2.29008124100006,2.2,-3.58426681000001));
#322133=CARTESIAN_POINT('Ctrl Pts',(-2.28874794800006,12.2,-3.58324994600002));
#322134=CARTESIAN_POINT('Ctrl Pts',(-2.28874794800006,5.2,-3.58324994600002));
#322135=CARTESIAN_POINT('Ctrl Pts',(-2.28874794800006,2.2,-3.58324994600002));
#322136=CARTESIAN_POINT('Ctrl Pts',(-2.28741938200006,12.2,-3.58223427200001));
#322137=CARTESIAN_POINT('Ctrl Pts',(-2.28741938200006,5.2,-3.58223427200001));
#322138=CARTESIAN_POINT('Ctrl Pts',(-2.28741938200006,2.2,-3.58223427200001));
#322139=CARTESIAN_POINT('Ctrl Pts',(-2.28609554300006,12.2,-3.58121980100002));
#322140=CARTESIAN_POINT('Ctrl Pts',(-2.28609554300006,5.2,-3.58121980100002));
#322141=CARTESIAN_POINT('Ctrl Pts',(-2.28609554300006,2.2,-3.58121980100002));
#322142=CARTESIAN_POINT('Ctrl Pts',(-2.28477643300006,12.2,-3.58020654600002));
#322143=CARTESIAN_POINT('Ctrl Pts',(-2.28477643300006,5.2,-3.58020654600002));
#322144=CARTESIAN_POINT('Ctrl Pts',(-2.28477643300006,2.2,-3.58020654600002));
#322145=CARTESIAN_POINT('Ctrl Pts',(-2.28346205200006,12.2,-3.57919451900001));
#322146=CARTESIAN_POINT('Ctrl Pts',(-2.28346205200006,5.2,-3.57919451900001));
#322147=CARTESIAN_POINT('Ctrl Pts',(-2.28346205200006,2.2,-3.57919451900001));
#322148=CARTESIAN_POINT('Ctrl Pts',(-2.28215239900006,12.2,-3.57818373200002));
#322149=CARTESIAN_POINT('Ctrl Pts',(-2.28215239900006,5.2,-3.57818373200002));
#322150=CARTESIAN_POINT('Ctrl Pts',(-2.28215239900006,2.2,-3.57818373200002));
#322151=CARTESIAN_POINT('Ctrl Pts',(-2.28084747800006,12.2,-3.57717419900001));
#322152=CARTESIAN_POINT('Ctrl Pts',(-2.28084747800006,5.2,-3.57717419900001));
#322153=CARTESIAN_POINT('Ctrl Pts',(-2.28084747800006,2.2,-3.57717419900001));
#322154=CARTESIAN_POINT('Ctrl Pts',(-2.27954728600006,12.2,-3.57616593100001));
#322155=CARTESIAN_POINT('Ctrl Pts',(-2.27954728600006,5.2,-3.57616593100001));
#322156=CARTESIAN_POINT('Ctrl Pts',(-2.27954728600006,2.2,-3.57616593100001));
#322157=CARTESIAN_POINT('Ctrl Pts',(-2.27825182700006,12.2,-3.57515894100001));
#322158=CARTESIAN_POINT('Ctrl Pts',(-2.27825182700006,5.2,-3.57515894100001));
#322159=CARTESIAN_POINT('Ctrl Pts',(-2.27825182700006,2.2,-3.57515894100001));
#322160=CARTESIAN_POINT('Ctrl Pts',(-2.27696109900006,12.2,-3.57415324200002));
#322161=CARTESIAN_POINT('Ctrl Pts',(-2.27696109900006,5.2,-3.57415324200002));
#322162=CARTESIAN_POINT('Ctrl Pts',(-2.27696109900006,2.2,-3.57415324200002));
#322163=CARTESIAN_POINT('Ctrl Pts',(-2.27567510500006,12.2,-3.57314884700001));
#322164=CARTESIAN_POINT('Ctrl Pts',(-2.27567510500006,5.2,-3.57314884700001));
#322165=CARTESIAN_POINT('Ctrl Pts',(-2.27567510500006,2.2,-3.57314884700001));
#322166=CARTESIAN_POINT('Ctrl Pts',(-2.27439384400005,12.2,-3.57214576600001));
#322167=CARTESIAN_POINT('Ctrl Pts',(-2.27439384400005,5.2,-3.57214576600001));
#322168=CARTESIAN_POINT('Ctrl Pts',(-2.27439384400005,2.2,-3.57214576600001));
#322169=CARTESIAN_POINT('Ctrl Pts',(-2.27311731600006,12.2,-3.57114401400001));
#322170=CARTESIAN_POINT('Ctrl Pts',(-2.27311731600006,5.2,-3.57114401400001));
#322171=CARTESIAN_POINT('Ctrl Pts',(-2.27311731600006,2.2,-3.57114401400001));
#322172=CARTESIAN_POINT('Ctrl Pts',(-2.27184552400006,12.2,-3.57014360500001));
#322173=CARTESIAN_POINT('Ctrl Pts',(-2.27184552400006,5.2,-3.57014360500001));
#322174=CARTESIAN_POINT('Ctrl Pts',(-2.27184552400006,2.2,-3.57014360500001));
#322175=CARTESIAN_POINT('Ctrl Pts',(-2.27057846700006,12.2,-3.56914454800001));
#322176=CARTESIAN_POINT('Ctrl Pts',(-2.27057846700006,5.2,-3.56914454800001));
#322177=CARTESIAN_POINT('Ctrl Pts',(-2.27057846700006,2.2,-3.56914454800001));
#322178=CARTESIAN_POINT('Ctrl Pts',(-2.26931614600006,12.2,-3.56814685800002));
#322179=CARTESIAN_POINT('Ctrl Pts',(-2.26931614600006,5.2,-3.56814685800002));
#322180=CARTESIAN_POINT('Ctrl Pts',(-2.26931614600006,2.2,-3.56814685800002));
#322181=CARTESIAN_POINT('Ctrl Pts',(-2.26805856000006,12.2,-3.56715054700001));
#322182=CARTESIAN_POINT('Ctrl Pts',(-2.26805856000006,5.2,-3.56715054700001));
#322183=CARTESIAN_POINT('Ctrl Pts',(-2.26805856000006,2.2,-3.56715054700001));
#322184=CARTESIAN_POINT('Ctrl Pts',(-2.26680571100006,12.2,-3.56615562900001));
#322185=CARTESIAN_POINT('Ctrl Pts',(-2.26680571100006,5.2,-3.56615562900001));
#322186=CARTESIAN_POINT('Ctrl Pts',(-2.26680571100006,2.2,-3.56615562900001));
#322187=CARTESIAN_POINT('Ctrl Pts',(-2.26555760000006,12.2,-3.56516211500002));
#322188=CARTESIAN_POINT('Ctrl Pts',(-2.26555760000006,5.2,-3.56516211500002));
#322189=CARTESIAN_POINT('Ctrl Pts',(-2.26555760000006,2.2,-3.56516211500002));
#322190=CARTESIAN_POINT('Ctrl Pts',(-2.26431422600006,12.2,-3.56417002000001));
#322191=CARTESIAN_POINT('Ctrl Pts',(-2.26431422600006,5.2,-3.56417002000001));
#322192=CARTESIAN_POINT('Ctrl Pts',(-2.26431422600006,2.2,-3.56417002000001));
#322193=CARTESIAN_POINT('Ctrl Pts',(-2.26307559100006,12.2,-3.56317935400002));
#322194=CARTESIAN_POINT('Ctrl Pts',(-2.26307559100006,5.2,-3.56317935400002));
#322195=CARTESIAN_POINT('Ctrl Pts',(-2.26307559100006,2.2,-3.56317935400002));
#322196=CARTESIAN_POINT('Ctrl Pts',(-2.26184169300006,12.2,-3.56219013200001));
#322197=CARTESIAN_POINT('Ctrl Pts',(-2.26184169300006,5.2,-3.56219013200001));
#322198=CARTESIAN_POINT('Ctrl Pts',(-2.26184169300006,2.2,-3.56219013200001));
#322199=CARTESIAN_POINT('Ctrl Pts',(-2.26061253600006,12.2,-3.56120236700002));
#322200=CARTESIAN_POINT('Ctrl Pts',(-2.26061253600006,5.2,-3.56120236700002));
#322201=CARTESIAN_POINT('Ctrl Pts',(-2.26061253600006,2.2,-3.56120236700002));
#322202=CARTESIAN_POINT('Ctrl Pts',(-2.25938811800006,12.2,-3.56021607000002));
#322203=CARTESIAN_POINT('Ctrl Pts',(-2.25938811800006,5.2,-3.56021607000002));
#322204=CARTESIAN_POINT('Ctrl Pts',(-2.25938811800006,2.2,-3.56021607000002));
#322205=CARTESIAN_POINT('Ctrl Pts',(-2.25816843900006,12.2,-3.55923125600001));
#322206=CARTESIAN_POINT('Ctrl Pts',(-2.25816843900006,5.2,-3.55923125600001));
#322207=CARTESIAN_POINT('Ctrl Pts',(-2.25816843900006,2.2,-3.55923125600001));
#322208=CARTESIAN_POINT('Ctrl Pts',(-2.25695350000006,12.2,-3.55824793700001));
#322209=CARTESIAN_POINT('Ctrl Pts',(-2.25695350000006,5.2,-3.55824793700001));
#322210=CARTESIAN_POINT('Ctrl Pts',(-2.25695350000006,2.2,-3.55824793700001));
#322211=CARTESIAN_POINT('Ctrl Pts',(-2.25574330200006,12.2,-3.55726612600002));
#322212=CARTESIAN_POINT('Ctrl Pts',(-2.25574330200006,5.2,-3.55726612600002));
#322213=CARTESIAN_POINT('Ctrl Pts',(-2.25574330200006,2.2,-3.55726612600002));
#322214=CARTESIAN_POINT('Ctrl Pts',(-2.25453784600006,12.2,-3.55628583600001));
#322215=CARTESIAN_POINT('Ctrl Pts',(-2.25453784600006,5.2,-3.55628583600001));
#322216=CARTESIAN_POINT('Ctrl Pts',(-2.25453784600006,2.2,-3.55628583600001));
#322217=CARTESIAN_POINT('Ctrl Pts',(-2.25333713000006,12.2,-3.55530708100002));
#322218=CARTESIAN_POINT('Ctrl Pts',(-2.25333713000006,5.2,-3.55530708100002));
#322219=CARTESIAN_POINT('Ctrl Pts',(-2.25333713000006,2.2,-3.55530708100002));
#322220=CARTESIAN_POINT('Ctrl Pts',(-2.25214115600005,12.2,-3.55432987300001));
#322221=CARTESIAN_POINT('Ctrl Pts',(-2.25214115600005,5.2,-3.55432987300001));
#322222=CARTESIAN_POINT('Ctrl Pts',(-2.25214115600005,2.2,-3.55432987300001));
#322223=CARTESIAN_POINT('Ctrl Pts',(-2.25094992400006,12.2,-3.55335422500001));
#322224=CARTESIAN_POINT('Ctrl Pts',(-2.25094992400006,5.2,-3.55335422500001));
#322225=CARTESIAN_POINT('Ctrl Pts',(-2.25094992400006,2.2,-3.55335422500001));
#322226=CARTESIAN_POINT('Ctrl Pts',(-2.24976343500006,12.2,-3.55238015100001));
#322227=CARTESIAN_POINT('Ctrl Pts',(-2.24976343500006,5.2,-3.55238015100001));
#322228=CARTESIAN_POINT('Ctrl Pts',(-2.24976343500006,2.2,-3.55238015100001));
#322229=CARTESIAN_POINT('Ctrl Pts',(-2.24858168800006,12.2,-3.55140766300002));
#322230=CARTESIAN_POINT('Ctrl Pts',(-2.24858168800006,5.2,-3.55140766300002));
#322231=CARTESIAN_POINT('Ctrl Pts',(-2.24858168800006,2.2,-3.55140766300002));
#322232=CARTESIAN_POINT('Ctrl Pts',(-2.24740468200006,12.2,-3.55043677600001));
#322233=CARTESIAN_POINT('Ctrl Pts',(-2.24740468200006,5.2,-3.55043677600001));
#322234=CARTESIAN_POINT('Ctrl Pts',(-2.24740468200006,2.2,-3.55043677600001));
#322235=CARTESIAN_POINT('Ctrl Pts',(-2.24623242100006,12.2,-3.54946750100002));
#322236=CARTESIAN_POINT('Ctrl Pts',(-2.24623242100006,5.2,-3.54946750100002));
#322237=CARTESIAN_POINT('Ctrl Pts',(-2.24623242100006,2.2,-3.54946750100002));
#322238=CARTESIAN_POINT('Ctrl Pts',(-2.24506490200006,12.2,-3.54849985200001));
#322239=CARTESIAN_POINT('Ctrl Pts',(-2.24506490200006,5.2,-3.54849985200001));
#322240=CARTESIAN_POINT('Ctrl Pts',(-2.24506490200006,2.2,-3.54849985200001));
#322241=CARTESIAN_POINT('Ctrl Pts',(-2.24390212800006,12.2,-3.54753384500002));
#322242=CARTESIAN_POINT('Ctrl Pts',(-2.24390212800006,5.2,-3.54753384500002));
#322243=CARTESIAN_POINT('Ctrl Pts',(-2.24390212800006,2.2,-3.54753384500002));
#322244=CARTESIAN_POINT('Ctrl Pts',(-2.24274409600006,12.2,-3.54656948900002));
#322245=CARTESIAN_POINT('Ctrl Pts',(-2.24274409600006,5.2,-3.54656948900002));
#322246=CARTESIAN_POINT('Ctrl Pts',(-2.24274409600006,2.2,-3.54656948900002));
#322247=CARTESIAN_POINT('Ctrl Pts',(-2.24159080800006,12.2,-3.54560679900001));
#322248=CARTESIAN_POINT('Ctrl Pts',(-2.24159080800006,5.2,-3.54560679900001));
#322249=CARTESIAN_POINT('Ctrl Pts',(-2.24159080800006,2.2,-3.54560679900001));
#322250=CARTESIAN_POINT('Ctrl Pts',(-2.24044226300005,12.2,-3.54464578800001));
#322251=CARTESIAN_POINT('Ctrl Pts',(-2.24044226300005,5.2,-3.54464578800001));
#322252=CARTESIAN_POINT('Ctrl Pts',(-2.24044226300005,2.2,-3.54464578800001));
#322253=CARTESIAN_POINT('Ctrl Pts',(-2.23929846300006,12.2,-3.54368647200001));
#322254=CARTESIAN_POINT('Ctrl Pts',(-2.23929846300006,5.2,-3.54368647200001));
#322255=CARTESIAN_POINT('Ctrl Pts',(-2.23929846300006,2.2,-3.54368647200001));
#322256=CARTESIAN_POINT('Ctrl Pts',(-2.23815940700006,12.2,-3.54272886000001));
#322257=CARTESIAN_POINT('Ctrl Pts',(-2.23815940700006,5.2,-3.54272886000001));
#322258=CARTESIAN_POINT('Ctrl Pts',(-2.23815940700006,2.2,-3.54272886000001));
#322259=CARTESIAN_POINT('Ctrl Pts',(-2.23702509400006,12.2,-3.54177296900001));
#322260=CARTESIAN_POINT('Ctrl Pts',(-2.23702509400006,5.2,-3.54177296900001));
#322261=CARTESIAN_POINT('Ctrl Pts',(-2.23702509400006,2.2,-3.54177296900001));
#322262=CARTESIAN_POINT('Ctrl Pts',(-2.23589552500005,12.2,-3.54081881000001));
#322263=CARTESIAN_POINT('Ctrl Pts',(-2.23589552500005,5.2,-3.54081881000001));
#322264=CARTESIAN_POINT('Ctrl Pts',(-2.23589552500005,2.2,-3.54081881000001));
#322265=CARTESIAN_POINT('Ctrl Pts',(-2.23477070200006,12.2,-3.53986640000001));
#322266=CARTESIAN_POINT('Ctrl Pts',(-2.23477070200006,5.2,-3.53986640000001));
#322267=CARTESIAN_POINT('Ctrl Pts',(-2.23477070200006,2.2,-3.53986640000001));
#322268=CARTESIAN_POINT('Ctrl Pts',(-2.23365062200005,12.2,-3.53891574700001));
#322269=CARTESIAN_POINT('Ctrl Pts',(-2.23365062200005,5.2,-3.53891574700001));
#322270=CARTESIAN_POINT('Ctrl Pts',(-2.23365062200005,2.2,-3.53891574700001));
#322271=CARTESIAN_POINT('Ctrl Pts',(-2.23253528700006,12.2,-3.53796687000001));
#322272=CARTESIAN_POINT('Ctrl Pts',(-2.23253528700006,5.2,-3.53796687000001));
#322273=CARTESIAN_POINT('Ctrl Pts',(-2.23253528700006,2.2,-3.53796687000001));
#322274=CARTESIAN_POINT('Ctrl Pts',(-2.23142469500006,12.2,-3.53701978000001));
#322275=CARTESIAN_POINT('Ctrl Pts',(-2.23142469500006,5.2,-3.53701978000001));
#322276=CARTESIAN_POINT('Ctrl Pts',(-2.23142469500006,2.2,-3.53701978000001));
#322277=CARTESIAN_POINT('Ctrl Pts',(-2.23031884900006,12.2,-3.53607449000001));
#322278=CARTESIAN_POINT('Ctrl Pts',(-2.23031884900006,5.2,-3.53607449000001));
#322279=CARTESIAN_POINT('Ctrl Pts',(-2.23031884900006,2.2,-3.53607449000001));
#322280=CARTESIAN_POINT('Ctrl Pts',(-2.22921774700006,12.2,-3.53513101400001));
#322281=CARTESIAN_POINT('Ctrl Pts',(-2.22921774700006,5.2,-3.53513101400001));
#322282=CARTESIAN_POINT('Ctrl Pts',(-2.22921774700006,2.2,-3.53513101400001));
#322283=CARTESIAN_POINT('Ctrl Pts',(-2.22812138900006,12.2,-3.53418936800002));
#322284=CARTESIAN_POINT('Ctrl Pts',(-2.22812138900006,5.2,-3.53418936800002));
#322285=CARTESIAN_POINT('Ctrl Pts',(-2.22812138900006,2.2,-3.53418936800002));
#322286=CARTESIAN_POINT('Ctrl Pts',(-2.22702977400006,12.2,-3.53324956200002));
#322287=CARTESIAN_POINT('Ctrl Pts',(-2.22702977400006,5.2,-3.53324956200002));
#322288=CARTESIAN_POINT('Ctrl Pts',(-2.22702977400006,2.2,-3.53324956200002));
#322289=CARTESIAN_POINT('Ctrl Pts',(-2.22594290400006,12.2,-3.53231161200001));
#322290=CARTESIAN_POINT('Ctrl Pts',(-2.22594290400006,5.2,-3.53231161200001));
#322291=CARTESIAN_POINT('Ctrl Pts',(-2.22594290400006,2.2,-3.53231161200001));
#322292=CARTESIAN_POINT('Ctrl Pts',(-2.22486077700006,12.2,-3.53137553200002));
#322293=CARTESIAN_POINT('Ctrl Pts',(-2.22486077700006,5.2,-3.53137553200002));
#322294=CARTESIAN_POINT('Ctrl Pts',(-2.22486077700006,2.2,-3.53137553200002));
#322295=CARTESIAN_POINT('Ctrl Pts',(-2.22378339500006,12.2,-3.53044133300001));
#322296=CARTESIAN_POINT('Ctrl Pts',(-2.22378339500006,5.2,-3.53044133300001));
#322297=CARTESIAN_POINT('Ctrl Pts',(-2.22378339500006,2.2,-3.53044133300001));
#322298=CARTESIAN_POINT('Ctrl Pts',(-2.22271075500006,12.2,-3.52950903200002));
#322299=CARTESIAN_POINT('Ctrl Pts',(-2.22271075500006,5.2,-3.52950903200002));
#322300=CARTESIAN_POINT('Ctrl Pts',(-2.22271075500006,2.2,-3.52950903200002));
#322301=CARTESIAN_POINT('Ctrl Pts',(-2.22164286100006,12.2,-3.52857864200002));
#322302=CARTESIAN_POINT('Ctrl Pts',(-2.22164286100006,5.2,-3.52857864200002));
#322303=CARTESIAN_POINT('Ctrl Pts',(-2.22164286100006,2.2,-3.52857864200002));
#322304=CARTESIAN_POINT('Ctrl Pts',(-2.22057970800006,12.2,-3.52765017500001));
#322305=CARTESIAN_POINT('Ctrl Pts',(-2.22057970800006,5.2,-3.52765017500001));
#322306=CARTESIAN_POINT('Ctrl Pts',(-2.22057970800006,2.2,-3.52765017500001));
#322307=CARTESIAN_POINT('Ctrl Pts',(-2.21952129900005,12.2,-3.52672364800001));
#322308=CARTESIAN_POINT('Ctrl Pts',(-2.21952129900005,5.2,-3.52672364800001));
#322309=CARTESIAN_POINT('Ctrl Pts',(-2.21952129900005,2.2,-3.52672364800001));
#322310=CARTESIAN_POINT('Ctrl Pts',(-2.21846763300006,12.2,-3.52579907200001));
#322311=CARTESIAN_POINT('Ctrl Pts',(-2.21846763300006,5.2,-3.52579907200001));
#322312=CARTESIAN_POINT('Ctrl Pts',(-2.21846763300006,2.2,-3.52579907200001));
#322313=CARTESIAN_POINT('Ctrl Pts',(-2.21741870900006,12.2,-3.52487646300002));
#322314=CARTESIAN_POINT('Ctrl Pts',(-2.21741870900006,5.2,-3.52487646300002));
#322315=CARTESIAN_POINT('Ctrl Pts',(-2.21741870900006,2.2,-3.52487646300002));
#322316=CARTESIAN_POINT('Ctrl Pts',(-2.21637452700006,12.2,-3.52395583300002));
#322317=CARTESIAN_POINT('Ctrl Pts',(-2.21637452700006,5.2,-3.52395583300002));
#322318=CARTESIAN_POINT('Ctrl Pts',(-2.21637452700006,2.2,-3.52395583300002));
#322319=CARTESIAN_POINT('Ctrl Pts',(-2.21533508800006,12.2,-3.52303719700001));
#322320=CARTESIAN_POINT('Ctrl Pts',(-2.21533508800006,5.2,-3.52303719700001));
#322321=CARTESIAN_POINT('Ctrl Pts',(-2.21533508800006,2.2,-3.52303719700001));
#322322=CARTESIAN_POINT('Ctrl Pts',(-2.21430039000006,12.2,-3.52212056900001));
#322323=CARTESIAN_POINT('Ctrl Pts',(-2.21430039000006,5.2,-3.52212056900001));
#322324=CARTESIAN_POINT('Ctrl Pts',(-2.21430039000006,2.2,-3.52212056900001));
#322325=CARTESIAN_POINT('Ctrl Pts',(-2.21327043400006,12.2,-3.52120596400002));
#322326=CARTESIAN_POINT('Ctrl Pts',(-2.21327043400006,5.2,-3.52120596400002));
#322327=CARTESIAN_POINT('Ctrl Pts',(-2.21327043400006,2.2,-3.52120596400002));
#322328=CARTESIAN_POINT('Ctrl Pts',(-2.21224521900006,12.2,-3.52029339500001));
#322329=CARTESIAN_POINT('Ctrl Pts',(-2.21224521900006,5.2,-3.52029339500001));
#322330=CARTESIAN_POINT('Ctrl Pts',(-2.21224521900006,2.2,-3.52029339500001));
#322331=CARTESIAN_POINT('Ctrl Pts',(-2.21122474400006,12.2,-3.51938287600001));
#322332=CARTESIAN_POINT('Ctrl Pts',(-2.21122474400006,5.2,-3.51938287600001));
#322333=CARTESIAN_POINT('Ctrl Pts',(-2.21122474400006,2.2,-3.51938287600001));
#322334=CARTESIAN_POINT('Ctrl Pts',(-2.21020901100006,12.2,-3.51847442100001));
#322335=CARTESIAN_POINT('Ctrl Pts',(-2.21020901100006,5.2,-3.51847442100001));
#322336=CARTESIAN_POINT('Ctrl Pts',(-2.21020901100006,2.2,-3.51847442100001));
#322337=CARTESIAN_POINT('Ctrl Pts',(-2.20919801800005,12.2,-3.51756804500001));
#322338=CARTESIAN_POINT('Ctrl Pts',(-2.20919801800005,5.2,-3.51756804500001));
#322339=CARTESIAN_POINT('Ctrl Pts',(-2.20919801800005,2.2,-3.51756804500001));
#322340=CARTESIAN_POINT('Ctrl Pts',(-2.20819176300005,12.2,-3.51666376200002));
#322341=CARTESIAN_POINT('Ctrl Pts',(-2.20819176300005,5.2,-3.51666376200002));
#322342=CARTESIAN_POINT('Ctrl Pts',(-2.20819176300005,2.2,-3.51666376200002));
#322343=CARTESIAN_POINT('Ctrl Pts',(-2.20719024800006,12.2,-3.51576158700002));
#322344=CARTESIAN_POINT('Ctrl Pts',(-2.20719024800006,5.2,-3.51576158700002));
#322345=CARTESIAN_POINT('Ctrl Pts',(-2.20719024800006,2.2,-3.51576158700002));
#322346=CARTESIAN_POINT('Ctrl Pts',(-2.20619347100006,12.2,-3.51486153100002));
#322347=CARTESIAN_POINT('Ctrl Pts',(-2.20619347100006,5.2,-3.51486153100002));
#322348=CARTESIAN_POINT('Ctrl Pts',(-2.20619347100006,2.2,-3.51486153100002));
#322349=CARTESIAN_POINT('Ctrl Pts',(-2.20520143300006,12.2,-3.51396361200001));
#322350=CARTESIAN_POINT('Ctrl Pts',(-2.20520143300006,5.2,-3.51396361200001));
#322351=CARTESIAN_POINT('Ctrl Pts',(-2.20520143300006,2.2,-3.51396361200001));
#322352=CARTESIAN_POINT('Ctrl Pts',(-2.20421413200006,12.2,-3.51306784200001));
#322353=CARTESIAN_POINT('Ctrl Pts',(-2.20421413200006,5.2,-3.51306784200001));
#322354=CARTESIAN_POINT('Ctrl Pts',(-2.20421413200006,2.2,-3.51306784200001));
#322355=CARTESIAN_POINT('Ctrl Pts',(-2.20323156900006,12.2,-3.51217423700001));
#322356=CARTESIAN_POINT('Ctrl Pts',(-2.20323156900006,5.2,-3.51217423700001));
#322357=CARTESIAN_POINT('Ctrl Pts',(-2.20323156900006,2.2,-3.51217423700001));
#322358=CARTESIAN_POINT('Ctrl Pts',(-2.20225374200006,12.2,-3.51128281000001));
#322359=CARTESIAN_POINT('Ctrl Pts',(-2.20225374200006,5.2,-3.51128281000001));
#322360=CARTESIAN_POINT('Ctrl Pts',(-2.20225374200006,2.2,-3.51128281000001));
#322361=CARTESIAN_POINT('Ctrl Pts',(-2.20128065100006,12.2,-3.51039357700001));
#322362=CARTESIAN_POINT('Ctrl Pts',(-2.20128065100006,5.2,-3.51039357700001));
#322363=CARTESIAN_POINT('Ctrl Pts',(-2.20128065100006,2.2,-3.51039357700001));
#322364=CARTESIAN_POINT('Ctrl Pts',(-2.20031229600006,12.2,-3.50950655100001));
#322365=CARTESIAN_POINT('Ctrl Pts',(-2.20031229600006,5.2,-3.50950655100001));
#322366=CARTESIAN_POINT('Ctrl Pts',(-2.20031229600006,2.2,-3.50950655100001));
#322367=CARTESIAN_POINT('Ctrl Pts',(-2.19934867500006,12.2,-3.50862174600001));
#322368=CARTESIAN_POINT('Ctrl Pts',(-2.19934867500006,5.2,-3.50862174600001));
#322369=CARTESIAN_POINT('Ctrl Pts',(-2.19934867500006,2.2,-3.50862174600001));
#322370=CARTESIAN_POINT('Ctrl Pts',(-2.19838978900006,12.2,-3.50773917800002));
#322371=CARTESIAN_POINT('Ctrl Pts',(-2.19838978900006,5.2,-3.50773917800002));
#322372=CARTESIAN_POINT('Ctrl Pts',(-2.19838978900006,2.2,-3.50773917800002));
#322373=CARTESIAN_POINT('Ctrl Pts',(-2.19743563700006,12.2,-3.50685886100001));
#322374=CARTESIAN_POINT('Ctrl Pts',(-2.19743563700006,5.2,-3.50685886100001));
#322375=CARTESIAN_POINT('Ctrl Pts',(-2.19743563700006,2.2,-3.50685886100001));
#322376=CARTESIAN_POINT('Ctrl Pts',(-2.19648621700005,12.2,-3.50598081000001));
#322377=CARTESIAN_POINT('Ctrl Pts',(-2.19648621700005,5.2,-3.50598081000001));
#322378=CARTESIAN_POINT('Ctrl Pts',(-2.19648621700005,2.2,-3.50598081000001));
#322379=CARTESIAN_POINT('Ctrl Pts',(-2.19554153100006,12.2,-3.50510503800002));
#322380=CARTESIAN_POINT('Ctrl Pts',(-2.19554153100006,5.2,-3.50510503800002));
#322381=CARTESIAN_POINT('Ctrl Pts',(-2.19554153100006,2.2,-3.50510503800002));
#322382=CARTESIAN_POINT('Ctrl Pts',(-2.19460157600006,12.2,-3.50423156200002));
#322383=CARTESIAN_POINT('Ctrl Pts',(-2.19460157600006,5.2,-3.50423156200002));
#322384=CARTESIAN_POINT('Ctrl Pts',(-2.19460157600006,2.2,-3.50423156200002));
#322385=CARTESIAN_POINT('Ctrl Pts',(-2.19366635100006,12.2,-3.50336039400001));
#322386=CARTESIAN_POINT('Ctrl Pts',(-2.19366635100006,5.2,-3.50336039400001));
#322387=CARTESIAN_POINT('Ctrl Pts',(-2.19366635100006,2.2,-3.50336039400001));
#322388=CARTESIAN_POINT('Ctrl Pts',(-2.19273585700006,12.2,-3.50249155100002));
#322389=CARTESIAN_POINT('Ctrl Pts',(-2.19273585700006,5.2,-3.50249155100002));
#322390=CARTESIAN_POINT('Ctrl Pts',(-2.19273585700006,2.2,-3.50249155100002));
#322391=CARTESIAN_POINT('Ctrl Pts',(-2.19181009200006,12.2,-3.50162504600001));
#322392=CARTESIAN_POINT('Ctrl Pts',(-2.19181009200006,5.2,-3.50162504600001));
#322393=CARTESIAN_POINT('Ctrl Pts',(-2.19181009200006,2.2,-3.50162504600001));
#322394=CARTESIAN_POINT('Ctrl Pts',(-2.19088905600006,12.2,-3.50076089500002));
#322395=CARTESIAN_POINT('Ctrl Pts',(-2.19088905600006,5.2,-3.50076089500002));
#322396=CARTESIAN_POINT('Ctrl Pts',(-2.19088905600006,2.2,-3.50076089500002));
#322397=CARTESIAN_POINT('Ctrl Pts',(-2.18997274800006,12.2,-3.49989911300002));
#322398=CARTESIAN_POINT('Ctrl Pts',(-2.18997274800006,5.2,-3.49989911300002));
#322399=CARTESIAN_POINT('Ctrl Pts',(-2.18997274800006,2.2,-3.49989911300002));
#322400=CARTESIAN_POINT('Ctrl Pts',(-2.18906116700006,12.2,-3.49903971300002));
#322401=CARTESIAN_POINT('Ctrl Pts',(-2.18906116700006,5.2,-3.49903971300002));
#322402=CARTESIAN_POINT('Ctrl Pts',(-2.18906116700006,2.2,-3.49903971300002));
#322403=CARTESIAN_POINT('Ctrl Pts',(-2.18815431200006,12.2,-3.49818271100002));
#322404=CARTESIAN_POINT('Ctrl Pts',(-2.18815431200006,5.2,-3.49818271100002));
#322405=CARTESIAN_POINT('Ctrl Pts',(-2.18815431200006,2.2,-3.49818271100002));
#322406=CARTESIAN_POINT('Ctrl Pts',(-2.18725218200006,12.2,-3.49732812300001));
#322407=CARTESIAN_POINT('Ctrl Pts',(-2.18725218200006,5.2,-3.49732812300001));
#322408=CARTESIAN_POINT('Ctrl Pts',(-2.18725218200006,2.2,-3.49732812300001));
#322409=CARTESIAN_POINT('Ctrl Pts',(-2.18635477700006,12.2,-3.49647596200001));
#322410=CARTESIAN_POINT('Ctrl Pts',(-2.18635477700006,5.2,-3.49647596200001));
#322411=CARTESIAN_POINT('Ctrl Pts',(-2.18635477700006,2.2,-3.49647596200001));
#322412=CARTESIAN_POINT('Ctrl Pts',(-2.18546209500006,12.2,-3.49562624400001));
#322413=CARTESIAN_POINT('Ctrl Pts',(-2.18546209500006,5.2,-3.49562624400001));
#322414=CARTESIAN_POINT('Ctrl Pts',(-2.18546209500006,2.2,-3.49562624400001));
#322415=CARTESIAN_POINT('Ctrl Pts',(-2.18457413600006,12.2,-3.49477898400002));
#322416=CARTESIAN_POINT('Ctrl Pts',(-2.18457413600006,5.2,-3.49477898400002));
#322417=CARTESIAN_POINT('Ctrl Pts',(-2.18457413600006,2.2,-3.49477898400002));
#322418=CARTESIAN_POINT('Ctrl Pts',(-2.18369089900006,12.2,-3.49393419600001));
#322419=CARTESIAN_POINT('Ctrl Pts',(-2.18369089900006,5.2,-3.49393419600001));
#322420=CARTESIAN_POINT('Ctrl Pts',(-2.18369089900006,2.2,-3.49393419600001));
#322421=CARTESIAN_POINT('Ctrl Pts',(-2.18281238100006,12.2,-3.49309189600001));
#322422=CARTESIAN_POINT('Ctrl Pts',(-2.18281238100006,5.2,-3.49309189600001));
#322423=CARTESIAN_POINT('Ctrl Pts',(-2.18281238100006,2.2,-3.49309189600001));
#322424=CARTESIAN_POINT('Ctrl Pts',(-2.18193858400006,12.2,-3.49225209900001));
#322425=CARTESIAN_POINT('Ctrl Pts',(-2.18193858400006,5.2,-3.49225209900001));
#322426=CARTESIAN_POINT('Ctrl Pts',(-2.18193858400006,2.2,-3.49225209900001));
#322427=CARTESIAN_POINT('Ctrl Pts',(-2.18106950600006,12.2,-3.49141482000002));
#322428=CARTESIAN_POINT('Ctrl Pts',(-2.18106950600006,5.2,-3.49141482000002));
#322429=CARTESIAN_POINT('Ctrl Pts',(-2.18106950600006,2.2,-3.49141482000002));
#322430=CARTESIAN_POINT('Ctrl Pts',(-2.18020514400005,12.2,-3.49058007400001));
#322431=CARTESIAN_POINT('Ctrl Pts',(-2.18020514400005,5.2,-3.49058007400001));
#322432=CARTESIAN_POINT('Ctrl Pts',(-2.18020514400005,2.2,-3.49058007400001));
#322433=CARTESIAN_POINT('Ctrl Pts',(-2.17934550000006,12.2,-3.48974787600001));
#322434=CARTESIAN_POINT('Ctrl Pts',(-2.17934550000006,5.2,-3.48974787600001));
#322435=CARTESIAN_POINT('Ctrl Pts',(-2.17934550000006,2.2,-3.48974787600001));
#322436=CARTESIAN_POINT('Ctrl Pts',(-2.17849057100006,12.2,-3.48891824200001));
#322437=CARTESIAN_POINT('Ctrl Pts',(-2.17849057100006,5.2,-3.48891824200001));
#322438=CARTESIAN_POINT('Ctrl Pts',(-2.17849057100006,2.2,-3.48891824200001));
#322439=CARTESIAN_POINT('Ctrl Pts',(-2.17764035600006,12.2,-3.48809118700002));
#322440=CARTESIAN_POINT('Ctrl Pts',(-2.17764035600006,5.2,-3.48809118700002));
#322441=CARTESIAN_POINT('Ctrl Pts',(-2.17764035600006,2.2,-3.48809118700002));
#322442=CARTESIAN_POINT('Ctrl Pts',(-2.17679485500006,12.2,-3.48726672600002));
#322443=CARTESIAN_POINT('Ctrl Pts',(-2.17679485500006,5.2,-3.48726672600002));
#322444=CARTESIAN_POINT('Ctrl Pts',(-2.17679485500006,2.2,-3.48726672600002));
#322445=CARTESIAN_POINT('Ctrl Pts',(-2.17595406600006,12.2,-3.48644487300001));
#322446=CARTESIAN_POINT('Ctrl Pts',(-2.17595406600006,5.2,-3.48644487300001));
#322447=CARTESIAN_POINT('Ctrl Pts',(-2.17595406600006,2.2,-3.48644487300001));
#322448=CARTESIAN_POINT('Ctrl Pts',(-2.17511798700006,12.2,-3.48562564600002));
#322449=CARTESIAN_POINT('Ctrl Pts',(-2.17511798700006,5.2,-3.48562564600002));
#322450=CARTESIAN_POINT('Ctrl Pts',(-2.17511798700006,2.2,-3.48562564600002));
#322451=CARTESIAN_POINT('Ctrl Pts',(-2.17428661800006,12.2,-3.48480905900002));
#322452=CARTESIAN_POINT('Ctrl Pts',(-2.17428661800006,5.2,-3.48480905900002));
#322453=CARTESIAN_POINT('Ctrl Pts',(-2.17428661800006,2.2,-3.48480905900002));
#322454=CARTESIAN_POINT('Ctrl Pts',(-2.17345995800006,12.2,-3.48399512700002));
#322455=CARTESIAN_POINT('Ctrl Pts',(-2.17345995800006,5.2,-3.48399512700002));
#322456=CARTESIAN_POINT('Ctrl Pts',(-2.17345995800006,2.2,-3.48399512700002));
#322457=CARTESIAN_POINT('Ctrl Pts',(-2.17263800500006,12.2,-3.48318386600001));
#322458=CARTESIAN_POINT('Ctrl Pts',(-2.17263800500006,5.2,-3.48318386600001));
#322459=CARTESIAN_POINT('Ctrl Pts',(-2.17263800500006,2.2,-3.48318386600001));
#322460=CARTESIAN_POINT('Ctrl Pts',(-2.17182075800006,12.2,-3.48237529200001));
#322461=CARTESIAN_POINT('Ctrl Pts',(-2.17182075800006,5.2,-3.48237529200001));
#322462=CARTESIAN_POINT('Ctrl Pts',(-2.17182075800006,2.2,-3.48237529200001));
#322463=CARTESIAN_POINT('Ctrl Pts',(-2.17100821500006,12.2,-3.48156941900001));
#322464=CARTESIAN_POINT('Ctrl Pts',(-2.17100821500006,5.2,-3.48156941900001));
#322465=CARTESIAN_POINT('Ctrl Pts',(-2.17100821500006,2.2,-3.48156941900001));
#322466=CARTESIAN_POINT('Ctrl Pts',(-2.17020037600005,12.2,-3.48076626400001));
#322467=CARTESIAN_POINT('Ctrl Pts',(-2.17020037600005,5.2,-3.48076626400001));
#322468=CARTESIAN_POINT('Ctrl Pts',(-2.17020037600005,2.2,-3.48076626400001));
#322469=CARTESIAN_POINT('Ctrl Pts',(-2.16939723900006,12.2,-3.47996584200001));
#322470=CARTESIAN_POINT('Ctrl Pts',(-2.16939723900006,5.2,-3.47996584200001));
#322471=CARTESIAN_POINT('Ctrl Pts',(-2.16939723900006,2.2,-3.47996584200001));
#322472=CARTESIAN_POINT('Ctrl Pts',(-2.16859880300006,12.2,-3.47916816900002));
#322473=CARTESIAN_POINT('Ctrl Pts',(-2.16859880300006,5.2,-3.47916816900002));
#322474=CARTESIAN_POINT('Ctrl Pts',(-2.16859880300006,2.2,-3.47916816900002));
#322475=CARTESIAN_POINT('Ctrl Pts',(-2.16780506500006,12.2,-3.47837326000001));
#322476=CARTESIAN_POINT('Ctrl Pts',(-2.16780506500006,5.2,-3.47837326000001));
#322477=CARTESIAN_POINT('Ctrl Pts',(-2.16780506500006,2.2,-3.47837326000001));
#322478=CARTESIAN_POINT('Ctrl Pts',(-2.16701602600006,12.2,-3.47758113100001));
#322479=CARTESIAN_POINT('Ctrl Pts',(-2.16701602600006,5.2,-3.47758113100001));
#322480=CARTESIAN_POINT('Ctrl Pts',(-2.16701602600006,2.2,-3.47758113100001));
#322481=CARTESIAN_POINT('Ctrl Pts',(-2.16623168300006,12.2,-3.47679179900001));
#322482=CARTESIAN_POINT('Ctrl Pts',(-2.16623168300006,5.2,-3.47679179900001));
#322483=CARTESIAN_POINT('Ctrl Pts',(-2.16623168300006,2.2,-3.47679179900001));
#322484=CARTESIAN_POINT('Ctrl Pts',(-2.16545203600006,12.2,-3.47600527800001));
#322485=CARTESIAN_POINT('Ctrl Pts',(-2.16545203600006,5.2,-3.47600527800001));
#322486=CARTESIAN_POINT('Ctrl Pts',(-2.16545203600006,2.2,-3.47600527800001));
#322487=CARTESIAN_POINT('Ctrl Pts',(-2.16467708200006,12.2,-3.47522158300002));
#322488=CARTESIAN_POINT('Ctrl Pts',(-2.16467708200006,5.2,-3.47522158300002));
#322489=CARTESIAN_POINT('Ctrl Pts',(-2.16467708200006,2.2,-3.47522158300002));
#322490=CARTESIAN_POINT('Ctrl Pts',(-2.16390682000006,12.2,-3.47444073300001));
#322491=CARTESIAN_POINT('Ctrl Pts',(-2.16390682000006,5.2,-3.47444073300001));
#322492=CARTESIAN_POINT('Ctrl Pts',(-2.16390682000006,2.2,-3.47444073300001));
#322493=CARTESIAN_POINT('Ctrl Pts',(-2.16314124800005,12.2,-3.47366274100001));
#322494=CARTESIAN_POINT('Ctrl Pts',(-2.16314124800005,5.2,-3.47366274100001));
#322495=CARTESIAN_POINT('Ctrl Pts',(-2.16314124800005,2.2,-3.47366274100001));
#322496=CARTESIAN_POINT('Ctrl Pts',(-2.16238036500005,12.2,-3.47288762500002));
#322497=CARTESIAN_POINT('Ctrl Pts',(-2.16238036500005,5.2,-3.47288762500002));
#322498=CARTESIAN_POINT('Ctrl Pts',(-2.16238036500005,2.2,-3.47288762500002));
#322499=CARTESIAN_POINT('Ctrl Pts',(-2.16162417000006,12.2,-3.47211539900002));
#322500=CARTESIAN_POINT('Ctrl Pts',(-2.16162417000006,5.2,-3.47211539900002));
#322501=CARTESIAN_POINT('Ctrl Pts',(-2.16162417000006,2.2,-3.47211539900002));
#322502=CARTESIAN_POINT('Ctrl Pts',(-2.16087266000006,12.2,-3.47134608100002));
#322503=CARTESIAN_POINT('Ctrl Pts',(-2.16087266000006,5.2,-3.47134608100002));
#322504=CARTESIAN_POINT('Ctrl Pts',(-2.16087266000006,2.2,-3.47134608100002));
#322505=CARTESIAN_POINT('Ctrl Pts',(-2.16012583500006,12.2,-3.47057968500001));
#322506=CARTESIAN_POINT('Ctrl Pts',(-2.16012583500006,5.2,-3.47057968500001));
#322507=CARTESIAN_POINT('Ctrl Pts',(-2.16012583500006,2.2,-3.47057968500001));
#322508=CARTESIAN_POINT('Ctrl Pts',(-2.15938369100006,12.2,-3.46981622800001));
#322509=CARTESIAN_POINT('Ctrl Pts',(-2.15938369100006,5.2,-3.46981622800001));
#322510=CARTESIAN_POINT('Ctrl Pts',(-2.15938369100006,2.2,-3.46981622800001));
#322511=CARTESIAN_POINT('Ctrl Pts',(-2.15864623000006,12.2,-3.46905572800001));
#322512=CARTESIAN_POINT('Ctrl Pts',(-2.15864623000006,5.2,-3.46905572800001));
#322513=CARTESIAN_POINT('Ctrl Pts',(-2.15864623000006,2.2,-3.46905572800001));
#322514=CARTESIAN_POINT('Ctrl Pts',(-2.15791344700006,12.2,-3.46829819800002));
#322515=CARTESIAN_POINT('Ctrl Pts',(-2.15791344700006,5.2,-3.46829819800002));
#322516=CARTESIAN_POINT('Ctrl Pts',(-2.15791344700006,2.2,-3.46829819800002));
#322517=CARTESIAN_POINT('Ctrl Pts',(-2.15718534100006,12.2,-3.46754365400002));
#322518=CARTESIAN_POINT('Ctrl Pts',(-2.15718534100006,5.2,-3.46754365400002));
#322519=CARTESIAN_POINT('Ctrl Pts',(-2.15718534100006,2.2,-3.46754365400002));
#322520=CARTESIAN_POINT('Ctrl Pts',(-2.15646191100006,12.2,-3.46679211500001));
#322521=CARTESIAN_POINT('Ctrl Pts',(-2.15646191100006,5.2,-3.46679211500001));
#322522=CARTESIAN_POINT('Ctrl Pts',(-2.15646191100006,2.2,-3.46679211500001));
#322523=CARTESIAN_POINT('Ctrl Pts',(-2.15574315500006,12.2,-3.46604359700001));
#322524=CARTESIAN_POINT('Ctrl Pts',(-2.15574315500006,5.2,-3.46604359700001));
#322525=CARTESIAN_POINT('Ctrl Pts',(-2.15574315500006,2.2,-3.46604359700001));
#322526=CARTESIAN_POINT('Ctrl Pts',(-2.15502907200006,12.2,-3.46529811400002));
#322527=CARTESIAN_POINT('Ctrl Pts',(-2.15502907200006,5.2,-3.46529811400002));
#322528=CARTESIAN_POINT('Ctrl Pts',(-2.15502907200006,2.2,-3.46529811400002));
#322529=CARTESIAN_POINT('Ctrl Pts',(-2.15431965800006,12.2,-3.46455568300001));
#322530=CARTESIAN_POINT('Ctrl Pts',(-2.15431965800006,5.2,-3.46455568300001));
#322531=CARTESIAN_POINT('Ctrl Pts',(-2.15431965800006,2.2,-3.46455568300001));
#322532=CARTESIAN_POINT('Ctrl Pts',(-2.15361491300006,12.2,-3.46381632200002));
#322533=CARTESIAN_POINT('Ctrl Pts',(-2.15361491300006,5.2,-3.46381632200002));
#322534=CARTESIAN_POINT('Ctrl Pts',(-2.15361491300006,2.2,-3.46381632200002));
#322535=CARTESIAN_POINT('Ctrl Pts',(-2.15291483500006,12.2,-3.46308004600001));
#322536=CARTESIAN_POINT('Ctrl Pts',(-2.15291483500006,5.2,-3.46308004600001));
#322537=CARTESIAN_POINT('Ctrl Pts',(-2.15291483500006,2.2,-3.46308004600001));
#322538=CARTESIAN_POINT('Ctrl Pts',(-2.15221942100006,12.2,-3.46234687200001));
#322539=CARTESIAN_POINT('Ctrl Pts',(-2.15221942100006,5.2,-3.46234687200001));
#322540=CARTESIAN_POINT('Ctrl Pts',(-2.15221942100006,2.2,-3.46234687200001));
#322541=CARTESIAN_POINT('Ctrl Pts',(-2.15152867000006,12.2,-3.46161681600002));
#322542=CARTESIAN_POINT('Ctrl Pts',(-2.15152867000006,5.2,-3.46161681600002));
#322543=CARTESIAN_POINT('Ctrl Pts',(-2.15152867000006,2.2,-3.46161681600002));
#322544=CARTESIAN_POINT('Ctrl Pts',(-2.15084257900005,12.2,-3.46088989500001));
#322545=CARTESIAN_POINT('Ctrl Pts',(-2.15084257900005,5.2,-3.46088989500001));
#322546=CARTESIAN_POINT('Ctrl Pts',(-2.15084257900005,2.2,-3.46088989500001));
#322547=CARTESIAN_POINT('Ctrl Pts',(-2.15016114900005,12.2,-3.46016612500001));
#322548=CARTESIAN_POINT('Ctrl Pts',(-2.15016114900005,5.2,-3.46016612500001));
#322549=CARTESIAN_POINT('Ctrl Pts',(-2.15016114900005,2.2,-3.46016612500001));
#322550=CARTESIAN_POINT('Ctrl Pts',(-2.14948437400006,12.2,-3.45944552300002));
#322551=CARTESIAN_POINT('Ctrl Pts',(-2.14948437400006,5.2,-3.45944552300002));
#322552=CARTESIAN_POINT('Ctrl Pts',(-2.14948437400006,2.2,-3.45944552300002));
#322553=CARTESIAN_POINT('Ctrl Pts',(-2.14881225400006,12.2,-3.45872810500001));
#322554=CARTESIAN_POINT('Ctrl Pts',(-2.14881225400006,5.2,-3.45872810500001));
#322555=CARTESIAN_POINT('Ctrl Pts',(-2.14881225400006,2.2,-3.45872810500001));
#322556=CARTESIAN_POINT('Ctrl Pts',(-2.14814478800006,12.2,-3.45801388900002));
#322557=CARTESIAN_POINT('Ctrl Pts',(-2.14814478800006,5.2,-3.45801388900002));
#322558=CARTESIAN_POINT('Ctrl Pts',(-2.14814478800006,2.2,-3.45801388900002));
#322559=CARTESIAN_POINT('Ctrl Pts',(-2.14748197100006,12.2,-3.45730289000001));
#322560=CARTESIAN_POINT('Ctrl Pts',(-2.14748197100006,5.2,-3.45730289000001));
#322561=CARTESIAN_POINT('Ctrl Pts',(-2.14748197100006,2.2,-3.45730289000001));
#322562=CARTESIAN_POINT('Ctrl Pts',(-2.14682380300005,12.2,-3.45659512600001));
#322563=CARTESIAN_POINT('Ctrl Pts',(-2.14682380300005,5.2,-3.45659512600001));
#322564=CARTESIAN_POINT('Ctrl Pts',(-2.14682380300005,2.2,-3.45659512600001));
#322565=CARTESIAN_POINT('Ctrl Pts',(-2.14617028200006,12.2,-3.45589061500001));
#322566=CARTESIAN_POINT('Ctrl Pts',(-2.14617028200006,5.2,-3.45589061500001));
#322567=CARTESIAN_POINT('Ctrl Pts',(-2.14617028200006,2.2,-3.45589061500001));
#322568=CARTESIAN_POINT('Ctrl Pts',(-2.14552140400006,12.2,-3.45518937000001));
#322569=CARTESIAN_POINT('Ctrl Pts',(-2.14552140400006,5.2,-3.45518937000001));
#322570=CARTESIAN_POINT('Ctrl Pts',(-2.14552140400006,2.2,-3.45518937000001));
#322571=CARTESIAN_POINT('Ctrl Pts',(-2.14487717000006,12.2,-3.45449141200001));
#322572=CARTESIAN_POINT('Ctrl Pts',(-2.14487717000006,5.2,-3.45449141200001));
#322573=CARTESIAN_POINT('Ctrl Pts',(-2.14487717000006,2.2,-3.45449141200001));
#322574=CARTESIAN_POINT('Ctrl Pts',(-2.14423757400006,12.2,-3.45379675600002));
#322575=CARTESIAN_POINT('Ctrl Pts',(-2.14423757400006,5.2,-3.45379675600002));
#322576=CARTESIAN_POINT('Ctrl Pts',(-2.14423757400006,2.2,-3.45379675600002));
#322577=CARTESIAN_POINT('Ctrl Pts',(-2.14360261700006,12.2,-3.45310541800002));
#322578=CARTESIAN_POINT('Ctrl Pts',(-2.14360261700006,5.2,-3.45310541800002));
#322579=CARTESIAN_POINT('Ctrl Pts',(-2.14360261700006,2.2,-3.45310541800002));
#322580=CARTESIAN_POINT('Ctrl Pts',(-2.14297229500006,12.2,-3.45241741600002));
#322581=CARTESIAN_POINT('Ctrl Pts',(-2.14297229500006,5.2,-3.45241741600002));
#322582=CARTESIAN_POINT('Ctrl Pts',(-2.14297229500006,2.2,-3.45241741600002));
#322583=CARTESIAN_POINT('Ctrl Pts',(-2.14234660600006,12.2,-3.45173276800002));
#322584=CARTESIAN_POINT('Ctrl Pts',(-2.14234660600006,5.2,-3.45173276800002));
#322585=CARTESIAN_POINT('Ctrl Pts',(-2.14234660600006,2.2,-3.45173276800002));
#322586=CARTESIAN_POINT('Ctrl Pts',(-2.14172554800005,12.2,-3.45105149000001));
#322587=CARTESIAN_POINT('Ctrl Pts',(-2.14172554800005,5.2,-3.45105149000001));
#322588=CARTESIAN_POINT('Ctrl Pts',(-2.14172554800005,2.2,-3.45105149000001));
#322589=CARTESIAN_POINT('Ctrl Pts',(-2.14110911800006,12.2,-3.45037359900001));
#322590=CARTESIAN_POINT('Ctrl Pts',(-2.14110911800006,5.2,-3.45037359900001));
#322591=CARTESIAN_POINT('Ctrl Pts',(-2.14110911800006,2.2,-3.45037359900001));
#322592=CARTESIAN_POINT('Ctrl Pts',(-2.14049731400006,12.2,-3.44969911300002));
#322593=CARTESIAN_POINT('Ctrl Pts',(-2.14049731400006,5.2,-3.44969911300002));
#322594=CARTESIAN_POINT('Ctrl Pts',(-2.14049731400006,2.2,-3.44969911300002));
#322595=CARTESIAN_POINT('Ctrl Pts',(-2.13989013300006,12.2,-3.44902804800002));
#322596=CARTESIAN_POINT('Ctrl Pts',(-2.13989013300006,5.2,-3.44902804800002));
#322597=CARTESIAN_POINT('Ctrl Pts',(-2.13989013300006,2.2,-3.44902804800002));
#322598=CARTESIAN_POINT('Ctrl Pts',(-2.13928757500006,12.2,-3.44836042300001));
#322599=CARTESIAN_POINT('Ctrl Pts',(-2.13928757500006,5.2,-3.44836042300001));
#322600=CARTESIAN_POINT('Ctrl Pts',(-2.13928757500006,2.2,-3.44836042300001));
#322601=CARTESIAN_POINT('Ctrl Pts',(-2.13868963400006,12.2,-3.44769625300001));
#322602=CARTESIAN_POINT('Ctrl Pts',(-2.13868963400006,5.2,-3.44769625300001));
#322603=CARTESIAN_POINT('Ctrl Pts',(-2.13868963400006,2.2,-3.44769625300001));
#322604=CARTESIAN_POINT('Ctrl Pts',(-2.13809631100006,12.2,-3.44703555800002));
#322605=CARTESIAN_POINT('Ctrl Pts',(-2.13809631100006,5.2,-3.44703555800002));
#322606=CARTESIAN_POINT('Ctrl Pts',(-2.13809631100006,2.2,-3.44703555800002));
#322607=CARTESIAN_POINT('Ctrl Pts',(-2.13750760000006,12.2,-3.44637835300002));
#322608=CARTESIAN_POINT('Ctrl Pts',(-2.13750760000006,5.2,-3.44637835300002));
#322609=CARTESIAN_POINT('Ctrl Pts',(-2.13750760000006,2.2,-3.44637835300002));
#322610=CARTESIAN_POINT('Ctrl Pts',(-2.13692350100006,12.2,-3.44572465600002));
#322611=CARTESIAN_POINT('Ctrl Pts',(-2.13692350100006,5.2,-3.44572465600002));
#322612=CARTESIAN_POINT('Ctrl Pts',(-2.13692350100006,2.2,-3.44572465600002));
#322613=CARTESIAN_POINT('Ctrl Pts',(-2.13634401000005,12.2,-3.44507448500002));
#322614=CARTESIAN_POINT('Ctrl Pts',(-2.13634401000005,5.2,-3.44507448500002));
#322615=CARTESIAN_POINT('Ctrl Pts',(-2.13634401000005,2.2,-3.44507448500002));
#322616=CARTESIAN_POINT('Ctrl Pts',(-2.13576912600006,12.2,-3.44442785800001));
#322617=CARTESIAN_POINT('Ctrl Pts',(-2.13576912600006,5.2,-3.44442785800001));
#322618=CARTESIAN_POINT('Ctrl Pts',(-2.13576912600006,2.2,-3.44442785800001));
#322619=CARTESIAN_POINT('Ctrl Pts',(-2.13519884400006,12.2,-3.44378479200001));
#322620=CARTESIAN_POINT('Ctrl Pts',(-2.13519884400006,5.2,-3.44378479200001));
#322621=CARTESIAN_POINT('Ctrl Pts',(-2.13519884400006,2.2,-3.44378479200001));
#322622=CARTESIAN_POINT('Ctrl Pts',(-2.13463316400006,12.2,-3.44314530400001));
#322623=CARTESIAN_POINT('Ctrl Pts',(-2.13463316400006,5.2,-3.44314530400001));
#322624=CARTESIAN_POINT('Ctrl Pts',(-2.13463316400006,2.2,-3.44314530400001));
#322625=CARTESIAN_POINT('Ctrl Pts',(-2.13407208100006,12.2,-3.44250941200002));
#322626=CARTESIAN_POINT('Ctrl Pts',(-2.13407208100006,5.2,-3.44250941200002));
#322627=CARTESIAN_POINT('Ctrl Pts',(-2.13407208100006,2.2,-3.44250941200002));
#322628=CARTESIAN_POINT('Ctrl Pts',(-2.13351559300006,12.2,-3.44187713400002));
#322629=CARTESIAN_POINT('Ctrl Pts',(-2.13351559300006,5.2,-3.44187713400002));
#322630=CARTESIAN_POINT('Ctrl Pts',(-2.13351559300006,2.2,-3.44187713400002));
#322631=CARTESIAN_POINT('Ctrl Pts',(-2.13296369900006,12.2,-3.44124848800002));
#322632=CARTESIAN_POINT('Ctrl Pts',(-2.13296369900006,5.2,-3.44124848800002));
#322633=CARTESIAN_POINT('Ctrl Pts',(-2.13296369900006,2.2,-3.44124848800002));
#322634=CARTESIAN_POINT('Ctrl Pts',(-2.13241639400006,12.2,-3.44062349100001));
#322635=CARTESIAN_POINT('Ctrl Pts',(-2.13241639400006,5.2,-3.44062349100001));
#322636=CARTESIAN_POINT('Ctrl Pts',(-2.13241639400006,2.2,-3.44062349100001));
#322637=CARTESIAN_POINT('Ctrl Pts',(-2.13187367600006,12.2,-3.44000216100001));
#322638=CARTESIAN_POINT('Ctrl Pts',(-2.13187367600006,5.2,-3.44000216100001));
#322639=CARTESIAN_POINT('Ctrl Pts',(-2.13187367600006,2.2,-3.44000216100001));
#322640=CARTESIAN_POINT('Ctrl Pts',(-2.13133554200006,12.2,-3.43938451500001));
#322641=CARTESIAN_POINT('Ctrl Pts',(-2.13133554200006,5.2,-3.43938451500001));
#322642=CARTESIAN_POINT('Ctrl Pts',(-2.13133554200006,2.2,-3.43938451500001));
#322643=CARTESIAN_POINT('Ctrl Pts',(-2.13080198900006,12.2,-3.43877057300002));
#322644=CARTESIAN_POINT('Ctrl Pts',(-2.13080198900006,5.2,-3.43877057300002));
#322645=CARTESIAN_POINT('Ctrl Pts',(-2.13080198900006,2.2,-3.43877057300002));
#322646=CARTESIAN_POINT('Ctrl Pts',(-2.13027301500006,12.2,-3.43816035200001));
#322647=CARTESIAN_POINT('Ctrl Pts',(-2.13027301500006,5.2,-3.43816035200001));
#322648=CARTESIAN_POINT('Ctrl Pts',(-2.13027301500006,2.2,-3.43816035200001));
#322649=CARTESIAN_POINT('Ctrl Pts',(-2.12974861500005,12.2,-3.43755386900002));
#322650=CARTESIAN_POINT('Ctrl Pts',(-2.12974861500005,5.2,-3.43755386900002));
#322651=CARTESIAN_POINT('Ctrl Pts',(-2.12974861500005,2.2,-3.43755386900002));
#322652=CARTESIAN_POINT('Ctrl Pts',(-2.12922878900006,12.2,-3.43695114400001));
#322653=CARTESIAN_POINT('Ctrl Pts',(-2.12922878900006,5.2,-3.43695114400001));
#322654=CARTESIAN_POINT('Ctrl Pts',(-2.12922878900006,2.2,-3.43695114400001));
#322655=CARTESIAN_POINT('Ctrl Pts',(-2.12871353300006,12.2,-3.43635219300001));
#322656=CARTESIAN_POINT('Ctrl Pts',(-2.12871353300006,5.2,-3.43635219300001));
#322657=CARTESIAN_POINT('Ctrl Pts',(-2.12871353300006,2.2,-3.43635219300001));
#322658=CARTESIAN_POINT('Ctrl Pts',(-2.12820284200005,12.2,-3.43575703600001));
#322659=CARTESIAN_POINT('Ctrl Pts',(-2.12820284200005,5.2,-3.43575703600001));
#322660=CARTESIAN_POINT('Ctrl Pts',(-2.12820284200005,2.2,-3.43575703600001));
#322661=CARTESIAN_POINT('Ctrl Pts',(-2.12769671400005,12.2,-3.43516569000001));
#322662=CARTESIAN_POINT('Ctrl Pts',(-2.12769671400005,5.2,-3.43516569000001));
#322663=CARTESIAN_POINT('Ctrl Pts',(-2.12769671400005,2.2,-3.43516569000001));
#322664=CARTESIAN_POINT('Ctrl Pts',(-2.12719514700006,12.2,-3.43457817300001));
#322665=CARTESIAN_POINT('Ctrl Pts',(-2.12719514700006,5.2,-3.43457817300001));
#322666=CARTESIAN_POINT('Ctrl Pts',(-2.12719514700006,2.2,-3.43457817300001));
#322667=CARTESIAN_POINT('Ctrl Pts',(-2.12669813800006,12.2,-3.43399450400002));
#322668=CARTESIAN_POINT('Ctrl Pts',(-2.12669813800006,5.2,-3.43399450400002));
#322669=CARTESIAN_POINT('Ctrl Pts',(-2.12669813800006,2.2,-3.43399450400002));
#322670=CARTESIAN_POINT('Ctrl Pts',(-2.12620568200005,12.2,-3.43341470100002));
#322671=CARTESIAN_POINT('Ctrl Pts',(-2.12620568200005,5.2,-3.43341470100002));
#322672=CARTESIAN_POINT('Ctrl Pts',(-2.12620568200005,2.2,-3.43341470100002));
#322673=CARTESIAN_POINT('Ctrl Pts',(-2.12571777800005,12.2,-3.43283878300001));
#322674=CARTESIAN_POINT('Ctrl Pts',(-2.12571777800005,5.2,-3.43283878300001));
#322675=CARTESIAN_POINT('Ctrl Pts',(-2.12571777800005,2.2,-3.43283878300001));
#322676=CARTESIAN_POINT('Ctrl Pts',(-2.12523442100006,12.2,-3.43226676700001));
#322677=CARTESIAN_POINT('Ctrl Pts',(-2.12523442100006,5.2,-3.43226676700001));
#322678=CARTESIAN_POINT('Ctrl Pts',(-2.12523442100006,2.2,-3.43226676700001));
#322679=CARTESIAN_POINT('Ctrl Pts',(-2.12475560800006,12.2,-3.43169867300002));
#322680=CARTESIAN_POINT('Ctrl Pts',(-2.12475560800006,5.2,-3.43169867300002));
#322681=CARTESIAN_POINT('Ctrl Pts',(-2.12475560800006,2.2,-3.43169867300002));
#322682=CARTESIAN_POINT('Ctrl Pts',(-2.12428133600006,12.2,-3.43113451900001));
#322683=CARTESIAN_POINT('Ctrl Pts',(-2.12428133600006,5.2,-3.43113451900001));
#322684=CARTESIAN_POINT('Ctrl Pts',(-2.12428133600006,2.2,-3.43113451900001));
#322685=CARTESIAN_POINT('Ctrl Pts',(-2.12381160300006,12.2,-3.43057432300002));
#322686=CARTESIAN_POINT('Ctrl Pts',(-2.12381160300006,5.2,-3.43057432300002));
#322687=CARTESIAN_POINT('Ctrl Pts',(-2.12381160300006,2.2,-3.43057432300002));
#322688=CARTESIAN_POINT('Ctrl Pts',(-2.12334640400006,12.2,-3.43001810500001));
#322689=CARTESIAN_POINT('Ctrl Pts',(-2.12334640400006,5.2,-3.43001810500001));
#322690=CARTESIAN_POINT('Ctrl Pts',(-2.12334640400006,2.2,-3.43001810500001));
#322691=CARTESIAN_POINT('Ctrl Pts',(-2.12288573600006,12.2,-3.42946588200002));
#322692=CARTESIAN_POINT('Ctrl Pts',(-2.12288573600006,5.2,-3.42946588200002));
#322693=CARTESIAN_POINT('Ctrl Pts',(-2.12288573600006,2.2,-3.42946588200002));
#322694=CARTESIAN_POINT('Ctrl Pts',(-2.12242959500006,12.2,-3.42891767300001));
#322695=CARTESIAN_POINT('Ctrl Pts',(-2.12242959500006,5.2,-3.42891767300001));
#322696=CARTESIAN_POINT('Ctrl Pts',(-2.12242959500006,2.2,-3.42891767300001));
#322697=CARTESIAN_POINT('Ctrl Pts',(-2.12197798100005,12.2,-3.42837349800002));
#322698=CARTESIAN_POINT('Ctrl Pts',(-2.12197798100005,5.2,-3.42837349800002));
#322699=CARTESIAN_POINT('Ctrl Pts',(-2.12197798100005,2.2,-3.42837349800002));
#322700=CARTESIAN_POINT('Ctrl Pts',(-2.12153088600005,12.2,-3.42783337400002));
#322701=CARTESIAN_POINT('Ctrl Pts',(-2.12153088600005,5.2,-3.42783337400002));
#322702=CARTESIAN_POINT('Ctrl Pts',(-2.12153088600005,2.2,-3.42783337400002));
#322703=CARTESIAN_POINT('Ctrl Pts',(-2.12108830800006,12.2,-3.42729732200001));
#322704=CARTESIAN_POINT('Ctrl Pts',(-2.12108830800006,5.2,-3.42729732200001));
#322705=CARTESIAN_POINT('Ctrl Pts',(-2.12108830800006,2.2,-3.42729732200001));
#322706=CARTESIAN_POINT('Ctrl Pts',(-2.12065024400005,12.2,-3.42676535900001));
#322707=CARTESIAN_POINT('Ctrl Pts',(-2.12065024400005,5.2,-3.42676535900001));
#322708=CARTESIAN_POINT('Ctrl Pts',(-2.12065024400005,2.2,-3.42676535900001));
#322709=CARTESIAN_POINT('Ctrl Pts',(-2.12021669100006,12.2,-3.42623750400001));
#322710=CARTESIAN_POINT('Ctrl Pts',(-2.12021669100006,5.2,-3.42623750400001));
#322711=CARTESIAN_POINT('Ctrl Pts',(-2.12021669100006,2.2,-3.42623750400001));
#322712=CARTESIAN_POINT('Ctrl Pts',(-2.11978764400006,12.2,-3.42571377800001));
#322713=CARTESIAN_POINT('Ctrl Pts',(-2.11978764400006,5.2,-3.42571377800001));
#322714=CARTESIAN_POINT('Ctrl Pts',(-2.11978764400006,2.2,-3.42571377800001));
#322715=CARTESIAN_POINT('Ctrl Pts',(-2.11936310100006,12.2,-3.42519419800002));
#322716=CARTESIAN_POINT('Ctrl Pts',(-2.11936310100006,5.2,-3.42519419800002));
#322717=CARTESIAN_POINT('Ctrl Pts',(-2.11936310100006,2.2,-3.42519419800002));
#322718=CARTESIAN_POINT('Ctrl Pts',(-2.11894305700006,12.2,-3.42467878500001));
#322719=CARTESIAN_POINT('Ctrl Pts',(-2.11894305700006,5.2,-3.42467878500001));
#322720=CARTESIAN_POINT('Ctrl Pts',(-2.11894305700006,2.2,-3.42467878500001));
#322721=CARTESIAN_POINT('Ctrl Pts',(-2.11852750900006,12.2,-3.42416755600001));
#322722=CARTESIAN_POINT('Ctrl Pts',(-2.11852750900006,5.2,-3.42416755600001));
#322723=CARTESIAN_POINT('Ctrl Pts',(-2.11852750900006,2.2,-3.42416755600001));
#322724=CARTESIAN_POINT('Ctrl Pts',(-2.11811645100005,12.2,-3.42366053200001));
#322725=CARTESIAN_POINT('Ctrl Pts',(-2.11811645100005,5.2,-3.42366053200001));
#322726=CARTESIAN_POINT('Ctrl Pts',(-2.11811645100005,2.2,-3.42366053200001));
#322727=CARTESIAN_POINT('Ctrl Pts',(-2.11770988300006,12.2,-3.42315773100001));
#322728=CARTESIAN_POINT('Ctrl Pts',(-2.11770988300006,5.2,-3.42315773100001));
#322729=CARTESIAN_POINT('Ctrl Pts',(-2.11770988300006,2.2,-3.42315773100001));
#322730=CARTESIAN_POINT('Ctrl Pts',(-2.11730780000006,12.2,-3.42265917200002));
#322731=CARTESIAN_POINT('Ctrl Pts',(-2.11730780000006,5.2,-3.42265917200002));
#322732=CARTESIAN_POINT('Ctrl Pts',(-2.11730780000006,2.2,-3.42265917200002));
#322733=CARTESIAN_POINT('Ctrl Pts',(-2.11691019700006,12.2,-3.42216487600002));
#322734=CARTESIAN_POINT('Ctrl Pts',(-2.11691019700006,5.2,-3.42216487600002));
#322735=CARTESIAN_POINT('Ctrl Pts',(-2.11691019700006,2.2,-3.42216487600002));
#322736=CARTESIAN_POINT('Ctrl Pts',(-2.11651707000006,12.2,-3.42167486200001));
#322737=CARTESIAN_POINT('Ctrl Pts',(-2.11651707000006,5.2,-3.42167486200001));
#322738=CARTESIAN_POINT('Ctrl Pts',(-2.11651707000006,2.2,-3.42167486200001));
#322739=CARTESIAN_POINT('Ctrl Pts',(-2.11612841600005,12.2,-3.42118914800002));
#322740=CARTESIAN_POINT('Ctrl Pts',(-2.11612841600005,5.2,-3.42118914800002));
#322741=CARTESIAN_POINT('Ctrl Pts',(-2.11612841600005,2.2,-3.42118914800002));
#322742=CARTESIAN_POINT('Ctrl Pts',(-2.11574423200006,12.2,-3.42070775600002));
#322743=CARTESIAN_POINT('Ctrl Pts',(-2.11574423200006,5.2,-3.42070775600002));
#322744=CARTESIAN_POINT('Ctrl Pts',(-2.11574423200006,2.2,-3.42070775600002));
#322745=CARTESIAN_POINT('Ctrl Pts',(-2.11536451200006,12.2,-3.42023070300002));
#322746=CARTESIAN_POINT('Ctrl Pts',(-2.11536451200006,5.2,-3.42023070300002));
#322747=CARTESIAN_POINT('Ctrl Pts',(-2.11536451200006,2.2,-3.42023070300002));
#322748=CARTESIAN_POINT('Ctrl Pts',(-2.11498925300006,12.2,-3.41975801000002));
#322749=CARTESIAN_POINT('Ctrl Pts',(-2.11498925300006,5.2,-3.41975801000002));
#322750=CARTESIAN_POINT('Ctrl Pts',(-2.11498925300006,2.2,-3.41975801000002));
#322751=CARTESIAN_POINT('Ctrl Pts',(-2.11461845100006,12.2,-3.41928969700001));
#322752=CARTESIAN_POINT('Ctrl Pts',(-2.11461845100006,5.2,-3.41928969700001));
#322753=CARTESIAN_POINT('Ctrl Pts',(-2.11461845100006,2.2,-3.41928969700001));
#322754=CARTESIAN_POINT('Ctrl Pts',(-2.11425210100006,12.2,-3.41882578300002));
#322755=CARTESIAN_POINT('Ctrl Pts',(-2.11425210100006,5.2,-3.41882578300002));
#322756=CARTESIAN_POINT('Ctrl Pts',(-2.11425210100006,2.2,-3.41882578300002));
#322757=CARTESIAN_POINT('Ctrl Pts',(-2.11389020000006,12.2,-3.41836628800001));
#322758=CARTESIAN_POINT('Ctrl Pts',(-2.11389020000006,5.2,-3.41836628800001));
#322759=CARTESIAN_POINT('Ctrl Pts',(-2.11389020000006,2.2,-3.41836628800001));
#322760=CARTESIAN_POINT('Ctrl Pts',(-2.11353274400006,12.2,-3.41791123100001));
#322761=CARTESIAN_POINT('Ctrl Pts',(-2.11353274400006,5.2,-3.41791123100001));
#322762=CARTESIAN_POINT('Ctrl Pts',(-2.11353274400006,2.2,-3.41791123100001));
#322763=CARTESIAN_POINT('Ctrl Pts',(-2.11317972800006,12.2,-3.41746063500001));
#322764=CARTESIAN_POINT('Ctrl Pts',(-2.11317972800006,5.2,-3.41746063500001));
#322765=CARTESIAN_POINT('Ctrl Pts',(-2.11317972800006,2.2,-3.41746063500001));
#322766=CARTESIAN_POINT('Ctrl Pts',(-2.11283114900006,12.2,-3.41701451600001));
#322767=CARTESIAN_POINT('Ctrl Pts',(-2.11283114900006,5.2,-3.41701451600001));
#322768=CARTESIAN_POINT('Ctrl Pts',(-2.11283114900006,2.2,-3.41701451600001));
#322769=CARTESIAN_POINT('Ctrl Pts',(-2.11248700100006,12.2,-3.41657289700001));
#322770=CARTESIAN_POINT('Ctrl Pts',(-2.11248700100006,5.2,-3.41657289700001));
#322771=CARTESIAN_POINT('Ctrl Pts',(-2.11248700100006,2.2,-3.41657289700001));
#322772=CARTESIAN_POINT('Ctrl Pts',(-2.11214728000006,12.2,-3.41613579500001));
#322773=CARTESIAN_POINT('Ctrl Pts',(-2.11214728000006,5.2,-3.41613579500001));
#322774=CARTESIAN_POINT('Ctrl Pts',(-2.11214728000006,2.2,-3.41613579500001));
#322775=CARTESIAN_POINT('Ctrl Pts',(-2.11181198300006,12.2,-3.41570323300001));
#322776=CARTESIAN_POINT('Ctrl Pts',(-2.11181198300006,5.2,-3.41570323300001));
#322777=CARTESIAN_POINT('Ctrl Pts',(-2.11181198300006,2.2,-3.41570323300001));
#322778=CARTESIAN_POINT('Ctrl Pts',(-2.11148110500006,12.2,-3.41527523000002));
#322779=CARTESIAN_POINT('Ctrl Pts',(-2.11148110500006,5.2,-3.41527523000002));
#322780=CARTESIAN_POINT('Ctrl Pts',(-2.11148110500006,2.2,-3.41527523000002));
#322781=CARTESIAN_POINT('Ctrl Pts',(-2.11115464100006,12.2,-3.41485180600001));
#322782=CARTESIAN_POINT('Ctrl Pts',(-2.11115464100006,5.2,-3.41485180600001));
#322783=CARTESIAN_POINT('Ctrl Pts',(-2.11115464100006,2.2,-3.41485180600001));
#322784=CARTESIAN_POINT('Ctrl Pts',(-2.11083258700006,12.2,-3.41443298300002));
#322785=CARTESIAN_POINT('Ctrl Pts',(-2.11083258700006,5.2,-3.41443298300002));
#322786=CARTESIAN_POINT('Ctrl Pts',(-2.11083258700006,2.2,-3.41443298300002));
#322787=CARTESIAN_POINT('Ctrl Pts',(-2.11051493900006,12.2,-3.41401877900001));
#322788=CARTESIAN_POINT('Ctrl Pts',(-2.11051493900006,5.2,-3.41401877900001));
#322789=CARTESIAN_POINT('Ctrl Pts',(-2.11051493900006,2.2,-3.41401877900001));
#322790=CARTESIAN_POINT('Ctrl Pts',(-2.11020169000005,12.2,-3.41360921600002));
#322791=CARTESIAN_POINT('Ctrl Pts',(-2.11020169000005,5.2,-3.41360921600002));
#322792=CARTESIAN_POINT('Ctrl Pts',(-2.11020169000005,2.2,-3.41360921600002));
#322793=CARTESIAN_POINT('Ctrl Pts',(-2.10989284000005,12.2,-3.41320431400002));
#322794=CARTESIAN_POINT('Ctrl Pts',(-2.10989284000005,5.2,-3.41320431400002));
#322795=CARTESIAN_POINT('Ctrl Pts',(-2.10989284000005,2.2,-3.41320431400002));
#322796=CARTESIAN_POINT('Ctrl Pts',(-2.10958838100006,12.2,-3.41280409200001));
#322797=CARTESIAN_POINT('Ctrl Pts',(-2.10958838100006,5.2,-3.41280409200001));
#322798=CARTESIAN_POINT('Ctrl Pts',(-2.10958838100006,2.2,-3.41280409200001));
#322799=CARTESIAN_POINT('Ctrl Pts',(-2.10928830800006,12.2,-3.41240857400001));
#322800=CARTESIAN_POINT('Ctrl Pts',(-2.10928830800006,5.2,-3.41240857400001));
#322801=CARTESIAN_POINT('Ctrl Pts',(-2.10928830800006,2.2,-3.41240857400001));
#322802=CARTESIAN_POINT('Ctrl Pts',(-2.10899261900006,12.2,-3.41201777800002));
#322803=CARTESIAN_POINT('Ctrl Pts',(-2.10899261900006,5.2,-3.41201777800002));
#322804=CARTESIAN_POINT('Ctrl Pts',(-2.10899261900006,2.2,-3.41201777800002));
#322805=CARTESIAN_POINT('Ctrl Pts',(-2.10870130700005,12.2,-3.41163172500002));
#322806=CARTESIAN_POINT('Ctrl Pts',(-2.10870130700005,5.2,-3.41163172500002));
#322807=CARTESIAN_POINT('Ctrl Pts',(-2.10870130700005,2.2,-3.41163172500002));
#322808=CARTESIAN_POINT('Ctrl Pts',(-2.10841436900005,12.2,-3.41125043600002));
#322809=CARTESIAN_POINT('Ctrl Pts',(-2.10841436900005,5.2,-3.41125043600002));
#322810=CARTESIAN_POINT('Ctrl Pts',(-2.10841436900005,2.2,-3.41125043600002));
#322811=CARTESIAN_POINT('Ctrl Pts',(-2.10813179800006,12.2,-3.41087393300001));
#322812=CARTESIAN_POINT('Ctrl Pts',(-2.10813179800006,5.2,-3.41087393300001));
#322813=CARTESIAN_POINT('Ctrl Pts',(-2.10813179800006,2.2,-3.41087393300001));
#322814=CARTESIAN_POINT('Ctrl Pts',(-2.10785359100006,12.2,-3.41050223400002));
#322815=CARTESIAN_POINT('Ctrl Pts',(-2.10785359100006,5.2,-3.41050223400002));
#322816=CARTESIAN_POINT('Ctrl Pts',(-2.10785359100006,2.2,-3.41050223400002));
#322817=CARTESIAN_POINT('Ctrl Pts',(-2.10757974300006,12.2,-3.41013536400002));
#322818=CARTESIAN_POINT('Ctrl Pts',(-2.10757974300006,5.2,-3.41013536400002));
#322819=CARTESIAN_POINT('Ctrl Pts',(-2.10757974300006,2.2,-3.41013536400002));
#322820=CARTESIAN_POINT('Ctrl Pts',(-2.10731024700006,12.2,-3.40977334100002));
#322821=CARTESIAN_POINT('Ctrl Pts',(-2.10731024700006,5.2,-3.40977334100002));
#322822=CARTESIAN_POINT('Ctrl Pts',(-2.10731024700006,2.2,-3.40977334100002));
#322823=CARTESIAN_POINT('Ctrl Pts',(-2.10704510100005,12.2,-3.40941618700001));
#322824=CARTESIAN_POINT('Ctrl Pts',(-2.10704510100005,5.2,-3.40941618700001));
#322825=CARTESIAN_POINT('Ctrl Pts',(-2.10704510100005,2.2,-3.40941618700001));
#322826=CARTESIAN_POINT('Ctrl Pts',(-2.10678429900006,12.2,-3.40906392200001));
#322827=CARTESIAN_POINT('Ctrl Pts',(-2.10678429900006,5.2,-3.40906392200001));
#322828=CARTESIAN_POINT('Ctrl Pts',(-2.10678429900006,2.2,-3.40906392200001));
#322829=CARTESIAN_POINT('Ctrl Pts',(-2.10652783500006,12.2,-3.40871657000001));
#322830=CARTESIAN_POINT('Ctrl Pts',(-2.10652783500006,5.2,-3.40871657000001));
#322831=CARTESIAN_POINT('Ctrl Pts',(-2.10652783500006,2.2,-3.40871657000001));
#322832=CARTESIAN_POINT('Ctrl Pts',(-2.10627570600006,12.2,-3.40837415000002));
#322833=CARTESIAN_POINT('Ctrl Pts',(-2.10627570600006,5.2,-3.40837415000002));
#322834=CARTESIAN_POINT('Ctrl Pts',(-2.10627570600006,2.2,-3.40837415000002));
#322835=CARTESIAN_POINT('Ctrl Pts',(-2.10602790400006,12.2,-3.40803668300001));
#322836=CARTESIAN_POINT('Ctrl Pts',(-2.10602790400006,5.2,-3.40803668300001));
#322837=CARTESIAN_POINT('Ctrl Pts',(-2.10602790400006,2.2,-3.40803668300001));
#322838=CARTESIAN_POINT('Ctrl Pts',(-2.10578442500006,12.2,-3.40770419100001));
#322839=CARTESIAN_POINT('Ctrl Pts',(-2.10578442500006,5.2,-3.40770419100001));
#322840=CARTESIAN_POINT('Ctrl Pts',(-2.10578442500006,2.2,-3.40770419100001));
#322841=CARTESIAN_POINT('Ctrl Pts',(-2.10554526400006,12.2,-3.40737669700002));
#322842=CARTESIAN_POINT('Ctrl Pts',(-2.10554526400006,5.2,-3.40737669700002));
#322843=CARTESIAN_POINT('Ctrl Pts',(-2.10554526400006,2.2,-3.40737669700002));
#322844=CARTESIAN_POINT('Ctrl Pts',(-2.10531041800006,12.2,-3.40705422000001));
#322845=CARTESIAN_POINT('Ctrl Pts',(-2.10531041800006,5.2,-3.40705422000001));
#322846=CARTESIAN_POINT('Ctrl Pts',(-2.10531041800006,2.2,-3.40705422000001));
#322847=CARTESIAN_POINT('Ctrl Pts',(-2.10507987800006,12.2,-3.40673678300002));
#322848=CARTESIAN_POINT('Ctrl Pts',(-2.10507987800006,5.2,-3.40673678300002));
#322849=CARTESIAN_POINT('Ctrl Pts',(-2.10507987800006,2.2,-3.40673678300002));
#322850=CARTESIAN_POINT('Ctrl Pts',(-2.10485364100006,12.2,-3.40642440800002));
#322851=CARTESIAN_POINT('Ctrl Pts',(-2.10485364100006,5.2,-3.40642440800002));
#322852=CARTESIAN_POINT('Ctrl Pts',(-2.10485364100006,2.2,-3.40642440800002));
#322853=CARTESIAN_POINT('Ctrl Pts',(-2.10463170000006,12.2,-3.40611711600001));
#322854=CARTESIAN_POINT('Ctrl Pts',(-2.10463170000006,5.2,-3.40611711600001));
#322855=CARTESIAN_POINT('Ctrl Pts',(-2.10463170000006,2.2,-3.40611711600001));
#322856=CARTESIAN_POINT('Ctrl Pts',(-2.10441405000005,12.2,-3.40581492800001));
#322857=CARTESIAN_POINT('Ctrl Pts',(-2.10441405000005,5.2,-3.40581492800001));
#322858=CARTESIAN_POINT('Ctrl Pts',(-2.10441405000005,2.2,-3.40581492800001));
#322859=CARTESIAN_POINT('Ctrl Pts',(-2.10420068800006,12.2,-3.40551786700001));
#322860=CARTESIAN_POINT('Ctrl Pts',(-2.10420068800006,5.2,-3.40551786700001));
#322861=CARTESIAN_POINT('Ctrl Pts',(-2.10420068800006,2.2,-3.40551786700001));
#322862=CARTESIAN_POINT('Ctrl Pts',(-2.10399160500006,12.2,-3.40522595500001));
#322863=CARTESIAN_POINT('Ctrl Pts',(-2.10399160500006,5.2,-3.40522595500001));
#322864=CARTESIAN_POINT('Ctrl Pts',(-2.10399160500006,2.2,-3.40522595500001));
#322865=CARTESIAN_POINT('Ctrl Pts',(-2.10378679800006,12.2,-3.40493921300002));
#322866=CARTESIAN_POINT('Ctrl Pts',(-2.10378679800006,5.2,-3.40493921300002));
#322867=CARTESIAN_POINT('Ctrl Pts',(-2.10378679800006,2.2,-3.40493921300002));
#322868=CARTESIAN_POINT('Ctrl Pts',(-2.10358626000006,12.2,-3.40465766400001));
#322869=CARTESIAN_POINT('Ctrl Pts',(-2.10358626000006,5.2,-3.40465766400001));
#322870=CARTESIAN_POINT('Ctrl Pts',(-2.10358626000006,2.2,-3.40465766400001));
#322871=CARTESIAN_POINT('Ctrl Pts',(-2.10338998700006,12.2,-3.40438132900001));
#322872=CARTESIAN_POINT('Ctrl Pts',(-2.10338998700006,5.2,-3.40438132900001));
#322873=CARTESIAN_POINT('Ctrl Pts',(-2.10338998700006,2.2,-3.40438132900001));
#322874=CARTESIAN_POINT('Ctrl Pts',(-2.10319797000006,12.2,-3.40411023100001));
#322875=CARTESIAN_POINT('Ctrl Pts',(-2.10319797000006,5.2,-3.40411023100001));
#322876=CARTESIAN_POINT('Ctrl Pts',(-2.10319797000006,2.2,-3.40411023100001));
#322877=CARTESIAN_POINT('Ctrl Pts',(-2.10301020700005,12.2,-3.40384439300002));
#322878=CARTESIAN_POINT('Ctrl Pts',(-2.10301020700005,5.2,-3.40384439300002));
#322879=CARTESIAN_POINT('Ctrl Pts',(-2.10301020700005,2.2,-3.40384439300002));
#322880=CARTESIAN_POINT('Ctrl Pts',(-2.10282669100006,12.2,-3.40358383500002));
#322881=CARTESIAN_POINT('Ctrl Pts',(-2.10282669100006,5.2,-3.40358383500002));
#322882=CARTESIAN_POINT('Ctrl Pts',(-2.10282669100006,2.2,-3.40358383500002));
#322883=CARTESIAN_POINT('Ctrl Pts',(-2.10264741500006,12.2,-3.40332858100002));
#322884=CARTESIAN_POINT('Ctrl Pts',(-2.10264741500006,5.2,-3.40332858100002));
#322885=CARTESIAN_POINT('Ctrl Pts',(-2.10264741500006,2.2,-3.40332858100002));
#322886=CARTESIAN_POINT('Ctrl Pts',(-2.10247237400006,12.2,-3.40307865400002));
#322887=CARTESIAN_POINT('Ctrl Pts',(-2.10247237400006,5.2,-3.40307865400002));
#322888=CARTESIAN_POINT('Ctrl Pts',(-2.10247237400006,2.2,-3.40307865400002));
#322889=CARTESIAN_POINT('Ctrl Pts',(-2.10230156200006,12.2,-3.40283407500001));
#322890=CARTESIAN_POINT('Ctrl Pts',(-2.10230156200006,5.2,-3.40283407500001));
#322891=CARTESIAN_POINT('Ctrl Pts',(-2.10230156200006,2.2,-3.40283407500001));
#322892=CARTESIAN_POINT('Ctrl Pts',(-2.10213497400006,12.2,-3.40259486800001));
#322893=CARTESIAN_POINT('Ctrl Pts',(-2.10213497400006,5.2,-3.40259486800001));
#322894=CARTESIAN_POINT('Ctrl Pts',(-2.10213497400006,2.2,-3.40259486800001));
#322895=CARTESIAN_POINT('Ctrl Pts',(-2.10197260400005,12.2,-3.40236105400002));
#322896=CARTESIAN_POINT('Ctrl Pts',(-2.10197260400005,5.2,-3.40236105400002));
#322897=CARTESIAN_POINT('Ctrl Pts',(-2.10197260400005,2.2,-3.40236105400002));
#322898=CARTESIAN_POINT('Ctrl Pts',(-2.10181444400006,12.2,-3.40213265700001));
#322899=CARTESIAN_POINT('Ctrl Pts',(-2.10181444400006,5.2,-3.40213265700001));
#322900=CARTESIAN_POINT('Ctrl Pts',(-2.10181444400006,2.2,-3.40213265700001));
#322901=CARTESIAN_POINT('Ctrl Pts',(-2.10166048900006,12.2,-3.40190970000001));
#322902=CARTESIAN_POINT('Ctrl Pts',(-2.10166048900006,5.2,-3.40190970000001));
#322903=CARTESIAN_POINT('Ctrl Pts',(-2.10166048900006,2.2,-3.40190970000001));
#322904=CARTESIAN_POINT('Ctrl Pts',(-2.10151073300006,12.2,-3.40169220500002));
#322905=CARTESIAN_POINT('Ctrl Pts',(-2.10151073300006,5.2,-3.40169220500002));
#322906=CARTESIAN_POINT('Ctrl Pts',(-2.10151073300006,2.2,-3.40169220500002));
#322907=CARTESIAN_POINT('Ctrl Pts',(-2.10136517100006,12.2,-3.40148019400001));
#322908=CARTESIAN_POINT('Ctrl Pts',(-2.10136517100006,5.2,-3.40148019400001));
#322909=CARTESIAN_POINT('Ctrl Pts',(-2.10136517100006,2.2,-3.40148019400001));
#322910=CARTESIAN_POINT('Ctrl Pts',(-2.10122379400006,12.2,-3.40127369300002));
#322911=CARTESIAN_POINT('Ctrl Pts',(-2.10122379400006,5.2,-3.40127369300002));
#322912=CARTESIAN_POINT('Ctrl Pts',(-2.10122379400006,2.2,-3.40127369300002));
#322913=CARTESIAN_POINT('Ctrl Pts',(-2.10108659900006,12.2,-3.40107272300001));
#322914=CARTESIAN_POINT('Ctrl Pts',(-2.10108659900006,5.2,-3.40107272300001));
#322915=CARTESIAN_POINT('Ctrl Pts',(-2.10108659900006,2.2,-3.40107272300001));
#322916=CARTESIAN_POINT('Ctrl Pts',(-2.10095357700005,12.2,-3.40087730700001));
#322917=CARTESIAN_POINT('Ctrl Pts',(-2.10095357700005,5.2,-3.40087730700001));
#322918=CARTESIAN_POINT('Ctrl Pts',(-2.10095357700005,2.2,-3.40087730700001));
#322919=CARTESIAN_POINT('Ctrl Pts',(-2.10082472400006,12.2,-3.40068746900001));
#322920=CARTESIAN_POINT('Ctrl Pts',(-2.10082472400006,5.2,-3.40068746900001));
#322921=CARTESIAN_POINT('Ctrl Pts',(-2.10082472400006,2.2,-3.40068746900001));
#322922=CARTESIAN_POINT('Ctrl Pts',(-2.10070003200005,12.2,-3.40050323100002));
#322923=CARTESIAN_POINT('Ctrl Pts',(-2.10070003200005,5.2,-3.40050323100002));
#322924=CARTESIAN_POINT('Ctrl Pts',(-2.10070003200005,2.2,-3.40050323100002));
#322925=CARTESIAN_POINT('Ctrl Pts',(-2.10057949400006,12.2,-3.40032461800002));
#322926=CARTESIAN_POINT('Ctrl Pts',(-2.10057949400006,5.2,-3.40032461800002));
#322927=CARTESIAN_POINT('Ctrl Pts',(-2.10057949400006,2.2,-3.40032461800002));
#322928=CARTESIAN_POINT('Ctrl Pts',(-2.10046310500006,12.2,-3.40015165400001));
#322929=CARTESIAN_POINT('Ctrl Pts',(-2.10046310500006,5.2,-3.40015165400001));
#322930=CARTESIAN_POINT('Ctrl Pts',(-2.10046310500006,2.2,-3.40015165400001));
#322931=CARTESIAN_POINT('Ctrl Pts',(-2.10035085800006,12.2,-3.39998436000001));
#322932=CARTESIAN_POINT('Ctrl Pts',(-2.10035085800006,5.2,-3.39998436000001));
#322933=CARTESIAN_POINT('Ctrl Pts',(-2.10035085800006,2.2,-3.39998436000001));
#322934=CARTESIAN_POINT('Ctrl Pts',(-2.10024274500006,12.2,-3.39982276200002));
#322935=CARTESIAN_POINT('Ctrl Pts',(-2.10024274500006,5.2,-3.39982276200002));
#322936=CARTESIAN_POINT('Ctrl Pts',(-2.10024274500006,2.2,-3.39982276200002));
#322937=CARTESIAN_POINT('Ctrl Pts',(-2.10013876200006,12.2,-3.39966688300001));
#322938=CARTESIAN_POINT('Ctrl Pts',(-2.10013876200006,5.2,-3.39966688300001));
#322939=CARTESIAN_POINT('Ctrl Pts',(-2.10013876200006,2.2,-3.39966688300001));
#322940=CARTESIAN_POINT('Ctrl Pts',(-2.10003890000006,12.2,-3.39951674700002));
#322941=CARTESIAN_POINT('Ctrl Pts',(-2.10003890000006,5.2,-3.39951674700002));
#322942=CARTESIAN_POINT('Ctrl Pts',(-2.10003890000006,2.2,-3.39951674700002));
#322943=CARTESIAN_POINT('Ctrl Pts',(-2.09994315400006,12.2,-3.39937237600001));
#322944=CARTESIAN_POINT('Ctrl Pts',(-2.09994315400006,5.2,-3.39937237600001));
#322945=CARTESIAN_POINT('Ctrl Pts',(-2.09994315400006,2.2,-3.39937237600001));
#322946=CARTESIAN_POINT('Ctrl Pts',(-2.09985151600006,12.2,-3.39923379500001));
#322947=CARTESIAN_POINT('Ctrl Pts',(-2.09985151600006,5.2,-3.39923379500001));
#322948=CARTESIAN_POINT('Ctrl Pts',(-2.09985151600006,2.2,-3.39923379500001));
#322949=CARTESIAN_POINT('Ctrl Pts',(-2.09976398000005,12.2,-3.39910102700001));
#322950=CARTESIAN_POINT('Ctrl Pts',(-2.09976398000005,5.2,-3.39910102700001));
#322951=CARTESIAN_POINT('Ctrl Pts',(-2.09976398000005,2.2,-3.39910102700001));
#322952=CARTESIAN_POINT('Ctrl Pts',(-2.09968053900006,12.2,-3.39897409600002));
#322953=CARTESIAN_POINT('Ctrl Pts',(-2.09968053900006,5.2,-3.39897409600002));
#322954=CARTESIAN_POINT('Ctrl Pts',(-2.09968053900006,2.2,-3.39897409600002));
#322955=CARTESIAN_POINT('Ctrl Pts',(-2.09960118500006,12.2,-3.39885302900001));
#322956=CARTESIAN_POINT('Ctrl Pts',(-2.09960118500006,5.2,-3.39885302900001));
#322957=CARTESIAN_POINT('Ctrl Pts',(-2.09960118500006,2.2,-3.39885302900001));
#322958=CARTESIAN_POINT('Ctrl Pts',(-2.09952591200006,12.2,-3.39873785000002));
#322959=CARTESIAN_POINT('Ctrl Pts',(-2.09952591200006,5.2,-3.39873785000002));
#322960=CARTESIAN_POINT('Ctrl Pts',(-2.09952591200006,2.2,-3.39873785000002));
#322961=CARTESIAN_POINT('Ctrl Pts',(-2.09945471100006,12.2,-3.39862858500001));
#322962=CARTESIAN_POINT('Ctrl Pts',(-2.09945471100006,5.2,-3.39862858500001));
#322963=CARTESIAN_POINT('Ctrl Pts',(-2.09945471100006,2.2,-3.39862858500001));
#322964=CARTESIAN_POINT('Ctrl Pts',(-2.09938757500006,12.2,-3.39852525600001));
#322965=CARTESIAN_POINT('Ctrl Pts',(-2.09938757500006,5.2,-3.39852525600001));
#322966=CARTESIAN_POINT('Ctrl Pts',(-2.09938757500006,2.2,-3.39852525600001));
#322967=CARTESIAN_POINT('Ctrl Pts',(-2.09932450100006,12.2,-3.39842788700001));
#322968=CARTESIAN_POINT('Ctrl Pts',(-2.09932450100006,5.2,-3.39842788700001));
#322969=CARTESIAN_POINT('Ctrl Pts',(-2.09932450100006,2.2,-3.39842788700001));
#322970=CARTESIAN_POINT('Ctrl Pts',(-2.09926547900006,12.2,-3.39833649900001));
#322971=CARTESIAN_POINT('Ctrl Pts',(-2.09926547900006,5.2,-3.39833649900001));
#322972=CARTESIAN_POINT('Ctrl Pts',(-2.09926547900006,2.2,-3.39833649900001));
#322973=CARTESIAN_POINT('Ctrl Pts',(-2.09921050200006,12.2,-3.39825111500001));
#322974=CARTESIAN_POINT('Ctrl Pts',(-2.09921050200006,5.2,-3.39825111500001));
#322975=CARTESIAN_POINT('Ctrl Pts',(-2.09921050200006,2.2,-3.39825111500001));
#322976=CARTESIAN_POINT('Ctrl Pts',(-2.09915956600006,12.2,-3.39817176000001));
#322977=CARTESIAN_POINT('Ctrl Pts',(-2.09915956600006,5.2,-3.39817176000001));
#322978=CARTESIAN_POINT('Ctrl Pts',(-2.09915956600006,2.2,-3.39817176000001));
#322979=CARTESIAN_POINT('Ctrl Pts',(-2.09911266000006,12.2,-3.39809846200001));
#322980=CARTESIAN_POINT('Ctrl Pts',(-2.09911266000006,5.2,-3.39809846200001));
#322981=CARTESIAN_POINT('Ctrl Pts',(-2.09911266000006,2.2,-3.39809846200001));
#322982=CARTESIAN_POINT('Ctrl Pts',(-2.09906977500005,12.2,-3.39803125200001));
#322983=CARTESIAN_POINT('Ctrl Pts',(-2.09906977500005,5.2,-3.39803125200001));
#322984=CARTESIAN_POINT('Ctrl Pts',(-2.09906977500005,2.2,-3.39803125200001));
#322985=CARTESIAN_POINT('Ctrl Pts',(-2.09903090200006,12.2,-3.39797016400002));
#322986=CARTESIAN_POINT('Ctrl Pts',(-2.09903090200006,5.2,-3.39797016400002));
#322987=CARTESIAN_POINT('Ctrl Pts',(-2.09903090200006,2.2,-3.39797016400002));
#322988=CARTESIAN_POINT('Ctrl Pts',(-2.09899603200005,12.2,-3.39791522200001));
#322989=CARTESIAN_POINT('Ctrl Pts',(-2.09899603200005,5.2,-3.39791522200001));
#322990=CARTESIAN_POINT('Ctrl Pts',(-2.09899603200005,2.2,-3.39791522200001));
#322991=CARTESIAN_POINT('Ctrl Pts',(-2.09896516000006,12.2,-3.39786644800002));
#322992=CARTESIAN_POINT('Ctrl Pts',(-2.09896516000006,5.2,-3.39786644800002));
#322993=CARTESIAN_POINT('Ctrl Pts',(-2.09896516000006,2.2,-3.39786644800002));
#322994=CARTESIAN_POINT('Ctrl Pts',(-2.0989354047251,12.2,-3.39781929544304));
#322995=CARTESIAN_POINT('Ctrl Pts',(-2.0989354047251,5.2,-3.39781929544304));
#322996=CARTESIAN_POINT('Ctrl Pts',(-2.0989354047251,2.2,-3.39781929544304));
#322997=CARTESIAN_POINT('Ctrl Pts',(-2.0989151302594,12.2,-3.39778702279926));
#322998=CARTESIAN_POINT('Ctrl Pts',(-2.0989151302594,5.2,-3.39778702279926));
#322999=CARTESIAN_POINT('Ctrl Pts',(-2.0989151302594,2.2,-3.39778702279926));
#323000=CARTESIAN_POINT('Ctrl Pts',(-2.09890181977372,12.2,-3.39776573310334));
#323001=CARTESIAN_POINT('Ctrl Pts',(-2.09890181977372,5.2,-3.39776573310334));
#323002=CARTESIAN_POINT('Ctrl Pts',(-2.09890181977372,2.2,-3.39776573310334));
#323003=CARTESIAN_POINT('Ctrl Pts',(-2.09889355742141,12.2,-3.39775245437597));
#323004=CARTESIAN_POINT('Ctrl Pts',(-2.09889355742141,5.2,-3.39775245437597));
#323005=CARTESIAN_POINT('Ctrl Pts',(-2.09889355742141,2.2,-3.39775245437597));
#323006=CARTESIAN_POINT('Ctrl Pts',(-2.09888845200005,12.2,-3.39774425600002));
#323007=CARTESIAN_POINT('Ctrl Pts',(-2.09888845200005,5.2,-3.39774425600002));
#323008=CARTESIAN_POINT('Ctrl Pts',(-2.09888845200005,2.2,-3.39774425600002));
#323009=CARTESIAN_POINT('',(-2.09888828100006,2.7,-3.39774436300001));
#323010=CARTESIAN_POINT('',(-2.09888828100006,12.2,-3.39774436300001));
#323011=CARTESIAN_POINT('Ctrl Pts',(-2.77990780000006,2.7,-3.85157274700001));
#323012=CARTESIAN_POINT('Ctrl Pts',(-2.5607296334765,2.7,-3.76566536820642));
#323013=CARTESIAN_POINT('Ctrl Pts',(-2.39555995610288,2.6999999999955,-3.66650574172274));
#323014=CARTESIAN_POINT('Ctrl Pts',(-2.15514138129518,2.6999999999955,-3.47929284706468));
#323015=CARTESIAN_POINT('Ctrl Pts',(-2.10572616940241,2.7,-3.40841675459135));
#323016=CARTESIAN_POINT('Ctrl Pts',(-2.09906882271441,2.7,-3.39803012695728));
#323017=CARTESIAN_POINT('Ctrl Pts',(-2.09897779197314,2.7,-3.39788771970969));
#323018=CARTESIAN_POINT('Ctrl Pts',(-2.09888845200005,2.7,-3.39774425600002));
#323019=CARTESIAN_POINT('Origin',(-2.09886131100005,15.2,-3.39770070400002));
#323020=CARTESIAN_POINT('',(-1.90509662000005,2.7,-3.08402851200002));
#323021=CARTESIAN_POINT('',(-1.90509662000005,2.2,-3.08402851200002));
#323022=CARTESIAN_POINT('',(-1.04943065555809,2.7,-1.69885035196417));
#323023=CARTESIAN_POINT('Origin',(-5.66300478732629E-14,15.2,-1.77635683940025E-14));
#323024=CARTESIAN_POINT('',(-1.40617553900006,2.7,-3.34115180000001));
#323025=CARTESIAN_POINT('',(-1.40617553900006,12.2,-3.34115180000001));
#323026=CARTESIAN_POINT('Origin',(-5.66300478732629E-14,2.7,-1.92943768261394E-14));
#323027=CARTESIAN_POINT('Origin',(-5.66300478732629E-14,15.2,-1.77635683940025E-14));
#323028=CARTESIAN_POINT('',(-1.54920894300006,2.7,-3.68100717000001));
#323029=CARTESIAN_POINT('',(-1.54920894300006,12.2,-3.68100717000001));
#323030=CARTESIAN_POINT('',(-5.63454419629576E-14,2.7,-1.86181372517296E-14));
#323031=CARTESIAN_POINT('Ctrl Pts',(-1.54920881500006,12.2,-3.68100722400001));
#323032=CARTESIAN_POINT('Ctrl Pts',(-1.54920881500006,5.2,-3.68100722400001));
#323033=CARTESIAN_POINT('Ctrl Pts',(-1.54920881500006,2.2,-3.68100722400001));
#323034=CARTESIAN_POINT('Ctrl Pts',(-1.54921144480716,12.2,-3.68101354053696));
#323035=CARTESIAN_POINT('Ctrl Pts',(-1.54921144480716,5.2,-3.68101354053696));
#323036=CARTESIAN_POINT('Ctrl Pts',(-1.54921144480716,2.2,-3.68101354053696));
#323037=CARTESIAN_POINT('Ctrl Pts',(-1.54921653367158,12.2,-3.6810257569059));
#323038=CARTESIAN_POINT('Ctrl Pts',(-1.54921653367158,5.2,-3.6810257569059));
#323039=CARTESIAN_POINT('Ctrl Pts',(-1.54921653367158,2.2,-3.6810257569059));
#323040=CARTESIAN_POINT('Ctrl Pts',(-1.54922407480527,12.2,-3.68104387907971));
#323041=CARTESIAN_POINT('Ctrl Pts',(-1.54922407480527,5.2,-3.68104387907971));
#323042=CARTESIAN_POINT('Ctrl Pts',(-1.54922407480527,2.2,-3.68104387907971));
#323043=CARTESIAN_POINT('Ctrl Pts',(-1.54923408213771,12.2,-3.68106787202714));
#323044=CARTESIAN_POINT('Ctrl Pts',(-1.54923408213771,5.19999999999999,
-3.68106787202714));
#323045=CARTESIAN_POINT('Ctrl Pts',(-1.54923408213771,2.2,-3.68106787202714));
#323046=CARTESIAN_POINT('Ctrl Pts',(-1.54925130100006,12.2,-3.68110978700001));
#323047=CARTESIAN_POINT('Ctrl Pts',(-1.54925130100006,5.2,-3.68110978700001));
#323048=CARTESIAN_POINT('Ctrl Pts',(-1.54925130100006,2.2,-3.68110978700001));
#323049=CARTESIAN_POINT('Ctrl Pts',(-1.54927039300006,12.2,-3.68115639400001));
#323050=CARTESIAN_POINT('Ctrl Pts',(-1.54927039300006,5.2,-3.68115639400001));
#323051=CARTESIAN_POINT('Ctrl Pts',(-1.54927039300006,2.2,-3.68115639400001));
#323052=CARTESIAN_POINT('Ctrl Pts',(-1.54929219900006,12.2,-3.68120983900001));
#323053=CARTESIAN_POINT('Ctrl Pts',(-1.54929219900006,5.2,-3.68120983900001));
#323054=CARTESIAN_POINT('Ctrl Pts',(-1.54929219900006,2.2,-3.68120983900001));
#323055=CARTESIAN_POINT('Ctrl Pts',(-1.54931671100006,12.2,-3.68127011900001));
#323056=CARTESIAN_POINT('Ctrl Pts',(-1.54931671100006,5.2,-3.68127011900001));
#323057=CARTESIAN_POINT('Ctrl Pts',(-1.54931671100006,2.2,-3.68127011900001));
#323058=CARTESIAN_POINT('Ctrl Pts',(-1.54934390400005,12.2,-3.68133722700001));
#323059=CARTESIAN_POINT('Ctrl Pts',(-1.54934390400005,5.2,-3.68133722700001));
#323060=CARTESIAN_POINT('Ctrl Pts',(-1.54934390400005,2.2,-3.68133722700001));
#323061=CARTESIAN_POINT('Ctrl Pts',(-1.54937375600006,12.2,-3.68141115300002));
#323062=CARTESIAN_POINT('Ctrl Pts',(-1.54937375600006,5.2,-3.68141115300002));
#323063=CARTESIAN_POINT('Ctrl Pts',(-1.54937375600006,2.2,-3.68141115300002));
#323064=CARTESIAN_POINT('Ctrl Pts',(-1.54940623200006,12.2,-3.68149188800002));
#323065=CARTESIAN_POINT('Ctrl Pts',(-1.54940623200006,5.2,-3.68149188800002));
#323066=CARTESIAN_POINT('Ctrl Pts',(-1.54940623200006,2.2,-3.68149188800002));
#323067=CARTESIAN_POINT('Ctrl Pts',(-1.54944130200006,12.2,-3.68157942000002));
#323068=CARTESIAN_POINT('Ctrl Pts',(-1.54944130200006,5.2,-3.68157942000002));
#323069=CARTESIAN_POINT('Ctrl Pts',(-1.54944130200006,2.2,-3.68157942000002));
#323070=CARTESIAN_POINT('Ctrl Pts',(-1.54947893900005,12.2,-3.68167374100001));
#323071=CARTESIAN_POINT('Ctrl Pts',(-1.54947893900005,5.2,-3.68167374100001));
#323072=CARTESIAN_POINT('Ctrl Pts',(-1.54947893900005,2.2,-3.68167374100001));
#323073=CARTESIAN_POINT('Ctrl Pts',(-1.54951911600006,12.2,-3.68177484000002));
#323074=CARTESIAN_POINT('Ctrl Pts',(-1.54951911600006,5.2,-3.68177484000002));
#323075=CARTESIAN_POINT('Ctrl Pts',(-1.54951911600006,2.2,-3.68177484000002));
#323076=CARTESIAN_POINT('Ctrl Pts',(-1.54956181300005,12.2,-3.68188271100002));
#323077=CARTESIAN_POINT('Ctrl Pts',(-1.54956181300005,5.2,-3.68188271100002));
#323078=CARTESIAN_POINT('Ctrl Pts',(-1.54956181300005,2.2,-3.68188271100002));
#323079=CARTESIAN_POINT('Ctrl Pts',(-1.54960700900005,12.2,-3.68199734600001));
#323080=CARTESIAN_POINT('Ctrl Pts',(-1.54960700900005,5.2,-3.68199734600001));
#323081=CARTESIAN_POINT('Ctrl Pts',(-1.54960700900005,2.2,-3.68199734600001));
#323082=CARTESIAN_POINT('Ctrl Pts',(-1.54965467900006,12.2,-3.68211873800002));
#323083=CARTESIAN_POINT('Ctrl Pts',(-1.54965467900006,5.2,-3.68211873800002));
#323084=CARTESIAN_POINT('Ctrl Pts',(-1.54965467900006,2.2,-3.68211873800002));
#323085=CARTESIAN_POINT('Ctrl Pts',(-1.54970480200005,12.2,-3.68224687900002));
#323086=CARTESIAN_POINT('Ctrl Pts',(-1.54970480200005,5.2,-3.68224687900002));
#323087=CARTESIAN_POINT('Ctrl Pts',(-1.54970480200005,2.2,-3.68224687900002));
#323088=CARTESIAN_POINT('Ctrl Pts',(-1.54975735300006,12.2,-3.68238175900002));
#323089=CARTESIAN_POINT('Ctrl Pts',(-1.54975735300006,5.2,-3.68238175900002));
#323090=CARTESIAN_POINT('Ctrl Pts',(-1.54975735300006,2.2,-3.68238175900002));
#323091=CARTESIAN_POINT('Ctrl Pts',(-1.54981230700006,12.2,-3.68252337000001));
#323092=CARTESIAN_POINT('Ctrl Pts',(-1.54981230700006,5.2,-3.68252337000001));
#323093=CARTESIAN_POINT('Ctrl Pts',(-1.54981230700006,2.2,-3.68252337000001));
#323094=CARTESIAN_POINT('Ctrl Pts',(-1.54986963900006,12.2,-3.68267170500001));
#323095=CARTESIAN_POINT('Ctrl Pts',(-1.54986963900006,5.2,-3.68267170500001));
#323096=CARTESIAN_POINT('Ctrl Pts',(-1.54986963900006,2.2,-3.68267170500001));
#323097=CARTESIAN_POINT('Ctrl Pts',(-1.54992932600006,12.2,-3.68282675200001));
#323098=CARTESIAN_POINT('Ctrl Pts',(-1.54992932600006,5.2,-3.68282675200001));
#323099=CARTESIAN_POINT('Ctrl Pts',(-1.54992932600006,2.2,-3.68282675200001));
#323100=CARTESIAN_POINT('Ctrl Pts',(-1.54999134300006,12.2,-3.68298850500001));
#323101=CARTESIAN_POINT('Ctrl Pts',(-1.54999134300006,5.2,-3.68298850500001));
#323102=CARTESIAN_POINT('Ctrl Pts',(-1.54999134300006,2.2,-3.68298850500001));
#323103=CARTESIAN_POINT('Ctrl Pts',(-1.55005566800006,12.2,-3.68315695700002));
#323104=CARTESIAN_POINT('Ctrl Pts',(-1.55005566800006,5.2,-3.68315695700002));
#323105=CARTESIAN_POINT('Ctrl Pts',(-1.55005566800006,2.2,-3.68315695700002));
#323106=CARTESIAN_POINT('Ctrl Pts',(-1.55012227800006,12.2,-3.68333209600001));
#323107=CARTESIAN_POINT('Ctrl Pts',(-1.55012227800006,5.2,-3.68333209600001));
#323108=CARTESIAN_POINT('Ctrl Pts',(-1.55012227800006,2.2,-3.68333209600001));
#323109=CARTESIAN_POINT('Ctrl Pts',(-1.55019114900006,12.2,-3.68351391700001));
#323110=CARTESIAN_POINT('Ctrl Pts',(-1.55019114900006,5.2,-3.68351391700001));
#323111=CARTESIAN_POINT('Ctrl Pts',(-1.55019114900006,2.2,-3.68351391700001));
#323112=CARTESIAN_POINT('Ctrl Pts',(-1.55026226000006,12.2,-3.68370241000001));
#323113=CARTESIAN_POINT('Ctrl Pts',(-1.55026226000006,5.2,-3.68370241000001));
#323114=CARTESIAN_POINT('Ctrl Pts',(-1.55026226000006,2.2,-3.68370241000001));
#323115=CARTESIAN_POINT('Ctrl Pts',(-1.55033558600006,12.2,-3.68389756800001));
#323116=CARTESIAN_POINT('Ctrl Pts',(-1.55033558600006,5.2,-3.68389756800001));
#323117=CARTESIAN_POINT('Ctrl Pts',(-1.55033558600006,2.2,-3.68389756800001));
#323118=CARTESIAN_POINT('Ctrl Pts',(-1.55041110500005,12.2,-3.68409938100001));
#323119=CARTESIAN_POINT('Ctrl Pts',(-1.55041110500005,5.2,-3.68409938100001));
#323120=CARTESIAN_POINT('Ctrl Pts',(-1.55041110500005,2.2,-3.68409938100001));
#323121=CARTESIAN_POINT('Ctrl Pts',(-1.55048879300006,12.2,-3.68430784300001));
#323122=CARTESIAN_POINT('Ctrl Pts',(-1.55048879300006,5.2,-3.68430784300001));
#323123=CARTESIAN_POINT('Ctrl Pts',(-1.55048879300006,2.2,-3.68430784300001));
#323124=CARTESIAN_POINT('Ctrl Pts',(-1.55056862800006,12.2,-3.68452294300001));
#323125=CARTESIAN_POINT('Ctrl Pts',(-1.55056862800006,5.2,-3.68452294300001));
#323126=CARTESIAN_POINT('Ctrl Pts',(-1.55056862800006,2.2,-3.68452294300001));
#323127=CARTESIAN_POINT('Ctrl Pts',(-1.55065058700006,12.2,-3.68474467500001));
#323128=CARTESIAN_POINT('Ctrl Pts',(-1.55065058700006,5.2,-3.68474467500001));
#323129=CARTESIAN_POINT('Ctrl Pts',(-1.55065058700006,2.2,-3.68474467500001));
#323130=CARTESIAN_POINT('Ctrl Pts',(-1.55073464700005,12.2,-3.68497302900002));
#323131=CARTESIAN_POINT('Ctrl Pts',(-1.55073464700005,5.2,-3.68497302900002));
#323132=CARTESIAN_POINT('Ctrl Pts',(-1.55073464700005,2.2,-3.68497302900002));
#323133=CARTESIAN_POINT('Ctrl Pts',(-1.55082078700006,12.2,-3.68520799800002));
#323134=CARTESIAN_POINT('Ctrl Pts',(-1.55082078700006,5.2,-3.68520799800002));
#323135=CARTESIAN_POINT('Ctrl Pts',(-1.55082078700006,2.2,-3.68520799800002));
#323136=CARTESIAN_POINT('Ctrl Pts',(-1.55090898200006,12.2,-3.68544957200001));
#323137=CARTESIAN_POINT('Ctrl Pts',(-1.55090898200006,5.2,-3.68544957200001));
#323138=CARTESIAN_POINT('Ctrl Pts',(-1.55090898200006,2.2,-3.68544957200001));
#323139=CARTESIAN_POINT('Ctrl Pts',(-1.55099921200006,12.2,-3.68569774400001));
#323140=CARTESIAN_POINT('Ctrl Pts',(-1.55099921200006,5.2,-3.68569774400001));
#323141=CARTESIAN_POINT('Ctrl Pts',(-1.55099921200006,2.2,-3.68569774400001));
#323142=CARTESIAN_POINT('Ctrl Pts',(-1.55109145400006,12.2,-3.68595250600002));
#323143=CARTESIAN_POINT('Ctrl Pts',(-1.55109145400006,5.2,-3.68595250600002));
#323144=CARTESIAN_POINT('Ctrl Pts',(-1.55109145400006,2.2,-3.68595250600002));
#323145=CARTESIAN_POINT('Ctrl Pts',(-1.55118568700006,12.2,-3.68621384800001));
#323146=CARTESIAN_POINT('Ctrl Pts',(-1.55118568700006,5.2,-3.68621384800001));
#323147=CARTESIAN_POINT('Ctrl Pts',(-1.55118568700006,2.2,-3.68621384800001));
#323148=CARTESIAN_POINT('Ctrl Pts',(-1.55128188600006,12.2,-3.68648176300002));
#323149=CARTESIAN_POINT('Ctrl Pts',(-1.55128188600006,5.2,-3.68648176300002));
#323150=CARTESIAN_POINT('Ctrl Pts',(-1.55128188600006,2.2,-3.68648176300002));
#323151=CARTESIAN_POINT('Ctrl Pts',(-1.55138003100005,12.2,-3.68675624400002));
#323152=CARTESIAN_POINT('Ctrl Pts',(-1.55138003100005,5.2,-3.68675624400002));
#323153=CARTESIAN_POINT('Ctrl Pts',(-1.55138003100005,2.2,-3.68675624400002));
#323154=CARTESIAN_POINT('Ctrl Pts',(-1.55148010000006,12.2,-3.68703728000002));
#323155=CARTESIAN_POINT('Ctrl Pts',(-1.55148010000006,5.2,-3.68703728000002));
#323156=CARTESIAN_POINT('Ctrl Pts',(-1.55148010000006,2.2,-3.68703728000002));
#323157=CARTESIAN_POINT('Ctrl Pts',(-1.55158207100006,12.2,-3.68732486500001));
#323158=CARTESIAN_POINT('Ctrl Pts',(-1.55158207100006,5.2,-3.68732486500001));
#323159=CARTESIAN_POINT('Ctrl Pts',(-1.55158207100006,2.2,-3.68732486500001));
#323160=CARTESIAN_POINT('Ctrl Pts',(-1.55168592200006,12.2,-3.68761899000001));
#323161=CARTESIAN_POINT('Ctrl Pts',(-1.55168592200006,5.2,-3.68761899000001));
#323162=CARTESIAN_POINT('Ctrl Pts',(-1.55168592200006,2.2,-3.68761899000001));
#323163=CARTESIAN_POINT('Ctrl Pts',(-1.55179163200006,12.2,-3.68791964500002));
#323164=CARTESIAN_POINT('Ctrl Pts',(-1.55179163200006,5.2,-3.68791964500002));
#323165=CARTESIAN_POINT('Ctrl Pts',(-1.55179163200006,2.2,-3.68791964500002));
#323166=CARTESIAN_POINT('Ctrl Pts',(-1.55189917800006,12.2,-3.68822682500001));
#323167=CARTESIAN_POINT('Ctrl Pts',(-1.55189917800006,5.2,-3.68822682500001));
#323168=CARTESIAN_POINT('Ctrl Pts',(-1.55189917800006,2.2,-3.68822682500001));
#323169=CARTESIAN_POINT('Ctrl Pts',(-1.55200854000005,12.2,-3.68854051900001));
#323170=CARTESIAN_POINT('Ctrl Pts',(-1.55200854000005,5.2,-3.68854051900001));
#323171=CARTESIAN_POINT('Ctrl Pts',(-1.55200854000005,2.2,-3.68854051900001));
#323172=CARTESIAN_POINT('Ctrl Pts',(-1.55211969500006,12.2,-3.68886072000001));
#323173=CARTESIAN_POINT('Ctrl Pts',(-1.55211969500006,5.2,-3.68886072000001));
#323174=CARTESIAN_POINT('Ctrl Pts',(-1.55211969500006,2.2,-3.68886072000001));
#323175=CARTESIAN_POINT('Ctrl Pts',(-1.55223262400006,12.2,-3.68918742000002));
#323176=CARTESIAN_POINT('Ctrl Pts',(-1.55223262400006,5.2,-3.68918742000002));
#323177=CARTESIAN_POINT('Ctrl Pts',(-1.55223262400006,2.2,-3.68918742000002));
#323178=CARTESIAN_POINT('Ctrl Pts',(-1.55234730400006,12.2,-3.68952060900002));
#323179=CARTESIAN_POINT('Ctrl Pts',(-1.55234730400006,5.2,-3.68952060900002));
#323180=CARTESIAN_POINT('Ctrl Pts',(-1.55234730400006,2.2,-3.68952060900002));
#323181=CARTESIAN_POINT('Ctrl Pts',(-1.55246371400006,12.2,-3.68986028200001));
#323182=CARTESIAN_POINT('Ctrl Pts',(-1.55246371400006,5.2,-3.68986028200001));
#323183=CARTESIAN_POINT('Ctrl Pts',(-1.55246371400006,2.2,-3.68986028200001));
#323184=CARTESIAN_POINT('Ctrl Pts',(-1.55258183200006,12.2,-3.69020642700002));
#323185=CARTESIAN_POINT('Ctrl Pts',(-1.55258183200006,5.2,-3.69020642700002));
#323186=CARTESIAN_POINT('Ctrl Pts',(-1.55258183200006,2.2,-3.69020642700002));
#323187=CARTESIAN_POINT('Ctrl Pts',(-1.55270163900005,12.2,-3.69055903800001));
#323188=CARTESIAN_POINT('Ctrl Pts',(-1.55270163900005,5.2,-3.69055903800001));
#323189=CARTESIAN_POINT('Ctrl Pts',(-1.55270163900005,2.2,-3.69055903800001));
#323190=CARTESIAN_POINT('Ctrl Pts',(-1.55282311500006,12.2,-3.69091810700001));
#323191=CARTESIAN_POINT('Ctrl Pts',(-1.55282311500006,5.2,-3.69091810700001));
#323192=CARTESIAN_POINT('Ctrl Pts',(-1.55282311500006,2.2,-3.69091810700001));
#323193=CARTESIAN_POINT('Ctrl Pts',(-1.55294623500006,12.2,-3.69128362500001));
#323194=CARTESIAN_POINT('Ctrl Pts',(-1.55294623500006,5.2,-3.69128362500001));
#323195=CARTESIAN_POINT('Ctrl Pts',(-1.55294623500006,2.2,-3.69128362500001));
#323196=CARTESIAN_POINT('Ctrl Pts',(-1.55307098100006,12.2,-3.69165558300002));
#323197=CARTESIAN_POINT('Ctrl Pts',(-1.55307098100006,5.2,-3.69165558300002));
#323198=CARTESIAN_POINT('Ctrl Pts',(-1.55307098100006,2.2,-3.69165558300002));
#323199=CARTESIAN_POINT('Ctrl Pts',(-1.55319733200006,12.2,-3.69203397300002));
#323200=CARTESIAN_POINT('Ctrl Pts',(-1.55319733200006,5.2,-3.69203397300002));
#323201=CARTESIAN_POINT('Ctrl Pts',(-1.55319733200006,2.2,-3.69203397300002));
#323202=CARTESIAN_POINT('Ctrl Pts',(-1.55332526700006,12.2,-3.69241878900001));
#323203=CARTESIAN_POINT('Ctrl Pts',(-1.55332526700006,5.2,-3.69241878900001));
#323204=CARTESIAN_POINT('Ctrl Pts',(-1.55332526700006,2.2,-3.69241878900001));
#323205=CARTESIAN_POINT('Ctrl Pts',(-1.55345476600006,12.2,-3.69281002200001));
#323206=CARTESIAN_POINT('Ctrl Pts',(-1.55345476600006,5.2,-3.69281002200001));
#323207=CARTESIAN_POINT('Ctrl Pts',(-1.55345476600006,2.2,-3.69281002200001));
#323208=CARTESIAN_POINT('Ctrl Pts',(-1.55358580700006,12.2,-3.69320766100001));
#323209=CARTESIAN_POINT('Ctrl Pts',(-1.55358580700006,5.2,-3.69320766100001));
#323210=CARTESIAN_POINT('Ctrl Pts',(-1.55358580700006,2.2,-3.69320766100001));
#323211=CARTESIAN_POINT('Ctrl Pts',(-1.55371837200006,12.2,-3.69361170100001));
#323212=CARTESIAN_POINT('Ctrl Pts',(-1.55371837200006,5.2,-3.69361170100001));
#323213=CARTESIAN_POINT('Ctrl Pts',(-1.55371837200006,2.2,-3.69361170100001));
#323214=CARTESIAN_POINT('Ctrl Pts',(-1.55385243800006,12.2,-3.69402213200001));
#323215=CARTESIAN_POINT('Ctrl Pts',(-1.55385243800006,5.2,-3.69402213200001));
#323216=CARTESIAN_POINT('Ctrl Pts',(-1.55385243800006,2.2,-3.69402213200001));
#323217=CARTESIAN_POINT('Ctrl Pts',(-1.55398798700006,12.2,-3.69443894600002));
#323218=CARTESIAN_POINT('Ctrl Pts',(-1.55398798700006,5.2,-3.69443894600002));
#323219=CARTESIAN_POINT('Ctrl Pts',(-1.55398798700006,2.2,-3.69443894600002));
#323220=CARTESIAN_POINT('Ctrl Pts',(-1.55412499800006,12.2,-3.69486213600001));
#323221=CARTESIAN_POINT('Ctrl Pts',(-1.55412499800006,5.2,-3.69486213600001));
#323222=CARTESIAN_POINT('Ctrl Pts',(-1.55412499800006,2.2,-3.69486213600001));
#323223=CARTESIAN_POINT('Ctrl Pts',(-1.55426345100006,12.2,-3.69529169300002));
#323224=CARTESIAN_POINT('Ctrl Pts',(-1.55426345100006,5.2,-3.69529169300002));
#323225=CARTESIAN_POINT('Ctrl Pts',(-1.55426345100006,2.2,-3.69529169300002));
#323226=CARTESIAN_POINT('Ctrl Pts',(-1.55440332500006,12.2,-3.69572760900001));
#323227=CARTESIAN_POINT('Ctrl Pts',(-1.55440332500006,5.2,-3.69572760900001));
#323228=CARTESIAN_POINT('Ctrl Pts',(-1.55440332500006,2.2,-3.69572760900001));
#323229=CARTESIAN_POINT('Ctrl Pts',(-1.55454460100006,12.2,-3.69616987500001));
#323230=CARTESIAN_POINT('Ctrl Pts',(-1.55454460100006,5.2,-3.69616987500001));
#323231=CARTESIAN_POINT('Ctrl Pts',(-1.55454460100006,2.2,-3.69616987500001));
#323232=CARTESIAN_POINT('Ctrl Pts',(-1.55468726000006,12.2,-3.69661848400002));
#323233=CARTESIAN_POINT('Ctrl Pts',(-1.55468726000006,5.2,-3.69661848400002));
#323234=CARTESIAN_POINT('Ctrl Pts',(-1.55468726000006,2.2,-3.69661848400002));
#323235=CARTESIAN_POINT('Ctrl Pts',(-1.55483128000005,12.2,-3.69707342600002));
#323236=CARTESIAN_POINT('Ctrl Pts',(-1.55483128000005,5.2,-3.69707342600002));
#323237=CARTESIAN_POINT('Ctrl Pts',(-1.55483128000005,2.2,-3.69707342600002));
#323238=CARTESIAN_POINT('Ctrl Pts',(-1.55497664300006,12.2,-3.69753469500001));
#323239=CARTESIAN_POINT('Ctrl Pts',(-1.55497664300006,5.2,-3.69753469500001));
#323240=CARTESIAN_POINT('Ctrl Pts',(-1.55497664300006,2.2,-3.69753469500001));
#323241=CARTESIAN_POINT('Ctrl Pts',(-1.55512332800006,12.2,-3.69800228200001));
#323242=CARTESIAN_POINT('Ctrl Pts',(-1.55512332800006,5.2,-3.69800228200001));
#323243=CARTESIAN_POINT('Ctrl Pts',(-1.55512332800006,2.2,-3.69800228200001));
#323244=CARTESIAN_POINT('Ctrl Pts',(-1.55527131700006,12.2,-3.69847617800001));
#323245=CARTESIAN_POINT('Ctrl Pts',(-1.55527131700006,5.2,-3.69847617800001));
#323246=CARTESIAN_POINT('Ctrl Pts',(-1.55527131700006,2.2,-3.69847617800001));
#323247=CARTESIAN_POINT('Ctrl Pts',(-1.55542058900005,12.2,-3.69895637600001));
#323248=CARTESIAN_POINT('Ctrl Pts',(-1.55542058900005,5.2,-3.69895637600001));
#323249=CARTESIAN_POINT('Ctrl Pts',(-1.55542058900005,2.2,-3.69895637600001));
#323250=CARTESIAN_POINT('Ctrl Pts',(-1.55557112500006,12.2,-3.69944286800001));
#323251=CARTESIAN_POINT('Ctrl Pts',(-1.55557112500006,5.2,-3.69944286800001));
#323252=CARTESIAN_POINT('Ctrl Pts',(-1.55557112500006,2.2,-3.69944286800001));
#323253=CARTESIAN_POINT('Ctrl Pts',(-1.55572290600006,12.2,-3.69993564400001));
#323254=CARTESIAN_POINT('Ctrl Pts',(-1.55572290600006,5.2,-3.69993564400001));
#323255=CARTESIAN_POINT('Ctrl Pts',(-1.55572290600006,2.2,-3.69993564400001));
#323256=CARTESIAN_POINT('Ctrl Pts',(-1.55587591300006,12.2,-3.70043469700001));
#323257=CARTESIAN_POINT('Ctrl Pts',(-1.55587591300006,5.2,-3.70043469700001));
#323258=CARTESIAN_POINT('Ctrl Pts',(-1.55587591300006,2.2,-3.70043469700001));
#323259=CARTESIAN_POINT('Ctrl Pts',(-1.55603012600006,12.2,-3.70094001900001));
#323260=CARTESIAN_POINT('Ctrl Pts',(-1.55603012600006,5.2,-3.70094001900001));
#323261=CARTESIAN_POINT('Ctrl Pts',(-1.55603012600006,2.2,-3.70094001900001));
#323262=CARTESIAN_POINT('Ctrl Pts',(-1.55618552500006,12.2,-3.70145160200002));
#323263=CARTESIAN_POINT('Ctrl Pts',(-1.55618552500006,5.2,-3.70145160200002));
#323264=CARTESIAN_POINT('Ctrl Pts',(-1.55618552500006,2.2,-3.70145160200002));
#323265=CARTESIAN_POINT('Ctrl Pts',(-1.55634209300006,12.2,-3.70196943800002));
#323266=CARTESIAN_POINT('Ctrl Pts',(-1.55634209300006,5.2,-3.70196943800002));
#323267=CARTESIAN_POINT('Ctrl Pts',(-1.55634209300006,2.2,-3.70196943800002));
#323268=CARTESIAN_POINT('Ctrl Pts',(-1.55649981000006,12.2,-3.70249351700001));
#323269=CARTESIAN_POINT('Ctrl Pts',(-1.55649981000006,5.2,-3.70249351700001));
#323270=CARTESIAN_POINT('Ctrl Pts',(-1.55649981000006,2.2,-3.70249351700001));
#323271=CARTESIAN_POINT('Ctrl Pts',(-1.55665865600006,12.2,-3.70302383400002));
#323272=CARTESIAN_POINT('Ctrl Pts',(-1.55665865600006,5.2,-3.70302383400002));
#323273=CARTESIAN_POINT('Ctrl Pts',(-1.55665865600006,2.2,-3.70302383400002));
#323274=CARTESIAN_POINT('Ctrl Pts',(-1.55681861300006,12.2,-3.70356037800001));
#323275=CARTESIAN_POINT('Ctrl Pts',(-1.55681861300006,5.2,-3.70356037800001));
#323276=CARTESIAN_POINT('Ctrl Pts',(-1.55681861300006,2.2,-3.70356037800001));
#323277=CARTESIAN_POINT('Ctrl Pts',(-1.55697966300006,12.2,-3.70410314200001));
#323278=CARTESIAN_POINT('Ctrl Pts',(-1.55697966300006,5.2,-3.70410314200001));
#323279=CARTESIAN_POINT('Ctrl Pts',(-1.55697966300006,2.2,-3.70410314200001));
#323280=CARTESIAN_POINT('Ctrl Pts',(-1.55714178500005,12.2,-3.70465211700001));
#323281=CARTESIAN_POINT('Ctrl Pts',(-1.55714178500005,5.2,-3.70465211700001));
#323282=CARTESIAN_POINT('Ctrl Pts',(-1.55714178500005,2.2,-3.70465211700001));
#323283=CARTESIAN_POINT('Ctrl Pts',(-1.55730496200006,12.2,-3.70520729600001));
#323284=CARTESIAN_POINT('Ctrl Pts',(-1.55730496200006,5.2,-3.70520729600001));
#323285=CARTESIAN_POINT('Ctrl Pts',(-1.55730496200006,2.2,-3.70520729600001));
#323286=CARTESIAN_POINT('Ctrl Pts',(-1.55746917600006,12.2,-3.70576867200001));
#323287=CARTESIAN_POINT('Ctrl Pts',(-1.55746917600006,5.2,-3.70576867200001));
#323288=CARTESIAN_POINT('Ctrl Pts',(-1.55746917600006,2.2,-3.70576867200001));
#323289=CARTESIAN_POINT('Ctrl Pts',(-1.55763440700006,12.2,-3.70633623300002));
#323290=CARTESIAN_POINT('Ctrl Pts',(-1.55763440700006,5.2,-3.70633623300002));
#323291=CARTESIAN_POINT('Ctrl Pts',(-1.55763440700006,2.2,-3.70633623300002));
#323292=CARTESIAN_POINT('Ctrl Pts',(-1.55780063700006,12.2,-3.70690997500001));
#323293=CARTESIAN_POINT('Ctrl Pts',(-1.55780063700006,5.2,-3.70690997500001));
#323294=CARTESIAN_POINT('Ctrl Pts',(-1.55780063700006,2.2,-3.70690997500001));
#323295=CARTESIAN_POINT('Ctrl Pts',(-1.55796784700006,12.2,-3.70748988700001));
#323296=CARTESIAN_POINT('Ctrl Pts',(-1.55796784700006,5.2,-3.70748988700001));
#323297=CARTESIAN_POINT('Ctrl Pts',(-1.55796784700006,2.2,-3.70748988700001));
#323298=CARTESIAN_POINT('Ctrl Pts',(-1.55813601900005,12.2,-3.70807596300001));
#323299=CARTESIAN_POINT('Ctrl Pts',(-1.55813601900005,5.2,-3.70807596300001));
#323300=CARTESIAN_POINT('Ctrl Pts',(-1.55813601900005,2.2,-3.70807596300001));
#323301=CARTESIAN_POINT('Ctrl Pts',(-1.55830513500006,12.2,-3.70866819300002));
#323302=CARTESIAN_POINT('Ctrl Pts',(-1.55830513500006,5.2,-3.70866819300002));
#323303=CARTESIAN_POINT('Ctrl Pts',(-1.55830513500006,2.2,-3.70866819300002));
#323304=CARTESIAN_POINT('Ctrl Pts',(-1.55847517600006,12.2,-3.70926657000001));
#323305=CARTESIAN_POINT('Ctrl Pts',(-1.55847517600006,5.2,-3.70926657000001));
#323306=CARTESIAN_POINT('Ctrl Pts',(-1.55847517600006,2.2,-3.70926657000001));
#323307=CARTESIAN_POINT('Ctrl Pts',(-1.55864612500005,12.2,-3.70987108600001));
#323308=CARTESIAN_POINT('Ctrl Pts',(-1.55864612500005,5.2,-3.70987108600001));
#323309=CARTESIAN_POINT('Ctrl Pts',(-1.55864612500005,2.2,-3.70987108600001));
#323310=CARTESIAN_POINT('Ctrl Pts',(-1.55881796400006,12.2,-3.71048173200001));
#323311=CARTESIAN_POINT('Ctrl Pts',(-1.55881796400006,5.2,-3.71048173200001));
#323312=CARTESIAN_POINT('Ctrl Pts',(-1.55881796400006,2.2,-3.71048173200001));
#323313=CARTESIAN_POINT('Ctrl Pts',(-1.55899067400005,12.2,-3.71109850100002));
#323314=CARTESIAN_POINT('Ctrl Pts',(-1.55899067400005,5.2,-3.71109850100002));
#323315=CARTESIAN_POINT('Ctrl Pts',(-1.55899067400005,2.2,-3.71109850100002));
#323316=CARTESIAN_POINT('Ctrl Pts',(-1.55916423600006,12.2,-3.71172138300001));
#323317=CARTESIAN_POINT('Ctrl Pts',(-1.55916423600006,5.2,-3.71172138300001));
#323318=CARTESIAN_POINT('Ctrl Pts',(-1.55916423600006,2.2,-3.71172138300001));
#323319=CARTESIAN_POINT('Ctrl Pts',(-1.55933863300006,12.2,-3.71235037100002));
#323320=CARTESIAN_POINT('Ctrl Pts',(-1.55933863300006,5.2,-3.71235037100002));
#323321=CARTESIAN_POINT('Ctrl Pts',(-1.55933863300006,2.2,-3.71235037100002));
#323322=CARTESIAN_POINT('Ctrl Pts',(-1.55951384900006,12.2,-3.71298545800002));
#323323=CARTESIAN_POINT('Ctrl Pts',(-1.55951384900006,5.2,-3.71298545800002));
#323324=CARTESIAN_POINT('Ctrl Pts',(-1.55951384900006,2.2,-3.71298545800002));
#323325=CARTESIAN_POINT('Ctrl Pts',(-1.55968986300006,12.2,-3.71362663500001));
#323326=CARTESIAN_POINT('Ctrl Pts',(-1.55968986300006,5.2,-3.71362663500001));
#323327=CARTESIAN_POINT('Ctrl Pts',(-1.55968986300006,2.2,-3.71362663500001));
#323328=CARTESIAN_POINT('Ctrl Pts',(-1.55986666000006,12.2,-3.71427389300001));
#323329=CARTESIAN_POINT('Ctrl Pts',(-1.55986666000006,5.2,-3.71427389300001));
#323330=CARTESIAN_POINT('Ctrl Pts',(-1.55986666000006,2.2,-3.71427389300001));
#323331=CARTESIAN_POINT('Ctrl Pts',(-1.56004422000006,12.2,-3.71492722500002));
#323332=CARTESIAN_POINT('Ctrl Pts',(-1.56004422000006,5.2,-3.71492722500002));
#323333=CARTESIAN_POINT('Ctrl Pts',(-1.56004422000006,2.2,-3.71492722500002));
#323334=CARTESIAN_POINT('Ctrl Pts',(-1.56022252800006,12.2,-3.71558662200002));
#323335=CARTESIAN_POINT('Ctrl Pts',(-1.56022252800006,5.2,-3.71558662200002));
#323336=CARTESIAN_POINT('Ctrl Pts',(-1.56022252800006,2.2,-3.71558662200002));
#323337=CARTESIAN_POINT('Ctrl Pts',(-1.56040156400006,12.2,-3.71625207700002));
#323338=CARTESIAN_POINT('Ctrl Pts',(-1.56040156400006,5.2,-3.71625207700002));
#323339=CARTESIAN_POINT('Ctrl Pts',(-1.56040156400006,2.2,-3.71625207700002));
#323340=CARTESIAN_POINT('Ctrl Pts',(-1.56058131100006,12.2,-3.71692358100002));
#323341=CARTESIAN_POINT('Ctrl Pts',(-1.56058131100006,5.2,-3.71692358100002));
#323342=CARTESIAN_POINT('Ctrl Pts',(-1.56058131100006,2.2,-3.71692358100002));
#323343=CARTESIAN_POINT('Ctrl Pts',(-1.56076175300006,12.2,-3.71760112700001));
#323344=CARTESIAN_POINT('Ctrl Pts',(-1.56076175300006,5.2,-3.71760112700001));
#323345=CARTESIAN_POINT('Ctrl Pts',(-1.56076175300006,2.2,-3.71760112700001));
#323346=CARTESIAN_POINT('Ctrl Pts',(-1.56094287100006,12.2,-3.71828470600001));
#323347=CARTESIAN_POINT('Ctrl Pts',(-1.56094287100006,5.2,-3.71828470600001));
#323348=CARTESIAN_POINT('Ctrl Pts',(-1.56094287100006,2.2,-3.71828470600001));
#323349=CARTESIAN_POINT('Ctrl Pts',(-1.56112464800006,12.2,-3.71897431000002));
#323350=CARTESIAN_POINT('Ctrl Pts',(-1.56112464800006,5.2,-3.71897431000002));
#323351=CARTESIAN_POINT('Ctrl Pts',(-1.56112464800006,2.2,-3.71897431000002));
#323352=CARTESIAN_POINT('Ctrl Pts',(-1.56130706700006,12.2,-3.71966993000001));
#323353=CARTESIAN_POINT('Ctrl Pts',(-1.56130706700006,5.2,-3.71966993000001));
#323354=CARTESIAN_POINT('Ctrl Pts',(-1.56130706700006,2.2,-3.71966993000001));
#323355=CARTESIAN_POINT('Ctrl Pts',(-1.56149011100006,12.2,-3.72037156100001));
#323356=CARTESIAN_POINT('Ctrl Pts',(-1.56149011100006,5.2,-3.72037156100001));
#323357=CARTESIAN_POINT('Ctrl Pts',(-1.56149011100006,2.2,-3.72037156100001));
#323358=CARTESIAN_POINT('Ctrl Pts',(-1.56167376300006,12.2,-3.72107919100001));
#323359=CARTESIAN_POINT('Ctrl Pts',(-1.56167376300006,5.2,-3.72107919100001));
#323360=CARTESIAN_POINT('Ctrl Pts',(-1.56167376300006,2.2,-3.72107919100001));
#323361=CARTESIAN_POINT('Ctrl Pts',(-1.56185800400006,12.2,-3.72179281400001));
#323362=CARTESIAN_POINT('Ctrl Pts',(-1.56185800400006,5.2,-3.72179281400001));
#323363=CARTESIAN_POINT('Ctrl Pts',(-1.56185800400006,2.2,-3.72179281400001));
#323364=CARTESIAN_POINT('Ctrl Pts',(-1.56204282100005,12.2,-3.72251242200001));
#323365=CARTESIAN_POINT('Ctrl Pts',(-1.56204282100005,5.2,-3.72251242200001));
#323366=CARTESIAN_POINT('Ctrl Pts',(-1.56204282100005,2.2,-3.72251242200001));
#323367=CARTESIAN_POINT('Ctrl Pts',(-1.56222819300006,12.2,-3.72323800600002));
#323368=CARTESIAN_POINT('Ctrl Pts',(-1.56222819300006,5.2,-3.72323800600002));
#323369=CARTESIAN_POINT('Ctrl Pts',(-1.56222819300006,2.2,-3.72323800600002));
#323370=CARTESIAN_POINT('Ctrl Pts',(-1.56241410500006,12.2,-3.72396955900001));
#323371=CARTESIAN_POINT('Ctrl Pts',(-1.56241410500006,5.2,-3.72396955900001));
#323372=CARTESIAN_POINT('Ctrl Pts',(-1.56241410500006,2.2,-3.72396955900001));
#323373=CARTESIAN_POINT('Ctrl Pts',(-1.56260053900006,12.2,-3.72470707300002));
#323374=CARTESIAN_POINT('Ctrl Pts',(-1.56260053900006,5.2,-3.72470707300002));
#323375=CARTESIAN_POINT('Ctrl Pts',(-1.56260053900006,2.2,-3.72470707300002));
#323376=CARTESIAN_POINT('Ctrl Pts',(-1.56278748000006,12.2,-3.72545053900001));
#323377=CARTESIAN_POINT('Ctrl Pts',(-1.56278748000006,5.2,-3.72545053900001));
#323378=CARTESIAN_POINT('Ctrl Pts',(-1.56278748000006,2.2,-3.72545053900001));
#323379=CARTESIAN_POINT('Ctrl Pts',(-1.56297490900006,12.2,-3.72619994800001));
#323380=CARTESIAN_POINT('Ctrl Pts',(-1.56297490900006,5.2,-3.72619994800001));
#323381=CARTESIAN_POINT('Ctrl Pts',(-1.56297490900006,2.2,-3.72619994800001));
#323382=CARTESIAN_POINT('Ctrl Pts',(-1.56316281100006,12.2,-3.72695529500001));
#323383=CARTESIAN_POINT('Ctrl Pts',(-1.56316281100006,5.2,-3.72695529500001));
#323384=CARTESIAN_POINT('Ctrl Pts',(-1.56316281100006,2.2,-3.72695529500001));
#323385=CARTESIAN_POINT('Ctrl Pts',(-1.56335117000005,12.2,-3.72771656800001));
#323386=CARTESIAN_POINT('Ctrl Pts',(-1.56335117000005,5.2,-3.72771656800001));
#323387=CARTESIAN_POINT('Ctrl Pts',(-1.56335117000005,2.2,-3.72771656800001));
#323388=CARTESIAN_POINT('Ctrl Pts',(-1.56353996800006,12.2,-3.72848376400002));
#323389=CARTESIAN_POINT('Ctrl Pts',(-1.56353996800006,5.2,-3.72848376400002));
#323390=CARTESIAN_POINT('Ctrl Pts',(-1.56353996800006,2.2,-3.72848376400002));
#323391=CARTESIAN_POINT('Ctrl Pts',(-1.56372918800006,12.2,-3.72925687000001));
#323392=CARTESIAN_POINT('Ctrl Pts',(-1.56372918800006,5.2,-3.72925687000001));
#323393=CARTESIAN_POINT('Ctrl Pts',(-1.56372918800006,2.2,-3.72925687000001));
#323394=CARTESIAN_POINT('Ctrl Pts',(-1.56391881500005,12.2,-3.73003588000001));
#323395=CARTESIAN_POINT('Ctrl Pts',(-1.56391881500005,5.2,-3.73003588000001));
#323396=CARTESIAN_POINT('Ctrl Pts',(-1.56391881500005,2.2,-3.73003588000001));
#323397=CARTESIAN_POINT('Ctrl Pts',(-1.56410883100006,12.2,-3.73082078600001));
#323398=CARTESIAN_POINT('Ctrl Pts',(-1.56410883100006,5.2,-3.73082078600001));
#323399=CARTESIAN_POINT('Ctrl Pts',(-1.56410883100006,2.2,-3.73082078600001));
#323400=CARTESIAN_POINT('Ctrl Pts',(-1.56429922100006,12.2,-3.73161158000002));
#323401=CARTESIAN_POINT('Ctrl Pts',(-1.56429922100006,5.2,-3.73161158000002));
#323402=CARTESIAN_POINT('Ctrl Pts',(-1.56429922100006,2.2,-3.73161158000002));
#323403=CARTESIAN_POINT('Ctrl Pts',(-1.56448996900005,12.2,-3.73240825400002));
#323404=CARTESIAN_POINT('Ctrl Pts',(-1.56448996900005,5.2,-3.73240825400002));
#323405=CARTESIAN_POINT('Ctrl Pts',(-1.56448996900005,2.2,-3.73240825400002));
#323406=CARTESIAN_POINT('Ctrl Pts',(-1.56468105700006,12.2,-3.73321079900002));
#323407=CARTESIAN_POINT('Ctrl Pts',(-1.56468105700006,5.2,-3.73321079900002));
#323408=CARTESIAN_POINT('Ctrl Pts',(-1.56468105700006,2.2,-3.73321079900002));
#323409=CARTESIAN_POINT('Ctrl Pts',(-1.56487247100005,12.2,-3.73401920800001));
#323410=CARTESIAN_POINT('Ctrl Pts',(-1.56487247100005,5.2,-3.73401920800001));
#323411=CARTESIAN_POINT('Ctrl Pts',(-1.56487247100005,2.2,-3.73401920800001));
#323412=CARTESIAN_POINT('Ctrl Pts',(-1.56506419200006,12.2,-3.73483347200001));
#323413=CARTESIAN_POINT('Ctrl Pts',(-1.56506419200006,5.2,-3.73483347200001));
#323414=CARTESIAN_POINT('Ctrl Pts',(-1.56506419200006,2.2,-3.73483347200001));
#323415=CARTESIAN_POINT('Ctrl Pts',(-1.56525620700006,12.2,-3.73565358500001));
#323416=CARTESIAN_POINT('Ctrl Pts',(-1.56525620700006,5.2,-3.73565358500001));
#323417=CARTESIAN_POINT('Ctrl Pts',(-1.56525620700006,2.2,-3.73565358500001));
#323418=CARTESIAN_POINT('Ctrl Pts',(-1.56544849800006,12.2,-3.73647953600001));
#323419=CARTESIAN_POINT('Ctrl Pts',(-1.56544849800006,5.2,-3.73647953600001));
#323420=CARTESIAN_POINT('Ctrl Pts',(-1.56544849800006,2.2,-3.73647953600001));
#323421=CARTESIAN_POINT('Ctrl Pts',(-1.56564104900006,12.2,-3.73731132000001));
#323422=CARTESIAN_POINT('Ctrl Pts',(-1.56564104900006,5.2,-3.73731132000001));
#323423=CARTESIAN_POINT('Ctrl Pts',(-1.56564104900006,2.2,-3.73731132000001));
#323424=CARTESIAN_POINT('Ctrl Pts',(-1.56583384600005,12.2,-3.73814892600001));
#323425=CARTESIAN_POINT('Ctrl Pts',(-1.56583384600005,5.2,-3.73814892600001));
#323426=CARTESIAN_POINT('Ctrl Pts',(-1.56583384600005,2.2,-3.73814892600001));
#323427=CARTESIAN_POINT('Ctrl Pts',(-1.56602687100006,12.2,-3.73899234800001));
#323428=CARTESIAN_POINT('Ctrl Pts',(-1.56602687100006,5.2,-3.73899234800001));
#323429=CARTESIAN_POINT('Ctrl Pts',(-1.56602687100006,2.2,-3.73899234800001));
#323430=CARTESIAN_POINT('Ctrl Pts',(-1.56622010900006,12.2,-3.73984157700002));
#323431=CARTESIAN_POINT('Ctrl Pts',(-1.56622010900006,5.2,-3.73984157700002));
#323432=CARTESIAN_POINT('Ctrl Pts',(-1.56622010900006,2.2,-3.73984157700002));
#323433=CARTESIAN_POINT('Ctrl Pts',(-1.56641354400006,12.2,-3.74069660600002));
#323434=CARTESIAN_POINT('Ctrl Pts',(-1.56641354400006,5.2,-3.74069660600002));
#323435=CARTESIAN_POINT('Ctrl Pts',(-1.56641354400006,2.2,-3.74069660600002));
#323436=CARTESIAN_POINT('Ctrl Pts',(-1.56660716100005,12.2,-3.74155742600002));
#323437=CARTESIAN_POINT('Ctrl Pts',(-1.56660716100005,5.2,-3.74155742600002));
#323438=CARTESIAN_POINT('Ctrl Pts',(-1.56660716100005,2.2,-3.74155742600002));
#323439=CARTESIAN_POINT('Ctrl Pts',(-1.56680094400006,12.2,-3.74242402900002));
#323440=CARTESIAN_POINT('Ctrl Pts',(-1.56680094400006,5.2,-3.74242402900002));
#323441=CARTESIAN_POINT('Ctrl Pts',(-1.56680094400006,2.2,-3.74242402900002));
#323442=CARTESIAN_POINT('Ctrl Pts',(-1.56699487700006,12.2,-3.74329640700001));
#323443=CARTESIAN_POINT('Ctrl Pts',(-1.56699487700006,5.2,-3.74329640700001));
#323444=CARTESIAN_POINT('Ctrl Pts',(-1.56699487700006,2.2,-3.74329640700001));
#323445=CARTESIAN_POINT('Ctrl Pts',(-1.56718894400006,12.2,-3.74417455200001));
#323446=CARTESIAN_POINT('Ctrl Pts',(-1.56718894400006,5.2,-3.74417455200001));
#323447=CARTESIAN_POINT('Ctrl Pts',(-1.56718894400006,2.2,-3.74417455200001));
#323448=CARTESIAN_POINT('Ctrl Pts',(-1.56738313100006,12.2,-3.74505845700002));
#323449=CARTESIAN_POINT('Ctrl Pts',(-1.56738313100006,5.2,-3.74505845700002));
#323450=CARTESIAN_POINT('Ctrl Pts',(-1.56738313100006,2.2,-3.74505845700002));
#323451=CARTESIAN_POINT('Ctrl Pts',(-1.56757742100006,12.2,-3.74594811200001));
#323452=CARTESIAN_POINT('Ctrl Pts',(-1.56757742100006,5.2,-3.74594811200001));
#323453=CARTESIAN_POINT('Ctrl Pts',(-1.56757742100006,2.2,-3.74594811200001));
#323454=CARTESIAN_POINT('Ctrl Pts',(-1.56777179900006,12.2,-3.74684351100001));
#323455=CARTESIAN_POINT('Ctrl Pts',(-1.56777179900006,5.2,-3.74684351100001));
#323456=CARTESIAN_POINT('Ctrl Pts',(-1.56777179900006,2.2,-3.74684351100001));
#323457=CARTESIAN_POINT('Ctrl Pts',(-1.56796625000006,12.2,-3.74774464500002));
#323458=CARTESIAN_POINT('Ctrl Pts',(-1.56796625000006,5.2,-3.74774464500002));
#323459=CARTESIAN_POINT('Ctrl Pts',(-1.56796625000006,2.2,-3.74774464500002));
#323460=CARTESIAN_POINT('Ctrl Pts',(-1.56816076000006,12.2,-3.74865150500002));
#323461=CARTESIAN_POINT('Ctrl Pts',(-1.56816076000006,5.2,-3.74865150500002));
#323462=CARTESIAN_POINT('Ctrl Pts',(-1.56816076000006,2.2,-3.74865150500002));
#323463=CARTESIAN_POINT('Ctrl Pts',(-1.56835531100006,12.2,-3.74956408500001));
#323464=CARTESIAN_POINT('Ctrl Pts',(-1.56835531100006,5.2,-3.74956408500001));
#323465=CARTESIAN_POINT('Ctrl Pts',(-1.56835531100006,2.2,-3.74956408500001));
#323466=CARTESIAN_POINT('Ctrl Pts',(-1.56854988800006,12.2,-3.75048237600001));
#323467=CARTESIAN_POINT('Ctrl Pts',(-1.56854988800006,5.2,-3.75048237600001));
#323468=CARTESIAN_POINT('Ctrl Pts',(-1.56854988800006,2.2,-3.75048237600001));
#323469=CARTESIAN_POINT('Ctrl Pts',(-1.56874447900006,12.2,-3.75140637000001));
#323470=CARTESIAN_POINT('Ctrl Pts',(-1.56874447900006,5.2,-3.75140637000001));
#323471=CARTESIAN_POINT('Ctrl Pts',(-1.56874447900006,2.2,-3.75140637000001));
#323472=CARTESIAN_POINT('Ctrl Pts',(-1.56893906600006,12.2,-3.75233605800001));
#323473=CARTESIAN_POINT('Ctrl Pts',(-1.56893906600006,5.2,-3.75233605800001));
#323474=CARTESIAN_POINT('Ctrl Pts',(-1.56893906600006,2.2,-3.75233605800001));
#323475=CARTESIAN_POINT('Ctrl Pts',(-1.56913363400006,12.2,-3.75327143400002));
#323476=CARTESIAN_POINT('Ctrl Pts',(-1.56913363400006,5.2,-3.75327143400002));
#323477=CARTESIAN_POINT('Ctrl Pts',(-1.56913363400006,2.2,-3.75327143400002));
#323478=CARTESIAN_POINT('Ctrl Pts',(-1.56932817100006,12.2,-3.75421248800002));
#323479=CARTESIAN_POINT('Ctrl Pts',(-1.56932817100006,5.2,-3.75421248800002));
#323480=CARTESIAN_POINT('Ctrl Pts',(-1.56932817100006,2.2,-3.75421248800002));
#323481=CARTESIAN_POINT('Ctrl Pts',(-1.56952265800005,12.2,-3.75515921400002));
#323482=CARTESIAN_POINT('Ctrl Pts',(-1.56952265800005,5.2,-3.75515921400002));
#323483=CARTESIAN_POINT('Ctrl Pts',(-1.56952265800005,2.2,-3.75515921400002));
#323484=CARTESIAN_POINT('Ctrl Pts',(-1.56971708200006,12.2,-3.75611160200001));
#323485=CARTESIAN_POINT('Ctrl Pts',(-1.56971708200006,5.2,-3.75611160200001));
#323486=CARTESIAN_POINT('Ctrl Pts',(-1.56971708200006,2.2,-3.75611160200001));
#323487=CARTESIAN_POINT('Ctrl Pts',(-1.56991142900006,12.2,-3.75706964400001));
#323488=CARTESIAN_POINT('Ctrl Pts',(-1.56991142900006,5.2,-3.75706964400001));
#323489=CARTESIAN_POINT('Ctrl Pts',(-1.56991142900006,2.2,-3.75706964400001));
#323490=CARTESIAN_POINT('Ctrl Pts',(-1.57010568200006,12.2,-3.75803333400002));
#323491=CARTESIAN_POINT('Ctrl Pts',(-1.57010568200006,5.2,-3.75803333400002));
#323492=CARTESIAN_POINT('Ctrl Pts',(-1.57010568200006,2.2,-3.75803333400002));
#323493=CARTESIAN_POINT('Ctrl Pts',(-1.57029982900006,12.2,-3.75900266300001));
#323494=CARTESIAN_POINT('Ctrl Pts',(-1.57029982900006,5.2,-3.75900266300001));
#323495=CARTESIAN_POINT('Ctrl Pts',(-1.57029982900006,2.2,-3.75900266300001));
#323496=CARTESIAN_POINT('Ctrl Pts',(-1.57049385200006,12.2,-3.75997762300001));
#323497=CARTESIAN_POINT('Ctrl Pts',(-1.57049385200006,5.2,-3.75997762300001));
#323498=CARTESIAN_POINT('Ctrl Pts',(-1.57049385200006,2.2,-3.75997762300001));
#323499=CARTESIAN_POINT('Ctrl Pts',(-1.57068773900006,12.2,-3.76095820600002));
#323500=CARTESIAN_POINT('Ctrl Pts',(-1.57068773900006,5.2,-3.76095820600002));
#323501=CARTESIAN_POINT('Ctrl Pts',(-1.57068773900006,2.2,-3.76095820600002));
#323502=CARTESIAN_POINT('Ctrl Pts',(-1.57088147400006,12.2,-3.76194440300001));
#323503=CARTESIAN_POINT('Ctrl Pts',(-1.57088147400006,5.2,-3.76194440300001));
#323504=CARTESIAN_POINT('Ctrl Pts',(-1.57088147400006,2.2,-3.76194440300001));
#323505=CARTESIAN_POINT('Ctrl Pts',(-1.57107504200006,12.2,-3.76293620800002));
#323506=CARTESIAN_POINT('Ctrl Pts',(-1.57107504200006,5.2,-3.76293620800002));
#323507=CARTESIAN_POINT('Ctrl Pts',(-1.57107504200006,2.2,-3.76293620800002));
#323508=CARTESIAN_POINT('Ctrl Pts',(-1.57126843100006,12.2,-3.76393361100002));
#323509=CARTESIAN_POINT('Ctrl Pts',(-1.57126843100006,5.2,-3.76393361100002));
#323510=CARTESIAN_POINT('Ctrl Pts',(-1.57126843100006,2.2,-3.76393361100002));
#323511=CARTESIAN_POINT('Ctrl Pts',(-1.57146162400006,12.2,-3.76493660500001));
#323512=CARTESIAN_POINT('Ctrl Pts',(-1.57146162400006,5.2,-3.76493660500001));
#323513=CARTESIAN_POINT('Ctrl Pts',(-1.57146162400006,2.2,-3.76493660500001));
#323514=CARTESIAN_POINT('Ctrl Pts',(-1.57165460600006,12.2,-3.76594518200001));
#323515=CARTESIAN_POINT('Ctrl Pts',(-1.57165460600006,5.2,-3.76594518200001));
#323516=CARTESIAN_POINT('Ctrl Pts',(-1.57165460600006,2.2,-3.76594518200001));
#323517=CARTESIAN_POINT('Ctrl Pts',(-1.57184736600006,12.2,-3.76695933400002));
#323518=CARTESIAN_POINT('Ctrl Pts',(-1.57184736600006,5.2,-3.76695933400002));
#323519=CARTESIAN_POINT('Ctrl Pts',(-1.57184736600006,2.2,-3.76695933400002));
#323520=CARTESIAN_POINT('Ctrl Pts',(-1.57203988700006,12.2,-3.76797905300001));
#323521=CARTESIAN_POINT('Ctrl Pts',(-1.57203988700006,5.2,-3.76797905300001));
#323522=CARTESIAN_POINT('Ctrl Pts',(-1.57203988700006,2.2,-3.76797905300001));
#323523=CARTESIAN_POINT('Ctrl Pts',(-1.57223215400006,12.2,-3.76900433100001));
#323524=CARTESIAN_POINT('Ctrl Pts',(-1.57223215400006,5.2,-3.76900433100001));
#323525=CARTESIAN_POINT('Ctrl Pts',(-1.57223215400006,2.2,-3.76900433100001));
#323526=CARTESIAN_POINT('Ctrl Pts',(-1.57242415500006,12.2,-3.77003516000002));
#323527=CARTESIAN_POINT('Ctrl Pts',(-1.57242415500006,5.2,-3.77003516000002));
#323528=CARTESIAN_POINT('Ctrl Pts',(-1.57242415500006,2.2,-3.77003516000002));
#323529=CARTESIAN_POINT('Ctrl Pts',(-1.57261587600006,12.2,-3.77107153100001));
#323530=CARTESIAN_POINT('Ctrl Pts',(-1.57261587600006,5.2,-3.77107153100001));
#323531=CARTESIAN_POINT('Ctrl Pts',(-1.57261587600006,2.2,-3.77107153100001));
#323532=CARTESIAN_POINT('Ctrl Pts',(-1.57280730000006,12.2,-3.77211343700001));
#323533=CARTESIAN_POINT('Ctrl Pts',(-1.57280730000006,5.2,-3.77211343700001));
#323534=CARTESIAN_POINT('Ctrl Pts',(-1.57280730000006,2.2,-3.77211343700001));
#323535=CARTESIAN_POINT('Ctrl Pts',(-1.57299841500006,12.2,-3.77316087100001));
#323536=CARTESIAN_POINT('Ctrl Pts',(-1.57299841500006,5.2,-3.77316087100001));
#323537=CARTESIAN_POINT('Ctrl Pts',(-1.57299841500006,2.2,-3.77316087100001));
#323538=CARTESIAN_POINT('Ctrl Pts',(-1.57318920600006,12.2,-3.77421382400001));
#323539=CARTESIAN_POINT('Ctrl Pts',(-1.57318920600006,5.2,-3.77421382400001));
#323540=CARTESIAN_POINT('Ctrl Pts',(-1.57318920600006,2.2,-3.77421382400001));
#323541=CARTESIAN_POINT('Ctrl Pts',(-1.57337966000005,12.2,-3.77527228700002));
#323542=CARTESIAN_POINT('Ctrl Pts',(-1.57337966000005,5.2,-3.77527228700002));
#323543=CARTESIAN_POINT('Ctrl Pts',(-1.57337966000005,2.2,-3.77527228700002));
#323544=CARTESIAN_POINT('Ctrl Pts',(-1.57356976200006,12.2,-3.77633625300001));
#323545=CARTESIAN_POINT('Ctrl Pts',(-1.57356976200006,5.2,-3.77633625300001));
#323546=CARTESIAN_POINT('Ctrl Pts',(-1.57356976200006,2.2,-3.77633625300001));
#323547=CARTESIAN_POINT('Ctrl Pts',(-1.57375949900006,12.2,-3.77740571600001));
#323548=CARTESIAN_POINT('Ctrl Pts',(-1.57375949900006,5.2,-3.77740571600001));
#323549=CARTESIAN_POINT('Ctrl Pts',(-1.57375949900006,2.2,-3.77740571600001));
#323550=CARTESIAN_POINT('Ctrl Pts',(-1.57394885500006,12.2,-3.77848066400002));
#323551=CARTESIAN_POINT('Ctrl Pts',(-1.57394885500006,5.2,-3.77848066400002));
#323552=CARTESIAN_POINT('Ctrl Pts',(-1.57394885500006,2.2,-3.77848066400002));
#323553=CARTESIAN_POINT('Ctrl Pts',(-1.57413781900006,12.2,-3.77956109200001));
#323554=CARTESIAN_POINT('Ctrl Pts',(-1.57413781900006,5.2,-3.77956109200001));
#323555=CARTESIAN_POINT('Ctrl Pts',(-1.57413781900006,2.2,-3.77956109200001));
#323556=CARTESIAN_POINT('Ctrl Pts',(-1.57432637600006,12.2,-3.78064699100001));
#323557=CARTESIAN_POINT('Ctrl Pts',(-1.57432637600006,5.2,-3.78064699100001));
#323558=CARTESIAN_POINT('Ctrl Pts',(-1.57432637600006,2.2,-3.78064699100001));
#323559=CARTESIAN_POINT('Ctrl Pts',(-1.57451451100005,12.2,-3.78173835300001));
#323560=CARTESIAN_POINT('Ctrl Pts',(-1.57451451100005,5.2,-3.78173835300001));
#323561=CARTESIAN_POINT('Ctrl Pts',(-1.57451451100005,2.2,-3.78173835300001));
#323562=CARTESIAN_POINT('Ctrl Pts',(-1.57470221200006,12.2,-3.78283517000002));
#323563=CARTESIAN_POINT('Ctrl Pts',(-1.57470221200006,5.2,-3.78283517000002));
#323564=CARTESIAN_POINT('Ctrl Pts',(-1.57470221200006,2.2,-3.78283517000002));
#323565=CARTESIAN_POINT('Ctrl Pts',(-1.57488946500006,12.2,-3.78393743500002));
#323566=CARTESIAN_POINT('Ctrl Pts',(-1.57488946500006,5.2,-3.78393743500002));
#323567=CARTESIAN_POINT('Ctrl Pts',(-1.57488946500006,2.2,-3.78393743500002));
#323568=CARTESIAN_POINT('Ctrl Pts',(-1.57507625600006,12.2,-3.78504513900001));
#323569=CARTESIAN_POINT('Ctrl Pts',(-1.57507625600006,5.2,-3.78504513900001));
#323570=CARTESIAN_POINT('Ctrl Pts',(-1.57507625600006,2.2,-3.78504513900001));
#323571=CARTESIAN_POINT('Ctrl Pts',(-1.57526257100006,12.2,-3.78615827400001));
#323572=CARTESIAN_POINT('Ctrl Pts',(-1.57526257100006,5.2,-3.78615827400001));
#323573=CARTESIAN_POINT('Ctrl Pts',(-1.57526257100006,2.2,-3.78615827400001));
#323574=CARTESIAN_POINT('Ctrl Pts',(-1.57544839700006,12.2,-3.78727683200001));
#323575=CARTESIAN_POINT('Ctrl Pts',(-1.57544839700006,5.2,-3.78727683200001));
#323576=CARTESIAN_POINT('Ctrl Pts',(-1.57544839700006,2.2,-3.78727683200001));
#323577=CARTESIAN_POINT('Ctrl Pts',(-1.57563372100005,12.2,-3.78840080700002));
#323578=CARTESIAN_POINT('Ctrl Pts',(-1.57563372100005,5.2,-3.78840080700002));
#323579=CARTESIAN_POINT('Ctrl Pts',(-1.57563372100005,2.2,-3.78840080700002));
#323580=CARTESIAN_POINT('Ctrl Pts',(-1.57581852800006,12.2,-3.78953018700001));
#323581=CARTESIAN_POINT('Ctrl Pts',(-1.57581852800006,5.2,-3.78953018700001));
#323582=CARTESIAN_POINT('Ctrl Pts',(-1.57581852800006,2.2,-3.78953018700001));
#323583=CARTESIAN_POINT('Ctrl Pts',(-1.57600280500006,12.2,-3.79066496800001));
#323584=CARTESIAN_POINT('Ctrl Pts',(-1.57600280500006,5.2,-3.79066496800001));
#323585=CARTESIAN_POINT('Ctrl Pts',(-1.57600280500006,2.2,-3.79066496800001));
#323586=CARTESIAN_POINT('Ctrl Pts',(-1.57618654000005,12.2,-3.79180514000002));
#323587=CARTESIAN_POINT('Ctrl Pts',(-1.57618654000005,5.2,-3.79180514000002));
#323588=CARTESIAN_POINT('Ctrl Pts',(-1.57618654000005,2.2,-3.79180514000002));
#323589=CARTESIAN_POINT('Ctrl Pts',(-1.57636971900006,12.2,-3.79295069600001));
#323590=CARTESIAN_POINT('Ctrl Pts',(-1.57636971900006,5.2,-3.79295069600001));
#323591=CARTESIAN_POINT('Ctrl Pts',(-1.57636971900006,2.2,-3.79295069600001));
#323592=CARTESIAN_POINT('Ctrl Pts',(-1.57655232800006,12.2,-3.79410162700001));
#323593=CARTESIAN_POINT('Ctrl Pts',(-1.57655232800006,5.2,-3.79410162700001));
#323594=CARTESIAN_POINT('Ctrl Pts',(-1.57655232800006,2.2,-3.79410162700001));
#323595=CARTESIAN_POINT('Ctrl Pts',(-1.57673435400006,12.2,-3.79525792600001));
#323596=CARTESIAN_POINT('Ctrl Pts',(-1.57673435400006,5.2,-3.79525792600001));
#323597=CARTESIAN_POINT('Ctrl Pts',(-1.57673435400006,2.2,-3.79525792600001));
#323598=CARTESIAN_POINT('Ctrl Pts',(-1.57691578400006,12.2,-3.79641958400001));
#323599=CARTESIAN_POINT('Ctrl Pts',(-1.57691578400006,5.2,-3.79641958400001));
#323600=CARTESIAN_POINT('Ctrl Pts',(-1.57691578400006,2.2,-3.79641958400001));
#323601=CARTESIAN_POINT('Ctrl Pts',(-1.57709660400006,12.2,-3.79758659500002));
#323602=CARTESIAN_POINT('Ctrl Pts',(-1.57709660400006,5.2,-3.79758659500002));
#323603=CARTESIAN_POINT('Ctrl Pts',(-1.57709660400006,2.2,-3.79758659500002));
#323604=CARTESIAN_POINT('Ctrl Pts',(-1.57727680300006,12.2,-3.79875894900001));
#323605=CARTESIAN_POINT('Ctrl Pts',(-1.57727680300006,5.2,-3.79875894900001));
#323606=CARTESIAN_POINT('Ctrl Pts',(-1.57727680300006,2.2,-3.79875894900001));
#323607=CARTESIAN_POINT('Ctrl Pts',(-1.57745636500006,12.2,-3.79993664000001));
#323608=CARTESIAN_POINT('Ctrl Pts',(-1.57745636500006,5.2,-3.79993664000001));
#323609=CARTESIAN_POINT('Ctrl Pts',(-1.57745636500006,2.2,-3.79993664000001));
#323610=CARTESIAN_POINT('Ctrl Pts',(-1.57763528000005,12.2,-3.80111965800001));
#323611=CARTESIAN_POINT('Ctrl Pts',(-1.57763528000005,5.2,-3.80111965800001));
#323612=CARTESIAN_POINT('Ctrl Pts',(-1.57763528000005,2.2,-3.80111965800001));
#323613=CARTESIAN_POINT('Ctrl Pts',(-1.57781353300006,12.2,-3.80230799500001));
#323614=CARTESIAN_POINT('Ctrl Pts',(-1.57781353300006,5.2,-3.80230799500001));
#323615=CARTESIAN_POINT('Ctrl Pts',(-1.57781353300006,2.2,-3.80230799500001));
#323616=CARTESIAN_POINT('Ctrl Pts',(-1.57799111000006,12.2,-3.80350164500001));
#323617=CARTESIAN_POINT('Ctrl Pts',(-1.57799111000006,5.2,-3.80350164500001));
#323618=CARTESIAN_POINT('Ctrl Pts',(-1.57799111000006,2.2,-3.80350164500001));
#323619=CARTESIAN_POINT('Ctrl Pts',(-1.57816800100006,12.2,-3.80470059800002));
#323620=CARTESIAN_POINT('Ctrl Pts',(-1.57816800100006,5.2,-3.80470059800002));
#323621=CARTESIAN_POINT('Ctrl Pts',(-1.57816800100006,2.2,-3.80470059800002));
#323622=CARTESIAN_POINT('Ctrl Pts',(-1.57834419200006,12.2,-3.80590484900001));
#323623=CARTESIAN_POINT('Ctrl Pts',(-1.57834419200006,5.2,-3.80590484900001));
#323624=CARTESIAN_POINT('Ctrl Pts',(-1.57834419200006,2.2,-3.80590484900001));
#323625=CARTESIAN_POINT('Ctrl Pts',(-1.57851966900005,12.2,-3.80711438700001));
#323626=CARTESIAN_POINT('Ctrl Pts',(-1.57851966900005,5.2,-3.80711438700001));
#323627=CARTESIAN_POINT('Ctrl Pts',(-1.57851966900005,2.2,-3.80711438700001));
#323628=CARTESIAN_POINT('Ctrl Pts',(-1.57869441900006,12.2,-3.80832920600001));
#323629=CARTESIAN_POINT('Ctrl Pts',(-1.57869441900006,5.2,-3.80832920600001));
#323630=CARTESIAN_POINT('Ctrl Pts',(-1.57869441900006,2.2,-3.80832920600001));
#323631=CARTESIAN_POINT('Ctrl Pts',(-1.57886843200005,12.2,-3.80954929600001));
#323632=CARTESIAN_POINT('Ctrl Pts',(-1.57886843200005,5.2,-3.80954929600001));
#323633=CARTESIAN_POINT('Ctrl Pts',(-1.57886843200005,2.2,-3.80954929600001));
#323634=CARTESIAN_POINT('Ctrl Pts',(-1.57904169200005,12.2,-3.81077465100002));
#323635=CARTESIAN_POINT('Ctrl Pts',(-1.57904169200005,5.2,-3.81077465100002));
#323636=CARTESIAN_POINT('Ctrl Pts',(-1.57904169200005,2.2,-3.81077465100002));
#323637=CARTESIAN_POINT('Ctrl Pts',(-1.57921418900006,12.2,-3.81200526300002));
#323638=CARTESIAN_POINT('Ctrl Pts',(-1.57921418900006,5.2,-3.81200526300002));
#323639=CARTESIAN_POINT('Ctrl Pts',(-1.57921418900006,2.2,-3.81200526300002));
#323640=CARTESIAN_POINT('Ctrl Pts',(-1.57938590800006,12.2,-3.81324112200002));
#323641=CARTESIAN_POINT('Ctrl Pts',(-1.57938590800006,5.2,-3.81324112200002));
#323642=CARTESIAN_POINT('Ctrl Pts',(-1.57938590800006,2.2,-3.81324112200002));
#323643=CARTESIAN_POINT('Ctrl Pts',(-1.57955683700005,12.2,-3.81448222300001));
#323644=CARTESIAN_POINT('Ctrl Pts',(-1.57955683700005,5.2,-3.81448222300001));
#323645=CARTESIAN_POINT('Ctrl Pts',(-1.57955683700005,2.2,-3.81448222300001));
#323646=CARTESIAN_POINT('Ctrl Pts',(-1.57972696400006,12.2,-3.81572855600002));
#323647=CARTESIAN_POINT('Ctrl Pts',(-1.57972696400006,5.2,-3.81572855600002));
#323648=CARTESIAN_POINT('Ctrl Pts',(-1.57972696400006,2.2,-3.81572855600002));
#323649=CARTESIAN_POINT('Ctrl Pts',(-1.57989627800006,12.2,-3.81698011500001));
#323650=CARTESIAN_POINT('Ctrl Pts',(-1.57989627800006,5.2,-3.81698011500001));
#323651=CARTESIAN_POINT('Ctrl Pts',(-1.57989627800006,2.2,-3.81698011500001));
#323652=CARTESIAN_POINT('Ctrl Pts',(-1.58006476400006,12.2,-3.81823689000001));
#323653=CARTESIAN_POINT('Ctrl Pts',(-1.58006476400006,5.2,-3.81823689000001));
#323654=CARTESIAN_POINT('Ctrl Pts',(-1.58006476400006,2.2,-3.81823689000001));
#323655=CARTESIAN_POINT('Ctrl Pts',(-1.58023240900006,12.2,-3.81949887400001));
#323656=CARTESIAN_POINT('Ctrl Pts',(-1.58023240900006,5.2,-3.81949887400001));
#323657=CARTESIAN_POINT('Ctrl Pts',(-1.58023240900006,2.2,-3.81949887400001));
#323658=CARTESIAN_POINT('Ctrl Pts',(-1.58039920300005,12.2,-3.82076605800002));
#323659=CARTESIAN_POINT('Ctrl Pts',(-1.58039920300005,5.2,-3.82076605800002));
#323660=CARTESIAN_POINT('Ctrl Pts',(-1.58039920300005,2.2,-3.82076605800002));
#323661=CARTESIAN_POINT('Ctrl Pts',(-1.58056513200005,12.2,-3.82203843600001));
#323662=CARTESIAN_POINT('Ctrl Pts',(-1.58056513200005,5.2,-3.82203843600001));
#323663=CARTESIAN_POINT('Ctrl Pts',(-1.58056513200005,2.2,-3.82203843600001));
#323664=CARTESIAN_POINT('Ctrl Pts',(-1.58073018500006,12.2,-3.82331599900001));
#323665=CARTESIAN_POINT('Ctrl Pts',(-1.58073018500006,5.2,-3.82331599900001));
#323666=CARTESIAN_POINT('Ctrl Pts',(-1.58073018500006,2.2,-3.82331599900001));
#323667=CARTESIAN_POINT('Ctrl Pts',(-1.58089434800006,12.2,-3.82459873900002));
#323668=CARTESIAN_POINT('Ctrl Pts',(-1.58089434800006,5.2,-3.82459873900002));
#323669=CARTESIAN_POINT('Ctrl Pts',(-1.58089434800006,2.2,-3.82459873900002));
#323670=CARTESIAN_POINT('Ctrl Pts',(-1.58105761000006,12.2,-3.82588664800001));
#323671=CARTESIAN_POINT('Ctrl Pts',(-1.58105761000006,5.2,-3.82588664800001));
#323672=CARTESIAN_POINT('Ctrl Pts',(-1.58105761000006,2.2,-3.82588664800001));
#323673=CARTESIAN_POINT('Ctrl Pts',(-1.58121995800005,12.2,-3.82717971800002));
#323674=CARTESIAN_POINT('Ctrl Pts',(-1.58121995800005,5.2,-3.82717971800002));
#323675=CARTESIAN_POINT('Ctrl Pts',(-1.58121995800005,2.2,-3.82717971800002));
#323676=CARTESIAN_POINT('Ctrl Pts',(-1.58138138000006,12.2,-3.82847794200002));
#323677=CARTESIAN_POINT('Ctrl Pts',(-1.58138138000006,5.2,-3.82847794200002));
#323678=CARTESIAN_POINT('Ctrl Pts',(-1.58138138000006,2.2,-3.82847794200002));
#323679=CARTESIAN_POINT('Ctrl Pts',(-1.58154186500005,12.2,-3.82978131200002));
#323680=CARTESIAN_POINT('Ctrl Pts',(-1.58154186500005,5.2,-3.82978131200002));
#323681=CARTESIAN_POINT('Ctrl Pts',(-1.58154186500005,2.2,-3.82978131200002));
#323682=CARTESIAN_POINT('Ctrl Pts',(-1.58170139800006,12.2,-3.83108981900001));
#323683=CARTESIAN_POINT('Ctrl Pts',(-1.58170139800006,5.2,-3.83108981900001));
#323684=CARTESIAN_POINT('Ctrl Pts',(-1.58170139800006,2.2,-3.83108981900001));
#323685=CARTESIAN_POINT('Ctrl Pts',(-1.58185997000006,12.2,-3.83240345600001));
#323686=CARTESIAN_POINT('Ctrl Pts',(-1.58185997000006,5.2,-3.83240345600001));
#323687=CARTESIAN_POINT('Ctrl Pts',(-1.58185997000006,2.2,-3.83240345600001));
#323688=CARTESIAN_POINT('Ctrl Pts',(-1.58201756800006,12.2,-3.83372221400001));
#323689=CARTESIAN_POINT('Ctrl Pts',(-1.58201756800006,5.2,-3.83372221400001));
#323690=CARTESIAN_POINT('Ctrl Pts',(-1.58201756800006,2.2,-3.83372221400001));
#323691=CARTESIAN_POINT('Ctrl Pts',(-1.58217417900006,12.2,-3.83504608800001));
#323692=CARTESIAN_POINT('Ctrl Pts',(-1.58217417900006,5.2,-3.83504608800001));
#323693=CARTESIAN_POINT('Ctrl Pts',(-1.58217417900006,2.2,-3.83504608800001));
#323694=CARTESIAN_POINT('Ctrl Pts',(-1.58232979100006,12.2,-3.83637506500001));
#323695=CARTESIAN_POINT('Ctrl Pts',(-1.58232979100006,5.2,-3.83637506500001));
#323696=CARTESIAN_POINT('Ctrl Pts',(-1.58232979100006,2.2,-3.83637506500001));
#323697=CARTESIAN_POINT('Ctrl Pts',(-1.58248439400006,12.2,-3.83770914200001));
#323698=CARTESIAN_POINT('Ctrl Pts',(-1.58248439400006,5.2,-3.83770914200001));
#323699=CARTESIAN_POINT('Ctrl Pts',(-1.58248439400006,2.2,-3.83770914200001));
#323700=CARTESIAN_POINT('Ctrl Pts',(-1.58263797400006,12.2,-3.83904831000002));
#323701=CARTESIAN_POINT('Ctrl Pts',(-1.58263797400006,5.2,-3.83904831000002));
#323702=CARTESIAN_POINT('Ctrl Pts',(-1.58263797400006,2.2,-3.83904831000002));
#323703=CARTESIAN_POINT('Ctrl Pts',(-1.58279052000006,12.2,-3.84039255800001));
#323704=CARTESIAN_POINT('Ctrl Pts',(-1.58279052000006,5.2,-3.84039255800001));
#323705=CARTESIAN_POINT('Ctrl Pts',(-1.58279052000006,2.2,-3.84039255800001));
#323706=CARTESIAN_POINT('Ctrl Pts',(-1.58294202100006,12.2,-3.84174188200001));
#323707=CARTESIAN_POINT('Ctrl Pts',(-1.58294202100006,5.2,-3.84174188200001));
#323708=CARTESIAN_POINT('Ctrl Pts',(-1.58294202100006,2.2,-3.84174188200001));
#323709=CARTESIAN_POINT('Ctrl Pts',(-1.58309246300006,12.2,-3.84309627200001));
#323710=CARTESIAN_POINT('Ctrl Pts',(-1.58309246300006,5.2,-3.84309627200001));
#323711=CARTESIAN_POINT('Ctrl Pts',(-1.58309246300006,2.2,-3.84309627200001));
#323712=CARTESIAN_POINT('Ctrl Pts',(-1.58324183600006,12.2,-3.84445572000002));
#323713=CARTESIAN_POINT('Ctrl Pts',(-1.58324183600006,5.2,-3.84445572000002));
#323714=CARTESIAN_POINT('Ctrl Pts',(-1.58324183600006,2.2,-3.84445572000002));
#323715=CARTESIAN_POINT('Ctrl Pts',(-1.58339012800006,12.2,-3.84582022000002));
#323716=CARTESIAN_POINT('Ctrl Pts',(-1.58339012800006,5.2,-3.84582022000002));
#323717=CARTESIAN_POINT('Ctrl Pts',(-1.58339012800006,2.2,-3.84582022000002));
#323718=CARTESIAN_POINT('Ctrl Pts',(-1.58353732700005,12.2,-3.84718976100002));
#323719=CARTESIAN_POINT('Ctrl Pts',(-1.58353732700005,5.2,-3.84718976100002));
#323720=CARTESIAN_POINT('Ctrl Pts',(-1.58353732700005,2.2,-3.84718976100002));
#323721=CARTESIAN_POINT('Ctrl Pts',(-1.58368342100006,12.2,-3.84856433800001));
#323722=CARTESIAN_POINT('Ctrl Pts',(-1.58368342100006,5.2,-3.84856433800001));
#323723=CARTESIAN_POINT('Ctrl Pts',(-1.58368342100006,2.2,-3.84856433800001));
#323724=CARTESIAN_POINT('Ctrl Pts',(-1.58382839900006,12.2,-3.84994394200001));
#323725=CARTESIAN_POINT('Ctrl Pts',(-1.58382839900006,5.2,-3.84994394200001));
#323726=CARTESIAN_POINT('Ctrl Pts',(-1.58382839900006,2.2,-3.84994394200001));
#323727=CARTESIAN_POINT('Ctrl Pts',(-1.58397225000006,12.2,-3.85132856500002));
#323728=CARTESIAN_POINT('Ctrl Pts',(-1.58397225000006,5.2,-3.85132856500002));
#323729=CARTESIAN_POINT('Ctrl Pts',(-1.58397225000006,2.2,-3.85132856500002));
#323730=CARTESIAN_POINT('Ctrl Pts',(-1.58411496100005,12.2,-3.85271819900002));
#323731=CARTESIAN_POINT('Ctrl Pts',(-1.58411496100005,5.2,-3.85271819900002));
#323732=CARTESIAN_POINT('Ctrl Pts',(-1.58411496100005,2.2,-3.85271819900002));
#323733=CARTESIAN_POINT('Ctrl Pts',(-1.58425652100005,12.2,-3.85411283600002));
#323734=CARTESIAN_POINT('Ctrl Pts',(-1.58425652100005,5.2,-3.85411283600002));
#323735=CARTESIAN_POINT('Ctrl Pts',(-1.58425652100005,2.2,-3.85411283600002));
#323736=CARTESIAN_POINT('Ctrl Pts',(-1.58439691900006,12.2,-3.85551247000001));
#323737=CARTESIAN_POINT('Ctrl Pts',(-1.58439691900006,5.2,-3.85551247000001));
#323738=CARTESIAN_POINT('Ctrl Pts',(-1.58439691900006,2.2,-3.85551247000001));
#323739=CARTESIAN_POINT('Ctrl Pts',(-1.58453614300006,12.2,-3.85691709000001));
#323740=CARTESIAN_POINT('Ctrl Pts',(-1.58453614300006,5.2,-3.85691709000001));
#323741=CARTESIAN_POINT('Ctrl Pts',(-1.58453614300006,2.2,-3.85691709000001));
#323742=CARTESIAN_POINT('Ctrl Pts',(-1.58467418200006,12.2,-3.85832669000001));
#323743=CARTESIAN_POINT('Ctrl Pts',(-1.58467418200006,5.2,-3.85832669000001));
#323744=CARTESIAN_POINT('Ctrl Pts',(-1.58467418200006,2.2,-3.85832669000001));
#323745=CARTESIAN_POINT('Ctrl Pts',(-1.58481102500006,12.2,-3.85974126200002));
#323746=CARTESIAN_POINT('Ctrl Pts',(-1.58481102500006,5.2,-3.85974126200002));
#323747=CARTESIAN_POINT('Ctrl Pts',(-1.58481102500006,2.2,-3.85974126200002));
#323748=CARTESIAN_POINT('Ctrl Pts',(-1.58494665900006,12.2,-3.86116079800002));
#323749=CARTESIAN_POINT('Ctrl Pts',(-1.58494665900006,5.2,-3.86116079800002));
#323750=CARTESIAN_POINT('Ctrl Pts',(-1.58494665900006,2.2,-3.86116079800002));
#323751=CARTESIAN_POINT('Ctrl Pts',(-1.58508107400006,12.2,-3.86258529000001));
#323752=CARTESIAN_POINT('Ctrl Pts',(-1.58508107400006,5.2,-3.86258529000001));
#323753=CARTESIAN_POINT('Ctrl Pts',(-1.58508107400006,2.2,-3.86258529000001));
#323754=CARTESIAN_POINT('Ctrl Pts',(-1.58521425900006,12.2,-3.86401473000001));
#323755=CARTESIAN_POINT('Ctrl Pts',(-1.58521425900006,5.2,-3.86401473000001));
#323756=CARTESIAN_POINT('Ctrl Pts',(-1.58521425900006,2.2,-3.86401473000001));
#323757=CARTESIAN_POINT('Ctrl Pts',(-1.58534620200005,12.2,-3.86544911100001));
#323758=CARTESIAN_POINT('Ctrl Pts',(-1.58534620200005,5.2,-3.86544911100001));
#323759=CARTESIAN_POINT('Ctrl Pts',(-1.58534620200005,2.2,-3.86544911100001));
#323760=CARTESIAN_POINT('Ctrl Pts',(-1.58547689100006,12.2,-3.86688842400002));
#323761=CARTESIAN_POINT('Ctrl Pts',(-1.58547689100006,5.2,-3.86688842400002));
#323762=CARTESIAN_POINT('Ctrl Pts',(-1.58547689100006,2.2,-3.86688842400002));
#323763=CARTESIAN_POINT('Ctrl Pts',(-1.58560631700006,12.2,-3.86833266100002));
#323764=CARTESIAN_POINT('Ctrl Pts',(-1.58560631700006,5.2,-3.86833266100002));
#323765=CARTESIAN_POINT('Ctrl Pts',(-1.58560631700006,2.2,-3.86833266100002));
#323766=CARTESIAN_POINT('Ctrl Pts',(-1.58573446800006,12.2,-3.86978181500002));
#323767=CARTESIAN_POINT('Ctrl Pts',(-1.58573446800006,5.2,-3.86978181500002));
#323768=CARTESIAN_POINT('Ctrl Pts',(-1.58573446800006,2.2,-3.86978181500002));
#323769=CARTESIAN_POINT('Ctrl Pts',(-1.58586133200005,12.2,-3.87123587800001));
#323770=CARTESIAN_POINT('Ctrl Pts',(-1.58586133200005,5.2,-3.87123587800001));
#323771=CARTESIAN_POINT('Ctrl Pts',(-1.58586133200005,2.2,-3.87123587800001));
#323772=CARTESIAN_POINT('Ctrl Pts',(-1.58598689800006,12.2,-3.87269484100001));
#323773=CARTESIAN_POINT('Ctrl Pts',(-1.58598689800006,5.2,-3.87269484100001));
#323774=CARTESIAN_POINT('Ctrl Pts',(-1.58598689800006,2.2,-3.87269484100001));
#323775=CARTESIAN_POINT('Ctrl Pts',(-1.58611115600006,12.2,-3.87415869700002));
#323776=CARTESIAN_POINT('Ctrl Pts',(-1.58611115600006,5.2,-3.87415869700002));
#323777=CARTESIAN_POINT('Ctrl Pts',(-1.58611115600006,2.2,-3.87415869700002));
#323778=CARTESIAN_POINT('Ctrl Pts',(-1.58623409500006,12.2,-3.87562744000002));
#323779=CARTESIAN_POINT('Ctrl Pts',(-1.58623409500006,5.2,-3.87562744000002));
#323780=CARTESIAN_POINT('Ctrl Pts',(-1.58623409500006,2.2,-3.87562744000002));
#323781=CARTESIAN_POINT('Ctrl Pts',(-1.58635570200006,12.2,-3.87710105900001));
#323782=CARTESIAN_POINT('Ctrl Pts',(-1.58635570200006,5.2,-3.87710105900001));
#323783=CARTESIAN_POINT('Ctrl Pts',(-1.58635570200006,2.2,-3.87710105900001));
#323784=CARTESIAN_POINT('Ctrl Pts',(-1.58647596900006,12.2,-3.87857954800001));
#323785=CARTESIAN_POINT('Ctrl Pts',(-1.58647596900006,5.2,-3.87857954800001));
#323786=CARTESIAN_POINT('Ctrl Pts',(-1.58647596900006,2.2,-3.87857954800001));
#323787=CARTESIAN_POINT('Ctrl Pts',(-1.58659488300006,12.2,-3.88006289700002));
#323788=CARTESIAN_POINT('Ctrl Pts',(-1.58659488300006,5.2,-3.88006289700002));
#323789=CARTESIAN_POINT('Ctrl Pts',(-1.58659488300006,2.2,-3.88006289700002));
#323790=CARTESIAN_POINT('Ctrl Pts',(-1.58671243300006,12.2,-3.88155110200001));
#323791=CARTESIAN_POINT('Ctrl Pts',(-1.58671243300006,5.2,-3.88155110200001));
#323792=CARTESIAN_POINT('Ctrl Pts',(-1.58671243300006,2.2,-3.88155110200001));
#323793=CARTESIAN_POINT('Ctrl Pts',(-1.58682861100006,12.2,-3.88304415200002));
#323794=CARTESIAN_POINT('Ctrl Pts',(-1.58682861100006,5.2,-3.88304415200002));
#323795=CARTESIAN_POINT('Ctrl Pts',(-1.58682861100006,2.2,-3.88304415200002));
#323796=CARTESIAN_POINT('Ctrl Pts',(-1.58694340200006,12.2,-3.88454203900002));
#323797=CARTESIAN_POINT('Ctrl Pts',(-1.58694340200006,5.2,-3.88454203900002));
#323798=CARTESIAN_POINT('Ctrl Pts',(-1.58694340200006,2.2,-3.88454203900002));
#323799=CARTESIAN_POINT('Ctrl Pts',(-1.58705679800006,12.2,-3.88604475700001));
#323800=CARTESIAN_POINT('Ctrl Pts',(-1.58705679800006,5.2,-3.88604475700001));
#323801=CARTESIAN_POINT('Ctrl Pts',(-1.58705679800006,2.2,-3.88604475700001));
#323802=CARTESIAN_POINT('Ctrl Pts',(-1.58716878700006,12.2,-3.88755229700001));
#323803=CARTESIAN_POINT('Ctrl Pts',(-1.58716878700006,5.2,-3.88755229700001));
#323804=CARTESIAN_POINT('Ctrl Pts',(-1.58716878700006,2.2,-3.88755229700001));
#323805=CARTESIAN_POINT('Ctrl Pts',(-1.58727936000005,12.2,-3.88906465100002));
#323806=CARTESIAN_POINT('Ctrl Pts',(-1.58727936000005,5.2,-3.88906465100002));
#323807=CARTESIAN_POINT('Ctrl Pts',(-1.58727936000005,2.2,-3.88906465100002));
#323808=CARTESIAN_POINT('Ctrl Pts',(-1.58738850400006,12.2,-3.89058181300001));
#323809=CARTESIAN_POINT('Ctrl Pts',(-1.58738850400006,5.2,-3.89058181300001));
#323810=CARTESIAN_POINT('Ctrl Pts',(-1.58738850400006,2.2,-3.89058181300001));
#323811=CARTESIAN_POINT('Ctrl Pts',(-1.58749621100006,12.2,-3.89210377300001));
#323812=CARTESIAN_POINT('Ctrl Pts',(-1.58749621100006,5.2,-3.89210377300001));
#323813=CARTESIAN_POINT('Ctrl Pts',(-1.58749621100006,2.2,-3.89210377300001));
#323814=CARTESIAN_POINT('Ctrl Pts',(-1.58760246700006,12.2,-3.89363052400002));
#323815=CARTESIAN_POINT('Ctrl Pts',(-1.58760246700006,5.2,-3.89363052400002));
#323816=CARTESIAN_POINT('Ctrl Pts',(-1.58760246700006,2.2,-3.89363052400002));
#323817=CARTESIAN_POINT('Ctrl Pts',(-1.58770726400005,12.2,-3.89516205800001));
#323818=CARTESIAN_POINT('Ctrl Pts',(-1.58770726400005,5.2,-3.89516205800001));
#323819=CARTESIAN_POINT('Ctrl Pts',(-1.58770726400005,2.2,-3.89516205800001));
#323820=CARTESIAN_POINT('Ctrl Pts',(-1.58781059000005,12.2,-3.89669836700001));
#323821=CARTESIAN_POINT('Ctrl Pts',(-1.58781059000005,5.2,-3.89669836700001));
#323822=CARTESIAN_POINT('Ctrl Pts',(-1.58781059000005,2.2,-3.89669836700001));
#323823=CARTESIAN_POINT('Ctrl Pts',(-1.58791243700006,12.2,-3.89823944300002));
#323824=CARTESIAN_POINT('Ctrl Pts',(-1.58791243700006,5.2,-3.89823944300002));
#323825=CARTESIAN_POINT('Ctrl Pts',(-1.58791243700006,2.2,-3.89823944300002));
#323826=CARTESIAN_POINT('Ctrl Pts',(-1.58801279100006,12.2,-3.89978528000002));
#323827=CARTESIAN_POINT('Ctrl Pts',(-1.58801279100006,5.2,-3.89978528000002));
#323828=CARTESIAN_POINT('Ctrl Pts',(-1.58801279100006,2.2,-3.89978528000002));
#323829=CARTESIAN_POINT('Ctrl Pts',(-1.58811164400006,12.2,-3.90133586700002));
#323830=CARTESIAN_POINT('Ctrl Pts',(-1.58811164400006,5.2,-3.90133586700002));
#323831=CARTESIAN_POINT('Ctrl Pts',(-1.58811164400006,2.2,-3.90133586700002));
#323832=CARTESIAN_POINT('Ctrl Pts',(-1.58820898400006,12.2,-3.90289119900002));
#323833=CARTESIAN_POINT('Ctrl Pts',(-1.58820898400006,5.2,-3.90289119900002));
#323834=CARTESIAN_POINT('Ctrl Pts',(-1.58820898400006,2.2,-3.90289119900002));
#323835=CARTESIAN_POINT('Ctrl Pts',(-1.58830480300006,12.2,-3.90445126600001));
#323836=CARTESIAN_POINT('Ctrl Pts',(-1.58830480300006,5.2,-3.90445126600001));
#323837=CARTESIAN_POINT('Ctrl Pts',(-1.58830480300006,2.2,-3.90445126600001));
#323838=CARTESIAN_POINT('Ctrl Pts',(-1.58839908700006,12.2,-3.90601606200002));
#323839=CARTESIAN_POINT('Ctrl Pts',(-1.58839908700006,5.2,-3.90601606200002));
#323840=CARTESIAN_POINT('Ctrl Pts',(-1.58839908700006,2.2,-3.90601606200002));
#323841=CARTESIAN_POINT('Ctrl Pts',(-1.58849182800005,12.2,-3.90758557700002));
#323842=CARTESIAN_POINT('Ctrl Pts',(-1.58849182800005,5.2,-3.90758557700002));
#323843=CARTESIAN_POINT('Ctrl Pts',(-1.58849182800005,2.2,-3.90758557700002));
#323844=CARTESIAN_POINT('Ctrl Pts',(-1.58858301700006,12.2,-3.90915980500001));
#323845=CARTESIAN_POINT('Ctrl Pts',(-1.58858301700006,5.2,-3.90915980500001));
#323846=CARTESIAN_POINT('Ctrl Pts',(-1.58858301700006,2.2,-3.90915980500001));
#323847=CARTESIAN_POINT('Ctrl Pts',(-1.58867264000006,12.2,-3.91073873900002));
#323848=CARTESIAN_POINT('Ctrl Pts',(-1.58867264000006,5.2,-3.91073873900002));
#323849=CARTESIAN_POINT('Ctrl Pts',(-1.58867264000006,2.2,-3.91073873900002));
#323850=CARTESIAN_POINT('Ctrl Pts',(-1.58876068900006,12.2,-3.91232236800001));
#323851=CARTESIAN_POINT('Ctrl Pts',(-1.58876068900006,5.2,-3.91232236800001));
#323852=CARTESIAN_POINT('Ctrl Pts',(-1.58876068900006,2.2,-3.91232236800001));
#323853=CARTESIAN_POINT('Ctrl Pts',(-1.58884715500006,12.2,-3.91391068700001));
#323854=CARTESIAN_POINT('Ctrl Pts',(-1.58884715500006,5.2,-3.91391068700001));
#323855=CARTESIAN_POINT('Ctrl Pts',(-1.58884715500006,2.2,-3.91391068700001));
#323856=CARTESIAN_POINT('Ctrl Pts',(-1.58893202500006,12.2,-3.91550368600001));
#323857=CARTESIAN_POINT('Ctrl Pts',(-1.58893202500006,5.2,-3.91550368600001));
#323858=CARTESIAN_POINT('Ctrl Pts',(-1.58893202500006,2.2,-3.91550368600001));
#323859=CARTESIAN_POINT('Ctrl Pts',(-1.58901529100006,12.2,-3.91710135900002));
#323860=CARTESIAN_POINT('Ctrl Pts',(-1.58901529100006,5.2,-3.91710135900002));
#323861=CARTESIAN_POINT('Ctrl Pts',(-1.58901529100006,2.2,-3.91710135900002));
#323862=CARTESIAN_POINT('Ctrl Pts',(-1.58909694200006,12.2,-3.91870369900001));
#323863=CARTESIAN_POINT('Ctrl Pts',(-1.58909694200006,5.2,-3.91870369900001));
#323864=CARTESIAN_POINT('Ctrl Pts',(-1.58909694200006,2.2,-3.91870369900001));
#323865=CARTESIAN_POINT('Ctrl Pts',(-1.58917696700006,12.2,-3.92031069400002));
#323866=CARTESIAN_POINT('Ctrl Pts',(-1.58917696700006,5.2,-3.92031069400002));
#323867=CARTESIAN_POINT('Ctrl Pts',(-1.58917696700006,2.2,-3.92031069400002));
#323868=CARTESIAN_POINT('Ctrl Pts',(-1.58925535800006,12.2,-3.92192234100001));
#323869=CARTESIAN_POINT('Ctrl Pts',(-1.58925535800006,5.2,-3.92192234100001));
#323870=CARTESIAN_POINT('Ctrl Pts',(-1.58925535800006,2.2,-3.92192234100001));
#323871=CARTESIAN_POINT('Ctrl Pts',(-1.58933210400006,12.2,-3.92353862800002));
#323872=CARTESIAN_POINT('Ctrl Pts',(-1.58933210400006,5.2,-3.92353862800002));
#323873=CARTESIAN_POINT('Ctrl Pts',(-1.58933210400006,2.2,-3.92353862800002));
#323874=CARTESIAN_POINT('Ctrl Pts',(-1.58940719400006,12.2,-3.92515955000002));
#323875=CARTESIAN_POINT('Ctrl Pts',(-1.58940719400006,5.2,-3.92515955000002));
#323876=CARTESIAN_POINT('Ctrl Pts',(-1.58940719400006,2.2,-3.92515955000002));
#323877=CARTESIAN_POINT('Ctrl Pts',(-1.58948062000006,12.2,-3.92678509900001));
#323878=CARTESIAN_POINT('Ctrl Pts',(-1.58948062000006,5.2,-3.92678509900001));
#323879=CARTESIAN_POINT('Ctrl Pts',(-1.58948062000006,2.2,-3.92678509900001));
#323880=CARTESIAN_POINT('Ctrl Pts',(-1.58955237000006,12.2,-3.92841526600002));
#323881=CARTESIAN_POINT('Ctrl Pts',(-1.58955237000006,5.2,-3.92841526600002));
#323882=CARTESIAN_POINT('Ctrl Pts',(-1.58955237000006,2.2,-3.92841526600002));
#323883=CARTESIAN_POINT('Ctrl Pts',(-1.58962243600006,12.2,-3.93005004400001));
#323884=CARTESIAN_POINT('Ctrl Pts',(-1.58962243600006,5.2,-3.93005004400001));
#323885=CARTESIAN_POINT('Ctrl Pts',(-1.58962243600006,2.2,-3.93005004400001));
#323886=CARTESIAN_POINT('Ctrl Pts',(-1.58969080700006,12.2,-3.93168942500001));
#323887=CARTESIAN_POINT('Ctrl Pts',(-1.58969080700006,5.2,-3.93168942500001));
#323888=CARTESIAN_POINT('Ctrl Pts',(-1.58969080700006,2.2,-3.93168942500001));
#323889=CARTESIAN_POINT('Ctrl Pts',(-1.58975747200006,12.2,-3.93333340100002));
#323890=CARTESIAN_POINT('Ctrl Pts',(-1.58975747200006,5.2,-3.93333340100002));
#323891=CARTESIAN_POINT('Ctrl Pts',(-1.58975747200006,2.2,-3.93333340100002));
#323892=CARTESIAN_POINT('Ctrl Pts',(-1.58982242300006,12.2,-3.93498196400001));
#323893=CARTESIAN_POINT('Ctrl Pts',(-1.58982242300006,5.2,-3.93498196400001));
#323894=CARTESIAN_POINT('Ctrl Pts',(-1.58982242300006,2.2,-3.93498196400001));
#323895=CARTESIAN_POINT('Ctrl Pts',(-1.58988565000006,12.2,-3.93663510600001));
#323896=CARTESIAN_POINT('Ctrl Pts',(-1.58988565000006,5.2,-3.93663510600001));
#323897=CARTESIAN_POINT('Ctrl Pts',(-1.58988565000006,2.2,-3.93663510600001));
#323898=CARTESIAN_POINT('Ctrl Pts',(-1.58994714200006,12.2,-3.93829282200001));
#323899=CARTESIAN_POINT('Ctrl Pts',(-1.58994714200006,5.2,-3.93829282200001));
#323900=CARTESIAN_POINT('Ctrl Pts',(-1.58994714200006,2.2,-3.93829282200001));
#323901=CARTESIAN_POINT('Ctrl Pts',(-1.59000689100006,12.2,-3.93995509900002));
#323902=CARTESIAN_POINT('Ctrl Pts',(-1.59000689100006,5.2,-3.93995509900002));
#323903=CARTESIAN_POINT('Ctrl Pts',(-1.59000689100006,2.2,-3.93995509900002));
#323904=CARTESIAN_POINT('Ctrl Pts',(-1.59006488600005,12.2,-3.94162193300001));
#323905=CARTESIAN_POINT('Ctrl Pts',(-1.59006488600005,5.2,-3.94162193300001));
#323906=CARTESIAN_POINT('Ctrl Pts',(-1.59006488600005,2.2,-3.94162193300001));
#323907=CARTESIAN_POINT('Ctrl Pts',(-1.59012111700006,12.2,-3.94329331600002));
#323908=CARTESIAN_POINT('Ctrl Pts',(-1.59012111700006,5.2,-3.94329331600002));
#323909=CARTESIAN_POINT('Ctrl Pts',(-1.59012111700006,2.2,-3.94329331600002));
#323910=CARTESIAN_POINT('Ctrl Pts',(-1.59017557600006,12.2,-3.94496923900002));
#323911=CARTESIAN_POINT('Ctrl Pts',(-1.59017557600006,5.2,-3.94496923900002));
#323912=CARTESIAN_POINT('Ctrl Pts',(-1.59017557600006,2.2,-3.94496923900002));
#323913=CARTESIAN_POINT('Ctrl Pts',(-1.59022825200006,12.2,-3.94664969400001));
#323914=CARTESIAN_POINT('Ctrl Pts',(-1.59022825200006,5.2,-3.94664969400001));
#323915=CARTESIAN_POINT('Ctrl Pts',(-1.59022825200006,2.2,-3.94664969400001));
#323916=CARTESIAN_POINT('Ctrl Pts',(-1.59027913600006,12.2,-3.94833467500002));
#323917=CARTESIAN_POINT('Ctrl Pts',(-1.59027913600006,5.2,-3.94833467500002));
#323918=CARTESIAN_POINT('Ctrl Pts',(-1.59027913600006,2.2,-3.94833467500002));
#323919=CARTESIAN_POINT('Ctrl Pts',(-1.59032821800006,12.2,-3.95002417200002));
#323920=CARTESIAN_POINT('Ctrl Pts',(-1.59032821800006,5.2,-3.95002417200002));
#323921=CARTESIAN_POINT('Ctrl Pts',(-1.59032821800006,2.2,-3.95002417200002));
#323922=CARTESIAN_POINT('Ctrl Pts',(-1.59037548900006,12.2,-3.95171817900001));
#323923=CARTESIAN_POINT('Ctrl Pts',(-1.59037548900006,5.2,-3.95171817900001));
#323924=CARTESIAN_POINT('Ctrl Pts',(-1.59037548900006,2.2,-3.95171817900001));
#323925=CARTESIAN_POINT('Ctrl Pts',(-1.59042093900006,12.2,-3.95341668700001));
#323926=CARTESIAN_POINT('Ctrl Pts',(-1.59042093900006,5.2,-3.95341668700001));
#323927=CARTESIAN_POINT('Ctrl Pts',(-1.59042093900006,2.2,-3.95341668700001));
#323928=CARTESIAN_POINT('Ctrl Pts',(-1.59046455800006,12.2,-3.95511968800002));
#323929=CARTESIAN_POINT('Ctrl Pts',(-1.59046455800006,5.2,-3.95511968800002));
#323930=CARTESIAN_POINT('Ctrl Pts',(-1.59046455800006,2.2,-3.95511968800002));
#323931=CARTESIAN_POINT('Ctrl Pts',(-1.59050633700006,12.2,-3.95682717600002));
#323932=CARTESIAN_POINT('Ctrl Pts',(-1.59050633700006,5.2,-3.95682717600002));
#323933=CARTESIAN_POINT('Ctrl Pts',(-1.59050633700006,2.2,-3.95682717600002));
#323934=CARTESIAN_POINT('Ctrl Pts',(-1.59054626700006,12.2,-3.95853914200002));
#323935=CARTESIAN_POINT('Ctrl Pts',(-1.59054626700006,5.2,-3.95853914200002));
#323936=CARTESIAN_POINT('Ctrl Pts',(-1.59054626700006,2.2,-3.95853914200002));
#323937=CARTESIAN_POINT('Ctrl Pts',(-1.59058434000006,12.2,-3.96025557800002));
#323938=CARTESIAN_POINT('Ctrl Pts',(-1.59058434000006,5.2,-3.96025557800002));
#323939=CARTESIAN_POINT('Ctrl Pts',(-1.59058434000006,2.2,-3.96025557800002));
#323940=CARTESIAN_POINT('Ctrl Pts',(-1.59062054300006,12.2,-3.96197647600002));
#323941=CARTESIAN_POINT('Ctrl Pts',(-1.59062054300006,5.2,-3.96197647600002));
#323942=CARTESIAN_POINT('Ctrl Pts',(-1.59062054300006,2.2,-3.96197647600002));
#323943=CARTESIAN_POINT('Ctrl Pts',(-1.59065486900006,12.2,-3.96370182900001));
#323944=CARTESIAN_POINT('Ctrl Pts',(-1.59065486900006,5.2,-3.96370182900001));
#323945=CARTESIAN_POINT('Ctrl Pts',(-1.59065486900006,2.2,-3.96370182900001));
#323946=CARTESIAN_POINT('Ctrl Pts',(-1.59068730800006,12.2,-3.96543163000001));
#323947=CARTESIAN_POINT('Ctrl Pts',(-1.59068730800006,5.2,-3.96543163000001));
#323948=CARTESIAN_POINT('Ctrl Pts',(-1.59068730800006,2.2,-3.96543163000001));
#323949=CARTESIAN_POINT('Ctrl Pts',(-1.59071785200006,12.2,-3.96716586900002));
#323950=CARTESIAN_POINT('Ctrl Pts',(-1.59071785200006,5.2,-3.96716586900002));
#323951=CARTESIAN_POINT('Ctrl Pts',(-1.59071785200006,2.2,-3.96716586900002));
#323952=CARTESIAN_POINT('Ctrl Pts',(-1.59074649000006,12.2,-3.96890453900001));
#323953=CARTESIAN_POINT('Ctrl Pts',(-1.59074649000006,5.2,-3.96890453900001));
#323954=CARTESIAN_POINT('Ctrl Pts',(-1.59074649000006,2.2,-3.96890453900001));
#323955=CARTESIAN_POINT('Ctrl Pts',(-1.59077321300006,12.2,-3.97064763300001));
#323956=CARTESIAN_POINT('Ctrl Pts',(-1.59077321300006,5.2,-3.97064763300001));
#323957=CARTESIAN_POINT('Ctrl Pts',(-1.59077321300006,2.2,-3.97064763300001));
#323958=CARTESIAN_POINT('Ctrl Pts',(-1.59079801300006,12.2,-3.97239514300002));
#323959=CARTESIAN_POINT('Ctrl Pts',(-1.59079801300006,5.2,-3.97239514300002));
#323960=CARTESIAN_POINT('Ctrl Pts',(-1.59079801300006,2.2,-3.97239514300002));
#323961=CARTESIAN_POINT('Ctrl Pts',(-1.59082087900006,12.2,-3.97414706000002));
#323962=CARTESIAN_POINT('Ctrl Pts',(-1.59082087900006,5.2,-3.97414706000002));
#323963=CARTESIAN_POINT('Ctrl Pts',(-1.59082087900006,2.2,-3.97414706000002));
#323964=CARTESIAN_POINT('Ctrl Pts',(-1.59084180300006,12.2,-3.97590337900001));
#323965=CARTESIAN_POINT('Ctrl Pts',(-1.59084180300006,5.2,-3.97590337900001));
#323966=CARTESIAN_POINT('Ctrl Pts',(-1.59084180300006,2.2,-3.97590337900001));
#323967=CARTESIAN_POINT('Ctrl Pts',(-1.59086077700006,12.2,-3.97766408900001));
#323968=CARTESIAN_POINT('Ctrl Pts',(-1.59086077700006,5.2,-3.97766408900001));
#323969=CARTESIAN_POINT('Ctrl Pts',(-1.59086077700006,2.2,-3.97766408900001));
#323970=CARTESIAN_POINT('Ctrl Pts',(-1.59087779000005,12.2,-3.97942918500001));
#323971=CARTESIAN_POINT('Ctrl Pts',(-1.59087779000005,5.2,-3.97942918500001));
#323972=CARTESIAN_POINT('Ctrl Pts',(-1.59087779000005,2.2,-3.97942918500001));
#323973=CARTESIAN_POINT('Ctrl Pts',(-1.59089283300006,12.2,-3.98119865700002));
#323974=CARTESIAN_POINT('Ctrl Pts',(-1.59089283300006,5.2,-3.98119865700002));
#323975=CARTESIAN_POINT('Ctrl Pts',(-1.59089283300006,2.2,-3.98119865700002));
#323976=CARTESIAN_POINT('Ctrl Pts',(-1.59090589800006,12.2,-3.98297249800001));
#323977=CARTESIAN_POINT('Ctrl Pts',(-1.59090589800006,5.2,-3.98297249800001));
#323978=CARTESIAN_POINT('Ctrl Pts',(-1.59090589800006,2.2,-3.98297249800001));
#323979=CARTESIAN_POINT('Ctrl Pts',(-1.59091697500006,12.2,-3.98475070100002));
#323980=CARTESIAN_POINT('Ctrl Pts',(-1.59091697500006,5.2,-3.98475070100002));
#323981=CARTESIAN_POINT('Ctrl Pts',(-1.59091697500006,2.2,-3.98475070100002));
#323982=CARTESIAN_POINT('Ctrl Pts',(-1.59092605600006,12.2,-3.98653325700002));
#323983=CARTESIAN_POINT('Ctrl Pts',(-1.59092605600006,5.2,-3.98653325700002));
#323984=CARTESIAN_POINT('Ctrl Pts',(-1.59092605600006,2.2,-3.98653325700002));
#323985=CARTESIAN_POINT('Ctrl Pts',(-1.59093313200006,12.2,-3.98832015800001));
#323986=CARTESIAN_POINT('Ctrl Pts',(-1.59093313200006,5.2,-3.98832015800001));
#323987=CARTESIAN_POINT('Ctrl Pts',(-1.59093313200006,2.2,-3.98832015800001));
#323988=CARTESIAN_POINT('Ctrl Pts',(-1.59093819200006,12.2,-3.99011139900002));
#323989=CARTESIAN_POINT('Ctrl Pts',(-1.59093819200006,5.2,-3.99011139900002));
#323990=CARTESIAN_POINT('Ctrl Pts',(-1.59093819200006,2.2,-3.99011139900002));
#323991=CARTESIAN_POINT('Ctrl Pts',(-1.59094123000005,12.2,-3.99190697000002));
#323992=CARTESIAN_POINT('Ctrl Pts',(-1.59094123000005,5.2,-3.99190697000002));
#323993=CARTESIAN_POINT('Ctrl Pts',(-1.59094123000005,2.2,-3.99190697000002));
#323994=CARTESIAN_POINT('Ctrl Pts',(-1.59094223500006,12.2,-3.99370686200001));
#323995=CARTESIAN_POINT('Ctrl Pts',(-1.59094223500006,5.2,-3.99370686200001));
#323996=CARTESIAN_POINT('Ctrl Pts',(-1.59094223500006,2.2,-3.99370686200001));
#323997=CARTESIAN_POINT('Ctrl Pts',(-1.59094120000006,12.2,-3.99551107000002));
#323998=CARTESIAN_POINT('Ctrl Pts',(-1.59094120000006,5.2,-3.99551107000002));
#323999=CARTESIAN_POINT('Ctrl Pts',(-1.59094120000006,2.2,-3.99551107000002));
#324000=CARTESIAN_POINT('Ctrl Pts',(-1.59093811300006,12.2,-3.99731958500002));
#324001=CARTESIAN_POINT('Ctrl Pts',(-1.59093811300006,5.2,-3.99731958500002));
#324002=CARTESIAN_POINT('Ctrl Pts',(-1.59093811300006,2.2,-3.99731958500002));
#324003=CARTESIAN_POINT('Ctrl Pts',(-1.59093296700005,12.2,-3.99913239900001));
#324004=CARTESIAN_POINT('Ctrl Pts',(-1.59093296700005,5.2,-3.99913239900001));
#324005=CARTESIAN_POINT('Ctrl Pts',(-1.59093296700005,2.2,-3.99913239900001));
#324006=CARTESIAN_POINT('Ctrl Pts',(-1.59092575600006,12.2,-4.00094950500002));
#324007=CARTESIAN_POINT('Ctrl Pts',(-1.59092575600006,5.2,-4.00094950500002));
#324008=CARTESIAN_POINT('Ctrl Pts',(-1.59092575600006,2.2,-4.00094950500002));
#324009=CARTESIAN_POINT('Ctrl Pts',(-1.59091646700006,12.2,-4.00277089400001));
#324010=CARTESIAN_POINT('Ctrl Pts',(-1.59091646700006,5.2,-4.00277089400001));
#324011=CARTESIAN_POINT('Ctrl Pts',(-1.59091646700006,2.2,-4.00277089400001));
#324012=CARTESIAN_POINT('Ctrl Pts',(-1.59090509200006,12.2,-4.00459656000002));
#324013=CARTESIAN_POINT('Ctrl Pts',(-1.59090509200006,5.2,-4.00459656000002));
#324014=CARTESIAN_POINT('Ctrl Pts',(-1.59090509200006,2.2,-4.00459656000002));
#324015=CARTESIAN_POINT('Ctrl Pts',(-1.59089162400006,12.2,-4.00642649300002));
#324016=CARTESIAN_POINT('Ctrl Pts',(-1.59089162400006,5.2,-4.00642649300002));
#324017=CARTESIAN_POINT('Ctrl Pts',(-1.59089162400006,2.2,-4.00642649300002));
#324018=CARTESIAN_POINT('Ctrl Pts',(-1.59087605400006,12.2,-4.00826068700002));
#324019=CARTESIAN_POINT('Ctrl Pts',(-1.59087605400006,5.2,-4.00826068700002));
#324020=CARTESIAN_POINT('Ctrl Pts',(-1.59087605400006,2.2,-4.00826068700002));
#324021=CARTESIAN_POINT('Ctrl Pts',(-1.59085837300006,12.2,-4.01009913300001));
#324022=CARTESIAN_POINT('Ctrl Pts',(-1.59085837300006,5.2,-4.01009913300001));
#324023=CARTESIAN_POINT('Ctrl Pts',(-1.59085837300006,2.2,-4.01009913300001));
#324024=CARTESIAN_POINT('Ctrl Pts',(-1.59083857100006,12.2,-4.01194182600001));
#324025=CARTESIAN_POINT('Ctrl Pts',(-1.59083857100006,5.2,-4.01194182600001));
#324026=CARTESIAN_POINT('Ctrl Pts',(-1.59083857100006,2.2,-4.01194182600001));
#324027=CARTESIAN_POINT('Ctrl Pts',(-1.59081664100006,12.2,-4.01378875500002));
#324028=CARTESIAN_POINT('Ctrl Pts',(-1.59081664100006,5.2,-4.01378875500002));
#324029=CARTESIAN_POINT('Ctrl Pts',(-1.59081664100006,2.2,-4.01378875500002));
#324030=CARTESIAN_POINT('Ctrl Pts',(-1.59079257400006,12.2,-4.01563991400002));
#324031=CARTESIAN_POINT('Ctrl Pts',(-1.59079257400006,5.2,-4.01563991400002));
#324032=CARTESIAN_POINT('Ctrl Pts',(-1.59079257400006,2.2,-4.01563991400002));
#324033=CARTESIAN_POINT('Ctrl Pts',(-1.59076636100006,12.2,-4.01749529400002));
#324034=CARTESIAN_POINT('Ctrl Pts',(-1.59076636100006,5.2,-4.01749529400002));
#324035=CARTESIAN_POINT('Ctrl Pts',(-1.59076636100006,2.2,-4.01749529400002));
#324036=CARTESIAN_POINT('Ctrl Pts',(-1.59073799500006,12.2,-4.01935488800001));
#324037=CARTESIAN_POINT('Ctrl Pts',(-1.59073799500006,5.2,-4.01935488800001));
#324038=CARTESIAN_POINT('Ctrl Pts',(-1.59073799500006,2.2,-4.01935488800001));
#324039=CARTESIAN_POINT('Ctrl Pts',(-1.59070746500006,12.2,-4.02121868900001));
#324040=CARTESIAN_POINT('Ctrl Pts',(-1.59070746500006,5.2,-4.02121868900001));
#324041=CARTESIAN_POINT('Ctrl Pts',(-1.59070746500006,2.2,-4.02121868900001));
#324042=CARTESIAN_POINT('Ctrl Pts',(-1.59067476500006,12.2,-4.02308668800002));
#324043=CARTESIAN_POINT('Ctrl Pts',(-1.59067476500006,5.2,-4.02308668800002));
#324044=CARTESIAN_POINT('Ctrl Pts',(-1.59067476500006,2.2,-4.02308668800002));
#324045=CARTESIAN_POINT('Ctrl Pts',(-1.59063988400006,12.2,-4.02495887800002));
#324046=CARTESIAN_POINT('Ctrl Pts',(-1.59063988400006,5.2,-4.02495887800002));
#324047=CARTESIAN_POINT('Ctrl Pts',(-1.59063988400006,2.2,-4.02495887800002));
#324048=CARTESIAN_POINT('Ctrl Pts',(-1.59060281600006,12.2,-4.02683525200001));
#324049=CARTESIAN_POINT('Ctrl Pts',(-1.59060281600006,5.2,-4.02683525200001));
#324050=CARTESIAN_POINT('Ctrl Pts',(-1.59060281600006,2.2,-4.02683525200001));
#324051=CARTESIAN_POINT('Ctrl Pts',(-1.59056355200006,12.2,-4.02871580100001));
#324052=CARTESIAN_POINT('Ctrl Pts',(-1.59056355200006,5.2,-4.02871580100001));
#324053=CARTESIAN_POINT('Ctrl Pts',(-1.59056355200006,2.2,-4.02871580100001));
#324054=CARTESIAN_POINT('Ctrl Pts',(-1.59052208200006,12.2,-4.03060051700002));
#324055=CARTESIAN_POINT('Ctrl Pts',(-1.59052208200006,5.2,-4.03060051700002));
#324056=CARTESIAN_POINT('Ctrl Pts',(-1.59052208200006,2.2,-4.03060051700002));
#324057=CARTESIAN_POINT('Ctrl Pts',(-1.59047840000006,12.2,-4.03248939400001));
#324058=CARTESIAN_POINT('Ctrl Pts',(-1.59047840000006,5.2,-4.03248939400001));
#324059=CARTESIAN_POINT('Ctrl Pts',(-1.59047840000006,2.2,-4.03248939400001));
#324060=CARTESIAN_POINT('Ctrl Pts',(-1.59043249400006,12.2,-4.03438242200002));
#324061=CARTESIAN_POINT('Ctrl Pts',(-1.59043249400006,5.2,-4.03438242200002));
#324062=CARTESIAN_POINT('Ctrl Pts',(-1.59043249400006,2.2,-4.03438242200002));
#324063=CARTESIAN_POINT('Ctrl Pts',(-1.59038436000006,12.2,-4.03627959500001));
#324064=CARTESIAN_POINT('Ctrl Pts',(-1.59038436000006,5.2,-4.03627959500001));
#324065=CARTESIAN_POINT('Ctrl Pts',(-1.59038436000006,2.2,-4.03627959500001));
#324066=CARTESIAN_POINT('Ctrl Pts',(-1.59033398800006,12.2,-4.03818090400001));
#324067=CARTESIAN_POINT('Ctrl Pts',(-1.59033398800006,5.2,-4.03818090400001));
#324068=CARTESIAN_POINT('Ctrl Pts',(-1.59033398800006,2.2,-4.03818090400001));
#324069=CARTESIAN_POINT('Ctrl Pts',(-1.59028137000006,12.2,-4.04008634300002));
#324070=CARTESIAN_POINT('Ctrl Pts',(-1.59028137000006,5.2,-4.04008634300002));
#324071=CARTESIAN_POINT('Ctrl Pts',(-1.59028137000006,2.2,-4.04008634300002));
#324072=CARTESIAN_POINT('Ctrl Pts',(-1.59022649600006,12.2,-4.04199590300002));
#324073=CARTESIAN_POINT('Ctrl Pts',(-1.59022649600006,5.2,-4.04199590300002));
#324074=CARTESIAN_POINT('Ctrl Pts',(-1.59022649600006,2.2,-4.04199590300002));
#324075=CARTESIAN_POINT('Ctrl Pts',(-1.59016936000006,12.2,-4.04390957600001));
#324076=CARTESIAN_POINT('Ctrl Pts',(-1.59016936000006,5.2,-4.04390957600001));
#324077=CARTESIAN_POINT('Ctrl Pts',(-1.59016936000006,2.2,-4.04390957600001));
#324078=CARTESIAN_POINT('Ctrl Pts',(-1.59010995200006,12.2,-4.04582735600002));
#324079=CARTESIAN_POINT('Ctrl Pts',(-1.59010995200006,5.2,-4.04582735600002));
#324080=CARTESIAN_POINT('Ctrl Pts',(-1.59010995200006,2.2,-4.04582735600002));
#324081=CARTESIAN_POINT('Ctrl Pts',(-1.59004826600006,12.2,-4.04774923300002));
#324082=CARTESIAN_POINT('Ctrl Pts',(-1.59004826600006,5.2,-4.04774923300002));
#324083=CARTESIAN_POINT('Ctrl Pts',(-1.59004826600006,2.2,-4.04774923300002));
#324084=CARTESIAN_POINT('Ctrl Pts',(-1.58998429200006,12.2,-4.04967520200001));
#324085=CARTESIAN_POINT('Ctrl Pts',(-1.58998429200006,5.2,-4.04967520200001));
#324086=CARTESIAN_POINT('Ctrl Pts',(-1.58998429200006,2.2,-4.04967520200001));
#324087=CARTESIAN_POINT('Ctrl Pts',(-1.58991802200006,12.2,-4.05160525300001));
#324088=CARTESIAN_POINT('Ctrl Pts',(-1.58991802200006,5.2,-4.05160525300001));
#324089=CARTESIAN_POINT('Ctrl Pts',(-1.58991802200006,2.2,-4.05160525300001));
#324090=CARTESIAN_POINT('Ctrl Pts',(-1.58984944900005,12.2,-4.05353937800002));
#324091=CARTESIAN_POINT('Ctrl Pts',(-1.58984944900005,5.2,-4.05353937800002));
#324092=CARTESIAN_POINT('Ctrl Pts',(-1.58984944900005,2.2,-4.05353937800002));
#324093=CARTESIAN_POINT('Ctrl Pts',(-1.58977856400006,12.2,-4.05547757100001));
#324094=CARTESIAN_POINT('Ctrl Pts',(-1.58977856400006,5.2,-4.05547757100001));
#324095=CARTESIAN_POINT('Ctrl Pts',(-1.58977856400006,2.2,-4.05547757100001));
#324096=CARTESIAN_POINT('Ctrl Pts',(-1.58970535900006,12.2,-4.05741982400002));
#324097=CARTESIAN_POINT('Ctrl Pts',(-1.58970535900006,5.2,-4.05741982400002));
#324098=CARTESIAN_POINT('Ctrl Pts',(-1.58970535900006,2.2,-4.05741982400002));
#324099=CARTESIAN_POINT('Ctrl Pts',(-1.58962982700006,12.2,-4.05936612800001));
#324100=CARTESIAN_POINT('Ctrl Pts',(-1.58962982700006,5.2,-4.05936612800001));
#324101=CARTESIAN_POINT('Ctrl Pts',(-1.58962982700006,2.2,-4.05936612800001));
#324102=CARTESIAN_POINT('Ctrl Pts',(-1.58955195800006,12.2,-4.06131647700001));
#324103=CARTESIAN_POINT('Ctrl Pts',(-1.58955195800006,5.2,-4.06131647700001));
#324104=CARTESIAN_POINT('Ctrl Pts',(-1.58955195800006,2.2,-4.06131647700001));
#324105=CARTESIAN_POINT('Ctrl Pts',(-1.58947174700006,12.2,-4.06327086300001));
#324106=CARTESIAN_POINT('Ctrl Pts',(-1.58947174700006,5.2,-4.06327086300001));
#324107=CARTESIAN_POINT('Ctrl Pts',(-1.58947174700006,2.2,-4.06327086300001));
#324108=CARTESIAN_POINT('Ctrl Pts',(-1.58938918300006,12.2,-4.06522927600002));
#324109=CARTESIAN_POINT('Ctrl Pts',(-1.58938918300006,5.2,-4.06522927600002));
#324110=CARTESIAN_POINT('Ctrl Pts',(-1.58938918300006,2.2,-4.06522927600002));
#324111=CARTESIAN_POINT('Ctrl Pts',(-1.58930425900006,12.2,-4.06719171200002));
#324112=CARTESIAN_POINT('Ctrl Pts',(-1.58930425900006,5.2,-4.06719171200002));
#324113=CARTESIAN_POINT('Ctrl Pts',(-1.58930425900006,2.2,-4.06719171200002));
#324114=CARTESIAN_POINT('Ctrl Pts',(-1.58921696800005,12.2,-4.06915816000001));
#324115=CARTESIAN_POINT('Ctrl Pts',(-1.58921696800005,5.2,-4.06915816000001));
#324116=CARTESIAN_POINT('Ctrl Pts',(-1.58921696800005,2.2,-4.06915816000001));
#324117=CARTESIAN_POINT('Ctrl Pts',(-1.58912730200006,12.2,-4.07112861400002));
#324118=CARTESIAN_POINT('Ctrl Pts',(-1.58912730200006,5.2,-4.07112861400002));
#324119=CARTESIAN_POINT('Ctrl Pts',(-1.58912730200006,2.2,-4.07112861400002));
#324120=CARTESIAN_POINT('Ctrl Pts',(-1.58903525200006,12.2,-4.07310306600001));
#324121=CARTESIAN_POINT('Ctrl Pts',(-1.58903525200006,5.2,-4.07310306600001));
#324122=CARTESIAN_POINT('Ctrl Pts',(-1.58903525200006,2.2,-4.07310306600001));
#324123=CARTESIAN_POINT('Ctrl Pts',(-1.58894081100006,12.2,-4.07508150900001));
#324124=CARTESIAN_POINT('Ctrl Pts',(-1.58894081100006,5.2,-4.07508150900001));
#324125=CARTESIAN_POINT('Ctrl Pts',(-1.58894081100006,2.2,-4.07508150900001));
#324126=CARTESIAN_POINT('Ctrl Pts',(-1.58884397200006,12.2,-4.07706393400002));
#324127=CARTESIAN_POINT('Ctrl Pts',(-1.58884397200006,5.2,-4.07706393400002));
#324128=CARTESIAN_POINT('Ctrl Pts',(-1.58884397200006,2.2,-4.07706393400002));
#324129=CARTESIAN_POINT('Ctrl Pts',(-1.58874472600006,12.2,-4.07905033500001));
#324130=CARTESIAN_POINT('Ctrl Pts',(-1.58874472600006,5.2,-4.07905033500001));
#324131=CARTESIAN_POINT('Ctrl Pts',(-1.58874472600006,2.2,-4.07905033500001));
#324132=CARTESIAN_POINT('Ctrl Pts',(-1.58864306500006,12.2,-4.08104070300002));
#324133=CARTESIAN_POINT('Ctrl Pts',(-1.58864306500006,5.2,-4.08104070300002));
#324134=CARTESIAN_POINT('Ctrl Pts',(-1.58864306500006,2.2,-4.08104070300002));
#324135=CARTESIAN_POINT('Ctrl Pts',(-1.58853898100005,12.2,-4.08303502800001));
#324136=CARTESIAN_POINT('Ctrl Pts',(-1.58853898100005,5.2,-4.08303502800001));
#324137=CARTESIAN_POINT('Ctrl Pts',(-1.58853898100005,2.2,-4.08303502800001));
#324138=CARTESIAN_POINT('Ctrl Pts',(-1.58843246800005,12.2,-4.08503330800002));
#324139=CARTESIAN_POINT('Ctrl Pts',(-1.58843246800005,5.2,-4.08503330800002));
#324140=CARTESIAN_POINT('Ctrl Pts',(-1.58843246800005,2.2,-4.08503330800002));
#324141=CARTESIAN_POINT('Ctrl Pts',(-1.58832351800006,12.2,-4.08703553000001));
#324142=CARTESIAN_POINT('Ctrl Pts',(-1.58832351800006,5.2,-4.08703553000001));
#324143=CARTESIAN_POINT('Ctrl Pts',(-1.58832351800006,2.2,-4.08703553000001));
#324144=CARTESIAN_POINT('Ctrl Pts',(-1.58821212100006,12.2,-4.08904169000001));
#324145=CARTESIAN_POINT('Ctrl Pts',(-1.58821212100006,5.2,-4.08904169000001));
#324146=CARTESIAN_POINT('Ctrl Pts',(-1.58821212100006,2.2,-4.08904169000001));
#324147=CARTESIAN_POINT('Ctrl Pts',(-1.58809827200006,12.2,-4.09105177800001));
#324148=CARTESIAN_POINT('Ctrl Pts',(-1.58809827200006,5.2,-4.09105177800001));
#324149=CARTESIAN_POINT('Ctrl Pts',(-1.58809827200006,2.2,-4.09105177800001));
#324150=CARTESIAN_POINT('Ctrl Pts',(-1.58798196200005,12.2,-4.09306578800001));
#324151=CARTESIAN_POINT('Ctrl Pts',(-1.58798196200005,5.2,-4.09306578800001));
#324152=CARTESIAN_POINT('Ctrl Pts',(-1.58798196200005,2.2,-4.09306578800001));
#324153=CARTESIAN_POINT('Ctrl Pts',(-1.58786318400006,12.2,-4.09508371000001));
#324154=CARTESIAN_POINT('Ctrl Pts',(-1.58786318400006,5.2,-4.09508371000001));
#324155=CARTESIAN_POINT('Ctrl Pts',(-1.58786318400006,2.2,-4.09508371000001));
#324156=CARTESIAN_POINT('Ctrl Pts',(-1.58774193000006,12.2,-4.09710553900001));
#324157=CARTESIAN_POINT('Ctrl Pts',(-1.58774193000006,5.2,-4.09710553900001));
#324158=CARTESIAN_POINT('Ctrl Pts',(-1.58774193000006,2.2,-4.09710553900001));
#324159=CARTESIAN_POINT('Ctrl Pts',(-1.58761819200006,12.2,-4.09913126700001));
#324160=CARTESIAN_POINT('Ctrl Pts',(-1.58761819200006,5.2,-4.09913126700001));
#324161=CARTESIAN_POINT('Ctrl Pts',(-1.58761819200006,2.2,-4.09913126700001));
#324162=CARTESIAN_POINT('Ctrl Pts',(-1.58749196400006,12.2,-4.10116088400001));
#324163=CARTESIAN_POINT('Ctrl Pts',(-1.58749196400006,5.2,-4.10116088400001));
#324164=CARTESIAN_POINT('Ctrl Pts',(-1.58749196400006,2.2,-4.10116088400001));
#324165=CARTESIAN_POINT('Ctrl Pts',(-1.58736323700006,12.2,-4.10319438400002));
#324166=CARTESIAN_POINT('Ctrl Pts',(-1.58736323700006,5.2,-4.10319438400002));
#324167=CARTESIAN_POINT('Ctrl Pts',(-1.58736323700006,2.2,-4.10319438400002));
#324168=CARTESIAN_POINT('Ctrl Pts',(-1.58723200500006,12.2,-4.10523176000002));
#324169=CARTESIAN_POINT('Ctrl Pts',(-1.58723200500006,5.2,-4.10523176000002));
#324170=CARTESIAN_POINT('Ctrl Pts',(-1.58723200500006,2.2,-4.10523176000002));
#324171=CARTESIAN_POINT('Ctrl Pts',(-1.58709825800006,12.2,-4.10727300300001));
#324172=CARTESIAN_POINT('Ctrl Pts',(-1.58709825800006,5.2,-4.10727300300001));
#324173=CARTESIAN_POINT('Ctrl Pts',(-1.58709825800006,2.2,-4.10727300300001));
#324174=CARTESIAN_POINT('Ctrl Pts',(-1.58696199100006,12.2,-4.10931810600002));
#324175=CARTESIAN_POINT('Ctrl Pts',(-1.58696199100006,5.2,-4.10931810600002));
#324176=CARTESIAN_POINT('Ctrl Pts',(-1.58696199100006,2.2,-4.10931810600002));
#324177=CARTESIAN_POINT('Ctrl Pts',(-1.58682319500006,12.2,-4.11136706100002));
#324178=CARTESIAN_POINT('Ctrl Pts',(-1.58682319500006,5.2,-4.11136706100002));
#324179=CARTESIAN_POINT('Ctrl Pts',(-1.58682319500006,2.2,-4.11136706100002));
#324180=CARTESIAN_POINT('Ctrl Pts',(-1.58668186400006,12.2,-4.11341985900001));
#324181=CARTESIAN_POINT('Ctrl Pts',(-1.58668186400006,5.2,-4.11341985900001));
#324182=CARTESIAN_POINT('Ctrl Pts',(-1.58668186400006,2.2,-4.11341985900001));
#324183=CARTESIAN_POINT('Ctrl Pts',(-1.58653799000006,12.2,-4.11547649600001));
#324184=CARTESIAN_POINT('Ctrl Pts',(-1.58653799000006,5.2,-4.11547649600001));
#324185=CARTESIAN_POINT('Ctrl Pts',(-1.58653799000006,2.2,-4.11547649600001));
#324186=CARTESIAN_POINT('Ctrl Pts',(-1.58639156500006,12.2,-4.11753696100002));
#324187=CARTESIAN_POINT('Ctrl Pts',(-1.58639156500006,5.2,-4.11753696100002));
#324188=CARTESIAN_POINT('Ctrl Pts',(-1.58639156500006,2.2,-4.11753696100002));
#324189=CARTESIAN_POINT('Ctrl Pts',(-1.58624258200006,12.2,-4.11960124800002));
#324190=CARTESIAN_POINT('Ctrl Pts',(-1.58624258200006,5.2,-4.11960124800002));
#324191=CARTESIAN_POINT('Ctrl Pts',(-1.58624258200006,2.2,-4.11960124800002));
#324192=CARTESIAN_POINT('Ctrl Pts',(-1.58609103400006,12.2,-4.12166934900001));
#324193=CARTESIAN_POINT('Ctrl Pts',(-1.58609103400006,5.2,-4.12166934900001));
#324194=CARTESIAN_POINT('Ctrl Pts',(-1.58609103400006,2.2,-4.12166934900001));
#324195=CARTESIAN_POINT('Ctrl Pts',(-1.58593691400006,12.2,-4.12374125600001));
#324196=CARTESIAN_POINT('Ctrl Pts',(-1.58593691400006,5.2,-4.12374125600001));
#324197=CARTESIAN_POINT('Ctrl Pts',(-1.58593691400006,2.2,-4.12374125600001));
#324198=CARTESIAN_POINT('Ctrl Pts',(-1.58578021300006,12.2,-4.12581696100002));
#324199=CARTESIAN_POINT('Ctrl Pts',(-1.58578021300006,5.2,-4.12581696100002));
#324200=CARTESIAN_POINT('Ctrl Pts',(-1.58578021300006,2.2,-4.12581696100002));
#324201=CARTESIAN_POINT('Ctrl Pts',(-1.58562092600006,12.2,-4.12789645800002));
#324202=CARTESIAN_POINT('Ctrl Pts',(-1.58562092600006,5.2,-4.12789645800002));
#324203=CARTESIAN_POINT('Ctrl Pts',(-1.58562092600006,2.2,-4.12789645800002));
#324204=CARTESIAN_POINT('Ctrl Pts',(-1.58545904500006,12.2,-4.12997973800001));
#324205=CARTESIAN_POINT('Ctrl Pts',(-1.58545904500006,5.2,-4.12997973800001));
#324206=CARTESIAN_POINT('Ctrl Pts',(-1.58545904500006,2.2,-4.12997973800001));
#324207=CARTESIAN_POINT('Ctrl Pts',(-1.58529456300006,12.2,-4.13206679300002));
#324208=CARTESIAN_POINT('Ctrl Pts',(-1.58529456300006,5.2,-4.13206679300002));
#324209=CARTESIAN_POINT('Ctrl Pts',(-1.58529456300006,2.2,-4.13206679300002));
#324210=CARTESIAN_POINT('Ctrl Pts',(-1.58512747100006,12.2,-4.13415761600001));
#324211=CARTESIAN_POINT('Ctrl Pts',(-1.58512747100006,5.2,-4.13415761600001));
#324212=CARTESIAN_POINT('Ctrl Pts',(-1.58512747100006,2.2,-4.13415761600001));
#324213=CARTESIAN_POINT('Ctrl Pts',(-1.58495776300006,12.2,-4.13625220100001));
#324214=CARTESIAN_POINT('Ctrl Pts',(-1.58495776300006,5.2,-4.13625220100001));
#324215=CARTESIAN_POINT('Ctrl Pts',(-1.58495776300006,2.2,-4.13625220100001));
#324216=CARTESIAN_POINT('Ctrl Pts',(-1.58478543300005,12.2,-4.13835053800002));
#324217=CARTESIAN_POINT('Ctrl Pts',(-1.58478543300005,5.2,-4.13835053800002));
#324218=CARTESIAN_POINT('Ctrl Pts',(-1.58478543300005,2.2,-4.13835053800002));
#324219=CARTESIAN_POINT('Ctrl Pts',(-1.58461047300006,12.2,-4.14045261900001));
#324220=CARTESIAN_POINT('Ctrl Pts',(-1.58461047300006,5.2,-4.14045261900001));
#324221=CARTESIAN_POINT('Ctrl Pts',(-1.58461047300006,2.2,-4.14045261900001));
#324222=CARTESIAN_POINT('Ctrl Pts',(-1.58443287500006,12.2,-4.14255843800001));
#324223=CARTESIAN_POINT('Ctrl Pts',(-1.58443287500006,5.2,-4.14255843800001));
#324224=CARTESIAN_POINT('Ctrl Pts',(-1.58443287500006,2.2,-4.14255843800001));
#324225=CARTESIAN_POINT('Ctrl Pts',(-1.58425263200005,12.2,-4.14466798700001));
#324226=CARTESIAN_POINT('Ctrl Pts',(-1.58425263200005,5.2,-4.14466798700001));
#324227=CARTESIAN_POINT('Ctrl Pts',(-1.58425263200005,2.2,-4.14466798700001));
#324228=CARTESIAN_POINT('Ctrl Pts',(-1.58406973900005,12.2,-4.14678125800001));
#324229=CARTESIAN_POINT('Ctrl Pts',(-1.58406973900005,5.2,-4.14678125800001));
#324230=CARTESIAN_POINT('Ctrl Pts',(-1.58406973900005,2.2,-4.14678125800001));
#324231=CARTESIAN_POINT('Ctrl Pts',(-1.58388418800006,12.2,-4.14889824300001));
#324232=CARTESIAN_POINT('Ctrl Pts',(-1.58388418800006,5.2,-4.14889824300001));
#324233=CARTESIAN_POINT('Ctrl Pts',(-1.58388418800006,2.2,-4.14889824300001));
#324234=CARTESIAN_POINT('Ctrl Pts',(-1.58369597100006,12.2,-4.15101893700002));
#324235=CARTESIAN_POINT('Ctrl Pts',(-1.58369597100006,5.2,-4.15101893700002));
#324236=CARTESIAN_POINT('Ctrl Pts',(-1.58369597100006,2.2,-4.15101893700002));
#324237=CARTESIAN_POINT('Ctrl Pts',(-1.58350508100006,12.2,-4.15314332800001));
#324238=CARTESIAN_POINT('Ctrl Pts',(-1.58350508100006,5.2,-4.15314332800001));
#324239=CARTESIAN_POINT('Ctrl Pts',(-1.58350508100006,2.2,-4.15314332800001));
#324240=CARTESIAN_POINT('Ctrl Pts',(-1.58331151200006,12.2,-4.15527141200001));
#324241=CARTESIAN_POINT('Ctrl Pts',(-1.58331151200006,5.2,-4.15527141200001));
#324242=CARTESIAN_POINT('Ctrl Pts',(-1.58331151200006,2.2,-4.15527141200001));
#324243=CARTESIAN_POINT('Ctrl Pts',(-1.58311525700006,12.2,-4.15740318000001));
#324244=CARTESIAN_POINT('Ctrl Pts',(-1.58311525700006,5.2,-4.15740318000001));
#324245=CARTESIAN_POINT('Ctrl Pts',(-1.58311525700006,2.2,-4.15740318000001));
#324246=CARTESIAN_POINT('Ctrl Pts',(-1.58291630800006,12.2,-4.15953862300002));
#324247=CARTESIAN_POINT('Ctrl Pts',(-1.58291630800006,5.2,-4.15953862300002));
#324248=CARTESIAN_POINT('Ctrl Pts',(-1.58291630800006,2.2,-4.15953862300002));
#324249=CARTESIAN_POINT('Ctrl Pts',(-1.58271465900006,12.2,-4.16167773700002));
#324250=CARTESIAN_POINT('Ctrl Pts',(-1.58271465900006,5.2,-4.16167773700002));
#324251=CARTESIAN_POINT('Ctrl Pts',(-1.58271465900006,2.2,-4.16167773700002));
#324252=CARTESIAN_POINT('Ctrl Pts',(-1.58251030300006,12.2,-4.16382051100001));
#324253=CARTESIAN_POINT('Ctrl Pts',(-1.58251030300006,5.2,-4.16382051100001));
#324254=CARTESIAN_POINT('Ctrl Pts',(-1.58251030300006,2.2,-4.16382051100001));
#324255=CARTESIAN_POINT('Ctrl Pts',(-1.58230323300006,12.2,-4.16596693800001));
#324256=CARTESIAN_POINT('Ctrl Pts',(-1.58230323300006,5.2,-4.16596693800001));
#324257=CARTESIAN_POINT('Ctrl Pts',(-1.58230323300006,2.2,-4.16596693800001));
#324258=CARTESIAN_POINT('Ctrl Pts',(-1.58209344200006,12.2,-4.16811701200002));
#324259=CARTESIAN_POINT('Ctrl Pts',(-1.58209344200006,5.2,-4.16811701200002));
#324260=CARTESIAN_POINT('Ctrl Pts',(-1.58209344200006,2.2,-4.16811701200002));
#324261=CARTESIAN_POINT('Ctrl Pts',(-1.58188092400006,12.2,-4.17027072500002));
#324262=CARTESIAN_POINT('Ctrl Pts',(-1.58188092400006,5.2,-4.17027072500002));
#324263=CARTESIAN_POINT('Ctrl Pts',(-1.58188092400006,2.2,-4.17027072500002));
#324264=CARTESIAN_POINT('Ctrl Pts',(-1.58166567100006,12.2,-4.17242806800001));
#324265=CARTESIAN_POINT('Ctrl Pts',(-1.58166567100006,5.2,-4.17242806800001));
#324266=CARTESIAN_POINT('Ctrl Pts',(-1.58166567100006,2.2,-4.17242806800001));
#324267=CARTESIAN_POINT('Ctrl Pts',(-1.58144767600006,12.2,-4.17458903300002));
#324268=CARTESIAN_POINT('Ctrl Pts',(-1.58144767600006,5.2,-4.17458903300002));
#324269=CARTESIAN_POINT('Ctrl Pts',(-1.58144767600006,2.2,-4.17458903300002));
#324270=CARTESIAN_POINT('Ctrl Pts',(-1.58122693300006,12.2,-4.17675361500002));
#324271=CARTESIAN_POINT('Ctrl Pts',(-1.58122693300006,5.2,-4.17675361500002));
#324272=CARTESIAN_POINT('Ctrl Pts',(-1.58122693300006,2.2,-4.17675361500002));
#324273=CARTESIAN_POINT('Ctrl Pts',(-1.58100343600006,12.2,-4.17892180400001));
#324274=CARTESIAN_POINT('Ctrl Pts',(-1.58100343600006,5.2,-4.17892180400001));
#324275=CARTESIAN_POINT('Ctrl Pts',(-1.58100343600006,2.2,-4.17892180400001));
#324276=CARTESIAN_POINT('Ctrl Pts',(-1.58077717700006,12.2,-4.18109359400002));
#324277=CARTESIAN_POINT('Ctrl Pts',(-1.58077717700006,5.2,-4.18109359400002));
#324278=CARTESIAN_POINT('Ctrl Pts',(-1.58077717700006,2.2,-4.18109359400002));
#324279=CARTESIAN_POINT('Ctrl Pts',(-1.58054815100006,12.2,-4.18326897700001));
#324280=CARTESIAN_POINT('Ctrl Pts',(-1.58054815100006,5.2,-4.18326897700001));
#324281=CARTESIAN_POINT('Ctrl Pts',(-1.58054815100006,2.2,-4.18326897700001));
#324282=CARTESIAN_POINT('Ctrl Pts',(-1.58031634800006,12.2,-4.18544794600002));
#324283=CARTESIAN_POINT('Ctrl Pts',(-1.58031634800006,5.2,-4.18544794600002));
#324284=CARTESIAN_POINT('Ctrl Pts',(-1.58031634800006,2.2,-4.18544794600002));
#324285=CARTESIAN_POINT('Ctrl Pts',(-1.58008176400006,12.2,-4.18763049100002));
#324286=CARTESIAN_POINT('Ctrl Pts',(-1.58008176400006,5.2,-4.18763049100002));
#324287=CARTESIAN_POINT('Ctrl Pts',(-1.58008176400006,2.2,-4.18763049100002));
#324288=CARTESIAN_POINT('Ctrl Pts',(-1.57984439200006,12.2,-4.18981660600001));
#324289=CARTESIAN_POINT('Ctrl Pts',(-1.57984439200006,5.2,-4.18981660600001));
#324290=CARTESIAN_POINT('Ctrl Pts',(-1.57984439200006,2.2,-4.18981660600001));
#324291=CARTESIAN_POINT('Ctrl Pts',(-1.57960422500006,12.2,-4.19200628400001));
#324292=CARTESIAN_POINT('Ctrl Pts',(-1.57960422500006,5.2,-4.19200628400001));
#324293=CARTESIAN_POINT('Ctrl Pts',(-1.57960422500006,2.2,-4.19200628400001));
#324294=CARTESIAN_POINT('Ctrl Pts',(-1.57936125600005,12.2,-4.19419951600001));
#324295=CARTESIAN_POINT('Ctrl Pts',(-1.57936125600005,5.2,-4.19419951600001));
#324296=CARTESIAN_POINT('Ctrl Pts',(-1.57936125600005,2.2,-4.19419951600001));
#324297=CARTESIAN_POINT('Ctrl Pts',(-1.57911547900006,12.2,-4.19639629700002));
#324298=CARTESIAN_POINT('Ctrl Pts',(-1.57911547900006,5.2,-4.19639629700002));
#324299=CARTESIAN_POINT('Ctrl Pts',(-1.57911547900006,2.2,-4.19639629700002));
#324300=CARTESIAN_POINT('Ctrl Pts',(-1.57886688700006,12.2,-4.19859661600002));
#324301=CARTESIAN_POINT('Ctrl Pts',(-1.57886688700006,5.2,-4.19859661600002));
#324302=CARTESIAN_POINT('Ctrl Pts',(-1.57886688700006,2.2,-4.19859661600002));
#324303=CARTESIAN_POINT('Ctrl Pts',(-1.57861547400006,12.2,-4.20080046700001));
#324304=CARTESIAN_POINT('Ctrl Pts',(-1.57861547400006,5.2,-4.20080046700001));
#324305=CARTESIAN_POINT('Ctrl Pts',(-1.57861547400006,2.2,-4.20080046700001));
#324306=CARTESIAN_POINT('Ctrl Pts',(-1.57836123400006,12.2,-4.20300784300002));
#324307=CARTESIAN_POINT('Ctrl Pts',(-1.57836123400006,5.2,-4.20300784300002));
#324308=CARTESIAN_POINT('Ctrl Pts',(-1.57836123400006,2.2,-4.20300784300002));
#324309=CARTESIAN_POINT('Ctrl Pts',(-1.57810415800005,12.2,-4.20521873600002));
#324310=CARTESIAN_POINT('Ctrl Pts',(-1.57810415800005,5.2,-4.20521873600002));
#324311=CARTESIAN_POINT('Ctrl Pts',(-1.57810415800005,2.2,-4.20521873600002));
#324312=CARTESIAN_POINT('Ctrl Pts',(-1.57784424200006,12.2,-4.20743313800001));
#324313=CARTESIAN_POINT('Ctrl Pts',(-1.57784424200006,5.2,-4.20743313800001));
#324314=CARTESIAN_POINT('Ctrl Pts',(-1.57784424200006,2.2,-4.20743313800001));
#324315=CARTESIAN_POINT('Ctrl Pts',(-1.57758148000006,12.2,-4.20965104200001));
#324316=CARTESIAN_POINT('Ctrl Pts',(-1.57758148000006,5.2,-4.20965104200001));
#324317=CARTESIAN_POINT('Ctrl Pts',(-1.57758148000006,2.2,-4.20965104200001));
#324318=CARTESIAN_POINT('Ctrl Pts',(-1.57731586300006,12.2,-4.21187243900001));
#324319=CARTESIAN_POINT('Ctrl Pts',(-1.57731586300006,5.2,-4.21187243900001));
#324320=CARTESIAN_POINT('Ctrl Pts',(-1.57731586300006,2.2,-4.21187243900001));
#324321=CARTESIAN_POINT('Ctrl Pts',(-1.57704738600006,12.2,-4.21409732500001));
#324322=CARTESIAN_POINT('Ctrl Pts',(-1.57704738600006,5.2,-4.21409732500001));
#324323=CARTESIAN_POINT('Ctrl Pts',(-1.57704738600006,2.2,-4.21409732500001));
#324324=CARTESIAN_POINT('Ctrl Pts',(-1.57677604200006,12.2,-4.21632568700002));
#324325=CARTESIAN_POINT('Ctrl Pts',(-1.57677604200006,5.2,-4.21632568700002));
#324326=CARTESIAN_POINT('Ctrl Pts',(-1.57677604200006,2.2,-4.21632568700002));
#324327=CARTESIAN_POINT('Ctrl Pts',(-1.57650182500006,12.2,-4.21855752300001));
#324328=CARTESIAN_POINT('Ctrl Pts',(-1.57650182500006,5.2,-4.21855752300001));
#324329=CARTESIAN_POINT('Ctrl Pts',(-1.57650182500006,2.2,-4.21855752300001));
#324330=CARTESIAN_POINT('Ctrl Pts',(-1.57622472900006,12.2,-4.22079282100002));
#324331=CARTESIAN_POINT('Ctrl Pts',(-1.57622472900006,5.2,-4.22079282100002));
#324332=CARTESIAN_POINT('Ctrl Pts',(-1.57622472900006,2.2,-4.22079282100002));
#324333=CARTESIAN_POINT('Ctrl Pts',(-1.57594474700006,12.2,-4.22303157600001));
#324334=CARTESIAN_POINT('Ctrl Pts',(-1.57594474700006,5.2,-4.22303157600001));
#324335=CARTESIAN_POINT('Ctrl Pts',(-1.57594474700006,2.2,-4.22303157600001));
#324336=CARTESIAN_POINT('Ctrl Pts',(-1.57566187300006,12.2,-4.22527378000002));
#324337=CARTESIAN_POINT('Ctrl Pts',(-1.57566187300006,5.2,-4.22527378000002));
#324338=CARTESIAN_POINT('Ctrl Pts',(-1.57566187300006,2.2,-4.22527378000002));
#324339=CARTESIAN_POINT('Ctrl Pts',(-1.57537610000006,12.2,-4.22751942500001));
#324340=CARTESIAN_POINT('Ctrl Pts',(-1.57537610000006,5.2,-4.22751942500001));
#324341=CARTESIAN_POINT('Ctrl Pts',(-1.57537610000006,2.2,-4.22751942500001));
#324342=CARTESIAN_POINT('Ctrl Pts',(-1.57508742400006,12.2,-4.22976850400001));
#324343=CARTESIAN_POINT('Ctrl Pts',(-1.57508742400006,5.2,-4.22976850400001));
#324344=CARTESIAN_POINT('Ctrl Pts',(-1.57508742400006,2.2,-4.22976850400001));
#324345=CARTESIAN_POINT('Ctrl Pts',(-1.57479583600006,12.2,-4.23202100900001));
#324346=CARTESIAN_POINT('Ctrl Pts',(-1.57479583600006,5.2,-4.23202100900001));
#324347=CARTESIAN_POINT('Ctrl Pts',(-1.57479583600006,2.2,-4.23202100900001));
#324348=CARTESIAN_POINT('Ctrl Pts',(-1.57450132900005,12.2,-4.23427693300002));
#324349=CARTESIAN_POINT('Ctrl Pts',(-1.57450132900005,5.2,-4.23427693300002));
#324350=CARTESIAN_POINT('Ctrl Pts',(-1.57450132900005,2.2,-4.23427693300002));
#324351=CARTESIAN_POINT('Ctrl Pts',(-1.57420390100006,12.2,-4.23653626600001));
#324352=CARTESIAN_POINT('Ctrl Pts',(-1.57420390100006,5.2,-4.23653626600001));
#324353=CARTESIAN_POINT('Ctrl Pts',(-1.57420390100006,2.2,-4.23653626600001));
#324354=CARTESIAN_POINT('Ctrl Pts',(-1.57390354300006,12.2,-4.23879900400001));
#324355=CARTESIAN_POINT('Ctrl Pts',(-1.57390354300006,5.2,-4.23879900400001));
#324356=CARTESIAN_POINT('Ctrl Pts',(-1.57390354300006,2.2,-4.23879900400001));
#324357=CARTESIAN_POINT('Ctrl Pts',(-1.57360024800006,12.2,-4.24106513700002));
#324358=CARTESIAN_POINT('Ctrl Pts',(-1.57360024800006,5.2,-4.24106513700002));
#324359=CARTESIAN_POINT('Ctrl Pts',(-1.57360024800006,2.2,-4.24106513700002));
#324360=CARTESIAN_POINT('Ctrl Pts',(-1.57329401100006,12.2,-4.24333465900002));
#324361=CARTESIAN_POINT('Ctrl Pts',(-1.57329401100006,5.2,-4.24333465900002));
#324362=CARTESIAN_POINT('Ctrl Pts',(-1.57329401100006,2.2,-4.24333465900002));
#324363=CARTESIAN_POINT('Ctrl Pts',(-1.57298482700006,12.2,-4.24560756200002));
#324364=CARTESIAN_POINT('Ctrl Pts',(-1.57298482700006,5.2,-4.24560756200002));
#324365=CARTESIAN_POINT('Ctrl Pts',(-1.57298482700006,2.2,-4.24560756200002));
#324366=CARTESIAN_POINT('Ctrl Pts',(-1.57267268700006,12.2,-4.24788383800002));
#324367=CARTESIAN_POINT('Ctrl Pts',(-1.57267268700006,5.2,-4.24788383800002));
#324368=CARTESIAN_POINT('Ctrl Pts',(-1.57267268700006,2.2,-4.24788383800002));
#324369=CARTESIAN_POINT('Ctrl Pts',(-1.57235758700006,12.2,-4.25016347900002));
#324370=CARTESIAN_POINT('Ctrl Pts',(-1.57235758700006,5.2,-4.25016347900002));
#324371=CARTESIAN_POINT('Ctrl Pts',(-1.57235758700006,2.2,-4.25016347900002));
#324372=CARTESIAN_POINT('Ctrl Pts',(-1.57203952100006,12.2,-4.25244647900001));
#324373=CARTESIAN_POINT('Ctrl Pts',(-1.57203952100006,5.2,-4.25244647900001));
#324374=CARTESIAN_POINT('Ctrl Pts',(-1.57203952100006,2.2,-4.25244647900001));
#324375=CARTESIAN_POINT('Ctrl Pts',(-1.57171848200006,12.2,-4.25473282900001));
#324376=CARTESIAN_POINT('Ctrl Pts',(-1.57171848200006,5.2,-4.25473282900001));
#324377=CARTESIAN_POINT('Ctrl Pts',(-1.57171848200006,2.2,-4.25473282900001));
#324378=CARTESIAN_POINT('Ctrl Pts',(-1.57139446300006,12.2,-4.25702252300002));
#324379=CARTESIAN_POINT('Ctrl Pts',(-1.57139446300006,5.2,-4.25702252300002));
#324380=CARTESIAN_POINT('Ctrl Pts',(-1.57139446300006,2.2,-4.25702252300002));
#324381=CARTESIAN_POINT('Ctrl Pts',(-1.57106746100005,12.2,-4.25931555100002));
#324382=CARTESIAN_POINT('Ctrl Pts',(-1.57106746100005,5.2,-4.25931555100002));
#324383=CARTESIAN_POINT('Ctrl Pts',(-1.57106746100005,2.2,-4.25931555100002));
#324384=CARTESIAN_POINT('Ctrl Pts',(-1.57073746600006,12.2,-4.26161190800002));
#324385=CARTESIAN_POINT('Ctrl Pts',(-1.57073746600006,5.2,-4.26161190800002));
#324386=CARTESIAN_POINT('Ctrl Pts',(-1.57073746600006,2.2,-4.26161190800002));
#324387=CARTESIAN_POINT('Ctrl Pts',(-1.57040447600005,12.2,-4.26391158500001));
#324388=CARTESIAN_POINT('Ctrl Pts',(-1.57040447600005,5.2,-4.26391158500001));
#324389=CARTESIAN_POINT('Ctrl Pts',(-1.57040447600005,2.2,-4.26391158500001));
#324390=CARTESIAN_POINT('Ctrl Pts',(-1.57006848200006,12.2,-4.26621457600001));
#324391=CARTESIAN_POINT('Ctrl Pts',(-1.57006848200006,5.2,-4.26621457600001));
#324392=CARTESIAN_POINT('Ctrl Pts',(-1.57006848200006,2.2,-4.26621457600001));
#324393=CARTESIAN_POINT('Ctrl Pts',(-1.56972947900006,12.2,-4.26852087100002));
#324394=CARTESIAN_POINT('Ctrl Pts',(-1.56972947900006,5.2,-4.26852087100002));
#324395=CARTESIAN_POINT('Ctrl Pts',(-1.56972947900006,2.2,-4.26852087100002));
#324396=CARTESIAN_POINT('Ctrl Pts',(-1.56938746200006,12.2,-4.27083046500002));
#324397=CARTESIAN_POINT('Ctrl Pts',(-1.56938746200006,5.2,-4.27083046500002));
#324398=CARTESIAN_POINT('Ctrl Pts',(-1.56938746200006,2.2,-4.27083046500002));
#324399=CARTESIAN_POINT('Ctrl Pts',(-1.56904242300006,12.2,-4.27314334800001));
#324400=CARTESIAN_POINT('Ctrl Pts',(-1.56904242300006,5.2,-4.27314334800001));
#324401=CARTESIAN_POINT('Ctrl Pts',(-1.56904242300006,2.2,-4.27314334800001));
#324402=CARTESIAN_POINT('Ctrl Pts',(-1.56869435800005,12.2,-4.27545951600001));
#324403=CARTESIAN_POINT('Ctrl Pts',(-1.56869435800005,5.2,-4.27545951600001));
#324404=CARTESIAN_POINT('Ctrl Pts',(-1.56869435800005,2.2,-4.27545951600001));
#324405=CARTESIAN_POINT('Ctrl Pts',(-1.56834326000005,12.2,-4.27777895800002));
#324406=CARTESIAN_POINT('Ctrl Pts',(-1.56834326000005,5.2,-4.27777895800002));
#324407=CARTESIAN_POINT('Ctrl Pts',(-1.56834326000005,2.2,-4.27777895800002));
#324408=CARTESIAN_POINT('Ctrl Pts',(-1.56798912400005,12.2,-4.28010166800001));
#324409=CARTESIAN_POINT('Ctrl Pts',(-1.56798912400005,5.2,-4.28010166800001));
#324410=CARTESIAN_POINT('Ctrl Pts',(-1.56798912400005,2.2,-4.28010166800001));
#324411=CARTESIAN_POINT('Ctrl Pts',(-1.56763194300006,12.2,-4.28242763800001));
#324412=CARTESIAN_POINT('Ctrl Pts',(-1.56763194300006,5.2,-4.28242763800001));
#324413=CARTESIAN_POINT('Ctrl Pts',(-1.56763194300006,2.2,-4.28242763800001));
#324414=CARTESIAN_POINT('Ctrl Pts',(-1.56727171100006,12.2,-4.28475686200001));
#324415=CARTESIAN_POINT('Ctrl Pts',(-1.56727171100006,5.2,-4.28475686200001));
#324416=CARTESIAN_POINT('Ctrl Pts',(-1.56727171100006,2.2,-4.28475686200001));
#324417=CARTESIAN_POINT('Ctrl Pts',(-1.56690842400006,12.2,-4.28708933000001));
#324418=CARTESIAN_POINT('Ctrl Pts',(-1.56690842400006,5.2,-4.28708933000001));
#324419=CARTESIAN_POINT('Ctrl Pts',(-1.56690842400006,2.2,-4.28708933000001));
#324420=CARTESIAN_POINT('Ctrl Pts',(-1.56654207500006,12.2,-4.28942503600001));
#324421=CARTESIAN_POINT('Ctrl Pts',(-1.56654207500006,5.2,-4.28942503600001));
#324422=CARTESIAN_POINT('Ctrl Pts',(-1.56654207500006,2.2,-4.28942503600001));
#324423=CARTESIAN_POINT('Ctrl Pts',(-1.56617265800006,12.2,-4.29176397300001));
#324424=CARTESIAN_POINT('Ctrl Pts',(-1.56617265800006,5.2,-4.29176397300001));
#324425=CARTESIAN_POINT('Ctrl Pts',(-1.56617265800006,2.2,-4.29176397300001));
#324426=CARTESIAN_POINT('Ctrl Pts',(-1.56580016900006,12.2,-4.29410613300002));
#324427=CARTESIAN_POINT('Ctrl Pts',(-1.56580016900006,5.2,-4.29410613300002));
#324428=CARTESIAN_POINT('Ctrl Pts',(-1.56580016900006,2.2,-4.29410613300002));
#324429=CARTESIAN_POINT('Ctrl Pts',(-1.56542459900006,12.2,-4.29645150700001));
#324430=CARTESIAN_POINT('Ctrl Pts',(-1.56542459900006,5.2,-4.29645150700001));
#324431=CARTESIAN_POINT('Ctrl Pts',(-1.56542459900006,2.2,-4.29645150700001));
#324432=CARTESIAN_POINT('Ctrl Pts',(-1.56504594300006,12.2,-4.29880009000001));
#324433=CARTESIAN_POINT('Ctrl Pts',(-1.56504594300006,5.2,-4.29880009000001));
#324434=CARTESIAN_POINT('Ctrl Pts',(-1.56504594300006,2.2,-4.29880009000001));
#324435=CARTESIAN_POINT('Ctrl Pts',(-1.56466419900006,12.2,-4.30115187200002));
#324436=CARTESIAN_POINT('Ctrl Pts',(-1.56466419900006,5.2,-4.30115187200002));
#324437=CARTESIAN_POINT('Ctrl Pts',(-1.56466419900006,2.2,-4.30115187200002));
#324438=CARTESIAN_POINT('Ctrl Pts',(-1.56427935700005,12.2,-4.30350684800001));
#324439=CARTESIAN_POINT('Ctrl Pts',(-1.56427935700005,5.2,-4.30350684800001));
#324440=CARTESIAN_POINT('Ctrl Pts',(-1.56427935700005,2.2,-4.30350684800001));
#324441=CARTESIAN_POINT('Ctrl Pts',(-1.56389141300005,12.2,-4.30586500900001));
#324442=CARTESIAN_POINT('Ctrl Pts',(-1.56389141300005,5.2,-4.30586500900001));
#324443=CARTESIAN_POINT('Ctrl Pts',(-1.56389141300005,2.2,-4.30586500900001));
#324444=CARTESIAN_POINT('Ctrl Pts',(-1.56350036100006,12.2,-4.30822634700001));
#324445=CARTESIAN_POINT('Ctrl Pts',(-1.56350036100006,5.2,-4.30822634700001));
#324446=CARTESIAN_POINT('Ctrl Pts',(-1.56350036100006,2.2,-4.30822634700001));
#324447=CARTESIAN_POINT('Ctrl Pts',(-1.56310619600006,12.2,-4.31059085600001));
#324448=CARTESIAN_POINT('Ctrl Pts',(-1.56310619600006,5.2,-4.31059085600001));
#324449=CARTESIAN_POINT('Ctrl Pts',(-1.56310619600006,2.2,-4.31059085600001));
#324450=CARTESIAN_POINT('Ctrl Pts',(-1.56270891100006,12.2,-4.31295852800002));
#324451=CARTESIAN_POINT('Ctrl Pts',(-1.56270891100006,5.2,-4.31295852800002));
#324452=CARTESIAN_POINT('Ctrl Pts',(-1.56270891100006,2.2,-4.31295852800002));
#324453=CARTESIAN_POINT('Ctrl Pts',(-1.56230850300005,12.2,-4.31532935500002));
#324454=CARTESIAN_POINT('Ctrl Pts',(-1.56230850300005,5.2,-4.31532935500002));
#324455=CARTESIAN_POINT('Ctrl Pts',(-1.56230850300005,2.2,-4.31532935500002));
#324456=CARTESIAN_POINT('Ctrl Pts',(-1.56190496300006,12.2,-4.31770333100001));
#324457=CARTESIAN_POINT('Ctrl Pts',(-1.56190496300006,5.2,-4.31770333100001));
#324458=CARTESIAN_POINT('Ctrl Pts',(-1.56190496300006,2.2,-4.31770333100001));
#324459=CARTESIAN_POINT('Ctrl Pts',(-1.56149828800005,12.2,-4.32008044700002));
#324460=CARTESIAN_POINT('Ctrl Pts',(-1.56149828800005,5.2,-4.32008044700002));
#324461=CARTESIAN_POINT('Ctrl Pts',(-1.56149828800005,2.2,-4.32008044700002));
#324462=CARTESIAN_POINT('Ctrl Pts',(-1.56108847100006,12.2,-4.32246069400001));
#324463=CARTESIAN_POINT('Ctrl Pts',(-1.56108847100006,5.2,-4.32246069400001));
#324464=CARTESIAN_POINT('Ctrl Pts',(-1.56108847100006,2.2,-4.32246069400001));
#324465=CARTESIAN_POINT('Ctrl Pts',(-1.56067550700006,12.2,-4.32484406800001));
#324466=CARTESIAN_POINT('Ctrl Pts',(-1.56067550700006,5.2,-4.32484406800001));
#324467=CARTESIAN_POINT('Ctrl Pts',(-1.56067550700006,2.2,-4.32484406800001));
#324468=CARTESIAN_POINT('Ctrl Pts',(-1.56025939000005,12.2,-4.32723056000002));
#324469=CARTESIAN_POINT('Ctrl Pts',(-1.56025939000005,5.2,-4.32723056000002));
#324470=CARTESIAN_POINT('Ctrl Pts',(-1.56025939000005,2.2,-4.32723056000002));
#324471=CARTESIAN_POINT('Ctrl Pts',(-1.55984011600005,12.2,-4.32962016300001));
#324472=CARTESIAN_POINT('Ctrl Pts',(-1.55984011600005,5.2,-4.32962016300001));
#324473=CARTESIAN_POINT('Ctrl Pts',(-1.55984011600005,2.2,-4.32962016300001));
#324474=CARTESIAN_POINT('Ctrl Pts',(-1.55941767800006,12.2,-4.33201286900001));
#324475=CARTESIAN_POINT('Ctrl Pts',(-1.55941767800006,5.2,-4.33201286900001));
#324476=CARTESIAN_POINT('Ctrl Pts',(-1.55941767800006,2.2,-4.33201286900001));
#324477=CARTESIAN_POINT('Ctrl Pts',(-1.55899207100005,12.2,-4.33440866900002));
#324478=CARTESIAN_POINT('Ctrl Pts',(-1.55899207100005,5.2,-4.33440866900002));
#324479=CARTESIAN_POINT('Ctrl Pts',(-1.55899207100005,2.2,-4.33440866900002));
#324480=CARTESIAN_POINT('Ctrl Pts',(-1.55856328800006,12.2,-4.33680755900001));
#324481=CARTESIAN_POINT('Ctrl Pts',(-1.55856328800006,5.2,-4.33680755900001));
#324482=CARTESIAN_POINT('Ctrl Pts',(-1.55856328800006,2.2,-4.33680755900001));
#324483=CARTESIAN_POINT('Ctrl Pts',(-1.55813132700006,12.2,-4.33920952900001));
#324484=CARTESIAN_POINT('Ctrl Pts',(-1.55813132700006,5.2,-4.33920952900001));
#324485=CARTESIAN_POINT('Ctrl Pts',(-1.55813132700006,2.2,-4.33920952900001));
#324486=CARTESIAN_POINT('Ctrl Pts',(-1.55769618000006,12.2,-4.34161457200001));
#324487=CARTESIAN_POINT('Ctrl Pts',(-1.55769618000006,5.2,-4.34161457200001));
#324488=CARTESIAN_POINT('Ctrl Pts',(-1.55769618000006,2.2,-4.34161457200001));
#324489=CARTESIAN_POINT('Ctrl Pts',(-1.55725784300006,12.2,-4.34402268000001));
#324490=CARTESIAN_POINT('Ctrl Pts',(-1.55725784300006,5.2,-4.34402268000001));
#324491=CARTESIAN_POINT('Ctrl Pts',(-1.55725784300006,2.2,-4.34402268000001));
#324492=CARTESIAN_POINT('Ctrl Pts',(-1.55681630800005,12.2,-4.34643384800002));
#324493=CARTESIAN_POINT('Ctrl Pts',(-1.55681630800005,5.2,-4.34643384800002));
#324494=CARTESIAN_POINT('Ctrl Pts',(-1.55681630800005,2.2,-4.34643384800002));
#324495=CARTESIAN_POINT('Ctrl Pts',(-1.55637157300006,12.2,-4.34884806500001));
#324496=CARTESIAN_POINT('Ctrl Pts',(-1.55637157300006,5.2,-4.34884806500001));
#324497=CARTESIAN_POINT('Ctrl Pts',(-1.55637157300006,2.2,-4.34884806500001));
#324498=CARTESIAN_POINT('Ctrl Pts',(-1.55592363000005,12.2,-4.35126532700002));
#324499=CARTESIAN_POINT('Ctrl Pts',(-1.55592363000005,5.2,-4.35126532700002));
#324500=CARTESIAN_POINT('Ctrl Pts',(-1.55592363000005,2.2,-4.35126532700002));
#324501=CARTESIAN_POINT('Ctrl Pts',(-1.55547247600006,12.2,-4.35368562300001));
#324502=CARTESIAN_POINT('Ctrl Pts',(-1.55547247600006,5.2,-4.35368562300001));
#324503=CARTESIAN_POINT('Ctrl Pts',(-1.55547247600006,2.2,-4.35368562300001));
#324504=CARTESIAN_POINT('Ctrl Pts',(-1.55501810200006,12.2,-4.35610894900002));
#324505=CARTESIAN_POINT('Ctrl Pts',(-1.55501810200006,5.2,-4.35610894900002));
#324506=CARTESIAN_POINT('Ctrl Pts',(-1.55501810200006,2.2,-4.35610894900002));
#324507=CARTESIAN_POINT('Ctrl Pts',(-1.55456050700006,12.2,-4.35853529600001));
#324508=CARTESIAN_POINT('Ctrl Pts',(-1.55456050700006,5.2,-4.35853529600001));
#324509=CARTESIAN_POINT('Ctrl Pts',(-1.55456050700006,2.2,-4.35853529600001));
#324510=CARTESIAN_POINT('Ctrl Pts',(-1.55409968300006,12.2,-4.36096465600002));
#324511=CARTESIAN_POINT('Ctrl Pts',(-1.55409968300006,5.2,-4.36096465600002));
#324512=CARTESIAN_POINT('Ctrl Pts',(-1.55409968300006,2.2,-4.36096465600002));
#324513=CARTESIAN_POINT('Ctrl Pts',(-1.55363562600006,12.2,-4.36339702300002));
#324514=CARTESIAN_POINT('Ctrl Pts',(-1.55363562600006,5.2,-4.36339702300002));
#324515=CARTESIAN_POINT('Ctrl Pts',(-1.55363562600006,2.2,-4.36339702300002));
#324516=CARTESIAN_POINT('Ctrl Pts',(-1.55316833000006,12.2,-4.36583238800001));
#324517=CARTESIAN_POINT('Ctrl Pts',(-1.55316833000006,5.2,-4.36583238800001));
#324518=CARTESIAN_POINT('Ctrl Pts',(-1.55316833000006,2.2,-4.36583238800001));
#324519=CARTESIAN_POINT('Ctrl Pts',(-1.55269779000006,12.2,-4.36827074500002));
#324520=CARTESIAN_POINT('Ctrl Pts',(-1.55269779000006,5.2,-4.36827074500002));
#324521=CARTESIAN_POINT('Ctrl Pts',(-1.55269779000006,2.2,-4.36827074500002));
#324522=CARTESIAN_POINT('Ctrl Pts',(-1.55222400100006,12.2,-4.37071208400001));
#324523=CARTESIAN_POINT('Ctrl Pts',(-1.55222400100006,5.2,-4.37071208400001));
#324524=CARTESIAN_POINT('Ctrl Pts',(-1.55222400100006,2.2,-4.37071208400001));
#324525=CARTESIAN_POINT('Ctrl Pts',(-1.55174695700006,12.2,-4.37315640100001));
#324526=CARTESIAN_POINT('Ctrl Pts',(-1.55174695700006,5.2,-4.37315640100001));
#324527=CARTESIAN_POINT('Ctrl Pts',(-1.55174695700006,2.2,-4.37315640100001));
#324528=CARTESIAN_POINT('Ctrl Pts',(-1.55126665400006,12.2,-4.37560368700002));
#324529=CARTESIAN_POINT('Ctrl Pts',(-1.55126665400006,5.2,-4.37560368700002));
#324530=CARTESIAN_POINT('Ctrl Pts',(-1.55126665400006,2.2,-4.37560368700002));
#324531=CARTESIAN_POINT('Ctrl Pts',(-1.55078308600005,12.2,-4.37805393400001));
#324532=CARTESIAN_POINT('Ctrl Pts',(-1.55078308600005,5.2,-4.37805393400001));
#324533=CARTESIAN_POINT('Ctrl Pts',(-1.55078308600005,2.2,-4.37805393400001));
#324534=CARTESIAN_POINT('Ctrl Pts',(-1.55029624800005,12.2,-4.38050713600001));
#324535=CARTESIAN_POINT('Ctrl Pts',(-1.55029624800005,5.2,-4.38050713600001));
#324536=CARTESIAN_POINT('Ctrl Pts',(-1.55029624800005,2.2,-4.38050713600001));
#324537=CARTESIAN_POINT('Ctrl Pts',(-1.54980613500005,12.2,-4.38296328300002));
#324538=CARTESIAN_POINT('Ctrl Pts',(-1.54980613500005,5.2,-4.38296328300002));
#324539=CARTESIAN_POINT('Ctrl Pts',(-1.54980613500005,2.2,-4.38296328300002));
#324540=CARTESIAN_POINT('Ctrl Pts',(-1.54931274100006,12.2,-4.38542237000001));
#324541=CARTESIAN_POINT('Ctrl Pts',(-1.54931274100006,5.2,-4.38542237000001));
#324542=CARTESIAN_POINT('Ctrl Pts',(-1.54931274100006,2.2,-4.38542237000001));
#324543=CARTESIAN_POINT('Ctrl Pts',(-1.54881606300005,12.2,-4.38788438900001));
#324544=CARTESIAN_POINT('Ctrl Pts',(-1.54881606300005,5.2,-4.38788438900001));
#324545=CARTESIAN_POINT('Ctrl Pts',(-1.54881606300005,2.2,-4.38788438900001));
#324546=CARTESIAN_POINT('Ctrl Pts',(-1.54831609400006,12.2,-4.39034933300002));
#324547=CARTESIAN_POINT('Ctrl Pts',(-1.54831609400006,5.2,-4.39034933300002));
#324548=CARTESIAN_POINT('Ctrl Pts',(-1.54831609400006,2.2,-4.39034933300002));
#324549=CARTESIAN_POINT('Ctrl Pts',(-1.54781282900006,12.2,-4.39281719400002));
#324550=CARTESIAN_POINT('Ctrl Pts',(-1.54781282900006,5.2,-4.39281719400002));
#324551=CARTESIAN_POINT('Ctrl Pts',(-1.54781282900006,2.2,-4.39281719400002));
#324552=CARTESIAN_POINT('Ctrl Pts',(-1.54730626400006,12.2,-4.39528796400001));
#324553=CARTESIAN_POINT('Ctrl Pts',(-1.54730626400006,5.2,-4.39528796400001));
#324554=CARTESIAN_POINT('Ctrl Pts',(-1.54730626400006,2.2,-4.39528796400001));
#324555=CARTESIAN_POINT('Ctrl Pts',(-1.54679639400006,12.2,-4.39776163600001));
#324556=CARTESIAN_POINT('Ctrl Pts',(-1.54679639400006,5.2,-4.39776163600001));
#324557=CARTESIAN_POINT('Ctrl Pts',(-1.54679639400006,2.2,-4.39776163600001));
#324558=CARTESIAN_POINT('Ctrl Pts',(-1.54628321200006,12.2,-4.40023820300001));
#324559=CARTESIAN_POINT('Ctrl Pts',(-1.54628321200006,5.2,-4.40023820300001));
#324560=CARTESIAN_POINT('Ctrl Pts',(-1.54628321200006,2.2,-4.40023820300001));
#324561=CARTESIAN_POINT('Ctrl Pts',(-1.54576671500006,12.2,-4.40271765800002));
#324562=CARTESIAN_POINT('Ctrl Pts',(-1.54576671500006,5.2,-4.40271765800002));
#324563=CARTESIAN_POINT('Ctrl Pts',(-1.54576671500006,2.2,-4.40271765800002));
#324564=CARTESIAN_POINT('Ctrl Pts',(-1.54524689700006,12.2,-4.40519999300002));
#324565=CARTESIAN_POINT('Ctrl Pts',(-1.54524689700006,5.2,-4.40519999300002));
#324566=CARTESIAN_POINT('Ctrl Pts',(-1.54524689700006,2.2,-4.40519999300002));
#324567=CARTESIAN_POINT('Ctrl Pts',(-1.54472375300006,12.2,-4.40768520000002));
#324568=CARTESIAN_POINT('Ctrl Pts',(-1.54472375300006,5.2,-4.40768520000002));
#324569=CARTESIAN_POINT('Ctrl Pts',(-1.54472375300006,2.2,-4.40768520000002));
#324570=CARTESIAN_POINT('Ctrl Pts',(-1.54419727900006,12.2,-4.41017327200001));
#324571=CARTESIAN_POINT('Ctrl Pts',(-1.54419727900006,5.2,-4.41017327200001));
#324572=CARTESIAN_POINT('Ctrl Pts',(-1.54419727900006,2.2,-4.41017327200001));
#324573=CARTESIAN_POINT('Ctrl Pts',(-1.54366747000006,12.2,-4.41266420300002));
#324574=CARTESIAN_POINT('Ctrl Pts',(-1.54366747000006,5.2,-4.41266420300002));
#324575=CARTESIAN_POINT('Ctrl Pts',(-1.54366747000006,2.2,-4.41266420300002));
#324576=CARTESIAN_POINT('Ctrl Pts',(-1.54313432000006,12.2,-4.41515798400001));
#324577=CARTESIAN_POINT('Ctrl Pts',(-1.54313432000006,5.2,-4.41515798400001));
#324578=CARTESIAN_POINT('Ctrl Pts',(-1.54313432000006,2.2,-4.41515798400001));
#324579=CARTESIAN_POINT('Ctrl Pts',(-1.54259782500006,12.2,-4.41765460700001));
#324580=CARTESIAN_POINT('Ctrl Pts',(-1.54259782500006,5.2,-4.41765460700001));
#324581=CARTESIAN_POINT('Ctrl Pts',(-1.54259782500006,2.2,-4.41765460700001));
#324582=CARTESIAN_POINT('Ctrl Pts',(-1.54205797900006,12.2,-4.42015406700001));
#324583=CARTESIAN_POINT('Ctrl Pts',(-1.54205797900006,5.2,-4.42015406700001));
#324584=CARTESIAN_POINT('Ctrl Pts',(-1.54205797900006,2.2,-4.42015406700001));
#324585=CARTESIAN_POINT('Ctrl Pts',(-1.54151477800006,12.2,-4.42265635500001));
#324586=CARTESIAN_POINT('Ctrl Pts',(-1.54151477800006,5.2,-4.42265635500001));
#324587=CARTESIAN_POINT('Ctrl Pts',(-1.54151477800006,2.2,-4.42265635500001));
#324588=CARTESIAN_POINT('Ctrl Pts',(-1.54096821700006,12.2,-4.42516146300001));
#324589=CARTESIAN_POINT('Ctrl Pts',(-1.54096821700006,5.2,-4.42516146300001));
#324590=CARTESIAN_POINT('Ctrl Pts',(-1.54096821700006,2.2,-4.42516146300001));
#324591=CARTESIAN_POINT('Ctrl Pts',(-1.54041829100006,12.2,-4.42766938500001));
#324592=CARTESIAN_POINT('Ctrl Pts',(-1.54041829100006,5.2,-4.42766938500001));
#324593=CARTESIAN_POINT('Ctrl Pts',(-1.54041829100006,2.2,-4.42766938500001));
#324594=CARTESIAN_POINT('Ctrl Pts',(-1.53986499500005,12.2,-4.43018011200001));
#324595=CARTESIAN_POINT('Ctrl Pts',(-1.53986499500005,5.2,-4.43018011200001));
#324596=CARTESIAN_POINT('Ctrl Pts',(-1.53986499500005,2.2,-4.43018011200001));
#324597=CARTESIAN_POINT('Ctrl Pts',(-1.53930832500006,12.2,-4.43269363900002));
#324598=CARTESIAN_POINT('Ctrl Pts',(-1.53930832500006,5.2,-4.43269363900002));
#324599=CARTESIAN_POINT('Ctrl Pts',(-1.53930832500006,2.2,-4.43269363900002));
#324600=CARTESIAN_POINT('Ctrl Pts',(-1.53874827600006,12.2,-4.43520995700001));
#324601=CARTESIAN_POINT('Ctrl Pts',(-1.53874827600006,5.2,-4.43520995700001));
#324602=CARTESIAN_POINT('Ctrl Pts',(-1.53874827600006,2.2,-4.43520995700001));
#324603=CARTESIAN_POINT('Ctrl Pts',(-1.53818484200006,12.2,-4.43772905900001));
#324604=CARTESIAN_POINT('Ctrl Pts',(-1.53818484200006,5.2,-4.43772905900001));
#324605=CARTESIAN_POINT('Ctrl Pts',(-1.53818484200006,2.2,-4.43772905900001));
#324606=CARTESIAN_POINT('Ctrl Pts',(-1.53761802000006,12.2,-4.44025093800001));
#324607=CARTESIAN_POINT('Ctrl Pts',(-1.53761802000006,5.2,-4.44025093800001));
#324608=CARTESIAN_POINT('Ctrl Pts',(-1.53761802000006,2.2,-4.44025093800001));
#324609=CARTESIAN_POINT('Ctrl Pts',(-1.53704780500005,12.2,-4.44277558600001));
#324610=CARTESIAN_POINT('Ctrl Pts',(-1.53704780500005,5.2,-4.44277558600001));
#324611=CARTESIAN_POINT('Ctrl Pts',(-1.53704780500005,2.2,-4.44277558600001));
#324612=CARTESIAN_POINT('Ctrl Pts',(-1.53647419100006,12.2,-4.44530299700002));
#324613=CARTESIAN_POINT('Ctrl Pts',(-1.53647419100006,5.2,-4.44530299700002));
#324614=CARTESIAN_POINT('Ctrl Pts',(-1.53647419100006,2.2,-4.44530299700002));
#324615=CARTESIAN_POINT('Ctrl Pts',(-1.53589717400005,12.2,-4.44783316200001));
#324616=CARTESIAN_POINT('Ctrl Pts',(-1.53589717400005,5.2,-4.44783316200001));
#324617=CARTESIAN_POINT('Ctrl Pts',(-1.53589717400005,2.2,-4.44783316200001));
#324618=CARTESIAN_POINT('Ctrl Pts',(-1.53531674800006,12.2,-4.45036607300001));
#324619=CARTESIAN_POINT('Ctrl Pts',(-1.53531674800006,5.2,-4.45036607300001));
#324620=CARTESIAN_POINT('Ctrl Pts',(-1.53531674800006,2.2,-4.45036607300001));
#324621=CARTESIAN_POINT('Ctrl Pts',(-1.53473291000006,12.2,-4.45290172400002));
#324622=CARTESIAN_POINT('Ctrl Pts',(-1.53473291000006,5.2,-4.45290172400002));
#324623=CARTESIAN_POINT('Ctrl Pts',(-1.53473291000006,2.2,-4.45290172400002));
#324624=CARTESIAN_POINT('Ctrl Pts',(-1.53414565400006,12.2,-4.45544010600001));
#324625=CARTESIAN_POINT('Ctrl Pts',(-1.53414565400006,5.2,-4.45544010600001));
#324626=CARTESIAN_POINT('Ctrl Pts',(-1.53414565400006,2.2,-4.45544010600001));
#324627=CARTESIAN_POINT('Ctrl Pts',(-1.53355497600006,12.2,-4.45798121300002));
#324628=CARTESIAN_POINT('Ctrl Pts',(-1.53355497600006,5.2,-4.45798121300002));
#324629=CARTESIAN_POINT('Ctrl Pts',(-1.53355497600006,2.2,-4.45798121300002));
#324630=CARTESIAN_POINT('Ctrl Pts',(-1.53296087100005,12.2,-4.46052503700002));
#324631=CARTESIAN_POINT('Ctrl Pts',(-1.53296087100005,5.2,-4.46052503700002));
#324632=CARTESIAN_POINT('Ctrl Pts',(-1.53296087100005,2.2,-4.46052503700002));
#324633=CARTESIAN_POINT('Ctrl Pts',(-1.53236333600006,12.2,-4.46307157300001));
#324634=CARTESIAN_POINT('Ctrl Pts',(-1.53236333600006,5.2,-4.46307157300001));
#324635=CARTESIAN_POINT('Ctrl Pts',(-1.53236333600006,2.2,-4.46307157300001));
#324636=CARTESIAN_POINT('Ctrl Pts',(-1.53176236500005,12.2,-4.46562081300002));
#324637=CARTESIAN_POINT('Ctrl Pts',(-1.53176236500005,5.2,-4.46562081300002));
#324638=CARTESIAN_POINT('Ctrl Pts',(-1.53176236500005,2.2,-4.46562081300002));
#324639=CARTESIAN_POINT('Ctrl Pts',(-1.53115795500006,12.2,-4.46817275000001));
#324640=CARTESIAN_POINT('Ctrl Pts',(-1.53115795500006,5.2,-4.46817275000001));
#324641=CARTESIAN_POINT('Ctrl Pts',(-1.53115795500006,2.2,-4.46817275000001));
#324642=CARTESIAN_POINT('Ctrl Pts',(-1.53055010200006,12.2,-4.47072737700001));
#324643=CARTESIAN_POINT('Ctrl Pts',(-1.53055010200006,5.2,-4.47072737700001));
#324644=CARTESIAN_POINT('Ctrl Pts',(-1.53055010200006,2.2,-4.47072737700001));
#324645=CARTESIAN_POINT('Ctrl Pts',(-1.52993880100006,12.2,-4.47328468700002));
#324646=CARTESIAN_POINT('Ctrl Pts',(-1.52993880100006,5.2,-4.47328468700002));
#324647=CARTESIAN_POINT('Ctrl Pts',(-1.52993880100006,2.2,-4.47328468700002));
#324648=CARTESIAN_POINT('Ctrl Pts',(-1.52932404500006,12.2,-4.47584467000001));
#324649=CARTESIAN_POINT('Ctrl Pts',(-1.52932404500006,5.2,-4.47584467000001));
#324650=CARTESIAN_POINT('Ctrl Pts',(-1.52932404500006,2.2,-4.47584467000001));
#324651=CARTESIAN_POINT('Ctrl Pts',(-1.52870582800006,12.2,-4.47840731700001));
#324652=CARTESIAN_POINT('Ctrl Pts',(-1.52870582800006,5.2,-4.47840731700001));
#324653=CARTESIAN_POINT('Ctrl Pts',(-1.52870582800006,2.2,-4.47840731700001));
#324654=CARTESIAN_POINT('Ctrl Pts',(-1.52808414600006,12.2,-4.48097261900001));
#324655=CARTESIAN_POINT('Ctrl Pts',(-1.52808414600006,5.2,-4.48097261900001));
#324656=CARTESIAN_POINT('Ctrl Pts',(-1.52808414600006,2.2,-4.48097261900001));
#324657=CARTESIAN_POINT('Ctrl Pts',(-1.52745899300006,12.2,-4.48354056900001));
#324658=CARTESIAN_POINT('Ctrl Pts',(-1.52745899300006,5.2,-4.48354056900001));
#324659=CARTESIAN_POINT('Ctrl Pts',(-1.52745899300006,2.2,-4.48354056900001));
#324660=CARTESIAN_POINT('Ctrl Pts',(-1.52683036500005,12.2,-4.48611115700002));
#324661=CARTESIAN_POINT('Ctrl Pts',(-1.52683036500005,5.2,-4.48611115700002));
#324662=CARTESIAN_POINT('Ctrl Pts',(-1.52683036500005,2.2,-4.48611115700002));
#324663=CARTESIAN_POINT('Ctrl Pts',(-1.52619825900006,12.2,-4.48868437900002));
#324664=CARTESIAN_POINT('Ctrl Pts',(-1.52619825900006,5.2,-4.48868437900002));
#324665=CARTESIAN_POINT('Ctrl Pts',(-1.52619825900006,2.2,-4.48868437900002));
#324666=CARTESIAN_POINT('Ctrl Pts',(-1.52556267200006,12.2,-4.49126023200002));
#324667=CARTESIAN_POINT('Ctrl Pts',(-1.52556267200006,5.2,-4.49126023200002));
#324668=CARTESIAN_POINT('Ctrl Pts',(-1.52556267200006,2.2,-4.49126023200002));
#324669=CARTESIAN_POINT('Ctrl Pts',(-1.52492360500006,12.2,-4.49383871500002));
#324670=CARTESIAN_POINT('Ctrl Pts',(-1.52492360500006,5.2,-4.49383871500002));
#324671=CARTESIAN_POINT('Ctrl Pts',(-1.52492360500006,2.2,-4.49383871500002));
#324672=CARTESIAN_POINT('Ctrl Pts',(-1.52440956500006,12.2,-4.49590360400002));
#324673=CARTESIAN_POINT('Ctrl Pts',(-1.52440956500006,5.2,-4.49590360400002));
#324674=CARTESIAN_POINT('Ctrl Pts',(-1.52440956500006,2.2,-4.49590360400002));
#324675=CARTESIAN_POINT('Ctrl Pts',(-1.52402246800006,12.2,-4.49745345200002));
#324676=CARTESIAN_POINT('Ctrl Pts',(-1.52402246800006,5.2,-4.49745345200002));
#324677=CARTESIAN_POINT('Ctrl Pts',(-1.52402246800006,2.2,-4.49745345200002));
#324678=CARTESIAN_POINT('Ctrl Pts',(-1.52376370700006,12.2,-4.49848720900001));
#324679=CARTESIAN_POINT('Ctrl Pts',(-1.52376370700006,5.2,-4.49848720900001));
#324680=CARTESIAN_POINT('Ctrl Pts',(-1.52376370700006,2.2,-4.49848720900001));
#324681=CARTESIAN_POINT('Ctrl Pts',(-1.52363415300006,12.2,-4.49900422000002));
#324682=CARTESIAN_POINT('Ctrl Pts',(-1.52363415300006,5.2,-4.49900422000002));
#324683=CARTESIAN_POINT('Ctrl Pts',(-1.52363415300006,2.2,-4.49900422000002));
#324684=CARTESIAN_POINT('',(-1.52363415200006,2.7,-4.49900422000002));
#324685=CARTESIAN_POINT('',(-1.52363415200006,12.2,-4.49900422000002));
#324686=CARTESIAN_POINT('Ctrl Pts',(-1.54920881500006,2.7,-3.68100722400001));
#324687=CARTESIAN_POINT('Ctrl Pts',(-1.5492699808608,2.7,-3.68115413835674));
#324688=CARTESIAN_POINT('Ctrl Pts',(-1.54932969519839,2.70000000000379,
-3.6813016557513));
#324689=CARTESIAN_POINT('Ctrl Pts',(-1.54951244654765,2.70000000000379,
-3.68175597959113));
#324690=CARTESIAN_POINT('Ctrl Pts',(-1.549639932611,2.70000000000408,-3.68207990099521));
#324691=CARTESIAN_POINT('Ctrl Pts',(-1.55017632519208,2.70000000000408,
-3.68345945901149));
#324692=CARTESIAN_POINT('Ctrl Pts',(-1.55060466855355,2.70000000000408,
-3.68461026767503));
#324693=CARTESIAN_POINT('Ctrl Pts',(-1.55244518831997,2.70000000000408,
-3.68968448235393));
#324694=CARTESIAN_POINT('Ctrl Pts',(-1.55386348666925,2.70000000000408,
-3.69397409267706));
#324695=CARTESIAN_POINT('Ctrl Pts',(-1.55978529038518,2.70000000000408,
-3.71291067441931));
#324696=CARTESIAN_POINT('Ctrl Pts',(-1.56386617840707,2.70000000000408,
-3.72905519462682));
#324697=CARTESIAN_POINT('Ctrl Pts',(-1.57685980730779,2.70000000000408,
-3.78818228384373));
#324698=CARTESIAN_POINT('Ctrl Pts',(-1.58522695273552,2.7,-3.8452561404863));
#324699=CARTESIAN_POINT('Ctrl Pts',(-1.59579187190059,2.7,-4.04559018005418));
#324700=CARTESIAN_POINT('Ctrl Pts',(-1.58808709236768,2.7,-4.24179194839253));
#324701=CARTESIAN_POINT('Ctrl Pts',(-1.52363415300006,2.7,-4.49900422000002));
#324702=CARTESIAN_POINT('Origin',(-5.66300478732629E-14,15.2,-1.77635683940025E-14));
#324703=CARTESIAN_POINT('',(-1.20083826600006,2.7,-4.59570315100002));
#324704=CARTESIAN_POINT('',(-1.20083826600006,12.2,-4.59570315100001));
#324705=CARTESIAN_POINT('Origin',(-5.66300478732629E-14,2.7,-1.92943768261394E-14));
#324706=CARTESIAN_POINT('Ctrl Pts',(-1.20083826600006,12.2,-4.59570315100001));
#324707=CARTESIAN_POINT('Ctrl Pts',(-1.20083826600006,5.2,-4.59570315100001));
#324708=CARTESIAN_POINT('Ctrl Pts',(-1.20083826600006,2.2,-4.59570315100001));
#324709=CARTESIAN_POINT('Ctrl Pts',(-1.20044580000006,12.2,-4.59534252100001));
#324710=CARTESIAN_POINT('Ctrl Pts',(-1.20044580000006,5.2,-4.59534252100001));
#324711=CARTESIAN_POINT('Ctrl Pts',(-1.20044580000006,2.2,-4.59534252100001));
#324712=CARTESIAN_POINT('Ctrl Pts',(-1.19966130200006,12.2,-4.59462129000002));
#324713=CARTESIAN_POINT('Ctrl Pts',(-1.19966130200006,5.2,-4.59462129000002));
#324714=CARTESIAN_POINT('Ctrl Pts',(-1.19966130200006,2.2,-4.59462129000002));
#324715=CARTESIAN_POINT('Ctrl Pts',(-1.19848586200006,12.2,-4.59353952500001));
#324716=CARTESIAN_POINT('Ctrl Pts',(-1.19848586200006,5.2,-4.59353952500001));
#324717=CARTESIAN_POINT('Ctrl Pts',(-1.19848586200006,2.2,-4.59353952500001));
#324718=CARTESIAN_POINT('Ctrl Pts',(-1.19692122000005,12.2,-4.59209734200002));
#324719=CARTESIAN_POINT('Ctrl Pts',(-1.19692122000005,5.2,-4.59209734200002));
#324720=CARTESIAN_POINT('Ctrl Pts',(-1.19692122000005,2.2,-4.59209734200002));
#324721=CARTESIAN_POINT('Ctrl Pts',(-1.19496977000005,12.2,-4.59029489100002));
#324722=CARTESIAN_POINT('Ctrl Pts',(-1.19496977000005,5.2,-4.59029489100002));
#324723=CARTESIAN_POINT('Ctrl Pts',(-1.19496977000005,2.2,-4.59029489100002));
#324724=CARTESIAN_POINT('Ctrl Pts',(-1.19302267400006,12.2,-4.58849272400002));
#324725=CARTESIAN_POINT('Ctrl Pts',(-1.19302267400006,5.2,-4.58849272400002));
#324726=CARTESIAN_POINT('Ctrl Pts',(-1.19302267400006,2.2,-4.58849272400002));
#324727=CARTESIAN_POINT('Ctrl Pts',(-1.19107993200006,12.2,-4.58669084000002));
#324728=CARTESIAN_POINT('Ctrl Pts',(-1.19107993200006,5.2,-4.58669084000002));
#324729=CARTESIAN_POINT('Ctrl Pts',(-1.19107993200006,2.2,-4.58669084000002));
#324730=CARTESIAN_POINT('Ctrl Pts',(-1.18914154200006,12.2,-4.58488924600001));
#324731=CARTESIAN_POINT('Ctrl Pts',(-1.18914154200006,5.2,-4.58488924600001));
#324732=CARTESIAN_POINT('Ctrl Pts',(-1.18914154200006,2.2,-4.58488924600001));
#324733=CARTESIAN_POINT('Ctrl Pts',(-1.18720750800006,12.2,-4.58308794500002));
#324734=CARTESIAN_POINT('Ctrl Pts',(-1.18720750800006,5.2,-4.58308794500002));
#324735=CARTESIAN_POINT('Ctrl Pts',(-1.18720750800006,2.2,-4.58308794500002));
#324736=CARTESIAN_POINT('Ctrl Pts',(-1.18527782700006,12.2,-4.58128694600001));
#324737=CARTESIAN_POINT('Ctrl Pts',(-1.18527782700006,5.2,-4.58128694600001));
#324738=CARTESIAN_POINT('Ctrl Pts',(-1.18527782700006,2.2,-4.58128694600001));
#324739=CARTESIAN_POINT('Ctrl Pts',(-1.18335250000006,12.2,-4.57948626000002));
#324740=CARTESIAN_POINT('Ctrl Pts',(-1.18335250000006,5.2,-4.57948626000002));
#324741=CARTESIAN_POINT('Ctrl Pts',(-1.18335250000006,2.2,-4.57948626000002));
#324742=CARTESIAN_POINT('Ctrl Pts',(-1.18143152900006,12.2,-4.57768589700001));
#324743=CARTESIAN_POINT('Ctrl Pts',(-1.18143152900006,5.2,-4.57768589700001));
#324744=CARTESIAN_POINT('Ctrl Pts',(-1.18143152900006,2.2,-4.57768589700001));
#324745=CARTESIAN_POINT('Ctrl Pts',(-1.17951491300005,12.2,-4.57588586700002));
#324746=CARTESIAN_POINT('Ctrl Pts',(-1.17951491300005,5.2,-4.57588586700002));
#324747=CARTESIAN_POINT('Ctrl Pts',(-1.17951491300005,2.2,-4.57588586700002));
#324748=CARTESIAN_POINT('Ctrl Pts',(-1.17760265200006,12.2,-4.57408618200001));
#324749=CARTESIAN_POINT('Ctrl Pts',(-1.17760265200006,5.2,-4.57408618200001));
#324750=CARTESIAN_POINT('Ctrl Pts',(-1.17760265200006,2.2,-4.57408618200001));
#324751=CARTESIAN_POINT('Ctrl Pts',(-1.17569474700006,12.2,-4.57228685000001));
#324752=CARTESIAN_POINT('Ctrl Pts',(-1.17569474700006,5.2,-4.57228685000001));
#324753=CARTESIAN_POINT('Ctrl Pts',(-1.17569474700006,2.2,-4.57228685000001));
#324754=CARTESIAN_POINT('Ctrl Pts',(-1.17379119700006,12.2,-4.57048788200002));
#324755=CARTESIAN_POINT('Ctrl Pts',(-1.17379119700006,5.2,-4.57048788200002));
#324756=CARTESIAN_POINT('Ctrl Pts',(-1.17379119700006,2.2,-4.57048788200002));
#324757=CARTESIAN_POINT('Ctrl Pts',(-1.17189200400006,12.2,-4.56868928400001));
#324758=CARTESIAN_POINT('Ctrl Pts',(-1.17189200400006,5.2,-4.56868928400001));
#324759=CARTESIAN_POINT('Ctrl Pts',(-1.17189200400006,2.2,-4.56868928400001));
#324760=CARTESIAN_POINT('Ctrl Pts',(-1.16999716800006,12.2,-4.56689106400002));
#324761=CARTESIAN_POINT('Ctrl Pts',(-1.16999716800006,5.2,-4.56689106400002));
#324762=CARTESIAN_POINT('Ctrl Pts',(-1.16999716800006,2.2,-4.56689106400002));
#324763=CARTESIAN_POINT('Ctrl Pts',(-1.16810668600006,12.2,-4.56509323000001));
#324764=CARTESIAN_POINT('Ctrl Pts',(-1.16810668600006,5.2,-4.56509323000001));
#324765=CARTESIAN_POINT('Ctrl Pts',(-1.16810668600006,2.2,-4.56509323000001));
#324766=CARTESIAN_POINT('Ctrl Pts',(-1.16622056200006,12.2,-4.56329579100001));
#324767=CARTESIAN_POINT('Ctrl Pts',(-1.16622056200006,5.2,-4.56329579100001));
#324768=CARTESIAN_POINT('Ctrl Pts',(-1.16622056200006,2.2,-4.56329579100001));
#324769=CARTESIAN_POINT('Ctrl Pts',(-1.16433879500006,12.2,-4.56149875400001));
#324770=CARTESIAN_POINT('Ctrl Pts',(-1.16433879500006,5.2,-4.56149875400001));
#324771=CARTESIAN_POINT('Ctrl Pts',(-1.16433879500006,2.2,-4.56149875400001));
#324772=CARTESIAN_POINT('Ctrl Pts',(-1.16246138400006,12.2,-4.55970212800001));
#324773=CARTESIAN_POINT('Ctrl Pts',(-1.16246138400006,5.2,-4.55970212800001));
#324774=CARTESIAN_POINT('Ctrl Pts',(-1.16246138400006,2.2,-4.55970212800001));
#324775=CARTESIAN_POINT('Ctrl Pts',(-1.16058832900006,12.2,-4.55790592300001));
#324776=CARTESIAN_POINT('Ctrl Pts',(-1.16058832900006,5.2,-4.55790592300001));
#324777=CARTESIAN_POINT('Ctrl Pts',(-1.16058832900006,2.2,-4.55790592300001));
#324778=CARTESIAN_POINT('Ctrl Pts',(-1.15871963300005,12.2,-4.55611014800001));
#324779=CARTESIAN_POINT('Ctrl Pts',(-1.15871963300005,5.2,-4.55611014800001));
#324780=CARTESIAN_POINT('Ctrl Pts',(-1.15871963300005,2.2,-4.55611014800001));
#324781=CARTESIAN_POINT('Ctrl Pts',(-1.15685529300006,12.2,-4.55431481100002));
#324782=CARTESIAN_POINT('Ctrl Pts',(-1.15685529300006,5.2,-4.55431481100002));
#324783=CARTESIAN_POINT('Ctrl Pts',(-1.15685529300006,2.2,-4.55431481100002));
#324784=CARTESIAN_POINT('Ctrl Pts',(-1.15499531100006,12.2,-4.55251992200001));
#324785=CARTESIAN_POINT('Ctrl Pts',(-1.15499531100006,5.2,-4.55251992200001));
#324786=CARTESIAN_POINT('Ctrl Pts',(-1.15499531100006,2.2,-4.55251992200001));
#324787=CARTESIAN_POINT('Ctrl Pts',(-1.15313968500006,12.2,-4.55072549000001));
#324788=CARTESIAN_POINT('Ctrl Pts',(-1.15313968500006,5.2,-4.55072549000001));
#324789=CARTESIAN_POINT('Ctrl Pts',(-1.15313968500006,2.2,-4.55072549000001));
#324790=CARTESIAN_POINT('Ctrl Pts',(-1.15128841800006,12.2,-4.54893152300002));
#324791=CARTESIAN_POINT('Ctrl Pts',(-1.15128841800006,5.2,-4.54893152300002));
#324792=CARTESIAN_POINT('Ctrl Pts',(-1.15128841800006,2.2,-4.54893152300002));
#324793=CARTESIAN_POINT('Ctrl Pts',(-1.14944150700006,12.2,-4.54713802900002));
#324794=CARTESIAN_POINT('Ctrl Pts',(-1.14944150700006,5.2,-4.54713802900002));
#324795=CARTESIAN_POINT('Ctrl Pts',(-1.14944150700006,2.2,-4.54713802900002));
#324796=CARTESIAN_POINT('Ctrl Pts',(-1.14759895400006,12.2,-4.54534501800001));
#324797=CARTESIAN_POINT('Ctrl Pts',(-1.14759895400006,5.2,-4.54534501800001));
#324798=CARTESIAN_POINT('Ctrl Pts',(-1.14759895400006,2.2,-4.54534501800001));
#324799=CARTESIAN_POINT('Ctrl Pts',(-1.14576075900006,12.2,-4.54355249800001));
#324800=CARTESIAN_POINT('Ctrl Pts',(-1.14576075900006,5.2,-4.54355249800001));
#324801=CARTESIAN_POINT('Ctrl Pts',(-1.14576075900006,2.2,-4.54355249800001));
#324802=CARTESIAN_POINT('Ctrl Pts',(-1.14392692100005,12.2,-4.54176047800001));
#324803=CARTESIAN_POINT('Ctrl Pts',(-1.14392692100005,5.2,-4.54176047800001));
#324804=CARTESIAN_POINT('Ctrl Pts',(-1.14392692100005,2.2,-4.54176047800001));
#324805=CARTESIAN_POINT('Ctrl Pts',(-1.14209744100006,12.2,-4.53996896700001));
#324806=CARTESIAN_POINT('Ctrl Pts',(-1.14209744100006,5.2,-4.53996896700001));
#324807=CARTESIAN_POINT('Ctrl Pts',(-1.14209744100006,2.2,-4.53996896700001));
#324808=CARTESIAN_POINT('Ctrl Pts',(-1.14027231800006,12.2,-4.53817797400001));
#324809=CARTESIAN_POINT('Ctrl Pts',(-1.14027231800006,5.2,-4.53817797400001));
#324810=CARTESIAN_POINT('Ctrl Pts',(-1.14027231800006,2.2,-4.53817797400001));
#324811=CARTESIAN_POINT('Ctrl Pts',(-1.13845155200006,12.2,-4.53638750700001));
#324812=CARTESIAN_POINT('Ctrl Pts',(-1.13845155200006,5.2,-4.53638750700001));
#324813=CARTESIAN_POINT('Ctrl Pts',(-1.13845155200006,2.2,-4.53638750700001));
#324814=CARTESIAN_POINT('Ctrl Pts',(-1.13663514400006,12.2,-4.53459757600001));
#324815=CARTESIAN_POINT('Ctrl Pts',(-1.13663514400006,5.2,-4.53459757600001));
#324816=CARTESIAN_POINT('Ctrl Pts',(-1.13663514400006,2.2,-4.53459757600001));
#324817=CARTESIAN_POINT('Ctrl Pts',(-1.13482309400006,12.2,-4.53280818900001));
#324818=CARTESIAN_POINT('Ctrl Pts',(-1.13482309400006,5.2,-4.53280818900001));
#324819=CARTESIAN_POINT('Ctrl Pts',(-1.13482309400006,2.2,-4.53280818900001));
#324820=CARTESIAN_POINT('Ctrl Pts',(-1.13301540100006,12.2,-4.53101935600001));
#324821=CARTESIAN_POINT('Ctrl Pts',(-1.13301540100006,5.2,-4.53101935600001));
#324822=CARTESIAN_POINT('Ctrl Pts',(-1.13301540100006,2.2,-4.53101935600001));
#324823=CARTESIAN_POINT('Ctrl Pts',(-1.13121206600006,12.2,-4.52923108400002));
#324824=CARTESIAN_POINT('Ctrl Pts',(-1.13121206600006,5.2,-4.52923108400002));
#324825=CARTESIAN_POINT('Ctrl Pts',(-1.13121206600006,2.2,-4.52923108400002));
#324826=CARTESIAN_POINT('Ctrl Pts',(-1.12941308600006,12.2,-4.52744338400001));
#324827=CARTESIAN_POINT('Ctrl Pts',(-1.12941308600006,5.2,-4.52744338400001));
#324828=CARTESIAN_POINT('Ctrl Pts',(-1.12941308600006,2.2,-4.52744338400001));
#324829=CARTESIAN_POINT('Ctrl Pts',(-1.12761846500006,12.2,-4.52565626400002));
#324830=CARTESIAN_POINT('Ctrl Pts',(-1.12761846500006,5.2,-4.52565626400002));
#324831=CARTESIAN_POINT('Ctrl Pts',(-1.12761846500006,2.2,-4.52565626400002));
#324832=CARTESIAN_POINT('Ctrl Pts',(-1.12582820100006,12.2,-4.52386973300001));
#324833=CARTESIAN_POINT('Ctrl Pts',(-1.12582820100006,5.2,-4.52386973300001));
#324834=CARTESIAN_POINT('Ctrl Pts',(-1.12582820100006,2.2,-4.52386973300001));
#324835=CARTESIAN_POINT('Ctrl Pts',(-1.12404229400005,12.2,-4.52208379900001));
#324836=CARTESIAN_POINT('Ctrl Pts',(-1.12404229400005,5.2,-4.52208379900001));
#324837=CARTESIAN_POINT('Ctrl Pts',(-1.12404229400005,2.2,-4.52208379900001));
#324838=CARTESIAN_POINT('Ctrl Pts',(-1.12226074300006,12.2,-4.52029847200001));
#324839=CARTESIAN_POINT('Ctrl Pts',(-1.12226074300006,5.2,-4.52029847200001));
#324840=CARTESIAN_POINT('Ctrl Pts',(-1.12226074300006,2.2,-4.52029847200001));
#324841=CARTESIAN_POINT('Ctrl Pts',(-1.12048354900006,12.2,-4.51851376100001));
#324842=CARTESIAN_POINT('Ctrl Pts',(-1.12048354900006,5.2,-4.51851376100001));
#324843=CARTESIAN_POINT('Ctrl Pts',(-1.12048354900006,2.2,-4.51851376100001));
#324844=CARTESIAN_POINT('Ctrl Pts',(-1.11871071100005,12.2,-4.51672967500001));
#324845=CARTESIAN_POINT('Ctrl Pts',(-1.11871071100005,5.2,-4.51672967500001));
#324846=CARTESIAN_POINT('Ctrl Pts',(-1.11871071100005,2.2,-4.51672967500001));
#324847=CARTESIAN_POINT('Ctrl Pts',(-1.11694223100006,12.2,-4.51494622200002));
#324848=CARTESIAN_POINT('Ctrl Pts',(-1.11694223100006,5.2,-4.51494622200002));
#324849=CARTESIAN_POINT('Ctrl Pts',(-1.11694223100006,2.2,-4.51494622200002));
#324850=CARTESIAN_POINT('Ctrl Pts',(-1.11517810600006,12.2,-4.51316341200001));
#324851=CARTESIAN_POINT('Ctrl Pts',(-1.11517810600006,5.2,-4.51316341200001));
#324852=CARTESIAN_POINT('Ctrl Pts',(-1.11517810600006,2.2,-4.51316341200001));
#324853=CARTESIAN_POINT('Ctrl Pts',(-1.11341833700005,12.2,-4.51138125500002));
#324854=CARTESIAN_POINT('Ctrl Pts',(-1.11341833700005,5.2,-4.51138125500002));
#324855=CARTESIAN_POINT('Ctrl Pts',(-1.11341833700005,2.2,-4.51138125500002));
#324856=CARTESIAN_POINT('Ctrl Pts',(-1.11166292300006,12.2,-4.50959975800002));
#324857=CARTESIAN_POINT('Ctrl Pts',(-1.11166292300006,5.2,-4.50959975800002));
#324858=CARTESIAN_POINT('Ctrl Pts',(-1.11166292300006,2.2,-4.50959975800002));
#324859=CARTESIAN_POINT('Ctrl Pts',(-1.10991186600006,12.2,-4.50781893000002));
#324860=CARTESIAN_POINT('Ctrl Pts',(-1.10991186600006,5.2,-4.50781893000002));
#324861=CARTESIAN_POINT('Ctrl Pts',(-1.10991186600006,2.2,-4.50781893000002));
#324862=CARTESIAN_POINT('Ctrl Pts',(-1.10816516400006,12.2,-4.50603878100001));
#324863=CARTESIAN_POINT('Ctrl Pts',(-1.10816516400006,5.2,-4.50603878100001));
#324864=CARTESIAN_POINT('Ctrl Pts',(-1.10816516400006,2.2,-4.50603878100001));
#324865=CARTESIAN_POINT('Ctrl Pts',(-1.10642281700006,12.2,-4.50425932100002));
#324866=CARTESIAN_POINT('Ctrl Pts',(-1.10642281700006,5.2,-4.50425932100002));
#324867=CARTESIAN_POINT('Ctrl Pts',(-1.10642281700006,2.2,-4.50425932100002));
#324868=CARTESIAN_POINT('Ctrl Pts',(-1.10468482400006,12.2,-4.50248055700001));
#324869=CARTESIAN_POINT('Ctrl Pts',(-1.10468482400006,5.2,-4.50248055700001));
#324870=CARTESIAN_POINT('Ctrl Pts',(-1.10468482400006,2.2,-4.50248055700001));
#324871=CARTESIAN_POINT('Ctrl Pts',(-1.10295118700006,12.2,-4.50070249900001));
#324872=CARTESIAN_POINT('Ctrl Pts',(-1.10295118700006,5.2,-4.50070249900001));
#324873=CARTESIAN_POINT('Ctrl Pts',(-1.10295118700006,2.2,-4.50070249900001));
#324874=CARTESIAN_POINT('Ctrl Pts',(-1.10122190400006,12.2,-4.49892515500002));
#324875=CARTESIAN_POINT('Ctrl Pts',(-1.10122190400006,5.2,-4.49892515500002));
#324876=CARTESIAN_POINT('Ctrl Pts',(-1.10122190400006,2.2,-4.49892515500002));
#324877=CARTESIAN_POINT('Ctrl Pts',(-1.09949697400006,12.2,-4.49714853700002));
#324878=CARTESIAN_POINT('Ctrl Pts',(-1.09949697400006,5.2,-4.49714853700002));
#324879=CARTESIAN_POINT('Ctrl Pts',(-1.09949697400006,2.2,-4.49714853700002));
#324880=CARTESIAN_POINT('Ctrl Pts',(-1.09777639800006,12.2,-4.49537265200001));
#324881=CARTESIAN_POINT('Ctrl Pts',(-1.09777639800006,5.2,-4.49537265200001));
#324882=CARTESIAN_POINT('Ctrl Pts',(-1.09777639800006,2.2,-4.49537265200001));
#324883=CARTESIAN_POINT('Ctrl Pts',(-1.09606017600006,12.2,-4.49359750800001));
#324884=CARTESIAN_POINT('Ctrl Pts',(-1.09606017600006,5.2,-4.49359750800001));
#324885=CARTESIAN_POINT('Ctrl Pts',(-1.09606017600006,2.2,-4.49359750800001));
#324886=CARTESIAN_POINT('Ctrl Pts',(-1.09434830700006,12.2,-4.49182311700001));
#324887=CARTESIAN_POINT('Ctrl Pts',(-1.09434830700006,5.2,-4.49182311700001));
#324888=CARTESIAN_POINT('Ctrl Pts',(-1.09434830700006,2.2,-4.49182311700001));
#324889=CARTESIAN_POINT('Ctrl Pts',(-1.09264079000006,12.2,-4.49004948600002));
#324890=CARTESIAN_POINT('Ctrl Pts',(-1.09264079000006,5.2,-4.49004948600002));
#324891=CARTESIAN_POINT('Ctrl Pts',(-1.09264079000006,2.2,-4.49004948600002));
#324892=CARTESIAN_POINT('Ctrl Pts',(-1.09093762600006,12.2,-4.48827662500001));
#324893=CARTESIAN_POINT('Ctrl Pts',(-1.09093762600006,5.2,-4.48827662500001));
#324894=CARTESIAN_POINT('Ctrl Pts',(-1.09093762600006,2.2,-4.48827662500001));
#324895=CARTESIAN_POINT('Ctrl Pts',(-1.08923881400006,12.2,-4.48650454200001));
#324896=CARTESIAN_POINT('Ctrl Pts',(-1.08923881400006,5.2,-4.48650454200001));
#324897=CARTESIAN_POINT('Ctrl Pts',(-1.08923881400006,2.2,-4.48650454200001));
#324898=CARTESIAN_POINT('Ctrl Pts',(-1.08754435300006,12.2,-4.48473324900001));
#324899=CARTESIAN_POINT('Ctrl Pts',(-1.08754435300006,5.2,-4.48473324900001));
#324900=CARTESIAN_POINT('Ctrl Pts',(-1.08754435300006,2.2,-4.48473324900001));
#324901=CARTESIAN_POINT('Ctrl Pts',(-1.08585424400006,12.2,-4.48296275200001));
#324902=CARTESIAN_POINT('Ctrl Pts',(-1.08585424400006,5.2,-4.48296275200001));
#324903=CARTESIAN_POINT('Ctrl Pts',(-1.08585424400006,2.2,-4.48296275200001));
#324904=CARTESIAN_POINT('Ctrl Pts',(-1.08416848500006,12.2,-4.48119306300002));
#324905=CARTESIAN_POINT('Ctrl Pts',(-1.08416848500006,5.2,-4.48119306300002));
#324906=CARTESIAN_POINT('Ctrl Pts',(-1.08416848500006,2.2,-4.48119306300002));
#324907=CARTESIAN_POINT('Ctrl Pts',(-1.08248707700006,12.2,-4.47942418800002));
#324908=CARTESIAN_POINT('Ctrl Pts',(-1.08248707700006,5.2,-4.47942418800002));
#324909=CARTESIAN_POINT('Ctrl Pts',(-1.08248707700006,2.2,-4.47942418800002));
#324910=CARTESIAN_POINT('Ctrl Pts',(-1.08081001900006,12.2,-4.47765613900001));
#324911=CARTESIAN_POINT('Ctrl Pts',(-1.08081001900006,5.2,-4.47765613900001));
#324912=CARTESIAN_POINT('Ctrl Pts',(-1.08081001900006,2.2,-4.47765613900001));
#324913=CARTESIAN_POINT('Ctrl Pts',(-1.07913731000005,12.2,-4.47588892300002));
#324914=CARTESIAN_POINT('Ctrl Pts',(-1.07913731000005,5.2,-4.47588892300002));
#324915=CARTESIAN_POINT('Ctrl Pts',(-1.07913731000005,2.2,-4.47588892300002));
#324916=CARTESIAN_POINT('Ctrl Pts',(-1.07746895100005,12.2,-4.47412255100001));
#324917=CARTESIAN_POINT('Ctrl Pts',(-1.07746895100005,5.2,-4.47412255100001));
#324918=CARTESIAN_POINT('Ctrl Pts',(-1.07746895100005,2.2,-4.47412255100001));
#324919=CARTESIAN_POINT('Ctrl Pts',(-1.07580494000006,12.2,-4.47235703200001));
#324920=CARTESIAN_POINT('Ctrl Pts',(-1.07580494000006,5.2,-4.47235703200001));
#324921=CARTESIAN_POINT('Ctrl Pts',(-1.07580494000006,2.2,-4.47235703200001));
#324922=CARTESIAN_POINT('Ctrl Pts',(-1.07414527700006,12.2,-4.47059237500001));
#324923=CARTESIAN_POINT('Ctrl Pts',(-1.07414527700006,5.2,-4.47059237500001));
#324924=CARTESIAN_POINT('Ctrl Pts',(-1.07414527700006,2.2,-4.47059237500001));
#324925=CARTESIAN_POINT('Ctrl Pts',(-1.07248996200005,12.2,-4.46882858800001));
#324926=CARTESIAN_POINT('Ctrl Pts',(-1.07248996200005,5.2,-4.46882858800001));
#324927=CARTESIAN_POINT('Ctrl Pts',(-1.07248996200005,2.2,-4.46882858800001));
#324928=CARTESIAN_POINT('Ctrl Pts',(-1.07083899300006,12.2,-4.46706568300002));
#324929=CARTESIAN_POINT('Ctrl Pts',(-1.07083899300006,5.2,-4.46706568300002));
#324930=CARTESIAN_POINT('Ctrl Pts',(-1.07083899300006,2.2,-4.46706568300002));
#324931=CARTESIAN_POINT('Ctrl Pts',(-1.06919237200006,12.2,-4.46530366700001));
#324932=CARTESIAN_POINT('Ctrl Pts',(-1.06919237200006,5.2,-4.46530366700001));
#324933=CARTESIAN_POINT('Ctrl Pts',(-1.06919237200006,2.2,-4.46530366700001));
#324934=CARTESIAN_POINT('Ctrl Pts',(-1.06755009600006,12.2,-4.46354255000001));
#324935=CARTESIAN_POINT('Ctrl Pts',(-1.06755009600006,5.2,-4.46354255000001));
#324936=CARTESIAN_POINT('Ctrl Pts',(-1.06755009600006,2.2,-4.46354255000001));
#324937=CARTESIAN_POINT('Ctrl Pts',(-1.06591216500005,12.2,-4.46178234200001));
#324938=CARTESIAN_POINT('Ctrl Pts',(-1.06591216500005,5.2,-4.46178234200001));
#324939=CARTESIAN_POINT('Ctrl Pts',(-1.06591216500005,2.2,-4.46178234200001));
#324940=CARTESIAN_POINT('Ctrl Pts',(-1.06427858000006,12.2,-4.46002305000002));
#324941=CARTESIAN_POINT('Ctrl Pts',(-1.06427858000006,5.2,-4.46002305000002));
#324942=CARTESIAN_POINT('Ctrl Pts',(-1.06427858000006,2.2,-4.46002305000002));
#324943=CARTESIAN_POINT('Ctrl Pts',(-1.06264933900006,12.2,-4.45826468700002));
#324944=CARTESIAN_POINT('Ctrl Pts',(-1.06264933900006,5.2,-4.45826468700002));
#324945=CARTESIAN_POINT('Ctrl Pts',(-1.06264933900006,2.2,-4.45826468700002));
#324946=CARTESIAN_POINT('Ctrl Pts',(-1.06102444200006,12.2,-4.45650725900002));
#324947=CARTESIAN_POINT('Ctrl Pts',(-1.06102444200006,5.2,-4.45650725900002));
#324948=CARTESIAN_POINT('Ctrl Pts',(-1.06102444200006,2.2,-4.45650725900002));
#324949=CARTESIAN_POINT('Ctrl Pts',(-1.05940388700006,12.2,-4.45475077800001));
#324950=CARTESIAN_POINT('Ctrl Pts',(-1.05940388700006,5.2,-4.45475077800001));
#324951=CARTESIAN_POINT('Ctrl Pts',(-1.05940388700006,2.2,-4.45475077800001));
#324952=CARTESIAN_POINT('Ctrl Pts',(-1.05778767600005,12.2,-4.45299525200001));
#324953=CARTESIAN_POINT('Ctrl Pts',(-1.05778767600005,5.2,-4.45299525200001));
#324954=CARTESIAN_POINT('Ctrl Pts',(-1.05778767600005,2.2,-4.45299525200001));
#324955=CARTESIAN_POINT('Ctrl Pts',(-1.05617580600006,12.2,-4.45124069000002));
#324956=CARTESIAN_POINT('Ctrl Pts',(-1.05617580600006,5.2,-4.45124069000002));
#324957=CARTESIAN_POINT('Ctrl Pts',(-1.05617580600006,2.2,-4.45124069000002));
#324958=CARTESIAN_POINT('Ctrl Pts',(-1.05456827700006,12.2,-4.44948710300002));
#324959=CARTESIAN_POINT('Ctrl Pts',(-1.05456827700006,5.2,-4.44948710300002));
#324960=CARTESIAN_POINT('Ctrl Pts',(-1.05456827700006,2.2,-4.44948710300002));
#324961=CARTESIAN_POINT('Ctrl Pts',(-1.05296508800006,12.2,-4.44773449800001));
#324962=CARTESIAN_POINT('Ctrl Pts',(-1.05296508800006,5.2,-4.44773449800001));
#324963=CARTESIAN_POINT('Ctrl Pts',(-1.05296508800006,2.2,-4.44773449800001));
#324964=CARTESIAN_POINT('Ctrl Pts',(-1.05136624100005,12.2,-4.44598288600002));
#324965=CARTESIAN_POINT('Ctrl Pts',(-1.05136624100005,5.2,-4.44598288600002));
#324966=CARTESIAN_POINT('Ctrl Pts',(-1.05136624100005,2.2,-4.44598288600002));
#324967=CARTESIAN_POINT('Ctrl Pts',(-1.04977173200006,12.2,-4.44423227700002));
#324968=CARTESIAN_POINT('Ctrl Pts',(-1.04977173200006,5.2,-4.44423227700002));
#324969=CARTESIAN_POINT('Ctrl Pts',(-1.04977173200006,2.2,-4.44423227700002));
#324970=CARTESIAN_POINT('Ctrl Pts',(-1.04818156000006,12.2,-4.44248267900001));
#324971=CARTESIAN_POINT('Ctrl Pts',(-1.04818156000006,5.2,-4.44248267900001));
#324972=CARTESIAN_POINT('Ctrl Pts',(-1.04818156000006,2.2,-4.44248267900001));
#324973=CARTESIAN_POINT('Ctrl Pts',(-1.04659572800006,12.2,-4.44073410200001));
#324974=CARTESIAN_POINT('Ctrl Pts',(-1.04659572800006,5.2,-4.44073410200001));
#324975=CARTESIAN_POINT('Ctrl Pts',(-1.04659572800006,2.2,-4.44073410200001));
#324976=CARTESIAN_POINT('Ctrl Pts',(-1.04501423200006,12.2,-4.43898655500002));
#324977=CARTESIAN_POINT('Ctrl Pts',(-1.04501423200006,5.2,-4.43898655500002));
#324978=CARTESIAN_POINT('Ctrl Pts',(-1.04501423200006,2.2,-4.43898655500002));
#324979=CARTESIAN_POINT('Ctrl Pts',(-1.04343707300006,12.2,-4.43724004900002));
#324980=CARTESIAN_POINT('Ctrl Pts',(-1.04343707300006,5.2,-4.43724004900002));
#324981=CARTESIAN_POINT('Ctrl Pts',(-1.04343707300006,2.2,-4.43724004900002));
#324982=CARTESIAN_POINT('Ctrl Pts',(-1.04186424800006,12.2,-4.43549459200002));
#324983=CARTESIAN_POINT('Ctrl Pts',(-1.04186424800006,5.2,-4.43549459200002));
#324984=CARTESIAN_POINT('Ctrl Pts',(-1.04186424800006,2.2,-4.43549459200002));
#324985=CARTESIAN_POINT('Ctrl Pts',(-1.04029575900006,12.2,-4.43375019500001));
#324986=CARTESIAN_POINT('Ctrl Pts',(-1.04029575900006,5.2,-4.43375019500001));
#324987=CARTESIAN_POINT('Ctrl Pts',(-1.04029575900006,2.2,-4.43375019500001));
#324988=CARTESIAN_POINT('Ctrl Pts',(-1.03873160300005,12.2,-4.43200686600001));
#324989=CARTESIAN_POINT('Ctrl Pts',(-1.03873160300005,5.2,-4.43200686600001));
#324990=CARTESIAN_POINT('Ctrl Pts',(-1.03873160300005,2.2,-4.43200686600001));
#324991=CARTESIAN_POINT('Ctrl Pts',(-1.03717178100006,12.2,-4.43026461500001));
#324992=CARTESIAN_POINT('Ctrl Pts',(-1.03717178100006,5.2,-4.43026461500001));
#324993=CARTESIAN_POINT('Ctrl Pts',(-1.03717178100006,2.2,-4.43026461500001));
#324994=CARTESIAN_POINT('Ctrl Pts',(-1.03561629200006,12.2,-4.42852345200002));
#324995=CARTESIAN_POINT('Ctrl Pts',(-1.03561629200006,5.2,-4.42852345200002));
#324996=CARTESIAN_POINT('Ctrl Pts',(-1.03561629200006,2.2,-4.42852345200002));
#324997=CARTESIAN_POINT('Ctrl Pts',(-1.03406513300005,12.2,-4.42678338600001));
#324998=CARTESIAN_POINT('Ctrl Pts',(-1.03406513300005,5.2,-4.42678338600001));
#324999=CARTESIAN_POINT('Ctrl Pts',(-1.03406513300005,2.2,-4.42678338600001));
#325000=CARTESIAN_POINT('Ctrl Pts',(-1.03251830500006,12.2,-4.42504442600002));
#325001=CARTESIAN_POINT('Ctrl Pts',(-1.03251830500006,5.2,-4.42504442600002));
#325002=CARTESIAN_POINT('Ctrl Pts',(-1.03251830500006,2.2,-4.42504442600002));
#325003=CARTESIAN_POINT('Ctrl Pts',(-1.03097580700006,12.2,-4.42330658300001));
#325004=CARTESIAN_POINT('Ctrl Pts',(-1.03097580700006,5.2,-4.42330658300001));
#325005=CARTESIAN_POINT('Ctrl Pts',(-1.03097580700006,2.2,-4.42330658300001));
#325006=CARTESIAN_POINT('Ctrl Pts',(-1.02943763800006,12.2,-4.42156986600001));
#325007=CARTESIAN_POINT('Ctrl Pts',(-1.02943763800006,5.2,-4.42156986600001));
#325008=CARTESIAN_POINT('Ctrl Pts',(-1.02943763800006,2.2,-4.42156986600001));
#325009=CARTESIAN_POINT('Ctrl Pts',(-1.02790379700005,12.2,-4.41983428400002));
#325010=CARTESIAN_POINT('Ctrl Pts',(-1.02790379700005,5.2,-4.41983428400002));
#325011=CARTESIAN_POINT('Ctrl Pts',(-1.02790379700005,2.2,-4.41983428400002));
#325012=CARTESIAN_POINT('Ctrl Pts',(-1.02637428300006,12.2,-4.41809984700001));
#325013=CARTESIAN_POINT('Ctrl Pts',(-1.02637428300006,5.2,-4.41809984700001));
#325014=CARTESIAN_POINT('Ctrl Pts',(-1.02637428300006,2.2,-4.41809984700001));
#325015=CARTESIAN_POINT('Ctrl Pts',(-1.02484909500006,12.2,-4.41636656500001));
#325016=CARTESIAN_POINT('Ctrl Pts',(-1.02484909500006,5.2,-4.41636656500001));
#325017=CARTESIAN_POINT('Ctrl Pts',(-1.02484909500006,2.2,-4.41636656500001));
#325018=CARTESIAN_POINT('Ctrl Pts',(-1.02332823300006,12.2,-4.41463444800001));
#325019=CARTESIAN_POINT('Ctrl Pts',(-1.02332823300006,5.2,-4.41463444800001));
#325020=CARTESIAN_POINT('Ctrl Pts',(-1.02332823300006,2.2,-4.41463444800001));
#325021=CARTESIAN_POINT('Ctrl Pts',(-1.02181169500006,12.2,-4.41290350400001));
#325022=CARTESIAN_POINT('Ctrl Pts',(-1.02181169500006,5.2,-4.41290350400001));
#325023=CARTESIAN_POINT('Ctrl Pts',(-1.02181169500006,2.2,-4.41290350400001));
#325024=CARTESIAN_POINT('Ctrl Pts',(-1.02029948100006,12.2,-4.41117374400001));
#325025=CARTESIAN_POINT('Ctrl Pts',(-1.02029948100006,5.2,-4.41117374400001));
#325026=CARTESIAN_POINT('Ctrl Pts',(-1.02029948100006,2.2,-4.41117374400001));
#325027=CARTESIAN_POINT('Ctrl Pts',(-1.01879158900006,12.2,-4.40944517800002));
#325028=CARTESIAN_POINT('Ctrl Pts',(-1.01879158900006,5.2,-4.40944517800002));
#325029=CARTESIAN_POINT('Ctrl Pts',(-1.01879158900006,2.2,-4.40944517800002));
#325030=CARTESIAN_POINT('Ctrl Pts',(-1.01728801800006,12.2,-4.40771781400001));
#325031=CARTESIAN_POINT('Ctrl Pts',(-1.01728801800006,5.2,-4.40771781400001));
#325032=CARTESIAN_POINT('Ctrl Pts',(-1.01728801800006,2.2,-4.40771781400001));
#325033=CARTESIAN_POINT('Ctrl Pts',(-1.01578876700006,12.2,-4.40599166300002));
#325034=CARTESIAN_POINT('Ctrl Pts',(-1.01578876700006,5.2,-4.40599166300002));
#325035=CARTESIAN_POINT('Ctrl Pts',(-1.01578876700006,2.2,-4.40599166300002));
#325036=CARTESIAN_POINT('Ctrl Pts',(-1.01429383600006,12.2,-4.40426673500002));
#325037=CARTESIAN_POINT('Ctrl Pts',(-1.01429383600006,5.2,-4.40426673500002));
#325038=CARTESIAN_POINT('Ctrl Pts',(-1.01429383600006,2.2,-4.40426673500002));
#325039=CARTESIAN_POINT('Ctrl Pts',(-1.01280322400006,12.2,-4.40254303900002));
#325040=CARTESIAN_POINT('Ctrl Pts',(-1.01280322400006,5.2,-4.40254303900002));
#325041=CARTESIAN_POINT('Ctrl Pts',(-1.01280322400006,2.2,-4.40254303900002));
#325042=CARTESIAN_POINT('Ctrl Pts',(-1.01131692900006,12.2,-4.40082058400002));
#325043=CARTESIAN_POINT('Ctrl Pts',(-1.01131692900006,5.2,-4.40082058400002));
#325044=CARTESIAN_POINT('Ctrl Pts',(-1.01131692900006,2.2,-4.40082058400002));
#325045=CARTESIAN_POINT('Ctrl Pts',(-1.00983494900006,12.2,-4.39909938100001));
#325046=CARTESIAN_POINT('Ctrl Pts',(-1.00983494900006,5.2,-4.39909938100001));
#325047=CARTESIAN_POINT('Ctrl Pts',(-1.00983494900006,2.2,-4.39909938100001));
#325048=CARTESIAN_POINT('Ctrl Pts',(-1.00835728600006,12.2,-4.39737943900001));
#325049=CARTESIAN_POINT('Ctrl Pts',(-1.00835728600006,5.2,-4.39737943900001));
#325050=CARTESIAN_POINT('Ctrl Pts',(-1.00835728600006,2.2,-4.39737943900001));
#325051=CARTESIAN_POINT('Ctrl Pts',(-1.00688393600006,12.2,-4.39566076900002));
#325052=CARTESIAN_POINT('Ctrl Pts',(-1.00688393600006,5.2,-4.39566076900002));
#325053=CARTESIAN_POINT('Ctrl Pts',(-1.00688393600006,2.2,-4.39566076900002));
#325054=CARTESIAN_POINT('Ctrl Pts',(-1.00541489900006,12.2,-4.39394337900001));
#325055=CARTESIAN_POINT('Ctrl Pts',(-1.00541489900006,5.2,-4.39394337900001));
#325056=CARTESIAN_POINT('Ctrl Pts',(-1.00541489900006,2.2,-4.39394337900001));
#325057=CARTESIAN_POINT('Ctrl Pts',(-1.00395017500006,12.2,-4.39222728000002));
#325058=CARTESIAN_POINT('Ctrl Pts',(-1.00395017500006,5.2,-4.39222728000002));
#325059=CARTESIAN_POINT('Ctrl Pts',(-1.00395017500006,2.2,-4.39222728000002));
#325060=CARTESIAN_POINT('Ctrl Pts',(-1.00248976100006,12.2,-4.39051248200002));
#325061=CARTESIAN_POINT('Ctrl Pts',(-1.00248976100006,5.2,-4.39051248200002));
#325062=CARTESIAN_POINT('Ctrl Pts',(-1.00248976100006,2.2,-4.39051248200002));
#325063=CARTESIAN_POINT('Ctrl Pts',(-1.00103365600006,12.2,-4.38879899400002));
#325064=CARTESIAN_POINT('Ctrl Pts',(-1.00103365600006,5.2,-4.38879899400002));
#325065=CARTESIAN_POINT('Ctrl Pts',(-1.00103365600006,2.2,-4.38879899400002));
#325066=CARTESIAN_POINT('Ctrl Pts',(-0.999581859000056,12.2,-4.38708682600002));
#325067=CARTESIAN_POINT('Ctrl Pts',(-0.999581859000056,5.2,-4.38708682600002));
#325068=CARTESIAN_POINT('Ctrl Pts',(-0.999581859000056,2.2,-4.38708682600002));
#325069=CARTESIAN_POINT('Ctrl Pts',(-0.998134371000056,12.2,-4.38537598800002));
#325070=CARTESIAN_POINT('Ctrl Pts',(-0.998134371000056,5.2,-4.38537598800002));
#325071=CARTESIAN_POINT('Ctrl Pts',(-0.998134371000056,2.2,-4.38537598800002));
#325072=CARTESIAN_POINT('Ctrl Pts',(-0.996691187000056,12.2,-4.38366649000002));
#325073=CARTESIAN_POINT('Ctrl Pts',(-0.996691187000056,5.2,-4.38366649000002));
#325074=CARTESIAN_POINT('Ctrl Pts',(-0.996691187000056,2.2,-4.38366649000002));
#325075=CARTESIAN_POINT('Ctrl Pts',(-0.995252310000057,12.2,-4.38195834100001));
#325076=CARTESIAN_POINT('Ctrl Pts',(-0.995252310000057,5.2,-4.38195834100001));
#325077=CARTESIAN_POINT('Ctrl Pts',(-0.995252310000057,2.2,-4.38195834100001));
#325078=CARTESIAN_POINT('Ctrl Pts',(-0.993817735000055,12.2,-4.38025155200001));
#325079=CARTESIAN_POINT('Ctrl Pts',(-0.993817735000055,5.2,-4.38025155200001));
#325080=CARTESIAN_POINT('Ctrl Pts',(-0.993817735000055,2.2,-4.38025155200001));
#325081=CARTESIAN_POINT('Ctrl Pts',(-0.992387463000056,12.2,-4.37854613300001));
#325082=CARTESIAN_POINT('Ctrl Pts',(-0.992387463000056,5.2,-4.37854613300001));
#325083=CARTESIAN_POINT('Ctrl Pts',(-0.992387463000056,2.2,-4.37854613300001));
#325084=CARTESIAN_POINT('Ctrl Pts',(-0.990961492000055,12.2,-4.37684209300001));
#325085=CARTESIAN_POINT('Ctrl Pts',(-0.990961492000055,5.2,-4.37684209300001));
#325086=CARTESIAN_POINT('Ctrl Pts',(-0.990961492000055,2.2,-4.37684209300001));
#325087=CARTESIAN_POINT('Ctrl Pts',(-0.989539821000056,12.2,-4.37513944100001));
#325088=CARTESIAN_POINT('Ctrl Pts',(-0.989539821000056,5.2,-4.37513944100001));
#325089=CARTESIAN_POINT('Ctrl Pts',(-0.989539821000056,2.2,-4.37513944100001));
#325090=CARTESIAN_POINT('Ctrl Pts',(-0.988122448000055,12.2,-4.37343819000001));
#325091=CARTESIAN_POINT('Ctrl Pts',(-0.988122448000055,5.2,-4.37343819000001));
#325092=CARTESIAN_POINT('Ctrl Pts',(-0.988122448000055,2.2,-4.37343819000001));
#325093=CARTESIAN_POINT('Ctrl Pts',(-0.986709372000056,12.2,-4.37173834700001));
#325094=CARTESIAN_POINT('Ctrl Pts',(-0.986709372000056,5.2,-4.37173834700001));
#325095=CARTESIAN_POINT('Ctrl Pts',(-0.986709372000056,2.2,-4.37173834700001));
#325096=CARTESIAN_POINT('Ctrl Pts',(-0.985300593000057,12.2,-4.37003992300002));
#325097=CARTESIAN_POINT('Ctrl Pts',(-0.985300593000057,5.2,-4.37003992300002));
#325098=CARTESIAN_POINT('Ctrl Pts',(-0.985300593000057,2.2,-4.37003992300002));
#325099=CARTESIAN_POINT('Ctrl Pts',(-0.983896107000056,12.2,-4.36834292900001));
#325100=CARTESIAN_POINT('Ctrl Pts',(-0.983896107000056,5.2,-4.36834292900001));
#325101=CARTESIAN_POINT('Ctrl Pts',(-0.983896107000056,2.2,-4.36834292900001));
#325102=CARTESIAN_POINT('Ctrl Pts',(-0.982495915000056,12.2,-4.36664737300001));
#325103=CARTESIAN_POINT('Ctrl Pts',(-0.982495915000056,5.2,-4.36664737300001));
#325104=CARTESIAN_POINT('Ctrl Pts',(-0.982495915000056,2.2,-4.36664737300001));
#325105=CARTESIAN_POINT('Ctrl Pts',(-0.981100015000056,12.2,-4.36495326700001));
#325106=CARTESIAN_POINT('Ctrl Pts',(-0.981100015000056,5.2,-4.36495326700001));
#325107=CARTESIAN_POINT('Ctrl Pts',(-0.981100015000056,2.2,-4.36495326700001));
#325108=CARTESIAN_POINT('Ctrl Pts',(-0.979708405000055,12.2,-4.36326061900001));
#325109=CARTESIAN_POINT('Ctrl Pts',(-0.979708405000055,5.2,-4.36326061900001));
#325110=CARTESIAN_POINT('Ctrl Pts',(-0.979708405000055,2.2,-4.36326061900001));
#325111=CARTESIAN_POINT('Ctrl Pts',(-0.978321085000056,12.2,-4.36156944000002));
#325112=CARTESIAN_POINT('Ctrl Pts',(-0.978321085000056,5.2,-4.36156944000002));
#325113=CARTESIAN_POINT('Ctrl Pts',(-0.978321085000056,2.2,-4.36156944000002));
#325114=CARTESIAN_POINT('Ctrl Pts',(-0.976938052000056,12.2,-4.35987974100001));
#325115=CARTESIAN_POINT('Ctrl Pts',(-0.976938052000056,5.2,-4.35987974100001));
#325116=CARTESIAN_POINT('Ctrl Pts',(-0.976938052000056,2.2,-4.35987974100001));
#325117=CARTESIAN_POINT('Ctrl Pts',(-0.975559305000055,12.2,-4.35819153100002));
#325118=CARTESIAN_POINT('Ctrl Pts',(-0.975559305000055,5.2,-4.35819153100002));
#325119=CARTESIAN_POINT('Ctrl Pts',(-0.975559305000055,2.2,-4.35819153100002));
#325120=CARTESIAN_POINT('Ctrl Pts',(-0.974184843000057,12.2,-4.35650481900002));
#325121=CARTESIAN_POINT('Ctrl Pts',(-0.974184843000057,5.2,-4.35650481900002));
#325122=CARTESIAN_POINT('Ctrl Pts',(-0.974184843000057,2.2,-4.35650481900002));
#325123=CARTESIAN_POINT('Ctrl Pts',(-0.972814664000056,12.2,-4.35481961700001));
#325124=CARTESIAN_POINT('Ctrl Pts',(-0.972814664000056,5.2,-4.35481961700001));
#325125=CARTESIAN_POINT('Ctrl Pts',(-0.972814664000056,2.2,-4.35481961700001));
#325126=CARTESIAN_POINT('Ctrl Pts',(-0.971448767000057,12.2,-4.35313593500001));
#325127=CARTESIAN_POINT('Ctrl Pts',(-0.971448767000057,5.2,-4.35313593500001));
#325128=CARTESIAN_POINT('Ctrl Pts',(-0.971448767000057,2.2,-4.35313593500001));
#325129=CARTESIAN_POINT('Ctrl Pts',(-0.970087150000056,12.2,-4.35145378100001));
#325130=CARTESIAN_POINT('Ctrl Pts',(-0.970087150000056,5.2,-4.35145378100001));
#325131=CARTESIAN_POINT('Ctrl Pts',(-0.970087150000056,2.2,-4.35145378100001));
#325132=CARTESIAN_POINT('Ctrl Pts',(-0.968729812000056,12.2,-4.34977316700001));
#325133=CARTESIAN_POINT('Ctrl Pts',(-0.968729812000056,5.2,-4.34977316700001));
#325134=CARTESIAN_POINT('Ctrl Pts',(-0.968729812000056,2.2,-4.34977316700001));
#325135=CARTESIAN_POINT('Ctrl Pts',(-0.967376751000056,12.2,-4.34809410300002));
#325136=CARTESIAN_POINT('Ctrl Pts',(-0.967376751000056,5.2,-4.34809410300002));
#325137=CARTESIAN_POINT('Ctrl Pts',(-0.967376751000056,2.2,-4.34809410300002));
#325138=CARTESIAN_POINT('Ctrl Pts',(-0.966027967000055,12.2,-4.34641659700001));
#325139=CARTESIAN_POINT('Ctrl Pts',(-0.966027967000055,5.2,-4.34641659700001));
#325140=CARTESIAN_POINT('Ctrl Pts',(-0.966027967000055,2.2,-4.34641659700001));
#325141=CARTESIAN_POINT('Ctrl Pts',(-0.964683457000056,12.2,-4.34474066300002));
#325142=CARTESIAN_POINT('Ctrl Pts',(-0.964683457000056,5.2,-4.34474066300002));
#325143=CARTESIAN_POINT('Ctrl Pts',(-0.964683457000056,2.2,-4.34474066300002));
#325144=CARTESIAN_POINT('Ctrl Pts',(-0.963343219000056,12.2,-4.34306630800001));
#325145=CARTESIAN_POINT('Ctrl Pts',(-0.963343219000056,5.2,-4.34306630800001));
#325146=CARTESIAN_POINT('Ctrl Pts',(-0.963343219000056,2.2,-4.34306630800001));
#325147=CARTESIAN_POINT('Ctrl Pts',(-0.962007251000055,12.2,-4.34139354300001));
#325148=CARTESIAN_POINT('Ctrl Pts',(-0.962007251000055,5.2,-4.34139354300001));
#325149=CARTESIAN_POINT('Ctrl Pts',(-0.962007251000055,2.2,-4.34139354300001));
#325150=CARTESIAN_POINT('Ctrl Pts',(-0.960675554000057,12.2,-4.33972237800001));
#325151=CARTESIAN_POINT('Ctrl Pts',(-0.960675554000057,5.2,-4.33972237800001));
#325152=CARTESIAN_POINT('Ctrl Pts',(-0.960675554000057,2.2,-4.33972237800001));
#325153=CARTESIAN_POINT('Ctrl Pts',(-0.959348124000057,12.2,-4.33805282500002));
#325154=CARTESIAN_POINT('Ctrl Pts',(-0.959348124000057,5.2,-4.33805282500002));
#325155=CARTESIAN_POINT('Ctrl Pts',(-0.959348124000057,2.2,-4.33805282500002));
#325156=CARTESIAN_POINT('Ctrl Pts',(-0.958024960000056,12.2,-4.33638489200002));
#325157=CARTESIAN_POINT('Ctrl Pts',(-0.958024960000056,5.2,-4.33638489200002));
#325158=CARTESIAN_POINT('Ctrl Pts',(-0.958024960000056,2.2,-4.33638489200002));
#325159=CARTESIAN_POINT('Ctrl Pts',(-0.956706062000056,12.2,-4.33471859000001));
#325160=CARTESIAN_POINT('Ctrl Pts',(-0.956706062000056,5.2,-4.33471859000001));
#325161=CARTESIAN_POINT('Ctrl Pts',(-0.956706062000056,2.2,-4.33471859000001));
#325162=CARTESIAN_POINT('Ctrl Pts',(-0.955391425000055,12.2,-4.33305392900001));
#325163=CARTESIAN_POINT('Ctrl Pts',(-0.955391425000055,5.2,-4.33305392900001));
#325164=CARTESIAN_POINT('Ctrl Pts',(-0.955391425000055,2.2,-4.33305392900001));
#325165=CARTESIAN_POINT('Ctrl Pts',(-0.954081050000056,12.2,-4.33139092000001));
#325166=CARTESIAN_POINT('Ctrl Pts',(-0.954081050000056,5.2,-4.33139092000001));
#325167=CARTESIAN_POINT('Ctrl Pts',(-0.954081050000056,2.2,-4.33139092000001));
#325168=CARTESIAN_POINT('Ctrl Pts',(-0.952774934000056,12.2,-4.32972957100001));
#325169=CARTESIAN_POINT('Ctrl Pts',(-0.952774934000056,5.2,-4.32972957100001));
#325170=CARTESIAN_POINT('Ctrl Pts',(-0.952774934000056,2.2,-4.32972957100001));
#325171=CARTESIAN_POINT('Ctrl Pts',(-0.951473076000056,12.2,-4.32806989600001));
#325172=CARTESIAN_POINT('Ctrl Pts',(-0.951473076000056,5.2,-4.32806989600001));
#325173=CARTESIAN_POINT('Ctrl Pts',(-0.951473076000056,2.2,-4.32806989600001));
#325174=CARTESIAN_POINT('Ctrl Pts',(-0.950175474000057,12.2,-4.32641190200002));
#325175=CARTESIAN_POINT('Ctrl Pts',(-0.950175474000057,5.2,-4.32641190200002));
#325176=CARTESIAN_POINT('Ctrl Pts',(-0.950175474000057,2.2,-4.32641190200002));
#325177=CARTESIAN_POINT('Ctrl Pts',(-0.948882126000056,12.2,-4.32475560100002));
#325178=CARTESIAN_POINT('Ctrl Pts',(-0.948882126000056,5.2,-4.32475560100002));
#325179=CARTESIAN_POINT('Ctrl Pts',(-0.948882126000056,2.2,-4.32475560100002));
#325180=CARTESIAN_POINT('Ctrl Pts',(-0.947593031000055,12.2,-4.32310100300001));
#325181=CARTESIAN_POINT('Ctrl Pts',(-0.947593031000055,5.2,-4.32310100300001));
#325182=CARTESIAN_POINT('Ctrl Pts',(-0.947593031000055,2.2,-4.32310100300001));
#325183=CARTESIAN_POINT('Ctrl Pts',(-0.946308186000057,12.2,-4.32144811800002));
#325184=CARTESIAN_POINT('Ctrl Pts',(-0.946308186000057,5.2,-4.32144811800002));
#325185=CARTESIAN_POINT('Ctrl Pts',(-0.946308186000057,2.2,-4.32144811800002));
#325186=CARTESIAN_POINT('Ctrl Pts',(-0.945027590000055,12.2,-4.31979695700001));
#325187=CARTESIAN_POINT('Ctrl Pts',(-0.945027590000055,5.2,-4.31979695700001));
#325188=CARTESIAN_POINT('Ctrl Pts',(-0.945027590000055,2.2,-4.31979695700001));
#325189=CARTESIAN_POINT('Ctrl Pts',(-0.943751240000056,12.2,-4.31814752900001));
#325190=CARTESIAN_POINT('Ctrl Pts',(-0.943751240000056,5.2,-4.31814752900001));
#325191=CARTESIAN_POINT('Ctrl Pts',(-0.943751240000056,2.2,-4.31814752900001));
#325192=CARTESIAN_POINT('Ctrl Pts',(-0.942479137000056,12.2,-4.31649984600002));
#325193=CARTESIAN_POINT('Ctrl Pts',(-0.942479137000056,5.2,-4.31649984600002));
#325194=CARTESIAN_POINT('Ctrl Pts',(-0.942479137000056,2.2,-4.31649984600002));
#325195=CARTESIAN_POINT('Ctrl Pts',(-0.941211276000056,12.2,-4.31485391700001));
#325196=CARTESIAN_POINT('Ctrl Pts',(-0.941211276000056,5.2,-4.31485391700001));
#325197=CARTESIAN_POINT('Ctrl Pts',(-0.941211276000056,2.2,-4.31485391700001));
#325198=CARTESIAN_POINT('Ctrl Pts',(-0.939947657000056,12.2,-4.31320975300002));
#325199=CARTESIAN_POINT('Ctrl Pts',(-0.939947657000056,5.2,-4.31320975300002));
#325200=CARTESIAN_POINT('Ctrl Pts',(-0.939947657000056,2.2,-4.31320975300002));
#325201=CARTESIAN_POINT('Ctrl Pts',(-0.938688278000056,12.2,-4.31156736500002));
#325202=CARTESIAN_POINT('Ctrl Pts',(-0.938688278000056,5.2,-4.31156736500002));
#325203=CARTESIAN_POINT('Ctrl Pts',(-0.938688278000056,2.2,-4.31156736500002));
#325204=CARTESIAN_POINT('Ctrl Pts',(-0.937433136000055,12.2,-4.30992676300002));
#325205=CARTESIAN_POINT('Ctrl Pts',(-0.937433136000055,5.2,-4.30992676300002));
#325206=CARTESIAN_POINT('Ctrl Pts',(-0.937433136000055,2.2,-4.30992676300002));
#325207=CARTESIAN_POINT('Ctrl Pts',(-0.936182229000057,12.2,-4.30828795600001));
#325208=CARTESIAN_POINT('Ctrl Pts',(-0.936182229000057,5.2,-4.30828795600001));
#325209=CARTESIAN_POINT('Ctrl Pts',(-0.936182229000057,2.2,-4.30828795600001));
#325210=CARTESIAN_POINT('Ctrl Pts',(-0.934935557000056,12.2,-4.30665095700002));
#325211=CARTESIAN_POINT('Ctrl Pts',(-0.934935557000056,5.2,-4.30665095700002));
#325212=CARTESIAN_POINT('Ctrl Pts',(-0.934935557000056,2.2,-4.30665095700002));
#325213=CARTESIAN_POINT('Ctrl Pts',(-0.933693116000055,12.2,-4.30501577500001));
#325214=CARTESIAN_POINT('Ctrl Pts',(-0.933693116000055,5.2,-4.30501577500001));
#325215=CARTESIAN_POINT('Ctrl Pts',(-0.933693116000055,2.2,-4.30501577500001));
#325216=CARTESIAN_POINT('Ctrl Pts',(-0.932454904000056,12.2,-4.30338242000001));
#325217=CARTESIAN_POINT('Ctrl Pts',(-0.932454904000056,5.2,-4.30338242000001));
#325218=CARTESIAN_POINT('Ctrl Pts',(-0.932454904000056,2.2,-4.30338242000001));
#325219=CARTESIAN_POINT('Ctrl Pts',(-0.931220922000057,12.2,-4.30175090400001));
#325220=CARTESIAN_POINT('Ctrl Pts',(-0.931220922000057,5.2,-4.30175090400001));
#325221=CARTESIAN_POINT('Ctrl Pts',(-0.931220922000057,2.2,-4.30175090400001));
#325222=CARTESIAN_POINT('Ctrl Pts',(-0.929991165000056,12.2,-4.30012123500001));
#325223=CARTESIAN_POINT('Ctrl Pts',(-0.929991165000056,5.2,-4.30012123500001));
#325224=CARTESIAN_POINT('Ctrl Pts',(-0.929991165000056,2.2,-4.30012123500001));
#325225=CARTESIAN_POINT('Ctrl Pts',(-0.928765631000056,12.2,-4.29849342700001));
#325226=CARTESIAN_POINT('Ctrl Pts',(-0.928765631000056,5.2,-4.29849342700001));
#325227=CARTESIAN_POINT('Ctrl Pts',(-0.928765631000056,2.2,-4.29849342700001));
#325228=CARTESIAN_POINT('Ctrl Pts',(-0.927544319000055,12.2,-4.29686748800002));
#325229=CARTESIAN_POINT('Ctrl Pts',(-0.927544319000055,5.2,-4.29686748800002));
#325230=CARTESIAN_POINT('Ctrl Pts',(-0.927544319000055,2.2,-4.29686748800002));
#325231=CARTESIAN_POINT('Ctrl Pts',(-0.926327227000057,12.2,-4.29524342900002));
#325232=CARTESIAN_POINT('Ctrl Pts',(-0.926327227000057,5.2,-4.29524342900002));
#325233=CARTESIAN_POINT('Ctrl Pts',(-0.926327227000057,2.2,-4.29524342900002));
#325234=CARTESIAN_POINT('Ctrl Pts',(-0.925114352000056,12.2,-4.29362126000001));
#325235=CARTESIAN_POINT('Ctrl Pts',(-0.925114352000056,5.2,-4.29362126000001));
#325236=CARTESIAN_POINT('Ctrl Pts',(-0.925114352000056,2.2,-4.29362126000001));
#325237=CARTESIAN_POINT('Ctrl Pts',(-0.923905693000057,12.2,-4.29200099300001));
#325238=CARTESIAN_POINT('Ctrl Pts',(-0.923905693000057,5.2,-4.29200099300001));
#325239=CARTESIAN_POINT('Ctrl Pts',(-0.923905693000057,2.2,-4.29200099300001));
#325240=CARTESIAN_POINT('Ctrl Pts',(-0.922701248000056,12.2,-4.29038263800001));
#325241=CARTESIAN_POINT('Ctrl Pts',(-0.922701248000056,5.2,-4.29038263800001));
#325242=CARTESIAN_POINT('Ctrl Pts',(-0.922701248000056,2.2,-4.29038263800001));
#325243=CARTESIAN_POINT('Ctrl Pts',(-0.921501014000056,12.2,-4.28876620600001));
#325244=CARTESIAN_POINT('Ctrl Pts',(-0.921501014000056,5.2,-4.28876620600001));
#325245=CARTESIAN_POINT('Ctrl Pts',(-0.921501014000056,2.2,-4.28876620600001));
#325246=CARTESIAN_POINT('Ctrl Pts',(-0.920304988000057,12.2,-4.28715170600002));
#325247=CARTESIAN_POINT('Ctrl Pts',(-0.920304988000057,5.2,-4.28715170600002));
#325248=CARTESIAN_POINT('Ctrl Pts',(-0.920304988000057,2.2,-4.28715170600002));
#325249=CARTESIAN_POINT('Ctrl Pts',(-0.919113169000055,12.2,-4.28553915100002));
#325250=CARTESIAN_POINT('Ctrl Pts',(-0.919113169000055,5.2,-4.28553915100002));
#325251=CARTESIAN_POINT('Ctrl Pts',(-0.919113169000055,2.2,-4.28553915100002));
#325252=CARTESIAN_POINT('Ctrl Pts',(-0.917925555000056,12.2,-4.28392854900002));
#325253=CARTESIAN_POINT('Ctrl Pts',(-0.917925555000056,5.2,-4.28392854900002));
#325254=CARTESIAN_POINT('Ctrl Pts',(-0.917925555000056,2.2,-4.28392854900002));
#325255=CARTESIAN_POINT('Ctrl Pts',(-0.916742144000056,12.2,-4.28231991300001));
#325256=CARTESIAN_POINT('Ctrl Pts',(-0.916742144000056,5.2,-4.28231991300001));
#325257=CARTESIAN_POINT('Ctrl Pts',(-0.916742144000056,2.2,-4.28231991300001));
#325258=CARTESIAN_POINT('Ctrl Pts',(-0.915562933000055,12.2,-4.28071325300001));
#325259=CARTESIAN_POINT('Ctrl Pts',(-0.915562933000055,5.2,-4.28071325300001));
#325260=CARTESIAN_POINT('Ctrl Pts',(-0.915562933000055,2.2,-4.28071325300001));
#325261=CARTESIAN_POINT('Ctrl Pts',(-0.914387920000056,12.2,-4.27910857900001));
#325262=CARTESIAN_POINT('Ctrl Pts',(-0.914387920000056,5.2,-4.27910857900001));
#325263=CARTESIAN_POINT('Ctrl Pts',(-0.914387920000056,2.2,-4.27910857900001));
#325264=CARTESIAN_POINT('Ctrl Pts',(-0.913217103000056,12.2,-4.27750590100001));
#325265=CARTESIAN_POINT('Ctrl Pts',(-0.913217103000056,5.2,-4.27750590100001));
#325266=CARTESIAN_POINT('Ctrl Pts',(-0.913217103000056,2.2,-4.27750590100001));
#325267=CARTESIAN_POINT('Ctrl Pts',(-0.912050479000056,12.2,-4.27590523100001));
#325268=CARTESIAN_POINT('Ctrl Pts',(-0.912050479000056,5.2,-4.27590523100001));
#325269=CARTESIAN_POINT('Ctrl Pts',(-0.912050479000056,2.2,-4.27590523100001));
#325270=CARTESIAN_POINT('Ctrl Pts',(-0.910888047000055,12.2,-4.27430658100001));
#325271=CARTESIAN_POINT('Ctrl Pts',(-0.910888047000055,5.2,-4.27430658100001));
#325272=CARTESIAN_POINT('Ctrl Pts',(-0.910888047000055,2.2,-4.27430658100001));
#325273=CARTESIAN_POINT('Ctrl Pts',(-0.909729802000055,12.2,-4.27270995800002));
#325274=CARTESIAN_POINT('Ctrl Pts',(-0.909729802000055,5.2,-4.27270995800002));
#325275=CARTESIAN_POINT('Ctrl Pts',(-0.909729802000055,2.2,-4.27270995800002));
#325276=CARTESIAN_POINT('Ctrl Pts',(-0.908575745000055,12.2,-4.27111537700001));
#325277=CARTESIAN_POINT('Ctrl Pts',(-0.908575745000055,5.2,-4.27111537700001));
#325278=CARTESIAN_POINT('Ctrl Pts',(-0.908575745000055,2.2,-4.27111537700001));
#325279=CARTESIAN_POINT('Ctrl Pts',(-0.907425872000056,12.2,-4.26952284600001));
#325280=CARTESIAN_POINT('Ctrl Pts',(-0.907425872000056,5.2,-4.26952284600001));
#325281=CARTESIAN_POINT('Ctrl Pts',(-0.907425872000056,2.2,-4.26952284600001));
#325282=CARTESIAN_POINT('Ctrl Pts',(-0.906280181000056,12.2,-4.26793237600001));
#325283=CARTESIAN_POINT('Ctrl Pts',(-0.906280181000056,5.2,-4.26793237600001));
#325284=CARTESIAN_POINT('Ctrl Pts',(-0.906280181000056,2.2,-4.26793237600001));
#325285=CARTESIAN_POINT('Ctrl Pts',(-0.905138668000056,12.2,-4.26634397900001));
#325286=CARTESIAN_POINT('Ctrl Pts',(-0.905138668000056,5.2,-4.26634397900001));
#325287=CARTESIAN_POINT('Ctrl Pts',(-0.905138668000056,2.2,-4.26634397900001));
#325288=CARTESIAN_POINT('Ctrl Pts',(-0.904001333000056,12.2,-4.26475766500001));
#325289=CARTESIAN_POINT('Ctrl Pts',(-0.904001333000056,5.2,-4.26475766500001));
#325290=CARTESIAN_POINT('Ctrl Pts',(-0.904001333000056,2.2,-4.26475766500001));
#325291=CARTESIAN_POINT('Ctrl Pts',(-0.902868173000057,12.2,-4.26317344500001));
#325292=CARTESIAN_POINT('Ctrl Pts',(-0.902868173000057,5.2,-4.26317344500001));
#325293=CARTESIAN_POINT('Ctrl Pts',(-0.902868173000057,2.2,-4.26317344500001));
#325294=CARTESIAN_POINT('Ctrl Pts',(-0.901739184000055,12.2,-4.26159132900001));
#325295=CARTESIAN_POINT('Ctrl Pts',(-0.901739184000055,5.2,-4.26159132900001));
#325296=CARTESIAN_POINT('Ctrl Pts',(-0.901739184000055,2.2,-4.26159132900001));
#325297=CARTESIAN_POINT('Ctrl Pts',(-0.900614366000055,12.2,-4.26001133000002));
#325298=CARTESIAN_POINT('Ctrl Pts',(-0.900614366000055,5.2,-4.26001133000002));
#325299=CARTESIAN_POINT('Ctrl Pts',(-0.900614366000055,2.2,-4.26001133000002));
#325300=CARTESIAN_POINT('Ctrl Pts',(-0.899493714000055,12.2,-4.25843345600001));
#325301=CARTESIAN_POINT('Ctrl Pts',(-0.899493714000055,5.2,-4.25843345600001));
#325302=CARTESIAN_POINT('Ctrl Pts',(-0.899493714000055,2.2,-4.25843345600001));
#325303=CARTESIAN_POINT('Ctrl Pts',(-0.898377227000056,12.2,-4.25685771900001));
#325304=CARTESIAN_POINT('Ctrl Pts',(-0.898377227000056,5.2,-4.25685771900001));
#325305=CARTESIAN_POINT('Ctrl Pts',(-0.898377227000056,2.2,-4.25685771900001));
#325306=CARTESIAN_POINT('Ctrl Pts',(-0.897264902000057,12.2,-4.25528413200002));
#325307=CARTESIAN_POINT('Ctrl Pts',(-0.897264902000057,5.2,-4.25528413200002));
#325308=CARTESIAN_POINT('Ctrl Pts',(-0.897264902000057,2.2,-4.25528413200002));
#325309=CARTESIAN_POINT('Ctrl Pts',(-0.896156737000057,12.2,-4.25371270300001));
#325310=CARTESIAN_POINT('Ctrl Pts',(-0.896156737000057,5.2,-4.25371270300001));
#325311=CARTESIAN_POINT('Ctrl Pts',(-0.896156737000057,2.2,-4.25371270300001));
#325312=CARTESIAN_POINT('Ctrl Pts',(-0.895052728000056,12.2,-4.25214344400001));
#325313=CARTESIAN_POINT('Ctrl Pts',(-0.895052728000056,5.2,-4.25214344400001));
#325314=CARTESIAN_POINT('Ctrl Pts',(-0.895052728000056,2.2,-4.25214344400001));
#325315=CARTESIAN_POINT('Ctrl Pts',(-0.893952874000057,12.2,-4.25057636600001));
#325316=CARTESIAN_POINT('Ctrl Pts',(-0.893952874000057,5.2,-4.25057636600001));
#325317=CARTESIAN_POINT('Ctrl Pts',(-0.893952874000057,2.2,-4.25057636600001));
#325318=CARTESIAN_POINT('Ctrl Pts',(-0.892857172000056,12.2,-4.24901148100002));
#325319=CARTESIAN_POINT('Ctrl Pts',(-0.892857172000056,5.2,-4.24901148100002));
#325320=CARTESIAN_POINT('Ctrl Pts',(-0.892857172000056,2.2,-4.24901148100002));
#325321=CARTESIAN_POINT('Ctrl Pts',(-0.891765620000056,12.2,-4.24744879800001));
#325322=CARTESIAN_POINT('Ctrl Pts',(-0.891765620000056,5.2,-4.24744879800001));
#325323=CARTESIAN_POINT('Ctrl Pts',(-0.891765620000056,2.2,-4.24744879800001));
#325324=CARTESIAN_POINT('Ctrl Pts',(-0.890678213000056,12.2,-4.24588832900001));
#325325=CARTESIAN_POINT('Ctrl Pts',(-0.890678213000056,5.2,-4.24588832900001));
#325326=CARTESIAN_POINT('Ctrl Pts',(-0.890678213000056,2.2,-4.24588832900001));
#325327=CARTESIAN_POINT('Ctrl Pts',(-0.889594950000056,12.2,-4.24433008500001));
#325328=CARTESIAN_POINT('Ctrl Pts',(-0.889594950000056,5.2,-4.24433008500001));
#325329=CARTESIAN_POINT('Ctrl Pts',(-0.889594950000056,2.2,-4.24433008500001));
#325330=CARTESIAN_POINT('Ctrl Pts',(-0.888515829000056,12.2,-4.24277407700002));
#325331=CARTESIAN_POINT('Ctrl Pts',(-0.888515829000056,5.2,-4.24277407700002));
#325332=CARTESIAN_POINT('Ctrl Pts',(-0.888515829000056,2.2,-4.24277407700002));
#325333=CARTESIAN_POINT('Ctrl Pts',(-0.887440846000055,12.2,-4.24122031600001));
#325334=CARTESIAN_POINT('Ctrl Pts',(-0.887440846000055,5.2,-4.24122031600001));
#325335=CARTESIAN_POINT('Ctrl Pts',(-0.887440846000055,2.2,-4.24122031600001));
#325336=CARTESIAN_POINT('Ctrl Pts',(-0.886370000000056,12.2,-4.23966881300001));
#325337=CARTESIAN_POINT('Ctrl Pts',(-0.886370000000056,5.2,-4.23966881300001));
#325338=CARTESIAN_POINT('Ctrl Pts',(-0.886370000000056,2.2,-4.23966881300001));
#325339=CARTESIAN_POINT('Ctrl Pts',(-0.885303286000055,12.2,-4.23811957800002));
#325340=CARTESIAN_POINT('Ctrl Pts',(-0.885303286000055,5.2,-4.23811957800002));
#325341=CARTESIAN_POINT('Ctrl Pts',(-0.885303286000055,2.2,-4.23811957800002));
#325342=CARTESIAN_POINT('Ctrl Pts',(-0.884240702000056,12.2,-4.23657262400001));
#325343=CARTESIAN_POINT('Ctrl Pts',(-0.884240702000056,5.2,-4.23657262400001));
#325344=CARTESIAN_POINT('Ctrl Pts',(-0.884240702000056,2.2,-4.23657262400001));
#325345=CARTESIAN_POINT('Ctrl Pts',(-0.883182246000055,12.2,-4.23502796100002));
#325346=CARTESIAN_POINT('Ctrl Pts',(-0.883182246000055,5.2,-4.23502796100002));
#325347=CARTESIAN_POINT('Ctrl Pts',(-0.883182246000055,2.2,-4.23502796100002));
#325348=CARTESIAN_POINT('Ctrl Pts',(-0.882127915000056,12.2,-4.23348560000001));
#325349=CARTESIAN_POINT('Ctrl Pts',(-0.882127915000056,5.2,-4.23348560000001));
#325350=CARTESIAN_POINT('Ctrl Pts',(-0.882127915000056,2.2,-4.23348560000001));
#325351=CARTESIAN_POINT('Ctrl Pts',(-0.881077706000056,12.2,-4.23194555300002));
#325352=CARTESIAN_POINT('Ctrl Pts',(-0.881077706000056,5.2,-4.23194555300002));
#325353=CARTESIAN_POINT('Ctrl Pts',(-0.881077706000056,2.2,-4.23194555300002));
#325354=CARTESIAN_POINT('Ctrl Pts',(-0.880031616000055,12.2,-4.23040783000001));
#325355=CARTESIAN_POINT('Ctrl Pts',(-0.880031616000055,5.2,-4.23040783000001));
#325356=CARTESIAN_POINT('Ctrl Pts',(-0.880031616000055,2.2,-4.23040783000001));
#325357=CARTESIAN_POINT('Ctrl Pts',(-0.878989642000055,12.2,-4.22887244300002));
#325358=CARTESIAN_POINT('Ctrl Pts',(-0.878989642000055,5.2,-4.22887244300002));
#325359=CARTESIAN_POINT('Ctrl Pts',(-0.878989642000055,2.2,-4.22887244300002));
#325360=CARTESIAN_POINT('Ctrl Pts',(-0.877951781000055,12.2,-4.22733940200001));
#325361=CARTESIAN_POINT('Ctrl Pts',(-0.877951781000055,5.2,-4.22733940200001));
#325362=CARTESIAN_POINT('Ctrl Pts',(-0.877951781000055,2.2,-4.22733940200001));
#325363=CARTESIAN_POINT('Ctrl Pts',(-0.876918030000056,12.2,-4.22580872000001));
#325364=CARTESIAN_POINT('Ctrl Pts',(-0.876918030000056,5.2,-4.22580872000001));
#325365=CARTESIAN_POINT('Ctrl Pts',(-0.876918030000056,2.2,-4.22580872000001));
#325366=CARTESIAN_POINT('Ctrl Pts',(-0.875888388000057,12.2,-4.22428040700002));
#325367=CARTESIAN_POINT('Ctrl Pts',(-0.875888388000057,5.2,-4.22428040700002));
#325368=CARTESIAN_POINT('Ctrl Pts',(-0.875888388000057,2.2,-4.22428040700002));
#325369=CARTESIAN_POINT('Ctrl Pts',(-0.874862850000057,12.2,-4.22275447400001));
#325370=CARTESIAN_POINT('Ctrl Pts',(-0.874862850000057,5.2,-4.22275447400001));
#325371=CARTESIAN_POINT('Ctrl Pts',(-0.874862850000057,2.2,-4.22275447400001));
#325372=CARTESIAN_POINT('Ctrl Pts',(-0.873841413000056,12.2,-4.22123093200002));
#325373=CARTESIAN_POINT('Ctrl Pts',(-0.873841413000056,5.2,-4.22123093200002));
#325374=CARTESIAN_POINT('Ctrl Pts',(-0.873841413000056,2.2,-4.22123093200002));
#325375=CARTESIAN_POINT('Ctrl Pts',(-0.872824076000055,12.2,-4.21970979500002));
#325376=CARTESIAN_POINT('Ctrl Pts',(-0.872824076000055,5.2,-4.21970979500002));
#325377=CARTESIAN_POINT('Ctrl Pts',(-0.872824076000055,2.2,-4.21970979500002));
#325378=CARTESIAN_POINT('Ctrl Pts',(-0.871810833000056,12.2,-4.21819107000001));
#325379=CARTESIAN_POINT('Ctrl Pts',(-0.871810833000056,5.2,-4.21819107000001));
#325380=CARTESIAN_POINT('Ctrl Pts',(-0.871810833000056,2.2,-4.21819107000001));
#325381=CARTESIAN_POINT('Ctrl Pts',(-0.870801684000057,12.2,-4.21667477100002));
#325382=CARTESIAN_POINT('Ctrl Pts',(-0.870801684000057,5.2,-4.21667477100002));
#325383=CARTESIAN_POINT('Ctrl Pts',(-0.870801684000057,2.2,-4.21667477100002));
#325384=CARTESIAN_POINT('Ctrl Pts',(-0.869796624000055,12.2,-4.21516090900001));
#325385=CARTESIAN_POINT('Ctrl Pts',(-0.869796624000055,5.2,-4.21516090900001));
#325386=CARTESIAN_POINT('Ctrl Pts',(-0.869796624000055,2.2,-4.21516090900001));
#325387=CARTESIAN_POINT('Ctrl Pts',(-0.868795651000056,12.2,-4.21364949400001));
#325388=CARTESIAN_POINT('Ctrl Pts',(-0.868795651000056,5.2,-4.21364949400001));
#325389=CARTESIAN_POINT('Ctrl Pts',(-0.868795651000056,2.2,-4.21364949400001));
#325390=CARTESIAN_POINT('Ctrl Pts',(-0.867798761000056,12.2,-4.21214053900002));
#325391=CARTESIAN_POINT('Ctrl Pts',(-0.867798761000056,5.2,-4.21214053900002));
#325392=CARTESIAN_POINT('Ctrl Pts',(-0.867798761000056,2.2,-4.21214053900002));
#325393=CARTESIAN_POINT('Ctrl Pts',(-0.866805951000057,12.2,-4.21063405500002));
#325394=CARTESIAN_POINT('Ctrl Pts',(-0.866805951000057,5.2,-4.21063405500002));
#325395=CARTESIAN_POINT('Ctrl Pts',(-0.866805951000057,2.2,-4.21063405500002));
#325396=CARTESIAN_POINT('Ctrl Pts',(-0.865817219000055,12.2,-4.20913005200001));
#325397=CARTESIAN_POINT('Ctrl Pts',(-0.865817219000055,5.2,-4.20913005200001));
#325398=CARTESIAN_POINT('Ctrl Pts',(-0.865817219000055,2.2,-4.20913005200001));
#325399=CARTESIAN_POINT('Ctrl Pts',(-0.864832560000056,12.2,-4.20762854200001));
#325400=CARTESIAN_POINT('Ctrl Pts',(-0.864832560000056,5.2,-4.20762854200001));
#325401=CARTESIAN_POINT('Ctrl Pts',(-0.864832560000056,2.2,-4.20762854200001));
#325402=CARTESIAN_POINT('Ctrl Pts',(-0.863851973000056,12.2,-4.20612953700001));
#325403=CARTESIAN_POINT('Ctrl Pts',(-0.863851973000056,5.2,-4.20612953700001));
#325404=CARTESIAN_POINT('Ctrl Pts',(-0.863851973000056,2.2,-4.20612953700001));
#325405=CARTESIAN_POINT('Ctrl Pts',(-0.862875453000056,12.2,-4.20463304800001));
#325406=CARTESIAN_POINT('Ctrl Pts',(-0.862875453000056,5.2,-4.20463304800001));
#325407=CARTESIAN_POINT('Ctrl Pts',(-0.862875453000056,2.2,-4.20463304800001));
#325408=CARTESIAN_POINT('Ctrl Pts',(-0.861902999000056,12.2,-4.20313908800001));
#325409=CARTESIAN_POINT('Ctrl Pts',(-0.861902999000056,5.2,-4.20313908800001));
#325410=CARTESIAN_POINT('Ctrl Pts',(-0.861902999000056,2.2,-4.20313908800001));
#325411=CARTESIAN_POINT('Ctrl Pts',(-0.860934605000055,12.2,-4.20164766600001));
#325412=CARTESIAN_POINT('Ctrl Pts',(-0.860934605000055,5.2,-4.20164766600001));
#325413=CARTESIAN_POINT('Ctrl Pts',(-0.860934605000055,2.2,-4.20164766600001));
#325414=CARTESIAN_POINT('Ctrl Pts',(-0.859970269000057,12.2,-4.20015879300002));
#325415=CARTESIAN_POINT('Ctrl Pts',(-0.859970269000057,5.2,-4.20015879300002));
#325416=CARTESIAN_POINT('Ctrl Pts',(-0.859970269000057,2.2,-4.20015879300002));
#325417=CARTESIAN_POINT('Ctrl Pts',(-0.859009988000056,12.2,-4.19867248200001));
#325418=CARTESIAN_POINT('Ctrl Pts',(-0.859009988000056,5.2,-4.19867248200001));
#325419=CARTESIAN_POINT('Ctrl Pts',(-0.859009988000056,2.2,-4.19867248200001));
#325420=CARTESIAN_POINT('Ctrl Pts',(-0.858053759000056,12.2,-4.19718874600001));
#325421=CARTESIAN_POINT('Ctrl Pts',(-0.858053759000056,5.2,-4.19718874600001));
#325422=CARTESIAN_POINT('Ctrl Pts',(-0.858053759000056,2.2,-4.19718874600001));
#325423=CARTESIAN_POINT('Ctrl Pts',(-0.857101578000057,12.2,-4.19570759300001));
#325424=CARTESIAN_POINT('Ctrl Pts',(-0.857101578000057,5.2,-4.19570759300001));
#325425=CARTESIAN_POINT('Ctrl Pts',(-0.857101578000057,2.2,-4.19570759300001));
#325426=CARTESIAN_POINT('Ctrl Pts',(-0.856153441000057,12.2,-4.19422903700001));
#325427=CARTESIAN_POINT('Ctrl Pts',(-0.856153441000057,5.2,-4.19422903700001));
#325428=CARTESIAN_POINT('Ctrl Pts',(-0.856153441000057,2.2,-4.19422903700001));
#325429=CARTESIAN_POINT('Ctrl Pts',(-0.855209346000055,12.2,-4.19275308800001));
#325430=CARTESIAN_POINT('Ctrl Pts',(-0.855209346000055,5.2,-4.19275308800001));
#325431=CARTESIAN_POINT('Ctrl Pts',(-0.855209346000055,2.2,-4.19275308800001));
#325432=CARTESIAN_POINT('Ctrl Pts',(-0.854269289000056,12.2,-4.19127975900001));
#325433=CARTESIAN_POINT('Ctrl Pts',(-0.854269289000056,5.2,-4.19127975900001));
#325434=CARTESIAN_POINT('Ctrl Pts',(-0.854269289000056,2.2,-4.19127975900001));
#325435=CARTESIAN_POINT('Ctrl Pts',(-0.853333268000057,12.2,-4.18980906100002));
#325436=CARTESIAN_POINT('Ctrl Pts',(-0.853333268000057,5.2,-4.18980906100002));
#325437=CARTESIAN_POINT('Ctrl Pts',(-0.853333268000057,2.2,-4.18980906100002));
#325438=CARTESIAN_POINT('Ctrl Pts',(-0.852401276000055,12.2,-4.18834100500002));
#325439=CARTESIAN_POINT('Ctrl Pts',(-0.852401276000055,5.2,-4.18834100500002));
#325440=CARTESIAN_POINT('Ctrl Pts',(-0.852401276000055,2.2,-4.18834100500002));
#325441=CARTESIAN_POINT('Ctrl Pts',(-0.851473313000056,12.2,-4.18687560300001));
#325442=CARTESIAN_POINT('Ctrl Pts',(-0.851473313000056,5.2,-4.18687560300001));
#325443=CARTESIAN_POINT('Ctrl Pts',(-0.851473313000056,2.2,-4.18687560300001));
#325444=CARTESIAN_POINT('Ctrl Pts',(-0.850549375000057,12.2,-4.18541286700002));
#325445=CARTESIAN_POINT('Ctrl Pts',(-0.850549375000057,5.2,-4.18541286700002));
#325446=CARTESIAN_POINT('Ctrl Pts',(-0.850549375000057,2.2,-4.18541286700002));
#325447=CARTESIAN_POINT('Ctrl Pts',(-0.849629457000055,12.2,-4.18395280800001));
#325448=CARTESIAN_POINT('Ctrl Pts',(-0.849629457000055,5.2,-4.18395280800001));
#325449=CARTESIAN_POINT('Ctrl Pts',(-0.849629457000055,2.2,-4.18395280800001));
#325450=CARTESIAN_POINT('Ctrl Pts',(-0.848713556000057,12.2,-4.18249543700002));
#325451=CARTESIAN_POINT('Ctrl Pts',(-0.848713556000057,5.2,-4.18249543700002));
#325452=CARTESIAN_POINT('Ctrl Pts',(-0.848713556000057,2.2,-4.18249543700002));
#325453=CARTESIAN_POINT('Ctrl Pts',(-0.847801670000056,12.2,-4.18104076700001));
#325454=CARTESIAN_POINT('Ctrl Pts',(-0.847801670000056,5.2,-4.18104076700001));
#325455=CARTESIAN_POINT('Ctrl Pts',(-0.847801670000056,2.2,-4.18104076700001));
#325456=CARTESIAN_POINT('Ctrl Pts',(-0.846893794000056,12.2,-4.17958880900001));
#325457=CARTESIAN_POINT('Ctrl Pts',(-0.846893794000056,5.2,-4.17958880900001));
#325458=CARTESIAN_POINT('Ctrl Pts',(-0.846893794000056,2.2,-4.17958880900001));
#325459=CARTESIAN_POINT('Ctrl Pts',(-0.845989925000056,12.2,-4.17813957500002));
#325460=CARTESIAN_POINT('Ctrl Pts',(-0.845989925000056,5.2,-4.17813957500002));
#325461=CARTESIAN_POINT('Ctrl Pts',(-0.845989925000056,2.2,-4.17813957500002));
#325462=CARTESIAN_POINT('Ctrl Pts',(-0.845090058000055,12.2,-4.17669307700002));
#325463=CARTESIAN_POINT('Ctrl Pts',(-0.845090058000055,5.2,-4.17669307700002));
#325464=CARTESIAN_POINT('Ctrl Pts',(-0.845090058000055,2.2,-4.17669307700002));
#325465=CARTESIAN_POINT('Ctrl Pts',(-0.844194192000056,12.2,-4.17524932500001));
#325466=CARTESIAN_POINT('Ctrl Pts',(-0.844194192000056,5.2,-4.17524932500001));
#325467=CARTESIAN_POINT('Ctrl Pts',(-0.844194192000056,2.2,-4.17524932500001));
#325468=CARTESIAN_POINT('Ctrl Pts',(-0.843302321000056,12.2,-4.17380833300002));
#325469=CARTESIAN_POINT('Ctrl Pts',(-0.843302321000056,5.2,-4.17380833300002));
#325470=CARTESIAN_POINT('Ctrl Pts',(-0.843302321000056,2.2,-4.17380833300002));
#325471=CARTESIAN_POINT('Ctrl Pts',(-0.842414442000056,12.2,-4.17237011100001));
#325472=CARTESIAN_POINT('Ctrl Pts',(-0.842414442000056,5.2,-4.17237011100001));
#325473=CARTESIAN_POINT('Ctrl Pts',(-0.842414442000056,2.2,-4.17237011100001));
#325474=CARTESIAN_POINT('Ctrl Pts',(-0.841530551000057,12.2,-4.17093467200001));
#325475=CARTESIAN_POINT('Ctrl Pts',(-0.841530551000057,5.2,-4.17093467200001));
#325476=CARTESIAN_POINT('Ctrl Pts',(-0.841530551000057,2.2,-4.17093467200001));
#325477=CARTESIAN_POINT('Ctrl Pts',(-0.840650646000055,12.2,-4.16950202700002));
#325478=CARTESIAN_POINT('Ctrl Pts',(-0.840650646000055,5.2,-4.16950202700002));
#325479=CARTESIAN_POINT('Ctrl Pts',(-0.840650646000055,2.2,-4.16950202700002));
#325480=CARTESIAN_POINT('Ctrl Pts',(-0.839774721000056,12.2,-4.16807218800002));
#325481=CARTESIAN_POINT('Ctrl Pts',(-0.839774721000056,5.2,-4.16807218800002));
#325482=CARTESIAN_POINT('Ctrl Pts',(-0.839774721000056,2.2,-4.16807218800002));
#325483=CARTESIAN_POINT('Ctrl Pts',(-0.838902774000055,12.2,-4.16664516700001));
#325484=CARTESIAN_POINT('Ctrl Pts',(-0.838902774000055,5.2,-4.16664516700001));
#325485=CARTESIAN_POINT('Ctrl Pts',(-0.838902774000055,2.2,-4.16664516700001));
#325486=CARTESIAN_POINT('Ctrl Pts',(-0.838034801000056,12.2,-4.16522097500001));
#325487=CARTESIAN_POINT('Ctrl Pts',(-0.838034801000056,5.2,-4.16522097500001));
#325488=CARTESIAN_POINT('Ctrl Pts',(-0.838034801000056,2.2,-4.16522097500001));
#325489=CARTESIAN_POINT('Ctrl Pts',(-0.837170796000055,12.2,-4.16379962500002));
#325490=CARTESIAN_POINT('Ctrl Pts',(-0.837170796000055,5.2,-4.16379962500002));
#325491=CARTESIAN_POINT('Ctrl Pts',(-0.837170796000055,2.2,-4.16379962500002));
#325492=CARTESIAN_POINT('Ctrl Pts',(-0.836310758000056,12.2,-4.16238112900002));
#325493=CARTESIAN_POINT('Ctrl Pts',(-0.836310758000056,5.2,-4.16238112900002));
#325494=CARTESIAN_POINT('Ctrl Pts',(-0.836310758000056,2.2,-4.16238112900002));
#325495=CARTESIAN_POINT('Ctrl Pts',(-0.835454681000056,12.2,-4.16096549800002));
#325496=CARTESIAN_POINT('Ctrl Pts',(-0.835454681000056,5.2,-4.16096549800002));
#325497=CARTESIAN_POINT('Ctrl Pts',(-0.835454681000056,2.2,-4.16096549800002));
#325498=CARTESIAN_POINT('Ctrl Pts',(-0.834602564000055,12.2,-4.15955274300002));
#325499=CARTESIAN_POINT('Ctrl Pts',(-0.834602564000055,5.2,-4.15955274300002));
#325500=CARTESIAN_POINT('Ctrl Pts',(-0.834602564000055,2.2,-4.15955274300002));
#325501=CARTESIAN_POINT('Ctrl Pts',(-0.833754401000055,12.2,-4.15814287900002));
#325502=CARTESIAN_POINT('Ctrl Pts',(-0.833754401000055,5.2,-4.15814287900002));
#325503=CARTESIAN_POINT('Ctrl Pts',(-0.833754401000055,2.2,-4.15814287900002));
#325504=CARTESIAN_POINT('Ctrl Pts',(-0.832910187000057,12.2,-4.15673591400001));
#325505=CARTESIAN_POINT('Ctrl Pts',(-0.832910187000057,5.2,-4.15673591400001));
#325506=CARTESIAN_POINT('Ctrl Pts',(-0.832910187000057,2.2,-4.15673591400001));
#325507=CARTESIAN_POINT('Ctrl Pts',(-0.832069920000055,12.2,-4.15533186300001));
#325508=CARTESIAN_POINT('Ctrl Pts',(-0.832069920000055,5.2,-4.15533186300001));
#325509=CARTESIAN_POINT('Ctrl Pts',(-0.832069920000055,2.2,-4.15533186300001));
#325510=CARTESIAN_POINT('Ctrl Pts',(-0.831233596000055,12.2,-4.15393073700002));
#325511=CARTESIAN_POINT('Ctrl Pts',(-0.831233596000055,5.2,-4.15393073700002));
#325512=CARTESIAN_POINT('Ctrl Pts',(-0.831233596000055,2.2,-4.15393073700002));
#325513=CARTESIAN_POINT('Ctrl Pts',(-0.830401209000057,12.2,-4.15253254800001));
#325514=CARTESIAN_POINT('Ctrl Pts',(-0.830401209000057,5.2,-4.15253254800001));
#325515=CARTESIAN_POINT('Ctrl Pts',(-0.830401209000057,2.2,-4.15253254800001));
#325516=CARTESIAN_POINT('Ctrl Pts',(-0.829572758000056,12.2,-4.15113730800002));
#325517=CARTESIAN_POINT('Ctrl Pts',(-0.829572758000056,5.2,-4.15113730800002));
#325518=CARTESIAN_POINT('Ctrl Pts',(-0.829572758000056,2.2,-4.15113730800002));
#325519=CARTESIAN_POINT('Ctrl Pts',(-0.828748237000055,12.2,-4.14974502800002));
#325520=CARTESIAN_POINT('Ctrl Pts',(-0.828748237000055,5.2,-4.14974502800002));
#325521=CARTESIAN_POINT('Ctrl Pts',(-0.828748237000055,2.2,-4.14974502800002));
#325522=CARTESIAN_POINT('Ctrl Pts',(-0.827927642000056,12.2,-4.14835572200001));
#325523=CARTESIAN_POINT('Ctrl Pts',(-0.827927642000056,5.2,-4.14835572200001));
#325524=CARTESIAN_POINT('Ctrl Pts',(-0.827927642000056,2.2,-4.14835572200001));
#325525=CARTESIAN_POINT('Ctrl Pts',(-0.827110969000057,12.2,-4.14696940100002));
#325526=CARTESIAN_POINT('Ctrl Pts',(-0.827110969000057,5.2,-4.14696940100002));
#325527=CARTESIAN_POINT('Ctrl Pts',(-0.827110969000057,2.2,-4.14696940100002));
#325528=CARTESIAN_POINT('Ctrl Pts',(-0.826298215000056,12.2,-4.14558607700001));
#325529=CARTESIAN_POINT('Ctrl Pts',(-0.826298215000056,5.2,-4.14558607700001));
#325530=CARTESIAN_POINT('Ctrl Pts',(-0.826298215000056,2.2,-4.14558607700001));
#325531=CARTESIAN_POINT('Ctrl Pts',(-0.825489374000057,12.2,-4.14420576200001));
#325532=CARTESIAN_POINT('Ctrl Pts',(-0.825489374000057,5.2,-4.14420576200001));
#325533=CARTESIAN_POINT('Ctrl Pts',(-0.825489374000057,2.2,-4.14420576200001));
#325534=CARTESIAN_POINT('Ctrl Pts',(-0.824684443000056,12.2,-4.14282846700001));
#325535=CARTESIAN_POINT('Ctrl Pts',(-0.824684443000056,5.2,-4.14282846700001));
#325536=CARTESIAN_POINT('Ctrl Pts',(-0.824684443000056,2.2,-4.14282846700001));
#325537=CARTESIAN_POINT('Ctrl Pts',(-0.823883418000056,12.2,-4.14145420800001));
#325538=CARTESIAN_POINT('Ctrl Pts',(-0.823883418000056,5.2,-4.14145420800001));
#325539=CARTESIAN_POINT('Ctrl Pts',(-0.823883418000056,2.2,-4.14145420800001));
#325540=CARTESIAN_POINT('Ctrl Pts',(-0.823086295000056,12.2,-4.14008299300002));
#325541=CARTESIAN_POINT('Ctrl Pts',(-0.823086295000056,5.2,-4.14008299300002));
#325542=CARTESIAN_POINT('Ctrl Pts',(-0.823086295000056,2.2,-4.14008299300002));
#325543=CARTESIAN_POINT('Ctrl Pts',(-0.822293068000055,12.2,-4.13871483500001));
#325544=CARTESIAN_POINT('Ctrl Pts',(-0.822293068000055,5.2,-4.13871483500001));
#325545=CARTESIAN_POINT('Ctrl Pts',(-0.822293068000055,2.2,-4.13871483500001));
#325546=CARTESIAN_POINT('Ctrl Pts',(-0.821503734000055,12.2,-4.13734974900001));
#325547=CARTESIAN_POINT('Ctrl Pts',(-0.821503734000055,5.2,-4.13734974900001));
#325548=CARTESIAN_POINT('Ctrl Pts',(-0.821503734000055,2.2,-4.13734974900001));
#325549=CARTESIAN_POINT('Ctrl Pts',(-0.820718289000055,12.2,-4.13598774400001));
#325550=CARTESIAN_POINT('Ctrl Pts',(-0.820718289000055,5.2,-4.13598774400001));
#325551=CARTESIAN_POINT('Ctrl Pts',(-0.820718289000055,2.2,-4.13598774400001));
#325552=CARTESIAN_POINT('Ctrl Pts',(-0.819936729000055,12.2,-4.13462883300001));
#325553=CARTESIAN_POINT('Ctrl Pts',(-0.819936729000055,5.2,-4.13462883300001));
#325554=CARTESIAN_POINT('Ctrl Pts',(-0.819936729000055,2.2,-4.13462883300001));
#325555=CARTESIAN_POINT('Ctrl Pts',(-0.819159048000057,12.2,-4.13327303000001));
#325556=CARTESIAN_POINT('Ctrl Pts',(-0.819159048000057,5.2,-4.13327303000001));
#325557=CARTESIAN_POINT('Ctrl Pts',(-0.819159048000057,2.2,-4.13327303000001));
#325558=CARTESIAN_POINT('Ctrl Pts',(-0.818385244000056,12.2,-4.13192034400002));
#325559=CARTESIAN_POINT('Ctrl Pts',(-0.818385244000056,5.2,-4.13192034400002));
#325560=CARTESIAN_POINT('Ctrl Pts',(-0.818385244000056,2.2,-4.13192034400002));
#325561=CARTESIAN_POINT('Ctrl Pts',(-0.817615311000056,12.2,-4.13057079000001));
#325562=CARTESIAN_POINT('Ctrl Pts',(-0.817615311000056,5.2,-4.13057079000001));
#325563=CARTESIAN_POINT('Ctrl Pts',(-0.817615311000056,2.2,-4.13057079000001));
#325564=CARTESIAN_POINT('Ctrl Pts',(-0.816849244000055,12.2,-4.12922438000002));
#325565=CARTESIAN_POINT('Ctrl Pts',(-0.816849244000055,5.2,-4.12922438000002));
#325566=CARTESIAN_POINT('Ctrl Pts',(-0.816849244000055,2.2,-4.12922438000002));
#325567=CARTESIAN_POINT('Ctrl Pts',(-0.816087040000056,12.2,-4.12788112400001));
#325568=CARTESIAN_POINT('Ctrl Pts',(-0.816087040000056,5.2,-4.12788112400001));
#325569=CARTESIAN_POINT('Ctrl Pts',(-0.816087040000056,2.2,-4.12788112400001));
#325570=CARTESIAN_POINT('Ctrl Pts',(-0.815328694000056,12.2,-4.12654103700001));
#325571=CARTESIAN_POINT('Ctrl Pts',(-0.815328694000056,5.2,-4.12654103700001));
#325572=CARTESIAN_POINT('Ctrl Pts',(-0.815328694000056,2.2,-4.12654103700001));
#325573=CARTESIAN_POINT('Ctrl Pts',(-0.814574201000056,12.2,-4.12520413000002));
#325574=CARTESIAN_POINT('Ctrl Pts',(-0.814574201000056,5.2,-4.12520413000002));
#325575=CARTESIAN_POINT('Ctrl Pts',(-0.814574201000056,2.2,-4.12520413000002));
#325576=CARTESIAN_POINT('Ctrl Pts',(-0.813823558000056,12.2,-4.12387041700002));
#325577=CARTESIAN_POINT('Ctrl Pts',(-0.813823558000056,5.2,-4.12387041700002));
#325578=CARTESIAN_POINT('Ctrl Pts',(-0.813823558000056,2.2,-4.12387041700002));
#325579=CARTESIAN_POINT('Ctrl Pts',(-0.813076758000056,12.2,-4.12253990800002));
#325580=CARTESIAN_POINT('Ctrl Pts',(-0.813076758000056,5.2,-4.12253990800002));
#325581=CARTESIAN_POINT('Ctrl Pts',(-0.813076758000056,2.2,-4.12253990800002));
#325582=CARTESIAN_POINT('Ctrl Pts',(-0.812333800000056,12.2,-4.12121261600001));
#325583=CARTESIAN_POINT('Ctrl Pts',(-0.812333800000056,5.2,-4.12121261600001));
#325584=CARTESIAN_POINT('Ctrl Pts',(-0.812333800000056,2.2,-4.12121261600001));
#325585=CARTESIAN_POINT('Ctrl Pts',(-0.811594676000055,12.2,-4.11988855500002));
#325586=CARTESIAN_POINT('Ctrl Pts',(-0.811594676000055,5.2,-4.11988855500002));
#325587=CARTESIAN_POINT('Ctrl Pts',(-0.811594676000055,2.2,-4.11988855500002));
#325588=CARTESIAN_POINT('Ctrl Pts',(-0.810859382000055,12.2,-4.11856773600002));
#325589=CARTESIAN_POINT('Ctrl Pts',(-0.810859382000055,5.2,-4.11856773600002));
#325590=CARTESIAN_POINT('Ctrl Pts',(-0.810859382000055,2.2,-4.11856773600002));
#325591=CARTESIAN_POINT('Ctrl Pts',(-0.810127916000055,12.2,-4.11725017200002));
#325592=CARTESIAN_POINT('Ctrl Pts',(-0.810127916000055,5.2,-4.11725017200002));
#325593=CARTESIAN_POINT('Ctrl Pts',(-0.810127916000055,2.2,-4.11725017200002));
#325594=CARTESIAN_POINT('Ctrl Pts',(-0.809400270000056,12.2,-4.11593587500001));
#325595=CARTESIAN_POINT('Ctrl Pts',(-0.809400270000056,5.2,-4.11593587500001));
#325596=CARTESIAN_POINT('Ctrl Pts',(-0.809400270000056,2.2,-4.11593587500001));
#325597=CARTESIAN_POINT('Ctrl Pts',(-0.808676442000056,12.2,-4.11462485700001));
#325598=CARTESIAN_POINT('Ctrl Pts',(-0.808676442000056,5.2,-4.11462485700001));
#325599=CARTESIAN_POINT('Ctrl Pts',(-0.808676442000056,2.2,-4.11462485700001));
#325600=CARTESIAN_POINT('Ctrl Pts',(-0.807956425000055,12.2,-4.11331713200001));
#325601=CARTESIAN_POINT('Ctrl Pts',(-0.807956425000055,5.2,-4.11331713200001));
#325602=CARTESIAN_POINT('Ctrl Pts',(-0.807956425000055,2.2,-4.11331713200001));
#325603=CARTESIAN_POINT('Ctrl Pts',(-0.807240215000055,12.2,-4.11201271100001));
#325604=CARTESIAN_POINT('Ctrl Pts',(-0.807240215000055,5.2,-4.11201271100001));
#325605=CARTESIAN_POINT('Ctrl Pts',(-0.807240215000055,2.2,-4.11201271100001));
#325606=CARTESIAN_POINT('Ctrl Pts',(-0.806527808000055,12.2,-4.11071160900002));
#325607=CARTESIAN_POINT('Ctrl Pts',(-0.806527808000055,5.2,-4.11071160900002));
#325608=CARTESIAN_POINT('Ctrl Pts',(-0.806527808000055,2.2,-4.11071160900002));
#325609=CARTESIAN_POINT('Ctrl Pts',(-0.805819199000056,12.2,-4.10941383600001));
#325610=CARTESIAN_POINT('Ctrl Pts',(-0.805819199000056,5.2,-4.10941383600001));
#325611=CARTESIAN_POINT('Ctrl Pts',(-0.805819199000056,2.2,-4.10941383600001));
#325612=CARTESIAN_POINT('Ctrl Pts',(-0.805114383000056,12.2,-4.10811940500002));
#325613=CARTESIAN_POINT('Ctrl Pts',(-0.805114383000056,5.2,-4.10811940500002));
#325614=CARTESIAN_POINT('Ctrl Pts',(-0.805114383000056,2.2,-4.10811940500002));
#325615=CARTESIAN_POINT('Ctrl Pts',(-0.804413354000056,12.2,-4.10682833000001));
#325616=CARTESIAN_POINT('Ctrl Pts',(-0.804413354000056,5.2,-4.10682833000001));
#325617=CARTESIAN_POINT('Ctrl Pts',(-0.804413354000056,2.2,-4.10682833000001));
#325618=CARTESIAN_POINT('Ctrl Pts',(-0.803716109000057,12.2,-4.10554062200001));
#325619=CARTESIAN_POINT('Ctrl Pts',(-0.803716109000057,5.2,-4.10554062200001));
#325620=CARTESIAN_POINT('Ctrl Pts',(-0.803716109000057,2.2,-4.10554062200001));
#325621=CARTESIAN_POINT('Ctrl Pts',(-0.803022642000055,12.2,-4.10425629400001));
#325622=CARTESIAN_POINT('Ctrl Pts',(-0.803022642000055,5.2,-4.10425629400001));
#325623=CARTESIAN_POINT('Ctrl Pts',(-0.803022642000055,2.2,-4.10425629400001));
#325624=CARTESIAN_POINT('Ctrl Pts',(-0.802332949000055,12.2,-4.10297536000002));
#325625=CARTESIAN_POINT('Ctrl Pts',(-0.802332949000055,5.2,-4.10297536000002));
#325626=CARTESIAN_POINT('Ctrl Pts',(-0.802332949000055,2.2,-4.10297536000002));
#325627=CARTESIAN_POINT('Ctrl Pts',(-0.801647024000056,12.2,-4.10169783100002));
#325628=CARTESIAN_POINT('Ctrl Pts',(-0.801647024000056,5.2,-4.10169783100002));
#325629=CARTESIAN_POINT('Ctrl Pts',(-0.801647024000056,2.2,-4.10169783100002));
#325630=CARTESIAN_POINT('Ctrl Pts',(-0.800964863000055,12.2,-4.10042372100001));
#325631=CARTESIAN_POINT('Ctrl Pts',(-0.800964863000055,5.2,-4.10042372100001));
#325632=CARTESIAN_POINT('Ctrl Pts',(-0.800964863000055,2.2,-4.10042372100001));
#325633=CARTESIAN_POINT('Ctrl Pts',(-0.800286459000056,12.2,-4.09915304200001));
#325634=CARTESIAN_POINT('Ctrl Pts',(-0.800286459000056,5.2,-4.09915304200001));
#325635=CARTESIAN_POINT('Ctrl Pts',(-0.800286459000056,2.2,-4.09915304200001));
#325636=CARTESIAN_POINT('Ctrl Pts',(-0.799611809000057,12.2,-4.09788580800001));
#325637=CARTESIAN_POINT('Ctrl Pts',(-0.799611809000057,5.2,-4.09788580800001));
#325638=CARTESIAN_POINT('Ctrl Pts',(-0.799611809000057,2.2,-4.09788580800001));
#325639=CARTESIAN_POINT('Ctrl Pts',(-0.798940908000055,12.2,-4.09662202900002));
#325640=CARTESIAN_POINT('Ctrl Pts',(-0.798940908000055,5.2,-4.09662202900002));
#325641=CARTESIAN_POINT('Ctrl Pts',(-0.798940908000055,2.2,-4.09662202900002));
#325642=CARTESIAN_POINT('Ctrl Pts',(-0.798273750000057,12.2,-4.09536172000001));
#325643=CARTESIAN_POINT('Ctrl Pts',(-0.798273750000057,5.2,-4.09536172000001));
#325644=CARTESIAN_POINT('Ctrl Pts',(-0.798273750000057,2.2,-4.09536172000001));
#325645=CARTESIAN_POINT('Ctrl Pts',(-0.797610330000056,12.2,-4.09410489300001));
#325646=CARTESIAN_POINT('Ctrl Pts',(-0.797610330000056,5.2,-4.09410489300001));
#325647=CARTESIAN_POINT('Ctrl Pts',(-0.797610330000056,2.2,-4.09410489300001));
#325648=CARTESIAN_POINT('Ctrl Pts',(-0.796950643000055,12.2,-4.09285156100001));
#325649=CARTESIAN_POINT('Ctrl Pts',(-0.796950643000055,5.2,-4.09285156100001));
#325650=CARTESIAN_POINT('Ctrl Pts',(-0.796950643000055,2.2,-4.09285156100001));
#325651=CARTESIAN_POINT('Ctrl Pts',(-0.796294684000056,12.2,-4.09160173700001));
#325652=CARTESIAN_POINT('Ctrl Pts',(-0.796294684000056,5.2,-4.09160173700001));
#325653=CARTESIAN_POINT('Ctrl Pts',(-0.796294684000056,2.2,-4.09160173700001));
#325654=CARTESIAN_POINT('Ctrl Pts',(-0.795642447000056,12.2,-4.09035543500002));
#325655=CARTESIAN_POINT('Ctrl Pts',(-0.795642447000056,5.2,-4.09035543500002));
#325656=CARTESIAN_POINT('Ctrl Pts',(-0.795642447000056,2.2,-4.09035543500002));
#325657=CARTESIAN_POINT('Ctrl Pts',(-0.794993928000055,12.2,-4.08911266500001));
#325658=CARTESIAN_POINT('Ctrl Pts',(-0.794993928000055,5.2,-4.08911266500001));
#325659=CARTESIAN_POINT('Ctrl Pts',(-0.794993928000055,2.2,-4.08911266500001));
#325660=CARTESIAN_POINT('Ctrl Pts',(-0.794349120000056,12.2,-4.08787344200002));
#325661=CARTESIAN_POINT('Ctrl Pts',(-0.794349120000056,5.2,-4.08787344200002));
#325662=CARTESIAN_POINT('Ctrl Pts',(-0.794349120000056,2.2,-4.08787344200002));
#325663=CARTESIAN_POINT('Ctrl Pts',(-0.793708020000056,12.2,-4.08663777800002));
#325664=CARTESIAN_POINT('Ctrl Pts',(-0.793708020000056,5.2,-4.08663777800002));
#325665=CARTESIAN_POINT('Ctrl Pts',(-0.793708020000056,2.2,-4.08663777800002));
#325666=CARTESIAN_POINT('Ctrl Pts',(-0.793070621000057,12.2,-4.08540568800001));
#325667=CARTESIAN_POINT('Ctrl Pts',(-0.793070621000057,5.2,-4.08540568800001));
#325668=CARTESIAN_POINT('Ctrl Pts',(-0.793070621000057,2.2,-4.08540568800001));
#325669=CARTESIAN_POINT('Ctrl Pts',(-0.792436919000057,12.2,-4.08417718200001));
#325670=CARTESIAN_POINT('Ctrl Pts',(-0.792436919000057,5.2,-4.08417718200001));
#325671=CARTESIAN_POINT('Ctrl Pts',(-0.792436919000057,2.2,-4.08417718200001));
#325672=CARTESIAN_POINT('Ctrl Pts',(-0.791806906000057,12.2,-4.08295227500002));
#325673=CARTESIAN_POINT('Ctrl Pts',(-0.791806906000057,5.2,-4.08295227500002));
#325674=CARTESIAN_POINT('Ctrl Pts',(-0.791806906000057,2.2,-4.08295227500002));
#325675=CARTESIAN_POINT('Ctrl Pts',(-0.791180580000056,12.2,-4.08173097900002));
#325676=CARTESIAN_POINT('Ctrl Pts',(-0.791180580000056,5.2,-4.08173097900002));
#325677=CARTESIAN_POINT('Ctrl Pts',(-0.791180580000056,2.2,-4.08173097900002));
#325678=CARTESIAN_POINT('Ctrl Pts',(-0.790557934000056,12.2,-4.08051330800001));
#325679=CARTESIAN_POINT('Ctrl Pts',(-0.790557934000056,5.2,-4.08051330800001));
#325680=CARTESIAN_POINT('Ctrl Pts',(-0.790557934000056,2.2,-4.08051330800001));
#325681=CARTESIAN_POINT('Ctrl Pts',(-0.789938961000055,12.2,-4.07929927400001));
#325682=CARTESIAN_POINT('Ctrl Pts',(-0.789938961000055,5.2,-4.07929927400001));
#325683=CARTESIAN_POINT('Ctrl Pts',(-0.789938961000055,2.2,-4.07929927400001));
#325684=CARTESIAN_POINT('Ctrl Pts',(-0.789323659000055,12.2,-4.07808889000002));
#325685=CARTESIAN_POINT('Ctrl Pts',(-0.789323659000055,5.2,-4.07808889000002));
#325686=CARTESIAN_POINT('Ctrl Pts',(-0.789323659000055,2.2,-4.07808889000002));
#325687=CARTESIAN_POINT('Ctrl Pts',(-0.788712019000056,12.2,-4.07688217000001));
#325688=CARTESIAN_POINT('Ctrl Pts',(-0.788712019000056,5.2,-4.07688217000001));
#325689=CARTESIAN_POINT('Ctrl Pts',(-0.788712019000056,2.2,-4.07688217000001));
#325690=CARTESIAN_POINT('Ctrl Pts',(-0.788104037000057,12.2,-4.07567912700001));
#325691=CARTESIAN_POINT('Ctrl Pts',(-0.788104037000057,5.2,-4.07567912700001));
#325692=CARTESIAN_POINT('Ctrl Pts',(-0.788104037000057,2.2,-4.07567912700001));
#325693=CARTESIAN_POINT('Ctrl Pts',(-0.787499708000056,12.2,-4.07447977400002));
#325694=CARTESIAN_POINT('Ctrl Pts',(-0.787499708000056,5.2,-4.07447977400002));
#325695=CARTESIAN_POINT('Ctrl Pts',(-0.787499708000056,2.2,-4.07447977400002));
#325696=CARTESIAN_POINT('Ctrl Pts',(-0.786899026000055,12.2,-4.07328412200001));
#325697=CARTESIAN_POINT('Ctrl Pts',(-0.786899026000055,5.2,-4.07328412200001));
#325698=CARTESIAN_POINT('Ctrl Pts',(-0.786899026000055,2.2,-4.07328412200001));
#325699=CARTESIAN_POINT('Ctrl Pts',(-0.786301985000056,12.2,-4.07209218900002));
#325700=CARTESIAN_POINT('Ctrl Pts',(-0.786301985000056,5.2,-4.07209218900002));
#325701=CARTESIAN_POINT('Ctrl Pts',(-0.786301985000056,2.2,-4.07209218900002));
#325702=CARTESIAN_POINT('Ctrl Pts',(-0.785708579000056,12.2,-4.07090398400001));
#325703=CARTESIAN_POINT('Ctrl Pts',(-0.785708579000056,5.2,-4.07090398400001));
#325704=CARTESIAN_POINT('Ctrl Pts',(-0.785708579000056,2.2,-4.07090398400001));
#325705=CARTESIAN_POINT('Ctrl Pts',(-0.785118804000057,12.2,-4.06971952100001));
#325706=CARTESIAN_POINT('Ctrl Pts',(-0.785118804000057,5.2,-4.06971952100001));
#325707=CARTESIAN_POINT('Ctrl Pts',(-0.785118804000057,2.2,-4.06971952100001));
#325708=CARTESIAN_POINT('Ctrl Pts',(-0.784532652000056,12.2,-4.06853881500002));
#325709=CARTESIAN_POINT('Ctrl Pts',(-0.784532652000056,5.2,-4.06853881500002));
#325710=CARTESIAN_POINT('Ctrl Pts',(-0.784532652000056,2.2,-4.06853881500002));
#325711=CARTESIAN_POINT('Ctrl Pts',(-0.783950118000056,12.2,-4.06736187600002));
#325712=CARTESIAN_POINT('Ctrl Pts',(-0.783950118000056,5.2,-4.06736187600002));
#325713=CARTESIAN_POINT('Ctrl Pts',(-0.783950118000056,2.2,-4.06736187600002));
#325714=CARTESIAN_POINT('Ctrl Pts',(-0.783371197000056,12.2,-4.06618872200001));
#325715=CARTESIAN_POINT('Ctrl Pts',(-0.783371197000056,5.2,-4.06618872200001));
#325716=CARTESIAN_POINT('Ctrl Pts',(-0.783371197000056,2.2,-4.06618872200001));
#325717=CARTESIAN_POINT('Ctrl Pts',(-0.782795883000055,12.2,-4.06501936200002));
#325718=CARTESIAN_POINT('Ctrl Pts',(-0.782795883000055,5.2,-4.06501936200002));
#325719=CARTESIAN_POINT('Ctrl Pts',(-0.782795883000055,2.2,-4.06501936200002));
#325720=CARTESIAN_POINT('Ctrl Pts',(-0.782224170000055,12.2,-4.06385381100002));
#325721=CARTESIAN_POINT('Ctrl Pts',(-0.782224170000055,5.2,-4.06385381100002));
#325722=CARTESIAN_POINT('Ctrl Pts',(-0.782224170000055,2.2,-4.06385381100002));
#325723=CARTESIAN_POINT('Ctrl Pts',(-0.781656052000056,12.2,-4.06269208200001));
#325724=CARTESIAN_POINT('Ctrl Pts',(-0.781656052000056,5.2,-4.06269208200001));
#325725=CARTESIAN_POINT('Ctrl Pts',(-0.781656052000056,2.2,-4.06269208200001));
#325726=CARTESIAN_POINT('Ctrl Pts',(-0.781091522000056,12.2,-4.06153418900002));
#325727=CARTESIAN_POINT('Ctrl Pts',(-0.781091522000056,5.2,-4.06153418900002));
#325728=CARTESIAN_POINT('Ctrl Pts',(-0.781091522000056,2.2,-4.06153418900002));
#325729=CARTESIAN_POINT('Ctrl Pts',(-0.780530576000055,12.2,-4.06038014600002));
#325730=CARTESIAN_POINT('Ctrl Pts',(-0.780530576000055,5.2,-4.06038014600002));
#325731=CARTESIAN_POINT('Ctrl Pts',(-0.780530576000055,2.2,-4.06038014600002));
#325732=CARTESIAN_POINT('Ctrl Pts',(-0.779973208000057,12.2,-4.05922996500002));
#325733=CARTESIAN_POINT('Ctrl Pts',(-0.779973208000057,5.2,-4.05922996500002));
#325734=CARTESIAN_POINT('Ctrl Pts',(-0.779973208000057,2.2,-4.05922996500002));
#325735=CARTESIAN_POINT('Ctrl Pts',(-0.779419410000056,12.2,-4.05808365900001));
#325736=CARTESIAN_POINT('Ctrl Pts',(-0.779419410000056,5.2,-4.05808365900001));
#325737=CARTESIAN_POINT('Ctrl Pts',(-0.779419410000056,2.2,-4.05808365900001));
#325738=CARTESIAN_POINT('Ctrl Pts',(-0.778869177000056,12.2,-4.05694124300001));
#325739=CARTESIAN_POINT('Ctrl Pts',(-0.778869177000056,5.2,-4.05694124300001));
#325740=CARTESIAN_POINT('Ctrl Pts',(-0.778869177000056,2.2,-4.05694124300001));
#325741=CARTESIAN_POINT('Ctrl Pts',(-0.778322505000055,12.2,-4.05580272900002));
#325742=CARTESIAN_POINT('Ctrl Pts',(-0.778322505000055,5.2,-4.05580272900002));
#325743=CARTESIAN_POINT('Ctrl Pts',(-0.778322505000055,2.2,-4.05580272900002));
#325744=CARTESIAN_POINT('Ctrl Pts',(-0.777779384000056,12.2,-4.05466813200002));
#325745=CARTESIAN_POINT('Ctrl Pts',(-0.777779384000056,5.2,-4.05466813200002));
#325746=CARTESIAN_POINT('Ctrl Pts',(-0.777779384000056,2.2,-4.05466813200002));
#325747=CARTESIAN_POINT('Ctrl Pts',(-0.777239810000055,12.2,-4.05353746500001));
#325748=CARTESIAN_POINT('Ctrl Pts',(-0.777239810000055,5.2,-4.05353746500001));
#325749=CARTESIAN_POINT('Ctrl Pts',(-0.777239810000055,2.2,-4.05353746500001));
#325750=CARTESIAN_POINT('Ctrl Pts',(-0.776703778000056,12.2,-4.05241074100001));
#325751=CARTESIAN_POINT('Ctrl Pts',(-0.776703778000056,5.2,-4.05241074100001));
#325752=CARTESIAN_POINT('Ctrl Pts',(-0.776703778000056,2.2,-4.05241074100001));
#325753=CARTESIAN_POINT('Ctrl Pts',(-0.776171280000056,12.2,-4.05128797400002));
#325754=CARTESIAN_POINT('Ctrl Pts',(-0.776171280000056,5.2,-4.05128797400002));
#325755=CARTESIAN_POINT('Ctrl Pts',(-0.776171280000056,2.2,-4.05128797400002));
#325756=CARTESIAN_POINT('Ctrl Pts',(-0.775642310000055,12.2,-4.05016917800001));
#325757=CARTESIAN_POINT('Ctrl Pts',(-0.775642310000055,5.2,-4.05016917800001));
#325758=CARTESIAN_POINT('Ctrl Pts',(-0.775642310000055,2.2,-4.05016917800001));
#325759=CARTESIAN_POINT('Ctrl Pts',(-0.775116863000056,12.2,-4.04905436500002));
#325760=CARTESIAN_POINT('Ctrl Pts',(-0.775116863000056,5.2,-4.04905436500002));
#325761=CARTESIAN_POINT('Ctrl Pts',(-0.775116863000056,2.2,-4.04905436500002));
#325762=CARTESIAN_POINT('Ctrl Pts',(-0.774594932000056,12.2,-4.04794355100002));
#325763=CARTESIAN_POINT('Ctrl Pts',(-0.774594932000056,5.2,-4.04794355100002));
#325764=CARTESIAN_POINT('Ctrl Pts',(-0.774594932000056,2.2,-4.04794355100002));
#325765=CARTESIAN_POINT('Ctrl Pts',(-0.774076510000056,12.2,-4.04683674800001));
#325766=CARTESIAN_POINT('Ctrl Pts',(-0.774076510000056,5.2,-4.04683674800001));
#325767=CARTESIAN_POINT('Ctrl Pts',(-0.774076510000056,2.2,-4.04683674800001));
#325768=CARTESIAN_POINT('Ctrl Pts',(-0.773561591000057,12.2,-4.04573397000001));
#325769=CARTESIAN_POINT('Ctrl Pts',(-0.773561591000057,5.2,-4.04573397000001));
#325770=CARTESIAN_POINT('Ctrl Pts',(-0.773561591000057,2.2,-4.04573397000001));
#325771=CARTESIAN_POINT('Ctrl Pts',(-0.773050169000056,12.2,-4.04463523000001));
#325772=CARTESIAN_POINT('Ctrl Pts',(-0.773050169000056,5.2,-4.04463523000001));
#325773=CARTESIAN_POINT('Ctrl Pts',(-0.773050169000056,2.2,-4.04463523000001));
#325774=CARTESIAN_POINT('Ctrl Pts',(-0.772542238000057,12.2,-4.04354054300001));
#325775=CARTESIAN_POINT('Ctrl Pts',(-0.772542238000057,5.2,-4.04354054300001));
#325776=CARTESIAN_POINT('Ctrl Pts',(-0.772542238000057,2.2,-4.04354054300001));
#325777=CARTESIAN_POINT('Ctrl Pts',(-0.772037790000055,12.2,-4.04244992300002));
#325778=CARTESIAN_POINT('Ctrl Pts',(-0.772037790000055,5.2,-4.04244992300002));
#325779=CARTESIAN_POINT('Ctrl Pts',(-0.772037790000055,2.2,-4.04244992300002));
#325780=CARTESIAN_POINT('Ctrl Pts',(-0.771536819000056,12.2,-4.04136338200002));
#325781=CARTESIAN_POINT('Ctrl Pts',(-0.771536819000056,5.2,-4.04136338200002));
#325782=CARTESIAN_POINT('Ctrl Pts',(-0.771536819000056,2.2,-4.04136338200002));
#325783=CARTESIAN_POINT('Ctrl Pts',(-0.771039320000056,12.2,-4.04028093500001));
#325784=CARTESIAN_POINT('Ctrl Pts',(-0.771039320000056,5.2,-4.04028093500001));
#325785=CARTESIAN_POINT('Ctrl Pts',(-0.771039320000056,2.2,-4.04028093500001));
#325786=CARTESIAN_POINT('Ctrl Pts',(-0.770545286000056,12.2,-4.03920259600001));
#325787=CARTESIAN_POINT('Ctrl Pts',(-0.770545286000056,5.2,-4.03920259600001));
#325788=CARTESIAN_POINT('Ctrl Pts',(-0.770545286000056,2.2,-4.03920259600001));
#325789=CARTESIAN_POINT('Ctrl Pts',(-0.770054709000056,12.2,-4.03812837800002));
#325790=CARTESIAN_POINT('Ctrl Pts',(-0.770054709000056,5.2,-4.03812837800002));
#325791=CARTESIAN_POINT('Ctrl Pts',(-0.770054709000056,2.2,-4.03812837800002));
#325792=CARTESIAN_POINT('Ctrl Pts',(-0.769567583000056,12.2,-4.03705829600002));
#325793=CARTESIAN_POINT('Ctrl Pts',(-0.769567583000056,5.2,-4.03705829600002));
#325794=CARTESIAN_POINT('Ctrl Pts',(-0.769567583000056,2.2,-4.03705829600002));
#325795=CARTESIAN_POINT('Ctrl Pts',(-0.769083902000055,12.2,-4.03599236300002));
#325796=CARTESIAN_POINT('Ctrl Pts',(-0.769083902000055,5.2,-4.03599236300002));
#325797=CARTESIAN_POINT('Ctrl Pts',(-0.769083902000055,2.2,-4.03599236300002));
#325798=CARTESIAN_POINT('Ctrl Pts',(-0.768603660000055,12.2,-4.03493059300001));
#325799=CARTESIAN_POINT('Ctrl Pts',(-0.768603660000055,5.2,-4.03493059300001));
#325800=CARTESIAN_POINT('Ctrl Pts',(-0.768603660000055,2.2,-4.03493059300001));
#325801=CARTESIAN_POINT('Ctrl Pts',(-0.768126848000056,12.2,-4.03387300000002));
#325802=CARTESIAN_POINT('Ctrl Pts',(-0.768126848000056,5.2,-4.03387300000002));
#325803=CARTESIAN_POINT('Ctrl Pts',(-0.768126848000056,2.2,-4.03387300000002));
#325804=CARTESIAN_POINT('Ctrl Pts',(-0.767653461000056,12.2,-4.03281959800001));
#325805=CARTESIAN_POINT('Ctrl Pts',(-0.767653461000056,5.2,-4.03281959800001));
#325806=CARTESIAN_POINT('Ctrl Pts',(-0.767653461000056,2.2,-4.03281959800001));
#325807=CARTESIAN_POINT('Ctrl Pts',(-0.767183491000055,12.2,-4.03177040100001));
#325808=CARTESIAN_POINT('Ctrl Pts',(-0.767183491000055,5.2,-4.03177040100001));
#325809=CARTESIAN_POINT('Ctrl Pts',(-0.767183491000055,2.2,-4.03177040100001));
#325810=CARTESIAN_POINT('Ctrl Pts',(-0.766716933000057,12.2,-4.03072542300002));
#325811=CARTESIAN_POINT('Ctrl Pts',(-0.766716933000057,5.2,-4.03072542300002));
#325812=CARTESIAN_POINT('Ctrl Pts',(-0.766716933000057,2.2,-4.03072542300002));
#325813=CARTESIAN_POINT('Ctrl Pts',(-0.766253778000056,12.2,-4.02968467800001));
#325814=CARTESIAN_POINT('Ctrl Pts',(-0.766253778000056,5.2,-4.02968467800001));
#325815=CARTESIAN_POINT('Ctrl Pts',(-0.766253778000056,2.2,-4.02968467800001));
#325816=CARTESIAN_POINT('Ctrl Pts',(-0.765794021000056,12.2,-4.02864818000001));
#325817=CARTESIAN_POINT('Ctrl Pts',(-0.765794021000056,5.2,-4.02864818000001));
#325818=CARTESIAN_POINT('Ctrl Pts',(-0.765794021000056,2.2,-4.02864818000001));
#325819=CARTESIAN_POINT('Ctrl Pts',(-0.765337654000057,12.2,-4.02761594400001));
#325820=CARTESIAN_POINT('Ctrl Pts',(-0.765337654000057,5.2,-4.02761594400001));
#325821=CARTESIAN_POINT('Ctrl Pts',(-0.765337654000057,2.2,-4.02761594400001));
#325822=CARTESIAN_POINT('Ctrl Pts',(-0.764884670000056,12.2,-4.02658798200001));
#325823=CARTESIAN_POINT('Ctrl Pts',(-0.764884670000056,5.2,-4.02658798200001));
#325824=CARTESIAN_POINT('Ctrl Pts',(-0.764884670000056,2.2,-4.02658798200001));
#325825=CARTESIAN_POINT('Ctrl Pts',(-0.764435063000055,12.2,-4.02556431100002));
#325826=CARTESIAN_POINT('Ctrl Pts',(-0.764435063000055,5.2,-4.02556431100002));
#325827=CARTESIAN_POINT('Ctrl Pts',(-0.764435063000055,2.2,-4.02556431100002));
#325828=CARTESIAN_POINT('Ctrl Pts',(-0.763988825000055,12.2,-4.02454494200001));
#325829=CARTESIAN_POINT('Ctrl Pts',(-0.763988825000055,5.2,-4.02454494200001));
#325830=CARTESIAN_POINT('Ctrl Pts',(-0.763988825000055,2.2,-4.02454494200001));
#325831=CARTESIAN_POINT('Ctrl Pts',(-0.763545950000056,12.2,-4.02352989200002));
#325832=CARTESIAN_POINT('Ctrl Pts',(-0.763545950000056,5.2,-4.02352989200002));
#325833=CARTESIAN_POINT('Ctrl Pts',(-0.763545950000056,2.2,-4.02352989200002));
#325834=CARTESIAN_POINT('Ctrl Pts',(-0.763106429000056,12.2,-4.02251917300001));
#325835=CARTESIAN_POINT('Ctrl Pts',(-0.763106429000056,5.2,-4.02251917300001));
#325836=CARTESIAN_POINT('Ctrl Pts',(-0.763106429000056,2.2,-4.02251917300001));
#325837=CARTESIAN_POINT('Ctrl Pts',(-0.762670257000057,12.2,-4.02151280100002));
#325838=CARTESIAN_POINT('Ctrl Pts',(-0.762670257000057,5.2,-4.02151280100002));
#325839=CARTESIAN_POINT('Ctrl Pts',(-0.762670257000057,2.2,-4.02151280100002));
#325840=CARTESIAN_POINT('Ctrl Pts',(-0.762237425000055,12.2,-4.02051078900001));
#325841=CARTESIAN_POINT('Ctrl Pts',(-0.762237425000055,5.2,-4.02051078900001));
#325842=CARTESIAN_POINT('Ctrl Pts',(-0.762237425000055,2.2,-4.02051078900001));
#325843=CARTESIAN_POINT('Ctrl Pts',(-0.761807927000057,12.2,-4.01951315200002));
#325844=CARTESIAN_POINT('Ctrl Pts',(-0.761807927000057,5.2,-4.01951315200002));
#325845=CARTESIAN_POINT('Ctrl Pts',(-0.761807927000057,2.2,-4.01951315200002));
#325846=CARTESIAN_POINT('Ctrl Pts',(-0.761381757000056,12.2,-4.01851990400001));
#325847=CARTESIAN_POINT('Ctrl Pts',(-0.761381757000056,5.2,-4.01851990400001));
#325848=CARTESIAN_POINT('Ctrl Pts',(-0.761381757000056,2.2,-4.01851990400001));
#325849=CARTESIAN_POINT('Ctrl Pts',(-0.760958905000055,12.2,-4.01753105900001));
#325850=CARTESIAN_POINT('Ctrl Pts',(-0.760958905000055,5.2,-4.01753105900001));
#325851=CARTESIAN_POINT('Ctrl Pts',(-0.760958905000055,2.2,-4.01753105900001));
#325852=CARTESIAN_POINT('Ctrl Pts',(-0.760539364000056,12.2,-4.01654663200001));
#325853=CARTESIAN_POINT('Ctrl Pts',(-0.760539364000056,5.2,-4.01654663200001));
#325854=CARTESIAN_POINT('Ctrl Pts',(-0.760539364000056,2.2,-4.01654663200001));
#325855=CARTESIAN_POINT('Ctrl Pts',(-0.760123129000055,12.2,-4.01556663700001));
#325856=CARTESIAN_POINT('Ctrl Pts',(-0.760123129000055,5.2,-4.01556663700001));
#325857=CARTESIAN_POINT('Ctrl Pts',(-0.760123129000055,2.2,-4.01556663700001));
#325858=CARTESIAN_POINT('Ctrl Pts',(-0.759710191000057,12.2,-4.01459108800001));
#325859=CARTESIAN_POINT('Ctrl Pts',(-0.759710191000057,5.2,-4.01459108800001));
#325860=CARTESIAN_POINT('Ctrl Pts',(-0.759710191000057,2.2,-4.01459108800001));
#325861=CARTESIAN_POINT('Ctrl Pts',(-0.759300543000055,12.2,-4.01362000100002));
#325862=CARTESIAN_POINT('Ctrl Pts',(-0.759300543000055,5.2,-4.01362000100002));
#325863=CARTESIAN_POINT('Ctrl Pts',(-0.759300543000055,2.2,-4.01362000100002));
#325864=CARTESIAN_POINT('Ctrl Pts',(-0.758894177000055,12.2,-4.01265338900001));
#325865=CARTESIAN_POINT('Ctrl Pts',(-0.758894177000055,5.2,-4.01265338900001));
#325866=CARTESIAN_POINT('Ctrl Pts',(-0.758894177000055,2.2,-4.01265338900001));
#325867=CARTESIAN_POINT('Ctrl Pts',(-0.758491086000056,12.2,-4.01169126700001));
#325868=CARTESIAN_POINT('Ctrl Pts',(-0.758491086000056,5.2,-4.01169126700001));
#325869=CARTESIAN_POINT('Ctrl Pts',(-0.758491086000056,2.2,-4.01169126700001));
#325870=CARTESIAN_POINT('Ctrl Pts',(-0.758091263000056,12.2,-4.01073364900002));
#325871=CARTESIAN_POINT('Ctrl Pts',(-0.758091263000056,5.2,-4.01073364900002));
#325872=CARTESIAN_POINT('Ctrl Pts',(-0.758091263000056,2.2,-4.01073364900002));
#325873=CARTESIAN_POINT('Ctrl Pts',(-0.757694698000057,12.2,-4.00978055000001));
#325874=CARTESIAN_POINT('Ctrl Pts',(-0.757694698000057,5.2,-4.00978055000001));
#325875=CARTESIAN_POINT('Ctrl Pts',(-0.757694698000057,2.2,-4.00978055000001));
#325876=CARTESIAN_POINT('Ctrl Pts',(-0.757301387000057,12.2,-4.00883198500001));
#325877=CARTESIAN_POINT('Ctrl Pts',(-0.757301387000057,5.2,-4.00883198500001));
#325878=CARTESIAN_POINT('Ctrl Pts',(-0.757301387000057,2.2,-4.00883198500001));
#325879=CARTESIAN_POINT('Ctrl Pts',(-0.756911320000055,12.2,-4.00788796800001));
#325880=CARTESIAN_POINT('Ctrl Pts',(-0.756911320000055,5.2,-4.00788796800001));
#325881=CARTESIAN_POINT('Ctrl Pts',(-0.756911320000055,2.2,-4.00788796800001));
#325882=CARTESIAN_POINT('Ctrl Pts',(-0.756524489000056,12.2,-4.00694851300001));
#325883=CARTESIAN_POINT('Ctrl Pts',(-0.756524489000056,5.2,-4.00694851300001));
#325884=CARTESIAN_POINT('Ctrl Pts',(-0.756524489000056,2.2,-4.00694851300001));
#325885=CARTESIAN_POINT('Ctrl Pts',(-0.756140888000055,12.2,-4.00601363600002));
#325886=CARTESIAN_POINT('Ctrl Pts',(-0.756140888000055,5.2,-4.00601363600002));
#325887=CARTESIAN_POINT('Ctrl Pts',(-0.756140888000055,2.2,-4.00601363600002));
#325888=CARTESIAN_POINT('Ctrl Pts',(-0.755760509000056,12.2,-4.00508335200001));
#325889=CARTESIAN_POINT('Ctrl Pts',(-0.755760509000056,5.2,-4.00508335200001));
#325890=CARTESIAN_POINT('Ctrl Pts',(-0.755760509000056,2.2,-4.00508335200001));
#325891=CARTESIAN_POINT('Ctrl Pts',(-0.755383344000055,12.2,-4.00415767300002));
#325892=CARTESIAN_POINT('Ctrl Pts',(-0.755383344000055,5.2,-4.00415767300002));
#325893=CARTESIAN_POINT('Ctrl Pts',(-0.755383344000055,2.2,-4.00415767300002));
#325894=CARTESIAN_POINT('Ctrl Pts',(-0.755009383000056,12.2,-4.00323661600002));
#325895=CARTESIAN_POINT('Ctrl Pts',(-0.755009383000056,5.2,-4.00323661600002));
#325896=CARTESIAN_POINT('Ctrl Pts',(-0.755009383000056,2.2,-4.00323661600002));
#325897=CARTESIAN_POINT('Ctrl Pts',(-0.754638622000057,12.2,-4.00232019600002));
#325898=CARTESIAN_POINT('Ctrl Pts',(-0.754638622000057,5.2,-4.00232019600002));
#325899=CARTESIAN_POINT('Ctrl Pts',(-0.754638622000057,2.2,-4.00232019600002));
#325900=CARTESIAN_POINT('Ctrl Pts',(-0.754271050000056,12.2,-4.00140842600001));
#325901=CARTESIAN_POINT('Ctrl Pts',(-0.754271050000056,5.2,-4.00140842600001));
#325902=CARTESIAN_POINT('Ctrl Pts',(-0.754271050000056,2.2,-4.00140842600001));
#325903=CARTESIAN_POINT('Ctrl Pts',(-0.753906660000055,12.2,-4.00050132300001));
#325904=CARTESIAN_POINT('Ctrl Pts',(-0.753906660000055,5.2,-4.00050132300001));
#325905=CARTESIAN_POINT('Ctrl Pts',(-0.753906660000055,2.2,-4.00050132300001));
#325906=CARTESIAN_POINT('Ctrl Pts',(-0.753545444000056,12.2,-3.99959889900002));
#325907=CARTESIAN_POINT('Ctrl Pts',(-0.753545444000056,5.2,-3.99959889900002));
#325908=CARTESIAN_POINT('Ctrl Pts',(-0.753545444000056,2.2,-3.99959889900002));
#325909=CARTESIAN_POINT('Ctrl Pts',(-0.753187395000056,12.2,-3.99870117100001));
#325910=CARTESIAN_POINT('Ctrl Pts',(-0.753187395000056,5.2,-3.99870117100001));
#325911=CARTESIAN_POINT('Ctrl Pts',(-0.753187395000056,2.2,-3.99870117100001));
#325912=CARTESIAN_POINT('Ctrl Pts',(-0.752832503000055,12.2,-3.99780815500002));
#325913=CARTESIAN_POINT('Ctrl Pts',(-0.752832503000055,5.2,-3.99780815500002));
#325914=CARTESIAN_POINT('Ctrl Pts',(-0.752832503000055,2.2,-3.99780815500002));
#325915=CARTESIAN_POINT('Ctrl Pts',(-0.752480762000056,12.2,-3.99691986300001));
#325916=CARTESIAN_POINT('Ctrl Pts',(-0.752480762000056,5.2,-3.99691986300001));
#325917=CARTESIAN_POINT('Ctrl Pts',(-0.752480762000056,2.2,-3.99691986300001));
#325918=CARTESIAN_POINT('Ctrl Pts',(-0.752132163000055,12.2,-3.99603631100002));
#325919=CARTESIAN_POINT('Ctrl Pts',(-0.752132163000055,5.2,-3.99603631100002));
#325920=CARTESIAN_POINT('Ctrl Pts',(-0.752132163000055,2.2,-3.99603631100002));
#325921=CARTESIAN_POINT('Ctrl Pts',(-0.751786697000056,12.2,-3.99515751500001));
#325922=CARTESIAN_POINT('Ctrl Pts',(-0.751786697000056,5.2,-3.99515751500001));
#325923=CARTESIAN_POINT('Ctrl Pts',(-0.751786697000056,2.2,-3.99515751500001));
#325924=CARTESIAN_POINT('Ctrl Pts',(-0.751444357000055,12.2,-3.99428348800001));
#325925=CARTESIAN_POINT('Ctrl Pts',(-0.751444357000055,5.2,-3.99428348800001));
#325926=CARTESIAN_POINT('Ctrl Pts',(-0.751444357000055,2.2,-3.99428348800001));
#325927=CARTESIAN_POINT('Ctrl Pts',(-0.751105134000056,12.2,-3.99341424700001));
#325928=CARTESIAN_POINT('Ctrl Pts',(-0.751105134000056,5.2,-3.99341424700001));
#325929=CARTESIAN_POINT('Ctrl Pts',(-0.751105134000056,2.2,-3.99341424700001));
#325930=CARTESIAN_POINT('Ctrl Pts',(-0.750769020000056,12.2,-3.99254980800002));
#325931=CARTESIAN_POINT('Ctrl Pts',(-0.750769020000056,5.2,-3.99254980800002));
#325932=CARTESIAN_POINT('Ctrl Pts',(-0.750769020000056,2.2,-3.99254980800002));
#325933=CARTESIAN_POINT('Ctrl Pts',(-0.750436006000056,12.2,-3.99169018200002));
#325934=CARTESIAN_POINT('Ctrl Pts',(-0.750436006000056,5.2,-3.99169018200002));
#325935=CARTESIAN_POINT('Ctrl Pts',(-0.750436006000056,2.2,-3.99169018200002));
#325936=CARTESIAN_POINT('Ctrl Pts',(-0.750106085000055,12.2,-3.99083538700001));
#325937=CARTESIAN_POINT('Ctrl Pts',(-0.750106085000055,5.2,-3.99083538700001));
#325938=CARTESIAN_POINT('Ctrl Pts',(-0.750106085000055,2.2,-3.99083538700001));
#325939=CARTESIAN_POINT('Ctrl Pts',(-0.749779247000056,12.2,-3.98998543900001));
#325940=CARTESIAN_POINT('Ctrl Pts',(-0.749779247000056,5.2,-3.98998543900001));
#325941=CARTESIAN_POINT('Ctrl Pts',(-0.749779247000056,2.2,-3.98998543900001));
#325942=CARTESIAN_POINT('Ctrl Pts',(-0.749455485000056,12.2,-3.98914035100002));
#325943=CARTESIAN_POINT('Ctrl Pts',(-0.749455485000056,5.2,-3.98914035100002));
#325944=CARTESIAN_POINT('Ctrl Pts',(-0.749455485000056,2.2,-3.98914035100002));
#325945=CARTESIAN_POINT('Ctrl Pts',(-0.749134790000056,12.2,-3.98830014000001));
#325946=CARTESIAN_POINT('Ctrl Pts',(-0.749134790000056,5.2,-3.98830014000001));
#325947=CARTESIAN_POINT('Ctrl Pts',(-0.749134790000056,2.2,-3.98830014000001));
#325948=CARTESIAN_POINT('Ctrl Pts',(-0.748817152000055,12.2,-3.98746481800002));
#325949=CARTESIAN_POINT('Ctrl Pts',(-0.748817152000055,5.2,-3.98746481800002));
#325950=CARTESIAN_POINT('Ctrl Pts',(-0.748817152000055,2.2,-3.98746481800002));
#325951=CARTESIAN_POINT('Ctrl Pts',(-0.748502565000055,12.2,-3.98663440500002));
#325952=CARTESIAN_POINT('Ctrl Pts',(-0.748502565000055,5.2,-3.98663440500002));
#325953=CARTESIAN_POINT('Ctrl Pts',(-0.748502565000055,2.2,-3.98663440500002));
#325954=CARTESIAN_POINT('Ctrl Pts',(-0.748191019000056,12.2,-3.98580891300002));
#325955=CARTESIAN_POINT('Ctrl Pts',(-0.748191019000056,5.2,-3.98580891300002));
#325956=CARTESIAN_POINT('Ctrl Pts',(-0.748191019000056,2.2,-3.98580891300002));
#325957=CARTESIAN_POINT('Ctrl Pts',(-0.747882505000056,12.2,-3.98498835800002));
#325958=CARTESIAN_POINT('Ctrl Pts',(-0.747882505000056,5.2,-3.98498835800002));
#325959=CARTESIAN_POINT('Ctrl Pts',(-0.747882505000056,2.2,-3.98498835800002));
#325960=CARTESIAN_POINT('Ctrl Pts',(-0.747577015000056,12.2,-3.98417275500002));
#325961=CARTESIAN_POINT('Ctrl Pts',(-0.747577015000056,5.2,-3.98417275500002));
#325962=CARTESIAN_POINT('Ctrl Pts',(-0.747577015000056,2.2,-3.98417275500002));
#325963=CARTESIAN_POINT('Ctrl Pts',(-0.747274539000056,12.2,-3.98336212200002));
#325964=CARTESIAN_POINT('Ctrl Pts',(-0.747274539000056,5.2,-3.98336212200002));
#325965=CARTESIAN_POINT('Ctrl Pts',(-0.747274539000056,2.2,-3.98336212200002));
#325966=CARTESIAN_POINT('Ctrl Pts',(-0.746975070000057,12.2,-3.98255647000001));
#325967=CARTESIAN_POINT('Ctrl Pts',(-0.746975070000057,5.2,-3.98255647000001));
#325968=CARTESIAN_POINT('Ctrl Pts',(-0.746975070000057,2.2,-3.98255647000001));
#325969=CARTESIAN_POINT('Ctrl Pts',(-0.746678599000056,12.2,-3.98175581800002));
#325970=CARTESIAN_POINT('Ctrl Pts',(-0.746678599000056,5.2,-3.98175581800002));
#325971=CARTESIAN_POINT('Ctrl Pts',(-0.746678599000056,2.2,-3.98175581800002));
#325972=CARTESIAN_POINT('Ctrl Pts',(-0.746385115000056,12.2,-3.98096018100001));
#325973=CARTESIAN_POINT('Ctrl Pts',(-0.746385115000056,5.2,-3.98096018100001));
#325974=CARTESIAN_POINT('Ctrl Pts',(-0.746385115000056,2.2,-3.98096018100001));
#325975=CARTESIAN_POINT('Ctrl Pts',(-0.746094611000055,12.2,-3.98016957200001));
#325976=CARTESIAN_POINT('Ctrl Pts',(-0.746094611000055,5.2,-3.98016957200001));
#325977=CARTESIAN_POINT('Ctrl Pts',(-0.746094611000055,2.2,-3.98016957200001));
#325978=CARTESIAN_POINT('Ctrl Pts',(-0.745807078000055,12.2,-3.97938401000001));
#325979=CARTESIAN_POINT('Ctrl Pts',(-0.745807078000055,5.2,-3.97938401000001));
#325980=CARTESIAN_POINT('Ctrl Pts',(-0.745807078000055,2.2,-3.97938401000001));
#325981=CARTESIAN_POINT('Ctrl Pts',(-0.745522507000055,12.2,-3.97860350800002));
#325982=CARTESIAN_POINT('Ctrl Pts',(-0.745522507000055,5.2,-3.97860350800002));
#325983=CARTESIAN_POINT('Ctrl Pts',(-0.745522507000055,2.2,-3.97860350800002));
#325984=CARTESIAN_POINT('Ctrl Pts',(-0.745240887000056,12.2,-3.97782808200001));
#325985=CARTESIAN_POINT('Ctrl Pts',(-0.745240887000056,5.2,-3.97782808200001));
#325986=CARTESIAN_POINT('Ctrl Pts',(-0.745240887000056,2.2,-3.97782808200001));
#325987=CARTESIAN_POINT('Ctrl Pts',(-0.744962211000055,12.2,-3.97705774900002));
#325988=CARTESIAN_POINT('Ctrl Pts',(-0.744962211000055,5.2,-3.97705774900002));
#325989=CARTESIAN_POINT('Ctrl Pts',(-0.744962211000055,2.2,-3.97705774900002));
#325990=CARTESIAN_POINT('Ctrl Pts',(-0.744686470000057,12.2,-3.97629252400002));
#325991=CARTESIAN_POINT('Ctrl Pts',(-0.744686470000057,5.2,-3.97629252400002));
#325992=CARTESIAN_POINT('Ctrl Pts',(-0.744686470000057,2.2,-3.97629252400002));
#325993=CARTESIAN_POINT('Ctrl Pts',(-0.744413653000056,12.2,-3.97553242100001));
#325994=CARTESIAN_POINT('Ctrl Pts',(-0.744413653000056,5.2,-3.97553242100001));
#325995=CARTESIAN_POINT('Ctrl Pts',(-0.744413653000056,2.2,-3.97553242100001));
#325996=CARTESIAN_POINT('Ctrl Pts',(-0.744143752000056,12.2,-3.97477745900002));
#325997=CARTESIAN_POINT('Ctrl Pts',(-0.744143752000056,5.2,-3.97477745900002));
#325998=CARTESIAN_POINT('Ctrl Pts',(-0.744143752000056,2.2,-3.97477745900002));
#325999=CARTESIAN_POINT('Ctrl Pts',(-0.743876758000056,12.2,-3.97402765100002));
#326000=CARTESIAN_POINT('Ctrl Pts',(-0.743876758000056,5.2,-3.97402765100002));
#326001=CARTESIAN_POINT('Ctrl Pts',(-0.743876758000056,2.2,-3.97402765100002));
#326002=CARTESIAN_POINT('Ctrl Pts',(-0.743612661000055,12.2,-3.97328301400002));
#326003=CARTESIAN_POINT('Ctrl Pts',(-0.743612661000055,5.2,-3.97328301400002));
#326004=CARTESIAN_POINT('Ctrl Pts',(-0.743612661000055,2.2,-3.97328301400002));
#326005=CARTESIAN_POINT('Ctrl Pts',(-0.743351452000055,12.2,-3.97254356300001));
#326006=CARTESIAN_POINT('Ctrl Pts',(-0.743351452000055,5.2,-3.97254356300001));
#326007=CARTESIAN_POINT('Ctrl Pts',(-0.743351452000055,2.2,-3.97254356300001));
#326008=CARTESIAN_POINT('Ctrl Pts',(-0.743093122000056,12.2,-3.97180931500001));
#326009=CARTESIAN_POINT('Ctrl Pts',(-0.743093122000056,5.2,-3.97180931500001));
#326010=CARTESIAN_POINT('Ctrl Pts',(-0.743093122000056,2.2,-3.97180931500001));
#326011=CARTESIAN_POINT('Ctrl Pts',(-0.742837660000056,12.2,-3.97108028500002));
#326012=CARTESIAN_POINT('Ctrl Pts',(-0.742837660000056,5.2,-3.97108028500002));
#326013=CARTESIAN_POINT('Ctrl Pts',(-0.742837660000056,2.2,-3.97108028500002));
#326014=CARTESIAN_POINT('Ctrl Pts',(-0.742585058000056,12.2,-3.97035649000001));
#326015=CARTESIAN_POINT('Ctrl Pts',(-0.742585058000056,5.2,-3.97035649000001));
#326016=CARTESIAN_POINT('Ctrl Pts',(-0.742585058000056,2.2,-3.97035649000001));
#326017=CARTESIAN_POINT('Ctrl Pts',(-0.742335305000056,12.2,-3.96963794400001));
#326018=CARTESIAN_POINT('Ctrl Pts',(-0.742335305000056,5.2,-3.96963794400001));
#326019=CARTESIAN_POINT('Ctrl Pts',(-0.742335305000056,2.2,-3.96963794400001));
#326020=CARTESIAN_POINT('Ctrl Pts',(-0.742088393000057,12.2,-3.96892466500002));
#326021=CARTESIAN_POINT('Ctrl Pts',(-0.742088393000057,5.2,-3.96892466500002));
#326022=CARTESIAN_POINT('Ctrl Pts',(-0.742088393000057,2.2,-3.96892466500002));
#326023=CARTESIAN_POINT('Ctrl Pts',(-0.741844312000056,12.2,-3.96821666800002));
#326024=CARTESIAN_POINT('Ctrl Pts',(-0.741844312000056,5.2,-3.96821666800002));
#326025=CARTESIAN_POINT('Ctrl Pts',(-0.741844312000056,2.2,-3.96821666800002));
#326026=CARTESIAN_POINT('Ctrl Pts',(-0.741603052000055,12.2,-3.96751396800001));
#326027=CARTESIAN_POINT('Ctrl Pts',(-0.741603052000055,5.2,-3.96751396800001));
#326028=CARTESIAN_POINT('Ctrl Pts',(-0.741603052000055,2.2,-3.96751396800001));
#326029=CARTESIAN_POINT('Ctrl Pts',(-0.741364603000055,12.2,-3.96681658300002));
#326030=CARTESIAN_POINT('Ctrl Pts',(-0.741364603000055,5.2,-3.96681658300002));
#326031=CARTESIAN_POINT('Ctrl Pts',(-0.741364603000055,2.2,-3.96681658300002));
#326032=CARTESIAN_POINT('Ctrl Pts',(-0.741128956000056,12.2,-3.96612452900001));
#326033=CARTESIAN_POINT('Ctrl Pts',(-0.741128956000056,5.2,-3.96612452900001));
#326034=CARTESIAN_POINT('Ctrl Pts',(-0.741128956000056,2.2,-3.96612452900001));
#326035=CARTESIAN_POINT('Ctrl Pts',(-0.740896100000056,12.2,-3.96543782100002));
#326036=CARTESIAN_POINT('Ctrl Pts',(-0.740896100000056,5.2,-3.96543782100002));
#326037=CARTESIAN_POINT('Ctrl Pts',(-0.740896100000056,2.2,-3.96543782100002));
#326038=CARTESIAN_POINT('Ctrl Pts',(-0.740666025000056,12.2,-3.96475647700001));
#326039=CARTESIAN_POINT('Ctrl Pts',(-0.740666025000056,5.2,-3.96475647700001));
#326040=CARTESIAN_POINT('Ctrl Pts',(-0.740666025000056,2.2,-3.96475647700001));
#326041=CARTESIAN_POINT('Ctrl Pts',(-0.740438724000055,12.2,-3.96408051000002));
#326042=CARTESIAN_POINT('Ctrl Pts',(-0.740438724000055,5.2,-3.96408051000002));
#326043=CARTESIAN_POINT('Ctrl Pts',(-0.740438724000055,2.2,-3.96408051000002));
#326044=CARTESIAN_POINT('Ctrl Pts',(-0.740214183000055,12.2,-3.96340994000001));
#326045=CARTESIAN_POINT('Ctrl Pts',(-0.740214183000055,5.2,-3.96340994000001));
#326046=CARTESIAN_POINT('Ctrl Pts',(-0.740214183000055,2.2,-3.96340994000001));
#326047=CARTESIAN_POINT('Ctrl Pts',(-0.739992395000056,12.2,-3.96274478100001));
#326048=CARTESIAN_POINT('Ctrl Pts',(-0.739992395000056,5.2,-3.96274478100001));
#326049=CARTESIAN_POINT('Ctrl Pts',(-0.739992395000056,2.2,-3.96274478100001));
#326050=CARTESIAN_POINT('Ctrl Pts',(-0.739773349000057,12.2,-3.96208504900001));
#326051=CARTESIAN_POINT('Ctrl Pts',(-0.739773349000057,5.2,-3.96208504900001));
#326052=CARTESIAN_POINT('Ctrl Pts',(-0.739773349000057,2.2,-3.96208504900001));
#326053=CARTESIAN_POINT('Ctrl Pts',(-0.739557033000056,12.2,-3.96143076100001));
#326054=CARTESIAN_POINT('Ctrl Pts',(-0.739557033000056,5.2,-3.96143076100001));
#326055=CARTESIAN_POINT('Ctrl Pts',(-0.739557033000056,2.2,-3.96143076100001));
#326056=CARTESIAN_POINT('Ctrl Pts',(-0.739343439000055,12.2,-3.96078193500002));
#326057=CARTESIAN_POINT('Ctrl Pts',(-0.739343439000055,5.2,-3.96078193500002));
#326058=CARTESIAN_POINT('Ctrl Pts',(-0.739343439000055,2.2,-3.96078193500002));
#326059=CARTESIAN_POINT('Ctrl Pts',(-0.739132557000056,12.2,-3.96013858500002));
#326060=CARTESIAN_POINT('Ctrl Pts',(-0.739132557000056,5.2,-3.96013858500002));
#326061=CARTESIAN_POINT('Ctrl Pts',(-0.739132557000056,2.2,-3.96013858500002));
#326062=CARTESIAN_POINT('Ctrl Pts',(-0.738924376000056,12.2,-3.95950072800002));
#326063=CARTESIAN_POINT('Ctrl Pts',(-0.738924376000056,5.2,-3.95950072800002));
#326064=CARTESIAN_POINT('Ctrl Pts',(-0.738924376000056,2.2,-3.95950072800002));
#326065=CARTESIAN_POINT('Ctrl Pts',(-0.738718886000056,12.2,-3.95886838100001));
#326066=CARTESIAN_POINT('Ctrl Pts',(-0.738718886000056,5.2,-3.95886838100001));
#326067=CARTESIAN_POINT('Ctrl Pts',(-0.738718886000056,2.2,-3.95886838100001));
#326068=CARTESIAN_POINT('Ctrl Pts',(-0.738516076000056,12.2,-3.95824156200002));
#326069=CARTESIAN_POINT('Ctrl Pts',(-0.738516076000056,5.2,-3.95824156200002));
#326070=CARTESIAN_POINT('Ctrl Pts',(-0.738516076000056,2.2,-3.95824156200002));
#326071=CARTESIAN_POINT('Ctrl Pts',(-0.738315935000056,12.2,-3.95762028500001));
#326072=CARTESIAN_POINT('Ctrl Pts',(-0.738315935000056,5.2,-3.95762028500001));
#326073=CARTESIAN_POINT('Ctrl Pts',(-0.738315935000056,2.2,-3.95762028500001));
#326074=CARTESIAN_POINT('Ctrl Pts',(-0.738118454000055,12.2,-3.95700456700002));
#326075=CARTESIAN_POINT('Ctrl Pts',(-0.738118454000055,5.2,-3.95700456700002));
#326076=CARTESIAN_POINT('Ctrl Pts',(-0.738118454000055,2.2,-3.95700456700002));
#326077=CARTESIAN_POINT('Ctrl Pts',(-0.737923622000055,12.2,-3.95639442600002));
#326078=CARTESIAN_POINT('Ctrl Pts',(-0.737923622000055,5.2,-3.95639442600002));
#326079=CARTESIAN_POINT('Ctrl Pts',(-0.737923622000055,2.2,-3.95639442600002));
#326080=CARTESIAN_POINT('Ctrl Pts',(-0.737731429000055,12.2,-3.95578987800001));
#326081=CARTESIAN_POINT('Ctrl Pts',(-0.737731429000055,5.2,-3.95578987800001));
#326082=CARTESIAN_POINT('Ctrl Pts',(-0.737731429000055,2.2,-3.95578987800001));
#326083=CARTESIAN_POINT('Ctrl Pts',(-0.737541863000055,12.2,-3.95519093900001));
#326084=CARTESIAN_POINT('Ctrl Pts',(-0.737541863000055,5.2,-3.95519093900001));
#326085=CARTESIAN_POINT('Ctrl Pts',(-0.737541863000055,2.2,-3.95519093900001));
#326086=CARTESIAN_POINT('Ctrl Pts',(-0.737354914000056,12.2,-3.95459762800002));
#326087=CARTESIAN_POINT('Ctrl Pts',(-0.737354914000056,5.2,-3.95459762800002));
#326088=CARTESIAN_POINT('Ctrl Pts',(-0.737354914000056,2.2,-3.95459762800002));
#326089=CARTESIAN_POINT('Ctrl Pts',(-0.737170572000055,12.2,-3.95400995800001));
#326090=CARTESIAN_POINT('Ctrl Pts',(-0.737170572000055,5.2,-3.95400995800001));
#326091=CARTESIAN_POINT('Ctrl Pts',(-0.737170572000055,2.2,-3.95400995800001));
#326092=CARTESIAN_POINT('Ctrl Pts',(-0.736988825000056,12.2,-3.95342795000001));
#326093=CARTESIAN_POINT('Ctrl Pts',(-0.736988825000056,5.2,-3.95342795000001));
#326094=CARTESIAN_POINT('Ctrl Pts',(-0.736988825000056,2.2,-3.95342795000001));
#326095=CARTESIAN_POINT('Ctrl Pts',(-0.736809662000055,12.2,-3.95285161700001));
#326096=CARTESIAN_POINT('Ctrl Pts',(-0.736809662000055,5.2,-3.95285161700001));
#326097=CARTESIAN_POINT('Ctrl Pts',(-0.736809662000055,2.2,-3.95285161700001));
#326098=CARTESIAN_POINT('Ctrl Pts',(-0.736633073000055,12.2,-3.95228097900001));
#326099=CARTESIAN_POINT('Ctrl Pts',(-0.736633073000055,5.2,-3.95228097900001));
#326100=CARTESIAN_POINT('Ctrl Pts',(-0.736633073000055,2.2,-3.95228097900001));
#326101=CARTESIAN_POINT('Ctrl Pts',(-0.736459048000055,12.2,-3.95171605100002));
#326102=CARTESIAN_POINT('Ctrl Pts',(-0.736459048000055,5.2,-3.95171605100002));
#326103=CARTESIAN_POINT('Ctrl Pts',(-0.736459048000055,2.2,-3.95171605100002));
#326104=CARTESIAN_POINT('Ctrl Pts',(-0.736287574000055,12.2,-3.95115685200001));
#326105=CARTESIAN_POINT('Ctrl Pts',(-0.736287574000055,5.2,-3.95115685200001));
#326106=CARTESIAN_POINT('Ctrl Pts',(-0.736287574000055,2.2,-3.95115685200001));
#326107=CARTESIAN_POINT('Ctrl Pts',(-0.736118641000055,12.2,-3.95060339600001));
#326108=CARTESIAN_POINT('Ctrl Pts',(-0.736118641000055,5.2,-3.95060339600001));
#326109=CARTESIAN_POINT('Ctrl Pts',(-0.736118641000055,2.2,-3.95060339600001));
#326110=CARTESIAN_POINT('Ctrl Pts',(-0.735952238000056,12.2,-3.95005570300001));
#326111=CARTESIAN_POINT('Ctrl Pts',(-0.735952238000056,5.2,-3.95005570300001));
#326112=CARTESIAN_POINT('Ctrl Pts',(-0.735952238000056,2.2,-3.95005570300001));
#326113=CARTESIAN_POINT('Ctrl Pts',(-0.735788355000055,12.2,-3.94951378800001));
#326114=CARTESIAN_POINT('Ctrl Pts',(-0.735788355000055,5.2,-3.94951378800001));
#326115=CARTESIAN_POINT('Ctrl Pts',(-0.735788355000055,2.2,-3.94951378800001));
#326116=CARTESIAN_POINT('Ctrl Pts',(-0.735626978000056,12.2,-3.94897766900002));
#326117=CARTESIAN_POINT('Ctrl Pts',(-0.735626978000056,5.2,-3.94897766900002));
#326118=CARTESIAN_POINT('Ctrl Pts',(-0.735626978000056,2.2,-3.94897766900002));
#326119=CARTESIAN_POINT('Ctrl Pts',(-0.735468096000057,12.2,-3.94844736400001));
#326120=CARTESIAN_POINT('Ctrl Pts',(-0.735468096000057,5.2,-3.94844736400001));
#326121=CARTESIAN_POINT('Ctrl Pts',(-0.735468096000057,2.2,-3.94844736400001));
#326122=CARTESIAN_POINT('Ctrl Pts',(-0.735311701000055,12.2,-3.94792288800002));
#326123=CARTESIAN_POINT('Ctrl Pts',(-0.735311701000055,5.2,-3.94792288800002));
#326124=CARTESIAN_POINT('Ctrl Pts',(-0.735311701000055,2.2,-3.94792288800002));
#326125=CARTESIAN_POINT('Ctrl Pts',(-0.735157778000056,12.2,-3.94740426000002));
#326126=CARTESIAN_POINT('Ctrl Pts',(-0.735157778000056,5.2,-3.94740426000002));
#326127=CARTESIAN_POINT('Ctrl Pts',(-0.735157778000056,2.2,-3.94740426000002));
#326128=CARTESIAN_POINT('Ctrl Pts',(-0.735006318000057,12.2,-3.94689149700001));
#326129=CARTESIAN_POINT('Ctrl Pts',(-0.735006318000057,5.2,-3.94689149700001));
#326130=CARTESIAN_POINT('Ctrl Pts',(-0.735006318000057,2.2,-3.94689149700001));
#326131=CARTESIAN_POINT('Ctrl Pts',(-0.734857308000055,12.2,-3.94638461600001));
#326132=CARTESIAN_POINT('Ctrl Pts',(-0.734857308000055,5.2,-3.94638461600001));
#326133=CARTESIAN_POINT('Ctrl Pts',(-0.734857308000055,2.2,-3.94638461600001));
#326134=CARTESIAN_POINT('Ctrl Pts',(-0.734710738000055,12.2,-3.94588363500001));
#326135=CARTESIAN_POINT('Ctrl Pts',(-0.734710738000055,5.2,-3.94588363500001));
#326136=CARTESIAN_POINT('Ctrl Pts',(-0.734710738000055,2.2,-3.94588363500001));
#326137=CARTESIAN_POINT('Ctrl Pts',(-0.734566594000056,12.2,-3.94538857000001));
#326138=CARTESIAN_POINT('Ctrl Pts',(-0.734566594000056,5.2,-3.94538857000001));
#326139=CARTESIAN_POINT('Ctrl Pts',(-0.734566594000056,2.2,-3.94538857000001));
#326140=CARTESIAN_POINT('Ctrl Pts',(-0.734424867000056,12.2,-3.94489944000001));
#326141=CARTESIAN_POINT('Ctrl Pts',(-0.734424867000056,5.2,-3.94489944000001));
#326142=CARTESIAN_POINT('Ctrl Pts',(-0.734424867000056,2.2,-3.94489944000001));
#326143=CARTESIAN_POINT('Ctrl Pts',(-0.734285544000055,12.2,-3.94441626200001));
#326144=CARTESIAN_POINT('Ctrl Pts',(-0.734285544000055,5.2,-3.94441626200001));
#326145=CARTESIAN_POINT('Ctrl Pts',(-0.734285544000055,2.2,-3.94441626200001));
#326146=CARTESIAN_POINT('Ctrl Pts',(-0.734148613000055,12.2,-3.94393905300001));
#326147=CARTESIAN_POINT('Ctrl Pts',(-0.734148613000055,5.2,-3.94393905300001));
#326148=CARTESIAN_POINT('Ctrl Pts',(-0.734148613000055,2.2,-3.94393905300001));
#326149=CARTESIAN_POINT('Ctrl Pts',(-0.734014063000057,12.2,-3.94346783100001));
#326150=CARTESIAN_POINT('Ctrl Pts',(-0.734014063000057,5.2,-3.94346783100001));
#326151=CARTESIAN_POINT('Ctrl Pts',(-0.734014063000057,2.2,-3.94346783100001));
#326152=CARTESIAN_POINT('Ctrl Pts',(-0.733881881000055,12.2,-3.94300261400002));
#326153=CARTESIAN_POINT('Ctrl Pts',(-0.733881881000055,5.2,-3.94300261400002));
#326154=CARTESIAN_POINT('Ctrl Pts',(-0.733881881000055,2.2,-3.94300261400002));
#326155=CARTESIAN_POINT('Ctrl Pts',(-0.733752055000056,12.2,-3.94254341900002));
#326156=CARTESIAN_POINT('Ctrl Pts',(-0.733752055000056,5.2,-3.94254341900002));
#326157=CARTESIAN_POINT('Ctrl Pts',(-0.733752055000056,2.2,-3.94254341900002));
#326158=CARTESIAN_POINT('Ctrl Pts',(-0.733624575000055,12.2,-3.94209026300001));
#326159=CARTESIAN_POINT('Ctrl Pts',(-0.733624575000055,5.2,-3.94209026300001));
#326160=CARTESIAN_POINT('Ctrl Pts',(-0.733624575000055,2.2,-3.94209026300001));
#326161=CARTESIAN_POINT('Ctrl Pts',(-0.733499428000056,12.2,-3.94164316600001));
#326162=CARTESIAN_POINT('Ctrl Pts',(-0.733499428000056,5.2,-3.94164316600001));
#326163=CARTESIAN_POINT('Ctrl Pts',(-0.733499428000056,2.2,-3.94164316600001));
#326164=CARTESIAN_POINT('Ctrl Pts',(-0.733376600000056,12.2,-3.94120214300001));
#326165=CARTESIAN_POINT('Ctrl Pts',(-0.733376600000056,5.2,-3.94120214300001));
#326166=CARTESIAN_POINT('Ctrl Pts',(-0.733376600000056,2.2,-3.94120214300001));
#326167=CARTESIAN_POINT('Ctrl Pts',(-0.733256082000056,12.2,-3.94076721300001));
#326168=CARTESIAN_POINT('Ctrl Pts',(-0.733256082000056,5.2,-3.94076721300001));
#326169=CARTESIAN_POINT('Ctrl Pts',(-0.733256082000056,2.2,-3.94076721300001));
#326170=CARTESIAN_POINT('Ctrl Pts',(-0.733137859000056,12.2,-3.94033839600001));
#326171=CARTESIAN_POINT('Ctrl Pts',(-0.733137859000056,5.2,-3.94033839600001));
#326172=CARTESIAN_POINT('Ctrl Pts',(-0.733137859000056,2.2,-3.94033839600001));
#326173=CARTESIAN_POINT('Ctrl Pts',(-0.733021920000055,12.2,-3.93991570600001));
#326174=CARTESIAN_POINT('Ctrl Pts',(-0.733021920000055,5.2,-3.93991570600001));
#326175=CARTESIAN_POINT('Ctrl Pts',(-0.733021920000055,2.2,-3.93991570600001));
#326176=CARTESIAN_POINT('Ctrl Pts',(-0.732908254000056,12.2,-3.93949916500001));
#326177=CARTESIAN_POINT('Ctrl Pts',(-0.732908254000056,5.2,-3.93949916500001));
#326178=CARTESIAN_POINT('Ctrl Pts',(-0.732908254000056,2.2,-3.93949916500001));
#326179=CARTESIAN_POINT('Ctrl Pts',(-0.732796846000056,12.2,-3.93908878700001));
#326180=CARTESIAN_POINT('Ctrl Pts',(-0.732796846000056,5.2,-3.93908878700001));
#326181=CARTESIAN_POINT('Ctrl Pts',(-0.732796846000056,2.2,-3.93908878700001));
#326182=CARTESIAN_POINT('Ctrl Pts',(-0.732687684000056,12.2,-3.93868459300001));
#326183=CARTESIAN_POINT('Ctrl Pts',(-0.732687684000056,5.2,-3.93868459300001));
#326184=CARTESIAN_POINT('Ctrl Pts',(-0.732687684000056,2.2,-3.93868459300001));
#326185=CARTESIAN_POINT('Ctrl Pts',(-0.732580758000055,12.2,-3.93828659900001));
#326186=CARTESIAN_POINT('Ctrl Pts',(-0.732580758000055,5.2,-3.93828659900001));
#326187=CARTESIAN_POINT('Ctrl Pts',(-0.732580758000055,2.2,-3.93828659900001));
#326188=CARTESIAN_POINT('Ctrl Pts',(-0.732476052000056,12.2,-3.93789482400001));
#326189=CARTESIAN_POINT('Ctrl Pts',(-0.732476052000056,5.2,-3.93789482400001));
#326190=CARTESIAN_POINT('Ctrl Pts',(-0.732476052000056,2.2,-3.93789482400001));
#326191=CARTESIAN_POINT('Ctrl Pts',(-0.732373555000055,12.2,-3.93750928800001));
#326192=CARTESIAN_POINT('Ctrl Pts',(-0.732373555000055,5.2,-3.93750928800001));
#326193=CARTESIAN_POINT('Ctrl Pts',(-0.732373555000055,2.2,-3.93750928800001));
#326194=CARTESIAN_POINT('Ctrl Pts',(-0.732273255000055,12.2,-3.93713000600002));
#326195=CARTESIAN_POINT('Ctrl Pts',(-0.732273255000055,5.2,-3.93713000600002));
#326196=CARTESIAN_POINT('Ctrl Pts',(-0.732273255000055,2.2,-3.93713000600002));
#326197=CARTESIAN_POINT('Ctrl Pts',(-0.732175138000055,12.2,-3.93675699800001));
#326198=CARTESIAN_POINT('Ctrl Pts',(-0.732175138000055,5.2,-3.93675699800001));
#326199=CARTESIAN_POINT('Ctrl Pts',(-0.732175138000055,2.2,-3.93675699800001));
#326200=CARTESIAN_POINT('Ctrl Pts',(-0.732079191000056,12.2,-3.93639028200001));
#326201=CARTESIAN_POINT('Ctrl Pts',(-0.732079191000056,5.2,-3.93639028200001));
#326202=CARTESIAN_POINT('Ctrl Pts',(-0.732079191000056,2.2,-3.93639028200001));
#326203=CARTESIAN_POINT('Ctrl Pts',(-0.731985402000056,12.2,-3.93602987700001));
#326204=CARTESIAN_POINT('Ctrl Pts',(-0.731985402000056,5.2,-3.93602987700001));
#326205=CARTESIAN_POINT('Ctrl Pts',(-0.731985402000056,2.2,-3.93602987700001));
#326206=CARTESIAN_POINT('Ctrl Pts',(-0.731893758000056,12.2,-3.93567580100001));
#326207=CARTESIAN_POINT('Ctrl Pts',(-0.731893758000056,5.2,-3.93567580100001));
#326208=CARTESIAN_POINT('Ctrl Pts',(-0.731893758000056,2.2,-3.93567580100001));
#326209=CARTESIAN_POINT('Ctrl Pts',(-0.731804245000056,12.2,-3.93532807100001));
#326210=CARTESIAN_POINT('Ctrl Pts',(-0.731804245000056,5.2,-3.93532807100001));
#326211=CARTESIAN_POINT('Ctrl Pts',(-0.731804245000056,2.2,-3.93532807100001));
#326212=CARTESIAN_POINT('Ctrl Pts',(-0.731716851000056,12.2,-3.93498670700001));
#326213=CARTESIAN_POINT('Ctrl Pts',(-0.731716851000056,5.2,-3.93498670700001));
#326214=CARTESIAN_POINT('Ctrl Pts',(-0.731716851000056,2.2,-3.93498670700001));
#326215=CARTESIAN_POINT('Ctrl Pts',(-0.731631562000056,12.2,-3.93465172700001));
#326216=CARTESIAN_POINT('Ctrl Pts',(-0.731631562000056,5.2,-3.93465172700001));
#326217=CARTESIAN_POINT('Ctrl Pts',(-0.731631562000056,2.2,-3.93465172700001));
#326218=CARTESIAN_POINT('Ctrl Pts',(-0.731548366000055,12.2,-3.93432315100001));
#326219=CARTESIAN_POINT('Ctrl Pts',(-0.731548366000055,5.2,-3.93432315100001));
#326220=CARTESIAN_POINT('Ctrl Pts',(-0.731548366000055,2.2,-3.93432315100001));
#326221=CARTESIAN_POINT('Ctrl Pts',(-0.731467248000056,12.2,-3.93400099600001));
#326222=CARTESIAN_POINT('Ctrl Pts',(-0.731467248000056,5.2,-3.93400099600001));
#326223=CARTESIAN_POINT('Ctrl Pts',(-0.731467248000056,2.2,-3.93400099600001));
#326224=CARTESIAN_POINT('Ctrl Pts',(-0.731388196000056,12.2,-3.93368528000002));
#326225=CARTESIAN_POINT('Ctrl Pts',(-0.731388196000056,5.2,-3.93368528000002));
#326226=CARTESIAN_POINT('Ctrl Pts',(-0.731388196000056,2.2,-3.93368528000002));
#326227=CARTESIAN_POINT('Ctrl Pts',(-0.731311196000056,12.2,-3.93337602400001));
#326228=CARTESIAN_POINT('Ctrl Pts',(-0.731311196000056,5.2,-3.93337602400001));
#326229=CARTESIAN_POINT('Ctrl Pts',(-0.731311196000056,2.2,-3.93337602400001));
#326230=CARTESIAN_POINT('Ctrl Pts',(-0.731236235000056,12.2,-3.93307324500002));
#326231=CARTESIAN_POINT('Ctrl Pts',(-0.731236235000056,5.2,-3.93307324500002));
#326232=CARTESIAN_POINT('Ctrl Pts',(-0.731236235000056,2.2,-3.93307324500002));
#326233=CARTESIAN_POINT('Ctrl Pts',(-0.731163299000055,12.2,-3.93277696300002));
#326234=CARTESIAN_POINT('Ctrl Pts',(-0.731163299000055,5.2,-3.93277696300002));
#326235=CARTESIAN_POINT('Ctrl Pts',(-0.731163299000055,2.2,-3.93277696300002));
#326236=CARTESIAN_POINT('Ctrl Pts',(-0.731092374000056,12.2,-3.93248719600002));
#326237=CARTESIAN_POINT('Ctrl Pts',(-0.731092374000056,5.2,-3.93248719600002));
#326238=CARTESIAN_POINT('Ctrl Pts',(-0.731092374000056,2.2,-3.93248719600002));
#326239=CARTESIAN_POINT('Ctrl Pts',(-0.731023446000056,12.2,-3.93220396300002));
#326240=CARTESIAN_POINT('Ctrl Pts',(-0.731023446000056,5.2,-3.93220396300002));
#326241=CARTESIAN_POINT('Ctrl Pts',(-0.731023446000056,2.2,-3.93220396300002));
#326242=CARTESIAN_POINT('Ctrl Pts',(-0.730956503000056,12.2,-3.93192728300002));
#326243=CARTESIAN_POINT('Ctrl Pts',(-0.730956503000056,5.2,-3.93192728300002));
#326244=CARTESIAN_POINT('Ctrl Pts',(-0.730956503000056,2.2,-3.93192728300002));
#326245=CARTESIAN_POINT('Ctrl Pts',(-0.730891530000056,12.2,-3.93165717500001));
#326246=CARTESIAN_POINT('Ctrl Pts',(-0.730891530000056,5.2,-3.93165717500001));
#326247=CARTESIAN_POINT('Ctrl Pts',(-0.730891530000056,2.2,-3.93165717500001));
#326248=CARTESIAN_POINT('Ctrl Pts',(-0.730828514000056,12.2,-3.93139365900002));
#326249=CARTESIAN_POINT('Ctrl Pts',(-0.730828514000056,5.2,-3.93139365900002));
#326250=CARTESIAN_POINT('Ctrl Pts',(-0.730828514000056,2.2,-3.93139365900002));
#326251=CARTESIAN_POINT('Ctrl Pts',(-0.730767439000056,12.2,-3.93113675200001));
#326252=CARTESIAN_POINT('Ctrl Pts',(-0.730767439000056,5.2,-3.93113675200001));
#326253=CARTESIAN_POINT('Ctrl Pts',(-0.730767439000056,2.2,-3.93113675200001));
#326254=CARTESIAN_POINT('Ctrl Pts',(-0.730708292000056,12.2,-3.93088647600001));
#326255=CARTESIAN_POINT('Ctrl Pts',(-0.730708292000056,5.2,-3.93088647600001));
#326256=CARTESIAN_POINT('Ctrl Pts',(-0.730708292000056,2.2,-3.93088647600001));
#326257=CARTESIAN_POINT('Ctrl Pts',(-0.730651060000056,12.2,-3.93064284800001));
#326258=CARTESIAN_POINT('Ctrl Pts',(-0.730651060000056,5.2,-3.93064284800001));
#326259=CARTESIAN_POINT('Ctrl Pts',(-0.730651060000056,2.2,-3.93064284800001));
#326260=CARTESIAN_POINT('Ctrl Pts',(-0.730595727000055,12.2,-3.93040588800002));
#326261=CARTESIAN_POINT('Ctrl Pts',(-0.730595727000055,5.2,-3.93040588800002));
#326262=CARTESIAN_POINT('Ctrl Pts',(-0.730595727000055,2.2,-3.93040588800002));
#326263=CARTESIAN_POINT('Ctrl Pts',(-0.730542281000056,12.2,-3.93017561500002));
#326264=CARTESIAN_POINT('Ctrl Pts',(-0.730542281000056,5.2,-3.93017561500002));
#326265=CARTESIAN_POINT('Ctrl Pts',(-0.730542281000056,2.2,-3.93017561500002));
#326266=CARTESIAN_POINT('Ctrl Pts',(-0.730490706000057,12.2,-3.92995204900001));
#326267=CARTESIAN_POINT('Ctrl Pts',(-0.730490706000057,5.2,-3.92995204900001));
#326268=CARTESIAN_POINT('Ctrl Pts',(-0.730490706000057,2.2,-3.92995204900001));
#326269=CARTESIAN_POINT('Ctrl Pts',(-0.730440988000056,12.2,-3.92973520900001));
#326270=CARTESIAN_POINT('Ctrl Pts',(-0.730440988000056,5.2,-3.92973520900001));
#326271=CARTESIAN_POINT('Ctrl Pts',(-0.730440988000056,2.2,-3.92973520900001));
#326272=CARTESIAN_POINT('Ctrl Pts',(-0.730393113000056,12.2,-3.92952511400001));
#326273=CARTESIAN_POINT('Ctrl Pts',(-0.730393113000056,5.2,-3.92952511400001));
#326274=CARTESIAN_POINT('Ctrl Pts',(-0.730393113000056,2.2,-3.92952511400001));
#326275=CARTESIAN_POINT('Ctrl Pts',(-0.730347066000056,12.2,-3.92932178500002));
#326276=CARTESIAN_POINT('Ctrl Pts',(-0.730347066000056,5.2,-3.92932178500002));
#326277=CARTESIAN_POINT('Ctrl Pts',(-0.730347066000056,2.2,-3.92932178500002));
#326278=CARTESIAN_POINT('Ctrl Pts',(-0.730302831000056,12.2,-3.92912523900002));
#326279=CARTESIAN_POINT('Ctrl Pts',(-0.730302831000056,5.2,-3.92912523900002));
#326280=CARTESIAN_POINT('Ctrl Pts',(-0.730302831000056,2.2,-3.92912523900002));
#326281=CARTESIAN_POINT('Ctrl Pts',(-0.730260396000055,12.2,-3.92893549900001));
#326282=CARTESIAN_POINT('Ctrl Pts',(-0.730260396000055,5.2,-3.92893549900001));
#326283=CARTESIAN_POINT('Ctrl Pts',(-0.730260396000055,2.2,-3.92893549900001));
#326284=CARTESIAN_POINT('Ctrl Pts',(-0.730219745000056,12.2,-3.92875258300001));
#326285=CARTESIAN_POINT('Ctrl Pts',(-0.730219745000056,5.2,-3.92875258300001));
#326286=CARTESIAN_POINT('Ctrl Pts',(-0.730219745000056,2.2,-3.92875258300001));
#326287=CARTESIAN_POINT('Ctrl Pts',(-0.730180862000056,12.2,-3.92857651100002));
#326288=CARTESIAN_POINT('Ctrl Pts',(-0.730180862000056,5.2,-3.92857651100002));
#326289=CARTESIAN_POINT('Ctrl Pts',(-0.730180862000056,2.2,-3.92857651100002));
#326290=CARTESIAN_POINT('Ctrl Pts',(-0.730143733000055,12.2,-3.92840730200001));
#326291=CARTESIAN_POINT('Ctrl Pts',(-0.730143733000055,5.2,-3.92840730200001));
#326292=CARTESIAN_POINT('Ctrl Pts',(-0.730143733000055,2.2,-3.92840730200001));
#326293=CARTESIAN_POINT('Ctrl Pts',(-0.730108344000057,12.2,-3.92824497500001));
#326294=CARTESIAN_POINT('Ctrl Pts',(-0.730108344000057,5.2,-3.92824497500001));
#326295=CARTESIAN_POINT('Ctrl Pts',(-0.730108344000057,2.2,-3.92824497500001));
#326296=CARTESIAN_POINT('Ctrl Pts',(-0.730074682000056,12.2,-3.92808955100001));
#326297=CARTESIAN_POINT('Ctrl Pts',(-0.730074682000056,5.2,-3.92808955100001));
#326298=CARTESIAN_POINT('Ctrl Pts',(-0.730074682000056,2.2,-3.92808955100001));
#326299=CARTESIAN_POINT('Ctrl Pts',(-0.730042727000055,12.2,-3.92794104900001));
#326300=CARTESIAN_POINT('Ctrl Pts',(-0.730042727000055,5.2,-3.92794104900001));
#326301=CARTESIAN_POINT('Ctrl Pts',(-0.730042727000055,2.2,-3.92794104900001));
#326302=CARTESIAN_POINT('Ctrl Pts',(-0.730012467000056,12.2,-3.92779949100001));
#326303=CARTESIAN_POINT('Ctrl Pts',(-0.730012467000056,5.2,-3.92779949100001));
#326304=CARTESIAN_POINT('Ctrl Pts',(-0.730012467000056,2.2,-3.92779949100001));
#326305=CARTESIAN_POINT('Ctrl Pts',(-0.729983883000056,12.2,-3.92766489800001));
#326306=CARTESIAN_POINT('Ctrl Pts',(-0.729983883000056,5.2,-3.92766489800001));
#326307=CARTESIAN_POINT('Ctrl Pts',(-0.729983883000056,2.2,-3.92766489800001));
#326308=CARTESIAN_POINT('Ctrl Pts',(-0.729956962000056,12.2,-3.92753729100002));
#326309=CARTESIAN_POINT('Ctrl Pts',(-0.729956962000056,5.2,-3.92753729100002));
#326310=CARTESIAN_POINT('Ctrl Pts',(-0.729956962000056,2.2,-3.92753729100002));
#326311=CARTESIAN_POINT('Ctrl Pts',(-0.729931687000055,12.2,-3.92741668800001));
#326312=CARTESIAN_POINT('Ctrl Pts',(-0.729931687000055,5.2,-3.92741668800001));
#326313=CARTESIAN_POINT('Ctrl Pts',(-0.729931687000055,2.2,-3.92741668800001));
#326314=CARTESIAN_POINT('Ctrl Pts',(-0.729908045000055,12.2,-3.92730311000001));
#326315=CARTESIAN_POINT('Ctrl Pts',(-0.729908045000055,5.2,-3.92730311000001));
#326316=CARTESIAN_POINT('Ctrl Pts',(-0.729908045000055,2.2,-3.92730311000001));
#326317=CARTESIAN_POINT('Ctrl Pts',(-0.729886021000056,12.2,-3.92719657100002));
#326318=CARTESIAN_POINT('Ctrl Pts',(-0.729886021000056,5.2,-3.92719657100002));
#326319=CARTESIAN_POINT('Ctrl Pts',(-0.729886021000056,2.2,-3.92719657100002));
#326320=CARTESIAN_POINT('Ctrl Pts',(-0.729865602000055,12.2,-3.92709709300001));
#326321=CARTESIAN_POINT('Ctrl Pts',(-0.729865602000055,5.2,-3.92709709300001));
#326322=CARTESIAN_POINT('Ctrl Pts',(-0.729865602000055,2.2,-3.92709709300001));
#326323=CARTESIAN_POINT('Ctrl Pts',(-0.729846772000055,12.2,-3.92700469600001));
#326324=CARTESIAN_POINT('Ctrl Pts',(-0.729846772000055,5.2,-3.92700469600001));
#326325=CARTESIAN_POINT('Ctrl Pts',(-0.729846772000055,2.2,-3.92700469600001));
#326326=CARTESIAN_POINT('Ctrl Pts',(-0.729829512000055,12.2,-3.92691940300002));
#326327=CARTESIAN_POINT('Ctrl Pts',(-0.729829512000055,5.2,-3.92691940300002));
#326328=CARTESIAN_POINT('Ctrl Pts',(-0.729829512000055,2.2,-3.92691940300002));
#326329=CARTESIAN_POINT('Ctrl Pts',(-0.729813802000056,12.2,-3.92684124000001));
#326330=CARTESIAN_POINT('Ctrl Pts',(-0.729813802000056,5.2,-3.92684124000001));
#326331=CARTESIAN_POINT('Ctrl Pts',(-0.729813802000056,2.2,-3.92684124000001));
#326332=CARTESIAN_POINT('Ctrl Pts',(-0.729799621000057,12.2,-3.92677023400001));
#326333=CARTESIAN_POINT('Ctrl Pts',(-0.729799621000057,5.2,-3.92677023400001));
#326334=CARTESIAN_POINT('Ctrl Pts',(-0.729799621000057,2.2,-3.92677023400001));
#326335=CARTESIAN_POINT('Ctrl Pts',(-0.729786954000057,12.2,-3.92670640600001));
#326336=CARTESIAN_POINT('Ctrl Pts',(-0.729786954000057,5.2,-3.92670640600001));
#326337=CARTESIAN_POINT('Ctrl Pts',(-0.729786954000057,2.2,-3.92670640600001));
#326338=CARTESIAN_POINT('Ctrl Pts',(-0.729775786000056,12.2,-3.92664977400001));
#326339=CARTESIAN_POINT('Ctrl Pts',(-0.729775786000056,5.2,-3.92664977400001));
#326340=CARTESIAN_POINT('Ctrl Pts',(-0.729775786000056,2.2,-3.92664977400001));
#326341=CARTESIAN_POINT('Ctrl Pts',(-0.729765073038284,12.2,-3.92659505674791));
#326342=CARTESIAN_POINT('Ctrl Pts',(-0.729765073038284,5.2,-3.92659505674791));
#326343=CARTESIAN_POINT('Ctrl Pts',(-0.729765073038284,2.2,-3.92659505674791));
#326344=CARTESIAN_POINT('Ctrl Pts',(-0.729757824757594,12.2,-3.92655763816102));
#326345=CARTESIAN_POINT('Ctrl Pts',(-0.729757824757594,5.2,-3.92655763816102));
#326346=CARTESIAN_POINT('Ctrl Pts',(-0.729757824757594,2.2,-3.92655763816102));
#326347=CARTESIAN_POINT('Ctrl Pts',(-0.729753103670104,12.2,-3.92653297916544));
#326348=CARTESIAN_POINT('Ctrl Pts',(-0.729753103670104,5.2,-3.92653297916544));
#326349=CARTESIAN_POINT('Ctrl Pts',(-0.729753103670104,2.2,-3.92653297916544));
#326350=CARTESIAN_POINT('Ctrl Pts',(-0.729750197519061,12.2,-3.92651761063945));
#326351=CARTESIAN_POINT('Ctrl Pts',(-0.729750197519061,5.2,-3.92651761063945));
#326352=CARTESIAN_POINT('Ctrl Pts',(-0.729750197519061,2.2,-3.92651761063945));
#326353=CARTESIAN_POINT('Ctrl Pts',(-0.729748397000056,12.2,-3.92650812200001));
#326354=CARTESIAN_POINT('Ctrl Pts',(-0.729748397000056,5.2,-3.92650812200001));
#326355=CARTESIAN_POINT('Ctrl Pts',(-0.729748397000056,2.2,-3.92650812200001));
#326356=CARTESIAN_POINT('',(-0.729748200000057,2.7,-3.92650816000002));
#326357=CARTESIAN_POINT('',(-0.729748200000057,12.2,-3.92650816000002));
#326358=CARTESIAN_POINT('Ctrl Pts',(-1.20083826600006,2.7,-4.59570315100001));
#326359=CARTESIAN_POINT('Ctrl Pts',(-0.99159571956929,2.7,-4.40343391106789));
#326360=CARTESIAN_POINT('Ctrl Pts',(-0.884170970210799,2.69999999999769,
-4.24256418392735));
#326361=CARTESIAN_POINT('Ctrl Pts',(-0.752547076732114,2.69999999999769,
-4.02218548569631));
#326362=CARTESIAN_POINT('Ctrl Pts',(-0.732215363126463,2.69999999999824,
-3.93874877259718));
#326363=CARTESIAN_POINT('Ctrl Pts',(-0.729801785768923,2.69999999999824,
-3.92678179258076));
#326364=CARTESIAN_POINT('Ctrl Pts',(-0.729774387723865,2.7,-3.92664509173279));
#326365=CARTESIAN_POINT('Ctrl Pts',(-0.729748397000056,2.7,-3.92650812200001));
#326366=CARTESIAN_POINT('Origin',(-0.729738823000057,15.2,-3.92645770700002));
#326367=CARTESIAN_POINT('',(-0.662370095000057,2.7,-3.56397122000002));
#326368=CARTESIAN_POINT('',(-0.662370095000057,2.2,-3.56397122000002));
#326369=CARTESIAN_POINT('',(-0.364869411202236,2.7,-1.96322885355537));
#326370=CARTESIAN_POINT('Origin',(-5.66300478732629E-14,15.2,-1.77635683940025E-14));
#326371=CARTESIAN_POINT('',(-0.104256396000055,2.7,-3.62350046200001));
#326372=CARTESIAN_POINT('',(-0.104256396000055,12.2,-3.62350046200001));
#326373=CARTESIAN_POINT('Origin',(-5.66300478732629E-14,2.7,-1.92943768261394E-14));
#326374=CARTESIAN_POINT('Origin',(-5.66300478732629E-14,15.2,-1.77635683940025E-14));
#326375=CARTESIAN_POINT('',(-0.114861152000056,2.7,-3.99207578300001));
#326376=CARTESIAN_POINT('',(-0.114861152000056,12.2,-3.99207578300001));
#326377=CARTESIAN_POINT('',(-5.66071634909361E-14,2.7,-1.84990148774464E-14));
#326378=CARTESIAN_POINT('Ctrl Pts',(-0.114861015000055,12.2,-3.99207578600001));
#326379=CARTESIAN_POINT('Ctrl Pts',(-0.114861015000055,5.2,-3.99207578600001));
#326380=CARTESIAN_POINT('Ctrl Pts',(-0.114861015000055,2.2,-3.99207578600001));
#326381=CARTESIAN_POINT('Ctrl Pts',(-0.114861185985858,12.2,-3.99208262642898));
#326382=CARTESIAN_POINT('Ctrl Pts',(-0.114861185985858,5.2,-3.99208262642898));
#326383=CARTESIAN_POINT('Ctrl Pts',(-0.114861185985858,2.2,-3.99208262642898));
#326384=CARTESIAN_POINT('Ctrl Pts',(-0.114861514799149,12.2,-3.99209585439877));
#326385=CARTESIAN_POINT('Ctrl Pts',(-0.114861514799149,5.2,-3.99209585439877));
#326386=CARTESIAN_POINT('Ctrl Pts',(-0.114861514799149,2.2,-3.99209585439877));
#326387=CARTESIAN_POINT('Ctrl Pts',(-0.11486200797077,12.2,-3.99211547674708));
#326388=CARTESIAN_POINT('Ctrl Pts',(-0.11486200797077,5.2,-3.99211547674708));
#326389=CARTESIAN_POINT('Ctrl Pts',(-0.11486200797077,2.2,-3.99211547674708));
#326390=CARTESIAN_POINT('Ctrl Pts',(-0.114862630472375,12.2,-3.99214150063735));
#326391=CARTESIAN_POINT('Ctrl Pts',(-0.114862630472375,5.2,-3.99214150063735));
#326392=CARTESIAN_POINT('Ctrl Pts',(-0.114862630472375,2.2,-3.99214150063735));
#326393=CARTESIAN_POINT('Ctrl Pts',(-0.114863582000057,12.2,-3.99218677200002));
#326394=CARTESIAN_POINT('Ctrl Pts',(-0.114863582000057,5.2,-3.99218677200002));
#326395=CARTESIAN_POINT('Ctrl Pts',(-0.114863582000057,2.2,-3.99218677200002));
#326396=CARTESIAN_POINT('Ctrl Pts',(-0.114864547000056,12.2,-3.99223712800001));
#326397=CARTESIAN_POINT('Ctrl Pts',(-0.114864547000056,5.2,-3.99223712800001));
#326398=CARTESIAN_POINT('Ctrl Pts',(-0.114864547000056,2.2,-3.99223712800001));
#326399=CARTESIAN_POINT('Ctrl Pts',(-0.114865575000056,12.2,-3.99229484100001));
#326400=CARTESIAN_POINT('Ctrl Pts',(-0.114865575000056,5.2,-3.99229484100001));
#326401=CARTESIAN_POINT('Ctrl Pts',(-0.114865575000056,2.2,-3.99229484100001));
#326402=CARTESIAN_POINT('Ctrl Pts',(-0.114866656000056,12.2,-3.99235990500001));
#326403=CARTESIAN_POINT('Ctrl Pts',(-0.114866656000056,5.2,-3.99235990500001));
#326404=CARTESIAN_POINT('Ctrl Pts',(-0.114866656000056,2.2,-3.99235990500001));
#326405=CARTESIAN_POINT('Ctrl Pts',(-0.114867771000055,12.2,-3.99243230500002));
#326406=CARTESIAN_POINT('Ctrl Pts',(-0.114867771000055,5.2,-3.99243230500002));
#326407=CARTESIAN_POINT('Ctrl Pts',(-0.114867771000055,2.2,-3.99243230500002));
#326408=CARTESIAN_POINT('Ctrl Pts',(-0.114868901000056,12.2,-3.99251202200002));
#326409=CARTESIAN_POINT('Ctrl Pts',(-0.114868901000056,5.2,-3.99251202200002));
#326410=CARTESIAN_POINT('Ctrl Pts',(-0.114868901000056,2.2,-3.99251202200002));
#326411=CARTESIAN_POINT('Ctrl Pts',(-0.114870019000056,12.2,-3.99259903700001));
#326412=CARTESIAN_POINT('Ctrl Pts',(-0.114870019000056,5.2,-3.99259903700001));
#326413=CARTESIAN_POINT('Ctrl Pts',(-0.114870019000056,2.2,-3.99259903700001));
#326414=CARTESIAN_POINT('Ctrl Pts',(-0.114871102000055,12.2,-3.99269332800001));
#326415=CARTESIAN_POINT('Ctrl Pts',(-0.114871102000055,5.2,-3.99269332800001));
#326416=CARTESIAN_POINT('Ctrl Pts',(-0.114871102000055,2.2,-3.99269332800001));
#326417=CARTESIAN_POINT('Ctrl Pts',(-0.114872125000056,12.2,-3.99279487500001));
#326418=CARTESIAN_POINT('Ctrl Pts',(-0.114872125000056,5.2,-3.99279487500001));
#326419=CARTESIAN_POINT('Ctrl Pts',(-0.114872125000056,2.2,-3.99279487500001));
#326420=CARTESIAN_POINT('Ctrl Pts',(-0.114873067000056,12.2,-3.99290366100002));
#326421=CARTESIAN_POINT('Ctrl Pts',(-0.114873067000056,5.2,-3.99290366100002));
#326422=CARTESIAN_POINT('Ctrl Pts',(-0.114873067000056,2.2,-3.99290366100002));
#326423=CARTESIAN_POINT('Ctrl Pts',(-0.114873913000055,12.2,-3.99301967100001));
#326424=CARTESIAN_POINT('Ctrl Pts',(-0.114873913000055,5.2,-3.99301967100001));
#326425=CARTESIAN_POINT('Ctrl Pts',(-0.114873913000055,2.2,-3.99301967100001));
#326426=CARTESIAN_POINT('Ctrl Pts',(-0.114874646000055,12.2,-3.99314289200001));
#326427=CARTESIAN_POINT('Ctrl Pts',(-0.114874646000055,5.2,-3.99314289200001));
#326428=CARTESIAN_POINT('Ctrl Pts',(-0.114874646000055,2.2,-3.99314289200001));
#326429=CARTESIAN_POINT('Ctrl Pts',(-0.114875245000056,12.2,-3.99327330700002));
#326430=CARTESIAN_POINT('Ctrl Pts',(-0.114875245000056,5.2,-3.99327330700002));
#326431=CARTESIAN_POINT('Ctrl Pts',(-0.114875245000056,2.2,-3.99327330700002));
#326432=CARTESIAN_POINT('Ctrl Pts',(-0.114875694000055,12.2,-3.99341090000001));
#326433=CARTESIAN_POINT('Ctrl Pts',(-0.114875694000055,5.2,-3.99341090000001));
#326434=CARTESIAN_POINT('Ctrl Pts',(-0.114875694000055,2.2,-3.99341090000001));
#326435=CARTESIAN_POINT('Ctrl Pts',(-0.114875972000055,12.2,-3.99355565600001));
#326436=CARTESIAN_POINT('Ctrl Pts',(-0.114875972000055,5.2,-3.99355565600001));
#326437=CARTESIAN_POINT('Ctrl Pts',(-0.114875972000055,2.2,-3.99355565600001));
#326438=CARTESIAN_POINT('Ctrl Pts',(-0.114876059000055,12.2,-3.99370755700001));
#326439=CARTESIAN_POINT('Ctrl Pts',(-0.114876059000055,5.2,-3.99370755700001));
#326440=CARTESIAN_POINT('Ctrl Pts',(-0.114876059000055,2.2,-3.99370755700001));
#326441=CARTESIAN_POINT('Ctrl Pts',(-0.114875936000055,12.2,-3.99386658500001));
#326442=CARTESIAN_POINT('Ctrl Pts',(-0.114875936000055,5.2,-3.99386658500001));
#326443=CARTESIAN_POINT('Ctrl Pts',(-0.114875936000055,2.2,-3.99386658500001));
#326444=CARTESIAN_POINT('Ctrl Pts',(-0.114875582000057,12.2,-3.99403272400002));
#326445=CARTESIAN_POINT('Ctrl Pts',(-0.114875582000057,5.2,-3.99403272400002));
#326446=CARTESIAN_POINT('Ctrl Pts',(-0.114875582000057,2.2,-3.99403272400002));
#326447=CARTESIAN_POINT('Ctrl Pts',(-0.114874979000056,12.2,-3.99420595800001));
#326448=CARTESIAN_POINT('Ctrl Pts',(-0.114874979000056,5.2,-3.99420595800001));
#326449=CARTESIAN_POINT('Ctrl Pts',(-0.114874979000056,2.2,-3.99420595800001));
#326450=CARTESIAN_POINT('Ctrl Pts',(-0.114874109000055,12.2,-3.99438627000002));
#326451=CARTESIAN_POINT('Ctrl Pts',(-0.114874109000055,5.2,-3.99438627000002));
#326452=CARTESIAN_POINT('Ctrl Pts',(-0.114874109000055,2.2,-3.99438627000002));
#326453=CARTESIAN_POINT('Ctrl Pts',(-0.114872952000056,12.2,-3.99457364500002));
#326454=CARTESIAN_POINT('Ctrl Pts',(-0.114872952000056,5.2,-3.99457364500002));
#326455=CARTESIAN_POINT('Ctrl Pts',(-0.114872952000056,2.2,-3.99457364500002));
#326456=CARTESIAN_POINT('Ctrl Pts',(-0.114871493000056,12.2,-3.99476806800001));
#326457=CARTESIAN_POINT('Ctrl Pts',(-0.114871493000056,5.2,-3.99476806800001));
#326458=CARTESIAN_POINT('Ctrl Pts',(-0.114871493000056,2.2,-3.99476806800001));
#326459=CARTESIAN_POINT('Ctrl Pts',(-0.114869709000055,12.2,-3.99496952100002));
#326460=CARTESIAN_POINT('Ctrl Pts',(-0.114869709000055,5.2,-3.99496952100002));
#326461=CARTESIAN_POINT('Ctrl Pts',(-0.114869709000055,2.2,-3.99496952100002));
#326462=CARTESIAN_POINT('Ctrl Pts',(-0.114867585000056,12.2,-3.99517798800002));
#326463=CARTESIAN_POINT('Ctrl Pts',(-0.114867585000056,5.2,-3.99517798800002));
#326464=CARTESIAN_POINT('Ctrl Pts',(-0.114867585000056,2.2,-3.99517798800002));
#326465=CARTESIAN_POINT('Ctrl Pts',(-0.114865100000056,12.2,-3.99539345500001));
#326466=CARTESIAN_POINT('Ctrl Pts',(-0.114865100000056,5.2,-3.99539345500001));
#326467=CARTESIAN_POINT('Ctrl Pts',(-0.114865100000056,2.2,-3.99539345500001));
#326468=CARTESIAN_POINT('Ctrl Pts',(-0.114862238000055,12.2,-3.99561590300001));
#326469=CARTESIAN_POINT('Ctrl Pts',(-0.114862238000055,5.2,-3.99561590300001));
#326470=CARTESIAN_POINT('Ctrl Pts',(-0.114862238000055,2.2,-3.99561590300001));
#326471=CARTESIAN_POINT('Ctrl Pts',(-0.114858978000055,12.2,-3.99584531900001));
#326472=CARTESIAN_POINT('Ctrl Pts',(-0.114858978000055,5.2,-3.99584531900001));
#326473=CARTESIAN_POINT('Ctrl Pts',(-0.114858978000055,2.2,-3.99584531900001));
#326474=CARTESIAN_POINT('Ctrl Pts',(-0.114855304000056,12.2,-3.99608168400002));
#326475=CARTESIAN_POINT('Ctrl Pts',(-0.114855304000056,5.2,-3.99608168400002));
#326476=CARTESIAN_POINT('Ctrl Pts',(-0.114855304000056,2.2,-3.99608168400002));
#326477=CARTESIAN_POINT('Ctrl Pts',(-0.114851197000055,12.2,-3.99632498400001));
#326478=CARTESIAN_POINT('Ctrl Pts',(-0.114851197000055,5.2,-3.99632498400001));
#326479=CARTESIAN_POINT('Ctrl Pts',(-0.114851197000055,2.2,-3.99632498400001));
#326480=CARTESIAN_POINT('Ctrl Pts',(-0.114846640000056,12.2,-3.99657520200002));
#326481=CARTESIAN_POINT('Ctrl Pts',(-0.114846640000056,5.2,-3.99657520200002));
#326482=CARTESIAN_POINT('Ctrl Pts',(-0.114846640000056,2.2,-3.99657520200002));
#326483=CARTESIAN_POINT('Ctrl Pts',(-0.114841613000056,12.2,-3.99683232300001));
#326484=CARTESIAN_POINT('Ctrl Pts',(-0.114841613000056,5.2,-3.99683232300001));
#326485=CARTESIAN_POINT('Ctrl Pts',(-0.114841613000056,2.2,-3.99683232300001));
#326486=CARTESIAN_POINT('Ctrl Pts',(-0.114836100000056,12.2,-3.99709633200001));
#326487=CARTESIAN_POINT('Ctrl Pts',(-0.114836100000056,5.2,-3.99709633200001));
#326488=CARTESIAN_POINT('Ctrl Pts',(-0.114836100000056,2.2,-3.99709633200001));
#326489=CARTESIAN_POINT('Ctrl Pts',(-0.114830082000056,12.2,-3.99736721100002));
#326490=CARTESIAN_POINT('Ctrl Pts',(-0.114830082000056,5.2,-3.99736721100002));
#326491=CARTESIAN_POINT('Ctrl Pts',(-0.114830082000056,2.2,-3.99736721100002));
#326492=CARTESIAN_POINT('Ctrl Pts',(-0.114823543000057,12.2,-3.99764494700001));
#326493=CARTESIAN_POINT('Ctrl Pts',(-0.114823543000057,5.2,-3.99764494700001));
#326494=CARTESIAN_POINT('Ctrl Pts',(-0.114823543000057,2.2,-3.99764494700001));
#326495=CARTESIAN_POINT('Ctrl Pts',(-0.114816464000055,12.2,-3.99792952200002));
#326496=CARTESIAN_POINT('Ctrl Pts',(-0.114816464000055,5.2,-3.99792952200002));
#326497=CARTESIAN_POINT('Ctrl Pts',(-0.114816464000055,2.2,-3.99792952200002));
#326498=CARTESIAN_POINT('Ctrl Pts',(-0.114808828000056,12.2,-3.99822092200001));
#326499=CARTESIAN_POINT('Ctrl Pts',(-0.114808828000056,5.2,-3.99822092200001));
#326500=CARTESIAN_POINT('Ctrl Pts',(-0.114808828000056,2.2,-3.99822092200001));
#326501=CARTESIAN_POINT('Ctrl Pts',(-0.114800617000055,12.2,-3.99851912900001));
#326502=CARTESIAN_POINT('Ctrl Pts',(-0.114800617000055,5.2,-3.99851912900001));
#326503=CARTESIAN_POINT('Ctrl Pts',(-0.114800617000055,2.2,-3.99851912900001));
#326504=CARTESIAN_POINT('Ctrl Pts',(-0.114791815000055,12.2,-3.99882413000002));
#326505=CARTESIAN_POINT('Ctrl Pts',(-0.114791815000055,5.2,-3.99882413000002));
#326506=CARTESIAN_POINT('Ctrl Pts',(-0.114791815000055,2.2,-3.99882413000002));
#326507=CARTESIAN_POINT('Ctrl Pts',(-0.114782402000057,12.2,-3.99913590800002));
#326508=CARTESIAN_POINT('Ctrl Pts',(-0.114782402000057,5.2,-3.99913590800002));
#326509=CARTESIAN_POINT('Ctrl Pts',(-0.114782402000057,2.2,-3.99913590800002));
#326510=CARTESIAN_POINT('Ctrl Pts',(-0.114772364000055,12.2,-3.99945444800001));
#326511=CARTESIAN_POINT('Ctrl Pts',(-0.114772364000055,5.2,-3.99945444800001));
#326512=CARTESIAN_POINT('Ctrl Pts',(-0.114772364000055,2.2,-3.99945444800001));
#326513=CARTESIAN_POINT('Ctrl Pts',(-0.114761683000056,12.2,-3.99977973400001));
#326514=CARTESIAN_POINT('Ctrl Pts',(-0.114761683000056,5.2,-3.99977973400001));
#326515=CARTESIAN_POINT('Ctrl Pts',(-0.114761683000056,2.2,-3.99977973400001));
#326516=CARTESIAN_POINT('Ctrl Pts',(-0.114750340000055,12.2,-4.00011175100001));
#326517=CARTESIAN_POINT('Ctrl Pts',(-0.114750340000055,5.2,-4.00011175100001));
#326518=CARTESIAN_POINT('Ctrl Pts',(-0.114750340000055,2.2,-4.00011175100001));
#326519=CARTESIAN_POINT('Ctrl Pts',(-0.114738319000055,12.2,-4.00045048400001));
#326520=CARTESIAN_POINT('Ctrl Pts',(-0.114738319000055,5.2,-4.00045048400001));
#326521=CARTESIAN_POINT('Ctrl Pts',(-0.114738319000055,2.2,-4.00045048400001));
#326522=CARTESIAN_POINT('Ctrl Pts',(-0.114725605000056,12.2,-4.00079591700001));
#326523=CARTESIAN_POINT('Ctrl Pts',(-0.114725605000056,5.2,-4.00079591700001));
#326524=CARTESIAN_POINT('Ctrl Pts',(-0.114725605000056,2.2,-4.00079591700001));
#326525=CARTESIAN_POINT('Ctrl Pts',(-0.114712179000056,12.2,-4.00114803400001));
#326526=CARTESIAN_POINT('Ctrl Pts',(-0.114712179000056,5.2,-4.00114803400001));
#326527=CARTESIAN_POINT('Ctrl Pts',(-0.114712179000056,2.2,-4.00114803400001));
#326528=CARTESIAN_POINT('Ctrl Pts',(-0.114698024000056,12.2,-4.00150682100001));
#326529=CARTESIAN_POINT('Ctrl Pts',(-0.114698024000056,5.2,-4.00150682100001));
#326530=CARTESIAN_POINT('Ctrl Pts',(-0.114698024000056,2.2,-4.00150682100001));
#326531=CARTESIAN_POINT('Ctrl Pts',(-0.114683124000056,12.2,-4.00187226200002));
#326532=CARTESIAN_POINT('Ctrl Pts',(-0.114683124000056,5.2,-4.00187226200002));
#326533=CARTESIAN_POINT('Ctrl Pts',(-0.114683124000056,2.2,-4.00187226200002));
#326534=CARTESIAN_POINT('Ctrl Pts',(-0.114667464000057,12.2,-4.00224434100001));
#326535=CARTESIAN_POINT('Ctrl Pts',(-0.114667464000057,5.2,-4.00224434100001));
#326536=CARTESIAN_POINT('Ctrl Pts',(-0.114667464000057,2.2,-4.00224434100001));
#326537=CARTESIAN_POINT('Ctrl Pts',(-0.114651025000055,12.2,-4.00262304400002));
#326538=CARTESIAN_POINT('Ctrl Pts',(-0.114651025000055,5.2,-4.00262304400002));
#326539=CARTESIAN_POINT('Ctrl Pts',(-0.114651025000055,2.2,-4.00262304400002));
#326540=CARTESIAN_POINT('Ctrl Pts',(-0.114633791000056,12.2,-4.00300835600001));
#326541=CARTESIAN_POINT('Ctrl Pts',(-0.114633791000056,5.2,-4.00300835600001));
#326542=CARTESIAN_POINT('Ctrl Pts',(-0.114633791000056,2.2,-4.00300835600001));
#326543=CARTESIAN_POINT('Ctrl Pts',(-0.114615747000055,12.2,-4.00340026000002));
#326544=CARTESIAN_POINT('Ctrl Pts',(-0.114615747000055,5.2,-4.00340026000002));
#326545=CARTESIAN_POINT('Ctrl Pts',(-0.114615747000055,2.2,-4.00340026000002));
#326546=CARTESIAN_POINT('Ctrl Pts',(-0.114596874000057,12.2,-4.00379874300001));
#326547=CARTESIAN_POINT('Ctrl Pts',(-0.114596874000057,5.2,-4.00379874300001));
#326548=CARTESIAN_POINT('Ctrl Pts',(-0.114596874000057,2.2,-4.00379874300001));
#326549=CARTESIAN_POINT('Ctrl Pts',(-0.114577159000057,12.2,-4.00420378800002));
#326550=CARTESIAN_POINT('Ctrl Pts',(-0.114577159000057,5.2,-4.00420378800002));
#326551=CARTESIAN_POINT('Ctrl Pts',(-0.114577159000057,2.2,-4.00420378800002));
#326552=CARTESIAN_POINT('Ctrl Pts',(-0.114556584000055,12.2,-4.00461538100001));
#326553=CARTESIAN_POINT('Ctrl Pts',(-0.114556584000055,5.2,-4.00461538100001));
#326554=CARTESIAN_POINT('Ctrl Pts',(-0.114556584000055,2.2,-4.00461538100001));
#326555=CARTESIAN_POINT('Ctrl Pts',(-0.114535132000055,12.2,-4.00503350700002));
#326556=CARTESIAN_POINT('Ctrl Pts',(-0.114535132000055,5.2,-4.00503350700002));
#326557=CARTESIAN_POINT('Ctrl Pts',(-0.114535132000055,2.2,-4.00503350700002));
#326558=CARTESIAN_POINT('Ctrl Pts',(-0.114512789000055,12.2,-4.00545815000001));
#326559=CARTESIAN_POINT('Ctrl Pts',(-0.114512789000055,5.2,-4.00545815000001));
#326560=CARTESIAN_POINT('Ctrl Pts',(-0.114512789000055,2.2,-4.00545815000001));
#326561=CARTESIAN_POINT('Ctrl Pts',(-0.114489538000055,12.2,-4.00588929700001));
#326562=CARTESIAN_POINT('Ctrl Pts',(-0.114489538000055,5.2,-4.00588929700001));
#326563=CARTESIAN_POINT('Ctrl Pts',(-0.114489538000055,2.2,-4.00588929700001));
#326564=CARTESIAN_POINT('Ctrl Pts',(-0.114465362000056,12.2,-4.00632693100002));
#326565=CARTESIAN_POINT('Ctrl Pts',(-0.114465362000056,5.2,-4.00632693100002));
#326566=CARTESIAN_POINT('Ctrl Pts',(-0.114465362000056,2.2,-4.00632693100002));
#326567=CARTESIAN_POINT('Ctrl Pts',(-0.114440247000056,12.2,-4.00677103800001));
#326568=CARTESIAN_POINT('Ctrl Pts',(-0.114440247000056,5.2,-4.00677103800001));
#326569=CARTESIAN_POINT('Ctrl Pts',(-0.114440247000056,2.2,-4.00677103800001));
#326570=CARTESIAN_POINT('Ctrl Pts',(-0.114414176000055,12.2,-4.00722160200001));
#326571=CARTESIAN_POINT('Ctrl Pts',(-0.114414176000055,5.2,-4.00722160200001));
#326572=CARTESIAN_POINT('Ctrl Pts',(-0.114414176000055,2.2,-4.00722160200001));
#326573=CARTESIAN_POINT('Ctrl Pts',(-0.114387135000056,12.2,-4.00767861000002));
#326574=CARTESIAN_POINT('Ctrl Pts',(-0.114387135000056,5.2,-4.00767861000002));
#326575=CARTESIAN_POINT('Ctrl Pts',(-0.114387135000056,2.2,-4.00767861000002));
#326576=CARTESIAN_POINT('Ctrl Pts',(-0.114359106000055,12.2,-4.00814204600001));
#326577=CARTESIAN_POINT('Ctrl Pts',(-0.114359106000055,5.2,-4.00814204600001));
#326578=CARTESIAN_POINT('Ctrl Pts',(-0.114359106000055,2.2,-4.00814204600001));
#326579=CARTESIAN_POINT('Ctrl Pts',(-0.114330074000056,12.2,-4.00861189500001));
#326580=CARTESIAN_POINT('Ctrl Pts',(-0.114330074000056,5.2,-4.00861189500001));
#326581=CARTESIAN_POINT('Ctrl Pts',(-0.114330074000056,2.2,-4.00861189500001));
#326582=CARTESIAN_POINT('Ctrl Pts',(-0.114300025000055,12.2,-4.00908814200001));
#326583=CARTESIAN_POINT('Ctrl Pts',(-0.114300025000055,5.2,-4.00908814200001));
#326584=CARTESIAN_POINT('Ctrl Pts',(-0.114300025000055,2.2,-4.00908814200001));
#326585=CARTESIAN_POINT('Ctrl Pts',(-0.114268943000055,12.2,-4.00957077400002));
#326586=CARTESIAN_POINT('Ctrl Pts',(-0.114268943000055,5.2,-4.00957077400002));
#326587=CARTESIAN_POINT('Ctrl Pts',(-0.114268943000055,2.2,-4.00957077400002));
#326588=CARTESIAN_POINT('Ctrl Pts',(-0.114236811000056,12.2,-4.01005977400001));
#326589=CARTESIAN_POINT('Ctrl Pts',(-0.114236811000056,5.2,-4.01005977400001));
#326590=CARTESIAN_POINT('Ctrl Pts',(-0.114236811000056,2.2,-4.01005977400001));
#326591=CARTESIAN_POINT('Ctrl Pts',(-0.114203615000056,12.2,-4.01055512900002));
#326592=CARTESIAN_POINT('Ctrl Pts',(-0.114203615000056,5.2,-4.01055512900002));
#326593=CARTESIAN_POINT('Ctrl Pts',(-0.114203615000056,2.2,-4.01055512900002));
#326594=CARTESIAN_POINT('Ctrl Pts',(-0.114169340000055,12.2,-4.01105682400001));
#326595=CARTESIAN_POINT('Ctrl Pts',(-0.114169340000055,5.2,-4.01105682400001));
#326596=CARTESIAN_POINT('Ctrl Pts',(-0.114169340000055,2.2,-4.01105682400001));
#326597=CARTESIAN_POINT('Ctrl Pts',(-0.114133970000055,12.2,-4.01156484400001));
#326598=CARTESIAN_POINT('Ctrl Pts',(-0.114133970000055,5.2,-4.01156484400001));
#326599=CARTESIAN_POINT('Ctrl Pts',(-0.114133970000055,2.2,-4.01156484400001));
#326600=CARTESIAN_POINT('Ctrl Pts',(-0.114097490000056,12.2,-4.01207917300002));
#326601=CARTESIAN_POINT('Ctrl Pts',(-0.114097490000056,5.2,-4.01207917300002));
#326602=CARTESIAN_POINT('Ctrl Pts',(-0.114097490000056,2.2,-4.01207917300002));
#326603=CARTESIAN_POINT('Ctrl Pts',(-0.114059886000056,12.2,-4.01259979900002));
#326604=CARTESIAN_POINT('Ctrl Pts',(-0.114059886000056,5.2,-4.01259979900002));
#326605=CARTESIAN_POINT('Ctrl Pts',(-0.114059886000056,2.2,-4.01259979900002));
#326606=CARTESIAN_POINT('Ctrl Pts',(-0.114021141000055,12.2,-4.01312670600001));
#326607=CARTESIAN_POINT('Ctrl Pts',(-0.114021141000055,5.2,-4.01312670600001));
#326608=CARTESIAN_POINT('Ctrl Pts',(-0.114021141000055,2.2,-4.01312670600001));
#326609=CARTESIAN_POINT('Ctrl Pts',(-0.113981242000056,12.2,-4.01365988000002));
#326610=CARTESIAN_POINT('Ctrl Pts',(-0.113981242000056,5.2,-4.01365988000002));
#326611=CARTESIAN_POINT('Ctrl Pts',(-0.113981242000056,2.2,-4.01365988000002));
#326612=CARTESIAN_POINT('Ctrl Pts',(-0.113940173000057,12.2,-4.01419930600001));
#326613=CARTESIAN_POINT('Ctrl Pts',(-0.113940173000057,5.2,-4.01419930600001));
#326614=CARTESIAN_POINT('Ctrl Pts',(-0.113940173000057,2.2,-4.01419930600001));
#326615=CARTESIAN_POINT('Ctrl Pts',(-0.113897920000056,12.2,-4.01474496900001));
#326616=CARTESIAN_POINT('Ctrl Pts',(-0.113897920000056,5.2,-4.01474496900001));
#326617=CARTESIAN_POINT('Ctrl Pts',(-0.113897920000056,2.2,-4.01474496900001));
#326618=CARTESIAN_POINT('Ctrl Pts',(-0.113854467000056,12.2,-4.01529685600002));
#326619=CARTESIAN_POINT('Ctrl Pts',(-0.113854467000056,5.2,-4.01529685600002));
#326620=CARTESIAN_POINT('Ctrl Pts',(-0.113854467000056,2.2,-4.01529685600002));
#326621=CARTESIAN_POINT('Ctrl Pts',(-0.113809801000055,12.2,-4.01585495100001));
#326622=CARTESIAN_POINT('Ctrl Pts',(-0.113809801000055,5.2,-4.01585495100001));
#326623=CARTESIAN_POINT('Ctrl Pts',(-0.113809801000055,2.2,-4.01585495100001));
#326624=CARTESIAN_POINT('Ctrl Pts',(-0.113763907000056,12.2,-4.01641924100002));
#326625=CARTESIAN_POINT('Ctrl Pts',(-0.113763907000056,5.2,-4.01641924100002));
#326626=CARTESIAN_POINT('Ctrl Pts',(-0.113763907000056,2.2,-4.01641924100002));
#326627=CARTESIAN_POINT('Ctrl Pts',(-0.113716768000056,12.2,-4.01698971200001));
#326628=CARTESIAN_POINT('Ctrl Pts',(-0.113716768000056,5.2,-4.01698971200001));
#326629=CARTESIAN_POINT('Ctrl Pts',(-0.113716768000056,2.2,-4.01698971200001));
#326630=CARTESIAN_POINT('Ctrl Pts',(-0.113668373000056,12.2,-4.01756634800002));
#326631=CARTESIAN_POINT('Ctrl Pts',(-0.113668373000056,5.2,-4.01756634800002));
#326632=CARTESIAN_POINT('Ctrl Pts',(-0.113668373000056,2.2,-4.01756634800002));
#326633=CARTESIAN_POINT('Ctrl Pts',(-0.113618705000055,12.2,-4.01814913500001));
#326634=CARTESIAN_POINT('Ctrl Pts',(-0.113618705000055,5.2,-4.01814913500001));
#326635=CARTESIAN_POINT('Ctrl Pts',(-0.113618705000055,2.2,-4.01814913500001));
#326636=CARTESIAN_POINT('Ctrl Pts',(-0.113567751000057,12.2,-4.01873805900001));
#326637=CARTESIAN_POINT('Ctrl Pts',(-0.113567751000057,5.2,-4.01873805900001));
#326638=CARTESIAN_POINT('Ctrl Pts',(-0.113567751000057,2.2,-4.01873805900001));
#326639=CARTESIAN_POINT('Ctrl Pts',(-0.113515496000056,12.2,-4.01933310600001));
#326640=CARTESIAN_POINT('Ctrl Pts',(-0.113515496000056,5.2,-4.01933310600001));
#326641=CARTESIAN_POINT('Ctrl Pts',(-0.113515496000056,2.2,-4.01933310600001));
#326642=CARTESIAN_POINT('Ctrl Pts',(-0.113461927000056,12.2,-4.01993426200002));
#326643=CARTESIAN_POINT('Ctrl Pts',(-0.113461927000056,5.2,-4.01993426200002));
#326644=CARTESIAN_POINT('Ctrl Pts',(-0.113461927000056,2.2,-4.01993426200002));
#326645=CARTESIAN_POINT('Ctrl Pts',(-0.113407028000055,12.2,-4.02054151200002));
#326646=CARTESIAN_POINT('Ctrl Pts',(-0.113407028000055,5.2,-4.02054151200002));
#326647=CARTESIAN_POINT('Ctrl Pts',(-0.113407028000055,2.2,-4.02054151200002));
#326648=CARTESIAN_POINT('Ctrl Pts',(-0.113350786000056,12.2,-4.02115484100001));
#326649=CARTESIAN_POINT('Ctrl Pts',(-0.113350786000056,5.2,-4.02115484100001));
#326650=CARTESIAN_POINT('Ctrl Pts',(-0.113350786000056,2.2,-4.02115484100001));
#326651=CARTESIAN_POINT('Ctrl Pts',(-0.113293186000056,12.2,-4.02177423700001));
#326652=CARTESIAN_POINT('Ctrl Pts',(-0.113293186000056,5.2,-4.02177423700001));
#326653=CARTESIAN_POINT('Ctrl Pts',(-0.113293186000056,2.2,-4.02177423700001));
#326654=CARTESIAN_POINT('Ctrl Pts',(-0.113234215000055,12.2,-4.02239968500002));
#326655=CARTESIAN_POINT('Ctrl Pts',(-0.113234215000055,5.2,-4.02239968500002));
#326656=CARTESIAN_POINT('Ctrl Pts',(-0.113234215000055,2.2,-4.02239968500002));
#326657=CARTESIAN_POINT('Ctrl Pts',(-0.113173859000056,12.2,-4.02303117100002));
#326658=CARTESIAN_POINT('Ctrl Pts',(-0.113173859000056,5.2,-4.02303117100002));
#326659=CARTESIAN_POINT('Ctrl Pts',(-0.113173859000056,2.2,-4.02303117100002));
#326660=CARTESIAN_POINT('Ctrl Pts',(-0.113112103000056,12.2,-4.02366868000001));
#326661=CARTESIAN_POINT('Ctrl Pts',(-0.113112103000056,5.2,-4.02366868000001));
#326662=CARTESIAN_POINT('Ctrl Pts',(-0.113112103000056,2.2,-4.02366868000001));
#326663=CARTESIAN_POINT('Ctrl Pts',(-0.113048934000056,12.2,-4.02431219900001));
#326664=CARTESIAN_POINT('Ctrl Pts',(-0.113048934000056,5.2,-4.02431219900001));
#326665=CARTESIAN_POINT('Ctrl Pts',(-0.113048934000056,2.2,-4.02431219900001));
#326666=CARTESIAN_POINT('Ctrl Pts',(-0.112984338000055,12.2,-4.02496171300001));
#326667=CARTESIAN_POINT('Ctrl Pts',(-0.112984338000055,5.2,-4.02496171300001));
#326668=CARTESIAN_POINT('Ctrl Pts',(-0.112984338000055,2.2,-4.02496171300001));
#326669=CARTESIAN_POINT('Ctrl Pts',(-0.112918302000056,12.2,-4.02561720900001));
#326670=CARTESIAN_POINT('Ctrl Pts',(-0.112918302000056,5.2,-4.02561720900001));
#326671=CARTESIAN_POINT('Ctrl Pts',(-0.112918302000056,2.2,-4.02561720900001));
#326672=CARTESIAN_POINT('Ctrl Pts',(-0.112850811000056,12.2,-4.02627867200001));
#326673=CARTESIAN_POINT('Ctrl Pts',(-0.112850811000056,5.2,-4.02627867200001));
#326674=CARTESIAN_POINT('Ctrl Pts',(-0.112850811000056,2.2,-4.02627867200001));
#326675=CARTESIAN_POINT('Ctrl Pts',(-0.112781853000056,12.2,-4.02694608900001));
#326676=CARTESIAN_POINT('Ctrl Pts',(-0.112781853000056,5.2,-4.02694608900001));
#326677=CARTESIAN_POINT('Ctrl Pts',(-0.112781853000056,2.2,-4.02694608900001));
#326678=CARTESIAN_POINT('Ctrl Pts',(-0.112711412000056,12.2,-4.02761944500002));
#326679=CARTESIAN_POINT('Ctrl Pts',(-0.112711412000056,5.2,-4.02761944500002));
#326680=CARTESIAN_POINT('Ctrl Pts',(-0.112711412000056,2.2,-4.02761944500002));
#326681=CARTESIAN_POINT('Ctrl Pts',(-0.112639476000057,12.2,-4.02829872600002));
#326682=CARTESIAN_POINT('Ctrl Pts',(-0.112639476000057,5.2,-4.02829872600002));
#326683=CARTESIAN_POINT('Ctrl Pts',(-0.112639476000057,2.2,-4.02829872600002));
#326684=CARTESIAN_POINT('Ctrl Pts',(-0.112566033000056,12.2,-4.02898392000001));
#326685=CARTESIAN_POINT('Ctrl Pts',(-0.112566033000056,5.2,-4.02898392000001));
#326686=CARTESIAN_POINT('Ctrl Pts',(-0.112566033000056,2.2,-4.02898392000001));
#326687=CARTESIAN_POINT('Ctrl Pts',(-0.112491067000056,12.2,-4.02967501100001));
#326688=CARTESIAN_POINT('Ctrl Pts',(-0.112491067000056,5.2,-4.02967501100001));
#326689=CARTESIAN_POINT('Ctrl Pts',(-0.112491067000056,2.2,-4.02967501100001));
#326690=CARTESIAN_POINT('Ctrl Pts',(-0.112414565000056,12.2,-4.03037198700002));
#326691=CARTESIAN_POINT('Ctrl Pts',(-0.112414565000056,5.2,-4.03037198700002));
#326692=CARTESIAN_POINT('Ctrl Pts',(-0.112414565000056,2.2,-4.03037198700002));
#326693=CARTESIAN_POINT('Ctrl Pts',(-0.112336516000056,12.2,-4.03107483200001));
#326694=CARTESIAN_POINT('Ctrl Pts',(-0.112336516000056,5.2,-4.03107483200001));
#326695=CARTESIAN_POINT('Ctrl Pts',(-0.112336516000056,2.2,-4.03107483200001));
#326696=CARTESIAN_POINT('Ctrl Pts',(-0.112256904000055,12.2,-4.03178353500001));
#326697=CARTESIAN_POINT('Ctrl Pts',(-0.112256904000055,5.2,-4.03178353500001));
#326698=CARTESIAN_POINT('Ctrl Pts',(-0.112256904000055,2.2,-4.03178353500001));
#326699=CARTESIAN_POINT('Ctrl Pts',(-0.112175718000056,12.2,-4.03249807800002));
#326700=CARTESIAN_POINT('Ctrl Pts',(-0.112175718000056,5.2,-4.03249807800002));
#326701=CARTESIAN_POINT('Ctrl Pts',(-0.112175718000056,2.2,-4.03249807800002));
#326702=CARTESIAN_POINT('Ctrl Pts',(-0.112092944000055,12.2,-4.03321845200002));
#326703=CARTESIAN_POINT('Ctrl Pts',(-0.112092944000055,5.2,-4.03321845200002));
#326704=CARTESIAN_POINT('Ctrl Pts',(-0.112092944000055,2.2,-4.03321845200002));
#326705=CARTESIAN_POINT('Ctrl Pts',(-0.112008568000055,12.2,-4.03394464100002));
#326706=CARTESIAN_POINT('Ctrl Pts',(-0.112008568000055,5.2,-4.03394464100002));
#326707=CARTESIAN_POINT('Ctrl Pts',(-0.112008568000055,2.2,-4.03394464100002));
#326708=CARTESIAN_POINT('Ctrl Pts',(-0.111922578000057,12.2,-4.03467663000002));
#326709=CARTESIAN_POINT('Ctrl Pts',(-0.111922578000057,5.2,-4.03467663000002));
#326710=CARTESIAN_POINT('Ctrl Pts',(-0.111922578000057,2.2,-4.03467663000002));
#326711=CARTESIAN_POINT('Ctrl Pts',(-0.111834961000056,12.2,-4.03541440800002));
#326712=CARTESIAN_POINT('Ctrl Pts',(-0.111834961000056,5.2,-4.03541440800002));
#326713=CARTESIAN_POINT('Ctrl Pts',(-0.111834961000056,2.2,-4.03541440800002));
#326714=CARTESIAN_POINT('Ctrl Pts',(-0.111745705000056,12.2,-4.03615796000001));
#326715=CARTESIAN_POINT('Ctrl Pts',(-0.111745705000056,5.2,-4.03615796000001));
#326716=CARTESIAN_POINT('Ctrl Pts',(-0.111745705000056,2.2,-4.03615796000001));
#326717=CARTESIAN_POINT('Ctrl Pts',(-0.111654795000057,12.2,-4.03690727100001));
#326718=CARTESIAN_POINT('Ctrl Pts',(-0.111654795000057,5.2,-4.03690727100001));
#326719=CARTESIAN_POINT('Ctrl Pts',(-0.111654795000057,2.2,-4.03690727100001));
#326720=CARTESIAN_POINT('Ctrl Pts',(-0.111562219000056,12.2,-4.03766233000002));
#326721=CARTESIAN_POINT('Ctrl Pts',(-0.111562219000056,5.2,-4.03766233000002));
#326722=CARTESIAN_POINT('Ctrl Pts',(-0.111562219000056,2.2,-4.03766233000002));
#326723=CARTESIAN_POINT('Ctrl Pts',(-0.111467966000056,12.2,-4.03842312200001));
#326724=CARTESIAN_POINT('Ctrl Pts',(-0.111467966000056,5.2,-4.03842312200001));
#326725=CARTESIAN_POINT('Ctrl Pts',(-0.111467966000056,2.2,-4.03842312200001));
#326726=CARTESIAN_POINT('Ctrl Pts',(-0.111372020000056,12.2,-4.03918963400002));
#326727=CARTESIAN_POINT('Ctrl Pts',(-0.111372020000056,5.2,-4.03918963400002));
#326728=CARTESIAN_POINT('Ctrl Pts',(-0.111372020000056,2.2,-4.03918963400002));
#326729=CARTESIAN_POINT('Ctrl Pts',(-0.111274372000055,12.2,-4.03996185000001));
#326730=CARTESIAN_POINT('Ctrl Pts',(-0.111274372000055,5.2,-4.03996185000001));
#326731=CARTESIAN_POINT('Ctrl Pts',(-0.111274372000055,2.2,-4.03996185000001));
#326732=CARTESIAN_POINT('Ctrl Pts',(-0.111175006000056,12.2,-4.04073976100001));
#326733=CARTESIAN_POINT('Ctrl Pts',(-0.111175006000056,5.2,-4.04073976100001));
#326734=CARTESIAN_POINT('Ctrl Pts',(-0.111175006000056,2.2,-4.04073976100001));
#326735=CARTESIAN_POINT('Ctrl Pts',(-0.111073912000055,12.2,-4.04152335000001));
#326736=CARTESIAN_POINT('Ctrl Pts',(-0.111073912000055,5.2,-4.04152335000001));
#326737=CARTESIAN_POINT('Ctrl Pts',(-0.111073912000055,2.2,-4.04152335000001));
#326738=CARTESIAN_POINT('Ctrl Pts',(-0.110971077000055,12.2,-4.04231260400001));
#326739=CARTESIAN_POINT('Ctrl Pts',(-0.110971077000055,5.2,-4.04231260400001));
#326740=CARTESIAN_POINT('Ctrl Pts',(-0.110971077000055,2.2,-4.04231260400001));
#326741=CARTESIAN_POINT('Ctrl Pts',(-0.110866488000055,12.2,-4.04310751100001));
#326742=CARTESIAN_POINT('Ctrl Pts',(-0.110866488000055,5.2,-4.04310751100001));
#326743=CARTESIAN_POINT('Ctrl Pts',(-0.110866488000055,2.2,-4.04310751100001));
#326744=CARTESIAN_POINT('Ctrl Pts',(-0.110760133000056,12.2,-4.04390805600002));
#326745=CARTESIAN_POINT('Ctrl Pts',(-0.110760133000056,5.2,-4.04390805600002));
#326746=CARTESIAN_POINT('Ctrl Pts',(-0.110760133000056,2.2,-4.04390805600002));
#326747=CARTESIAN_POINT('Ctrl Pts',(-0.110651998000056,12.2,-4.04471422600002));
#326748=CARTESIAN_POINT('Ctrl Pts',(-0.110651998000056,5.2,-4.04471422600002));
#326749=CARTESIAN_POINT('Ctrl Pts',(-0.110651998000056,2.2,-4.04471422600002));
#326750=CARTESIAN_POINT('Ctrl Pts',(-0.110542073000056,12.2,-4.04552600800002));
#326751=CARTESIAN_POINT('Ctrl Pts',(-0.110542073000056,5.2,-4.04552600800002));
#326752=CARTESIAN_POINT('Ctrl Pts',(-0.110542073000056,2.2,-4.04552600800002));
#326753=CARTESIAN_POINT('Ctrl Pts',(-0.110430344000055,12.2,-4.04634338900001));
#326754=CARTESIAN_POINT('Ctrl Pts',(-0.110430344000055,5.2,-4.04634338900001));
#326755=CARTESIAN_POINT('Ctrl Pts',(-0.110430344000055,2.2,-4.04634338900001));
#326756=CARTESIAN_POINT('Ctrl Pts',(-0.110316801000057,12.2,-4.04716635400002));
#326757=CARTESIAN_POINT('Ctrl Pts',(-0.110316801000057,5.2,-4.04716635400002));
#326758=CARTESIAN_POINT('Ctrl Pts',(-0.110316801000057,2.2,-4.04716635400002));
#326759=CARTESIAN_POINT('Ctrl Pts',(-0.110201430000056,12.2,-4.04799489100002));
#326760=CARTESIAN_POINT('Ctrl Pts',(-0.110201430000056,5.2,-4.04799489100002));
#326761=CARTESIAN_POINT('Ctrl Pts',(-0.110201430000056,2.2,-4.04799489100002));
#326762=CARTESIAN_POINT('Ctrl Pts',(-0.110084220000056,12.2,-4.04882898600002));
#326763=CARTESIAN_POINT('Ctrl Pts',(-0.110084220000056,5.2,-4.04882898600002));
#326764=CARTESIAN_POINT('Ctrl Pts',(-0.110084220000056,2.2,-4.04882898600002));
#326765=CARTESIAN_POINT('Ctrl Pts',(-0.109965157000056,12.2,-4.04966862700002));
#326766=CARTESIAN_POINT('Ctrl Pts',(-0.109965157000056,5.2,-4.04966862700002));
#326767=CARTESIAN_POINT('Ctrl Pts',(-0.109965157000056,2.2,-4.04966862700002));
#326768=CARTESIAN_POINT('Ctrl Pts',(-0.109844232000055,12.2,-4.05051379900002));
#326769=CARTESIAN_POINT('Ctrl Pts',(-0.109844232000055,5.2,-4.05051379900002));
#326770=CARTESIAN_POINT('Ctrl Pts',(-0.109844232000055,2.2,-4.05051379900002));
#326771=CARTESIAN_POINT('Ctrl Pts',(-0.109721430000055,12.2,-4.05136449100001));
#326772=CARTESIAN_POINT('Ctrl Pts',(-0.109721430000055,5.2,-4.05136449100001));
#326773=CARTESIAN_POINT('Ctrl Pts',(-0.109721430000055,2.2,-4.05136449100001));
#326774=CARTESIAN_POINT('Ctrl Pts',(-0.109596742000055,12.2,-4.05222068700001));
#326775=CARTESIAN_POINT('Ctrl Pts',(-0.109596742000055,5.2,-4.05222068700001));
#326776=CARTESIAN_POINT('Ctrl Pts',(-0.109596742000055,2.2,-4.05222068700001));
#326777=CARTESIAN_POINT('Ctrl Pts',(-0.109470154000055,12.2,-4.05308237500002));
#326778=CARTESIAN_POINT('Ctrl Pts',(-0.109470154000055,5.2,-4.05308237500002));
#326779=CARTESIAN_POINT('Ctrl Pts',(-0.109470154000055,2.2,-4.05308237500002));
#326780=CARTESIAN_POINT('Ctrl Pts',(-0.109341655000056,12.2,-4.05394954200001));
#326781=CARTESIAN_POINT('Ctrl Pts',(-0.109341655000056,5.2,-4.05394954200001));
#326782=CARTESIAN_POINT('Ctrl Pts',(-0.109341655000056,2.2,-4.05394954200001));
#326783=CARTESIAN_POINT('Ctrl Pts',(-0.109211234000056,12.2,-4.05482217500001));
#326784=CARTESIAN_POINT('Ctrl Pts',(-0.109211234000056,5.2,-4.05482217500001));
#326785=CARTESIAN_POINT('Ctrl Pts',(-0.109211234000056,2.2,-4.05482217500001));
#326786=CARTESIAN_POINT('Ctrl Pts',(-0.109078877000056,12.2,-4.05570026000001));
#326787=CARTESIAN_POINT('Ctrl Pts',(-0.109078877000056,5.2,-4.05570026000001));
#326788=CARTESIAN_POINT('Ctrl Pts',(-0.109078877000056,2.2,-4.05570026000001));
#326789=CARTESIAN_POINT('Ctrl Pts',(-0.108944575000055,12.2,-4.05658378600001));
#326790=CARTESIAN_POINT('Ctrl Pts',(-0.108944575000055,5.2,-4.05658378600001));
#326791=CARTESIAN_POINT('Ctrl Pts',(-0.108944575000055,2.2,-4.05658378600001));
#326792=CARTESIAN_POINT('Ctrl Pts',(-0.108808314000056,12.2,-4.05747273700001));
#326793=CARTESIAN_POINT('Ctrl Pts',(-0.108808314000056,5.2,-4.05747273700001));
#326794=CARTESIAN_POINT('Ctrl Pts',(-0.108808314000056,2.2,-4.05747273700001));
#326795=CARTESIAN_POINT('Ctrl Pts',(-0.108670085000057,12.2,-4.05836710200001));
#326796=CARTESIAN_POINT('Ctrl Pts',(-0.108670085000057,5.2,-4.05836710200001));
#326797=CARTESIAN_POINT('Ctrl Pts',(-0.108670085000057,2.2,-4.05836710200001));
#326798=CARTESIAN_POINT('Ctrl Pts',(-0.108529875000055,12.2,-4.05926686700001));
#326799=CARTESIAN_POINT('Ctrl Pts',(-0.108529875000055,5.2,-4.05926686700001));
#326800=CARTESIAN_POINT('Ctrl Pts',(-0.108529875000055,2.2,-4.05926686700001));
#326801=CARTESIAN_POINT('Ctrl Pts',(-0.108387672000055,12.2,-4.06017201800001));
#326802=CARTESIAN_POINT('Ctrl Pts',(-0.108387672000055,5.2,-4.06017201800001));
#326803=CARTESIAN_POINT('Ctrl Pts',(-0.108387672000055,2.2,-4.06017201800001));
#326804=CARTESIAN_POINT('Ctrl Pts',(-0.108243465000056,12.2,-4.06108254500001));
#326805=CARTESIAN_POINT('Ctrl Pts',(-0.108243465000056,5.2,-4.06108254500001));
#326806=CARTESIAN_POINT('Ctrl Pts',(-0.108243465000056,2.2,-4.06108254500001));
#326807=CARTESIAN_POINT('Ctrl Pts',(-0.108097244000056,12.2,-4.06199843200001));
#326808=CARTESIAN_POINT('Ctrl Pts',(-0.108097244000056,5.2,-4.06199843200001));
#326809=CARTESIAN_POINT('Ctrl Pts',(-0.108097244000056,2.2,-4.06199843200001));
#326810=CARTESIAN_POINT('Ctrl Pts',(-0.107948995000056,12.2,-4.06291966700001));
#326811=CARTESIAN_POINT('Ctrl Pts',(-0.107948995000056,5.2,-4.06291966700001));
#326812=CARTESIAN_POINT('Ctrl Pts',(-0.107948995000056,2.2,-4.06291966700001));
#326813=CARTESIAN_POINT('Ctrl Pts',(-0.107798709000055,12.2,-4.06384623800002));
#326814=CARTESIAN_POINT('Ctrl Pts',(-0.107798709000055,5.2,-4.06384623800002));
#326815=CARTESIAN_POINT('Ctrl Pts',(-0.107798709000055,2.2,-4.06384623800002));
#326816=CARTESIAN_POINT('Ctrl Pts',(-0.107646374000057,12.2,-4.06477813000001));
#326817=CARTESIAN_POINT('Ctrl Pts',(-0.107646374000057,5.2,-4.06477813000001));
#326818=CARTESIAN_POINT('Ctrl Pts',(-0.107646374000057,2.2,-4.06477813000001));
#326819=CARTESIAN_POINT('Ctrl Pts',(-0.107491979000055,12.2,-4.06571533200002));
#326820=CARTESIAN_POINT('Ctrl Pts',(-0.107491979000055,5.2,-4.06571533200002));
#326821=CARTESIAN_POINT('Ctrl Pts',(-0.107491979000055,2.2,-4.06571533200002));
#326822=CARTESIAN_POINT('Ctrl Pts',(-0.107335513000055,12.2,-4.06665783000001));
#326823=CARTESIAN_POINT('Ctrl Pts',(-0.107335513000055,5.2,-4.06665783000001));
#326824=CARTESIAN_POINT('Ctrl Pts',(-0.107335513000055,2.2,-4.06665783000001));
#326825=CARTESIAN_POINT('Ctrl Pts',(-0.107176964000055,12.2,-4.06760561100001));
#326826=CARTESIAN_POINT('Ctrl Pts',(-0.107176964000055,5.2,-4.06760561100001));
#326827=CARTESIAN_POINT('Ctrl Pts',(-0.107176964000055,2.2,-4.06760561100001));
#326828=CARTESIAN_POINT('Ctrl Pts',(-0.107016321000056,12.2,-4.06855866300001));
#326829=CARTESIAN_POINT('Ctrl Pts',(-0.107016321000056,5.2,-4.06855866300001));
#326830=CARTESIAN_POINT('Ctrl Pts',(-0.107016321000056,2.2,-4.06855866300001));
#326831=CARTESIAN_POINT('Ctrl Pts',(-0.106853574000055,12.2,-4.06951697300002));
#326832=CARTESIAN_POINT('Ctrl Pts',(-0.106853574000055,5.2,-4.06951697300002));
#326833=CARTESIAN_POINT('Ctrl Pts',(-0.106853574000055,2.2,-4.06951697300002));
#326834=CARTESIAN_POINT('Ctrl Pts',(-0.106688711000055,12.2,-4.07048052800001));
#326835=CARTESIAN_POINT('Ctrl Pts',(-0.106688711000055,5.2,-4.07048052800001));
#326836=CARTESIAN_POINT('Ctrl Pts',(-0.106688711000055,2.2,-4.07048052800001));
#326837=CARTESIAN_POINT('Ctrl Pts',(-0.106521723000055,12.2,-4.07144931400001));
#326838=CARTESIAN_POINT('Ctrl Pts',(-0.106521723000055,5.2,-4.07144931400001));
#326839=CARTESIAN_POINT('Ctrl Pts',(-0.106521723000055,2.2,-4.07144931400001));
#326840=CARTESIAN_POINT('Ctrl Pts',(-0.106352597000056,12.2,-4.07242332000001));
#326841=CARTESIAN_POINT('Ctrl Pts',(-0.106352597000056,5.2,-4.07242332000001));
#326842=CARTESIAN_POINT('Ctrl Pts',(-0.106352597000056,2.2,-4.07242332000001));
#326843=CARTESIAN_POINT('Ctrl Pts',(-0.106181322000056,12.2,-4.07340253300001));
#326844=CARTESIAN_POINT('Ctrl Pts',(-0.106181322000056,5.2,-4.07340253300001));
#326845=CARTESIAN_POINT('Ctrl Pts',(-0.106181322000056,2.2,-4.07340253300001));
#326846=CARTESIAN_POINT('Ctrl Pts',(-0.106007888000056,12.2,-4.07438693900001));
#326847=CARTESIAN_POINT('Ctrl Pts',(-0.106007888000056,5.2,-4.07438693900001));
#326848=CARTESIAN_POINT('Ctrl Pts',(-0.106007888000056,2.2,-4.07438693900001));
#326849=CARTESIAN_POINT('Ctrl Pts',(-0.105832285000057,12.2,-4.07537652600002));
#326850=CARTESIAN_POINT('Ctrl Pts',(-0.105832285000057,5.2,-4.07537652600002));
#326851=CARTESIAN_POINT('Ctrl Pts',(-0.105832285000057,2.2,-4.07537652600002));
#326852=CARTESIAN_POINT('Ctrl Pts',(-0.105654502000055,12.2,-4.07637128100002));
#326853=CARTESIAN_POINT('Ctrl Pts',(-0.105654502000055,5.2,-4.07637128100002));
#326854=CARTESIAN_POINT('Ctrl Pts',(-0.105654502000055,2.2,-4.07637128100002));
#326855=CARTESIAN_POINT('Ctrl Pts',(-0.105474527000055,12.2,-4.07737119100001));
#326856=CARTESIAN_POINT('Ctrl Pts',(-0.105474527000055,5.2,-4.07737119100001));
#326857=CARTESIAN_POINT('Ctrl Pts',(-0.105474527000055,2.2,-4.07737119100001));
#326858=CARTESIAN_POINT('Ctrl Pts',(-0.105292351000056,12.2,-4.07837624500001));
#326859=CARTESIAN_POINT('Ctrl Pts',(-0.105292351000056,5.2,-4.07837624500001));
#326860=CARTESIAN_POINT('Ctrl Pts',(-0.105292351000056,2.2,-4.07837624500001));
#326861=CARTESIAN_POINT('Ctrl Pts',(-0.105107963000056,12.2,-4.07938642800001));
#326862=CARTESIAN_POINT('Ctrl Pts',(-0.105107963000056,5.2,-4.07938642800001));
#326863=CARTESIAN_POINT('Ctrl Pts',(-0.105107963000056,2.2,-4.07938642800001));
#326864=CARTESIAN_POINT('Ctrl Pts',(-0.104921351000057,12.2,-4.08040173000002));
#326865=CARTESIAN_POINT('Ctrl Pts',(-0.104921351000057,5.2,-4.08040173000002));
#326866=CARTESIAN_POINT('Ctrl Pts',(-0.104921351000057,2.2,-4.08040173000002));
#326867=CARTESIAN_POINT('Ctrl Pts',(-0.104732506000056,12.2,-4.08142213600001));
#326868=CARTESIAN_POINT('Ctrl Pts',(-0.104732506000056,5.2,-4.08142213600001));
#326869=CARTESIAN_POINT('Ctrl Pts',(-0.104732506000056,2.2,-4.08142213600001));
#326870=CARTESIAN_POINT('Ctrl Pts',(-0.104541418000055,12.2,-4.08244763400001));
#326871=CARTESIAN_POINT('Ctrl Pts',(-0.104541418000055,5.2,-4.08244763400001));
#326872=CARTESIAN_POINT('Ctrl Pts',(-0.104541418000055,2.2,-4.08244763400001));
#326873=CARTESIAN_POINT('Ctrl Pts',(-0.104348076000056,12.2,-4.08347821100001));
#326874=CARTESIAN_POINT('Ctrl Pts',(-0.104348076000056,5.2,-4.08347821100001));
#326875=CARTESIAN_POINT('Ctrl Pts',(-0.104348076000056,2.2,-4.08347821100001));
#326876=CARTESIAN_POINT('Ctrl Pts',(-0.104152469000055,12.2,-4.08451385700001));
#326877=CARTESIAN_POINT('Ctrl Pts',(-0.104152469000055,5.2,-4.08451385700001));
#326878=CARTESIAN_POINT('Ctrl Pts',(-0.104152469000055,2.2,-4.08451385700001));
#326879=CARTESIAN_POINT('Ctrl Pts',(-0.103954586000056,12.2,-4.08555455600002));
#326880=CARTESIAN_POINT('Ctrl Pts',(-0.103954586000056,5.2,-4.08555455600002));
#326881=CARTESIAN_POINT('Ctrl Pts',(-0.103954586000056,2.2,-4.08555455600002));
#326882=CARTESIAN_POINT('Ctrl Pts',(-0.103754419000056,12.2,-4.08660029800001));
#326883=CARTESIAN_POINT('Ctrl Pts',(-0.103754419000056,5.2,-4.08660029800001));
#326884=CARTESIAN_POINT('Ctrl Pts',(-0.103754419000056,2.2,-4.08660029800001));
#326885=CARTESIAN_POINT('Ctrl Pts',(-0.103551956000055,12.2,-4.08765106800002));
#326886=CARTESIAN_POINT('Ctrl Pts',(-0.103551956000055,5.2,-4.08765106800002));
#326887=CARTESIAN_POINT('Ctrl Pts',(-0.103551956000055,2.2,-4.08765106800002));
#326888=CARTESIAN_POINT('Ctrl Pts',(-0.103347188000056,12.2,-4.08870685700002));
#326889=CARTESIAN_POINT('Ctrl Pts',(-0.103347188000056,5.2,-4.08870685700002));
#326890=CARTESIAN_POINT('Ctrl Pts',(-0.103347188000056,2.2,-4.08870685700002));
#326891=CARTESIAN_POINT('Ctrl Pts',(-0.103140103000056,12.2,-4.08976764800002));
#326892=CARTESIAN_POINT('Ctrl Pts',(-0.103140103000056,5.2,-4.08976764800002));
#326893=CARTESIAN_POINT('Ctrl Pts',(-0.103140103000056,2.2,-4.08976764800002));
#326894=CARTESIAN_POINT('Ctrl Pts',(-0.102930694000056,12.2,-4.09083343200002));
#326895=CARTESIAN_POINT('Ctrl Pts',(-0.102930694000056,5.2,-4.09083343200002));
#326896=CARTESIAN_POINT('Ctrl Pts',(-0.102930694000056,2.2,-4.09083343200002));
#326897=CARTESIAN_POINT('Ctrl Pts',(-0.102718947000057,12.2,-4.09190419600002));
#326898=CARTESIAN_POINT('Ctrl Pts',(-0.102718947000057,5.2,-4.09190419600002));
#326899=CARTESIAN_POINT('Ctrl Pts',(-0.102718947000057,2.2,-4.09190419600002));
#326900=CARTESIAN_POINT('Ctrl Pts',(-0.102504855000056,12.2,-4.09297992600001));
#326901=CARTESIAN_POINT('Ctrl Pts',(-0.102504855000056,5.2,-4.09297992600001));
#326902=CARTESIAN_POINT('Ctrl Pts',(-0.102504855000056,2.2,-4.09297992600001));
#326903=CARTESIAN_POINT('Ctrl Pts',(-0.102288407000056,12.2,-4.09406061100002));
#326904=CARTESIAN_POINT('Ctrl Pts',(-0.102288407000056,5.2,-4.09406061100002));
#326905=CARTESIAN_POINT('Ctrl Pts',(-0.102288407000056,2.2,-4.09406061100002));
#326906=CARTESIAN_POINT('Ctrl Pts',(-0.102069593000056,12.2,-4.09514623900002));
#326907=CARTESIAN_POINT('Ctrl Pts',(-0.102069593000056,5.2,-4.09514623900002));
#326908=CARTESIAN_POINT('Ctrl Pts',(-0.102069593000056,2.2,-4.09514623900002));
#326909=CARTESIAN_POINT('Ctrl Pts',(-0.101848403000057,12.2,-4.09623679600001));
#326910=CARTESIAN_POINT('Ctrl Pts',(-0.101848403000057,5.2,-4.09623679600001));
#326911=CARTESIAN_POINT('Ctrl Pts',(-0.101848403000057,2.2,-4.09623679600001));
#326912=CARTESIAN_POINT('Ctrl Pts',(-0.101624827000055,12.2,-4.09733227000002));
#326913=CARTESIAN_POINT('Ctrl Pts',(-0.101624827000055,5.2,-4.09733227000002));
#326914=CARTESIAN_POINT('Ctrl Pts',(-0.101624827000055,2.2,-4.09733227000002));
#326915=CARTESIAN_POINT('Ctrl Pts',(-0.101398855000056,12.2,-4.09843264900001));
#326916=CARTESIAN_POINT('Ctrl Pts',(-0.101398855000056,5.2,-4.09843264900001));
#326917=CARTESIAN_POINT('Ctrl Pts',(-0.101398855000056,2.2,-4.09843264900001));
#326918=CARTESIAN_POINT('Ctrl Pts',(-0.101170479000056,12.2,-4.09953792200001));
#326919=CARTESIAN_POINT('Ctrl Pts',(-0.101170479000056,5.2,-4.09953792200001));
#326920=CARTESIAN_POINT('Ctrl Pts',(-0.101170479000056,2.2,-4.09953792200001));
#326921=CARTESIAN_POINT('Ctrl Pts',(-0.100939686000056,12.2,-4.10064807500001));
#326922=CARTESIAN_POINT('Ctrl Pts',(-0.100939686000056,5.2,-4.10064807500001));
#326923=CARTESIAN_POINT('Ctrl Pts',(-0.100939686000056,2.2,-4.10064807500001));
#326924=CARTESIAN_POINT('Ctrl Pts',(-0.100706469000055,12.2,-4.10176309600002));
#326925=CARTESIAN_POINT('Ctrl Pts',(-0.100706469000055,5.2,-4.10176309600002));
#326926=CARTESIAN_POINT('Ctrl Pts',(-0.100706469000055,2.2,-4.10176309600002));
#326927=CARTESIAN_POINT('Ctrl Pts',(-0.100470817000057,12.2,-4.10288297300001));
#326928=CARTESIAN_POINT('Ctrl Pts',(-0.100470817000057,5.2,-4.10288297300001));
#326929=CARTESIAN_POINT('Ctrl Pts',(-0.100470817000057,2.2,-4.10288297300001));
#326930=CARTESIAN_POINT('Ctrl Pts',(-0.100232720000056,12.2,-4.10400769300002));
#326931=CARTESIAN_POINT('Ctrl Pts',(-0.100232720000056,5.2,-4.10400769300002));
#326932=CARTESIAN_POINT('Ctrl Pts',(-0.100232720000056,2.2,-4.10400769300002));
#326933=CARTESIAN_POINT('Ctrl Pts',(-0.0999921710000551,12.2,-4.10513724500001));
#326934=CARTESIAN_POINT('Ctrl Pts',(-0.0999921710000551,5.2,-4.10513724500001));
#326935=CARTESIAN_POINT('Ctrl Pts',(-0.0999921710000551,2.2,-4.10513724500001));
#326936=CARTESIAN_POINT('Ctrl Pts',(-0.0997491570000564,12.2,-4.10627161500001));
#326937=CARTESIAN_POINT('Ctrl Pts',(-0.0997491570000564,5.2,-4.10627161500001));
#326938=CARTESIAN_POINT('Ctrl Pts',(-0.0997491570000564,2.2,-4.10627161500001));
#326939=CARTESIAN_POINT('Ctrl Pts',(-0.0995036710000552,12.2,-4.10741079300001));
#326940=CARTESIAN_POINT('Ctrl Pts',(-0.0995036710000552,5.2,-4.10741079300001));
#326941=CARTESIAN_POINT('Ctrl Pts',(-0.0995036710000552,2.2,-4.10741079300001));
#326942=CARTESIAN_POINT('Ctrl Pts',(-0.099255701000055,12.2,-4.10855476500001));
#326943=CARTESIAN_POINT('Ctrl Pts',(-0.099255701000055,5.2,-4.10855476500001));
#326944=CARTESIAN_POINT('Ctrl Pts',(-0.099255701000055,2.2,-4.10855476500001));
#326945=CARTESIAN_POINT('Ctrl Pts',(-0.0990052400000552,12.2,-4.10970351900001));
#326946=CARTESIAN_POINT('Ctrl Pts',(-0.0990052400000552,5.2,-4.10970351900001));
#326947=CARTESIAN_POINT('Ctrl Pts',(-0.0990052400000552,2.2,-4.10970351900001));
#326948=CARTESIAN_POINT('Ctrl Pts',(-0.098752278000056,12.2,-4.11085704400001));
#326949=CARTESIAN_POINT('Ctrl Pts',(-0.098752278000056,5.2,-4.11085704400001));
#326950=CARTESIAN_POINT('Ctrl Pts',(-0.098752278000056,2.2,-4.11085704400001));
#326951=CARTESIAN_POINT('Ctrl Pts',(-0.0984968050000568,12.2,-4.11201532700002));
#326952=CARTESIAN_POINT('Ctrl Pts',(-0.0984968050000568,5.2,-4.11201532700002));
#326953=CARTESIAN_POINT('Ctrl Pts',(-0.0984968050000568,2.2,-4.11201532700002));
#326954=CARTESIAN_POINT('Ctrl Pts',(-0.0982388110000565,12.2,-4.11317835500002));
#326955=CARTESIAN_POINT('Ctrl Pts',(-0.0982388110000565,5.2,-4.11317835500002));
#326956=CARTESIAN_POINT('Ctrl Pts',(-0.0982388110000565,2.2,-4.11317835500002));
#326957=CARTESIAN_POINT('Ctrl Pts',(-0.0979782880000546,12.2,-4.11434611800002));
#326958=CARTESIAN_POINT('Ctrl Pts',(-0.0979782880000546,5.2,-4.11434611800002));
#326959=CARTESIAN_POINT('Ctrl Pts',(-0.0979782880000546,2.2,-4.11434611800002));
#326960=CARTESIAN_POINT('Ctrl Pts',(-0.0977152270000547,12.2,-4.11551860300001));
#326961=CARTESIAN_POINT('Ctrl Pts',(-0.0977152270000547,5.2,-4.11551860300001));
#326962=CARTESIAN_POINT('Ctrl Pts',(-0.0977152270000547,2.2,-4.11551860300001));
#326963=CARTESIAN_POINT('Ctrl Pts',(-0.097449618000055,12.2,-4.11669579600002));
#326964=CARTESIAN_POINT('Ctrl Pts',(-0.097449618000055,5.2,-4.11669579600002));
#326965=CARTESIAN_POINT('Ctrl Pts',(-0.097449618000055,2.2,-4.11669579600002));
#326966=CARTESIAN_POINT('Ctrl Pts',(-0.0971814510000557,12.2,-4.11787768800002));
#326967=CARTESIAN_POINT('Ctrl Pts',(-0.0971814510000557,5.2,-4.11787768800002));
#326968=CARTESIAN_POINT('Ctrl Pts',(-0.0971814510000557,2.2,-4.11787768800002));
#326969=CARTESIAN_POINT('Ctrl Pts',(-0.096910718000055,12.2,-4.11906426500002));
#326970=CARTESIAN_POINT('Ctrl Pts',(-0.096910718000055,5.2,-4.11906426500002));
#326971=CARTESIAN_POINT('Ctrl Pts',(-0.096910718000055,2.2,-4.11906426500002));
#326972=CARTESIAN_POINT('Ctrl Pts',(-0.0966374100000567,12.2,-4.12025551500002));
#326973=CARTESIAN_POINT('Ctrl Pts',(-0.0966374100000567,5.2,-4.12025551500002));
#326974=CARTESIAN_POINT('Ctrl Pts',(-0.0966374100000567,2.2,-4.12025551500002));
#326975=CARTESIAN_POINT('Ctrl Pts',(-0.0963615180000554,12.2,-4.12145142700002));
#326976=CARTESIAN_POINT('Ctrl Pts',(-0.0963615180000554,5.2,-4.12145142700002));
#326977=CARTESIAN_POINT('Ctrl Pts',(-0.0963615180000554,2.2,-4.12145142700002));
#326978=CARTESIAN_POINT('Ctrl Pts',(-0.096083031000056,12.2,-4.12265198800001));
#326979=CARTESIAN_POINT('Ctrl Pts',(-0.096083031000056,5.2,-4.12265198800001));
#326980=CARTESIAN_POINT('Ctrl Pts',(-0.096083031000056,2.2,-4.12265198800001));
#326981=CARTESIAN_POINT('Ctrl Pts',(-0.0958019420000567,12.2,-4.12385718700001));
#326982=CARTESIAN_POINT('Ctrl Pts',(-0.0958019420000567,5.2,-4.12385718700001));
#326983=CARTESIAN_POINT('Ctrl Pts',(-0.0958019420000567,2.2,-4.12385718700001));
#326984=CARTESIAN_POINT('Ctrl Pts',(-0.0955182420000555,12.2,-4.12506701100002));
#326985=CARTESIAN_POINT('Ctrl Pts',(-0.0955182420000555,5.2,-4.12506701100002));
#326986=CARTESIAN_POINT('Ctrl Pts',(-0.0955182420000555,2.2,-4.12506701100002));
#326987=CARTESIAN_POINT('Ctrl Pts',(-0.0952319210000563,12.2,-4.12628144800002));
#326988=CARTESIAN_POINT('Ctrl Pts',(-0.0952319210000563,5.2,-4.12628144800002));
#326989=CARTESIAN_POINT('Ctrl Pts',(-0.0952319210000563,2.2,-4.12628144800002));
#326990=CARTESIAN_POINT('Ctrl Pts',(-0.094942972000055,12.2,-4.12750048600001));
#326991=CARTESIAN_POINT('Ctrl Pts',(-0.094942972000055,5.2,-4.12750048600001));
#326992=CARTESIAN_POINT('Ctrl Pts',(-0.094942972000055,2.2,-4.12750048600001));
#326993=CARTESIAN_POINT('Ctrl Pts',(-0.094651383000055,12.2,-4.12872411500001));
#326994=CARTESIAN_POINT('Ctrl Pts',(-0.094651383000055,5.2,-4.12872411500001));
#326995=CARTESIAN_POINT('Ctrl Pts',(-0.094651383000055,2.2,-4.12872411500001));
#326996=CARTESIAN_POINT('Ctrl Pts',(-0.0943571480000549,12.2,-4.12995232000001));
#326997=CARTESIAN_POINT('Ctrl Pts',(-0.0943571480000549,5.2,-4.12995232000001));
#326998=CARTESIAN_POINT('Ctrl Pts',(-0.0943571480000549,2.2,-4.12995232000001));
#326999=CARTESIAN_POINT('Ctrl Pts',(-0.0940602560000559,12.2,-4.13118509300002));
#327000=CARTESIAN_POINT('Ctrl Pts',(-0.0940602560000559,5.2,-4.13118509300002));
#327001=CARTESIAN_POINT('Ctrl Pts',(-0.0940602560000559,2.2,-4.13118509300002));
#327002=CARTESIAN_POINT('Ctrl Pts',(-0.0937607010000552,12.2,-4.13242241800001));
#327003=CARTESIAN_POINT('Ctrl Pts',(-0.0937607010000552,5.2,-4.13242241800001));
#327004=CARTESIAN_POINT('Ctrl Pts',(-0.0937607010000552,2.2,-4.13242241800001));
#327005=CARTESIAN_POINT('Ctrl Pts',(-0.0934584710000563,12.2,-4.13366428600002));
#327006=CARTESIAN_POINT('Ctrl Pts',(-0.0934584710000563,5.2,-4.13366428600002));
#327007=CARTESIAN_POINT('Ctrl Pts',(-0.0934584710000563,2.2,-4.13366428600002));
#327008=CARTESIAN_POINT('Ctrl Pts',(-0.0931535600000555,12.2,-4.13491068300001));
#327009=CARTESIAN_POINT('Ctrl Pts',(-0.0931535600000555,5.2,-4.13491068300001));
#327010=CARTESIAN_POINT('Ctrl Pts',(-0.0931535600000555,2.2,-4.13491068300001));
#327011=CARTESIAN_POINT('Ctrl Pts',(-0.0928459580000562,12.2,-4.13616159800001));
#327012=CARTESIAN_POINT('Ctrl Pts',(-0.0928459580000562,5.2,-4.13616159800001));
#327013=CARTESIAN_POINT('Ctrl Pts',(-0.0928459580000562,2.2,-4.13616159800001));
#327014=CARTESIAN_POINT('Ctrl Pts',(-0.0925356570000557,12.2,-4.13741702000001));
#327015=CARTESIAN_POINT('Ctrl Pts',(-0.0925356570000557,5.2,-4.13741702000001));
#327016=CARTESIAN_POINT('Ctrl Pts',(-0.0925356570000557,2.2,-4.13741702000001));
#327017=CARTESIAN_POINT('Ctrl Pts',(-0.0922226470000564,12.2,-4.13867693700002));
#327018=CARTESIAN_POINT('Ctrl Pts',(-0.0922226470000564,5.2,-4.13867693700002));
#327019=CARTESIAN_POINT('Ctrl Pts',(-0.0922226470000564,2.2,-4.13867693700002));
#327020=CARTESIAN_POINT('Ctrl Pts',(-0.0919069210000567,12.2,-4.13994133600001));
#327021=CARTESIAN_POINT('Ctrl Pts',(-0.0919069210000567,5.2,-4.13994133600001));
#327022=CARTESIAN_POINT('Ctrl Pts',(-0.0919069210000567,2.2,-4.13994133600001));
#327023=CARTESIAN_POINT('Ctrl Pts',(-0.0915884700000558,12.2,-4.14121020700001));
#327024=CARTESIAN_POINT('Ctrl Pts',(-0.0915884700000558,5.2,-4.14121020700001));
#327025=CARTESIAN_POINT('Ctrl Pts',(-0.0915884700000558,2.2,-4.14121020700001));
#327026=CARTESIAN_POINT('Ctrl Pts',(-0.0912672860000552,12.2,-4.14248353600001));
#327027=CARTESIAN_POINT('Ctrl Pts',(-0.0912672860000552,5.2,-4.14248353600001));
#327028=CARTESIAN_POINT('Ctrl Pts',(-0.0912672860000552,2.2,-4.14248353600001));
#327029=CARTESIAN_POINT('Ctrl Pts',(-0.0909433590000552,12.2,-4.14376131300001));
#327030=CARTESIAN_POINT('Ctrl Pts',(-0.0909433590000552,5.2,-4.14376131300001));
#327031=CARTESIAN_POINT('Ctrl Pts',(-0.0909433590000552,2.2,-4.14376131300001));
#327032=CARTESIAN_POINT('Ctrl Pts',(-0.0906166830000554,12.2,-4.14504352500002));
#327033=CARTESIAN_POINT('Ctrl Pts',(-0.0906166830000554,5.2,-4.14504352500002));
#327034=CARTESIAN_POINT('Ctrl Pts',(-0.0906166830000554,2.2,-4.14504352500002));
#327035=CARTESIAN_POINT('Ctrl Pts',(-0.0902872480000561,12.2,-4.14633016200002));
#327036=CARTESIAN_POINT('Ctrl Pts',(-0.0902872480000561,5.2,-4.14633016200002));
#327037=CARTESIAN_POINT('Ctrl Pts',(-0.0902872480000561,2.2,-4.14633016200002));
#327038=CARTESIAN_POINT('Ctrl Pts',(-0.0899550450000564,12.2,-4.14762121100001));
#327039=CARTESIAN_POINT('Ctrl Pts',(-0.0899550450000564,5.2,-4.14762121100001));
#327040=CARTESIAN_POINT('Ctrl Pts',(-0.0899550450000564,2.2,-4.14762121100001));
#327041=CARTESIAN_POINT('Ctrl Pts',(-0.0896200680000547,12.2,-4.14891666000001));
#327042=CARTESIAN_POINT('Ctrl Pts',(-0.0896200680000547,5.2,-4.14891666000001));
#327043=CARTESIAN_POINT('Ctrl Pts',(-0.0896200680000547,2.2,-4.14891666000001));
#327044=CARTESIAN_POINT('Ctrl Pts',(-0.0892823060000558,12.2,-4.15021649900002));
#327045=CARTESIAN_POINT('Ctrl Pts',(-0.0892823060000558,5.2,-4.15021649900002));
#327046=CARTESIAN_POINT('Ctrl Pts',(-0.0892823060000558,2.2,-4.15021649900002));
#327047=CARTESIAN_POINT('Ctrl Pts',(-0.0889417520000546,12.2,-4.15152071400001));
#327048=CARTESIAN_POINT('Ctrl Pts',(-0.0889417520000546,5.2,-4.15152071400001));
#327049=CARTESIAN_POINT('Ctrl Pts',(-0.0889417520000546,2.2,-4.15152071400001));
#327050=CARTESIAN_POINT('Ctrl Pts',(-0.0885983980000549,12.2,-4.15282929600002));
#327051=CARTESIAN_POINT('Ctrl Pts',(-0.0885983980000549,5.2,-4.15282929600002));
#327052=CARTESIAN_POINT('Ctrl Pts',(-0.0885983980000549,2.2,-4.15282929600002));
#327053=CARTESIAN_POINT('Ctrl Pts',(-0.0882522360000559,12.2,-4.15414223000001));
#327054=CARTESIAN_POINT('Ctrl Pts',(-0.0882522360000559,5.2,-4.15414223000001));
#327055=CARTESIAN_POINT('Ctrl Pts',(-0.0882522360000559,2.2,-4.15414223000001));
#327056=CARTESIAN_POINT('Ctrl Pts',(-0.0879032580000561,12.2,-4.15545950800002));
#327057=CARTESIAN_POINT('Ctrl Pts',(-0.0879032580000561,5.2,-4.15545950800002));
#327058=CARTESIAN_POINT('Ctrl Pts',(-0.0879032580000561,2.2,-4.15545950800002));
#327059=CARTESIAN_POINT('Ctrl Pts',(-0.0875514550000567,12.2,-4.15678111500001));
#327060=CARTESIAN_POINT('Ctrl Pts',(-0.0875514550000567,5.2,-4.15678111500001));
#327061=CARTESIAN_POINT('Ctrl Pts',(-0.0875514550000567,2.2,-4.15678111500001));
#327062=CARTESIAN_POINT('Ctrl Pts',(-0.087196818000056,12.2,-4.15810704200001));
#327063=CARTESIAN_POINT('Ctrl Pts',(-0.087196818000056,5.2,-4.15810704200001));
#327064=CARTESIAN_POINT('Ctrl Pts',(-0.087196818000056,2.2,-4.15810704200001));
#327065=CARTESIAN_POINT('Ctrl Pts',(-0.0868393420000557,12.2,-4.15943727600002));
#327066=CARTESIAN_POINT('Ctrl Pts',(-0.0868393420000557,5.2,-4.15943727600002));
#327067=CARTESIAN_POINT('Ctrl Pts',(-0.0868393420000557,2.2,-4.15943727600002));
#327068=CARTESIAN_POINT('Ctrl Pts',(-0.086479016000055,12.2,-4.16077180600002));
#327069=CARTESIAN_POINT('Ctrl Pts',(-0.086479016000055,5.2,-4.16077180600002));
#327070=CARTESIAN_POINT('Ctrl Pts',(-0.086479016000055,2.2,-4.16077180600002));
#327071=CARTESIAN_POINT('Ctrl Pts',(-0.0861158340000556,12.2,-4.16211062100002));
#327072=CARTESIAN_POINT('Ctrl Pts',(-0.0861158340000556,5.2,-4.16211062100002));
#327073=CARTESIAN_POINT('Ctrl Pts',(-0.0861158340000556,2.2,-4.16211062100002));
#327074=CARTESIAN_POINT('Ctrl Pts',(-0.0857497870000556,12.2,-4.16345370800002));
#327075=CARTESIAN_POINT('Ctrl Pts',(-0.0857497870000556,5.2,-4.16345370800002));
#327076=CARTESIAN_POINT('Ctrl Pts',(-0.0857497870000556,2.2,-4.16345370800002));
#327077=CARTESIAN_POINT('Ctrl Pts',(-0.0853808670000566,12.2,-4.16480105700002));
#327078=CARTESIAN_POINT('Ctrl Pts',(-0.0853808670000566,5.2,-4.16480105700002));
#327079=CARTESIAN_POINT('Ctrl Pts',(-0.0853808670000566,2.2,-4.16480105700002));
#327080=CARTESIAN_POINT('Ctrl Pts',(-0.0850090670000558,12.2,-4.16615265500001));
#327081=CARTESIAN_POINT('Ctrl Pts',(-0.0850090670000558,5.2,-4.16615265500001));
#327082=CARTESIAN_POINT('Ctrl Pts',(-0.0850090670000558,2.2,-4.16615265500001));
#327083=CARTESIAN_POINT('Ctrl Pts',(-0.0846343790000559,12.2,-4.16750849100001));
#327084=CARTESIAN_POINT('Ctrl Pts',(-0.0846343790000559,5.2,-4.16750849100001));
#327085=CARTESIAN_POINT('Ctrl Pts',(-0.0846343790000559,2.2,-4.16750849100001));
#327086=CARTESIAN_POINT('Ctrl Pts',(-0.084256794000056,12.2,-4.16886855400001));
#327087=CARTESIAN_POINT('Ctrl Pts',(-0.084256794000056,5.2,-4.16886855400001));
#327088=CARTESIAN_POINT('Ctrl Pts',(-0.084256794000056,2.2,-4.16886855400001));
#327089=CARTESIAN_POINT('Ctrl Pts',(-0.0838763050000557,12.2,-4.17023283200002));
#327090=CARTESIAN_POINT('Ctrl Pts',(-0.0838763050000557,5.2,-4.17023283200002));
#327091=CARTESIAN_POINT('Ctrl Pts',(-0.0838763050000557,2.2,-4.17023283200002));
#327092=CARTESIAN_POINT('Ctrl Pts',(-0.0834929050000566,12.2,-4.17160131500002));
#327093=CARTESIAN_POINT('Ctrl Pts',(-0.0834929050000566,5.2,-4.17160131500002));
#327094=CARTESIAN_POINT('Ctrl Pts',(-0.0834929050000566,2.2,-4.17160131500002));
#327095=CARTESIAN_POINT('Ctrl Pts',(-0.0831065840000556,12.2,-4.17297398900002));
#327096=CARTESIAN_POINT('Ctrl Pts',(-0.0831065840000556,5.2,-4.17297398900002));
#327097=CARTESIAN_POINT('Ctrl Pts',(-0.0831065840000556,2.2,-4.17297398900002));
#327098=CARTESIAN_POINT('Ctrl Pts',(-0.0827173360000566,12.2,-4.17435084500001));
#327099=CARTESIAN_POINT('Ctrl Pts',(-0.0827173360000566,5.2,-4.17435084500001));
#327100=CARTESIAN_POINT('Ctrl Pts',(-0.0827173360000566,2.2,-4.17435084500001));
#327101=CARTESIAN_POINT('Ctrl Pts',(-0.0823251550000559,12.2,-4.17573187000002));
#327102=CARTESIAN_POINT('Ctrl Pts',(-0.0823251550000559,5.2,-4.17573187000002));
#327103=CARTESIAN_POINT('Ctrl Pts',(-0.0823251550000559,2.2,-4.17573187000002));
#327104=CARTESIAN_POINT('Ctrl Pts',(-0.0819300290000557,12.2,-4.17711705300002));
#327105=CARTESIAN_POINT('Ctrl Pts',(-0.0819300290000557,5.2,-4.17711705300002));
#327106=CARTESIAN_POINT('Ctrl Pts',(-0.0819300290000557,2.2,-4.17711705300002));
#327107=CARTESIAN_POINT('Ctrl Pts',(-0.0815319540000559,12.2,-4.17850638300001));
#327108=CARTESIAN_POINT('Ctrl Pts',(-0.0815319540000559,5.2,-4.17850638300001));
#327109=CARTESIAN_POINT('Ctrl Pts',(-0.0815319540000559,2.2,-4.17850638300001));
#327110=CARTESIAN_POINT('Ctrl Pts',(-0.0811309220000567,12.2,-4.17989984800001));
#327111=CARTESIAN_POINT('Ctrl Pts',(-0.0811309220000567,5.2,-4.17989984800001));
#327112=CARTESIAN_POINT('Ctrl Pts',(-0.0811309220000567,2.2,-4.17989984800001));
#327113=CARTESIAN_POINT('Ctrl Pts',(-0.0807269240000552,12.2,-4.18129743700002));
#327114=CARTESIAN_POINT('Ctrl Pts',(-0.0807269240000552,5.2,-4.18129743700002));
#327115=CARTESIAN_POINT('Ctrl Pts',(-0.0807269240000552,2.2,-4.18129743700002));
#327116=CARTESIAN_POINT('Ctrl Pts',(-0.0803199530000565,12.2,-4.18269913800001));
#327117=CARTESIAN_POINT('Ctrl Pts',(-0.0803199530000565,5.2,-4.18269913800001));
#327118=CARTESIAN_POINT('Ctrl Pts',(-0.0803199530000565,2.2,-4.18269913800001));
#327119=CARTESIAN_POINT('Ctrl Pts',(-0.0799100020000565,12.2,-4.18410494100002));
#327120=CARTESIAN_POINT('Ctrl Pts',(-0.0799100020000565,5.2,-4.18410494100002));
#327121=CARTESIAN_POINT('Ctrl Pts',(-0.0799100020000565,2.2,-4.18410494100002));
#327122=CARTESIAN_POINT('Ctrl Pts',(-0.0794970630000569,12.2,-4.18551483500002));
#327123=CARTESIAN_POINT('Ctrl Pts',(-0.0794970630000569,5.2,-4.18551483500002));
#327124=CARTESIAN_POINT('Ctrl Pts',(-0.0794970630000569,2.2,-4.18551483500002));
#327125=CARTESIAN_POINT('Ctrl Pts',(-0.0790811280000547,12.2,-4.18692880600001));
#327126=CARTESIAN_POINT('Ctrl Pts',(-0.0790811280000547,5.2,-4.18692880600001));
#327127=CARTESIAN_POINT('Ctrl Pts',(-0.0790811280000547,2.2,-4.18692880600001));
#327128=CARTESIAN_POINT('Ctrl Pts',(-0.0786621920000563,12.2,-4.18834684500001));
#327129=CARTESIAN_POINT('Ctrl Pts',(-0.0786621920000563,5.2,-4.18834684500001));
#327130=CARTESIAN_POINT('Ctrl Pts',(-0.0786621920000563,2.2,-4.18834684500001));
#327131=CARTESIAN_POINT('Ctrl Pts',(-0.0782402460000564,12.2,-4.18976894000001));
#327132=CARTESIAN_POINT('Ctrl Pts',(-0.0782402460000564,5.2,-4.18976894000001));
#327133=CARTESIAN_POINT('Ctrl Pts',(-0.0782402460000564,2.2,-4.18976894000001));
#327134=CARTESIAN_POINT('Ctrl Pts',(-0.0778152820000566,12.2,-4.19119507900001));
#327135=CARTESIAN_POINT('Ctrl Pts',(-0.0778152820000566,5.2,-4.19119507900001));
#327136=CARTESIAN_POINT('Ctrl Pts',(-0.0778152820000566,2.2,-4.19119507900001));
#327137=CARTESIAN_POINT('Ctrl Pts',(-0.0773872930000563,12.2,-4.19262525300002));
#327138=CARTESIAN_POINT('Ctrl Pts',(-0.0773872930000563,5.2,-4.19262525300002));
#327139=CARTESIAN_POINT('Ctrl Pts',(-0.0773872930000563,2.2,-4.19262525300002));
#327140=CARTESIAN_POINT('Ctrl Pts',(-0.076956273000055,12.2,-4.19405944800001));
#327141=CARTESIAN_POINT('Ctrl Pts',(-0.076956273000055,5.2,-4.19405944800001));
#327142=CARTESIAN_POINT('Ctrl Pts',(-0.076956273000055,2.2,-4.19405944800001));
#327143=CARTESIAN_POINT('Ctrl Pts',(-0.0765222130000554,12.2,-4.19549765400001));
#327144=CARTESIAN_POINT('Ctrl Pts',(-0.0765222130000554,5.2,-4.19549765400001));
#327145=CARTESIAN_POINT('Ctrl Pts',(-0.0765222130000554,2.2,-4.19549765400001));
#327146=CARTESIAN_POINT('Ctrl Pts',(-0.0760851080000558,12.2,-4.19693986000001));
#327147=CARTESIAN_POINT('Ctrl Pts',(-0.0760851080000558,5.2,-4.19693986000001));
#327148=CARTESIAN_POINT('Ctrl Pts',(-0.0760851080000558,2.2,-4.19693986000001));
#327149=CARTESIAN_POINT('Ctrl Pts',(-0.0756449490000555,12.2,-4.19838605500002));
#327150=CARTESIAN_POINT('Ctrl Pts',(-0.0756449490000555,5.2,-4.19838605500002));
#327151=CARTESIAN_POINT('Ctrl Pts',(-0.0756449490000555,2.2,-4.19838605500002));
#327152=CARTESIAN_POINT('Ctrl Pts',(-0.0752017290000562,12.2,-4.19983622700002));
#327153=CARTESIAN_POINT('Ctrl Pts',(-0.0752017290000562,5.2,-4.19983622700002));
#327154=CARTESIAN_POINT('Ctrl Pts',(-0.0752017290000562,2.2,-4.19983622700002));
#327155=CARTESIAN_POINT('Ctrl Pts',(-0.0747554410000551,12.2,-4.20129036500001));
#327156=CARTESIAN_POINT('Ctrl Pts',(-0.0747554410000551,5.2,-4.20129036500001));
#327157=CARTESIAN_POINT('Ctrl Pts',(-0.0747554410000551,2.2,-4.20129036500001));
#327158=CARTESIAN_POINT('Ctrl Pts',(-0.074306079000056,12.2,-4.20274845800002));
#327159=CARTESIAN_POINT('Ctrl Pts',(-0.074306079000056,5.2,-4.20274845800002));
#327160=CARTESIAN_POINT('Ctrl Pts',(-0.074306079000056,2.2,-4.20274845800002));
#327161=CARTESIAN_POINT('Ctrl Pts',(-0.0738536340000551,12.2,-4.20421049600002));
#327162=CARTESIAN_POINT('Ctrl Pts',(-0.0738536340000551,5.2,-4.20421049600002));
#327163=CARTESIAN_POINT('Ctrl Pts',(-0.0738536340000551,2.2,-4.20421049600002));
#327164=CARTESIAN_POINT('Ctrl Pts',(-0.0733981010000551,12.2,-4.20567646600002));
#327165=CARTESIAN_POINT('Ctrl Pts',(-0.0733981010000551,5.2,-4.20567646600002));
#327166=CARTESIAN_POINT('Ctrl Pts',(-0.0733981010000551,2.2,-4.20567646600002));
#327167=CARTESIAN_POINT('Ctrl Pts',(-0.0729394710000564,12.2,-4.20714635600001));
#327168=CARTESIAN_POINT('Ctrl Pts',(-0.0729394710000564,5.2,-4.20714635600001));
#327169=CARTESIAN_POINT('Ctrl Pts',(-0.0729394710000564,2.2,-4.20714635600001));
#327170=CARTESIAN_POINT('Ctrl Pts',(-0.0724777380000563,12.2,-4.20862015900001));
#327171=CARTESIAN_POINT('Ctrl Pts',(-0.0724777380000563,5.2,-4.20862015900001));
#327172=CARTESIAN_POINT('Ctrl Pts',(-0.0724777380000563,2.2,-4.20862015900001));
#327173=CARTESIAN_POINT('Ctrl Pts',(-0.0720128950000554,12.2,-4.21009786100001));
#327174=CARTESIAN_POINT('Ctrl Pts',(-0.0720128950000554,5.2,-4.21009786100001));
#327175=CARTESIAN_POINT('Ctrl Pts',(-0.0720128950000554,2.2,-4.21009786100001));
#327176=CARTESIAN_POINT('Ctrl Pts',(-0.0715449360000553,12.2,-4.21157945000001));
#327177=CARTESIAN_POINT('Ctrl Pts',(-0.0715449360000553,5.2,-4.21157945000001));
#327178=CARTESIAN_POINT('Ctrl Pts',(-0.0715449360000553,2.2,-4.21157945000001));
#327179=CARTESIAN_POINT('Ctrl Pts',(-0.0710738530000565,12.2,-4.21306491700001));
#327180=CARTESIAN_POINT('Ctrl Pts',(-0.0710738530000565,5.2,-4.21306491700001));
#327181=CARTESIAN_POINT('Ctrl Pts',(-0.0710738530000565,2.2,-4.21306491700001));
#327182=CARTESIAN_POINT('Ctrl Pts',(-0.0705996390000563,12.2,-4.21455424900001));
#327183=CARTESIAN_POINT('Ctrl Pts',(-0.0705996390000563,5.2,-4.21455424900001));
#327184=CARTESIAN_POINT('Ctrl Pts',(-0.0705996390000563,2.2,-4.21455424900001));
#327185=CARTESIAN_POINT('Ctrl Pts',(-0.0701222880000552,12.2,-4.21604743700001));
#327186=CARTESIAN_POINT('Ctrl Pts',(-0.0701222880000552,5.2,-4.21604743700001));
#327187=CARTESIAN_POINT('Ctrl Pts',(-0.0701222880000552,2.2,-4.21604743700001));
#327188=CARTESIAN_POINT('Ctrl Pts',(-0.0696417920000558,12.2,-4.21754447000001));
#327189=CARTESIAN_POINT('Ctrl Pts',(-0.0696417920000558,5.2,-4.21754447000001));
#327190=CARTESIAN_POINT('Ctrl Pts',(-0.0696417920000558,2.2,-4.21754447000001));
#327191=CARTESIAN_POINT('Ctrl Pts',(-0.0691581460000557,12.2,-4.21904533400001));
#327192=CARTESIAN_POINT('Ctrl Pts',(-0.0691581460000557,5.2,-4.21904533400001));
#327193=CARTESIAN_POINT('Ctrl Pts',(-0.0691581460000557,2.2,-4.21904533400001));
#327194=CARTESIAN_POINT('Ctrl Pts',(-0.0686713410000561,12.2,-4.22055002100001));
#327195=CARTESIAN_POINT('Ctrl Pts',(-0.0686713410000561,5.2,-4.22055002100001));
#327196=CARTESIAN_POINT('Ctrl Pts',(-0.0686713410000561,2.2,-4.22055002100001));
#327197=CARTESIAN_POINT('Ctrl Pts',(-0.0681813710000567,12.2,-4.22205851900001));
#327198=CARTESIAN_POINT('Ctrl Pts',(-0.0681813710000567,5.2,-4.22205851900001));
#327199=CARTESIAN_POINT('Ctrl Pts',(-0.0681813710000567,2.2,-4.22205851900001));
#327200=CARTESIAN_POINT('Ctrl Pts',(-0.0676882310000571,12.2,-4.22357081700001));
#327201=CARTESIAN_POINT('Ctrl Pts',(-0.0676882310000571,5.2,-4.22357081700001));
#327202=CARTESIAN_POINT('Ctrl Pts',(-0.0676882310000571,2.2,-4.22357081700001));
#327203=CARTESIAN_POINT('Ctrl Pts',(-0.0671919130000554,12.2,-4.22508690400001));
#327204=CARTESIAN_POINT('Ctrl Pts',(-0.0671919130000554,5.2,-4.22508690400001));
#327205=CARTESIAN_POINT('Ctrl Pts',(-0.0671919130000554,2.2,-4.22508690400001));
#327206=CARTESIAN_POINT('Ctrl Pts',(-0.0666924100000566,12.2,-4.22660676900001));
#327207=CARTESIAN_POINT('Ctrl Pts',(-0.0666924100000566,5.2,-4.22660676900001));
#327208=CARTESIAN_POINT('Ctrl Pts',(-0.0666924100000566,2.2,-4.22660676900001));
#327209=CARTESIAN_POINT('Ctrl Pts',(-0.0661897150000546,12.2,-4.22813040100001));
#327210=CARTESIAN_POINT('Ctrl Pts',(-0.0661897150000546,5.2,-4.22813040100001));
#327211=CARTESIAN_POINT('Ctrl Pts',(-0.0661897150000546,2.2,-4.22813040100001));
#327212=CARTESIAN_POINT('Ctrl Pts',(-0.0656838230000556,12.2,-4.22965778900001));
#327213=CARTESIAN_POINT('Ctrl Pts',(-0.0656838230000556,5.2,-4.22965778900001));
#327214=CARTESIAN_POINT('Ctrl Pts',(-0.0656838230000556,2.2,-4.22965778900001));
#327215=CARTESIAN_POINT('Ctrl Pts',(-0.0651747270000558,12.2,-4.23118892200002));
#327216=CARTESIAN_POINT('Ctrl Pts',(-0.0651747270000558,5.2,-4.23118892200002));
#327217=CARTESIAN_POINT('Ctrl Pts',(-0.0651747270000558,2.2,-4.23118892200002));
#327218=CARTESIAN_POINT('Ctrl Pts',(-0.0646624190000556,12.2,-4.23272378900001));
#327219=CARTESIAN_POINT('Ctrl Pts',(-0.0646624190000556,5.2,-4.23272378900001));
#327220=CARTESIAN_POINT('Ctrl Pts',(-0.0646624190000556,2.2,-4.23272378900001));
#327221=CARTESIAN_POINT('Ctrl Pts',(-0.0641468940000556,12.2,-4.23426238000001));
#327222=CARTESIAN_POINT('Ctrl Pts',(-0.0641468940000556,5.2,-4.23426238000001));
#327223=CARTESIAN_POINT('Ctrl Pts',(-0.0641468940000556,2.2,-4.23426238000001));
#327224=CARTESIAN_POINT('Ctrl Pts',(-0.0636281460000554,12.2,-4.23580468300001));
#327225=CARTESIAN_POINT('Ctrl Pts',(-0.0636281460000554,5.2,-4.23580468300001));
#327226=CARTESIAN_POINT('Ctrl Pts',(-0.0636281460000554,2.2,-4.23580468300001));
#327227=CARTESIAN_POINT('Ctrl Pts',(-0.0631061670000555,12.2,-4.23735068900001));
#327228=CARTESIAN_POINT('Ctrl Pts',(-0.0631061670000555,5.2,-4.23735068900001));
#327229=CARTESIAN_POINT('Ctrl Pts',(-0.0631061670000555,2.2,-4.23735068900001));
#327230=CARTESIAN_POINT('Ctrl Pts',(-0.0625809500000563,12.2,-4.23890038400002));
#327231=CARTESIAN_POINT('Ctrl Pts',(-0.0625809500000563,5.2,-4.23890038400002));
#327232=CARTESIAN_POINT('Ctrl Pts',(-0.0625809500000563,2.2,-4.23890038400002));
#327233=CARTESIAN_POINT('Ctrl Pts',(-0.0620524920000565,12.2,-4.24045376000001));
#327234=CARTESIAN_POINT('Ctrl Pts',(-0.0620524920000565,5.2,-4.24045376000001));
#327235=CARTESIAN_POINT('Ctrl Pts',(-0.0620524920000565,2.2,-4.24045376000001));
#327236=CARTESIAN_POINT('Ctrl Pts',(-0.0615207820000552,12.2,-4.24201080300001));
#327237=CARTESIAN_POINT('Ctrl Pts',(-0.0615207820000552,5.2,-4.24201080300001));
#327238=CARTESIAN_POINT('Ctrl Pts',(-0.0615207820000552,2.2,-4.24201080300001));
#327239=CARTESIAN_POINT('Ctrl Pts',(-0.0609858180000555,12.2,-4.24357150600001));
#327240=CARTESIAN_POINT('Ctrl Pts',(-0.0609858180000555,5.2,-4.24357150600001));
#327241=CARTESIAN_POINT('Ctrl Pts',(-0.0609858180000555,2.2,-4.24357150600001));
#327242=CARTESIAN_POINT('Ctrl Pts',(-0.0604475910000557,12.2,-4.24513585500002));
#327243=CARTESIAN_POINT('Ctrl Pts',(-0.0604475910000557,5.2,-4.24513585500002));
#327244=CARTESIAN_POINT('Ctrl Pts',(-0.0604475910000557,2.2,-4.24513585500002));
#327245=CARTESIAN_POINT('Ctrl Pts',(-0.0599060960000553,12.2,-4.24670384200001));
#327246=CARTESIAN_POINT('Ctrl Pts',(-0.0599060960000553,5.2,-4.24670384200001));
#327247=CARTESIAN_POINT('Ctrl Pts',(-0.0599060960000553,2.2,-4.24670384200001));
#327248=CARTESIAN_POINT('Ctrl Pts',(-0.0593613260000558,12.2,-4.24827545300001));
#327249=CARTESIAN_POINT('Ctrl Pts',(-0.0593613260000558,5.2,-4.24827545300001));
#327250=CARTESIAN_POINT('Ctrl Pts',(-0.0593613260000558,2.2,-4.24827545300001));
#327251=CARTESIAN_POINT('Ctrl Pts',(-0.0588132750000547,12.2,-4.24985068100002));
#327252=CARTESIAN_POINT('Ctrl Pts',(-0.0588132750000547,5.2,-4.24985068100002));
#327253=CARTESIAN_POINT('Ctrl Pts',(-0.0588132750000547,2.2,-4.24985068100002));
#327254=CARTESIAN_POINT('Ctrl Pts',(-0.0582619360000558,12.2,-4.25142951200002));
#327255=CARTESIAN_POINT('Ctrl Pts',(-0.0582619360000558,5.2,-4.25142951200002));
#327256=CARTESIAN_POINT('Ctrl Pts',(-0.0582619360000558,2.2,-4.25142951200002));
#327257=CARTESIAN_POINT('Ctrl Pts',(-0.0577073040000553,12.2,-4.25301193500002));
#327258=CARTESIAN_POINT('Ctrl Pts',(-0.0577073040000553,5.2,-4.25301193500002));
#327259=CARTESIAN_POINT('Ctrl Pts',(-0.0577073040000553,2.2,-4.25301193500002));
#327260=CARTESIAN_POINT('Ctrl Pts',(-0.057149372000056,12.2,-4.25459794200002));
#327261=CARTESIAN_POINT('Ctrl Pts',(-0.057149372000056,5.2,-4.25459794200002));
#327262=CARTESIAN_POINT('Ctrl Pts',(-0.057149372000056,2.2,-4.25459794200002));
#327263=CARTESIAN_POINT('Ctrl Pts',(-0.0565881350000552,12.2,-4.25618752100001));
#327264=CARTESIAN_POINT('Ctrl Pts',(-0.0565881350000552,5.2,-4.25618752100001));
#327265=CARTESIAN_POINT('Ctrl Pts',(-0.0565881350000552,2.2,-4.25618752100001));
#327266=CARTESIAN_POINT('Ctrl Pts',(-0.0560235860000546,12.2,-4.25778066100001));
#327267=CARTESIAN_POINT('Ctrl Pts',(-0.0560235860000546,5.2,-4.25778066100001));
#327268=CARTESIAN_POINT('Ctrl Pts',(-0.0560235860000546,2.2,-4.25778066100001));
#327269=CARTESIAN_POINT('Ctrl Pts',(-0.0554557180000559,12.2,-4.25937735100002));
#327270=CARTESIAN_POINT('Ctrl Pts',(-0.0554557180000559,5.2,-4.25937735100002));
#327271=CARTESIAN_POINT('Ctrl Pts',(-0.0554557180000559,2.2,-4.25937735100002));
#327272=CARTESIAN_POINT('Ctrl Pts',(-0.0548845270000553,12.2,-4.26097758100001));
#327273=CARTESIAN_POINT('Ctrl Pts',(-0.0548845270000553,5.2,-4.26097758100001));
#327274=CARTESIAN_POINT('Ctrl Pts',(-0.0548845270000553,2.2,-4.26097758100001));
#327275=CARTESIAN_POINT('Ctrl Pts',(-0.0543100050000567,12.2,-4.26258134100001));
#327276=CARTESIAN_POINT('Ctrl Pts',(-0.0543100050000567,5.2,-4.26258134100001));
#327277=CARTESIAN_POINT('Ctrl Pts',(-0.0543100050000567,2.2,-4.26258134100001));
#327278=CARTESIAN_POINT('Ctrl Pts',(-0.0537321480000563,12.2,-4.26418861700002));
#327279=CARTESIAN_POINT('Ctrl Pts',(-0.0537321480000563,5.2,-4.26418861700002));
#327280=CARTESIAN_POINT('Ctrl Pts',(-0.0537321480000563,2.2,-4.26418861700002));
#327281=CARTESIAN_POINT('Ctrl Pts',(-0.0531509480000558,12.2,-4.26579940300002));
#327282=CARTESIAN_POINT('Ctrl Pts',(-0.0531509480000558,5.2,-4.26579940300002));
#327283=CARTESIAN_POINT('Ctrl Pts',(-0.0531509480000558,2.2,-4.26579940300002));
#327284=CARTESIAN_POINT('Ctrl Pts',(-0.0525664010000571,12.2,-4.26741368500001));
#327285=CARTESIAN_POINT('Ctrl Pts',(-0.0525664010000571,5.2,-4.26741368500001));
#327286=CARTESIAN_POINT('Ctrl Pts',(-0.0525664010000571,2.2,-4.26741368500001));
#327287=CARTESIAN_POINT('Ctrl Pts',(-0.051978500000055,12.2,-4.26903145300002));
#327288=CARTESIAN_POINT('Ctrl Pts',(-0.051978500000055,5.2,-4.26903145300002));
#327289=CARTESIAN_POINT('Ctrl Pts',(-0.051978500000055,2.2,-4.26903145300002));
#327290=CARTESIAN_POINT('Ctrl Pts',(-0.0513872380000546,12.2,-4.27065269700002));
#327291=CARTESIAN_POINT('Ctrl Pts',(-0.0513872380000546,5.2,-4.27065269700002));
#327292=CARTESIAN_POINT('Ctrl Pts',(-0.0513872380000546,2.2,-4.27065269700002));
#327293=CARTESIAN_POINT('Ctrl Pts',(-0.0507926120000557,12.2,-4.27227740600001));
#327294=CARTESIAN_POINT('Ctrl Pts',(-0.0507926120000557,5.2,-4.27227740600001));
#327295=CARTESIAN_POINT('Ctrl Pts',(-0.0507926120000557,2.2,-4.27227740600001));
#327296=CARTESIAN_POINT('Ctrl Pts',(-0.0501946120000552,12.2,-4.27390556900002));
#327297=CARTESIAN_POINT('Ctrl Pts',(-0.0501946120000552,5.2,-4.27390556900002));
#327298=CARTESIAN_POINT('Ctrl Pts',(-0.0501946120000552,2.2,-4.27390556900002));
#327299=CARTESIAN_POINT('Ctrl Pts',(-0.0495932360000562,12.2,-4.27553717600002));
#327300=CARTESIAN_POINT('Ctrl Pts',(-0.0495932360000562,5.2,-4.27553717600002));
#327301=CARTESIAN_POINT('Ctrl Pts',(-0.0495932360000562,2.2,-4.27553717600002));
#327302=CARTESIAN_POINT('Ctrl Pts',(-0.048988477000057,12.2,-4.27717221600002));
#327303=CARTESIAN_POINT('Ctrl Pts',(-0.048988477000057,5.2,-4.27717221600002));
#327304=CARTESIAN_POINT('Ctrl Pts',(-0.048988477000057,2.2,-4.27717221600002));
#327305=CARTESIAN_POINT('Ctrl Pts',(-0.0483803290000551,12.2,-4.27881068000001));
#327306=CARTESIAN_POINT('Ctrl Pts',(-0.0483803290000551,5.2,-4.27881068000001));
#327307=CARTESIAN_POINT('Ctrl Pts',(-0.0483803290000551,2.2,-4.27881068000001));
#327308=CARTESIAN_POINT('Ctrl Pts',(-0.0477687860000553,12.2,-4.28045255500002));
#327309=CARTESIAN_POINT('Ctrl Pts',(-0.0477687860000553,5.2,-4.28045255500002));
#327310=CARTESIAN_POINT('Ctrl Pts',(-0.0477687860000553,2.2,-4.28045255500002));
#327311=CARTESIAN_POINT('Ctrl Pts',(-0.047153842000055,12.2,-4.28209783100002));
#327312=CARTESIAN_POINT('Ctrl Pts',(-0.047153842000055,5.2,-4.28209783100002));
#327313=CARTESIAN_POINT('Ctrl Pts',(-0.047153842000055,2.2,-4.28209783100002));
#327314=CARTESIAN_POINT('Ctrl Pts',(-0.0465354920000549,12.2,-4.28374649900002));
#327315=CARTESIAN_POINT('Ctrl Pts',(-0.0465354920000549,5.2,-4.28374649900002));
#327316=CARTESIAN_POINT('Ctrl Pts',(-0.0465354920000549,2.2,-4.28374649900002));
#327317=CARTESIAN_POINT('Ctrl Pts',(-0.0459137300000556,12.2,-4.28539854700002));
#327318=CARTESIAN_POINT('Ctrl Pts',(-0.0459137300000556,5.2,-4.28539854700002));
#327319=CARTESIAN_POINT('Ctrl Pts',(-0.0459137300000556,2.2,-4.28539854700002));
#327320=CARTESIAN_POINT('Ctrl Pts',(-0.0452885500000555,12.2,-4.28705396500002));
#327321=CARTESIAN_POINT('Ctrl Pts',(-0.0452885500000555,5.2,-4.28705396500002));
#327322=CARTESIAN_POINT('Ctrl Pts',(-0.0452885500000555,2.2,-4.28705396500002));
#327323=CARTESIAN_POINT('Ctrl Pts',(-0.0446599480000565,12.2,-4.28871274200001));
#327324=CARTESIAN_POINT('Ctrl Pts',(-0.0446599480000565,5.2,-4.28871274200001));
#327325=CARTESIAN_POINT('Ctrl Pts',(-0.0446599480000565,2.2,-4.28871274200001));
#327326=CARTESIAN_POINT('Ctrl Pts',(-0.0440279170000557,12.2,-4.29037486800001));
#327327=CARTESIAN_POINT('Ctrl Pts',(-0.0440279170000557,5.2,-4.29037486800001));
#327328=CARTESIAN_POINT('Ctrl Pts',(-0.0440279170000557,2.2,-4.29037486800001));
#327329=CARTESIAN_POINT('Ctrl Pts',(-0.043392450000056,12.2,-4.29204033300001));
#327330=CARTESIAN_POINT('Ctrl Pts',(-0.043392450000056,5.2,-4.29204033300001));
#327331=CARTESIAN_POINT('Ctrl Pts',(-0.043392450000056,2.2,-4.29204033300001));
#327332=CARTESIAN_POINT('Ctrl Pts',(-0.0427535450000571,12.2,-4.29370912600001));
#327333=CARTESIAN_POINT('Ctrl Pts',(-0.0427535450000571,5.2,-4.29370912600001));
#327334=CARTESIAN_POINT('Ctrl Pts',(-0.0427535450000571,2.2,-4.29370912600001));
#327335=CARTESIAN_POINT('Ctrl Pts',(-0.0421111930000551,12.2,-4.29538123500001));
#327336=CARTESIAN_POINT('Ctrl Pts',(-0.0421111930000551,5.2,-4.29538123500001));
#327337=CARTESIAN_POINT('Ctrl Pts',(-0.0421111930000551,2.2,-4.29538123500001));
#327338=CARTESIAN_POINT('Ctrl Pts',(-0.0414653900000561,12.2,-4.29705665200002));
#327339=CARTESIAN_POINT('Ctrl Pts',(-0.0414653900000561,5.2,-4.29705665200002));
#327340=CARTESIAN_POINT('Ctrl Pts',(-0.0414653900000561,2.2,-4.29705665200002));
#327341=CARTESIAN_POINT('Ctrl Pts',(-0.0408161310000566,12.2,-4.29873536500001));
#327342=CARTESIAN_POINT('Ctrl Pts',(-0.0408161310000566,5.2,-4.29873536500001));
#327343=CARTESIAN_POINT('Ctrl Pts',(-0.0408161310000566,2.2,-4.29873536500001));
#327344=CARTESIAN_POINT('Ctrl Pts',(-0.0401634110000571,12.2,-4.30041736500002));
#327345=CARTESIAN_POINT('Ctrl Pts',(-0.0401634110000571,5.2,-4.30041736500002));
#327346=CARTESIAN_POINT('Ctrl Pts',(-0.0401634110000571,2.2,-4.30041736500002));
#327347=CARTESIAN_POINT('Ctrl Pts',(-0.0395072220000559,12.2,-4.30210263900001));
#327348=CARTESIAN_POINT('Ctrl Pts',(-0.0395072220000559,5.2,-4.30210263900001));
#327349=CARTESIAN_POINT('Ctrl Pts',(-0.0395072220000559,2.2,-4.30210263900001));
#327350=CARTESIAN_POINT('Ctrl Pts',(-0.038847561000056,12.2,-4.30379117900001));
#327351=CARTESIAN_POINT('Ctrl Pts',(-0.038847561000056,5.2,-4.30379117900001));
#327352=CARTESIAN_POINT('Ctrl Pts',(-0.038847561000056,2.2,-4.30379117900001));
#327353=CARTESIAN_POINT('Ctrl Pts',(-0.0381844200000547,12.2,-4.30548297500001));
#327354=CARTESIAN_POINT('Ctrl Pts',(-0.0381844200000547,5.2,-4.30548297500001));
#327355=CARTESIAN_POINT('Ctrl Pts',(-0.0381844200000547,2.2,-4.30548297500001));
#327356=CARTESIAN_POINT('Ctrl Pts',(-0.0375177970000562,12.2,-4.30717801400001));
#327357=CARTESIAN_POINT('Ctrl Pts',(-0.0375177970000562,5.2,-4.30717801400001));
#327358=CARTESIAN_POINT('Ctrl Pts',(-0.0375177970000562,2.2,-4.30717801400001));
#327359=CARTESIAN_POINT('Ctrl Pts',(-0.0368476850000565,12.2,-4.30887628700001));
#327360=CARTESIAN_POINT('Ctrl Pts',(-0.0368476850000565,5.2,-4.30887628700001));
#327361=CARTESIAN_POINT('Ctrl Pts',(-0.0368476850000565,2.2,-4.30887628700001));
#327362=CARTESIAN_POINT('Ctrl Pts',(-0.0361740780000552,12.2,-4.31057778500001));
#327363=CARTESIAN_POINT('Ctrl Pts',(-0.0361740780000552,5.2,-4.31057778500001));
#327364=CARTESIAN_POINT('Ctrl Pts',(-0.0361740780000552,2.2,-4.31057778500001));
#327365=CARTESIAN_POINT('Ctrl Pts',(-0.0354969720000553,12.2,-4.31228249500001));
#327366=CARTESIAN_POINT('Ctrl Pts',(-0.0354969720000553,5.2,-4.31228249500001));
#327367=CARTESIAN_POINT('Ctrl Pts',(-0.0354969720000553,2.2,-4.31228249500001));
#327368=CARTESIAN_POINT('Ctrl Pts',(-0.0348163610000551,12.2,-4.31399040900001));
#327369=CARTESIAN_POINT('Ctrl Pts',(-0.0348163610000551,5.2,-4.31399040900001));
#327370=CARTESIAN_POINT('Ctrl Pts',(-0.0348163610000551,2.2,-4.31399040900001));
#327371=CARTESIAN_POINT('Ctrl Pts',(-0.0341322390000565,12.2,-4.31570151500001));
#327372=CARTESIAN_POINT('Ctrl Pts',(-0.0341322390000565,5.2,-4.31570151500001));
#327373=CARTESIAN_POINT('Ctrl Pts',(-0.0341322390000565,2.2,-4.31570151500001));
#327374=CARTESIAN_POINT('Ctrl Pts',(-0.0334446030000557,12.2,-4.31741580200002));
#327375=CARTESIAN_POINT('Ctrl Pts',(-0.0334446030000557,5.2,-4.31741580200002));
#327376=CARTESIAN_POINT('Ctrl Pts',(-0.0334446030000557,2.2,-4.31741580200002));
#327377=CARTESIAN_POINT('Ctrl Pts',(-0.0327534450000555,12.2,-4.31913326200001));
#327378=CARTESIAN_POINT('Ctrl Pts',(-0.0327534450000555,5.2,-4.31913326200001));
#327379=CARTESIAN_POINT('Ctrl Pts',(-0.0327534450000555,2.2,-4.31913326200001));
#327380=CARTESIAN_POINT('Ctrl Pts',(-0.0320587610000567,12.2,-4.32085388300001));
#327381=CARTESIAN_POINT('Ctrl Pts',(-0.0320587610000567,5.2,-4.32085388300001));
#327382=CARTESIAN_POINT('Ctrl Pts',(-0.0320587610000567,2.2,-4.32085388300001));
#327383=CARTESIAN_POINT('Ctrl Pts',(-0.0313605480000556,12.2,-4.32257765700002));
#327384=CARTESIAN_POINT('Ctrl Pts',(-0.0313605480000556,5.2,-4.32257765700002));
#327385=CARTESIAN_POINT('Ctrl Pts',(-0.0313605480000556,2.2,-4.32257765700002));
#327386=CARTESIAN_POINT('Ctrl Pts',(-0.030658797000056,12.2,-4.32430457100001));
#327387=CARTESIAN_POINT('Ctrl Pts',(-0.030658797000056,5.2,-4.32430457100001));
#327388=CARTESIAN_POINT('Ctrl Pts',(-0.030658797000056,2.2,-4.32430457100001));
#327389=CARTESIAN_POINT('Ctrl Pts',(-0.0299535050000566,12.2,-4.32603461600001));
#327390=CARTESIAN_POINT('Ctrl Pts',(-0.0299535050000566,5.2,-4.32603461600001));
#327391=CARTESIAN_POINT('Ctrl Pts',(-0.0299535050000566,2.2,-4.32603461600001));
#327392=CARTESIAN_POINT('Ctrl Pts',(-0.0292446680000558,12.2,-4.32776778100001));
#327393=CARTESIAN_POINT('Ctrl Pts',(-0.0292446680000558,5.2,-4.32776778100001));
#327394=CARTESIAN_POINT('Ctrl Pts',(-0.0292446680000558,2.2,-4.32776778100001));
#327395=CARTESIAN_POINT('Ctrl Pts',(-0.0285322780000552,12.2,-4.32950405600002));
#327396=CARTESIAN_POINT('Ctrl Pts',(-0.0285322780000552,5.2,-4.32950405600002));
#327397=CARTESIAN_POINT('Ctrl Pts',(-0.0285322780000552,2.2,-4.32950405600002));
#327398=CARTESIAN_POINT('Ctrl Pts',(-0.0278163330000558,12.2,-4.33124343200001));
#327399=CARTESIAN_POINT('Ctrl Pts',(-0.0278163330000558,5.2,-4.33124343200001));
#327400=CARTESIAN_POINT('Ctrl Pts',(-0.0278163330000558,2.2,-4.33124343200001));
#327401=CARTESIAN_POINT('Ctrl Pts',(-0.0270968250000558,12.2,-4.33298589700001));
#327402=CARTESIAN_POINT('Ctrl Pts',(-0.0270968250000558,5.2,-4.33298589700001));
#327403=CARTESIAN_POINT('Ctrl Pts',(-0.0270968250000558,2.2,-4.33298589700001));
#327404=CARTESIAN_POINT('Ctrl Pts',(-0.0263737510000561,12.2,-4.33473144100001));
#327405=CARTESIAN_POINT('Ctrl Pts',(-0.0263737510000561,5.2,-4.33473144100001));
#327406=CARTESIAN_POINT('Ctrl Pts',(-0.0263737510000561,2.2,-4.33473144100001));
#327407=CARTESIAN_POINT('Ctrl Pts',(-0.0256471060000563,12.2,-4.33648005500002));
#327408=CARTESIAN_POINT('Ctrl Pts',(-0.0256471060000563,5.2,-4.33648005500002));
#327409=CARTESIAN_POINT('Ctrl Pts',(-0.0256471060000563,2.2,-4.33648005500002));
#327410=CARTESIAN_POINT('Ctrl Pts',(-0.0249168840000558,12.2,-4.33823172900001));
#327411=CARTESIAN_POINT('Ctrl Pts',(-0.0249168840000558,5.2,-4.33823172900001));
#327412=CARTESIAN_POINT('Ctrl Pts',(-0.0249168840000558,2.2,-4.33823172900001));
#327413=CARTESIAN_POINT('Ctrl Pts',(-0.0241830820000555,12.2,-4.33998645000001));
#327414=CARTESIAN_POINT('Ctrl Pts',(-0.0241830820000555,5.2,-4.33998645000001));
#327415=CARTESIAN_POINT('Ctrl Pts',(-0.0241830820000555,2.2,-4.33998645000001));
#327416=CARTESIAN_POINT('Ctrl Pts',(-0.0234456920000559,12.2,-4.34174421100002));
#327417=CARTESIAN_POINT('Ctrl Pts',(-0.0234456920000559,5.2,-4.34174421100002));
#327418=CARTESIAN_POINT('Ctrl Pts',(-0.0234456920000559,2.2,-4.34174421100002));
#327419=CARTESIAN_POINT('Ctrl Pts',(-0.0227047110000556,12.2,-4.34350500000001));
#327420=CARTESIAN_POINT('Ctrl Pts',(-0.0227047110000556,5.2,-4.34350500000001));
#327421=CARTESIAN_POINT('Ctrl Pts',(-0.0227047110000556,2.2,-4.34350500000001));
#327422=CARTESIAN_POINT('Ctrl Pts',(-0.0219601350000553,12.2,-4.34526880800002));
#327423=CARTESIAN_POINT('Ctrl Pts',(-0.0219601350000553,5.2,-4.34526880800002));
#327424=CARTESIAN_POINT('Ctrl Pts',(-0.0219601350000553,2.2,-4.34526880800002));
#327425=CARTESIAN_POINT('Ctrl Pts',(-0.0212119570000546,12.2,-4.34703562300002));
#327426=CARTESIAN_POINT('Ctrl Pts',(-0.0212119570000546,5.2,-4.34703562300002));
#327427=CARTESIAN_POINT('Ctrl Pts',(-0.0212119570000546,2.2,-4.34703562300002));
#327428=CARTESIAN_POINT('Ctrl Pts',(-0.0204601740000554,12.2,-4.34880543700002));
#327429=CARTESIAN_POINT('Ctrl Pts',(-0.0204601740000554,5.2,-4.34880543700002));
#327430=CARTESIAN_POINT('Ctrl Pts',(-0.0204601740000554,2.2,-4.34880543700002));
#327431=CARTESIAN_POINT('Ctrl Pts',(-0.019704779000056,12.2,-4.35057823800001));
#327432=CARTESIAN_POINT('Ctrl Pts',(-0.019704779000056,5.2,-4.35057823800001));
#327433=CARTESIAN_POINT('Ctrl Pts',(-0.019704779000056,2.2,-4.35057823800001));
#327434=CARTESIAN_POINT('Ctrl Pts',(-0.018945770000055,12.2,-4.35235401800002));
#327435=CARTESIAN_POINT('Ctrl Pts',(-0.018945770000055,5.2,-4.35235401800002));
#327436=CARTESIAN_POINT('Ctrl Pts',(-0.018945770000055,2.2,-4.35235401800002));
#327437=CARTESIAN_POINT('Ctrl Pts',(-0.0181831400000565,12.2,-4.35413276500002));
#327438=CARTESIAN_POINT('Ctrl Pts',(-0.0181831400000565,5.2,-4.35413276500002));
#327439=CARTESIAN_POINT('Ctrl Pts',(-0.0181831400000565,2.2,-4.35413276500002));
#327440=CARTESIAN_POINT('Ctrl Pts',(-0.0174168870000557,12.2,-4.35591446900002));
#327441=CARTESIAN_POINT('Ctrl Pts',(-0.0174168870000557,5.2,-4.35591446900002));
#327442=CARTESIAN_POINT('Ctrl Pts',(-0.0174168870000557,2.2,-4.35591446900002));
#327443=CARTESIAN_POINT('Ctrl Pts',(-0.0166470020000553,12.2,-4.35769912100001));
#327444=CARTESIAN_POINT('Ctrl Pts',(-0.0166470020000553,5.2,-4.35769912100001));
#327445=CARTESIAN_POINT('Ctrl Pts',(-0.0166470020000553,2.2,-4.35769912100001));
#327446=CARTESIAN_POINT('Ctrl Pts',(-0.0158734840000552,12.2,-4.35948671100002));
#327447=CARTESIAN_POINT('Ctrl Pts',(-0.0158734840000552,5.2,-4.35948671100002));
#327448=CARTESIAN_POINT('Ctrl Pts',(-0.0158734840000552,2.2,-4.35948671100002));
#327449=CARTESIAN_POINT('Ctrl Pts',(-0.0150963270000548,12.2,-4.36127722800002));
#327450=CARTESIAN_POINT('Ctrl Pts',(-0.0150963270000548,5.2,-4.36127722800002));
#327451=CARTESIAN_POINT('Ctrl Pts',(-0.0150963270000548,2.2,-4.36127722800002));
#327452=CARTESIAN_POINT('Ctrl Pts',(-0.014315526000056,12.2,-4.36307066200001));
#327453=CARTESIAN_POINT('Ctrl Pts',(-0.014315526000056,5.2,-4.36307066200001));
#327454=CARTESIAN_POINT('Ctrl Pts',(-0.014315526000056,2.2,-4.36307066200001));
#327455=CARTESIAN_POINT('Ctrl Pts',(-0.0135310770000563,12.2,-4.36486700300001));
#327456=CARTESIAN_POINT('Ctrl Pts',(-0.0135310770000563,5.2,-4.36486700300001));
#327457=CARTESIAN_POINT('Ctrl Pts',(-0.0135310770000563,2.2,-4.36486700300001));
#327458=CARTESIAN_POINT('Ctrl Pts',(-0.0127429750000552,12.2,-4.36666624200001));
#327459=CARTESIAN_POINT('Ctrl Pts',(-0.0127429750000552,5.2,-4.36666624200001));
#327460=CARTESIAN_POINT('Ctrl Pts',(-0.0127429750000552,2.2,-4.36666624200001));
#327461=CARTESIAN_POINT('Ctrl Pts',(-0.0119512150000567,12.2,-4.36846836700001));
#327462=CARTESIAN_POINT('Ctrl Pts',(-0.0119512150000567,5.2,-4.36846836700001));
#327463=CARTESIAN_POINT('Ctrl Pts',(-0.0119512150000567,2.2,-4.36846836700001));
#327464=CARTESIAN_POINT('Ctrl Pts',(-0.0111557950000552,12.2,-4.37027336900002));
#327465=CARTESIAN_POINT('Ctrl Pts',(-0.0111557950000552,5.2,-4.37027336900002));
#327466=CARTESIAN_POINT('Ctrl Pts',(-0.0111557950000552,2.2,-4.37027336900002));
#327467=CARTESIAN_POINT('Ctrl Pts',(-0.0103567060000565,12.2,-4.37208123900001));
#327468=CARTESIAN_POINT('Ctrl Pts',(-0.0103567060000565,5.2,-4.37208123900001));
#327469=CARTESIAN_POINT('Ctrl Pts',(-0.0103567060000565,2.2,-4.37208123900001));
#327470=CARTESIAN_POINT('Ctrl Pts',(-0.00955394600005489,12.2,-4.37389196600002));
#327471=CARTESIAN_POINT('Ctrl Pts',(-0.00955394600005489,5.2,-4.37389196600002));
#327472=CARTESIAN_POINT('Ctrl Pts',(-0.00955394600005489,2.2,-4.37389196600002));
#327473=CARTESIAN_POINT('Ctrl Pts',(-0.00874751200005575,12.2,-4.37570554000001));
#327474=CARTESIAN_POINT('Ctrl Pts',(-0.00874751200005575,5.2,-4.37570554000001));
#327475=CARTESIAN_POINT('Ctrl Pts',(-0.00874751200005575,2.2,-4.37570554000001));
#327476=CARTESIAN_POINT('Ctrl Pts',(-0.00793739600005617,12.2,-4.37752195100002));
#327477=CARTESIAN_POINT('Ctrl Pts',(-0.00793739600005617,5.2,-4.37752195100002));
#327478=CARTESIAN_POINT('Ctrl Pts',(-0.00793739600005617,2.2,-4.37752195100002));
#327479=CARTESIAN_POINT('Ctrl Pts',(-0.00712359700005606,12.2,-4.37934118900001));
#327480=CARTESIAN_POINT('Ctrl Pts',(-0.00712359700005606,5.2,-4.37934118900001));
#327481=CARTESIAN_POINT('Ctrl Pts',(-0.00712359700005606,2.2,-4.37934118900001));
#327482=CARTESIAN_POINT('Ctrl Pts',(-0.00630610800005483,12.2,-4.38116324500001));
#327483=CARTESIAN_POINT('Ctrl Pts',(-0.00630610800005483,5.2,-4.38116324500001));
#327484=CARTESIAN_POINT('Ctrl Pts',(-0.00630610800005483,2.2,-4.38116324500001));
#327485=CARTESIAN_POINT('Ctrl Pts',(-0.00548492600005558,12.2,-4.38298810700001));
#327486=CARTESIAN_POINT('Ctrl Pts',(-0.00548492600005558,5.2,-4.38298810700001));
#327487=CARTESIAN_POINT('Ctrl Pts',(-0.00548492600005558,2.2,-4.38298810700001));
#327488=CARTESIAN_POINT('Ctrl Pts',(-0.00466004600005677,12.2,-4.38481576600001));
#327489=CARTESIAN_POINT('Ctrl Pts',(-0.00466004600005677,5.2,-4.38481576600001));
#327490=CARTESIAN_POINT('Ctrl Pts',(-0.00466004600005677,2.2,-4.38481576600001));
#327491=CARTESIAN_POINT('Ctrl Pts',(-0.00383146400005586,12.2,-4.38664621400001));
#327492=CARTESIAN_POINT('Ctrl Pts',(-0.00383146400005586,5.2,-4.38664621400001));
#327493=CARTESIAN_POINT('Ctrl Pts',(-0.00383146400005586,2.2,-4.38664621400001));
#327494=CARTESIAN_POINT('Ctrl Pts',(-0.00299917500005576,12.2,-4.38847943800001));
#327495=CARTESIAN_POINT('Ctrl Pts',(-0.00299917500005576,5.2,-4.38847943800001));
#327496=CARTESIAN_POINT('Ctrl Pts',(-0.00299917500005576,2.2,-4.38847943800001));
#327497=CARTESIAN_POINT('Ctrl Pts',(-0.00216317600005623,12.2,-4.39031543100001));
#327498=CARTESIAN_POINT('Ctrl Pts',(-0.00216317600005623,5.2,-4.39031543100001));
#327499=CARTESIAN_POINT('Ctrl Pts',(-0.00216317600005623,2.2,-4.39031543100001));
#327500=CARTESIAN_POINT('Ctrl Pts',(-0.00132346000005668,12.2,-4.39215418000002));
#327501=CARTESIAN_POINT('Ctrl Pts',(-0.00132346000005668,5.2,-4.39215418000002));
#327502=CARTESIAN_POINT('Ctrl Pts',(-0.00132346000005668,2.2,-4.39215418000002));
#327503=CARTESIAN_POINT('Ctrl Pts',(-0.000480025000056958,12.2,-4.39399567700002));
#327504=CARTESIAN_POINT('Ctrl Pts',(-0.000480025000056958,5.2,-4.39399567700002));
#327505=CARTESIAN_POINT('Ctrl Pts',(-0.000480025000056958,2.2,-4.39399567700002));
#327506=CARTESIAN_POINT('Ctrl Pts',(0.000367133999944471,12.2,-4.39583991200001));
#327507=CARTESIAN_POINT('Ctrl Pts',(0.000367133999944471,5.2,-4.39583991200001));
#327508=CARTESIAN_POINT('Ctrl Pts',(0.000367133999944471,2.2,-4.39583991200001));
#327509=CARTESIAN_POINT('Ctrl Pts',(0.00121801999994452,12.2,-4.39768687500001));
#327510=CARTESIAN_POINT('Ctrl Pts',(0.00121801999994452,5.2,-4.39768687500001));
#327511=CARTESIAN_POINT('Ctrl Pts',(0.00121801999994452,2.2,-4.39768687500001));
#327512=CARTESIAN_POINT('Ctrl Pts',(0.00207263999994488,12.2,-4.39953655500001));
#327513=CARTESIAN_POINT('Ctrl Pts',(0.00207263999994488,5.2,-4.39953655500001));
#327514=CARTESIAN_POINT('Ctrl Pts',(0.00207263999994488,2.2,-4.39953655500001));
#327515=CARTESIAN_POINT('Ctrl Pts',(0.00293099499994453,12.2,-4.40138894500001));
#327516=CARTESIAN_POINT('Ctrl Pts',(0.00293099499994453,5.2,-4.40138894500001));
#327517=CARTESIAN_POINT('Ctrl Pts',(0.00293099499994453,2.2,-4.40138894500001));
#327518=CARTESIAN_POINT('Ctrl Pts',(0.00379309099994395,12.2,-4.40324403300002));
#327519=CARTESIAN_POINT('Ctrl Pts',(0.00379309099994395,5.2,-4.40324403300002));
#327520=CARTESIAN_POINT('Ctrl Pts',(0.00379309099994395,2.2,-4.40324403300002));
#327521=CARTESIAN_POINT('Ctrl Pts',(0.00465893399994365,12.2,-4.40510180900001));
#327522=CARTESIAN_POINT('Ctrl Pts',(0.00465893399994365,5.2,-4.40510180900001));
#327523=CARTESIAN_POINT('Ctrl Pts',(0.00465893399994365,2.2,-4.40510180900001));
#327524=CARTESIAN_POINT('Ctrl Pts',(0.00552852499994371,12.2,-4.40696226300001));
#327525=CARTESIAN_POINT('Ctrl Pts',(0.00552852499994371,5.2,-4.40696226300001));
#327526=CARTESIAN_POINT('Ctrl Pts',(0.00552852499994371,2.2,-4.40696226300001));
#327527=CARTESIAN_POINT('Ctrl Pts',(0.00640186899994454,12.2,-4.40882538700002));
#327528=CARTESIAN_POINT('Ctrl Pts',(0.00640186899994454,5.2,-4.40882538700002));
#327529=CARTESIAN_POINT('Ctrl Pts',(0.00640186899994454,2.2,-4.40882538700002));
#327530=CARTESIAN_POINT('Ctrl Pts',(0.00727896999994536,12.2,-4.41069117000001));
#327531=CARTESIAN_POINT('Ctrl Pts',(0.00727896999994536,5.2,-4.41069117000001));
#327532=CARTESIAN_POINT('Ctrl Pts',(0.00727896999994536,2.2,-4.41069117000001));
#327533=CARTESIAN_POINT('Ctrl Pts',(0.00815983399994446,12.2,-4.41255960200001));
#327534=CARTESIAN_POINT('Ctrl Pts',(0.00815983399994446,5.2,-4.41255960200001));
#327535=CARTESIAN_POINT('Ctrl Pts',(0.00815983399994446,2.2,-4.41255960200001));
#327536=CARTESIAN_POINT('Ctrl Pts',(0.00904446199994412,12.2,-4.41443067300002));
#327537=CARTESIAN_POINT('Ctrl Pts',(0.00904446199994412,5.2,-4.41443067300002));
#327538=CARTESIAN_POINT('Ctrl Pts',(0.00904446199994412,2.2,-4.41443067300002));
#327539=CARTESIAN_POINT('Ctrl Pts',(0.00993286099994494,12.2,-4.41630437500002));
#327540=CARTESIAN_POINT('Ctrl Pts',(0.00993286099994494,5.2,-4.41630437500002));
#327541=CARTESIAN_POINT('Ctrl Pts',(0.00993286099994494,2.2,-4.41630437500002));
#327542=CARTESIAN_POINT('Ctrl Pts',(0.0108250329999449,12.2,-4.41818069600002));
#327543=CARTESIAN_POINT('Ctrl Pts',(0.0108250329999449,5.2,-4.41818069600002));
#327544=CARTESIAN_POINT('Ctrl Pts',(0.0108250329999449,2.2,-4.41818069600002));
#327545=CARTESIAN_POINT('Ctrl Pts',(0.0117209829999432,12.2,-4.42005962600001));
#327546=CARTESIAN_POINT('Ctrl Pts',(0.0117209829999432,5.2,-4.42005962600001));
#327547=CARTESIAN_POINT('Ctrl Pts',(0.0117209829999432,2.2,-4.42005962600001));
#327548=CARTESIAN_POINT('Ctrl Pts',(0.0126207139999435,12.2,-4.42194115800001));
#327549=CARTESIAN_POINT('Ctrl Pts',(0.0126207139999435,5.2,-4.42194115800001));
#327550=CARTESIAN_POINT('Ctrl Pts',(0.0126207139999435,2.2,-4.42194115800001));
#327551=CARTESIAN_POINT('Ctrl Pts',(0.013524230999945,12.2,-4.42382528100001));
#327552=CARTESIAN_POINT('Ctrl Pts',(0.013524230999945,5.2,-4.42382528100001));
#327553=CARTESIAN_POINT('Ctrl Pts',(0.013524230999945,2.2,-4.42382528100001));
#327554=CARTESIAN_POINT('Ctrl Pts',(0.0144315379999438,12.2,-4.42571198400001));
#327555=CARTESIAN_POINT('Ctrl Pts',(0.0144315379999438,5.2,-4.42571198400001));
#327556=CARTESIAN_POINT('Ctrl Pts',(0.0144315379999438,2.2,-4.42571198400001));
#327557=CARTESIAN_POINT('Ctrl Pts',(0.0153426389999434,12.2,-4.42760125800001));
#327558=CARTESIAN_POINT('Ctrl Pts',(0.0153426389999434,5.2,-4.42760125800001));
#327559=CARTESIAN_POINT('Ctrl Pts',(0.0153426389999434,2.2,-4.42760125800001));
#327560=CARTESIAN_POINT('Ctrl Pts',(0.0162575369999451,12.2,-4.42949309400001));
#327561=CARTESIAN_POINT('Ctrl Pts',(0.0162575369999451,5.2,-4.42949309400001));
#327562=CARTESIAN_POINT('Ctrl Pts',(0.0162575369999451,2.2,-4.42949309400001));
#327563=CARTESIAN_POINT('Ctrl Pts',(0.017176236999944,12.2,-4.43138748200001));
#327564=CARTESIAN_POINT('Ctrl Pts',(0.017176236999944,5.2,-4.43138748200001));
#327565=CARTESIAN_POINT('Ctrl Pts',(0.017176236999944,2.2,-4.43138748200001));
#327566=CARTESIAN_POINT('Ctrl Pts',(0.0180987419999445,12.2,-4.43328441100002));
#327567=CARTESIAN_POINT('Ctrl Pts',(0.0180987419999445,5.2,-4.43328441100002));
#327568=CARTESIAN_POINT('Ctrl Pts',(0.0180987419999445,2.2,-4.43328441100002));
#327569=CARTESIAN_POINT('Ctrl Pts',(0.0190250569999439,12.2,-4.43518387300001));
#327570=CARTESIAN_POINT('Ctrl Pts',(0.0190250569999439,5.2,-4.43518387300001));
#327571=CARTESIAN_POINT('Ctrl Pts',(0.0190250569999439,2.2,-4.43518387300001));
#327572=CARTESIAN_POINT('Ctrl Pts',(0.0199551849999435,12.2,-4.43708585900001));
#327573=CARTESIAN_POINT('Ctrl Pts',(0.0199551849999435,5.2,-4.43708585900001));
#327574=CARTESIAN_POINT('Ctrl Pts',(0.0199551849999435,2.2,-4.43708585900001));
#327575=CARTESIAN_POINT('Ctrl Pts',(0.0208891289999435,12.2,-4.43899035600001));
#327576=CARTESIAN_POINT('Ctrl Pts',(0.0208891289999435,5.2,-4.43899035600001));
#327577=CARTESIAN_POINT('Ctrl Pts',(0.0208891289999435,2.2,-4.43899035600001));
#327578=CARTESIAN_POINT('Ctrl Pts',(0.0218268949999434,12.2,-4.44089735800001));
#327579=CARTESIAN_POINT('Ctrl Pts',(0.0218268949999434,5.2,-4.44089735800001));
#327580=CARTESIAN_POINT('Ctrl Pts',(0.0218268949999434,2.2,-4.44089735800001));
#327581=CARTESIAN_POINT('Ctrl Pts',(0.0227684839999431,12.2,-4.44280685300001));
#327582=CARTESIAN_POINT('Ctrl Pts',(0.0227684839999431,5.2,-4.44280685300001));
#327583=CARTESIAN_POINT('Ctrl Pts',(0.0227684839999431,2.2,-4.44280685300001));
#327584=CARTESIAN_POINT('Ctrl Pts',(0.0237139019999444,12.2,-4.44471883200002));
#327585=CARTESIAN_POINT('Ctrl Pts',(0.0237139019999444,5.2,-4.44471883200002));
#327586=CARTESIAN_POINT('Ctrl Pts',(0.0237139019999444,2.2,-4.44471883200002));
#327587=CARTESIAN_POINT('Ctrl Pts',(0.0246631529999441,12.2,-4.44663328500001));
#327588=CARTESIAN_POINT('Ctrl Pts',(0.0246631529999441,5.2,-4.44663328500001));
#327589=CARTESIAN_POINT('Ctrl Pts',(0.0246631529999441,2.2,-4.44663328500001));
#327590=CARTESIAN_POINT('Ctrl Pts',(0.0256162389999448,12.2,-4.44855020400002));
#327591=CARTESIAN_POINT('Ctrl Pts',(0.0256162389999448,5.2,-4.44855020400002));
#327592=CARTESIAN_POINT('Ctrl Pts',(0.0256162389999448,2.2,-4.44855020400002));
#327593=CARTESIAN_POINT('Ctrl Pts',(0.0265731639999434,12.2,-4.45046957800002));
#327594=CARTESIAN_POINT('Ctrl Pts',(0.0265731639999434,5.2,-4.45046957800002));
#327595=CARTESIAN_POINT('Ctrl Pts',(0.0265731639999434,2.2,-4.45046957800002));
#327596=CARTESIAN_POINT('Ctrl Pts',(0.0275339329999447,12.2,-4.45239139700002));
#327597=CARTESIAN_POINT('Ctrl Pts',(0.0275339329999447,5.2,-4.45239139700002));
#327598=CARTESIAN_POINT('Ctrl Pts',(0.0275339329999447,2.2,-4.45239139700002));
#327599=CARTESIAN_POINT('Ctrl Pts',(0.0284985489999434,12.2,-4.45431565300002));
#327600=CARTESIAN_POINT('Ctrl Pts',(0.0284985489999434,5.2,-4.45431565300002));
#327601=CARTESIAN_POINT('Ctrl Pts',(0.0284985489999434,2.2,-4.45431565300002));
#327602=CARTESIAN_POINT('Ctrl Pts',(0.0294670149999454,12.2,-4.45624233500002));
#327603=CARTESIAN_POINT('Ctrl Pts',(0.0294670149999454,5.2,-4.45624233500002));
#327604=CARTESIAN_POINT('Ctrl Pts',(0.0294670149999454,2.2,-4.45624233500002));
#327605=CARTESIAN_POINT('Ctrl Pts',(0.0304393349999443,12.2,-4.45817143400001));
#327606=CARTESIAN_POINT('Ctrl Pts',(0.0304393349999443,5.2,-4.45817143400001));
#327607=CARTESIAN_POINT('Ctrl Pts',(0.0304393349999443,2.2,-4.45817143400001));
#327608=CARTESIAN_POINT('Ctrl Pts',(0.0314155129999438,12.2,-4.46010294100001));
#327609=CARTESIAN_POINT('Ctrl Pts',(0.0314155129999438,5.2,-4.46010294100001));
#327610=CARTESIAN_POINT('Ctrl Pts',(0.0314155129999438,2.2,-4.46010294100001));
#327611=CARTESIAN_POINT('Ctrl Pts',(0.0323955529999442,12.2,-4.46203684400002));
#327612=CARTESIAN_POINT('Ctrl Pts',(0.0323955529999442,5.2,-4.46203684400002));
#327613=CARTESIAN_POINT('Ctrl Pts',(0.0323955529999442,2.2,-4.46203684400002));
#327614=CARTESIAN_POINT('Ctrl Pts',(0.0333794569999435,12.2,-4.46397313600002));
#327615=CARTESIAN_POINT('Ctrl Pts',(0.0333794569999435,5.2,-4.46397313600002));
#327616=CARTESIAN_POINT('Ctrl Pts',(0.0333794569999435,2.2,-4.46397313600002));
#327617=CARTESIAN_POINT('Ctrl Pts',(0.0343672309999443,12.2,-4.46591180700001));
#327618=CARTESIAN_POINT('Ctrl Pts',(0.0343672309999443,5.2,-4.46591180700001));
#327619=CARTESIAN_POINT('Ctrl Pts',(0.0343672309999443,2.2,-4.46591180700001));
#327620=CARTESIAN_POINT('Ctrl Pts',(0.0353588759999435,12.2,-4.46785284800002));
#327621=CARTESIAN_POINT('Ctrl Pts',(0.0353588759999435,5.2,-4.46785284800002));
#327622=CARTESIAN_POINT('Ctrl Pts',(0.0353588759999435,2.2,-4.46785284800002));
#327623=CARTESIAN_POINT('Ctrl Pts',(0.0363543979999437,12.2,-4.46979624600001));
#327624=CARTESIAN_POINT('Ctrl Pts',(0.0363543979999437,5.2,-4.46979624600001));
#327625=CARTESIAN_POINT('Ctrl Pts',(0.0363543979999437,2.2,-4.46979624600001));
#327626=CARTESIAN_POINT('Ctrl Pts',(0.037353797999945,12.2,-4.47174199600001));
#327627=CARTESIAN_POINT('Ctrl Pts',(0.037353797999945,5.2,-4.47174199600001));
#327628=CARTESIAN_POINT('Ctrl Pts',(0.037353797999945,2.2,-4.47174199600001));
#327629=CARTESIAN_POINT('Ctrl Pts',(0.0383570819999446,12.2,-4.47369008700001));
#327630=CARTESIAN_POINT('Ctrl Pts',(0.0383570819999446,5.2,-4.47369008700001));
#327631=CARTESIAN_POINT('Ctrl Pts',(0.0383570819999446,2.2,-4.47369008700001));
#327632=CARTESIAN_POINT('Ctrl Pts',(0.0393642509999437,12.2,-4.47564050800001));
#327633=CARTESIAN_POINT('Ctrl Pts',(0.0393642509999437,5.2,-4.47564050800001));
#327634=CARTESIAN_POINT('Ctrl Pts',(0.0393642509999437,2.2,-4.47564050800001));
#327635=CARTESIAN_POINT('Ctrl Pts',(0.0403753099999438,12.2,-4.47759325200002));
#327636=CARTESIAN_POINT('Ctrl Pts',(0.0403753099999438,5.2,-4.47759325200002));
#327637=CARTESIAN_POINT('Ctrl Pts',(0.0403753099999438,2.2,-4.47759325200002));
#327638=CARTESIAN_POINT('Ctrl Pts',(0.041390261999944,12.2,-4.47954830700001));
#327639=CARTESIAN_POINT('Ctrl Pts',(0.041390261999944,5.2,-4.47954830700001));
#327640=CARTESIAN_POINT('Ctrl Pts',(0.041390261999944,2.2,-4.47954830700001));
#327641=CARTESIAN_POINT('Ctrl Pts',(0.0424091099999446,12.2,-4.48150566500002));
#327642=CARTESIAN_POINT('Ctrl Pts',(0.0424091099999446,5.2,-4.48150566500002));
#327643=CARTESIAN_POINT('Ctrl Pts',(0.0424091099999446,2.2,-4.48150566500002));
#327644=CARTESIAN_POINT('Ctrl Pts',(0.0434318589999438,12.2,-4.48346531700002));
#327645=CARTESIAN_POINT('Ctrl Pts',(0.0434318589999438,5.2,-4.48346531700002));
#327646=CARTESIAN_POINT('Ctrl Pts',(0.0434318589999438,2.2,-4.48346531700002));
#327647=CARTESIAN_POINT('Ctrl Pts',(0.044458510999944,12.2,-4.48542725200001));
#327648=CARTESIAN_POINT('Ctrl Pts',(0.044458510999944,5.2,-4.48542725200001));
#327649=CARTESIAN_POINT('Ctrl Pts',(0.044458510999944,2.2,-4.48542725200001));
#327650=CARTESIAN_POINT('Ctrl Pts',(0.0454890689999432,12.2,-4.48739146100001));
#327651=CARTESIAN_POINT('Ctrl Pts',(0.0454890689999432,5.2,-4.48739146100001));
#327652=CARTESIAN_POINT('Ctrl Pts',(0.0454890689999432,2.2,-4.48739146100001));
#327653=CARTESIAN_POINT('Ctrl Pts',(0.046523537999944,12.2,-4.48935793600001));
#327654=CARTESIAN_POINT('Ctrl Pts',(0.046523537999944,5.2,-4.48935793600001));
#327655=CARTESIAN_POINT('Ctrl Pts',(0.046523537999944,2.2,-4.48935793600001));
#327656=CARTESIAN_POINT('Ctrl Pts',(0.0475619189999443,12.2,-4.49132666500001));
#327657=CARTESIAN_POINT('Ctrl Pts',(0.0475619189999443,5.2,-4.49132666500001));
#327658=CARTESIAN_POINT('Ctrl Pts',(0.0475619189999443,2.2,-4.49132666500001));
#327659=CARTESIAN_POINT('Ctrl Pts',(0.0486042179999446,12.2,-4.49329764200002));
#327660=CARTESIAN_POINT('Ctrl Pts',(0.0486042179999446,5.2,-4.49329764200002));
#327661=CARTESIAN_POINT('Ctrl Pts',(0.0486042179999446,2.2,-4.49329764200002));
#327662=CARTESIAN_POINT('Ctrl Pts',(0.049650436999944,12.2,-4.49527085400002));
#327663=CARTESIAN_POINT('Ctrl Pts',(0.049650436999944,5.2,-4.49527085400002));
#327664=CARTESIAN_POINT('Ctrl Pts',(0.049650436999944,2.2,-4.49527085400002));
#327665=CARTESIAN_POINT('Ctrl Pts',(0.0507005789999437,12.2,-4.49724629400002));
#327666=CARTESIAN_POINT('Ctrl Pts',(0.0507005789999437,5.2,-4.49724629400002));
#327667=CARTESIAN_POINT('Ctrl Pts',(0.0507005789999437,2.2,-4.49724629400002));
#327668=CARTESIAN_POINT('Ctrl Pts',(0.0517546479999442,12.2,-4.49922395100002));
#327669=CARTESIAN_POINT('Ctrl Pts',(0.0517546479999442,5.2,-4.49922395100002));
#327670=CARTESIAN_POINT('Ctrl Pts',(0.0517546479999442,2.2,-4.49922395100002));
#327671=CARTESIAN_POINT('Ctrl Pts',(0.0528126449999444,12.2,-4.50120381900001));
#327672=CARTESIAN_POINT('Ctrl Pts',(0.0528126449999444,5.2,-4.50120381900001));
#327673=CARTESIAN_POINT('Ctrl Pts',(0.0528126449999444,2.2,-4.50120381900001));
#327674=CARTESIAN_POINT('Ctrl Pts',(0.0538745769999438,12.2,-4.50318588400001));
#327675=CARTESIAN_POINT('Ctrl Pts',(0.0538745769999438,5.2,-4.50318588400001));
#327676=CARTESIAN_POINT('Ctrl Pts',(0.0538745769999438,2.2,-4.50318588400001));
#327677=CARTESIAN_POINT('Ctrl Pts',(0.0549404449999447,12.2,-4.50517014000001));
#327678=CARTESIAN_POINT('Ctrl Pts',(0.0549404449999447,5.2,-4.50517014000001));
#327679=CARTESIAN_POINT('Ctrl Pts',(0.0549404449999447,2.2,-4.50517014000001));
#327680=CARTESIAN_POINT('Ctrl Pts',(0.0560102509999438,12.2,-4.50715657500002));
#327681=CARTESIAN_POINT('Ctrl Pts',(0.0560102509999438,5.2,-4.50715657500002));
#327682=CARTESIAN_POINT('Ctrl Pts',(0.0560102509999438,2.2,-4.50715657500002));
#327683=CARTESIAN_POINT('Ctrl Pts',(0.0570840009999451,12.2,-4.50914518300001));
#327684=CARTESIAN_POINT('Ctrl Pts',(0.0570840009999451,5.2,-4.50914518300001));
#327685=CARTESIAN_POINT('Ctrl Pts',(0.0570840009999451,2.2,-4.50914518300001));
#327686=CARTESIAN_POINT('Ctrl Pts',(0.0581616969999443,12.2,-4.51113595100002));
#327687=CARTESIAN_POINT('Ctrl Pts',(0.0581616969999443,5.2,-4.51113595100002));
#327688=CARTESIAN_POINT('Ctrl Pts',(0.0581616969999443,2.2,-4.51113595100002));
#327689=CARTESIAN_POINT('Ctrl Pts',(0.0592433409999438,12.2,-4.51312887200002));
#327690=CARTESIAN_POINT('Ctrl Pts',(0.0592433409999438,5.2,-4.51312887200002));
#327691=CARTESIAN_POINT('Ctrl Pts',(0.0592433409999438,2.2,-4.51312887200002));
#327692=CARTESIAN_POINT('Ctrl Pts',(0.0603289369999449,12.2,-4.51512393600002));
#327693=CARTESIAN_POINT('Ctrl Pts',(0.0603289369999449,5.2,-4.51512393600002));
#327694=CARTESIAN_POINT('Ctrl Pts',(0.0603289369999449,2.2,-4.51512393600002));
#327695=CARTESIAN_POINT('Ctrl Pts',(0.0614184889999447,12.2,-4.51712113400002));
#327696=CARTESIAN_POINT('Ctrl Pts',(0.0614184889999447,5.2,-4.51712113400002));
#327697=CARTESIAN_POINT('Ctrl Pts',(0.0614184889999447,2.2,-4.51712113400002));
#327698=CARTESIAN_POINT('Ctrl Pts',(0.0625119979999444,12.2,-4.51912045700002));
#327699=CARTESIAN_POINT('Ctrl Pts',(0.0625119979999444,5.2,-4.51912045700002));
#327700=CARTESIAN_POINT('Ctrl Pts',(0.0625119979999444,2.2,-4.51912045700002));
#327701=CARTESIAN_POINT('Ctrl Pts',(0.0636094699999445,12.2,-4.52112189500002));
#327702=CARTESIAN_POINT('Ctrl Pts',(0.0636094699999445,5.2,-4.52112189500002));
#327703=CARTESIAN_POINT('Ctrl Pts',(0.0636094699999445,2.2,-4.52112189500002));
#327704=CARTESIAN_POINT('Ctrl Pts',(0.0647109049999439,12.2,-4.52312544000002));
#327705=CARTESIAN_POINT('Ctrl Pts',(0.0647109049999439,5.2,-4.52312544000002));
#327706=CARTESIAN_POINT('Ctrl Pts',(0.0647109049999439,2.2,-4.52312544000002));
#327707=CARTESIAN_POINT('Ctrl Pts',(0.0658163089999442,12.2,-4.52513108000002));
#327708=CARTESIAN_POINT('Ctrl Pts',(0.0658163089999442,5.2,-4.52513108000002));
#327709=CARTESIAN_POINT('Ctrl Pts',(0.0658163089999442,2.2,-4.52513108000002));
#327710=CARTESIAN_POINT('Ctrl Pts',(0.0669256809999441,12.2,-4.52713880800002));
#327711=CARTESIAN_POINT('Ctrl Pts',(0.0669256809999441,5.2,-4.52713880800002));
#327712=CARTESIAN_POINT('Ctrl Pts',(0.0669256809999441,2.2,-4.52713880800002));
#327713=CARTESIAN_POINT('Ctrl Pts',(0.0680390289999444,12.2,-4.52914861400001));
#327714=CARTESIAN_POINT('Ctrl Pts',(0.0680390289999444,5.2,-4.52914861400001));
#327715=CARTESIAN_POINT('Ctrl Pts',(0.0680390289999444,2.2,-4.52914861400001));
#327716=CARTESIAN_POINT('Ctrl Pts',(0.0691563519999438,12.2,-4.53116048900001));
#327717=CARTESIAN_POINT('Ctrl Pts',(0.0691563519999438,5.2,-4.53116048900001));
#327718=CARTESIAN_POINT('Ctrl Pts',(0.0691563519999438,2.2,-4.53116048900001));
#327719=CARTESIAN_POINT('Ctrl Pts',(0.070277653999945,12.2,-4.53317442400001));
#327720=CARTESIAN_POINT('Ctrl Pts',(0.070277653999945,5.2,-4.53317442400001));
#327721=CARTESIAN_POINT('Ctrl Pts',(0.070277653999945,2.2,-4.53317442400001));
#327722=CARTESIAN_POINT('Ctrl Pts',(0.0714029399999438,12.2,-4.53519041000002));
#327723=CARTESIAN_POINT('Ctrl Pts',(0.0714029399999438,5.2,-4.53519041000002));
#327724=CARTESIAN_POINT('Ctrl Pts',(0.0714029399999438,2.2,-4.53519041000002));
#327725=CARTESIAN_POINT('Ctrl Pts',(0.0725322099999437,12.2,-4.53720843600002));
#327726=CARTESIAN_POINT('Ctrl Pts',(0.0725322099999437,5.2,-4.53720843600002));
#327727=CARTESIAN_POINT('Ctrl Pts',(0.0725322099999437,2.2,-4.53720843600002));
#327728=CARTESIAN_POINT('Ctrl Pts',(0.073665468999945,12.2,-4.53922849500001));
#327729=CARTESIAN_POINT('Ctrl Pts',(0.073665468999945,5.2,-4.53922849500001));
#327730=CARTESIAN_POINT('Ctrl Pts',(0.073665468999945,2.2,-4.53922849500001));
#327731=CARTESIAN_POINT('Ctrl Pts',(0.0748027189999445,12.2,-4.54125057700002));
#327732=CARTESIAN_POINT('Ctrl Pts',(0.0748027189999445,5.2,-4.54125057700002));
#327733=CARTESIAN_POINT('Ctrl Pts',(0.0748027189999445,2.2,-4.54125057700002));
#327734=CARTESIAN_POINT('Ctrl Pts',(0.0759439619999436,12.2,-4.54327467100001));
#327735=CARTESIAN_POINT('Ctrl Pts',(0.0759439619999436,5.2,-4.54327467100001));
#327736=CARTESIAN_POINT('Ctrl Pts',(0.0759439619999436,2.2,-4.54327467100001));
#327737=CARTESIAN_POINT('Ctrl Pts',(0.0770892039999438,12.2,-4.54530077100001));
#327738=CARTESIAN_POINT('Ctrl Pts',(0.0770892039999438,5.2,-4.54530077100001));
#327739=CARTESIAN_POINT('Ctrl Pts',(0.0770892039999438,2.2,-4.54530077100001));
#327740=CARTESIAN_POINT('Ctrl Pts',(0.078238444999944,12.2,-4.54732886600001));
#327741=CARTESIAN_POINT('Ctrl Pts',(0.078238444999944,5.2,-4.54732886600001));
#327742=CARTESIAN_POINT('Ctrl Pts',(0.078238444999944,2.2,-4.54732886600001));
#327743=CARTESIAN_POINT('Ctrl Pts',(0.0793916879999446,12.2,-4.54935894600002));
#327744=CARTESIAN_POINT('Ctrl Pts',(0.0793916879999446,5.2,-4.54935894600002));
#327745=CARTESIAN_POINT('Ctrl Pts',(0.0793916879999446,2.2,-4.54935894600002));
#327746=CARTESIAN_POINT('Ctrl Pts',(0.0805489369999446,12.2,-4.55139100400002));
#327747=CARTESIAN_POINT('Ctrl Pts',(0.0805489369999446,5.2,-4.55139100400002));
#327748=CARTESIAN_POINT('Ctrl Pts',(0.0805489369999446,2.2,-4.55139100400002));
#327749=CARTESIAN_POINT('Ctrl Pts',(0.0817101939999443,12.2,-4.55342503000002));
#327750=CARTESIAN_POINT('Ctrl Pts',(0.0817101939999443,5.2,-4.55342503000002));
#327751=CARTESIAN_POINT('Ctrl Pts',(0.0817101939999443,2.2,-4.55342503000002));
#327752=CARTESIAN_POINT('Ctrl Pts',(0.0828754619999439,12.2,-4.55546101400001));
#327753=CARTESIAN_POINT('Ctrl Pts',(0.0828754619999439,5.2,-4.55546101400001));
#327754=CARTESIAN_POINT('Ctrl Pts',(0.0828754619999439,2.2,-4.55546101400001));
#327755=CARTESIAN_POINT('Ctrl Pts',(0.0840447429999447,12.2,-4.55749894800002));
#327756=CARTESIAN_POINT('Ctrl Pts',(0.0840447429999447,5.2,-4.55749894800002));
#327757=CARTESIAN_POINT('Ctrl Pts',(0.0840447429999447,2.2,-4.55749894800002));
#327758=CARTESIAN_POINT('Ctrl Pts',(0.0852180419999449,12.2,-4.55953882200001));
#327759=CARTESIAN_POINT('Ctrl Pts',(0.0852180419999449,5.2,-4.55953882200001));
#327760=CARTESIAN_POINT('Ctrl Pts',(0.0852180419999449,2.2,-4.55953882200001));
#327761=CARTESIAN_POINT('Ctrl Pts',(0.0863953609999446,12.2,-4.56158062800001));
#327762=CARTESIAN_POINT('Ctrl Pts',(0.0863953609999446,5.2,-4.56158062800001));
#327763=CARTESIAN_POINT('Ctrl Pts',(0.0863953609999446,2.2,-4.56158062800001));
#327764=CARTESIAN_POINT('Ctrl Pts',(0.087576699999945,12.2,-4.56362435600001));
#327765=CARTESIAN_POINT('Ctrl Pts',(0.087576699999945,5.2,-4.56362435600001));
#327766=CARTESIAN_POINT('Ctrl Pts',(0.087576699999945,2.2,-4.56362435600001));
#327767=CARTESIAN_POINT('Ctrl Pts',(0.0887620659999444,12.2,-4.56566999600001));
#327768=CARTESIAN_POINT('Ctrl Pts',(0.0887620659999444,5.2,-4.56566999600001));
#327769=CARTESIAN_POINT('Ctrl Pts',(0.0887620659999444,2.2,-4.56566999600001));
#327770=CARTESIAN_POINT('Ctrl Pts',(0.089951457999945,12.2,-4.56771754100001));
#327771=CARTESIAN_POINT('Ctrl Pts',(0.089951457999945,5.2,-4.56771754100001));
#327772=CARTESIAN_POINT('Ctrl Pts',(0.089951457999945,2.2,-4.56771754100001));
#327773=CARTESIAN_POINT('Ctrl Pts',(0.0911448799999448,12.2,-4.56976698000001));
#327774=CARTESIAN_POINT('Ctrl Pts',(0.0911448799999448,5.2,-4.56976698000001));
#327775=CARTESIAN_POINT('Ctrl Pts',(0.0911448799999448,2.2,-4.56976698000001));
#327776=CARTESIAN_POINT('Ctrl Pts',(0.0923423349999453,12.2,-4.57181830600002));
#327777=CARTESIAN_POINT('Ctrl Pts',(0.0923423349999453,5.2,-4.57181830600002));
#327778=CARTESIAN_POINT('Ctrl Pts',(0.0923423349999453,2.2,-4.57181830600002));
#327779=CARTESIAN_POINT('Ctrl Pts',(0.0935438259999444,12.2,-4.57387150700002));
#327780=CARTESIAN_POINT('Ctrl Pts',(0.0935438259999444,5.2,-4.57387150700002));
#327781=CARTESIAN_POINT('Ctrl Pts',(0.0935438259999444,2.2,-4.57387150700002));
#327782=CARTESIAN_POINT('Ctrl Pts',(0.0947493549999445,12.2,-4.57592657700001));
#327783=CARTESIAN_POINT('Ctrl Pts',(0.0947493549999445,5.2,-4.57592657700001));
#327784=CARTESIAN_POINT('Ctrl Pts',(0.0947493549999445,2.2,-4.57592657700001));
#327785=CARTESIAN_POINT('Ctrl Pts',(0.0959589249999449,12.2,-4.57798350600001));
#327786=CARTESIAN_POINT('Ctrl Pts',(0.0959589249999449,5.2,-4.57798350600001));
#327787=CARTESIAN_POINT('Ctrl Pts',(0.0959589249999449,2.2,-4.57798350600001));
#327788=CARTESIAN_POINT('Ctrl Pts',(0.0971725369999443,12.2,-4.58004228400001));
#327789=CARTESIAN_POINT('Ctrl Pts',(0.0971725369999443,5.2,-4.58004228400001));
#327790=CARTESIAN_POINT('Ctrl Pts',(0.0971725369999443,2.2,-4.58004228400001));
#327791=CARTESIAN_POINT('Ctrl Pts',(0.0983901959999434,12.2,-4.58210290300002));
#327792=CARTESIAN_POINT('Ctrl Pts',(0.0983901959999434,5.2,-4.58210290300002));
#327793=CARTESIAN_POINT('Ctrl Pts',(0.0983901959999434,2.2,-4.58210290300002));
#327794=CARTESIAN_POINT('Ctrl Pts',(0.0996119039999444,12.2,-4.58416535200001));
#327795=CARTESIAN_POINT('Ctrl Pts',(0.0996119039999444,5.2,-4.58416535200001));
#327796=CARTESIAN_POINT('Ctrl Pts',(0.0996119039999444,2.2,-4.58416535200001));
#327797=CARTESIAN_POINT('Ctrl Pts',(0.100837662999943,12.2,-4.58622962500002));
#327798=CARTESIAN_POINT('Ctrl Pts',(0.100837662999943,5.2,-4.58622962500002));
#327799=CARTESIAN_POINT('Ctrl Pts',(0.100837662999943,2.2,-4.58622962500002));
#327800=CARTESIAN_POINT('Ctrl Pts',(0.102067473999944,12.2,-4.58829571100001));
#327801=CARTESIAN_POINT('Ctrl Pts',(0.102067473999944,5.2,-4.58829571100001));
#327802=CARTESIAN_POINT('Ctrl Pts',(0.102067473999944,2.2,-4.58829571100001));
#327803=CARTESIAN_POINT('Ctrl Pts',(0.103301341999943,12.2,-4.59036360200002));
#327804=CARTESIAN_POINT('Ctrl Pts',(0.103301341999943,5.2,-4.59036360200002));
#327805=CARTESIAN_POINT('Ctrl Pts',(0.103301341999943,2.2,-4.59036360200002));
#327806=CARTESIAN_POINT('Ctrl Pts',(0.104539268999944,12.2,-4.59243328800001));
#327807=CARTESIAN_POINT('Ctrl Pts',(0.104539268999944,5.2,-4.59243328800001));
#327808=CARTESIAN_POINT('Ctrl Pts',(0.104539268999944,2.2,-4.59243328800001));
#327809=CARTESIAN_POINT('Ctrl Pts',(0.105781256999944,12.2,-4.59450476100002));
#327810=CARTESIAN_POINT('Ctrl Pts',(0.105781256999944,5.2,-4.59450476100002));
#327811=CARTESIAN_POINT('Ctrl Pts',(0.105781256999944,2.2,-4.59450476100002));
#327812=CARTESIAN_POINT('Ctrl Pts',(0.107027308999944,12.2,-4.59657801100001));
#327813=CARTESIAN_POINT('Ctrl Pts',(0.107027308999944,5.2,-4.59657801100001));
#327814=CARTESIAN_POINT('Ctrl Pts',(0.107027308999944,2.2,-4.59657801100001));
#327815=CARTESIAN_POINT('Ctrl Pts',(0.108277424999944,12.2,-4.59865303000001));
#327816=CARTESIAN_POINT('Ctrl Pts',(0.108277424999944,5.2,-4.59865303000001));
#327817=CARTESIAN_POINT('Ctrl Pts',(0.108277424999944,2.2,-4.59865303000001));
#327818=CARTESIAN_POINT('Ctrl Pts',(0.109531610999944,12.2,-4.60072980900001));
#327819=CARTESIAN_POINT('Ctrl Pts',(0.109531610999944,5.2,-4.60072980900001));
#327820=CARTESIAN_POINT('Ctrl Pts',(0.109531610999944,2.2,-4.60072980900001));
#327821=CARTESIAN_POINT('Ctrl Pts',(0.110789867999944,12.2,-4.60280833800002));
#327822=CARTESIAN_POINT('Ctrl Pts',(0.110789867999944,5.2,-4.60280833800002));
#327823=CARTESIAN_POINT('Ctrl Pts',(0.110789867999944,2.2,-4.60280833800002));
#327824=CARTESIAN_POINT('Ctrl Pts',(0.112052197999944,12.2,-4.60488860800002));
#327825=CARTESIAN_POINT('Ctrl Pts',(0.112052197999944,5.2,-4.60488860800002));
#327826=CARTESIAN_POINT('Ctrl Pts',(0.112052197999944,2.2,-4.60488860800002));
#327827=CARTESIAN_POINT('Ctrl Pts',(0.113318603999945,12.2,-4.60697061200001));
#327828=CARTESIAN_POINT('Ctrl Pts',(0.113318603999945,5.2,-4.60697061200001));
#327829=CARTESIAN_POINT('Ctrl Pts',(0.113318603999945,2.2,-4.60697061200001));
#327830=CARTESIAN_POINT('Ctrl Pts',(0.114589087999944,12.2,-4.60905434000002));
#327831=CARTESIAN_POINT('Ctrl Pts',(0.114589087999944,5.2,-4.60905434000002));
#327832=CARTESIAN_POINT('Ctrl Pts',(0.114589087999944,2.2,-4.60905434000002));
#327833=CARTESIAN_POINT('Ctrl Pts',(0.115863651999945,12.2,-4.61113978200002));
#327834=CARTESIAN_POINT('Ctrl Pts',(0.115863651999945,5.2,-4.61113978200002));
#327835=CARTESIAN_POINT('Ctrl Pts',(0.115863651999945,2.2,-4.61113978200002));
#327836=CARTESIAN_POINT('Ctrl Pts',(0.117142298999945,12.2,-4.61322693100001));
#327837=CARTESIAN_POINT('Ctrl Pts',(0.117142298999945,5.2,-4.61322693100001));
#327838=CARTESIAN_POINT('Ctrl Pts',(0.117142298999945,2.2,-4.61322693100001));
#327839=CARTESIAN_POINT('Ctrl Pts',(0.118425031999945,12.2,-4.61531577700002));
#327840=CARTESIAN_POINT('Ctrl Pts',(0.118425031999945,5.2,-4.61531577700002));
#327841=CARTESIAN_POINT('Ctrl Pts',(0.118425031999945,2.2,-4.61531577700002));
#327842=CARTESIAN_POINT('Ctrl Pts',(0.119711850999943,12.2,-4.61740631000001));
#327843=CARTESIAN_POINT('Ctrl Pts',(0.119711850999943,5.2,-4.61740631000001));
#327844=CARTESIAN_POINT('Ctrl Pts',(0.119711850999943,2.2,-4.61740631000001));
#327845=CARTESIAN_POINT('Ctrl Pts',(0.121002760999945,12.2,-4.61949852400001));
#327846=CARTESIAN_POINT('Ctrl Pts',(0.121002760999945,5.2,-4.61949852400001));
#327847=CARTESIAN_POINT('Ctrl Pts',(0.121002760999945,2.2,-4.61949852400001));
#327848=CARTESIAN_POINT('Ctrl Pts',(0.122297761999944,12.2,-4.62159240800001));
#327849=CARTESIAN_POINT('Ctrl Pts',(0.122297761999944,5.2,-4.62159240800001));
#327850=CARTESIAN_POINT('Ctrl Pts',(0.122297761999944,2.2,-4.62159240800001));
#327851=CARTESIAN_POINT('Ctrl Pts',(0.123596857999945,12.2,-4.62368795400002));
#327852=CARTESIAN_POINT('Ctrl Pts',(0.123596857999945,5.2,-4.62368795400002));
#327853=CARTESIAN_POINT('Ctrl Pts',(0.123596857999945,2.2,-4.62368795400002));
#327854=CARTESIAN_POINT('Ctrl Pts',(0.124900049999944,12.2,-4.62578515200001));
#327855=CARTESIAN_POINT('Ctrl Pts',(0.124900049999944,5.2,-4.62578515200001));
#327856=CARTESIAN_POINT('Ctrl Pts',(0.124900049999944,2.2,-4.62578515200001));
#327857=CARTESIAN_POINT('Ctrl Pts',(0.126207341999944,12.2,-4.62788399400001));
#327858=CARTESIAN_POINT('Ctrl Pts',(0.126207341999944,5.2,-4.62788399400001));
#327859=CARTESIAN_POINT('Ctrl Pts',(0.126207341999944,2.2,-4.62788399400001));
#327860=CARTESIAN_POINT('Ctrl Pts',(0.127518733999944,12.2,-4.62998447200002));
#327861=CARTESIAN_POINT('Ctrl Pts',(0.127518733999944,5.2,-4.62998447200002));
#327862=CARTESIAN_POINT('Ctrl Pts',(0.127518733999944,2.2,-4.62998447200002));
#327863=CARTESIAN_POINT('Ctrl Pts',(0.128834229999945,12.2,-4.63208657500001));
#327864=CARTESIAN_POINT('Ctrl Pts',(0.128834229999945,5.2,-4.63208657500001));
#327865=CARTESIAN_POINT('Ctrl Pts',(0.128834229999945,2.2,-4.63208657500001));
#327866=CARTESIAN_POINT('Ctrl Pts',(0.130153831999945,12.2,-4.63419029600002));
#327867=CARTESIAN_POINT('Ctrl Pts',(0.130153831999945,5.2,-4.63419029600002));
#327868=CARTESIAN_POINT('Ctrl Pts',(0.130153831999945,2.2,-4.63419029600002));
#327869=CARTESIAN_POINT('Ctrl Pts',(0.131477540999944,12.2,-4.63629562500001));
#327870=CARTESIAN_POINT('Ctrl Pts',(0.131477540999944,5.2,-4.63629562500001));
#327871=CARTESIAN_POINT('Ctrl Pts',(0.131477540999944,2.2,-4.63629562500001));
#327872=CARTESIAN_POINT('Ctrl Pts',(0.132805359999945,12.2,-4.63840255500001));
#327873=CARTESIAN_POINT('Ctrl Pts',(0.132805359999945,5.2,-4.63840255500001));
#327874=CARTESIAN_POINT('Ctrl Pts',(0.132805359999945,2.2,-4.63840255500001));
#327875=CARTESIAN_POINT('Ctrl Pts',(0.134137289999944,12.2,-4.64051107500001));
#327876=CARTESIAN_POINT('Ctrl Pts',(0.134137289999944,5.2,-4.64051107500001));
#327877=CARTESIAN_POINT('Ctrl Pts',(0.134137289999944,2.2,-4.64051107500001));
#327878=CARTESIAN_POINT('Ctrl Pts',(0.135473335999944,12.2,-4.64262117800001));
#327879=CARTESIAN_POINT('Ctrl Pts',(0.135473335999944,5.2,-4.64262117800001));
#327880=CARTESIAN_POINT('Ctrl Pts',(0.135473335999944,2.2,-4.64262117800001));
#327881=CARTESIAN_POINT('Ctrl Pts',(0.136813497999944,12.2,-4.64473285400001));
#327882=CARTESIAN_POINT('Ctrl Pts',(0.136813497999944,5.2,-4.64473285400001));
#327883=CARTESIAN_POINT('Ctrl Pts',(0.136813497999944,2.2,-4.64473285400001));
#327884=CARTESIAN_POINT('Ctrl Pts',(0.138157777999943,12.2,-4.64684609400001));
#327885=CARTESIAN_POINT('Ctrl Pts',(0.138157777999943,5.2,-4.64684609400001));
#327886=CARTESIAN_POINT('Ctrl Pts',(0.138157777999943,2.2,-4.64684609400001));
#327887=CARTESIAN_POINT('Ctrl Pts',(0.139506177999945,12.2,-4.64896089100002));
#327888=CARTESIAN_POINT('Ctrl Pts',(0.139506177999945,5.2,-4.64896089100002));
#327889=CARTESIAN_POINT('Ctrl Pts',(0.139506177999945,2.2,-4.64896089100002));
#327890=CARTESIAN_POINT('Ctrl Pts',(0.140858699999944,12.2,-4.65107723400001));
#327891=CARTESIAN_POINT('Ctrl Pts',(0.140858699999944,5.2,-4.65107723400001));
#327892=CARTESIAN_POINT('Ctrl Pts',(0.140858699999944,2.2,-4.65107723400001));
#327893=CARTESIAN_POINT('Ctrl Pts',(0.142215347999944,12.2,-4.65319511600002));
#327894=CARTESIAN_POINT('Ctrl Pts',(0.142215347999944,5.2,-4.65319511600002));
#327895=CARTESIAN_POINT('Ctrl Pts',(0.142215347999944,2.2,-4.65319511600002));
#327896=CARTESIAN_POINT('Ctrl Pts',(0.143576121999944,12.2,-4.65531452700001));
#327897=CARTESIAN_POINT('Ctrl Pts',(0.143576121999944,5.2,-4.65531452700001));
#327898=CARTESIAN_POINT('Ctrl Pts',(0.143576121999944,2.2,-4.65531452700001));
#327899=CARTESIAN_POINT('Ctrl Pts',(0.144941025999945,12.2,-4.65743546000001));
#327900=CARTESIAN_POINT('Ctrl Pts',(0.144941025999945,5.2,-4.65743546000001));
#327901=CARTESIAN_POINT('Ctrl Pts',(0.144941025999945,2.2,-4.65743546000001));
#327902=CARTESIAN_POINT('Ctrl Pts',(0.146310058999944,12.2,-4.65955790400002));
#327903=CARTESIAN_POINT('Ctrl Pts',(0.146310058999944,5.2,-4.65955790400002));
#327904=CARTESIAN_POINT('Ctrl Pts',(0.146310058999944,2.2,-4.65955790400002));
#327905=CARTESIAN_POINT('Ctrl Pts',(0.147683225999945,12.2,-4.66168185200001));
#327906=CARTESIAN_POINT('Ctrl Pts',(0.147683225999945,5.2,-4.66168185200001));
#327907=CARTESIAN_POINT('Ctrl Pts',(0.147683225999945,2.2,-4.66168185200001));
#327908=CARTESIAN_POINT('Ctrl Pts',(0.149060527999945,12.2,-4.66380729400001));
#327909=CARTESIAN_POINT('Ctrl Pts',(0.149060527999945,5.2,-4.66380729400001));
#327910=CARTESIAN_POINT('Ctrl Pts',(0.149060527999945,2.2,-4.66380729400001));
#327911=CARTESIAN_POINT('Ctrl Pts',(0.150441966999945,12.2,-4.66593422200001));
#327912=CARTESIAN_POINT('Ctrl Pts',(0.150441966999945,5.2,-4.66593422200001));
#327913=CARTESIAN_POINT('Ctrl Pts',(0.150441966999945,2.2,-4.66593422200001));
#327914=CARTESIAN_POINT('Ctrl Pts',(0.151827543999945,12.2,-4.66806262700001));
#327915=CARTESIAN_POINT('Ctrl Pts',(0.151827543999945,5.2,-4.66806262700001));
#327916=CARTESIAN_POINT('Ctrl Pts',(0.151827543999945,2.2,-4.66806262700001));
#327917=CARTESIAN_POINT('Ctrl Pts',(0.153217260999944,12.2,-4.67019250200002));
#327918=CARTESIAN_POINT('Ctrl Pts',(0.153217260999944,5.2,-4.67019250200002));
#327919=CARTESIAN_POINT('Ctrl Pts',(0.153217260999944,2.2,-4.67019250200002));
#327920=CARTESIAN_POINT('Ctrl Pts',(0.154611121999944,12.2,-4.67232383600001));
#327921=CARTESIAN_POINT('Ctrl Pts',(0.154611121999944,5.2,-4.67232383600001));
#327922=CARTESIAN_POINT('Ctrl Pts',(0.154611121999944,2.2,-4.67232383600001));
#327923=CARTESIAN_POINT('Ctrl Pts',(0.156009126999944,12.2,-4.67445662200001));
#327924=CARTESIAN_POINT('Ctrl Pts',(0.156009126999944,5.2,-4.67445662200001));
#327925=CARTESIAN_POINT('Ctrl Pts',(0.156009126999944,2.2,-4.67445662200001));
#327926=CARTESIAN_POINT('Ctrl Pts',(0.157411277999945,12.2,-4.67659084900002));
#327927=CARTESIAN_POINT('Ctrl Pts',(0.157411277999945,5.2,-4.67659084900002));
#327928=CARTESIAN_POINT('Ctrl Pts',(0.157411277999945,2.2,-4.67659084900002));
#327929=CARTESIAN_POINT('Ctrl Pts',(0.158817578999945,12.2,-4.67872651000001));
#327930=CARTESIAN_POINT('Ctrl Pts',(0.158817578999945,5.2,-4.67872651000001));
#327931=CARTESIAN_POINT('Ctrl Pts',(0.158817578999945,2.2,-4.67872651000001));
#327932=CARTESIAN_POINT('Ctrl Pts',(0.160228028999944,12.2,-4.68086359800001));
#327933=CARTESIAN_POINT('Ctrl Pts',(0.160228028999944,5.2,-4.68086359800001));
#327934=CARTESIAN_POINT('Ctrl Pts',(0.160228028999944,2.2,-4.68086359800001));
#327935=CARTESIAN_POINT('Ctrl Pts',(0.161642630999944,12.2,-4.68300210100002));
#327936=CARTESIAN_POINT('Ctrl Pts',(0.161642630999944,5.2,-4.68300210100002));
#327937=CARTESIAN_POINT('Ctrl Pts',(0.161642630999944,2.2,-4.68300210100002));
#327938=CARTESIAN_POINT('Ctrl Pts',(0.163061386999944,12.2,-4.68514201200001));
#327939=CARTESIAN_POINT('Ctrl Pts',(0.163061386999944,5.2,-4.68514201200001));
#327940=CARTESIAN_POINT('Ctrl Pts',(0.163061386999944,2.2,-4.68514201200001));
#327941=CARTESIAN_POINT('Ctrl Pts',(0.164484299999945,12.2,-4.68728332300001));
#327942=CARTESIAN_POINT('Ctrl Pts',(0.164484299999945,5.2,-4.68728332300001));
#327943=CARTESIAN_POINT('Ctrl Pts',(0.164484299999945,2.2,-4.68728332300001));
#327944=CARTESIAN_POINT('Ctrl Pts',(0.165911369999945,12.2,-4.68942602400002));
#327945=CARTESIAN_POINT('Ctrl Pts',(0.165911369999945,5.2,-4.68942602400002));
#327946=CARTESIAN_POINT('Ctrl Pts',(0.165911369999945,2.2,-4.68942602400002));
#327947=CARTESIAN_POINT('Ctrl Pts',(0.167342598999944,12.2,-4.69157010700001));
#327948=CARTESIAN_POINT('Ctrl Pts',(0.167342598999944,5.2,-4.69157010700001));
#327949=CARTESIAN_POINT('Ctrl Pts',(0.167342598999944,2.2,-4.69157010700001));
#327950=CARTESIAN_POINT('Ctrl Pts',(0.168777989999944,12.2,-4.69371556500001));
#327951=CARTESIAN_POINT('Ctrl Pts',(0.168777989999944,5.2,-4.69371556500001));
#327952=CARTESIAN_POINT('Ctrl Pts',(0.168777989999944,2.2,-4.69371556500001));
#327953=CARTESIAN_POINT('Ctrl Pts',(0.170217542999945,12.2,-4.69586238700002));
#327954=CARTESIAN_POINT('Ctrl Pts',(0.170217542999945,5.2,-4.69586238700002));
#327955=CARTESIAN_POINT('Ctrl Pts',(0.170217542999945,2.2,-4.69586238700002));
#327956=CARTESIAN_POINT('Ctrl Pts',(0.171661261999944,12.2,-4.69801056600001));
#327957=CARTESIAN_POINT('Ctrl Pts',(0.171661261999944,5.2,-4.69801056600001));
#327958=CARTESIAN_POINT('Ctrl Pts',(0.171661261999944,2.2,-4.69801056600001));
#327959=CARTESIAN_POINT('Ctrl Pts',(0.173109147999944,12.2,-4.70016009300001));
#327960=CARTESIAN_POINT('Ctrl Pts',(0.173109147999944,5.2,-4.70016009300001));
#327961=CARTESIAN_POINT('Ctrl Pts',(0.173109147999944,2.2,-4.70016009300001));
#327962=CARTESIAN_POINT('Ctrl Pts',(0.174561200999944,12.2,-4.70231095900001));
#327963=CARTESIAN_POINT('Ctrl Pts',(0.174561200999944,5.2,-4.70231095900001));
#327964=CARTESIAN_POINT('Ctrl Pts',(0.174561200999944,2.2,-4.70231095900001));
#327965=CARTESIAN_POINT('Ctrl Pts',(0.176017423999945,12.2,-4.70446315400002));
#327966=CARTESIAN_POINT('Ctrl Pts',(0.176017423999945,5.2,-4.70446315400002));
#327967=CARTESIAN_POINT('Ctrl Pts',(0.176017423999945,2.2,-4.70446315400002));
#327968=CARTESIAN_POINT('Ctrl Pts',(0.177477819999944,12.2,-4.70661667200002));
#327969=CARTESIAN_POINT('Ctrl Pts',(0.177477819999944,5.2,-4.70661667200002));
#327970=CARTESIAN_POINT('Ctrl Pts',(0.177477819999944,2.2,-4.70661667200002));
#327971=CARTESIAN_POINT('Ctrl Pts',(0.178942388999944,12.2,-4.70877150100002));
#327972=CARTESIAN_POINT('Ctrl Pts',(0.178942388999944,5.2,-4.70877150100002));
#327973=CARTESIAN_POINT('Ctrl Pts',(0.178942388999944,2.2,-4.70877150100002));
#327974=CARTESIAN_POINT('Ctrl Pts',(0.180411133999945,12.2,-4.71092763500002));
#327975=CARTESIAN_POINT('Ctrl Pts',(0.180411133999945,5.2,-4.71092763500002));
#327976=CARTESIAN_POINT('Ctrl Pts',(0.180411133999945,2.2,-4.71092763500002));
#327977=CARTESIAN_POINT('Ctrl Pts',(0.181884055999945,12.2,-4.71308506500002));
#327978=CARTESIAN_POINT('Ctrl Pts',(0.181884055999945,5.2,-4.71308506500002));
#327979=CARTESIAN_POINT('Ctrl Pts',(0.181884055999945,2.2,-4.71308506500002));
#327980=CARTESIAN_POINT('Ctrl Pts',(0.183361154999944,12.2,-4.71524378400002));
#327981=CARTESIAN_POINT('Ctrl Pts',(0.183361154999944,5.2,-4.71524378400002));
#327982=CARTESIAN_POINT('Ctrl Pts',(0.183361154999944,2.2,-4.71524378400002));
#327983=CARTESIAN_POINT('Ctrl Pts',(0.184842434999943,12.2,-4.71740378300002));
#327984=CARTESIAN_POINT('Ctrl Pts',(0.184842434999943,5.2,-4.71740378300002));
#327985=CARTESIAN_POINT('Ctrl Pts',(0.184842434999943,2.2,-4.71740378300002));
#327986=CARTESIAN_POINT('Ctrl Pts',(0.186327895999945,12.2,-4.71956505600001));
#327987=CARTESIAN_POINT('Ctrl Pts',(0.186327895999945,5.2,-4.71956505600001));
#327988=CARTESIAN_POINT('Ctrl Pts',(0.186327895999945,2.2,-4.71956505600001));
#327989=CARTESIAN_POINT('Ctrl Pts',(0.187817540999945,12.2,-4.72172759400001));
#327990=CARTESIAN_POINT('Ctrl Pts',(0.187817540999945,5.2,-4.72172759400001));
#327991=CARTESIAN_POINT('Ctrl Pts',(0.187817540999945,2.2,-4.72172759400001));
#327992=CARTESIAN_POINT('Ctrl Pts',(0.189311369999944,12.2,-4.72389138700001));
#327993=CARTESIAN_POINT('Ctrl Pts',(0.189311369999944,5.2,-4.72389138700001));
#327994=CARTESIAN_POINT('Ctrl Pts',(0.189311369999944,2.2,-4.72389138700001));
#327995=CARTESIAN_POINT('Ctrl Pts',(0.190809384999945,12.2,-4.72605642400001));
#327996=CARTESIAN_POINT('Ctrl Pts',(0.190809384999945,5.2,-4.72605642400001));
#327997=CARTESIAN_POINT('Ctrl Pts',(0.190809384999945,2.2,-4.72605642400001));
#327998=CARTESIAN_POINT('Ctrl Pts',(0.192311589999944,12.2,-4.72822269600002));
#327999=CARTESIAN_POINT('Ctrl Pts',(0.192311589999944,5.2,-4.72822269600002));
#328000=CARTESIAN_POINT('Ctrl Pts',(0.192311589999944,2.2,-4.72822269600002));
#328001=CARTESIAN_POINT('Ctrl Pts',(0.193817984999944,12.2,-4.73039019200002));
#328002=CARTESIAN_POINT('Ctrl Pts',(0.193817984999944,5.2,-4.73039019200002));
#328003=CARTESIAN_POINT('Ctrl Pts',(0.193817984999944,2.2,-4.73039019200002));
#328004=CARTESIAN_POINT('Ctrl Pts',(0.195328572999944,12.2,-4.73255890000001));
#328005=CARTESIAN_POINT('Ctrl Pts',(0.195328572999944,5.2,-4.73255890000001));
#328006=CARTESIAN_POINT('Ctrl Pts',(0.195328572999944,2.2,-4.73255890000001));
#328007=CARTESIAN_POINT('Ctrl Pts',(0.196843354999944,12.2,-4.73472881600001));
#328008=CARTESIAN_POINT('Ctrl Pts',(0.196843354999944,5.2,-4.73472881600001));
#328009=CARTESIAN_POINT('Ctrl Pts',(0.196843354999944,2.2,-4.73472881600001));
#328010=CARTESIAN_POINT('Ctrl Pts',(0.198362330999944,12.2,-4.73689993200002));
#328011=CARTESIAN_POINT('Ctrl Pts',(0.198362330999944,5.2,-4.73689993200002));
#328012=CARTESIAN_POINT('Ctrl Pts',(0.198362330999944,2.2,-4.73689993200002));
#328013=CARTESIAN_POINT('Ctrl Pts',(0.199885503999945,12.2,-4.73907224400001));
#328014=CARTESIAN_POINT('Ctrl Pts',(0.199885503999945,5.2,-4.73907224400001));
#328015=CARTESIAN_POINT('Ctrl Pts',(0.199885503999945,2.2,-4.73907224400001));
#328016=CARTESIAN_POINT('Ctrl Pts',(0.201412871999944,12.2,-4.74124574900001));
#328017=CARTESIAN_POINT('Ctrl Pts',(0.201412871999944,5.2,-4.74124574900001));
#328018=CARTESIAN_POINT('Ctrl Pts',(0.201412871999944,2.2,-4.74124574900001));
#328019=CARTESIAN_POINT('Ctrl Pts',(0.202638122999945,12.2,-4.74298550700002));
#328020=CARTESIAN_POINT('Ctrl Pts',(0.202638122999945,5.2,-4.74298550700002));
#328021=CARTESIAN_POINT('Ctrl Pts',(0.202638122999945,2.2,-4.74298550700002));
#328022=CARTESIAN_POINT('Ctrl Pts',(0.203558949999945,12.2,-4.74429086200002));
#328023=CARTESIAN_POINT('Ctrl Pts',(0.203558949999945,5.2,-4.74429086200002));
#328024=CARTESIAN_POINT('Ctrl Pts',(0.203558949999945,2.2,-4.74429086200002));
#328025=CARTESIAN_POINT('Ctrl Pts',(0.204173673999944,12.2,-4.74516133800002));
#328026=CARTESIAN_POINT('Ctrl Pts',(0.204173673999944,5.2,-4.74516133800002));
#328027=CARTESIAN_POINT('Ctrl Pts',(0.204173673999944,2.2,-4.74516133800002));
#328028=CARTESIAN_POINT('Ctrl Pts',(0.204481245999943,12.2,-4.74559663400001));
#328029=CARTESIAN_POINT('Ctrl Pts',(0.204481245999943,5.2,-4.74559663400001));
#328030=CARTESIAN_POINT('Ctrl Pts',(0.204481245999943,2.2,-4.74559663400001));
#328031=CARTESIAN_POINT('',(0.204481245999943,2.7,-4.74559663400001));
#328032=CARTESIAN_POINT('',(0.204481245999943,12.2,-4.74559663400001));
#328033=CARTESIAN_POINT('Ctrl Pts',(-0.114861015000055,2.7,-3.99207578600001));
#328034=CARTESIAN_POINT('Ctrl Pts',(-0.114872757025975,2.7,-3.99254553549219));
#328035=CARTESIAN_POINT('Ctrl Pts',(-0.114899241427072,2.70000000000408,
-3.99417468340611));
#328036=CARTESIAN_POINT('Ctrl Pts',(-0.114744299208137,2.70000000000408,
-4.00133406504499));
#328037=CARTESIAN_POINT('Ctrl Pts',(-0.114517346149866,2.70000000000408,
-4.00584622983241));
#328038=CARTESIAN_POINT('Ctrl Pts',(-0.113198568136949,2.70000000000408,
-4.025643335709));
#328039=CARTESIAN_POINT('Ctrl Pts',(-0.111172638029036,2.70000000000408,
-4.04216774748531));
#328040=CARTESIAN_POINT('Ctrl Pts',(-0.101894823642615,2.70000000000408,
-4.10222156454465));
#328041=CARTESIAN_POINT('Ctrl Pts',(-0.0890316803033102,2.7,-4.15849363694796));
#328042=CARTESIAN_POINT('Ctrl Pts',(-0.0185693674509617,2.7,-4.37334076837332));
#328043=CARTESIAN_POINT('Ctrl Pts',(0.0678106861394203,2.7,-4.55217152370141));
#328044=CARTESIAN_POINT('Ctrl Pts',(0.204481245999943,2.7,-4.74559663400001));
#328045=CARTESIAN_POINT('Origin',(-5.66300478732629E-14,15.2,-1.77635683940025E-14));
#328046=CARTESIAN_POINT('',(0.540411127999944,2.7,-4.71915837900002));
#328047=CARTESIAN_POINT('',(0.540411127999944,12.2,-4.71915837900001));
#328048=CARTESIAN_POINT('Origin',(-5.66300478732629E-14,2.7,-1.92943768261394E-14));
#328049=CARTESIAN_POINT('Ctrl Pts',(0.540411127999944,12.2,-4.71915838000001));
#328050=CARTESIAN_POINT('Ctrl Pts',(0.540411127999944,5.2,-4.71915838000001));
#328051=CARTESIAN_POINT('Ctrl Pts',(0.540411127999944,2.2,-4.71915838000001));
#328052=CARTESIAN_POINT('Ctrl Pts',(0.540646816999945,12.2,-4.71868032600002));
#328053=CARTESIAN_POINT('Ctrl Pts',(0.540646816999945,5.2,-4.71868032600002));
#328054=CARTESIAN_POINT('Ctrl Pts',(0.540646816999945,2.2,-4.71868032600002));
#328055=CARTESIAN_POINT('Ctrl Pts',(0.541117799999945,12.2,-4.71772440400001));
#328056=CARTESIAN_POINT('Ctrl Pts',(0.541117799999945,5.2,-4.71772440400001));
#328057=CARTESIAN_POINT('Ctrl Pts',(0.541117799999945,2.2,-4.71772440400001));
#328058=CARTESIAN_POINT('Ctrl Pts',(0.541823087999944,12.2,-4.71629107100001));
#328059=CARTESIAN_POINT('Ctrl Pts',(0.541823087999944,5.2,-4.71629107100001));
#328060=CARTESIAN_POINT('Ctrl Pts',(0.541823087999944,2.2,-4.71629107100001));
#328061=CARTESIAN_POINT('Ctrl Pts',(0.542761095999944,12.2,-4.71438106100001));
#328062=CARTESIAN_POINT('Ctrl Pts',(0.542761095999944,5.2,-4.71438106100001));
#328063=CARTESIAN_POINT('Ctrl Pts',(0.542761095999944,2.2,-4.71438106100001));
#328064=CARTESIAN_POINT('Ctrl Pts',(0.543929649999945,12.2,-4.71199538200001));
#328065=CARTESIAN_POINT('Ctrl Pts',(0.543929649999945,5.2,-4.71199538200001));
#328066=CARTESIAN_POINT('Ctrl Pts',(0.543929649999945,2.2,-4.71199538200001));
#328067=CARTESIAN_POINT('Ctrl Pts',(0.545094244999944,12.2,-4.70961153900001));
#328068=CARTESIAN_POINT('Ctrl Pts',(0.545094244999944,5.2,-4.70961153900001));
#328069=CARTESIAN_POINT('Ctrl Pts',(0.545094244999944,2.2,-4.70961153900001));
#328070=CARTESIAN_POINT('Ctrl Pts',(0.546254882999944,12.2,-4.70722953300001));
#328071=CARTESIAN_POINT('Ctrl Pts',(0.546254882999944,5.2,-4.70722953300001));
#328072=CARTESIAN_POINT('Ctrl Pts',(0.546254882999944,2.2,-4.70722953300001));
#328073=CARTESIAN_POINT('Ctrl Pts',(0.547411564999944,12.2,-4.70484936900001));
#328074=CARTESIAN_POINT('Ctrl Pts',(0.547411564999944,5.2,-4.70484936900001));
#328075=CARTESIAN_POINT('Ctrl Pts',(0.547411564999944,2.2,-4.70484936900001));
#328076=CARTESIAN_POINT('Ctrl Pts',(0.548564294999945,12.2,-4.70247105100002));
#328077=CARTESIAN_POINT('Ctrl Pts',(0.548564294999945,5.2,-4.70247105100002));
#328078=CARTESIAN_POINT('Ctrl Pts',(0.548564294999945,2.2,-4.70247105100002));
#328079=CARTESIAN_POINT('Ctrl Pts',(0.549713072999943,12.2,-4.70009458900002));
#328080=CARTESIAN_POINT('Ctrl Pts',(0.549713072999943,5.2,-4.70009458900002));
#328081=CARTESIAN_POINT('Ctrl Pts',(0.549713072999943,2.2,-4.70009458900002));
#328082=CARTESIAN_POINT('Ctrl Pts',(0.550857902999944,12.2,-4.69771999200002));
#328083=CARTESIAN_POINT('Ctrl Pts',(0.550857902999944,5.2,-4.69771999200002));
#328084=CARTESIAN_POINT('Ctrl Pts',(0.550857902999944,2.2,-4.69771999200002));
#328085=CARTESIAN_POINT('Ctrl Pts',(0.551998788999944,12.2,-4.69534726800001));
#328086=CARTESIAN_POINT('Ctrl Pts',(0.551998788999944,5.2,-4.69534726800001));
#328087=CARTESIAN_POINT('Ctrl Pts',(0.551998788999944,2.2,-4.69534726800001));
#328088=CARTESIAN_POINT('Ctrl Pts',(0.553135733999944,12.2,-4.69297642900001));
#328089=CARTESIAN_POINT('Ctrl Pts',(0.553135733999944,5.2,-4.69297642900001));
#328090=CARTESIAN_POINT('Ctrl Pts',(0.553135733999944,2.2,-4.69297642900001));
#328091=CARTESIAN_POINT('Ctrl Pts',(0.554268742999944,12.2,-4.69060748400001));
#328092=CARTESIAN_POINT('Ctrl Pts',(0.554268742999944,5.2,-4.69060748400001));
#328093=CARTESIAN_POINT('Ctrl Pts',(0.554268742999944,2.2,-4.69060748400001));
#328094=CARTESIAN_POINT('Ctrl Pts',(0.555397818999944,12.2,-4.68824044200002));
#328095=CARTESIAN_POINT('Ctrl Pts',(0.555397818999944,5.2,-4.68824044200002));
#328096=CARTESIAN_POINT('Ctrl Pts',(0.555397818999944,2.2,-4.68824044200002));
#328097=CARTESIAN_POINT('Ctrl Pts',(0.556522961999945,12.2,-4.68587531300001));
#328098=CARTESIAN_POINT('Ctrl Pts',(0.556522961999945,5.2,-4.68587531300001));
#328099=CARTESIAN_POINT('Ctrl Pts',(0.556522961999945,2.2,-4.68587531300001));
#328100=CARTESIAN_POINT('Ctrl Pts',(0.557644178999944,12.2,-4.68351210200002));
#328101=CARTESIAN_POINT('Ctrl Pts',(0.557644178999944,5.2,-4.68351210200002));
#328102=CARTESIAN_POINT('Ctrl Pts',(0.557644178999944,2.2,-4.68351210200002));
#328103=CARTESIAN_POINT('Ctrl Pts',(0.558761469999944,12.2,-4.68115081800001));
#328104=CARTESIAN_POINT('Ctrl Pts',(0.558761469999944,5.2,-4.68115081800001));
#328105=CARTESIAN_POINT('Ctrl Pts',(0.558761469999944,2.2,-4.68115081800001));
#328106=CARTESIAN_POINT('Ctrl Pts',(0.559874837999944,12.2,-4.67879146700001));
#328107=CARTESIAN_POINT('Ctrl Pts',(0.559874837999944,5.2,-4.67879146700001));
#328108=CARTESIAN_POINT('Ctrl Pts',(0.559874837999944,2.2,-4.67879146700001));
#328109=CARTESIAN_POINT('Ctrl Pts',(0.560984286999945,12.2,-4.67643405800001));
#328110=CARTESIAN_POINT('Ctrl Pts',(0.560984286999945,5.2,-4.67643405800001));
#328111=CARTESIAN_POINT('Ctrl Pts',(0.560984286999945,2.2,-4.67643405800001));
#328112=CARTESIAN_POINT('Ctrl Pts',(0.562089818999943,12.2,-4.67407859900002));
#328113=CARTESIAN_POINT('Ctrl Pts',(0.562089818999943,5.2,-4.67407859900002));
#328114=CARTESIAN_POINT('Ctrl Pts',(0.562089818999943,2.2,-4.67407859900002));
#328115=CARTESIAN_POINT('Ctrl Pts',(0.563191435999945,12.2,-4.67172509600001));
#328116=CARTESIAN_POINT('Ctrl Pts',(0.563191435999945,5.2,-4.67172509600001));
#328117=CARTESIAN_POINT('Ctrl Pts',(0.563191435999945,2.2,-4.67172509600001));
#328118=CARTESIAN_POINT('Ctrl Pts',(0.564289141999944,12.2,-4.66937355900002));
#328119=CARTESIAN_POINT('Ctrl Pts',(0.564289141999944,5.2,-4.66937355900002));
#328120=CARTESIAN_POINT('Ctrl Pts',(0.564289141999944,2.2,-4.66937355900002));
#328121=CARTESIAN_POINT('Ctrl Pts',(0.565382941999945,12.2,-4.66702399800001));
#328122=CARTESIAN_POINT('Ctrl Pts',(0.565382941999945,5.2,-4.66702399800001));
#328123=CARTESIAN_POINT('Ctrl Pts',(0.565382941999945,2.2,-4.66702399800001));
#328124=CARTESIAN_POINT('Ctrl Pts',(0.566472835999944,12.2,-4.66467641900001));
#328125=CARTESIAN_POINT('Ctrl Pts',(0.566472835999944,5.2,-4.66467641900001));
#328126=CARTESIAN_POINT('Ctrl Pts',(0.566472835999944,2.2,-4.66467641900001));
#328127=CARTESIAN_POINT('Ctrl Pts',(0.567558829999945,12.2,-4.66233083200001));
#328128=CARTESIAN_POINT('Ctrl Pts',(0.567558829999945,5.2,-4.66233083200001));
#328129=CARTESIAN_POINT('Ctrl Pts',(0.567558829999945,2.2,-4.66233083200001));
#328130=CARTESIAN_POINT('Ctrl Pts',(0.568640924999944,12.2,-4.65998724400002));
#328131=CARTESIAN_POINT('Ctrl Pts',(0.568640924999944,5.2,-4.65998724400002));
#328132=CARTESIAN_POINT('Ctrl Pts',(0.568640924999944,2.2,-4.65998724400002));
#328133=CARTESIAN_POINT('Ctrl Pts',(0.569719124999944,12.2,-4.65764566400001));
#328134=CARTESIAN_POINT('Ctrl Pts',(0.569719124999944,5.2,-4.65764566400001));
#328135=CARTESIAN_POINT('Ctrl Pts',(0.569719124999944,2.2,-4.65764566400001));
#328136=CARTESIAN_POINT('Ctrl Pts',(0.570793433999944,12.2,-4.65530610000001));
#328137=CARTESIAN_POINT('Ctrl Pts',(0.570793433999944,5.2,-4.65530610000001));
#328138=CARTESIAN_POINT('Ctrl Pts',(0.570793433999944,2.2,-4.65530610000001));
#328139=CARTESIAN_POINT('Ctrl Pts',(0.571863851999944,12.2,-4.65296856000001));
#328140=CARTESIAN_POINT('Ctrl Pts',(0.571863851999944,5.2,-4.65296856000001));
#328141=CARTESIAN_POINT('Ctrl Pts',(0.571863851999944,2.2,-4.65296856000001));
#328142=CARTESIAN_POINT('Ctrl Pts',(0.572930385999944,12.2,-4.65063305300002));
#328143=CARTESIAN_POINT('Ctrl Pts',(0.572930385999944,5.2,-4.65063305300002));
#328144=CARTESIAN_POINT('Ctrl Pts',(0.572930385999944,2.2,-4.65063305300002));
#328145=CARTESIAN_POINT('Ctrl Pts',(0.573993035999945,12.2,-4.64829958600002));
#328146=CARTESIAN_POINT('Ctrl Pts',(0.573993035999945,5.2,-4.64829958600002));
#328147=CARTESIAN_POINT('Ctrl Pts',(0.573993035999945,2.2,-4.64829958600002));
#328148=CARTESIAN_POINT('Ctrl Pts',(0.575051807999943,12.2,-4.64596816700002));
#328149=CARTESIAN_POINT('Ctrl Pts',(0.575051807999943,5.2,-4.64596816700002));
#328150=CARTESIAN_POINT('Ctrl Pts',(0.575051807999943,2.2,-4.64596816700002));
#328151=CARTESIAN_POINT('Ctrl Pts',(0.576106702999944,12.2,-4.64363880500001));
#328152=CARTESIAN_POINT('Ctrl Pts',(0.576106702999944,5.2,-4.64363880500001));
#328153=CARTESIAN_POINT('Ctrl Pts',(0.576106702999944,2.2,-4.64363880500001));
#328154=CARTESIAN_POINT('Ctrl Pts',(0.577157724999945,12.2,-4.64131150800001));
#328155=CARTESIAN_POINT('Ctrl Pts',(0.577157724999945,5.2,-4.64131150800001));
#328156=CARTESIAN_POINT('Ctrl Pts',(0.577157724999945,2.2,-4.64131150800001));
#328157=CARTESIAN_POINT('Ctrl Pts',(0.578204876999945,12.2,-4.63898628500001));
#328158=CARTESIAN_POINT('Ctrl Pts',(0.578204876999945,5.2,-4.63898628500001));
#328159=CARTESIAN_POINT('Ctrl Pts',(0.578204876999945,2.2,-4.63898628500001));
#328160=CARTESIAN_POINT('Ctrl Pts',(0.579248161999945,12.2,-4.63666314300001));
#328161=CARTESIAN_POINT('Ctrl Pts',(0.579248161999945,5.2,-4.63666314300001));
#328162=CARTESIAN_POINT('Ctrl Pts',(0.579248161999945,2.2,-4.63666314300001));
#328163=CARTESIAN_POINT('Ctrl Pts',(0.580287583999944,12.2,-4.63434209100001));
#328164=CARTESIAN_POINT('Ctrl Pts',(0.580287583999944,5.2,-4.63434209100001));
#328165=CARTESIAN_POINT('Ctrl Pts',(0.580287583999944,2.2,-4.63434209100001));
#328166=CARTESIAN_POINT('Ctrl Pts',(0.581323146999945,12.2,-4.63202313700001));
#328167=CARTESIAN_POINT('Ctrl Pts',(0.581323146999945,5.2,-4.63202313700001));
#328168=CARTESIAN_POINT('Ctrl Pts',(0.581323146999945,2.2,-4.63202313700001));
#328169=CARTESIAN_POINT('Ctrl Pts',(0.582354852999944,12.2,-4.62970629100001));
#328170=CARTESIAN_POINT('Ctrl Pts',(0.582354852999944,5.2,-4.62970629100001));
#328171=CARTESIAN_POINT('Ctrl Pts',(0.582354852999944,2.2,-4.62970629100001));
#328172=CARTESIAN_POINT('Ctrl Pts',(0.583382704999944,12.2,-4.62739155900001));
#328173=CARTESIAN_POINT('Ctrl Pts',(0.583382704999944,5.2,-4.62739155900001));
#328174=CARTESIAN_POINT('Ctrl Pts',(0.583382704999944,2.2,-4.62739155900001));
#328175=CARTESIAN_POINT('Ctrl Pts',(0.584406706999945,12.2,-4.62507895000002));
#328176=CARTESIAN_POINT('Ctrl Pts',(0.584406706999945,5.2,-4.62507895000002));
#328177=CARTESIAN_POINT('Ctrl Pts',(0.584406706999945,2.2,-4.62507895000002));
#328178=CARTESIAN_POINT('Ctrl Pts',(0.585426862999944,12.2,-4.62276847200001));
#328179=CARTESIAN_POINT('Ctrl Pts',(0.585426862999944,5.2,-4.62276847200001));
#328180=CARTESIAN_POINT('Ctrl Pts',(0.585426862999944,2.2,-4.62276847200001));
#328181=CARTESIAN_POINT('Ctrl Pts',(0.586443174999944,12.2,-4.62046013400002));
#328182=CARTESIAN_POINT('Ctrl Pts',(0.586443174999944,5.2,-4.62046013400002));
#328183=CARTESIAN_POINT('Ctrl Pts',(0.586443174999944,2.2,-4.62046013400002));
#328184=CARTESIAN_POINT('Ctrl Pts',(0.587455645999944,12.2,-4.61815394400002));
#328185=CARTESIAN_POINT('Ctrl Pts',(0.587455645999944,5.2,-4.61815394400002));
#328186=CARTESIAN_POINT('Ctrl Pts',(0.587455645999944,2.2,-4.61815394400002));
#328187=CARTESIAN_POINT('Ctrl Pts',(0.588464282999944,12.2,-4.61584991100001));
#328188=CARTESIAN_POINT('Ctrl Pts',(0.588464282999944,5.2,-4.61584991100001));
#328189=CARTESIAN_POINT('Ctrl Pts',(0.588464282999944,2.2,-4.61584991100001));
#328190=CARTESIAN_POINT('Ctrl Pts',(0.589469083999944,12.2,-4.61354804200001));
#328191=CARTESIAN_POINT('Ctrl Pts',(0.589469083999944,5.2,-4.61354804200001));
#328192=CARTESIAN_POINT('Ctrl Pts',(0.589469083999944,2.2,-4.61354804200001));
#328193=CARTESIAN_POINT('Ctrl Pts',(0.590470056999944,12.2,-4.61124834600001));
#328194=CARTESIAN_POINT('Ctrl Pts',(0.590470056999944,5.2,-4.61124834600001));
#328195=CARTESIAN_POINT('Ctrl Pts',(0.590470056999944,2.2,-4.61124834600001));
#328196=CARTESIAN_POINT('Ctrl Pts',(0.591467202999943,12.2,-4.60895083100001));
#328197=CARTESIAN_POINT('Ctrl Pts',(0.591467202999943,5.2,-4.60895083100001));
#328198=CARTESIAN_POINT('Ctrl Pts',(0.591467202999943,2.2,-4.60895083100001));
#328199=CARTESIAN_POINT('Ctrl Pts',(0.592460524999944,12.2,-4.60665550600002));
#328200=CARTESIAN_POINT('Ctrl Pts',(0.592460524999944,5.2,-4.60665550600002));
#328201=CARTESIAN_POINT('Ctrl Pts',(0.592460524999944,2.2,-4.60665550600002));
#328202=CARTESIAN_POINT('Ctrl Pts',(0.593450028999943,12.2,-4.60436237900002));
#328203=CARTESIAN_POINT('Ctrl Pts',(0.593450028999943,5.2,-4.60436237900002));
#328204=CARTESIAN_POINT('Ctrl Pts',(0.593450028999943,2.2,-4.60436237900002));
#328205=CARTESIAN_POINT('Ctrl Pts',(0.594435716999944,12.2,-4.60207145800001));
#328206=CARTESIAN_POINT('Ctrl Pts',(0.594435716999944,5.2,-4.60207145800001));
#328207=CARTESIAN_POINT('Ctrl Pts',(0.594435716999944,2.2,-4.60207145800001));
#328208=CARTESIAN_POINT('Ctrl Pts',(0.595417591999944,12.2,-4.59978275200001));
#328209=CARTESIAN_POINT('Ctrl Pts',(0.595417591999944,5.2,-4.59978275200001));
#328210=CARTESIAN_POINT('Ctrl Pts',(0.595417591999944,2.2,-4.59978275200001));
#328211=CARTESIAN_POINT('Ctrl Pts',(0.596395656999944,12.2,-4.59749626800001));
#328212=CARTESIAN_POINT('Ctrl Pts',(0.596395656999944,5.2,-4.59749626800001));
#328213=CARTESIAN_POINT('Ctrl Pts',(0.596395656999944,2.2,-4.59749626800001));
#328214=CARTESIAN_POINT('Ctrl Pts',(0.597369917999945,12.2,-4.59521201700001));
#328215=CARTESIAN_POINT('Ctrl Pts',(0.597369917999945,5.2,-4.59521201700001));
#328216=CARTESIAN_POINT('Ctrl Pts',(0.597369917999945,2.2,-4.59521201700001));
#328217=CARTESIAN_POINT('Ctrl Pts',(0.598340375999945,12.2,-4.59293000500002));
#328218=CARTESIAN_POINT('Ctrl Pts',(0.598340375999945,5.2,-4.59293000500002));
#328219=CARTESIAN_POINT('Ctrl Pts',(0.598340375999945,2.2,-4.59293000500002));
#328220=CARTESIAN_POINT('Ctrl Pts',(0.599307035999944,12.2,-4.59065024100001));
#328221=CARTESIAN_POINT('Ctrl Pts',(0.599307035999944,5.2,-4.59065024100001));
#328222=CARTESIAN_POINT('Ctrl Pts',(0.599307035999944,2.2,-4.59065024100001));
#328223=CARTESIAN_POINT('Ctrl Pts',(0.600269900999945,12.2,-4.58837273300002));
#328224=CARTESIAN_POINT('Ctrl Pts',(0.600269900999945,5.2,-4.58837273300002));
#328225=CARTESIAN_POINT('Ctrl Pts',(0.600269900999945,2.2,-4.58837273300002));
#328226=CARTESIAN_POINT('Ctrl Pts',(0.601228974999944,12.2,-4.58609749100002));
#328227=CARTESIAN_POINT('Ctrl Pts',(0.601228974999944,5.2,-4.58609749100002));
#328228=CARTESIAN_POINT('Ctrl Pts',(0.601228974999944,2.2,-4.58609749100002));
#328229=CARTESIAN_POINT('Ctrl Pts',(0.602184260999944,12.2,-4.58382452200001));
#328230=CARTESIAN_POINT('Ctrl Pts',(0.602184260999944,5.2,-4.58382452200001));
#328231=CARTESIAN_POINT('Ctrl Pts',(0.602184260999944,2.2,-4.58382452200001));
#328232=CARTESIAN_POINT('Ctrl Pts',(0.603135763999945,12.2,-4.58155383400001));
#328233=CARTESIAN_POINT('Ctrl Pts',(0.603135763999945,5.2,-4.58155383400001));
#328234=CARTESIAN_POINT('Ctrl Pts',(0.603135763999945,2.2,-4.58155383400001));
#328235=CARTESIAN_POINT('Ctrl Pts',(0.604083485999943,12.2,-4.57928543600001));
#328236=CARTESIAN_POINT('Ctrl Pts',(0.604083485999943,5.2,-4.57928543600001));
#328237=CARTESIAN_POINT('Ctrl Pts',(0.604083485999943,2.2,-4.57928543600001));
#328238=CARTESIAN_POINT('Ctrl Pts',(0.605027431999944,12.2,-4.57701933800001));
#328239=CARTESIAN_POINT('Ctrl Pts',(0.605027431999944,5.2,-4.57701933800001));
#328240=CARTESIAN_POINT('Ctrl Pts',(0.605027431999944,2.2,-4.57701933800001));
#328241=CARTESIAN_POINT('Ctrl Pts',(0.605967602999944,12.2,-4.57475554500002));
#328242=CARTESIAN_POINT('Ctrl Pts',(0.605967602999944,5.2,-4.57475554500002));
#328243=CARTESIAN_POINT('Ctrl Pts',(0.605967602999944,2.2,-4.57475554500002));
#328244=CARTESIAN_POINT('Ctrl Pts',(0.606904005999944,12.2,-4.57249406800001));
#328245=CARTESIAN_POINT('Ctrl Pts',(0.606904005999944,5.2,-4.57249406800001));
#328246=CARTESIAN_POINT('Ctrl Pts',(0.606904005999944,2.2,-4.57249406800001));
#328247=CARTESIAN_POINT('Ctrl Pts',(0.607836643999944,12.2,-4.57023491600001));
#328248=CARTESIAN_POINT('Ctrl Pts',(0.607836643999944,5.2,-4.57023491600001));
#328249=CARTESIAN_POINT('Ctrl Pts',(0.607836643999944,2.2,-4.57023491600001));
#328250=CARTESIAN_POINT('Ctrl Pts',(0.608765518999944,12.2,-4.56797809500001));
#328251=CARTESIAN_POINT('Ctrl Pts',(0.608765518999944,5.2,-4.56797809500001));
#328252=CARTESIAN_POINT('Ctrl Pts',(0.608765518999944,2.2,-4.56797809500001));
#328253=CARTESIAN_POINT('Ctrl Pts',(0.609690635999944,12.2,-4.56572361400001));
#328254=CARTESIAN_POINT('Ctrl Pts',(0.609690635999944,5.2,-4.56572361400001));
#328255=CARTESIAN_POINT('Ctrl Pts',(0.609690635999944,2.2,-4.56572361400001));
#328256=CARTESIAN_POINT('Ctrl Pts',(0.610611998999944,12.2,-4.56347148200001));
#328257=CARTESIAN_POINT('Ctrl Pts',(0.610611998999944,5.2,-4.56347148200001));
#328258=CARTESIAN_POINT('Ctrl Pts',(0.610611998999944,2.2,-4.56347148200001));
#328259=CARTESIAN_POINT('Ctrl Pts',(0.611529610999945,12.2,-4.56122170900001));
#328260=CARTESIAN_POINT('Ctrl Pts',(0.611529610999945,5.2,-4.56122170900001));
#328261=CARTESIAN_POINT('Ctrl Pts',(0.611529610999945,2.2,-4.56122170900001));
#328262=CARTESIAN_POINT('Ctrl Pts',(0.612443475999944,12.2,-4.55897430100002));
#328263=CARTESIAN_POINT('Ctrl Pts',(0.612443475999944,5.2,-4.55897430100002));
#328264=CARTESIAN_POINT('Ctrl Pts',(0.612443475999944,2.2,-4.55897430100002));
#328265=CARTESIAN_POINT('Ctrl Pts',(0.613353596999944,12.2,-4.55672926800001));
#328266=CARTESIAN_POINT('Ctrl Pts',(0.613353596999944,5.2,-4.55672926800001));
#328267=CARTESIAN_POINT('Ctrl Pts',(0.613353596999944,2.2,-4.55672926800001));
#328268=CARTESIAN_POINT('Ctrl Pts',(0.614259979999944,12.2,-4.55448661800002));
#328269=CARTESIAN_POINT('Ctrl Pts',(0.614259979999944,5.2,-4.55448661800002));
#328270=CARTESIAN_POINT('Ctrl Pts',(0.614259979999944,2.2,-4.55448661800002));
#328271=CARTESIAN_POINT('Ctrl Pts',(0.615162626999944,12.2,-4.55224635800001));
#328272=CARTESIAN_POINT('Ctrl Pts',(0.615162626999944,5.2,-4.55224635800001));
#328273=CARTESIAN_POINT('Ctrl Pts',(0.615162626999944,2.2,-4.55224635800001));
#328274=CARTESIAN_POINT('Ctrl Pts',(0.616061541999944,12.2,-4.55000849900001));
#328275=CARTESIAN_POINT('Ctrl Pts',(0.616061541999944,5.2,-4.55000849900001));
#328276=CARTESIAN_POINT('Ctrl Pts',(0.616061541999944,2.2,-4.55000849900001));
#328277=CARTESIAN_POINT('Ctrl Pts',(0.616956729999945,12.2,-4.54777304800002));
#328278=CARTESIAN_POINT('Ctrl Pts',(0.616956729999945,5.2,-4.54777304800002));
#328279=CARTESIAN_POINT('Ctrl Pts',(0.616956729999945,2.2,-4.54777304800002));
#328280=CARTESIAN_POINT('Ctrl Pts',(0.617848193999944,12.2,-4.54554001400002));
#328281=CARTESIAN_POINT('Ctrl Pts',(0.617848193999944,5.2,-4.54554001400002));
#328282=CARTESIAN_POINT('Ctrl Pts',(0.617848193999944,2.2,-4.54554001400002));
#328283=CARTESIAN_POINT('Ctrl Pts',(0.618735937999944,12.2,-4.54330940500002));
#328284=CARTESIAN_POINT('Ctrl Pts',(0.618735937999944,5.2,-4.54330940500002));
#328285=CARTESIAN_POINT('Ctrl Pts',(0.618735937999944,2.2,-4.54330940500002));
#328286=CARTESIAN_POINT('Ctrl Pts',(0.619619964999945,12.2,-4.54108123000001));
#328287=CARTESIAN_POINT('Ctrl Pts',(0.619619964999945,5.2,-4.54108123000001));
#328288=CARTESIAN_POINT('Ctrl Pts',(0.619619964999945,2.2,-4.54108123000001));
#328289=CARTESIAN_POINT('Ctrl Pts',(0.620500280999944,12.2,-4.53885549700002));
#328290=CARTESIAN_POINT('Ctrl Pts',(0.620500280999944,5.2,-4.53885549700002));
#328291=CARTESIAN_POINT('Ctrl Pts',(0.620500280999944,2.2,-4.53885549700002));
#328292=CARTESIAN_POINT('Ctrl Pts',(0.621376888999944,12.2,-4.53663221500001));
#328293=CARTESIAN_POINT('Ctrl Pts',(0.621376888999944,5.2,-4.53663221500001));
#328294=CARTESIAN_POINT('Ctrl Pts',(0.621376888999944,2.2,-4.53663221500001));
#328295=CARTESIAN_POINT('Ctrl Pts',(0.622249792999944,12.2,-4.53441139300002));
#328296=CARTESIAN_POINT('Ctrl Pts',(0.622249792999944,5.2,-4.53441139300002));
#328297=CARTESIAN_POINT('Ctrl Pts',(0.622249792999944,2.2,-4.53441139300002));
#328298=CARTESIAN_POINT('Ctrl Pts',(0.623118994999944,12.2,-4.53219303800001));
#328299=CARTESIAN_POINT('Ctrl Pts',(0.623118994999944,5.2,-4.53219303800001));
#328300=CARTESIAN_POINT('Ctrl Pts',(0.623118994999944,2.2,-4.53219303800001));
#328301=CARTESIAN_POINT('Ctrl Pts',(0.623984501999945,12.2,-4.52997715900001));
#328302=CARTESIAN_POINT('Ctrl Pts',(0.623984501999945,5.2,-4.52997715900001));
#328303=CARTESIAN_POINT('Ctrl Pts',(0.623984501999945,2.2,-4.52997715900001));
#328304=CARTESIAN_POINT('Ctrl Pts',(0.624846316999944,12.2,-4.52776376600001));
#328305=CARTESIAN_POINT('Ctrl Pts',(0.624846316999944,5.2,-4.52776376600001));
#328306=CARTESIAN_POINT('Ctrl Pts',(0.624846316999944,2.2,-4.52776376600001));
#328307=CARTESIAN_POINT('Ctrl Pts',(0.625704442999945,12.2,-4.52555286600001));
#328308=CARTESIAN_POINT('Ctrl Pts',(0.625704442999945,5.2,-4.52555286600001));
#328309=CARTESIAN_POINT('Ctrl Pts',(0.625704442999945,2.2,-4.52555286600001));
#328310=CARTESIAN_POINT('Ctrl Pts',(0.626558884999944,12.2,-4.52334446800001));
#328311=CARTESIAN_POINT('Ctrl Pts',(0.626558884999944,5.2,-4.52334446800001));
#328312=CARTESIAN_POINT('Ctrl Pts',(0.626558884999944,2.2,-4.52334446800001));
#328313=CARTESIAN_POINT('Ctrl Pts',(0.627409647999944,12.2,-4.52113858100001));
#328314=CARTESIAN_POINT('Ctrl Pts',(0.627409647999944,5.2,-4.52113858100001));
#328315=CARTESIAN_POINT('Ctrl Pts',(0.627409647999944,2.2,-4.52113858100001));
#328316=CARTESIAN_POINT('Ctrl Pts',(0.628256733999945,12.2,-4.51893521300001));
#328317=CARTESIAN_POINT('Ctrl Pts',(0.628256733999945,5.2,-4.51893521300001));
#328318=CARTESIAN_POINT('Ctrl Pts',(0.628256733999945,2.2,-4.51893521300001));
#328319=CARTESIAN_POINT('Ctrl Pts',(0.629100147999945,12.2,-4.51673437200002));
#328320=CARTESIAN_POINT('Ctrl Pts',(0.629100147999945,5.2,-4.51673437200002));
#328321=CARTESIAN_POINT('Ctrl Pts',(0.629100147999945,2.2,-4.51673437200002));
#328322=CARTESIAN_POINT('Ctrl Pts',(0.629939894999944,12.2,-4.51453606800001));
#328323=CARTESIAN_POINT('Ctrl Pts',(0.629939894999944,5.2,-4.51453606800001));
#328324=CARTESIAN_POINT('Ctrl Pts',(0.629939894999944,2.2,-4.51453606800001));
#328325=CARTESIAN_POINT('Ctrl Pts',(0.630775978999945,12.2,-4.51234030800002));
#328326=CARTESIAN_POINT('Ctrl Pts',(0.630775978999945,5.2,-4.51234030800002));
#328327=CARTESIAN_POINT('Ctrl Pts',(0.630775978999945,2.2,-4.51234030800002));
#328328=CARTESIAN_POINT('Ctrl Pts',(0.631608402999944,12.2,-4.51014710200001));
#328329=CARTESIAN_POINT('Ctrl Pts',(0.631608402999944,5.2,-4.51014710200001));
#328330=CARTESIAN_POINT('Ctrl Pts',(0.631608402999944,2.2,-4.51014710200001));
#328331=CARTESIAN_POINT('Ctrl Pts',(0.632437170999944,12.2,-4.50795645800001));
#328332=CARTESIAN_POINT('Ctrl Pts',(0.632437170999944,5.2,-4.50795645800001));
#328333=CARTESIAN_POINT('Ctrl Pts',(0.632437170999944,2.2,-4.50795645800001));
#328334=CARTESIAN_POINT('Ctrl Pts',(0.633262287999944,12.2,-4.50576838500002));
#328335=CARTESIAN_POINT('Ctrl Pts',(0.633262287999944,5.2,-4.50576838500002));
#328336=CARTESIAN_POINT('Ctrl Pts',(0.633262287999944,2.2,-4.50576838500002));
#328337=CARTESIAN_POINT('Ctrl Pts',(0.634083757999945,12.2,-4.50358289100001));
#328338=CARTESIAN_POINT('Ctrl Pts',(0.634083757999945,5.2,-4.50358289100001));
#328339=CARTESIAN_POINT('Ctrl Pts',(0.634083757999945,2.2,-4.50358289100001));
#328340=CARTESIAN_POINT('Ctrl Pts',(0.634901585999944,12.2,-4.50139998400001));
#328341=CARTESIAN_POINT('Ctrl Pts',(0.634901585999944,5.2,-4.50139998400001));
#328342=CARTESIAN_POINT('Ctrl Pts',(0.634901585999944,2.2,-4.50139998400001));
#328343=CARTESIAN_POINT('Ctrl Pts',(0.635715774999944,12.2,-4.49921967400002));
#328344=CARTESIAN_POINT('Ctrl Pts',(0.635715774999944,5.2,-4.49921967400002));
#328345=CARTESIAN_POINT('Ctrl Pts',(0.635715774999944,2.2,-4.49921967400002));
#328346=CARTESIAN_POINT('Ctrl Pts',(0.636526330999944,12.2,-4.49704196900001));
#328347=CARTESIAN_POINT('Ctrl Pts',(0.636526330999944,5.2,-4.49704196900001));
#328348=CARTESIAN_POINT('Ctrl Pts',(0.636526330999944,2.2,-4.49704196900001));
#328349=CARTESIAN_POINT('Ctrl Pts',(0.637333255999945,12.2,-4.49486687800002));
#328350=CARTESIAN_POINT('Ctrl Pts',(0.637333255999945,5.2,-4.49486687800002));
#328351=CARTESIAN_POINT('Ctrl Pts',(0.637333255999945,2.2,-4.49486687800002));
#328352=CARTESIAN_POINT('Ctrl Pts',(0.638136555999944,12.2,-4.49269440900002));
#328353=CARTESIAN_POINT('Ctrl Pts',(0.638136555999944,5.2,-4.49269440900002));
#328354=CARTESIAN_POINT('Ctrl Pts',(0.638136555999944,2.2,-4.49269440900002));
#328355=CARTESIAN_POINT('Ctrl Pts',(0.638936233999944,12.2,-4.49052457000001));
#328356=CARTESIAN_POINT('Ctrl Pts',(0.638936233999944,5.2,-4.49052457000001));
#328357=CARTESIAN_POINT('Ctrl Pts',(0.638936233999944,2.2,-4.49052457000001));
#328358=CARTESIAN_POINT('Ctrl Pts',(0.639732295999944,12.2,-4.48835737200001));
#328359=CARTESIAN_POINT('Ctrl Pts',(0.639732295999944,5.2,-4.48835737200001));
#328360=CARTESIAN_POINT('Ctrl Pts',(0.639732295999944,2.2,-4.48835737200001));
#328361=CARTESIAN_POINT('Ctrl Pts',(0.640524743999944,12.2,-4.48619282100001));
#328362=CARTESIAN_POINT('Ctrl Pts',(0.640524743999944,5.2,-4.48619282100001));
#328363=CARTESIAN_POINT('Ctrl Pts',(0.640524743999944,2.2,-4.48619282100001));
#328364=CARTESIAN_POINT('Ctrl Pts',(0.641313584999944,12.2,-4.48403092800001));
#328365=CARTESIAN_POINT('Ctrl Pts',(0.641313584999944,5.2,-4.48403092800001));
#328366=CARTESIAN_POINT('Ctrl Pts',(0.641313584999944,2.2,-4.48403092800001));
#328367=CARTESIAN_POINT('Ctrl Pts',(0.642098820999945,12.2,-4.48187170000002));
#328368=CARTESIAN_POINT('Ctrl Pts',(0.642098820999945,5.2,-4.48187170000002));
#328369=CARTESIAN_POINT('Ctrl Pts',(0.642098820999945,2.2,-4.48187170000002));
#328370=CARTESIAN_POINT('Ctrl Pts',(0.642880458999944,12.2,-4.47971514600002));
#328371=CARTESIAN_POINT('Ctrl Pts',(0.642880458999944,5.2,-4.47971514600002));
#328372=CARTESIAN_POINT('Ctrl Pts',(0.642880458999944,2.2,-4.47971514600002));
#328373=CARTESIAN_POINT('Ctrl Pts',(0.643658500999944,12.2,-4.47756127500002));
#328374=CARTESIAN_POINT('Ctrl Pts',(0.643658500999944,5.2,-4.47756127500002));
#328375=CARTESIAN_POINT('Ctrl Pts',(0.643658500999944,2.2,-4.47756127500002));
#328376=CARTESIAN_POINT('Ctrl Pts',(0.644432952999944,12.2,-4.47541009600001));
#328377=CARTESIAN_POINT('Ctrl Pts',(0.644432952999944,5.2,-4.47541009600001));
#328378=CARTESIAN_POINT('Ctrl Pts',(0.644432952999944,2.2,-4.47541009600001));
#328379=CARTESIAN_POINT('Ctrl Pts',(0.645203818999944,12.2,-4.47326161700001));
#328380=CARTESIAN_POINT('Ctrl Pts',(0.645203818999944,5.2,-4.47326161700001));
#328381=CARTESIAN_POINT('Ctrl Pts',(0.645203818999944,2.2,-4.47326161700001));
#328382=CARTESIAN_POINT('Ctrl Pts',(0.645971102999944,12.2,-4.47111584600002));
#328383=CARTESIAN_POINT('Ctrl Pts',(0.645971102999944,5.2,-4.47111584600002));
#328384=CARTESIAN_POINT('Ctrl Pts',(0.645971102999944,2.2,-4.47111584600002));
#328385=CARTESIAN_POINT('Ctrl Pts',(0.646734808999944,12.2,-4.46897279400002));
#328386=CARTESIAN_POINT('Ctrl Pts',(0.646734808999944,5.2,-4.46897279400002));
#328387=CARTESIAN_POINT('Ctrl Pts',(0.646734808999944,2.2,-4.46897279400002));
#328388=CARTESIAN_POINT('Ctrl Pts',(0.647494942999944,12.2,-4.46683246700001));
#328389=CARTESIAN_POINT('Ctrl Pts',(0.647494942999944,5.2,-4.46683246700001));
#328390=CARTESIAN_POINT('Ctrl Pts',(0.647494942999944,2.2,-4.46683246700001));
#328391=CARTESIAN_POINT('Ctrl Pts',(0.648251508999944,12.2,-4.46469487600002));
#328392=CARTESIAN_POINT('Ctrl Pts',(0.648251508999944,5.2,-4.46469487600002));
#328393=CARTESIAN_POINT('Ctrl Pts',(0.648251508999944,2.2,-4.46469487600002));
#328394=CARTESIAN_POINT('Ctrl Pts',(0.649004510999944,12.2,-4.46256002700002));
#328395=CARTESIAN_POINT('Ctrl Pts',(0.649004510999944,5.2,-4.46256002700002));
#328396=CARTESIAN_POINT('Ctrl Pts',(0.649004510999944,2.2,-4.46256002700002));
#328397=CARTESIAN_POINT('Ctrl Pts',(0.649753954999944,12.2,-4.46042793300002));
#328398=CARTESIAN_POINT('Ctrl Pts',(0.649753954999944,5.2,-4.46042793300002));
#328399=CARTESIAN_POINT('Ctrl Pts',(0.649753954999944,2.2,-4.46042793300002));
#328400=CARTESIAN_POINT('Ctrl Pts',(0.650499842999944,12.2,-4.45829859800002));
#328401=CARTESIAN_POINT('Ctrl Pts',(0.650499842999944,5.2,-4.45829859800002));
#328402=CARTESIAN_POINT('Ctrl Pts',(0.650499842999944,2.2,-4.45829859800002));
#328403=CARTESIAN_POINT('Ctrl Pts',(0.651242182999944,12.2,-4.45617203400001));
#328404=CARTESIAN_POINT('Ctrl Pts',(0.651242182999944,5.2,-4.45617203400001));
#328405=CARTESIAN_POINT('Ctrl Pts',(0.651242182999944,2.2,-4.45617203400001));
#328406=CARTESIAN_POINT('Ctrl Pts',(0.651980975999944,12.2,-4.45404824800002));
#328407=CARTESIAN_POINT('Ctrl Pts',(0.651980975999944,5.2,-4.45404824800002));
#328408=CARTESIAN_POINT('Ctrl Pts',(0.651980975999944,2.2,-4.45404824800002));
#328409=CARTESIAN_POINT('Ctrl Pts',(0.652716228999944,12.2,-4.45192725000001));
#328410=CARTESIAN_POINT('Ctrl Pts',(0.652716228999944,5.2,-4.45192725000001));
#328411=CARTESIAN_POINT('Ctrl Pts',(0.652716228999944,2.2,-4.45192725000001));
#328412=CARTESIAN_POINT('Ctrl Pts',(0.653447946999944,12.2,-4.44980904800001));
#328413=CARTESIAN_POINT('Ctrl Pts',(0.653447946999944,5.2,-4.44980904800001));
#328414=CARTESIAN_POINT('Ctrl Pts',(0.653447946999944,2.2,-4.44980904800001));
#328415=CARTESIAN_POINT('Ctrl Pts',(0.654176132999944,12.2,-4.44769365000001));
#328416=CARTESIAN_POINT('Ctrl Pts',(0.654176132999944,5.2,-4.44769365000001));
#328417=CARTESIAN_POINT('Ctrl Pts',(0.654176132999944,2.2,-4.44769365000001));
#328418=CARTESIAN_POINT('Ctrl Pts',(0.654900792999944,12.2,-4.44558106600002));
#328419=CARTESIAN_POINT('Ctrl Pts',(0.654900792999944,5.2,-4.44558106600002));
#328420=CARTESIAN_POINT('Ctrl Pts',(0.654900792999944,2.2,-4.44558106600002));
#328421=CARTESIAN_POINT('Ctrl Pts',(0.655621929999944,12.2,-4.44347130500002));
#328422=CARTESIAN_POINT('Ctrl Pts',(0.655621929999944,5.2,-4.44347130500002));
#328423=CARTESIAN_POINT('Ctrl Pts',(0.655621929999944,2.2,-4.44347130500002));
#328424=CARTESIAN_POINT('Ctrl Pts',(0.656339550999945,12.2,-4.44136437500001));
#328425=CARTESIAN_POINT('Ctrl Pts',(0.656339550999945,5.2,-4.44136437500001));
#328426=CARTESIAN_POINT('Ctrl Pts',(0.656339550999945,2.2,-4.44136437500001));
#328427=CARTESIAN_POINT('Ctrl Pts',(0.657053658999944,12.2,-4.43926028400002));
#328428=CARTESIAN_POINT('Ctrl Pts',(0.657053658999944,5.2,-4.43926028400002));
#328429=CARTESIAN_POINT('Ctrl Pts',(0.657053658999944,2.2,-4.43926028400002));
#328430=CARTESIAN_POINT('Ctrl Pts',(0.657764258999943,12.2,-4.43715904200001));
#328431=CARTESIAN_POINT('Ctrl Pts',(0.657764258999943,5.2,-4.43715904200001));
#328432=CARTESIAN_POINT('Ctrl Pts',(0.657764258999943,2.2,-4.43715904200001));
#328433=CARTESIAN_POINT('Ctrl Pts',(0.658471356999945,12.2,-4.43506065900001));
#328434=CARTESIAN_POINT('Ctrl Pts',(0.658471356999945,5.2,-4.43506065900001));
#328435=CARTESIAN_POINT('Ctrl Pts',(0.658471356999945,2.2,-4.43506065900001));
#328436=CARTESIAN_POINT('Ctrl Pts',(0.659174956999945,12.2,-4.43296514000002));
#328437=CARTESIAN_POINT('Ctrl Pts',(0.659174956999945,5.2,-4.43296514000002));
#328438=CARTESIAN_POINT('Ctrl Pts',(0.659174956999945,2.2,-4.43296514000002));
#328439=CARTESIAN_POINT('Ctrl Pts',(0.659875062999945,12.2,-4.43087249800001));
#328440=CARTESIAN_POINT('Ctrl Pts',(0.659875062999945,5.2,-4.43087249800001));
#328441=CARTESIAN_POINT('Ctrl Pts',(0.659875062999945,2.2,-4.43087249800001));
#328442=CARTESIAN_POINT('Ctrl Pts',(0.660571681999944,12.2,-4.42878273800002));
#328443=CARTESIAN_POINT('Ctrl Pts',(0.660571681999944,5.2,-4.42878273800002));
#328444=CARTESIAN_POINT('Ctrl Pts',(0.660571681999944,2.2,-4.42878273800002));
#328445=CARTESIAN_POINT('Ctrl Pts',(0.661264816999945,12.2,-4.42669587300001));
#328446=CARTESIAN_POINT('Ctrl Pts',(0.661264816999945,5.2,-4.42669587300001));
#328447=CARTESIAN_POINT('Ctrl Pts',(0.661264816999945,2.2,-4.42669587300001));
#328448=CARTESIAN_POINT('Ctrl Pts',(0.661954472999944,12.2,-4.42461190800001));
#328449=CARTESIAN_POINT('Ctrl Pts',(0.661954472999944,5.2,-4.42461190800001));
#328450=CARTESIAN_POINT('Ctrl Pts',(0.661954472999944,2.2,-4.42461190800001));
#328451=CARTESIAN_POINT('Ctrl Pts',(0.662640655999944,12.2,-4.42253085400001));
#328452=CARTESIAN_POINT('Ctrl Pts',(0.662640655999944,5.2,-4.42253085400001));
#328453=CARTESIAN_POINT('Ctrl Pts',(0.662640655999944,2.2,-4.42253085400001));
#328454=CARTESIAN_POINT('Ctrl Pts',(0.663323368999944,12.2,-4.42045271900001));
#328455=CARTESIAN_POINT('Ctrl Pts',(0.663323368999944,5.2,-4.42045271900001));
#328456=CARTESIAN_POINT('Ctrl Pts',(0.663323368999944,2.2,-4.42045271900001));
#328457=CARTESIAN_POINT('Ctrl Pts',(0.664002618999944,12.2,-4.41837751200001));
#328458=CARTESIAN_POINT('Ctrl Pts',(0.664002618999944,5.2,-4.41837751200001));
#328459=CARTESIAN_POINT('Ctrl Pts',(0.664002618999944,2.2,-4.41837751200001));
#328460=CARTESIAN_POINT('Ctrl Pts',(0.664678409999944,12.2,-4.41630524100002));
#328461=CARTESIAN_POINT('Ctrl Pts',(0.664678409999944,5.2,-4.41630524100002));
#328462=CARTESIAN_POINT('Ctrl Pts',(0.664678409999944,2.2,-4.41630524100002));
#328463=CARTESIAN_POINT('Ctrl Pts',(0.665350747999944,12.2,-4.41423591700001));
#328464=CARTESIAN_POINT('Ctrl Pts',(0.665350747999944,5.2,-4.41423591700001));
#328465=CARTESIAN_POINT('Ctrl Pts',(0.665350747999944,2.2,-4.41423591700001));
#328466=CARTESIAN_POINT('Ctrl Pts',(0.666019636999944,12.2,-4.41216954700002));
#328467=CARTESIAN_POINT('Ctrl Pts',(0.666019636999944,5.2,-4.41216954700002));
#328468=CARTESIAN_POINT('Ctrl Pts',(0.666019636999944,2.2,-4.41216954700002));
#328469=CARTESIAN_POINT('Ctrl Pts',(0.666685079999944,12.2,-4.41010614100001));
#328470=CARTESIAN_POINT('Ctrl Pts',(0.666685079999944,5.2,-4.41010614100001));
#328471=CARTESIAN_POINT('Ctrl Pts',(0.666685079999944,2.2,-4.41010614100001));
#328472=CARTESIAN_POINT('Ctrl Pts',(0.667347085999944,12.2,-4.40804570700001));
#328473=CARTESIAN_POINT('Ctrl Pts',(0.667347085999944,5.2,-4.40804570700001));
#328474=CARTESIAN_POINT('Ctrl Pts',(0.667347085999944,2.2,-4.40804570700001));
#328475=CARTESIAN_POINT('Ctrl Pts',(0.668005658999945,12.2,-4.40598825400001));
#328476=CARTESIAN_POINT('Ctrl Pts',(0.668005658999945,5.2,-4.40598825400001));
#328477=CARTESIAN_POINT('Ctrl Pts',(0.668005658999945,2.2,-4.40598825400001));
#328478=CARTESIAN_POINT('Ctrl Pts',(0.668660801999944,12.2,-4.40393379100001));
#328479=CARTESIAN_POINT('Ctrl Pts',(0.668660801999944,5.2,-4.40393379100001));
#328480=CARTESIAN_POINT('Ctrl Pts',(0.668660801999944,2.2,-4.40393379100001));
#328481=CARTESIAN_POINT('Ctrl Pts',(0.669312520999944,12.2,-4.40188232700002));
#328482=CARTESIAN_POINT('Ctrl Pts',(0.669312520999944,5.2,-4.40188232700002));
#328483=CARTESIAN_POINT('Ctrl Pts',(0.669312520999944,2.2,-4.40188232700002));
#328484=CARTESIAN_POINT('Ctrl Pts',(0.669960822999944,12.2,-4.39983387200002));
#328485=CARTESIAN_POINT('Ctrl Pts',(0.669960822999944,5.2,-4.39983387200002));
#328486=CARTESIAN_POINT('Ctrl Pts',(0.669960822999944,2.2,-4.39983387200002));
#328487=CARTESIAN_POINT('Ctrl Pts',(0.670605710999944,12.2,-4.39778843200001));
#328488=CARTESIAN_POINT('Ctrl Pts',(0.670605710999944,5.2,-4.39778843200001));
#328489=CARTESIAN_POINT('Ctrl Pts',(0.670605710999944,2.2,-4.39778843200001));
#328490=CARTESIAN_POINT('Ctrl Pts',(0.671247190999944,12.2,-4.39574601800001));
#328491=CARTESIAN_POINT('Ctrl Pts',(0.671247190999944,5.2,-4.39574601800001));
#328492=CARTESIAN_POINT('Ctrl Pts',(0.671247190999944,2.2,-4.39574601800001));
#328493=CARTESIAN_POINT('Ctrl Pts',(0.671885266999944,12.2,-4.39370664000001));
#328494=CARTESIAN_POINT('Ctrl Pts',(0.671885266999944,5.2,-4.39370664000001));
#328495=CARTESIAN_POINT('Ctrl Pts',(0.671885266999944,2.2,-4.39370664000001));
#328496=CARTESIAN_POINT('Ctrl Pts',(0.672519945999944,12.2,-4.39167030400001));
#328497=CARTESIAN_POINT('Ctrl Pts',(0.672519945999944,5.2,-4.39167030400001));
#328498=CARTESIAN_POINT('Ctrl Pts',(0.672519945999944,2.2,-4.39167030400001));
#328499=CARTESIAN_POINT('Ctrl Pts',(0.673151232999943,12.2,-4.38963702100001));
#328500=CARTESIAN_POINT('Ctrl Pts',(0.673151232999943,5.2,-4.38963702100001));
#328501=CARTESIAN_POINT('Ctrl Pts',(0.673151232999943,2.2,-4.38963702100001));
#328502=CARTESIAN_POINT('Ctrl Pts',(0.673779131999944,12.2,-4.38760679800001));
#328503=CARTESIAN_POINT('Ctrl Pts',(0.673779131999944,5.2,-4.38760679800001));
#328504=CARTESIAN_POINT('Ctrl Pts',(0.673779131999944,2.2,-4.38760679800001));
#328505=CARTESIAN_POINT('Ctrl Pts',(0.674403648999945,12.2,-4.38557964800002));
#328506=CARTESIAN_POINT('Ctrl Pts',(0.674403648999945,5.2,-4.38557964800002));
#328507=CARTESIAN_POINT('Ctrl Pts',(0.674403648999945,2.2,-4.38557964800002));
#328508=CARTESIAN_POINT('Ctrl Pts',(0.675024788999944,12.2,-4.38355557500001));
#328509=CARTESIAN_POINT('Ctrl Pts',(0.675024788999944,5.2,-4.38355557500001));
#328510=CARTESIAN_POINT('Ctrl Pts',(0.675024788999944,2.2,-4.38355557500001));
#328511=CARTESIAN_POINT('Ctrl Pts',(0.675642557999944,12.2,-4.38153459100001));
#328512=CARTESIAN_POINT('Ctrl Pts',(0.675642557999944,5.2,-4.38153459100001));
#328513=CARTESIAN_POINT('Ctrl Pts',(0.675642557999944,2.2,-4.38153459100001));
#328514=CARTESIAN_POINT('Ctrl Pts',(0.676256959999945,12.2,-4.37951670400002));
#328515=CARTESIAN_POINT('Ctrl Pts',(0.676256959999945,5.2,-4.37951670400002));
#328516=CARTESIAN_POINT('Ctrl Pts',(0.676256959999945,2.2,-4.37951670400002));
#328517=CARTESIAN_POINT('Ctrl Pts',(0.676868000999944,12.2,-4.37750192300001));
#328518=CARTESIAN_POINT('Ctrl Pts',(0.676868000999944,5.2,-4.37750192300001));
#328519=CARTESIAN_POINT('Ctrl Pts',(0.676868000999944,2.2,-4.37750192300001));
#328520=CARTESIAN_POINT('Ctrl Pts',(0.677475687999943,12.2,-4.37549025700001));
#328521=CARTESIAN_POINT('Ctrl Pts',(0.677475687999943,5.2,-4.37549025700001));
#328522=CARTESIAN_POINT('Ctrl Pts',(0.677475687999943,2.2,-4.37549025700001));
#328523=CARTESIAN_POINT('Ctrl Pts',(0.678080023999944,12.2,-4.37348171500001));
#328524=CARTESIAN_POINT('Ctrl Pts',(0.678080023999944,5.2,-4.37348171500001));
#328525=CARTESIAN_POINT('Ctrl Pts',(0.678080023999944,2.2,-4.37348171500001));
#328526=CARTESIAN_POINT('Ctrl Pts',(0.678681014999943,12.2,-4.37147630700002));
#328527=CARTESIAN_POINT('Ctrl Pts',(0.678681014999943,5.2,-4.37147630700002));
#328528=CARTESIAN_POINT('Ctrl Pts',(0.678681014999943,2.2,-4.37147630700002));
#328529=CARTESIAN_POINT('Ctrl Pts',(0.679278665999944,12.2,-4.36947404000001));
#328530=CARTESIAN_POINT('Ctrl Pts',(0.679278665999944,5.2,-4.36947404000001));
#328531=CARTESIAN_POINT('Ctrl Pts',(0.679278665999944,2.2,-4.36947404000001));
#328532=CARTESIAN_POINT('Ctrl Pts',(0.679872984999944,12.2,-4.36747492400002));
#328533=CARTESIAN_POINT('Ctrl Pts',(0.679872984999944,5.2,-4.36747492400002));
#328534=CARTESIAN_POINT('Ctrl Pts',(0.679872984999944,2.2,-4.36747492400002));
#328535=CARTESIAN_POINT('Ctrl Pts',(0.680463973999944,12.2,-4.36547896800001));
#328536=CARTESIAN_POINT('Ctrl Pts',(0.680463973999944,5.2,-4.36547896800001));
#328537=CARTESIAN_POINT('Ctrl Pts',(0.680463973999944,2.2,-4.36547896800001));
#328538=CARTESIAN_POINT('Ctrl Pts',(0.681051641999945,12.2,-4.36348618100002));
#328539=CARTESIAN_POINT('Ctrl Pts',(0.681051641999945,5.2,-4.36348618100002));
#328540=CARTESIAN_POINT('Ctrl Pts',(0.681051641999945,2.2,-4.36348618100002));
#328541=CARTESIAN_POINT('Ctrl Pts',(0.681635990999945,12.2,-4.36149657200001));
#328542=CARTESIAN_POINT('Ctrl Pts',(0.681635990999945,5.2,-4.36149657200001));
#328543=CARTESIAN_POINT('Ctrl Pts',(0.681635990999945,2.2,-4.36149657200001));
#328544=CARTESIAN_POINT('Ctrl Pts',(0.682217027999944,12.2,-4.35951015100001));
#328545=CARTESIAN_POINT('Ctrl Pts',(0.682217027999944,5.2,-4.35951015100001));
#328546=CARTESIAN_POINT('Ctrl Pts',(0.682217027999944,2.2,-4.35951015100001));
#328547=CARTESIAN_POINT('Ctrl Pts',(0.682794759999944,12.2,-4.35752692500001));
#328548=CARTESIAN_POINT('Ctrl Pts',(0.682794759999944,5.2,-4.35752692500001));
#328549=CARTESIAN_POINT('Ctrl Pts',(0.682794759999944,2.2,-4.35752692500001));
#328550=CARTESIAN_POINT('Ctrl Pts',(0.683369188999944,12.2,-4.35554690300001));
#328551=CARTESIAN_POINT('Ctrl Pts',(0.683369188999944,5.2,-4.35554690300001));
#328552=CARTESIAN_POINT('Ctrl Pts',(0.683369188999944,2.2,-4.35554690300001));
#328553=CARTESIAN_POINT('Ctrl Pts',(0.683940323999944,12.2,-4.35357009800001));
#328554=CARTESIAN_POINT('Ctrl Pts',(0.683940323999944,5.2,-4.35357009800001));
#328555=CARTESIAN_POINT('Ctrl Pts',(0.683940323999944,2.2,-4.35357009800001));
#328556=CARTESIAN_POINT('Ctrl Pts',(0.684508169999944,12.2,-4.35159651300001));
#328557=CARTESIAN_POINT('Ctrl Pts',(0.684508169999944,5.2,-4.35159651300001));
#328558=CARTESIAN_POINT('Ctrl Pts',(0.684508169999944,2.2,-4.35159651300001));
#328559=CARTESIAN_POINT('Ctrl Pts',(0.685072730999944,12.2,-4.34962616200002));
#328560=CARTESIAN_POINT('Ctrl Pts',(0.685072730999944,5.2,-4.34962616200002));
#328561=CARTESIAN_POINT('Ctrl Pts',(0.685072730999944,2.2,-4.34962616200002));
#328562=CARTESIAN_POINT('Ctrl Pts',(0.685634014999944,12.2,-4.34765905300001));
#328563=CARTESIAN_POINT('Ctrl Pts',(0.685634014999944,5.2,-4.34765905300001));
#328564=CARTESIAN_POINT('Ctrl Pts',(0.685634014999944,2.2,-4.34765905300001));
#328565=CARTESIAN_POINT('Ctrl Pts',(0.686192024999944,12.2,-4.34569519300001));
#328566=CARTESIAN_POINT('Ctrl Pts',(0.686192024999944,5.2,-4.34569519300001));
#328567=CARTESIAN_POINT('Ctrl Pts',(0.686192024999944,2.2,-4.34569519300001));
#328568=CARTESIAN_POINT('Ctrl Pts',(0.686746768999944,12.2,-4.34373459300001));
#328569=CARTESIAN_POINT('Ctrl Pts',(0.686746768999944,5.2,-4.34373459300001));
#328570=CARTESIAN_POINT('Ctrl Pts',(0.686746768999944,2.2,-4.34373459300001));
#328571=CARTESIAN_POINT('Ctrl Pts',(0.687298250999944,12.2,-4.34177726100001));
#328572=CARTESIAN_POINT('Ctrl Pts',(0.687298250999944,5.2,-4.34177726100001));
#328573=CARTESIAN_POINT('Ctrl Pts',(0.687298250999944,2.2,-4.34177726100001));
#328574=CARTESIAN_POINT('Ctrl Pts',(0.687846477999944,12.2,-4.33982320600002));
#328575=CARTESIAN_POINT('Ctrl Pts',(0.687846477999944,5.2,-4.33982320600002));
#328576=CARTESIAN_POINT('Ctrl Pts',(0.687846477999944,2.2,-4.33982320600002));
#328577=CARTESIAN_POINT('Ctrl Pts',(0.688391454999944,12.2,-4.33787243900001));
#328578=CARTESIAN_POINT('Ctrl Pts',(0.688391454999944,5.2,-4.33787243900001));
#328579=CARTESIAN_POINT('Ctrl Pts',(0.688391454999944,2.2,-4.33787243900001));
#328580=CARTESIAN_POINT('Ctrl Pts',(0.688933188999944,12.2,-4.33592496700001));
#328581=CARTESIAN_POINT('Ctrl Pts',(0.688933188999944,5.2,-4.33592496700001));
#328582=CARTESIAN_POINT('Ctrl Pts',(0.688933188999944,2.2,-4.33592496700001));
#328583=CARTESIAN_POINT('Ctrl Pts',(0.689471683999944,12.2,-4.33398080000002));
#328584=CARTESIAN_POINT('Ctrl Pts',(0.689471683999944,5.2,-4.33398080000002));
#328585=CARTESIAN_POINT('Ctrl Pts',(0.689471683999944,2.2,-4.33398080000002));
#328586=CARTESIAN_POINT('Ctrl Pts',(0.690006945999944,12.2,-4.33203994700001));
#328587=CARTESIAN_POINT('Ctrl Pts',(0.690006945999944,5.2,-4.33203994700001));
#328588=CARTESIAN_POINT('Ctrl Pts',(0.690006945999944,2.2,-4.33203994700001));
#328589=CARTESIAN_POINT('Ctrl Pts',(0.690538980999944,12.2,-4.33010241700002));
#328590=CARTESIAN_POINT('Ctrl Pts',(0.690538980999944,5.2,-4.33010241700002));
#328591=CARTESIAN_POINT('Ctrl Pts',(0.690538980999944,2.2,-4.33010241700002));
#328592=CARTESIAN_POINT('Ctrl Pts',(0.691067796999943,12.2,-4.32816821900001));
#328593=CARTESIAN_POINT('Ctrl Pts',(0.691067796999943,5.2,-4.32816821900001));
#328594=CARTESIAN_POINT('Ctrl Pts',(0.691067796999943,2.2,-4.32816821900001));
#328595=CARTESIAN_POINT('Ctrl Pts',(0.691593397999944,12.2,-4.32623736200001));
#328596=CARTESIAN_POINT('Ctrl Pts',(0.691593397999944,5.2,-4.32623736200001));
#328597=CARTESIAN_POINT('Ctrl Pts',(0.691593397999944,2.2,-4.32623736200001));
#328598=CARTESIAN_POINT('Ctrl Pts',(0.692115789999944,12.2,-4.32430985600002));
#328599=CARTESIAN_POINT('Ctrl Pts',(0.692115789999944,5.2,-4.32430985600002));
#328600=CARTESIAN_POINT('Ctrl Pts',(0.692115789999944,2.2,-4.32430985600002));
#328601=CARTESIAN_POINT('Ctrl Pts',(0.692634977999944,12.2,-4.32238570900001));
#328602=CARTESIAN_POINT('Ctrl Pts',(0.692634977999944,5.2,-4.32238570900001));
#328603=CARTESIAN_POINT('Ctrl Pts',(0.692634977999944,2.2,-4.32238570900001));
#328604=CARTESIAN_POINT('Ctrl Pts',(0.693150969999944,12.2,-4.32046493100001));
#328605=CARTESIAN_POINT('Ctrl Pts',(0.693150969999944,5.2,-4.32046493100001));
#328606=CARTESIAN_POINT('Ctrl Pts',(0.693150969999944,2.2,-4.32046493100001));
#328607=CARTESIAN_POINT('Ctrl Pts',(0.693663770999944,12.2,-4.31854753200001));
#328608=CARTESIAN_POINT('Ctrl Pts',(0.693663770999944,5.2,-4.31854753200001));
#328609=CARTESIAN_POINT('Ctrl Pts',(0.693663770999944,2.2,-4.31854753200001));
#328610=CARTESIAN_POINT('Ctrl Pts',(0.694173386999944,12.2,-4.31663351900001));
#328611=CARTESIAN_POINT('Ctrl Pts',(0.694173386999944,5.2,-4.31663351900001));
#328612=CARTESIAN_POINT('Ctrl Pts',(0.694173386999944,2.2,-4.31663351900001));
#328613=CARTESIAN_POINT('Ctrl Pts',(0.694679823999944,12.2,-4.31472290200002));
#328614=CARTESIAN_POINT('Ctrl Pts',(0.694679823999944,5.2,-4.31472290200002));
#328615=CARTESIAN_POINT('Ctrl Pts',(0.694679823999944,2.2,-4.31472290200002));
#328616=CARTESIAN_POINT('Ctrl Pts',(0.695183087999944,12.2,-4.31281569100001));
#328617=CARTESIAN_POINT('Ctrl Pts',(0.695183087999944,5.2,-4.31281569100001));
#328618=CARTESIAN_POINT('Ctrl Pts',(0.695183087999944,2.2,-4.31281569100001));
#328619=CARTESIAN_POINT('Ctrl Pts',(0.695683184999945,12.2,-4.31091189300002));
#328620=CARTESIAN_POINT('Ctrl Pts',(0.695683184999945,5.2,-4.31091189300002));
#328621=CARTESIAN_POINT('Ctrl Pts',(0.695683184999945,2.2,-4.31091189300002));
#328622=CARTESIAN_POINT('Ctrl Pts',(0.696180120999944,12.2,-4.30901152000001));
#328623=CARTESIAN_POINT('Ctrl Pts',(0.696180120999944,5.2,-4.30901152000001));
#328624=CARTESIAN_POINT('Ctrl Pts',(0.696180120999944,2.2,-4.30901152000001));
#328625=CARTESIAN_POINT('Ctrl Pts',(0.696673901999944,12.2,-4.30711458000001));
#328626=CARTESIAN_POINT('Ctrl Pts',(0.696673901999944,5.2,-4.30711458000001));
#328627=CARTESIAN_POINT('Ctrl Pts',(0.696673901999944,2.2,-4.30711458000001));
#328628=CARTESIAN_POINT('Ctrl Pts',(0.697164535999945,12.2,-4.30522108300002));
#328629=CARTESIAN_POINT('Ctrl Pts',(0.697164535999945,5.2,-4.30522108300002));
#328630=CARTESIAN_POINT('Ctrl Pts',(0.697164535999945,2.2,-4.30522108300002));
#328631=CARTESIAN_POINT('Ctrl Pts',(0.697652025999944,12.2,-4.30333103500002));
#328632=CARTESIAN_POINT('Ctrl Pts',(0.697652025999944,5.2,-4.30333103500002));
#328633=CARTESIAN_POINT('Ctrl Pts',(0.697652025999944,2.2,-4.30333103500002));
#328634=CARTESIAN_POINT('Ctrl Pts',(0.698136379999944,12.2,-4.30144444900002));
#328635=CARTESIAN_POINT('Ctrl Pts',(0.698136379999944,5.2,-4.30144444900002));
#328636=CARTESIAN_POINT('Ctrl Pts',(0.698136379999944,2.2,-4.30144444900002));
#328637=CARTESIAN_POINT('Ctrl Pts',(0.698617604999944,12.2,-4.29956133300001));
#328638=CARTESIAN_POINT('Ctrl Pts',(0.698617604999944,5.2,-4.29956133300001));
#328639=CARTESIAN_POINT('Ctrl Pts',(0.698617604999944,2.2,-4.29956133300001));
#328640=CARTESIAN_POINT('Ctrl Pts',(0.699095704999944,12.2,-4.29768169500001));
#328641=CARTESIAN_POINT('Ctrl Pts',(0.699095704999944,5.2,-4.29768169500001));
#328642=CARTESIAN_POINT('Ctrl Pts',(0.699095704999944,2.2,-4.29768169500001));
#328643=CARTESIAN_POINT('Ctrl Pts',(0.699570687999944,12.2,-4.29580554600001));
#328644=CARTESIAN_POINT('Ctrl Pts',(0.699570687999944,5.2,-4.29580554600001));
#328645=CARTESIAN_POINT('Ctrl Pts',(0.699570687999944,2.2,-4.29580554600001));
#328646=CARTESIAN_POINT('Ctrl Pts',(0.700042559999944,12.2,-4.29393289400001));
#328647=CARTESIAN_POINT('Ctrl Pts',(0.700042559999944,5.2,-4.29393289400001));
#328648=CARTESIAN_POINT('Ctrl Pts',(0.700042559999944,2.2,-4.29393289400001));
#328649=CARTESIAN_POINT('Ctrl Pts',(0.700511326999944,12.2,-4.29206374900001));
#328650=CARTESIAN_POINT('Ctrl Pts',(0.700511326999944,5.2,-4.29206374900001));
#328651=CARTESIAN_POINT('Ctrl Pts',(0.700511326999944,2.2,-4.29206374900001));
#328652=CARTESIAN_POINT('Ctrl Pts',(0.700976993999943,12.2,-4.29019811900002));
#328653=CARTESIAN_POINT('Ctrl Pts',(0.700976993999943,5.2,-4.29019811900002));
#328654=CARTESIAN_POINT('Ctrl Pts',(0.700976993999943,2.2,-4.29019811900002));
#328655=CARTESIAN_POINT('Ctrl Pts',(0.701439569999944,12.2,-4.28833601600001));
#328656=CARTESIAN_POINT('Ctrl Pts',(0.701439569999944,5.2,-4.28833601600001));
#328657=CARTESIAN_POINT('Ctrl Pts',(0.701439569999944,2.2,-4.28833601600001));
#328658=CARTESIAN_POINT('Ctrl Pts',(0.701899058999944,12.2,-4.28647744700001));
#328659=CARTESIAN_POINT('Ctrl Pts',(0.701899058999944,5.2,-4.28647744700001));
#328660=CARTESIAN_POINT('Ctrl Pts',(0.701899058999944,2.2,-4.28647744700001));
#328661=CARTESIAN_POINT('Ctrl Pts',(0.702355468999943,12.2,-4.28462242100002));
#328662=CARTESIAN_POINT('Ctrl Pts',(0.702355468999943,5.2,-4.28462242100002));
#328663=CARTESIAN_POINT('Ctrl Pts',(0.702355468999943,2.2,-4.28462242100002));
#328664=CARTESIAN_POINT('Ctrl Pts',(0.702808804999945,12.2,-4.28277094800002));
#328665=CARTESIAN_POINT('Ctrl Pts',(0.702808804999945,5.2,-4.28277094800002));
#328666=CARTESIAN_POINT('Ctrl Pts',(0.702808804999945,2.2,-4.28277094800002));
#328667=CARTESIAN_POINT('Ctrl Pts',(0.703259075999945,12.2,-4.28092303800002));
#328668=CARTESIAN_POINT('Ctrl Pts',(0.703259075999945,5.2,-4.28092303800002));
#328669=CARTESIAN_POINT('Ctrl Pts',(0.703259075999945,2.2,-4.28092303800002));
#328670=CARTESIAN_POINT('Ctrl Pts',(0.703706284999944,12.2,-4.27907869900002));
#328671=CARTESIAN_POINT('Ctrl Pts',(0.703706284999944,5.2,-4.27907869900002));
#328672=CARTESIAN_POINT('Ctrl Pts',(0.703706284999944,2.2,-4.27907869900002));
#328673=CARTESIAN_POINT('Ctrl Pts',(0.704150439999944,12.2,-4.27723794100002));
#328674=CARTESIAN_POINT('Ctrl Pts',(0.704150439999944,5.2,-4.27723794100002));
#328675=CARTESIAN_POINT('Ctrl Pts',(0.704150439999944,2.2,-4.27723794100002));
#328676=CARTESIAN_POINT('Ctrl Pts',(0.704591548999944,12.2,-4.27540077300002));
#328677=CARTESIAN_POINT('Ctrl Pts',(0.704591548999944,5.2,-4.27540077300002));
#328678=CARTESIAN_POINT('Ctrl Pts',(0.704591548999944,2.2,-4.27540077300002));
#328679=CARTESIAN_POINT('Ctrl Pts',(0.705029615999945,12.2,-4.27356720500002));
#328680=CARTESIAN_POINT('Ctrl Pts',(0.705029615999945,5.2,-4.27356720500002));
#328681=CARTESIAN_POINT('Ctrl Pts',(0.705029615999945,2.2,-4.27356720500002));
#328682=CARTESIAN_POINT('Ctrl Pts',(0.705464648999944,12.2,-4.27173724500001));
#328683=CARTESIAN_POINT('Ctrl Pts',(0.705464648999944,5.2,-4.27173724500001));
#328684=CARTESIAN_POINT('Ctrl Pts',(0.705464648999944,2.2,-4.27173724500001));
#328685=CARTESIAN_POINT('Ctrl Pts',(0.705896653999945,12.2,-4.26991090400001));
#328686=CARTESIAN_POINT('Ctrl Pts',(0.705896653999945,5.2,-4.26991090400001));
#328687=CARTESIAN_POINT('Ctrl Pts',(0.705896653999945,2.2,-4.26991090400001));
#328688=CARTESIAN_POINT('Ctrl Pts',(0.706325638999944,12.2,-4.26808819000001));
#328689=CARTESIAN_POINT('Ctrl Pts',(0.706325638999944,5.2,-4.26808819000001));
#328690=CARTESIAN_POINT('Ctrl Pts',(0.706325638999944,2.2,-4.26808819000001));
#328691=CARTESIAN_POINT('Ctrl Pts',(0.706751607999945,12.2,-4.26626911400001));
#328692=CARTESIAN_POINT('Ctrl Pts',(0.706751607999945,5.2,-4.26626911400001));
#328693=CARTESIAN_POINT('Ctrl Pts',(0.706751607999945,2.2,-4.26626911400001));
#328694=CARTESIAN_POINT('Ctrl Pts',(0.707174569999944,12.2,-4.26445368300001));
#328695=CARTESIAN_POINT('Ctrl Pts',(0.707174569999944,5.2,-4.26445368300001));
#328696=CARTESIAN_POINT('Ctrl Pts',(0.707174569999944,2.2,-4.26445368300001));
#328697=CARTESIAN_POINT('Ctrl Pts',(0.707594530999944,12.2,-4.26264190800001));
#328698=CARTESIAN_POINT('Ctrl Pts',(0.707594530999944,5.2,-4.26264190800001));
#328699=CARTESIAN_POINT('Ctrl Pts',(0.707594530999944,2.2,-4.26264190800001));
#328700=CARTESIAN_POINT('Ctrl Pts',(0.708011496999944,12.2,-4.26083379800001));
#328701=CARTESIAN_POINT('Ctrl Pts',(0.708011496999944,5.2,-4.26083379800001));
#328702=CARTESIAN_POINT('Ctrl Pts',(0.708011496999944,2.2,-4.26083379800001));
#328703=CARTESIAN_POINT('Ctrl Pts',(0.708425474999944,12.2,-4.25902936100002));
#328704=CARTESIAN_POINT('Ctrl Pts',(0.708425474999944,5.2,-4.25902936100002));
#328705=CARTESIAN_POINT('Ctrl Pts',(0.708425474999944,2.2,-4.25902936100002));
#328706=CARTESIAN_POINT('Ctrl Pts',(0.708836471999944,12.2,-4.25722860900001));
#328707=CARTESIAN_POINT('Ctrl Pts',(0.708836471999944,5.2,-4.25722860900001));
#328708=CARTESIAN_POINT('Ctrl Pts',(0.708836471999944,2.2,-4.25722860900001));
#328709=CARTESIAN_POINT('Ctrl Pts',(0.709244494999944,12.2,-4.25543154900001));
#328710=CARTESIAN_POINT('Ctrl Pts',(0.709244494999944,5.2,-4.25543154900001));
#328711=CARTESIAN_POINT('Ctrl Pts',(0.709244494999944,2.2,-4.25543154900001));
#328712=CARTESIAN_POINT('Ctrl Pts',(0.709649549999944,12.2,-4.25363819200001));
#328713=CARTESIAN_POINT('Ctrl Pts',(0.709649549999944,5.2,-4.25363819200001));
#328714=CARTESIAN_POINT('Ctrl Pts',(0.709649549999944,2.2,-4.25363819200001));
#328715=CARTESIAN_POINT('Ctrl Pts',(0.710051644999944,12.2,-4.25184854700001));
#328716=CARTESIAN_POINT('Ctrl Pts',(0.710051644999944,5.2,-4.25184854700001));
#328717=CARTESIAN_POINT('Ctrl Pts',(0.710051644999944,2.2,-4.25184854700001));
#328718=CARTESIAN_POINT('Ctrl Pts',(0.710450784999944,12.2,-4.25006262200001));
#328719=CARTESIAN_POINT('Ctrl Pts',(0.710450784999944,5.2,-4.25006262200001));
#328720=CARTESIAN_POINT('Ctrl Pts',(0.710450784999944,2.2,-4.25006262200001));
#328721=CARTESIAN_POINT('Ctrl Pts',(0.710846977999945,12.2,-4.24828042900002));
#328722=CARTESIAN_POINT('Ctrl Pts',(0.710846977999945,5.2,-4.24828042900002));
#328723=CARTESIAN_POINT('Ctrl Pts',(0.710846977999945,2.2,-4.24828042900002));
#328724=CARTESIAN_POINT('Ctrl Pts',(0.711240232999945,12.2,-4.24650197500001));
#328725=CARTESIAN_POINT('Ctrl Pts',(0.711240232999945,5.2,-4.24650197500001));
#328726=CARTESIAN_POINT('Ctrl Pts',(0.711240232999945,2.2,-4.24650197500001));
#328727=CARTESIAN_POINT('Ctrl Pts',(0.711630551999944,12.2,-4.24472727100001));
#328728=CARTESIAN_POINT('Ctrl Pts',(0.711630551999944,5.2,-4.24472727100001));
#328729=CARTESIAN_POINT('Ctrl Pts',(0.711630551999944,2.2,-4.24472727100001));
#328730=CARTESIAN_POINT('Ctrl Pts',(0.712017946999944,12.2,-4.24295632600002));
#328731=CARTESIAN_POINT('Ctrl Pts',(0.712017946999944,5.2,-4.24295632600002));
#328732=CARTESIAN_POINT('Ctrl Pts',(0.712017946999944,2.2,-4.24295632600002));
#328733=CARTESIAN_POINT('Ctrl Pts',(0.712402421999945,12.2,-4.24118915000002));
#328734=CARTESIAN_POINT('Ctrl Pts',(0.712402421999945,5.2,-4.24118915000002));
#328735=CARTESIAN_POINT('Ctrl Pts',(0.712402421999945,2.2,-4.24118915000002));
#328736=CARTESIAN_POINT('Ctrl Pts',(0.712783982999944,12.2,-4.23942575000002));
#328737=CARTESIAN_POINT('Ctrl Pts',(0.712783982999944,5.2,-4.23942575000002));
#328738=CARTESIAN_POINT('Ctrl Pts',(0.712783982999944,2.2,-4.23942575000002));
#328739=CARTESIAN_POINT('Ctrl Pts',(0.713162640999945,12.2,-4.23766613800002));
#328740=CARTESIAN_POINT('Ctrl Pts',(0.713162640999945,5.2,-4.23766613800002));
#328741=CARTESIAN_POINT('Ctrl Pts',(0.713162640999945,2.2,-4.23766613800002));
#328742=CARTESIAN_POINT('Ctrl Pts',(0.713538398999944,12.2,-4.23591032200001));
#328743=CARTESIAN_POINT('Ctrl Pts',(0.713538398999944,5.2,-4.23591032200001));
#328744=CARTESIAN_POINT('Ctrl Pts',(0.713538398999944,2.2,-4.23591032200001));
#328745=CARTESIAN_POINT('Ctrl Pts',(0.713911265999945,12.2,-4.23415831300002));
#328746=CARTESIAN_POINT('Ctrl Pts',(0.713911265999945,5.2,-4.23415831300002));
#328747=CARTESIAN_POINT('Ctrl Pts',(0.713911265999945,2.2,-4.23415831300002));
#328748=CARTESIAN_POINT('Ctrl Pts',(0.714281250999944,12.2,-4.23241011900001));
#328749=CARTESIAN_POINT('Ctrl Pts',(0.714281250999944,5.2,-4.23241011900001));
#328750=CARTESIAN_POINT('Ctrl Pts',(0.714281250999944,2.2,-4.23241011900001));
#328751=CARTESIAN_POINT('Ctrl Pts',(0.714648356999944,12.2,-4.23066575100002));
#328752=CARTESIAN_POINT('Ctrl Pts',(0.714648356999944,5.2,-4.23066575100002));
#328753=CARTESIAN_POINT('Ctrl Pts',(0.714648356999944,2.2,-4.23066575100002));
#328754=CARTESIAN_POINT('Ctrl Pts',(0.715012592999944,12.2,-4.22892521700001));
#328755=CARTESIAN_POINT('Ctrl Pts',(0.715012592999944,5.2,-4.22892521700001));
#328756=CARTESIAN_POINT('Ctrl Pts',(0.715012592999944,2.2,-4.22892521700001));
#328757=CARTESIAN_POINT('Ctrl Pts',(0.715373966999944,12.2,-4.22718852600001));
#328758=CARTESIAN_POINT('Ctrl Pts',(0.715373966999944,5.2,-4.22718852600001));
#328759=CARTESIAN_POINT('Ctrl Pts',(0.715373966999944,2.2,-4.22718852600001));
#328760=CARTESIAN_POINT('Ctrl Pts',(0.715732484999945,12.2,-4.22545569000001));
#328761=CARTESIAN_POINT('Ctrl Pts',(0.715732484999945,5.2,-4.22545569000001));
#328762=CARTESIAN_POINT('Ctrl Pts',(0.715732484999945,2.2,-4.22545569000001));
#328763=CARTESIAN_POINT('Ctrl Pts',(0.716088154999944,12.2,-4.22372671600002));
#328764=CARTESIAN_POINT('Ctrl Pts',(0.716088154999944,5.2,-4.22372671600002));
#328765=CARTESIAN_POINT('Ctrl Pts',(0.716088154999944,2.2,-4.22372671600002));
#328766=CARTESIAN_POINT('Ctrl Pts',(0.716440982999944,12.2,-4.22200161500002));
#328767=CARTESIAN_POINT('Ctrl Pts',(0.716440982999944,5.2,-4.22200161500002));
#328768=CARTESIAN_POINT('Ctrl Pts',(0.716440982999944,2.2,-4.22200161500002));
#328769=CARTESIAN_POINT('Ctrl Pts',(0.716790976999944,12.2,-4.22028039700002));
#328770=CARTESIAN_POINT('Ctrl Pts',(0.716790976999944,5.2,-4.22028039700002));
#328771=CARTESIAN_POINT('Ctrl Pts',(0.716790976999944,2.2,-4.22028039700002));
#328772=CARTESIAN_POINT('Ctrl Pts',(0.717138145999944,12.2,-4.21856306900001));
#328773=CARTESIAN_POINT('Ctrl Pts',(0.717138145999944,5.2,-4.21856306900001));
#328774=CARTESIAN_POINT('Ctrl Pts',(0.717138145999944,2.2,-4.21856306900001));
#328775=CARTESIAN_POINT('Ctrl Pts',(0.717482494999944,12.2,-4.21684964300002));
#328776=CARTESIAN_POINT('Ctrl Pts',(0.717482494999944,5.2,-4.21684964300002));
#328777=CARTESIAN_POINT('Ctrl Pts',(0.717482494999944,2.2,-4.21684964300002));
#328778=CARTESIAN_POINT('Ctrl Pts',(0.717824032999944,12.2,-4.21514012700001));
#328779=CARTESIAN_POINT('Ctrl Pts',(0.717824032999944,5.2,-4.21514012700001));
#328780=CARTESIAN_POINT('Ctrl Pts',(0.717824032999944,2.2,-4.21514012700001));
#328781=CARTESIAN_POINT('Ctrl Pts',(0.718162764999944,12.2,-4.21343453200001));
#328782=CARTESIAN_POINT('Ctrl Pts',(0.718162764999944,5.2,-4.21343453200001));
#328783=CARTESIAN_POINT('Ctrl Pts',(0.718162764999944,2.2,-4.21343453200001));
#328784=CARTESIAN_POINT('Ctrl Pts',(0.718498699999944,12.2,-4.21173286600002));
#328785=CARTESIAN_POINT('Ctrl Pts',(0.718498699999944,5.2,-4.21173286600002));
#328786=CARTESIAN_POINT('Ctrl Pts',(0.718498699999944,2.2,-4.21173286600002));
#328787=CARTESIAN_POINT('Ctrl Pts',(0.718831845999944,12.2,-4.21003514000001));
#328788=CARTESIAN_POINT('Ctrl Pts',(0.718831845999944,5.2,-4.21003514000001));
#328789=CARTESIAN_POINT('Ctrl Pts',(0.718831845999944,2.2,-4.21003514000001));
#328790=CARTESIAN_POINT('Ctrl Pts',(0.719162208999945,12.2,-4.20834136300002));
#328791=CARTESIAN_POINT('Ctrl Pts',(0.719162208999945,5.2,-4.20834136300002));
#328792=CARTESIAN_POINT('Ctrl Pts',(0.719162208999945,2.2,-4.20834136300002));
#328793=CARTESIAN_POINT('Ctrl Pts',(0.719489797999944,12.2,-4.20665154400002));
#328794=CARTESIAN_POINT('Ctrl Pts',(0.719489797999944,5.2,-4.20665154400002));
#328795=CARTESIAN_POINT('Ctrl Pts',(0.719489797999944,2.2,-4.20665154400002));
#328796=CARTESIAN_POINT('Ctrl Pts',(0.719814618999944,12.2,-4.20496569300001));
#328797=CARTESIAN_POINT('Ctrl Pts',(0.719814618999944,5.2,-4.20496569300001));
#328798=CARTESIAN_POINT('Ctrl Pts',(0.719814618999944,2.2,-4.20496569300001));
#328799=CARTESIAN_POINT('Ctrl Pts',(0.720136680999944,12.2,-4.20328382000001));
#328800=CARTESIAN_POINT('Ctrl Pts',(0.720136680999944,5.2,-4.20328382000001));
#328801=CARTESIAN_POINT('Ctrl Pts',(0.720136680999944,2.2,-4.20328382000001));
#328802=CARTESIAN_POINT('Ctrl Pts',(0.720455989999944,12.2,-4.20160593400002));
#328803=CARTESIAN_POINT('Ctrl Pts',(0.720455989999944,5.2,-4.20160593400002));
#328804=CARTESIAN_POINT('Ctrl Pts',(0.720455989999944,2.2,-4.20160593400002));
#328805=CARTESIAN_POINT('Ctrl Pts',(0.720772555999944,12.2,-4.19993204500001));
#328806=CARTESIAN_POINT('Ctrl Pts',(0.720772555999944,5.2,-4.19993204500001));
#328807=CARTESIAN_POINT('Ctrl Pts',(0.720772555999944,2.2,-4.19993204500001));
#328808=CARTESIAN_POINT('Ctrl Pts',(0.721086382999945,12.2,-4.19826216300001));
#328809=CARTESIAN_POINT('Ctrl Pts',(0.721086382999945,5.2,-4.19826216300001));
#328810=CARTESIAN_POINT('Ctrl Pts',(0.721086382999945,2.2,-4.19826216300001));
#328811=CARTESIAN_POINT('Ctrl Pts',(0.721397480999945,12.2,-4.19659629700002));
#328812=CARTESIAN_POINT('Ctrl Pts',(0.721397480999945,5.2,-4.19659629700002));
#328813=CARTESIAN_POINT('Ctrl Pts',(0.721397480999945,2.2,-4.19659629700002));
#328814=CARTESIAN_POINT('Ctrl Pts',(0.721705857999945,12.2,-4.19493445500001));
#328815=CARTESIAN_POINT('Ctrl Pts',(0.721705857999945,5.2,-4.19493445500001));
#328816=CARTESIAN_POINT('Ctrl Pts',(0.721705857999945,2.2,-4.19493445500001));
#328817=CARTESIAN_POINT('Ctrl Pts',(0.722011521999945,12.2,-4.19327665100001));
#328818=CARTESIAN_POINT('Ctrl Pts',(0.722011521999945,5.2,-4.19327665100001));
#328819=CARTESIAN_POINT('Ctrl Pts',(0.722011521999945,2.2,-4.19327665100001));
#328820=CARTESIAN_POINT('Ctrl Pts',(0.722314477999944,12.2,-4.19162289000001));
#328821=CARTESIAN_POINT('Ctrl Pts',(0.722314477999944,5.2,-4.19162289000001));
#328822=CARTESIAN_POINT('Ctrl Pts',(0.722314477999944,2.2,-4.19162289000001));
#328823=CARTESIAN_POINT('Ctrl Pts',(0.722614734999943,12.2,-4.18997318500002));
#328824=CARTESIAN_POINT('Ctrl Pts',(0.722614734999943,5.2,-4.18997318500002));
#328825=CARTESIAN_POINT('Ctrl Pts',(0.722614734999943,2.2,-4.18997318500002));
#328826=CARTESIAN_POINT('Ctrl Pts',(0.722912302999944,12.2,-4.18832754300002));
#328827=CARTESIAN_POINT('Ctrl Pts',(0.722912302999944,5.2,-4.18832754300002));
#328828=CARTESIAN_POINT('Ctrl Pts',(0.722912302999944,2.2,-4.18832754300002));
#328829=CARTESIAN_POINT('Ctrl Pts',(0.723207185999944,12.2,-4.18668597600002));
#328830=CARTESIAN_POINT('Ctrl Pts',(0.723207185999944,5.2,-4.18668597600002));
#328831=CARTESIAN_POINT('Ctrl Pts',(0.723207185999944,2.2,-4.18668597600002));
#328832=CARTESIAN_POINT('Ctrl Pts',(0.723499394999945,12.2,-4.18504849200001));
#328833=CARTESIAN_POINT('Ctrl Pts',(0.723499394999945,5.2,-4.18504849200001));
#328834=CARTESIAN_POINT('Ctrl Pts',(0.723499394999945,2.2,-4.18504849200001));
#328835=CARTESIAN_POINT('Ctrl Pts',(0.723788936999944,12.2,-4.18341510300001));
#328836=CARTESIAN_POINT('Ctrl Pts',(0.723788936999944,5.2,-4.18341510300001));
#328837=CARTESIAN_POINT('Ctrl Pts',(0.723788936999944,2.2,-4.18341510300001));
#328838=CARTESIAN_POINT('Ctrl Pts',(0.724075819999944,12.2,-4.18178581500001));
#328839=CARTESIAN_POINT('Ctrl Pts',(0.724075819999944,5.2,-4.18178581500001));
#328840=CARTESIAN_POINT('Ctrl Pts',(0.724075819999944,2.2,-4.18178581500001));
#328841=CARTESIAN_POINT('Ctrl Pts',(0.724360049999944,12.2,-4.18016064100001));
#328842=CARTESIAN_POINT('Ctrl Pts',(0.724360049999944,5.2,-4.18016064100001));
#328843=CARTESIAN_POINT('Ctrl Pts',(0.724360049999944,2.2,-4.18016064100001));
#328844=CARTESIAN_POINT('Ctrl Pts',(0.724641636999944,12.2,-4.17853958900002));
#328845=CARTESIAN_POINT('Ctrl Pts',(0.724641636999944,5.2,-4.17853958900002));
#328846=CARTESIAN_POINT('Ctrl Pts',(0.724641636999944,2.2,-4.17853958900002));
#328847=CARTESIAN_POINT('Ctrl Pts',(0.724920587999944,12.2,-4.17692266800001));
#328848=CARTESIAN_POINT('Ctrl Pts',(0.724920587999944,5.2,-4.17692266800001));
#328849=CARTESIAN_POINT('Ctrl Pts',(0.724920587999944,2.2,-4.17692266800001));
#328850=CARTESIAN_POINT('Ctrl Pts',(0.725196911999944,12.2,-4.17530989100001));
#328851=CARTESIAN_POINT('Ctrl Pts',(0.725196911999944,5.2,-4.17530989100001));
#328852=CARTESIAN_POINT('Ctrl Pts',(0.725196911999944,2.2,-4.17530989100001));
#328853=CARTESIAN_POINT('Ctrl Pts',(0.725470616999945,12.2,-4.17370126400002));
#328854=CARTESIAN_POINT('Ctrl Pts',(0.725470616999945,5.2,-4.17370126400002));
#328855=CARTESIAN_POINT('Ctrl Pts',(0.725470616999945,2.2,-4.17370126400002));
#328856=CARTESIAN_POINT('Ctrl Pts',(0.725741709999944,12.2,-4.17209679900001));
#328857=CARTESIAN_POINT('Ctrl Pts',(0.725741709999944,5.2,-4.17209679900001));
#328858=CARTESIAN_POINT('Ctrl Pts',(0.725741709999944,2.2,-4.17209679900001));
#328859=CARTESIAN_POINT('Ctrl Pts',(0.726010198999945,12.2,-4.17049650500001));
#328860=CARTESIAN_POINT('Ctrl Pts',(0.726010198999945,5.2,-4.17049650500001));
#328861=CARTESIAN_POINT('Ctrl Pts',(0.726010198999945,2.2,-4.17049650500001));
#328862=CARTESIAN_POINT('Ctrl Pts',(0.726276091999944,12.2,-4.16890039200001));
#328863=CARTESIAN_POINT('Ctrl Pts',(0.726276091999944,5.2,-4.16890039200001));
#328864=CARTESIAN_POINT('Ctrl Pts',(0.726276091999944,2.2,-4.16890039200001));
#328865=CARTESIAN_POINT('Ctrl Pts',(0.726539398999945,12.2,-4.16730846900002));
#328866=CARTESIAN_POINT('Ctrl Pts',(0.726539398999945,5.2,-4.16730846900002));
#328867=CARTESIAN_POINT('Ctrl Pts',(0.726539398999945,2.2,-4.16730846900002));
#328868=CARTESIAN_POINT('Ctrl Pts',(0.726800126999944,12.2,-4.16572074700001));
#328869=CARTESIAN_POINT('Ctrl Pts',(0.726800126999944,5.2,-4.16572074700001));
#328870=CARTESIAN_POINT('Ctrl Pts',(0.726800126999944,2.2,-4.16572074700001));
#328871=CARTESIAN_POINT('Ctrl Pts',(0.727058282999944,12.2,-4.16413723500002));
#328872=CARTESIAN_POINT('Ctrl Pts',(0.727058282999944,5.2,-4.16413723500002));
#328873=CARTESIAN_POINT('Ctrl Pts',(0.727058282999944,2.2,-4.16413723500002));
#328874=CARTESIAN_POINT('Ctrl Pts',(0.727313877999943,12.2,-4.16255794200001));
#328875=CARTESIAN_POINT('Ctrl Pts',(0.727313877999943,5.2,-4.16255794200001));
#328876=CARTESIAN_POINT('Ctrl Pts',(0.727313877999943,2.2,-4.16255794200001));
#328877=CARTESIAN_POINT('Ctrl Pts',(0.727566916999944,12.2,-4.16098288000001));
#328878=CARTESIAN_POINT('Ctrl Pts',(0.727566916999944,5.2,-4.16098288000001));
#328879=CARTESIAN_POINT('Ctrl Pts',(0.727566916999944,2.2,-4.16098288000001));
#328880=CARTESIAN_POINT('Ctrl Pts',(0.727817410999945,12.2,-4.15941205600001));
#328881=CARTESIAN_POINT('Ctrl Pts',(0.727817410999945,5.2,-4.15941205600001));
#328882=CARTESIAN_POINT('Ctrl Pts',(0.727817410999945,2.2,-4.15941205600001));
#328883=CARTESIAN_POINT('Ctrl Pts',(0.728065366999945,12.2,-4.15784548300001));
#328884=CARTESIAN_POINT('Ctrl Pts',(0.728065366999945,5.2,-4.15784548300001));
#328885=CARTESIAN_POINT('Ctrl Pts',(0.728065366999945,2.2,-4.15784548300001));
#328886=CARTESIAN_POINT('Ctrl Pts',(0.728310792999943,12.2,-4.15628316800001));
#328887=CARTESIAN_POINT('Ctrl Pts',(0.728310792999943,5.2,-4.15628316800001));
#328888=CARTESIAN_POINT('Ctrl Pts',(0.728310792999943,2.2,-4.15628316800001));
#328889=CARTESIAN_POINT('Ctrl Pts',(0.728553698999944,12.2,-4.15472512200001));
#328890=CARTESIAN_POINT('Ctrl Pts',(0.728553698999944,5.2,-4.15472512200001));
#328891=CARTESIAN_POINT('Ctrl Pts',(0.728553698999944,2.2,-4.15472512200001));
#328892=CARTESIAN_POINT('Ctrl Pts',(0.728794090999945,12.2,-4.15317135500001));
#328893=CARTESIAN_POINT('Ctrl Pts',(0.728794090999945,5.2,-4.15317135500001));
#328894=CARTESIAN_POINT('Ctrl Pts',(0.728794090999945,2.2,-4.15317135500001));
#328895=CARTESIAN_POINT('Ctrl Pts',(0.729031978999944,12.2,-4.15162187600002));
#328896=CARTESIAN_POINT('Ctrl Pts',(0.729031978999944,5.2,-4.15162187600002));
#328897=CARTESIAN_POINT('Ctrl Pts',(0.729031978999944,2.2,-4.15162187600002));
#328898=CARTESIAN_POINT('Ctrl Pts',(0.729267370999944,12.2,-4.15007669700001));
#328899=CARTESIAN_POINT('Ctrl Pts',(0.729267370999944,5.2,-4.15007669700001));
#328900=CARTESIAN_POINT('Ctrl Pts',(0.729267370999944,2.2,-4.15007669700001));
#328901=CARTESIAN_POINT('Ctrl Pts',(0.729500276999944,12.2,-4.14853582400001));
#328902=CARTESIAN_POINT('Ctrl Pts',(0.729500276999944,5.2,-4.14853582400001));
#328903=CARTESIAN_POINT('Ctrl Pts',(0.729500276999944,2.2,-4.14853582400001));
#328904=CARTESIAN_POINT('Ctrl Pts',(0.729730702999943,12.2,-4.14699927100001));
#328905=CARTESIAN_POINT('Ctrl Pts',(0.729730702999943,5.2,-4.14699927100001));
#328906=CARTESIAN_POINT('Ctrl Pts',(0.729730702999943,2.2,-4.14699927100001));
#328907=CARTESIAN_POINT('Ctrl Pts',(0.729958658999944,12.2,-4.14546704400002));
#328908=CARTESIAN_POINT('Ctrl Pts',(0.729958658999944,5.2,-4.14546704400002));
#328909=CARTESIAN_POINT('Ctrl Pts',(0.729958658999944,2.2,-4.14546704400002));
#328910=CARTESIAN_POINT('Ctrl Pts',(0.730184153999944,12.2,-4.14393915700002));
#328911=CARTESIAN_POINT('Ctrl Pts',(0.730184153999944,5.2,-4.14393915700002));
#328912=CARTESIAN_POINT('Ctrl Pts',(0.730184153999944,2.2,-4.14393915700002));
#328913=CARTESIAN_POINT('Ctrl Pts',(0.730407194999944,12.2,-4.14241561600001));
#328914=CARTESIAN_POINT('Ctrl Pts',(0.730407194999944,5.2,-4.14241561600001));
#328915=CARTESIAN_POINT('Ctrl Pts',(0.730407194999944,2.2,-4.14241561600001));
#328916=CARTESIAN_POINT('Ctrl Pts',(0.730627791999944,12.2,-4.14089643400001));
#328917=CARTESIAN_POINT('Ctrl Pts',(0.730627791999944,5.2,-4.14089643400001));
#328918=CARTESIAN_POINT('Ctrl Pts',(0.730627791999944,2.2,-4.14089643400001));
#328919=CARTESIAN_POINT('Ctrl Pts',(0.730845953999945,12.2,-4.13938161900001));
#328920=CARTESIAN_POINT('Ctrl Pts',(0.730845953999945,5.2,-4.13938161900001));
#328921=CARTESIAN_POINT('Ctrl Pts',(0.730845953999945,2.2,-4.13938161900001));
#328922=CARTESIAN_POINT('Ctrl Pts',(0.731061687999944,12.2,-4.13787118200001));
#328923=CARTESIAN_POINT('Ctrl Pts',(0.731061687999944,5.2,-4.13787118200001));
#328924=CARTESIAN_POINT('Ctrl Pts',(0.731061687999944,2.2,-4.13787118200001));
#328925=CARTESIAN_POINT('Ctrl Pts',(0.731275002999944,12.2,-4.13636513200001));
#328926=CARTESIAN_POINT('Ctrl Pts',(0.731275002999944,5.2,-4.13636513200001));
#328927=CARTESIAN_POINT('Ctrl Pts',(0.731275002999944,2.2,-4.13636513200001));
#328928=CARTESIAN_POINT('Ctrl Pts',(0.731485909999944,12.2,-4.13486347900001));
#328929=CARTESIAN_POINT('Ctrl Pts',(0.731485909999944,5.2,-4.13486347900001));
#328930=CARTESIAN_POINT('Ctrl Pts',(0.731485909999944,2.2,-4.13486347900001));
#328931=CARTESIAN_POINT('Ctrl Pts',(0.731694414999944,12.2,-4.13336623300002));
#328932=CARTESIAN_POINT('Ctrl Pts',(0.731694414999944,5.2,-4.13336623300002));
#328933=CARTESIAN_POINT('Ctrl Pts',(0.731694414999944,2.2,-4.13336623300002));
#328934=CARTESIAN_POINT('Ctrl Pts',(0.731900528999944,12.2,-4.13187340400002));
#328935=CARTESIAN_POINT('Ctrl Pts',(0.731900528999944,5.2,-4.13187340400002));
#328936=CARTESIAN_POINT('Ctrl Pts',(0.731900528999944,2.2,-4.13187340400002));
#328937=CARTESIAN_POINT('Ctrl Pts',(0.732104258999944,12.2,-4.13038500300001));
#328938=CARTESIAN_POINT('Ctrl Pts',(0.732104258999944,5.2,-4.13038500300001));
#328939=CARTESIAN_POINT('Ctrl Pts',(0.732104258999944,2.2,-4.13038500300001));
#328940=CARTESIAN_POINT('Ctrl Pts',(0.732305614999944,12.2,-4.12890103900001));
#328941=CARTESIAN_POINT('Ctrl Pts',(0.732305614999944,5.2,-4.12890103900001));
#328942=CARTESIAN_POINT('Ctrl Pts',(0.732305614999944,2.2,-4.12890103900001));
#328943=CARTESIAN_POINT('Ctrl Pts',(0.732504605999944,12.2,-4.12742152100002));
#328944=CARTESIAN_POINT('Ctrl Pts',(0.732504605999944,5.2,-4.12742152100002));
#328945=CARTESIAN_POINT('Ctrl Pts',(0.732504605999944,2.2,-4.12742152100002));
#328946=CARTESIAN_POINT('Ctrl Pts',(0.732701239999944,12.2,-4.12594646000001));
#328947=CARTESIAN_POINT('Ctrl Pts',(0.732701239999944,5.2,-4.12594646000001));
#328948=CARTESIAN_POINT('Ctrl Pts',(0.732701239999944,2.2,-4.12594646000001));
#328949=CARTESIAN_POINT('Ctrl Pts',(0.732895527999945,12.2,-4.12447586700001));
#328950=CARTESIAN_POINT('Ctrl Pts',(0.732895527999945,5.2,-4.12447586700001));
#328951=CARTESIAN_POINT('Ctrl Pts',(0.732895527999945,2.2,-4.12447586700001));
#328952=CARTESIAN_POINT('Ctrl Pts',(0.733087475999944,12.2,-4.12300975000001));
#328953=CARTESIAN_POINT('Ctrl Pts',(0.733087475999944,5.2,-4.12300975000001));
#328954=CARTESIAN_POINT('Ctrl Pts',(0.733087475999944,2.2,-4.12300975000001));
#328955=CARTESIAN_POINT('Ctrl Pts',(0.733277095999945,12.2,-4.12154812100002));
#328956=CARTESIAN_POINT('Ctrl Pts',(0.733277095999945,5.2,-4.12154812100002));
#328957=CARTESIAN_POINT('Ctrl Pts',(0.733277095999945,2.2,-4.12154812100002));
#328958=CARTESIAN_POINT('Ctrl Pts',(0.733464394999944,12.2,-4.12009098900001));
#328959=CARTESIAN_POINT('Ctrl Pts',(0.733464394999944,5.2,-4.12009098900001));
#328960=CARTESIAN_POINT('Ctrl Pts',(0.733464394999944,2.2,-4.12009098900001));
#328961=CARTESIAN_POINT('Ctrl Pts',(0.733649382999944,12.2,-4.11863836300002));
#328962=CARTESIAN_POINT('Ctrl Pts',(0.733649382999944,5.2,-4.11863836300002));
#328963=CARTESIAN_POINT('Ctrl Pts',(0.733649382999944,2.2,-4.11863836300002));
#328964=CARTESIAN_POINT('Ctrl Pts',(0.733832068999944,12.2,-4.11719025400001));
#328965=CARTESIAN_POINT('Ctrl Pts',(0.733832068999944,5.2,-4.11719025400001));
#328966=CARTESIAN_POINT('Ctrl Pts',(0.733832068999944,2.2,-4.11719025400001));
#328967=CARTESIAN_POINT('Ctrl Pts',(0.734012461999944,12.2,-4.11574667300002));
#328968=CARTESIAN_POINT('Ctrl Pts',(0.734012461999944,5.2,-4.11574667300002));
#328969=CARTESIAN_POINT('Ctrl Pts',(0.734012461999944,2.2,-4.11574667300002));
#328970=CARTESIAN_POINT('Ctrl Pts',(0.734190571999944,12.2,-4.11430762700002));
#328971=CARTESIAN_POINT('Ctrl Pts',(0.734190571999944,5.2,-4.11430762700002));
#328972=CARTESIAN_POINT('Ctrl Pts',(0.734190571999944,2.2,-4.11430762700002));
#328973=CARTESIAN_POINT('Ctrl Pts',(0.734366405999943,12.2,-4.11287313100001));
#328974=CARTESIAN_POINT('Ctrl Pts',(0.734366405999943,5.2,-4.11287313100001));
#328975=CARTESIAN_POINT('Ctrl Pts',(0.734366405999943,2.2,-4.11287313100001));
#328976=CARTESIAN_POINT('Ctrl Pts',(0.734539975999944,12.2,-4.11144319000002));
#328977=CARTESIAN_POINT('Ctrl Pts',(0.734539975999944,5.2,-4.11144319000002));
#328978=CARTESIAN_POINT('Ctrl Pts',(0.734539975999944,2.2,-4.11144319000002));
#328979=CARTESIAN_POINT('Ctrl Pts',(0.734711289999944,12.2,-4.11001781700001));
#328980=CARTESIAN_POINT('Ctrl Pts',(0.734711289999944,5.2,-4.11001781700001));
#328981=CARTESIAN_POINT('Ctrl Pts',(0.734711289999944,2.2,-4.11001781700001));
#328982=CARTESIAN_POINT('Ctrl Pts',(0.734880356999944,12.2,-4.10859702100002));
#328983=CARTESIAN_POINT('Ctrl Pts',(0.734880356999944,5.2,-4.10859702100002));
#328984=CARTESIAN_POINT('Ctrl Pts',(0.734880356999944,2.2,-4.10859702100002));
#328985=CARTESIAN_POINT('Ctrl Pts',(0.735047187999944,12.2,-4.10718081300002));
#328986=CARTESIAN_POINT('Ctrl Pts',(0.735047187999944,5.2,-4.10718081300002));
#328987=CARTESIAN_POINT('Ctrl Pts',(0.735047187999944,2.2,-4.10718081300002));
#328988=CARTESIAN_POINT('Ctrl Pts',(0.735211790999944,12.2,-4.10576920200001));
#328989=CARTESIAN_POINT('Ctrl Pts',(0.735211790999944,5.2,-4.10576920200001));
#328990=CARTESIAN_POINT('Ctrl Pts',(0.735211790999944,2.2,-4.10576920200001));
#328991=CARTESIAN_POINT('Ctrl Pts',(0.735374174999944,12.2,-4.10436219900001));
#328992=CARTESIAN_POINT('Ctrl Pts',(0.735374174999944,5.2,-4.10436219900001));
#328993=CARTESIAN_POINT('Ctrl Pts',(0.735374174999944,2.2,-4.10436219900001));
#328994=CARTESIAN_POINT('Ctrl Pts',(0.735534349999944,12.2,-4.10295981200001));
#328995=CARTESIAN_POINT('Ctrl Pts',(0.735534349999944,5.2,-4.10295981200001));
#328996=CARTESIAN_POINT('Ctrl Pts',(0.735534349999944,2.2,-4.10295981200001));
#328997=CARTESIAN_POINT('Ctrl Pts',(0.735692325999944,12.2,-4.10156205400002));
#328998=CARTESIAN_POINT('Ctrl Pts',(0.735692325999944,5.2,-4.10156205400002));
#328999=CARTESIAN_POINT('Ctrl Pts',(0.735692325999944,2.2,-4.10156205400002));
#329000=CARTESIAN_POINT('Ctrl Pts',(0.735848111999945,12.2,-4.10016893300002));
#329001=CARTESIAN_POINT('Ctrl Pts',(0.735848111999945,5.2,-4.10016893300002));
#329002=CARTESIAN_POINT('Ctrl Pts',(0.735848111999945,2.2,-4.10016893300002));
#329003=CARTESIAN_POINT('Ctrl Pts',(0.736001718999945,12.2,-4.09878046200001));
#329004=CARTESIAN_POINT('Ctrl Pts',(0.736001718999945,5.2,-4.09878046200001));
#329005=CARTESIAN_POINT('Ctrl Pts',(0.736001718999945,2.2,-4.09878046200001));
#329006=CARTESIAN_POINT('Ctrl Pts',(0.736153152999944,12.2,-4.09739664800002));
#329007=CARTESIAN_POINT('Ctrl Pts',(0.736153152999944,5.2,-4.09739664800002));
#329008=CARTESIAN_POINT('Ctrl Pts',(0.736153152999944,2.2,-4.09739664800002));
#329009=CARTESIAN_POINT('Ctrl Pts',(0.736302427999944,12.2,-4.09601750200002));
#329010=CARTESIAN_POINT('Ctrl Pts',(0.736302427999944,5.2,-4.09601750200002));
#329011=CARTESIAN_POINT('Ctrl Pts',(0.736302427999944,2.2,-4.09601750200002));
#329012=CARTESIAN_POINT('Ctrl Pts',(0.736449549999943,12.2,-4.09464303500001));
#329013=CARTESIAN_POINT('Ctrl Pts',(0.736449549999943,5.2,-4.09464303500001));
#329014=CARTESIAN_POINT('Ctrl Pts',(0.736449549999943,2.2,-4.09464303500001));
#329015=CARTESIAN_POINT('Ctrl Pts',(0.736594531999945,12.2,-4.09327325700001));
#329016=CARTESIAN_POINT('Ctrl Pts',(0.736594531999945,5.2,-4.09327325700001));
#329017=CARTESIAN_POINT('Ctrl Pts',(0.736594531999945,2.2,-4.09327325700001));
#329018=CARTESIAN_POINT('Ctrl Pts',(0.736737380999944,12.2,-4.09190817700001));
#329019=CARTESIAN_POINT('Ctrl Pts',(0.736737380999944,5.2,-4.09190817700001));
#329020=CARTESIAN_POINT('Ctrl Pts',(0.736737380999944,2.2,-4.09190817700001));
#329021=CARTESIAN_POINT('Ctrl Pts',(0.736878106999944,12.2,-4.09054780600002));
#329022=CARTESIAN_POINT('Ctrl Pts',(0.736878106999944,5.2,-4.09054780600002));
#329023=CARTESIAN_POINT('Ctrl Pts',(0.736878106999944,2.2,-4.09054780600002));
#329024=CARTESIAN_POINT('Ctrl Pts',(0.737016721999945,12.2,-4.08919215500001));
#329025=CARTESIAN_POINT('Ctrl Pts',(0.737016721999945,5.2,-4.08919215500001));
#329026=CARTESIAN_POINT('Ctrl Pts',(0.737016721999945,2.2,-4.08919215500001));
#329027=CARTESIAN_POINT('Ctrl Pts',(0.737153233999944,12.2,-4.08784123200002));
#329028=CARTESIAN_POINT('Ctrl Pts',(0.737153233999944,5.2,-4.08784123200002));
#329029=CARTESIAN_POINT('Ctrl Pts',(0.737153233999944,2.2,-4.08784123200002));
#329030=CARTESIAN_POINT('Ctrl Pts',(0.737287653999944,12.2,-4.08649505000001));
#329031=CARTESIAN_POINT('Ctrl Pts',(0.737287653999944,5.2,-4.08649505000001));
#329032=CARTESIAN_POINT('Ctrl Pts',(0.737287653999944,2.2,-4.08649505000001));
#329033=CARTESIAN_POINT('Ctrl Pts',(0.737419989999945,12.2,-4.08515361700001));
#329034=CARTESIAN_POINT('Ctrl Pts',(0.737419989999945,5.2,-4.08515361700001));
#329035=CARTESIAN_POINT('Ctrl Pts',(0.737419989999945,2.2,-4.08515361700001));
#329036=CARTESIAN_POINT('Ctrl Pts',(0.737550252999944,12.2,-4.08381694400001));
#329037=CARTESIAN_POINT('Ctrl Pts',(0.737550252999944,5.2,-4.08381694400001));
#329038=CARTESIAN_POINT('Ctrl Pts',(0.737550252999944,2.2,-4.08381694400001));
#329039=CARTESIAN_POINT('Ctrl Pts',(0.737678454999945,12.2,-4.08248504200001));
#329040=CARTESIAN_POINT('Ctrl Pts',(0.737678454999945,5.2,-4.08248504200001));
#329041=CARTESIAN_POINT('Ctrl Pts',(0.737678454999945,2.2,-4.08248504200001));
#329042=CARTESIAN_POINT('Ctrl Pts',(0.737804602999944,12.2,-4.08115792000002));
#329043=CARTESIAN_POINT('Ctrl Pts',(0.737804602999944,5.2,-4.08115792000002));
#329044=CARTESIAN_POINT('Ctrl Pts',(0.737804602999944,2.2,-4.08115792000002));
#329045=CARTESIAN_POINT('Ctrl Pts',(0.737928706999944,12.2,-4.07983558900002));
#329046=CARTESIAN_POINT('Ctrl Pts',(0.737928706999944,5.2,-4.07983558900002));
#329047=CARTESIAN_POINT('Ctrl Pts',(0.737928706999944,2.2,-4.07983558900002));
#329048=CARTESIAN_POINT('Ctrl Pts',(0.738050778999945,12.2,-4.07851805900001));
#329049=CARTESIAN_POINT('Ctrl Pts',(0.738050778999945,5.2,-4.07851805900001));
#329050=CARTESIAN_POINT('Ctrl Pts',(0.738050778999945,2.2,-4.07851805900001));
#329051=CARTESIAN_POINT('Ctrl Pts',(0.738170829999943,12.2,-4.07720534100001));
#329052=CARTESIAN_POINT('Ctrl Pts',(0.738170829999943,5.2,-4.07720534100001));
#329053=CARTESIAN_POINT('Ctrl Pts',(0.738170829999943,2.2,-4.07720534100001));
#329054=CARTESIAN_POINT('Ctrl Pts',(0.738288867999944,12.2,-4.07589744400001));
#329055=CARTESIAN_POINT('Ctrl Pts',(0.738288867999944,5.2,-4.07589744400001));
#329056=CARTESIAN_POINT('Ctrl Pts',(0.738288867999944,2.2,-4.07589744400001));
#329057=CARTESIAN_POINT('Ctrl Pts',(0.738404901999944,12.2,-4.07459437900001));
#329058=CARTESIAN_POINT('Ctrl Pts',(0.738404901999944,5.2,-4.07459437900001));
#329059=CARTESIAN_POINT('Ctrl Pts',(0.738404901999944,2.2,-4.07459437900001));
#329060=CARTESIAN_POINT('Ctrl Pts',(0.738518944999944,12.2,-4.07329615600001));
#329061=CARTESIAN_POINT('Ctrl Pts',(0.738518944999944,5.2,-4.07329615600001));
#329062=CARTESIAN_POINT('Ctrl Pts',(0.738518944999944,2.2,-4.07329615600001));
#329063=CARTESIAN_POINT('Ctrl Pts',(0.738631005999945,12.2,-4.07200278500001));
#329064=CARTESIAN_POINT('Ctrl Pts',(0.738631005999945,5.2,-4.07200278500001));
#329065=CARTESIAN_POINT('Ctrl Pts',(0.738631005999945,2.2,-4.07200278500001));
#329066=CARTESIAN_POINT('Ctrl Pts',(0.738741095999944,12.2,-4.07071427800001));
#329067=CARTESIAN_POINT('Ctrl Pts',(0.738741095999944,5.2,-4.07071427800001));
#329068=CARTESIAN_POINT('Ctrl Pts',(0.738741095999944,2.2,-4.07071427800001));
#329069=CARTESIAN_POINT('Ctrl Pts',(0.738849224999945,12.2,-4.06943064400001));
#329070=CARTESIAN_POINT('Ctrl Pts',(0.738849224999945,5.2,-4.06943064400001));
#329071=CARTESIAN_POINT('Ctrl Pts',(0.738849224999945,2.2,-4.06943064400001));
#329072=CARTESIAN_POINT('Ctrl Pts',(0.738955402999945,12.2,-4.06815189300001));
#329073=CARTESIAN_POINT('Ctrl Pts',(0.738955402999945,5.2,-4.06815189300001));
#329074=CARTESIAN_POINT('Ctrl Pts',(0.738955402999945,2.2,-4.06815189300001));
#329075=CARTESIAN_POINT('Ctrl Pts',(0.739059639999944,12.2,-4.06687803500001));
#329076=CARTESIAN_POINT('Ctrl Pts',(0.739059639999944,5.2,-4.06687803500001));
#329077=CARTESIAN_POINT('Ctrl Pts',(0.739059639999944,2.2,-4.06687803500001));
#329078=CARTESIAN_POINT('Ctrl Pts',(0.739161947999943,12.2,-4.06560908300001));
#329079=CARTESIAN_POINT('Ctrl Pts',(0.739161947999943,5.2,-4.06560908300001));
#329080=CARTESIAN_POINT('Ctrl Pts',(0.739161947999943,2.2,-4.06560908300001));
#329081=CARTESIAN_POINT('Ctrl Pts',(0.739262335999944,12.2,-4.06434504400002));
#329082=CARTESIAN_POINT('Ctrl Pts',(0.739262335999944,5.2,-4.06434504400002));
#329083=CARTESIAN_POINT('Ctrl Pts',(0.739262335999944,2.2,-4.06434504400002));
#329084=CARTESIAN_POINT('Ctrl Pts',(0.739360815999944,12.2,-4.06308593100002));
#329085=CARTESIAN_POINT('Ctrl Pts',(0.739360815999944,5.2,-4.06308593100002));
#329086=CARTESIAN_POINT('Ctrl Pts',(0.739360815999944,2.2,-4.06308593100002));
#329087=CARTESIAN_POINT('Ctrl Pts',(0.739457395999944,12.2,-4.06183175400002));
#329088=CARTESIAN_POINT('Ctrl Pts',(0.739457395999944,5.2,-4.06183175400002));
#329089=CARTESIAN_POINT('Ctrl Pts',(0.739457395999944,2.2,-4.06183175400002));
#329090=CARTESIAN_POINT('Ctrl Pts',(0.739552088999944,12.2,-4.06058252100001));
#329091=CARTESIAN_POINT('Ctrl Pts',(0.739552088999944,5.2,-4.06058252100001));
#329092=CARTESIAN_POINT('Ctrl Pts',(0.739552088999944,2.2,-4.06058252100001));
#329093=CARTESIAN_POINT('Ctrl Pts',(0.739644903999944,12.2,-4.05933824500002));
#329094=CARTESIAN_POINT('Ctrl Pts',(0.739644903999944,5.2,-4.05933824500002));
#329095=CARTESIAN_POINT('Ctrl Pts',(0.739644903999944,2.2,-4.05933824500002));
#329096=CARTESIAN_POINT('Ctrl Pts',(0.739735853999944,12.2,-4.05809893600001));
#329097=CARTESIAN_POINT('Ctrl Pts',(0.739735853999944,5.2,-4.05809893600001));
#329098=CARTESIAN_POINT('Ctrl Pts',(0.739735853999944,2.2,-4.05809893600001));
#329099=CARTESIAN_POINT('Ctrl Pts',(0.739824947999944,12.2,-4.05686460300001));
#329100=CARTESIAN_POINT('Ctrl Pts',(0.739824947999944,5.2,-4.05686460300001));
#329101=CARTESIAN_POINT('Ctrl Pts',(0.739824947999944,2.2,-4.05686460300001));
#329102=CARTESIAN_POINT('Ctrl Pts',(0.739912195999944,12.2,-4.05563525900002));
#329103=CARTESIAN_POINT('Ctrl Pts',(0.739912195999944,5.2,-4.05563525900002));
#329104=CARTESIAN_POINT('Ctrl Pts',(0.739912195999944,2.2,-4.05563525900002));
#329105=CARTESIAN_POINT('Ctrl Pts',(0.739997609999944,12.2,-4.05441091100001));
#329106=CARTESIAN_POINT('Ctrl Pts',(0.739997609999944,5.2,-4.05441091100001));
#329107=CARTESIAN_POINT('Ctrl Pts',(0.739997609999944,2.2,-4.05441091100001));
#329108=CARTESIAN_POINT('Ctrl Pts',(0.740081200999944,12.2,-4.05319157200001));
#329109=CARTESIAN_POINT('Ctrl Pts',(0.740081200999944,5.2,-4.05319157200001));
#329110=CARTESIAN_POINT('Ctrl Pts',(0.740081200999944,2.2,-4.05319157200001));
#329111=CARTESIAN_POINT('Ctrl Pts',(0.740162978999944,12.2,-4.05197725200001));
#329112=CARTESIAN_POINT('Ctrl Pts',(0.740162978999944,5.2,-4.05197725200001));
#329113=CARTESIAN_POINT('Ctrl Pts',(0.740162978999944,2.2,-4.05197725200001));
#329114=CARTESIAN_POINT('Ctrl Pts',(0.740242954999945,12.2,-4.05076796100001));
#329115=CARTESIAN_POINT('Ctrl Pts',(0.740242954999945,5.2,-4.05076796100001));
#329116=CARTESIAN_POINT('Ctrl Pts',(0.740242954999945,2.2,-4.05076796100001));
#329117=CARTESIAN_POINT('Ctrl Pts',(0.740321139999944,12.2,-4.04956371000001));
#329118=CARTESIAN_POINT('Ctrl Pts',(0.740321139999944,5.2,-4.04956371000001));
#329119=CARTESIAN_POINT('Ctrl Pts',(0.740321139999944,2.2,-4.04956371000001));
#329120=CARTESIAN_POINT('Ctrl Pts',(0.740397545999943,12.2,-4.04836450900001));
#329121=CARTESIAN_POINT('Ctrl Pts',(0.740397545999943,5.2,-4.04836450900001));
#329122=CARTESIAN_POINT('Ctrl Pts',(0.740397545999943,2.2,-4.04836450900001));
#329123=CARTESIAN_POINT('Ctrl Pts',(0.740472182999944,12.2,-4.04717036800001));
#329124=CARTESIAN_POINT('Ctrl Pts',(0.740472182999944,5.2,-4.04717036800001));
#329125=CARTESIAN_POINT('Ctrl Pts',(0.740472182999944,2.2,-4.04717036800001));
#329126=CARTESIAN_POINT('Ctrl Pts',(0.740545062999944,12.2,-4.04598130000001));
#329127=CARTESIAN_POINT('Ctrl Pts',(0.740545062999944,5.2,-4.04598130000001));
#329128=CARTESIAN_POINT('Ctrl Pts',(0.740545062999944,2.2,-4.04598130000001));
#329129=CARTESIAN_POINT('Ctrl Pts',(0.740616194999945,12.2,-4.04479731300002));
#329130=CARTESIAN_POINT('Ctrl Pts',(0.740616194999945,5.2,-4.04479731300002));
#329131=CARTESIAN_POINT('Ctrl Pts',(0.740616194999945,2.2,-4.04479731300002));
#329132=CARTESIAN_POINT('Ctrl Pts',(0.740685591999944,12.2,-4.04361841700001));
#329133=CARTESIAN_POINT('Ctrl Pts',(0.740685591999944,5.2,-4.04361841700001));
#329134=CARTESIAN_POINT('Ctrl Pts',(0.740685591999944,2.2,-4.04361841700001));
#329135=CARTESIAN_POINT('Ctrl Pts',(0.740753264999944,12.2,-4.04244462600001));
#329136=CARTESIAN_POINT('Ctrl Pts',(0.740753264999944,5.2,-4.04244462600001));
#329137=CARTESIAN_POINT('Ctrl Pts',(0.740753264999944,2.2,-4.04244462600001));
#329138=CARTESIAN_POINT('Ctrl Pts',(0.740819223999944,12.2,-4.04127594600002));
#329139=CARTESIAN_POINT('Ctrl Pts',(0.740819223999944,5.2,-4.04127594600002));
#329140=CARTESIAN_POINT('Ctrl Pts',(0.740819223999944,2.2,-4.04127594600002));
#329141=CARTESIAN_POINT('Ctrl Pts',(0.740883481999944,12.2,-4.04011239200001));
#329142=CARTESIAN_POINT('Ctrl Pts',(0.740883481999944,5.2,-4.04011239200001));
#329143=CARTESIAN_POINT('Ctrl Pts',(0.740883481999944,2.2,-4.04011239200001));
#329144=CARTESIAN_POINT('Ctrl Pts',(0.740946048999944,12.2,-4.03895397100001));
#329145=CARTESIAN_POINT('Ctrl Pts',(0.740946048999944,5.2,-4.03895397100001));
#329146=CARTESIAN_POINT('Ctrl Pts',(0.740946048999944,2.2,-4.03895397100001));
#329147=CARTESIAN_POINT('Ctrl Pts',(0.741006936999944,12.2,-4.03780069600002));
#329148=CARTESIAN_POINT('Ctrl Pts',(0.741006936999944,5.2,-4.03780069600002));
#329149=CARTESIAN_POINT('Ctrl Pts',(0.741006936999944,2.2,-4.03780069600002));
#329150=CARTESIAN_POINT('Ctrl Pts',(0.741066156999944,12.2,-4.03665257700002));
#329151=CARTESIAN_POINT('Ctrl Pts',(0.741066156999944,5.2,-4.03665257700002));
#329152=CARTESIAN_POINT('Ctrl Pts',(0.741066156999944,2.2,-4.03665257700002));
#329153=CARTESIAN_POINT('Ctrl Pts',(0.741123719999944,12.2,-4.03550962400002));
#329154=CARTESIAN_POINT('Ctrl Pts',(0.741123719999944,5.2,-4.03550962400002));
#329155=CARTESIAN_POINT('Ctrl Pts',(0.741123719999944,2.2,-4.03550962400002));
#329156=CARTESIAN_POINT('Ctrl Pts',(0.741179638999945,12.2,-4.03437184700001));
#329157=CARTESIAN_POINT('Ctrl Pts',(0.741179638999945,5.2,-4.03437184700001));
#329158=CARTESIAN_POINT('Ctrl Pts',(0.741179638999945,2.2,-4.03437184700001));
#329159=CARTESIAN_POINT('Ctrl Pts',(0.741233922999944,12.2,-4.03323925800001));
#329160=CARTESIAN_POINT('Ctrl Pts',(0.741233922999944,5.2,-4.03323925800001));
#329161=CARTESIAN_POINT('Ctrl Pts',(0.741233922999944,2.2,-4.03323925800001));
#329162=CARTESIAN_POINT('Ctrl Pts',(0.741286585999944,12.2,-4.03211186800001));
#329163=CARTESIAN_POINT('Ctrl Pts',(0.741286585999944,5.2,-4.03211186800001));
#329164=CARTESIAN_POINT('Ctrl Pts',(0.741286585999944,2.2,-4.03211186800001));
#329165=CARTESIAN_POINT('Ctrl Pts',(0.741337637999945,12.2,-4.03098968600001));
#329166=CARTESIAN_POINT('Ctrl Pts',(0.741337637999945,5.2,-4.03098968600001));
#329167=CARTESIAN_POINT('Ctrl Pts',(0.741337637999945,2.2,-4.03098968600001));
#329168=CARTESIAN_POINT('Ctrl Pts',(0.741387091999944,12.2,-4.02987272300001));
#329169=CARTESIAN_POINT('Ctrl Pts',(0.741387091999944,5.2,-4.02987272300001));
#329170=CARTESIAN_POINT('Ctrl Pts',(0.741387091999944,2.2,-4.02987272300001));
#329171=CARTESIAN_POINT('Ctrl Pts',(0.741434957999945,12.2,-4.02876099100002));
#329172=CARTESIAN_POINT('Ctrl Pts',(0.741434957999945,5.2,-4.02876099100002));
#329173=CARTESIAN_POINT('Ctrl Pts',(0.741434957999945,2.2,-4.02876099100002));
#329174=CARTESIAN_POINT('Ctrl Pts',(0.741481247999943,12.2,-4.02765449900001));
#329175=CARTESIAN_POINT('Ctrl Pts',(0.741481247999943,5.2,-4.02765449900001));
#329176=CARTESIAN_POINT('Ctrl Pts',(0.741481247999943,2.2,-4.02765449900001));
#329177=CARTESIAN_POINT('Ctrl Pts',(0.741525974999945,12.2,-4.02655326000001));
#329178=CARTESIAN_POINT('Ctrl Pts',(0.741525974999945,5.2,-4.02655326000001));
#329179=CARTESIAN_POINT('Ctrl Pts',(0.741525974999945,2.2,-4.02655326000001));
#329180=CARTESIAN_POINT('Ctrl Pts',(0.741569149999944,12.2,-4.02545728100002));
#329181=CARTESIAN_POINT('Ctrl Pts',(0.741569149999944,5.2,-4.02545728100002));
#329182=CARTESIAN_POINT('Ctrl Pts',(0.741569149999944,2.2,-4.02545728100002));
#329183=CARTESIAN_POINT('Ctrl Pts',(0.741610784999944,12.2,-4.02436657600001));
#329184=CARTESIAN_POINT('Ctrl Pts',(0.741610784999944,5.2,-4.02436657600001));
#329185=CARTESIAN_POINT('Ctrl Pts',(0.741610784999944,2.2,-4.02436657600001));
#329186=CARTESIAN_POINT('Ctrl Pts',(0.741650891999944,12.2,-4.02328115500001));
#329187=CARTESIAN_POINT('Ctrl Pts',(0.741650891999944,5.2,-4.02328115500001));
#329188=CARTESIAN_POINT('Ctrl Pts',(0.741650891999944,2.2,-4.02328115500001));
#329189=CARTESIAN_POINT('Ctrl Pts',(0.741689481999944,12.2,-4.02220102700001));
#329190=CARTESIAN_POINT('Ctrl Pts',(0.741689481999944,5.2,-4.02220102700001));
#329191=CARTESIAN_POINT('Ctrl Pts',(0.741689481999944,2.2,-4.02220102700001));
#329192=CARTESIAN_POINT('Ctrl Pts',(0.741726566999944,12.2,-4.02112620600001));
#329193=CARTESIAN_POINT('Ctrl Pts',(0.741726566999944,5.2,-4.02112620600001));
#329194=CARTESIAN_POINT('Ctrl Pts',(0.741726566999944,2.2,-4.02112620600001));
#329195=CARTESIAN_POINT('Ctrl Pts',(0.741762160999944,12.2,-4.02005670000001));
#329196=CARTESIAN_POINT('Ctrl Pts',(0.741762160999944,5.2,-4.02005670000001));
#329197=CARTESIAN_POINT('Ctrl Pts',(0.741762160999944,2.2,-4.02005670000001));
#329198=CARTESIAN_POINT('Ctrl Pts',(0.741796273999944,12.2,-4.01899252000002));
#329199=CARTESIAN_POINT('Ctrl Pts',(0.741796273999944,5.2,-4.01899252000002));
#329200=CARTESIAN_POINT('Ctrl Pts',(0.741796273999944,2.2,-4.01899252000002));
#329201=CARTESIAN_POINT('Ctrl Pts',(0.741828917999944,12.2,-4.01793367800002));
#329202=CARTESIAN_POINT('Ctrl Pts',(0.741828917999944,5.2,-4.01793367800002));
#329203=CARTESIAN_POINT('Ctrl Pts',(0.741828917999944,2.2,-4.01793367800002));
#329204=CARTESIAN_POINT('Ctrl Pts',(0.741860106999944,12.2,-4.01688018300002));
#329205=CARTESIAN_POINT('Ctrl Pts',(0.741860106999944,5.2,-4.01688018300002));
#329206=CARTESIAN_POINT('Ctrl Pts',(0.741860106999944,2.2,-4.01688018300002));
#329207=CARTESIAN_POINT('Ctrl Pts',(0.741889850999944,12.2,-4.01583204800001));
#329208=CARTESIAN_POINT('Ctrl Pts',(0.741889850999944,5.2,-4.01583204800001));
#329209=CARTESIAN_POINT('Ctrl Pts',(0.741889850999944,2.2,-4.01583204800001));
#329210=CARTESIAN_POINT('Ctrl Pts',(0.741918163999945,12.2,-4.01478928300001));
#329211=CARTESIAN_POINT('Ctrl Pts',(0.741918163999945,5.2,-4.01478928300001));
#329212=CARTESIAN_POINT('Ctrl Pts',(0.741918163999945,2.2,-4.01478928300001));
#329213=CARTESIAN_POINT('Ctrl Pts',(0.741945055999944,12.2,-4.01375189800001));
#329214=CARTESIAN_POINT('Ctrl Pts',(0.741945055999944,5.2,-4.01375189800001));
#329215=CARTESIAN_POINT('Ctrl Pts',(0.741945055999944,2.2,-4.01375189800001));
#329216=CARTESIAN_POINT('Ctrl Pts',(0.741970542999945,12.2,-4.01271990400001));
#329217=CARTESIAN_POINT('Ctrl Pts',(0.741970542999945,5.2,-4.01271990400001));
#329218=CARTESIAN_POINT('Ctrl Pts',(0.741970542999945,2.2,-4.01271990400001));
#329219=CARTESIAN_POINT('Ctrl Pts',(0.741994632999944,12.2,-4.01169331300002));
#329220=CARTESIAN_POINT('Ctrl Pts',(0.741994632999944,5.2,-4.01169331300002));
#329221=CARTESIAN_POINT('Ctrl Pts',(0.741994632999944,2.2,-4.01169331300002));
#329222=CARTESIAN_POINT('Ctrl Pts',(0.742017340999944,12.2,-4.01067213400002));
#329223=CARTESIAN_POINT('Ctrl Pts',(0.742017340999944,5.2,-4.01067213400002));
#329224=CARTESIAN_POINT('Ctrl Pts',(0.742017340999944,2.2,-4.01067213400002));
#329225=CARTESIAN_POINT('Ctrl Pts',(0.742038679999945,12.2,-4.00965638100002));
#329226=CARTESIAN_POINT('Ctrl Pts',(0.742038679999945,5.2,-4.00965638100002));
#329227=CARTESIAN_POINT('Ctrl Pts',(0.742038679999945,2.2,-4.00965638100002));
#329228=CARTESIAN_POINT('Ctrl Pts',(0.742058659999943,12.2,-4.00864606100001));
#329229=CARTESIAN_POINT('Ctrl Pts',(0.742058659999943,5.2,-4.00864606100001));
#329230=CARTESIAN_POINT('Ctrl Pts',(0.742058659999943,2.2,-4.00864606100001));
#329231=CARTESIAN_POINT('Ctrl Pts',(0.742077295999944,12.2,-4.00764118700002));
#329232=CARTESIAN_POINT('Ctrl Pts',(0.742077295999944,5.2,-4.00764118700002));
#329233=CARTESIAN_POINT('Ctrl Pts',(0.742077295999944,2.2,-4.00764118700002));
#329234=CARTESIAN_POINT('Ctrl Pts',(0.742094599999944,12.2,-4.00664177000001));
#329235=CARTESIAN_POINT('Ctrl Pts',(0.742094599999944,5.2,-4.00664177000001));
#329236=CARTESIAN_POINT('Ctrl Pts',(0.742094599999944,2.2,-4.00664177000001));
#329237=CARTESIAN_POINT('Ctrl Pts',(0.742110582999944,12.2,-4.00564782000002));
#329238=CARTESIAN_POINT('Ctrl Pts',(0.742110582999944,5.2,-4.00564782000002));
#329239=CARTESIAN_POINT('Ctrl Pts',(0.742110582999944,2.2,-4.00564782000002));
#329240=CARTESIAN_POINT('Ctrl Pts',(0.742125258999944,12.2,-4.00465934800001));
#329241=CARTESIAN_POINT('Ctrl Pts',(0.742125258999944,5.2,-4.00465934800001));
#329242=CARTESIAN_POINT('Ctrl Pts',(0.742125258999944,2.2,-4.00465934800001));
#329243=CARTESIAN_POINT('Ctrl Pts',(0.742138639999944,12.2,-4.00367636600001));
#329244=CARTESIAN_POINT('Ctrl Pts',(0.742138639999944,5.2,-4.00367636600001));
#329245=CARTESIAN_POINT('Ctrl Pts',(0.742138639999944,2.2,-4.00367636600001));
#329246=CARTESIAN_POINT('Ctrl Pts',(0.742150738999944,12.2,-4.00269888500001));
#329247=CARTESIAN_POINT('Ctrl Pts',(0.742150738999944,5.2,-4.00269888500001));
#329248=CARTESIAN_POINT('Ctrl Pts',(0.742150738999944,2.2,-4.00269888500001));
#329249=CARTESIAN_POINT('Ctrl Pts',(0.742161569999944,12.2,-4.00172691400002));
#329250=CARTESIAN_POINT('Ctrl Pts',(0.742161569999944,5.2,-4.00172691400002));
#329251=CARTESIAN_POINT('Ctrl Pts',(0.742161569999944,2.2,-4.00172691400002));
#329252=CARTESIAN_POINT('Ctrl Pts',(0.742171144999944,12.2,-4.00076046600002));
#329253=CARTESIAN_POINT('Ctrl Pts',(0.742171144999944,5.2,-4.00076046600002));
#329254=CARTESIAN_POINT('Ctrl Pts',(0.742171144999944,2.2,-4.00076046600002));
#329255=CARTESIAN_POINT('Ctrl Pts',(0.742179474999943,12.2,-3.99979955000001));
#329256=CARTESIAN_POINT('Ctrl Pts',(0.742179474999943,5.2,-3.99979955000001));
#329257=CARTESIAN_POINT('Ctrl Pts',(0.742179474999943,2.2,-3.99979955000001));
#329258=CARTESIAN_POINT('Ctrl Pts',(0.742186576999945,12.2,-3.99884418000001));
#329259=CARTESIAN_POINT('Ctrl Pts',(0.742186576999945,5.2,-3.99884418000001));
#329260=CARTESIAN_POINT('Ctrl Pts',(0.742186576999945,2.2,-3.99884418000001));
#329261=CARTESIAN_POINT('Ctrl Pts',(0.742192459999944,12.2,-3.99789436300001));
#329262=CARTESIAN_POINT('Ctrl Pts',(0.742192459999944,5.2,-3.99789436300001));
#329263=CARTESIAN_POINT('Ctrl Pts',(0.742192459999944,2.2,-3.99789436300001));
#329264=CARTESIAN_POINT('Ctrl Pts',(0.742197139999944,12.2,-3.99695011400001));
#329265=CARTESIAN_POINT('Ctrl Pts',(0.742197139999944,5.2,-3.99695011400001));
#329266=CARTESIAN_POINT('Ctrl Pts',(0.742197139999944,2.2,-3.99695011400001));
#329267=CARTESIAN_POINT('Ctrl Pts',(0.742200627999944,12.2,-3.99601144100002));
#329268=CARTESIAN_POINT('Ctrl Pts',(0.742200627999944,5.2,-3.99601144100002));
#329269=CARTESIAN_POINT('Ctrl Pts',(0.742200627999944,2.2,-3.99601144100002));
#329270=CARTESIAN_POINT('Ctrl Pts',(0.742202937999944,12.2,-3.99507835700001));
#329271=CARTESIAN_POINT('Ctrl Pts',(0.742202937999944,5.2,-3.99507835700001));
#329272=CARTESIAN_POINT('Ctrl Pts',(0.742202937999944,2.2,-3.99507835700001));
#329273=CARTESIAN_POINT('Ctrl Pts',(0.742204082999944,12.2,-3.99415087100001));
#329274=CARTESIAN_POINT('Ctrl Pts',(0.742204082999944,5.2,-3.99415087100001));
#329275=CARTESIAN_POINT('Ctrl Pts',(0.742204082999944,2.2,-3.99415087100001));
#329276=CARTESIAN_POINT('Ctrl Pts',(0.742204076999945,12.2,-3.99322899600001));
#329277=CARTESIAN_POINT('Ctrl Pts',(0.742204076999945,5.2,-3.99322899600001));
#329278=CARTESIAN_POINT('Ctrl Pts',(0.742204076999945,2.2,-3.99322899600001));
#329279=CARTESIAN_POINT('Ctrl Pts',(0.742202931999943,12.2,-3.99231274300002));
#329280=CARTESIAN_POINT('Ctrl Pts',(0.742202931999943,5.2,-3.99231274300002));
#329281=CARTESIAN_POINT('Ctrl Pts',(0.742202931999943,2.2,-3.99231274300002));
#329282=CARTESIAN_POINT('Ctrl Pts',(0.742200661999944,12.2,-3.99140212200002));
#329283=CARTESIAN_POINT('Ctrl Pts',(0.742200661999944,5.2,-3.99140212200002));
#329284=CARTESIAN_POINT('Ctrl Pts',(0.742200661999944,2.2,-3.99140212200002));
#329285=CARTESIAN_POINT('Ctrl Pts',(0.742197279999944,12.2,-3.99049714400002));
#329286=CARTESIAN_POINT('Ctrl Pts',(0.742197279999944,5.2,-3.99049714400002));
#329287=CARTESIAN_POINT('Ctrl Pts',(0.742197279999944,2.2,-3.99049714400002));
#329288=CARTESIAN_POINT('Ctrl Pts',(0.742192799999944,12.2,-3.98959782100002));
#329289=CARTESIAN_POINT('Ctrl Pts',(0.742192799999944,5.2,-3.98959782100002));
#329290=CARTESIAN_POINT('Ctrl Pts',(0.742192799999944,2.2,-3.98959782100002));
#329291=CARTESIAN_POINT('Ctrl Pts',(0.742187234999945,12.2,-3.98870416500001));
#329292=CARTESIAN_POINT('Ctrl Pts',(0.742187234999945,5.2,-3.98870416500001));
#329293=CARTESIAN_POINT('Ctrl Pts',(0.742187234999945,2.2,-3.98870416500001));
#329294=CARTESIAN_POINT('Ctrl Pts',(0.742180598999944,12.2,-3.98781618500001));
#329295=CARTESIAN_POINT('Ctrl Pts',(0.742180598999944,5.2,-3.98781618500001));
#329296=CARTESIAN_POINT('Ctrl Pts',(0.742180598999944,2.2,-3.98781618500001));
#329297=CARTESIAN_POINT('Ctrl Pts',(0.742172904999945,12.2,-3.98693389300002));
#329298=CARTESIAN_POINT('Ctrl Pts',(0.742172904999945,5.2,-3.98693389300002));
#329299=CARTESIAN_POINT('Ctrl Pts',(0.742172904999945,2.2,-3.98693389300002));
#329300=CARTESIAN_POINT('Ctrl Pts',(0.742164167999944,12.2,-3.98605730100002));
#329301=CARTESIAN_POINT('Ctrl Pts',(0.742164167999944,5.2,-3.98605730100002));
#329302=CARTESIAN_POINT('Ctrl Pts',(0.742164167999944,2.2,-3.98605730100002));
#329303=CARTESIAN_POINT('Ctrl Pts',(0.742154399999944,12.2,-3.98518641800001));
#329304=CARTESIAN_POINT('Ctrl Pts',(0.742154399999944,5.2,-3.98518641800001));
#329305=CARTESIAN_POINT('Ctrl Pts',(0.742154399999944,2.2,-3.98518641800001));
#329306=CARTESIAN_POINT('Ctrl Pts',(0.742143613999944,12.2,-3.98432125700001));
#329307=CARTESIAN_POINT('Ctrl Pts',(0.742143613999944,5.2,-3.98432125700001));
#329308=CARTESIAN_POINT('Ctrl Pts',(0.742143613999944,2.2,-3.98432125700001));
#329309=CARTESIAN_POINT('Ctrl Pts',(0.742131825999944,12.2,-3.98346182900001));
#329310=CARTESIAN_POINT('Ctrl Pts',(0.742131825999944,5.2,-3.98346182900001));
#329311=CARTESIAN_POINT('Ctrl Pts',(0.742131825999944,2.2,-3.98346182900001));
#329312=CARTESIAN_POINT('Ctrl Pts',(0.742119048999944,12.2,-3.98260814600001));
#329313=CARTESIAN_POINT('Ctrl Pts',(0.742119048999944,5.2,-3.98260814600001));
#329314=CARTESIAN_POINT('Ctrl Pts',(0.742119048999944,2.2,-3.98260814600001));
#329315=CARTESIAN_POINT('Ctrl Pts',(0.742105296999944,12.2,-3.98176021700001));
#329316=CARTESIAN_POINT('Ctrl Pts',(0.742105296999944,5.2,-3.98176021700001));
#329317=CARTESIAN_POINT('Ctrl Pts',(0.742105296999944,2.2,-3.98176021700001));
#329318=CARTESIAN_POINT('Ctrl Pts',(0.742090582999944,12.2,-3.98091805500002));
#329319=CARTESIAN_POINT('Ctrl Pts',(0.742090582999944,5.2,-3.98091805500002));
#329320=CARTESIAN_POINT('Ctrl Pts',(0.742090582999944,2.2,-3.98091805500002));
#329321=CARTESIAN_POINT('Ctrl Pts',(0.742074920999943,12.2,-3.98008167000001));
#329322=CARTESIAN_POINT('Ctrl Pts',(0.742074920999943,5.2,-3.98008167000001));
#329323=CARTESIAN_POINT('Ctrl Pts',(0.742074920999943,2.2,-3.98008167000001));
#329324=CARTESIAN_POINT('Ctrl Pts',(0.742058326999944,12.2,-3.97925107500001));
#329325=CARTESIAN_POINT('Ctrl Pts',(0.742058326999944,5.2,-3.97925107500001));
#329326=CARTESIAN_POINT('Ctrl Pts',(0.742058326999944,2.2,-3.97925107500001));
#329327=CARTESIAN_POINT('Ctrl Pts',(0.742040812999945,12.2,-3.97842628000001));
#329328=CARTESIAN_POINT('Ctrl Pts',(0.742040812999945,5.2,-3.97842628000001));
#329329=CARTESIAN_POINT('Ctrl Pts',(0.742040812999945,2.2,-3.97842628000001));
#329330=CARTESIAN_POINT('Ctrl Pts',(0.742022392999945,12.2,-3.97760729600002));
#329331=CARTESIAN_POINT('Ctrl Pts',(0.742022392999945,5.2,-3.97760729600002));
#329332=CARTESIAN_POINT('Ctrl Pts',(0.742022392999945,2.2,-3.97760729600002));
#329333=CARTESIAN_POINT('Ctrl Pts',(0.742003082999945,12.2,-3.97679413600001));
#329334=CARTESIAN_POINT('Ctrl Pts',(0.742003082999945,5.2,-3.97679413600001));
#329335=CARTESIAN_POINT('Ctrl Pts',(0.742003082999945,2.2,-3.97679413600001));
#329336=CARTESIAN_POINT('Ctrl Pts',(0.741982896999944,12.2,-3.97598680900002));
#329337=CARTESIAN_POINT('Ctrl Pts',(0.741982896999944,5.2,-3.97598680900002));
#329338=CARTESIAN_POINT('Ctrl Pts',(0.741982896999944,2.2,-3.97598680900002));
#329339=CARTESIAN_POINT('Ctrl Pts',(0.741961847999945,12.2,-3.97518532700001));
#329340=CARTESIAN_POINT('Ctrl Pts',(0.741961847999945,5.2,-3.97518532700001));
#329341=CARTESIAN_POINT('Ctrl Pts',(0.741961847999945,2.2,-3.97518532700001));
#329342=CARTESIAN_POINT('Ctrl Pts',(0.741939950999945,12.2,-3.97438970300001));
#329343=CARTESIAN_POINT('Ctrl Pts',(0.741939950999945,5.2,-3.97438970300001));
#329344=CARTESIAN_POINT('Ctrl Pts',(0.741939950999945,2.2,-3.97438970300001));
#329345=CARTESIAN_POINT('Ctrl Pts',(0.741917219999944,12.2,-3.97359994600002));
#329346=CARTESIAN_POINT('Ctrl Pts',(0.741917219999944,5.2,-3.97359994600002));
#329347=CARTESIAN_POINT('Ctrl Pts',(0.741917219999944,2.2,-3.97359994600002));
#329348=CARTESIAN_POINT('Ctrl Pts',(0.741893669999943,12.2,-3.97281606900002));
#329349=CARTESIAN_POINT('Ctrl Pts',(0.741893669999943,5.2,-3.97281606900002));
#329350=CARTESIAN_POINT('Ctrl Pts',(0.741893669999943,2.2,-3.97281606900002));
#329351=CARTESIAN_POINT('Ctrl Pts',(0.741869314999944,12.2,-3.97203808400001));
#329352=CARTESIAN_POINT('Ctrl Pts',(0.741869314999944,5.2,-3.97203808400001));
#329353=CARTESIAN_POINT('Ctrl Pts',(0.741869314999944,2.2,-3.97203808400001));
#329354=CARTESIAN_POINT('Ctrl Pts',(0.741844169999945,12.2,-3.97126600100002));
#329355=CARTESIAN_POINT('Ctrl Pts',(0.741844169999945,5.2,-3.97126600100002));
#329356=CARTESIAN_POINT('Ctrl Pts',(0.741844169999945,2.2,-3.97126600100002));
#329357=CARTESIAN_POINT('Ctrl Pts',(0.741818249999944,12.2,-3.97049983000001));
#329358=CARTESIAN_POINT('Ctrl Pts',(0.741818249999944,5.2,-3.97049983000001));
#329359=CARTESIAN_POINT('Ctrl Pts',(0.741818249999944,2.2,-3.97049983000001));
#329360=CARTESIAN_POINT('Ctrl Pts',(0.741791566999944,12.2,-3.96973958600002));
#329361=CARTESIAN_POINT('Ctrl Pts',(0.741791566999944,5.2,-3.96973958600002));
#329362=CARTESIAN_POINT('Ctrl Pts',(0.741791566999944,2.2,-3.96973958600002));
#329363=CARTESIAN_POINT('Ctrl Pts',(0.741764139999944,12.2,-3.96898527800001));
#329364=CARTESIAN_POINT('Ctrl Pts',(0.741764139999944,5.2,-3.96898527800001));
#329365=CARTESIAN_POINT('Ctrl Pts',(0.741764139999944,2.2,-3.96898527800001));
#329366=CARTESIAN_POINT('Ctrl Pts',(0.741735980999944,12.2,-3.96823691800002));
#329367=CARTESIAN_POINT('Ctrl Pts',(0.741735980999944,5.2,-3.96823691800002));
#329368=CARTESIAN_POINT('Ctrl Pts',(0.741735980999944,2.2,-3.96823691800002));
#329369=CARTESIAN_POINT('Ctrl Pts',(0.741707104999944,12.2,-3.96749451800002));
#329370=CARTESIAN_POINT('Ctrl Pts',(0.741707104999944,5.2,-3.96749451800002));
#329371=CARTESIAN_POINT('Ctrl Pts',(0.741707104999944,2.2,-3.96749451800002));
#329372=CARTESIAN_POINT('Ctrl Pts',(0.741677527999944,12.2,-3.96675808800001));
#329373=CARTESIAN_POINT('Ctrl Pts',(0.741677527999944,5.2,-3.96675808800001));
#329374=CARTESIAN_POINT('Ctrl Pts',(0.741677527999944,2.2,-3.96675808800001));
#329375=CARTESIAN_POINT('Ctrl Pts',(0.741647263999944,12.2,-3.96602764100002));
#329376=CARTESIAN_POINT('Ctrl Pts',(0.741647263999944,5.2,-3.96602764100002));
#329377=CARTESIAN_POINT('Ctrl Pts',(0.741647263999944,2.2,-3.96602764100002));
#329378=CARTESIAN_POINT('Ctrl Pts',(0.741616327999944,12.2,-3.96530318800002));
#329379=CARTESIAN_POINT('Ctrl Pts',(0.741616327999944,5.2,-3.96530318800002));
#329380=CARTESIAN_POINT('Ctrl Pts',(0.741616327999944,2.2,-3.96530318800002));
#329381=CARTESIAN_POINT('Ctrl Pts',(0.741584735999944,12.2,-3.96458474000001));
#329382=CARTESIAN_POINT('Ctrl Pts',(0.741584735999944,5.2,-3.96458474000001));
#329383=CARTESIAN_POINT('Ctrl Pts',(0.741584735999944,2.2,-3.96458474000001));
#329384=CARTESIAN_POINT('Ctrl Pts',(0.741552500999945,12.2,-3.96387230900002));
#329385=CARTESIAN_POINT('Ctrl Pts',(0.741552500999945,5.2,-3.96387230900002));
#329386=CARTESIAN_POINT('Ctrl Pts',(0.741552500999945,2.2,-3.96387230900002));
#329387=CARTESIAN_POINT('Ctrl Pts',(0.741519640999945,12.2,-3.96316590700001));
#329388=CARTESIAN_POINT('Ctrl Pts',(0.741519640999945,5.2,-3.96316590700001));
#329389=CARTESIAN_POINT('Ctrl Pts',(0.741519640999945,2.2,-3.96316590700001));
#329390=CARTESIAN_POINT('Ctrl Pts',(0.741486168999944,12.2,-3.96246554600001));
#329391=CARTESIAN_POINT('Ctrl Pts',(0.741486168999944,5.2,-3.96246554600001));
#329392=CARTESIAN_POINT('Ctrl Pts',(0.741486168999944,2.2,-3.96246554600001));
#329393=CARTESIAN_POINT('Ctrl Pts',(0.741452101999944,12.2,-3.96177123600001));
#329394=CARTESIAN_POINT('Ctrl Pts',(0.741452101999944,5.2,-3.96177123600001));
#329395=CARTESIAN_POINT('Ctrl Pts',(0.741452101999944,2.2,-3.96177123600001));
#329396=CARTESIAN_POINT('Ctrl Pts',(0.741417452999944,12.2,-3.96108298900002));
#329397=CARTESIAN_POINT('Ctrl Pts',(0.741417452999944,5.2,-3.96108298900002));
#329398=CARTESIAN_POINT('Ctrl Pts',(0.741417452999944,2.2,-3.96108298900002));
#329399=CARTESIAN_POINT('Ctrl Pts',(0.741382239999945,12.2,-3.96040081700002));
#329400=CARTESIAN_POINT('Ctrl Pts',(0.741382239999945,5.2,-3.96040081700002));
#329401=CARTESIAN_POINT('Ctrl Pts',(0.741382239999945,2.2,-3.96040081700002));
#329402=CARTESIAN_POINT('Ctrl Pts',(0.741346476999943,12.2,-3.95972473100001));
#329403=CARTESIAN_POINT('Ctrl Pts',(0.741346476999943,5.2,-3.95972473100001));
#329404=CARTESIAN_POINT('Ctrl Pts',(0.741346476999943,2.2,-3.95972473100001));
#329405=CARTESIAN_POINT('Ctrl Pts',(0.741310179999944,12.2,-3.95905474400001));
#329406=CARTESIAN_POINT('Ctrl Pts',(0.741310179999944,5.2,-3.95905474400001));
#329407=CARTESIAN_POINT('Ctrl Pts',(0.741310179999944,2.2,-3.95905474400001));
#329408=CARTESIAN_POINT('Ctrl Pts',(0.741273364999944,12.2,-3.95839086700001));
#329409=CARTESIAN_POINT('Ctrl Pts',(0.741273364999944,5.2,-3.95839086700001));
#329410=CARTESIAN_POINT('Ctrl Pts',(0.741273364999944,2.2,-3.95839086700001));
#329411=CARTESIAN_POINT('Ctrl Pts',(0.741236044999944,12.2,-3.95773311200001));
#329412=CARTESIAN_POINT('Ctrl Pts',(0.741236044999944,5.2,-3.95773311200001));
#329413=CARTESIAN_POINT('Ctrl Pts',(0.741236044999944,2.2,-3.95773311200001));
#329414=CARTESIAN_POINT('Ctrl Pts',(0.741198239999944,12.2,-3.95708148800002));
#329415=CARTESIAN_POINT('Ctrl Pts',(0.741198239999944,5.2,-3.95708148800002));
#329416=CARTESIAN_POINT('Ctrl Pts',(0.741198239999944,2.2,-3.95708148800002));
#329417=CARTESIAN_POINT('Ctrl Pts',(0.741159961999944,12.2,-3.95643601100002));
#329418=CARTESIAN_POINT('Ctrl Pts',(0.741159961999944,5.2,-3.95643601100002));
#329419=CARTESIAN_POINT('Ctrl Pts',(0.741159961999944,2.2,-3.95643601100002));
#329420=CARTESIAN_POINT('Ctrl Pts',(0.741121229999945,12.2,-3.95579668900002));
#329421=CARTESIAN_POINT('Ctrl Pts',(0.741121229999945,5.2,-3.95579668900002));
#329422=CARTESIAN_POINT('Ctrl Pts',(0.741121229999945,2.2,-3.95579668900002));
#329423=CARTESIAN_POINT('Ctrl Pts',(0.741082055999944,12.2,-3.95516353700001));
#329424=CARTESIAN_POINT('Ctrl Pts',(0.741082055999944,5.2,-3.95516353700001));
#329425=CARTESIAN_POINT('Ctrl Pts',(0.741082055999944,2.2,-3.95516353700001));
#329426=CARTESIAN_POINT('Ctrl Pts',(0.741042459999944,12.2,-3.95453656400001));
#329427=CARTESIAN_POINT('Ctrl Pts',(0.741042459999944,5.2,-3.95453656400001));
#329428=CARTESIAN_POINT('Ctrl Pts',(0.741042459999944,2.2,-3.95453656400001));
#329429=CARTESIAN_POINT('Ctrl Pts',(0.741002455999944,12.2,-3.95391578400002));
#329430=CARTESIAN_POINT('Ctrl Pts',(0.741002455999944,5.2,-3.95391578400002));
#329431=CARTESIAN_POINT('Ctrl Pts',(0.741002455999944,2.2,-3.95391578400002));
#329432=CARTESIAN_POINT('Ctrl Pts',(0.740962058999944,12.2,-3.95330120700002));
#329433=CARTESIAN_POINT('Ctrl Pts',(0.740962058999944,5.2,-3.95330120700002));
#329434=CARTESIAN_POINT('Ctrl Pts',(0.740962058999944,2.2,-3.95330120700002));
#329435=CARTESIAN_POINT('Ctrl Pts',(0.740921286999944,12.2,-3.95269284500001));
#329436=CARTESIAN_POINT('Ctrl Pts',(0.740921286999944,5.2,-3.95269284500001));
#329437=CARTESIAN_POINT('Ctrl Pts',(0.740921286999944,2.2,-3.95269284500001));
#329438=CARTESIAN_POINT('Ctrl Pts',(0.740880156999945,12.2,-3.95209071000002));
#329439=CARTESIAN_POINT('Ctrl Pts',(0.740880156999945,5.2,-3.95209071000002));
#329440=CARTESIAN_POINT('Ctrl Pts',(0.740880156999945,2.2,-3.95209071000002));
#329441=CARTESIAN_POINT('Ctrl Pts',(0.740838681999944,12.2,-3.95149481500002));
#329442=CARTESIAN_POINT('Ctrl Pts',(0.740838681999944,5.2,-3.95149481500002));
#329443=CARTESIAN_POINT('Ctrl Pts',(0.740838681999944,2.2,-3.95149481500002));
#329444=CARTESIAN_POINT('Ctrl Pts',(0.740796879999944,12.2,-3.95090517000002));
#329445=CARTESIAN_POINT('Ctrl Pts',(0.740796879999944,5.2,-3.95090517000002));
#329446=CARTESIAN_POINT('Ctrl Pts',(0.740796879999944,2.2,-3.95090517000002));
#329447=CARTESIAN_POINT('Ctrl Pts',(0.740754768999944,12.2,-3.95032178800002));
#329448=CARTESIAN_POINT('Ctrl Pts',(0.740754768999944,5.2,-3.95032178800002));
#329449=CARTESIAN_POINT('Ctrl Pts',(0.740754768999944,2.2,-3.95032178800002));
#329450=CARTESIAN_POINT('Ctrl Pts',(0.740712361999945,12.2,-3.94974468100001));
#329451=CARTESIAN_POINT('Ctrl Pts',(0.740712361999945,5.2,-3.94974468100001));
#329452=CARTESIAN_POINT('Ctrl Pts',(0.740712361999945,2.2,-3.94974468100001));
#329453=CARTESIAN_POINT('Ctrl Pts',(0.740669678999945,12.2,-3.94917386000001));
#329454=CARTESIAN_POINT('Ctrl Pts',(0.740669678999945,5.2,-3.94917386000001));
#329455=CARTESIAN_POINT('Ctrl Pts',(0.740669678999945,2.2,-3.94917386000001));
#329456=CARTESIAN_POINT('Ctrl Pts',(0.740626733999944,12.2,-3.94860933800001));
#329457=CARTESIAN_POINT('Ctrl Pts',(0.740626733999944,5.2,-3.94860933800001));
#329458=CARTESIAN_POINT('Ctrl Pts',(0.740626733999944,2.2,-3.94860933800001));
#329459=CARTESIAN_POINT('Ctrl Pts',(0.740583544999944,12.2,-3.94805112600002));
#329460=CARTESIAN_POINT('Ctrl Pts',(0.740583544999944,5.2,-3.94805112600002));
#329461=CARTESIAN_POINT('Ctrl Pts',(0.740583544999944,2.2,-3.94805112600002));
#329462=CARTESIAN_POINT('Ctrl Pts',(0.740540128999945,12.2,-3.94749923600001));
#329463=CARTESIAN_POINT('Ctrl Pts',(0.740540128999945,5.2,-3.94749923600001));
#329464=CARTESIAN_POINT('Ctrl Pts',(0.740540128999945,2.2,-3.94749923600001));
#329465=CARTESIAN_POINT('Ctrl Pts',(0.740496500999944,12.2,-3.94695368100002));
#329466=CARTESIAN_POINT('Ctrl Pts',(0.740496500999944,5.2,-3.94695368100002));
#329467=CARTESIAN_POINT('Ctrl Pts',(0.740496500999944,2.2,-3.94695368100002));
#329468=CARTESIAN_POINT('Ctrl Pts',(0.740452678999944,12.2,-3.94641447100001));
#329469=CARTESIAN_POINT('Ctrl Pts',(0.740452678999944,5.2,-3.94641447100001));
#329470=CARTESIAN_POINT('Ctrl Pts',(0.740452678999944,2.2,-3.94641447100001));
#329471=CARTESIAN_POINT('Ctrl Pts',(0.740408679999944,12.2,-3.94588162100002));
#329472=CARTESIAN_POINT('Ctrl Pts',(0.740408679999944,5.2,-3.94588162100002));
#329473=CARTESIAN_POINT('Ctrl Pts',(0.740408679999944,2.2,-3.94588162100002));
#329474=CARTESIAN_POINT('Ctrl Pts',(0.740364520999944,12.2,-3.94535513900002));
#329475=CARTESIAN_POINT('Ctrl Pts',(0.740364520999944,5.2,-3.94535513900002));
#329476=CARTESIAN_POINT('Ctrl Pts',(0.740364520999944,2.2,-3.94535513900002));
#329477=CARTESIAN_POINT('Ctrl Pts',(0.740320218999945,12.2,-3.94483504100001));
#329478=CARTESIAN_POINT('Ctrl Pts',(0.740320218999945,5.2,-3.94483504100001));
#329479=CARTESIAN_POINT('Ctrl Pts',(0.740320218999945,2.2,-3.94483504100001));
#329480=CARTESIAN_POINT('Ctrl Pts',(0.740275790999945,12.2,-3.94432133700001));
#329481=CARTESIAN_POINT('Ctrl Pts',(0.740275790999945,5.2,-3.94432133700001));
#329482=CARTESIAN_POINT('Ctrl Pts',(0.740275790999945,2.2,-3.94432133700001));
#329483=CARTESIAN_POINT('Ctrl Pts',(0.740231253999944,12.2,-3.94381403900002));
#329484=CARTESIAN_POINT('Ctrl Pts',(0.740231253999944,5.2,-3.94381403900002));
#329485=CARTESIAN_POINT('Ctrl Pts',(0.740231253999944,2.2,-3.94381403900002));
#329486=CARTESIAN_POINT('Ctrl Pts',(0.740186624999944,12.2,-3.94331315900001));
#329487=CARTESIAN_POINT('Ctrl Pts',(0.740186624999944,5.2,-3.94331315900001));
#329488=CARTESIAN_POINT('Ctrl Pts',(0.740186624999944,2.2,-3.94331315900001));
#329489=CARTESIAN_POINT('Ctrl Pts',(0.740141921999945,12.2,-3.94281871000001));
#329490=CARTESIAN_POINT('Ctrl Pts',(0.740141921999945,5.2,-3.94281871000001));
#329491=CARTESIAN_POINT('Ctrl Pts',(0.740141921999945,2.2,-3.94281871000001));
#329492=CARTESIAN_POINT('Ctrl Pts',(0.740097160999944,12.2,-3.94233070300002));
#329493=CARTESIAN_POINT('Ctrl Pts',(0.740097160999944,5.2,-3.94233070300002));
#329494=CARTESIAN_POINT('Ctrl Pts',(0.740097160999944,2.2,-3.94233070300002));
#329495=CARTESIAN_POINT('Ctrl Pts',(0.740052360999944,12.2,-3.94184915200002));
#329496=CARTESIAN_POINT('Ctrl Pts',(0.740052360999944,5.2,-3.94184915200002));
#329497=CARTESIAN_POINT('Ctrl Pts',(0.740052360999944,2.2,-3.94184915200002));
#329498=CARTESIAN_POINT('Ctrl Pts',(0.740007537999944,12.2,-3.94137406700001));
#329499=CARTESIAN_POINT('Ctrl Pts',(0.740007537999944,5.2,-3.94137406700001));
#329500=CARTESIAN_POINT('Ctrl Pts',(0.740007537999944,2.2,-3.94137406700001));
#329501=CARTESIAN_POINT('Ctrl Pts',(0.739962711999944,12.2,-3.94090546000001));
#329502=CARTESIAN_POINT('Ctrl Pts',(0.739962711999944,5.2,-3.94090546000001));
#329503=CARTESIAN_POINT('Ctrl Pts',(0.739962711999944,2.2,-3.94090546000001));
#329504=CARTESIAN_POINT('Ctrl Pts',(0.739917897999944,12.2,-3.94044334500002));
#329505=CARTESIAN_POINT('Ctrl Pts',(0.739917897999944,5.2,-3.94044334500002));
#329506=CARTESIAN_POINT('Ctrl Pts',(0.739917897999944,2.2,-3.94044334500002));
#329507=CARTESIAN_POINT('Ctrl Pts',(0.739873114999944,12.2,-3.93998773400002));
#329508=CARTESIAN_POINT('Ctrl Pts',(0.739873114999944,5.2,-3.93998773400002));
#329509=CARTESIAN_POINT('Ctrl Pts',(0.739873114999944,2.2,-3.93998773400002));
#329510=CARTESIAN_POINT('Ctrl Pts',(0.739828380999944,12.2,-3.93953863800002));
#329511=CARTESIAN_POINT('Ctrl Pts',(0.739828380999944,5.2,-3.93953863800002));
#329512=CARTESIAN_POINT('Ctrl Pts',(0.739828380999944,2.2,-3.93953863800002));
#329513=CARTESIAN_POINT('Ctrl Pts',(0.739783712999944,12.2,-3.93909607000001));
#329514=CARTESIAN_POINT('Ctrl Pts',(0.739783712999944,5.2,-3.93909607000001));
#329515=CARTESIAN_POINT('Ctrl Pts',(0.739783712999944,2.2,-3.93909607000001));
#329516=CARTESIAN_POINT('Ctrl Pts',(0.739739128999944,12.2,-3.93866004200001));
#329517=CARTESIAN_POINT('Ctrl Pts',(0.739739128999944,5.2,-3.93866004200001));
#329518=CARTESIAN_POINT('Ctrl Pts',(0.739739128999944,2.2,-3.93866004200001));
#329519=CARTESIAN_POINT('Ctrl Pts',(0.739694648999943,12.2,-3.93823056700001));
#329520=CARTESIAN_POINT('Ctrl Pts',(0.739694648999943,5.2,-3.93823056700001));
#329521=CARTESIAN_POINT('Ctrl Pts',(0.739694648999943,2.2,-3.93823056700001));
#329522=CARTESIAN_POINT('Ctrl Pts',(0.739650287999944,12.2,-3.93780765600001));
#329523=CARTESIAN_POINT('Ctrl Pts',(0.739650287999944,5.2,-3.93780765600001));
#329524=CARTESIAN_POINT('Ctrl Pts',(0.739650287999944,2.2,-3.93780765600001));
#329525=CARTESIAN_POINT('Ctrl Pts',(0.739606065999945,12.2,-3.93739132200002));
#329526=CARTESIAN_POINT('Ctrl Pts',(0.739606065999945,5.2,-3.93739132200002));
#329527=CARTESIAN_POINT('Ctrl Pts',(0.739606065999945,2.2,-3.93739132200002));
#329528=CARTESIAN_POINT('Ctrl Pts',(0.739562000999944,12.2,-3.93698157800001));
#329529=CARTESIAN_POINT('Ctrl Pts',(0.739562000999944,5.2,-3.93698157800001));
#329530=CARTESIAN_POINT('Ctrl Pts',(0.739562000999944,2.2,-3.93698157800001));
#329531=CARTESIAN_POINT('Ctrl Pts',(0.739518110999944,12.2,-3.93657843600002));
#329532=CARTESIAN_POINT('Ctrl Pts',(0.739518110999944,5.2,-3.93657843600002));
#329533=CARTESIAN_POINT('Ctrl Pts',(0.739518110999944,2.2,-3.93657843600002));
#329534=CARTESIAN_POINT('Ctrl Pts',(0.739474413999944,12.2,-3.93618190600002));
#329535=CARTESIAN_POINT('Ctrl Pts',(0.739474413999944,5.2,-3.93618190600002));
#329536=CARTESIAN_POINT('Ctrl Pts',(0.739474413999944,2.2,-3.93618190600002));
#329537=CARTESIAN_POINT('Ctrl Pts',(0.739430928999945,12.2,-3.93579200400001));
#329538=CARTESIAN_POINT('Ctrl Pts',(0.739430928999945,5.2,-3.93579200400001));
#329539=CARTESIAN_POINT('Ctrl Pts',(0.739430928999945,2.2,-3.93579200400001));
#329540=CARTESIAN_POINT('Ctrl Pts',(0.739387674999944,12.2,-3.93540874100001));
#329541=CARTESIAN_POINT('Ctrl Pts',(0.739387674999944,5.2,-3.93540874100001));
#329542=CARTESIAN_POINT('Ctrl Pts',(0.739387674999944,2.2,-3.93540874100001));
#329543=CARTESIAN_POINT('Ctrl Pts',(0.739344668999945,12.2,-3.93503212900002));
#329544=CARTESIAN_POINT('Ctrl Pts',(0.739344668999945,5.2,-3.93503212900002));
#329545=CARTESIAN_POINT('Ctrl Pts',(0.739344668999945,2.2,-3.93503212900002));
#329546=CARTESIAN_POINT('Ctrl Pts',(0.739301930999944,12.2,-3.93466218000002));
#329547=CARTESIAN_POINT('Ctrl Pts',(0.739301930999944,5.2,-3.93466218000002));
#329548=CARTESIAN_POINT('Ctrl Pts',(0.739301930999944,2.2,-3.93466218000002));
#329549=CARTESIAN_POINT('Ctrl Pts',(0.739259478999944,12.2,-3.93429890800002));
#329550=CARTESIAN_POINT('Ctrl Pts',(0.739259478999944,5.2,-3.93429890800002));
#329551=CARTESIAN_POINT('Ctrl Pts',(0.739259478999944,2.2,-3.93429890800002));
#329552=CARTESIAN_POINT('Ctrl Pts',(0.739217332999944,12.2,-3.93394232400002));
#329553=CARTESIAN_POINT('Ctrl Pts',(0.739217332999944,5.2,-3.93394232400002));
#329554=CARTESIAN_POINT('Ctrl Pts',(0.739217332999944,2.2,-3.93394232400002));
#329555=CARTESIAN_POINT('Ctrl Pts',(0.739175509999944,12.2,-3.93359244200001));
#329556=CARTESIAN_POINT('Ctrl Pts',(0.739175509999944,5.2,-3.93359244200001));
#329557=CARTESIAN_POINT('Ctrl Pts',(0.739175509999944,2.2,-3.93359244200001));
#329558=CARTESIAN_POINT('Ctrl Pts',(0.739134030999944,12.2,-3.93324927300001));
#329559=CARTESIAN_POINT('Ctrl Pts',(0.739134030999944,5.2,-3.93324927300001));
#329560=CARTESIAN_POINT('Ctrl Pts',(0.739134030999944,2.2,-3.93324927300001));
#329561=CARTESIAN_POINT('Ctrl Pts',(0.739092914999944,12.2,-3.93291283000002));
#329562=CARTESIAN_POINT('Ctrl Pts',(0.739092914999944,5.2,-3.93291283000002));
#329563=CARTESIAN_POINT('Ctrl Pts',(0.739092914999944,2.2,-3.93291283000002));
#329564=CARTESIAN_POINT('Ctrl Pts',(0.739052177999944,12.2,-3.93258312600001));
#329565=CARTESIAN_POINT('Ctrl Pts',(0.739052177999944,5.2,-3.93258312600001));
#329566=CARTESIAN_POINT('Ctrl Pts',(0.739052177999944,2.2,-3.93258312600001));
#329567=CARTESIAN_POINT('Ctrl Pts',(0.739011842999945,12.2,-3.93226017400002));
#329568=CARTESIAN_POINT('Ctrl Pts',(0.739011842999945,5.2,-3.93226017400002));
#329569=CARTESIAN_POINT('Ctrl Pts',(0.739011842999945,2.2,-3.93226017400002));
#329570=CARTESIAN_POINT('Ctrl Pts',(0.738971926999944,12.2,-3.93194398500002));
#329571=CARTESIAN_POINT('Ctrl Pts',(0.738971926999944,5.2,-3.93194398500002));
#329572=CARTESIAN_POINT('Ctrl Pts',(0.738971926999944,2.2,-3.93194398500002));
#329573=CARTESIAN_POINT('Ctrl Pts',(0.738932449999944,12.2,-3.93163457300002));
#329574=CARTESIAN_POINT('Ctrl Pts',(0.738932449999944,5.2,-3.93163457300002));
#329575=CARTESIAN_POINT('Ctrl Pts',(0.738932449999944,2.2,-3.93163457300002));
#329576=CARTESIAN_POINT('Ctrl Pts',(0.738893430999944,12.2,-3.93133195000001));
#329577=CARTESIAN_POINT('Ctrl Pts',(0.738893430999944,5.2,-3.93133195000001));
#329578=CARTESIAN_POINT('Ctrl Pts',(0.738893430999944,2.2,-3.93133195000001));
#329579=CARTESIAN_POINT('Ctrl Pts',(0.738854890999944,12.2,-3.93103612900001));
#329580=CARTESIAN_POINT('Ctrl Pts',(0.738854890999944,5.2,-3.93103612900001));
#329581=CARTESIAN_POINT('Ctrl Pts',(0.738854890999944,2.2,-3.93103612900001));
#329582=CARTESIAN_POINT('Ctrl Pts',(0.738816847999945,12.2,-3.93074712400002));
#329583=CARTESIAN_POINT('Ctrl Pts',(0.738816847999945,5.2,-3.93074712400002));
#329584=CARTESIAN_POINT('Ctrl Pts',(0.738816847999945,2.2,-3.93074712400002));
#329585=CARTESIAN_POINT('Ctrl Pts',(0.738779321999944,12.2,-3.93046494500001));
#329586=CARTESIAN_POINT('Ctrl Pts',(0.738779321999944,5.2,-3.93046494500001));
#329587=CARTESIAN_POINT('Ctrl Pts',(0.738779321999944,2.2,-3.93046494500001));
#329588=CARTESIAN_POINT('Ctrl Pts',(0.738742333999944,12.2,-3.93018960500001));
#329589=CARTESIAN_POINT('Ctrl Pts',(0.738742333999944,5.2,-3.93018960500001));
#329590=CARTESIAN_POINT('Ctrl Pts',(0.738742333999944,2.2,-3.93018960500001));
#329591=CARTESIAN_POINT('Ctrl Pts',(0.738705901999944,12.2,-3.92992111900002));
#329592=CARTESIAN_POINT('Ctrl Pts',(0.738705901999944,5.2,-3.92992111900002));
#329593=CARTESIAN_POINT('Ctrl Pts',(0.738705901999944,2.2,-3.92992111900002));
#329594=CARTESIAN_POINT('Ctrl Pts',(0.738670047999944,12.2,-3.92965949900002));
#329595=CARTESIAN_POINT('Ctrl Pts',(0.738670047999944,5.2,-3.92965949900002));
#329596=CARTESIAN_POINT('Ctrl Pts',(0.738670047999944,2.2,-3.92965949900002));
#329597=CARTESIAN_POINT('Ctrl Pts',(0.738634788999945,12.2,-3.92940475700001));
#329598=CARTESIAN_POINT('Ctrl Pts',(0.738634788999945,5.2,-3.92940475700001));
#329599=CARTESIAN_POINT('Ctrl Pts',(0.738634788999945,2.2,-3.92940475700001));
#329600=CARTESIAN_POINT('Ctrl Pts',(0.738600147999944,12.2,-3.92915690600002));
#329601=CARTESIAN_POINT('Ctrl Pts',(0.738600147999944,5.2,-3.92915690600002));
#329602=CARTESIAN_POINT('Ctrl Pts',(0.738600147999944,2.2,-3.92915690600002));
#329603=CARTESIAN_POINT('Ctrl Pts',(0.738566144999945,12.2,-3.92891595800001));
#329604=CARTESIAN_POINT('Ctrl Pts',(0.738566144999945,5.2,-3.92891595800001));
#329605=CARTESIAN_POINT('Ctrl Pts',(0.738566144999945,2.2,-3.92891595800001));
#329606=CARTESIAN_POINT('Ctrl Pts',(0.738532797999943,12.2,-3.92868192900002));
#329607=CARTESIAN_POINT('Ctrl Pts',(0.738532797999943,5.2,-3.92868192900002));
#329608=CARTESIAN_POINT('Ctrl Pts',(0.738532797999943,2.2,-3.92868192900002));
#329609=CARTESIAN_POINT('Ctrl Pts',(0.738500128999945,12.2,-3.92845482900002));
#329610=CARTESIAN_POINT('Ctrl Pts',(0.738500128999945,5.2,-3.92845482900002));
#329611=CARTESIAN_POINT('Ctrl Pts',(0.738500128999945,2.2,-3.92845482900002));
#329612=CARTESIAN_POINT('Ctrl Pts',(0.738468156999944,12.2,-3.92823467100001));
#329613=CARTESIAN_POINT('Ctrl Pts',(0.738468156999944,5.2,-3.92823467100001));
#329614=CARTESIAN_POINT('Ctrl Pts',(0.738468156999944,2.2,-3.92823467100001));
#329615=CARTESIAN_POINT('Ctrl Pts',(0.738436904999944,12.2,-3.92802146900001));
#329616=CARTESIAN_POINT('Ctrl Pts',(0.738436904999944,5.2,-3.92802146900001));
#329617=CARTESIAN_POINT('Ctrl Pts',(0.738436904999944,2.2,-3.92802146900001));
#329618=CARTESIAN_POINT('Ctrl Pts',(0.738406391999944,12.2,-3.92781523500001));
#329619=CARTESIAN_POINT('Ctrl Pts',(0.738406391999944,5.2,-3.92781523500001));
#329620=CARTESIAN_POINT('Ctrl Pts',(0.738406391999944,2.2,-3.92781523500001));
#329621=CARTESIAN_POINT('Ctrl Pts',(0.738376637999945,12.2,-3.92761598300002));
#329622=CARTESIAN_POINT('Ctrl Pts',(0.738376637999945,5.2,-3.92761598300002));
#329623=CARTESIAN_POINT('Ctrl Pts',(0.738376637999945,2.2,-3.92761598300002));
#329624=CARTESIAN_POINT('Ctrl Pts',(0.738347665999944,12.2,-3.92742372600001));
#329625=CARTESIAN_POINT('Ctrl Pts',(0.738347665999944,5.2,-3.92742372600001));
#329626=CARTESIAN_POINT('Ctrl Pts',(0.738347665999944,2.2,-3.92742372600001));
#329627=CARTESIAN_POINT('Ctrl Pts',(0.738319495999944,12.2,-3.92723847700001));
#329628=CARTESIAN_POINT('Ctrl Pts',(0.738319495999944,5.2,-3.92723847700001));
#329629=CARTESIAN_POINT('Ctrl Pts',(0.738319495999944,2.2,-3.92723847700001));
#329630=CARTESIAN_POINT('Ctrl Pts',(0.738292148999945,12.2,-3.92706024900002));
#329631=CARTESIAN_POINT('Ctrl Pts',(0.738292148999945,5.2,-3.92706024900002));
#329632=CARTESIAN_POINT('Ctrl Pts',(0.738292148999945,2.2,-3.92706024900002));
#329633=CARTESIAN_POINT('Ctrl Pts',(0.738265644999945,12.2,-3.92688905300002));
#329634=CARTESIAN_POINT('Ctrl Pts',(0.738265644999945,5.2,-3.92688905300002));
#329635=CARTESIAN_POINT('Ctrl Pts',(0.738265644999945,2.2,-3.92688905300002));
#329636=CARTESIAN_POINT('Ctrl Pts',(0.738240003999944,12.2,-3.92672490400002));
#329637=CARTESIAN_POINT('Ctrl Pts',(0.738240003999944,5.2,-3.92672490400002));
#329638=CARTESIAN_POINT('Ctrl Pts',(0.738240003999944,2.2,-3.92672490400002));
#329639=CARTESIAN_POINT('Ctrl Pts',(0.738215248999944,12.2,-3.92656781500001));
#329640=CARTESIAN_POINT('Ctrl Pts',(0.738215248999944,5.2,-3.92656781500001));
#329641=CARTESIAN_POINT('Ctrl Pts',(0.738215248999944,2.2,-3.92656781500001));
#329642=CARTESIAN_POINT('Ctrl Pts',(0.738191399999945,12.2,-3.92641779800002));
#329643=CARTESIAN_POINT('Ctrl Pts',(0.738191399999945,5.2,-3.92641779800002));
#329644=CARTESIAN_POINT('Ctrl Pts',(0.738191399999945,2.2,-3.92641779800002));
#329645=CARTESIAN_POINT('Ctrl Pts',(0.738168480999944,12.2,-3.92627486800002));
#329646=CARTESIAN_POINT('Ctrl Pts',(0.738168480999944,5.2,-3.92627486800002));
#329647=CARTESIAN_POINT('Ctrl Pts',(0.738168480999944,2.2,-3.92627486800002));
#329648=CARTESIAN_POINT('Ctrl Pts',(0.738146512999944,12.2,-3.92613903800001));
#329649=CARTESIAN_POINT('Ctrl Pts',(0.738146512999944,5.2,-3.92613903800001));
#329650=CARTESIAN_POINT('Ctrl Pts',(0.738146512999944,2.2,-3.92613903800001));
#329651=CARTESIAN_POINT('Ctrl Pts',(0.738125519999944,12.2,-3.92601032300002));
#329652=CARTESIAN_POINT('Ctrl Pts',(0.738125519999944,5.2,-3.92601032300002));
#329653=CARTESIAN_POINT('Ctrl Pts',(0.738125519999944,2.2,-3.92601032300002));
#329654=CARTESIAN_POINT('Ctrl Pts',(0.738105520999944,12.2,-3.92588873400001));
#329655=CARTESIAN_POINT('Ctrl Pts',(0.738105520999944,5.2,-3.92588873400001));
#329656=CARTESIAN_POINT('Ctrl Pts',(0.738105520999944,2.2,-3.92588873400001));
#329657=CARTESIAN_POINT('Ctrl Pts',(0.738086536999945,12.2,-3.92577428400001));
#329658=CARTESIAN_POINT('Ctrl Pts',(0.738086536999945,5.2,-3.92577428400001));
#329659=CARTESIAN_POINT('Ctrl Pts',(0.738086536999945,2.2,-3.92577428400001));
#329660=CARTESIAN_POINT('Ctrl Pts',(0.738068587999944,12.2,-3.92566698400001));
#329661=CARTESIAN_POINT('Ctrl Pts',(0.738068587999944,5.2,-3.92566698400001));
#329662=CARTESIAN_POINT('Ctrl Pts',(0.738068587999944,2.2,-3.92566698400001));
#329663=CARTESIAN_POINT('Ctrl Pts',(0.738051691999945,12.2,-3.92556684800001));
#329664=CARTESIAN_POINT('Ctrl Pts',(0.738051691999945,5.2,-3.92556684800001));
#329665=CARTESIAN_POINT('Ctrl Pts',(0.738051691999945,2.2,-3.92556684800001));
#329666=CARTESIAN_POINT('Ctrl Pts',(0.738035872999945,12.2,-3.92547388800002));
#329667=CARTESIAN_POINT('Ctrl Pts',(0.738035872999945,5.2,-3.92547388800002));
#329668=CARTESIAN_POINT('Ctrl Pts',(0.738035872999945,2.2,-3.92547388800002));
#329669=CARTESIAN_POINT('Ctrl Pts',(0.738021155999945,12.2,-3.92538811900002));
#329670=CARTESIAN_POINT('Ctrl Pts',(0.738021155999945,5.2,-3.92538811900002));
#329671=CARTESIAN_POINT('Ctrl Pts',(0.738021155999945,2.2,-3.92538811900002));
#329672=CARTESIAN_POINT('Ctrl Pts',(0.738007569999944,12.2,-3.92530956000002));
#329673=CARTESIAN_POINT('Ctrl Pts',(0.738007569999944,5.2,-3.92530956000002));
#329674=CARTESIAN_POINT('Ctrl Pts',(0.738007569999944,2.2,-3.92530956000002));
#329675=CARTESIAN_POINT('Ctrl Pts',(0.737995141999944,12.2,-3.92523822500001));
#329676=CARTESIAN_POINT('Ctrl Pts',(0.737995141999944,5.2,-3.92523822500001));
#329677=CARTESIAN_POINT('Ctrl Pts',(0.737995141999944,2.2,-3.92523822500001));
#329678=CARTESIAN_POINT('Ctrl Pts',(0.737983896999944,12.2,-3.92517413200002));
#329679=CARTESIAN_POINT('Ctrl Pts',(0.737983896999944,5.2,-3.92517413200002));
#329680=CARTESIAN_POINT('Ctrl Pts',(0.737983896999944,2.2,-3.92517413200002));
#329681=CARTESIAN_POINT('Ctrl Pts',(0.737973852999944,12.2,-3.92511728900002));
#329682=CARTESIAN_POINT('Ctrl Pts',(0.737973852999944,5.2,-3.92511728900002));
#329683=CARTESIAN_POINT('Ctrl Pts',(0.737973852999944,2.2,-3.92511728900002));
#329684=CARTESIAN_POINT('Ctrl Pts',(0.737964075508447,12.2,-3.92506239688743));
#329685=CARTESIAN_POINT('Ctrl Pts',(0.737964075508447,5.2,-3.92506239688743));
#329686=CARTESIAN_POINT('Ctrl Pts',(0.737964075508447,2.2,-3.92506239688743));
#329687=CARTESIAN_POINT('Ctrl Pts',(0.737957318588985,12.2,-3.92502488824354));
#329688=CARTESIAN_POINT('Ctrl Pts',(0.737957318588985,5.2,-3.92502488824354));
#329689=CARTESIAN_POINT('Ctrl Pts',(0.737957318588985,2.2,-3.92502488824354));
#329690=CARTESIAN_POINT('Ctrl Pts',(0.737952809879958,12.2,-3.92500018886681));
#329691=CARTESIAN_POINT('Ctrl Pts',(0.737952809879958,5.2,-3.92500018886681));
#329692=CARTESIAN_POINT('Ctrl Pts',(0.737952809879958,2.2,-3.92500018886681));
#329693=CARTESIAN_POINT('Ctrl Pts',(0.737949974070314,12.2,-3.9249848052472));
#329694=CARTESIAN_POINT('Ctrl Pts',(0.737949974070314,5.2,-3.9249848052472));
#329695=CARTESIAN_POINT('Ctrl Pts',(0.737949974070314,2.2,-3.9249848052472));
#329696=CARTESIAN_POINT('Ctrl Pts',(0.737948220999944,12.2,-3.92497531000001));
#329697=CARTESIAN_POINT('Ctrl Pts',(0.737948220999944,5.2,-3.92497531000001));
#329698=CARTESIAN_POINT('Ctrl Pts',(0.737948220999944,2.2,-3.92497531000001));
#329699=CARTESIAN_POINT('',(0.737948419999944,2.7,-3.92497527300002));
#329700=CARTESIAN_POINT('',(0.737948419999944,12.2,-3.92497527300002));
#329701=CARTESIAN_POINT('Ctrl Pts',(0.540411127999944,2.7,-4.71915838000001));
#329702=CARTESIAN_POINT('Ctrl Pts',(0.665652104973256,2.7,-4.46512891742156));
#329703=CARTESIAN_POINT('Ctrl Pts',(0.707703770492112,2.70000000000005,
-4.27722825213315));
#329704=CARTESIAN_POINT('Ctrl Pts',(0.751313867273993,2.70000000000005,
-4.02314857199238));
#329705=CARTESIAN_POINT('Ctrl Pts',(0.740087973051188,2.70000000000455,
-3.93748559824036));
#329706=CARTESIAN_POINT('Ctrl Pts',(0.738030284168778,2.70000000000455,
-3.92544135994311));
#329707=CARTESIAN_POINT('Ctrl Pts',(0.737990568056458,2.7,-3.92520467658791));
#329708=CARTESIAN_POINT('Ctrl Pts',(0.737948220999944,2.7,-3.92497531000001));
#329709=CARTESIAN_POINT('Origin',(0.737938937999945,15.2,-3.92492484000002));
#329710=CARTESIAN_POINT('',(0.669813182999944,2.7,-3.56257986500002));
#329711=CARTESIAN_POINT('',(0.669813182999944,2.2,-3.56257986500002));
#329712=CARTESIAN_POINT('',(0.368969468486324,2.7,-1.96246242009659));
#329713=CARTESIAN_POINT('Origin',(-5.66300478732629E-14,2.7,-1.7702336056717E-14));
#329714=CARTESIAN_POINT('',(1.21174314999994,2.7,-3.41647530900001));
#329715=CARTESIAN_POINT('Origin',(-5.66300478732629E-14,2.7,-1.92943768261394E-14));
#329716=CARTESIAN_POINT('',(1.33499927399995,2.7,-3.76399243800002));
#329717=CARTESIAN_POINT('',(-5.68808302581349E-14,2.7,-1.85873030340881E-14));
#329718=CARTESIAN_POINT('',(1.90498031899994,2.7,-4.35126992700001));
#329719=CARTESIAN_POINT('Ctrl Pts',(1.33499940099994,2.7,-3.76399239200001));
#329720=CARTESIAN_POINT('Ctrl Pts',(1.33505318590947,2.7,-3.76414216657697));
#329721=CARTESIAN_POINT('Ctrl Pts',(1.33510842838262,2.70000000000379,-3.76429141658972));
#329722=CARTESIAN_POINT('Ctrl Pts',(1.3352798572439,2.70000000000379,-3.76475137816303));
#329723=CARTESIAN_POINT('Ctrl Pts',(1.33540406083887,2.70000000000408,-3.76507710840355));
#329724=CARTESIAN_POINT('Ctrl Pts',(1.33593626418945,2.70000000000408,-3.76645590419181));
#329725=CARTESIAN_POINT('Ctrl Pts',(1.3363951343922,2.70000000000408,-3.76759527567173));
#329726=CARTESIAN_POINT('Ctrl Pts',(1.33845293758698,2.70000000000408,-3.77258387700579));
#329727=CARTESIAN_POINT('Ctrl Pts',(1.34029389818348,2.70000000000408,-3.77670788059791));
#329728=CARTESIAN_POINT('Ctrl Pts',(1.34867811834044,2.70000000000408,-3.79469813505244));
#329729=CARTESIAN_POINT('Ctrl Pts',(1.35653894621658,2.70000000000408,-3.80937791673359));
#329730=CARTESIAN_POINT('Ctrl Pts',(1.38680573533928,2.70000000000408,-3.86188878113129));
#329731=CARTESIAN_POINT('Ctrl Pts',(1.41908990349611,2.7,-3.90970550382703));
#329732=CARTESIAN_POINT('Ctrl Pts',(1.55514657451191,2.7,-4.07573224600064));
#329733=CARTESIAN_POINT('Ctrl Pts',(1.69711667034069,2.7,-4.21327383678026));
#329734=CARTESIAN_POINT('Ctrl Pts',(1.90498031899994,2.7,-4.35126992800001));
#329735=CARTESIAN_POINT('',(2.20867500599994,2.7,-4.20526511800002));
#329736=CARTESIAN_POINT('Origin',(-5.66300478732629E-14,2.7,-1.92943768261394E-14));
#329737=CARTESIAN_POINT('',(2.10598101599994,2.7,-3.39335272700002));
#329738=CARTESIAN_POINT('Ctrl Pts',(2.20867500599994,2.7,-4.20526511900002));
#329739=CARTESIAN_POINT('Ctrl Pts',(2.23054550490679,2.7,-3.95864099641364));
#329740=CARTESIAN_POINT('Ctrl Pts',(2.21200258882908,2.7,-3.76641859286599));
#329741=CARTESIAN_POINT('Ctrl Pts',(2.15359897116276,2.7,-3.47945049981984));
#329742=CARTESIAN_POINT('Ctrl Pts',(2.11239855701061,2.7,-3.40405190689996));
#329743=CARTESIAN_POINT('Ctrl Pts',(2.10612617646059,2.7,-3.39359173223168));
#329744=CARTESIAN_POINT('Ctrl Pts',(2.10605412404705,2.7,-3.39347190592633));
#329745=CARTESIAN_POINT('Ctrl Pts',(2.10598084399995,2.7,-3.39335283300001));
#329746=CARTESIAN_POINT('',(1.91153447899994,2.7,-3.08004235900002));
#329747=CARTESIAN_POINT('',(1.05297697809741,2.7,-1.69665456162922));
#329748=CARTESIAN_POINT('',(2.36409006999994,2.7,-2.74803623300001));
#329749=CARTESIAN_POINT('Origin',(-5.66300478732629E-14,2.7,-1.92943768261394E-14));
#329750=CARTESIAN_POINT('',(2.60456064899994,2.7,-3.02756105800002));
#329751=CARTESIAN_POINT('',(-5.70235930926259E-14,2.7,-1.88369168773884E-14));
#329752=CARTESIAN_POINT('',(3.34820124399994,2.7,-3.36928010500001));
#329753=CARTESIAN_POINT('Ctrl Pts',(2.60456075099994,2.7,-3.02756096900001));
#329754=CARTESIAN_POINT('Ctrl Pts',(2.60466500709798,2.7,-3.02768120188421));
#329755=CARTESIAN_POINT('Ctrl Pts',(2.6047704354198,2.69999999999987,-3.02780041686978));
#329756=CARTESIAN_POINT('Ctrl Pts',(2.60509625096573,2.69999999999987,-3.02816717075809));
#329757=CARTESIAN_POINT('Ctrl Pts',(2.60532946277246,2.7,-3.02842574326169));
#329758=CARTESIAN_POINT('Ctrl Pts',(2.60632500711197,2.7,-3.02952050165491));
#329759=CARTESIAN_POINT('Ctrl Pts',(2.60716450668402,2.7,-3.03041715663214));
#329760=CARTESIAN_POINT('Ctrl Pts',(2.61088625784452,2.7,-3.03432639867292));
#329761=CARTESIAN_POINT('Ctrl Pts',(2.61409560992509,2.7,-3.03750956461736));
#329762=CARTESIAN_POINT('Ctrl Pts',(2.62840201211911,2.7,-3.05124616104321));
#329763=CARTESIAN_POINT('Ctrl Pts',(2.64103233645551,2.7,-3.0620938237245));
#329764=CARTESIAN_POINT('Ctrl Pts',(2.68823087033611,2.7,-3.10013029786383));
#329765=CARTESIAN_POINT('Ctrl Pts',(2.73560912439619,2.7,-3.13305665019956));
#329766=CARTESIAN_POINT('Ctrl Pts',(2.9319957262991,2.7,-3.24411877831512));
#329767=CARTESIAN_POINT('Ctrl Pts',(3.11606392248859,2.7,-3.3182297564467));
#329768=CARTESIAN_POINT('Ctrl Pts',(3.34820124399994,2.7,-3.36928010500001));
#329769=CARTESIAN_POINT('',(3.57864508499994,2.7,-3.12342750100001));
#329770=CARTESIAN_POINT('Origin',(-5.66300478732629E-14,2.7,-1.92943768261394E-14));
#329771=CARTESIAN_POINT('',(3.18958920499994,2.7,-2.40343909200002));
#329772=CARTESIAN_POINT('Ctrl Pts',(3.57864508499994,2.7,-3.12342750100001));
#329773=CARTESIAN_POINT('Ctrl Pts',(3.51005252440388,2.7,-2.88591939399924));
#329774=CARTESIAN_POINT('Ctrl Pts',(3.42511647090323,2.69999999999088,-2.71873794461971));
#329775=CARTESIAN_POINT('Ctrl Pts',(3.27332372189986,2.69999999999088,-2.4763086239477));
#329776=CARTESIAN_POINT('Ctrl Pts',(3.20549137962071,2.69999999999088,-2.41612390951146));
#329777=CARTESIAN_POINT('Ctrl Pts',(3.19023885271594,2.69999999999088,-2.40394068962246));
#329778=CARTESIAN_POINT('Ctrl Pts',(3.18967095409694,2.7,-2.40350137821559));
#329779=CARTESIAN_POINT('Ctrl Pts',(3.18958908308186,2.7,-2.40343925206217));
#329780=CARTESIAN_POINT('',(2.89509244999994,2.7,-2.18152806500001));
#329781=CARTESIAN_POINT('',(1.59477411092506,2.7,-1.20170410393585));
#329782=CARTESIAN_POINT('',(3.19715352599995,2.7,-1.70845963700002));
#329783=CARTESIAN_POINT('Origin',(-5.66300478732629E-14,2.7,-1.92943768261394E-14));
#329784=CARTESIAN_POINT('',(3.52236167599994,2.7,-1.88224078000002));
#329785=CARTESIAN_POINT('',(-5.69609323413902E-14,2.7,-1.91175624338592E-14));
#329786=CARTESIAN_POINT('',(4.33922903699994,2.7,-1.93225033600002));
#329787=CARTESIAN_POINT('Ctrl Pts',(3.52236173899994,2.7,-1.88224066100001));
#329788=CARTESIAN_POINT('Ctrl Pts',(3.52250239789438,2.7,-1.88231509464184));
#329789=CARTESIAN_POINT('Ctrl Pts',(3.52264376260884,2.69999999999987,-1.88238819257901));
#329790=CARTESIAN_POINT('Ctrl Pts',(3.52307936983357,2.69999999999987,-1.88261212568366));
#329791=CARTESIAN_POINT('Ctrl Pts',(3.52338953221521,2.7,-1.88276864836628));
#329792=CARTESIAN_POINT('Ctrl Pts',(3.524715395624,2.7,-1.88343088035005));
#329793=CARTESIAN_POINT('Ctrl Pts',(3.52582171235091,2.7,-1.88396352252172));
#329794=CARTESIAN_POINT('Ctrl Pts',(3.53070391512716,2.7,-1.88626411944967));
#329795=CARTESIAN_POINT('Ctrl Pts',(3.53484594800583,2.7,-1.88807280192899));
#329796=CARTESIAN_POINT('Ctrl Pts',(3.55314920490717,2.7,-1.89571400990757));
#329797=CARTESIAN_POINT('Ctrl Pts',(3.56885036242802,2.7,-1.90126819174153));
#329798=CARTESIAN_POINT('Ctrl Pts',(3.62652324888264,2.7,-1.91966091085629));
#329799=CARTESIAN_POINT('Ctrl Pts',(3.68259524212757,2.7,-1.93326135998433));
#329800=CARTESIAN_POINT('Ctrl Pts',(3.88845402391619,2.7,-1.96334031610243));
#329801=CARTESIAN_POINT('Ctrl Pts',(4.0855706716694,2.7,-1.97139908700959));
#329802=CARTESIAN_POINT('Ctrl Pts',(4.33922903699994,2.7,-1.93225033600001));
#329803=CARTESIAN_POINT('',(4.46529931499995,2.7,-1.61975369200002));
#329804=CARTESIAN_POINT('Origin',(-5.66300478732629E-14,2.7,-1.92943768261394E-14));
#329805=CARTESIAN_POINT('',(3.84242569899994,2.7,-1.08892768900002));
#329806=CARTESIAN_POINT('Ctrl Pts',(4.46529931499995,2.7,-1.61975369200002));
#329807=CARTESIAN_POINT('Ctrl Pts',(4.29358758119907,2.7,-1.39422941109806));
#329808=CARTESIAN_POINT('Ctrl Pts',(4.14405887002337,2.69999999999094,-1.27286083842864));
#329809=CARTESIAN_POINT('Ctrl Pts',(3.93634800541175,2.69999999999094,-1.12078426790825));
#329810=CARTESIAN_POINT('Ctrl Pts',(3.85463885449721,2.69999999999544,-1.09260715575166));
#329811=CARTESIAN_POINT('Ctrl Pts',(3.84274996213715,2.69999999999544,-1.08902313452261));
#329812=CARTESIAN_POINT('Ctrl Pts',(3.84258808458359,2.7,-1.08897453261456));
#329813=CARTESIAN_POINT('Ctrl Pts',(3.84242564299994,2.7,-1.08892788300002));
#329814=CARTESIAN_POINT('',(3.48765214499994,2.7,-0.988386318000014));
#329815=CARTESIAN_POINT('',(1.92118816307637,2.7,-0.544456849994655));
#329816=CARTESIAN_POINT('',(3.59842368199994,2.7,-0.438146099000015));
#329817=CARTESIAN_POINT('Origin',(-5.66300478732629E-14,2.7,-1.92943768261394E-14));
#329818=CARTESIAN_POINT('',(3.96444824099994,2.7,-0.482713455000018));
#329819=CARTESIAN_POINT('',(-5.67255557987442E-14,2.7,-1.92827477272514E-14));
#329820=CARTESIAN_POINT('',(4.74421990499994,2.7,-0.234259451000015));
#329821=CARTESIAN_POINT('Ctrl Pts',(3.96444825599994,2.7,-0.482713322000015));
#329822=CARTESIAN_POINT('Ctrl Pts',(3.96497547528596,2.7,-0.482775452743841));
#329823=CARTESIAN_POINT('Ctrl Pts',(3.96655962681762,2.70000000000098,-0.482946807487822));
#329824=CARTESIAN_POINT('Ctrl Pts',(3.9736780106965,2.70000000000098,-0.483451374626115));
#329825=CARTESIAN_POINT('Ctrl Pts',(3.97819360075364,2.7,-0.483641747904727));
#329826=CARTESIAN_POINT('Ctrl Pts',(3.99802246284191,2.7,-0.484155087954969));
#329827=CARTESIAN_POINT('Ctrl Pts',(4.01466717880949,2.7,-0.483662565437282));
#329828=CARTESIAN_POINT('Ctrl Pts',(4.07519067554633,2.7,-0.479973318483465));
#329829=CARTESIAN_POINT('Ctrl Pts',(4.13240045706223,2.7,-0.472381001980205));
#329830=CARTESIAN_POINT('Ctrl Pts',(4.32840548403216,2.7,-0.427621068241287));
#329831=CARTESIAN_POINT('Ctrl Pts',(4.51557914880521,2.7,-0.365999725911413));
#329832=CARTESIAN_POINT('Ctrl Pts',(4.74421990499994,2.7,-0.234259451000014));
#329833=CARTESIAN_POINT('',(4.74889012999994,2.7,0.102676828999985));
#329834=CARTESIAN_POINT('Origin',(-5.66300478732629E-14,2.7,-1.92943768261394E-14));
#329835=CARTESIAN_POINT('',(3.97632130999995,2.7,0.372649431999984));
#329836=CARTESIAN_POINT('Ctrl Pts',(4.74889012999994,2.7,0.102676827999986));
#329837=CARTESIAN_POINT('Ctrl Pts',(4.53436175012147,2.7,0.234337488975898));
#329838=CARTESIAN_POINT('Ctrl Pts',(4.35470102702024,2.70000000000136,0.301734470466299));
#329839=CARTESIAN_POINT('Ctrl Pts',(4.07614478832924,2.70000000000136,0.376824070144407));
#329840=CARTESIAN_POINT('Ctrl Pts',(3.9893662305862,2.70000000000136,0.373641676368157));
#329841=CARTESIAN_POINT('Ctrl Pts',(3.97670805493192,2.70000000000136,0.372681581585382));
#329842=CARTESIAN_POINT('Ctrl Pts',(3.9765145886927,2.7,0.37266656994227));
#329843=CARTESIAN_POINT('Ctrl Pts',(3.97632132799994,2.7,0.372649231999986));
#329844=CARTESIAN_POINT('',(3.60918509199994,2.7,0.338242477999984));
#329845=CARTESIAN_POINT('',(1.98813510850398,2.7,0.186322321956948));
#329846=CARTESIAN_POINT('',(3.51370677999994,2.7,0.891341496999986));
#329847=CARTESIAN_POINT('Origin',(-5.66300478732629E-14,2.7,-1.92943768261394E-14));
#329848=CARTESIAN_POINT('',(3.87111410199994,2.7,0.982006995999985));
#329849=CARTESIAN_POINT('',(-5.64403258229752E-14,2.7,-1.9246248980943E-14));
#329850=CARTESIAN_POINT('',(4.50847758599994,2.7,1.49536946999998));
#329851=CARTESIAN_POINT('Ctrl Pts',(3.87111406899994,2.7,0.982007125999989));
#329852=CARTESIAN_POINT('Ctrl Pts',(3.87126816493785,2.7,0.982046870939275));
#329853=CARTESIAN_POINT('Ctrl Pts',(3.87142187737795,2.69999999999987,0.982088098741952));
#329854=CARTESIAN_POINT('Ctrl Pts',(3.87189501533044,2.69999999999987,0.982216169587049));
#329855=CARTESIAN_POINT('Ctrl Pts',(3.87223055398195,2.7,0.982309707816934));
#329856=CARTESIAN_POINT('Ctrl Pts',(3.87365399687205,2.7,0.982712826320259));
#329857=CARTESIAN_POINT('Ctrl Pts',(3.87483183053987,2.7,0.983064923222153));
#329858=CARTESIAN_POINT('Ctrl Pts',(3.87998483279679,2.7,0.984652376245422));
#329859=CARTESIAN_POINT('Ctrl Pts',(3.88426244359151,2.69999999986206,0.986105300970037));
#329860=CARTESIAN_POINT('Ctrl Pts',(3.90294453748838,2.69999999986206,0.992792044582336));
#329861=CARTESIAN_POINT('Ctrl Pts',(3.91828518273234,2.69999999986206,0.999263364476566));
#329862=CARTESIAN_POINT('Ctrl Pts',(3.97345252689468,2.69999999986206,1.02459627187225));
#329863=CARTESIAN_POINT('Ctrl Pts',(4.02405430856334,2.69999999986206,1.05235489225042));
#329864=CARTESIAN_POINT('Ctrl Pts',(4.19593946187621,2.69999999986206,1.16846769640984));
#329865=CARTESIAN_POINT('Ctrl Pts',(4.34710585219733,2.7,1.2951894823555));
#329866=CARTESIAN_POINT('Ctrl Pts',(4.50847758551134,2.7,1.49536947039387));
#329867=CARTESIAN_POINT('',(4.39111701799995,2.7,1.81124027399999));
#329868=CARTESIAN_POINT('Origin',(-5.66300478732629E-14,2.7,-1.92943768261394E-14));
#329869=CARTESIAN_POINT('',(3.57319269599994,2.7,1.78389818299998));
#329870=CARTESIAN_POINT('Ctrl Pts',(4.39111701799995,2.7,1.81124027399999));
#329871=CARTESIAN_POINT('Ctrl Pts',(4.16446456139502,2.7,1.85268289602666));
#329872=CARTESIAN_POINT('Ctrl Pts',(3.98092498875472,2.6999999999957,1.85499572109631));
#329873=CARTESIAN_POINT('Ctrl Pts',(3.68606585001811,2.6999999999957,1.82867373173923));
#329874=CARTESIAN_POINT('Ctrl Pts',(3.59791443406951,2.6999999999957,1.79511456173619));
#329875=CARTESIAN_POINT('Ctrl Pts',(3.57422435482557,2.6999999999957,1.78440390906306));
#329876=CARTESIAN_POINT('Ctrl Pts',(3.5733518983807,2.7,1.78397669582644));
#329877=CARTESIAN_POINT('Ctrl Pts',(3.57320811899994,2.7,1.78390558399999));
#329878=CARTESIAN_POINT('',(3.24327759199994,2.7,1.61918975399999));
#329879=CARTESIAN_POINT('',(1.78657339171225,2.7,0.89193763007472));
#329880=CARTESIAN_POINT('',(2.95444430699995,2.7,2.10044848399999));
#329881=CARTESIAN_POINT('Origin',(-5.66300478732629E-14,2.7,-1.92943768261394E-14));
#329882=CARTESIAN_POINT('',(3.25496455399994,2.7,2.31410196199999));
#329883=CARTESIAN_POINT('',(-5.62541273730178E-14,2.7,-1.90271178888999E-14));
#329884=CARTESIAN_POINT('',(3.66384038699994,2.7,3.02304045899999));
#329885=CARTESIAN_POINT('Ctrl Pts',(3.25496447599994,2.7,2.31410207099998));
#329886=CARTESIAN_POINT('Ctrl Pts',(3.25509380911664,2.7,2.31419479733641));
#329887=CARTESIAN_POINT('Ctrl Pts',(3.25522224824814,2.7,2.31428876886345));
#329888=CARTESIAN_POINT('Ctrl Pts',(3.25561768780298,2.7,2.31457948816326));
#329889=CARTESIAN_POINT('Ctrl Pts',(3.25589686040589,2.7,2.31478799213888));
#329890=CARTESIAN_POINT('Ctrl Pts',(3.25707841110901,2.7,2.31567798214903));
#329891=CARTESIAN_POINT('Ctrl Pts',(3.25804922226441,2.7,2.31643157262964));
#329892=CARTESIAN_POINT('Ctrl Pts',(3.26228208001726,2.7,2.31977431503512));
#329893=CARTESIAN_POINT('Ctrl Pts',(3.26574629644654,2.7,2.32267476697699));
#329894=CARTESIAN_POINT('Ctrl Pts',(3.28074968457772,2.7,2.3356573222311));
#329895=CARTESIAN_POINT('Ctrl Pts',(3.29271501724893,2.7,2.34723161070611));
#329896=CARTESIAN_POINT('Ctrl Pts',(3.33492074366084,2.7,2.3906951000267));
#329897=CARTESIAN_POINT('Ctrl Pts',(3.37207270647139,2.7,2.43481567022442));
#329898=CARTESIAN_POINT('Ctrl Pts',(3.50029625949204,2.7,2.61941870425912));
#329899=CARTESIAN_POINT('Ctrl Pts',(3.5912406264507,2.7,2.79551317498595));
#329900=CARTESIAN_POINT('Ctrl Pts',(3.66384038671035,2.7,3.02304045909239));
#329901=CARTESIAN_POINT('',(3.44029922199995,2.7,3.27518568399999));
#329902=CARTESIAN_POINT('Origin',(-5.66300478732629E-14,2.7,-1.92943768261394E-14));
#329903=CARTESIAN_POINT('',(2.68748460699994,2.7,2.95422159799998));
#329904=CARTESIAN_POINT('Ctrl Pts',(3.44029922199995,2.7,3.27518568399999));
#329905=CARTESIAN_POINT('Ctrl Pts',(3.21786882806739,2.7,3.23269647807893));
#329906=CARTESIAN_POINT('Ctrl Pts',(3.03797835476827,2.69999999991388,3.16794335198484));
#329907=CARTESIAN_POINT('Ctrl Pts',(2.76277297310063,2.69999999991388,3.02746870010843));
#329908=CARTESIAN_POINT('Ctrl Pts',(2.6988645801551,2.7,2.96618934843886));
#329909=CARTESIAN_POINT('Ctrl Pts',(2.68791813750504,2.7,2.95468644111427));
#329910=CARTESIAN_POINT('Ctrl Pts',(2.68769951805849,2.7,2.95445572616322));
#329911=CARTESIAN_POINT('Ctrl Pts',(2.68748475499994,2.7,2.95422146199999));
#329912=CARTESIAN_POINT('',(2.43934748299994,2.7,2.68145648099999));
#329913=CARTESIAN_POINT('',(1.34372503703575,2.7,1.47709181992227));
#329914=CARTESIAN_POINT('',(1.99616775999994,2.7,3.02587826499998));
#329915=CARTESIAN_POINT('Origin',(-5.66300478732629E-14,2.7,-1.92943768261394E-14));
#329916=CARTESIAN_POINT('',(2.19921400599994,2.7,3.33366463399998));
#329917=CARTESIAN_POINT('',(-5.62641527204106E-14,2.7,-1.87397369739548E-14));
#329918=CARTESIAN_POINT('',(2.32438124199994,2.7,4.14243308299999));
#329919=CARTESIAN_POINT('Ctrl Pts',(2.19921389299994,2.7,3.33366470799999));
#329920=CARTESIAN_POINT('Ctrl Pts',(2.19931588681345,2.7,3.33382057043879));
#329921=CARTESIAN_POINT('Ctrl Pts',(2.19945522257332,2.7,3.33403928857926));
#329922=CARTESIAN_POINT('Ctrl Pts',(2.19965044880653,2.7,3.33434572647333));
#329923=CARTESIAN_POINT('Ctrl Pts',(2.1998356694566,2.70000000003935,3.33464134712214));
#329924=CARTESIAN_POINT('Ctrl Pts',(2.20061503722166,2.70000000003935,3.33589661910806));
#329925=CARTESIAN_POINT('Ctrl Pts',(2.20124779639401,2.70000000003925,3.33694950778106));
#329926=CARTESIAN_POINT('Ctrl Pts',(2.2039889246851,2.70000000003925,3.34159838370012));
#329927=CARTESIAN_POINT('Ctrl Pts',(2.20617219748561,2.70000000003925,3.34555593602161));
#329928=CARTESIAN_POINT('Ctrl Pts',(2.21546987923668,2.70000000003925,3.36307652428032));
#329929=CARTESIAN_POINT('Ctrl Pts',(2.22244615778148,2.70000000004265,3.37819108197411));
#329930=CARTESIAN_POINT('Ctrl Pts',(2.24613361740207,2.70000000004265,3.43404298918454));
#329931=CARTESIAN_POINT('Ctrl Pts',(2.26483106300591,2.7,3.48862949035665));
#329932=CARTESIAN_POINT('Ctrl Pts',(2.31198289469397,2.7,3.68342718120813));
#329933=CARTESIAN_POINT('Ctrl Pts',(2.34044050484888,2.7,3.87831359748762));
#329934=CARTESIAN_POINT('Ctrl Pts',(2.32438124099994,2.7,4.14243308299999));
#329935=CARTESIAN_POINT('',(2.02484994999994,2.7,4.29679911999998));
#329936=CARTESIAN_POINT('Origin',(-5.66300478732629E-14,2.7,-1.92943768261394E-14));
#329937=CARTESIAN_POINT('',(1.43881682999994,2.7,3.72556101799999));
#329938=CARTESIAN_POINT('Ctrl Pts',(2.02484995099994,2.7,4.29679911999998));
#329939=CARTESIAN_POINT('Ctrl Pts',(1.8076091663063,2.7,4.16109889870302));
#329940=CARTESIAN_POINT('Ctrl Pts',(1.66719638754842,2.69999999999827,4.02884779679555));
#329941=CARTESIAN_POINT('Ctrl Pts',(1.47880267972745,2.69999999999827,3.81539272798213));
#329942=CARTESIAN_POINT('Ctrl Pts',(1.44348902206156,2.69999999999827,3.73713776031853));
#329943=CARTESIAN_POINT('Ctrl Pts',(1.43891818135105,2.69999999999827,3.72581613794803));
#329944=CARTESIAN_POINT('Ctrl Pts',(1.43886694677176,2.7,3.72568879689252));
#329945=CARTESIAN_POINT('Ctrl Pts',(1.43881701799994,2.7,3.72556094399998));
#329946=CARTESIAN_POINT('',(1.30596997799994,2.7,3.38157765299999));
#329947=CARTESIAN_POINT('',(0.719399171412685,2.7,1.86275657353368));
#329948=CARTESIAN_POINT('',(0.768297694999944,2.7,3.54264641999999));
#329949=CARTESIAN_POINT('Origin',(-5.66300478732629E-14,2.7,-1.92943768261394E-14));
#329950=CARTESIAN_POINT('',(0.846447418999944,2.7,3.90299742599998));
#329951=CARTESIAN_POINT('',(-5.6465168812309E-14,2.7,-1.85341139478339E-14));
#329952=CARTESIAN_POINT('',(0.671001528999944,2.7,4.70236716499999));
#329953=CARTESIAN_POINT('Ctrl Pts',(0.846447287999944,2.7,3.90299745399999));
#329954=CARTESIAN_POINT('Ctrl Pts',(0.846467846681651,2.7,3.90309401488272));
#329955=CARTESIAN_POINT('Ctrl Pts',(0.846597772797866,2.70000000003935,
3.90372626137044));
#329956=CARTESIAN_POINT('Ctrl Pts',(0.846948074033169,2.70000000003935,
3.9055875681682));
#329957=CARTESIAN_POINT('Ctrl Pts',(0.847157926835858,2.70000000003925,
3.90679934491583));
#329958=CARTESIAN_POINT('Ctrl Pts',(0.848033633711593,2.70000000003925,
3.91211870052104));
#329959=CARTESIAN_POINT('Ctrl Pts',(0.848639829978756,2.70000000003925,
3.91659698430345));
#329960=CARTESIAN_POINT('Ctrl Pts',(0.850980875269782,2.70000000003925,
3.9362963901345));
#329961=CARTESIAN_POINT('Ctrl Pts',(0.852026119632535,2.70000000004265,
3.95291500911878));
#329962=CARTESIAN_POINT('Ctrl Pts',(0.853935255767777,2.70000000004265,
4.01346555886468));
#329963=CARTESIAN_POINT('Ctrl Pts',(0.851665052634113,2.7,4.07111646661862));
#329964=CARTESIAN_POINT('Ctrl Pts',(0.823079825617721,2.7,4.28622758807126));
#329965=CARTESIAN_POINT('Ctrl Pts',(0.774023401236597,2.7,4.47792766603638));
#329966=CARTESIAN_POINT('Ctrl Pts',(0.671001528999944,2.7,4.70236716399998));
#329967=CARTESIAN_POINT('',(0.335933473999944,2.7,4.73810602499999));
#329968=CARTESIAN_POINT('Origin',(-5.66300478732629E-14,2.7,-1.92943768261394E-14));
#329969=CARTESIAN_POINT('',(-0.00417113200005593,2.7,3.99374277699999));
#329970=CARTESIAN_POINT('Ctrl Pts',(0.335933474999944,2.7,4.73810602399999));
#329971=CARTESIAN_POINT('Ctrl Pts',(0.191001992066463,2.7,4.54460111419137));
#329972=CARTESIAN_POINT('Ctrl Pts',(0.104334236466074,2.69999999999544,
4.37236491648483));
#329973=CARTESIAN_POINT('Ctrl Pts',(0.000727985133453244,2.69999999999544,
4.09269413395091));
#329974=CARTESIAN_POINT('Ctrl Pts',(-0.00397622061450719,2.69999999999544,
4.00638406225539));
#329975=CARTESIAN_POINT('Ctrl Pts',(-0.00416806805312489,2.69999999999544,
3.99408078084134));
#329976=CARTESIAN_POINT('Ctrl Pts',(-0.00417050122958008,2.7,3.9939117830049));
#329977=CARTESIAN_POINT('Ctrl Pts',(-0.00417093000005587,2.7,3.99374277699999));
#329978=CARTESIAN_POINT('',(-0.00378600900005525,2.7,3.62499802299999));
#329979=CARTESIAN_POINT('',(-0.00208553923349334,2.7,1.99684572999974));
#329980=CARTESIAN_POINT('',(-0.563335230000056,2.7,3.58096054499998));
#329981=CARTESIAN_POINT('Origin',(-5.66300478732629E-14,2.7,-1.92943768261394E-14));
#329982=CARTESIAN_POINT('',(-0.620636577000055,2.7,3.94520878799998));
#329983=CARTESIAN_POINT('',(-5.67522488325669E-14,2.7,-1.85175803632247E-14));
#329984=CARTESIAN_POINT('Ctrl Pts',(-0.620636713000057,2.7,3.94520876599999));
#329985=CARTESIAN_POINT('Ctrl Pts',(-0.62073983719734,2.7,3.94584843905133));
#329986=CARTESIAN_POINT('Ctrl Pts',(-0.621830449136101,2.70000000003925,
3.95215994345551));
#329987=CARTESIAN_POINT('Ctrl Pts',(-0.628437841084849,2.70000000003925,
3.97789527472828));
#329988=CARTESIAN_POINT('Ctrl Pts',(-0.633466261820168,2.70000000004265,
3.99376897413103));
#329989=CARTESIAN_POINT('Ctrl Pts',(-0.653589700676736,2.70000000004265,
4.05100641397367));
#329990=CARTESIAN_POINT('Ctrl Pts',(-0.676556548929634,2.7,4.10395776250158));
#329991=CARTESIAN_POINT('Ctrl Pts',(-0.759803833912682,2.7,4.25572319419894));
#329992=CARTESIAN_POINT('Ctrl Pts',(-0.863318865366222,2.7,4.42354419280542));
#329993=CARTESIAN_POINT('Ctrl Pts',(-1.07300065800006,2.7,4.62722050399999));
#329994=CARTESIAN_POINT('Origin',(-5.66300478732629E-14,15.2,-1.77635683940025E-14));
#329995=CARTESIAN_POINT('',(-0.620636577000055,12.2,3.94520878799998));
#329996=CARTESIAN_POINT('',(-0.563335230000056,12.2,3.58096054499998));
#329997=CARTESIAN_POINT('Ctrl Pts',(-0.620636713000057,12.2,3.94520876599999));
#329998=CARTESIAN_POINT('Ctrl Pts',(-0.620636713000057,5.2,3.94520876599999));
#329999=CARTESIAN_POINT('Ctrl Pts',(-0.620636713000057,2.2,3.94520876599999));
#330000=CARTESIAN_POINT('Ctrl Pts',(-0.620637801933522,12.2,3.94521552058728));
#330001=CARTESIAN_POINT('Ctrl Pts',(-0.620637801933522,5.2,3.94521552058728));
#330002=CARTESIAN_POINT('Ctrl Pts',(-0.620637801933522,2.2,3.94521552058728));
#330003=CARTESIAN_POINT('Ctrl Pts',(-0.620639908278723,12.2,3.94522858611743));
#330004=CARTESIAN_POINT('Ctrl Pts',(-0.620639908278723,5.2,3.94522858611743));
#330005=CARTESIAN_POINT('Ctrl Pts',(-0.620639908278723,2.2,3.94522858611743));
#330006=CARTESIAN_POINT('Ctrl Pts',(-0.620643037501306,12.2,3.94524796762661));
#330007=CARTESIAN_POINT('Ctrl Pts',(-0.620643037501306,5.2,3.94524796762661));
#330008=CARTESIAN_POINT('Ctrl Pts',(-0.620643037501306,2.2,3.94524796762661));
#330009=CARTESIAN_POINT('Ctrl Pts',(-0.620647175670436,12.2,3.94527360898568));
#330010=CARTESIAN_POINT('Ctrl Pts',(-0.620647175670436,5.2,3.94527360898568));
#330011=CARTESIAN_POINT('Ctrl Pts',(-0.620647175670436,2.2,3.94527360898568));
#330012=CARTESIAN_POINT('Ctrl Pts',(-0.620654584000055,12.2,3.94531833299999));
#330013=CARTESIAN_POINT('Ctrl Pts',(-0.620654584000055,5.2,3.94531833299999));
#330014=CARTESIAN_POINT('Ctrl Pts',(-0.620654584000055,2.2,3.94531833299999));
#330015=CARTESIAN_POINT('Ctrl Pts',(-0.620662887000056,12.2,3.94536800899999));
#330016=CARTESIAN_POINT('Ctrl Pts',(-0.620662887000056,5.2,3.94536800899999));
#330017=CARTESIAN_POINT('Ctrl Pts',(-0.620662887000056,2.2,3.94536800899999));
#330018=CARTESIAN_POINT('Ctrl Pts',(-0.620672482000056,12.2,3.94542492999998));
#330019=CARTESIAN_POINT('Ctrl Pts',(-0.620672482000056,5.2,3.94542492999998));
#330020=CARTESIAN_POINT('Ctrl Pts',(-0.620672482000056,2.2,3.94542492999998));
#330021=CARTESIAN_POINT('Ctrl Pts',(-0.620683376000055,12.2,3.94548908399998));
#330022=CARTESIAN_POINT('Ctrl Pts',(-0.620683376000055,5.2,3.94548908399998));
#330023=CARTESIAN_POINT('Ctrl Pts',(-0.620683376000055,2.2,3.94548908399998));
#330024=CARTESIAN_POINT('Ctrl Pts',(-0.620695582000056,12.2,3.94556045499999));
#330025=CARTESIAN_POINT('Ctrl Pts',(-0.620695582000056,5.2,3.94556045499999));
#330026=CARTESIAN_POINT('Ctrl Pts',(-0.620695582000056,2.2,3.94556045499999));
#330027=CARTESIAN_POINT('Ctrl Pts',(-0.620709120000056,12.2,3.94563902299998));
#330028=CARTESIAN_POINT('Ctrl Pts',(-0.620709120000056,5.2,3.94563902299998));
#330029=CARTESIAN_POINT('Ctrl Pts',(-0.620709120000056,2.2,3.94563902299998));
#330030=CARTESIAN_POINT('Ctrl Pts',(-0.620724009000057,12.2,3.94572476199999));
#330031=CARTESIAN_POINT('Ctrl Pts',(-0.620724009000057,5.2,3.94572476199999));
#330032=CARTESIAN_POINT('Ctrl Pts',(-0.620724009000057,2.2,3.94572476199999));
#330033=CARTESIAN_POINT('Ctrl Pts',(-0.620740272000055,12.2,3.94581764599998));
#330034=CARTESIAN_POINT('Ctrl Pts',(-0.620740272000055,5.2,3.94581764599998));
#330035=CARTESIAN_POINT('Ctrl Pts',(-0.620740272000055,2.2,3.94581764599998));
#330036=CARTESIAN_POINT('Ctrl Pts',(-0.620757926000056,12.2,3.94591765199999));
#330037=CARTESIAN_POINT('Ctrl Pts',(-0.620757926000056,5.2,3.94591765199999));
#330038=CARTESIAN_POINT('Ctrl Pts',(-0.620757926000056,2.2,3.94591765199999));
#330039=CARTESIAN_POINT('Ctrl Pts',(-0.620776988000056,12.2,3.94602475899998));
#330040=CARTESIAN_POINT('Ctrl Pts',(-0.620776988000056,5.2,3.94602475899998));
#330041=CARTESIAN_POINT('Ctrl Pts',(-0.620776988000056,2.2,3.94602475899998));
#330042=CARTESIAN_POINT('Ctrl Pts',(-0.620797473000056,12.2,3.94613894999999));
#330043=CARTESIAN_POINT('Ctrl Pts',(-0.620797473000056,5.2,3.94613894999999));
#330044=CARTESIAN_POINT('Ctrl Pts',(-0.620797473000056,2.2,3.94613894999999));
#330045=CARTESIAN_POINT('Ctrl Pts',(-0.620819395000056,12.2,3.94626020699998));
#330046=CARTESIAN_POINT('Ctrl Pts',(-0.620819395000056,5.2,3.94626020699998));
#330047=CARTESIAN_POINT('Ctrl Pts',(-0.620819395000056,2.2,3.94626020699998));
#330048=CARTESIAN_POINT('Ctrl Pts',(-0.620842770000056,12.2,3.94638851099998));
#330049=CARTESIAN_POINT('Ctrl Pts',(-0.620842770000056,5.2,3.94638851099998));
#330050=CARTESIAN_POINT('Ctrl Pts',(-0.620842770000056,2.2,3.94638851099998));
#330051=CARTESIAN_POINT('Ctrl Pts',(-0.620867612000057,12.2,3.94652384499998));
#330052=CARTESIAN_POINT('Ctrl Pts',(-0.620867612000057,5.2,3.94652384499998));
#330053=CARTESIAN_POINT('Ctrl Pts',(-0.620867612000057,2.2,3.94652384499998));
#330054=CARTESIAN_POINT('Ctrl Pts',(-0.620893937000057,12.2,3.94666618599998));
#330055=CARTESIAN_POINT('Ctrl Pts',(-0.620893937000057,5.2,3.94666618599998));
#330056=CARTESIAN_POINT('Ctrl Pts',(-0.620893937000057,2.2,3.94666618599998));
#330057=CARTESIAN_POINT('Ctrl Pts',(-0.620921763000055,12.2,3.94681551699998));
#330058=CARTESIAN_POINT('Ctrl Pts',(-0.620921763000055,5.2,3.94681551699998));
#330059=CARTESIAN_POINT('Ctrl Pts',(-0.620921763000055,2.2,3.94681551699998));
#330060=CARTESIAN_POINT('Ctrl Pts',(-0.620951105000056,12.2,3.94697181399999));
#330061=CARTESIAN_POINT('Ctrl Pts',(-0.620951105000056,5.2,3.94697181399999));
#330062=CARTESIAN_POINT('Ctrl Pts',(-0.620951105000056,2.2,3.94697181399999));
#330063=CARTESIAN_POINT('Ctrl Pts',(-0.620981981000056,12.2,3.94713505999999));
#330064=CARTESIAN_POINT('Ctrl Pts',(-0.620981981000056,5.2,3.94713505999999));
#330065=CARTESIAN_POINT('Ctrl Pts',(-0.620981981000056,2.2,3.94713505999999));
#330066=CARTESIAN_POINT('Ctrl Pts',(-0.621014405000055,12.2,3.94730523299998));
#330067=CARTESIAN_POINT('Ctrl Pts',(-0.621014405000055,5.2,3.94730523299998));
#330068=CARTESIAN_POINT('Ctrl Pts',(-0.621014405000055,2.2,3.94730523299998));
#330069=CARTESIAN_POINT('Ctrl Pts',(-0.621048393000055,12.2,3.94748231499998));
#330070=CARTESIAN_POINT('Ctrl Pts',(-0.621048393000055,5.2,3.94748231499998));
#330071=CARTESIAN_POINT('Ctrl Pts',(-0.621048393000055,2.2,3.94748231499998));
#330072=CARTESIAN_POINT('Ctrl Pts',(-0.621083959000056,12.2,3.94766628699998));
#330073=CARTESIAN_POINT('Ctrl Pts',(-0.621083959000056,5.2,3.94766628699998));
#330074=CARTESIAN_POINT('Ctrl Pts',(-0.621083959000056,2.2,3.94766628699998));
#330075=CARTESIAN_POINT('Ctrl Pts',(-0.621121120000057,12.2,3.94785713099999));
#330076=CARTESIAN_POINT('Ctrl Pts',(-0.621121120000057,5.2,3.94785713099999));
#330077=CARTESIAN_POINT('Ctrl Pts',(-0.621121120000057,2.2,3.94785713099999));
#330078=CARTESIAN_POINT('Ctrl Pts',(-0.621159890000056,12.2,3.94805482699999));
#330079=CARTESIAN_POINT('Ctrl Pts',(-0.621159890000056,5.2,3.94805482699999));
#330080=CARTESIAN_POINT('Ctrl Pts',(-0.621159890000056,2.2,3.94805482699999));
#330081=CARTESIAN_POINT('Ctrl Pts',(-0.621200283000055,12.2,3.94825935499998));
#330082=CARTESIAN_POINT('Ctrl Pts',(-0.621200283000055,5.2,3.94825935499998));
#330083=CARTESIAN_POINT('Ctrl Pts',(-0.621200283000055,2.2,3.94825935499998));
#330084=CARTESIAN_POINT('Ctrl Pts',(-0.621242317000057,12.2,3.94847069599999));
#330085=CARTESIAN_POINT('Ctrl Pts',(-0.621242317000057,5.2,3.94847069599999));
#330086=CARTESIAN_POINT('Ctrl Pts',(-0.621242317000057,2.2,3.94847069599999));
#330087=CARTESIAN_POINT('Ctrl Pts',(-0.621286006000057,12.2,3.94868882999998));
#330088=CARTESIAN_POINT('Ctrl Pts',(-0.621286006000057,5.2,3.94868882999998));
#330089=CARTESIAN_POINT('Ctrl Pts',(-0.621286006000057,2.2,3.94868882999998));
#330090=CARTESIAN_POINT('Ctrl Pts',(-0.621331365000056,12.2,3.94891373999998));
#330091=CARTESIAN_POINT('Ctrl Pts',(-0.621331365000056,5.2,3.94891373999998));
#330092=CARTESIAN_POINT('Ctrl Pts',(-0.621331365000056,2.2,3.94891373999998));
#330093=CARTESIAN_POINT('Ctrl Pts',(-0.621378409000056,12.2,3.94914540499999));
#330094=CARTESIAN_POINT('Ctrl Pts',(-0.621378409000056,5.2,3.94914540499999));
#330095=CARTESIAN_POINT('Ctrl Pts',(-0.621378409000056,2.2,3.94914540499999));
#330096=CARTESIAN_POINT('Ctrl Pts',(-0.621427152000056,12.2,3.94938380899998));
#330097=CARTESIAN_POINT('Ctrl Pts',(-0.621427152000056,5.2,3.94938380899998));
#330098=CARTESIAN_POINT('Ctrl Pts',(-0.621427152000056,2.2,3.94938380899998));
#330099=CARTESIAN_POINT('Ctrl Pts',(-0.621477610000056,12.2,3.94962892899999));
#330100=CARTESIAN_POINT('Ctrl Pts',(-0.621477610000056,5.2,3.94962892899999));
#330101=CARTESIAN_POINT('Ctrl Pts',(-0.621477610000056,2.2,3.94962892899999));
#330102=CARTESIAN_POINT('Ctrl Pts',(-0.621529797000056,12.2,3.94988074799999));
#330103=CARTESIAN_POINT('Ctrl Pts',(-0.621529797000056,5.2,3.94988074799999));
#330104=CARTESIAN_POINT('Ctrl Pts',(-0.621529797000056,2.2,3.94988074799999));
#330105=CARTESIAN_POINT('Ctrl Pts',(-0.621583728000056,12.2,3.95013924799999));
#330106=CARTESIAN_POINT('Ctrl Pts',(-0.621583728000056,5.2,3.95013924799999));
#330107=CARTESIAN_POINT('Ctrl Pts',(-0.621583728000056,2.2,3.95013924799999));
#330108=CARTESIAN_POINT('Ctrl Pts',(-0.621639416000056,12.2,3.95040441099999));
#330109=CARTESIAN_POINT('Ctrl Pts',(-0.621639416000056,5.2,3.95040441099999));
#330110=CARTESIAN_POINT('Ctrl Pts',(-0.621639416000056,2.2,3.95040441099999));
#330111=CARTESIAN_POINT('Ctrl Pts',(-0.621696878000056,12.2,3.95067621599999));
#330112=CARTESIAN_POINT('Ctrl Pts',(-0.621696878000056,5.2,3.95067621599999));
#330113=CARTESIAN_POINT('Ctrl Pts',(-0.621696878000056,2.2,3.95067621599999));
#330114=CARTESIAN_POINT('Ctrl Pts',(-0.621756127000056,12.2,3.95095464499998));
#330115=CARTESIAN_POINT('Ctrl Pts',(-0.621756127000056,5.2,3.95095464499998));
#330116=CARTESIAN_POINT('Ctrl Pts',(-0.621756127000056,2.2,3.95095464499998));
#330117=CARTESIAN_POINT('Ctrl Pts',(-0.621817178000056,12.2,3.95123967899998));
#330118=CARTESIAN_POINT('Ctrl Pts',(-0.621817178000056,5.2,3.95123967899998));
#330119=CARTESIAN_POINT('Ctrl Pts',(-0.621817178000056,2.2,3.95123967899998));
#330120=CARTESIAN_POINT('Ctrl Pts',(-0.621880043000056,12.2,3.95153129999999));
#330121=CARTESIAN_POINT('Ctrl Pts',(-0.621880043000056,5.2,3.95153129999999));
#330122=CARTESIAN_POINT('Ctrl Pts',(-0.621880043000056,2.2,3.95153129999999));
#330123=CARTESIAN_POINT('Ctrl Pts',(-0.621944740000057,12.2,3.95182949099999));
#330124=CARTESIAN_POINT('Ctrl Pts',(-0.621944740000057,5.2,3.95182949099999));
#330125=CARTESIAN_POINT('Ctrl Pts',(-0.621944740000057,2.2,3.95182949099999));
#330126=CARTESIAN_POINT('Ctrl Pts',(-0.622011281000056,12.2,3.95213423099998));
#330127=CARTESIAN_POINT('Ctrl Pts',(-0.622011281000056,5.2,3.95213423099998));
#330128=CARTESIAN_POINT('Ctrl Pts',(-0.622011281000056,2.2,3.95213423099998));
#330129=CARTESIAN_POINT('Ctrl Pts',(-0.622079680000055,12.2,3.95244550299999));
#330130=CARTESIAN_POINT('Ctrl Pts',(-0.622079680000055,5.2,3.95244550299999));
#330131=CARTESIAN_POINT('Ctrl Pts',(-0.622079680000055,2.2,3.95244550299999));
#330132=CARTESIAN_POINT('Ctrl Pts',(-0.622149951000056,12.2,3.95276328699998));
#330133=CARTESIAN_POINT('Ctrl Pts',(-0.622149951000056,5.2,3.95276328699998));
#330134=CARTESIAN_POINT('Ctrl Pts',(-0.622149951000056,2.2,3.95276328699998));
#330135=CARTESIAN_POINT('Ctrl Pts',(-0.622222109000056,12.2,3.95308756699999));
#330136=CARTESIAN_POINT('Ctrl Pts',(-0.622222109000056,5.2,3.95308756699999));
#330137=CARTESIAN_POINT('Ctrl Pts',(-0.622222109000056,2.2,3.95308756699999));
#330138=CARTESIAN_POINT('Ctrl Pts',(-0.622296167000057,12.2,3.95341832299999));
#330139=CARTESIAN_POINT('Ctrl Pts',(-0.622296167000057,5.2,3.95341832299999));
#330140=CARTESIAN_POINT('Ctrl Pts',(-0.622296167000057,2.2,3.95341832299999));
#330141=CARTESIAN_POINT('Ctrl Pts',(-0.622372137000056,12.2,3.95375553799998));
#330142=CARTESIAN_POINT('Ctrl Pts',(-0.622372137000056,5.2,3.95375553799998));
#330143=CARTESIAN_POINT('Ctrl Pts',(-0.622372137000056,2.2,3.95375553799998));
#330144=CARTESIAN_POINT('Ctrl Pts',(-0.622450037000055,12.2,3.95409919299999));
#330145=CARTESIAN_POINT('Ctrl Pts',(-0.622450037000055,5.2,3.95409919299999));
#330146=CARTESIAN_POINT('Ctrl Pts',(-0.622450037000055,2.2,3.95409919299999));
#330147=CARTESIAN_POINT('Ctrl Pts',(-0.622529878000057,12.2,3.95444926999998));
#330148=CARTESIAN_POINT('Ctrl Pts',(-0.622529878000057,5.2,3.95444926999998));
#330149=CARTESIAN_POINT('Ctrl Pts',(-0.622529878000057,2.2,3.95444926999998));
#330150=CARTESIAN_POINT('Ctrl Pts',(-0.622611672000056,12.2,3.95480575099998));
#330151=CARTESIAN_POINT('Ctrl Pts',(-0.622611672000056,5.2,3.95480575099998));
#330152=CARTESIAN_POINT('Ctrl Pts',(-0.622611672000056,2.2,3.95480575099998));
#330153=CARTESIAN_POINT('Ctrl Pts',(-0.622695436000056,12.2,3.95516861799998));
#330154=CARTESIAN_POINT('Ctrl Pts',(-0.622695436000056,5.2,3.95516861799998));
#330155=CARTESIAN_POINT('Ctrl Pts',(-0.622695436000056,2.2,3.95516861799998));
#330156=CARTESIAN_POINT('Ctrl Pts',(-0.622781182000055,12.2,3.95553785199999));
#330157=CARTESIAN_POINT('Ctrl Pts',(-0.622781182000055,5.2,3.95553785199999));
#330158=CARTESIAN_POINT('Ctrl Pts',(-0.622781182000055,2.2,3.95553785199999));
#330159=CARTESIAN_POINT('Ctrl Pts',(-0.622868923000055,12.2,3.95591343599998));
#330160=CARTESIAN_POINT('Ctrl Pts',(-0.622868923000055,5.2,3.95591343599998));
#330161=CARTESIAN_POINT('Ctrl Pts',(-0.622868923000055,2.2,3.95591343599998));
#330162=CARTESIAN_POINT('Ctrl Pts',(-0.622958672000056,12.2,3.95629535099999));
#330163=CARTESIAN_POINT('Ctrl Pts',(-0.622958672000056,5.2,3.95629535099999));
#330164=CARTESIAN_POINT('Ctrl Pts',(-0.622958672000056,2.2,3.95629535099999));
#330165=CARTESIAN_POINT('Ctrl Pts',(-0.623050444000055,12.2,3.95668358099999));
#330166=CARTESIAN_POINT('Ctrl Pts',(-0.623050444000055,5.2,3.95668358099999));
#330167=CARTESIAN_POINT('Ctrl Pts',(-0.623050444000055,2.2,3.95668358099999));
#330168=CARTESIAN_POINT('Ctrl Pts',(-0.623144251000056,12.2,3.95707810699999));
#330169=CARTESIAN_POINT('Ctrl Pts',(-0.623144251000056,5.2,3.95707810699999));
#330170=CARTESIAN_POINT('Ctrl Pts',(-0.623144251000056,2.2,3.95707810699999));
#330171=CARTESIAN_POINT('Ctrl Pts',(-0.623240106000056,12.2,3.95747891199999));
#330172=CARTESIAN_POINT('Ctrl Pts',(-0.623240106000056,5.2,3.95747891199999));
#330173=CARTESIAN_POINT('Ctrl Pts',(-0.623240106000056,2.2,3.95747891199999));
#330174=CARTESIAN_POINT('Ctrl Pts',(-0.623338022000055,12.2,3.95788597599999));
#330175=CARTESIAN_POINT('Ctrl Pts',(-0.623338022000055,5.2,3.95788597599999));
#330176=CARTESIAN_POINT('Ctrl Pts',(-0.623338022000055,2.2,3.95788597599999));
#330177=CARTESIAN_POINT('Ctrl Pts',(-0.623438013000056,12.2,3.95829928399999));
#330178=CARTESIAN_POINT('Ctrl Pts',(-0.623438013000056,5.2,3.95829928399999));
#330179=CARTESIAN_POINT('Ctrl Pts',(-0.623438013000056,2.2,3.95829928399999));
#330180=CARTESIAN_POINT('Ctrl Pts',(-0.623540092000056,12.2,3.95871881699998));
#330181=CARTESIAN_POINT('Ctrl Pts',(-0.623540092000056,5.2,3.95871881699998));
#330182=CARTESIAN_POINT('Ctrl Pts',(-0.623540092000056,2.2,3.95871881699998));
#330183=CARTESIAN_POINT('Ctrl Pts',(-0.623644270000057,12.2,3.95914455699998));
#330184=CARTESIAN_POINT('Ctrl Pts',(-0.623644270000057,5.2,3.95914455699998));
#330185=CARTESIAN_POINT('Ctrl Pts',(-0.623644270000057,2.2,3.95914455699998));
#330186=CARTESIAN_POINT('Ctrl Pts',(-0.623750562000056,12.2,3.95957648599998));
#330187=CARTESIAN_POINT('Ctrl Pts',(-0.623750562000056,5.2,3.95957648599998));
#330188=CARTESIAN_POINT('Ctrl Pts',(-0.623750562000056,2.2,3.95957648599998));
#330189=CARTESIAN_POINT('Ctrl Pts',(-0.623858980000056,12.2,3.96001458899998));
#330190=CARTESIAN_POINT('Ctrl Pts',(-0.623858980000056,5.2,3.96001458899998));
#330191=CARTESIAN_POINT('Ctrl Pts',(-0.623858980000056,2.2,3.96001458899998));
#330192=CARTESIAN_POINT('Ctrl Pts',(-0.623969536000055,12.2,3.96045884699999));
#330193=CARTESIAN_POINT('Ctrl Pts',(-0.623969536000055,5.2,3.96045884699999));
#330194=CARTESIAN_POINT('Ctrl Pts',(-0.623969536000055,2.2,3.96045884699999));
#330195=CARTESIAN_POINT('Ctrl Pts',(-0.624082244000055,12.2,3.96090924099998));
#330196=CARTESIAN_POINT('Ctrl Pts',(-0.624082244000055,5.2,3.96090924099998));
#330197=CARTESIAN_POINT('Ctrl Pts',(-0.624082244000055,2.2,3.96090924099998));
#330198=CARTESIAN_POINT('Ctrl Pts',(-0.624197116000056,12.2,3.96136575499998));
#330199=CARTESIAN_POINT('Ctrl Pts',(-0.624197116000056,5.2,3.96136575499998));
#330200=CARTESIAN_POINT('Ctrl Pts',(-0.624197116000056,2.2,3.96136575499998));
#330201=CARTESIAN_POINT('Ctrl Pts',(-0.624314163000056,12.2,3.96182837299998));
#330202=CARTESIAN_POINT('Ctrl Pts',(-0.624314163000056,5.2,3.96182837299998));
#330203=CARTESIAN_POINT('Ctrl Pts',(-0.624314163000056,2.2,3.96182837299998));
#330204=CARTESIAN_POINT('Ctrl Pts',(-0.624433400000056,12.2,3.96229707499998));
#330205=CARTESIAN_POINT('Ctrl Pts',(-0.624433400000056,5.2,3.96229707499998));
#330206=CARTESIAN_POINT('Ctrl Pts',(-0.624433400000056,2.2,3.96229707499998));
#330207=CARTESIAN_POINT('Ctrl Pts',(-0.624554838000057,12.2,3.96277184599998));
#330208=CARTESIAN_POINT('Ctrl Pts',(-0.624554838000057,5.2,3.96277184599998));
#330209=CARTESIAN_POINT('Ctrl Pts',(-0.624554838000057,2.2,3.96277184599998));
#330210=CARTESIAN_POINT('Ctrl Pts',(-0.624678490000056,12.2,3.96325266599998));
#330211=CARTESIAN_POINT('Ctrl Pts',(-0.624678490000056,5.2,3.96325266599998));
#330212=CARTESIAN_POINT('Ctrl Pts',(-0.624678490000056,2.2,3.96325266599998));
#330213=CARTESIAN_POINT('Ctrl Pts',(-0.624804368000056,12.2,3.96373951999998));
#330214=CARTESIAN_POINT('Ctrl Pts',(-0.624804368000056,5.2,3.96373951999998));
#330215=CARTESIAN_POINT('Ctrl Pts',(-0.624804368000056,2.2,3.96373951999998));
#330216=CARTESIAN_POINT('Ctrl Pts',(-0.624932484000055,12.2,3.96423239099998));
#330217=CARTESIAN_POINT('Ctrl Pts',(-0.624932484000055,5.2,3.96423239099998));
#330218=CARTESIAN_POINT('Ctrl Pts',(-0.624932484000055,2.2,3.96423239099998));
#330219=CARTESIAN_POINT('Ctrl Pts',(-0.625062850000055,12.2,3.96473125899998));
#330220=CARTESIAN_POINT('Ctrl Pts',(-0.625062850000055,5.2,3.96473125899998));
#330221=CARTESIAN_POINT('Ctrl Pts',(-0.625062850000055,2.2,3.96473125899998));
#330222=CARTESIAN_POINT('Ctrl Pts',(-0.625195479000055,12.2,3.96523611099998));
#330223=CARTESIAN_POINT('Ctrl Pts',(-0.625195479000055,5.2,3.96523611099998));
#330224=CARTESIAN_POINT('Ctrl Pts',(-0.625195479000055,2.2,3.96523611099998));
#330225=CARTESIAN_POINT('Ctrl Pts',(-0.625330383000057,12.2,3.96574692699998));
#330226=CARTESIAN_POINT('Ctrl Pts',(-0.625330383000057,5.2,3.96574692699998));
#330227=CARTESIAN_POINT('Ctrl Pts',(-0.625330383000057,2.2,3.96574692699998));
#330228=CARTESIAN_POINT('Ctrl Pts',(-0.625467573000057,12.2,3.96626369099998));
#330229=CARTESIAN_POINT('Ctrl Pts',(-0.625467573000057,5.2,3.96626369099998));
#330230=CARTESIAN_POINT('Ctrl Pts',(-0.625467573000057,2.2,3.96626369099998));
#330231=CARTESIAN_POINT('Ctrl Pts',(-0.625607062000055,12.2,3.96678638599998));
#330232=CARTESIAN_POINT('Ctrl Pts',(-0.625607062000055,5.2,3.96678638599998));
#330233=CARTESIAN_POINT('Ctrl Pts',(-0.625607062000055,2.2,3.96678638599998));
#330234=CARTESIAN_POINT('Ctrl Pts',(-0.625748861000056,12.2,3.96731499499998));
#330235=CARTESIAN_POINT('Ctrl Pts',(-0.625748861000056,5.2,3.96731499499998));
#330236=CARTESIAN_POINT('Ctrl Pts',(-0.625748861000056,2.2,3.96731499499998));
#330237=CARTESIAN_POINT('Ctrl Pts',(-0.625892983000057,12.2,3.96784949999999));
#330238=CARTESIAN_POINT('Ctrl Pts',(-0.625892983000057,5.2,3.96784949999999));
#330239=CARTESIAN_POINT('Ctrl Pts',(-0.625892983000057,2.2,3.96784949999999));
#330240=CARTESIAN_POINT('Ctrl Pts',(-0.626039438000056,12.2,3.96838988599999));
#330241=CARTESIAN_POINT('Ctrl Pts',(-0.626039438000056,5.2,3.96838988599999));
#330242=CARTESIAN_POINT('Ctrl Pts',(-0.626039438000056,2.2,3.96838988599999));
#330243=CARTESIAN_POINT('Ctrl Pts',(-0.626188240000056,12.2,3.96893613399998));
#330244=CARTESIAN_POINT('Ctrl Pts',(-0.626188240000056,5.2,3.96893613399998));
#330245=CARTESIAN_POINT('Ctrl Pts',(-0.626188240000056,2.2,3.96893613399998));
#330246=CARTESIAN_POINT('Ctrl Pts',(-0.626339399000055,12.2,3.96948822899999));
#330247=CARTESIAN_POINT('Ctrl Pts',(-0.626339399000055,5.2,3.96948822899999));
#330248=CARTESIAN_POINT('Ctrl Pts',(-0.626339399000055,2.2,3.96948822899999));
#330249=CARTESIAN_POINT('Ctrl Pts',(-0.626492927000056,12.2,3.97004615499998));
#330250=CARTESIAN_POINT('Ctrl Pts',(-0.626492927000056,5.2,3.97004615499998));
#330251=CARTESIAN_POINT('Ctrl Pts',(-0.626492927000056,2.2,3.97004615499998));
#330252=CARTESIAN_POINT('Ctrl Pts',(-0.626648836000055,12.2,3.97060989199999));
#330253=CARTESIAN_POINT('Ctrl Pts',(-0.626648836000055,5.2,3.97060989199999));
#330254=CARTESIAN_POINT('Ctrl Pts',(-0.626648836000055,2.2,3.97060989199999));
#330255=CARTESIAN_POINT('Ctrl Pts',(-0.626807136000057,12.2,3.97117942599999));
#330256=CARTESIAN_POINT('Ctrl Pts',(-0.626807136000057,5.2,3.97117942599999));
#330257=CARTESIAN_POINT('Ctrl Pts',(-0.626807136000057,2.2,3.97117942599999));
#330258=CARTESIAN_POINT('Ctrl Pts',(-0.626967841000056,12.2,3.97175473999998));
#330259=CARTESIAN_POINT('Ctrl Pts',(-0.626967841000056,5.2,3.97175473999998));
#330260=CARTESIAN_POINT('Ctrl Pts',(-0.626967841000056,2.2,3.97175473999998));
#330261=CARTESIAN_POINT('Ctrl Pts',(-0.627130961000055,12.2,3.97233581699999));
#330262=CARTESIAN_POINT('Ctrl Pts',(-0.627130961000055,5.2,3.97233581699999));
#330263=CARTESIAN_POINT('Ctrl Pts',(-0.627130961000055,2.2,3.97233581699999));
#330264=CARTESIAN_POINT('Ctrl Pts',(-0.627296507000056,12.2,3.97292263899998));
#330265=CARTESIAN_POINT('Ctrl Pts',(-0.627296507000056,5.2,3.97292263899998));
#330266=CARTESIAN_POINT('Ctrl Pts',(-0.627296507000056,2.2,3.97292263899998));
#330267=CARTESIAN_POINT('Ctrl Pts',(-0.627464491000056,12.2,3.97351519199999));
#330268=CARTESIAN_POINT('Ctrl Pts',(-0.627464491000056,5.2,3.97351519199999));
#330269=CARTESIAN_POINT('Ctrl Pts',(-0.627464491000056,2.2,3.97351519199999));
#330270=CARTESIAN_POINT('Ctrl Pts',(-0.627634923000056,12.2,3.97411345799998));
#330271=CARTESIAN_POINT('Ctrl Pts',(-0.627634923000056,5.2,3.97411345799998));
#330272=CARTESIAN_POINT('Ctrl Pts',(-0.627634923000056,2.2,3.97411345799998));
#330273=CARTESIAN_POINT('Ctrl Pts',(-0.627807816000056,12.2,3.97471741999999));
#330274=CARTESIAN_POINT('Ctrl Pts',(-0.627807816000056,5.2,3.97471741999999));
#330275=CARTESIAN_POINT('Ctrl Pts',(-0.627807816000056,2.2,3.97471741999999));
#330276=CARTESIAN_POINT('Ctrl Pts',(-0.627983180000056,12.2,3.97532706299998));
#330277=CARTESIAN_POINT('Ctrl Pts',(-0.627983180000056,5.2,3.97532706299998));
#330278=CARTESIAN_POINT('Ctrl Pts',(-0.627983180000056,2.2,3.97532706299998));
#330279=CARTESIAN_POINT('Ctrl Pts',(-0.628161026000056,12.2,3.97594236899998));
#330280=CARTESIAN_POINT('Ctrl Pts',(-0.628161026000056,5.2,3.97594236899998));
#330281=CARTESIAN_POINT('Ctrl Pts',(-0.628161026000056,2.2,3.97594236899998));
#330282=CARTESIAN_POINT('Ctrl Pts',(-0.628341365000056,12.2,3.97656332399999));
#330283=CARTESIAN_POINT('Ctrl Pts',(-0.628341365000056,5.2,3.97656332399999));
#330284=CARTESIAN_POINT('Ctrl Pts',(-0.628341365000056,2.2,3.97656332399999));
#330285=CARTESIAN_POINT('Ctrl Pts',(-0.628524210000055,12.2,3.97718990899998));
#330286=CARTESIAN_POINT('Ctrl Pts',(-0.628524210000055,5.2,3.97718990899998));
#330287=CARTESIAN_POINT('Ctrl Pts',(-0.628524210000055,2.2,3.97718990899998));
#330288=CARTESIAN_POINT('Ctrl Pts',(-0.628709569000057,12.2,3.97782210999999));
#330289=CARTESIAN_POINT('Ctrl Pts',(-0.628709569000057,5.2,3.97782210999999));
#330290=CARTESIAN_POINT('Ctrl Pts',(-0.628709569000057,2.2,3.97782210999999));
#330291=CARTESIAN_POINT('Ctrl Pts',(-0.628897453000056,12.2,3.97845990899999));
#330292=CARTESIAN_POINT('Ctrl Pts',(-0.628897453000056,5.2,3.97845990899999));
#330293=CARTESIAN_POINT('Ctrl Pts',(-0.628897453000056,2.2,3.97845990899999));
#330294=CARTESIAN_POINT('Ctrl Pts',(-0.629087876000056,12.2,3.97910328999998));
#330295=CARTESIAN_POINT('Ctrl Pts',(-0.629087876000056,5.2,3.97910328999998));
#330296=CARTESIAN_POINT('Ctrl Pts',(-0.629087876000056,2.2,3.97910328999998));
#330297=CARTESIAN_POINT('Ctrl Pts',(-0.629280845000055,12.2,3.97975223799998));
#330298=CARTESIAN_POINT('Ctrl Pts',(-0.629280845000055,5.2,3.97975223799998));
#330299=CARTESIAN_POINT('Ctrl Pts',(-0.629280845000055,2.2,3.97975223799998));
#330300=CARTESIAN_POINT('Ctrl Pts',(-0.629476374000056,12.2,3.98040673499998));
#330301=CARTESIAN_POINT('Ctrl Pts',(-0.629476374000056,5.2,3.98040673499998));
#330302=CARTESIAN_POINT('Ctrl Pts',(-0.629476374000056,2.2,3.98040673499998));
#330303=CARTESIAN_POINT('Ctrl Pts',(-0.629674471000056,12.2,3.98106676699998));
#330304=CARTESIAN_POINT('Ctrl Pts',(-0.629674471000056,5.2,3.98106676699998));
#330305=CARTESIAN_POINT('Ctrl Pts',(-0.629674471000056,2.2,3.98106676699998));
#330306=CARTESIAN_POINT('Ctrl Pts',(-0.629875149000056,12.2,3.98173231599999));
#330307=CARTESIAN_POINT('Ctrl Pts',(-0.629875149000056,5.2,3.98173231599999));
#330308=CARTESIAN_POINT('Ctrl Pts',(-0.629875149000056,2.2,3.98173231599999));
#330309=CARTESIAN_POINT('Ctrl Pts',(-0.630078416000056,12.2,3.98240336699998));
#330310=CARTESIAN_POINT('Ctrl Pts',(-0.630078416000056,5.2,3.98240336699998));
#330311=CARTESIAN_POINT('Ctrl Pts',(-0.630078416000056,2.2,3.98240336699998));
#330312=CARTESIAN_POINT('Ctrl Pts',(-0.630284284000057,12.2,3.98307990399999));
#330313=CARTESIAN_POINT('Ctrl Pts',(-0.630284284000057,5.2,3.98307990399999));
#330314=CARTESIAN_POINT('Ctrl Pts',(-0.630284284000057,2.2,3.98307990399999));
#330315=CARTESIAN_POINT('Ctrl Pts',(-0.630492764000056,12.2,3.98376190999999));
#330316=CARTESIAN_POINT('Ctrl Pts',(-0.630492764000056,5.2,3.98376190999999));
#330317=CARTESIAN_POINT('Ctrl Pts',(-0.630492764000056,2.2,3.98376190999999));
#330318=CARTESIAN_POINT('Ctrl Pts',(-0.630703865000056,12.2,3.98444936999999));
#330319=CARTESIAN_POINT('Ctrl Pts',(-0.630703865000056,5.2,3.98444936999999));
#330320=CARTESIAN_POINT('Ctrl Pts',(-0.630703865000056,2.2,3.98444936999999));
#330321=CARTESIAN_POINT('Ctrl Pts',(-0.630917599000057,12.2,3.98514226799998));
#330322=CARTESIAN_POINT('Ctrl Pts',(-0.630917599000057,5.2,3.98514226799998));
#330323=CARTESIAN_POINT('Ctrl Pts',(-0.630917599000057,2.2,3.98514226799998));
#330324=CARTESIAN_POINT('Ctrl Pts',(-0.631133974000055,12.2,3.98584058799998));
#330325=CARTESIAN_POINT('Ctrl Pts',(-0.631133974000055,5.2,3.98584058799998));
#330326=CARTESIAN_POINT('Ctrl Pts',(-0.631133974000055,2.2,3.98584058799998));
#330327=CARTESIAN_POINT('Ctrl Pts',(-0.631353003000056,12.2,3.98654431399999));
#330328=CARTESIAN_POINT('Ctrl Pts',(-0.631353003000056,5.2,3.98654431399999));
#330329=CARTESIAN_POINT('Ctrl Pts',(-0.631353003000056,2.2,3.98654431399999));
#330330=CARTESIAN_POINT('Ctrl Pts',(-0.631574693000055,12.2,3.98725342999998));
#330331=CARTESIAN_POINT('Ctrl Pts',(-0.631574693000055,5.2,3.98725342999998));
#330332=CARTESIAN_POINT('Ctrl Pts',(-0.631574693000055,2.2,3.98725342999998));
#330333=CARTESIAN_POINT('Ctrl Pts',(-0.631799058000055,12.2,3.98796791999998));
#330334=CARTESIAN_POINT('Ctrl Pts',(-0.631799058000055,5.2,3.98796791999998));
#330335=CARTESIAN_POINT('Ctrl Pts',(-0.631799058000055,2.2,3.98796791999998));
#330336=CARTESIAN_POINT('Ctrl Pts',(-0.632026106000056,12.2,3.98868776899998));
#330337=CARTESIAN_POINT('Ctrl Pts',(-0.632026106000056,5.2,3.98868776899998));
#330338=CARTESIAN_POINT('Ctrl Pts',(-0.632026106000056,2.2,3.98868776899998));
#330339=CARTESIAN_POINT('Ctrl Pts',(-0.632255847000056,12.2,3.98941295999999));
#330340=CARTESIAN_POINT('Ctrl Pts',(-0.632255847000056,5.2,3.98941295999999));
#330341=CARTESIAN_POINT('Ctrl Pts',(-0.632255847000056,2.2,3.98941295999999));
#330342=CARTESIAN_POINT('Ctrl Pts',(-0.632488291000056,12.2,3.99014347899998));
#330343=CARTESIAN_POINT('Ctrl Pts',(-0.632488291000056,5.2,3.99014347899998));
#330344=CARTESIAN_POINT('Ctrl Pts',(-0.632488291000056,2.2,3.99014347899998));
#330345=CARTESIAN_POINT('Ctrl Pts',(-0.632723447000056,12.2,3.99087930899999));
#330346=CARTESIAN_POINT('Ctrl Pts',(-0.632723447000056,5.2,3.99087930899999));
#330347=CARTESIAN_POINT('Ctrl Pts',(-0.632723447000056,2.2,3.99087930899999));
#330348=CARTESIAN_POINT('Ctrl Pts',(-0.632961328000056,12.2,3.99162043499998));
#330349=CARTESIAN_POINT('Ctrl Pts',(-0.632961328000056,5.2,3.99162043499998));
#330350=CARTESIAN_POINT('Ctrl Pts',(-0.632961328000056,2.2,3.99162043499998));
#330351=CARTESIAN_POINT('Ctrl Pts',(-0.633201942000056,12.2,3.99236684199998));
#330352=CARTESIAN_POINT('Ctrl Pts',(-0.633201942000056,5.2,3.99236684199998));
#330353=CARTESIAN_POINT('Ctrl Pts',(-0.633201942000056,2.2,3.99236684199998));
#330354=CARTESIAN_POINT('Ctrl Pts',(-0.633445299000056,12.2,3.99311851299998));
#330355=CARTESIAN_POINT('Ctrl Pts',(-0.633445299000056,5.2,3.99311851299998));
#330356=CARTESIAN_POINT('Ctrl Pts',(-0.633445299000056,2.2,3.99311851299998));
#330357=CARTESIAN_POINT('Ctrl Pts',(-0.633691409000056,12.2,3.99387543199998));
#330358=CARTESIAN_POINT('Ctrl Pts',(-0.633691409000056,5.2,3.99387543199998));
#330359=CARTESIAN_POINT('Ctrl Pts',(-0.633691409000056,2.2,3.99387543199998));
#330360=CARTESIAN_POINT('Ctrl Pts',(-0.633940281000056,12.2,3.99463758599998));
#330361=CARTESIAN_POINT('Ctrl Pts',(-0.633940281000056,5.2,3.99463758599998));
#330362=CARTESIAN_POINT('Ctrl Pts',(-0.633940281000056,2.2,3.99463758599998));
#330363=CARTESIAN_POINT('Ctrl Pts',(-0.634191925000056,12.2,3.99540495699998));
#330364=CARTESIAN_POINT('Ctrl Pts',(-0.634191925000056,5.2,3.99540495699998));
#330365=CARTESIAN_POINT('Ctrl Pts',(-0.634191925000056,2.2,3.99540495699998));
#330366=CARTESIAN_POINT('Ctrl Pts',(-0.634446352000057,12.2,3.99617753199998));
#330367=CARTESIAN_POINT('Ctrl Pts',(-0.634446352000057,5.2,3.99617753199998));
#330368=CARTESIAN_POINT('Ctrl Pts',(-0.634446352000057,2.2,3.99617753199998));
#330369=CARTESIAN_POINT('Ctrl Pts',(-0.634703570000056,12.2,3.99695529299999));
#330370=CARTESIAN_POINT('Ctrl Pts',(-0.634703570000056,5.2,3.99695529299999));
#330371=CARTESIAN_POINT('Ctrl Pts',(-0.634703570000056,2.2,3.99695529299999));
#330372=CARTESIAN_POINT('Ctrl Pts',(-0.634963589000056,12.2,3.99773822599998));
#330373=CARTESIAN_POINT('Ctrl Pts',(-0.634963589000056,5.2,3.99773822599998));
#330374=CARTESIAN_POINT('Ctrl Pts',(-0.634963589000056,2.2,3.99773822599998));
#330375=CARTESIAN_POINT('Ctrl Pts',(-0.635226419000056,12.2,3.99852631499999));
#330376=CARTESIAN_POINT('Ctrl Pts',(-0.635226419000056,5.2,3.99852631499999));
#330377=CARTESIAN_POINT('Ctrl Pts',(-0.635226419000056,2.2,3.99852631499999));
#330378=CARTESIAN_POINT('Ctrl Pts',(-0.635492068000056,12.2,3.99931954599998));
#330379=CARTESIAN_POINT('Ctrl Pts',(-0.635492068000056,5.2,3.99931954599998));
#330380=CARTESIAN_POINT('Ctrl Pts',(-0.635492068000056,2.2,3.99931954599998));
#330381=CARTESIAN_POINT('Ctrl Pts',(-0.635760548000055,12.2,4.00011790099998));
#330382=CARTESIAN_POINT('Ctrl Pts',(-0.635760548000055,5.2,4.00011790099998));
#330383=CARTESIAN_POINT('Ctrl Pts',(-0.635760548000055,2.2,4.00011790099998));
#330384=CARTESIAN_POINT('Ctrl Pts',(-0.636031867000056,12.2,4.00092136699998));
#330385=CARTESIAN_POINT('Ctrl Pts',(-0.636031867000056,5.2,4.00092136699998));
#330386=CARTESIAN_POINT('Ctrl Pts',(-0.636031867000056,2.2,4.00092136699998));
#330387=CARTESIAN_POINT('Ctrl Pts',(-0.636306033000055,12.2,4.00172992899999));
#330388=CARTESIAN_POINT('Ctrl Pts',(-0.636306033000055,5.2,4.00172992899999));
#330389=CARTESIAN_POINT('Ctrl Pts',(-0.636306033000055,2.2,4.00172992899999));
#330390=CARTESIAN_POINT('Ctrl Pts',(-0.636583058000056,12.2,4.00254357099998));
#330391=CARTESIAN_POINT('Ctrl Pts',(-0.636583058000056,5.2,4.00254357099998));
#330392=CARTESIAN_POINT('Ctrl Pts',(-0.636583058000056,2.2,4.00254357099998));
#330393=CARTESIAN_POINT('Ctrl Pts',(-0.636862948000055,12.2,4.00336227799999));
#330394=CARTESIAN_POINT('Ctrl Pts',(-0.636862948000055,5.2,4.00336227799999));
#330395=CARTESIAN_POINT('Ctrl Pts',(-0.636862948000055,2.2,4.00336227799999));
#330396=CARTESIAN_POINT('Ctrl Pts',(-0.637145716000056,12.2,4.00418603399999));
#330397=CARTESIAN_POINT('Ctrl Pts',(-0.637145716000056,5.2,4.00418603399999));
#330398=CARTESIAN_POINT('Ctrl Pts',(-0.637145716000056,2.2,4.00418603399999));
#330399=CARTESIAN_POINT('Ctrl Pts',(-0.637431369000057,12.2,4.00501482399999));
#330400=CARTESIAN_POINT('Ctrl Pts',(-0.637431369000057,5.2,4.00501482399999));
#330401=CARTESIAN_POINT('Ctrl Pts',(-0.637431369000057,2.2,4.00501482399999));
#330402=CARTESIAN_POINT('Ctrl Pts',(-0.637719916000057,12.2,4.00584863399998));
#330403=CARTESIAN_POINT('Ctrl Pts',(-0.637719916000057,5.2,4.00584863399998));
#330404=CARTESIAN_POINT('Ctrl Pts',(-0.637719916000057,2.2,4.00584863399998));
#330405=CARTESIAN_POINT('Ctrl Pts',(-0.638011366000055,12.2,4.00668744799999));
#330406=CARTESIAN_POINT('Ctrl Pts',(-0.638011366000055,5.2,4.00668744799999));
#330407=CARTESIAN_POINT('Ctrl Pts',(-0.638011366000055,2.2,4.00668744799999));
#330408=CARTESIAN_POINT('Ctrl Pts',(-0.638305729000056,12.2,4.00753125199999));
#330409=CARTESIAN_POINT('Ctrl Pts',(-0.638305729000056,5.2,4.00753125199999));
#330410=CARTESIAN_POINT('Ctrl Pts',(-0.638305729000056,2.2,4.00753125199999));
#330411=CARTESIAN_POINT('Ctrl Pts',(-0.638603013000055,12.2,4.00838002899999));
#330412=CARTESIAN_POINT('Ctrl Pts',(-0.638603013000055,5.2,4.00838002899999));
#330413=CARTESIAN_POINT('Ctrl Pts',(-0.638603013000055,2.2,4.00838002899999));
#330414=CARTESIAN_POINT('Ctrl Pts',(-0.638903229000055,12.2,4.00923376599999));
#330415=CARTESIAN_POINT('Ctrl Pts',(-0.638903229000055,5.2,4.00923376599999));
#330416=CARTESIAN_POINT('Ctrl Pts',(-0.638903229000055,2.2,4.00923376599999));
#330417=CARTESIAN_POINT('Ctrl Pts',(-0.639206383000056,12.2,4.01009244699999));
#330418=CARTESIAN_POINT('Ctrl Pts',(-0.639206383000056,5.2,4.01009244699999));
#330419=CARTESIAN_POINT('Ctrl Pts',(-0.639206383000056,2.2,4.01009244699999));
#330420=CARTESIAN_POINT('Ctrl Pts',(-0.639512486000056,12.2,4.01095605699999));
#330421=CARTESIAN_POINT('Ctrl Pts',(-0.639512486000056,5.2,4.01095605699999));
#330422=CARTESIAN_POINT('Ctrl Pts',(-0.639512486000056,2.2,4.01095605699999));
#330423=CARTESIAN_POINT('Ctrl Pts',(-0.639821545000056,12.2,4.01182458199998));
#330424=CARTESIAN_POINT('Ctrl Pts',(-0.639821545000056,5.2,4.01182458199998));
#330425=CARTESIAN_POINT('Ctrl Pts',(-0.639821545000056,2.2,4.01182458199998));
#330426=CARTESIAN_POINT('Ctrl Pts',(-0.640133571000057,12.2,4.01269800599999));
#330427=CARTESIAN_POINT('Ctrl Pts',(-0.640133571000057,5.2,4.01269800599999));
#330428=CARTESIAN_POINT('Ctrl Pts',(-0.640133571000057,2.2,4.01269800599999));
#330429=CARTESIAN_POINT('Ctrl Pts',(-0.640448571000055,12.2,4.01357631499998));
#330430=CARTESIAN_POINT('Ctrl Pts',(-0.640448571000055,5.2,4.01357631499998));
#330431=CARTESIAN_POINT('Ctrl Pts',(-0.640448571000055,2.2,4.01357631499998));
#330432=CARTESIAN_POINT('Ctrl Pts',(-0.640766556000055,12.2,4.01445949299998));
#330433=CARTESIAN_POINT('Ctrl Pts',(-0.640766556000055,5.2,4.01445949299998));
#330434=CARTESIAN_POINT('Ctrl Pts',(-0.640766556000055,2.2,4.01445949299998));
#330435=CARTESIAN_POINT('Ctrl Pts',(-0.641087532000055,12.2,4.01534752699998));
#330436=CARTESIAN_POINT('Ctrl Pts',(-0.641087532000055,5.2,4.01534752699998));
#330437=CARTESIAN_POINT('Ctrl Pts',(-0.641087532000055,2.2,4.01534752699998));
#330438=CARTESIAN_POINT('Ctrl Pts',(-0.641411509000056,12.2,4.01624040099998));
#330439=CARTESIAN_POINT('Ctrl Pts',(-0.641411509000056,5.2,4.01624040099998));
#330440=CARTESIAN_POINT('Ctrl Pts',(-0.641411509000056,2.2,4.01624040099998));
#330441=CARTESIAN_POINT('Ctrl Pts',(-0.641738495000055,12.2,4.01713810099999));
#330442=CARTESIAN_POINT('Ctrl Pts',(-0.641738495000055,5.2,4.01713810099999));
#330443=CARTESIAN_POINT('Ctrl Pts',(-0.641738495000055,2.2,4.01713810099999));
#330444=CARTESIAN_POINT('Ctrl Pts',(-0.642068498000056,12.2,4.01804061099998));
#330445=CARTESIAN_POINT('Ctrl Pts',(-0.642068498000056,5.2,4.01804061099998));
#330446=CARTESIAN_POINT('Ctrl Pts',(-0.642068498000056,2.2,4.01804061099998));
#330447=CARTESIAN_POINT('Ctrl Pts',(-0.642401528000055,12.2,4.01894791799998));
#330448=CARTESIAN_POINT('Ctrl Pts',(-0.642401528000055,5.2,4.01894791799998));
#330449=CARTESIAN_POINT('Ctrl Pts',(-0.642401528000055,2.2,4.01894791799998));
#330450=CARTESIAN_POINT('Ctrl Pts',(-0.642737593000057,12.2,4.01986000599998));
#330451=CARTESIAN_POINT('Ctrl Pts',(-0.642737593000057,5.2,4.01986000599998));
#330452=CARTESIAN_POINT('Ctrl Pts',(-0.642737593000057,2.2,4.01986000599998));
#330453=CARTESIAN_POINT('Ctrl Pts',(-0.643076701000057,12.2,4.02077686099998));
#330454=CARTESIAN_POINT('Ctrl Pts',(-0.643076701000057,5.2,4.02077686099998));
#330455=CARTESIAN_POINT('Ctrl Pts',(-0.643076701000057,2.2,4.02077686099998));
#330456=CARTESIAN_POINT('Ctrl Pts',(-0.643418861000056,12.2,4.02169846799998));
#330457=CARTESIAN_POINT('Ctrl Pts',(-0.643418861000056,5.2,4.02169846799998));
#330458=CARTESIAN_POINT('Ctrl Pts',(-0.643418861000056,2.2,4.02169846799998));
#330459=CARTESIAN_POINT('Ctrl Pts',(-0.643764080000055,12.2,4.02262481199998));
#330460=CARTESIAN_POINT('Ctrl Pts',(-0.643764080000055,5.2,4.02262481199998));
#330461=CARTESIAN_POINT('Ctrl Pts',(-0.643764080000055,2.2,4.02262481199998));
#330462=CARTESIAN_POINT('Ctrl Pts',(-0.644112369000055,12.2,4.02355587999998));
#330463=CARTESIAN_POINT('Ctrl Pts',(-0.644112369000055,5.2,4.02355587999998));
#330464=CARTESIAN_POINT('Ctrl Pts',(-0.644112369000055,2.2,4.02355587999998));
#330465=CARTESIAN_POINT('Ctrl Pts',(-0.644463733000055,12.2,4.02449165699998));
#330466=CARTESIAN_POINT('Ctrl Pts',(-0.644463733000055,5.2,4.02449165699998));
#330467=CARTESIAN_POINT('Ctrl Pts',(-0.644463733000055,2.2,4.02449165699998));
#330468=CARTESIAN_POINT('Ctrl Pts',(-0.644818182000056,12.2,4.02543212699998));
#330469=CARTESIAN_POINT('Ctrl Pts',(-0.644818182000056,5.2,4.02543212699998));
#330470=CARTESIAN_POINT('Ctrl Pts',(-0.644818182000056,2.2,4.02543212699998));
#330471=CARTESIAN_POINT('Ctrl Pts',(-0.645175724000057,12.2,4.02637727699998));
#330472=CARTESIAN_POINT('Ctrl Pts',(-0.645175724000057,5.2,4.02637727699998));
#330473=CARTESIAN_POINT('Ctrl Pts',(-0.645175724000057,2.2,4.02637727699998));
#330474=CARTESIAN_POINT('Ctrl Pts',(-0.645536368000055,12.2,4.02732709299999));
#330475=CARTESIAN_POINT('Ctrl Pts',(-0.645536368000055,5.2,4.02732709299999));
#330476=CARTESIAN_POINT('Ctrl Pts',(-0.645536368000055,2.2,4.02732709299999));
#330477=CARTESIAN_POINT('Ctrl Pts',(-0.645900120000055,12.2,4.02828155799998));
#330478=CARTESIAN_POINT('Ctrl Pts',(-0.645900120000055,5.2,4.02828155799998));
#330479=CARTESIAN_POINT('Ctrl Pts',(-0.645900120000055,2.2,4.02828155799998));
#330480=CARTESIAN_POINT('Ctrl Pts',(-0.646266990000056,12.2,4.02924065999999));
#330481=CARTESIAN_POINT('Ctrl Pts',(-0.646266990000056,5.2,4.02924065999999));
#330482=CARTESIAN_POINT('Ctrl Pts',(-0.646266990000056,2.2,4.02924065999999));
#330483=CARTESIAN_POINT('Ctrl Pts',(-0.646636985000055,12.2,4.03020438399999));
#330484=CARTESIAN_POINT('Ctrl Pts',(-0.646636985000055,5.2,4.03020438399999));
#330485=CARTESIAN_POINT('Ctrl Pts',(-0.646636985000055,2.2,4.03020438399999));
#330486=CARTESIAN_POINT('Ctrl Pts',(-0.647010113000055,12.2,4.03117271499998));
#330487=CARTESIAN_POINT('Ctrl Pts',(-0.647010113000055,5.2,4.03117271499998));
#330488=CARTESIAN_POINT('Ctrl Pts',(-0.647010113000055,2.2,4.03117271499998));
#330489=CARTESIAN_POINT('Ctrl Pts',(-0.647386383000056,12.2,4.03214563999998));
#330490=CARTESIAN_POINT('Ctrl Pts',(-0.647386383000056,5.2,4.03214563999998));
#330491=CARTESIAN_POINT('Ctrl Pts',(-0.647386383000056,2.2,4.03214563999998));
#330492=CARTESIAN_POINT('Ctrl Pts',(-0.647765802000055,12.2,4.03312314399999));
#330493=CARTESIAN_POINT('Ctrl Pts',(-0.647765802000055,5.2,4.03312314399999));
#330494=CARTESIAN_POINT('Ctrl Pts',(-0.647765802000055,2.2,4.03312314399999));
#330495=CARTESIAN_POINT('Ctrl Pts',(-0.648148378000055,12.2,4.03410521199999));
#330496=CARTESIAN_POINT('Ctrl Pts',(-0.648148378000055,5.2,4.03410521199999));
#330497=CARTESIAN_POINT('Ctrl Pts',(-0.648148378000055,2.2,4.03410521199999));
#330498=CARTESIAN_POINT('Ctrl Pts',(-0.648534119000056,12.2,4.03509183099998));
#330499=CARTESIAN_POINT('Ctrl Pts',(-0.648534119000056,5.2,4.03509183099998));
#330500=CARTESIAN_POINT('Ctrl Pts',(-0.648534119000056,2.2,4.03509183099998));
#330501=CARTESIAN_POINT('Ctrl Pts',(-0.648923032000056,12.2,4.03608298599998));
#330502=CARTESIAN_POINT('Ctrl Pts',(-0.648923032000056,5.2,4.03608298599998));
#330503=CARTESIAN_POINT('Ctrl Pts',(-0.648923032000056,2.2,4.03608298599998));
#330504=CARTESIAN_POINT('Ctrl Pts',(-0.649315126000056,12.2,4.03707866299998));
#330505=CARTESIAN_POINT('Ctrl Pts',(-0.649315126000056,5.2,4.03707866299998));
#330506=CARTESIAN_POINT('Ctrl Pts',(-0.649315126000056,2.2,4.03707866299998));
#330507=CARTESIAN_POINT('Ctrl Pts',(-0.649710408000056,12.2,4.03807884799999));
#330508=CARTESIAN_POINT('Ctrl Pts',(-0.649710408000056,5.2,4.03807884799999));
#330509=CARTESIAN_POINT('Ctrl Pts',(-0.649710408000056,2.2,4.03807884799999));
#330510=CARTESIAN_POINT('Ctrl Pts',(-0.650108887000057,12.2,4.03908352699998));
#330511=CARTESIAN_POINT('Ctrl Pts',(-0.650108887000057,5.2,4.03908352699998));
#330512=CARTESIAN_POINT('Ctrl Pts',(-0.650108887000057,2.2,4.03908352699998));
#330513=CARTESIAN_POINT('Ctrl Pts',(-0.650510568000057,12.2,4.04009268399999));
#330514=CARTESIAN_POINT('Ctrl Pts',(-0.650510568000057,5.2,4.04009268399999));
#330515=CARTESIAN_POINT('Ctrl Pts',(-0.650510568000057,2.2,4.04009268399999));
#330516=CARTESIAN_POINT('Ctrl Pts',(-0.650915461000056,12.2,4.04110630799998));
#330517=CARTESIAN_POINT('Ctrl Pts',(-0.650915461000056,5.2,4.04110630799998));
#330518=CARTESIAN_POINT('Ctrl Pts',(-0.650915461000056,2.2,4.04110630799998));
#330519=CARTESIAN_POINT('Ctrl Pts',(-0.651323572000055,12.2,4.04212438299999));
#330520=CARTESIAN_POINT('Ctrl Pts',(-0.651323572000055,5.2,4.04212438299999));
#330521=CARTESIAN_POINT('Ctrl Pts',(-0.651323572000055,2.2,4.04212438299999));
#330522=CARTESIAN_POINT('Ctrl Pts',(-0.651734911000055,12.2,4.04314689499999));
#330523=CARTESIAN_POINT('Ctrl Pts',(-0.651734911000055,5.2,4.04314689499999));
#330524=CARTESIAN_POINT('Ctrl Pts',(-0.651734911000055,2.2,4.04314689499999));
#330525=CARTESIAN_POINT('Ctrl Pts',(-0.652149483000055,12.2,4.04417382999998));
#330526=CARTESIAN_POINT('Ctrl Pts',(-0.652149483000055,5.2,4.04417382999998));
#330527=CARTESIAN_POINT('Ctrl Pts',(-0.652149483000055,2.2,4.04417382999998));
#330528=CARTESIAN_POINT('Ctrl Pts',(-0.652567296000056,12.2,4.04520517499999));
#330529=CARTESIAN_POINT('Ctrl Pts',(-0.652567296000056,5.2,4.04520517499999));
#330530=CARTESIAN_POINT('Ctrl Pts',(-0.652567296000056,2.2,4.04520517499999));
#330531=CARTESIAN_POINT('Ctrl Pts',(-0.652988358000056,12.2,4.04624091499999));
#330532=CARTESIAN_POINT('Ctrl Pts',(-0.652988358000056,5.2,4.04624091499999));
#330533=CARTESIAN_POINT('Ctrl Pts',(-0.652988358000056,2.2,4.04624091499999));
#330534=CARTESIAN_POINT('Ctrl Pts',(-0.653412676000055,12.2,4.04728103699998));
#330535=CARTESIAN_POINT('Ctrl Pts',(-0.653412676000055,5.2,4.04728103699998));
#330536=CARTESIAN_POINT('Ctrl Pts',(-0.653412676000055,2.2,4.04728103699998));
#330537=CARTESIAN_POINT('Ctrl Pts',(-0.653840258000056,12.2,4.04832552499998));
#330538=CARTESIAN_POINT('Ctrl Pts',(-0.653840258000056,5.2,4.04832552499998));
#330539=CARTESIAN_POINT('Ctrl Pts',(-0.653840258000056,2.2,4.04832552499998));
#330540=CARTESIAN_POINT('Ctrl Pts',(-0.654271111000057,12.2,4.04937436799998));
#330541=CARTESIAN_POINT('Ctrl Pts',(-0.654271111000057,5.2,4.04937436799998));
#330542=CARTESIAN_POINT('Ctrl Pts',(-0.654271111000057,2.2,4.04937436799998));
#330543=CARTESIAN_POINT('Ctrl Pts',(-0.654705242000055,12.2,4.05042754999998));
#330544=CARTESIAN_POINT('Ctrl Pts',(-0.654705242000055,5.2,4.05042754999998));
#330545=CARTESIAN_POINT('Ctrl Pts',(-0.654705242000055,2.2,4.05042754999998));
#330546=CARTESIAN_POINT('Ctrl Pts',(-0.655142658000055,12.2,4.05148505699999));
#330547=CARTESIAN_POINT('Ctrl Pts',(-0.655142658000055,5.2,4.05148505699999));
#330548=CARTESIAN_POINT('Ctrl Pts',(-0.655142658000055,2.2,4.05148505699999));
#330549=CARTESIAN_POINT('Ctrl Pts',(-0.655583367000055,12.2,4.05254687799999));
#330550=CARTESIAN_POINT('Ctrl Pts',(-0.655583367000055,5.2,4.05254687799999));
#330551=CARTESIAN_POINT('Ctrl Pts',(-0.655583367000055,2.2,4.05254687799999));
#330552=CARTESIAN_POINT('Ctrl Pts',(-0.656027376000056,12.2,4.05361299499998));
#330553=CARTESIAN_POINT('Ctrl Pts',(-0.656027376000056,5.2,4.05361299499998));
#330554=CARTESIAN_POINT('Ctrl Pts',(-0.656027376000056,2.2,4.05361299499998));
#330555=CARTESIAN_POINT('Ctrl Pts',(-0.656474692000056,12.2,4.05468339699999));
#330556=CARTESIAN_POINT('Ctrl Pts',(-0.656474692000056,5.2,4.05468339699999));
#330557=CARTESIAN_POINT('Ctrl Pts',(-0.656474692000056,2.2,4.05468339699999));
#330558=CARTESIAN_POINT('Ctrl Pts',(-0.656925322000056,12.2,4.05575806999998));
#330559=CARTESIAN_POINT('Ctrl Pts',(-0.656925322000056,5.2,4.05575806999998));
#330560=CARTESIAN_POINT('Ctrl Pts',(-0.656925322000056,2.2,4.05575806999998));
#330561=CARTESIAN_POINT('Ctrl Pts',(-0.657379273000057,12.2,4.05683699999998));
#330562=CARTESIAN_POINT('Ctrl Pts',(-0.657379273000057,5.2,4.05683699999998));
#330563=CARTESIAN_POINT('Ctrl Pts',(-0.657379273000057,2.2,4.05683699999998));
#330564=CARTESIAN_POINT('Ctrl Pts',(-0.657836552000056,12.2,4.05792017199998));
#330565=CARTESIAN_POINT('Ctrl Pts',(-0.657836552000056,5.2,4.05792017199998));
#330566=CARTESIAN_POINT('Ctrl Pts',(-0.657836552000056,2.2,4.05792017199998));
#330567=CARTESIAN_POINT('Ctrl Pts',(-0.658297168000056,12.2,4.05900757499998));
#330568=CARTESIAN_POINT('Ctrl Pts',(-0.658297168000056,5.2,4.05900757499998));
#330569=CARTESIAN_POINT('Ctrl Pts',(-0.658297168000056,2.2,4.05900757499998));
#330570=CARTESIAN_POINT('Ctrl Pts',(-0.658761125000057,12.2,4.06009919199998));
#330571=CARTESIAN_POINT('Ctrl Pts',(-0.658761125000057,5.2,4.06009919199998));
#330572=CARTESIAN_POINT('Ctrl Pts',(-0.658761125000057,2.2,4.06009919199998));
#330573=CARTESIAN_POINT('Ctrl Pts',(-0.659228431000055,12.2,4.06119501299998));
#330574=CARTESIAN_POINT('Ctrl Pts',(-0.659228431000055,5.2,4.06119501299998));
#330575=CARTESIAN_POINT('Ctrl Pts',(-0.659228431000055,2.2,4.06119501299998));
#330576=CARTESIAN_POINT('Ctrl Pts',(-0.659699094000056,12.2,4.06229501999999));
#330577=CARTESIAN_POINT('Ctrl Pts',(-0.659699094000056,5.2,4.06229501999999));
#330578=CARTESIAN_POINT('Ctrl Pts',(-0.659699094000056,2.2,4.06229501999999));
#330579=CARTESIAN_POINT('Ctrl Pts',(-0.660173120000056,12.2,4.06339920299998));
#330580=CARTESIAN_POINT('Ctrl Pts',(-0.660173120000056,5.2,4.06339920299998));
#330581=CARTESIAN_POINT('Ctrl Pts',(-0.660173120000056,2.2,4.06339920299998));
#330582=CARTESIAN_POINT('Ctrl Pts',(-0.660650515000055,12.2,4.06450754799998));
#330583=CARTESIAN_POINT('Ctrl Pts',(-0.660650515000055,5.2,4.06450754799998));
#330584=CARTESIAN_POINT('Ctrl Pts',(-0.660650515000055,2.2,4.06450754799998));
#330585=CARTESIAN_POINT('Ctrl Pts',(-0.661131288000056,12.2,4.06562003999999));
#330586=CARTESIAN_POINT('Ctrl Pts',(-0.661131288000056,5.2,4.06562003999999));
#330587=CARTESIAN_POINT('Ctrl Pts',(-0.661131288000056,2.2,4.06562003999999));
#330588=CARTESIAN_POINT('Ctrl Pts',(-0.661615444000055,12.2,4.06673666599998));
#330589=CARTESIAN_POINT('Ctrl Pts',(-0.661615444000055,5.2,4.06673666599998));
#330590=CARTESIAN_POINT('Ctrl Pts',(-0.661615444000055,2.2,4.06673666599998));
#330591=CARTESIAN_POINT('Ctrl Pts',(-0.662102990000056,12.2,4.06785741199998));
#330592=CARTESIAN_POINT('Ctrl Pts',(-0.662102990000056,5.2,4.06785741199998));
#330593=CARTESIAN_POINT('Ctrl Pts',(-0.662102990000056,2.2,4.06785741199998));
#330594=CARTESIAN_POINT('Ctrl Pts',(-0.662593934000055,12.2,4.06898226699998));
#330595=CARTESIAN_POINT('Ctrl Pts',(-0.662593934000055,5.2,4.06898226699998));
#330596=CARTESIAN_POINT('Ctrl Pts',(-0.662593934000055,2.2,4.06898226699998));
#330597=CARTESIAN_POINT('Ctrl Pts',(-0.663088280000055,12.2,4.07011121399999));
#330598=CARTESIAN_POINT('Ctrl Pts',(-0.663088280000055,5.2,4.07011121399999));
#330599=CARTESIAN_POINT('Ctrl Pts',(-0.663088280000055,2.2,4.07011121399999));
#330600=CARTESIAN_POINT('Ctrl Pts',(-0.663586038000057,12.2,4.07124424199999));
#330601=CARTESIAN_POINT('Ctrl Pts',(-0.663586038000057,5.2,4.07124424199999));
#330602=CARTESIAN_POINT('Ctrl Pts',(-0.663586038000057,2.2,4.07124424199999));
#330603=CARTESIAN_POINT('Ctrl Pts',(-0.664087212000056,12.2,4.07238133699998));
#330604=CARTESIAN_POINT('Ctrl Pts',(-0.664087212000056,5.2,4.07238133699998));
#330605=CARTESIAN_POINT('Ctrl Pts',(-0.664087212000056,2.2,4.07238133699998));
#330606=CARTESIAN_POINT('Ctrl Pts',(-0.664591809000056,12.2,4.07352248499999));
#330607=CARTESIAN_POINT('Ctrl Pts',(-0.664591809000056,5.2,4.07352248499999));
#330608=CARTESIAN_POINT('Ctrl Pts',(-0.664591809000056,2.2,4.07352248499999));
#330609=CARTESIAN_POINT('Ctrl Pts',(-0.665099838000056,12.2,4.07466767299999));
#330610=CARTESIAN_POINT('Ctrl Pts',(-0.665099838000056,5.2,4.07466767299999));
#330611=CARTESIAN_POINT('Ctrl Pts',(-0.665099838000056,2.2,4.07466767299999));
#330612=CARTESIAN_POINT('Ctrl Pts',(-0.665611302000055,12.2,4.07581688699998));
#330613=CARTESIAN_POINT('Ctrl Pts',(-0.665611302000055,5.2,4.07581688699998));
#330614=CARTESIAN_POINT('Ctrl Pts',(-0.665611302000055,2.2,4.07581688699998));
#330615=CARTESIAN_POINT('Ctrl Pts',(-0.666126210000056,12.2,4.07697011499998));
#330616=CARTESIAN_POINT('Ctrl Pts',(-0.666126210000056,5.2,4.07697011499998));
#330617=CARTESIAN_POINT('Ctrl Pts',(-0.666126210000056,2.2,4.07697011499998));
#330618=CARTESIAN_POINT('Ctrl Pts',(-0.666644568000055,12.2,4.07812734299998));
#330619=CARTESIAN_POINT('Ctrl Pts',(-0.666644568000055,5.2,4.07812734299998));
#330620=CARTESIAN_POINT('Ctrl Pts',(-0.666644568000055,2.2,4.07812734299998));
#330621=CARTESIAN_POINT('Ctrl Pts',(-0.667166381000056,12.2,4.07928855699998));
#330622=CARTESIAN_POINT('Ctrl Pts',(-0.667166381000056,5.2,4.07928855699998));
#330623=CARTESIAN_POINT('Ctrl Pts',(-0.667166381000056,2.2,4.07928855699998));
#330624=CARTESIAN_POINT('Ctrl Pts',(-0.667691657000056,12.2,4.08045374499999));
#330625=CARTESIAN_POINT('Ctrl Pts',(-0.667691657000056,5.2,4.08045374499999));
#330626=CARTESIAN_POINT('Ctrl Pts',(-0.667691657000056,2.2,4.08045374499999));
#330627=CARTESIAN_POINT('Ctrl Pts',(-0.668220401000056,12.2,4.08162289299998));
#330628=CARTESIAN_POINT('Ctrl Pts',(-0.668220401000056,5.2,4.08162289299998));
#330629=CARTESIAN_POINT('Ctrl Pts',(-0.668220401000056,2.2,4.08162289299998));
#330630=CARTESIAN_POINT('Ctrl Pts',(-0.668752621000056,12.2,4.08279598699998));
#330631=CARTESIAN_POINT('Ctrl Pts',(-0.668752621000056,5.2,4.08279598699998));
#330632=CARTESIAN_POINT('Ctrl Pts',(-0.668752621000056,2.2,4.08279598699998));
#330633=CARTESIAN_POINT('Ctrl Pts',(-0.669288322000057,12.2,4.08397301599998));
#330634=CARTESIAN_POINT('Ctrl Pts',(-0.669288322000057,5.2,4.08397301599998));
#330635=CARTESIAN_POINT('Ctrl Pts',(-0.669288322000057,2.2,4.08397301599998));
#330636=CARTESIAN_POINT('Ctrl Pts',(-0.669827511000056,12.2,4.08515396399999));
#330637=CARTESIAN_POINT('Ctrl Pts',(-0.669827511000056,5.2,4.08515396399999));
#330638=CARTESIAN_POINT('Ctrl Pts',(-0.669827511000056,2.2,4.08515396399999));
#330639=CARTESIAN_POINT('Ctrl Pts',(-0.670370194000055,12.2,4.08633882099998));
#330640=CARTESIAN_POINT('Ctrl Pts',(-0.670370194000055,5.2,4.08633882099998));
#330641=CARTESIAN_POINT('Ctrl Pts',(-0.670370194000055,2.2,4.08633882099998));
#330642=CARTESIAN_POINT('Ctrl Pts',(-0.670916377000056,12.2,4.08752756999998));
#330643=CARTESIAN_POINT('Ctrl Pts',(-0.670916377000056,5.2,4.08752756999998));
#330644=CARTESIAN_POINT('Ctrl Pts',(-0.670916377000056,2.2,4.08752756999998));
#330645=CARTESIAN_POINT('Ctrl Pts',(-0.671466066000056,12.2,4.08872020199999));
#330646=CARTESIAN_POINT('Ctrl Pts',(-0.671466066000056,5.2,4.08872020199999));
#330647=CARTESIAN_POINT('Ctrl Pts',(-0.671466066000056,2.2,4.08872020199999));
#330648=CARTESIAN_POINT('Ctrl Pts',(-0.672019267000056,12.2,4.08991670099999));
#330649=CARTESIAN_POINT('Ctrl Pts',(-0.672019267000056,5.2,4.08991670099999));
#330650=CARTESIAN_POINT('Ctrl Pts',(-0.672019267000056,2.2,4.08991670099999));
#330651=CARTESIAN_POINT('Ctrl Pts',(-0.672575988000055,12.2,4.09111705399998));
#330652=CARTESIAN_POINT('Ctrl Pts',(-0.672575988000055,5.2,4.09111705399998));
#330653=CARTESIAN_POINT('Ctrl Pts',(-0.672575988000055,2.2,4.09111705399998));
#330654=CARTESIAN_POINT('Ctrl Pts',(-0.673136233000056,12.2,4.09232124999999));
#330655=CARTESIAN_POINT('Ctrl Pts',(-0.673136233000056,5.2,4.09232124999999));
#330656=CARTESIAN_POINT('Ctrl Pts',(-0.673136233000056,2.2,4.09232124999999));
#330657=CARTESIAN_POINT('Ctrl Pts',(-0.673700008000055,12.2,4.09352927399999));
#330658=CARTESIAN_POINT('Ctrl Pts',(-0.673700008000055,5.2,4.09352927399999));
#330659=CARTESIAN_POINT('Ctrl Pts',(-0.673700008000055,2.2,4.09352927399999));
#330660=CARTESIAN_POINT('Ctrl Pts',(-0.674267321000055,12.2,4.09474111499998));
#330661=CARTESIAN_POINT('Ctrl Pts',(-0.674267321000055,5.2,4.09474111499998));
#330662=CARTESIAN_POINT('Ctrl Pts',(-0.674267321000055,2.2,4.09474111499998));
#330663=CARTESIAN_POINT('Ctrl Pts',(-0.674838176000057,12.2,4.09595675699999));
#330664=CARTESIAN_POINT('Ctrl Pts',(-0.674838176000057,5.2,4.09595675699999));
#330665=CARTESIAN_POINT('Ctrl Pts',(-0.674838176000057,2.2,4.09595675699999));
#330666=CARTESIAN_POINT('Ctrl Pts',(-0.675412580000057,12.2,4.09717618899998));
#330667=CARTESIAN_POINT('Ctrl Pts',(-0.675412580000057,5.2,4.09717618899998));
#330668=CARTESIAN_POINT('Ctrl Pts',(-0.675412580000057,2.2,4.09717618899998));
#330669=CARTESIAN_POINT('Ctrl Pts',(-0.675990538000055,12.2,4.09839939799999));
#330670=CARTESIAN_POINT('Ctrl Pts',(-0.675990538000055,5.2,4.09839939799999));
#330671=CARTESIAN_POINT('Ctrl Pts',(-0.675990538000055,2.2,4.09839939799999));
#330672=CARTESIAN_POINT('Ctrl Pts',(-0.676572058000057,12.2,4.09962637099999));
#330673=CARTESIAN_POINT('Ctrl Pts',(-0.676572058000057,5.2,4.09962637099999));
#330674=CARTESIAN_POINT('Ctrl Pts',(-0.676572058000057,2.2,4.09962637099999));
#330675=CARTESIAN_POINT('Ctrl Pts',(-0.677157144000056,12.2,4.10085709399999));
#330676=CARTESIAN_POINT('Ctrl Pts',(-0.677157144000056,5.2,4.10085709399999));
#330677=CARTESIAN_POINT('Ctrl Pts',(-0.677157144000056,2.2,4.10085709399999));
#330678=CARTESIAN_POINT('Ctrl Pts',(-0.677745802000055,12.2,4.10209155499999));
#330679=CARTESIAN_POINT('Ctrl Pts',(-0.677745802000055,5.2,4.10209155499999));
#330680=CARTESIAN_POINT('Ctrl Pts',(-0.677745802000055,2.2,4.10209155499999));
#330681=CARTESIAN_POINT('Ctrl Pts',(-0.678338038000056,12.2,4.10332974099998));
#330682=CARTESIAN_POINT('Ctrl Pts',(-0.678338038000056,5.2,4.10332974099998));
#330683=CARTESIAN_POINT('Ctrl Pts',(-0.678338038000056,2.2,4.10332974099998));
#330684=CARTESIAN_POINT('Ctrl Pts',(-0.678933857000056,12.2,4.10457163999999));
#330685=CARTESIAN_POINT('Ctrl Pts',(-0.678933857000056,5.2,4.10457163999999));
#330686=CARTESIAN_POINT('Ctrl Pts',(-0.678933857000056,2.2,4.10457163999999));
#330687=CARTESIAN_POINT('Ctrl Pts',(-0.679533266000056,12.2,4.10581723699998));
#330688=CARTESIAN_POINT('Ctrl Pts',(-0.679533266000056,5.2,4.10581723699998));
#330689=CARTESIAN_POINT('Ctrl Pts',(-0.679533266000056,2.2,4.10581723699998));
#330690=CARTESIAN_POINT('Ctrl Pts',(-0.680136271000055,12.2,4.10706652199998));
#330691=CARTESIAN_POINT('Ctrl Pts',(-0.680136271000055,5.2,4.10706652199998));
#330692=CARTESIAN_POINT('Ctrl Pts',(-0.680136271000055,2.2,4.10706652199998));
#330693=CARTESIAN_POINT('Ctrl Pts',(-0.680742878000055,12.2,4.10831947899998));
#330694=CARTESIAN_POINT('Ctrl Pts',(-0.680742878000055,5.2,4.10831947899998));
#330695=CARTESIAN_POINT('Ctrl Pts',(-0.680742878000055,2.2,4.10831947899998));
#330696=CARTESIAN_POINT('Ctrl Pts',(-0.681353090000056,12.2,4.10957609699998));
#330697=CARTESIAN_POINT('Ctrl Pts',(-0.681353090000056,5.2,4.10957609699998));
#330698=CARTESIAN_POINT('Ctrl Pts',(-0.681353090000056,2.2,4.10957609699998));
#330699=CARTESIAN_POINT('Ctrl Pts',(-0.681966916000055,12.2,4.11083636399999));
#330700=CARTESIAN_POINT('Ctrl Pts',(-0.681966916000055,5.2,4.11083636399999));
#330701=CARTESIAN_POINT('Ctrl Pts',(-0.681966916000055,2.2,4.11083636399999));
#330702=CARTESIAN_POINT('Ctrl Pts',(-0.682584358000057,12.2,4.11210026599999));
#330703=CARTESIAN_POINT('Ctrl Pts',(-0.682584358000057,5.2,4.11210026599999));
#330704=CARTESIAN_POINT('Ctrl Pts',(-0.682584358000057,2.2,4.11210026599999));
#330705=CARTESIAN_POINT('Ctrl Pts',(-0.683205425000055,12.2,4.11336778999999));
#330706=CARTESIAN_POINT('Ctrl Pts',(-0.683205425000055,5.2,4.11336778999999));
#330707=CARTESIAN_POINT('Ctrl Pts',(-0.683205425000055,2.2,4.11336778999999));
#330708=CARTESIAN_POINT('Ctrl Pts',(-0.683830121000056,12.2,4.11463892399999));
#330709=CARTESIAN_POINT('Ctrl Pts',(-0.683830121000056,5.2,4.11463892399999));
#330710=CARTESIAN_POINT('Ctrl Pts',(-0.683830121000056,2.2,4.11463892399999));
#330711=CARTESIAN_POINT('Ctrl Pts',(-0.684458451000056,12.2,4.11591365699999));
#330712=CARTESIAN_POINT('Ctrl Pts',(-0.684458451000056,5.2,4.11591365699999));
#330713=CARTESIAN_POINT('Ctrl Pts',(-0.684458451000056,2.2,4.11591365699999));
#330714=CARTESIAN_POINT('Ctrl Pts',(-0.685090423000055,12.2,4.11719197299998));
#330715=CARTESIAN_POINT('Ctrl Pts',(-0.685090423000055,5.2,4.11719197299998));
#330716=CARTESIAN_POINT('Ctrl Pts',(-0.685090423000055,2.2,4.11719197299998));
#330717=CARTESIAN_POINT('Ctrl Pts',(-0.685726038000055,12.2,4.11847385999998));
#330718=CARTESIAN_POINT('Ctrl Pts',(-0.685726038000055,5.2,4.11847385999998));
#330719=CARTESIAN_POINT('Ctrl Pts',(-0.685726038000055,2.2,4.11847385999998));
#330720=CARTESIAN_POINT('Ctrl Pts',(-0.686365306000055,12.2,4.11975930699998));
#330721=CARTESIAN_POINT('Ctrl Pts',(-0.686365306000055,5.2,4.11975930699998));
#330722=CARTESIAN_POINT('Ctrl Pts',(-0.686365306000055,2.2,4.11975930699998));
#330723=CARTESIAN_POINT('Ctrl Pts',(-0.687008229000057,12.2,4.12104830099998));
#330724=CARTESIAN_POINT('Ctrl Pts',(-0.687008229000057,5.2,4.12104830099998));
#330725=CARTESIAN_POINT('Ctrl Pts',(-0.687008229000057,2.2,4.12104830099998));
#330726=CARTESIAN_POINT('Ctrl Pts',(-0.687654816000055,12.2,4.12234082799999));
#330727=CARTESIAN_POINT('Ctrl Pts',(-0.687654816000055,5.2,4.12234082799999));
#330728=CARTESIAN_POINT('Ctrl Pts',(-0.687654816000055,2.2,4.12234082799999));
#330729=CARTESIAN_POINT('Ctrl Pts',(-0.688305069000055,12.2,4.12363687799999));
#330730=CARTESIAN_POINT('Ctrl Pts',(-0.688305069000055,5.2,4.12363687799999));
#330731=CARTESIAN_POINT('Ctrl Pts',(-0.688305069000055,2.2,4.12363687799999));
#330732=CARTESIAN_POINT('Ctrl Pts',(-0.688958994000056,12.2,4.12493643499998));
#330733=CARTESIAN_POINT('Ctrl Pts',(-0.688958994000056,5.2,4.12493643499998));
#330734=CARTESIAN_POINT('Ctrl Pts',(-0.688958994000056,2.2,4.12493643499998));
#330735=CARTESIAN_POINT('Ctrl Pts',(-0.689616598000056,12.2,4.12623949099999));
#330736=CARTESIAN_POINT('Ctrl Pts',(-0.689616598000056,5.2,4.12623949099999));
#330737=CARTESIAN_POINT('Ctrl Pts',(-0.689616598000056,2.2,4.12623949099999));
#330738=CARTESIAN_POINT('Ctrl Pts',(-0.690277884000056,12.2,4.12754602799998));
#330739=CARTESIAN_POINT('Ctrl Pts',(-0.690277884000056,5.2,4.12754602799998));
#330740=CARTESIAN_POINT('Ctrl Pts',(-0.690277884000056,2.2,4.12754602799998));
#330741=CARTESIAN_POINT('Ctrl Pts',(-0.690942859000057,12.2,4.12885603799998));
#330742=CARTESIAN_POINT('Ctrl Pts',(-0.690942859000057,5.2,4.12885603799998));
#330743=CARTESIAN_POINT('Ctrl Pts',(-0.690942859000057,2.2,4.12885603799998));
#330744=CARTESIAN_POINT('Ctrl Pts',(-0.691611527000056,12.2,4.13016950599999));
#330745=CARTESIAN_POINT('Ctrl Pts',(-0.691611527000056,5.2,4.13016950599999));
#330746=CARTESIAN_POINT('Ctrl Pts',(-0.691611527000056,2.2,4.13016950599999));
#330747=CARTESIAN_POINT('Ctrl Pts',(-0.692283895000055,12.2,4.13148642099999));
#330748=CARTESIAN_POINT('Ctrl Pts',(-0.692283895000055,5.2,4.13148642099999));
#330749=CARTESIAN_POINT('Ctrl Pts',(-0.692283895000055,2.2,4.13148642099999));
#330750=CARTESIAN_POINT('Ctrl Pts',(-0.692959966000056,12.2,4.13280676999998));
#330751=CARTESIAN_POINT('Ctrl Pts',(-0.692959966000056,5.2,4.13280676999998));
#330752=CARTESIAN_POINT('Ctrl Pts',(-0.692959966000056,2.2,4.13280676999998));
#330753=CARTESIAN_POINT('Ctrl Pts',(-0.693639747000055,12.2,4.13413053899998));
#330754=CARTESIAN_POINT('Ctrl Pts',(-0.693639747000055,5.2,4.13413053899998));
#330755=CARTESIAN_POINT('Ctrl Pts',(-0.693639747000055,2.2,4.13413053899998));
#330756=CARTESIAN_POINT('Ctrl Pts',(-0.694323241000055,12.2,4.13545771799999));
#330757=CARTESIAN_POINT('Ctrl Pts',(-0.694323241000055,5.2,4.13545771799999));
#330758=CARTESIAN_POINT('Ctrl Pts',(-0.694323241000055,2.2,4.13545771799999));
#330759=CARTESIAN_POINT('Ctrl Pts',(-0.695010455000055,12.2,4.13678829299998));
#330760=CARTESIAN_POINT('Ctrl Pts',(-0.695010455000055,5.2,4.13678829299998));
#330761=CARTESIAN_POINT('Ctrl Pts',(-0.695010455000055,2.2,4.13678829299998));
#330762=CARTESIAN_POINT('Ctrl Pts',(-0.695701394000056,12.2,4.13812225399998));
#330763=CARTESIAN_POINT('Ctrl Pts',(-0.695701394000056,5.2,4.13812225399998));
#330764=CARTESIAN_POINT('Ctrl Pts',(-0.695701394000056,2.2,4.13812225399998));
#330765=CARTESIAN_POINT('Ctrl Pts',(-0.696396062000056,12.2,4.13945958499998));
#330766=CARTESIAN_POINT('Ctrl Pts',(-0.696396062000056,5.2,4.13945958499998));
#330767=CARTESIAN_POINT('Ctrl Pts',(-0.696396062000056,2.2,4.13945958499998));
#330768=CARTESIAN_POINT('Ctrl Pts',(-0.697094464000055,12.2,4.14080027599999));
#330769=CARTESIAN_POINT('Ctrl Pts',(-0.697094464000055,5.2,4.14080027599999));
#330770=CARTESIAN_POINT('Ctrl Pts',(-0.697094464000055,2.2,4.14080027599999));
#330771=CARTESIAN_POINT('Ctrl Pts',(-0.697796606000055,12.2,4.14214431499998));
#330772=CARTESIAN_POINT('Ctrl Pts',(-0.697796606000055,5.2,4.14214431499998));
#330773=CARTESIAN_POINT('Ctrl Pts',(-0.697796606000055,2.2,4.14214431499998));
#330774=CARTESIAN_POINT('Ctrl Pts',(-0.698502492000056,12.2,4.14349168899999));
#330775=CARTESIAN_POINT('Ctrl Pts',(-0.698502492000056,5.2,4.14349168899999));
#330776=CARTESIAN_POINT('Ctrl Pts',(-0.698502492000056,2.2,4.14349168899999));
#330777=CARTESIAN_POINT('Ctrl Pts',(-0.699212127000056,12.2,4.14484238499998));
#330778=CARTESIAN_POINT('Ctrl Pts',(-0.699212127000056,5.2,4.14484238499998));
#330779=CARTESIAN_POINT('Ctrl Pts',(-0.699212127000056,2.2,4.14484238499998));
#330780=CARTESIAN_POINT('Ctrl Pts',(-0.699925517000055,12.2,4.14619639199999));
#330781=CARTESIAN_POINT('Ctrl Pts',(-0.699925517000055,5.2,4.14619639199999));
#330782=CARTESIAN_POINT('Ctrl Pts',(-0.699925517000055,2.2,4.14619639199999));
#330783=CARTESIAN_POINT('Ctrl Pts',(-0.700642665000055,12.2,4.14755369699999));
#330784=CARTESIAN_POINT('Ctrl Pts',(-0.700642665000055,5.2,4.14755369699999));
#330785=CARTESIAN_POINT('Ctrl Pts',(-0.700642665000055,2.2,4.14755369699999));
#330786=CARTESIAN_POINT('Ctrl Pts',(-0.701363578000055,12.2,4.14891428699999));
#330787=CARTESIAN_POINT('Ctrl Pts',(-0.701363578000055,5.2,4.14891428699999));
#330788=CARTESIAN_POINT('Ctrl Pts',(-0.701363578000055,2.2,4.14891428699999));
#330789=CARTESIAN_POINT('Ctrl Pts',(-0.702088258000056,12.2,4.15027815199998));
#330790=CARTESIAN_POINT('Ctrl Pts',(-0.702088258000056,5.2,4.15027815199998));
#330791=CARTESIAN_POINT('Ctrl Pts',(-0.702088258000056,2.2,4.15027815199998));
#330792=CARTESIAN_POINT('Ctrl Pts',(-0.702816713000055,12.2,4.15164527899999));
#330793=CARTESIAN_POINT('Ctrl Pts',(-0.702816713000055,5.2,4.15164527899999));
#330794=CARTESIAN_POINT('Ctrl Pts',(-0.702816713000055,2.2,4.15164527899999));
#330795=CARTESIAN_POINT('Ctrl Pts',(-0.703548946000057,12.2,4.15301565399999));
#330796=CARTESIAN_POINT('Ctrl Pts',(-0.703548946000057,5.2,4.15301565399999));
#330797=CARTESIAN_POINT('Ctrl Pts',(-0.703548946000057,2.2,4.15301565399999));
#330798=CARTESIAN_POINT('Ctrl Pts',(-0.704284962000056,12.2,4.15438926699998));
#330799=CARTESIAN_POINT('Ctrl Pts',(-0.704284962000056,5.2,4.15438926699998));
#330800=CARTESIAN_POINT('Ctrl Pts',(-0.704284962000056,2.2,4.15438926699998));
#330801=CARTESIAN_POINT('Ctrl Pts',(-0.705024766000056,12.2,4.15576610399999));
#330802=CARTESIAN_POINT('Ctrl Pts',(-0.705024766000056,5.2,4.15576610399999));
#330803=CARTESIAN_POINT('Ctrl Pts',(-0.705024766000056,2.2,4.15576610399999));
#330804=CARTESIAN_POINT('Ctrl Pts',(-0.705768362000055,12.2,4.15714615499999));
#330805=CARTESIAN_POINT('Ctrl Pts',(-0.705768362000055,5.2,4.15714615499999));
#330806=CARTESIAN_POINT('Ctrl Pts',(-0.705768362000055,2.2,4.15714615499999));
#330807=CARTESIAN_POINT('Ctrl Pts',(-0.706515755000057,12.2,4.15852940599999));
#330808=CARTESIAN_POINT('Ctrl Pts',(-0.706515755000057,5.2,4.15852940599999));
#330809=CARTESIAN_POINT('Ctrl Pts',(-0.706515755000057,2.2,4.15852940599999));
#330810=CARTESIAN_POINT('Ctrl Pts',(-0.707266950000056,12.2,4.15991584599999));
#330811=CARTESIAN_POINT('Ctrl Pts',(-0.707266950000056,5.2,4.15991584599999));
#330812=CARTESIAN_POINT('Ctrl Pts',(-0.707266950000056,2.2,4.15991584599999));
#330813=CARTESIAN_POINT('Ctrl Pts',(-0.708021951000056,12.2,4.16130546299998));
#330814=CARTESIAN_POINT('Ctrl Pts',(-0.708021951000056,5.2,4.16130546299998));
#330815=CARTESIAN_POINT('Ctrl Pts',(-0.708021951000056,2.2,4.16130546299998));
#330816=CARTESIAN_POINT('Ctrl Pts',(-0.708780763000056,12.2,4.16269824399999));
#330817=CARTESIAN_POINT('Ctrl Pts',(-0.708780763000056,5.2,4.16269824399999));
#330818=CARTESIAN_POINT('Ctrl Pts',(-0.708780763000056,2.2,4.16269824399999));
#330819=CARTESIAN_POINT('Ctrl Pts',(-0.709543392000055,12.2,4.16409417799999));
#330820=CARTESIAN_POINT('Ctrl Pts',(-0.709543392000055,5.2,4.16409417799999));
#330821=CARTESIAN_POINT('Ctrl Pts',(-0.709543392000055,2.2,4.16409417799999));
#330822=CARTESIAN_POINT('Ctrl Pts',(-0.710309839000055,12.2,4.16549325299999));
#330823=CARTESIAN_POINT('Ctrl Pts',(-0.710309839000055,5.2,4.16549325299999));
#330824=CARTESIAN_POINT('Ctrl Pts',(-0.710309839000055,2.2,4.16549325299999));
#330825=CARTESIAN_POINT('Ctrl Pts',(-0.711080112000056,12.2,4.16689545499998));
#330826=CARTESIAN_POINT('Ctrl Pts',(-0.711080112000056,5.2,4.16689545499998));
#330827=CARTESIAN_POINT('Ctrl Pts',(-0.711080112000056,2.2,4.16689545499998));
#330828=CARTESIAN_POINT('Ctrl Pts',(-0.711854213000055,12.2,4.16830077499998));
#330829=CARTESIAN_POINT('Ctrl Pts',(-0.711854213000055,5.2,4.16830077499998));
#330830=CARTESIAN_POINT('Ctrl Pts',(-0.711854213000055,2.2,4.16830077499998));
#330831=CARTESIAN_POINT('Ctrl Pts',(-0.712632149000055,12.2,4.16970919899998));
#330832=CARTESIAN_POINT('Ctrl Pts',(-0.712632149000055,5.2,4.16970919899998));
#330833=CARTESIAN_POINT('Ctrl Pts',(-0.712632149000055,2.2,4.16970919899998));
#330834=CARTESIAN_POINT('Ctrl Pts',(-0.713413922000056,12.2,4.17112071399998));
#330835=CARTESIAN_POINT('Ctrl Pts',(-0.713413922000056,5.2,4.17112071399998));
#330836=CARTESIAN_POINT('Ctrl Pts',(-0.713413922000056,2.2,4.17112071399998));
#330837=CARTESIAN_POINT('Ctrl Pts',(-0.714199538000055,12.2,4.17253531199999));
#330838=CARTESIAN_POINT('Ctrl Pts',(-0.714199538000055,5.2,4.17253531199999));
#330839=CARTESIAN_POINT('Ctrl Pts',(-0.714199538000055,2.2,4.17253531199999));
#330840=CARTESIAN_POINT('Ctrl Pts',(-0.714988999000056,12.2,4.17395297699999));
#330841=CARTESIAN_POINT('Ctrl Pts',(-0.714988999000056,5.2,4.17395297699999));
#330842=CARTESIAN_POINT('Ctrl Pts',(-0.714988999000056,2.2,4.17395297699999));
#330843=CARTESIAN_POINT('Ctrl Pts',(-0.715782313000056,12.2,4.17537369999998));
#330844=CARTESIAN_POINT('Ctrl Pts',(-0.715782313000056,5.2,4.17537369999998));
#330845=CARTESIAN_POINT('Ctrl Pts',(-0.715782313000056,2.2,4.17537369999998));
#330846=CARTESIAN_POINT('Ctrl Pts',(-0.716579482000055,12.2,4.17679746799998));
#330847=CARTESIAN_POINT('Ctrl Pts',(-0.716579482000055,5.2,4.17679746799998));
#330848=CARTESIAN_POINT('Ctrl Pts',(-0.716579482000055,2.2,4.17679746799998));
#330849=CARTESIAN_POINT('Ctrl Pts',(-0.717380511000056,12.2,4.17822426999999));
#330850=CARTESIAN_POINT('Ctrl Pts',(-0.717380511000056,5.2,4.17822426999999));
#330851=CARTESIAN_POINT('Ctrl Pts',(-0.717380511000056,2.2,4.17822426999999));
#330852=CARTESIAN_POINT('Ctrl Pts',(-0.718185404000057,12.2,4.17965409099998));
#330853=CARTESIAN_POINT('Ctrl Pts',(-0.718185404000057,5.2,4.17965409099998));
#330854=CARTESIAN_POINT('Ctrl Pts',(-0.718185404000057,2.2,4.17965409099998));
#330855=CARTESIAN_POINT('Ctrl Pts',(-0.718994165000056,12.2,4.18108692299998));
#330856=CARTESIAN_POINT('Ctrl Pts',(-0.718994165000056,5.2,4.18108692299998));
#330857=CARTESIAN_POINT('Ctrl Pts',(-0.718994165000056,2.2,4.18108692299998));
#330858=CARTESIAN_POINT('Ctrl Pts',(-0.719806800000056,12.2,4.18252275099999));
#330859=CARTESIAN_POINT('Ctrl Pts',(-0.719806800000056,5.2,4.18252275099999));
#330860=CARTESIAN_POINT('Ctrl Pts',(-0.719806800000056,2.2,4.18252275099999));
#330861=CARTESIAN_POINT('Ctrl Pts',(-0.720623311000056,12.2,4.18396156599999));
#330862=CARTESIAN_POINT('Ctrl Pts',(-0.720623311000056,5.2,4.18396156599999));
#330863=CARTESIAN_POINT('Ctrl Pts',(-0.720623311000056,2.2,4.18396156599999));
#330864=CARTESIAN_POINT('Ctrl Pts',(-0.721443703000055,12.2,4.18540335499999));
#330865=CARTESIAN_POINT('Ctrl Pts',(-0.721443703000055,5.2,4.18540335499999));
#330866=CARTESIAN_POINT('Ctrl Pts',(-0.721443703000055,2.2,4.18540335499999));
#330867=CARTESIAN_POINT('Ctrl Pts',(-0.722267980000056,12.2,4.18684810599999));
#330868=CARTESIAN_POINT('Ctrl Pts',(-0.722267980000056,5.2,4.18684810599999));
#330869=CARTESIAN_POINT('Ctrl Pts',(-0.722267980000056,2.2,4.18684810599999));
#330870=CARTESIAN_POINT('Ctrl Pts',(-0.723096147000056,12.2,4.18829580799999));
#330871=CARTESIAN_POINT('Ctrl Pts',(-0.723096147000056,5.2,4.18829580799999));
#330872=CARTESIAN_POINT('Ctrl Pts',(-0.723096147000056,2.2,4.18829580799999));
#330873=CARTESIAN_POINT('Ctrl Pts',(-0.723928208000055,12.2,4.18974644799999));
#330874=CARTESIAN_POINT('Ctrl Pts',(-0.723928208000055,5.2,4.18974644799999));
#330875=CARTESIAN_POINT('Ctrl Pts',(-0.723928208000055,2.2,4.18974644799999));
#330876=CARTESIAN_POINT('Ctrl Pts',(-0.724764166000057,12.2,4.19120001499999));
#330877=CARTESIAN_POINT('Ctrl Pts',(-0.724764166000057,5.2,4.19120001499999));
#330878=CARTESIAN_POINT('Ctrl Pts',(-0.724764166000057,2.2,4.19120001499999));
#330879=CARTESIAN_POINT('Ctrl Pts',(-0.725604025000056,12.2,4.19265649699998));
#330880=CARTESIAN_POINT('Ctrl Pts',(-0.725604025000056,5.2,4.19265649699998));
#330881=CARTESIAN_POINT('Ctrl Pts',(-0.725604025000056,2.2,4.19265649699998));
#330882=CARTESIAN_POINT('Ctrl Pts',(-0.726447791000057,12.2,4.19411588299998));
#330883=CARTESIAN_POINT('Ctrl Pts',(-0.726447791000057,5.2,4.19411588299998));
#330884=CARTESIAN_POINT('Ctrl Pts',(-0.726447791000057,2.2,4.19411588299998));
#330885=CARTESIAN_POINT('Ctrl Pts',(-0.727295466000056,12.2,4.19557816099999));
#330886=CARTESIAN_POINT('Ctrl Pts',(-0.727295466000056,5.2,4.19557816099999));
#330887=CARTESIAN_POINT('Ctrl Pts',(-0.727295466000056,2.2,4.19557816099999));
#330888=CARTESIAN_POINT('Ctrl Pts',(-0.728147055000056,12.2,4.19704331899998));
#330889=CARTESIAN_POINT('Ctrl Pts',(-0.728147055000056,5.2,4.19704331899998));
#330890=CARTESIAN_POINT('Ctrl Pts',(-0.728147055000056,2.2,4.19704331899998));
#330891=CARTESIAN_POINT('Ctrl Pts',(-0.729002563000056,12.2,4.19851134599998));
#330892=CARTESIAN_POINT('Ctrl Pts',(-0.729002563000056,5.2,4.19851134599998));
#330893=CARTESIAN_POINT('Ctrl Pts',(-0.729002563000056,2.2,4.19851134599998));
#330894=CARTESIAN_POINT('Ctrl Pts',(-0.729861992000057,12.2,4.19998222999999));
#330895=CARTESIAN_POINT('Ctrl Pts',(-0.729861992000057,5.2,4.19998222999999));
#330896=CARTESIAN_POINT('Ctrl Pts',(-0.729861992000057,2.2,4.19998222999999));
#330897=CARTESIAN_POINT('Ctrl Pts',(-0.730725346000056,12.2,4.20145595999998));
#330898=CARTESIAN_POINT('Ctrl Pts',(-0.730725346000056,5.2,4.20145595999998));
#330899=CARTESIAN_POINT('Ctrl Pts',(-0.730725346000056,2.2,4.20145595999998));
#330900=CARTESIAN_POINT('Ctrl Pts',(-0.731592631000056,12.2,4.20293252199999));
#330901=CARTESIAN_POINT('Ctrl Pts',(-0.731592631000056,5.2,4.20293252199999));
#330902=CARTESIAN_POINT('Ctrl Pts',(-0.731592631000056,2.2,4.20293252199999));
#330903=CARTESIAN_POINT('Ctrl Pts',(-0.732463849000055,12.2,4.20441190799998));
#330904=CARTESIAN_POINT('Ctrl Pts',(-0.732463849000055,5.2,4.20441190799998));
#330905=CARTESIAN_POINT('Ctrl Pts',(-0.732463849000055,2.2,4.20441190799998));
#330906=CARTESIAN_POINT('Ctrl Pts',(-0.733339005000057,12.2,4.20589410399998));
#330907=CARTESIAN_POINT('Ctrl Pts',(-0.733339005000057,5.2,4.20589410399998));
#330908=CARTESIAN_POINT('Ctrl Pts',(-0.733339005000057,2.2,4.20589410399998));
#330909=CARTESIAN_POINT('Ctrl Pts',(-0.734218101000056,12.2,4.20737909899999));
#330910=CARTESIAN_POINT('Ctrl Pts',(-0.734218101000056,5.2,4.20737909899999));
#330911=CARTESIAN_POINT('Ctrl Pts',(-0.734218101000056,2.2,4.20737909899999));
#330912=CARTESIAN_POINT('Ctrl Pts',(-0.735101143000056,12.2,4.20886688199998));
#330913=CARTESIAN_POINT('Ctrl Pts',(-0.735101143000056,5.2,4.20886688199998));
#330914=CARTESIAN_POINT('Ctrl Pts',(-0.735101143000056,2.2,4.20886688199998));
#330915=CARTESIAN_POINT('Ctrl Pts',(-0.735988134000056,12.2,4.21035744099999));
#330916=CARTESIAN_POINT('Ctrl Pts',(-0.735988134000056,5.2,4.21035744099999));
#330917=CARTESIAN_POINT('Ctrl Pts',(-0.735988134000056,2.2,4.21035744099999));
#330918=CARTESIAN_POINT('Ctrl Pts',(-0.736879077000056,12.2,4.21185076399999));
#330919=CARTESIAN_POINT('Ctrl Pts',(-0.736879077000056,5.2,4.21185076399999));
#330920=CARTESIAN_POINT('Ctrl Pts',(-0.736879077000056,2.2,4.21185076399999));
#330921=CARTESIAN_POINT('Ctrl Pts',(-0.737773977000057,12.2,4.21334684099998));
#330922=CARTESIAN_POINT('Ctrl Pts',(-0.737773977000057,5.2,4.21334684099998));
#330923=CARTESIAN_POINT('Ctrl Pts',(-0.737773977000057,2.2,4.21334684099998));
#330924=CARTESIAN_POINT('Ctrl Pts',(-0.738672837000056,12.2,4.21484565899998));
#330925=CARTESIAN_POINT('Ctrl Pts',(-0.738672837000056,5.2,4.21484565899998));
#330926=CARTESIAN_POINT('Ctrl Pts',(-0.738672837000056,2.2,4.21484565899998));
#330927=CARTESIAN_POINT('Ctrl Pts',(-0.739575662000057,12.2,4.21634720699998));
#330928=CARTESIAN_POINT('Ctrl Pts',(-0.739575662000057,5.2,4.21634720699998));
#330929=CARTESIAN_POINT('Ctrl Pts',(-0.739575662000057,2.2,4.21634720699998));
#330930=CARTESIAN_POINT('Ctrl Pts',(-0.740482454000055,12.2,4.21785147499998));
#330931=CARTESIAN_POINT('Ctrl Pts',(-0.740482454000055,5.2,4.21785147499998));
#330932=CARTESIAN_POINT('Ctrl Pts',(-0.740482454000055,2.2,4.21785147499998));
#330933=CARTESIAN_POINT('Ctrl Pts',(-0.741393217000056,12.2,4.21935844899998));
#330934=CARTESIAN_POINT('Ctrl Pts',(-0.741393217000056,5.2,4.21935844899998));
#330935=CARTESIAN_POINT('Ctrl Pts',(-0.741393217000056,2.2,4.21935844899998));
#330936=CARTESIAN_POINT('Ctrl Pts',(-0.742307956000056,12.2,4.22086811899998));
#330937=CARTESIAN_POINT('Ctrl Pts',(-0.742307956000056,5.2,4.22086811899998));
#330938=CARTESIAN_POINT('Ctrl Pts',(-0.742307956000056,2.2,4.22086811899998));
#330939=CARTESIAN_POINT('Ctrl Pts',(-0.743226673000056,12.2,4.22238047399999));
#330940=CARTESIAN_POINT('Ctrl Pts',(-0.743226673000056,5.2,4.22238047399999));
#330941=CARTESIAN_POINT('Ctrl Pts',(-0.743226673000056,2.2,4.22238047399999));
#330942=CARTESIAN_POINT('Ctrl Pts',(-0.744149371000056,12.2,4.22389550199998));
#330943=CARTESIAN_POINT('Ctrl Pts',(-0.744149371000056,5.2,4.22389550199998));
#330944=CARTESIAN_POINT('Ctrl Pts',(-0.744149371000056,2.2,4.22389550199998));
#330945=CARTESIAN_POINT('Ctrl Pts',(-0.745076057000055,12.2,4.22541319099999));
#330946=CARTESIAN_POINT('Ctrl Pts',(-0.745076057000055,5.2,4.22541319099999));
#330947=CARTESIAN_POINT('Ctrl Pts',(-0.745076057000055,2.2,4.22541319099999));
#330948=CARTESIAN_POINT('Ctrl Pts',(-0.746006730000056,12.2,4.22693353199998));
#330949=CARTESIAN_POINT('Ctrl Pts',(-0.746006730000056,5.2,4.22693353199998));
#330950=CARTESIAN_POINT('Ctrl Pts',(-0.746006730000056,2.2,4.22693353199998));
#330951=CARTESIAN_POINT('Ctrl Pts',(-0.746941397000055,12.2,4.22845651199999));
#330952=CARTESIAN_POINT('Ctrl Pts',(-0.746941397000055,5.2,4.22845651199999));
#330953=CARTESIAN_POINT('Ctrl Pts',(-0.746941397000055,2.2,4.22845651199999));
#330954=CARTESIAN_POINT('Ctrl Pts',(-0.747880061000057,12.2,4.22998211899999));
#330955=CARTESIAN_POINT('Ctrl Pts',(-0.747880061000057,5.2,4.22998211899999));
#330956=CARTESIAN_POINT('Ctrl Pts',(-0.747880061000057,2.2,4.22998211899999));
#330957=CARTESIAN_POINT('Ctrl Pts',(-0.748822725000055,12.2,4.23151034299998));
#330958=CARTESIAN_POINT('Ctrl Pts',(-0.748822725000055,5.2,4.23151034299998));
#330959=CARTESIAN_POINT('Ctrl Pts',(-0.748822725000055,2.2,4.23151034299998));
#330960=CARTESIAN_POINT('Ctrl Pts',(-0.749769392000056,12.2,4.23304117199999));
#330961=CARTESIAN_POINT('Ctrl Pts',(-0.749769392000056,5.2,4.23304117199999));
#330962=CARTESIAN_POINT('Ctrl Pts',(-0.749769392000056,2.2,4.23304117199999));
#330963=CARTESIAN_POINT('Ctrl Pts',(-0.750720065000056,12.2,4.23457459399999));
#330964=CARTESIAN_POINT('Ctrl Pts',(-0.750720065000056,5.2,4.23457459399999));
#330965=CARTESIAN_POINT('Ctrl Pts',(-0.750720065000056,2.2,4.23457459399999));
#330966=CARTESIAN_POINT('Ctrl Pts',(-0.751674750000056,12.2,4.23611059999998));
#330967=CARTESIAN_POINT('Ctrl Pts',(-0.751674750000056,5.2,4.23611059999998));
#330968=CARTESIAN_POINT('Ctrl Pts',(-0.751674750000056,2.2,4.23611059999998));
#330969=CARTESIAN_POINT('Ctrl Pts',(-0.752633448000056,12.2,4.23764917699998));
#330970=CARTESIAN_POINT('Ctrl Pts',(-0.752633448000056,5.2,4.23764917699998));
#330971=CARTESIAN_POINT('Ctrl Pts',(-0.752633448000056,2.2,4.23764917699998));
#330972=CARTESIAN_POINT('Ctrl Pts',(-0.753596163000055,12.2,4.23919031499998));
#330973=CARTESIAN_POINT('Ctrl Pts',(-0.753596163000055,5.2,4.23919031499998));
#330974=CARTESIAN_POINT('Ctrl Pts',(-0.753596163000055,2.2,4.23919031499998));
#330975=CARTESIAN_POINT('Ctrl Pts',(-0.754562898000056,12.2,4.24073399999998));
#330976=CARTESIAN_POINT('Ctrl Pts',(-0.754562898000056,5.2,4.24073399999998));
#330977=CARTESIAN_POINT('Ctrl Pts',(-0.754562898000056,2.2,4.24073399999998));
#330978=CARTESIAN_POINT('Ctrl Pts',(-0.755533657000056,12.2,4.24228022499998));
#330979=CARTESIAN_POINT('Ctrl Pts',(-0.755533657000056,5.2,4.24228022499998));
#330980=CARTESIAN_POINT('Ctrl Pts',(-0.755533657000056,2.2,4.24228022499998));
#330981=CARTESIAN_POINT('Ctrl Pts',(-0.756508444000056,12.2,4.24382897599998));
#330982=CARTESIAN_POINT('Ctrl Pts',(-0.756508444000056,5.2,4.24382897599998));
#330983=CARTESIAN_POINT('Ctrl Pts',(-0.756508444000056,2.2,4.24382897599998));
#330984=CARTESIAN_POINT('Ctrl Pts',(-0.757487261000056,12.2,4.24538024199999));
#330985=CARTESIAN_POINT('Ctrl Pts',(-0.757487261000056,5.2,4.24538024199999));
#330986=CARTESIAN_POINT('Ctrl Pts',(-0.757487261000056,2.2,4.24538024199999));
#330987=CARTESIAN_POINT('Ctrl Pts',(-0.758470112000056,12.2,4.24693401299999));
#330988=CARTESIAN_POINT('Ctrl Pts',(-0.758470112000056,5.2,4.24693401299999));
#330989=CARTESIAN_POINT('Ctrl Pts',(-0.758470112000056,2.2,4.24693401299999));
#330990=CARTESIAN_POINT('Ctrl Pts',(-0.759457000000056,12.2,4.24849027799999));
#330991=CARTESIAN_POINT('Ctrl Pts',(-0.759457000000056,5.2,4.24849027799999));
#330992=CARTESIAN_POINT('Ctrl Pts',(-0.759457000000056,2.2,4.24849027799999));
#330993=CARTESIAN_POINT('Ctrl Pts',(-0.760447928000056,12.2,4.25004902299998));
#330994=CARTESIAN_POINT('Ctrl Pts',(-0.760447928000056,5.2,4.25004902299998));
#330995=CARTESIAN_POINT('Ctrl Pts',(-0.760447928000056,2.2,4.25004902299998));
#330996=CARTESIAN_POINT('Ctrl Pts',(-0.761442900000056,12.2,4.25161024099998));
#330997=CARTESIAN_POINT('Ctrl Pts',(-0.761442900000056,5.2,4.25161024099998));
#330998=CARTESIAN_POINT('Ctrl Pts',(-0.761442900000056,2.2,4.25161024099998));
#330999=CARTESIAN_POINT('Ctrl Pts',(-0.762441918000055,12.2,4.25317391799998));
#331000=CARTESIAN_POINT('Ctrl Pts',(-0.762441918000055,5.2,4.25317391799998));
#331001=CARTESIAN_POINT('Ctrl Pts',(-0.762441918000055,2.2,4.25317391799998));
#331002=CARTESIAN_POINT('Ctrl Pts',(-0.763444986000056,12.2,4.25474004399998));
#331003=CARTESIAN_POINT('Ctrl Pts',(-0.763444986000056,5.2,4.25474004399998));
#331004=CARTESIAN_POINT('Ctrl Pts',(-0.763444986000056,2.2,4.25474004399998));
#331005=CARTESIAN_POINT('Ctrl Pts',(-0.764452107000055,12.2,4.25630860699999));
#331006=CARTESIAN_POINT('Ctrl Pts',(-0.764452107000055,5.2,4.25630860699999));
#331007=CARTESIAN_POINT('Ctrl Pts',(-0.764452107000055,2.2,4.25630860699999));
#331008=CARTESIAN_POINT('Ctrl Pts',(-0.765463285000055,12.2,4.25787959799998));
#331009=CARTESIAN_POINT('Ctrl Pts',(-0.765463285000055,5.2,4.25787959799998));
#331010=CARTESIAN_POINT('Ctrl Pts',(-0.765463285000055,2.2,4.25787959799998));
#331011=CARTESIAN_POINT('Ctrl Pts',(-0.766478522000057,12.2,4.25945300399999));
#331012=CARTESIAN_POINT('Ctrl Pts',(-0.766478522000057,5.2,4.25945300399999));
#331013=CARTESIAN_POINT('Ctrl Pts',(-0.766478522000057,2.2,4.25945300399999));
#331014=CARTESIAN_POINT('Ctrl Pts',(-0.767497821000056,12.2,4.26102881499999));
#331015=CARTESIAN_POINT('Ctrl Pts',(-0.767497821000056,5.2,4.26102881499999));
#331016=CARTESIAN_POINT('Ctrl Pts',(-0.767497821000056,2.2,4.26102881499999));
#331017=CARTESIAN_POINT('Ctrl Pts',(-0.768521186000056,12.2,4.26260701899999));
#331018=CARTESIAN_POINT('Ctrl Pts',(-0.768521186000056,5.2,4.26260701899999));
#331019=CARTESIAN_POINT('Ctrl Pts',(-0.768521186000056,2.2,4.26260701899999));
#331020=CARTESIAN_POINT('Ctrl Pts',(-0.769548620000055,12.2,4.26418760599999));
#331021=CARTESIAN_POINT('Ctrl Pts',(-0.769548620000055,5.2,4.26418760599999));
#331022=CARTESIAN_POINT('Ctrl Pts',(-0.769548620000055,2.2,4.26418760599999));
#331023=CARTESIAN_POINT('Ctrl Pts',(-0.770580124000055,12.2,4.26577056599999));
#331024=CARTESIAN_POINT('Ctrl Pts',(-0.770580124000055,5.2,4.26577056599999));
#331025=CARTESIAN_POINT('Ctrl Pts',(-0.770580124000055,2.2,4.26577056599999));
#331026=CARTESIAN_POINT('Ctrl Pts',(-0.771615704000055,12.2,4.26735588499999));
#331027=CARTESIAN_POINT('Ctrl Pts',(-0.771615704000055,5.2,4.26735588499999));
#331028=CARTESIAN_POINT('Ctrl Pts',(-0.771615704000055,2.2,4.26735588499999));
#331029=CARTESIAN_POINT('Ctrl Pts',(-0.772655361000056,12.2,4.26894355499999));
#331030=CARTESIAN_POINT('Ctrl Pts',(-0.772655361000056,5.2,4.26894355499999));
#331031=CARTESIAN_POINT('Ctrl Pts',(-0.772655361000056,2.2,4.26894355499999));
#331032=CARTESIAN_POINT('Ctrl Pts',(-0.773699100000057,12.2,4.27053356399998));
#331033=CARTESIAN_POINT('Ctrl Pts',(-0.773699100000057,5.2,4.27053356399998));
#331034=CARTESIAN_POINT('Ctrl Pts',(-0.773699100000057,2.2,4.27053356399998));
#331035=CARTESIAN_POINT('Ctrl Pts',(-0.774746921000055,12.2,4.27212589999999));
#331036=CARTESIAN_POINT('Ctrl Pts',(-0.774746921000055,5.2,4.27212589999999));
#331037=CARTESIAN_POINT('Ctrl Pts',(-0.774746921000055,2.2,4.27212589999999));
#331038=CARTESIAN_POINT('Ctrl Pts',(-0.775798829000056,12.2,4.27372055299998));
#331039=CARTESIAN_POINT('Ctrl Pts',(-0.775798829000056,5.2,4.27372055299998));
#331040=CARTESIAN_POINT('Ctrl Pts',(-0.775798829000056,2.2,4.27372055299998));
#331041=CARTESIAN_POINT('Ctrl Pts',(-0.776854827000056,12.2,4.27531751299998));
#331042=CARTESIAN_POINT('Ctrl Pts',(-0.776854827000056,5.2,4.27531751299998));
#331043=CARTESIAN_POINT('Ctrl Pts',(-0.776854827000056,2.2,4.27531751299998));
#331044=CARTESIAN_POINT('Ctrl Pts',(-0.777914917000055,12.2,4.27691676699999));
#331045=CARTESIAN_POINT('Ctrl Pts',(-0.777914917000055,5.2,4.27691676699999));
#331046=CARTESIAN_POINT('Ctrl Pts',(-0.777914917000055,2.2,4.27691676699999));
#331047=CARTESIAN_POINT('Ctrl Pts',(-0.778979103000056,12.2,4.27851830699999));
#331048=CARTESIAN_POINT('Ctrl Pts',(-0.778979103000056,5.2,4.27851830699999));
#331049=CARTESIAN_POINT('Ctrl Pts',(-0.778979103000056,2.2,4.27851830699999));
#331050=CARTESIAN_POINT('Ctrl Pts',(-0.780047386000057,12.2,4.28012212099999));
#331051=CARTESIAN_POINT('Ctrl Pts',(-0.780047386000057,5.2,4.28012212099999));
#331052=CARTESIAN_POINT('Ctrl Pts',(-0.780047386000057,2.2,4.28012212099999));
#331053=CARTESIAN_POINT('Ctrl Pts',(-0.781119770000055,12.2,4.28172819599999));
#331054=CARTESIAN_POINT('Ctrl Pts',(-0.781119770000055,5.2,4.28172819599999));
#331055=CARTESIAN_POINT('Ctrl Pts',(-0.781119770000055,2.2,4.28172819599999));
#331056=CARTESIAN_POINT('Ctrl Pts',(-0.782196258000055,12.2,4.28333652299998));
#331057=CARTESIAN_POINT('Ctrl Pts',(-0.782196258000055,5.2,4.28333652299998));
#331058=CARTESIAN_POINT('Ctrl Pts',(-0.782196258000055,2.2,4.28333652299998));
#331059=CARTESIAN_POINT('Ctrl Pts',(-0.783276853000056,12.2,4.28494709199998));
#331060=CARTESIAN_POINT('Ctrl Pts',(-0.783276853000056,5.2,4.28494709199998));
#331061=CARTESIAN_POINT('Ctrl Pts',(-0.783276853000056,2.2,4.28494709199998));
#331062=CARTESIAN_POINT('Ctrl Pts',(-0.784361558000055,12.2,4.28655989199999));
#331063=CARTESIAN_POINT('Ctrl Pts',(-0.784361558000055,5.2,4.28655989199999));
#331064=CARTESIAN_POINT('Ctrl Pts',(-0.784361558000055,2.2,4.28655989199999));
#331065=CARTESIAN_POINT('Ctrl Pts',(-0.785450374000056,12.2,4.28817490999998));
#331066=CARTESIAN_POINT('Ctrl Pts',(-0.785450374000056,5.2,4.28817490999998));
#331067=CARTESIAN_POINT('Ctrl Pts',(-0.785450374000056,2.2,4.28817490999998));
#331068=CARTESIAN_POINT('Ctrl Pts',(-0.786543305000055,12.2,4.28979213799998));
#331069=CARTESIAN_POINT('Ctrl Pts',(-0.786543305000055,5.2,4.28979213799998));
#331070=CARTESIAN_POINT('Ctrl Pts',(-0.786543305000055,2.2,4.28979213799998));
#331071=CARTESIAN_POINT('Ctrl Pts',(-0.787640354000055,12.2,4.29141156299998));
#331072=CARTESIAN_POINT('Ctrl Pts',(-0.787640354000055,5.2,4.29141156299998));
#331073=CARTESIAN_POINT('Ctrl Pts',(-0.787640354000055,2.2,4.29141156299998));
#331074=CARTESIAN_POINT('Ctrl Pts',(-0.788741523000055,12.2,4.29303317699999));
#331075=CARTESIAN_POINT('Ctrl Pts',(-0.788741523000055,5.2,4.29303317699999));
#331076=CARTESIAN_POINT('Ctrl Pts',(-0.788741523000055,2.2,4.29303317699999));
#331077=CARTESIAN_POINT('Ctrl Pts',(-0.789846815000056,12.2,4.29465696599999));
#331078=CARTESIAN_POINT('Ctrl Pts',(-0.789846815000056,5.2,4.29465696599999));
#331079=CARTESIAN_POINT('Ctrl Pts',(-0.789846815000056,2.2,4.29465696599999));
#331080=CARTESIAN_POINT('Ctrl Pts',(-0.790956233000056,12.2,4.29628292199999));
#331081=CARTESIAN_POINT('Ctrl Pts',(-0.790956233000056,5.2,4.29628292199999));
#331082=CARTESIAN_POINT('Ctrl Pts',(-0.790956233000056,2.2,4.29628292199999));
#331083=CARTESIAN_POINT('Ctrl Pts',(-0.792069779000055,12.2,4.29791103299999));
#331084=CARTESIAN_POINT('Ctrl Pts',(-0.792069779000055,5.2,4.29791103299999));
#331085=CARTESIAN_POINT('Ctrl Pts',(-0.792069779000055,2.2,4.29791103299999));
#331086=CARTESIAN_POINT('Ctrl Pts',(-0.793187456000056,12.2,4.29954128799999));
#331087=CARTESIAN_POINT('Ctrl Pts',(-0.793187456000056,5.2,4.29954128799999));
#331088=CARTESIAN_POINT('Ctrl Pts',(-0.793187456000056,2.2,4.29954128799999));
#331089=CARTESIAN_POINT('Ctrl Pts',(-0.794309268000056,12.2,4.30117367699999));
#331090=CARTESIAN_POINT('Ctrl Pts',(-0.794309268000056,5.2,4.30117367699999));
#331091=CARTESIAN_POINT('Ctrl Pts',(-0.794309268000056,2.2,4.30117367699999));
#331092=CARTESIAN_POINT('Ctrl Pts',(-0.795435215000057,12.2,4.30280818899998));
#331093=CARTESIAN_POINT('Ctrl Pts',(-0.795435215000057,5.2,4.30280818899998));
#331094=CARTESIAN_POINT('Ctrl Pts',(-0.795435215000057,2.2,4.30280818899998));
#331095=CARTESIAN_POINT('Ctrl Pts',(-0.796565301000056,12.2,4.30444481399999));
#331096=CARTESIAN_POINT('Ctrl Pts',(-0.796565301000056,5.2,4.30444481399999));
#331097=CARTESIAN_POINT('Ctrl Pts',(-0.796565301000056,2.2,4.30444481399999));
#331098=CARTESIAN_POINT('Ctrl Pts',(-0.797699528000055,12.2,4.30608354099999));
#331099=CARTESIAN_POINT('Ctrl Pts',(-0.797699528000055,5.2,4.30608354099999));
#331100=CARTESIAN_POINT('Ctrl Pts',(-0.797699528000055,2.2,4.30608354099999));
#331101=CARTESIAN_POINT('Ctrl Pts',(-0.798837899000056,12.2,4.30772435899998));
#331102=CARTESIAN_POINT('Ctrl Pts',(-0.798837899000056,5.2,4.30772435899998));
#331103=CARTESIAN_POINT('Ctrl Pts',(-0.798837899000056,2.2,4.30772435899998));
#331104=CARTESIAN_POINT('Ctrl Pts',(-0.799980417000056,12.2,4.30936725799998));
#331105=CARTESIAN_POINT('Ctrl Pts',(-0.799980417000056,5.2,4.30936725799998));
#331106=CARTESIAN_POINT('Ctrl Pts',(-0.799980417000056,2.2,4.30936725799998));
#331107=CARTESIAN_POINT('Ctrl Pts',(-0.801127083000056,12.2,4.31101222699999));
#331108=CARTESIAN_POINT('Ctrl Pts',(-0.801127083000056,5.2,4.31101222699999));
#331109=CARTESIAN_POINT('Ctrl Pts',(-0.801127083000056,2.2,4.31101222699999));
#331110=CARTESIAN_POINT('Ctrl Pts',(-0.802277901000057,12.2,4.31265925599998));
#331111=CARTESIAN_POINT('Ctrl Pts',(-0.802277901000057,5.2,4.31265925599998));
#331112=CARTESIAN_POINT('Ctrl Pts',(-0.802277901000057,2.2,4.31265925599998));
#331113=CARTESIAN_POINT('Ctrl Pts',(-0.803432873000055,12.2,4.31430833399999));
#331114=CARTESIAN_POINT('Ctrl Pts',(-0.803432873000055,5.2,4.31430833399999));
#331115=CARTESIAN_POINT('Ctrl Pts',(-0.803432873000055,2.2,4.31430833399999));
#331116=CARTESIAN_POINT('Ctrl Pts',(-0.804592000000056,12.2,4.31595944899998));
#331117=CARTESIAN_POINT('Ctrl Pts',(-0.804592000000056,5.2,4.31595944899998));
#331118=CARTESIAN_POINT('Ctrl Pts',(-0.804592000000056,2.2,4.31595944899998));
#331119=CARTESIAN_POINT('Ctrl Pts',(-0.805755288000055,12.2,4.31761259299999));
#331120=CARTESIAN_POINT('Ctrl Pts',(-0.805755288000055,5.2,4.31761259299999));
#331121=CARTESIAN_POINT('Ctrl Pts',(-0.805755288000055,2.2,4.31761259299999));
#331122=CARTESIAN_POINT('Ctrl Pts',(-0.806922735000055,12.2,4.31926775499999));
#331123=CARTESIAN_POINT('Ctrl Pts',(-0.806922735000055,5.2,4.31926775499999));
#331124=CARTESIAN_POINT('Ctrl Pts',(-0.806922735000055,2.2,4.31926775499999));
#331125=CARTESIAN_POINT('Ctrl Pts',(-0.808094347000056,12.2,4.32092492399998));
#331126=CARTESIAN_POINT('Ctrl Pts',(-0.808094347000056,5.2,4.32092492399998));
#331127=CARTESIAN_POINT('Ctrl Pts',(-0.808094347000056,2.2,4.32092492399998));
#331128=CARTESIAN_POINT('Ctrl Pts',(-0.809270125000056,12.2,4.32258408799999));
#331129=CARTESIAN_POINT('Ctrl Pts',(-0.809270125000056,5.2,4.32258408799999));
#331130=CARTESIAN_POINT('Ctrl Pts',(-0.809270125000056,2.2,4.32258408799999));
#331131=CARTESIAN_POINT('Ctrl Pts',(-0.810450070000056,12.2,4.32424523999998));
#331132=CARTESIAN_POINT('Ctrl Pts',(-0.810450070000056,5.2,4.32424523999998));
#331133=CARTESIAN_POINT('Ctrl Pts',(-0.810450070000056,2.2,4.32424523999998));
#331134=CARTESIAN_POINT('Ctrl Pts',(-0.811634187000055,12.2,4.32590836599999));
#331135=CARTESIAN_POINT('Ctrl Pts',(-0.811634187000055,5.2,4.32590836599999));
#331136=CARTESIAN_POINT('Ctrl Pts',(-0.811634187000055,2.2,4.32590836599999));
#331137=CARTESIAN_POINT('Ctrl Pts',(-0.812822475000056,12.2,4.32757345699999));
#331138=CARTESIAN_POINT('Ctrl Pts',(-0.812822475000056,5.2,4.32757345699999));
#331139=CARTESIAN_POINT('Ctrl Pts',(-0.812822475000056,2.2,4.32757345699999));
#331140=CARTESIAN_POINT('Ctrl Pts',(-0.814014940000056,12.2,4.32924050299999));
#331141=CARTESIAN_POINT('Ctrl Pts',(-0.814014940000056,5.2,4.32924050299999));
#331142=CARTESIAN_POINT('Ctrl Pts',(-0.814014940000056,2.2,4.32924050299999));
#331143=CARTESIAN_POINT('Ctrl Pts',(-0.815211583000056,12.2,4.33090949299999));
#331144=CARTESIAN_POINT('Ctrl Pts',(-0.815211583000056,5.2,4.33090949299999));
#331145=CARTESIAN_POINT('Ctrl Pts',(-0.815211583000056,2.2,4.33090949299999));
#331146=CARTESIAN_POINT('Ctrl Pts',(-0.816412405000057,12.2,4.33258041699998));
#331147=CARTESIAN_POINT('Ctrl Pts',(-0.816412405000057,5.2,4.33258041699998));
#331148=CARTESIAN_POINT('Ctrl Pts',(-0.816412405000057,2.2,4.33258041699998));
#331149=CARTESIAN_POINT('Ctrl Pts',(-0.817617408000055,12.2,4.33425326399998));
#331150=CARTESIAN_POINT('Ctrl Pts',(-0.817617408000055,5.2,4.33425326399998));
#331151=CARTESIAN_POINT('Ctrl Pts',(-0.817617408000055,2.2,4.33425326399998));
#331152=CARTESIAN_POINT('Ctrl Pts',(-0.818826596000056,12.2,4.33592802399998));
#331153=CARTESIAN_POINT('Ctrl Pts',(-0.818826596000056,5.2,4.33592802399998));
#331154=CARTESIAN_POINT('Ctrl Pts',(-0.818826596000056,2.2,4.33592802399998));
#331155=CARTESIAN_POINT('Ctrl Pts',(-0.820039971000056,12.2,4.33760468699998));
#331156=CARTESIAN_POINT('Ctrl Pts',(-0.820039971000056,5.2,4.33760468699998));
#331157=CARTESIAN_POINT('Ctrl Pts',(-0.820039971000056,2.2,4.33760468699998));
#331158=CARTESIAN_POINT('Ctrl Pts',(-0.821257535000056,12.2,4.33928324199999));
#331159=CARTESIAN_POINT('Ctrl Pts',(-0.821257535000056,5.2,4.33928324199999));
#331160=CARTESIAN_POINT('Ctrl Pts',(-0.821257535000056,2.2,4.33928324199999));
#331161=CARTESIAN_POINT('Ctrl Pts',(-0.822479289000055,12.2,4.34096367899999));
#331162=CARTESIAN_POINT('Ctrl Pts',(-0.822479289000055,5.2,4.34096367899999));
#331163=CARTESIAN_POINT('Ctrl Pts',(-0.822479289000055,2.2,4.34096367899999));
#331164=CARTESIAN_POINT('Ctrl Pts',(-0.823705236000055,12.2,4.34264598699999));
#331165=CARTESIAN_POINT('Ctrl Pts',(-0.823705236000055,5.2,4.34264598699999));
#331166=CARTESIAN_POINT('Ctrl Pts',(-0.823705236000055,2.2,4.34264598699999));
#331167=CARTESIAN_POINT('Ctrl Pts',(-0.824935379000056,12.2,4.34433015699998));
#331168=CARTESIAN_POINT('Ctrl Pts',(-0.824935379000056,5.2,4.34433015699998));
#331169=CARTESIAN_POINT('Ctrl Pts',(-0.824935379000056,2.2,4.34433015699998));
#331170=CARTESIAN_POINT('Ctrl Pts',(-0.826169719000056,12.2,4.34601617799999));
#331171=CARTESIAN_POINT('Ctrl Pts',(-0.826169719000056,5.2,4.34601617799999));
#331172=CARTESIAN_POINT('Ctrl Pts',(-0.826169719000056,2.2,4.34601617799999));
#331173=CARTESIAN_POINT('Ctrl Pts',(-0.827408258000055,12.2,4.34770403899999));
#331174=CARTESIAN_POINT('Ctrl Pts',(-0.827408258000055,5.2,4.34770403899999));
#331175=CARTESIAN_POINT('Ctrl Pts',(-0.827408258000055,2.2,4.34770403899999));
#331176=CARTESIAN_POINT('Ctrl Pts',(-0.828650998000056,12.2,4.34939372999998));
#331177=CARTESIAN_POINT('Ctrl Pts',(-0.828650998000056,5.2,4.34939372999998));
#331178=CARTESIAN_POINT('Ctrl Pts',(-0.828650998000056,2.2,4.34939372999998));
#331179=CARTESIAN_POINT('Ctrl Pts',(-0.829897943000055,12.2,4.35108524199999));
#331180=CARTESIAN_POINT('Ctrl Pts',(-0.829897943000055,5.2,4.35108524199999));
#331181=CARTESIAN_POINT('Ctrl Pts',(-0.829897943000055,2.2,4.35108524199999));
#331182=CARTESIAN_POINT('Ctrl Pts',(-0.831149093000055,12.2,4.35277856399999));
#331183=CARTESIAN_POINT('Ctrl Pts',(-0.831149093000055,5.2,4.35277856399999));
#331184=CARTESIAN_POINT('Ctrl Pts',(-0.831149093000055,2.2,4.35277856399999));
#331185=CARTESIAN_POINT('Ctrl Pts',(-0.832404451000055,12.2,4.35447368499998));
#331186=CARTESIAN_POINT('Ctrl Pts',(-0.832404451000055,5.2,4.35447368499998));
#331187=CARTESIAN_POINT('Ctrl Pts',(-0.832404451000055,2.2,4.35447368499998));
#331188=CARTESIAN_POINT('Ctrl Pts',(-0.833664018000055,12.2,4.35617059399998));
#331189=CARTESIAN_POINT('Ctrl Pts',(-0.833664018000055,5.2,4.35617059399998));
#331190=CARTESIAN_POINT('Ctrl Pts',(-0.833664018000055,2.2,4.35617059399998));
#331191=CARTESIAN_POINT('Ctrl Pts',(-0.834927797000056,12.2,4.35786928399998));
#331192=CARTESIAN_POINT('Ctrl Pts',(-0.834927797000056,5.2,4.35786928399998));
#331193=CARTESIAN_POINT('Ctrl Pts',(-0.834927797000056,2.2,4.35786928399998));
#331194=CARTESIAN_POINT('Ctrl Pts',(-0.836195790000056,12.2,4.35956974299998));
#331195=CARTESIAN_POINT('Ctrl Pts',(-0.836195790000056,5.2,4.35956974299998));
#331196=CARTESIAN_POINT('Ctrl Pts',(-0.836195790000056,2.2,4.35956974299998));
#331197=CARTESIAN_POINT('Ctrl Pts',(-0.837467999000056,12.2,4.36127195899999));
#331198=CARTESIAN_POINT('Ctrl Pts',(-0.837467999000056,5.2,4.36127195899999));
#331199=CARTESIAN_POINT('Ctrl Pts',(-0.837467999000056,2.2,4.36127195899999));
#331200=CARTESIAN_POINT('Ctrl Pts',(-0.838744426000056,12.2,4.36297592499999));
#331201=CARTESIAN_POINT('Ctrl Pts',(-0.838744426000056,5.2,4.36297592499999));
#331202=CARTESIAN_POINT('Ctrl Pts',(-0.838744426000056,2.2,4.36297592499999));
#331203=CARTESIAN_POINT('Ctrl Pts',(-0.840025071000056,12.2,4.36468162899998));
#331204=CARTESIAN_POINT('Ctrl Pts',(-0.840025071000056,5.2,4.36468162899998));
#331205=CARTESIAN_POINT('Ctrl Pts',(-0.840025071000056,2.2,4.36468162899998));
#331206=CARTESIAN_POINT('Ctrl Pts',(-0.841309938000055,12.2,4.36638906199998));
#331207=CARTESIAN_POINT('Ctrl Pts',(-0.841309938000055,5.2,4.36638906199998));
#331208=CARTESIAN_POINT('Ctrl Pts',(-0.841309938000055,2.2,4.36638906199998));
#331209=CARTESIAN_POINT('Ctrl Pts',(-0.842599029000055,12.2,4.36809821199999));
#331210=CARTESIAN_POINT('Ctrl Pts',(-0.842599029000055,5.2,4.36809821199999));
#331211=CARTESIAN_POINT('Ctrl Pts',(-0.842599029000055,2.2,4.36809821199999));
#331212=CARTESIAN_POINT('Ctrl Pts',(-0.843892345000056,12.2,4.36980906999998));
#331213=CARTESIAN_POINT('Ctrl Pts',(-0.843892345000056,5.2,4.36980906999998));
#331214=CARTESIAN_POINT('Ctrl Pts',(-0.843892345000056,2.2,4.36980906999998));
#331215=CARTESIAN_POINT('Ctrl Pts',(-0.845189888000055,12.2,4.37152162599999));
#331216=CARTESIAN_POINT('Ctrl Pts',(-0.845189888000055,5.2,4.37152162599999));
#331217=CARTESIAN_POINT('Ctrl Pts',(-0.845189888000055,2.2,4.37152162599999));
#331218=CARTESIAN_POINT('Ctrl Pts',(-0.846491661000056,12.2,4.37323586999998));
#331219=CARTESIAN_POINT('Ctrl Pts',(-0.846491661000056,5.2,4.37323586999998));
#331220=CARTESIAN_POINT('Ctrl Pts',(-0.846491661000056,2.2,4.37323586999998));
#331221=CARTESIAN_POINT('Ctrl Pts',(-0.847797664000056,12.2,4.37495179199999));
#331222=CARTESIAN_POINT('Ctrl Pts',(-0.847797664000056,5.2,4.37495179199999));
#331223=CARTESIAN_POINT('Ctrl Pts',(-0.847797664000056,2.2,4.37495179199999));
#331224=CARTESIAN_POINT('Ctrl Pts',(-0.849107900000057,12.2,4.37666937999998));
#331225=CARTESIAN_POINT('Ctrl Pts',(-0.849107900000057,5.2,4.37666937999998));
#331226=CARTESIAN_POINT('Ctrl Pts',(-0.849107900000057,2.2,4.37666937999998));
#331227=CARTESIAN_POINT('Ctrl Pts',(-0.850422370000056,12.2,4.37838862699999));
#331228=CARTESIAN_POINT('Ctrl Pts',(-0.850422370000056,5.2,4.37838862699999));
#331229=CARTESIAN_POINT('Ctrl Pts',(-0.850422370000056,2.2,4.37838862699999));
#331230=CARTESIAN_POINT('Ctrl Pts',(-0.851741076000057,12.2,4.38010951999999));
#331231=CARTESIAN_POINT('Ctrl Pts',(-0.851741076000057,5.2,4.38010951999999));
#331232=CARTESIAN_POINT('Ctrl Pts',(-0.851741076000057,2.2,4.38010951999999));
#331233=CARTESIAN_POINT('Ctrl Pts',(-0.853064021000056,12.2,4.38183205199999));
#331234=CARTESIAN_POINT('Ctrl Pts',(-0.853064021000056,5.2,4.38183205199999));
#331235=CARTESIAN_POINT('Ctrl Pts',(-0.853064021000056,2.2,4.38183205199999));
#331236=CARTESIAN_POINT('Ctrl Pts',(-0.854391206000056,12.2,4.38355620999998));
#331237=CARTESIAN_POINT('Ctrl Pts',(-0.854391206000056,5.2,4.38355620999998));
#331238=CARTESIAN_POINT('Ctrl Pts',(-0.854391206000056,2.2,4.38355620999998));
#331239=CARTESIAN_POINT('Ctrl Pts',(-0.855722632000055,12.2,4.38528198599998));
#331240=CARTESIAN_POINT('Ctrl Pts',(-0.855722632000055,5.2,4.38528198599998));
#331241=CARTESIAN_POINT('Ctrl Pts',(-0.855722632000055,2.2,4.38528198599998));
#331242=CARTESIAN_POINT('Ctrl Pts',(-0.857058301000055,12.2,4.38700936899998));
#331243=CARTESIAN_POINT('Ctrl Pts',(-0.857058301000055,5.2,4.38700936899998));
#331244=CARTESIAN_POINT('Ctrl Pts',(-0.857058301000055,2.2,4.38700936899998));
#331245=CARTESIAN_POINT('Ctrl Pts',(-0.858398215000056,12.2,4.38873834899999));
#331246=CARTESIAN_POINT('Ctrl Pts',(-0.858398215000056,5.2,4.38873834899999));
#331247=CARTESIAN_POINT('Ctrl Pts',(-0.858398215000056,2.2,4.38873834899999));
#331248=CARTESIAN_POINT('Ctrl Pts',(-0.859742376000057,12.2,4.39046891699999));
#331249=CARTESIAN_POINT('Ctrl Pts',(-0.859742376000057,5.2,4.39046891699999));
#331250=CARTESIAN_POINT('Ctrl Pts',(-0.859742376000057,2.2,4.39046891699999));
#331251=CARTESIAN_POINT('Ctrl Pts',(-0.861090785000057,12.2,4.39220106199999));
#331252=CARTESIAN_POINT('Ctrl Pts',(-0.861090785000057,5.2,4.39220106199999));
#331253=CARTESIAN_POINT('Ctrl Pts',(-0.861090785000057,2.2,4.39220106199999));
#331254=CARTESIAN_POINT('Ctrl Pts',(-0.862443445000055,12.2,4.39393477399998));
#331255=CARTESIAN_POINT('Ctrl Pts',(-0.862443445000055,5.2,4.39393477399998));
#331256=CARTESIAN_POINT('Ctrl Pts',(-0.862443445000055,2.2,4.39393477399998));
#331257=CARTESIAN_POINT('Ctrl Pts',(-0.863800356000055,12.2,4.39567004399999));
#331258=CARTESIAN_POINT('Ctrl Pts',(-0.863800356000055,5.2,4.39567004399999));
#331259=CARTESIAN_POINT('Ctrl Pts',(-0.863800356000055,2.2,4.39567004399999));
#331260=CARTESIAN_POINT('Ctrl Pts',(-0.865161520000056,12.2,4.39740686199999));
#331261=CARTESIAN_POINT('Ctrl Pts',(-0.865161520000056,5.2,4.39740686199999));
#331262=CARTESIAN_POINT('Ctrl Pts',(-0.865161520000056,2.2,4.39740686199999));
#331263=CARTESIAN_POINT('Ctrl Pts',(-0.866526939000056,12.2,4.39914521599999));
#331264=CARTESIAN_POINT('Ctrl Pts',(-0.866526939000056,5.2,4.39914521599999));
#331265=CARTESIAN_POINT('Ctrl Pts',(-0.866526939000056,2.2,4.39914521599999));
#331266=CARTESIAN_POINT('Ctrl Pts',(-0.867896616000056,12.2,4.40088509899999));
#331267=CARTESIAN_POINT('Ctrl Pts',(-0.867896616000056,5.2,4.40088509899999));
#331268=CARTESIAN_POINT('Ctrl Pts',(-0.867896616000056,2.2,4.40088509899999));
#331269=CARTESIAN_POINT('Ctrl Pts',(-0.869270549000056,12.2,4.40262649999998));
#331270=CARTESIAN_POINT('Ctrl Pts',(-0.869270549000056,5.2,4.40262649999998));
#331271=CARTESIAN_POINT('Ctrl Pts',(-0.869270549000056,2.2,4.40262649999998));
#331272=CARTESIAN_POINT('Ctrl Pts',(-0.870648743000055,12.2,4.40436940799999));
#331273=CARTESIAN_POINT('Ctrl Pts',(-0.870648743000055,5.2,4.40436940799999));
#331274=CARTESIAN_POINT('Ctrl Pts',(-0.870648743000055,2.2,4.40436940799999));
#331275=CARTESIAN_POINT('Ctrl Pts',(-0.872031197000057,12.2,4.40611381399999));
#331276=CARTESIAN_POINT('Ctrl Pts',(-0.872031197000057,5.2,4.40611381399999));
#331277=CARTESIAN_POINT('Ctrl Pts',(-0.872031197000057,2.2,4.40611381399999));
#331278=CARTESIAN_POINT('Ctrl Pts',(-0.873417915000055,12.2,4.40785970899999));
#331279=CARTESIAN_POINT('Ctrl Pts',(-0.873417915000055,5.2,4.40785970899999));
#331280=CARTESIAN_POINT('Ctrl Pts',(-0.873417915000055,2.2,4.40785970899999));
#331281=CARTESIAN_POINT('Ctrl Pts',(-0.874808897000056,12.2,4.40960708199999));
#331282=CARTESIAN_POINT('Ctrl Pts',(-0.874808897000056,5.2,4.40960708199999));
#331283=CARTESIAN_POINT('Ctrl Pts',(-0.874808897000056,2.2,4.40960708199999));
#331284=CARTESIAN_POINT('Ctrl Pts',(-0.876204144000056,12.2,4.41135592299998));
#331285=CARTESIAN_POINT('Ctrl Pts',(-0.876204144000056,5.2,4.41135592299998));
#331286=CARTESIAN_POINT('Ctrl Pts',(-0.876204144000056,2.2,4.41135592299998));
#331287=CARTESIAN_POINT('Ctrl Pts',(-0.877603659000057,12.2,4.41310622299999));
#331288=CARTESIAN_POINT('Ctrl Pts',(-0.877603659000057,5.2,4.41310622299999));
#331289=CARTESIAN_POINT('Ctrl Pts',(-0.877603659000057,2.2,4.41310622299999));
#331290=CARTESIAN_POINT('Ctrl Pts',(-0.879007443000056,12.2,4.41485797199999));
#331291=CARTESIAN_POINT('Ctrl Pts',(-0.879007443000056,5.2,4.41485797199999));
#331292=CARTESIAN_POINT('Ctrl Pts',(-0.879007443000056,2.2,4.41485797199999));
#331293=CARTESIAN_POINT('Ctrl Pts',(-0.880415495000056,12.2,4.41661115999998));
#331294=CARTESIAN_POINT('Ctrl Pts',(-0.880415495000056,5.2,4.41661115999998));
#331295=CARTESIAN_POINT('Ctrl Pts',(-0.880415495000056,2.2,4.41661115999998));
#331296=CARTESIAN_POINT('Ctrl Pts',(-0.881827821000056,12.2,4.41836577599998));
#331297=CARTESIAN_POINT('Ctrl Pts',(-0.881827821000056,5.2,4.41836577599998));
#331298=CARTESIAN_POINT('Ctrl Pts',(-0.881827821000056,2.2,4.41836577599998));
#331299=CARTESIAN_POINT('Ctrl Pts',(-0.883244419000055,12.2,4.42012181299998));
#331300=CARTESIAN_POINT('Ctrl Pts',(-0.883244419000055,5.2,4.42012181299998));
#331301=CARTESIAN_POINT('Ctrl Pts',(-0.883244419000055,2.2,4.42012181299998));
#331302=CARTESIAN_POINT('Ctrl Pts',(-0.884665291000056,12.2,4.42187925899999));
#331303=CARTESIAN_POINT('Ctrl Pts',(-0.884665291000056,5.2,4.42187925899999));
#331304=CARTESIAN_POINT('Ctrl Pts',(-0.884665291000056,2.2,4.42187925899999));
#331305=CARTESIAN_POINT('Ctrl Pts',(-0.886090440000055,12.2,4.42363810499998));
#331306=CARTESIAN_POINT('Ctrl Pts',(-0.886090440000055,5.2,4.42363810499998));
#331307=CARTESIAN_POINT('Ctrl Pts',(-0.886090440000055,2.2,4.42363810499998));
#331308=CARTESIAN_POINT('Ctrl Pts',(-0.887519865000056,12.2,4.42539834199999));
#331309=CARTESIAN_POINT('Ctrl Pts',(-0.887519865000056,5.2,4.42539834199999));
#331310=CARTESIAN_POINT('Ctrl Pts',(-0.887519865000056,2.2,4.42539834199999));
#331311=CARTESIAN_POINT('Ctrl Pts',(-0.888953570000056,12.2,4.42715995899999));
#331312=CARTESIAN_POINT('Ctrl Pts',(-0.888953570000056,5.2,4.42715995899999));
#331313=CARTESIAN_POINT('Ctrl Pts',(-0.888953570000056,2.2,4.42715995899999));
#331314=CARTESIAN_POINT('Ctrl Pts',(-0.890391553000055,12.2,4.42892294599999));
#331315=CARTESIAN_POINT('Ctrl Pts',(-0.890391553000055,5.2,4.42892294599999));
#331316=CARTESIAN_POINT('Ctrl Pts',(-0.890391553000055,2.2,4.42892294599999));
#331317=CARTESIAN_POINT('Ctrl Pts',(-0.891833819000055,12.2,4.43068729499998));
#331318=CARTESIAN_POINT('Ctrl Pts',(-0.891833819000055,5.2,4.43068729499998));
#331319=CARTESIAN_POINT('Ctrl Pts',(-0.891833819000055,2.2,4.43068729499998));
#331320=CARTESIAN_POINT('Ctrl Pts',(-0.893280366000055,12.2,4.43245299399998));
#331321=CARTESIAN_POINT('Ctrl Pts',(-0.893280366000055,5.2,4.43245299399998));
#331322=CARTESIAN_POINT('Ctrl Pts',(-0.893280366000055,2.2,4.43245299399998));
#331323=CARTESIAN_POINT('Ctrl Pts',(-0.894731198000055,12.2,4.43422003599999));
#331324=CARTESIAN_POINT('Ctrl Pts',(-0.894731198000055,5.2,4.43422003599999));
#331325=CARTESIAN_POINT('Ctrl Pts',(-0.894731198000055,2.2,4.43422003599999));
#331326=CARTESIAN_POINT('Ctrl Pts',(-0.896186315000056,12.2,4.43598840999999));
#331327=CARTESIAN_POINT('Ctrl Pts',(-0.896186315000056,5.2,4.43598840999999));
#331328=CARTESIAN_POINT('Ctrl Pts',(-0.896186315000056,2.2,4.43598840999999));
#331329=CARTESIAN_POINT('Ctrl Pts',(-0.897645718000056,12.2,4.43775810499999));
#331330=CARTESIAN_POINT('Ctrl Pts',(-0.897645718000056,5.2,4.43775810499999));
#331331=CARTESIAN_POINT('Ctrl Pts',(-0.897645718000056,2.2,4.43775810499999));
#331332=CARTESIAN_POINT('Ctrl Pts',(-0.899109409000056,12.2,4.43952911299998));
#331333=CARTESIAN_POINT('Ctrl Pts',(-0.899109409000056,5.2,4.43952911299998));
#331334=CARTESIAN_POINT('Ctrl Pts',(-0.899109409000056,2.2,4.43952911299998));
#331335=CARTESIAN_POINT('Ctrl Pts',(-0.900577389000056,12.2,4.44130142499999));
#331336=CARTESIAN_POINT('Ctrl Pts',(-0.900577389000056,5.2,4.44130142499999));
#331337=CARTESIAN_POINT('Ctrl Pts',(-0.900577389000056,2.2,4.44130142499999));
#331338=CARTESIAN_POINT('Ctrl Pts',(-0.902049660000056,12.2,4.44307502999998));
#331339=CARTESIAN_POINT('Ctrl Pts',(-0.902049660000056,5.2,4.44307502999998));
#331340=CARTESIAN_POINT('Ctrl Pts',(-0.902049660000056,2.2,4.44307502999998));
#331341=CARTESIAN_POINT('Ctrl Pts',(-0.903526221000056,12.2,4.44484991899999));
#331342=CARTESIAN_POINT('Ctrl Pts',(-0.903526221000056,5.2,4.44484991899999));
#331343=CARTESIAN_POINT('Ctrl Pts',(-0.903526221000056,2.2,4.44484991899999));
#331344=CARTESIAN_POINT('Ctrl Pts',(-0.905007075000055,12.2,4.44662608099998));
#331345=CARTESIAN_POINT('Ctrl Pts',(-0.905007075000055,5.2,4.44662608099998));
#331346=CARTESIAN_POINT('Ctrl Pts',(-0.905007075000055,2.2,4.44662608099998));
#331347=CARTESIAN_POINT('Ctrl Pts',(-0.906492222000056,12.2,4.44840350899998));
#331348=CARTESIAN_POINT('Ctrl Pts',(-0.906492222000056,5.2,4.44840350899998));
#331349=CARTESIAN_POINT('Ctrl Pts',(-0.906492222000056,2.2,4.44840350899998));
#331350=CARTESIAN_POINT('Ctrl Pts',(-0.907981665000056,12.2,4.45018219199999));
#331351=CARTESIAN_POINT('Ctrl Pts',(-0.907981665000056,5.2,4.45018219199999));
#331352=CARTESIAN_POINT('Ctrl Pts',(-0.907981665000056,2.2,4.45018219199999));
#331353=CARTESIAN_POINT('Ctrl Pts',(-0.909475403000056,12.2,4.45196211899999));
#331354=CARTESIAN_POINT('Ctrl Pts',(-0.909475403000056,5.2,4.45196211899999));
#331355=CARTESIAN_POINT('Ctrl Pts',(-0.909475403000056,2.2,4.45196211899999));
#331356=CARTESIAN_POINT('Ctrl Pts',(-0.910973439000056,12.2,4.45374328299999));
#331357=CARTESIAN_POINT('Ctrl Pts',(-0.910973439000056,5.2,4.45374328299999));
#331358=CARTESIAN_POINT('Ctrl Pts',(-0.910973439000056,2.2,4.45374328299999));
#331359=CARTESIAN_POINT('Ctrl Pts',(-0.912475773000055,12.2,4.45552567399999));
#331360=CARTESIAN_POINT('Ctrl Pts',(-0.912475773000055,5.2,4.45552567399999));
#331361=CARTESIAN_POINT('Ctrl Pts',(-0.912475773000055,2.2,4.45552567399999));
#331362=CARTESIAN_POINT('Ctrl Pts',(-0.913982407000056,12.2,4.45730928099999));
#331363=CARTESIAN_POINT('Ctrl Pts',(-0.913982407000056,5.2,4.45730928099999));
#331364=CARTESIAN_POINT('Ctrl Pts',(-0.913982407000056,2.2,4.45730928099999));
#331365=CARTESIAN_POINT('Ctrl Pts',(-0.915493341000057,12.2,4.45909409499999));
#331366=CARTESIAN_POINT('Ctrl Pts',(-0.915493341000057,5.2,4.45909409499999));
#331367=CARTESIAN_POINT('Ctrl Pts',(-0.915493341000057,2.2,4.45909409499999));
#331368=CARTESIAN_POINT('Ctrl Pts',(-0.917008577000056,12.2,4.46088010699999));
#331369=CARTESIAN_POINT('Ctrl Pts',(-0.917008577000056,5.2,4.46088010699999));
#331370=CARTESIAN_POINT('Ctrl Pts',(-0.917008577000056,2.2,4.46088010699999));
#331371=CARTESIAN_POINT('Ctrl Pts',(-0.918528116000056,12.2,4.46266730699998));
#331372=CARTESIAN_POINT('Ctrl Pts',(-0.918528116000056,5.2,4.46266730699998));
#331373=CARTESIAN_POINT('Ctrl Pts',(-0.918528116000056,2.2,4.46266730699998));
#331374=CARTESIAN_POINT('Ctrl Pts',(-0.920051957000056,12.2,4.46445568599999));
#331375=CARTESIAN_POINT('Ctrl Pts',(-0.920051957000056,5.2,4.46445568599999));
#331376=CARTESIAN_POINT('Ctrl Pts',(-0.920051957000056,2.2,4.46445568599999));
#331377=CARTESIAN_POINT('Ctrl Pts',(-0.921580104000055,12.2,4.46624523499998));
#331378=CARTESIAN_POINT('Ctrl Pts',(-0.921580104000055,5.2,4.46624523499998));
#331379=CARTESIAN_POINT('Ctrl Pts',(-0.921580104000055,2.2,4.46624523499998));
#331380=CARTESIAN_POINT('Ctrl Pts',(-0.923112557000056,12.2,4.46803594299999));
#331381=CARTESIAN_POINT('Ctrl Pts',(-0.923112557000056,5.2,4.46803594299999));
#331382=CARTESIAN_POINT('Ctrl Pts',(-0.923112557000056,2.2,4.46803594299999));
#331383=CARTESIAN_POINT('Ctrl Pts',(-0.924649317000057,12.2,4.46982780199999));
#331384=CARTESIAN_POINT('Ctrl Pts',(-0.924649317000057,5.2,4.46982780199999));
#331385=CARTESIAN_POINT('Ctrl Pts',(-0.924649317000057,2.2,4.46982780199999));
#331386=CARTESIAN_POINT('Ctrl Pts',(-0.926190383000056,12.2,4.47162080099999));
#331387=CARTESIAN_POINT('Ctrl Pts',(-0.926190383000056,5.2,4.47162080099999));
#331388=CARTESIAN_POINT('Ctrl Pts',(-0.926190383000056,2.2,4.47162080099999));
#331389=CARTESIAN_POINT('Ctrl Pts',(-0.927735760000056,12.2,4.47341493299999));
#331390=CARTESIAN_POINT('Ctrl Pts',(-0.927735760000056,5.2,4.47341493299999));
#331391=CARTESIAN_POINT('Ctrl Pts',(-0.927735760000056,2.2,4.47341493299999));
#331392=CARTESIAN_POINT('Ctrl Pts',(-0.929285445000056,12.2,4.47521018599998));
#331393=CARTESIAN_POINT('Ctrl Pts',(-0.929285445000056,5.2,4.47521018599998));
#331394=CARTESIAN_POINT('Ctrl Pts',(-0.929285445000056,2.2,4.47521018599998));
#331395=CARTESIAN_POINT('Ctrl Pts',(-0.930839442000057,12.2,4.47700655099998));
#331396=CARTESIAN_POINT('Ctrl Pts',(-0.930839442000057,5.2,4.47700655099998));
#331397=CARTESIAN_POINT('Ctrl Pts',(-0.930839442000057,2.2,4.47700655099998));
#331398=CARTESIAN_POINT('Ctrl Pts',(-0.932397750000057,12.2,4.47880401999999));
#331399=CARTESIAN_POINT('Ctrl Pts',(-0.932397750000057,5.2,4.47880401999999));
#331400=CARTESIAN_POINT('Ctrl Pts',(-0.932397750000057,2.2,4.47880401999999));
#331401=CARTESIAN_POINT('Ctrl Pts',(-0.933960370000056,12.2,4.48060258399998));
#331402=CARTESIAN_POINT('Ctrl Pts',(-0.933960370000056,5.2,4.48060258399998));
#331403=CARTESIAN_POINT('Ctrl Pts',(-0.933960370000056,2.2,4.48060258399998));
#331404=CARTESIAN_POINT('Ctrl Pts',(-0.935527304000056,12.2,4.48240223099998));
#331405=CARTESIAN_POINT('Ctrl Pts',(-0.935527304000056,5.2,4.48240223099998));
#331406=CARTESIAN_POINT('Ctrl Pts',(-0.935527304000056,2.2,4.48240223099998));
#331407=CARTESIAN_POINT('Ctrl Pts',(-0.937098553000055,12.2,4.48420295299999));
#331408=CARTESIAN_POINT('Ctrl Pts',(-0.937098553000055,5.2,4.48420295299999));
#331409=CARTESIAN_POINT('Ctrl Pts',(-0.937098553000055,2.2,4.48420295299999));
#331410=CARTESIAN_POINT('Ctrl Pts',(-0.938674116000057,12.2,4.48600474199999));
#331411=CARTESIAN_POINT('Ctrl Pts',(-0.938674116000057,5.2,4.48600474199999));
#331412=CARTESIAN_POINT('Ctrl Pts',(-0.938674116000057,2.2,4.48600474199999));
#331413=CARTESIAN_POINT('Ctrl Pts',(-0.940253996000056,12.2,4.48780758699999));
#331414=CARTESIAN_POINT('Ctrl Pts',(-0.940253996000056,5.2,4.48780758699999));
#331415=CARTESIAN_POINT('Ctrl Pts',(-0.940253996000056,2.2,4.48780758699999));
#331416=CARTESIAN_POINT('Ctrl Pts',(-0.941838193000055,12.2,4.48961147899999));
#331417=CARTESIAN_POINT('Ctrl Pts',(-0.941838193000055,5.2,4.48961147899999));
#331418=CARTESIAN_POINT('Ctrl Pts',(-0.941838193000055,2.2,4.48961147899999));
#331419=CARTESIAN_POINT('Ctrl Pts',(-0.943426707000056,12.2,4.49141640799999));
#331420=CARTESIAN_POINT('Ctrl Pts',(-0.943426707000056,5.2,4.49141640799999));
#331421=CARTESIAN_POINT('Ctrl Pts',(-0.943426707000056,2.2,4.49141640799999));
#331422=CARTESIAN_POINT('Ctrl Pts',(-0.945019539000055,12.2,4.49322236599999));
#331423=CARTESIAN_POINT('Ctrl Pts',(-0.945019539000055,5.2,4.49322236599999));
#331424=CARTESIAN_POINT('Ctrl Pts',(-0.945019539000055,2.2,4.49322236599999));
#331425=CARTESIAN_POINT('Ctrl Pts',(-0.946616692000056,12.2,4.49502934399998));
#331426=CARTESIAN_POINT('Ctrl Pts',(-0.946616692000056,5.2,4.49502934399998));
#331427=CARTESIAN_POINT('Ctrl Pts',(-0.946616692000056,2.2,4.49502934399998));
#331428=CARTESIAN_POINT('Ctrl Pts',(-0.948218165000055,12.2,4.49683733099998));
#331429=CARTESIAN_POINT('Ctrl Pts',(-0.948218165000055,5.2,4.49683733099998));
#331430=CARTESIAN_POINT('Ctrl Pts',(-0.948218165000055,2.2,4.49683733099998));
#331431=CARTESIAN_POINT('Ctrl Pts',(-0.949823959000057,12.2,4.49864631999999));
#331432=CARTESIAN_POINT('Ctrl Pts',(-0.949823959000057,5.2,4.49864631999999));
#331433=CARTESIAN_POINT('Ctrl Pts',(-0.949823959000057,2.2,4.49864631999999));
#331434=CARTESIAN_POINT('Ctrl Pts',(-0.951434074000056,12.2,4.50045629899999));
#331435=CARTESIAN_POINT('Ctrl Pts',(-0.951434074000056,5.2,4.50045629899999));
#331436=CARTESIAN_POINT('Ctrl Pts',(-0.951434074000056,2.2,4.50045629899999));
#331437=CARTESIAN_POINT('Ctrl Pts',(-0.953048512000055,12.2,4.50226725999999));
#331438=CARTESIAN_POINT('Ctrl Pts',(-0.953048512000055,5.2,4.50226725999999));
#331439=CARTESIAN_POINT('Ctrl Pts',(-0.953048512000055,2.2,4.50226725999999));
#331440=CARTESIAN_POINT('Ctrl Pts',(-0.954667273000057,12.2,4.50407919399999));
#331441=CARTESIAN_POINT('Ctrl Pts',(-0.954667273000057,5.2,4.50407919399999));
#331442=CARTESIAN_POINT('Ctrl Pts',(-0.954667273000057,2.2,4.50407919399999));
#331443=CARTESIAN_POINT('Ctrl Pts',(-0.956290358000055,12.2,4.50589209199999));
#331444=CARTESIAN_POINT('Ctrl Pts',(-0.956290358000055,5.2,4.50589209199999));
#331445=CARTESIAN_POINT('Ctrl Pts',(-0.956290358000055,2.2,4.50589209199999));
#331446=CARTESIAN_POINT('Ctrl Pts',(-0.957917768000056,12.2,4.50770594399999));
#331447=CARTESIAN_POINT('Ctrl Pts',(-0.957917768000056,5.2,4.50770594399999));
#331448=CARTESIAN_POINT('Ctrl Pts',(-0.957917768000056,2.2,4.50770594399999));
#331449=CARTESIAN_POINT('Ctrl Pts',(-0.959549503000057,12.2,4.50952074099998));
#331450=CARTESIAN_POINT('Ctrl Pts',(-0.959549503000057,5.2,4.50952074099998));
#331451=CARTESIAN_POINT('Ctrl Pts',(-0.959549503000057,2.2,4.50952074099998));
#331452=CARTESIAN_POINT('Ctrl Pts',(-0.961185565000056,12.2,4.51133647499999));
#331453=CARTESIAN_POINT('Ctrl Pts',(-0.961185565000056,5.2,4.51133647499999));
#331454=CARTESIAN_POINT('Ctrl Pts',(-0.961185565000056,2.2,4.51133647499999));
#331455=CARTESIAN_POINT('Ctrl Pts',(-0.962825953000056,12.2,4.51315313599999));
#331456=CARTESIAN_POINT('Ctrl Pts',(-0.962825953000056,5.2,4.51315313599999));
#331457=CARTESIAN_POINT('Ctrl Pts',(-0.962825953000056,2.2,4.51315313599999));
#331458=CARTESIAN_POINT('Ctrl Pts',(-0.964470669000056,12.2,4.51497071299999));
#331459=CARTESIAN_POINT('Ctrl Pts',(-0.964470669000056,5.2,4.51497071299999));
#331460=CARTESIAN_POINT('Ctrl Pts',(-0.964470669000056,2.2,4.51497071299999));
#331461=CARTESIAN_POINT('Ctrl Pts',(-0.966119713000057,12.2,4.51678919899998));
#331462=CARTESIAN_POINT('Ctrl Pts',(-0.966119713000057,5.2,4.51678919899998));
#331463=CARTESIAN_POINT('Ctrl Pts',(-0.966119713000057,2.2,4.51678919899998));
#331464=CARTESIAN_POINT('Ctrl Pts',(-0.967773085000055,12.2,4.51860858499998));
#331465=CARTESIAN_POINT('Ctrl Pts',(-0.967773085000055,5.2,4.51860858499998));
#331466=CARTESIAN_POINT('Ctrl Pts',(-0.967773085000055,2.2,4.51860858499998));
#331467=CARTESIAN_POINT('Ctrl Pts',(-0.969430788000055,12.2,4.52042885999998));
#331468=CARTESIAN_POINT('Ctrl Pts',(-0.969430788000055,5.2,4.52042885999998));
#331469=CARTESIAN_POINT('Ctrl Pts',(-0.969430788000055,2.2,4.52042885999998));
#331470=CARTESIAN_POINT('Ctrl Pts',(-0.971092819000056,12.2,4.52225001699999));
#331471=CARTESIAN_POINT('Ctrl Pts',(-0.971092819000056,5.2,4.52225001699999));
#331472=CARTESIAN_POINT('Ctrl Pts',(-0.971092819000056,2.2,4.52225001699999));
#331473=CARTESIAN_POINT('Ctrl Pts',(-0.972759181000056,12.2,4.52407204499998));
#331474=CARTESIAN_POINT('Ctrl Pts',(-0.972759181000056,5.2,4.52407204499998));
#331475=CARTESIAN_POINT('Ctrl Pts',(-0.972759181000056,2.2,4.52407204499998));
#331476=CARTESIAN_POINT('Ctrl Pts',(-0.974429875000055,12.2,4.52589493699998));
#331477=CARTESIAN_POINT('Ctrl Pts',(-0.974429875000055,5.2,4.52589493699998));
#331478=CARTESIAN_POINT('Ctrl Pts',(-0.974429875000055,2.2,4.52589493699998));
#331479=CARTESIAN_POINT('Ctrl Pts',(-0.976104901000056,12.2,4.52771868199999));
#331480=CARTESIAN_POINT('Ctrl Pts',(-0.976104901000056,5.2,4.52771868199999));
#331481=CARTESIAN_POINT('Ctrl Pts',(-0.976104901000056,2.2,4.52771868199999));
#331482=CARTESIAN_POINT('Ctrl Pts',(-0.977784258000056,12.2,4.52954327099999));
#331483=CARTESIAN_POINT('Ctrl Pts',(-0.977784258000056,5.2,4.52954327099999));
#331484=CARTESIAN_POINT('Ctrl Pts',(-0.977784258000056,2.2,4.52954327099999));
#331485=CARTESIAN_POINT('Ctrl Pts',(-0.979467948000057,12.2,4.53136869699998));
#331486=CARTESIAN_POINT('Ctrl Pts',(-0.979467948000057,5.2,4.53136869699998));
#331487=CARTESIAN_POINT('Ctrl Pts',(-0.979467948000057,2.2,4.53136869699998));
#331488=CARTESIAN_POINT('Ctrl Pts',(-0.981155972000056,12.2,4.53319494799998));
#331489=CARTESIAN_POINT('Ctrl Pts',(-0.981155972000056,5.2,4.53319494799998));
#331490=CARTESIAN_POINT('Ctrl Pts',(-0.981155972000056,2.2,4.53319494799998));
#331491=CARTESIAN_POINT('Ctrl Pts',(-0.982848330000056,12.2,4.53502201599999));
#331492=CARTESIAN_POINT('Ctrl Pts',(-0.982848330000056,5.2,4.53502201599999));
#331493=CARTESIAN_POINT('Ctrl Pts',(-0.982848330000056,2.2,4.53502201599999));
#331494=CARTESIAN_POINT('Ctrl Pts',(-0.984545022000055,12.2,4.53684989399999));
#331495=CARTESIAN_POINT('Ctrl Pts',(-0.984545022000055,5.2,4.53684989399999));
#331496=CARTESIAN_POINT('Ctrl Pts',(-0.984545022000055,2.2,4.53684989399999));
#331497=CARTESIAN_POINT('Ctrl Pts',(-0.986246049000057,12.2,4.53867856999998));
#331498=CARTESIAN_POINT('Ctrl Pts',(-0.986246049000057,5.2,4.53867856999998));
#331499=CARTESIAN_POINT('Ctrl Pts',(-0.986246049000057,2.2,4.53867856999998));
#331500=CARTESIAN_POINT('Ctrl Pts',(-0.987951411000055,12.2,4.54050803599999));
#331501=CARTESIAN_POINT('Ctrl Pts',(-0.987951411000055,5.2,4.54050803599999));
#331502=CARTESIAN_POINT('Ctrl Pts',(-0.987951411000055,2.2,4.54050803599999));
#331503=CARTESIAN_POINT('Ctrl Pts',(-0.989661108000056,12.2,4.54233828499999));
#331504=CARTESIAN_POINT('Ctrl Pts',(-0.989661108000056,5.2,4.54233828499999));
#331505=CARTESIAN_POINT('Ctrl Pts',(-0.989661108000056,2.2,4.54233828499999));
#331506=CARTESIAN_POINT('Ctrl Pts',(-0.991375143000056,12.2,4.54416930499999));
#331507=CARTESIAN_POINT('Ctrl Pts',(-0.991375143000056,5.2,4.54416930499999));
#331508=CARTESIAN_POINT('Ctrl Pts',(-0.991375143000056,2.2,4.54416930499999));
#331509=CARTESIAN_POINT('Ctrl Pts',(-0.993093514000056,12.2,4.54600108699999));
#331510=CARTESIAN_POINT('Ctrl Pts',(-0.993093514000056,5.2,4.54600108699999));
#331511=CARTESIAN_POINT('Ctrl Pts',(-0.993093514000056,2.2,4.54600108699999));
#331512=CARTESIAN_POINT('Ctrl Pts',(-0.994816221000056,12.2,4.54783362499998));
#331513=CARTESIAN_POINT('Ctrl Pts',(-0.994816221000056,5.2,4.54783362499998));
#331514=CARTESIAN_POINT('Ctrl Pts',(-0.994816221000056,2.2,4.54783362499998));
#331515=CARTESIAN_POINT('Ctrl Pts',(-0.996543267000056,12.2,4.54966690799999));
#331516=CARTESIAN_POINT('Ctrl Pts',(-0.996543267000056,5.2,4.54966690799999));
#331517=CARTESIAN_POINT('Ctrl Pts',(-0.996543267000056,2.2,4.54966690799999));
#331518=CARTESIAN_POINT('Ctrl Pts',(-0.998274650000056,12.2,4.55150092699999));
#331519=CARTESIAN_POINT('Ctrl Pts',(-0.998274650000056,5.2,4.55150092699999));
#331520=CARTESIAN_POINT('Ctrl Pts',(-0.998274650000056,2.2,4.55150092699999));
#331521=CARTESIAN_POINT('Ctrl Pts',(-1.00001037100006,12.2,4.55333567299999));
#331522=CARTESIAN_POINT('Ctrl Pts',(-1.00001037100006,5.2,4.55333567299999));
#331523=CARTESIAN_POINT('Ctrl Pts',(-1.00001037100006,2.2,4.55333567299999));
#331524=CARTESIAN_POINT('Ctrl Pts',(-1.00175043200006,12.2,4.55517113699998));
#331525=CARTESIAN_POINT('Ctrl Pts',(-1.00175043200006,5.2,4.55517113699998));
#331526=CARTESIAN_POINT('Ctrl Pts',(-1.00175043200006,2.2,4.55517113699998));
#331527=CARTESIAN_POINT('Ctrl Pts',(-1.00349483100006,12.2,4.55700731099999));
#331528=CARTESIAN_POINT('Ctrl Pts',(-1.00349483100006,5.2,4.55700731099999));
#331529=CARTESIAN_POINT('Ctrl Pts',(-1.00349483100006,2.2,4.55700731099999));
#331530=CARTESIAN_POINT('Ctrl Pts',(-1.00524357000006,12.2,4.55884418699998));
#331531=CARTESIAN_POINT('Ctrl Pts',(-1.00524357000006,5.2,4.55884418699998));
#331532=CARTESIAN_POINT('Ctrl Pts',(-1.00524357000006,2.2,4.55884418699998));
#331533=CARTESIAN_POINT('Ctrl Pts',(-1.00699664800006,12.2,4.56068175199999));
#331534=CARTESIAN_POINT('Ctrl Pts',(-1.00699664800006,5.2,4.56068175199999));
#331535=CARTESIAN_POINT('Ctrl Pts',(-1.00699664800006,2.2,4.56068175199999));
#331536=CARTESIAN_POINT('Ctrl Pts',(-1.00875406700006,12.2,4.56252000199999));
#331537=CARTESIAN_POINT('Ctrl Pts',(-1.00875406700006,5.2,4.56252000199999));
#331538=CARTESIAN_POINT('Ctrl Pts',(-1.00875406700006,2.2,4.56252000199999));
#331539=CARTESIAN_POINT('Ctrl Pts',(-1.01051582600006,12.2,4.56435892399998));
#331540=CARTESIAN_POINT('Ctrl Pts',(-1.01051582600006,5.2,4.56435892399998));
#331541=CARTESIAN_POINT('Ctrl Pts',(-1.01051582600006,2.2,4.56435892399998));
#331542=CARTESIAN_POINT('Ctrl Pts',(-1.01228192600006,12.2,4.56619851199999));
#331543=CARTESIAN_POINT('Ctrl Pts',(-1.01228192600006,5.2,4.56619851199999));
#331544=CARTESIAN_POINT('Ctrl Pts',(-1.01228192600006,2.2,4.56619851199999));
#331545=CARTESIAN_POINT('Ctrl Pts',(-1.01405236700006,12.2,4.56803875599999));
#331546=CARTESIAN_POINT('Ctrl Pts',(-1.01405236700006,5.2,4.56803875599999));
#331547=CARTESIAN_POINT('Ctrl Pts',(-1.01405236700006,2.2,4.56803875599999));
#331548=CARTESIAN_POINT('Ctrl Pts',(-1.01582714800006,12.2,4.56987964799998));
#331549=CARTESIAN_POINT('Ctrl Pts',(-1.01582714800006,5.2,4.56987964799998));
#331550=CARTESIAN_POINT('Ctrl Pts',(-1.01582714800006,2.2,4.56987964799998));
#331551=CARTESIAN_POINT('Ctrl Pts',(-1.01760627200006,12.2,4.57172117699999));
#331552=CARTESIAN_POINT('Ctrl Pts',(-1.01760627200006,5.2,4.57172117699999));
#331553=CARTESIAN_POINT('Ctrl Pts',(-1.01760627200006,2.2,4.57172117699999));
#331554=CARTESIAN_POINT('Ctrl Pts',(-1.01938973700006,12.2,4.57356333599999));
#331555=CARTESIAN_POINT('Ctrl Pts',(-1.01938973700006,5.2,4.57356333599999));
#331556=CARTESIAN_POINT('Ctrl Pts',(-1.01938973700006,2.2,4.57356333599999));
#331557=CARTESIAN_POINT('Ctrl Pts',(-1.02117754400005,12.2,4.57540611499999));
#331558=CARTESIAN_POINT('Ctrl Pts',(-1.02117754400005,5.2,4.57540611499999));
#331559=CARTESIAN_POINT('Ctrl Pts',(-1.02117754400005,2.2,4.57540611499999));
#331560=CARTESIAN_POINT('Ctrl Pts',(-1.02296969300006,12.2,4.57724950599999));
#331561=CARTESIAN_POINT('Ctrl Pts',(-1.02296969300006,5.2,4.57724950599999));
#331562=CARTESIAN_POINT('Ctrl Pts',(-1.02296969300006,2.2,4.57724950599999));
#331563=CARTESIAN_POINT('Ctrl Pts',(-1.02476618500006,12.2,4.57909349999999));
#331564=CARTESIAN_POINT('Ctrl Pts',(-1.02476618500006,5.2,4.57909349999999));
#331565=CARTESIAN_POINT('Ctrl Pts',(-1.02476618500006,2.2,4.57909349999999));
#331566=CARTESIAN_POINT('Ctrl Pts',(-1.02656701900006,12.2,4.58093808899999));
#331567=CARTESIAN_POINT('Ctrl Pts',(-1.02656701900006,5.2,4.58093808899999));
#331568=CARTESIAN_POINT('Ctrl Pts',(-1.02656701900006,2.2,4.58093808899999));
#331569=CARTESIAN_POINT('Ctrl Pts',(-1.02837219600006,12.2,4.58278326299999));
#331570=CARTESIAN_POINT('Ctrl Pts',(-1.02837219600006,5.2,4.58278326299999));
#331571=CARTESIAN_POINT('Ctrl Pts',(-1.02837219600006,2.2,4.58278326299999));
#331572=CARTESIAN_POINT('Ctrl Pts',(-1.03018171600006,12.2,4.58462901499999));
#331573=CARTESIAN_POINT('Ctrl Pts',(-1.03018171600006,5.2,4.58462901499999));
#331574=CARTESIAN_POINT('Ctrl Pts',(-1.03018171600006,2.2,4.58462901499999));
#331575=CARTESIAN_POINT('Ctrl Pts',(-1.03199558000005,12.2,4.58647533399999));
#331576=CARTESIAN_POINT('Ctrl Pts',(-1.03199558000005,5.2,4.58647533399999));
#331577=CARTESIAN_POINT('Ctrl Pts',(-1.03199558000005,2.2,4.58647533399999));
#331578=CARTESIAN_POINT('Ctrl Pts',(-1.03381378600006,12.2,4.58832221299998));
#331579=CARTESIAN_POINT('Ctrl Pts',(-1.03381378600006,5.2,4.58832221299998));
#331580=CARTESIAN_POINT('Ctrl Pts',(-1.03381378600006,2.2,4.58832221299998));
#331581=CARTESIAN_POINT('Ctrl Pts',(-1.03563633600006,12.2,4.59016964299998));
#331582=CARTESIAN_POINT('Ctrl Pts',(-1.03563633600006,5.2,4.59016964299998));
#331583=CARTESIAN_POINT('Ctrl Pts',(-1.03563633600006,2.2,4.59016964299998));
#331584=CARTESIAN_POINT('Ctrl Pts',(-1.03746322900006,12.2,4.59201761299998));
#331585=CARTESIAN_POINT('Ctrl Pts',(-1.03746322900006,5.2,4.59201761299998));
#331586=CARTESIAN_POINT('Ctrl Pts',(-1.03746322900006,2.2,4.59201761299998));
#331587=CARTESIAN_POINT('Ctrl Pts',(-1.03929446800006,12.2,4.59386611499998));
#331588=CARTESIAN_POINT('Ctrl Pts',(-1.03929446800006,5.2,4.59386611499998));
#331589=CARTESIAN_POINT('Ctrl Pts',(-1.03929446800006,2.2,4.59386611499998));
#331590=CARTESIAN_POINT('Ctrl Pts',(-1.04113004900006,12.2,4.59571514099999));
#331591=CARTESIAN_POINT('Ctrl Pts',(-1.04113004900006,5.2,4.59571514099999));
#331592=CARTESIAN_POINT('Ctrl Pts',(-1.04113004900006,2.2,4.59571514099999));
#331593=CARTESIAN_POINT('Ctrl Pts',(-1.04296997400006,12.2,4.59756468099998));
#331594=CARTESIAN_POINT('Ctrl Pts',(-1.04296997400006,5.2,4.59756468099998));
#331595=CARTESIAN_POINT('Ctrl Pts',(-1.04296997400006,2.2,4.59756468099998));
#331596=CARTESIAN_POINT('Ctrl Pts',(-1.04481424200006,12.2,4.59941472799999));
#331597=CARTESIAN_POINT('Ctrl Pts',(-1.04481424200006,5.2,4.59941472799999));
#331598=CARTESIAN_POINT('Ctrl Pts',(-1.04481424200006,2.2,4.59941472799999));
#331599=CARTESIAN_POINT('Ctrl Pts',(-1.04666285500006,12.2,4.60126527399999));
#331600=CARTESIAN_POINT('Ctrl Pts',(-1.04666285500006,5.2,4.60126527399999));
#331601=CARTESIAN_POINT('Ctrl Pts',(-1.04666285500006,2.2,4.60126527399999));
#331602=CARTESIAN_POINT('Ctrl Pts',(-1.04851581200006,12.2,4.60311631099999));
#331603=CARTESIAN_POINT('Ctrl Pts',(-1.04851581200006,5.2,4.60311631099999));
#331604=CARTESIAN_POINT('Ctrl Pts',(-1.04851581200006,2.2,4.60311631099999));
#331605=CARTESIAN_POINT('Ctrl Pts',(-1.05037311400006,12.2,4.60496783199999));
#331606=CARTESIAN_POINT('Ctrl Pts',(-1.05037311400006,5.2,4.60496783199999));
#331607=CARTESIAN_POINT('Ctrl Pts',(-1.05037311400006,2.2,4.60496783199999));
#331608=CARTESIAN_POINT('Ctrl Pts',(-1.05223475900006,12.2,4.60681982699998));
#331609=CARTESIAN_POINT('Ctrl Pts',(-1.05223475900006,5.2,4.60681982699998));
#331610=CARTESIAN_POINT('Ctrl Pts',(-1.05223475900006,2.2,4.60681982699998));
#331611=CARTESIAN_POINT('Ctrl Pts',(-1.05410074900006,12.2,4.60867228699998));
#331612=CARTESIAN_POINT('Ctrl Pts',(-1.05410074900006,5.2,4.60867228699998));
#331613=CARTESIAN_POINT('Ctrl Pts',(-1.05410074900006,2.2,4.60867228699998));
#331614=CARTESIAN_POINT('Ctrl Pts',(-1.05597108200006,12.2,4.61052519999999));
#331615=CARTESIAN_POINT('Ctrl Pts',(-1.05597108200006,5.2,4.61052519999999));
#331616=CARTESIAN_POINT('Ctrl Pts',(-1.05597108200006,2.2,4.61052519999999));
#331617=CARTESIAN_POINT('Ctrl Pts',(-1.05784576100006,12.2,4.61237855699999));
#331618=CARTESIAN_POINT('Ctrl Pts',(-1.05784576100006,5.2,4.61237855699999));
#331619=CARTESIAN_POINT('Ctrl Pts',(-1.05784576100006,2.2,4.61237855699999));
#331620=CARTESIAN_POINT('Ctrl Pts',(-1.05972478300006,12.2,4.61423234699998));
#331621=CARTESIAN_POINT('Ctrl Pts',(-1.05972478300006,5.2,4.61423234699998));
#331622=CARTESIAN_POINT('Ctrl Pts',(-1.05972478300006,2.2,4.61423234699998));
#331623=CARTESIAN_POINT('Ctrl Pts',(-1.06160814900006,12.2,4.61608656099998));
#331624=CARTESIAN_POINT('Ctrl Pts',(-1.06160814900006,5.2,4.61608656099998));
#331625=CARTESIAN_POINT('Ctrl Pts',(-1.06160814900006,2.2,4.61608656099998));
#331626=CARTESIAN_POINT('Ctrl Pts',(-1.06349586000006,12.2,4.61794118999999));
#331627=CARTESIAN_POINT('Ctrl Pts',(-1.06349586000006,5.2,4.61794118999999));
#331628=CARTESIAN_POINT('Ctrl Pts',(-1.06349586000006,2.2,4.61794118999999));
#331629=CARTESIAN_POINT('Ctrl Pts',(-1.06538791400006,12.2,4.61979622599999));
#331630=CARTESIAN_POINT('Ctrl Pts',(-1.06538791400006,5.2,4.61979622599999));
#331631=CARTESIAN_POINT('Ctrl Pts',(-1.06538791400006,2.2,4.61979622599999));
#331632=CARTESIAN_POINT('Ctrl Pts',(-1.06728431400006,12.2,4.62165166799998));
#331633=CARTESIAN_POINT('Ctrl Pts',(-1.06728431400006,5.2,4.62165166799998));
#331634=CARTESIAN_POINT('Ctrl Pts',(-1.06728431400006,2.2,4.62165166799998));
#331635=CARTESIAN_POINT('Ctrl Pts',(-1.06918505607982,12.2,4.62350751207786));
#331636=CARTESIAN_POINT('Ctrl Pts',(-1.06918505607982,5.2,4.62350751207786));
#331637=CARTESIAN_POINT('Ctrl Pts',(-1.06918505607982,2.2,4.62350751207786));
#331638=CARTESIAN_POINT('Ctrl Pts',(-1.07070912515995,12.2,4.62499250815578));
#331639=CARTESIAN_POINT('Ctrl Pts',(-1.07070912515995,5.2,4.62499250815578));
#331640=CARTESIAN_POINT('Ctrl Pts',(-1.07070912515995,2.2,4.62499250815578));
#331641=CARTESIAN_POINT('Ctrl Pts',(-1.07185413124031,12.2,4.62610643623372));
#331642=CARTESIAN_POINT('Ctrl Pts',(-1.07185413124031,5.2,4.62610643623372));
#331643=CARTESIAN_POINT('Ctrl Pts',(-1.07185413124031,2.2,4.62610643623372));
#331644=CARTESIAN_POINT('Ctrl Pts',(-1.07261833832076,12.2,4.62684913431167));
#331645=CARTESIAN_POINT('Ctrl Pts',(-1.07261833832076,5.2,4.62684913431167));
#331646=CARTESIAN_POINT('Ctrl Pts',(-1.07261833832076,2.2,4.62684913431167));
#331647=CARTESIAN_POINT('Ctrl Pts',(-1.07300065800006,12.2,4.62722050399999));
#331648=CARTESIAN_POINT('Ctrl Pts',(-1.07300065800006,5.2,4.62722050399999));
#331649=CARTESIAN_POINT('Ctrl Pts',(-1.07300065800006,2.2,4.62722050399999));
#331650=CARTESIAN_POINT('Origin',(-5.66300478732629E-14,15.2,-1.77635683940025E-14));
#331651=CARTESIAN_POINT('',(-0.00378600900005522,2.2,3.62499802299999));
#331652=CARTESIAN_POINT('Origin',(-0.0041710780000559,15.2,3.99369145999999));
#331653=CARTESIAN_POINT('',(-0.00417113200005593,12.2,3.99374277699999));
#331654=CARTESIAN_POINT('Ctrl Pts',(0.335933474999944,12.2,4.73810602399999));
#331655=CARTESIAN_POINT('Ctrl Pts',(0.335933474999944,5.2,4.73810602399999));
#331656=CARTESIAN_POINT('Ctrl Pts',(0.335933474999944,2.2,4.73810602399999));
#331657=CARTESIAN_POINT('Ctrl Pts',(0.335613955999945,12.2,4.73767941899998));
#331658=CARTESIAN_POINT('Ctrl Pts',(0.335613955999945,5.2,4.73767941899998));
#331659=CARTESIAN_POINT('Ctrl Pts',(0.335613955999945,2.2,4.73767941899998));
#331660=CARTESIAN_POINT('Ctrl Pts',(0.334975341999945,12.2,4.73682631699998));
#331661=CARTESIAN_POINT('Ctrl Pts',(0.334975341999945,5.2,4.73682631699998));
#331662=CARTESIAN_POINT('Ctrl Pts',(0.334975341999945,2.2,4.73682631699998));
#331663=CARTESIAN_POINT('Ctrl Pts',(0.334018688999944,12.2,4.73554698499999));
#331664=CARTESIAN_POINT('Ctrl Pts',(0.334018688999944,5.2,4.73554698499999));
#331665=CARTESIAN_POINT('Ctrl Pts',(0.334018688999944,2.2,4.73554698499999));
#331666=CARTESIAN_POINT('Ctrl Pts',(0.332745688999945,12.2,4.73384185399999));
#331667=CARTESIAN_POINT('Ctrl Pts',(0.332745688999945,5.2,4.73384185399999));
#331668=CARTESIAN_POINT('Ctrl Pts',(0.332745688999945,2.2,4.73384185399999));
#331669=CARTESIAN_POINT('Ctrl Pts',(0.331158665999943,12.2,4.73171151799999));
#331670=CARTESIAN_POINT('Ctrl Pts',(0.331158665999943,5.2,4.73171151799999));
#331671=CARTESIAN_POINT('Ctrl Pts',(0.331158665999943,2.2,4.73171151799999));
#331672=CARTESIAN_POINT('Ctrl Pts',(0.329575868999944,12.2,4.72958225699998));
#331673=CARTESIAN_POINT('Ctrl Pts',(0.329575868999944,5.2,4.72958225699998));
#331674=CARTESIAN_POINT('Ctrl Pts',(0.329575868999944,2.2,4.72958225699998));
#331675=CARTESIAN_POINT('Ctrl Pts',(0.327997300999944,12.2,4.72745407599999));
#331676=CARTESIAN_POINT('Ctrl Pts',(0.327997300999944,5.2,4.72745407599999));
#331677=CARTESIAN_POINT('Ctrl Pts',(0.327997300999944,2.2,4.72745407599999));
#331678=CARTESIAN_POINT('Ctrl Pts',(0.326422958999943,12.2,4.72532697899998));
#331679=CARTESIAN_POINT('Ctrl Pts',(0.326422958999943,5.2,4.72532697899998));
#331680=CARTESIAN_POINT('Ctrl Pts',(0.326422958999943,2.2,4.72532697899998));
#331681=CARTESIAN_POINT('Ctrl Pts',(0.324852842999944,12.2,4.72320096999999));
#331682=CARTESIAN_POINT('Ctrl Pts',(0.324852842999944,5.2,4.72320096999999));
#331683=CARTESIAN_POINT('Ctrl Pts',(0.324852842999944,2.2,4.72320096999999));
#331684=CARTESIAN_POINT('Ctrl Pts',(0.323286950999944,12.2,4.72107605899998));
#331685=CARTESIAN_POINT('Ctrl Pts',(0.323286950999944,5.2,4.72107605899998));
#331686=CARTESIAN_POINT('Ctrl Pts',(0.323286950999944,2.2,4.72107605899998));
#331687=CARTESIAN_POINT('Ctrl Pts',(0.321725282999944,12.2,4.71895225599999));
#331688=CARTESIAN_POINT('Ctrl Pts',(0.321725282999944,5.2,4.71895225599999));
#331689=CARTESIAN_POINT('Ctrl Pts',(0.321725282999944,2.2,4.71895225599999));
#331690=CARTESIAN_POINT('Ctrl Pts',(0.320167835999945,12.2,4.71682956899999));
#331691=CARTESIAN_POINT('Ctrl Pts',(0.320167835999945,5.2,4.71682956899999));
#331692=CARTESIAN_POINT('Ctrl Pts',(0.320167835999945,2.2,4.71682956899999));
#331693=CARTESIAN_POINT('Ctrl Pts',(0.318614607999944,12.2,4.71470801099999));
#331694=CARTESIAN_POINT('Ctrl Pts',(0.318614607999944,5.2,4.71470801099999));
#331695=CARTESIAN_POINT('Ctrl Pts',(0.318614607999944,2.2,4.71470801099999));
#331696=CARTESIAN_POINT('Ctrl Pts',(0.317065597999945,12.2,4.71258759299998));
#331697=CARTESIAN_POINT('Ctrl Pts',(0.317065597999945,5.2,4.71258759299998));
#331698=CARTESIAN_POINT('Ctrl Pts',(0.317065597999945,2.2,4.71258759299998));
#331699=CARTESIAN_POINT('Ctrl Pts',(0.315520804999944,12.2,4.71046832199999));
#331700=CARTESIAN_POINT('Ctrl Pts',(0.315520804999944,5.2,4.71046832199999));
#331701=CARTESIAN_POINT('Ctrl Pts',(0.315520804999944,2.2,4.71046832199999));
#331702=CARTESIAN_POINT('Ctrl Pts',(0.313980226999944,12.2,4.70835020699998));
#331703=CARTESIAN_POINT('Ctrl Pts',(0.313980226999944,5.2,4.70835020699998));
#331704=CARTESIAN_POINT('Ctrl Pts',(0.313980226999944,2.2,4.70835020699998));
#331705=CARTESIAN_POINT('Ctrl Pts',(0.312443861999944,12.2,4.70623325799998));
#331706=CARTESIAN_POINT('Ctrl Pts',(0.312443861999944,5.2,4.70623325799998));
#331707=CARTESIAN_POINT('Ctrl Pts',(0.312443861999944,2.2,4.70623325799998));
#331708=CARTESIAN_POINT('Ctrl Pts',(0.310911710999945,12.2,4.70411747999999));
#331709=CARTESIAN_POINT('Ctrl Pts',(0.310911710999945,5.2,4.70411747999999));
#331710=CARTESIAN_POINT('Ctrl Pts',(0.310911710999945,2.2,4.70411747999999));
#331711=CARTESIAN_POINT('Ctrl Pts',(0.309383769999944,12.2,4.70200288399998));
#331712=CARTESIAN_POINT('Ctrl Pts',(0.309383769999944,5.2,4.70200288399998));
#331713=CARTESIAN_POINT('Ctrl Pts',(0.309383769999944,2.2,4.70200288399998));
#331714=CARTESIAN_POINT('Ctrl Pts',(0.307860039999944,12.2,4.69988947399998));
#331715=CARTESIAN_POINT('Ctrl Pts',(0.307860039999944,5.2,4.69988947399998));
#331716=CARTESIAN_POINT('Ctrl Pts',(0.307860039999944,2.2,4.69988947399998));
#331717=CARTESIAN_POINT('Ctrl Pts',(0.306340516999944,12.2,4.69777726199998));
#331718=CARTESIAN_POINT('Ctrl Pts',(0.306340516999944,5.2,4.69777726199998));
#331719=CARTESIAN_POINT('Ctrl Pts',(0.306340516999944,2.2,4.69777726199998));
#331720=CARTESIAN_POINT('Ctrl Pts',(0.304825201999943,12.2,4.69566625299999));
#331721=CARTESIAN_POINT('Ctrl Pts',(0.304825201999943,5.2,4.69566625299999));
#331722=CARTESIAN_POINT('Ctrl Pts',(0.304825201999943,2.2,4.69566625299999));
#331723=CARTESIAN_POINT('Ctrl Pts',(0.303314091999944,12.2,4.69355645999999));
#331724=CARTESIAN_POINT('Ctrl Pts',(0.303314091999944,5.2,4.69355645999999));
#331725=CARTESIAN_POINT('Ctrl Pts',(0.303314091999944,2.2,4.69355645999999));
#331726=CARTESIAN_POINT('Ctrl Pts',(0.301807185999945,12.2,4.69144788799999));
#331727=CARTESIAN_POINT('Ctrl Pts',(0.301807185999945,5.2,4.69144788799999));
#331728=CARTESIAN_POINT('Ctrl Pts',(0.301807185999945,2.2,4.69144788799999));
#331729=CARTESIAN_POINT('Ctrl Pts',(0.300304481999945,12.2,4.68934054899999));
#331730=CARTESIAN_POINT('Ctrl Pts',(0.300304481999945,5.2,4.68934054899999));
#331731=CARTESIAN_POINT('Ctrl Pts',(0.300304481999945,2.2,4.68934054899999));
#331732=CARTESIAN_POINT('Ctrl Pts',(0.298805979999944,12.2,4.68723445099998));
#331733=CARTESIAN_POINT('Ctrl Pts',(0.298805979999944,5.2,4.68723445099998));
#331734=CARTESIAN_POINT('Ctrl Pts',(0.298805979999944,2.2,4.68723445099998));
#331735=CARTESIAN_POINT('Ctrl Pts',(0.297311675999945,12.2,4.68512960199998));
#331736=CARTESIAN_POINT('Ctrl Pts',(0.297311675999945,5.2,4.68512960199998));
#331737=CARTESIAN_POINT('Ctrl Pts',(0.297311675999945,2.2,4.68512960199998));
#331738=CARTESIAN_POINT('Ctrl Pts',(0.295821569999944,12.2,4.68302601099998));
#331739=CARTESIAN_POINT('Ctrl Pts',(0.295821569999944,5.2,4.68302601099998));
#331740=CARTESIAN_POINT('Ctrl Pts',(0.295821569999944,2.2,4.68302601099998));
#331741=CARTESIAN_POINT('Ctrl Pts',(0.294335659999945,12.2,4.68092368599999));
#331742=CARTESIAN_POINT('Ctrl Pts',(0.294335659999945,5.2,4.68092368599999));
#331743=CARTESIAN_POINT('Ctrl Pts',(0.294335659999945,2.2,4.68092368599999));
#331744=CARTESIAN_POINT('Ctrl Pts',(0.292853944999945,12.2,4.67882263599999));
#331745=CARTESIAN_POINT('Ctrl Pts',(0.292853944999945,5.2,4.67882263599999));
#331746=CARTESIAN_POINT('Ctrl Pts',(0.292853944999945,2.2,4.67882263599999));
#331747=CARTESIAN_POINT('Ctrl Pts',(0.291376422999944,12.2,4.67672286999999));
#331748=CARTESIAN_POINT('Ctrl Pts',(0.291376422999944,5.2,4.67672286999999));
#331749=CARTESIAN_POINT('Ctrl Pts',(0.291376422999944,2.2,4.67672286999999));
#331750=CARTESIAN_POINT('Ctrl Pts',(0.289903092999945,12.2,4.67462439599998));
#331751=CARTESIAN_POINT('Ctrl Pts',(0.289903092999945,5.2,4.67462439599998));
#331752=CARTESIAN_POINT('Ctrl Pts',(0.289903092999945,2.2,4.67462439599998));
#331753=CARTESIAN_POINT('Ctrl Pts',(0.288433951999943,12.2,4.67252722199999));
#331754=CARTESIAN_POINT('Ctrl Pts',(0.288433951999943,5.2,4.67252722199999));
#331755=CARTESIAN_POINT('Ctrl Pts',(0.288433951999943,2.2,4.67252722199999));
#331756=CARTESIAN_POINT('Ctrl Pts',(0.286968998999945,12.2,4.67043135899999));
#331757=CARTESIAN_POINT('Ctrl Pts',(0.286968998999945,5.2,4.67043135899999));
#331758=CARTESIAN_POINT('Ctrl Pts',(0.286968998999945,2.2,4.67043135899999));
#331759=CARTESIAN_POINT('Ctrl Pts',(0.285508232999945,12.2,4.66833681299998));
#331760=CARTESIAN_POINT('Ctrl Pts',(0.285508232999945,5.2,4.66833681299998));
#331761=CARTESIAN_POINT('Ctrl Pts',(0.285508232999945,2.2,4.66833681299998));
#331762=CARTESIAN_POINT('Ctrl Pts',(0.284051652999944,12.2,4.66624359399999));
#331763=CARTESIAN_POINT('Ctrl Pts',(0.284051652999944,5.2,4.66624359399999));
#331764=CARTESIAN_POINT('Ctrl Pts',(0.284051652999944,2.2,4.66624359399999));
#331765=CARTESIAN_POINT('Ctrl Pts',(0.282599253999944,12.2,4.66415171199999));
#331766=CARTESIAN_POINT('Ctrl Pts',(0.282599253999944,5.2,4.66415171199999));
#331767=CARTESIAN_POINT('Ctrl Pts',(0.282599253999944,2.2,4.66415171199999));
#331768=CARTESIAN_POINT('Ctrl Pts',(0.281151037999944,12.2,4.66206117399998));
#331769=CARTESIAN_POINT('Ctrl Pts',(0.281151037999944,5.2,4.66206117399998));
#331770=CARTESIAN_POINT('Ctrl Pts',(0.281151037999944,2.2,4.66206117399998));
#331771=CARTESIAN_POINT('Ctrl Pts',(0.279707001999944,12.2,4.65997198899998));
#331772=CARTESIAN_POINT('Ctrl Pts',(0.279707001999944,5.2,4.65997198899998));
#331773=CARTESIAN_POINT('Ctrl Pts',(0.279707001999944,2.2,4.65997198899998));
#331774=CARTESIAN_POINT('Ctrl Pts',(0.278267143999944,12.2,4.65788416699999));
#331775=CARTESIAN_POINT('Ctrl Pts',(0.278267143999944,5.2,4.65788416699999));
#331776=CARTESIAN_POINT('Ctrl Pts',(0.278267143999944,2.2,4.65788416699999));
#331777=CARTESIAN_POINT('Ctrl Pts',(0.276831460999943,12.2,4.65579771499999));
#331778=CARTESIAN_POINT('Ctrl Pts',(0.276831460999943,5.2,4.65579771499999));
#331779=CARTESIAN_POINT('Ctrl Pts',(0.276831460999943,2.2,4.65579771499999));
#331780=CARTESIAN_POINT('Ctrl Pts',(0.275399953999944,12.2,4.65371264199998));
#331781=CARTESIAN_POINT('Ctrl Pts',(0.275399953999944,5.2,4.65371264199998));
#331782=CARTESIAN_POINT('Ctrl Pts',(0.275399953999944,2.2,4.65371264199998));
#331783=CARTESIAN_POINT('Ctrl Pts',(0.273972618999944,12.2,4.65162895899999));
#331784=CARTESIAN_POINT('Ctrl Pts',(0.273972618999944,5.2,4.65162895899999));
#331785=CARTESIAN_POINT('Ctrl Pts',(0.273972618999944,2.2,4.65162895899999));
#331786=CARTESIAN_POINT('Ctrl Pts',(0.272549455999943,12.2,4.64954667099998));
#331787=CARTESIAN_POINT('Ctrl Pts',(0.272549455999943,5.2,4.64954667099998));
#331788=CARTESIAN_POINT('Ctrl Pts',(0.272549455999943,2.2,4.64954667099998));
#331789=CARTESIAN_POINT('Ctrl Pts',(0.271130461999943,12.2,4.64746578999998));
#331790=CARTESIAN_POINT('Ctrl Pts',(0.271130461999943,5.2,4.64746578999998));
#331791=CARTESIAN_POINT('Ctrl Pts',(0.271130461999943,2.2,4.64746578999998));
#331792=CARTESIAN_POINT('Ctrl Pts',(0.269715634999944,12.2,4.64538632299998));
#331793=CARTESIAN_POINT('Ctrl Pts',(0.269715634999944,5.2,4.64538632299998));
#331794=CARTESIAN_POINT('Ctrl Pts',(0.269715634999944,2.2,4.64538632299998));
#331795=CARTESIAN_POINT('Ctrl Pts',(0.268304974999944,12.2,4.64330827999999));
#331796=CARTESIAN_POINT('Ctrl Pts',(0.268304974999944,5.2,4.64330827999999));
#331797=CARTESIAN_POINT('Ctrl Pts',(0.268304974999944,2.2,4.64330827999999));
#331798=CARTESIAN_POINT('Ctrl Pts',(0.266898477999945,12.2,4.64123166799999));
#331799=CARTESIAN_POINT('Ctrl Pts',(0.266898477999945,5.2,4.64123166799999));
#331800=CARTESIAN_POINT('Ctrl Pts',(0.266898477999945,2.2,4.64123166799999));
#331801=CARTESIAN_POINT('Ctrl Pts',(0.265496142999944,12.2,4.63915649899998));
#331802=CARTESIAN_POINT('Ctrl Pts',(0.265496142999944,5.2,4.63915649899998));
#331803=CARTESIAN_POINT('Ctrl Pts',(0.265496142999944,2.2,4.63915649899998));
#331804=CARTESIAN_POINT('Ctrl Pts',(0.264097967999944,12.2,4.63708277799999));
#331805=CARTESIAN_POINT('Ctrl Pts',(0.264097967999944,5.2,4.63708277799999));
#331806=CARTESIAN_POINT('Ctrl Pts',(0.264097967999944,2.2,4.63708277799999));
#331807=CARTESIAN_POINT('Ctrl Pts',(0.262703951999944,12.2,4.63501051699998));
#331808=CARTESIAN_POINT('Ctrl Pts',(0.262703951999944,5.2,4.63501051699998));
#331809=CARTESIAN_POINT('Ctrl Pts',(0.262703951999944,2.2,4.63501051699998));
#331810=CARTESIAN_POINT('Ctrl Pts',(0.261314091999945,12.2,4.63293972199998));
#331811=CARTESIAN_POINT('Ctrl Pts',(0.261314091999945,5.2,4.63293972199998));
#331812=CARTESIAN_POINT('Ctrl Pts',(0.261314091999945,2.2,4.63293972199998));
#331813=CARTESIAN_POINT('Ctrl Pts',(0.259928386999944,12.2,4.63087040499998));
#331814=CARTESIAN_POINT('Ctrl Pts',(0.259928386999944,5.2,4.63087040499998));
#331815=CARTESIAN_POINT('Ctrl Pts',(0.259928386999944,2.2,4.63087040499998));
#331816=CARTESIAN_POINT('Ctrl Pts',(0.258546834999944,12.2,4.62880257299998));
#331817=CARTESIAN_POINT('Ctrl Pts',(0.258546834999944,5.2,4.62880257299998));
#331818=CARTESIAN_POINT('Ctrl Pts',(0.258546834999944,2.2,4.62880257299998));
#331819=CARTESIAN_POINT('Ctrl Pts',(0.257169431999945,12.2,4.62673623399999));
#331820=CARTESIAN_POINT('Ctrl Pts',(0.257169431999945,5.2,4.62673623399999));
#331821=CARTESIAN_POINT('Ctrl Pts',(0.257169431999945,2.2,4.62673623399999));
#331822=CARTESIAN_POINT('Ctrl Pts',(0.255796178999944,12.2,4.62467139899999));
#331823=CARTESIAN_POINT('Ctrl Pts',(0.255796178999944,5.2,4.62467139899999));
#331824=CARTESIAN_POINT('Ctrl Pts',(0.255796178999944,2.2,4.62467139899999));
#331825=CARTESIAN_POINT('Ctrl Pts',(0.254427072999944,12.2,4.62260807599999));
#331826=CARTESIAN_POINT('Ctrl Pts',(0.254427072999944,5.2,4.62260807599999));
#331827=CARTESIAN_POINT('Ctrl Pts',(0.254427072999944,2.2,4.62260807599999));
#331828=CARTESIAN_POINT('Ctrl Pts',(0.253062110999943,12.2,4.62054627299998));
#331829=CARTESIAN_POINT('Ctrl Pts',(0.253062110999943,5.2,4.62054627299998));
#331830=CARTESIAN_POINT('Ctrl Pts',(0.253062110999943,2.2,4.62054627299998));
#331831=CARTESIAN_POINT('Ctrl Pts',(0.251701291999943,12.2,4.61848599999998));
#331832=CARTESIAN_POINT('Ctrl Pts',(0.251701291999943,5.2,4.61848599999998));
#331833=CARTESIAN_POINT('Ctrl Pts',(0.251701291999943,2.2,4.61848599999998));
#331834=CARTESIAN_POINT('Ctrl Pts',(0.250344613999944,12.2,4.61642726599998));
#331835=CARTESIAN_POINT('Ctrl Pts',(0.250344613999944,5.2,4.61642726599998));
#331836=CARTESIAN_POINT('Ctrl Pts',(0.250344613999944,2.2,4.61642726599998));
#331837=CARTESIAN_POINT('Ctrl Pts',(0.248992075999944,12.2,4.61437007899999));
#331838=CARTESIAN_POINT('Ctrl Pts',(0.248992075999944,5.2,4.61437007899999));
#331839=CARTESIAN_POINT('Ctrl Pts',(0.248992075999944,2.2,4.61437007899999));
#331840=CARTESIAN_POINT('Ctrl Pts',(0.247643673999944,12.2,4.61231444999999));
#331841=CARTESIAN_POINT('Ctrl Pts',(0.247643673999944,5.2,4.61231444999999));
#331842=CARTESIAN_POINT('Ctrl Pts',(0.247643673999944,2.2,4.61231444999999));
#331843=CARTESIAN_POINT('Ctrl Pts',(0.246299405999943,12.2,4.61026038399999));
#331844=CARTESIAN_POINT('Ctrl Pts',(0.246299405999943,5.2,4.61026038399999));
#331845=CARTESIAN_POINT('Ctrl Pts',(0.246299405999943,2.2,4.61026038399999));
#331846=CARTESIAN_POINT('Ctrl Pts',(0.244959270999944,12.2,4.60820789399998));
#331847=CARTESIAN_POINT('Ctrl Pts',(0.244959270999944,5.2,4.60820789399998));
#331848=CARTESIAN_POINT('Ctrl Pts',(0.244959270999944,2.2,4.60820789399998));
#331849=CARTESIAN_POINT('Ctrl Pts',(0.243623266999944,12.2,4.60615698599998));
#331850=CARTESIAN_POINT('Ctrl Pts',(0.243623266999944,5.2,4.60615698599998));
#331851=CARTESIAN_POINT('Ctrl Pts',(0.243623266999944,2.2,4.60615698599998));
#331852=CARTESIAN_POINT('Ctrl Pts',(0.242291391999944,12.2,4.60410767099999));
#331853=CARTESIAN_POINT('Ctrl Pts',(0.242291391999944,5.2,4.60410767099999));
#331854=CARTESIAN_POINT('Ctrl Pts',(0.242291391999944,2.2,4.60410767099999));
#331855=CARTESIAN_POINT('Ctrl Pts',(0.240963642999944,12.2,4.60205995699998));
#331856=CARTESIAN_POINT('Ctrl Pts',(0.240963642999944,5.2,4.60205995699998));
#331857=CARTESIAN_POINT('Ctrl Pts',(0.240963642999944,2.2,4.60205995699998));
#331858=CARTESIAN_POINT('Ctrl Pts',(0.239640017999945,12.2,4.60001385399998));
#331859=CARTESIAN_POINT('Ctrl Pts',(0.239640017999945,5.2,4.60001385399998));
#331860=CARTESIAN_POINT('Ctrl Pts',(0.239640017999945,2.2,4.60001385399998));
#331861=CARTESIAN_POINT('Ctrl Pts',(0.238320514999945,12.2,4.59796936899998));
#331862=CARTESIAN_POINT('Ctrl Pts',(0.238320514999945,5.2,4.59796936899998));
#331863=CARTESIAN_POINT('Ctrl Pts',(0.238320514999945,2.2,4.59796936899998));
#331864=CARTESIAN_POINT('Ctrl Pts',(0.237005132999943,12.2,4.59592651299998));
#331865=CARTESIAN_POINT('Ctrl Pts',(0.237005132999943,5.2,4.59592651299998));
#331866=CARTESIAN_POINT('Ctrl Pts',(0.237005132999943,2.2,4.59592651299998));
#331867=CARTESIAN_POINT('Ctrl Pts',(0.235693867999943,12.2,4.59388529299999));
#331868=CARTESIAN_POINT('Ctrl Pts',(0.235693867999943,5.2,4.59388529299999));
#331869=CARTESIAN_POINT('Ctrl Pts',(0.235693867999943,2.2,4.59388529299999));
#331870=CARTESIAN_POINT('Ctrl Pts',(0.234386717999945,12.2,4.59184572099999));
#331871=CARTESIAN_POINT('Ctrl Pts',(0.234386717999945,5.2,4.59184572099999));
#331872=CARTESIAN_POINT('Ctrl Pts',(0.234386717999945,2.2,4.59184572099999));
#331873=CARTESIAN_POINT('Ctrl Pts',(0.233083682999944,12.2,4.58980780299999));
#331874=CARTESIAN_POINT('Ctrl Pts',(0.233083682999944,5.2,4.58980780299999));
#331875=CARTESIAN_POINT('Ctrl Pts',(0.233083682999944,2.2,4.58980780299999));
#331876=CARTESIAN_POINT('Ctrl Pts',(0.231784757999945,12.2,4.58777154899998));
#331877=CARTESIAN_POINT('Ctrl Pts',(0.231784757999945,5.2,4.58777154899998));
#331878=CARTESIAN_POINT('Ctrl Pts',(0.231784757999945,2.2,4.58777154899998));
#331879=CARTESIAN_POINT('Ctrl Pts',(0.230489942999944,12.2,4.58573696899998));
#331880=CARTESIAN_POINT('Ctrl Pts',(0.230489942999944,5.2,4.58573696899998));
#331881=CARTESIAN_POINT('Ctrl Pts',(0.230489942999944,2.2,4.58573696899998));
#331882=CARTESIAN_POINT('Ctrl Pts',(0.229199234999945,12.2,4.58370407099999));
#331883=CARTESIAN_POINT('Ctrl Pts',(0.229199234999945,5.2,4.58370407099999));
#331884=CARTESIAN_POINT('Ctrl Pts',(0.229199234999945,2.2,4.58370407099999));
#331885=CARTESIAN_POINT('Ctrl Pts',(0.227912629999943,12.2,4.58167286499998));
#331886=CARTESIAN_POINT('Ctrl Pts',(0.227912629999943,5.2,4.58167286499998));
#331887=CARTESIAN_POINT('Ctrl Pts',(0.227912629999943,2.2,4.58167286499998));
#331888=CARTESIAN_POINT('Ctrl Pts',(0.226630128999944,12.2,4.57964335899998));
#331889=CARTESIAN_POINT('Ctrl Pts',(0.226630128999944,5.2,4.57964335899998));
#331890=CARTESIAN_POINT('Ctrl Pts',(0.226630128999944,2.2,4.57964335899998));
#331891=CARTESIAN_POINT('Ctrl Pts',(0.225351726999945,12.2,4.57761556199999));
#331892=CARTESIAN_POINT('Ctrl Pts',(0.225351726999945,5.2,4.57761556199999));
#331893=CARTESIAN_POINT('Ctrl Pts',(0.225351726999945,2.2,4.57761556199999));
#331894=CARTESIAN_POINT('Ctrl Pts',(0.224077423999944,12.2,4.57558948499998));
#331895=CARTESIAN_POINT('Ctrl Pts',(0.224077423999944,5.2,4.57558948499998));
#331896=CARTESIAN_POINT('Ctrl Pts',(0.224077423999944,2.2,4.57558948499998));
#331897=CARTESIAN_POINT('Ctrl Pts',(0.222807214999945,12.2,4.57356513499998));
#331898=CARTESIAN_POINT('Ctrl Pts',(0.222807214999945,5.2,4.57356513499998));
#331899=CARTESIAN_POINT('Ctrl Pts',(0.222807214999945,2.2,4.57356513499998));
#331900=CARTESIAN_POINT('Ctrl Pts',(0.221541099999945,12.2,4.57154252199999));
#331901=CARTESIAN_POINT('Ctrl Pts',(0.221541099999945,5.2,4.57154252199999));
#331902=CARTESIAN_POINT('Ctrl Pts',(0.221541099999945,2.2,4.57154252199999));
#331903=CARTESIAN_POINT('Ctrl Pts',(0.220279073999944,12.2,4.56952165399999));
#331904=CARTESIAN_POINT('Ctrl Pts',(0.220279073999944,5.2,4.56952165399999));
#331905=CARTESIAN_POINT('Ctrl Pts',(0.220279073999944,2.2,4.56952165399999));
#331906=CARTESIAN_POINT('Ctrl Pts',(0.219021137999944,12.2,4.56750254099998));
#331907=CARTESIAN_POINT('Ctrl Pts',(0.219021137999944,5.2,4.56750254099998));
#331908=CARTESIAN_POINT('Ctrl Pts',(0.219021137999944,2.2,4.56750254099998));
#331909=CARTESIAN_POINT('Ctrl Pts',(0.217767286999945,12.2,4.56548519299999));
#331910=CARTESIAN_POINT('Ctrl Pts',(0.217767286999945,5.2,4.56548519299999));
#331911=CARTESIAN_POINT('Ctrl Pts',(0.217767286999945,2.2,4.56548519299999));
#331912=CARTESIAN_POINT('Ctrl Pts',(0.216517519999944,12.2,4.56346961899998));
#331913=CARTESIAN_POINT('Ctrl Pts',(0.216517519999944,5.2,4.56346961899998));
#331914=CARTESIAN_POINT('Ctrl Pts',(0.216517519999944,2.2,4.56346961899998));
#331915=CARTESIAN_POINT('Ctrl Pts',(0.215271834999945,12.2,4.56145582599999));
#331916=CARTESIAN_POINT('Ctrl Pts',(0.215271834999945,5.2,4.56145582599999));
#331917=CARTESIAN_POINT('Ctrl Pts',(0.215271834999945,2.2,4.56145582599999));
#331918=CARTESIAN_POINT('Ctrl Pts',(0.214030226999944,12.2,4.55944382499998));
#331919=CARTESIAN_POINT('Ctrl Pts',(0.214030226999944,5.2,4.55944382499998));
#331920=CARTESIAN_POINT('Ctrl Pts',(0.214030226999944,2.2,4.55944382499998));
#331921=CARTESIAN_POINT('Ctrl Pts',(0.212792695999945,12.2,4.55743362599998));
#331922=CARTESIAN_POINT('Ctrl Pts',(0.212792695999945,5.2,4.55743362599998));
#331923=CARTESIAN_POINT('Ctrl Pts',(0.212792695999945,2.2,4.55743362599998));
#331924=CARTESIAN_POINT('Ctrl Pts',(0.211559238999944,12.2,4.55542523499999));
#331925=CARTESIAN_POINT('Ctrl Pts',(0.211559238999944,5.2,4.55542523499999));
#331926=CARTESIAN_POINT('Ctrl Pts',(0.211559238999944,2.2,4.55542523499999));
#331927=CARTESIAN_POINT('Ctrl Pts',(0.210329852999944,12.2,4.55341866399999));
#331928=CARTESIAN_POINT('Ctrl Pts',(0.210329852999944,5.2,4.55341866399999));
#331929=CARTESIAN_POINT('Ctrl Pts',(0.210329852999944,2.2,4.55341866399999));
#331930=CARTESIAN_POINT('Ctrl Pts',(0.209104535999945,12.2,4.55141392199998));
#331931=CARTESIAN_POINT('Ctrl Pts',(0.209104535999945,5.2,4.55141392199998));
#331932=CARTESIAN_POINT('Ctrl Pts',(0.209104535999945,2.2,4.55141392199998));
#331933=CARTESIAN_POINT('Ctrl Pts',(0.207883285999945,12.2,4.54941101699998));
#331934=CARTESIAN_POINT('Ctrl Pts',(0.207883285999945,5.2,4.54941101699998));
#331935=CARTESIAN_POINT('Ctrl Pts',(0.207883285999945,2.2,4.54941101699998));
#331936=CARTESIAN_POINT('Ctrl Pts',(0.206666098999945,12.2,4.54740995799998));
#331937=CARTESIAN_POINT('Ctrl Pts',(0.206666098999945,5.2,4.54740995799998));
#331938=CARTESIAN_POINT('Ctrl Pts',(0.206666098999945,2.2,4.54740995799998));
#331939=CARTESIAN_POINT('Ctrl Pts',(0.205452972999945,12.2,4.54541075599998));
#331940=CARTESIAN_POINT('Ctrl Pts',(0.205452972999945,5.2,4.54541075599998));
#331941=CARTESIAN_POINT('Ctrl Pts',(0.205452972999945,2.2,4.54541075599998));
#331942=CARTESIAN_POINT('Ctrl Pts',(0.204243906999944,12.2,4.54341341899998));
#331943=CARTESIAN_POINT('Ctrl Pts',(0.204243906999944,5.2,4.54341341899998));
#331944=CARTESIAN_POINT('Ctrl Pts',(0.204243906999944,2.2,4.54341341899998));
#331945=CARTESIAN_POINT('Ctrl Pts',(0.203038895999944,12.2,4.54141795499999));
#331946=CARTESIAN_POINT('Ctrl Pts',(0.203038895999944,5.2,4.54141795499999));
#331947=CARTESIAN_POINT('Ctrl Pts',(0.203038895999944,2.2,4.54141795499999));
#331948=CARTESIAN_POINT('Ctrl Pts',(0.201837938999944,12.2,4.53942437699999));
#331949=CARTESIAN_POINT('Ctrl Pts',(0.201837938999944,5.2,4.53942437699999));
#331950=CARTESIAN_POINT('Ctrl Pts',(0.201837938999944,2.2,4.53942437699999));
#331951=CARTESIAN_POINT('Ctrl Pts',(0.200641032999943,12.2,4.53743268999999));
#331952=CARTESIAN_POINT('Ctrl Pts',(0.200641032999943,5.2,4.53743268999999));
#331953=CARTESIAN_POINT('Ctrl Pts',(0.200641032999943,2.2,4.53743268999999));
#331954=CARTESIAN_POINT('Ctrl Pts',(0.199448174999944,12.2,4.53544290599999));
#331955=CARTESIAN_POINT('Ctrl Pts',(0.199448174999944,5.2,4.53544290599999));
#331956=CARTESIAN_POINT('Ctrl Pts',(0.199448174999944,2.2,4.53544290599999));
#331957=CARTESIAN_POINT('Ctrl Pts',(0.198259362999943,12.2,4.53345503399999));
#331958=CARTESIAN_POINT('Ctrl Pts',(0.198259362999943,5.2,4.53345503399999));
#331959=CARTESIAN_POINT('Ctrl Pts',(0.198259362999943,2.2,4.53345503399999));
#331960=CARTESIAN_POINT('Ctrl Pts',(0.197074592999943,12.2,4.53146908099999));
#331961=CARTESIAN_POINT('Ctrl Pts',(0.197074592999943,5.2,4.53146908099999));
#331962=CARTESIAN_POINT('Ctrl Pts',(0.197074592999943,2.2,4.53146908099999));
#331963=CARTESIAN_POINT('Ctrl Pts',(0.195893864999944,12.2,4.52948505899998));
#331964=CARTESIAN_POINT('Ctrl Pts',(0.195893864999944,5.2,4.52948505899998));
#331965=CARTESIAN_POINT('Ctrl Pts',(0.195893864999944,2.2,4.52948505899998));
#331966=CARTESIAN_POINT('Ctrl Pts',(0.194717173999944,12.2,4.52750297699998));
#331967=CARTESIAN_POINT('Ctrl Pts',(0.194717173999944,5.2,4.52750297699998));
#331968=CARTESIAN_POINT('Ctrl Pts',(0.194717173999944,2.2,4.52750297699998));
#331969=CARTESIAN_POINT('Ctrl Pts',(0.193544517999945,12.2,4.52552284299998));
#331970=CARTESIAN_POINT('Ctrl Pts',(0.193544517999945,5.2,4.52552284299998));
#331971=CARTESIAN_POINT('Ctrl Pts',(0.193544517999945,2.2,4.52552284299998));
#331972=CARTESIAN_POINT('Ctrl Pts',(0.192375894999944,12.2,4.52354466699998));
#331973=CARTESIAN_POINT('Ctrl Pts',(0.192375894999944,5.2,4.52354466699998));
#331974=CARTESIAN_POINT('Ctrl Pts',(0.192375894999944,2.2,4.52354466699998));
#331975=CARTESIAN_POINT('Ctrl Pts',(0.191211299999944,12.2,4.52156845699999));
#331976=CARTESIAN_POINT('Ctrl Pts',(0.191211299999944,5.2,4.52156845699999));
#331977=CARTESIAN_POINT('Ctrl Pts',(0.191211299999944,2.2,4.52156845699999));
#331978=CARTESIAN_POINT('Ctrl Pts',(0.190050732999945,12.2,4.51959422499999));
#331979=CARTESIAN_POINT('Ctrl Pts',(0.190050732999945,5.2,4.51959422499999));
#331980=CARTESIAN_POINT('Ctrl Pts',(0.190050732999945,2.2,4.51959422499999));
#331981=CARTESIAN_POINT('Ctrl Pts',(0.188894189999944,12.2,4.51762197899999));
#331982=CARTESIAN_POINT('Ctrl Pts',(0.188894189999944,5.2,4.51762197899999));
#331983=CARTESIAN_POINT('Ctrl Pts',(0.188894189999944,2.2,4.51762197899999));
#331984=CARTESIAN_POINT('Ctrl Pts',(0.187741667999944,12.2,4.51565172799998));
#331985=CARTESIAN_POINT('Ctrl Pts',(0.187741667999944,5.2,4.51565172799998));
#331986=CARTESIAN_POINT('Ctrl Pts',(0.187741667999944,2.2,4.51565172799998));
#331987=CARTESIAN_POINT('Ctrl Pts',(0.186593162999945,12.2,4.51368348099999));
#331988=CARTESIAN_POINT('Ctrl Pts',(0.186593162999945,5.2,4.51368348099999));
#331989=CARTESIAN_POINT('Ctrl Pts',(0.186593162999945,2.2,4.51368348099999));
#331990=CARTESIAN_POINT('Ctrl Pts',(0.185448674999943,12.2,4.51171724899999));
#331991=CARTESIAN_POINT('Ctrl Pts',(0.185448674999943,5.2,4.51171724899999));
#331992=CARTESIAN_POINT('Ctrl Pts',(0.185448674999943,2.2,4.51171724899999));
#331993=CARTESIAN_POINT('Ctrl Pts',(0.184308199999944,12.2,4.50975303999999));
#331994=CARTESIAN_POINT('Ctrl Pts',(0.184308199999944,5.2,4.50975303999999));
#331995=CARTESIAN_POINT('Ctrl Pts',(0.184308199999944,2.2,4.50975303999999));
#331996=CARTESIAN_POINT('Ctrl Pts',(0.183171734999944,12.2,4.50779086399999));
#331997=CARTESIAN_POINT('Ctrl Pts',(0.183171734999944,5.2,4.50779086399999));
#331998=CARTESIAN_POINT('Ctrl Pts',(0.183171734999944,2.2,4.50779086399999));
#331999=CARTESIAN_POINT('Ctrl Pts',(0.182039276999945,12.2,4.50583072899998));
#332000=CARTESIAN_POINT('Ctrl Pts',(0.182039276999945,5.2,4.50583072899998));
#332001=CARTESIAN_POINT('Ctrl Pts',(0.182039276999945,2.2,4.50583072899998));
#332002=CARTESIAN_POINT('Ctrl Pts',(0.180910821999944,12.2,4.50387264599998));
#332003=CARTESIAN_POINT('Ctrl Pts',(0.180910821999944,5.2,4.50387264599998));
#332004=CARTESIAN_POINT('Ctrl Pts',(0.180910821999944,2.2,4.50387264599998));
#332005=CARTESIAN_POINT('Ctrl Pts',(0.179786368999943,12.2,4.50191662499999));
#332006=CARTESIAN_POINT('Ctrl Pts',(0.179786368999943,5.2,4.50191662499999));
#332007=CARTESIAN_POINT('Ctrl Pts',(0.179786368999943,2.2,4.50191662499999));
#332008=CARTESIAN_POINT('Ctrl Pts',(0.178665914999945,12.2,4.49996267399998));
#332009=CARTESIAN_POINT('Ctrl Pts',(0.178665914999945,5.2,4.49996267399998));
#332010=CARTESIAN_POINT('Ctrl Pts',(0.178665914999945,2.2,4.49996267399998));
#332011=CARTESIAN_POINT('Ctrl Pts',(0.177549455999945,12.2,4.49801080299999));
#332012=CARTESIAN_POINT('Ctrl Pts',(0.177549455999945,5.2,4.49801080299999));
#332013=CARTESIAN_POINT('Ctrl Pts',(0.177549455999945,2.2,4.49801080299999));
#332014=CARTESIAN_POINT('Ctrl Pts',(0.176436989999944,12.2,4.49606102099998));
#332015=CARTESIAN_POINT('Ctrl Pts',(0.176436989999944,5.2,4.49606102099998));
#332016=CARTESIAN_POINT('Ctrl Pts',(0.176436989999944,2.2,4.49606102099998));
#332017=CARTESIAN_POINT('Ctrl Pts',(0.175328511999944,12.2,4.49411333799999));
#332018=CARTESIAN_POINT('Ctrl Pts',(0.175328511999944,5.2,4.49411333799999));
#332019=CARTESIAN_POINT('Ctrl Pts',(0.175328511999944,2.2,4.49411333799999));
#332020=CARTESIAN_POINT('Ctrl Pts',(0.174224021999944,12.2,4.49216776299998));
#332021=CARTESIAN_POINT('Ctrl Pts',(0.174224021999944,5.2,4.49216776299998));
#332022=CARTESIAN_POINT('Ctrl Pts',(0.174224021999944,2.2,4.49216776299998));
#332023=CARTESIAN_POINT('Ctrl Pts',(0.173123514999943,12.2,4.49022430599998));
#332024=CARTESIAN_POINT('Ctrl Pts',(0.173123514999943,5.2,4.49022430599998));
#332025=CARTESIAN_POINT('Ctrl Pts',(0.173123514999943,2.2,4.49022430599998));
#332026=CARTESIAN_POINT('Ctrl Pts',(0.172026987999944,12.2,4.48828297499999));
#332027=CARTESIAN_POINT('Ctrl Pts',(0.172026987999944,5.2,4.48828297499999));
#332028=CARTESIAN_POINT('Ctrl Pts',(0.172026987999944,2.2,4.48828297499999));
#332029=CARTESIAN_POINT('Ctrl Pts',(0.170934438999945,12.2,4.48634378299998));
#332030=CARTESIAN_POINT('Ctrl Pts',(0.170934438999945,5.2,4.48634378299998));
#332031=CARTESIAN_POINT('Ctrl Pts',(0.170934438999945,2.2,4.48634378299998));
#332032=CARTESIAN_POINT('Ctrl Pts',(0.169845864999945,12.2,4.48440673499999));
#332033=CARTESIAN_POINT('Ctrl Pts',(0.169845864999945,5.2,4.48440673499999));
#332034=CARTESIAN_POINT('Ctrl Pts',(0.169845864999945,2.2,4.48440673499999));
#332035=CARTESIAN_POINT('Ctrl Pts',(0.168761260999943,12.2,4.48247184299999));
#332036=CARTESIAN_POINT('Ctrl Pts',(0.168761260999943,5.2,4.48247184299999));
#332037=CARTESIAN_POINT('Ctrl Pts',(0.168761260999943,2.2,4.48247184299999));
#332038=CARTESIAN_POINT('Ctrl Pts',(0.167680625999944,12.2,4.48053911699999));
#332039=CARTESIAN_POINT('Ctrl Pts',(0.167680625999944,5.2,4.48053911699999));
#332040=CARTESIAN_POINT('Ctrl Pts',(0.167680625999944,2.2,4.48053911699999));
#332041=CARTESIAN_POINT('Ctrl Pts',(0.166603955999944,12.2,4.47860856599998));
#332042=CARTESIAN_POINT('Ctrl Pts',(0.166603955999944,5.2,4.47860856599998));
#332043=CARTESIAN_POINT('Ctrl Pts',(0.166603955999944,2.2,4.47860856599998));
#332044=CARTESIAN_POINT('Ctrl Pts',(0.165531247999944,12.2,4.47668019799998));
#332045=CARTESIAN_POINT('Ctrl Pts',(0.165531247999944,5.2,4.47668019799998));
#332046=CARTESIAN_POINT('Ctrl Pts',(0.165531247999944,2.2,4.47668019799998));
#332047=CARTESIAN_POINT('Ctrl Pts',(0.164462497999944,12.2,4.47475402499999));
#332048=CARTESIAN_POINT('Ctrl Pts',(0.164462497999944,5.2,4.47475402499999));
#332049=CARTESIAN_POINT('Ctrl Pts',(0.164462497999944,2.2,4.47475402499999));
#332050=CARTESIAN_POINT('Ctrl Pts',(0.163397704999945,12.2,4.47283005399999));
#332051=CARTESIAN_POINT('Ctrl Pts',(0.163397704999945,5.2,4.47283005399999));
#332052=CARTESIAN_POINT('Ctrl Pts',(0.163397704999945,2.2,4.47283005399999));
#332053=CARTESIAN_POINT('Ctrl Pts',(0.162336863999943,12.2,4.47090829699999));
#332054=CARTESIAN_POINT('Ctrl Pts',(0.162336863999943,5.2,4.47090829699999));
#332055=CARTESIAN_POINT('Ctrl Pts',(0.162336863999943,2.2,4.47090829699999));
#332056=CARTESIAN_POINT('Ctrl Pts',(0.161279971999945,12.2,4.46898876299999));
#332057=CARTESIAN_POINT('Ctrl Pts',(0.161279971999945,5.2,4.46898876299999));
#332058=CARTESIAN_POINT('Ctrl Pts',(0.161279971999945,2.2,4.46898876299999));
#332059=CARTESIAN_POINT('Ctrl Pts',(0.160227026999945,12.2,4.46707146099998));
#332060=CARTESIAN_POINT('Ctrl Pts',(0.160227026999945,5.2,4.46707146099998));
#332061=CARTESIAN_POINT('Ctrl Pts',(0.160227026999945,2.2,4.46707146099998));
#332062=CARTESIAN_POINT('Ctrl Pts',(0.159178023999944,12.2,4.46515639899999));
#332063=CARTESIAN_POINT('Ctrl Pts',(0.159178023999944,5.2,4.46515639899999));
#332064=CARTESIAN_POINT('Ctrl Pts',(0.159178023999944,2.2,4.46515639899999));
#332065=CARTESIAN_POINT('Ctrl Pts',(0.158132960999945,12.2,4.46324358999998));
#332066=CARTESIAN_POINT('Ctrl Pts',(0.158132960999945,5.2,4.46324358999998));
#332067=CARTESIAN_POINT('Ctrl Pts',(0.158132960999945,2.2,4.46324358999998));
#332068=CARTESIAN_POINT('Ctrl Pts',(0.157091832999944,12.2,4.46133304099998));
#332069=CARTESIAN_POINT('Ctrl Pts',(0.157091832999944,5.2,4.46133304099998));
#332070=CARTESIAN_POINT('Ctrl Pts',(0.157091832999944,2.2,4.46133304099998));
#332071=CARTESIAN_POINT('Ctrl Pts',(0.156054640999944,12.2,4.45942476299999));
#332072=CARTESIAN_POINT('Ctrl Pts',(0.156054640999944,5.2,4.45942476299999));
#332073=CARTESIAN_POINT('Ctrl Pts',(0.156054640999944,2.2,4.45942476299999));
#332074=CARTESIAN_POINT('Ctrl Pts',(0.155021375999944,12.2,4.45751876499998));
#332075=CARTESIAN_POINT('Ctrl Pts',(0.155021375999944,5.2,4.45751876499998));
#332076=CARTESIAN_POINT('Ctrl Pts',(0.155021375999944,2.2,4.45751876499998));
#332077=CARTESIAN_POINT('Ctrl Pts',(0.153992038999944,12.2,4.45561505699998));
#332078=CARTESIAN_POINT('Ctrl Pts',(0.153992038999944,5.2,4.45561505699998));
#332079=CARTESIAN_POINT('Ctrl Pts',(0.153992038999944,2.2,4.45561505699998));
#332080=CARTESIAN_POINT('Ctrl Pts',(0.152966623999945,12.2,4.45371364899999));
#332081=CARTESIAN_POINT('Ctrl Pts',(0.152966623999945,5.2,4.45371364899999));
#332082=CARTESIAN_POINT('Ctrl Pts',(0.152966623999945,2.2,4.45371364899999));
#332083=CARTESIAN_POINT('Ctrl Pts',(0.151945128999945,12.2,4.45181454999998));
#332084=CARTESIAN_POINT('Ctrl Pts',(0.151945128999945,5.2,4.45181454999998));
#332085=CARTESIAN_POINT('Ctrl Pts',(0.151945128999945,2.2,4.45181454999998));
#332086=CARTESIAN_POINT('Ctrl Pts',(0.150927550999944,12.2,4.44991776899998));
#332087=CARTESIAN_POINT('Ctrl Pts',(0.150927550999944,5.2,4.44991776899998));
#332088=CARTESIAN_POINT('Ctrl Pts',(0.150927550999944,2.2,4.44991776899998));
#332089=CARTESIAN_POINT('Ctrl Pts',(0.149913884999944,12.2,4.44802331699999));
#332090=CARTESIAN_POINT('Ctrl Pts',(0.149913884999944,5.2,4.44802331699999));
#332091=CARTESIAN_POINT('Ctrl Pts',(0.149913884999944,2.2,4.44802331699999));
#332092=CARTESIAN_POINT('Ctrl Pts',(0.148904129999944,12.2,4.44613120299999));
#332093=CARTESIAN_POINT('Ctrl Pts',(0.148904129999944,5.2,4.44613120299999));
#332094=CARTESIAN_POINT('Ctrl Pts',(0.148904129999944,2.2,4.44613120299999));
#332095=CARTESIAN_POINT('Ctrl Pts',(0.147898278999945,12.2,4.44424143699998));
#332096=CARTESIAN_POINT('Ctrl Pts',(0.147898278999945,5.2,4.44424143699998));
#332097=CARTESIAN_POINT('Ctrl Pts',(0.147898278999945,2.2,4.44424143699998));
#332098=CARTESIAN_POINT('Ctrl Pts',(0.146896331999944,12.2,4.44235402799999));
#332099=CARTESIAN_POINT('Ctrl Pts',(0.146896331999944,5.2,4.44235402799999));
#332100=CARTESIAN_POINT('Ctrl Pts',(0.146896331999944,2.2,4.44235402799999));
#332101=CARTESIAN_POINT('Ctrl Pts',(0.145898283999945,12.2,4.44046898699998));
#332102=CARTESIAN_POINT('Ctrl Pts',(0.145898283999945,5.2,4.44046898699998));
#332103=CARTESIAN_POINT('Ctrl Pts',(0.145898283999945,2.2,4.44046898699998));
#332104=CARTESIAN_POINT('Ctrl Pts',(0.144904131999944,12.2,4.43858632299998));
#332105=CARTESIAN_POINT('Ctrl Pts',(0.144904131999944,5.2,4.43858632299998));
#332106=CARTESIAN_POINT('Ctrl Pts',(0.144904131999944,2.2,4.43858632299998));
#332107=CARTESIAN_POINT('Ctrl Pts',(0.143913870999944,12.2,4.43670604599999));
#332108=CARTESIAN_POINT('Ctrl Pts',(0.143913870999944,5.2,4.43670604599999));
#332109=CARTESIAN_POINT('Ctrl Pts',(0.143913870999944,2.2,4.43670604599999));
#332110=CARTESIAN_POINT('Ctrl Pts',(0.142927499999944,12.2,4.43482816499999));
#332111=CARTESIAN_POINT('Ctrl Pts',(0.142927499999944,5.2,4.43482816499999));
#332112=CARTESIAN_POINT('Ctrl Pts',(0.142927499999944,2.2,4.43482816499999));
#332113=CARTESIAN_POINT('Ctrl Pts',(0.141945013999945,12.2,4.43295269099998));
#332114=CARTESIAN_POINT('Ctrl Pts',(0.141945013999945,5.2,4.43295269099998));
#332115=CARTESIAN_POINT('Ctrl Pts',(0.141945013999945,2.2,4.43295269099998));
#332116=CARTESIAN_POINT('Ctrl Pts',(0.140966408999944,12.2,4.43107963199999));
#332117=CARTESIAN_POINT('Ctrl Pts',(0.140966408999944,5.2,4.43107963199999));
#332118=CARTESIAN_POINT('Ctrl Pts',(0.140966408999944,2.2,4.43107963199999));
#332119=CARTESIAN_POINT('Ctrl Pts',(0.139991681999945,12.2,4.42920899999999));
#332120=CARTESIAN_POINT('Ctrl Pts',(0.139991681999945,5.2,4.42920899999999));
#332121=CARTESIAN_POINT('Ctrl Pts',(0.139991681999945,2.2,4.42920899999999));
#332122=CARTESIAN_POINT('Ctrl Pts',(0.139020829999945,12.2,4.42734080299999));
#332123=CARTESIAN_POINT('Ctrl Pts',(0.139020829999945,5.2,4.42734080299999));
#332124=CARTESIAN_POINT('Ctrl Pts',(0.139020829999945,2.2,4.42734080299999));
#332125=CARTESIAN_POINT('Ctrl Pts',(0.138053847999944,12.2,4.42547505199999));
#332126=CARTESIAN_POINT('Ctrl Pts',(0.138053847999944,5.2,4.42547505199999));
#332127=CARTESIAN_POINT('Ctrl Pts',(0.138053847999944,2.2,4.42547505199999));
#332128=CARTESIAN_POINT('Ctrl Pts',(0.137090732999944,12.2,4.42361175499999));
#332129=CARTESIAN_POINT('Ctrl Pts',(0.137090732999944,5.2,4.42361175499999));
#332130=CARTESIAN_POINT('Ctrl Pts',(0.137090732999944,2.2,4.42361175499999));
#332131=CARTESIAN_POINT('Ctrl Pts',(0.136131481999945,12.2,4.42175092399999));
#332132=CARTESIAN_POINT('Ctrl Pts',(0.136131481999945,5.2,4.42175092399999));
#332133=CARTESIAN_POINT('Ctrl Pts',(0.136131481999945,2.2,4.42175092399999));
#332134=CARTESIAN_POINT('Ctrl Pts',(0.135176090999943,12.2,4.41989256899999));
#332135=CARTESIAN_POINT('Ctrl Pts',(0.135176090999943,5.2,4.41989256899999));
#332136=CARTESIAN_POINT('Ctrl Pts',(0.135176090999943,2.2,4.41989256899999));
#332137=CARTESIAN_POINT('Ctrl Pts',(0.134224555999944,12.2,4.41803669699999));
#332138=CARTESIAN_POINT('Ctrl Pts',(0.134224555999944,5.2,4.41803669699999));
#332139=CARTESIAN_POINT('Ctrl Pts',(0.134224555999944,2.2,4.41803669699999));
#332140=CARTESIAN_POINT('Ctrl Pts',(0.133276872999945,12.2,4.41618331999998));
#332141=CARTESIAN_POINT('Ctrl Pts',(0.133276872999945,5.2,4.41618331999998));
#332142=CARTESIAN_POINT('Ctrl Pts',(0.133276872999945,2.2,4.41618331999998));
#332143=CARTESIAN_POINT('Ctrl Pts',(0.132333037999944,12.2,4.41433244799998));
#332144=CARTESIAN_POINT('Ctrl Pts',(0.132333037999944,5.2,4.41433244799998));
#332145=CARTESIAN_POINT('Ctrl Pts',(0.132333037999944,2.2,4.41433244799998));
#332146=CARTESIAN_POINT('Ctrl Pts',(0.131393048999945,12.2,4.41248408899998));
#332147=CARTESIAN_POINT('Ctrl Pts',(0.131393048999945,5.2,4.41248408899998));
#332148=CARTESIAN_POINT('Ctrl Pts',(0.131393048999945,2.2,4.41248408899998));
#332149=CARTESIAN_POINT('Ctrl Pts',(0.130456900999943,12.2,4.41063825499998));
#332150=CARTESIAN_POINT('Ctrl Pts',(0.130456900999943,5.2,4.41063825499998));
#332151=CARTESIAN_POINT('Ctrl Pts',(0.130456900999943,2.2,4.41063825499998));
#332152=CARTESIAN_POINT('Ctrl Pts',(0.129524589999944,12.2,4.40879495599999));
#332153=CARTESIAN_POINT('Ctrl Pts',(0.129524589999944,5.2,4.40879495599999));
#332154=CARTESIAN_POINT('Ctrl Pts',(0.129524589999944,2.2,4.40879495599999));
#332155=CARTESIAN_POINT('Ctrl Pts',(0.128596111999943,12.2,4.40695419999999));
#332156=CARTESIAN_POINT('Ctrl Pts',(0.128596111999943,5.2,4.40695419999999));
#332157=CARTESIAN_POINT('Ctrl Pts',(0.128596111999943,2.2,4.40695419999999));
#332158=CARTESIAN_POINT('Ctrl Pts',(0.127671463999944,12.2,4.40511599799999));
#332159=CARTESIAN_POINT('Ctrl Pts',(0.127671463999944,5.2,4.40511599799999));
#332160=CARTESIAN_POINT('Ctrl Pts',(0.127671463999944,2.2,4.40511599799999));
#332161=CARTESIAN_POINT('Ctrl Pts',(0.126750642999944,12.2,4.40328035999999));
#332162=CARTESIAN_POINT('Ctrl Pts',(0.126750642999944,5.2,4.40328035999999));
#332163=CARTESIAN_POINT('Ctrl Pts',(0.126750642999944,2.2,4.40328035999999));
#332164=CARTESIAN_POINT('Ctrl Pts',(0.125833642999943,12.2,4.40144729499998));
#332165=CARTESIAN_POINT('Ctrl Pts',(0.125833642999943,5.2,4.40144729499998));
#332166=CARTESIAN_POINT('Ctrl Pts',(0.125833642999943,2.2,4.40144729499998));
#332167=CARTESIAN_POINT('Ctrl Pts',(0.124920460999943,12.2,4.39961681499998));
#332168=CARTESIAN_POINT('Ctrl Pts',(0.124920460999943,5.2,4.39961681499998));
#332169=CARTESIAN_POINT('Ctrl Pts',(0.124920460999943,2.2,4.39961681499998));
#332170=CARTESIAN_POINT('Ctrl Pts',(0.124011093999944,12.2,4.39778892799998));
#332171=CARTESIAN_POINT('Ctrl Pts',(0.124011093999944,5.2,4.39778892799998));
#332172=CARTESIAN_POINT('Ctrl Pts',(0.124011093999944,2.2,4.39778892799998));
#332173=CARTESIAN_POINT('Ctrl Pts',(0.123105536999945,12.2,4.39596364399998));
#332174=CARTESIAN_POINT('Ctrl Pts',(0.123105536999945,5.2,4.39596364399998));
#332175=CARTESIAN_POINT('Ctrl Pts',(0.123105536999945,2.2,4.39596364399998));
#332176=CARTESIAN_POINT('Ctrl Pts',(0.122203784999944,12.2,4.39414097499998));
#332177=CARTESIAN_POINT('Ctrl Pts',(0.122203784999944,5.2,4.39414097499998));
#332178=CARTESIAN_POINT('Ctrl Pts',(0.122203784999944,2.2,4.39414097499998));
#332179=CARTESIAN_POINT('Ctrl Pts',(0.121305836999944,12.2,4.39232092799998));
#332180=CARTESIAN_POINT('Ctrl Pts',(0.121305836999944,5.2,4.39232092799998));
#332181=CARTESIAN_POINT('Ctrl Pts',(0.121305836999944,2.2,4.39232092799998));
#332182=CARTESIAN_POINT('Ctrl Pts',(0.120411685999944,12.2,4.39050351499999));
#332183=CARTESIAN_POINT('Ctrl Pts',(0.120411685999944,5.2,4.39050351499999));
#332184=CARTESIAN_POINT('Ctrl Pts',(0.120411685999944,2.2,4.39050351499999));
#332185=CARTESIAN_POINT('Ctrl Pts',(0.119521329999944,12.2,4.38868874599999));
#332186=CARTESIAN_POINT('Ctrl Pts',(0.119521329999944,5.2,4.38868874599999));
#332187=CARTESIAN_POINT('Ctrl Pts',(0.119521329999944,2.2,4.38868874599999));
#332188=CARTESIAN_POINT('Ctrl Pts',(0.118634763999944,12.2,4.38687662999998));
#332189=CARTESIAN_POINT('Ctrl Pts',(0.118634763999944,5.2,4.38687662999998));
#332190=CARTESIAN_POINT('Ctrl Pts',(0.118634763999944,2.2,4.38687662999998));
#332191=CARTESIAN_POINT('Ctrl Pts',(0.117751984999943,12.2,4.38506717799999));
#332192=CARTESIAN_POINT('Ctrl Pts',(0.117751984999943,5.2,4.38506717799999));
#332193=CARTESIAN_POINT('Ctrl Pts',(0.117751984999943,2.2,4.38506717799999));
#332194=CARTESIAN_POINT('Ctrl Pts',(0.116872986999944,12.2,4.38326039899999));
#332195=CARTESIAN_POINT('Ctrl Pts',(0.116872986999944,5.2,4.38326039899999));
#332196=CARTESIAN_POINT('Ctrl Pts',(0.116872986999944,2.2,4.38326039899999));
#332197=CARTESIAN_POINT('Ctrl Pts',(0.115997767999945,12.2,4.38145630499999));
#332198=CARTESIAN_POINT('Ctrl Pts',(0.115997767999945,5.2,4.38145630499999));
#332199=CARTESIAN_POINT('Ctrl Pts',(0.115997767999945,2.2,4.38145630499999));
#332200=CARTESIAN_POINT('Ctrl Pts',(0.115126322999943,12.2,4.37965490299998));
#332201=CARTESIAN_POINT('Ctrl Pts',(0.115126322999943,5.2,4.37965490299998));
#332202=CARTESIAN_POINT('Ctrl Pts',(0.115126322999943,2.2,4.37965490299998));
#332203=CARTESIAN_POINT('Ctrl Pts',(0.114258647999945,12.2,4.37785620599998));
#332204=CARTESIAN_POINT('Ctrl Pts',(0.114258647999945,5.2,4.37785620599998));
#332205=CARTESIAN_POINT('Ctrl Pts',(0.114258647999945,2.2,4.37785620599998));
#332206=CARTESIAN_POINT('Ctrl Pts',(0.113394737999943,12.2,4.37606022199999));
#332207=CARTESIAN_POINT('Ctrl Pts',(0.113394737999943,5.2,4.37606022199999));
#332208=CARTESIAN_POINT('Ctrl Pts',(0.113394737999943,2.2,4.37606022199999));
#332209=CARTESIAN_POINT('Ctrl Pts',(0.112534589999944,12.2,4.37426696199999));
#332210=CARTESIAN_POINT('Ctrl Pts',(0.112534589999944,5.2,4.37426696199999));
#332211=CARTESIAN_POINT('Ctrl Pts',(0.112534589999944,2.2,4.37426696199999));
#332212=CARTESIAN_POINT('Ctrl Pts',(0.111678198999944,12.2,4.37247643699998));
#332213=CARTESIAN_POINT('Ctrl Pts',(0.111678198999944,5.2,4.37247643699998));
#332214=CARTESIAN_POINT('Ctrl Pts',(0.111678198999944,2.2,4.37247643699998));
#332215=CARTESIAN_POINT('Ctrl Pts',(0.110825560999944,12.2,4.37068865499998));
#332216=CARTESIAN_POINT('Ctrl Pts',(0.110825560999944,5.2,4.37068865499998));
#332217=CARTESIAN_POINT('Ctrl Pts',(0.110825560999944,2.2,4.37068865499998));
#332218=CARTESIAN_POINT('Ctrl Pts',(0.109976672999944,12.2,4.36890362799998));
#332219=CARTESIAN_POINT('Ctrl Pts',(0.109976672999944,5.2,4.36890362799998));
#332220=CARTESIAN_POINT('Ctrl Pts',(0.109976672999944,2.2,4.36890362799998));
#332221=CARTESIAN_POINT('Ctrl Pts',(0.109131527999944,12.2,4.36712136499998));
#332222=CARTESIAN_POINT('Ctrl Pts',(0.109131527999944,5.2,4.36712136499998));
#332223=CARTESIAN_POINT('Ctrl Pts',(0.109131527999944,2.2,4.36712136499998));
#332224=CARTESIAN_POINT('Ctrl Pts',(0.108290123999945,12.2,4.36534187599998));
#332225=CARTESIAN_POINT('Ctrl Pts',(0.108290123999945,5.2,4.36534187599998));
#332226=CARTESIAN_POINT('Ctrl Pts',(0.108290123999945,2.2,4.36534187599998));
#332227=CARTESIAN_POINT('Ctrl Pts',(0.107452456999945,12.2,4.36356517299998));
#332228=CARTESIAN_POINT('Ctrl Pts',(0.107452456999945,5.2,4.36356517299998));
#332229=CARTESIAN_POINT('Ctrl Pts',(0.107452456999945,2.2,4.36356517299998));
#332230=CARTESIAN_POINT('Ctrl Pts',(0.106618521999945,12.2,4.36179126299999));
#332231=CARTESIAN_POINT('Ctrl Pts',(0.106618521999945,5.2,4.36179126299999));
#332232=CARTESIAN_POINT('Ctrl Pts',(0.106618521999945,2.2,4.36179126299999));
#332233=CARTESIAN_POINT('Ctrl Pts',(0.105788312999945,12.2,4.36002015999998));
#332234=CARTESIAN_POINT('Ctrl Pts',(0.105788312999945,5.2,4.36002015999998));
#332235=CARTESIAN_POINT('Ctrl Pts',(0.105788312999945,2.2,4.36002015999998));
#332236=CARTESIAN_POINT('Ctrl Pts',(0.104961826999944,12.2,4.35825186999999));
#332237=CARTESIAN_POINT('Ctrl Pts',(0.104961826999944,5.2,4.35825186999999));
#332238=CARTESIAN_POINT('Ctrl Pts',(0.104961826999944,2.2,4.35825186999999));
#332239=CARTESIAN_POINT('Ctrl Pts',(0.104139060999945,12.2,4.35648640699998));
#332240=CARTESIAN_POINT('Ctrl Pts',(0.104139060999945,5.2,4.35648640699998));
#332241=CARTESIAN_POINT('Ctrl Pts',(0.104139060999945,2.2,4.35648640699998));
#332242=CARTESIAN_POINT('Ctrl Pts',(0.103320008999944,12.2,4.35472377899998));
#332243=CARTESIAN_POINT('Ctrl Pts',(0.103320008999944,5.2,4.35472377899998));
#332244=CARTESIAN_POINT('Ctrl Pts',(0.103320008999944,2.2,4.35472377899998));
#332245=CARTESIAN_POINT('Ctrl Pts',(0.102504665999945,12.2,4.35296399599999));
#332246=CARTESIAN_POINT('Ctrl Pts',(0.102504665999945,5.2,4.35296399599999));
#332247=CARTESIAN_POINT('Ctrl Pts',(0.102504665999945,2.2,4.35296399599999));
#332248=CARTESIAN_POINT('Ctrl Pts',(0.101693028999945,12.2,4.35120706999999));
#332249=CARTESIAN_POINT('Ctrl Pts',(0.101693028999945,5.2,4.35120706999999));
#332250=CARTESIAN_POINT('Ctrl Pts',(0.101693028999945,2.2,4.35120706999999));
#332251=CARTESIAN_POINT('Ctrl Pts',(0.100885093999944,12.2,4.34945300999999));
#332252=CARTESIAN_POINT('Ctrl Pts',(0.100885093999944,5.2,4.34945300999999));
#332253=CARTESIAN_POINT('Ctrl Pts',(0.100885093999944,2.2,4.34945300999999));
#332254=CARTESIAN_POINT('Ctrl Pts',(0.100080853999945,12.2,4.34770182599999));
#332255=CARTESIAN_POINT('Ctrl Pts',(0.100080853999945,5.2,4.34770182599999));
#332256=CARTESIAN_POINT('Ctrl Pts',(0.100080853999945,2.2,4.34770182599999));
#332257=CARTESIAN_POINT('Ctrl Pts',(0.0992803059999436,12.2,4.34595352899999));
#332258=CARTESIAN_POINT('Ctrl Pts',(0.0992803059999436,5.2,4.34595352899999));
#332259=CARTESIAN_POINT('Ctrl Pts',(0.0992803059999436,2.2,4.34595352899999));
#332260=CARTESIAN_POINT('Ctrl Pts',(0.0984834469999452,12.2,4.34420812899998));
#332261=CARTESIAN_POINT('Ctrl Pts',(0.0984834469999452,5.2,4.34420812899998));
#332262=CARTESIAN_POINT('Ctrl Pts',(0.0984834469999452,2.2,4.34420812899998));
#332263=CARTESIAN_POINT('Ctrl Pts',(0.0976902699999449,12.2,4.34246563599999));
#332264=CARTESIAN_POINT('Ctrl Pts',(0.0976902699999449,5.2,4.34246563599999));
#332265=CARTESIAN_POINT('Ctrl Pts',(0.0976902699999449,2.2,4.34246563599999));
#332266=CARTESIAN_POINT('Ctrl Pts',(0.0969007709999448,12.2,4.34072606099999));
#332267=CARTESIAN_POINT('Ctrl Pts',(0.0969007709999448,5.2,4.34072606099999));
#332268=CARTESIAN_POINT('Ctrl Pts',(0.0969007709999448,2.2,4.34072606099999));
#332269=CARTESIAN_POINT('Ctrl Pts',(0.0961149459999433,12.2,4.33898941299999));
#332270=CARTESIAN_POINT('Ctrl Pts',(0.0961149459999433,5.2,4.33898941299999));
#332271=CARTESIAN_POINT('Ctrl Pts',(0.0961149459999433,2.2,4.33898941299999));
#332272=CARTESIAN_POINT('Ctrl Pts',(0.0953327899999434,12.2,4.33725570399999));
#332273=CARTESIAN_POINT('Ctrl Pts',(0.0953327899999434,5.2,4.33725570399999));
#332274=CARTESIAN_POINT('Ctrl Pts',(0.0953327899999434,2.2,4.33725570399999));
#332275=CARTESIAN_POINT('Ctrl Pts',(0.0945542979999436,12.2,4.33552494299998));
#332276=CARTESIAN_POINT('Ctrl Pts',(0.0945542979999436,5.2,4.33552494299998));
#332277=CARTESIAN_POINT('Ctrl Pts',(0.0945542979999436,2.2,4.33552494299998));
#332278=CARTESIAN_POINT('Ctrl Pts',(0.0937794679999449,12.2,4.33379714099999));
#332279=CARTESIAN_POINT('Ctrl Pts',(0.0937794679999449,5.2,4.33379714099999));
#332280=CARTESIAN_POINT('Ctrl Pts',(0.0937794679999449,2.2,4.33379714099999));
#332281=CARTESIAN_POINT('Ctrl Pts',(0.0930082919999442,12.2,4.33207230799999));
#332282=CARTESIAN_POINT('Ctrl Pts',(0.0930082919999442,5.2,4.33207230799999));
#332283=CARTESIAN_POINT('Ctrl Pts',(0.0930082919999442,2.2,4.33207230799999));
#332284=CARTESIAN_POINT('Ctrl Pts',(0.0922407659999447,12.2,4.33035045399999));
#332285=CARTESIAN_POINT('Ctrl Pts',(0.0922407659999447,5.2,4.33035045399999));
#332286=CARTESIAN_POINT('Ctrl Pts',(0.0922407659999447,2.2,4.33035045399999));
#332287=CARTESIAN_POINT('Ctrl Pts',(0.0914768859999437,12.2,4.32863159099998));
#332288=CARTESIAN_POINT('Ctrl Pts',(0.0914768859999437,5.2,4.32863159099998));
#332289=CARTESIAN_POINT('Ctrl Pts',(0.0914768859999437,2.2,4.32863159099998));
#332290=CARTESIAN_POINT('Ctrl Pts',(0.0907166469999443,12.2,4.32691572699999));
#332291=CARTESIAN_POINT('Ctrl Pts',(0.0907166469999443,5.2,4.32691572699999));
#332292=CARTESIAN_POINT('Ctrl Pts',(0.0907166469999443,2.2,4.32691572699999));
#332293=CARTESIAN_POINT('Ctrl Pts',(0.0899600449999449,12.2,4.32520287399999));
#332294=CARTESIAN_POINT('Ctrl Pts',(0.0899600449999449,5.2,4.32520287399999));
#332295=CARTESIAN_POINT('Ctrl Pts',(0.0899600449999449,2.2,4.32520287399999));
#332296=CARTESIAN_POINT('Ctrl Pts',(0.0892070729999439,12.2,4.32349304199998));
#332297=CARTESIAN_POINT('Ctrl Pts',(0.0892070729999439,5.2,4.32349304199998));
#332298=CARTESIAN_POINT('Ctrl Pts',(0.0892070729999439,2.2,4.32349304199998));
#332299=CARTESIAN_POINT('Ctrl Pts',(0.0884577279999454,12.2,4.32178624099999));
#332300=CARTESIAN_POINT('Ctrl Pts',(0.0884577279999454,5.2,4.32178624099999));
#332301=CARTESIAN_POINT('Ctrl Pts',(0.0884577279999454,2.2,4.32178624099999));
#332302=CARTESIAN_POINT('Ctrl Pts',(0.0877120049999436,12.2,4.32008248299999));
#332303=CARTESIAN_POINT('Ctrl Pts',(0.0877120049999436,5.2,4.32008248299999));
#332304=CARTESIAN_POINT('Ctrl Pts',(0.0877120049999436,2.2,4.32008248299999));
#332305=CARTESIAN_POINT('Ctrl Pts',(0.0869698999999446,12.2,4.31838177599998));
#332306=CARTESIAN_POINT('Ctrl Pts',(0.0869698999999446,5.2,4.31838177599998));
#332307=CARTESIAN_POINT('Ctrl Pts',(0.0869698999999446,2.2,4.31838177599998));
#332308=CARTESIAN_POINT('Ctrl Pts',(0.0862314059999447,12.2,4.31668413199999));
#332309=CARTESIAN_POINT('Ctrl Pts',(0.0862314059999447,5.2,4.31668413199999));
#332310=CARTESIAN_POINT('Ctrl Pts',(0.0862314059999447,2.2,4.31668413199999));
#332311=CARTESIAN_POINT('Ctrl Pts',(0.0854965199999447,12.2,4.31498956099999));
#332312=CARTESIAN_POINT('Ctrl Pts',(0.0854965199999447,5.2,4.31498956099999));
#332313=CARTESIAN_POINT('Ctrl Pts',(0.0854965199999447,2.2,4.31498956099999));
#332314=CARTESIAN_POINT('Ctrl Pts',(0.084765235999944,12.2,4.31329807399998));
#332315=CARTESIAN_POINT('Ctrl Pts',(0.084765235999944,5.2,4.31329807399998));
#332316=CARTESIAN_POINT('Ctrl Pts',(0.084765235999944,2.2,4.31329807399998));
#332317=CARTESIAN_POINT('Ctrl Pts',(0.0840375479999445,12.2,4.31160968099999));
#332318=CARTESIAN_POINT('Ctrl Pts',(0.0840375479999445,5.2,4.31160968099999));
#332319=CARTESIAN_POINT('Ctrl Pts',(0.0840375479999445,2.2,4.31160968099999));
#332320=CARTESIAN_POINT('Ctrl Pts',(0.0833134539999436,12.2,4.30992439199999));
#332321=CARTESIAN_POINT('Ctrl Pts',(0.0833134539999436,5.2,4.30992439199999));
#332322=CARTESIAN_POINT('Ctrl Pts',(0.0833134539999436,2.2,4.30992439199999));
#332323=CARTESIAN_POINT('Ctrl Pts',(0.0825929469999431,12.2,4.30824221899999));
#332324=CARTESIAN_POINT('Ctrl Pts',(0.0825929469999431,5.2,4.30824221899999));
#332325=CARTESIAN_POINT('Ctrl Pts',(0.0825929469999431,2.2,4.30824221899999));
#332326=CARTESIAN_POINT('Ctrl Pts',(0.0818760219999448,12.2,4.30656317199999));
#332327=CARTESIAN_POINT('Ctrl Pts',(0.0818760219999448,5.2,4.30656317199999));
#332328=CARTESIAN_POINT('Ctrl Pts',(0.0818760219999448,2.2,4.30656317199999));
#332329=CARTESIAN_POINT('Ctrl Pts',(0.0811626739999449,12.2,4.30488725899998));
#332330=CARTESIAN_POINT('Ctrl Pts',(0.0811626739999449,5.2,4.30488725899998));
#332331=CARTESIAN_POINT('Ctrl Pts',(0.0811626739999449,2.2,4.30488725899998));
#332332=CARTESIAN_POINT('Ctrl Pts',(0.0804528979999442,12.2,4.30321449499999));
#332333=CARTESIAN_POINT('Ctrl Pts',(0.0804528979999442,5.2,4.30321449499999));
#332334=CARTESIAN_POINT('Ctrl Pts',(0.0804528979999442,2.2,4.30321449499999));
#332335=CARTESIAN_POINT('Ctrl Pts',(0.0797466899999433,12.2,4.30154488699999));
#332336=CARTESIAN_POINT('Ctrl Pts',(0.0797466899999433,5.2,4.30154488699999));
#332337=CARTESIAN_POINT('Ctrl Pts',(0.0797466899999433,2.2,4.30154488699999));
#332338=CARTESIAN_POINT('Ctrl Pts',(0.0790440439999451,12.2,4.29987844599999));
#332339=CARTESIAN_POINT('Ctrl Pts',(0.0790440439999451,5.2,4.29987844599999));
#332340=CARTESIAN_POINT('Ctrl Pts',(0.0790440439999451,2.2,4.29987844599999));
#332341=CARTESIAN_POINT('Ctrl Pts',(0.0783449549999438,12.2,4.29821518399999));
#332342=CARTESIAN_POINT('Ctrl Pts',(0.0783449549999438,5.2,4.29821518399999));
#332343=CARTESIAN_POINT('Ctrl Pts',(0.0783449549999438,2.2,4.29821518399999));
#332344=CARTESIAN_POINT('Ctrl Pts',(0.0776494169999431,12.2,4.29655511099998));
#332345=CARTESIAN_POINT('Ctrl Pts',(0.0776494169999431,5.2,4.29655511099998));
#332346=CARTESIAN_POINT('Ctrl Pts',(0.0776494169999431,2.2,4.29655511099998));
#332347=CARTESIAN_POINT('Ctrl Pts',(0.076957425999945,12.2,4.29489823699999));
#332348=CARTESIAN_POINT('Ctrl Pts',(0.076957425999945,5.2,4.29489823699999));
#332349=CARTESIAN_POINT('Ctrl Pts',(0.076957425999945,2.2,4.29489823699999));
#332350=CARTESIAN_POINT('Ctrl Pts',(0.0762689769999447,12.2,4.29324457299998));
#332351=CARTESIAN_POINT('Ctrl Pts',(0.0762689769999447,5.2,4.29324457299998));
#332352=CARTESIAN_POINT('Ctrl Pts',(0.0762689769999447,2.2,4.29324457299998));
#332353=CARTESIAN_POINT('Ctrl Pts',(0.0755840629999438,12.2,4.29159412999999));
#332354=CARTESIAN_POINT('Ctrl Pts',(0.0755840629999438,5.2,4.29159412999999));
#332355=CARTESIAN_POINT('Ctrl Pts',(0.0755840629999438,2.2,4.29159412999999));
#332356=CARTESIAN_POINT('Ctrl Pts',(0.0749026809999442,12.2,4.28994691799998));
#332357=CARTESIAN_POINT('Ctrl Pts',(0.0749026809999442,5.2,4.28994691799998));
#332358=CARTESIAN_POINT('Ctrl Pts',(0.0749026809999442,2.2,4.28994691799998));
#332359=CARTESIAN_POINT('Ctrl Pts',(0.0742248239999454,12.2,4.28830294699999));
#332360=CARTESIAN_POINT('Ctrl Pts',(0.0742248239999454,5.2,4.28830294699999));
#332361=CARTESIAN_POINT('Ctrl Pts',(0.0742248239999454,2.2,4.28830294699999));
#332362=CARTESIAN_POINT('Ctrl Pts',(0.0735504879999438,12.2,4.28666222999999));
#332363=CARTESIAN_POINT('Ctrl Pts',(0.0735504879999438,5.2,4.28666222999999));
#332364=CARTESIAN_POINT('Ctrl Pts',(0.0735504879999438,2.2,4.28666222999999));
#332365=CARTESIAN_POINT('Ctrl Pts',(0.0728796659999442,12.2,4.28502477699999));
#332366=CARTESIAN_POINT('Ctrl Pts',(0.0728796659999442,5.2,4.28502477699999));
#332367=CARTESIAN_POINT('Ctrl Pts',(0.0728796659999442,2.2,4.28502477699999));
#332368=CARTESIAN_POINT('Ctrl Pts',(0.0722123539999442,12.2,4.28339059599999));
#332369=CARTESIAN_POINT('Ctrl Pts',(0.0722123539999442,5.2,4.28339059599999));
#332370=CARTESIAN_POINT('Ctrl Pts',(0.0722123539999442,2.2,4.28339059599999));
#332371=CARTESIAN_POINT('Ctrl Pts',(0.0715485469999444,12.2,4.28175969999998));
#332372=CARTESIAN_POINT('Ctrl Pts',(0.0715485469999444,5.2,4.28175969999998));
#332373=CARTESIAN_POINT('Ctrl Pts',(0.0715485469999444,2.2,4.28175969999998));
#332374=CARTESIAN_POINT('Ctrl Pts',(0.0708882379999431,12.2,4.28013209899999));
#332375=CARTESIAN_POINT('Ctrl Pts',(0.0708882379999431,5.2,4.28013209899999));
#332376=CARTESIAN_POINT('Ctrl Pts',(0.0708882379999431,2.2,4.28013209899999));
#332377=CARTESIAN_POINT('Ctrl Pts',(0.0702314229999445,12.2,4.27850780499998));
#332378=CARTESIAN_POINT('Ctrl Pts',(0.0702314229999445,5.2,4.27850780499998));
#332379=CARTESIAN_POINT('Ctrl Pts',(0.0702314229999445,2.2,4.27850780499998));
#332380=CARTESIAN_POINT('Ctrl Pts',(0.0695780959999437,12.2,4.27688682699999));
#332381=CARTESIAN_POINT('Ctrl Pts',(0.0695780959999437,5.2,4.27688682699999));
#332382=CARTESIAN_POINT('Ctrl Pts',(0.0695780959999437,2.2,4.27688682699999));
#332383=CARTESIAN_POINT('Ctrl Pts',(0.0689282519999446,12.2,4.27526917599998));
#332384=CARTESIAN_POINT('Ctrl Pts',(0.0689282519999446,5.2,4.27526917599998));
#332385=CARTESIAN_POINT('Ctrl Pts',(0.0689282519999446,2.2,4.27526917599998));
#332386=CARTESIAN_POINT('Ctrl Pts',(0.0682818839999444,12.2,4.27365486399999));
#332387=CARTESIAN_POINT('Ctrl Pts',(0.0682818839999444,5.2,4.27365486399999));
#332388=CARTESIAN_POINT('Ctrl Pts',(0.0682818839999444,2.2,4.27365486399999));
#332389=CARTESIAN_POINT('Ctrl Pts',(0.067638988999944,12.2,4.27204390099998));
#332390=CARTESIAN_POINT('Ctrl Pts',(0.067638988999944,5.2,4.27204390099998));
#332391=CARTESIAN_POINT('Ctrl Pts',(0.067638988999944,2.2,4.27204390099998));
#332392=CARTESIAN_POINT('Ctrl Pts',(0.0669995589999439,12.2,4.27043629599999));
#332393=CARTESIAN_POINT('Ctrl Pts',(0.0669995589999439,5.2,4.27043629599999));
#332394=CARTESIAN_POINT('Ctrl Pts',(0.0669995589999439,2.2,4.27043629599999));
#332395=CARTESIAN_POINT('Ctrl Pts',(0.0663635899999437,12.2,4.26883206299999));
#332396=CARTESIAN_POINT('Ctrl Pts',(0.0663635899999437,5.2,4.26883206299999));
#332397=CARTESIAN_POINT('Ctrl Pts',(0.0663635899999437,2.2,4.26883206299999));
#332398=CARTESIAN_POINT('Ctrl Pts',(0.065731074999944,12.2,4.26723121099998));
#332399=CARTESIAN_POINT('Ctrl Pts',(0.065731074999944,5.2,4.26723121099998));
#332400=CARTESIAN_POINT('Ctrl Pts',(0.065731074999944,2.2,4.26723121099998));
#332401=CARTESIAN_POINT('Ctrl Pts',(0.0651020109999434,12.2,4.26563375099998));
#332402=CARTESIAN_POINT('Ctrl Pts',(0.0651020109999434,5.2,4.26563375099998));
#332403=CARTESIAN_POINT('Ctrl Pts',(0.0651020109999434,2.2,4.26563375099998));
#332404=CARTESIAN_POINT('Ctrl Pts',(0.0644763889999444,12.2,4.26403969299999));
#332405=CARTESIAN_POINT('Ctrl Pts',(0.0644763889999444,5.2,4.26403969299999));
#332406=CARTESIAN_POINT('Ctrl Pts',(0.0644763889999444,2.2,4.26403969299999));
#332407=CARTESIAN_POINT('Ctrl Pts',(0.0638542059999436,12.2,4.26244904999999));
#332408=CARTESIAN_POINT('Ctrl Pts',(0.0638542059999436,5.2,4.26244904999999));
#332409=CARTESIAN_POINT('Ctrl Pts',(0.0638542059999436,2.2,4.26244904999999));
#332410=CARTESIAN_POINT('Ctrl Pts',(0.0632354539999447,12.2,4.26086183099999));
#332411=CARTESIAN_POINT('Ctrl Pts',(0.0632354539999447,5.2,4.26086183099999));
#332412=CARTESIAN_POINT('Ctrl Pts',(0.0632354539999447,2.2,4.26086183099999));
#332413=CARTESIAN_POINT('Ctrl Pts',(0.062620129999944,12.2,4.25927804699998));
#332414=CARTESIAN_POINT('Ctrl Pts',(0.062620129999944,5.2,4.25927804699998));
#332415=CARTESIAN_POINT('Ctrl Pts',(0.062620129999944,2.2,4.25927804699998));
#332416=CARTESIAN_POINT('Ctrl Pts',(0.0620082269999445,12.2,4.25769770899999));
#332417=CARTESIAN_POINT('Ctrl Pts',(0.0620082269999445,5.2,4.25769770899999));
#332418=CARTESIAN_POINT('Ctrl Pts',(0.0620082269999445,2.2,4.25769770899999));
#332419=CARTESIAN_POINT('Ctrl Pts',(0.0613997379999442,12.2,4.25612082899999));
#332420=CARTESIAN_POINT('Ctrl Pts',(0.0613997379999442,5.2,4.25612082899999));
#332421=CARTESIAN_POINT('Ctrl Pts',(0.0613997379999442,2.2,4.25612082899999));
#332422=CARTESIAN_POINT('Ctrl Pts',(0.0607946599999443,12.2,4.25454741599999));
#332423=CARTESIAN_POINT('Ctrl Pts',(0.0607946599999443,5.2,4.25454741599999));
#332424=CARTESIAN_POINT('Ctrl Pts',(0.0607946599999443,2.2,4.25454741599999));
#332425=CARTESIAN_POINT('Ctrl Pts',(0.0601929839999438,12.2,4.25297748199998));
#332426=CARTESIAN_POINT('Ctrl Pts',(0.0601929839999438,5.2,4.25297748199998));
#332427=CARTESIAN_POINT('Ctrl Pts',(0.0601929839999438,2.2,4.25297748199998));
#332428=CARTESIAN_POINT('Ctrl Pts',(0.0595947059999435,12.2,4.25141103799999));
#332429=CARTESIAN_POINT('Ctrl Pts',(0.0595947059999435,5.2,4.25141103799999));
#332430=CARTESIAN_POINT('Ctrl Pts',(0.0595947059999435,2.2,4.25141103799999));
#332431=CARTESIAN_POINT('Ctrl Pts',(0.0589998189999441,12.2,4.24984809499998));
#332432=CARTESIAN_POINT('Ctrl Pts',(0.0589998189999441,5.2,4.24984809499998));
#332433=CARTESIAN_POINT('Ctrl Pts',(0.0589998189999441,2.2,4.24984809499998));
#332434=CARTESIAN_POINT('Ctrl Pts',(0.0584083189999451,12.2,4.24828866399999));
#332435=CARTESIAN_POINT('Ctrl Pts',(0.0584083189999451,5.2,4.24828866399999));
#332436=CARTESIAN_POINT('Ctrl Pts',(0.0584083189999451,2.2,4.24828866399999));
#332437=CARTESIAN_POINT('Ctrl Pts',(0.0578201979999437,12.2,4.24673275499998));
#332438=CARTESIAN_POINT('Ctrl Pts',(0.0578201979999437,5.2,4.24673275499998));
#332439=CARTESIAN_POINT('Ctrl Pts',(0.0578201979999437,2.2,4.24673275499998));
#332440=CARTESIAN_POINT('Ctrl Pts',(0.0572354519999441,12.2,4.24518037899999));
#332441=CARTESIAN_POINT('Ctrl Pts',(0.0572354519999441,5.2,4.24518037899999));
#332442=CARTESIAN_POINT('Ctrl Pts',(0.0572354519999441,2.2,4.24518037899999));
#332443=CARTESIAN_POINT('Ctrl Pts',(0.0566540739999444,12.2,4.24363154799998));
#332444=CARTESIAN_POINT('Ctrl Pts',(0.0566540739999444,5.2,4.24363154799998));
#332445=CARTESIAN_POINT('Ctrl Pts',(0.0566540739999444,2.2,4.24363154799998));
#332446=CARTESIAN_POINT('Ctrl Pts',(0.0560760579999442,12.2,4.24208627199998));
#332447=CARTESIAN_POINT('Ctrl Pts',(0.0560760579999442,5.2,4.24208627199998));
#332448=CARTESIAN_POINT('Ctrl Pts',(0.0560760579999442,2.2,4.24208627199998));
#332449=CARTESIAN_POINT('Ctrl Pts',(0.0555013979999441,12.2,4.24054456199999));
#332450=CARTESIAN_POINT('Ctrl Pts',(0.0555013979999441,5.2,4.24054456199999));
#332451=CARTESIAN_POINT('Ctrl Pts',(0.0555013979999441,2.2,4.24054456199999));
#332452=CARTESIAN_POINT('Ctrl Pts',(0.0549300879999437,12.2,4.23900643199998));
#332453=CARTESIAN_POINT('Ctrl Pts',(0.0549300879999437,5.2,4.23900643199998));
#332454=CARTESIAN_POINT('Ctrl Pts',(0.0549300879999437,2.2,4.23900643199998));
#332455=CARTESIAN_POINT('Ctrl Pts',(0.0543621219999435,12.2,4.23747188799998));
#332456=CARTESIAN_POINT('Ctrl Pts',(0.0543621219999435,5.2,4.23747188799998));
#332457=CARTESIAN_POINT('Ctrl Pts',(0.0543621219999435,2.2,4.23747188799998));
#332458=CARTESIAN_POINT('Ctrl Pts',(0.0537974939999442,12.2,4.23594094499999));
#332459=CARTESIAN_POINT('Ctrl Pts',(0.0537974939999442,5.2,4.23594094499999));
#332460=CARTESIAN_POINT('Ctrl Pts',(0.0537974939999442,2.2,4.23594094499999));
#332461=CARTESIAN_POINT('Ctrl Pts',(0.053236196999944,12.2,4.23441361199998));
#332462=CARTESIAN_POINT('Ctrl Pts',(0.053236196999944,5.2,4.23441361199998));
#332463=CARTESIAN_POINT('Ctrl Pts',(0.053236196999944,2.2,4.23441361199998));
#332464=CARTESIAN_POINT('Ctrl Pts',(0.0526782259999448,12.2,4.23288990099999));
#332465=CARTESIAN_POINT('Ctrl Pts',(0.0526782259999448,5.2,4.23288990099999));
#332466=CARTESIAN_POINT('Ctrl Pts',(0.0526782259999448,2.2,4.23288990099999));
#332467=CARTESIAN_POINT('Ctrl Pts',(0.0521235739999448,12.2,4.23136982199999));
#332468=CARTESIAN_POINT('Ctrl Pts',(0.0521235739999448,5.2,4.23136982199999));
#332469=CARTESIAN_POINT('Ctrl Pts',(0.0521235739999448,2.2,4.23136982199999));
#332470=CARTESIAN_POINT('Ctrl Pts',(0.0515722369999438,12.2,4.22985338699998));
#332471=CARTESIAN_POINT('Ctrl Pts',(0.0515722369999438,5.2,4.22985338699998));
#332472=CARTESIAN_POINT('Ctrl Pts',(0.0515722369999438,2.2,4.22985338699998));
#332473=CARTESIAN_POINT('Ctrl Pts',(0.0510242039999442,12.2,4.22834060799998));
#332474=CARTESIAN_POINT('Ctrl Pts',(0.0510242039999442,5.2,4.22834060799998));
#332475=CARTESIAN_POINT('Ctrl Pts',(0.0510242039999442,2.2,4.22834060799998));
#332476=CARTESIAN_POINT('Ctrl Pts',(0.0504794739999448,12.2,4.22683149399998));
#332477=CARTESIAN_POINT('Ctrl Pts',(0.0504794739999448,5.2,4.22683149399998));
#332478=CARTESIAN_POINT('Ctrl Pts',(0.0504794739999448,2.2,4.22683149399998));
#332479=CARTESIAN_POINT('Ctrl Pts',(0.0499380369999436,12.2,4.22532605799999));
#332480=CARTESIAN_POINT('Ctrl Pts',(0.0499380369999436,5.2,4.22532605799999));
#332481=CARTESIAN_POINT('Ctrl Pts',(0.0499380369999436,2.2,4.22532605799999));
#332482=CARTESIAN_POINT('Ctrl Pts',(0.0493998889999436,12.2,4.22382430899999));
#332483=CARTESIAN_POINT('Ctrl Pts',(0.0493998889999436,5.2,4.22382430899999));
#332484=CARTESIAN_POINT('Ctrl Pts',(0.0493998889999436,2.2,4.22382430899999));
#332485=CARTESIAN_POINT('Ctrl Pts',(0.0488650229999443,12.2,4.22232625999998));
#332486=CARTESIAN_POINT('Ctrl Pts',(0.0488650229999443,5.2,4.22232625999998));
#332487=CARTESIAN_POINT('Ctrl Pts',(0.0488650229999443,2.2,4.22232625999998));
#332488=CARTESIAN_POINT('Ctrl Pts',(0.0483334319999451,12.2,4.22083192199998));
#332489=CARTESIAN_POINT('Ctrl Pts',(0.0483334319999451,5.2,4.22083192199998));
#332490=CARTESIAN_POINT('Ctrl Pts',(0.0483334319999451,2.2,4.22083192199998));
#332491=CARTESIAN_POINT('Ctrl Pts',(0.0478051099999444,12.2,4.21934130599999));
#332492=CARTESIAN_POINT('Ctrl Pts',(0.0478051099999444,5.2,4.21934130599999));
#332493=CARTESIAN_POINT('Ctrl Pts',(0.0478051099999444,2.2,4.21934130599999));
#332494=CARTESIAN_POINT('Ctrl Pts',(0.0472800499999448,12.2,4.21785442199998));
#332495=CARTESIAN_POINT('Ctrl Pts',(0.0472800499999448,5.2,4.21785442199998));
#332496=CARTESIAN_POINT('Ctrl Pts',(0.0472800499999448,2.2,4.21785442199998));
#332497=CARTESIAN_POINT('Ctrl Pts',(0.046758246999945,12.2,4.21637128399999));
#332498=CARTESIAN_POINT('Ctrl Pts',(0.046758246999945,5.2,4.21637128399999));
#332499=CARTESIAN_POINT('Ctrl Pts',(0.046758246999945,2.2,4.21637128399999));
#332500=CARTESIAN_POINT('Ctrl Pts',(0.0462396929999442,12.2,4.21489189899999));
#332501=CARTESIAN_POINT('Ctrl Pts',(0.0462396929999442,5.2,4.21489189899999));
#332502=CARTESIAN_POINT('Ctrl Pts',(0.0462396929999442,2.2,4.21489189899999));
#332503=CARTESIAN_POINT('Ctrl Pts',(0.0457243829999443,12.2,4.21341628199999));
#332504=CARTESIAN_POINT('Ctrl Pts',(0.0457243829999443,5.2,4.21341628199999));
#332505=CARTESIAN_POINT('Ctrl Pts',(0.0457243829999443,2.2,4.21341628199999));
#332506=CARTESIAN_POINT('Ctrl Pts',(0.0452123089999434,12.2,4.21194444299999));
#332507=CARTESIAN_POINT('Ctrl Pts',(0.0452123089999434,5.2,4.21194444299999));
#332508=CARTESIAN_POINT('Ctrl Pts',(0.0452123089999434,2.2,4.21194444299999));
#332509=CARTESIAN_POINT('Ctrl Pts',(0.0447034649999445,12.2,4.21047639199998));
#332510=CARTESIAN_POINT('Ctrl Pts',(0.0447034649999445,5.2,4.21047639199998));
#332511=CARTESIAN_POINT('Ctrl Pts',(0.0447034649999445,2.2,4.21047639199998));
#332512=CARTESIAN_POINT('Ctrl Pts',(0.0441978439999446,12.2,4.20901214299998));
#332513=CARTESIAN_POINT('Ctrl Pts',(0.0441978439999446,5.2,4.20901214299998));
#332514=CARTESIAN_POINT('Ctrl Pts',(0.0441978439999446,2.2,4.20901214299998));
#332515=CARTESIAN_POINT('Ctrl Pts',(0.0436954399999434,12.2,4.20755170399998));
#332516=CARTESIAN_POINT('Ctrl Pts',(0.0436954399999434,5.2,4.20755170399998));
#332517=CARTESIAN_POINT('Ctrl Pts',(0.0436954399999434,2.2,4.20755170399998));
#332518=CARTESIAN_POINT('Ctrl Pts',(0.0431962469999447,12.2,4.20609508999998));
#332519=CARTESIAN_POINT('Ctrl Pts',(0.0431962469999447,5.2,4.20609508999998));
#332520=CARTESIAN_POINT('Ctrl Pts',(0.0431962469999447,2.2,4.20609508999998));
#332521=CARTESIAN_POINT('Ctrl Pts',(0.0427002569999435,12.2,4.20464230799999));
#332522=CARTESIAN_POINT('Ctrl Pts',(0.0427002569999435,5.2,4.20464230799999));
#332523=CARTESIAN_POINT('Ctrl Pts',(0.0427002569999435,2.2,4.20464230799999));
#332524=CARTESIAN_POINT('Ctrl Pts',(0.0422074639999437,12.2,4.20319337299999));
#332525=CARTESIAN_POINT('Ctrl Pts',(0.0422074639999437,5.2,4.20319337299999));
#332526=CARTESIAN_POINT('Ctrl Pts',(0.0422074639999437,2.2,4.20319337299999));
#332527=CARTESIAN_POINT('Ctrl Pts',(0.0417178609999436,12.2,4.20174829399999));
#332528=CARTESIAN_POINT('Ctrl Pts',(0.0417178609999436,5.2,4.20174829399999));
#332529=CARTESIAN_POINT('Ctrl Pts',(0.0417178609999436,2.2,4.20174829399999));
#332530=CARTESIAN_POINT('Ctrl Pts',(0.0412314409999437,12.2,4.20030708399998));
#332531=CARTESIAN_POINT('Ctrl Pts',(0.0412314409999437,5.2,4.20030708399998));
#332532=CARTESIAN_POINT('Ctrl Pts',(0.0412314409999437,2.2,4.20030708399998));
#332533=CARTESIAN_POINT('Ctrl Pts',(0.0407481979999447,12.2,4.19886975299999));
#332534=CARTESIAN_POINT('Ctrl Pts',(0.0407481979999447,5.2,4.19886975299999));
#332535=CARTESIAN_POINT('Ctrl Pts',(0.0407481979999447,2.2,4.19886975299999));
#332536=CARTESIAN_POINT('Ctrl Pts',(0.0402681239999436,12.2,4.19743631399999));
#332537=CARTESIAN_POINT('Ctrl Pts',(0.0402681239999436,5.2,4.19743631399999));
#332538=CARTESIAN_POINT('Ctrl Pts',(0.0402681239999436,2.2,4.19743631399999));
#332539=CARTESIAN_POINT('Ctrl Pts',(0.0397912139999446,12.2,4.19600677699999));
#332540=CARTESIAN_POINT('Ctrl Pts',(0.0397912139999446,5.2,4.19600677699999));
#332541=CARTESIAN_POINT('Ctrl Pts',(0.0397912139999446,2.2,4.19600677699999));
#332542=CARTESIAN_POINT('Ctrl Pts',(0.0393174589999445,12.2,4.19458115399999));
#332543=CARTESIAN_POINT('Ctrl Pts',(0.0393174589999445,5.2,4.19458115399999));
#332544=CARTESIAN_POINT('Ctrl Pts',(0.0393174589999445,2.2,4.19458115399999));
#332545=CARTESIAN_POINT('Ctrl Pts',(0.0388468539999442,12.2,4.19315945499999));
#332546=CARTESIAN_POINT('Ctrl Pts',(0.0388468539999442,5.2,4.19315945499999));
#332547=CARTESIAN_POINT('Ctrl Pts',(0.0388468539999442,2.2,4.19315945499999));
#332548=CARTESIAN_POINT('Ctrl Pts',(0.0383793899999441,12.2,4.19174169399999));
#332549=CARTESIAN_POINT('Ctrl Pts',(0.0383793899999441,5.2,4.19174169399999));
#332550=CARTESIAN_POINT('Ctrl Pts',(0.0383793899999441,2.2,4.19174169399999));
#332551=CARTESIAN_POINT('Ctrl Pts',(0.0379150629999447,12.2,4.19032788099998));
#332552=CARTESIAN_POINT('Ctrl Pts',(0.0379150629999447,5.2,4.19032788099998));
#332553=CARTESIAN_POINT('Ctrl Pts',(0.0379150629999447,2.2,4.19032788099998));
#332554=CARTESIAN_POINT('Ctrl Pts',(0.0374538629999443,12.2,4.18891802799998));
#332555=CARTESIAN_POINT('Ctrl Pts',(0.0374538629999443,5.2,4.18891802799998));
#332556=CARTESIAN_POINT('Ctrl Pts',(0.0374538629999443,2.2,4.18891802799998));
#332557=CARTESIAN_POINT('Ctrl Pts',(0.0369957849999436,12.2,4.18751214499999));
#332558=CARTESIAN_POINT('Ctrl Pts',(0.0369957849999436,5.2,4.18751214499999));
#332559=CARTESIAN_POINT('Ctrl Pts',(0.0369957849999436,2.2,4.18751214499999));
#332560=CARTESIAN_POINT('Ctrl Pts',(0.036540819999944,12.2,4.18611024499998));
#332561=CARTESIAN_POINT('Ctrl Pts',(0.036540819999944,5.2,4.18611024499998));
#332562=CARTESIAN_POINT('Ctrl Pts',(0.036540819999944,2.2,4.18611024499998));
#332563=CARTESIAN_POINT('Ctrl Pts',(0.0360889629999439,12.2,4.18471233899999));
#332564=CARTESIAN_POINT('Ctrl Pts',(0.0360889629999439,5.2,4.18471233899999));
#332565=CARTESIAN_POINT('Ctrl Pts',(0.0360889629999439,2.2,4.18471233899999));
#332566=CARTESIAN_POINT('Ctrl Pts',(0.0356402039999448,12.2,4.18331843899999));
#332567=CARTESIAN_POINT('Ctrl Pts',(0.0356402039999448,5.2,4.18331843899999));
#332568=CARTESIAN_POINT('Ctrl Pts',(0.0356402039999448,2.2,4.18331843899999));
#332569=CARTESIAN_POINT('Ctrl Pts',(0.0351945409999443,12.2,4.18192855499999));
#332570=CARTESIAN_POINT('Ctrl Pts',(0.0351945409999443,5.2,4.18192855499999));
#332571=CARTESIAN_POINT('Ctrl Pts',(0.0351945409999443,2.2,4.18192855499999));
#332572=CARTESIAN_POINT('Ctrl Pts',(0.0347519609999447,12.2,4.18054269999999));
#332573=CARTESIAN_POINT('Ctrl Pts',(0.0347519609999447,5.2,4.18054269999999));
#332574=CARTESIAN_POINT('Ctrl Pts',(0.0347519609999447,2.2,4.18054269999999));
#332575=CARTESIAN_POINT('Ctrl Pts',(0.0343124599999445,12.2,4.17916088499998));
#332576=CARTESIAN_POINT('Ctrl Pts',(0.0343124599999445,5.2,4.17916088499998));
#332577=CARTESIAN_POINT('Ctrl Pts',(0.0343124599999445,2.2,4.17916088499998));
#332578=CARTESIAN_POINT('Ctrl Pts',(0.0338760309999431,12.2,4.17778312299999));
#332579=CARTESIAN_POINT('Ctrl Pts',(0.0338760309999431,5.2,4.17778312299999));
#332580=CARTESIAN_POINT('Ctrl Pts',(0.0338760309999431,2.2,4.17778312299999));
#332581=CARTESIAN_POINT('Ctrl Pts',(0.0334426659999443,12.2,4.17640942299998));
#332582=CARTESIAN_POINT('Ctrl Pts',(0.0334426659999443,5.2,4.17640942299998));
#332583=CARTESIAN_POINT('Ctrl Pts',(0.0334426659999443,2.2,4.17640942299998));
#332584=CARTESIAN_POINT('Ctrl Pts',(0.0330123569999441,12.2,4.17503979899998));
#332585=CARTESIAN_POINT('Ctrl Pts',(0.0330123569999441,5.2,4.17503979899998));
#332586=CARTESIAN_POINT('Ctrl Pts',(0.0330123569999441,2.2,4.17503979899998));
#332587=CARTESIAN_POINT('Ctrl Pts',(0.0325850979999431,12.2,4.17367426099998));
#332588=CARTESIAN_POINT('Ctrl Pts',(0.0325850979999431,5.2,4.17367426099998));
#332589=CARTESIAN_POINT('Ctrl Pts',(0.0325850979999431,2.2,4.17367426099998));
#332590=CARTESIAN_POINT('Ctrl Pts',(0.032160879999944,12.2,4.17231282099999));
#332591=CARTESIAN_POINT('Ctrl Pts',(0.032160879999944,5.2,4.17231282099999));
#332592=CARTESIAN_POINT('Ctrl Pts',(0.032160879999944,2.2,4.17231282099999));
#332593=CARTESIAN_POINT('Ctrl Pts',(0.031739697999944,12.2,4.17095549099999));
#332594=CARTESIAN_POINT('Ctrl Pts',(0.031739697999944,5.2,4.17095549099999));
#332595=CARTESIAN_POINT('Ctrl Pts',(0.031739697999944,2.2,4.17095549099999));
#332596=CARTESIAN_POINT('Ctrl Pts',(0.0313215419999435,12.2,4.16960228199999));
#332597=CARTESIAN_POINT('Ctrl Pts',(0.0313215419999435,5.2,4.16960228199999));
#332598=CARTESIAN_POINT('Ctrl Pts',(0.0313215419999435,2.2,4.16960228199999));
#332599=CARTESIAN_POINT('Ctrl Pts',(0.0309064059999453,12.2,4.16825320699999));
#332600=CARTESIAN_POINT('Ctrl Pts',(0.0309064059999453,5.2,4.16825320699999));
#332601=CARTESIAN_POINT('Ctrl Pts',(0.0309064059999453,2.2,4.16825320699999));
#332602=CARTESIAN_POINT('Ctrl Pts',(0.0304942829999444,12.2,4.16690827599999));
#332603=CARTESIAN_POINT('Ctrl Pts',(0.0304942829999444,5.2,4.16690827599999));
#332604=CARTESIAN_POINT('Ctrl Pts',(0.0304942829999444,2.2,4.16690827599999));
#332605=CARTESIAN_POINT('Ctrl Pts',(0.0300851639999444,12.2,4.16556750299999));
#332606=CARTESIAN_POINT('Ctrl Pts',(0.0300851639999444,5.2,4.16556750299999));
#332607=CARTESIAN_POINT('Ctrl Pts',(0.0300851639999444,2.2,4.16556750299999));
#332608=CARTESIAN_POINT('Ctrl Pts',(0.0296790429999449,12.2,4.16423089699999));
#332609=CARTESIAN_POINT('Ctrl Pts',(0.0296790429999449,5.2,4.16423089699999));
#332610=CARTESIAN_POINT('Ctrl Pts',(0.0296790429999449,2.2,4.16423089699999));
#332611=CARTESIAN_POINT('Ctrl Pts',(0.0292759109999441,12.2,4.16289846999998));
#332612=CARTESIAN_POINT('Ctrl Pts',(0.0292759109999441,5.2,4.16289846999998));
#332613=CARTESIAN_POINT('Ctrl Pts',(0.0292759109999441,2.2,4.16289846999998));
#332614=CARTESIAN_POINT('Ctrl Pts',(0.0288757609999435,12.2,4.16157023699999));
#332615=CARTESIAN_POINT('Ctrl Pts',(0.0288757609999435,5.2,4.16157023699999));
#332616=CARTESIAN_POINT('Ctrl Pts',(0.0288757609999435,2.2,4.16157023699999));
#332617=CARTESIAN_POINT('Ctrl Pts',(0.0284785859999437,12.2,4.16024620599998));
#332618=CARTESIAN_POINT('Ctrl Pts',(0.0284785859999437,5.2,4.16024620599998));
#332619=CARTESIAN_POINT('Ctrl Pts',(0.0284785859999437,2.2,4.16024620599998));
#332620=CARTESIAN_POINT('Ctrl Pts',(0.0280843769999439,12.2,4.15892639099999));
#332621=CARTESIAN_POINT('Ctrl Pts',(0.0280843769999439,5.2,4.15892639099999));
#332622=CARTESIAN_POINT('Ctrl Pts',(0.0280843769999439,2.2,4.15892639099999));
#332623=CARTESIAN_POINT('Ctrl Pts',(0.0276931269999447,12.2,4.15761080299998));
#332624=CARTESIAN_POINT('Ctrl Pts',(0.0276931269999447,5.2,4.15761080299998));
#332625=CARTESIAN_POINT('Ctrl Pts',(0.0276931269999447,2.2,4.15761080299998));
#332626=CARTESIAN_POINT('Ctrl Pts',(0.0273048289999433,12.2,4.15629945299998));
#332627=CARTESIAN_POINT('Ctrl Pts',(0.0273048289999433,5.2,4.15629945299998));
#332628=CARTESIAN_POINT('Ctrl Pts',(0.0273048289999433,2.2,4.15629945299998));
#332629=CARTESIAN_POINT('Ctrl Pts',(0.0269194739999445,12.2,4.15499235399999));
#332630=CARTESIAN_POINT('Ctrl Pts',(0.0269194739999445,5.2,4.15499235399999));
#332631=CARTESIAN_POINT('Ctrl Pts',(0.0269194739999445,2.2,4.15499235399999));
#332632=CARTESIAN_POINT('Ctrl Pts',(0.0265370559999434,12.2,4.15368951899998));
#332633=CARTESIAN_POINT('Ctrl Pts',(0.0265370559999434,5.2,4.15368951899998));
#332634=CARTESIAN_POINT('Ctrl Pts',(0.0265370559999434,2.2,4.15368951899998));
#332635=CARTESIAN_POINT('Ctrl Pts',(0.0261575649999435,12.2,4.15239095699998));
#332636=CARTESIAN_POINT('Ctrl Pts',(0.0261575649999435,5.2,4.15239095699998));
#332637=CARTESIAN_POINT('Ctrl Pts',(0.0261575649999435,2.2,4.15239095699998));
#332638=CARTESIAN_POINT('Ctrl Pts',(0.0257809939999454,12.2,4.15109668199998));
#332639=CARTESIAN_POINT('Ctrl Pts',(0.0257809939999454,5.2,4.15109668199998));
#332640=CARTESIAN_POINT('Ctrl Pts',(0.0257809939999454,2.2,4.15109668199998));
#332641=CARTESIAN_POINT('Ctrl Pts',(0.025407334999944,12.2,4.14980670399999));
#332642=CARTESIAN_POINT('Ctrl Pts',(0.025407334999944,5.2,4.14980670399999));
#332643=CARTESIAN_POINT('Ctrl Pts',(0.025407334999944,2.2,4.14980670399999));
#332644=CARTESIAN_POINT('Ctrl Pts',(0.0250365809999431,12.2,4.14852103699998));
#332645=CARTESIAN_POINT('Ctrl Pts',(0.0250365809999431,5.2,4.14852103699998));
#332646=CARTESIAN_POINT('Ctrl Pts',(0.0250365809999431,2.2,4.14852103699998));
#332647=CARTESIAN_POINT('Ctrl Pts',(0.0246687219999442,12.2,4.14723969099998));
#332648=CARTESIAN_POINT('Ctrl Pts',(0.0246687219999442,5.2,4.14723969099998));
#332649=CARTESIAN_POINT('Ctrl Pts',(0.0246687219999442,2.2,4.14723969099998));
#332650=CARTESIAN_POINT('Ctrl Pts',(0.0243037529999446,12.2,4.14596267999999));
#332651=CARTESIAN_POINT('Ctrl Pts',(0.0243037529999446,5.2,4.14596267999999));
#332652=CARTESIAN_POINT('Ctrl Pts',(0.0243037529999446,2.2,4.14596267999999));
#332653=CARTESIAN_POINT('Ctrl Pts',(0.0239416629999434,12.2,4.14469001399999));
#332654=CARTESIAN_POINT('Ctrl Pts',(0.0239416629999434,5.2,4.14469001399999));
#332655=CARTESIAN_POINT('Ctrl Pts',(0.0239416629999434,2.2,4.14469001399999));
#332656=CARTESIAN_POINT('Ctrl Pts',(0.0235824469999446,12.2,4.14342170599999));
#332657=CARTESIAN_POINT('Ctrl Pts',(0.0235824469999446,5.2,4.14342170599999));
#332658=CARTESIAN_POINT('Ctrl Pts',(0.0235824469999446,2.2,4.14342170599999));
#332659=CARTESIAN_POINT('Ctrl Pts',(0.023226092999945,12.2,4.14215776799999));
#332660=CARTESIAN_POINT('Ctrl Pts',(0.023226092999945,5.2,4.14215776799999));
#332661=CARTESIAN_POINT('Ctrl Pts',(0.023226092999945,2.2,4.14215776799999));
#332662=CARTESIAN_POINT('Ctrl Pts',(0.0228725969999444,12.2,4.14089821099999));
#332663=CARTESIAN_POINT('Ctrl Pts',(0.0228725969999444,5.2,4.14089821099999));
#332664=CARTESIAN_POINT('Ctrl Pts',(0.0228725969999444,2.2,4.14089821099999));
#332665=CARTESIAN_POINT('Ctrl Pts',(0.0225219469999449,12.2,4.13964304799999));
#332666=CARTESIAN_POINT('Ctrl Pts',(0.0225219469999449,5.2,4.13964304799999));
#332667=CARTESIAN_POINT('Ctrl Pts',(0.0225219469999449,2.2,4.13964304799999));
#332668=CARTESIAN_POINT('Ctrl Pts',(0.022174136999944,12.2,4.13839229099998));
#332669=CARTESIAN_POINT('Ctrl Pts',(0.022174136999944,5.2,4.13839229099998));
#332670=CARTESIAN_POINT('Ctrl Pts',(0.022174136999944,2.2,4.13839229099998));
#332671=CARTESIAN_POINT('Ctrl Pts',(0.0218291599999443,12.2,4.13714595299999));
#332672=CARTESIAN_POINT('Ctrl Pts',(0.0218291599999443,5.2,4.13714595299999));
#332673=CARTESIAN_POINT('Ctrl Pts',(0.0218291599999443,2.2,4.13714595299999));
#332674=CARTESIAN_POINT('Ctrl Pts',(0.0214870049999438,12.2,4.13590404299998));
#332675=CARTESIAN_POINT('Ctrl Pts',(0.0214870049999438,5.2,4.13590404299998));
#332676=CARTESIAN_POINT('Ctrl Pts',(0.0214870049999438,2.2,4.13590404299998));
#332677=CARTESIAN_POINT('Ctrl Pts',(0.0211476659999443,12.2,4.13466657499999));
#332678=CARTESIAN_POINT('Ctrl Pts',(0.0211476659999443,5.2,4.13466657499999));
#332679=CARTESIAN_POINT('Ctrl Pts',(0.0211476659999443,2.2,4.13466657499999));
#332680=CARTESIAN_POINT('Ctrl Pts',(0.0208111309999437,12.2,4.13343356199999));
#332681=CARTESIAN_POINT('Ctrl Pts',(0.0208111309999437,5.2,4.13343356199999));
#332682=CARTESIAN_POINT('Ctrl Pts',(0.0208111309999437,2.2,4.13343356199999));
#332683=CARTESIAN_POINT('Ctrl Pts',(0.0204773969999439,12.2,4.13220501399999));
#332684=CARTESIAN_POINT('Ctrl Pts',(0.0204773969999439,5.2,4.13220501399999));
#332685=CARTESIAN_POINT('Ctrl Pts',(0.0204773969999439,2.2,4.13220501399999));
#332686=CARTESIAN_POINT('Ctrl Pts',(0.0201464519999439,12.2,4.13098094499999));
#332687=CARTESIAN_POINT('Ctrl Pts',(0.0201464519999439,5.2,4.13098094499999));
#332688=CARTESIAN_POINT('Ctrl Pts',(0.0201464519999439,2.2,4.13098094499999));
#332689=CARTESIAN_POINT('Ctrl Pts',(0.0198182879999453,12.2,4.12976136599998));
#332690=CARTESIAN_POINT('Ctrl Pts',(0.0198182879999453,5.2,4.12976136599998));
#332691=CARTESIAN_POINT('Ctrl Pts',(0.0198182879999453,2.2,4.12976136599998));
#332692=CARTESIAN_POINT('Ctrl Pts',(0.0194928969999442,12.2,4.12854628899999));
#332693=CARTESIAN_POINT('Ctrl Pts',(0.0194928969999442,5.2,4.12854628899999));
#332694=CARTESIAN_POINT('Ctrl Pts',(0.0194928969999442,2.2,4.12854628899999));
#332695=CARTESIAN_POINT('Ctrl Pts',(0.019170269999943,12.2,4.12733572799999));
#332696=CARTESIAN_POINT('Ctrl Pts',(0.019170269999943,5.2,4.12733572799999));
#332697=CARTESIAN_POINT('Ctrl Pts',(0.019170269999943,2.2,4.12733572799999));
#332698=CARTESIAN_POINT('Ctrl Pts',(0.0188503999999445,12.2,4.12612969199999));
#332699=CARTESIAN_POINT('Ctrl Pts',(0.0188503999999445,5.2,4.12612969199999));
#332700=CARTESIAN_POINT('Ctrl Pts',(0.0188503999999445,2.2,4.12612969199999));
#332701=CARTESIAN_POINT('Ctrl Pts',(0.0185332769999447,12.2,4.12492819699998));
#332702=CARTESIAN_POINT('Ctrl Pts',(0.0185332769999447,5.2,4.12492819699998));
#332703=CARTESIAN_POINT('Ctrl Pts',(0.0185332769999447,2.2,4.12492819699998));
#332704=CARTESIAN_POINT('Ctrl Pts',(0.0182188929999438,12.2,4.12373125199998));
#332705=CARTESIAN_POINT('Ctrl Pts',(0.0182188929999438,5.2,4.12373125199998));
#332706=CARTESIAN_POINT('Ctrl Pts',(0.0182188929999438,2.2,4.12373125199998));
#332707=CARTESIAN_POINT('Ctrl Pts',(0.0179072379999445,12.2,4.12253887099999));
#332708=CARTESIAN_POINT('Ctrl Pts',(0.0179072379999445,5.2,4.12253887099999));
#332709=CARTESIAN_POINT('Ctrl Pts',(0.0179072379999445,2.2,4.12253887099999));
#332710=CARTESIAN_POINT('Ctrl Pts',(0.0175983049999429,12.2,4.12135106499999));
#332711=CARTESIAN_POINT('Ctrl Pts',(0.0175983049999429,5.2,4.12135106499999));
#332712=CARTESIAN_POINT('Ctrl Pts',(0.0175983049999429,2.2,4.12135106499999));
#332713=CARTESIAN_POINT('Ctrl Pts',(0.0172920849999447,12.2,4.12016784699999));
#332714=CARTESIAN_POINT('Ctrl Pts',(0.0172920849999447,5.2,4.12016784699999));
#332715=CARTESIAN_POINT('Ctrl Pts',(0.0172920849999447,2.2,4.12016784699999));
#332716=CARTESIAN_POINT('Ctrl Pts',(0.0169885679999437,12.2,4.11898922899999));
#332717=CARTESIAN_POINT('Ctrl Pts',(0.0169885679999437,5.2,4.11898922899999));
#332718=CARTESIAN_POINT('Ctrl Pts',(0.0169885679999437,2.2,4.11898922899999));
#332719=CARTESIAN_POINT('Ctrl Pts',(0.0166877469999438,12.2,4.11781522499999));
#332720=CARTESIAN_POINT('Ctrl Pts',(0.0166877469999438,5.2,4.11781522499999));
#332721=CARTESIAN_POINT('Ctrl Pts',(0.0166877469999438,2.2,4.11781522499999));
#332722=CARTESIAN_POINT('Ctrl Pts',(0.0163896129999441,12.2,4.11664584499999));
#332723=CARTESIAN_POINT('Ctrl Pts',(0.0163896129999441,5.2,4.11664584499999));
#332724=CARTESIAN_POINT('Ctrl Pts',(0.0163896129999441,2.2,4.11664584499999));
#332725=CARTESIAN_POINT('Ctrl Pts',(0.0160941549999449,12.2,4.11548110199998));
#332726=CARTESIAN_POINT('Ctrl Pts',(0.0160941549999449,5.2,4.11548110199998));
#332727=CARTESIAN_POINT('Ctrl Pts',(0.0160941549999449,2.2,4.11548110199998));
#332728=CARTESIAN_POINT('Ctrl Pts',(0.0158013659999445,12.2,4.11432100899999));
#332729=CARTESIAN_POINT('Ctrl Pts',(0.0158013659999445,5.2,4.11432100899999));
#332730=CARTESIAN_POINT('Ctrl Pts',(0.0158013659999445,2.2,4.11432100899999));
#332731=CARTESIAN_POINT('Ctrl Pts',(0.0155112359999432,12.2,4.11316557799999));
#332732=CARTESIAN_POINT('Ctrl Pts',(0.0155112359999432,5.2,4.11316557799999));
#332733=CARTESIAN_POINT('Ctrl Pts',(0.0155112359999432,2.2,4.11316557799999));
#332734=CARTESIAN_POINT('Ctrl Pts',(0.0152237589999449,12.2,4.11201482099998));
#332735=CARTESIAN_POINT('Ctrl Pts',(0.0152237589999449,5.2,4.11201482099998));
#332736=CARTESIAN_POINT('Ctrl Pts',(0.0152237589999449,2.2,4.11201482099998));
#332737=CARTESIAN_POINT('Ctrl Pts',(0.014938920999944,12.2,4.11086874999998));
#332738=CARTESIAN_POINT('Ctrl Pts',(0.014938920999944,5.2,4.11086874999998));
#332739=CARTESIAN_POINT('Ctrl Pts',(0.014938920999944,2.2,4.11086874999998));
#332740=CARTESIAN_POINT('Ctrl Pts',(0.0146567169999445,12.2,4.10972737899999));
#332741=CARTESIAN_POINT('Ctrl Pts',(0.0146567169999445,5.2,4.10972737899999));
#332742=CARTESIAN_POINT('Ctrl Pts',(0.0146567169999445,2.2,4.10972737899999));
#332743=CARTESIAN_POINT('Ctrl Pts',(0.0143771369999435,12.2,4.10859071899999));
#332744=CARTESIAN_POINT('Ctrl Pts',(0.0143771369999435,5.2,4.10859071899999));
#332745=CARTESIAN_POINT('Ctrl Pts',(0.0143771369999435,2.2,4.10859071899999));
#332746=CARTESIAN_POINT('Ctrl Pts',(0.0141001709999444,12.2,4.10745878299998));
#332747=CARTESIAN_POINT('Ctrl Pts',(0.0141001709999444,5.2,4.10745878299998));
#332748=CARTESIAN_POINT('Ctrl Pts',(0.0141001709999444,2.2,4.10745878299998));
#332749=CARTESIAN_POINT('Ctrl Pts',(0.0138258089999432,12.2,4.10633158399998));
#332750=CARTESIAN_POINT('Ctrl Pts',(0.0138258089999432,5.2,4.10633158399998));
#332751=CARTESIAN_POINT('Ctrl Pts',(0.0138258089999432,2.2,4.10633158399998));
#332752=CARTESIAN_POINT('Ctrl Pts',(0.0135540449999449,12.2,4.10520913399999));
#332753=CARTESIAN_POINT('Ctrl Pts',(0.0135540449999449,5.2,4.10520913399999));
#332754=CARTESIAN_POINT('Ctrl Pts',(0.0135540449999449,2.2,4.10520913399999));
#332755=CARTESIAN_POINT('Ctrl Pts',(0.013284865999944,12.2,4.10409144399999));
#332756=CARTESIAN_POINT('Ctrl Pts',(0.013284865999944,5.2,4.10409144399999));
#332757=CARTESIAN_POINT('Ctrl Pts',(0.013284865999944,2.2,4.10409144399999));
#332758=CARTESIAN_POINT('Ctrl Pts',(0.0130182669999446,12.2,4.10297852999999));
#332759=CARTESIAN_POINT('Ctrl Pts',(0.0130182669999446,5.2,4.10297852999999));
#332760=CARTESIAN_POINT('Ctrl Pts',(0.0130182669999446,2.2,4.10297852999999));
#332761=CARTESIAN_POINT('Ctrl Pts',(0.0127542339999442,12.2,4.10187040099999));
#332762=CARTESIAN_POINT('Ctrl Pts',(0.0127542339999442,5.2,4.10187040099999));
#332763=CARTESIAN_POINT('Ctrl Pts',(0.0127542339999442,2.2,4.10187040099999));
#332764=CARTESIAN_POINT('Ctrl Pts',(0.0124927609999437,12.2,4.10076707099999));
#332765=CARTESIAN_POINT('Ctrl Pts',(0.0124927609999437,5.2,4.10076707099999));
#332766=CARTESIAN_POINT('Ctrl Pts',(0.0124927609999437,2.2,4.10076707099999));
#332767=CARTESIAN_POINT('Ctrl Pts',(0.0122338369999431,12.2,4.09966855299999));
#332768=CARTESIAN_POINT('Ctrl Pts',(0.0122338369999431,5.2,4.09966855299999));
#332769=CARTESIAN_POINT('Ctrl Pts',(0.0122338369999431,2.2,4.09966855299999));
#332770=CARTESIAN_POINT('Ctrl Pts',(0.0119774549999441,12.2,4.09857485999999));
#332771=CARTESIAN_POINT('Ctrl Pts',(0.0119774549999441,5.2,4.09857485999999));
#332772=CARTESIAN_POINT('Ctrl Pts',(0.0119774549999441,2.2,4.09857485999999));
#332773=CARTESIAN_POINT('Ctrl Pts',(0.0117236019999434,12.2,4.09748600299999));
#332774=CARTESIAN_POINT('Ctrl Pts',(0.0117236019999434,5.2,4.09748600299999));
#332775=CARTESIAN_POINT('Ctrl Pts',(0.0117236019999434,2.2,4.09748600299999));
#332776=CARTESIAN_POINT('Ctrl Pts',(0.0114722699999437,12.2,4.09640199399998));
#332777=CARTESIAN_POINT('Ctrl Pts',(0.0114722699999437,5.2,4.09640199399998));
#332778=CARTESIAN_POINT('Ctrl Pts',(0.0114722699999437,2.2,4.09640199399998));
#332779=CARTESIAN_POINT('Ctrl Pts',(0.0112234509999443,12.2,4.09532284999998));
#332780=CARTESIAN_POINT('Ctrl Pts',(0.0112234509999443,5.2,4.09532284999998));
#332781=CARTESIAN_POINT('Ctrl Pts',(0.0112234509999443,2.2,4.09532284999998));
#332782=CARTESIAN_POINT('Ctrl Pts',(0.0109771329999442,12.2,4.09424857899998));
#332783=CARTESIAN_POINT('Ctrl Pts',(0.0109771329999442,5.2,4.09424857899998));
#332784=CARTESIAN_POINT('Ctrl Pts',(0.0109771329999442,2.2,4.09424857899998));
#332785=CARTESIAN_POINT('Ctrl Pts',(0.0107333079999439,12.2,4.09317919499999));
#332786=CARTESIAN_POINT('Ctrl Pts',(0.0107333079999439,5.2,4.09317919499999));
#332787=CARTESIAN_POINT('Ctrl Pts',(0.0107333079999439,2.2,4.09317919499999));
#332788=CARTESIAN_POINT('Ctrl Pts',(0.0104919659999436,12.2,4.09211471199999));
#332789=CARTESIAN_POINT('Ctrl Pts',(0.0104919659999436,5.2,4.09211471199999));
#332790=CARTESIAN_POINT('Ctrl Pts',(0.0104919659999436,2.2,4.09211471199999));
#332791=CARTESIAN_POINT('Ctrl Pts',(0.0102530959999447,12.2,4.09105514199998));
#332792=CARTESIAN_POINT('Ctrl Pts',(0.0102530959999447,5.2,4.09105514199998));
#332793=CARTESIAN_POINT('Ctrl Pts',(0.0102530959999447,2.2,4.09105514199998));
#332794=CARTESIAN_POINT('Ctrl Pts',(0.0100166899999443,12.2,4.09000049599998));
#332795=CARTESIAN_POINT('Ctrl Pts',(0.0100166899999443,5.2,4.09000049599998));
#332796=CARTESIAN_POINT('Ctrl Pts',(0.0100166899999443,2.2,4.09000049599998));
#332797=CARTESIAN_POINT('Ctrl Pts',(0.00978273799994377,12.2,4.08895078999999));
#332798=CARTESIAN_POINT('Ctrl Pts',(0.00978273799994377,5.2,4.08895078999999));
#332799=CARTESIAN_POINT('Ctrl Pts',(0.00978273799994377,2.2,4.08895078999999));
#332800=CARTESIAN_POINT('Ctrl Pts',(0.0095512299999445,12.2,4.08790603499998));
#332801=CARTESIAN_POINT('Ctrl Pts',(0.0095512299999445,5.2,4.08790603499998));
#332802=CARTESIAN_POINT('Ctrl Pts',(0.0095512299999445,2.2,4.08790603499998));
#332803=CARTESIAN_POINT('Ctrl Pts',(0.00932215499994448,12.2,4.08686624199999));
#332804=CARTESIAN_POINT('Ctrl Pts',(0.00932215499994448,5.2,4.08686624199999));
#332805=CARTESIAN_POINT('Ctrl Pts',(0.00932215499994448,2.2,4.08686624199999));
#332806=CARTESIAN_POINT('Ctrl Pts',(0.00909550499994415,12.2,4.08583142799999));
#332807=CARTESIAN_POINT('Ctrl Pts',(0.00909550499994415,5.2,4.08583142799999));
#332808=CARTESIAN_POINT('Ctrl Pts',(0.00909550499994415,2.2,4.08583142799999));
#332809=CARTESIAN_POINT('Ctrl Pts',(0.00887126799994364,12.2,4.08480160199999));
#332810=CARTESIAN_POINT('Ctrl Pts',(0.00887126799994364,5.2,4.08480160199999));
#332811=CARTESIAN_POINT('Ctrl Pts',(0.00887126799994364,2.2,4.08480160199999));
#332812=CARTESIAN_POINT('Ctrl Pts',(0.00864943599994449,12.2,4.08377677799999));
#332813=CARTESIAN_POINT('Ctrl Pts',(0.00864943599994449,5.2,4.08377677799999));
#332814=CARTESIAN_POINT('Ctrl Pts',(0.00864943599994449,2.2,4.08377677799999));
#332815=CARTESIAN_POINT('Ctrl Pts',(0.00842999799994359,12.2,4.08275697099998));
#332816=CARTESIAN_POINT('Ctrl Pts',(0.00842999799994359,5.2,4.08275697099998));
#332817=CARTESIAN_POINT('Ctrl Pts',(0.00842999799994359,2.2,4.08275697099998));
#332818=CARTESIAN_POINT('Ctrl Pts',(0.00821294299994334,12.2,4.08174219099998));
#332819=CARTESIAN_POINT('Ctrl Pts',(0.00821294299994334,5.2,4.08174219099998));
#332820=CARTESIAN_POINT('Ctrl Pts',(0.00821294299994334,2.2,4.08174219099998));
#332821=CARTESIAN_POINT('Ctrl Pts',(0.00799826299994421,12.2,4.08073245199999));
#332822=CARTESIAN_POINT('Ctrl Pts',(0.00799826299994421,5.2,4.08073245199999));
#332823=CARTESIAN_POINT('Ctrl Pts',(0.00799826299994421,2.2,4.08073245199999));
#332824=CARTESIAN_POINT('Ctrl Pts',(0.00778594599994408,12.2,4.07972776699999));
#332825=CARTESIAN_POINT('Ctrl Pts',(0.00778594599994408,5.2,4.07972776699999));
#332826=CARTESIAN_POINT('Ctrl Pts',(0.00778594599994408,2.2,4.07972776699999));
#332827=CARTESIAN_POINT('Ctrl Pts',(0.0075759849999446,12.2,4.07872814899999));
#332828=CARTESIAN_POINT('Ctrl Pts',(0.0075759849999446,5.2,4.07872814899999));
#332829=CARTESIAN_POINT('Ctrl Pts',(0.0075759849999446,2.2,4.07872814899999));
#332830=CARTESIAN_POINT('Ctrl Pts',(0.00736836499994452,12.2,4.07773361099999));
#332831=CARTESIAN_POINT('Ctrl Pts',(0.00736836499994452,5.2,4.07773361099999));
#332832=CARTESIAN_POINT('Ctrl Pts',(0.00736836499994452,2.2,4.07773361099999));
#332833=CARTESIAN_POINT('Ctrl Pts',(0.00716307899994439,12.2,4.07674416499999));
#332834=CARTESIAN_POINT('Ctrl Pts',(0.00716307899994439,5.2,4.07674416499999));
#332835=CARTESIAN_POINT('Ctrl Pts',(0.00716307899994439,2.2,4.07674416499999));
#332836=CARTESIAN_POINT('Ctrl Pts',(0.00696011599994328,12.2,4.07575982599998));
#332837=CARTESIAN_POINT('Ctrl Pts',(0.00696011599994328,5.2,4.07575982599998));
#332838=CARTESIAN_POINT('Ctrl Pts',(0.00696011599994328,2.2,4.07575982599998));
#332839=CARTESIAN_POINT('Ctrl Pts',(0.00675946399994353,12.2,4.07478060399999));
#332840=CARTESIAN_POINT('Ctrl Pts',(0.00675946399994353,5.2,4.07478060399999));
#332841=CARTESIAN_POINT('Ctrl Pts',(0.00675946399994353,2.2,4.07478060399999));
#332842=CARTESIAN_POINT('Ctrl Pts',(0.00656111499994338,12.2,4.07380651499999));
#332843=CARTESIAN_POINT('Ctrl Pts',(0.00656111499994338,5.2,4.07380651499999));
#332844=CARTESIAN_POINT('Ctrl Pts',(0.00656111499994338,2.2,4.07380651499999));
#332845=CARTESIAN_POINT('Ctrl Pts',(0.00636505799994302,12.2,4.07283757099999));
#332846=CARTESIAN_POINT('Ctrl Pts',(0.00636505799994302,5.2,4.07283757099999));
#332847=CARTESIAN_POINT('Ctrl Pts',(0.00636505799994302,2.2,4.07283757099999));
#332848=CARTESIAN_POINT('Ctrl Pts',(0.00617128199994376,12.2,4.07187378599998));
#332849=CARTESIAN_POINT('Ctrl Pts',(0.00617128199994376,5.2,4.07187378599998));
#332850=CARTESIAN_POINT('Ctrl Pts',(0.00617128199994376,2.2,4.07187378599998));
#332851=CARTESIAN_POINT('Ctrl Pts',(0.00597977699994367,12.2,4.07091516999999));
#332852=CARTESIAN_POINT('Ctrl Pts',(0.00597977699994367,5.2,4.07091516999999));
#332853=CARTESIAN_POINT('Ctrl Pts',(0.00597977699994367,2.2,4.07091516999999));
#332854=CARTESIAN_POINT('Ctrl Pts',(0.00579053099994397,12.2,4.06996173999998));
#332855=CARTESIAN_POINT('Ctrl Pts',(0.00579053099994397,5.2,4.06996173999998));
#332856=CARTESIAN_POINT('Ctrl Pts',(0.00579053099994397,2.2,4.06996173999998));
#332857=CARTESIAN_POINT('Ctrl Pts',(0.00560353499994392,12.2,4.06901350599998));
#332858=CARTESIAN_POINT('Ctrl Pts',(0.00560353499994392,5.2,4.06901350599998));
#332859=CARTESIAN_POINT('Ctrl Pts',(0.00560353499994392,2.2,4.06901350599998));
#332860=CARTESIAN_POINT('Ctrl Pts',(0.00541877899994491,12.2,4.06807048299999));
#332861=CARTESIAN_POINT('Ctrl Pts',(0.00541877899994491,5.2,4.06807048299999));
#332862=CARTESIAN_POINT('Ctrl Pts',(0.00541877899994491,2.2,4.06807048299999));
#332863=CARTESIAN_POINT('Ctrl Pts',(0.00523624899994467,12.2,4.06713268299999));
#332864=CARTESIAN_POINT('Ctrl Pts',(0.00523624899994467,5.2,4.06713268299999));
#332865=CARTESIAN_POINT('Ctrl Pts',(0.00523624899994467,2.2,4.06713268299999));
#332866=CARTESIAN_POINT('Ctrl Pts',(0.00505593799994374,12.2,4.06620012199999));
#332867=CARTESIAN_POINT('Ctrl Pts',(0.00505593799994374,5.2,4.06620012199999));
#332868=CARTESIAN_POINT('Ctrl Pts',(0.00505593799994374,2.2,4.06620012199999));
#332869=CARTESIAN_POINT('Ctrl Pts',(0.00487783199994317,12.2,4.06527280899999));
#332870=CARTESIAN_POINT('Ctrl Pts',(0.00487783199994317,5.2,4.06527280899999));
#332871=CARTESIAN_POINT('Ctrl Pts',(0.00487783199994317,2.2,4.06527280899999));
#332872=CARTESIAN_POINT('Ctrl Pts',(0.00470192299994453,12.2,4.06435075999998));
#332873=CARTESIAN_POINT('Ctrl Pts',(0.00470192299994453,5.2,4.06435075999998));
#332874=CARTESIAN_POINT('Ctrl Pts',(0.00470192299994453,2.2,4.06435075999998));
#332875=CARTESIAN_POINT('Ctrl Pts',(0.0045281989999446,12.2,4.06343398799999));
#332876=CARTESIAN_POINT('Ctrl Pts',(0.0045281989999446,5.2,4.06343398799999));
#332877=CARTESIAN_POINT('Ctrl Pts',(0.0045281989999446,2.2,4.06343398799999));
#332878=CARTESIAN_POINT('Ctrl Pts',(0.0043566479999435,12.2,4.06252250499998));
#332879=CARTESIAN_POINT('Ctrl Pts',(0.0043566479999435,5.2,4.06252250499998));
#332880=CARTESIAN_POINT('Ctrl Pts',(0.0043566479999435,2.2,4.06252250499998));
#332881=CARTESIAN_POINT('Ctrl Pts',(0.00418725999994373,12.2,4.06161632599999));
#332882=CARTESIAN_POINT('Ctrl Pts',(0.00418725999994373,5.2,4.06161632599999));
#332883=CARTESIAN_POINT('Ctrl Pts',(0.00418725999994373,2.2,4.06161632599999));
#332884=CARTESIAN_POINT('Ctrl Pts',(0.00402002399994438,12.2,4.06071546299999));
#332885=CARTESIAN_POINT('Ctrl Pts',(0.00402002399994438,5.2,4.06071546299999));
#332886=CARTESIAN_POINT('Ctrl Pts',(0.00402002399994438,2.2,4.06071546299999));
#332887=CARTESIAN_POINT('Ctrl Pts',(0.00385492899994454,12.2,4.05981992999998));
#332888=CARTESIAN_POINT('Ctrl Pts',(0.00385492899994454,5.2,4.05981992999998));
#332889=CARTESIAN_POINT('Ctrl Pts',(0.00385492899994454,2.2,4.05981992999998));
#332890=CARTESIAN_POINT('Ctrl Pts',(0.00369196399994442,12.2,4.05892973999999));
#332891=CARTESIAN_POINT('Ctrl Pts',(0.00369196399994442,5.2,4.05892973999999));
#332892=CARTESIAN_POINT('Ctrl Pts',(0.00369196399994442,2.2,4.05892973999999));
#332893=CARTESIAN_POINT('Ctrl Pts',(0.00353111799994531,12.2,4.05804490699998));
#332894=CARTESIAN_POINT('Ctrl Pts',(0.00353111799994531,5.2,4.05804490699998));
#332895=CARTESIAN_POINT('Ctrl Pts',(0.00353111799994531,2.2,4.05804490699998));
#332896=CARTESIAN_POINT('Ctrl Pts',(0.00337237899994291,12.2,4.05716544299998));
#332897=CARTESIAN_POINT('Ctrl Pts',(0.00337237899994291,5.2,4.05716544299998));
#332898=CARTESIAN_POINT('Ctrl Pts',(0.00337237899994291,2.2,4.05716544299998));
#332899=CARTESIAN_POINT('Ctrl Pts',(0.00321573599994517,12.2,4.05629136299999));
#332900=CARTESIAN_POINT('Ctrl Pts',(0.00321573599994517,5.2,4.05629136299999));
#332901=CARTESIAN_POINT('Ctrl Pts',(0.00321573599994517,2.2,4.05629136299999));
#332902=CARTESIAN_POINT('Ctrl Pts',(0.00306117799994453,12.2,4.05542268099998));
#332903=CARTESIAN_POINT('Ctrl Pts',(0.00306117799994453,5.2,4.05542268099998));
#332904=CARTESIAN_POINT('Ctrl Pts',(0.00306117799994453,2.2,4.05542268099998));
#332905=CARTESIAN_POINT('Ctrl Pts',(0.00290869399994341,12.2,4.05455940799998));
#332906=CARTESIAN_POINT('Ctrl Pts',(0.00290869399994341,5.2,4.05455940799998));
#332907=CARTESIAN_POINT('Ctrl Pts',(0.00290869399994341,2.2,4.05455940799998));
#332908=CARTESIAN_POINT('Ctrl Pts',(0.00275827199994415,12.2,4.05370155899998));
#332909=CARTESIAN_POINT('Ctrl Pts',(0.00275827199994415,5.2,4.05370155899998));
#332910=CARTESIAN_POINT('Ctrl Pts',(0.00275827199994415,2.2,4.05370155899998));
#332911=CARTESIAN_POINT('Ctrl Pts',(0.00260990099994473,12.2,4.05284914799999));
#332912=CARTESIAN_POINT('Ctrl Pts',(0.00260990099994473,5.2,4.05284914799999));
#332913=CARTESIAN_POINT('Ctrl Pts',(0.00260990099994473,2.2,4.05284914799999));
#332914=CARTESIAN_POINT('Ctrl Pts',(0.00246356899994526,12.2,4.05200218699999));
#332915=CARTESIAN_POINT('Ctrl Pts',(0.00246356899994526,5.2,4.05200218699999));
#332916=CARTESIAN_POINT('Ctrl Pts',(0.00246356899994526,2.2,4.05200218699999));
#332917=CARTESIAN_POINT('Ctrl Pts',(0.00231926399994364,12.2,4.05116069199998));
#332918=CARTESIAN_POINT('Ctrl Pts',(0.00231926399994364,5.2,4.05116069199998));
#332919=CARTESIAN_POINT('Ctrl Pts',(0.00231926399994364,2.2,4.05116069199998));
#332920=CARTESIAN_POINT('Ctrl Pts',(0.00217697599994459,12.2,4.05032467299999));
#332921=CARTESIAN_POINT('Ctrl Pts',(0.00217697599994459,5.2,4.05032467299999));
#332922=CARTESIAN_POINT('Ctrl Pts',(0.00217697599994459,2.2,4.05032467299999));
#332923=CARTESIAN_POINT('Ctrl Pts',(0.00203669299994379,12.2,4.04949414699999));
#332924=CARTESIAN_POINT('Ctrl Pts',(0.00203669299994379,5.2,4.04949414699999));
#332925=CARTESIAN_POINT('Ctrl Pts',(0.00203669299994379,2.2,4.04949414699999));
#332926=CARTESIAN_POINT('Ctrl Pts',(0.0018984019999435,12.2,4.04866912499998));
#332927=CARTESIAN_POINT('Ctrl Pts',(0.0018984019999435,5.2,4.04866912499998));
#332928=CARTESIAN_POINT('Ctrl Pts',(0.0018984019999435,2.2,4.04866912499998));
#332929=CARTESIAN_POINT('Ctrl Pts',(0.00176209299994289,12.2,4.04784962399999));
#332930=CARTESIAN_POINT('Ctrl Pts',(0.00176209299994289,5.2,4.04784962399999));
#332931=CARTESIAN_POINT('Ctrl Pts',(0.00176209299994289,2.2,4.04784962399999));
#332932=CARTESIAN_POINT('Ctrl Pts',(0.00162775199994413,12.2,4.04703565399998));
#332933=CARTESIAN_POINT('Ctrl Pts',(0.00162775199994413,5.2,4.04703565399998));
#332934=CARTESIAN_POINT('Ctrl Pts',(0.00162775199994413,2.2,4.04703565399998));
#332935=CARTESIAN_POINT('Ctrl Pts',(0.00149536999994425,12.2,4.04622722999999));
#332936=CARTESIAN_POINT('Ctrl Pts',(0.00149536999994425,5.2,4.04622722999999));
#332937=CARTESIAN_POINT('Ctrl Pts',(0.00149536999994425,2.2,4.04622722999999));
#332938=CARTESIAN_POINT('Ctrl Pts',(0.00136493299994433,12.2,4.04542436699998));
#332939=CARTESIAN_POINT('Ctrl Pts',(0.00136493299994433,5.2,4.04542436699998));
#332940=CARTESIAN_POINT('Ctrl Pts',(0.00136493299994433,2.2,4.04542436699998));
#332941=CARTESIAN_POINT('Ctrl Pts',(0.00123642999994344,12.2,4.04462707699999));
#332942=CARTESIAN_POINT('Ctrl Pts',(0.00123642999994344,5.2,4.04462707699999));
#332943=CARTESIAN_POINT('Ctrl Pts',(0.00123642999994344,2.2,4.04462707699999));
#332944=CARTESIAN_POINT('Ctrl Pts',(0.00110984899994392,12.2,4.04383537399998));
#332945=CARTESIAN_POINT('Ctrl Pts',(0.00110984899994392,5.2,4.04383537399998));
#332946=CARTESIAN_POINT('Ctrl Pts',(0.00110984899994392,2.2,4.04383537399998));
#332947=CARTESIAN_POINT('Ctrl Pts',(0.000985176999943596,12.2,4.04304927399998));
#332948=CARTESIAN_POINT('Ctrl Pts',(0.000985176999943596,5.2,4.04304927399998));
#332949=CARTESIAN_POINT('Ctrl Pts',(0.000985176999943596,2.2,4.04304927399998));
#332950=CARTESIAN_POINT('Ctrl Pts',(0.000862403999944963,12.2,4.04226878799999));
#332951=CARTESIAN_POINT('Ctrl Pts',(0.000862403999944963,5.2,4.04226878799999));
#332952=CARTESIAN_POINT('Ctrl Pts',(0.000862403999944963,2.2,4.04226878799999));
#332953=CARTESIAN_POINT('Ctrl Pts',(0.000741515999944644,12.2,4.04149393099999));
#332954=CARTESIAN_POINT('Ctrl Pts',(0.000741515999944644,5.2,4.04149393099999));
#332955=CARTESIAN_POINT('Ctrl Pts',(0.000741515999944644,2.2,4.04149393099999));
#332956=CARTESIAN_POINT('Ctrl Pts',(0.00062250199994395,12.2,4.04072471599999));
#332957=CARTESIAN_POINT('Ctrl Pts',(0.00062250199994395,5.2,4.04072471599999));
#332958=CARTESIAN_POINT('Ctrl Pts',(0.00062250199994395,2.2,4.04072471599999));
#332959=CARTESIAN_POINT('Ctrl Pts',(0.000505348999944024,12.2,4.03996115799998));
#332960=CARTESIAN_POINT('Ctrl Pts',(0.000505348999944024,5.2,4.03996115799998));
#332961=CARTESIAN_POINT('Ctrl Pts',(0.000505348999944024,2.2,4.03996115799998));
#332962=CARTESIAN_POINT('Ctrl Pts',(0.000390043999944903,12.2,4.03920327199998));
#332963=CARTESIAN_POINT('Ctrl Pts',(0.000390043999944903,5.2,4.03920327199998));
#332964=CARTESIAN_POINT('Ctrl Pts',(0.000390043999944903,2.2,4.03920327199998));
#332965=CARTESIAN_POINT('Ctrl Pts',(0.000276576999944647,12.2,4.03845106799999));
#332966=CARTESIAN_POINT('Ctrl Pts',(0.000276576999944647,5.2,4.03845106799999));
#332967=CARTESIAN_POINT('Ctrl Pts',(0.000276576999944647,2.2,4.03845106799999));
#332968=CARTESIAN_POINT('Ctrl Pts',(0.000164934999944402,12.2,4.03770456499998));
#332969=CARTESIAN_POINT('Ctrl Pts',(0.000164934999944402,5.2,4.03770456499998));
#332970=CARTESIAN_POINT('Ctrl Pts',(0.000164934999944402,2.2,4.03770456499998));
#332971=CARTESIAN_POINT('Ctrl Pts',(5.51029999440369E-5,12.2,4.03696377299998));
#332972=CARTESIAN_POINT('Ctrl Pts',(5.51029999440369E-5,5.2,4.03696377299998));
#332973=CARTESIAN_POINT('Ctrl Pts',(5.51029999440369E-5,2.2,4.03696377299998));
#332974=CARTESIAN_POINT('Ctrl Pts',(-5.29290000550551E-5,12.2,4.03622870699999));
#332975=CARTESIAN_POINT('Ctrl Pts',(-5.29290000550551E-5,5.2,4.03622870699999));
#332976=CARTESIAN_POINT('Ctrl Pts',(-5.29290000550551E-5,2.2,4.03622870699999));
#332977=CARTESIAN_POINT('Ctrl Pts',(-0.000159173000054977,12.2,4.03549938199999));
#332978=CARTESIAN_POINT('Ctrl Pts',(-0.000159173000054977,5.2,4.03549938199999));
#332979=CARTESIAN_POINT('Ctrl Pts',(-0.000159173000054977,2.2,4.03549938199999));
#332980=CARTESIAN_POINT('Ctrl Pts',(-0.00026364400005475,12.2,4.03477581099998));
#332981=CARTESIAN_POINT('Ctrl Pts',(-0.00026364400005475,5.2,4.03477581099998));
#332982=CARTESIAN_POINT('Ctrl Pts',(-0.00026364400005475,2.2,4.03477581099998));
#332983=CARTESIAN_POINT('Ctrl Pts',(-0.000366352000055201,12.2,4.03405800899999));
#332984=CARTESIAN_POINT('Ctrl Pts',(-0.000366352000055201,5.2,4.03405800899999));
#332985=CARTESIAN_POINT('Ctrl Pts',(-0.000366352000055201,2.2,4.03405800899999));
#332986=CARTESIAN_POINT('Ctrl Pts',(-0.000467312000056461,12.2,4.03334598799999));
#332987=CARTESIAN_POINT('Ctrl Pts',(-0.000467312000056461,5.2,4.03334598799999));
#332988=CARTESIAN_POINT('Ctrl Pts',(-0.000467312000056461,2.2,4.03334598799999));
#332989=CARTESIAN_POINT('Ctrl Pts',(-0.000566536000056192,12.2,4.03263976499999));
#332990=CARTESIAN_POINT('Ctrl Pts',(-0.000566536000056192,5.2,4.03263976499999));
#332991=CARTESIAN_POINT('Ctrl Pts',(-0.000566536000056192,2.2,4.03263976499999));
#332992=CARTESIAN_POINT('Ctrl Pts',(-0.000664036000056498,12.2,4.03193935299999));
#332993=CARTESIAN_POINT('Ctrl Pts',(-0.000664036000056498,5.2,4.03193935299999));
#332994=CARTESIAN_POINT('Ctrl Pts',(-0.000664036000056498,2.2,4.03193935299999));
#332995=CARTESIAN_POINT('Ctrl Pts',(-0.000759825000056233,12.2,4.03124476599999));
#332996=CARTESIAN_POINT('Ctrl Pts',(-0.000759825000056233,5.2,4.03124476599999));
#332997=CARTESIAN_POINT('Ctrl Pts',(-0.000759825000056233,2.2,4.03124476599999));
#332998=CARTESIAN_POINT('Ctrl Pts',(-0.000853916000055363,12.2,4.03055601799998));
#332999=CARTESIAN_POINT('Ctrl Pts',(-0.000853916000055363,5.2,4.03055601799998));
#333000=CARTESIAN_POINT('Ctrl Pts',(-0.000853916000055363,2.2,4.03055601799998));
#333001=CARTESIAN_POINT('Ctrl Pts',(-0.00094632400005624,12.2,4.02987312299998));
#333002=CARTESIAN_POINT('Ctrl Pts',(-0.00094632400005624,5.2,4.02987312299998));
#333003=CARTESIAN_POINT('Ctrl Pts',(-0.00094632400005624,2.2,4.02987312299998));
#333004=CARTESIAN_POINT('Ctrl Pts',(-0.00103705900005636,12.2,4.02919609599999));
#333005=CARTESIAN_POINT('Ctrl Pts',(-0.00103705900005636,5.2,4.02919609599999));
#333006=CARTESIAN_POINT('Ctrl Pts',(-0.00103705900005636,2.2,4.02919609599999));
#333007=CARTESIAN_POINT('Ctrl Pts',(-0.0011261340000568,12.2,4.02852495099999));
#333008=CARTESIAN_POINT('Ctrl Pts',(-0.0011261340000568,5.2,4.02852495099999));
#333009=CARTESIAN_POINT('Ctrl Pts',(-0.0011261340000568,2.2,4.02852495099999));
#333010=CARTESIAN_POINT('Ctrl Pts',(-0.00121356600005563,12.2,4.02785970199999));
#333011=CARTESIAN_POINT('Ctrl Pts',(-0.00121356600005563,5.2,4.02785970199999));
#333012=CARTESIAN_POINT('Ctrl Pts',(-0.00121356600005563,2.2,4.02785970199999));
#333013=CARTESIAN_POINT('Ctrl Pts',(-0.00129936400005582,12.2,4.02720036299999));
#333014=CARTESIAN_POINT('Ctrl Pts',(-0.00129936400005582,5.2,4.02720036299999));
#333015=CARTESIAN_POINT('Ctrl Pts',(-0.00129936400005582,2.2,4.02720036299999));
#333016=CARTESIAN_POINT('Ctrl Pts',(-0.0013835430000564,12.2,4.02654694999999));
#333017=CARTESIAN_POINT('Ctrl Pts',(-0.0013835430000564,5.2,4.02654694999999));
#333018=CARTESIAN_POINT('Ctrl Pts',(-0.0013835430000564,2.2,4.02654694999999));
#333019=CARTESIAN_POINT('Ctrl Pts',(-0.0014661160000562,12.2,4.02589947499998));
#333020=CARTESIAN_POINT('Ctrl Pts',(-0.0014661160000562,5.2,4.02589947499998));
#333021=CARTESIAN_POINT('Ctrl Pts',(-0.0014661160000562,2.2,4.02589947499998));
#333022=CARTESIAN_POINT('Ctrl Pts',(-0.00154709700005641,12.2,4.02525795499999));
#333023=CARTESIAN_POINT('Ctrl Pts',(-0.00154709700005641,5.2,4.02525795499999));
#333024=CARTESIAN_POINT('Ctrl Pts',(-0.00154709700005641,2.2,4.02525795499999));
#333025=CARTESIAN_POINT('Ctrl Pts',(-0.00162649800005466,12.2,4.02462240299998));
#333026=CARTESIAN_POINT('Ctrl Pts',(-0.00162649800005466,5.2,4.02462240299998));
#333027=CARTESIAN_POINT('Ctrl Pts',(-0.00162649800005466,2.2,4.02462240299998));
#333028=CARTESIAN_POINT('Ctrl Pts',(-0.00170433400005555,12.2,4.02399283199999));
#333029=CARTESIAN_POINT('Ctrl Pts',(-0.00170433400005555,5.2,4.02399283199999));
#333030=CARTESIAN_POINT('Ctrl Pts',(-0.00170433400005555,2.2,4.02399283199999));
#333031=CARTESIAN_POINT('Ctrl Pts',(-0.00178061700005673,12.2,4.02336925899998));
#333032=CARTESIAN_POINT('Ctrl Pts',(-0.00178061700005673,5.2,4.02336925899998));
#333033=CARTESIAN_POINT('Ctrl Pts',(-0.00178061700005673,2.2,4.02336925899998));
#333034=CARTESIAN_POINT('Ctrl Pts',(-0.00185536300005507,12.2,4.02275169799999));
#333035=CARTESIAN_POINT('Ctrl Pts',(-0.00185536300005507,5.2,4.02275169799999));
#333036=CARTESIAN_POINT('Ctrl Pts',(-0.00185536300005507,2.2,4.02275169799999));
#333037=CARTESIAN_POINT('Ctrl Pts',(-0.00192858300005595,12.2,4.02214016199999));
#333038=CARTESIAN_POINT('Ctrl Pts',(-0.00192858300005595,5.2,4.02214016199999));
#333039=CARTESIAN_POINT('Ctrl Pts',(-0.00192858300005595,2.2,4.02214016199999));
#333040=CARTESIAN_POINT('Ctrl Pts',(-0.00200029100005606,12.2,4.02153466699998));
#333041=CARTESIAN_POINT('Ctrl Pts',(-0.00200029100005606,5.2,4.02153466699998));
#333042=CARTESIAN_POINT('Ctrl Pts',(-0.00200029100005606,2.2,4.02153466699998));
#333043=CARTESIAN_POINT('Ctrl Pts',(-0.00207050200005555,12.2,4.02093522699998));
#333044=CARTESIAN_POINT('Ctrl Pts',(-0.00207050200005555,5.2,4.02093522699998));
#333045=CARTESIAN_POINT('Ctrl Pts',(-0.00207050200005555,2.2,4.02093522699998));
#333046=CARTESIAN_POINT('Ctrl Pts',(-0.00213922900005548,12.2,4.02034185699998));
#333047=CARTESIAN_POINT('Ctrl Pts',(-0.00213922900005548,5.2,4.02034185699998));
#333048=CARTESIAN_POINT('Ctrl Pts',(-0.00213922900005548,2.2,4.02034185699998));
#333049=CARTESIAN_POINT('Ctrl Pts',(-0.00220648600005481,12.2,4.01975457099999));
#333050=CARTESIAN_POINT('Ctrl Pts',(-0.00220648600005481,5.2,4.01975457099999));
#333051=CARTESIAN_POINT('Ctrl Pts',(-0.00220648600005481,2.2,4.01975457099999));
#333052=CARTESIAN_POINT('Ctrl Pts',(-0.00227228800005475,12.2,4.01917338499998));
#333053=CARTESIAN_POINT('Ctrl Pts',(-0.00227228800005475,5.2,4.01917338499998));
#333054=CARTESIAN_POINT('Ctrl Pts',(-0.00227228800005475,2.2,4.01917338499998));
#333055=CARTESIAN_POINT('Ctrl Pts',(-0.00233664700005632,12.2,4.01859831199998));
#333056=CARTESIAN_POINT('Ctrl Pts',(-0.00233664700005632,5.2,4.01859831199998));
#333057=CARTESIAN_POINT('Ctrl Pts',(-0.00233664700005632,2.2,4.01859831199998));
#333058=CARTESIAN_POINT('Ctrl Pts',(-0.0023995780000552,12.2,4.01802936699998));
#333059=CARTESIAN_POINT('Ctrl Pts',(-0.0023995780000552,5.2,4.01802936699998));
#333060=CARTESIAN_POINT('Ctrl Pts',(-0.0023995780000552,2.2,4.01802936699998));
#333061=CARTESIAN_POINT('Ctrl Pts',(-0.00246109500005588,12.2,4.01746656599999));
#333062=CARTESIAN_POINT('Ctrl Pts',(-0.00246109500005588,5.2,4.01746656599999));
#333063=CARTESIAN_POINT('Ctrl Pts',(-0.00246109500005588,2.2,4.01746656599999));
#333064=CARTESIAN_POINT('Ctrl Pts',(-0.00252121300005626,12.2,4.01690992299999));
#333065=CARTESIAN_POINT('Ctrl Pts',(-0.00252121300005626,5.2,4.01690992299999));
#333066=CARTESIAN_POINT('Ctrl Pts',(-0.00252121300005626,2.2,4.01690992299999));
#333067=CARTESIAN_POINT('Ctrl Pts',(-0.00257994500005521,12.2,4.01635945199998));
#333068=CARTESIAN_POINT('Ctrl Pts',(-0.00257994500005521,5.2,4.01635945199998));
#333069=CARTESIAN_POINT('Ctrl Pts',(-0.00257994500005521,2.2,4.01635945199998));
#333070=CARTESIAN_POINT('Ctrl Pts',(-0.00263730600005508,12.2,4.01581516899999));
#333071=CARTESIAN_POINT('Ctrl Pts',(-0.00263730600005508,5.2,4.01581516899999));
#333072=CARTESIAN_POINT('Ctrl Pts',(-0.00263730600005508,2.2,4.01581516899999));
#333073=CARTESIAN_POINT('Ctrl Pts',(-0.00269331000005591,12.2,4.01527708799998));
#333074=CARTESIAN_POINT('Ctrl Pts',(-0.00269331000005591,5.2,4.01527708799998));
#333075=CARTESIAN_POINT('Ctrl Pts',(-0.00269331000005591,2.2,4.01527708799998));
#333076=CARTESIAN_POINT('Ctrl Pts',(-0.00274797200005673,12.2,4.01474522599998));
#333077=CARTESIAN_POINT('Ctrl Pts',(-0.00274797200005673,5.2,4.01474522599998));
#333078=CARTESIAN_POINT('Ctrl Pts',(-0.00274797200005673,2.2,4.01474522599998));
#333079=CARTESIAN_POINT('Ctrl Pts',(-0.00280130500005527,12.2,4.01421959499999));
#333080=CARTESIAN_POINT('Ctrl Pts',(-0.00280130500005527,5.2,4.01421959499999));
#333081=CARTESIAN_POINT('Ctrl Pts',(-0.00280130500005527,2.2,4.01421959499999));
#333082=CARTESIAN_POINT('Ctrl Pts',(-0.00285332500005509,12.2,4.01370021099999));
#333083=CARTESIAN_POINT('Ctrl Pts',(-0.00285332500005509,5.2,4.01370021099999));
#333084=CARTESIAN_POINT('Ctrl Pts',(-0.00285332500005509,2.2,4.01370021099999));
#333085=CARTESIAN_POINT('Ctrl Pts',(-0.00290404600005623,12.2,4.01318708999998));
#333086=CARTESIAN_POINT('Ctrl Pts',(-0.00290404600005623,5.2,4.01318708999998));
#333087=CARTESIAN_POINT('Ctrl Pts',(-0.00290404600005623,2.2,4.01318708999998));
#333088=CARTESIAN_POINT('Ctrl Pts',(-0.0029534830000555,12.2,4.01268024599998));
#333089=CARTESIAN_POINT('Ctrl Pts',(-0.0029534830000555,5.2,4.01268024599998));
#333090=CARTESIAN_POINT('Ctrl Pts',(-0.0029534830000555,2.2,4.01268024599998));
#333091=CARTESIAN_POINT('Ctrl Pts',(-0.00300165000005626,12.2,4.01217969399998));
#333092=CARTESIAN_POINT('Ctrl Pts',(-0.00300165000005626,5.2,4.01217969399998));
#333093=CARTESIAN_POINT('Ctrl Pts',(-0.00300165000005626,2.2,4.01217969399998));
#333094=CARTESIAN_POINT('Ctrl Pts',(-0.00304856200005644,12.2,4.01168544899999));
#333095=CARTESIAN_POINT('Ctrl Pts',(-0.00304856200005644,5.2,4.01168544899999));
#333096=CARTESIAN_POINT('Ctrl Pts',(-0.00304856200005644,2.2,4.01168544899999));
#333097=CARTESIAN_POINT('Ctrl Pts',(-0.00309423600005521,12.2,4.01119752799998));
#333098=CARTESIAN_POINT('Ctrl Pts',(-0.00309423600005521,5.2,4.01119752799998));
#333099=CARTESIAN_POINT('Ctrl Pts',(-0.00309423600005521,2.2,4.01119752799998));
#333100=CARTESIAN_POINT('Ctrl Pts',(-0.00313868200005563,12.2,4.01071594299999));
#333101=CARTESIAN_POINT('Ctrl Pts',(-0.00313868200005563,5.2,4.01071594299999));
#333102=CARTESIAN_POINT('Ctrl Pts',(-0.00313868200005563,2.2,4.01071594299999));
#333103=CARTESIAN_POINT('Ctrl Pts',(-0.00318192000005602,12.2,4.01024071099998));
#333104=CARTESIAN_POINT('Ctrl Pts',(-0.00318192000005602,5.2,4.01024071099998));
#333105=CARTESIAN_POINT('Ctrl Pts',(-0.00318192000005602,2.2,4.01024071099998));
#333106=CARTESIAN_POINT('Ctrl Pts',(-0.00322396300005635,12.2,4.00977184799999));
#333107=CARTESIAN_POINT('Ctrl Pts',(-0.00322396300005635,5.2,4.00977184799999));
#333108=CARTESIAN_POINT('Ctrl Pts',(-0.00322396300005635,2.2,4.00977184799999));
#333109=CARTESIAN_POINT('Ctrl Pts',(-0.00326482500005555,12.2,4.00930936699999));
#333110=CARTESIAN_POINT('Ctrl Pts',(-0.00326482500005555,5.2,4.00930936699999));
#333111=CARTESIAN_POINT('Ctrl Pts',(-0.00326482500005555,2.2,4.00930936699999));
#333112=CARTESIAN_POINT('Ctrl Pts',(-0.00330452400005511,12.2,4.00885328399998));
#333113=CARTESIAN_POINT('Ctrl Pts',(-0.00330452400005511,5.2,4.00885328399998));
#333114=CARTESIAN_POINT('Ctrl Pts',(-0.00330452400005511,2.2,4.00885328399998));
#333115=CARTESIAN_POINT('Ctrl Pts',(-0.00334307200005602,12.2,4.00840361499998));
#333116=CARTESIAN_POINT('Ctrl Pts',(-0.00334307200005602,5.2,4.00840361499998));
#333117=CARTESIAN_POINT('Ctrl Pts',(-0.00334307200005602,2.2,4.00840361499998));
#333118=CARTESIAN_POINT('Ctrl Pts',(-0.00338048600005637,12.2,4.00796037499998));
#333119=CARTESIAN_POINT('Ctrl Pts',(-0.00338048600005637,5.2,4.00796037499998));
#333120=CARTESIAN_POINT('Ctrl Pts',(-0.00338048600005637,2.2,4.00796037499998));
#333121=CARTESIAN_POINT('Ctrl Pts',(-0.00341678200005525,12.2,4.00752357899999));
#333122=CARTESIAN_POINT('Ctrl Pts',(-0.00341678200005525,5.2,4.00752357899999));
#333123=CARTESIAN_POINT('Ctrl Pts',(-0.00341678200005525,2.2,4.00752357899999));
#333124=CARTESIAN_POINT('Ctrl Pts',(-0.00345197500005613,12.2,4.00709324299999));
#333125=CARTESIAN_POINT('Ctrl Pts',(-0.00345197500005613,5.2,4.00709324299999));
#333126=CARTESIAN_POINT('Ctrl Pts',(-0.00345197500005613,2.2,4.00709324299999));
#333127=CARTESIAN_POINT('Ctrl Pts',(-0.00348607900005683,12.2,4.00666938199999));
#333128=CARTESIAN_POINT('Ctrl Pts',(-0.00348607900005683,5.2,4.00666938199999));
#333129=CARTESIAN_POINT('Ctrl Pts',(-0.00348607900005683,2.2,4.00666938199999));
#333130=CARTESIAN_POINT('Ctrl Pts',(-0.00351911100005543,12.2,4.00625201199999));
#333131=CARTESIAN_POINT('Ctrl Pts',(-0.00351911100005543,5.2,4.00625201199999));
#333132=CARTESIAN_POINT('Ctrl Pts',(-0.00351911100005543,2.2,4.00625201199999));
#333133=CARTESIAN_POINT('Ctrl Pts',(-0.0035510860000565,12.2,4.00584114699999));
#333134=CARTESIAN_POINT('Ctrl Pts',(-0.0035510860000565,5.2,4.00584114699999));
#333135=CARTESIAN_POINT('Ctrl Pts',(-0.0035510860000565,2.2,4.00584114699999));
#333136=CARTESIAN_POINT('Ctrl Pts',(-0.0035820210000559,12.2,4.00543680299998));
#333137=CARTESIAN_POINT('Ctrl Pts',(-0.0035820210000559,5.2,4.00543680299998));
#333138=CARTESIAN_POINT('Ctrl Pts',(-0.0035820210000559,2.2,4.00543680299998));
#333139=CARTESIAN_POINT('Ctrl Pts',(-0.003611930000057,12.2,4.00503899699999));
#333140=CARTESIAN_POINT('Ctrl Pts',(-0.003611930000057,5.2,4.00503899699999));
#333141=CARTESIAN_POINT('Ctrl Pts',(-0.003611930000057,2.2,4.00503899699999));
#333142=CARTESIAN_POINT('Ctrl Pts',(-0.00364083000005456,12.2,4.00464774299999));
#333143=CARTESIAN_POINT('Ctrl Pts',(-0.00364083000005456,5.2,4.00464774299999));
#333144=CARTESIAN_POINT('Ctrl Pts',(-0.00364083000005456,2.2,4.00464774299999));
#333145=CARTESIAN_POINT('Ctrl Pts',(-0.00366873600005647,12.2,4.00426305799999));
#333146=CARTESIAN_POINT('Ctrl Pts',(-0.00366873600005647,5.2,4.00426305799999));
#333147=CARTESIAN_POINT('Ctrl Pts',(-0.00366873600005647,2.2,4.00426305799999));
#333148=CARTESIAN_POINT('Ctrl Pts',(-0.00369566500005526,12.2,4.00388495599999));
#333149=CARTESIAN_POINT('Ctrl Pts',(-0.00369566500005526,5.2,4.00388495599999));
#333150=CARTESIAN_POINT('Ctrl Pts',(-0.00369566500005526,2.2,4.00388495599999));
#333151=CARTESIAN_POINT('Ctrl Pts',(-0.00372163300005669,12.2,4.00351345299998));
#333152=CARTESIAN_POINT('Ctrl Pts',(-0.00372163300005669,5.2,4.00351345299998));
#333153=CARTESIAN_POINT('Ctrl Pts',(-0.00372163300005669,2.2,4.00351345299998));
#333154=CARTESIAN_POINT('Ctrl Pts',(-0.00374665500005534,12.2,4.00314856599999));
#333155=CARTESIAN_POINT('Ctrl Pts',(-0.00374665500005534,5.2,4.00314856599999));
#333156=CARTESIAN_POINT('Ctrl Pts',(-0.00374665500005534,2.2,4.00314856599999));
#333157=CARTESIAN_POINT('Ctrl Pts',(-0.00377074800005595,12.2,4.00279030999998));
#333158=CARTESIAN_POINT('Ctrl Pts',(-0.00377074800005595,5.2,4.00279030999998));
#333159=CARTESIAN_POINT('Ctrl Pts',(-0.00377074800005595,2.2,4.00279030999998));
#333160=CARTESIAN_POINT('Ctrl Pts',(-0.00379393000005558,12.2,4.00243869999999));
#333161=CARTESIAN_POINT('Ctrl Pts',(-0.00379393000005558,5.2,4.00243869999999));
#333162=CARTESIAN_POINT('Ctrl Pts',(-0.00379393000005558,2.2,4.00243869999999));
#333163=CARTESIAN_POINT('Ctrl Pts',(-0.00381621400005528,12.2,4.00209375199999));
#333164=CARTESIAN_POINT('Ctrl Pts',(-0.00381621400005528,5.2,4.00209375199999));
#333165=CARTESIAN_POINT('Ctrl Pts',(-0.00381621400005528,2.2,4.00209375199999));
#333166=CARTESIAN_POINT('Ctrl Pts',(-0.00383761700005537,12.2,4.00175548199999));
#333167=CARTESIAN_POINT('Ctrl Pts',(-0.00383761700005537,5.2,4.00175548199999));
#333168=CARTESIAN_POINT('Ctrl Pts',(-0.00383761700005537,2.2,4.00175548199999));
#333169=CARTESIAN_POINT('Ctrl Pts',(-0.0038581580000563,12.2,4.00142390699998));
#333170=CARTESIAN_POINT('Ctrl Pts',(-0.0038581580000563,5.2,4.00142390699998));
#333171=CARTESIAN_POINT('Ctrl Pts',(-0.0038581580000563,2.2,4.00142390699998));
#333172=CARTESIAN_POINT('Ctrl Pts',(-0.00387785200005487,12.2,4.00109904099998));
#333173=CARTESIAN_POINT('Ctrl Pts',(-0.00387785200005487,5.2,4.00109904099998));
#333174=CARTESIAN_POINT('Ctrl Pts',(-0.00387785200005487,2.2,4.00109904099998));
#333175=CARTESIAN_POINT('Ctrl Pts',(-0.00389671400005676,12.2,4.00078090299999));
#333176=CARTESIAN_POINT('Ctrl Pts',(-0.00389671400005676,5.2,4.00078090299999));
#333177=CARTESIAN_POINT('Ctrl Pts',(-0.00389671400005676,2.2,4.00078090299999));
#333178=CARTESIAN_POINT('Ctrl Pts',(-0.00391476500005595,12.2,4.00046950499998));
#333179=CARTESIAN_POINT('Ctrl Pts',(-0.00391476500005595,5.2,4.00046950499998));
#333180=CARTESIAN_POINT('Ctrl Pts',(-0.00391476500005595,2.2,4.00046950499998));
#333181=CARTESIAN_POINT('Ctrl Pts',(-0.00393201700005564,12.2,4.00016486499998));
#333182=CARTESIAN_POINT('Ctrl Pts',(-0.00393201700005564,5.2,4.00016486499998));
#333183=CARTESIAN_POINT('Ctrl Pts',(-0.00393201700005564,2.2,4.00016486499998));
#333184=CARTESIAN_POINT('Ctrl Pts',(-0.00394849000005527,12.2,3.99986699899999));
#333185=CARTESIAN_POINT('Ctrl Pts',(-0.00394849000005527,5.2,3.99986699899999));
#333186=CARTESIAN_POINT('Ctrl Pts',(-0.00394849000005527,2.2,3.99986699899999));
#333187=CARTESIAN_POINT('Ctrl Pts',(-0.00396419900005497,12.2,3.99957592299998));
#333188=CARTESIAN_POINT('Ctrl Pts',(-0.00396419900005497,5.2,3.99957592299998));
#333189=CARTESIAN_POINT('Ctrl Pts',(-0.00396419900005497,2.2,3.99957592299998));
#333190=CARTESIAN_POINT('Ctrl Pts',(-0.00397916300005519,12.2,3.99929165399998));
#333191=CARTESIAN_POINT('Ctrl Pts',(-0.00397916300005519,5.2,3.99929165399998));
#333192=CARTESIAN_POINT('Ctrl Pts',(-0.00397916300005519,2.2,3.99929165399998));
#333193=CARTESIAN_POINT('Ctrl Pts',(-0.00399339700005497,12.2,3.99901420599999));
#333194=CARTESIAN_POINT('Ctrl Pts',(-0.00399339700005497,5.2,3.99901420599999));
#333195=CARTESIAN_POINT('Ctrl Pts',(-0.00399339700005497,2.2,3.99901420599999));
#333196=CARTESIAN_POINT('Ctrl Pts',(-0.00400692000005477,12.2,3.99874359799998));
#333197=CARTESIAN_POINT('Ctrl Pts',(-0.00400692000005477,5.2,3.99874359799998));
#333198=CARTESIAN_POINT('Ctrl Pts',(-0.00400692000005477,2.2,3.99874359799998));
#333199=CARTESIAN_POINT('Ctrl Pts',(-0.00401974900005598,12.2,3.99847984399998));
#333200=CARTESIAN_POINT('Ctrl Pts',(-0.00401974900005598,5.2,3.99847984399998));
#333201=CARTESIAN_POINT('Ctrl Pts',(-0.00401974900005598,2.2,3.99847984399998));
#333202=CARTESIAN_POINT('Ctrl Pts',(-0.0040319000000555,12.2,3.99822295999999));
#333203=CARTESIAN_POINT('Ctrl Pts',(-0.0040319000000555,5.2,3.99822295999999));
#333204=CARTESIAN_POINT('Ctrl Pts',(-0.0040319000000555,2.2,3.99822295999999));
#333205=CARTESIAN_POINT('Ctrl Pts',(-0.00404339100005592,12.2,3.99797296399999));
#333206=CARTESIAN_POINT('Ctrl Pts',(-0.00404339100005592,5.2,3.99797296399999));
#333207=CARTESIAN_POINT('Ctrl Pts',(-0.00404339100005592,2.2,3.99797296399999));
#333208=CARTESIAN_POINT('Ctrl Pts',(-0.0040542400000554,12.2,3.99772987199999));
#333209=CARTESIAN_POINT('Ctrl Pts',(-0.0040542400000554,5.2,3.99772987199999));
#333210=CARTESIAN_POINT('Ctrl Pts',(-0.0040542400000554,2.2,3.99772987199999));
#333211=CARTESIAN_POINT('Ctrl Pts',(-0.00406446400005534,12.2,3.99749369899999));
#333212=CARTESIAN_POINT('Ctrl Pts',(-0.00406446400005534,5.2,3.99749369899999));
#333213=CARTESIAN_POINT('Ctrl Pts',(-0.00406446400005534,2.2,3.99749369899999));
#333214=CARTESIAN_POINT('Ctrl Pts',(-0.00407408100005503,12.2,3.99726446299999));
#333215=CARTESIAN_POINT('Ctrl Pts',(-0.00407408100005503,5.2,3.99726446299999));
#333216=CARTESIAN_POINT('Ctrl Pts',(-0.00407408100005503,2.2,3.99726446299999));
#333217=CARTESIAN_POINT('Ctrl Pts',(-0.00408310700005577,12.2,3.99704217899998));
#333218=CARTESIAN_POINT('Ctrl Pts',(-0.00408310700005577,5.2,3.99704217899998));
#333219=CARTESIAN_POINT('Ctrl Pts',(-0.00408310700005577,2.2,3.99704217899998));
#333220=CARTESIAN_POINT('Ctrl Pts',(-0.00409156300005598,12.2,3.99682686399998));
#333221=CARTESIAN_POINT('Ctrl Pts',(-0.00409156300005598,5.2,3.99682686399998));
#333222=CARTESIAN_POINT('Ctrl Pts',(-0.00409156300005598,2.2,3.99682686399998));
#333223=CARTESIAN_POINT('Ctrl Pts',(-0.00409946400005579,12.2,3.99661853599999));
#333224=CARTESIAN_POINT('Ctrl Pts',(-0.00409946400005579,5.2,3.99661853599999));
#333225=CARTESIAN_POINT('Ctrl Pts',(-0.00409946400005579,2.2,3.99661853599999));
#333226=CARTESIAN_POINT('Ctrl Pts',(-0.00410683100005583,12.2,3.99641720899999));
#333227=CARTESIAN_POINT('Ctrl Pts',(-0.00410683100005583,5.2,3.99641720899999));
#333228=CARTESIAN_POINT('Ctrl Pts',(-0.00410683100005583,2.2,3.99641720899999));
#333229=CARTESIAN_POINT('Ctrl Pts',(-0.00411367900005622,12.2,3.99622290199999));
#333230=CARTESIAN_POINT('Ctrl Pts',(-0.00411367900005622,5.2,3.99622290199999));
#333231=CARTESIAN_POINT('Ctrl Pts',(-0.00411367900005622,2.2,3.99622290199999));
#333232=CARTESIAN_POINT('Ctrl Pts',(-0.0041200280000553,12.2,3.99603563099999));
#333233=CARTESIAN_POINT('Ctrl Pts',(-0.0041200280000553,5.2,3.99603563099999));
#333234=CARTESIAN_POINT('Ctrl Pts',(-0.0041200280000553,2.2,3.99603563099999));
#333235=CARTESIAN_POINT('Ctrl Pts',(-0.00412589600005676,12.2,3.99585541199999));
#333236=CARTESIAN_POINT('Ctrl Pts',(-0.00412589600005676,5.2,3.99585541199999));
#333237=CARTESIAN_POINT('Ctrl Pts',(-0.00412589600005676,2.2,3.99585541199999));
#333238=CARTESIAN_POINT('Ctrl Pts',(-0.00413130000005536,12.2,3.99568226099999));
#333239=CARTESIAN_POINT('Ctrl Pts',(-0.00413130000005536,5.2,3.99568226099999));
#333240=CARTESIAN_POINT('Ctrl Pts',(-0.00413130000005536,2.2,3.99568226099999));
#333241=CARTESIAN_POINT('Ctrl Pts',(-0.00413625800005591,12.2,3.99551619599999));
#333242=CARTESIAN_POINT('Ctrl Pts',(-0.00413625800005591,5.2,3.99551619599999));
#333243=CARTESIAN_POINT('Ctrl Pts',(-0.00413625800005591,2.2,3.99551619599999));
#333244=CARTESIAN_POINT('Ctrl Pts',(-0.00414079000005564,12.2,3.99535723299999));
#333245=CARTESIAN_POINT('Ctrl Pts',(-0.00414079000005564,5.2,3.99535723299999));
#333246=CARTESIAN_POINT('Ctrl Pts',(-0.00414079000005564,2.2,3.99535723299999));
#333247=CARTESIAN_POINT('Ctrl Pts',(-0.00414491200005585,12.2,3.99520538699999));
#333248=CARTESIAN_POINT('Ctrl Pts',(-0.00414491200005585,5.2,3.99520538699999));
#333249=CARTESIAN_POINT('Ctrl Pts',(-0.00414491200005585,2.2,3.99520538699999));
#333250=CARTESIAN_POINT('Ctrl Pts',(-0.00414864600005616,12.2,3.99506067999998));
#333251=CARTESIAN_POINT('Ctrl Pts',(-0.00414864600005616,5.2,3.99506067999998));
#333252=CARTESIAN_POINT('Ctrl Pts',(-0.00414864600005616,2.2,3.99506067999998));
#333253=CARTESIAN_POINT('Ctrl Pts',(-0.00415201100005481,12.2,3.99492312699999));
#333254=CARTESIAN_POINT('Ctrl Pts',(-0.00415201100005481,5.2,3.99492312699999));
#333255=CARTESIAN_POINT('Ctrl Pts',(-0.00415201100005481,2.2,3.99492312699999));
#333256=CARTESIAN_POINT('Ctrl Pts',(-0.00415502700005566,12.2,3.99479274399998));
#333257=CARTESIAN_POINT('Ctrl Pts',(-0.00415502700005566,5.2,3.99479274399998));
#333258=CARTESIAN_POINT('Ctrl Pts',(-0.00415502700005566,2.2,3.99479274399998));
#333259=CARTESIAN_POINT('Ctrl Pts',(-0.00415771000005561,12.2,3.99466955099999));
#333260=CARTESIAN_POINT('Ctrl Pts',(-0.00415771000005561,5.2,3.99466955099999));
#333261=CARTESIAN_POINT('Ctrl Pts',(-0.00415771000005561,2.2,3.99466955099999));
#333262=CARTESIAN_POINT('Ctrl Pts',(-0.0041600800000552,12.2,3.99455356199999));
#333263=CARTESIAN_POINT('Ctrl Pts',(-0.0041600800000552,5.2,3.99455356199999));
#333264=CARTESIAN_POINT('Ctrl Pts',(-0.0041600800000552,2.2,3.99455356199999));
#333265=CARTESIAN_POINT('Ctrl Pts',(-0.00416215300005574,12.2,3.99444479099999));
#333266=CARTESIAN_POINT('Ctrl Pts',(-0.00416215300005574,5.2,3.99444479099999));
#333267=CARTESIAN_POINT('Ctrl Pts',(-0.00416215300005574,2.2,3.99444479099999));
#333268=CARTESIAN_POINT('Ctrl Pts',(-0.00416394400005627,12.2,3.99434325499998));
#333269=CARTESIAN_POINT('Ctrl Pts',(-0.00416394400005627,5.2,3.99434325499998));
#333270=CARTESIAN_POINT('Ctrl Pts',(-0.00416394400005627,2.2,3.99434325499998));
#333271=CARTESIAN_POINT('Ctrl Pts',(-0.00416547700005544,12.2,3.99424897099999));
#333272=CARTESIAN_POINT('Ctrl Pts',(-0.00416547700005544,5.2,3.99424897099999));
#333273=CARTESIAN_POINT('Ctrl Pts',(-0.00416547700005544,2.2,3.99424897099999));
#333274=CARTESIAN_POINT('Ctrl Pts',(-0.00416677000005584,12.2,3.99416195899998));
#333275=CARTESIAN_POINT('Ctrl Pts',(-0.00416677000005584,5.2,3.99416195899998));
#333276=CARTESIAN_POINT('Ctrl Pts',(-0.00416677000005584,2.2,3.99416195899998));
#333277=CARTESIAN_POINT('Ctrl Pts',(-0.00416785000005638,12.2,3.99408223999998));
#333278=CARTESIAN_POINT('Ctrl Pts',(-0.00416785000005638,5.2,3.99408223999998));
#333279=CARTESIAN_POINT('Ctrl Pts',(-0.00416785000005638,2.2,3.99408223999998));
#333280=CARTESIAN_POINT('Ctrl Pts',(-0.0041687420000558,12.2,3.99400983799998));
#333281=CARTESIAN_POINT('Ctrl Pts',(-0.0041687420000558,5.2,3.99400983799998));
#333282=CARTESIAN_POINT('Ctrl Pts',(-0.0041687420000558,2.2,3.99400983799998));
#333283=CARTESIAN_POINT('Ctrl Pts',(-0.00416946500005567,12.2,3.99394476899998));
#333284=CARTESIAN_POINT('Ctrl Pts',(-0.00416946500005567,5.2,3.99394476899998));
#333285=CARTESIAN_POINT('Ctrl Pts',(-0.00416946500005567,2.2,3.99394476899998));
#333286=CARTESIAN_POINT('Ctrl Pts',(-0.00417003700005637,12.2,3.99388704899999));
#333287=CARTESIAN_POINT('Ctrl Pts',(-0.00417003700005637,5.2,3.99388704899999));
#333288=CARTESIAN_POINT('Ctrl Pts',(-0.00417003700005637,2.2,3.99388704899999));
#333289=CARTESIAN_POINT('Ctrl Pts',(-0.00417051303328587,12.2,3.99383129333122));
#333290=CARTESIAN_POINT('Ctrl Pts',(-0.00417051303328587,5.2,3.99383129333122));
#333291=CARTESIAN_POINT('Ctrl Pts',(-0.00417051303328587,2.2,3.99383129333122));
#333292=CARTESIAN_POINT('Ctrl Pts',(-0.00417076165687092,12.2,3.99379318127802));
#333293=CARTESIAN_POINT('Ctrl Pts',(-0.00417076165687092,5.2,3.99379318127802));
#333294=CARTESIAN_POINT('Ctrl Pts',(-0.00417076165687092,2.2,3.99379318127802));
#333295=CARTESIAN_POINT('Ctrl Pts',(-0.00417087178589682,12.2,3.99376807430458));
#333296=CARTESIAN_POINT('Ctrl Pts',(-0.00417087178589682,5.2,3.99376807430458));
#333297=CARTESIAN_POINT('Ctrl Pts',(-0.00417087178589682,2.2,3.99376807430458));
#333298=CARTESIAN_POINT('Ctrl Pts',(-0.00417090550046129,12.2,3.99375243386499));
#333299=CARTESIAN_POINT('Ctrl Pts',(-0.00417090550046129,5.2,3.99375243386499));
#333300=CARTESIAN_POINT('Ctrl Pts',(-0.00417090550046129,2.2,3.99375243386499));
#333301=CARTESIAN_POINT('Ctrl Pts',(-0.00417093000005587,12.2,3.99374277699999));
#333302=CARTESIAN_POINT('Ctrl Pts',(-0.00417093000005587,5.2,3.99374277699999));
#333303=CARTESIAN_POINT('Ctrl Pts',(-0.00417093000005587,2.2,3.99374277699999));
#333304=CARTESIAN_POINT('',(0.335933473999944,12.2,4.73810602499999));
#333305=CARTESIAN_POINT('Origin',(-5.66300478732629E-14,15.2,-1.77635683940025E-14));
#333306=CARTESIAN_POINT('',(0.671001528999944,12.2,4.70236716499999));
#333307=CARTESIAN_POINT('Ctrl Pts',(0.846447287999944,12.2,3.90299745399999));
#333308=CARTESIAN_POINT('Ctrl Pts',(0.846447287999944,5.2,3.90299745399999));
#333309=CARTESIAN_POINT('Ctrl Pts',(0.846447287999944,2.2,3.90299745399999));
#333310=CARTESIAN_POINT('Ctrl Pts',(0.846448712915784,12.2,3.90300414660476));
#333311=CARTESIAN_POINT('Ctrl Pts',(0.846448712915784,5.2,3.90300414660476));
#333312=CARTESIAN_POINT('Ctrl Pts',(0.846448712915784,2.2,3.90300414660476));
#333313=CARTESIAN_POINT('Ctrl Pts',(0.846451469166328,12.2,3.90301709034366));
#333314=CARTESIAN_POINT('Ctrl Pts',(0.846451469166328,5.2,3.90301709034366));
#333315=CARTESIAN_POINT('Ctrl Pts',(0.846451469166328,2.2,3.90301709034366));
#333316=CARTESIAN_POINT('Ctrl Pts',(0.846455551098625,12.2,3.90303629127475));
#333317=CARTESIAN_POINT('Ctrl Pts',(0.846455551098625,5.19999999999999,
3.90303629127475));
#333318=CARTESIAN_POINT('Ctrl Pts',(0.846455551098625,2.2,3.90303629127475));
#333319=CARTESIAN_POINT('Ctrl Pts',(0.846460993740913,12.2,3.90306169326758));
#333320=CARTESIAN_POINT('Ctrl Pts',(0.846460993740913,5.2,3.90306169326758));
#333321=CARTESIAN_POINT('Ctrl Pts',(0.846460993740913,2.2,3.90306169326758));
#333322=CARTESIAN_POINT('Ctrl Pts',(0.846470204999944,12.2,3.90310607699998));
#333323=CARTESIAN_POINT('Ctrl Pts',(0.846470204999944,5.2,3.90310607699998));
#333324=CARTESIAN_POINT('Ctrl Pts',(0.846470204999944,2.2,3.90310607699998));
#333325=CARTESIAN_POINT('Ctrl Pts',(0.846480406999944,12.2,3.90315539799998));
#333326=CARTESIAN_POINT('Ctrl Pts',(0.846480406999944,5.2,3.90315539799998));
#333327=CARTESIAN_POINT('Ctrl Pts',(0.846480406999944,2.2,3.90315539799998));
#333328=CARTESIAN_POINT('Ctrl Pts',(0.846492022999944,12.2,3.90321194099998));
#333329=CARTESIAN_POINT('Ctrl Pts',(0.846492022999944,5.2,3.90321194099998));
#333330=CARTESIAN_POINT('Ctrl Pts',(0.846492022999944,2.2,3.90321194099998));
#333331=CARTESIAN_POINT('Ctrl Pts',(0.846505039999944,12.2,3.90327569799998));
#333332=CARTESIAN_POINT('Ctrl Pts',(0.846505039999944,5.2,3.90327569799998));
#333333=CARTESIAN_POINT('Ctrl Pts',(0.846505039999944,2.2,3.90327569799998));
#333334=CARTESIAN_POINT('Ctrl Pts',(0.846519438999944,12.2,3.90334666099999));
#333335=CARTESIAN_POINT('Ctrl Pts',(0.846519438999944,5.2,3.90334666099999));
#333336=CARTESIAN_POINT('Ctrl Pts',(0.846519438999944,2.2,3.90334666099999));
#333337=CARTESIAN_POINT('Ctrl Pts',(0.846535197999944,12.2,3.90342481399998));
#333338=CARTESIAN_POINT('Ctrl Pts',(0.846535197999944,5.2,3.90342481399998));
#333339=CARTESIAN_POINT('Ctrl Pts',(0.846535197999944,2.2,3.90342481399998));
#333340=CARTESIAN_POINT('Ctrl Pts',(0.846552286999944,12.2,3.90351014099998));
#333341=CARTESIAN_POINT('Ctrl Pts',(0.846552286999944,5.2,3.90351014099998));
#333342=CARTESIAN_POINT('Ctrl Pts',(0.846552286999944,2.2,3.90351014099998));
#333343=CARTESIAN_POINT('Ctrl Pts',(0.846570675999944,12.2,3.90360262699998));
#333344=CARTESIAN_POINT('Ctrl Pts',(0.846570675999944,5.2,3.90360262699998));
#333345=CARTESIAN_POINT('Ctrl Pts',(0.846570675999944,2.2,3.90360262699998));
#333346=CARTESIAN_POINT('Ctrl Pts',(0.846590339999944,12.2,3.90370225599998));
#333347=CARTESIAN_POINT('Ctrl Pts',(0.846590339999944,5.2,3.90370225599998));
#333348=CARTESIAN_POINT('Ctrl Pts',(0.846590339999944,2.2,3.90370225599998));
#333349=CARTESIAN_POINT('Ctrl Pts',(0.846611256999944,12.2,3.90380901799999));
#333350=CARTESIAN_POINT('Ctrl Pts',(0.846611256999944,5.2,3.90380901799999));
#333351=CARTESIAN_POINT('Ctrl Pts',(0.846611256999944,2.2,3.90380901799999));
#333352=CARTESIAN_POINT('Ctrl Pts',(0.846633405999944,12.2,3.90392289699999));
#333353=CARTESIAN_POINT('Ctrl Pts',(0.846633405999944,5.2,3.90392289699999));
#333354=CARTESIAN_POINT('Ctrl Pts',(0.846633405999944,2.2,3.90392289699999));
#333355=CARTESIAN_POINT('Ctrl Pts',(0.846656765999944,12.2,3.90404388499999));
#333356=CARTESIAN_POINT('Ctrl Pts',(0.846656765999944,5.2,3.90404388499999));
#333357=CARTESIAN_POINT('Ctrl Pts',(0.846656765999944,2.2,3.90404388499999));
#333358=CARTESIAN_POINT('Ctrl Pts',(0.846681319999945,12.2,3.90417196899998));
#333359=CARTESIAN_POINT('Ctrl Pts',(0.846681319999945,5.2,3.90417196899998));
#333360=CARTESIAN_POINT('Ctrl Pts',(0.846681319999945,2.2,3.90417196899998));
#333361=CARTESIAN_POINT('Ctrl Pts',(0.846707043999944,12.2,3.90430713799999));
#333362=CARTESIAN_POINT('Ctrl Pts',(0.846707043999944,5.2,3.90430713799999));
#333363=CARTESIAN_POINT('Ctrl Pts',(0.846707043999944,2.2,3.90430713799999));
#333364=CARTESIAN_POINT('Ctrl Pts',(0.846733914999944,12.2,3.90444937799998));
#333365=CARTESIAN_POINT('Ctrl Pts',(0.846733914999944,5.2,3.90444937799998));
#333366=CARTESIAN_POINT('Ctrl Pts',(0.846733914999944,2.2,3.90444937799998));
#333367=CARTESIAN_POINT('Ctrl Pts',(0.846761912999944,12.2,3.90459867599999));
#333368=CARTESIAN_POINT('Ctrl Pts',(0.846761912999944,5.2,3.90459867599999));
#333369=CARTESIAN_POINT('Ctrl Pts',(0.846761912999944,2.2,3.90459867599999));
#333370=CARTESIAN_POINT('Ctrl Pts',(0.846791012999945,12.2,3.90475501999998));
#333371=CARTESIAN_POINT('Ctrl Pts',(0.846791012999945,5.2,3.90475501999998));
#333372=CARTESIAN_POINT('Ctrl Pts',(0.846791012999945,2.2,3.90475501999998));
#333373=CARTESIAN_POINT('Ctrl Pts',(0.846821192999945,12.2,3.90491839499998));
#333374=CARTESIAN_POINT('Ctrl Pts',(0.846821192999945,5.2,3.90491839499998));
#333375=CARTESIAN_POINT('Ctrl Pts',(0.846821192999945,2.2,3.90491839499998));
#333376=CARTESIAN_POINT('Ctrl Pts',(0.846852431999944,12.2,3.90508878899999));
#333377=CARTESIAN_POINT('Ctrl Pts',(0.846852431999944,5.2,3.90508878899999));
#333378=CARTESIAN_POINT('Ctrl Pts',(0.846852431999944,2.2,3.90508878899999));
#333379=CARTESIAN_POINT('Ctrl Pts',(0.846884708999944,12.2,3.90526619099998));
#333380=CARTESIAN_POINT('Ctrl Pts',(0.846884708999944,5.2,3.90526619099998));
#333381=CARTESIAN_POINT('Ctrl Pts',(0.846884708999944,2.2,3.90526619099998));
#333382=CARTESIAN_POINT('Ctrl Pts',(0.846918002999945,12.2,3.90545058899999));
#333383=CARTESIAN_POINT('Ctrl Pts',(0.846918002999945,5.2,3.90545058899999));
#333384=CARTESIAN_POINT('Ctrl Pts',(0.846918002999945,2.2,3.90545058899999));
#333385=CARTESIAN_POINT('Ctrl Pts',(0.846952291999944,12.2,3.90564196899999));
#333386=CARTESIAN_POINT('Ctrl Pts',(0.846952291999944,5.2,3.90564196899999));
#333387=CARTESIAN_POINT('Ctrl Pts',(0.846952291999944,2.2,3.90564196899999));
#333388=CARTESIAN_POINT('Ctrl Pts',(0.846987556999944,12.2,3.90584031899999));
#333389=CARTESIAN_POINT('Ctrl Pts',(0.846987556999944,5.2,3.90584031899999));
#333390=CARTESIAN_POINT('Ctrl Pts',(0.846987556999944,2.2,3.90584031899999));
#333391=CARTESIAN_POINT('Ctrl Pts',(0.847023773999944,12.2,3.90604562799999));
#333392=CARTESIAN_POINT('Ctrl Pts',(0.847023773999944,5.2,3.90604562799999));
#333393=CARTESIAN_POINT('Ctrl Pts',(0.847023773999944,2.2,3.90604562799999));
#333394=CARTESIAN_POINT('Ctrl Pts',(0.847060923999944,12.2,3.90625788299998));
#333395=CARTESIAN_POINT('Ctrl Pts',(0.847060923999944,5.2,3.90625788299998));
#333396=CARTESIAN_POINT('Ctrl Pts',(0.847060923999944,2.2,3.90625788299998));
#333397=CARTESIAN_POINT('Ctrl Pts',(0.847098984999944,12.2,3.90647706899999));
#333398=CARTESIAN_POINT('Ctrl Pts',(0.847098984999944,5.2,3.90647706899999));
#333399=CARTESIAN_POINT('Ctrl Pts',(0.847098984999944,2.2,3.90647706899999));
#333400=CARTESIAN_POINT('Ctrl Pts',(0.847137935999944,12.2,3.90670317699998));
#333401=CARTESIAN_POINT('Ctrl Pts',(0.847137935999944,5.2,3.90670317699998));
#333402=CARTESIAN_POINT('Ctrl Pts',(0.847137935999944,2.2,3.90670317699998));
#333403=CARTESIAN_POINT('Ctrl Pts',(0.847177756999944,12.2,3.90693619299999));
#333404=CARTESIAN_POINT('Ctrl Pts',(0.847177756999944,5.2,3.90693619299999));
#333405=CARTESIAN_POINT('Ctrl Pts',(0.847177756999944,2.2,3.90693619299999));
#333406=CARTESIAN_POINT('Ctrl Pts',(0.847218424999945,12.2,3.90717610499999));
#333407=CARTESIAN_POINT('Ctrl Pts',(0.847218424999945,5.2,3.90717610499999));
#333408=CARTESIAN_POINT('Ctrl Pts',(0.847218424999945,2.2,3.90717610499999));
#333409=CARTESIAN_POINT('Ctrl Pts',(0.847259921999944,12.2,3.90742289999999));
#333410=CARTESIAN_POINT('Ctrl Pts',(0.847259921999944,5.2,3.90742289999999));
#333411=CARTESIAN_POINT('Ctrl Pts',(0.847259921999944,2.2,3.90742289999999));
#333412=CARTESIAN_POINT('Ctrl Pts',(0.847302226999944,12.2,3.90767656699998));
#333413=CARTESIAN_POINT('Ctrl Pts',(0.847302226999944,5.2,3.90767656699998));
#333414=CARTESIAN_POINT('Ctrl Pts',(0.847302226999944,2.2,3.90767656699998));
#333415=CARTESIAN_POINT('Ctrl Pts',(0.847345319999944,12.2,3.90793709299999));
#333416=CARTESIAN_POINT('Ctrl Pts',(0.847345319999944,5.2,3.90793709299999));
#333417=CARTESIAN_POINT('Ctrl Pts',(0.847345319999944,2.2,3.90793709299999));
#333418=CARTESIAN_POINT('Ctrl Pts',(0.847389178999944,12.2,3.90820446699998));
#333419=CARTESIAN_POINT('Ctrl Pts',(0.847389178999944,5.2,3.90820446699998));
#333420=CARTESIAN_POINT('Ctrl Pts',(0.847389178999944,2.2,3.90820446699998));
#333421=CARTESIAN_POINT('Ctrl Pts',(0.847433784999944,12.2,3.90847867499998));
#333422=CARTESIAN_POINT('Ctrl Pts',(0.847433784999944,5.2,3.90847867499998));
#333423=CARTESIAN_POINT('Ctrl Pts',(0.847433784999944,2.2,3.90847867499998));
#333424=CARTESIAN_POINT('Ctrl Pts',(0.847479116999944,12.2,3.90875970499999));
#333425=CARTESIAN_POINT('Ctrl Pts',(0.847479116999944,5.2,3.90875970499999));
#333426=CARTESIAN_POINT('Ctrl Pts',(0.847479116999944,2.2,3.90875970499999));
#333427=CARTESIAN_POINT('Ctrl Pts',(0.847525154999944,12.2,3.90904754499999));
#333428=CARTESIAN_POINT('Ctrl Pts',(0.847525154999944,5.2,3.90904754499999));
#333429=CARTESIAN_POINT('Ctrl Pts',(0.847525154999944,2.2,3.90904754499999));
#333430=CARTESIAN_POINT('Ctrl Pts',(0.847571879999944,12.2,3.90934218499999));
#333431=CARTESIAN_POINT('Ctrl Pts',(0.847571879999944,5.2,3.90934218499999));
#333432=CARTESIAN_POINT('Ctrl Pts',(0.847571879999944,2.2,3.90934218499999));
#333433=CARTESIAN_POINT('Ctrl Pts',(0.847619270999944,12.2,3.90964360999998));
#333434=CARTESIAN_POINT('Ctrl Pts',(0.847619270999944,5.2,3.90964360999998));
#333435=CARTESIAN_POINT('Ctrl Pts',(0.847619270999944,2.2,3.90964360999998));
#333436=CARTESIAN_POINT('Ctrl Pts',(0.847667308999944,12.2,3.90995180799998));
#333437=CARTESIAN_POINT('Ctrl Pts',(0.847667308999944,5.2,3.90995180799998));
#333438=CARTESIAN_POINT('Ctrl Pts',(0.847667308999944,2.2,3.90995180799998));
#333439=CARTESIAN_POINT('Ctrl Pts',(0.847715972999944,12.2,3.91026676999999));
#333440=CARTESIAN_POINT('Ctrl Pts',(0.847715972999944,5.2,3.91026676999999));
#333441=CARTESIAN_POINT('Ctrl Pts',(0.847715972999944,2.2,3.91026676999999));
#333442=CARTESIAN_POINT('Ctrl Pts',(0.847765243999944,12.2,3.91058847999999));
#333443=CARTESIAN_POINT('Ctrl Pts',(0.847765243999944,5.2,3.91058847999999));
#333444=CARTESIAN_POINT('Ctrl Pts',(0.847765243999944,2.2,3.91058847999999));
#333445=CARTESIAN_POINT('Ctrl Pts',(0.847815101999945,12.2,3.91091692899998));
#333446=CARTESIAN_POINT('Ctrl Pts',(0.847815101999945,5.2,3.91091692899998));
#333447=CARTESIAN_POINT('Ctrl Pts',(0.847815101999945,2.2,3.91091692899998));
#333448=CARTESIAN_POINT('Ctrl Pts',(0.847865527999944,12.2,3.91125210199998));
#333449=CARTESIAN_POINT('Ctrl Pts',(0.847865527999944,5.2,3.91125210199998));
#333450=CARTESIAN_POINT('Ctrl Pts',(0.847865527999944,2.2,3.91125210199998));
#333451=CARTESIAN_POINT('Ctrl Pts',(0.847916502999944,12.2,3.91159398899998));
#333452=CARTESIAN_POINT('Ctrl Pts',(0.847916502999944,5.2,3.91159398899998));
#333453=CARTESIAN_POINT('Ctrl Pts',(0.847916502999944,2.2,3.91159398899998));
#333454=CARTESIAN_POINT('Ctrl Pts',(0.847968007999944,12.2,3.91194257899999));
#333455=CARTESIAN_POINT('Ctrl Pts',(0.847968007999944,5.2,3.91194257899999));
#333456=CARTESIAN_POINT('Ctrl Pts',(0.847968007999944,2.2,3.91194257899999));
#333457=CARTESIAN_POINT('Ctrl Pts',(0.848020020999944,12.2,3.91229785699998));
#333458=CARTESIAN_POINT('Ctrl Pts',(0.848020020999944,5.2,3.91229785699998));
#333459=CARTESIAN_POINT('Ctrl Pts',(0.848020020999944,2.2,3.91229785699998));
#333460=CARTESIAN_POINT('Ctrl Pts',(0.848072523999944,12.2,3.91265981299998));
#333461=CARTESIAN_POINT('Ctrl Pts',(0.848072523999944,5.2,3.91265981299998));
#333462=CARTESIAN_POINT('Ctrl Pts',(0.848072523999944,2.2,3.91265981299998));
#333463=CARTESIAN_POINT('Ctrl Pts',(0.848125499999944,12.2,3.91302843499999));
#333464=CARTESIAN_POINT('Ctrl Pts',(0.848125499999944,5.2,3.91302843499999));
#333465=CARTESIAN_POINT('Ctrl Pts',(0.848125499999944,2.2,3.91302843499999));
#333466=CARTESIAN_POINT('Ctrl Pts',(0.848178926999944,12.2,3.91340370999998));
#333467=CARTESIAN_POINT('Ctrl Pts',(0.848178926999944,5.2,3.91340370999998));
#333468=CARTESIAN_POINT('Ctrl Pts',(0.848178926999944,2.2,3.91340370999998));
#333469=CARTESIAN_POINT('Ctrl Pts',(0.848232787999944,12.2,3.91378562799999));
#333470=CARTESIAN_POINT('Ctrl Pts',(0.848232787999944,5.2,3.91378562799999));
#333471=CARTESIAN_POINT('Ctrl Pts',(0.848232787999944,2.2,3.91378562799999));
#333472=CARTESIAN_POINT('Ctrl Pts',(0.848287061999944,12.2,3.91417417499999));
#333473=CARTESIAN_POINT('Ctrl Pts',(0.848287061999944,5.2,3.91417417499999));
#333474=CARTESIAN_POINT('Ctrl Pts',(0.848287061999944,2.2,3.91417417499999));
#333475=CARTESIAN_POINT('Ctrl Pts',(0.848341732999944,12.2,3.91456933999999));
#333476=CARTESIAN_POINT('Ctrl Pts',(0.848341732999944,5.2,3.91456933999999));
#333477=CARTESIAN_POINT('Ctrl Pts',(0.848341732999944,2.2,3.91456933999999));
#333478=CARTESIAN_POINT('Ctrl Pts',(0.848396778999944,12.2,3.91497111199998));
#333479=CARTESIAN_POINT('Ctrl Pts',(0.848396778999944,5.2,3.91497111199998));
#333480=CARTESIAN_POINT('Ctrl Pts',(0.848396778999944,2.2,3.91497111199998));
#333481=CARTESIAN_POINT('Ctrl Pts',(0.848452184999945,12.2,3.91537947699998));
#333482=CARTESIAN_POINT('Ctrl Pts',(0.848452184999945,5.2,3.91537947699998));
#333483=CARTESIAN_POINT('Ctrl Pts',(0.848452184999945,2.2,3.91537947699998));
#333484=CARTESIAN_POINT('Ctrl Pts',(0.848507928999944,12.2,3.91579442499999));
#333485=CARTESIAN_POINT('Ctrl Pts',(0.848507928999944,5.2,3.91579442499999));
#333486=CARTESIAN_POINT('Ctrl Pts',(0.848507928999944,2.2,3.91579442499999));
#333487=CARTESIAN_POINT('Ctrl Pts',(0.848563993999945,12.2,3.91621594399999));
#333488=CARTESIAN_POINT('Ctrl Pts',(0.848563993999945,5.2,3.91621594399999));
#333489=CARTESIAN_POINT('Ctrl Pts',(0.848563993999945,2.2,3.91621594399999));
#333490=CARTESIAN_POINT('Ctrl Pts',(0.848620361999944,12.2,3.91664402199999));
#333491=CARTESIAN_POINT('Ctrl Pts',(0.848620361999944,5.2,3.91664402199999));
#333492=CARTESIAN_POINT('Ctrl Pts',(0.848620361999944,2.2,3.91664402199999));
#333493=CARTESIAN_POINT('Ctrl Pts',(0.848677012999944,12.2,3.91707864699999));
#333494=CARTESIAN_POINT('Ctrl Pts',(0.848677012999944,5.2,3.91707864699999));
#333495=CARTESIAN_POINT('Ctrl Pts',(0.848677012999944,2.2,3.91707864699999));
#333496=CARTESIAN_POINT('Ctrl Pts',(0.848733929999944,12.2,3.91751980599999));
#333497=CARTESIAN_POINT('Ctrl Pts',(0.848733929999944,5.2,3.91751980599999));
#333498=CARTESIAN_POINT('Ctrl Pts',(0.848733929999944,2.2,3.91751980599999));
#333499=CARTESIAN_POINT('Ctrl Pts',(0.848791094999944,12.2,3.91796748999998));
#333500=CARTESIAN_POINT('Ctrl Pts',(0.848791094999944,5.2,3.91796748999998));
#333501=CARTESIAN_POINT('Ctrl Pts',(0.848791094999944,2.2,3.91796748999998));
#333502=CARTESIAN_POINT('Ctrl Pts',(0.848848487999944,12.2,3.91842168499998));
#333503=CARTESIAN_POINT('Ctrl Pts',(0.848848487999944,5.2,3.91842168499998));
#333504=CARTESIAN_POINT('Ctrl Pts',(0.848848487999944,2.2,3.91842168499998));
#333505=CARTESIAN_POINT('Ctrl Pts',(0.848906091999945,12.2,3.91888237999999));
#333506=CARTESIAN_POINT('Ctrl Pts',(0.848906091999945,5.2,3.91888237999999));
#333507=CARTESIAN_POINT('Ctrl Pts',(0.848906091999945,2.2,3.91888237999999));
#333508=CARTESIAN_POINT('Ctrl Pts',(0.848963890999944,12.2,3.91934956299998));
#333509=CARTESIAN_POINT('Ctrl Pts',(0.848963890999944,5.2,3.91934956299998));
#333510=CARTESIAN_POINT('Ctrl Pts',(0.848963890999944,2.2,3.91934956299998));
#333511=CARTESIAN_POINT('Ctrl Pts',(0.849021862999945,12.2,3.91982322299998));
#333512=CARTESIAN_POINT('Ctrl Pts',(0.849021862999945,5.2,3.91982322299998));
#333513=CARTESIAN_POINT('Ctrl Pts',(0.849021862999945,2.2,3.91982322299998));
#333514=CARTESIAN_POINT('Ctrl Pts',(0.849079992999945,12.2,3.92030334899999));
#333515=CARTESIAN_POINT('Ctrl Pts',(0.849079992999945,5.2,3.92030334899999));
#333516=CARTESIAN_POINT('Ctrl Pts',(0.849079992999945,2.2,3.92030334899999));
#333517=CARTESIAN_POINT('Ctrl Pts',(0.849138261999944,12.2,3.92078992799998));
#333518=CARTESIAN_POINT('Ctrl Pts',(0.849138261999944,5.2,3.92078992799998));
#333519=CARTESIAN_POINT('Ctrl Pts',(0.849138261999944,2.2,3.92078992799998));
#333520=CARTESIAN_POINT('Ctrl Pts',(0.849196652999944,12.2,3.92128294799999));
#333521=CARTESIAN_POINT('Ctrl Pts',(0.849196652999944,5.2,3.92128294799999));
#333522=CARTESIAN_POINT('Ctrl Pts',(0.849196652999944,2.2,3.92128294799999));
#333523=CARTESIAN_POINT('Ctrl Pts',(0.849255145999944,12.2,3.92178239799998));
#333524=CARTESIAN_POINT('Ctrl Pts',(0.849255145999944,5.2,3.92178239799998));
#333525=CARTESIAN_POINT('Ctrl Pts',(0.849255145999944,2.2,3.92178239799998));
#333526=CARTESIAN_POINT('Ctrl Pts',(0.849313727999944,12.2,3.92228826699998));
#333527=CARTESIAN_POINT('Ctrl Pts',(0.849313727999944,5.2,3.92228826699998));
#333528=CARTESIAN_POINT('Ctrl Pts',(0.849313727999944,2.2,3.92228826699998));
#333529=CARTESIAN_POINT('Ctrl Pts',(0.849372375999944,12.2,3.92280054199999));
#333530=CARTESIAN_POINT('Ctrl Pts',(0.849372375999944,5.2,3.92280054199999));
#333531=CARTESIAN_POINT('Ctrl Pts',(0.849372375999944,2.2,3.92280054199999));
#333532=CARTESIAN_POINT('Ctrl Pts',(0.849431077999945,12.2,3.92331921299998));
#333533=CARTESIAN_POINT('Ctrl Pts',(0.849431077999945,5.2,3.92331921299998));
#333534=CARTESIAN_POINT('Ctrl Pts',(0.849431077999945,2.2,3.92331921299998));
#333535=CARTESIAN_POINT('Ctrl Pts',(0.849489810999944,12.2,3.92384426799998));
#333536=CARTESIAN_POINT('Ctrl Pts',(0.849489810999944,5.2,3.92384426799998));
#333537=CARTESIAN_POINT('Ctrl Pts',(0.849489810999944,2.2,3.92384426799998));
#333538=CARTESIAN_POINT('Ctrl Pts',(0.849548561999944,12.2,3.92437569399998));
#333539=CARTESIAN_POINT('Ctrl Pts',(0.849548561999944,5.2,3.92437569399998));
#333540=CARTESIAN_POINT('Ctrl Pts',(0.849548561999944,2.2,3.92437569399998));
#333541=CARTESIAN_POINT('Ctrl Pts',(0.849607310999944,12.2,3.92491348299998));
#333542=CARTESIAN_POINT('Ctrl Pts',(0.849607310999944,5.2,3.92491348299998));
#333543=CARTESIAN_POINT('Ctrl Pts',(0.849607310999944,2.2,3.92491348299998));
#333544=CARTESIAN_POINT('Ctrl Pts',(0.849666042999945,12.2,3.92545761799998));
#333545=CARTESIAN_POINT('Ctrl Pts',(0.849666042999945,5.2,3.92545761799998));
#333546=CARTESIAN_POINT('Ctrl Pts',(0.849666042999945,2.2,3.92545761799998));
#333547=CARTESIAN_POINT('Ctrl Pts',(0.849724738999944,12.2,3.92600809299999));
#333548=CARTESIAN_POINT('Ctrl Pts',(0.849724738999944,5.2,3.92600809299999));
#333549=CARTESIAN_POINT('Ctrl Pts',(0.849724738999944,2.2,3.92600809299999));
#333550=CARTESIAN_POINT('Ctrl Pts',(0.849783383999945,12.2,3.92656489399998));
#333551=CARTESIAN_POINT('Ctrl Pts',(0.849783383999945,5.2,3.92656489399998));
#333552=CARTESIAN_POINT('Ctrl Pts',(0.849783383999945,2.2,3.92656489399998));
#333553=CARTESIAN_POINT('Ctrl Pts',(0.849841957999944,12.2,3.92712800899999));
#333554=CARTESIAN_POINT('Ctrl Pts',(0.849841957999944,5.2,3.92712800899999));
#333555=CARTESIAN_POINT('Ctrl Pts',(0.849841957999944,2.2,3.92712800899999));
#333556=CARTESIAN_POINT('Ctrl Pts',(0.849900445999944,12.2,3.92769742699999));
#333557=CARTESIAN_POINT('Ctrl Pts',(0.849900445999944,5.2,3.92769742699999));
#333558=CARTESIAN_POINT('Ctrl Pts',(0.849900445999944,2.2,3.92769742699999));
#333559=CARTESIAN_POINT('Ctrl Pts',(0.849958830999944,12.2,3.92827313699998));
#333560=CARTESIAN_POINT('Ctrl Pts',(0.849958830999944,5.2,3.92827313699998));
#333561=CARTESIAN_POINT('Ctrl Pts',(0.849958830999944,2.2,3.92827313699998));
#333562=CARTESIAN_POINT('Ctrl Pts',(0.850017095999944,12.2,3.92885512799998));
#333563=CARTESIAN_POINT('Ctrl Pts',(0.850017095999944,5.2,3.92885512799998));
#333564=CARTESIAN_POINT('Ctrl Pts',(0.850017095999944,2.2,3.92885512799998));
#333565=CARTESIAN_POINT('Ctrl Pts',(0.850075223999944,12.2,3.92944338699999));
#333566=CARTESIAN_POINT('Ctrl Pts',(0.850075223999944,5.2,3.92944338699999));
#333567=CARTESIAN_POINT('Ctrl Pts',(0.850075223999944,2.2,3.92944338699999));
#333568=CARTESIAN_POINT('Ctrl Pts',(0.850133198999944,12.2,3.93003790399998));
#333569=CARTESIAN_POINT('Ctrl Pts',(0.850133198999944,5.2,3.93003790399998));
#333570=CARTESIAN_POINT('Ctrl Pts',(0.850133198999944,2.2,3.93003790399998));
#333571=CARTESIAN_POINT('Ctrl Pts',(0.850191003999944,12.2,3.93063866799999));
#333572=CARTESIAN_POINT('Ctrl Pts',(0.850191003999944,5.2,3.93063866799999));
#333573=CARTESIAN_POINT('Ctrl Pts',(0.850191003999944,2.2,3.93063866799999));
#333574=CARTESIAN_POINT('Ctrl Pts',(0.850248621999944,12.2,3.93124566599998));
#333575=CARTESIAN_POINT('Ctrl Pts',(0.850248621999944,5.2,3.93124566599998));
#333576=CARTESIAN_POINT('Ctrl Pts',(0.850248621999944,2.2,3.93124566599998));
#333577=CARTESIAN_POINT('Ctrl Pts',(0.850306036999945,12.2,3.93185888699998));
#333578=CARTESIAN_POINT('Ctrl Pts',(0.850306036999945,5.2,3.93185888699998));
#333579=CARTESIAN_POINT('Ctrl Pts',(0.850306036999945,2.2,3.93185888699998));
#333580=CARTESIAN_POINT('Ctrl Pts',(0.850363230999944,12.2,3.93247832099998));
#333581=CARTESIAN_POINT('Ctrl Pts',(0.850363230999944,5.2,3.93247832099998));
#333582=CARTESIAN_POINT('Ctrl Pts',(0.850363230999944,2.2,3.93247832099998));
#333583=CARTESIAN_POINT('Ctrl Pts',(0.850420188999944,12.2,3.93310395499999));
#333584=CARTESIAN_POINT('Ctrl Pts',(0.850420188999944,5.2,3.93310395499999));
#333585=CARTESIAN_POINT('Ctrl Pts',(0.850420188999944,2.2,3.93310395499999));
#333586=CARTESIAN_POINT('Ctrl Pts',(0.850476895999944,12.2,3.93373577899998));
#333587=CARTESIAN_POINT('Ctrl Pts',(0.850476895999944,5.2,3.93373577899998));
#333588=CARTESIAN_POINT('Ctrl Pts',(0.850476895999944,2.2,3.93373577899998));
#333589=CARTESIAN_POINT('Ctrl Pts',(0.850533333999944,12.2,3.93437378099998));
#333590=CARTESIAN_POINT('Ctrl Pts',(0.850533333999944,5.2,3.93437378099998));
#333591=CARTESIAN_POINT('Ctrl Pts',(0.850533333999944,2.2,3.93437378099998));
#333592=CARTESIAN_POINT('Ctrl Pts',(0.850589486999944,12.2,3.93501794899999));
#333593=CARTESIAN_POINT('Ctrl Pts',(0.850589486999944,5.2,3.93501794899999));
#333594=CARTESIAN_POINT('Ctrl Pts',(0.850589486999944,2.2,3.93501794899999));
#333595=CARTESIAN_POINT('Ctrl Pts',(0.850645338999944,12.2,3.93566827399999));
#333596=CARTESIAN_POINT('Ctrl Pts',(0.850645338999944,5.2,3.93566827399999));
#333597=CARTESIAN_POINT('Ctrl Pts',(0.850645338999944,2.2,3.93566827399999));
#333598=CARTESIAN_POINT('Ctrl Pts',(0.850700872999944,12.2,3.93632474299999));
#333599=CARTESIAN_POINT('Ctrl Pts',(0.850700872999944,5.2,3.93632474299999));
#333600=CARTESIAN_POINT('Ctrl Pts',(0.850700872999944,2.2,3.93632474299999));
#333601=CARTESIAN_POINT('Ctrl Pts',(0.850756075999944,12.2,3.93698734399998));
#333602=CARTESIAN_POINT('Ctrl Pts',(0.850756075999944,5.2,3.93698734399998));
#333603=CARTESIAN_POINT('Ctrl Pts',(0.850756075999944,2.2,3.93698734399998));
#333604=CARTESIAN_POINT('Ctrl Pts',(0.850810928999944,12.2,3.93765606799998));
#333605=CARTESIAN_POINT('Ctrl Pts',(0.850810928999944,5.2,3.93765606799998));
#333606=CARTESIAN_POINT('Ctrl Pts',(0.850810928999944,2.2,3.93765606799998));
#333607=CARTESIAN_POINT('Ctrl Pts',(0.850865416999944,12.2,3.93833090199998));
#333608=CARTESIAN_POINT('Ctrl Pts',(0.850865416999944,5.2,3.93833090199998));
#333609=CARTESIAN_POINT('Ctrl Pts',(0.850865416999944,2.2,3.93833090199998));
#333610=CARTESIAN_POINT('Ctrl Pts',(0.850919522999944,12.2,3.93901183599999));
#333611=CARTESIAN_POINT('Ctrl Pts',(0.850919522999944,5.2,3.93901183599999));
#333612=CARTESIAN_POINT('Ctrl Pts',(0.850919522999944,2.2,3.93901183599999));
#333613=CARTESIAN_POINT('Ctrl Pts',(0.850973233999944,12.2,3.93969885899998));
#333614=CARTESIAN_POINT('Ctrl Pts',(0.850973233999944,5.2,3.93969885899998));
#333615=CARTESIAN_POINT('Ctrl Pts',(0.850973233999944,2.2,3.93969885899998));
#333616=CARTESIAN_POINT('Ctrl Pts',(0.851026531999944,12.2,3.94039195799999));
#333617=CARTESIAN_POINT('Ctrl Pts',(0.851026531999944,5.2,3.94039195799999));
#333618=CARTESIAN_POINT('Ctrl Pts',(0.851026531999944,2.2,3.94039195799999));
#333619=CARTESIAN_POINT('Ctrl Pts',(0.851079402999945,12.2,3.94109112299999));
#333620=CARTESIAN_POINT('Ctrl Pts',(0.851079402999945,5.2,3.94109112299999));
#333621=CARTESIAN_POINT('Ctrl Pts',(0.851079402999945,2.2,3.94109112299999));
#333622=CARTESIAN_POINT('Ctrl Pts',(0.851131829999944,12.2,3.94179634299999));
#333623=CARTESIAN_POINT('Ctrl Pts',(0.851131829999944,5.2,3.94179634299999));
#333624=CARTESIAN_POINT('Ctrl Pts',(0.851131829999944,2.2,3.94179634299999));
#333625=CARTESIAN_POINT('Ctrl Pts',(0.851183796999945,12.2,3.94250760599999));
#333626=CARTESIAN_POINT('Ctrl Pts',(0.851183796999945,5.2,3.94250760599999));
#333627=CARTESIAN_POINT('Ctrl Pts',(0.851183796999945,2.2,3.94250760599999));
#333628=CARTESIAN_POINT('Ctrl Pts',(0.851235289999944,12.2,3.94322490199999));
#333629=CARTESIAN_POINT('Ctrl Pts',(0.851235289999944,5.2,3.94322490199999));
#333630=CARTESIAN_POINT('Ctrl Pts',(0.851235289999944,2.2,3.94322490199999));
#333631=CARTESIAN_POINT('Ctrl Pts',(0.851286293999944,12.2,3.94394821999998));
#333632=CARTESIAN_POINT('Ctrl Pts',(0.851286293999944,5.2,3.94394821999998));
#333633=CARTESIAN_POINT('Ctrl Pts',(0.851286293999944,2.2,3.94394821999998));
#333634=CARTESIAN_POINT('Ctrl Pts',(0.851336790999944,12.2,3.94467754799999));
#333635=CARTESIAN_POINT('Ctrl Pts',(0.851336790999944,5.2,3.94467754799999));
#333636=CARTESIAN_POINT('Ctrl Pts',(0.851336790999944,2.2,3.94467754799999));
#333637=CARTESIAN_POINT('Ctrl Pts',(0.851386768999944,12.2,3.94541287499998));
#333638=CARTESIAN_POINT('Ctrl Pts',(0.851386768999944,5.2,3.94541287499998));
#333639=CARTESIAN_POINT('Ctrl Pts',(0.851386768999944,2.2,3.94541287499998));
#333640=CARTESIAN_POINT('Ctrl Pts',(0.851436209999944,12.2,3.94615418899999));
#333641=CARTESIAN_POINT('Ctrl Pts',(0.851436209999944,5.2,3.94615418899999));
#333642=CARTESIAN_POINT('Ctrl Pts',(0.851436209999944,2.2,3.94615418899999));
#333643=CARTESIAN_POINT('Ctrl Pts',(0.851485099999943,12.2,3.94690148199999));
#333644=CARTESIAN_POINT('Ctrl Pts',(0.851485099999943,5.2,3.94690148199999));
#333645=CARTESIAN_POINT('Ctrl Pts',(0.851485099999943,2.2,3.94690148199999));
#333646=CARTESIAN_POINT('Ctrl Pts',(0.851533423999945,12.2,3.94765473999998));
#333647=CARTESIAN_POINT('Ctrl Pts',(0.851533423999945,5.2,3.94765473999998));
#333648=CARTESIAN_POINT('Ctrl Pts',(0.851533423999945,2.2,3.94765473999998));
#333649=CARTESIAN_POINT('Ctrl Pts',(0.851581165999944,12.2,3.94841395299999));
#333650=CARTESIAN_POINT('Ctrl Pts',(0.851581165999944,5.2,3.94841395299999));
#333651=CARTESIAN_POINT('Ctrl Pts',(0.851581165999944,2.2,3.94841395299999));
#333652=CARTESIAN_POINT('Ctrl Pts',(0.851628312999945,12.2,3.94917910899999));
#333653=CARTESIAN_POINT('Ctrl Pts',(0.851628312999945,5.2,3.94917910899999));
#333654=CARTESIAN_POINT('Ctrl Pts',(0.851628312999945,2.2,3.94917910899999));
#333655=CARTESIAN_POINT('Ctrl Pts',(0.851674847999945,12.2,3.94995019899999));
#333656=CARTESIAN_POINT('Ctrl Pts',(0.851674847999945,5.2,3.94995019899999));
#333657=CARTESIAN_POINT('Ctrl Pts',(0.851674847999945,2.2,3.94995019899999));
#333658=CARTESIAN_POINT('Ctrl Pts',(0.851720754999944,12.2,3.95072721099999));
#333659=CARTESIAN_POINT('Ctrl Pts',(0.851720754999944,5.2,3.95072721099999));
#333660=CARTESIAN_POINT('Ctrl Pts',(0.851720754999944,2.2,3.95072721099999));
#333661=CARTESIAN_POINT('Ctrl Pts',(0.851766022999944,12.2,3.95151013399998));
#333662=CARTESIAN_POINT('Ctrl Pts',(0.851766022999944,5.2,3.95151013399998));
#333663=CARTESIAN_POINT('Ctrl Pts',(0.851766022999944,2.2,3.95151013399998));
#333664=CARTESIAN_POINT('Ctrl Pts',(0.851810633999944,12.2,3.95229895699998));
#333665=CARTESIAN_POINT('Ctrl Pts',(0.851810633999944,5.2,3.95229895699998));
#333666=CARTESIAN_POINT('Ctrl Pts',(0.851810633999944,2.2,3.95229895699998));
#333667=CARTESIAN_POINT('Ctrl Pts',(0.851854574999944,12.2,3.95309366899999));
#333668=CARTESIAN_POINT('Ctrl Pts',(0.851854574999944,5.2,3.95309366899999));
#333669=CARTESIAN_POINT('Ctrl Pts',(0.851854574999944,2.2,3.95309366899999));
#333670=CARTESIAN_POINT('Ctrl Pts',(0.851897829999944,12.2,3.95389425899998));
#333671=CARTESIAN_POINT('Ctrl Pts',(0.851897829999944,5.2,3.95389425899998));
#333672=CARTESIAN_POINT('Ctrl Pts',(0.851897829999944,2.2,3.95389425899998));
#333673=CARTESIAN_POINT('Ctrl Pts',(0.851940384999944,12.2,3.95470071599998));
#333674=CARTESIAN_POINT('Ctrl Pts',(0.851940384999944,5.2,3.95470071599998));
#333675=CARTESIAN_POINT('Ctrl Pts',(0.851940384999944,2.2,3.95470071599998));
#333676=CARTESIAN_POINT('Ctrl Pts',(0.851982225999944,12.2,3.95551302999999));
#333677=CARTESIAN_POINT('Ctrl Pts',(0.851982225999944,5.2,3.95551302999999));
#333678=CARTESIAN_POINT('Ctrl Pts',(0.851982225999944,2.2,3.95551302999999));
#333679=CARTESIAN_POINT('Ctrl Pts',(0.852023336999944,12.2,3.95633118699998));
#333680=CARTESIAN_POINT('Ctrl Pts',(0.852023336999944,5.2,3.95633118699998));
#333681=CARTESIAN_POINT('Ctrl Pts',(0.852023336999944,2.2,3.95633118699998));
#333682=CARTESIAN_POINT('Ctrl Pts',(0.852063703999945,12.2,3.95715518099998));
#333683=CARTESIAN_POINT('Ctrl Pts',(0.852063703999945,5.2,3.95715518099998));
#333684=CARTESIAN_POINT('Ctrl Pts',(0.852063703999945,2.2,3.95715518099998));
#333685=CARTESIAN_POINT('Ctrl Pts',(0.852103313999945,12.2,3.95798499699998));
#333686=CARTESIAN_POINT('Ctrl Pts',(0.852103313999945,5.2,3.95798499699998));
#333687=CARTESIAN_POINT('Ctrl Pts',(0.852103313999945,2.2,3.95798499699998));
#333688=CARTESIAN_POINT('Ctrl Pts',(0.852142149999944,12.2,3.95882062599998));
#333689=CARTESIAN_POINT('Ctrl Pts',(0.852142149999944,5.2,3.95882062599998));
#333690=CARTESIAN_POINT('Ctrl Pts',(0.852142149999944,2.2,3.95882062599998));
#333691=CARTESIAN_POINT('Ctrl Pts',(0.852180199999945,12.2,3.95966205699998));
#333692=CARTESIAN_POINT('Ctrl Pts',(0.852180199999945,5.2,3.95966205699998));
#333693=CARTESIAN_POINT('Ctrl Pts',(0.852180199999945,2.2,3.95966205699998));
#333694=CARTESIAN_POINT('Ctrl Pts',(0.852217448999945,12.2,3.96050927799998));
#333695=CARTESIAN_POINT('Ctrl Pts',(0.852217448999945,5.2,3.96050927799998));
#333696=CARTESIAN_POINT('Ctrl Pts',(0.852217448999945,2.2,3.96050927799998));
#333697=CARTESIAN_POINT('Ctrl Pts',(0.852253881999945,12.2,3.96136228099999));
#333698=CARTESIAN_POINT('Ctrl Pts',(0.852253881999945,5.2,3.96136228099999));
#333699=CARTESIAN_POINT('Ctrl Pts',(0.852253881999945,2.2,3.96136228099999));
#333700=CARTESIAN_POINT('Ctrl Pts',(0.852289485999944,12.2,3.96222105099999));
#333701=CARTESIAN_POINT('Ctrl Pts',(0.852289485999944,5.2,3.96222105099999));
#333702=CARTESIAN_POINT('Ctrl Pts',(0.852289485999944,2.2,3.96222105099999));
#333703=CARTESIAN_POINT('Ctrl Pts',(0.852324245999945,12.2,3.96308557999999));
#333704=CARTESIAN_POINT('Ctrl Pts',(0.852324245999945,5.2,3.96308557999999));
#333705=CARTESIAN_POINT('Ctrl Pts',(0.852324245999945,2.2,3.96308557999999));
#333706=CARTESIAN_POINT('Ctrl Pts',(0.852358147999944,12.2,3.96395585799999));
#333707=CARTESIAN_POINT('Ctrl Pts',(0.852358147999944,5.2,3.96395585799999));
#333708=CARTESIAN_POINT('Ctrl Pts',(0.852358147999944,2.2,3.96395585799999));
#333709=CARTESIAN_POINT('Ctrl Pts',(0.852391178999944,12.2,3.96483187099999));
#333710=CARTESIAN_POINT('Ctrl Pts',(0.852391178999944,5.2,3.96483187099999));
#333711=CARTESIAN_POINT('Ctrl Pts',(0.852391178999944,2.2,3.96483187099999));
#333712=CARTESIAN_POINT('Ctrl Pts',(0.852423323999945,12.2,3.96571361099999));
#333713=CARTESIAN_POINT('Ctrl Pts',(0.852423323999945,5.2,3.96571361099999));
#333714=CARTESIAN_POINT('Ctrl Pts',(0.852423323999945,2.2,3.96571361099999));
#333715=CARTESIAN_POINT('Ctrl Pts',(0.852454568999944,12.2,3.96660106599998));
#333716=CARTESIAN_POINT('Ctrl Pts',(0.852454568999944,5.2,3.96660106599998));
#333717=CARTESIAN_POINT('Ctrl Pts',(0.852454568999944,2.2,3.96660106599998));
#333718=CARTESIAN_POINT('Ctrl Pts',(0.852484900999944,12.2,3.96749422499998));
#333719=CARTESIAN_POINT('Ctrl Pts',(0.852484900999944,5.2,3.96749422499998));
#333720=CARTESIAN_POINT('Ctrl Pts',(0.852484900999944,2.2,3.96749422499998));
#333721=CARTESIAN_POINT('Ctrl Pts',(0.852514304999944,12.2,3.96839307799999));
#333722=CARTESIAN_POINT('Ctrl Pts',(0.852514304999944,5.2,3.96839307799999));
#333723=CARTESIAN_POINT('Ctrl Pts',(0.852514304999944,2.2,3.96839307799999));
#333724=CARTESIAN_POINT('Ctrl Pts',(0.852542767999944,12.2,3.96929761499998));
#333725=CARTESIAN_POINT('Ctrl Pts',(0.852542767999944,5.2,3.96929761499998));
#333726=CARTESIAN_POINT('Ctrl Pts',(0.852542767999944,2.2,3.96929761499998));
#333727=CARTESIAN_POINT('Ctrl Pts',(0.852570275999944,12.2,3.97020782199998));
#333728=CARTESIAN_POINT('Ctrl Pts',(0.852570275999944,5.2,3.97020782199998));
#333729=CARTESIAN_POINT('Ctrl Pts',(0.852570275999944,2.2,3.97020782199998));
#333730=CARTESIAN_POINT('Ctrl Pts',(0.852596815999944,12.2,3.97112369199998));
#333731=CARTESIAN_POINT('Ctrl Pts',(0.852596815999944,5.2,3.97112369199998));
#333732=CARTESIAN_POINT('Ctrl Pts',(0.852596815999944,2.2,3.97112369199998));
#333733=CARTESIAN_POINT('Ctrl Pts',(0.852622373999944,12.2,3.97204521299999));
#333734=CARTESIAN_POINT('Ctrl Pts',(0.852622373999944,5.2,3.97204521299999));
#333735=CARTESIAN_POINT('Ctrl Pts',(0.852622373999944,2.2,3.97204521299999));
#333736=CARTESIAN_POINT('Ctrl Pts',(0.852646935999944,12.2,3.97297237299998));
#333737=CARTESIAN_POINT('Ctrl Pts',(0.852646935999944,5.2,3.97297237299998));
#333738=CARTESIAN_POINT('Ctrl Pts',(0.852646935999944,2.2,3.97297237299998));
#333739=CARTESIAN_POINT('Ctrl Pts',(0.852670487999945,12.2,3.97390516399999));
#333740=CARTESIAN_POINT('Ctrl Pts',(0.852670487999945,5.2,3.97390516399999));
#333741=CARTESIAN_POINT('Ctrl Pts',(0.852670487999945,2.2,3.97390516399999));
#333742=CARTESIAN_POINT('Ctrl Pts',(0.852693017999945,12.2,3.97484357199998));
#333743=CARTESIAN_POINT('Ctrl Pts',(0.852693017999945,5.2,3.97484357199998));
#333744=CARTESIAN_POINT('Ctrl Pts',(0.852693017999945,2.2,3.97484357199998));
#333745=CARTESIAN_POINT('Ctrl Pts',(0.852714510999945,12.2,3.97578758899999));
#333746=CARTESIAN_POINT('Ctrl Pts',(0.852714510999945,5.2,3.97578758899999));
#333747=CARTESIAN_POINT('Ctrl Pts',(0.852714510999945,2.2,3.97578758899999));
#333748=CARTESIAN_POINT('Ctrl Pts',(0.852734954999944,12.2,3.97673720299998));
#333749=CARTESIAN_POINT('Ctrl Pts',(0.852734954999944,5.2,3.97673720299998));
#333750=CARTESIAN_POINT('Ctrl Pts',(0.852734954999944,2.2,3.97673720299998));
#333751=CARTESIAN_POINT('Ctrl Pts',(0.852754335999945,12.2,3.97769240399998));
#333752=CARTESIAN_POINT('Ctrl Pts',(0.852754335999945,5.2,3.97769240399998));
#333753=CARTESIAN_POINT('Ctrl Pts',(0.852754335999945,2.2,3.97769240399998));
#333754=CARTESIAN_POINT('Ctrl Pts',(0.852772641999944,12.2,3.97865318099999));
#333755=CARTESIAN_POINT('Ctrl Pts',(0.852772641999944,5.2,3.97865318099999));
#333756=CARTESIAN_POINT('Ctrl Pts',(0.852772641999944,2.2,3.97865318099999));
#333757=CARTESIAN_POINT('Ctrl Pts',(0.852789856999945,12.2,3.97961952299998));
#333758=CARTESIAN_POINT('Ctrl Pts',(0.852789856999945,5.2,3.97961952299998));
#333759=CARTESIAN_POINT('Ctrl Pts',(0.852789856999945,2.2,3.97961952299998));
#333760=CARTESIAN_POINT('Ctrl Pts',(0.852805969999944,12.2,3.98059142099999));
#333761=CARTESIAN_POINT('Ctrl Pts',(0.852805969999944,5.2,3.98059142099999));
#333762=CARTESIAN_POINT('Ctrl Pts',(0.852805969999944,2.2,3.98059142099999));
#333763=CARTESIAN_POINT('Ctrl Pts',(0.852820967999944,12.2,3.98156886199998));
#333764=CARTESIAN_POINT('Ctrl Pts',(0.852820967999944,5.2,3.98156886199998));
#333765=CARTESIAN_POINT('Ctrl Pts',(0.852820967999944,2.2,3.98156886199998));
#333766=CARTESIAN_POINT('Ctrl Pts',(0.852834834999944,12.2,3.98255183799999));
#333767=CARTESIAN_POINT('Ctrl Pts',(0.852834834999944,5.2,3.98255183799999));
#333768=CARTESIAN_POINT('Ctrl Pts',(0.852834834999944,2.2,3.98255183799999));
#333769=CARTESIAN_POINT('Ctrl Pts',(0.852847561999944,12.2,3.98354033699999));
#333770=CARTESIAN_POINT('Ctrl Pts',(0.852847561999944,5.2,3.98354033699999));
#333771=CARTESIAN_POINT('Ctrl Pts',(0.852847561999944,2.2,3.98354033699999));
#333772=CARTESIAN_POINT('Ctrl Pts',(0.852859133999945,12.2,3.98453434699999));
#333773=CARTESIAN_POINT('Ctrl Pts',(0.852859133999945,5.2,3.98453434699999));
#333774=CARTESIAN_POINT('Ctrl Pts',(0.852859133999945,2.2,3.98453434699999));
#333775=CARTESIAN_POINT('Ctrl Pts',(0.852869537999944,12.2,3.98553385999998));
#333776=CARTESIAN_POINT('Ctrl Pts',(0.852869537999944,5.2,3.98553385999998));
#333777=CARTESIAN_POINT('Ctrl Pts',(0.852869537999944,2.2,3.98553385999998));
#333778=CARTESIAN_POINT('Ctrl Pts',(0.852878760999943,12.2,3.98653886499999));
#333779=CARTESIAN_POINT('Ctrl Pts',(0.852878760999943,5.2,3.98653886499999));
#333780=CARTESIAN_POINT('Ctrl Pts',(0.852878760999943,2.2,3.98653886499999));
#333781=CARTESIAN_POINT('Ctrl Pts',(0.852886789999945,12.2,3.98754934899999));
#333782=CARTESIAN_POINT('Ctrl Pts',(0.852886789999945,5.2,3.98754934899999));
#333783=CARTESIAN_POINT('Ctrl Pts',(0.852886789999945,2.2,3.98754934899999));
#333784=CARTESIAN_POINT('Ctrl Pts',(0.852893612999944,12.2,3.98856530599998));
#333785=CARTESIAN_POINT('Ctrl Pts',(0.852893612999944,5.2,3.98856530599998));
#333786=CARTESIAN_POINT('Ctrl Pts',(0.852893612999944,2.2,3.98856530599998));
#333787=CARTESIAN_POINT('Ctrl Pts',(0.852899216999944,12.2,3.98958671999999));
#333788=CARTESIAN_POINT('Ctrl Pts',(0.852899216999944,5.2,3.98958671999999));
#333789=CARTESIAN_POINT('Ctrl Pts',(0.852899216999944,2.2,3.98958671999999));
#333790=CARTESIAN_POINT('Ctrl Pts',(0.852903588999945,12.2,3.99061358499999));
#333791=CARTESIAN_POINT('Ctrl Pts',(0.852903588999945,5.2,3.99061358499999));
#333792=CARTESIAN_POINT('Ctrl Pts',(0.852903588999945,2.2,3.99061358499999));
#333793=CARTESIAN_POINT('Ctrl Pts',(0.852906715999944,12.2,3.99164588899998));
#333794=CARTESIAN_POINT('Ctrl Pts',(0.852906715999944,5.2,3.99164588899998));
#333795=CARTESIAN_POINT('Ctrl Pts',(0.852906715999944,2.2,3.99164588899998));
#333796=CARTESIAN_POINT('Ctrl Pts',(0.852908584999944,12.2,3.99268361999999));
#333797=CARTESIAN_POINT('Ctrl Pts',(0.852908584999944,5.2,3.99268361999999));
#333798=CARTESIAN_POINT('Ctrl Pts',(0.852908584999944,2.2,3.99268361999999));
#333799=CARTESIAN_POINT('Ctrl Pts',(0.852909184999944,12.2,3.99372676999998));
#333800=CARTESIAN_POINT('Ctrl Pts',(0.852909184999944,5.2,3.99372676999998));
#333801=CARTESIAN_POINT('Ctrl Pts',(0.852909184999944,2.2,3.99372676999998));
#333802=CARTESIAN_POINT('Ctrl Pts',(0.852908502999944,12.2,3.99477532799998));
#333803=CARTESIAN_POINT('Ctrl Pts',(0.852908502999944,5.2,3.99477532799998));
#333804=CARTESIAN_POINT('Ctrl Pts',(0.852908502999944,2.2,3.99477532799998));
#333805=CARTESIAN_POINT('Ctrl Pts',(0.852906525999945,12.2,3.99582927999998));
#333806=CARTESIAN_POINT('Ctrl Pts',(0.852906525999945,5.2,3.99582927999998));
#333807=CARTESIAN_POINT('Ctrl Pts',(0.852906525999945,2.2,3.99582927999998));
#333808=CARTESIAN_POINT('Ctrl Pts',(0.852903240999944,12.2,3.99688862099998));
#333809=CARTESIAN_POINT('Ctrl Pts',(0.852903240999944,5.2,3.99688862099998));
#333810=CARTESIAN_POINT('Ctrl Pts',(0.852903240999944,2.2,3.99688862099998));
#333811=CARTESIAN_POINT('Ctrl Pts',(0.852898635999945,12.2,3.99795333699998));
#333812=CARTESIAN_POINT('Ctrl Pts',(0.852898635999945,5.2,3.99795333699998));
#333813=CARTESIAN_POINT('Ctrl Pts',(0.852898635999945,2.2,3.99795333699998));
#333814=CARTESIAN_POINT('Ctrl Pts',(0.852892698999944,12.2,3.99902341999999));
#333815=CARTESIAN_POINT('Ctrl Pts',(0.852892698999944,5.2,3.99902341999999));
#333816=CARTESIAN_POINT('Ctrl Pts',(0.852892698999944,2.2,3.99902341999999));
#333817=CARTESIAN_POINT('Ctrl Pts',(0.852885417999943,12.2,4.00009885599999));
#333818=CARTESIAN_POINT('Ctrl Pts',(0.852885417999943,5.2,4.00009885599999));
#333819=CARTESIAN_POINT('Ctrl Pts',(0.852885417999943,2.2,4.00009885599999));
#333820=CARTESIAN_POINT('Ctrl Pts',(0.852876779999944,12.2,4.00117963799998));
#333821=CARTESIAN_POINT('Ctrl Pts',(0.852876779999944,5.2,4.00117963799998));
#333822=CARTESIAN_POINT('Ctrl Pts',(0.852876779999944,2.2,4.00117963799998));
#333823=CARTESIAN_POINT('Ctrl Pts',(0.852866772999944,12.2,4.00226575399999));
#333824=CARTESIAN_POINT('Ctrl Pts',(0.852866772999944,5.2,4.00226575399999));
#333825=CARTESIAN_POINT('Ctrl Pts',(0.852866772999944,2.2,4.00226575399999));
#333826=CARTESIAN_POINT('Ctrl Pts',(0.852855384999944,12.2,4.00335719399998));
#333827=CARTESIAN_POINT('Ctrl Pts',(0.852855384999944,5.2,4.00335719399998));
#333828=CARTESIAN_POINT('Ctrl Pts',(0.852855384999944,2.2,4.00335719399998));
#333829=CARTESIAN_POINT('Ctrl Pts',(0.852842602999945,12.2,4.00445394799998));
#333830=CARTESIAN_POINT('Ctrl Pts',(0.852842602999945,5.2,4.00445394799998));
#333831=CARTESIAN_POINT('Ctrl Pts',(0.852842602999945,2.2,4.00445394799998));
#333832=CARTESIAN_POINT('Ctrl Pts',(0.852828414999944,12.2,4.00555600399999));
#333833=CARTESIAN_POINT('Ctrl Pts',(0.852828414999944,5.2,4.00555600399999));
#333834=CARTESIAN_POINT('Ctrl Pts',(0.852828414999944,2.2,4.00555600399999));
#333835=CARTESIAN_POINT('Ctrl Pts',(0.852812809999944,12.2,4.00666335299999));
#333836=CARTESIAN_POINT('Ctrl Pts',(0.852812809999944,5.2,4.00666335299999));
#333837=CARTESIAN_POINT('Ctrl Pts',(0.852812809999944,2.2,4.00666335299999));
#333838=CARTESIAN_POINT('Ctrl Pts',(0.852795775999944,12.2,4.00777598499998));
#333839=CARTESIAN_POINT('Ctrl Pts',(0.852795775999944,5.2,4.00777598499998));
#333840=CARTESIAN_POINT('Ctrl Pts',(0.852795775999944,2.2,4.00777598499998));
#333841=CARTESIAN_POINT('Ctrl Pts',(0.852777298999944,12.2,4.00889388999998));
#333842=CARTESIAN_POINT('Ctrl Pts',(0.852777298999944,5.2,4.00889388999998));
#333843=CARTESIAN_POINT('Ctrl Pts',(0.852777298999944,2.2,4.00889388999998));
#333844=CARTESIAN_POINT('Ctrl Pts',(0.852757369999945,12.2,4.01001705599998));
#333845=CARTESIAN_POINT('Ctrl Pts',(0.852757369999945,5.2,4.01001705599998));
#333846=CARTESIAN_POINT('Ctrl Pts',(0.852757369999945,2.2,4.01001705599998));
#333847=CARTESIAN_POINT('Ctrl Pts',(0.852735973999944,12.2,4.01114547299999));
#333848=CARTESIAN_POINT('Ctrl Pts',(0.852735973999944,5.2,4.01114547299999));
#333849=CARTESIAN_POINT('Ctrl Pts',(0.852735973999944,2.2,4.01114547299999));
#333850=CARTESIAN_POINT('Ctrl Pts',(0.852713101999945,12.2,4.01227913099999));
#333851=CARTESIAN_POINT('Ctrl Pts',(0.852713101999945,5.2,4.01227913099999));
#333852=CARTESIAN_POINT('Ctrl Pts',(0.852713101999945,2.2,4.01227913099999));
#333853=CARTESIAN_POINT('Ctrl Pts',(0.852688740999944,12.2,4.01341801999998));
#333854=CARTESIAN_POINT('Ctrl Pts',(0.852688740999944,5.2,4.01341801999998));
#333855=CARTESIAN_POINT('Ctrl Pts',(0.852688740999944,2.2,4.01341801999998));
#333856=CARTESIAN_POINT('Ctrl Pts',(0.852662876999944,12.2,4.01456212999998));
#333857=CARTESIAN_POINT('Ctrl Pts',(0.852662876999944,5.2,4.01456212999998));
#333858=CARTESIAN_POINT('Ctrl Pts',(0.852662876999944,2.2,4.01456212999998));
#333859=CARTESIAN_POINT('Ctrl Pts',(0.852635501999944,12.2,4.01571144899999));
#333860=CARTESIAN_POINT('Ctrl Pts',(0.852635501999944,5.2,4.01571144899999));
#333861=CARTESIAN_POINT('Ctrl Pts',(0.852635501999944,2.2,4.01571144899999));
#333862=CARTESIAN_POINT('Ctrl Pts',(0.852606601999945,12.2,4.01686596899999));
#333863=CARTESIAN_POINT('Ctrl Pts',(0.852606601999945,5.2,4.01686596899999));
#333864=CARTESIAN_POINT('Ctrl Pts',(0.852606601999945,2.2,4.01686596899999));
#333865=CARTESIAN_POINT('Ctrl Pts',(0.852576166999944,12.2,4.01802567799999));
#333866=CARTESIAN_POINT('Ctrl Pts',(0.852576166999944,5.2,4.01802567799999));
#333867=CARTESIAN_POINT('Ctrl Pts',(0.852576166999944,2.2,4.01802567799999));
#333868=CARTESIAN_POINT('Ctrl Pts',(0.852544183999945,12.2,4.01919056699998));
#333869=CARTESIAN_POINT('Ctrl Pts',(0.852544183999945,5.2,4.01919056699998));
#333870=CARTESIAN_POINT('Ctrl Pts',(0.852544183999945,2.2,4.01919056699998));
#333871=CARTESIAN_POINT('Ctrl Pts',(0.852510640999945,12.2,4.02036062599999));
#333872=CARTESIAN_POINT('Ctrl Pts',(0.852510640999945,5.2,4.02036062599999));
#333873=CARTESIAN_POINT('Ctrl Pts',(0.852510640999945,2.2,4.02036062599999));
#333874=CARTESIAN_POINT('Ctrl Pts',(0.852475527999944,12.2,4.02153584299998));
#333875=CARTESIAN_POINT('Ctrl Pts',(0.852475527999944,5.2,4.02153584299998));
#333876=CARTESIAN_POINT('Ctrl Pts',(0.852475527999944,2.2,4.02153584299998));
#333877=CARTESIAN_POINT('Ctrl Pts',(0.852438831999944,12.2,4.02271620799999));
#333878=CARTESIAN_POINT('Ctrl Pts',(0.852438831999944,5.2,4.02271620799999));
#333879=CARTESIAN_POINT('Ctrl Pts',(0.852438831999944,2.2,4.02271620799999));
#333880=CARTESIAN_POINT('Ctrl Pts',(0.852400542999944,12.2,4.02390171199999));
#333881=CARTESIAN_POINT('Ctrl Pts',(0.852400542999944,5.2,4.02390171199999));
#333882=CARTESIAN_POINT('Ctrl Pts',(0.852400542999944,2.2,4.02390171199999));
#333883=CARTESIAN_POINT('Ctrl Pts',(0.852360646999945,12.2,4.02509234399999));
#333884=CARTESIAN_POINT('Ctrl Pts',(0.852360646999945,5.2,4.02509234399999));
#333885=CARTESIAN_POINT('Ctrl Pts',(0.852360646999945,2.2,4.02509234399999));
#333886=CARTESIAN_POINT('Ctrl Pts',(0.852319135999945,12.2,4.02628809399998));
#333887=CARTESIAN_POINT('Ctrl Pts',(0.852319135999945,5.2,4.02628809399998));
#333888=CARTESIAN_POINT('Ctrl Pts',(0.852319135999945,2.2,4.02628809399998));
#333889=CARTESIAN_POINT('Ctrl Pts',(0.852275997999944,12.2,4.02748895199998));
#333890=CARTESIAN_POINT('Ctrl Pts',(0.852275997999944,5.2,4.02748895199998));
#333891=CARTESIAN_POINT('Ctrl Pts',(0.852275997999944,2.2,4.02748895199998));
#333892=CARTESIAN_POINT('Ctrl Pts',(0.852231218999945,12.2,4.02869490799999));
#333893=CARTESIAN_POINT('Ctrl Pts',(0.852231218999945,5.2,4.02869490799999));
#333894=CARTESIAN_POINT('Ctrl Pts',(0.852231218999945,2.2,4.02869490799999));
#333895=CARTESIAN_POINT('Ctrl Pts',(0.852184791999945,12.2,4.02990594999999));
#333896=CARTESIAN_POINT('Ctrl Pts',(0.852184791999945,5.2,4.02990594999999));
#333897=CARTESIAN_POINT('Ctrl Pts',(0.852184791999945,2.2,4.02990594999999));
#333898=CARTESIAN_POINT('Ctrl Pts',(0.852136700999945,12.2,4.03112206999998));
#333899=CARTESIAN_POINT('Ctrl Pts',(0.852136700999945,5.2,4.03112206999998));
#333900=CARTESIAN_POINT('Ctrl Pts',(0.852136700999945,2.2,4.03112206999998));
#333901=CARTESIAN_POINT('Ctrl Pts',(0.852086937999944,12.2,4.03234325799998));
#333902=CARTESIAN_POINT('Ctrl Pts',(0.852086937999944,5.2,4.03234325799998));
#333903=CARTESIAN_POINT('Ctrl Pts',(0.852086937999944,2.2,4.03234325799998));
#333904=CARTESIAN_POINT('Ctrl Pts',(0.852035490999944,12.2,4.03356950199999));
#333905=CARTESIAN_POINT('Ctrl Pts',(0.852035490999944,5.2,4.03356950199999));
#333906=CARTESIAN_POINT('Ctrl Pts',(0.852035490999944,2.2,4.03356950199999));
#333907=CARTESIAN_POINT('Ctrl Pts',(0.851982348999945,12.2,4.03480079299998));
#333908=CARTESIAN_POINT('Ctrl Pts',(0.851982348999945,5.2,4.03480079299998));
#333909=CARTESIAN_POINT('Ctrl Pts',(0.851982348999945,2.2,4.03480079299998));
#333910=CARTESIAN_POINT('Ctrl Pts',(0.851927500999944,12.2,4.03603712099999));
#333911=CARTESIAN_POINT('Ctrl Pts',(0.851927500999944,5.2,4.03603712099999));
#333912=CARTESIAN_POINT('Ctrl Pts',(0.851927500999944,2.2,4.03603712099999));
#333913=CARTESIAN_POINT('Ctrl Pts',(0.851870935999944,12.2,4.03727847499999));
#333914=CARTESIAN_POINT('Ctrl Pts',(0.851870935999944,5.2,4.03727847499999));
#333915=CARTESIAN_POINT('Ctrl Pts',(0.851870935999944,2.2,4.03727847499999));
#333916=CARTESIAN_POINT('Ctrl Pts',(0.851812641999944,12.2,4.03852484599999));
#333917=CARTESIAN_POINT('Ctrl Pts',(0.851812641999944,5.2,4.03852484599999));
#333918=CARTESIAN_POINT('Ctrl Pts',(0.851812641999944,2.2,4.03852484599999));
#333919=CARTESIAN_POINT('Ctrl Pts',(0.851752610999944,12.2,4.03977622199999));
#333920=CARTESIAN_POINT('Ctrl Pts',(0.851752610999944,5.2,4.03977622199999));
#333921=CARTESIAN_POINT('Ctrl Pts',(0.851752610999944,2.2,4.03977622199999));
#333922=CARTESIAN_POINT('Ctrl Pts',(0.851690827999944,12.2,4.04103259599999));
#333923=CARTESIAN_POINT('Ctrl Pts',(0.851690827999944,5.2,4.04103259599999));
#333924=CARTESIAN_POINT('Ctrl Pts',(0.851690827999944,2.2,4.04103259599999));
#333925=CARTESIAN_POINT('Ctrl Pts',(0.851627284999944,12.2,4.04229395399998));
#333926=CARTESIAN_POINT('Ctrl Pts',(0.851627284999944,5.2,4.04229395399998));
#333927=CARTESIAN_POINT('Ctrl Pts',(0.851627284999944,2.2,4.04229395399998));
#333928=CARTESIAN_POINT('Ctrl Pts',(0.851561969999944,12.2,4.04356028899999));
#333929=CARTESIAN_POINT('Ctrl Pts',(0.851561969999944,5.2,4.04356028899999));
#333930=CARTESIAN_POINT('Ctrl Pts',(0.851561969999944,2.2,4.04356028899999));
#333931=CARTESIAN_POINT('Ctrl Pts',(0.851494872999944,12.2,4.04483158999999));
#333932=CARTESIAN_POINT('Ctrl Pts',(0.851494872999944,5.2,4.04483158999999));
#333933=CARTESIAN_POINT('Ctrl Pts',(0.851494872999944,2.2,4.04483158999999));
#333934=CARTESIAN_POINT('Ctrl Pts',(0.851425981999945,12.2,4.04610784699998));
#333935=CARTESIAN_POINT('Ctrl Pts',(0.851425981999945,5.2,4.04610784699998));
#333936=CARTESIAN_POINT('Ctrl Pts',(0.851425981999945,2.2,4.04610784699998));
#333937=CARTESIAN_POINT('Ctrl Pts',(0.851355286999944,12.2,4.04738904899999));
#333938=CARTESIAN_POINT('Ctrl Pts',(0.851355286999944,5.2,4.04738904899999));
#333939=CARTESIAN_POINT('Ctrl Pts',(0.851355286999944,2.2,4.04738904899999));
#333940=CARTESIAN_POINT('Ctrl Pts',(0.851282776999944,12.2,4.04867518799998));
#333941=CARTESIAN_POINT('Ctrl Pts',(0.851282776999944,5.2,4.04867518799998));
#333942=CARTESIAN_POINT('Ctrl Pts',(0.851282776999944,2.2,4.04867518799998));
#333943=CARTESIAN_POINT('Ctrl Pts',(0.851208441999944,12.2,4.04996625099999));
#333944=CARTESIAN_POINT('Ctrl Pts',(0.851208441999944,5.2,4.04996625099999));
#333945=CARTESIAN_POINT('Ctrl Pts',(0.851208441999944,2.2,4.04996625099999));
#333946=CARTESIAN_POINT('Ctrl Pts',(0.851132271999945,12.2,4.05126223099998));
#333947=CARTESIAN_POINT('Ctrl Pts',(0.851132271999945,5.2,4.05126223099998));
#333948=CARTESIAN_POINT('Ctrl Pts',(0.851132271999945,2.2,4.05126223099998));
#333949=CARTESIAN_POINT('Ctrl Pts',(0.851054254999944,12.2,4.05256311499999));
#333950=CARTESIAN_POINT('Ctrl Pts',(0.851054254999944,5.2,4.05256311499999));
#333951=CARTESIAN_POINT('Ctrl Pts',(0.851054254999944,2.2,4.05256311499999));
#333952=CARTESIAN_POINT('Ctrl Pts',(0.850974380999945,12.2,4.05386889599999));
#333953=CARTESIAN_POINT('Ctrl Pts',(0.850974380999945,5.2,4.05386889599999));
#333954=CARTESIAN_POINT('Ctrl Pts',(0.850974380999945,2.2,4.05386889599999));
#333955=CARTESIAN_POINT('Ctrl Pts',(0.850892638999944,12.2,4.05517956199999));
#333956=CARTESIAN_POINT('Ctrl Pts',(0.850892638999944,5.2,4.05517956199999));
#333957=CARTESIAN_POINT('Ctrl Pts',(0.850892638999944,2.2,4.05517956199999));
#333958=CARTESIAN_POINT('Ctrl Pts',(0.850809018999944,12.2,4.05649510399999));
#333959=CARTESIAN_POINT('Ctrl Pts',(0.850809018999944,5.2,4.05649510399999));
#333960=CARTESIAN_POINT('Ctrl Pts',(0.850809018999944,2.2,4.05649510399999));
#333961=CARTESIAN_POINT('Ctrl Pts',(0.850723510999944,12.2,4.05781551099999));
#333962=CARTESIAN_POINT('Ctrl Pts',(0.850723510999944,5.2,4.05781551099999));
#333963=CARTESIAN_POINT('Ctrl Pts',(0.850723510999944,2.2,4.05781551099999));
#333964=CARTESIAN_POINT('Ctrl Pts',(0.850636103999944,12.2,4.05914077399999));
#333965=CARTESIAN_POINT('Ctrl Pts',(0.850636103999944,5.2,4.05914077399999));
#333966=CARTESIAN_POINT('Ctrl Pts',(0.850636103999944,2.2,4.05914077399999));
#333967=CARTESIAN_POINT('Ctrl Pts',(0.850546785999944,12.2,4.06047088299999));
#333968=CARTESIAN_POINT('Ctrl Pts',(0.850546785999944,5.2,4.06047088299999));
#333969=CARTESIAN_POINT('Ctrl Pts',(0.850546785999944,2.2,4.06047088299999));
#333970=CARTESIAN_POINT('Ctrl Pts',(0.850455550999943,12.2,4.06180582599998));
#333971=CARTESIAN_POINT('Ctrl Pts',(0.850455550999943,5.2,4.06180582599998));
#333972=CARTESIAN_POINT('Ctrl Pts',(0.850455550999943,2.2,4.06180582599998));
#333973=CARTESIAN_POINT('Ctrl Pts',(0.850362384999944,12.2,4.06314559499998));
#333974=CARTESIAN_POINT('Ctrl Pts',(0.850362384999944,5.2,4.06314559499998));
#333975=CARTESIAN_POINT('Ctrl Pts',(0.850362384999944,2.2,4.06314559499998));
#333976=CARTESIAN_POINT('Ctrl Pts',(0.850267278999944,12.2,4.06449018099998));
#333977=CARTESIAN_POINT('Ctrl Pts',(0.850267278999944,5.2,4.06449018099998));
#333978=CARTESIAN_POINT('Ctrl Pts',(0.850267278999944,2.2,4.06449018099998));
#333979=CARTESIAN_POINT('Ctrl Pts',(0.850170222999944,12.2,4.06583957199998));
#333980=CARTESIAN_POINT('Ctrl Pts',(0.850170222999944,5.2,4.06583957199998));
#333981=CARTESIAN_POINT('Ctrl Pts',(0.850170222999944,2.2,4.06583957199998));
#333982=CARTESIAN_POINT('Ctrl Pts',(0.850071204999944,12.2,4.06719375799998));
#333983=CARTESIAN_POINT('Ctrl Pts',(0.850071204999944,5.2,4.06719375799998));
#333984=CARTESIAN_POINT('Ctrl Pts',(0.850071204999944,2.2,4.06719375799998));
#333985=CARTESIAN_POINT('Ctrl Pts',(0.849970217999945,12.2,4.06855273199999));
#333986=CARTESIAN_POINT('Ctrl Pts',(0.849970217999945,5.2,4.06855273199999));
#333987=CARTESIAN_POINT('Ctrl Pts',(0.849970217999945,2.2,4.06855273199999));
#333988=CARTESIAN_POINT('Ctrl Pts',(0.849867249999944,12.2,4.06991647999998));
#333989=CARTESIAN_POINT('Ctrl Pts',(0.849867249999944,5.2,4.06991647999998));
#333990=CARTESIAN_POINT('Ctrl Pts',(0.849867249999944,2.2,4.06991647999998));
#333991=CARTESIAN_POINT('Ctrl Pts',(0.849762289999945,12.2,4.07128499499999));
#333992=CARTESIAN_POINT('Ctrl Pts',(0.849762289999945,5.2,4.07128499499999));
#333993=CARTESIAN_POINT('Ctrl Pts',(0.849762289999945,2.2,4.07128499499999));
#333994=CARTESIAN_POINT('Ctrl Pts',(0.849655330999944,12.2,4.07265826499999));
#333995=CARTESIAN_POINT('Ctrl Pts',(0.849655330999944,5.2,4.07265826499999));
#333996=CARTESIAN_POINT('Ctrl Pts',(0.849655330999944,2.2,4.07265826499999));
#333997=CARTESIAN_POINT('Ctrl Pts',(0.849546358999944,12.2,4.07403628199998));
#333998=CARTESIAN_POINT('Ctrl Pts',(0.849546358999944,5.2,4.07403628199998));
#333999=CARTESIAN_POINT('Ctrl Pts',(0.849546358999944,2.2,4.07403628199998));
#334000=CARTESIAN_POINT('Ctrl Pts',(0.849435366999944,12.2,4.07541903499999));
#334001=CARTESIAN_POINT('Ctrl Pts',(0.849435366999944,5.2,4.07541903499999));
#334002=CARTESIAN_POINT('Ctrl Pts',(0.849435366999944,2.2,4.07541903499999));
#334003=CARTESIAN_POINT('Ctrl Pts',(0.849322344999944,12.2,4.07680651499999));
#334004=CARTESIAN_POINT('Ctrl Pts',(0.849322344999944,5.2,4.07680651499999));
#334005=CARTESIAN_POINT('Ctrl Pts',(0.849322344999944,2.2,4.07680651499999));
#334006=CARTESIAN_POINT('Ctrl Pts',(0.849207281999944,12.2,4.07819871099999));
#334007=CARTESIAN_POINT('Ctrl Pts',(0.849207281999944,5.2,4.07819871099999));
#334008=CARTESIAN_POINT('Ctrl Pts',(0.849207281999944,2.2,4.07819871099999));
#334009=CARTESIAN_POINT('Ctrl Pts',(0.849090166999944,12.2,4.07959561399998));
#334010=CARTESIAN_POINT('Ctrl Pts',(0.849090166999944,5.2,4.07959561399998));
#334011=CARTESIAN_POINT('Ctrl Pts',(0.849090166999944,2.2,4.07959561399998));
#334012=CARTESIAN_POINT('Ctrl Pts',(0.848970992999944,12.2,4.08099721399999));
#334013=CARTESIAN_POINT('Ctrl Pts',(0.848970992999944,5.2,4.08099721399999));
#334014=CARTESIAN_POINT('Ctrl Pts',(0.848970992999944,2.2,4.08099721399999));
#334015=CARTESIAN_POINT('Ctrl Pts',(0.848849747999945,12.2,4.08240349999998));
#334016=CARTESIAN_POINT('Ctrl Pts',(0.848849747999945,5.2,4.08240349999998));
#334017=CARTESIAN_POINT('Ctrl Pts',(0.848849747999945,2.2,4.08240349999998));
#334018=CARTESIAN_POINT('Ctrl Pts',(0.848726422999944,12.2,4.08381446399999));
#334019=CARTESIAN_POINT('Ctrl Pts',(0.848726422999944,5.2,4.08381446399999));
#334020=CARTESIAN_POINT('Ctrl Pts',(0.848726422999944,2.2,4.08381446399999));
#334021=CARTESIAN_POINT('Ctrl Pts',(0.848601007999944,12.2,4.08523009399998));
#334022=CARTESIAN_POINT('Ctrl Pts',(0.848601007999944,5.2,4.08523009399998));
#334023=CARTESIAN_POINT('Ctrl Pts',(0.848601007999944,2.2,4.08523009399998));
#334024=CARTESIAN_POINT('Ctrl Pts',(0.848473494999944,12.2,4.08665038299999));
#334025=CARTESIAN_POINT('Ctrl Pts',(0.848473494999944,5.2,4.08665038299999));
#334026=CARTESIAN_POINT('Ctrl Pts',(0.848473494999944,2.2,4.08665038299999));
#334027=CARTESIAN_POINT('Ctrl Pts',(0.848343870999945,12.2,4.08807531799999));
#334028=CARTESIAN_POINT('Ctrl Pts',(0.848343870999945,5.2,4.08807531799999));
#334029=CARTESIAN_POINT('Ctrl Pts',(0.848343870999945,2.2,4.08807531799999));
#334030=CARTESIAN_POINT('Ctrl Pts',(0.848212129999945,12.2,4.08950489299999));
#334031=CARTESIAN_POINT('Ctrl Pts',(0.848212129999945,5.2,4.08950489299999));
#334032=CARTESIAN_POINT('Ctrl Pts',(0.848212129999945,2.2,4.08950489299999));
#334033=CARTESIAN_POINT('Ctrl Pts',(0.848078258999945,12.2,4.09093909399999));
#334034=CARTESIAN_POINT('Ctrl Pts',(0.848078258999945,5.2,4.09093909399999));
#334035=CARTESIAN_POINT('Ctrl Pts',(0.848078258999945,2.2,4.09093909399999));
#334036=CARTESIAN_POINT('Ctrl Pts',(0.847942250999945,12.2,4.09237791399998));
#334037=CARTESIAN_POINT('Ctrl Pts',(0.847942250999945,5.2,4.09237791399998));
#334038=CARTESIAN_POINT('Ctrl Pts',(0.847942250999945,2.2,4.09237791399998));
#334039=CARTESIAN_POINT('Ctrl Pts',(0.847804094999944,12.2,4.09382134299998));
#334040=CARTESIAN_POINT('Ctrl Pts',(0.847804094999944,5.2,4.09382134299998));
#334041=CARTESIAN_POINT('Ctrl Pts',(0.847804094999944,2.2,4.09382134299998));
#334042=CARTESIAN_POINT('Ctrl Pts',(0.847663781999944,12.2,4.09526936999999));
#334043=CARTESIAN_POINT('Ctrl Pts',(0.847663781999944,5.2,4.09526936999999));
#334044=CARTESIAN_POINT('Ctrl Pts',(0.847663781999944,2.2,4.09526936999999));
#334045=CARTESIAN_POINT('Ctrl Pts',(0.847521301999944,12.2,4.09672198499998));
#334046=CARTESIAN_POINT('Ctrl Pts',(0.847521301999944,5.2,4.09672198499998));
#334047=CARTESIAN_POINT('Ctrl Pts',(0.847521301999944,2.2,4.09672198499998));
#334048=CARTESIAN_POINT('Ctrl Pts',(0.847376646999944,12.2,4.09817917999998));
#334049=CARTESIAN_POINT('Ctrl Pts',(0.847376646999944,5.2,4.09817917999998));
#334050=CARTESIAN_POINT('Ctrl Pts',(0.847376646999944,2.2,4.09817917999998));
#334051=CARTESIAN_POINT('Ctrl Pts',(0.847229806999944,12.2,4.09964094399999));
#334052=CARTESIAN_POINT('Ctrl Pts',(0.847229806999944,5.2,4.09964094399999));
#334053=CARTESIAN_POINT('Ctrl Pts',(0.847229806999944,2.2,4.09964094399999));
#334054=CARTESIAN_POINT('Ctrl Pts',(0.847080770999944,12.2,4.10110726699998));
#334055=CARTESIAN_POINT('Ctrl Pts',(0.847080770999944,5.2,4.10110726699998));
#334056=CARTESIAN_POINT('Ctrl Pts',(0.847080770999944,2.2,4.10110726699998));
#334057=CARTESIAN_POINT('Ctrl Pts',(0.846929531999944,12.2,4.10257814099998));
#334058=CARTESIAN_POINT('Ctrl Pts',(0.846929531999944,5.2,4.10257814099998));
#334059=CARTESIAN_POINT('Ctrl Pts',(0.846929531999944,2.2,4.10257814099998));
#334060=CARTESIAN_POINT('Ctrl Pts',(0.846776077999943,12.2,4.10405355399998));
#334061=CARTESIAN_POINT('Ctrl Pts',(0.846776077999943,5.2,4.10405355399998));
#334062=CARTESIAN_POINT('Ctrl Pts',(0.846776077999943,2.2,4.10405355399998));
#334063=CARTESIAN_POINT('Ctrl Pts',(0.846620402999945,12.2,4.10553349899998));
#334064=CARTESIAN_POINT('Ctrl Pts',(0.846620402999945,5.2,4.10553349899998));
#334065=CARTESIAN_POINT('Ctrl Pts',(0.846620402999945,2.2,4.10553349899998));
#334066=CARTESIAN_POINT('Ctrl Pts',(0.846462495999944,12.2,4.10701796199999));
#334067=CARTESIAN_POINT('Ctrl Pts',(0.846462495999944,5.2,4.10701796199999));
#334068=CARTESIAN_POINT('Ctrl Pts',(0.846462495999944,2.2,4.10701796199999));
#334069=CARTESIAN_POINT('Ctrl Pts',(0.846302346999944,12.2,4.10850693699999));
#334070=CARTESIAN_POINT('Ctrl Pts',(0.846302346999944,5.2,4.10850693699999));
#334071=CARTESIAN_POINT('Ctrl Pts',(0.846302346999944,2.2,4.10850693699999));
#334072=CARTESIAN_POINT('Ctrl Pts',(0.846139947999944,12.2,4.11000041399999));
#334073=CARTESIAN_POINT('Ctrl Pts',(0.846139947999944,5.2,4.11000041399999));
#334074=CARTESIAN_POINT('Ctrl Pts',(0.846139947999944,2.2,4.11000041399999));
#334075=CARTESIAN_POINT('Ctrl Pts',(0.845975289999944,12.2,4.11149838199999));
#334076=CARTESIAN_POINT('Ctrl Pts',(0.845975289999944,5.2,4.11149838199999));
#334077=CARTESIAN_POINT('Ctrl Pts',(0.845975289999944,2.2,4.11149838199999));
#334078=CARTESIAN_POINT('Ctrl Pts',(0.845808361999943,12.2,4.11300083099999));
#334079=CARTESIAN_POINT('Ctrl Pts',(0.845808361999943,5.2,4.11300083099999));
#334080=CARTESIAN_POINT('Ctrl Pts',(0.845808361999943,2.2,4.11300083099999));
#334081=CARTESIAN_POINT('Ctrl Pts',(0.845639156999944,12.2,4.11450775199998));
#334082=CARTESIAN_POINT('Ctrl Pts',(0.845639156999944,5.2,4.11450775199998));
#334083=CARTESIAN_POINT('Ctrl Pts',(0.845639156999944,2.2,4.11450775199998));
#334084=CARTESIAN_POINT('Ctrl Pts',(0.845467665999945,12.2,4.11601913699998));
#334085=CARTESIAN_POINT('Ctrl Pts',(0.845467665999945,5.2,4.11601913699998));
#334086=CARTESIAN_POINT('Ctrl Pts',(0.845467665999945,2.2,4.11601913699998));
#334087=CARTESIAN_POINT('Ctrl Pts',(0.845293878999944,12.2,4.11753497299999));
#334088=CARTESIAN_POINT('Ctrl Pts',(0.845293878999944,5.2,4.11753497299999));
#334089=CARTESIAN_POINT('Ctrl Pts',(0.845293878999944,2.2,4.11753497299999));
#334090=CARTESIAN_POINT('Ctrl Pts',(0.845117785999945,12.2,4.11905525299999));
#334091=CARTESIAN_POINT('Ctrl Pts',(0.845117785999945,5.2,4.11905525299999));
#334092=CARTESIAN_POINT('Ctrl Pts',(0.845117785999945,2.2,4.11905525299999));
#334093=CARTESIAN_POINT('Ctrl Pts',(0.844939379999944,12.2,4.12057996599999));
#334094=CARTESIAN_POINT('Ctrl Pts',(0.844939379999944,5.2,4.12057996599999));
#334095=CARTESIAN_POINT('Ctrl Pts',(0.844939379999944,2.2,4.12057996599999));
#334096=CARTESIAN_POINT('Ctrl Pts',(0.844758650999945,12.2,4.12210910299999));
#334097=CARTESIAN_POINT('Ctrl Pts',(0.844758650999945,5.2,4.12210910299999));
#334098=CARTESIAN_POINT('Ctrl Pts',(0.844758650999945,2.2,4.12210910299999));
#334099=CARTESIAN_POINT('Ctrl Pts',(0.844575590999944,12.2,4.12364265299999));
#334100=CARTESIAN_POINT('Ctrl Pts',(0.844575590999944,5.2,4.12364265299999));
#334101=CARTESIAN_POINT('Ctrl Pts',(0.844575590999944,2.2,4.12364265299999));
#334102=CARTESIAN_POINT('Ctrl Pts',(0.844390189999944,12.2,4.12518060899998));
#334103=CARTESIAN_POINT('Ctrl Pts',(0.844390189999944,5.2,4.12518060899998));
#334104=CARTESIAN_POINT('Ctrl Pts',(0.844390189999944,2.2,4.12518060899998));
#334105=CARTESIAN_POINT('Ctrl Pts',(0.844202440999945,12.2,4.12672295999998));
#334106=CARTESIAN_POINT('Ctrl Pts',(0.844202440999945,5.2,4.12672295999998));
#334107=CARTESIAN_POINT('Ctrl Pts',(0.844202440999945,2.2,4.12672295999998));
#334108=CARTESIAN_POINT('Ctrl Pts',(0.844012331999945,12.2,4.12826969399998));
#334109=CARTESIAN_POINT('Ctrl Pts',(0.844012331999945,5.2,4.12826969399998));
#334110=CARTESIAN_POINT('Ctrl Pts',(0.844012331999945,2.2,4.12826969399998));
#334111=CARTESIAN_POINT('Ctrl Pts',(0.843819855999944,12.2,4.12982080499999));
#334112=CARTESIAN_POINT('Ctrl Pts',(0.843819855999944,5.2,4.12982080499999));
#334113=CARTESIAN_POINT('Ctrl Pts',(0.843819855999944,2.2,4.12982080499999));
#334114=CARTESIAN_POINT('Ctrl Pts',(0.843625005999944,12.2,4.13137628199999));
#334115=CARTESIAN_POINT('Ctrl Pts',(0.843625005999944,5.2,4.13137628199999));
#334116=CARTESIAN_POINT('Ctrl Pts',(0.843625005999944,2.2,4.13137628199999));
#334117=CARTESIAN_POINT('Ctrl Pts',(0.843427769999944,12.2,4.13293611499999));
#334118=CARTESIAN_POINT('Ctrl Pts',(0.843427769999944,5.2,4.13293611499999));
#334119=CARTESIAN_POINT('Ctrl Pts',(0.843427769999944,2.2,4.13293611499999));
#334120=CARTESIAN_POINT('Ctrl Pts',(0.843228141999944,12.2,4.13450029499998));
#334121=CARTESIAN_POINT('Ctrl Pts',(0.843228141999944,5.2,4.13450029499998));
#334122=CARTESIAN_POINT('Ctrl Pts',(0.843228141999944,2.2,4.13450029499998));
#334123=CARTESIAN_POINT('Ctrl Pts',(0.843026111999944,12.2,4.13606881099999));
#334124=CARTESIAN_POINT('Ctrl Pts',(0.843026111999944,5.2,4.13606881099999));
#334125=CARTESIAN_POINT('Ctrl Pts',(0.843026111999944,2.2,4.13606881099999));
#334126=CARTESIAN_POINT('Ctrl Pts',(0.842821670999945,12.2,4.13764165599999));
#334127=CARTESIAN_POINT('Ctrl Pts',(0.842821670999945,5.2,4.13764165599999));
#334128=CARTESIAN_POINT('Ctrl Pts',(0.842821670999945,2.2,4.13764165599999));
#334129=CARTESIAN_POINT('Ctrl Pts',(0.842614809999944,12.2,4.13921881899999));
#334130=CARTESIAN_POINT('Ctrl Pts',(0.842614809999944,5.2,4.13921881899999));
#334131=CARTESIAN_POINT('Ctrl Pts',(0.842614809999944,2.2,4.13921881899999));
#334132=CARTESIAN_POINT('Ctrl Pts',(0.842405522999944,12.2,4.14080028899999));
#334133=CARTESIAN_POINT('Ctrl Pts',(0.842405522999944,5.2,4.14080028899999));
#334134=CARTESIAN_POINT('Ctrl Pts',(0.842405522999944,2.2,4.14080028899999));
#334135=CARTESIAN_POINT('Ctrl Pts',(0.842193798999944,12.2,4.14238605799999));
#334136=CARTESIAN_POINT('Ctrl Pts',(0.842193798999944,5.2,4.14238605799999));
#334137=CARTESIAN_POINT('Ctrl Pts',(0.842193798999944,2.2,4.14238605799999));
#334138=CARTESIAN_POINT('Ctrl Pts',(0.841979630999944,12.2,4.14397611799998));
#334139=CARTESIAN_POINT('Ctrl Pts',(0.841979630999944,5.2,4.14397611799998));
#334140=CARTESIAN_POINT('Ctrl Pts',(0.841979630999944,2.2,4.14397611799998));
#334141=CARTESIAN_POINT('Ctrl Pts',(0.841763009999944,12.2,4.14557045599998));
#334142=CARTESIAN_POINT('Ctrl Pts',(0.841763009999944,5.2,4.14557045599998));
#334143=CARTESIAN_POINT('Ctrl Pts',(0.841763009999944,2.2,4.14557045599998));
#334144=CARTESIAN_POINT('Ctrl Pts',(0.841543926999945,12.2,4.14716906499999));
#334145=CARTESIAN_POINT('Ctrl Pts',(0.841543926999945,5.2,4.14716906499999));
#334146=CARTESIAN_POINT('Ctrl Pts',(0.841543926999945,2.2,4.14716906499999));
#334147=CARTESIAN_POINT('Ctrl Pts',(0.841322372999944,12.2,4.14877193599998));
#334148=CARTESIAN_POINT('Ctrl Pts',(0.841322372999944,5.2,4.14877193599998));
#334149=CARTESIAN_POINT('Ctrl Pts',(0.841322372999944,2.2,4.14877193599998));
#334150=CARTESIAN_POINT('Ctrl Pts',(0.841098341999944,12.2,4.15037905699998));
#334151=CARTESIAN_POINT('Ctrl Pts',(0.841098341999944,5.2,4.15037905699998));
#334152=CARTESIAN_POINT('Ctrl Pts',(0.841098341999944,2.2,4.15037905699998));
#334153=CARTESIAN_POINT('Ctrl Pts',(0.840871822999943,12.2,4.15199041799998));
#334154=CARTESIAN_POINT('Ctrl Pts',(0.840871822999943,5.2,4.15199041799998));
#334155=CARTESIAN_POINT('Ctrl Pts',(0.840871822999943,2.2,4.15199041799998));
#334156=CARTESIAN_POINT('Ctrl Pts',(0.840642809999944,12.2,4.15360601399998));
#334157=CARTESIAN_POINT('Ctrl Pts',(0.840642809999944,5.2,4.15360601399998));
#334158=CARTESIAN_POINT('Ctrl Pts',(0.840642809999944,2.2,4.15360601399998));
#334159=CARTESIAN_POINT('Ctrl Pts',(0.840411292999944,12.2,4.15522582999999));
#334160=CARTESIAN_POINT('Ctrl Pts',(0.840411292999944,5.2,4.15522582999999));
#334161=CARTESIAN_POINT('Ctrl Pts',(0.840411292999944,2.2,4.15522582999999));
#334162=CARTESIAN_POINT('Ctrl Pts',(0.840177262999945,12.2,4.15684985999999));
#334163=CARTESIAN_POINT('Ctrl Pts',(0.840177262999945,5.2,4.15684985999999));
#334164=CARTESIAN_POINT('Ctrl Pts',(0.840177262999945,2.2,4.15684985999999));
#334165=CARTESIAN_POINT('Ctrl Pts',(0.839940712999944,12.2,4.15847809399998));
#334166=CARTESIAN_POINT('Ctrl Pts',(0.839940712999944,5.2,4.15847809399998));
#334167=CARTESIAN_POINT('Ctrl Pts',(0.839940712999944,2.2,4.15847809399998));
#334168=CARTESIAN_POINT('Ctrl Pts',(0.839701635999944,12.2,4.16011052199998));
#334169=CARTESIAN_POINT('Ctrl Pts',(0.839701635999944,5.2,4.16011052199998));
#334170=CARTESIAN_POINT('Ctrl Pts',(0.839701635999944,2.2,4.16011052199998));
#334171=CARTESIAN_POINT('Ctrl Pts',(0.839460021999944,12.2,4.16174713499998));
#334172=CARTESIAN_POINT('Ctrl Pts',(0.839460021999944,5.2,4.16174713499998));
#334173=CARTESIAN_POINT('Ctrl Pts',(0.839460021999944,2.2,4.16174713499998));
#334174=CARTESIAN_POINT('Ctrl Pts',(0.839215862999944,12.2,4.16338792299998));
#334175=CARTESIAN_POINT('Ctrl Pts',(0.839215862999944,5.2,4.16338792299998));
#334176=CARTESIAN_POINT('Ctrl Pts',(0.839215862999944,2.2,4.16338792299998));
#334177=CARTESIAN_POINT('Ctrl Pts',(0.838969151999944,12.2,4.16503287599999));
#334178=CARTESIAN_POINT('Ctrl Pts',(0.838969151999944,5.2,4.16503287599999));
#334179=CARTESIAN_POINT('Ctrl Pts',(0.838969151999944,2.2,4.16503287599999));
#334180=CARTESIAN_POINT('Ctrl Pts',(0.838719879999944,12.2,4.16668198599999));
#334181=CARTESIAN_POINT('Ctrl Pts',(0.838719879999944,5.2,4.16668198599999));
#334182=CARTESIAN_POINT('Ctrl Pts',(0.838719879999944,2.2,4.16668198599999));
#334183=CARTESIAN_POINT('Ctrl Pts',(0.838468037999944,12.2,4.16833524199999));
#334184=CARTESIAN_POINT('Ctrl Pts',(0.838468037999944,5.2,4.16833524199999));
#334185=CARTESIAN_POINT('Ctrl Pts',(0.838468037999944,2.2,4.16833524199999));
#334186=CARTESIAN_POINT('Ctrl Pts',(0.838213618999945,12.2,4.16999263699999));
#334187=CARTESIAN_POINT('Ctrl Pts',(0.838213618999945,5.2,4.16999263699999));
#334188=CARTESIAN_POINT('Ctrl Pts',(0.838213618999945,2.2,4.16999263699999));
#334189=CARTESIAN_POINT('Ctrl Pts',(0.837956614999944,12.2,4.17165415799998));
#334190=CARTESIAN_POINT('Ctrl Pts',(0.837956614999944,5.2,4.17165415799998));
#334191=CARTESIAN_POINT('Ctrl Pts',(0.837956614999944,2.2,4.17165415799998));
#334192=CARTESIAN_POINT('Ctrl Pts',(0.837697017999944,12.2,4.17331979799999));
#334193=CARTESIAN_POINT('Ctrl Pts',(0.837697017999944,5.2,4.17331979799999));
#334194=CARTESIAN_POINT('Ctrl Pts',(0.837697017999944,2.2,4.17331979799999));
#334195=CARTESIAN_POINT('Ctrl Pts',(0.837434820999944,12.2,4.17498954799999));
#334196=CARTESIAN_POINT('Ctrl Pts',(0.837434820999944,5.2,4.17498954799999));
#334197=CARTESIAN_POINT('Ctrl Pts',(0.837434820999944,2.2,4.17498954799999));
#334198=CARTESIAN_POINT('Ctrl Pts',(0.837170012999944,12.2,4.17666339699998));
#334199=CARTESIAN_POINT('Ctrl Pts',(0.837170012999944,5.2,4.17666339699998));
#334200=CARTESIAN_POINT('Ctrl Pts',(0.837170012999944,2.2,4.17666339699998));
#334201=CARTESIAN_POINT('Ctrl Pts',(0.836902588999945,12.2,4.17834133499999));
#334202=CARTESIAN_POINT('Ctrl Pts',(0.836902588999945,5.2,4.17834133499999));
#334203=CARTESIAN_POINT('Ctrl Pts',(0.836902588999945,2.2,4.17834133499999));
#334204=CARTESIAN_POINT('Ctrl Pts',(0.836632540999944,12.2,4.18002335599999));
#334205=CARTESIAN_POINT('Ctrl Pts',(0.836632540999944,5.2,4.18002335599999));
#334206=CARTESIAN_POINT('Ctrl Pts',(0.836632540999944,2.2,4.18002335599999));
#334207=CARTESIAN_POINT('Ctrl Pts',(0.836359857999944,12.2,4.18170944799999));
#334208=CARTESIAN_POINT('Ctrl Pts',(0.836359857999944,5.2,4.18170944799999));
#334209=CARTESIAN_POINT('Ctrl Pts',(0.836359857999944,2.2,4.18170944799999));
#334210=CARTESIAN_POINT('Ctrl Pts',(0.836084535999944,12.2,4.18339959999999));
#334211=CARTESIAN_POINT('Ctrl Pts',(0.836084535999944,5.2,4.18339959999999));
#334212=CARTESIAN_POINT('Ctrl Pts',(0.836084535999944,2.2,4.18339959999999));
#334213=CARTESIAN_POINT('Ctrl Pts',(0.835806564999944,12.2,4.18509380699999));
#334214=CARTESIAN_POINT('Ctrl Pts',(0.835806564999944,5.2,4.18509380699999));
#334215=CARTESIAN_POINT('Ctrl Pts',(0.835806564999944,2.2,4.18509380699999));
#334216=CARTESIAN_POINT('Ctrl Pts',(0.835525937999945,12.2,4.18679205599998));
#334217=CARTESIAN_POINT('Ctrl Pts',(0.835525937999945,5.2,4.18679205599998));
#334218=CARTESIAN_POINT('Ctrl Pts',(0.835525937999945,2.2,4.18679205599998));
#334219=CARTESIAN_POINT('Ctrl Pts',(0.835242646999944,12.2,4.18849433899998));
#334220=CARTESIAN_POINT('Ctrl Pts',(0.835242646999944,5.2,4.18849433899998));
#334221=CARTESIAN_POINT('Ctrl Pts',(0.835242646999944,2.2,4.18849433899998));
#334222=CARTESIAN_POINT('Ctrl Pts',(0.834956683999944,12.2,4.19020064599999));
#334223=CARTESIAN_POINT('Ctrl Pts',(0.834956683999944,5.2,4.19020064599999));
#334224=CARTESIAN_POINT('Ctrl Pts',(0.834956683999944,2.2,4.19020064599999));
#334225=CARTESIAN_POINT('Ctrl Pts',(0.834668041999944,12.2,4.19191096899999));
#334226=CARTESIAN_POINT('Ctrl Pts',(0.834668041999944,5.2,4.19191096899999));
#334227=CARTESIAN_POINT('Ctrl Pts',(0.834668041999944,2.2,4.19191096899999));
#334228=CARTESIAN_POINT('Ctrl Pts',(0.834376710999944,12.2,4.19362529799999));
#334229=CARTESIAN_POINT('Ctrl Pts',(0.834376710999944,5.2,4.19362529799999));
#334230=CARTESIAN_POINT('Ctrl Pts',(0.834376710999944,2.2,4.19362529799999));
#334231=CARTESIAN_POINT('Ctrl Pts',(0.834082687999944,12.2,4.19534362299999));
#334232=CARTESIAN_POINT('Ctrl Pts',(0.834082687999944,5.2,4.19534362299999));
#334233=CARTESIAN_POINT('Ctrl Pts',(0.834082687999944,2.2,4.19534362299999));
#334234=CARTESIAN_POINT('Ctrl Pts',(0.833785959999944,12.2,4.19706593499999));
#334235=CARTESIAN_POINT('Ctrl Pts',(0.833785959999944,5.2,4.19706593499999));
#334236=CARTESIAN_POINT('Ctrl Pts',(0.833785959999944,2.2,4.19706593499999));
#334237=CARTESIAN_POINT('Ctrl Pts',(0.833486523999943,12.2,4.19879222499999));
#334238=CARTESIAN_POINT('Ctrl Pts',(0.833486523999943,5.2,4.19879222499999));
#334239=CARTESIAN_POINT('Ctrl Pts',(0.833486523999943,2.2,4.19879222499999));
#334240=CARTESIAN_POINT('Ctrl Pts',(0.833184369999944,12.2,4.20052248299999));
#334241=CARTESIAN_POINT('Ctrl Pts',(0.833184369999944,5.2,4.20052248299999));
#334242=CARTESIAN_POINT('Ctrl Pts',(0.833184369999944,2.2,4.20052248299999));
#334243=CARTESIAN_POINT('Ctrl Pts',(0.832879489999944,12.2,4.20225669999999));
#334244=CARTESIAN_POINT('Ctrl Pts',(0.832879489999944,5.2,4.20225669999999));
#334245=CARTESIAN_POINT('Ctrl Pts',(0.832879489999944,2.2,4.20225669999999));
#334246=CARTESIAN_POINT('Ctrl Pts',(0.832571877999944,12.2,4.20399486699999));
#334247=CARTESIAN_POINT('Ctrl Pts',(0.832571877999944,5.2,4.20399486699999));
#334248=CARTESIAN_POINT('Ctrl Pts',(0.832571877999944,2.2,4.20399486699999));
#334249=CARTESIAN_POINT('Ctrl Pts',(0.832261524999944,12.2,4.20573697499999));
#334250=CARTESIAN_POINT('Ctrl Pts',(0.832261524999944,5.2,4.20573697499999));
#334251=CARTESIAN_POINT('Ctrl Pts',(0.832261524999944,2.2,4.20573697499999));
#334252=CARTESIAN_POINT('Ctrl Pts',(0.831948425999944,12.2,4.20748301399998));
#334253=CARTESIAN_POINT('Ctrl Pts',(0.831948425999944,5.2,4.20748301399998));
#334254=CARTESIAN_POINT('Ctrl Pts',(0.831948425999944,2.2,4.20748301399998));
#334255=CARTESIAN_POINT('Ctrl Pts',(0.831632569999944,12.2,4.20923297499999));
#334256=CARTESIAN_POINT('Ctrl Pts',(0.831632569999944,5.2,4.20923297499999));
#334257=CARTESIAN_POINT('Ctrl Pts',(0.831632569999944,2.2,4.20923297499999));
#334258=CARTESIAN_POINT('Ctrl Pts',(0.831313951999944,12.2,4.21098684799999));
#334259=CARTESIAN_POINT('Ctrl Pts',(0.831313951999944,5.2,4.21098684799999));
#334260=CARTESIAN_POINT('Ctrl Pts',(0.831313951999944,2.2,4.21098684799999));
#334261=CARTESIAN_POINT('Ctrl Pts',(0.830992564999944,12.2,4.21274462499999));
#334262=CARTESIAN_POINT('Ctrl Pts',(0.830992564999944,5.2,4.21274462499999));
#334263=CARTESIAN_POINT('Ctrl Pts',(0.830992564999944,2.2,4.21274462499999));
#334264=CARTESIAN_POINT('Ctrl Pts',(0.830668399999944,12.2,4.21450629599998));
#334265=CARTESIAN_POINT('Ctrl Pts',(0.830668399999944,5.2,4.21450629599998));
#334266=CARTESIAN_POINT('Ctrl Pts',(0.830668399999944,2.2,4.21450629599998));
#334267=CARTESIAN_POINT('Ctrl Pts',(0.830341450999944,12.2,4.21627185199998));
#334268=CARTESIAN_POINT('Ctrl Pts',(0.830341450999944,5.2,4.21627185199998));
#334269=CARTESIAN_POINT('Ctrl Pts',(0.830341450999944,2.2,4.21627185199998));
#334270=CARTESIAN_POINT('Ctrl Pts',(0.830011708999944,12.2,4.21804128199998));
#334271=CARTESIAN_POINT('Ctrl Pts',(0.830011708999944,5.2,4.21804128199998));
#334272=CARTESIAN_POINT('Ctrl Pts',(0.830011708999944,2.2,4.21804128199998));
#334273=CARTESIAN_POINT('Ctrl Pts',(0.829679168999945,12.2,4.21981457999999));
#334274=CARTESIAN_POINT('Ctrl Pts',(0.829679168999945,5.2,4.21981457999999));
#334275=CARTESIAN_POINT('Ctrl Pts',(0.829679168999945,2.2,4.21981457999999));
#334276=CARTESIAN_POINT('Ctrl Pts',(0.829343820999945,12.2,4.22159173399999));
#334277=CARTESIAN_POINT('Ctrl Pts',(0.829343820999945,5.2,4.22159173399999));
#334278=CARTESIAN_POINT('Ctrl Pts',(0.829343820999945,2.2,4.22159173399999));
#334279=CARTESIAN_POINT('Ctrl Pts',(0.829005659999944,12.2,4.22337273599998));
#334280=CARTESIAN_POINT('Ctrl Pts',(0.829005659999944,5.2,4.22337273599998));
#334281=CARTESIAN_POINT('Ctrl Pts',(0.829005659999944,2.2,4.22337273599998));
#334282=CARTESIAN_POINT('Ctrl Pts',(0.828664677999944,12.2,4.22515757699998));
#334283=CARTESIAN_POINT('Ctrl Pts',(0.828664677999944,5.2,4.22515757699998));
#334284=CARTESIAN_POINT('Ctrl Pts',(0.828664677999944,2.2,4.22515757699998));
#334285=CARTESIAN_POINT('Ctrl Pts',(0.828320867999944,12.2,4.22694624699999));
#334286=CARTESIAN_POINT('Ctrl Pts',(0.828320867999944,5.2,4.22694624699999));
#334287=CARTESIAN_POINT('Ctrl Pts',(0.828320867999944,2.2,4.22694624699999));
#334288=CARTESIAN_POINT('Ctrl Pts',(0.827974222999944,12.2,4.22873873599999));
#334289=CARTESIAN_POINT('Ctrl Pts',(0.827974222999944,5.2,4.22873873599999));
#334290=CARTESIAN_POINT('Ctrl Pts',(0.827974222999944,2.2,4.22873873599999));
#334291=CARTESIAN_POINT('Ctrl Pts',(0.827624734999944,12.2,4.23053503799999));
#334292=CARTESIAN_POINT('Ctrl Pts',(0.827624734999944,5.2,4.23053503799999));
#334293=CARTESIAN_POINT('Ctrl Pts',(0.827624734999944,2.2,4.23053503799999));
#334294=CARTESIAN_POINT('Ctrl Pts',(0.827272396999944,12.2,4.23233513899999));
#334295=CARTESIAN_POINT('Ctrl Pts',(0.827272396999944,5.2,4.23233513899999));
#334296=CARTESIAN_POINT('Ctrl Pts',(0.827272396999944,2.2,4.23233513899999));
#334297=CARTESIAN_POINT('Ctrl Pts',(0.826917202999944,12.2,4.23413903399998));
#334298=CARTESIAN_POINT('Ctrl Pts',(0.826917202999944,5.2,4.23413903399998));
#334299=CARTESIAN_POINT('Ctrl Pts',(0.826917202999944,2.2,4.23413903399998));
#334300=CARTESIAN_POINT('Ctrl Pts',(0.826559144999944,12.2,4.23594671199999));
#334301=CARTESIAN_POINT('Ctrl Pts',(0.826559144999944,5.2,4.23594671199999));
#334302=CARTESIAN_POINT('Ctrl Pts',(0.826559144999944,2.2,4.23594671199999));
#334303=CARTESIAN_POINT('Ctrl Pts',(0.826198215999944,12.2,4.23775816399999));
#334304=CARTESIAN_POINT('Ctrl Pts',(0.826198215999944,5.2,4.23775816399999));
#334305=CARTESIAN_POINT('Ctrl Pts',(0.826198215999944,2.2,4.23775816399999));
#334306=CARTESIAN_POINT('Ctrl Pts',(0.825834408999944,12.2,4.23957338099999));
#334307=CARTESIAN_POINT('Ctrl Pts',(0.825834408999944,5.2,4.23957338099999));
#334308=CARTESIAN_POINT('Ctrl Pts',(0.825834408999944,2.2,4.23957338099999));
#334309=CARTESIAN_POINT('Ctrl Pts',(0.825467717999944,12.2,4.24139235399998));
#334310=CARTESIAN_POINT('Ctrl Pts',(0.825467717999944,5.2,4.24139235399998));
#334311=CARTESIAN_POINT('Ctrl Pts',(0.825467717999944,2.2,4.24139235399998));
#334312=CARTESIAN_POINT('Ctrl Pts',(0.825098134999944,12.2,4.24321507299998));
#334313=CARTESIAN_POINT('Ctrl Pts',(0.825098134999944,5.2,4.24321507299998));
#334314=CARTESIAN_POINT('Ctrl Pts',(0.825098134999944,2.2,4.24321507299998));
#334315=CARTESIAN_POINT('Ctrl Pts',(0.824725651999944,12.2,4.24504152999998));
#334316=CARTESIAN_POINT('Ctrl Pts',(0.824725651999944,5.2,4.24504152999998));
#334317=CARTESIAN_POINT('Ctrl Pts',(0.824725651999944,2.2,4.24504152999998));
#334318=CARTESIAN_POINT('Ctrl Pts',(0.824350264999943,12.2,4.24687171399999));
#334319=CARTESIAN_POINT('Ctrl Pts',(0.824350264999943,5.2,4.24687171399999));
#334320=CARTESIAN_POINT('Ctrl Pts',(0.824350264999943,2.2,4.24687171399999));
#334321=CARTESIAN_POINT('Ctrl Pts',(0.823971964999944,12.2,4.24870561699999));
#334322=CARTESIAN_POINT('Ctrl Pts',(0.823971964999944,5.2,4.24870561699999));
#334323=CARTESIAN_POINT('Ctrl Pts',(0.823971964999944,2.2,4.24870561699999));
#334324=CARTESIAN_POINT('Ctrl Pts',(0.823590743999943,12.2,4.25054322999999));
#334325=CARTESIAN_POINT('Ctrl Pts',(0.823590743999943,5.2,4.25054322999999));
#334326=CARTESIAN_POINT('Ctrl Pts',(0.823590743999943,2.2,4.25054322999999));
#334327=CARTESIAN_POINT('Ctrl Pts',(0.823206597999944,12.2,4.25238454399998));
#334328=CARTESIAN_POINT('Ctrl Pts',(0.823206597999944,5.2,4.25238454399998));
#334329=CARTESIAN_POINT('Ctrl Pts',(0.823206597999944,2.2,4.25238454399998));
#334330=CARTESIAN_POINT('Ctrl Pts',(0.822819518999944,12.2,4.25422954999998));
#334331=CARTESIAN_POINT('Ctrl Pts',(0.822819518999944,5.2,4.25422954999998));
#334332=CARTESIAN_POINT('Ctrl Pts',(0.822819518999944,2.2,4.25422954999998));
#334333=CARTESIAN_POINT('Ctrl Pts',(0.822429499999945,12.2,4.25607823699998));
#334334=CARTESIAN_POINT('Ctrl Pts',(0.822429499999945,5.2,4.25607823699998));
#334335=CARTESIAN_POINT('Ctrl Pts',(0.822429499999945,2.2,4.25607823699998));
#334336=CARTESIAN_POINT('Ctrl Pts',(0.822036533999944,12.2,4.25793059899998));
#334337=CARTESIAN_POINT('Ctrl Pts',(0.822036533999944,5.2,4.25793059899998));
#334338=CARTESIAN_POINT('Ctrl Pts',(0.822036533999944,2.2,4.25793059899998));
#334339=CARTESIAN_POINT('Ctrl Pts',(0.821640614999944,12.2,4.25978662399999));
#334340=CARTESIAN_POINT('Ctrl Pts',(0.821640614999944,5.2,4.25978662399999));
#334341=CARTESIAN_POINT('Ctrl Pts',(0.821640614999944,2.2,4.25978662399999));
#334342=CARTESIAN_POINT('Ctrl Pts',(0.821241735999945,12.2,4.26164630399998));
#334343=CARTESIAN_POINT('Ctrl Pts',(0.821241735999945,5.2,4.26164630399998));
#334344=CARTESIAN_POINT('Ctrl Pts',(0.821241735999945,2.2,4.26164630399998));
#334345=CARTESIAN_POINT('Ctrl Pts',(0.820839888999945,12.2,4.26350963099999));
#334346=CARTESIAN_POINT('Ctrl Pts',(0.820839888999945,5.2,4.26350963099999));
#334347=CARTESIAN_POINT('Ctrl Pts',(0.820839888999945,2.2,4.26350963099999));
#334348=CARTESIAN_POINT('Ctrl Pts',(0.820435068999944,12.2,4.26537659399998));
#334349=CARTESIAN_POINT('Ctrl Pts',(0.820435068999944,5.2,4.26537659399998));
#334350=CARTESIAN_POINT('Ctrl Pts',(0.820435068999944,2.2,4.26537659399998));
#334351=CARTESIAN_POINT('Ctrl Pts',(0.820027268999944,12.2,4.26724718499998));
#334352=CARTESIAN_POINT('Ctrl Pts',(0.820027268999944,5.2,4.26724718499998));
#334353=CARTESIAN_POINT('Ctrl Pts',(0.820027268999944,2.2,4.26724718499998));
#334354=CARTESIAN_POINT('Ctrl Pts',(0.819616481999944,12.2,4.26912139399998));
#334355=CARTESIAN_POINT('Ctrl Pts',(0.819616481999944,5.2,4.26912139399998));
#334356=CARTESIAN_POINT('Ctrl Pts',(0.819616481999944,2.2,4.26912139399998));
#334357=CARTESIAN_POINT('Ctrl Pts',(0.819202701999945,12.2,4.27099921299998));
#334358=CARTESIAN_POINT('Ctrl Pts',(0.819202701999945,5.2,4.27099921299998));
#334359=CARTESIAN_POINT('Ctrl Pts',(0.819202701999945,2.2,4.27099921299998));
#334360=CARTESIAN_POINT('Ctrl Pts',(0.818785921999944,12.2,4.27288063199998));
#334361=CARTESIAN_POINT('Ctrl Pts',(0.818785921999944,5.2,4.27288063199998));
#334362=CARTESIAN_POINT('Ctrl Pts',(0.818785921999944,2.2,4.27288063199998));
#334363=CARTESIAN_POINT('Ctrl Pts',(0.818366133999944,12.2,4.27476564299998));
#334364=CARTESIAN_POINT('Ctrl Pts',(0.818366133999944,5.2,4.27476564299998));
#334365=CARTESIAN_POINT('Ctrl Pts',(0.818366133999944,2.2,4.27476564299998));
#334366=CARTESIAN_POINT('Ctrl Pts',(0.817943333999944,12.2,4.27665423699998));
#334367=CARTESIAN_POINT('Ctrl Pts',(0.817943333999944,5.2,4.27665423699998));
#334368=CARTESIAN_POINT('Ctrl Pts',(0.817943333999944,2.2,4.27665423699998));
#334369=CARTESIAN_POINT('Ctrl Pts',(0.817517513999944,12.2,4.27854640299999));
#334370=CARTESIAN_POINT('Ctrl Pts',(0.817517513999944,5.2,4.27854640299999));
#334371=CARTESIAN_POINT('Ctrl Pts',(0.817517513999944,2.2,4.27854640299999));
#334372=CARTESIAN_POINT('Ctrl Pts',(0.817088667999945,12.2,4.28044213499999));
#334373=CARTESIAN_POINT('Ctrl Pts',(0.817088667999945,5.2,4.28044213499999));
#334374=CARTESIAN_POINT('Ctrl Pts',(0.817088667999945,2.2,4.28044213499999));
#334375=CARTESIAN_POINT('Ctrl Pts',(0.816656787999944,12.2,4.28234141999998));
#334376=CARTESIAN_POINT('Ctrl Pts',(0.816656787999944,5.2,4.28234141999998));
#334377=CARTESIAN_POINT('Ctrl Pts',(0.816656787999944,2.2,4.28234141999998));
#334378=CARTESIAN_POINT('Ctrl Pts',(0.816221870999944,12.2,4.28424425199999));
#334379=CARTESIAN_POINT('Ctrl Pts',(0.816221870999944,5.2,4.28424425199999));
#334380=CARTESIAN_POINT('Ctrl Pts',(0.816221870999944,2.2,4.28424425199999));
#334381=CARTESIAN_POINT('Ctrl Pts',(0.815783906999944,12.2,4.28615062199999));
#334382=CARTESIAN_POINT('Ctrl Pts',(0.815783906999944,5.2,4.28615062199999));
#334383=CARTESIAN_POINT('Ctrl Pts',(0.815783906999944,2.2,4.28615062199999));
#334384=CARTESIAN_POINT('Ctrl Pts',(0.815342891999945,12.2,4.28806051899999));
#334385=CARTESIAN_POINT('Ctrl Pts',(0.815342891999945,5.2,4.28806051899999));
#334386=CARTESIAN_POINT('Ctrl Pts',(0.815342891999945,2.2,4.28806051899999));
#334387=CARTESIAN_POINT('Ctrl Pts',(0.814898817999944,12.2,4.28997393599998));
#334388=CARTESIAN_POINT('Ctrl Pts',(0.814898817999944,5.2,4.28997393599998));
#334389=CARTESIAN_POINT('Ctrl Pts',(0.814898817999944,2.2,4.28997393599998));
#334390=CARTESIAN_POINT('Ctrl Pts',(0.814451678999945,12.2,4.29189086099999));
#334391=CARTESIAN_POINT('Ctrl Pts',(0.814451678999945,5.2,4.29189086099999));
#334392=CARTESIAN_POINT('Ctrl Pts',(0.814451678999945,2.2,4.29189086099999));
#334393=CARTESIAN_POINT('Ctrl Pts',(0.814001469999944,12.2,4.29381128899998));
#334394=CARTESIAN_POINT('Ctrl Pts',(0.814001469999944,5.2,4.29381128899998));
#334395=CARTESIAN_POINT('Ctrl Pts',(0.814001469999944,2.2,4.29381128899998));
#334396=CARTESIAN_POINT('Ctrl Pts',(0.813548181999945,12.2,4.29573520799998));
#334397=CARTESIAN_POINT('Ctrl Pts',(0.813548181999945,5.2,4.29573520799998));
#334398=CARTESIAN_POINT('Ctrl Pts',(0.813548181999945,2.2,4.29573520799998));
#334399=CARTESIAN_POINT('Ctrl Pts',(0.813091811999944,12.2,4.29766260999998));
#334400=CARTESIAN_POINT('Ctrl Pts',(0.813091811999944,5.2,4.29766260999998));
#334401=CARTESIAN_POINT('Ctrl Pts',(0.813091811999944,2.2,4.29766260999998));
#334402=CARTESIAN_POINT('Ctrl Pts',(0.812632351999943,12.2,4.29959348699998));
#334403=CARTESIAN_POINT('Ctrl Pts',(0.812632351999943,5.2,4.29959348699998));
#334404=CARTESIAN_POINT('Ctrl Pts',(0.812632351999943,2.2,4.29959348699998));
#334405=CARTESIAN_POINT('Ctrl Pts',(0.812169794999944,12.2,4.30152782799999));
#334406=CARTESIAN_POINT('Ctrl Pts',(0.812169794999944,5.2,4.30152782799999));
#334407=CARTESIAN_POINT('Ctrl Pts',(0.812169794999944,2.2,4.30152782799999));
#334408=CARTESIAN_POINT('Ctrl Pts',(0.811704135999943,12.2,4.30346562599999));
#334409=CARTESIAN_POINT('Ctrl Pts',(0.811704135999943,5.2,4.30346562599999));
#334410=CARTESIAN_POINT('Ctrl Pts',(0.811704135999943,2.2,4.30346562599999));
#334411=CARTESIAN_POINT('Ctrl Pts',(0.811235367999944,12.2,4.30540686999999));
#334412=CARTESIAN_POINT('Ctrl Pts',(0.811235367999944,5.2,4.30540686999999));
#334413=CARTESIAN_POINT('Ctrl Pts',(0.811235367999944,2.2,4.30540686999999));
#334414=CARTESIAN_POINT('Ctrl Pts',(0.810763485999945,12.2,4.30735155199999));
#334415=CARTESIAN_POINT('Ctrl Pts',(0.810763485999945,5.2,4.30735155199999));
#334416=CARTESIAN_POINT('Ctrl Pts',(0.810763485999945,2.2,4.30735155199999));
#334417=CARTESIAN_POINT('Ctrl Pts',(0.810288482999945,12.2,4.30929966499999));
#334418=CARTESIAN_POINT('Ctrl Pts',(0.810288482999945,5.2,4.30929966499999));
#334419=CARTESIAN_POINT('Ctrl Pts',(0.810288482999945,2.2,4.30929966499999));
#334420=CARTESIAN_POINT('Ctrl Pts',(0.809810351999943,12.2,4.31125119599999));
#334421=CARTESIAN_POINT('Ctrl Pts',(0.809810351999943,5.2,4.31125119599999));
#334422=CARTESIAN_POINT('Ctrl Pts',(0.809810351999943,2.2,4.31125119599999));
#334423=CARTESIAN_POINT('Ctrl Pts',(0.809329088999945,12.2,4.31320613999999));
#334424=CARTESIAN_POINT('Ctrl Pts',(0.809329088999945,5.2,4.31320613999999));
#334425=CARTESIAN_POINT('Ctrl Pts',(0.809329088999945,2.2,4.31320613999999));
#334426=CARTESIAN_POINT('Ctrl Pts',(0.808844685999944,12.2,4.31516448499998));
#334427=CARTESIAN_POINT('Ctrl Pts',(0.808844685999944,5.2,4.31516448499998));
#334428=CARTESIAN_POINT('Ctrl Pts',(0.808844685999944,2.2,4.31516448499998));
#334429=CARTESIAN_POINT('Ctrl Pts',(0.808357137999944,12.2,4.31712622399999));
#334430=CARTESIAN_POINT('Ctrl Pts',(0.808357137999944,5.2,4.31712622399999));
#334431=CARTESIAN_POINT('Ctrl Pts',(0.808357137999944,2.2,4.31712622399999));
#334432=CARTESIAN_POINT('Ctrl Pts',(0.807866437999943,12.2,4.31909134599999));
#334433=CARTESIAN_POINT('Ctrl Pts',(0.807866437999943,5.2,4.31909134599999));
#334434=CARTESIAN_POINT('Ctrl Pts',(0.807866437999943,2.2,4.31909134599999));
#334435=CARTESIAN_POINT('Ctrl Pts',(0.807372581999944,12.2,4.32105984499999));
#334436=CARTESIAN_POINT('Ctrl Pts',(0.807372581999944,5.2,4.32105984499999));
#334437=CARTESIAN_POINT('Ctrl Pts',(0.807372581999944,2.2,4.32105984499999));
#334438=CARTESIAN_POINT('Ctrl Pts',(0.806875560999945,12.2,4.32303170999998));
#334439=CARTESIAN_POINT('Ctrl Pts',(0.806875560999945,5.2,4.32303170999998));
#334440=CARTESIAN_POINT('Ctrl Pts',(0.806875560999945,2.2,4.32303170999998));
#334441=CARTESIAN_POINT('Ctrl Pts',(0.806375370999944,12.2,4.32500693299998));
#334442=CARTESIAN_POINT('Ctrl Pts',(0.806375370999944,5.2,4.32500693299998));
#334443=CARTESIAN_POINT('Ctrl Pts',(0.806375370999944,2.2,4.32500693299998));
#334444=CARTESIAN_POINT('Ctrl Pts',(0.805872006999944,12.2,4.32698550299998));
#334445=CARTESIAN_POINT('Ctrl Pts',(0.805872006999944,5.2,4.32698550299998));
#334446=CARTESIAN_POINT('Ctrl Pts',(0.805872006999944,2.2,4.32698550299998));
#334447=CARTESIAN_POINT('Ctrl Pts',(0.805365458999944,12.2,4.32896741499999));
#334448=CARTESIAN_POINT('Ctrl Pts',(0.805365458999944,5.2,4.32896741499999));
#334449=CARTESIAN_POINT('Ctrl Pts',(0.805365458999944,2.2,4.32896741499999));
#334450=CARTESIAN_POINT('Ctrl Pts',(0.804855725999943,12.2,4.33095265599999));
#334451=CARTESIAN_POINT('Ctrl Pts',(0.804855725999943,5.2,4.33095265599999));
#334452=CARTESIAN_POINT('Ctrl Pts',(0.804855725999943,2.2,4.33095265599999));
#334453=CARTESIAN_POINT('Ctrl Pts',(0.804342799999944,12.2,4.33294121999998));
#334454=CARTESIAN_POINT('Ctrl Pts',(0.804342799999944,5.2,4.33294121999998));
#334455=CARTESIAN_POINT('Ctrl Pts',(0.804342799999944,2.2,4.33294121999998));
#334456=CARTESIAN_POINT('Ctrl Pts',(0.803826673999944,12.2,4.33493309799999));
#334457=CARTESIAN_POINT('Ctrl Pts',(0.803826673999944,5.2,4.33493309799999));
#334458=CARTESIAN_POINT('Ctrl Pts',(0.803826673999944,2.2,4.33493309799999));
#334459=CARTESIAN_POINT('Ctrl Pts',(0.803307342999945,12.2,4.33692827799998));
#334460=CARTESIAN_POINT('Ctrl Pts',(0.803307342999945,5.2,4.33692827799998));
#334461=CARTESIAN_POINT('Ctrl Pts',(0.803307342999945,2.2,4.33692827799998));
#334462=CARTESIAN_POINT('Ctrl Pts',(0.802784801999944,12.2,4.33892675499998));
#334463=CARTESIAN_POINT('Ctrl Pts',(0.802784801999944,5.2,4.33892675499998));
#334464=CARTESIAN_POINT('Ctrl Pts',(0.802784801999944,2.2,4.33892675499998));
#334465=CARTESIAN_POINT('Ctrl Pts',(0.802259043999943,12.2,4.34092851799999));
#334466=CARTESIAN_POINT('Ctrl Pts',(0.802259043999943,5.2,4.34092851799999));
#334467=CARTESIAN_POINT('Ctrl Pts',(0.802259043999943,2.2,4.34092851799999));
#334468=CARTESIAN_POINT('Ctrl Pts',(0.801730063999945,12.2,4.34293355899998));
#334469=CARTESIAN_POINT('Ctrl Pts',(0.801730063999945,5.2,4.34293355899998));
#334470=CARTESIAN_POINT('Ctrl Pts',(0.801730063999945,2.2,4.34293355899998));
#334471=CARTESIAN_POINT('Ctrl Pts',(0.801197855999944,12.2,4.34494186799999));
#334472=CARTESIAN_POINT('Ctrl Pts',(0.801197855999944,5.2,4.34494186799999));
#334473=CARTESIAN_POINT('Ctrl Pts',(0.801197855999944,2.2,4.34494186799999));
#334474=CARTESIAN_POINT('Ctrl Pts',(0.800662413999944,12.2,4.34695343699998));
#334475=CARTESIAN_POINT('Ctrl Pts',(0.800662413999944,5.2,4.34695343699998));
#334476=CARTESIAN_POINT('Ctrl Pts',(0.800662413999944,2.2,4.34695343699998));
#334477=CARTESIAN_POINT('Ctrl Pts',(0.800123732999943,12.2,4.34896825699998));
#334478=CARTESIAN_POINT('Ctrl Pts',(0.800123732999943,5.2,4.34896825699998));
#334479=CARTESIAN_POINT('Ctrl Pts',(0.800123732999943,2.2,4.34896825699998));
#334480=CARTESIAN_POINT('Ctrl Pts',(0.799581806999944,12.2,4.35098631899999));
#334481=CARTESIAN_POINT('Ctrl Pts',(0.799581806999944,5.2,4.35098631899999));
#334482=CARTESIAN_POINT('Ctrl Pts',(0.799581806999944,2.2,4.35098631899999));
#334483=CARTESIAN_POINT('Ctrl Pts',(0.799036627999944,12.2,4.35300761599999));
#334484=CARTESIAN_POINT('Ctrl Pts',(0.799036627999944,5.2,4.35300761599999));
#334485=CARTESIAN_POINT('Ctrl Pts',(0.799036627999944,2.2,4.35300761599999));
#334486=CARTESIAN_POINT('Ctrl Pts',(0.798488193999944,12.2,4.35503213599999));
#334487=CARTESIAN_POINT('Ctrl Pts',(0.798488193999944,5.2,4.35503213599999));
#334488=CARTESIAN_POINT('Ctrl Pts',(0.798488193999944,2.2,4.35503213599999));
#334489=CARTESIAN_POINT('Ctrl Pts',(0.797936496999945,12.2,4.35705987099999));
#334490=CARTESIAN_POINT('Ctrl Pts',(0.797936496999945,5.2,4.35705987099999));
#334491=CARTESIAN_POINT('Ctrl Pts',(0.797936496999945,2.2,4.35705987099999));
#334492=CARTESIAN_POINT('Ctrl Pts',(0.797381532999945,12.2,4.35909081499998));
#334493=CARTESIAN_POINT('Ctrl Pts',(0.797381532999945,5.2,4.35909081499998));
#334494=CARTESIAN_POINT('Ctrl Pts',(0.797381532999945,2.2,4.35909081499998));
#334495=CARTESIAN_POINT('Ctrl Pts',(0.796823294999944,12.2,4.36112495599998));
#334496=CARTESIAN_POINT('Ctrl Pts',(0.796823294999944,5.2,4.36112495599998));
#334497=CARTESIAN_POINT('Ctrl Pts',(0.796823294999944,2.2,4.36112495599998));
#334498=CARTESIAN_POINT('Ctrl Pts',(0.796261777999944,12.2,4.36316228499999));
#334499=CARTESIAN_POINT('Ctrl Pts',(0.796261777999944,5.2,4.36316228499999));
#334500=CARTESIAN_POINT('Ctrl Pts',(0.796261777999944,2.2,4.36316228499999));
#334501=CARTESIAN_POINT('Ctrl Pts',(0.795696975999944,12.2,4.36520279599999));
#334502=CARTESIAN_POINT('Ctrl Pts',(0.795696975999944,5.2,4.36520279599999));
#334503=CARTESIAN_POINT('Ctrl Pts',(0.795696975999944,2.2,4.36520279599999));
#334504=CARTESIAN_POINT('Ctrl Pts',(0.795128884999944,12.2,4.36724647799998));
#334505=CARTESIAN_POINT('Ctrl Pts',(0.795128884999944,5.2,4.36724647799998));
#334506=CARTESIAN_POINT('Ctrl Pts',(0.795128884999944,2.2,4.36724647799998));
#334507=CARTESIAN_POINT('Ctrl Pts',(0.794557497999944,12.2,4.36929332299999));
#334508=CARTESIAN_POINT('Ctrl Pts',(0.794557497999944,5.2,4.36929332299999));
#334509=CARTESIAN_POINT('Ctrl Pts',(0.794557497999944,2.2,4.36929332299999));
#334510=CARTESIAN_POINT('Ctrl Pts',(0.793982808999945,12.2,4.37134332199999));
#334511=CARTESIAN_POINT('Ctrl Pts',(0.793982808999945,5.2,4.37134332199999));
#334512=CARTESIAN_POINT('Ctrl Pts',(0.793982808999945,2.2,4.37134332199999));
#334513=CARTESIAN_POINT('Ctrl Pts',(0.793404813999944,12.2,4.37339646599998));
#334514=CARTESIAN_POINT('Ctrl Pts',(0.793404813999944,5.2,4.37339646599998));
#334515=CARTESIAN_POINT('Ctrl Pts',(0.793404813999944,2.2,4.37339646599998));
#334516=CARTESIAN_POINT('Ctrl Pts',(0.792823505999943,12.2,4.37545274699998));
#334517=CARTESIAN_POINT('Ctrl Pts',(0.792823505999943,5.2,4.37545274699998));
#334518=CARTESIAN_POINT('Ctrl Pts',(0.792823505999943,2.2,4.37545274699998));
#334519=CARTESIAN_POINT('Ctrl Pts',(0.792238880999945,12.2,4.37751215499999));
#334520=CARTESIAN_POINT('Ctrl Pts',(0.792238880999945,5.2,4.37751215499999));
#334521=CARTESIAN_POINT('Ctrl Pts',(0.792238880999945,2.2,4.37751215499999));
#334522=CARTESIAN_POINT('Ctrl Pts',(0.791650932999944,12.2,4.37957468199999));
#334523=CARTESIAN_POINT('Ctrl Pts',(0.791650932999944,5.2,4.37957468199999));
#334524=CARTESIAN_POINT('Ctrl Pts',(0.791650932999944,2.2,4.37957468199999));
#334525=CARTESIAN_POINT('Ctrl Pts',(0.791059655999944,12.2,4.38164031999998));
#334526=CARTESIAN_POINT('Ctrl Pts',(0.791059655999944,5.2,4.38164031999998));
#334527=CARTESIAN_POINT('Ctrl Pts',(0.791059655999944,2.2,4.38164031999998));
#334528=CARTESIAN_POINT('Ctrl Pts',(0.790465045999944,12.2,4.38370905999999));
#334529=CARTESIAN_POINT('Ctrl Pts',(0.790465045999944,5.2,4.38370905999999));
#334530=CARTESIAN_POINT('Ctrl Pts',(0.790465045999944,2.2,4.38370905999999));
#334531=CARTESIAN_POINT('Ctrl Pts',(0.789867097999944,12.2,4.38578089099998));
#334532=CARTESIAN_POINT('Ctrl Pts',(0.789867097999944,5.2,4.38578089099998));
#334533=CARTESIAN_POINT('Ctrl Pts',(0.789867097999944,2.2,4.38578089099998));
#334534=CARTESIAN_POINT('Ctrl Pts',(0.789265802999944,12.2,4.38785580699999));
#334535=CARTESIAN_POINT('Ctrl Pts',(0.789265802999944,5.2,4.38785580699999));
#334536=CARTESIAN_POINT('Ctrl Pts',(0.789265802999944,2.2,4.38785580699999));
#334537=CARTESIAN_POINT('Ctrl Pts',(0.788661159999945,12.2,4.38993379799999));
#334538=CARTESIAN_POINT('Ctrl Pts',(0.788661159999945,5.2,4.38993379799999));
#334539=CARTESIAN_POINT('Ctrl Pts',(0.788661159999945,2.2,4.38993379799999));
#334540=CARTESIAN_POINT('Ctrl Pts',(0.788053160999944,12.2,4.39201485499999));
#334541=CARTESIAN_POINT('Ctrl Pts',(0.788053160999944,5.2,4.39201485499999));
#334542=CARTESIAN_POINT('Ctrl Pts',(0.788053160999944,2.2,4.39201485499999));
#334543=CARTESIAN_POINT('Ctrl Pts',(0.787441801999944,12.2,4.39409896999998));
#334544=CARTESIAN_POINT('Ctrl Pts',(0.787441801999944,5.2,4.39409896999998));
#334545=CARTESIAN_POINT('Ctrl Pts',(0.787441801999944,2.2,4.39409896999998));
#334546=CARTESIAN_POINT('Ctrl Pts',(0.786827076999944,12.2,4.39618613399999));
#334547=CARTESIAN_POINT('Ctrl Pts',(0.786827076999944,5.2,4.39618613399999));
#334548=CARTESIAN_POINT('Ctrl Pts',(0.786827076999944,2.2,4.39618613399999));
#334549=CARTESIAN_POINT('Ctrl Pts',(0.786208980999944,12.2,4.39827633899998));
#334550=CARTESIAN_POINT('Ctrl Pts',(0.786208980999944,5.2,4.39827633899998));
#334551=CARTESIAN_POINT('Ctrl Pts',(0.786208980999944,2.2,4.39827633899998));
#334552=CARTESIAN_POINT('Ctrl Pts',(0.785587508999944,12.2,4.40036957499998));
#334553=CARTESIAN_POINT('Ctrl Pts',(0.785587508999944,5.2,4.40036957499998));
#334554=CARTESIAN_POINT('Ctrl Pts',(0.785587508999944,2.2,4.40036957499998));
#334555=CARTESIAN_POINT('Ctrl Pts',(0.784962655999945,12.2,4.40246583399999));
#334556=CARTESIAN_POINT('Ctrl Pts',(0.784962655999945,5.2,4.40246583399999));
#334557=CARTESIAN_POINT('Ctrl Pts',(0.784962655999945,2.2,4.40246583399999));
#334558=CARTESIAN_POINT('Ctrl Pts',(0.784334416999944,12.2,4.40456510699998));
#334559=CARTESIAN_POINT('Ctrl Pts',(0.784334416999944,5.2,4.40456510699998));
#334560=CARTESIAN_POINT('Ctrl Pts',(0.784334416999944,2.2,4.40456510699998));
#334561=CARTESIAN_POINT('Ctrl Pts',(0.783702784999945,12.2,4.40666738599998));
#334562=CARTESIAN_POINT('Ctrl Pts',(0.783702784999945,5.2,4.40666738599998));
#334563=CARTESIAN_POINT('Ctrl Pts',(0.783702784999945,2.2,4.40666738599998));
#334564=CARTESIAN_POINT('Ctrl Pts',(0.783067756999943,12.2,4.40877266199998));
#334565=CARTESIAN_POINT('Ctrl Pts',(0.783067756999943,5.2,4.40877266199998));
#334566=CARTESIAN_POINT('Ctrl Pts',(0.783067756999943,2.2,4.40877266199998));
#334567=CARTESIAN_POINT('Ctrl Pts',(0.782429326999944,12.2,4.41088092599998));
#334568=CARTESIAN_POINT('Ctrl Pts',(0.782429326999944,5.2,4.41088092599998));
#334569=CARTESIAN_POINT('Ctrl Pts',(0.782429326999944,2.2,4.41088092599998));
#334570=CARTESIAN_POINT('Ctrl Pts',(0.781787488999944,12.2,4.41299216899999));
#334571=CARTESIAN_POINT('Ctrl Pts',(0.781787488999944,5.2,4.41299216899999));
#334572=CARTESIAN_POINT('Ctrl Pts',(0.781787488999944,2.2,4.41299216899999));
#334573=CARTESIAN_POINT('Ctrl Pts',(0.781142240999944,12.2,4.41510638199999));
#334574=CARTESIAN_POINT('Ctrl Pts',(0.781142240999944,5.2,4.41510638199999));
#334575=CARTESIAN_POINT('Ctrl Pts',(0.781142240999944,2.2,4.41510638199999));
#334576=CARTESIAN_POINT('Ctrl Pts',(0.780493573999944,12.2,4.41722355899999));
#334577=CARTESIAN_POINT('Ctrl Pts',(0.780493573999944,5.2,4.41722355899999));
#334578=CARTESIAN_POINT('Ctrl Pts',(0.780493573999944,2.2,4.41722355899999));
#334579=CARTESIAN_POINT('Ctrl Pts',(0.779841484999944,12.2,4.41934368899998));
#334580=CARTESIAN_POINT('Ctrl Pts',(0.779841484999944,5.2,4.41934368899998));
#334581=CARTESIAN_POINT('Ctrl Pts',(0.779841484999944,2.2,4.41934368899998));
#334582=CARTESIAN_POINT('Ctrl Pts',(0.779185969999945,12.2,4.42146676299998));
#334583=CARTESIAN_POINT('Ctrl Pts',(0.779185969999945,5.2,4.42146676299998));
#334584=CARTESIAN_POINT('Ctrl Pts',(0.779185969999945,2.2,4.42146676299998));
#334585=CARTESIAN_POINT('Ctrl Pts',(0.778527020999944,12.2,4.42359277399999));
#334586=CARTESIAN_POINT('Ctrl Pts',(0.778527020999944,5.2,4.42359277399999));
#334587=CARTESIAN_POINT('Ctrl Pts',(0.778527020999944,2.2,4.42359277399999));
#334588=CARTESIAN_POINT('Ctrl Pts',(0.777864634999944,12.2,4.42572171199998));
#334589=CARTESIAN_POINT('Ctrl Pts',(0.777864634999944,5.2,4.42572171199998));
#334590=CARTESIAN_POINT('Ctrl Pts',(0.777864634999944,2.2,4.42572171199998));
#334591=CARTESIAN_POINT('Ctrl Pts',(0.777198807999944,12.2,4.42785356899999));
#334592=CARTESIAN_POINT('Ctrl Pts',(0.777198807999944,5.2,4.42785356899999));
#334593=CARTESIAN_POINT('Ctrl Pts',(0.777198807999944,2.2,4.42785356899999));
#334594=CARTESIAN_POINT('Ctrl Pts',(0.776529531999944,12.2,4.42998833699999));
#334595=CARTESIAN_POINT('Ctrl Pts',(0.776529531999944,5.2,4.42998833699999));
#334596=CARTESIAN_POINT('Ctrl Pts',(0.776529531999944,2.2,4.42998833699999));
#334597=CARTESIAN_POINT('Ctrl Pts',(0.775856804999945,12.2,4.43212600599999));
#334598=CARTESIAN_POINT('Ctrl Pts',(0.775856804999945,5.2,4.43212600599999));
#334599=CARTESIAN_POINT('Ctrl Pts',(0.775856804999945,2.2,4.43212600599999));
#334600=CARTESIAN_POINT('Ctrl Pts',(0.775180620999943,12.2,4.43426656799998));
#334601=CARTESIAN_POINT('Ctrl Pts',(0.775180620999943,5.2,4.43426656799998));
#334602=CARTESIAN_POINT('Ctrl Pts',(0.775180620999943,2.2,4.43426656799998));
#334603=CARTESIAN_POINT('Ctrl Pts',(0.774500973999944,12.2,4.43641001499999));
#334604=CARTESIAN_POINT('Ctrl Pts',(0.774500973999944,5.2,4.43641001499999));
#334605=CARTESIAN_POINT('Ctrl Pts',(0.774500973999944,2.2,4.43641001499999));
#334606=CARTESIAN_POINT('Ctrl Pts',(0.773817860999944,12.2,4.43855633799998));
#334607=CARTESIAN_POINT('Ctrl Pts',(0.773817860999944,5.2,4.43855633799998));
#334608=CARTESIAN_POINT('Ctrl Pts',(0.773817860999944,2.2,4.43855633799998));
#334609=CARTESIAN_POINT('Ctrl Pts',(0.773131275999944,12.2,4.44070552699999));
#334610=CARTESIAN_POINT('Ctrl Pts',(0.773131275999944,5.2,4.44070552699999));
#334611=CARTESIAN_POINT('Ctrl Pts',(0.773131275999944,2.2,4.44070552699999));
#334612=CARTESIAN_POINT('Ctrl Pts',(0.772441214999944,12.2,4.44285757499999));
#334613=CARTESIAN_POINT('Ctrl Pts',(0.772441214999944,5.2,4.44285757499999));
#334614=CARTESIAN_POINT('Ctrl Pts',(0.772441214999944,2.2,4.44285757499999));
#334615=CARTESIAN_POINT('Ctrl Pts',(0.771747671999944,12.2,4.44501247299999));
#334616=CARTESIAN_POINT('Ctrl Pts',(0.771747671999944,5.2,4.44501247299999));
#334617=CARTESIAN_POINT('Ctrl Pts',(0.771747671999944,2.2,4.44501247299999));
#334618=CARTESIAN_POINT('Ctrl Pts',(0.771050642999944,12.2,4.44717021199998));
#334619=CARTESIAN_POINT('Ctrl Pts',(0.771050642999944,5.2,4.44717021199998));
#334620=CARTESIAN_POINT('Ctrl Pts',(0.771050642999944,2.2,4.44717021199998));
#334621=CARTESIAN_POINT('Ctrl Pts',(0.770350122999944,12.2,4.44933078499999));
#334622=CARTESIAN_POINT('Ctrl Pts',(0.770350122999944,5.2,4.44933078499999));
#334623=CARTESIAN_POINT('Ctrl Pts',(0.770350122999944,2.2,4.44933078499999));
#334624=CARTESIAN_POINT('Ctrl Pts',(0.769646107999944,12.2,4.45149418099999));
#334625=CARTESIAN_POINT('Ctrl Pts',(0.769646107999944,5.2,4.45149418099999));
#334626=CARTESIAN_POINT('Ctrl Pts',(0.769646107999944,2.2,4.45149418099999));
#334627=CARTESIAN_POINT('Ctrl Pts',(0.768938590999944,12.2,4.45366039399998));
#334628=CARTESIAN_POINT('Ctrl Pts',(0.768938590999944,5.2,4.45366039399998));
#334629=CARTESIAN_POINT('Ctrl Pts',(0.768938590999944,2.2,4.45366039399998));
#334630=CARTESIAN_POINT('Ctrl Pts',(0.768227569999944,12.2,4.45582941299998));
#334631=CARTESIAN_POINT('Ctrl Pts',(0.768227569999944,5.2,4.45582941299998));
#334632=CARTESIAN_POINT('Ctrl Pts',(0.768227569999944,2.2,4.45582941299998));
#334633=CARTESIAN_POINT('Ctrl Pts',(0.767513038999944,12.2,4.45800123099998));
#334634=CARTESIAN_POINT('Ctrl Pts',(0.767513038999944,5.2,4.45800123099998));
#334635=CARTESIAN_POINT('Ctrl Pts',(0.767513038999944,2.2,4.45800123099998));
#334636=CARTESIAN_POINT('Ctrl Pts',(0.766794991999945,12.2,4.46017583899998));
#334637=CARTESIAN_POINT('Ctrl Pts',(0.766794991999945,5.2,4.46017583899998));
#334638=CARTESIAN_POINT('Ctrl Pts',(0.766794991999945,2.2,4.46017583899998));
#334639=CARTESIAN_POINT('Ctrl Pts',(0.766073427999945,12.2,4.46235322799998));
#334640=CARTESIAN_POINT('Ctrl Pts',(0.766073427999945,5.2,4.46235322799998));
#334641=CARTESIAN_POINT('Ctrl Pts',(0.766073427999945,2.2,4.46235322799998));
#334642=CARTESIAN_POINT('Ctrl Pts',(0.765348338999944,12.2,4.46453339099998));
#334643=CARTESIAN_POINT('Ctrl Pts',(0.765348338999944,5.2,4.46453339099998));
#334644=CARTESIAN_POINT('Ctrl Pts',(0.765348338999944,2.2,4.46453339099998));
#334645=CARTESIAN_POINT('Ctrl Pts',(0.764619720999944,12.2,4.46671631799998));
#334646=CARTESIAN_POINT('Ctrl Pts',(0.764619720999944,5.2,4.46671631799998));
#334647=CARTESIAN_POINT('Ctrl Pts',(0.764619720999944,2.2,4.46671631799998));
#334648=CARTESIAN_POINT('Ctrl Pts',(0.763887570999944,12.2,4.46890199999999));
#334649=CARTESIAN_POINT('Ctrl Pts',(0.763887570999944,5.2,4.46890199999999));
#334650=CARTESIAN_POINT('Ctrl Pts',(0.763887570999944,2.2,4.46890199999999));
#334651=CARTESIAN_POINT('Ctrl Pts',(0.763151880999944,12.2,4.47109042999998));
#334652=CARTESIAN_POINT('Ctrl Pts',(0.763151880999944,5.2,4.47109042999998));
#334653=CARTESIAN_POINT('Ctrl Pts',(0.763151880999944,2.2,4.47109042999998));
#334654=CARTESIAN_POINT('Ctrl Pts',(0.762412649999944,12.2,4.47328159899998));
#334655=CARTESIAN_POINT('Ctrl Pts',(0.762412649999944,5.2,4.47328159899998));
#334656=CARTESIAN_POINT('Ctrl Pts',(0.762412649999944,2.2,4.47328159899998));
#334657=CARTESIAN_POINT('Ctrl Pts',(0.761669871999944,12.2,4.47547549799998));
#334658=CARTESIAN_POINT('Ctrl Pts',(0.761669871999944,5.2,4.47547549799998));
#334659=CARTESIAN_POINT('Ctrl Pts',(0.761669871999944,2.2,4.47547549799998));
#334660=CARTESIAN_POINT('Ctrl Pts',(0.760923542999944,12.2,4.47767211899999));
#334661=CARTESIAN_POINT('Ctrl Pts',(0.760923542999944,5.2,4.47767211899999));
#334662=CARTESIAN_POINT('Ctrl Pts',(0.760923542999944,2.2,4.47767211899999));
#334663=CARTESIAN_POINT('Ctrl Pts',(0.760173656999944,12.2,4.47987145299999));
#334664=CARTESIAN_POINT('Ctrl Pts',(0.760173656999944,5.2,4.47987145299999));
#334665=CARTESIAN_POINT('Ctrl Pts',(0.760173656999944,2.2,4.47987145299999));
#334666=CARTESIAN_POINT('Ctrl Pts',(0.759420210999945,12.2,4.48207349099999));
#334667=CARTESIAN_POINT('Ctrl Pts',(0.759420210999945,5.2,4.48207349099999));
#334668=CARTESIAN_POINT('Ctrl Pts',(0.759420210999945,2.2,4.48207349099999));
#334669=CARTESIAN_POINT('Ctrl Pts',(0.758663198999944,12.2,4.48427822699998));
#334670=CARTESIAN_POINT('Ctrl Pts',(0.758663198999944,5.2,4.48427822699998));
#334671=CARTESIAN_POINT('Ctrl Pts',(0.758663198999944,2.2,4.48427822699998));
#334672=CARTESIAN_POINT('Ctrl Pts',(0.757902617999945,12.2,4.48648564999999));
#334673=CARTESIAN_POINT('Ctrl Pts',(0.757902617999945,5.2,4.48648564999999));
#334674=CARTESIAN_POINT('Ctrl Pts',(0.757902617999945,2.2,4.48648564999999));
#334675=CARTESIAN_POINT('Ctrl Pts',(0.757138463999943,12.2,4.48869575199998));
#334676=CARTESIAN_POINT('Ctrl Pts',(0.757138463999943,5.2,4.48869575199998));
#334677=CARTESIAN_POINT('Ctrl Pts',(0.757138463999943,2.2,4.48869575199998));
#334678=CARTESIAN_POINT('Ctrl Pts',(0.756370729999943,12.2,4.49090852399999));
#334679=CARTESIAN_POINT('Ctrl Pts',(0.756370729999943,5.2,4.49090852399999));
#334680=CARTESIAN_POINT('Ctrl Pts',(0.756370729999943,2.2,4.49090852399999));
#334681=CARTESIAN_POINT('Ctrl Pts',(0.755599414999945,12.2,4.49312395999999));
#334682=CARTESIAN_POINT('Ctrl Pts',(0.755599414999945,5.2,4.49312395999999));
#334683=CARTESIAN_POINT('Ctrl Pts',(0.755599414999945,2.2,4.49312395999999));
#334684=CARTESIAN_POINT('Ctrl Pts',(0.754824510999944,12.2,4.49534204999999));
#334685=CARTESIAN_POINT('Ctrl Pts',(0.754824510999944,5.2,4.49534204999999));
#334686=CARTESIAN_POINT('Ctrl Pts',(0.754824510999944,2.2,4.49534204999999));
#334687=CARTESIAN_POINT('Ctrl Pts',(0.754046015999944,12.2,4.49756278299999));
#334688=CARTESIAN_POINT('Ctrl Pts',(0.754046015999944,5.2,4.49756278299999));
#334689=CARTESIAN_POINT('Ctrl Pts',(0.754046015999944,2.2,4.49756278299999));
#334690=CARTESIAN_POINT('Ctrl Pts',(0.753263923999944,12.2,4.49978615499998));
#334691=CARTESIAN_POINT('Ctrl Pts',(0.753263923999944,5.2,4.49978615499998));
#334692=CARTESIAN_POINT('Ctrl Pts',(0.753263923999944,2.2,4.49978615499998));
#334693=CARTESIAN_POINT('Ctrl Pts',(0.752478233999944,12.2,4.50201215499998));
#334694=CARTESIAN_POINT('Ctrl Pts',(0.752478233999944,5.2,4.50201215499998));
#334695=CARTESIAN_POINT('Ctrl Pts',(0.752478233999944,2.2,4.50201215499998));
#334696=CARTESIAN_POINT('Ctrl Pts',(0.751688936999945,12.2,4.50424077499999));
#334697=CARTESIAN_POINT('Ctrl Pts',(0.751688936999945,5.2,4.50424077499999));
#334698=CARTESIAN_POINT('Ctrl Pts',(0.751688936999945,2.2,4.50424077499999));
#334699=CARTESIAN_POINT('Ctrl Pts',(0.750896031999945,12.2,4.50647200599998));
#334700=CARTESIAN_POINT('Ctrl Pts',(0.750896031999945,5.2,4.50647200599998));
#334701=CARTESIAN_POINT('Ctrl Pts',(0.750896031999945,2.2,4.50647200599998));
#334702=CARTESIAN_POINT('Ctrl Pts',(0.750099512999944,12.2,4.50870584099999));
#334703=CARTESIAN_POINT('Ctrl Pts',(0.750099512999944,5.2,4.50870584099999));
#334704=CARTESIAN_POINT('Ctrl Pts',(0.750099512999944,2.2,4.50870584099999));
#334705=CARTESIAN_POINT('Ctrl Pts',(0.749299376999945,12.2,4.51094227099999));
#334706=CARTESIAN_POINT('Ctrl Pts',(0.749299376999945,5.2,4.51094227099999));
#334707=CARTESIAN_POINT('Ctrl Pts',(0.749299376999945,2.2,4.51094227099999));
#334708=CARTESIAN_POINT('Ctrl Pts',(0.748495618999944,12.2,4.51318128699998));
#334709=CARTESIAN_POINT('Ctrl Pts',(0.748495618999944,5.2,4.51318128699998));
#334710=CARTESIAN_POINT('Ctrl Pts',(0.748495618999944,2.2,4.51318128699998));
#334711=CARTESIAN_POINT('Ctrl Pts',(0.747688233999945,12.2,4.51542287999998));
#334712=CARTESIAN_POINT('Ctrl Pts',(0.747688233999945,5.2,4.51542287999998));
#334713=CARTESIAN_POINT('Ctrl Pts',(0.747688233999945,2.2,4.51542287999998));
#334714=CARTESIAN_POINT('Ctrl Pts',(0.746877218999944,12.2,4.51766704299998));
#334715=CARTESIAN_POINT('Ctrl Pts',(0.746877218999944,5.2,4.51766704299998));
#334716=CARTESIAN_POINT('Ctrl Pts',(0.746877218999944,2.2,4.51766704299998));
#334717=CARTESIAN_POINT('Ctrl Pts',(0.746062569999945,12.2,4.51991376699999));
#334718=CARTESIAN_POINT('Ctrl Pts',(0.746062569999945,5.2,4.51991376699999));
#334719=CARTESIAN_POINT('Ctrl Pts',(0.746062569999945,2.2,4.51991376699999));
#334720=CARTESIAN_POINT('Ctrl Pts',(0.745244281999944,12.2,4.52216304399998));
#334721=CARTESIAN_POINT('Ctrl Pts',(0.745244281999944,5.2,4.52216304399998));
#334722=CARTESIAN_POINT('Ctrl Pts',(0.745244281999944,2.2,4.52216304399998));
#334723=CARTESIAN_POINT('Ctrl Pts',(0.744422349999944,12.2,4.52441486499998));
#334724=CARTESIAN_POINT('Ctrl Pts',(0.744422349999944,5.2,4.52441486499998));
#334725=CARTESIAN_POINT('Ctrl Pts',(0.744422349999944,2.2,4.52441486499998));
#334726=CARTESIAN_POINT('Ctrl Pts',(0.743596771999945,12.2,4.52666922199998));
#334727=CARTESIAN_POINT('Ctrl Pts',(0.743596771999945,5.2,4.52666922199998));
#334728=CARTESIAN_POINT('Ctrl Pts',(0.743596771999945,2.2,4.52666922199998));
#334729=CARTESIAN_POINT('Ctrl Pts',(0.742767542999945,12.2,4.52892610699998));
#334730=CARTESIAN_POINT('Ctrl Pts',(0.742767542999945,5.2,4.52892610699998));
#334731=CARTESIAN_POINT('Ctrl Pts',(0.742767542999945,2.2,4.52892610699998));
#334732=CARTESIAN_POINT('Ctrl Pts',(0.741934656999944,12.2,4.53118550999999));
#334733=CARTESIAN_POINT('Ctrl Pts',(0.741934656999944,5.2,4.53118550999999));
#334734=CARTESIAN_POINT('Ctrl Pts',(0.741934656999944,2.2,4.53118550999999));
#334735=CARTESIAN_POINT('Ctrl Pts',(0.741098112999944,12.2,4.53344742499999));
#334736=CARTESIAN_POINT('Ctrl Pts',(0.741098112999944,5.2,4.53344742499999));
#334737=CARTESIAN_POINT('Ctrl Pts',(0.741098112999944,2.2,4.53344742499999));
#334738=CARTESIAN_POINT('Ctrl Pts',(0.740257903999945,12.2,4.53571184099999));
#334739=CARTESIAN_POINT('Ctrl Pts',(0.740257903999945,5.2,4.53571184099999));
#334740=CARTESIAN_POINT('Ctrl Pts',(0.740257903999945,2.2,4.53571184099999));
#334741=CARTESIAN_POINT('Ctrl Pts',(0.739414027999944,12.2,4.53797875199999));
#334742=CARTESIAN_POINT('Ctrl Pts',(0.739414027999944,5.2,4.53797875199999));
#334743=CARTESIAN_POINT('Ctrl Pts',(0.739414027999944,2.2,4.53797875199999));
#334744=CARTESIAN_POINT('Ctrl Pts',(0.738566478999945,12.2,4.54024814799999));
#334745=CARTESIAN_POINT('Ctrl Pts',(0.738566478999945,5.2,4.54024814799999));
#334746=CARTESIAN_POINT('Ctrl Pts',(0.738566478999945,2.2,4.54024814799999));
#334747=CARTESIAN_POINT('Ctrl Pts',(0.737715255999943,12.2,4.54252002199999));
#334748=CARTESIAN_POINT('Ctrl Pts',(0.737715255999943,5.2,4.54252002199999));
#334749=CARTESIAN_POINT('Ctrl Pts',(0.737715255999943,2.2,4.54252002199999));
#334750=CARTESIAN_POINT('Ctrl Pts',(0.736860351999944,12.2,4.54479436399998));
#334751=CARTESIAN_POINT('Ctrl Pts',(0.736860351999944,5.2,4.54479436399998));
#334752=CARTESIAN_POINT('Ctrl Pts',(0.736860351999944,2.2,4.54479436399998));
#334753=CARTESIAN_POINT('Ctrl Pts',(0.736001763999944,12.2,4.54707116699999));
#334754=CARTESIAN_POINT('Ctrl Pts',(0.736001763999944,5.2,4.54707116699999));
#334755=CARTESIAN_POINT('Ctrl Pts',(0.736001763999944,2.2,4.54707116699999));
#334756=CARTESIAN_POINT('Ctrl Pts',(0.735139488999944,12.2,4.54935042199998));
#334757=CARTESIAN_POINT('Ctrl Pts',(0.735139488999944,5.2,4.54935042199998));
#334758=CARTESIAN_POINT('Ctrl Pts',(0.735139488999944,2.2,4.54935042199998));
#334759=CARTESIAN_POINT('Ctrl Pts',(0.734273520999944,12.2,4.55163212099999));
#334760=CARTESIAN_POINT('Ctrl Pts',(0.734273520999944,5.2,4.55163212099999));
#334761=CARTESIAN_POINT('Ctrl Pts',(0.734273520999944,2.2,4.55163212099999));
#334762=CARTESIAN_POINT('Ctrl Pts',(0.733403857999945,12.2,4.55391625599999));
#334763=CARTESIAN_POINT('Ctrl Pts',(0.733403857999945,5.2,4.55391625599999));
#334764=CARTESIAN_POINT('Ctrl Pts',(0.733403857999945,2.2,4.55391625599999));
#334765=CARTESIAN_POINT('Ctrl Pts',(0.732530494999944,12.2,4.55620281699999));
#334766=CARTESIAN_POINT('Ctrl Pts',(0.732530494999944,5.2,4.55620281699999));
#334767=CARTESIAN_POINT('Ctrl Pts',(0.732530494999944,2.2,4.55620281699999));
#334768=CARTESIAN_POINT('Ctrl Pts',(0.731653427999944,12.2,4.55849179699998));
#334769=CARTESIAN_POINT('Ctrl Pts',(0.731653427999944,5.2,4.55849179699998));
#334770=CARTESIAN_POINT('Ctrl Pts',(0.731653427999944,2.2,4.55849179699998));
#334771=CARTESIAN_POINT('Ctrl Pts',(0.730772652999944,12.2,4.56078318899999));
#334772=CARTESIAN_POINT('Ctrl Pts',(0.730772652999944,5.2,4.56078318899999));
#334773=CARTESIAN_POINT('Ctrl Pts',(0.730772652999944,2.2,4.56078318899999));
#334774=CARTESIAN_POINT('Ctrl Pts',(0.729888166999944,12.2,4.56307698199999));
#334775=CARTESIAN_POINT('Ctrl Pts',(0.729888166999944,5.2,4.56307698199999));
#334776=CARTESIAN_POINT('Ctrl Pts',(0.729888166999944,2.2,4.56307698199999));
#334777=CARTESIAN_POINT('Ctrl Pts',(0.728999964999945,12.2,4.56537316999999));
#334778=CARTESIAN_POINT('Ctrl Pts',(0.728999964999945,5.2,4.56537316999999));
#334779=CARTESIAN_POINT('Ctrl Pts',(0.728999964999945,2.2,4.56537316999999));
#334780=CARTESIAN_POINT('Ctrl Pts',(0.728108044999944,12.2,4.56767174299999));
#334781=CARTESIAN_POINT('Ctrl Pts',(0.728108044999944,5.2,4.56767174299999));
#334782=CARTESIAN_POINT('Ctrl Pts',(0.728108044999944,2.2,4.56767174299999));
#334783=CARTESIAN_POINT('Ctrl Pts',(0.727212399999945,12.2,4.56997269299999));
#334784=CARTESIAN_POINT('Ctrl Pts',(0.727212399999945,5.2,4.56997269299999));
#334785=CARTESIAN_POINT('Ctrl Pts',(0.727212399999945,2.2,4.56997269299999));
#334786=CARTESIAN_POINT('Ctrl Pts',(0.726313029999944,12.2,4.57227601299999));
#334787=CARTESIAN_POINT('Ctrl Pts',(0.726313029999944,5.2,4.57227601299999));
#334788=CARTESIAN_POINT('Ctrl Pts',(0.726313029999944,2.2,4.57227601299999));
#334789=CARTESIAN_POINT('Ctrl Pts',(0.725409927999944,12.2,4.57458169399998));
#334790=CARTESIAN_POINT('Ctrl Pts',(0.725409927999944,5.2,4.57458169399998));
#334791=CARTESIAN_POINT('Ctrl Pts',(0.725409927999944,2.2,4.57458169399998));
#334792=CARTESIAN_POINT('Ctrl Pts',(0.724503090999944,12.2,4.57688972699999));
#334793=CARTESIAN_POINT('Ctrl Pts',(0.724503090999944,5.2,4.57688972699999));
#334794=CARTESIAN_POINT('Ctrl Pts',(0.724503090999944,2.2,4.57688972699999));
#334795=CARTESIAN_POINT('Ctrl Pts',(0.723592515999945,12.2,4.57920010399998));
#334796=CARTESIAN_POINT('Ctrl Pts',(0.723592515999945,5.2,4.57920010399998));
#334797=CARTESIAN_POINT('Ctrl Pts',(0.723592515999945,2.2,4.57920010399998));
#334798=CARTESIAN_POINT('Ctrl Pts',(0.722678199999944,12.2,4.58151281799999));
#334799=CARTESIAN_POINT('Ctrl Pts',(0.722678199999944,5.2,4.58151281799999));
#334800=CARTESIAN_POINT('Ctrl Pts',(0.722678199999944,2.2,4.58151281799999));
#334801=CARTESIAN_POINT('Ctrl Pts',(0.721760135999945,12.2,4.58382785899998));
#334802=CARTESIAN_POINT('Ctrl Pts',(0.721760135999945,5.2,4.58382785899998));
#334803=CARTESIAN_POINT('Ctrl Pts',(0.721760135999945,2.2,4.58382785899998));
#334804=CARTESIAN_POINT('Ctrl Pts',(0.720838322999944,12.2,4.58614521899998));
#334805=CARTESIAN_POINT('Ctrl Pts',(0.720838322999944,5.2,4.58614521899998));
#334806=CARTESIAN_POINT('Ctrl Pts',(0.720838322999944,2.2,4.58614521899998));
#334807=CARTESIAN_POINT('Ctrl Pts',(0.719912756999944,12.2,4.58846488999999));
#334808=CARTESIAN_POINT('Ctrl Pts',(0.719912756999944,5.2,4.58846488999999));
#334809=CARTESIAN_POINT('Ctrl Pts',(0.719912756999944,2.2,4.58846488999999));
#334810=CARTESIAN_POINT('Ctrl Pts',(0.718983433999945,12.2,4.59078686499999));
#334811=CARTESIAN_POINT('Ctrl Pts',(0.718983433999945,5.2,4.59078686499999));
#334812=CARTESIAN_POINT('Ctrl Pts',(0.718983433999945,2.2,4.59078686499999));
#334813=CARTESIAN_POINT('Ctrl Pts',(0.718050349999944,12.2,4.59311113399998));
#334814=CARTESIAN_POINT('Ctrl Pts',(0.718050349999944,5.2,4.59311113399998));
#334815=CARTESIAN_POINT('Ctrl Pts',(0.718050349999944,2.2,4.59311113399998));
#334816=CARTESIAN_POINT('Ctrl Pts',(0.717113500999944,12.2,4.59543768999998));
#334817=CARTESIAN_POINT('Ctrl Pts',(0.717113500999944,5.2,4.59543768999998));
#334818=CARTESIAN_POINT('Ctrl Pts',(0.717113500999944,2.2,4.59543768999998));
#334819=CARTESIAN_POINT('Ctrl Pts',(0.716172884999944,12.2,4.59776652499999));
#334820=CARTESIAN_POINT('Ctrl Pts',(0.716172884999944,5.2,4.59776652499999));
#334821=CARTESIAN_POINT('Ctrl Pts',(0.716172884999944,2.2,4.59776652499999));
#334822=CARTESIAN_POINT('Ctrl Pts',(0.715228496999945,12.2,4.60009762899999));
#334823=CARTESIAN_POINT('Ctrl Pts',(0.715228496999945,5.2,4.60009762899999));
#334824=CARTESIAN_POINT('Ctrl Pts',(0.715228496999945,2.2,4.60009762899999));
#334825=CARTESIAN_POINT('Ctrl Pts',(0.714280331999944,12.2,4.60243099399998));
#334826=CARTESIAN_POINT('Ctrl Pts',(0.714280331999944,5.2,4.60243099399998));
#334827=CARTESIAN_POINT('Ctrl Pts',(0.714280331999944,2.2,4.60243099399998));
#334828=CARTESIAN_POINT('Ctrl Pts',(0.713328389999944,12.2,4.60476661399999));
#334829=CARTESIAN_POINT('Ctrl Pts',(0.713328389999944,5.2,4.60476661399999));
#334830=CARTESIAN_POINT('Ctrl Pts',(0.713328389999944,2.2,4.60476661399999));
#334831=CARTESIAN_POINT('Ctrl Pts',(0.712372663999944,12.2,4.60710447899999));
#334832=CARTESIAN_POINT('Ctrl Pts',(0.712372663999944,5.2,4.60710447899999));
#334833=CARTESIAN_POINT('Ctrl Pts',(0.712372663999944,2.2,4.60710447899999));
#334834=CARTESIAN_POINT('Ctrl Pts',(0.711413152999943,12.2,4.60944458099998));
#334835=CARTESIAN_POINT('Ctrl Pts',(0.711413152999943,5.2,4.60944458099998));
#334836=CARTESIAN_POINT('Ctrl Pts',(0.711413152999943,2.2,4.60944458099998));
#334837=CARTESIAN_POINT('Ctrl Pts',(0.710449851999945,12.2,4.61178691299998));
#334838=CARTESIAN_POINT('Ctrl Pts',(0.710449851999945,5.2,4.61178691299998));
#334839=CARTESIAN_POINT('Ctrl Pts',(0.710449851999945,2.2,4.61178691299998));
#334840=CARTESIAN_POINT('Ctrl Pts',(0.709482756999944,12.2,4.61413146499999));
#334841=CARTESIAN_POINT('Ctrl Pts',(0.709482756999944,5.2,4.61413146499999));
#334842=CARTESIAN_POINT('Ctrl Pts',(0.709482756999944,2.2,4.61413146499999));
#334843=CARTESIAN_POINT('Ctrl Pts',(0.708511864999944,12.2,4.61647822799998));
#334844=CARTESIAN_POINT('Ctrl Pts',(0.708511864999944,5.2,4.61647822799998));
#334845=CARTESIAN_POINT('Ctrl Pts',(0.708511864999944,2.2,4.61647822799998));
#334846=CARTESIAN_POINT('Ctrl Pts',(0.707537173999944,12.2,4.61882719699998));
#334847=CARTESIAN_POINT('Ctrl Pts',(0.707537173999944,5.2,4.61882719699998));
#334848=CARTESIAN_POINT('Ctrl Pts',(0.707537173999944,2.2,4.61882719699998));
#334849=CARTESIAN_POINT('Ctrl Pts',(0.706558677999943,12.2,4.62117836299999));
#334850=CARTESIAN_POINT('Ctrl Pts',(0.706558677999943,5.2,4.62117836299999));
#334851=CARTESIAN_POINT('Ctrl Pts',(0.706558677999943,2.2,4.62117836299999));
#334852=CARTESIAN_POINT('Ctrl Pts',(0.705576373999944,12.2,4.62353171699998));
#334853=CARTESIAN_POINT('Ctrl Pts',(0.705576373999944,5.2,4.62353171699998));
#334854=CARTESIAN_POINT('Ctrl Pts',(0.705576373999944,2.2,4.62353171699998));
#334855=CARTESIAN_POINT('Ctrl Pts',(0.704590260999944,12.2,4.62588724999998));
#334856=CARTESIAN_POINT('Ctrl Pts',(0.704590260999944,5.2,4.62588724999998));
#334857=CARTESIAN_POINT('Ctrl Pts',(0.704590260999944,2.2,4.62588724999998));
#334858=CARTESIAN_POINT('Ctrl Pts',(0.703600331999944,12.2,4.62824495499999));
#334859=CARTESIAN_POINT('Ctrl Pts',(0.703600331999944,5.2,4.62824495499999));
#334860=CARTESIAN_POINT('Ctrl Pts',(0.703600331999944,2.2,4.62824495499999));
#334861=CARTESIAN_POINT('Ctrl Pts',(0.702606586999944,12.2,4.63060482299999));
#334862=CARTESIAN_POINT('Ctrl Pts',(0.702606586999944,5.2,4.63060482299999));
#334863=CARTESIAN_POINT('Ctrl Pts',(0.702606586999944,2.2,4.63060482299999));
#334864=CARTESIAN_POINT('Ctrl Pts',(0.701609018999945,12.2,4.63296684699999));
#334865=CARTESIAN_POINT('Ctrl Pts',(0.701609018999945,5.2,4.63296684699999));
#334866=CARTESIAN_POINT('Ctrl Pts',(0.701609018999945,2.2,4.63296684699999));
#334867=CARTESIAN_POINT('Ctrl Pts',(0.700607627999944,12.2,4.63533101799998));
#334868=CARTESIAN_POINT('Ctrl Pts',(0.700607627999944,5.2,4.63533101799998));
#334869=CARTESIAN_POINT('Ctrl Pts',(0.700607627999944,2.2,4.63533101799998));
#334870=CARTESIAN_POINT('Ctrl Pts',(0.699602407999944,12.2,4.63769732799998));
#334871=CARTESIAN_POINT('Ctrl Pts',(0.699602407999944,5.2,4.63769732799998));
#334872=CARTESIAN_POINT('Ctrl Pts',(0.699602407999944,2.2,4.63769732799998));
#334873=CARTESIAN_POINT('Ctrl Pts',(0.698593355999945,12.2,4.64006576799999));
#334874=CARTESIAN_POINT('Ctrl Pts',(0.698593355999945,5.2,4.64006576799999));
#334875=CARTESIAN_POINT('Ctrl Pts',(0.698593355999945,2.2,4.64006576799999));
#334876=CARTESIAN_POINT('Ctrl Pts',(0.697580470999944,12.2,4.64243633299999));
#334877=CARTESIAN_POINT('Ctrl Pts',(0.697580470999944,5.2,4.64243633299999));
#334878=CARTESIAN_POINT('Ctrl Pts',(0.697580470999944,2.2,4.64243633299999));
#334879=CARTESIAN_POINT('Ctrl Pts',(0.696563746999944,12.2,4.64480901199998));
#334880=CARTESIAN_POINT('Ctrl Pts',(0.696563746999944,5.2,4.64480901199998));
#334881=CARTESIAN_POINT('Ctrl Pts',(0.696563746999944,2.2,4.64480901199998));
#334882=CARTESIAN_POINT('Ctrl Pts',(0.695543181999944,12.2,4.64718379799999));
#334883=CARTESIAN_POINT('Ctrl Pts',(0.695543181999944,5.2,4.64718379799999));
#334884=CARTESIAN_POINT('Ctrl Pts',(0.695543181999944,2.2,4.64718379799999));
#334885=CARTESIAN_POINT('Ctrl Pts',(0.694518772999944,12.2,4.64956068299998));
#334886=CARTESIAN_POINT('Ctrl Pts',(0.694518772999944,5.2,4.64956068299998));
#334887=CARTESIAN_POINT('Ctrl Pts',(0.694518772999944,2.2,4.64956068299998));
#334888=CARTESIAN_POINT('Ctrl Pts',(0.693490514999944,12.2,4.65193965799998));
#334889=CARTESIAN_POINT('Ctrl Pts',(0.693490514999944,5.2,4.65193965799998));
#334890=CARTESIAN_POINT('Ctrl Pts',(0.693490514999944,2.2,4.65193965799998));
#334891=CARTESIAN_POINT('Ctrl Pts',(0.692458406999944,12.2,4.65432071499999));
#334892=CARTESIAN_POINT('Ctrl Pts',(0.692458406999944,5.2,4.65432071499999));
#334893=CARTESIAN_POINT('Ctrl Pts',(0.692458406999944,2.2,4.65432071499999));
#334894=CARTESIAN_POINT('Ctrl Pts',(0.691422441999944,12.2,4.65670384699998));
#334895=CARTESIAN_POINT('Ctrl Pts',(0.691422441999944,5.2,4.65670384699998));
#334896=CARTESIAN_POINT('Ctrl Pts',(0.691422441999944,2.2,4.65670384699998));
#334897=CARTESIAN_POINT('Ctrl Pts',(0.690382619999944,12.2,4.65908904299998));
#334898=CARTESIAN_POINT('Ctrl Pts',(0.690382619999944,5.2,4.65908904299998));
#334899=CARTESIAN_POINT('Ctrl Pts',(0.690382619999944,2.2,4.65908904299998));
#334900=CARTESIAN_POINT('Ctrl Pts',(0.689338937999944,12.2,4.66147629599998));
#334901=CARTESIAN_POINT('Ctrl Pts',(0.689338937999944,5.2,4.66147629599998));
#334902=CARTESIAN_POINT('Ctrl Pts',(0.689338937999944,2.2,4.66147629599998));
#334903=CARTESIAN_POINT('Ctrl Pts',(0.688291388999944,12.2,4.66386559899998));
#334904=CARTESIAN_POINT('Ctrl Pts',(0.688291388999944,5.2,4.66386559899998));
#334905=CARTESIAN_POINT('Ctrl Pts',(0.688291388999944,2.2,4.66386559899998));
#334906=CARTESIAN_POINT('Ctrl Pts',(0.687239972999943,12.2,4.66625694299999));
#334907=CARTESIAN_POINT('Ctrl Pts',(0.687239972999943,5.2,4.66625694299999));
#334908=CARTESIAN_POINT('Ctrl Pts',(0.687239972999943,2.2,4.66625694299999));
#334909=CARTESIAN_POINT('Ctrl Pts',(0.686184687999944,12.2,4.66865032199999));
#334910=CARTESIAN_POINT('Ctrl Pts',(0.686184687999944,5.2,4.66865032199999));
#334911=CARTESIAN_POINT('Ctrl Pts',(0.686184687999944,2.2,4.66865032199999));
#334912=CARTESIAN_POINT('Ctrl Pts',(0.685125528999944,12.2,4.67104572799999));
#334913=CARTESIAN_POINT('Ctrl Pts',(0.685125528999944,5.2,4.67104572799999));
#334914=CARTESIAN_POINT('Ctrl Pts',(0.685125528999944,2.2,4.67104572799999));
#334915=CARTESIAN_POINT('Ctrl Pts',(0.684062492999944,12.2,4.67344315399998));
#334916=CARTESIAN_POINT('Ctrl Pts',(0.684062492999944,5.2,4.67344315399998));
#334917=CARTESIAN_POINT('Ctrl Pts',(0.684062492999944,2.2,4.67344315399998));
#334918=CARTESIAN_POINT('Ctrl Pts',(0.682995577999944,12.2,4.67584259099999));
#334919=CARTESIAN_POINT('Ctrl Pts',(0.682995577999944,5.2,4.67584259099999));
#334920=CARTESIAN_POINT('Ctrl Pts',(0.682995577999944,2.2,4.67584259099999));
#334921=CARTESIAN_POINT('Ctrl Pts',(0.681924779999944,12.2,4.67824403199998));
#334922=CARTESIAN_POINT('Ctrl Pts',(0.681924779999944,5.2,4.67824403199998));
#334923=CARTESIAN_POINT('Ctrl Pts',(0.681924779999944,2.2,4.67824403199998));
#334924=CARTESIAN_POINT('Ctrl Pts',(0.680850095999944,12.2,4.68064746499999));
#334925=CARTESIAN_POINT('Ctrl Pts',(0.680850095999944,5.2,4.68064746499999));
#334926=CARTESIAN_POINT('Ctrl Pts',(0.680850095999944,2.2,4.68064746499999));
#334927=CARTESIAN_POINT('Ctrl Pts',(0.679771519999944,12.2,4.68305288099998));
#334928=CARTESIAN_POINT('Ctrl Pts',(0.679771519999944,5.2,4.68305288099998));
#334929=CARTESIAN_POINT('Ctrl Pts',(0.679771519999944,2.2,4.68305288099998));
#334930=CARTESIAN_POINT('Ctrl Pts',(0.678689050999944,12.2,4.68546026999999));
#334931=CARTESIAN_POINT('Ctrl Pts',(0.678689050999944,5.2,4.68546026999999));
#334932=CARTESIAN_POINT('Ctrl Pts',(0.678689050999944,2.2,4.68546026999999));
#334933=CARTESIAN_POINT('Ctrl Pts',(0.677602681999944,12.2,4.68786962299998));
#334934=CARTESIAN_POINT('Ctrl Pts',(0.677602681999944,5.2,4.68786962299998));
#334935=CARTESIAN_POINT('Ctrl Pts',(0.677602681999944,2.2,4.68786962299998));
#334936=CARTESIAN_POINT('Ctrl Pts',(0.676512413999945,12.2,4.69028093199999));
#334937=CARTESIAN_POINT('Ctrl Pts',(0.676512413999945,5.2,4.69028093199999));
#334938=CARTESIAN_POINT('Ctrl Pts',(0.676512413999945,2.2,4.69028093199999));
#334939=CARTESIAN_POINT('Ctrl Pts',(0.675418241999944,12.2,4.69269419199998));
#334940=CARTESIAN_POINT('Ctrl Pts',(0.675418241999944,5.2,4.69269419199998));
#334941=CARTESIAN_POINT('Ctrl Pts',(0.675418241999944,2.2,4.69269419199998));
#334942=CARTESIAN_POINT('Ctrl Pts',(0.674320165999944,12.2,4.69510939799999));
#334943=CARTESIAN_POINT('Ctrl Pts',(0.674320165999944,5.2,4.69510939799999));
#334944=CARTESIAN_POINT('Ctrl Pts',(0.674320165999944,2.2,4.69510939799999));
#334945=CARTESIAN_POINT('Ctrl Pts',(0.673218184999944,12.2,4.69752654799999));
#334946=CARTESIAN_POINT('Ctrl Pts',(0.673218184999944,5.2,4.69752654799999));
#334947=CARTESIAN_POINT('Ctrl Pts',(0.673218184999944,2.2,4.69752654799999));
#334948=CARTESIAN_POINT('Ctrl Pts',(0.672333474999944,12.2,4.69946182299999));
#334949=CARTESIAN_POINT('Ctrl Pts',(0.672333474999944,5.2,4.69946182299999));
#334950=CARTESIAN_POINT('Ctrl Pts',(0.672333474999944,2.2,4.69946182299999));
#334951=CARTESIAN_POINT('Ctrl Pts',(0.671668184999944,12.2,4.70091415399998));
#334952=CARTESIAN_POINT('Ctrl Pts',(0.671668184999944,5.2,4.70091415399998));
#334953=CARTESIAN_POINT('Ctrl Pts',(0.671668184999944,2.2,4.70091415399998));
#334954=CARTESIAN_POINT('Ctrl Pts',(0.671223877999945,12.2,4.70188276299999));
#334955=CARTESIAN_POINT('Ctrl Pts',(0.671223877999945,5.2,4.70188276299999));
#334956=CARTESIAN_POINT('Ctrl Pts',(0.671223877999945,2.2,4.70188276299999));
#334957=CARTESIAN_POINT('Ctrl Pts',(0.671001528999944,12.2,4.70236716399998));
#334958=CARTESIAN_POINT('Ctrl Pts',(0.671001528999944,5.2,4.70236716399998));
#334959=CARTESIAN_POINT('Ctrl Pts',(0.671001528999944,2.2,4.70236716399998));
#334960=CARTESIAN_POINT('',(0.846447418999944,12.2,3.90299742599999));
#334961=CARTESIAN_POINT('Origin',(-5.66300478732629E-14,15.2,-1.77635683940025E-14));
#334962=CARTESIAN_POINT('',(0.768297694999944,12.2,3.54264641999999));
#334963=CARTESIAN_POINT('Origin',(-5.66300478732629E-14,15.2,-1.77635683940025E-14));
#334964=CARTESIAN_POINT('',(1.30596997799994,2.2,3.38157765299999));
#334965=CARTESIAN_POINT('Origin',(-5.66300478732629E-14,15.2,-1.77635683940025E-14));
#334966=CARTESIAN_POINT('',(2.19921400599994,12.2,3.33366463399998));
#334967=CARTESIAN_POINT('',(1.99616775999994,12.2,3.02587826499998));
#334968=CARTESIAN_POINT('Origin',(1.43879834299994,15.2,3.72551314699999));
#334969=CARTESIAN_POINT('',(1.43881682999994,12.2,3.72556101799999));
#334970=CARTESIAN_POINT('Ctrl Pts',(2.02484995099994,12.2,4.29679911999998));
#334971=CARTESIAN_POINT('Ctrl Pts',(2.02484995099994,5.2,4.29679911999998));
#334972=CARTESIAN_POINT('Ctrl Pts',(2.02484995099994,2.2,4.29679911999998));
#334973=CARTESIAN_POINT('Ctrl Pts',(2.02439790199994,12.2,4.29651674599998));
#334974=CARTESIAN_POINT('Ctrl Pts',(2.02439790199994,5.2,4.29651674599998));
#334975=CARTESIAN_POINT('Ctrl Pts',(2.02439790199994,2.2,4.29651674599998));
#334976=CARTESIAN_POINT('Ctrl Pts',(2.02349423499994,12.2,4.29595194499999));
#334977=CARTESIAN_POINT('Ctrl Pts',(2.02349423499994,5.2,4.29595194499999));
#334978=CARTESIAN_POINT('Ctrl Pts',(2.02349423499994,2.2,4.29595194499999));
#334979=CARTESIAN_POINT('Ctrl Pts',(2.02214003499994,12.2,4.29510458699998));
#334980=CARTESIAN_POINT('Ctrl Pts',(2.02214003499994,5.2,4.29510458699998));
#334981=CARTESIAN_POINT('Ctrl Pts',(2.02214003499994,2.2,4.29510458699998));
#334982=CARTESIAN_POINT('Ctrl Pts',(2.02033703299994,12.2,4.29397446099999));
#334983=CARTESIAN_POINT('Ctrl Pts',(2.02033703299994,5.2,4.29397446099999));
#334984=CARTESIAN_POINT('Ctrl Pts',(2.02033703299994,2.2,4.29397446099999));
#334985=CARTESIAN_POINT('Ctrl Pts',(2.01808761199994,12.2,4.29256127999999));
#334986=CARTESIAN_POINT('Ctrl Pts',(2.01808761199994,5.2,4.29256127999999));
#334987=CARTESIAN_POINT('Ctrl Pts',(2.01808761199994,2.2,4.29256127999999));
#334988=CARTESIAN_POINT('Ctrl Pts',(2.01584252099994,12.2,4.29114757499999));
#334989=CARTESIAN_POINT('Ctrl Pts',(2.01584252099994,5.2,4.29114757499999));
#334990=CARTESIAN_POINT('Ctrl Pts',(2.01584252099994,2.2,4.29114757499999));
#334991=CARTESIAN_POINT('Ctrl Pts',(2.01360176199994,12.2,4.28973334999998));
#334992=CARTESIAN_POINT('Ctrl Pts',(2.01360176199994,5.2,4.28973334999998));
#334993=CARTESIAN_POINT('Ctrl Pts',(2.01360176199994,2.2,4.28973334999998));
#334994=CARTESIAN_POINT('Ctrl Pts',(2.01136533499994,12.2,4.28831860799999));
#334995=CARTESIAN_POINT('Ctrl Pts',(2.01136533499994,5.2,4.28831860799999));
#334996=CARTESIAN_POINT('Ctrl Pts',(2.01136533499994,2.2,4.28831860799999));
#334997=CARTESIAN_POINT('Ctrl Pts',(2.00913324299994,12.2,4.28690335699999));
#334998=CARTESIAN_POINT('Ctrl Pts',(2.00913324299994,5.2,4.28690335699999));
#334999=CARTESIAN_POINT('Ctrl Pts',(2.00913324299994,2.2,4.28690335699999));
#335000=CARTESIAN_POINT('Ctrl Pts',(2.00690548599994,12.2,4.28548760099999));
#335001=CARTESIAN_POINT('Ctrl Pts',(2.00690548599994,5.2,4.28548760099999));
#335002=CARTESIAN_POINT('Ctrl Pts',(2.00690548599994,2.2,4.28548760099999));
#335003=CARTESIAN_POINT('Ctrl Pts',(2.00468206699994,12.2,4.28407135299998));
#335004=CARTESIAN_POINT('Ctrl Pts',(2.00468206699994,5.2,4.28407135299998));
#335005=CARTESIAN_POINT('Ctrl Pts',(2.00468206699994,2.2,4.28407135299998));
#335006=CARTESIAN_POINT('Ctrl Pts',(2.00246298799994,12.2,4.28265462199998));
#335007=CARTESIAN_POINT('Ctrl Pts',(2.00246298799994,5.2,4.28265462199998));
#335008=CARTESIAN_POINT('Ctrl Pts',(2.00246298799994,2.2,4.28265462199998));
#335009=CARTESIAN_POINT('Ctrl Pts',(2.00024825099994,12.2,4.28123741899999));
#335010=CARTESIAN_POINT('Ctrl Pts',(2.00024825099994,5.2,4.28123741899999));
#335011=CARTESIAN_POINT('Ctrl Pts',(2.00024825099994,2.2,4.28123741899999));
#335012=CARTESIAN_POINT('Ctrl Pts',(1.99803785899994,12.2,4.27981975299998));
#335013=CARTESIAN_POINT('Ctrl Pts',(1.99803785899994,5.2,4.27981975299998));
#335014=CARTESIAN_POINT('Ctrl Pts',(1.99803785899994,2.2,4.27981975299998));
#335015=CARTESIAN_POINT('Ctrl Pts',(1.99583181299994,12.2,4.27840163599999));
#335016=CARTESIAN_POINT('Ctrl Pts',(1.99583181299994,5.2,4.27840163599999));
#335017=CARTESIAN_POINT('Ctrl Pts',(1.99583181299994,2.2,4.27840163599999));
#335018=CARTESIAN_POINT('Ctrl Pts',(1.99363011599994,12.2,4.27698307399999));
#335019=CARTESIAN_POINT('Ctrl Pts',(1.99363011599994,5.2,4.27698307399999));
#335020=CARTESIAN_POINT('Ctrl Pts',(1.99363011599994,2.2,4.27698307399999));
#335021=CARTESIAN_POINT('Ctrl Pts',(1.99143276799994,12.2,4.27556407599998));
#335022=CARTESIAN_POINT('Ctrl Pts',(1.99143276799994,5.2,4.27556407599998));
#335023=CARTESIAN_POINT('Ctrl Pts',(1.99143276799994,2.2,4.27556407599998));
#335024=CARTESIAN_POINT('Ctrl Pts',(1.98923977299994,12.2,4.27414464999998));
#335025=CARTESIAN_POINT('Ctrl Pts',(1.98923977299994,5.2,4.27414464999998));
#335026=CARTESIAN_POINT('Ctrl Pts',(1.98923977299994,2.2,4.27414464999998));
#335027=CARTESIAN_POINT('Ctrl Pts',(1.98705112999994,12.2,4.27272480299998));
#335028=CARTESIAN_POINT('Ctrl Pts',(1.98705112999994,5.2,4.27272480299998));
#335029=CARTESIAN_POINT('Ctrl Pts',(1.98705112999994,2.2,4.27272480299998));
#335030=CARTESIAN_POINT('Ctrl Pts',(1.98486684199994,12.2,4.27130454199999));
#335031=CARTESIAN_POINT('Ctrl Pts',(1.98486684199994,5.2,4.27130454199999));
#335032=CARTESIAN_POINT('Ctrl Pts',(1.98486684199994,2.2,4.27130454199999));
#335033=CARTESIAN_POINT('Ctrl Pts',(1.98268690899994,12.2,4.26988387799998));
#335034=CARTESIAN_POINT('Ctrl Pts',(1.98268690899994,5.2,4.26988387799998));
#335035=CARTESIAN_POINT('Ctrl Pts',(1.98268690899994,2.2,4.26988387799998));
#335036=CARTESIAN_POINT('Ctrl Pts',(1.98051133699994,12.2,4.26846281599998));
#335037=CARTESIAN_POINT('Ctrl Pts',(1.98051133699994,5.2,4.26846281599998));
#335038=CARTESIAN_POINT('Ctrl Pts',(1.98051133699994,2.2,4.26846281599998));
#335039=CARTESIAN_POINT('Ctrl Pts',(1.97834012299994,12.2,4.26704136799999));
#335040=CARTESIAN_POINT('Ctrl Pts',(1.97834012299994,5.2,4.26704136799999));
#335041=CARTESIAN_POINT('Ctrl Pts',(1.97834012299994,2.2,4.26704136799999));
#335042=CARTESIAN_POINT('Ctrl Pts',(1.97617327099994,12.2,4.26561954099999));
#335043=CARTESIAN_POINT('Ctrl Pts',(1.97617327099994,5.2,4.26561954099999));
#335044=CARTESIAN_POINT('Ctrl Pts',(1.97617327099994,2.2,4.26561954099999));
#335045=CARTESIAN_POINT('Ctrl Pts',(1.97401078399994,12.2,4.26419734499999));
#335046=CARTESIAN_POINT('Ctrl Pts',(1.97401078399994,5.2,4.26419734499999));
#335047=CARTESIAN_POINT('Ctrl Pts',(1.97401078399994,2.2,4.26419734499999));
#335048=CARTESIAN_POINT('Ctrl Pts',(1.97185265999994,12.2,4.26277478799998));
#335049=CARTESIAN_POINT('Ctrl Pts',(1.97185265999994,5.2,4.26277478799998));
#335050=CARTESIAN_POINT('Ctrl Pts',(1.97185265999994,2.2,4.26277478799998));
#335051=CARTESIAN_POINT('Ctrl Pts',(1.96969890499994,12.2,4.26135187899998));
#335052=CARTESIAN_POINT('Ctrl Pts',(1.96969890499994,5.2,4.26135187899998));
#335053=CARTESIAN_POINT('Ctrl Pts',(1.96969890499994,2.2,4.26135187899998));
#335054=CARTESIAN_POINT('Ctrl Pts',(1.96754951799994,12.2,4.25992862799998));
#335055=CARTESIAN_POINT('Ctrl Pts',(1.96754951799994,5.2,4.25992862799998));
#335056=CARTESIAN_POINT('Ctrl Pts',(1.96754951799994,2.2,4.25992862799998));
#335057=CARTESIAN_POINT('Ctrl Pts',(1.96540450099994,12.2,4.25850504099999));
#335058=CARTESIAN_POINT('Ctrl Pts',(1.96540450099994,5.2,4.25850504099999));
#335059=CARTESIAN_POINT('Ctrl Pts',(1.96540450099994,2.2,4.25850504099999));
#335060=CARTESIAN_POINT('Ctrl Pts',(1.96326385599994,12.2,4.25708112799998));
#335061=CARTESIAN_POINT('Ctrl Pts',(1.96326385599994,5.2,4.25708112799998));
#335062=CARTESIAN_POINT('Ctrl Pts',(1.96326385599994,2.2,4.25708112799998));
#335063=CARTESIAN_POINT('Ctrl Pts',(1.96112758399994,12.2,4.25565689599999));
#335064=CARTESIAN_POINT('Ctrl Pts',(1.96112758399994,5.2,4.25565689599999));
#335065=CARTESIAN_POINT('Ctrl Pts',(1.96112758399994,2.2,4.25565689599999));
#335066=CARTESIAN_POINT('Ctrl Pts',(1.95899568899994,12.2,4.25423235599999));
#335067=CARTESIAN_POINT('Ctrl Pts',(1.95899568899994,5.2,4.25423235599999));
#335068=CARTESIAN_POINT('Ctrl Pts',(1.95899568899994,2.2,4.25423235599999));
#335069=CARTESIAN_POINT('Ctrl Pts',(1.95686816899994,12.2,4.25280751499999));
#335070=CARTESIAN_POINT('Ctrl Pts',(1.95686816899994,5.2,4.25280751499999));
#335071=CARTESIAN_POINT('Ctrl Pts',(1.95686816899994,2.2,4.25280751499999));
#335072=CARTESIAN_POINT('Ctrl Pts',(1.95474502799994,12.2,4.25138238199998));
#335073=CARTESIAN_POINT('Ctrl Pts',(1.95474502799994,5.2,4.25138238199998));
#335074=CARTESIAN_POINT('Ctrl Pts',(1.95474502799994,2.2,4.25138238199998));
#335075=CARTESIAN_POINT('Ctrl Pts',(1.95262626799994,12.2,4.24995696599999));
#335076=CARTESIAN_POINT('Ctrl Pts',(1.95262626799994,5.2,4.24995696599999));
#335077=CARTESIAN_POINT('Ctrl Pts',(1.95262626799994,2.2,4.24995696599999));
#335078=CARTESIAN_POINT('Ctrl Pts',(1.95051188799995,12.2,4.24853127599999));
#335079=CARTESIAN_POINT('Ctrl Pts',(1.95051188799995,5.2,4.24853127599999));
#335080=CARTESIAN_POINT('Ctrl Pts',(1.95051188799995,2.2,4.24853127599999));
#335081=CARTESIAN_POINT('Ctrl Pts',(1.94840189199994,12.2,4.24710531999998));
#335082=CARTESIAN_POINT('Ctrl Pts',(1.94840189199994,5.2,4.24710531999998));
#335083=CARTESIAN_POINT('Ctrl Pts',(1.94840189199994,2.2,4.24710531999998));
#335084=CARTESIAN_POINT('Ctrl Pts',(1.94629628199994,12.2,4.24567910799999));
#335085=CARTESIAN_POINT('Ctrl Pts',(1.94629628199994,5.2,4.24567910799999));
#335086=CARTESIAN_POINT('Ctrl Pts',(1.94629628199994,2.2,4.24567910799999));
#335087=CARTESIAN_POINT('Ctrl Pts',(1.94419505699994,12.2,4.24425264599999));
#335088=CARTESIAN_POINT('Ctrl Pts',(1.94419505699994,5.2,4.24425264599999));
#335089=CARTESIAN_POINT('Ctrl Pts',(1.94419505699994,2.2,4.24425264599999));
#335090=CARTESIAN_POINT('Ctrl Pts',(1.94209821999994,12.2,4.24282594599998));
#335091=CARTESIAN_POINT('Ctrl Pts',(1.94209821999994,5.2,4.24282594599998));
#335092=CARTESIAN_POINT('Ctrl Pts',(1.94209821999994,2.2,4.24282594599998));
#335093=CARTESIAN_POINT('Ctrl Pts',(1.94000577299994,12.2,4.24139901599998));
#335094=CARTESIAN_POINT('Ctrl Pts',(1.94000577299994,5.2,4.24139901599998));
#335095=CARTESIAN_POINT('Ctrl Pts',(1.94000577299994,2.2,4.24139901599998));
#335096=CARTESIAN_POINT('Ctrl Pts',(1.93791771799994,12.2,4.23997186399999));
#335097=CARTESIAN_POINT('Ctrl Pts',(1.93791771799994,5.2,4.23997186399999));
#335098=CARTESIAN_POINT('Ctrl Pts',(1.93791771799994,2.2,4.23997186399999));
#335099=CARTESIAN_POINT('Ctrl Pts',(1.93583405399994,12.2,4.23854449999999));
#335100=CARTESIAN_POINT('Ctrl Pts',(1.93583405399994,5.2,4.23854449999999));
#335101=CARTESIAN_POINT('Ctrl Pts',(1.93583405399994,2.2,4.23854449999999));
#335102=CARTESIAN_POINT('Ctrl Pts',(1.93375478499994,12.2,4.23711693099998));
#335103=CARTESIAN_POINT('Ctrl Pts',(1.93375478499994,5.2,4.23711693099998));
#335104=CARTESIAN_POINT('Ctrl Pts',(1.93375478499994,2.2,4.23711693099998));
#335105=CARTESIAN_POINT('Ctrl Pts',(1.93167991099994,12.2,4.23568916599999));
#335106=CARTESIAN_POINT('Ctrl Pts',(1.93167991099994,5.2,4.23568916599999));
#335107=CARTESIAN_POINT('Ctrl Pts',(1.93167991099994,2.2,4.23568916599999));
#335108=CARTESIAN_POINT('Ctrl Pts',(1.92960943499994,12.2,4.23426121599999));
#335109=CARTESIAN_POINT('Ctrl Pts',(1.92960943499994,5.2,4.23426121599999));
#335110=CARTESIAN_POINT('Ctrl Pts',(1.92960943499994,2.2,4.23426121599999));
#335111=CARTESIAN_POINT('Ctrl Pts',(1.92754335699994,12.2,4.23283308699999));
#335112=CARTESIAN_POINT('Ctrl Pts',(1.92754335699994,5.2,4.23283308699999));
#335113=CARTESIAN_POINT('Ctrl Pts',(1.92754335699994,2.2,4.23283308699999));
#335114=CARTESIAN_POINT('Ctrl Pts',(1.92548167999994,12.2,4.23140478999999));
#335115=CARTESIAN_POINT('Ctrl Pts',(1.92548167999994,5.2,4.23140478999999));
#335116=CARTESIAN_POINT('Ctrl Pts',(1.92548167999994,2.2,4.23140478999999));
#335117=CARTESIAN_POINT('Ctrl Pts',(1.92342440299994,12.2,4.22997633299998));
#335118=CARTESIAN_POINT('Ctrl Pts',(1.92342440299994,5.2,4.22997633299998));
#335119=CARTESIAN_POINT('Ctrl Pts',(1.92342440299994,2.2,4.22997633299998));
#335120=CARTESIAN_POINT('Ctrl Pts',(1.92137152999994,12.2,4.22854772599998));
#335121=CARTESIAN_POINT('Ctrl Pts',(1.92137152999994,5.2,4.22854772599998));
#335122=CARTESIAN_POINT('Ctrl Pts',(1.92137152999994,2.2,4.22854772599998));
#335123=CARTESIAN_POINT('Ctrl Pts',(1.91932306199994,12.2,4.22711897599999));
#335124=CARTESIAN_POINT('Ctrl Pts',(1.91932306199994,5.2,4.22711897599999));
#335125=CARTESIAN_POINT('Ctrl Pts',(1.91932306199994,2.2,4.22711897599999));
#335126=CARTESIAN_POINT('Ctrl Pts',(1.91727899899994,12.2,4.22569009299998));
#335127=CARTESIAN_POINT('Ctrl Pts',(1.91727899899994,5.2,4.22569009299998));
#335128=CARTESIAN_POINT('Ctrl Pts',(1.91727899899994,2.2,4.22569009299998));
#335129=CARTESIAN_POINT('Ctrl Pts',(1.91523934399994,12.2,4.22426108799999));
#335130=CARTESIAN_POINT('Ctrl Pts',(1.91523934399994,5.2,4.22426108799999));
#335131=CARTESIAN_POINT('Ctrl Pts',(1.91523934399994,2.2,4.22426108799999));
#335132=CARTESIAN_POINT('Ctrl Pts',(1.91320409699994,12.2,4.22283196599999));
#335133=CARTESIAN_POINT('Ctrl Pts',(1.91320409699994,5.2,4.22283196599999));
#335134=CARTESIAN_POINT('Ctrl Pts',(1.91320409699994,2.2,4.22283196599999));
#335135=CARTESIAN_POINT('Ctrl Pts',(1.91117325999994,12.2,4.22140273799998));
#335136=CARTESIAN_POINT('Ctrl Pts',(1.91117325999994,5.2,4.22140273799998));
#335137=CARTESIAN_POINT('Ctrl Pts',(1.91117325999994,2.2,4.22140273799998));
#335138=CARTESIAN_POINT('Ctrl Pts',(1.90914683499994,12.2,4.21997341099999));
#335139=CARTESIAN_POINT('Ctrl Pts',(1.90914683499994,5.2,4.21997341099999));
#335140=CARTESIAN_POINT('Ctrl Pts',(1.90914683499994,2.2,4.21997341099999));
#335141=CARTESIAN_POINT('Ctrl Pts',(1.90712482299994,12.2,4.21854399799999));
#335142=CARTESIAN_POINT('Ctrl Pts',(1.90712482299994,5.2,4.21854399799999));
#335143=CARTESIAN_POINT('Ctrl Pts',(1.90712482299994,2.2,4.21854399799999));
#335144=CARTESIAN_POINT('Ctrl Pts',(1.90510722499994,12.2,4.21711450499998));
#335145=CARTESIAN_POINT('Ctrl Pts',(1.90510722499994,5.2,4.21711450499998));
#335146=CARTESIAN_POINT('Ctrl Pts',(1.90510722499994,2.2,4.21711450499998));
#335147=CARTESIAN_POINT('Ctrl Pts',(1.90309404399994,12.2,4.21568494399998));
#335148=CARTESIAN_POINT('Ctrl Pts',(1.90309404399994,5.2,4.21568494399998));
#335149=CARTESIAN_POINT('Ctrl Pts',(1.90309404399994,2.2,4.21568494399998));
#335150=CARTESIAN_POINT('Ctrl Pts',(1.90108527799994,12.2,4.21425531899998));
#335151=CARTESIAN_POINT('Ctrl Pts',(1.90108527799994,5.2,4.21425531899998));
#335152=CARTESIAN_POINT('Ctrl Pts',(1.90108527799994,2.2,4.21425531899998));
#335153=CARTESIAN_POINT('Ctrl Pts',(1.89908093199994,12.2,4.21282564299998));
#335154=CARTESIAN_POINT('Ctrl Pts',(1.89908093199994,5.2,4.21282564299998));
#335155=CARTESIAN_POINT('Ctrl Pts',(1.89908093199994,2.2,4.21282564299998));
#335156=CARTESIAN_POINT('Ctrl Pts',(1.89708100499994,12.2,4.21139592399999));
#335157=CARTESIAN_POINT('Ctrl Pts',(1.89708100499994,5.2,4.21139592399999));
#335158=CARTESIAN_POINT('Ctrl Pts',(1.89708100499994,2.2,4.21139592399999));
#335159=CARTESIAN_POINT('Ctrl Pts',(1.89508549899994,12.2,4.20996617099998));
#335160=CARTESIAN_POINT('Ctrl Pts',(1.89508549899994,5.2,4.20996617099998));
#335161=CARTESIAN_POINT('Ctrl Pts',(1.89508549899994,2.2,4.20996617099998));
#335162=CARTESIAN_POINT('Ctrl Pts',(1.89309441499994,12.2,4.20853639299998));
#335163=CARTESIAN_POINT('Ctrl Pts',(1.89309441499994,5.2,4.20853639299998));
#335164=CARTESIAN_POINT('Ctrl Pts',(1.89309441499994,2.2,4.20853639299998));
#335165=CARTESIAN_POINT('Ctrl Pts',(1.89110775499994,12.2,4.20710659899999));
#335166=CARTESIAN_POINT('Ctrl Pts',(1.89110775499994,5.2,4.20710659899999));
#335167=CARTESIAN_POINT('Ctrl Pts',(1.89110775499994,2.2,4.20710659899999));
#335168=CARTESIAN_POINT('Ctrl Pts',(1.88912552099994,12.2,4.20567679799999));
#335169=CARTESIAN_POINT('Ctrl Pts',(1.88912552099994,5.2,4.20567679799999));
#335170=CARTESIAN_POINT('Ctrl Pts',(1.88912552099994,2.2,4.20567679799999));
#335171=CARTESIAN_POINT('Ctrl Pts',(1.88714771199994,12.2,4.20424700099999));
#335172=CARTESIAN_POINT('Ctrl Pts',(1.88714771199994,5.2,4.20424700099999));
#335173=CARTESIAN_POINT('Ctrl Pts',(1.88714771199994,2.2,4.20424700099999));
#335174=CARTESIAN_POINT('Ctrl Pts',(1.88517432999994,12.2,4.20281721399999));
#335175=CARTESIAN_POINT('Ctrl Pts',(1.88517432999994,5.2,4.20281721399999));
#335176=CARTESIAN_POINT('Ctrl Pts',(1.88517432999994,2.2,4.20281721399999));
#335177=CARTESIAN_POINT('Ctrl Pts',(1.88320537699994,12.2,4.20138744899998));
#335178=CARTESIAN_POINT('Ctrl Pts',(1.88320537699994,5.2,4.20138744899998));
#335179=CARTESIAN_POINT('Ctrl Pts',(1.88320537699994,2.2,4.20138744899998));
#335180=CARTESIAN_POINT('Ctrl Pts',(1.88124085599994,12.2,4.19995771299998));
#335181=CARTESIAN_POINT('Ctrl Pts',(1.88124085599994,5.2,4.19995771299998));
#335182=CARTESIAN_POINT('Ctrl Pts',(1.88124085599994,2.2,4.19995771299998));
#335183=CARTESIAN_POINT('Ctrl Pts',(1.87928076399994,12.2,4.19852801599998));
#335184=CARTESIAN_POINT('Ctrl Pts',(1.87928076399994,5.2,4.19852801599998));
#335185=CARTESIAN_POINT('Ctrl Pts',(1.87928076399994,2.2,4.19852801599998));
#335186=CARTESIAN_POINT('Ctrl Pts',(1.87732510499994,12.2,4.19709836799999));
#335187=CARTESIAN_POINT('Ctrl Pts',(1.87732510499994,5.2,4.19709836799999));
#335188=CARTESIAN_POINT('Ctrl Pts',(1.87732510499994,2.2,4.19709836799999));
#335189=CARTESIAN_POINT('Ctrl Pts',(1.87537387899994,12.2,4.19566877599999));
#335190=CARTESIAN_POINT('Ctrl Pts',(1.87537387899994,5.2,4.19566877599999));
#335191=CARTESIAN_POINT('Ctrl Pts',(1.87537387899994,2.2,4.19566877599999));
#335192=CARTESIAN_POINT('Ctrl Pts',(1.87342708999994,12.2,4.19423925199998));
#335193=CARTESIAN_POINT('Ctrl Pts',(1.87342708999994,5.2,4.19423925199998));
#335194=CARTESIAN_POINT('Ctrl Pts',(1.87342708999994,2.2,4.19423925199998));
#335195=CARTESIAN_POINT('Ctrl Pts',(1.87148473399994,12.2,4.19280980399999));
#335196=CARTESIAN_POINT('Ctrl Pts',(1.87148473399994,5.2,4.19280980399999));
#335197=CARTESIAN_POINT('Ctrl Pts',(1.87148473399994,2.2,4.19280980399999));
#335198=CARTESIAN_POINT('Ctrl Pts',(1.86954681799994,12.2,4.19138044099999));
#335199=CARTESIAN_POINT('Ctrl Pts',(1.86954681799994,5.2,4.19138044099999));
#335200=CARTESIAN_POINT('Ctrl Pts',(1.86954681799994,2.2,4.19138044099999));
#335201=CARTESIAN_POINT('Ctrl Pts',(1.86761333799994,12.2,4.18995117199999));
#335202=CARTESIAN_POINT('Ctrl Pts',(1.86761333799994,5.2,4.18995117199999));
#335203=CARTESIAN_POINT('Ctrl Pts',(1.86761333799994,2.2,4.18995117199999));
#335204=CARTESIAN_POINT('Ctrl Pts',(1.86568429899994,12.2,4.18852200699998));
#335205=CARTESIAN_POINT('Ctrl Pts',(1.86568429899994,5.2,4.18852200699998));
#335206=CARTESIAN_POINT('Ctrl Pts',(1.86568429899994,2.2,4.18852200699998));
#335207=CARTESIAN_POINT('Ctrl Pts',(1.86375969999994,12.2,4.18709295499998));
#335208=CARTESIAN_POINT('Ctrl Pts',(1.86375969999994,5.2,4.18709295499998));
#335209=CARTESIAN_POINT('Ctrl Pts',(1.86375969999994,2.2,4.18709295499998));
#335210=CARTESIAN_POINT('Ctrl Pts',(1.86183954399994,12.2,4.18566402599998));
#335211=CARTESIAN_POINT('Ctrl Pts',(1.86183954399994,5.2,4.18566402599998));
#335212=CARTESIAN_POINT('Ctrl Pts',(1.86183954399994,2.2,4.18566402599998));
#335213=CARTESIAN_POINT('Ctrl Pts',(1.85992382999994,12.2,4.18423522799999));
#335214=CARTESIAN_POINT('Ctrl Pts',(1.85992382999994,5.2,4.18423522799999));
#335215=CARTESIAN_POINT('Ctrl Pts',(1.85992382999994,2.2,4.18423522799999));
#335216=CARTESIAN_POINT('Ctrl Pts',(1.85801255999994,12.2,4.18280657099999));
#335217=CARTESIAN_POINT('Ctrl Pts',(1.85801255999994,5.2,4.18280657099999));
#335218=CARTESIAN_POINT('Ctrl Pts',(1.85801255999994,2.2,4.18280657099999));
#335219=CARTESIAN_POINT('Ctrl Pts',(1.85610573599994,12.2,4.18137806399999));
#335220=CARTESIAN_POINT('Ctrl Pts',(1.85610573599994,5.2,4.18137806399999));
#335221=CARTESIAN_POINT('Ctrl Pts',(1.85610573599994,2.2,4.18137806399999));
#335222=CARTESIAN_POINT('Ctrl Pts',(1.85420335799994,12.2,4.17994971699999));
#335223=CARTESIAN_POINT('Ctrl Pts',(1.85420335799994,5.2,4.17994971699999));
#335224=CARTESIAN_POINT('Ctrl Pts',(1.85420335799994,2.2,4.17994971699999));
#335225=CARTESIAN_POINT('Ctrl Pts',(1.85230542599994,12.2,4.17852153899998));
#335226=CARTESIAN_POINT('Ctrl Pts',(1.85230542599994,5.2,4.17852153899998));
#335227=CARTESIAN_POINT('Ctrl Pts',(1.85230542599994,2.2,4.17852153899998));
#335228=CARTESIAN_POINT('Ctrl Pts',(1.85041194399994,12.2,4.17709353899999));
#335229=CARTESIAN_POINT('Ctrl Pts',(1.85041194399994,5.2,4.17709353899999));
#335230=CARTESIAN_POINT('Ctrl Pts',(1.85041194399994,2.2,4.17709353899999));
#335231=CARTESIAN_POINT('Ctrl Pts',(1.84852290999994,12.2,4.17566572799998));
#335232=CARTESIAN_POINT('Ctrl Pts',(1.84852290999994,5.2,4.17566572799998));
#335233=CARTESIAN_POINT('Ctrl Pts',(1.84852290999994,2.2,4.17566572799998));
#335234=CARTESIAN_POINT('Ctrl Pts',(1.84663832699994,12.2,4.17423811299999));
#335235=CARTESIAN_POINT('Ctrl Pts',(1.84663832699994,5.2,4.17423811299999));
#335236=CARTESIAN_POINT('Ctrl Pts',(1.84663832699994,2.2,4.17423811299999));
#335237=CARTESIAN_POINT('Ctrl Pts',(1.84475819699994,12.2,4.17281070499998));
#335238=CARTESIAN_POINT('Ctrl Pts',(1.84475819699994,5.2,4.17281070499998));
#335239=CARTESIAN_POINT('Ctrl Pts',(1.84475819699994,2.2,4.17281070499998));
#335240=CARTESIAN_POINT('Ctrl Pts',(1.84288251799994,12.2,4.17138351299998));
#335241=CARTESIAN_POINT('Ctrl Pts',(1.84288251799994,5.2,4.17138351299998));
#335242=CARTESIAN_POINT('Ctrl Pts',(1.84288251799994,2.2,4.17138351299998));
#335243=CARTESIAN_POINT('Ctrl Pts',(1.84101129199994,12.2,4.16995654599998));
#335244=CARTESIAN_POINT('Ctrl Pts',(1.84101129199994,5.2,4.16995654599998));
#335245=CARTESIAN_POINT('Ctrl Pts',(1.84101129199994,2.2,4.16995654599998));
#335246=CARTESIAN_POINT('Ctrl Pts',(1.83914452199994,12.2,4.16852981599998));
#335247=CARTESIAN_POINT('Ctrl Pts',(1.83914452199994,5.2,4.16852981599998));
#335248=CARTESIAN_POINT('Ctrl Pts',(1.83914452199994,2.2,4.16852981599998));
#335249=CARTESIAN_POINT('Ctrl Pts',(1.83728220699995,12.2,4.16710332899999));
#335250=CARTESIAN_POINT('Ctrl Pts',(1.83728220699995,5.2,4.16710332899999));
#335251=CARTESIAN_POINT('Ctrl Pts',(1.83728220699995,2.2,4.16710332899999));
#335252=CARTESIAN_POINT('Ctrl Pts',(1.83542434799994,12.2,4.16567709499999));
#335253=CARTESIAN_POINT('Ctrl Pts',(1.83542434799994,5.2,4.16567709499999));
#335254=CARTESIAN_POINT('Ctrl Pts',(1.83542434799994,2.2,4.16567709499999));
#335255=CARTESIAN_POINT('Ctrl Pts',(1.83357094699994,12.2,4.16425112599998));
#335256=CARTESIAN_POINT('Ctrl Pts',(1.83357094699994,5.2,4.16425112599998));
#335257=CARTESIAN_POINT('Ctrl Pts',(1.83357094699994,2.2,4.16425112599998));
#335258=CARTESIAN_POINT('Ctrl Pts',(1.83172200399994,12.2,4.16282543099998));
#335259=CARTESIAN_POINT('Ctrl Pts',(1.83172200399994,5.2,4.16282543099998));
#335260=CARTESIAN_POINT('Ctrl Pts',(1.83172200399994,2.2,4.16282543099998));
#335261=CARTESIAN_POINT('Ctrl Pts',(1.82987752099994,12.2,4.16140001599998));
#335262=CARTESIAN_POINT('Ctrl Pts',(1.82987752099994,5.2,4.16140001599998));
#335263=CARTESIAN_POINT('Ctrl Pts',(1.82987752099994,2.2,4.16140001599998));
#335264=CARTESIAN_POINT('Ctrl Pts',(1.82803749799994,12.2,4.15997489499999));
#335265=CARTESIAN_POINT('Ctrl Pts',(1.82803749799994,5.2,4.15997489499999));
#335266=CARTESIAN_POINT('Ctrl Pts',(1.82803749799994,2.2,4.15997489499999));
#335267=CARTESIAN_POINT('Ctrl Pts',(1.82620193699994,12.2,4.15855007599998));
#335268=CARTESIAN_POINT('Ctrl Pts',(1.82620193699994,5.2,4.15855007599998));
#335269=CARTESIAN_POINT('Ctrl Pts',(1.82620193699994,2.2,4.15855007599998));
#335270=CARTESIAN_POINT('Ctrl Pts',(1.82437083599994,12.2,4.15712556699999));
#335271=CARTESIAN_POINT('Ctrl Pts',(1.82437083599994,5.2,4.15712556699999));
#335272=CARTESIAN_POINT('Ctrl Pts',(1.82437083599994,2.2,4.15712556699999));
#335273=CARTESIAN_POINT('Ctrl Pts',(1.82254419999994,12.2,4.15570137999998));
#335274=CARTESIAN_POINT('Ctrl Pts',(1.82254419999994,5.2,4.15570137999998));
#335275=CARTESIAN_POINT('Ctrl Pts',(1.82254419999994,2.2,4.15570137999998));
#335276=CARTESIAN_POINT('Ctrl Pts',(1.82072202699994,12.2,4.15427752199999));
#335277=CARTESIAN_POINT('Ctrl Pts',(1.82072202699994,5.2,4.15427752199999));
#335278=CARTESIAN_POINT('Ctrl Pts',(1.82072202699994,2.2,4.15427752199999));
#335279=CARTESIAN_POINT('Ctrl Pts',(1.81890431799994,12.2,4.15285400499998));
#335280=CARTESIAN_POINT('Ctrl Pts',(1.81890431799994,5.2,4.15285400499998));
#335281=CARTESIAN_POINT('Ctrl Pts',(1.81890431799994,2.2,4.15285400499998));
#335282=CARTESIAN_POINT('Ctrl Pts',(1.81709107599994,12.2,4.15143083799999));
#335283=CARTESIAN_POINT('Ctrl Pts',(1.81709107599994,5.2,4.15143083799999));
#335284=CARTESIAN_POINT('Ctrl Pts',(1.81709107599994,2.2,4.15143083799999));
#335285=CARTESIAN_POINT('Ctrl Pts',(1.81528230099994,12.2,4.15000802999998));
#335286=CARTESIAN_POINT('Ctrl Pts',(1.81528230099994,5.2,4.15000802999998));
#335287=CARTESIAN_POINT('Ctrl Pts',(1.81528230099994,2.2,4.15000802999998));
#335288=CARTESIAN_POINT('Ctrl Pts',(1.81347799099994,12.2,4.14858559099999));
#335289=CARTESIAN_POINT('Ctrl Pts',(1.81347799099994,5.2,4.14858559099999));
#335290=CARTESIAN_POINT('Ctrl Pts',(1.81347799099994,2.2,4.14858559099999));
#335291=CARTESIAN_POINT('Ctrl Pts',(1.81167815099994,12.2,4.14716353099998));
#335292=CARTESIAN_POINT('Ctrl Pts',(1.81167815099994,5.2,4.14716353099998));
#335293=CARTESIAN_POINT('Ctrl Pts',(1.81167815099994,2.2,4.14716353099998));
#335294=CARTESIAN_POINT('Ctrl Pts',(1.80988277899994,12.2,4.14574185999999));
#335295=CARTESIAN_POINT('Ctrl Pts',(1.80988277899994,5.2,4.14574185999999));
#335296=CARTESIAN_POINT('Ctrl Pts',(1.80988277899994,2.2,4.14574185999999));
#335297=CARTESIAN_POINT('Ctrl Pts',(1.80809187599994,12.2,4.14432058599999));
#335298=CARTESIAN_POINT('Ctrl Pts',(1.80809187599994,5.2,4.14432058599999));
#335299=CARTESIAN_POINT('Ctrl Pts',(1.80809187599994,2.2,4.14432058599999));
#335300=CARTESIAN_POINT('Ctrl Pts',(1.80630544499994,12.2,4.14289972099999));
#335301=CARTESIAN_POINT('Ctrl Pts',(1.80630544499994,5.2,4.14289972099999));
#335302=CARTESIAN_POINT('Ctrl Pts',(1.80630544499994,2.2,4.14289972099999));
#335303=CARTESIAN_POINT('Ctrl Pts',(1.80452348399994,12.2,4.14147927299998));
#335304=CARTESIAN_POINT('Ctrl Pts',(1.80452348399994,5.2,4.14147927299998));
#335305=CARTESIAN_POINT('Ctrl Pts',(1.80452348399994,2.2,4.14147927299998));
#335306=CARTESIAN_POINT('Ctrl Pts',(1.80274599599994,12.2,4.14005925299998));
#335307=CARTESIAN_POINT('Ctrl Pts',(1.80274599599994,5.2,4.14005925299998));
#335308=CARTESIAN_POINT('Ctrl Pts',(1.80274599599994,2.2,4.14005925299998));
#335309=CARTESIAN_POINT('Ctrl Pts',(1.80097298099994,12.2,4.13863966899999));
#335310=CARTESIAN_POINT('Ctrl Pts',(1.80097298099994,5.2,4.13863966899999));
#335311=CARTESIAN_POINT('Ctrl Pts',(1.80097298099994,2.2,4.13863966899999));
#335312=CARTESIAN_POINT('Ctrl Pts',(1.79920443899994,12.2,4.13722053299999));
#335313=CARTESIAN_POINT('Ctrl Pts',(1.79920443899994,5.2,4.13722053299999));
#335314=CARTESIAN_POINT('Ctrl Pts',(1.79920443899994,2.2,4.13722053299999));
#335315=CARTESIAN_POINT('Ctrl Pts',(1.79744036999994,12.2,4.13580185399999));
#335316=CARTESIAN_POINT('Ctrl Pts',(1.79744036999994,5.2,4.13580185399999));
#335317=CARTESIAN_POINT('Ctrl Pts',(1.79744036999994,2.2,4.13580185399999));
#335318=CARTESIAN_POINT('Ctrl Pts',(1.79568077699994,12.2,4.13438364099999));
#335319=CARTESIAN_POINT('Ctrl Pts',(1.79568077699994,5.2,4.13438364099999));
#335320=CARTESIAN_POINT('Ctrl Pts',(1.79568077699994,2.2,4.13438364099999));
#335321=CARTESIAN_POINT('Ctrl Pts',(1.79392565999994,12.2,4.13296590499999));
#335322=CARTESIAN_POINT('Ctrl Pts',(1.79392565999994,5.2,4.13296590499999));
#335323=CARTESIAN_POINT('Ctrl Pts',(1.79392565999994,2.2,4.13296590499999));
#335324=CARTESIAN_POINT('Ctrl Pts',(1.79217501899994,12.2,4.13154865399999));
#335325=CARTESIAN_POINT('Ctrl Pts',(1.79217501899994,5.2,4.13154865399999));
#335326=CARTESIAN_POINT('Ctrl Pts',(1.79217501899994,2.2,4.13154865399999));
#335327=CARTESIAN_POINT('Ctrl Pts',(1.79042885499994,12.2,4.13013189999998));
#335328=CARTESIAN_POINT('Ctrl Pts',(1.79042885499994,5.2,4.13013189999998));
#335329=CARTESIAN_POINT('Ctrl Pts',(1.79042885499994,2.2,4.13013189999998));
#335330=CARTESIAN_POINT('Ctrl Pts',(1.78868716699994,12.2,4.12871565099999));
#335331=CARTESIAN_POINT('Ctrl Pts',(1.78868716699994,5.2,4.12871565099999));
#335332=CARTESIAN_POINT('Ctrl Pts',(1.78868716699994,2.2,4.12871565099999));
#335333=CARTESIAN_POINT('Ctrl Pts',(1.78694995899994,12.2,4.12729991899998));
#335334=CARTESIAN_POINT('Ctrl Pts',(1.78694995899994,5.2,4.12729991899998));
#335335=CARTESIAN_POINT('Ctrl Pts',(1.78694995899994,2.2,4.12729991899998));
#335336=CARTESIAN_POINT('Ctrl Pts',(1.78521722999994,12.2,4.12588471199999));
#335337=CARTESIAN_POINT('Ctrl Pts',(1.78521722999994,5.2,4.12588471199999));
#335338=CARTESIAN_POINT('Ctrl Pts',(1.78521722999994,2.2,4.12588471199999));
#335339=CARTESIAN_POINT('Ctrl Pts',(1.78348897899994,12.2,4.12447004199999));
#335340=CARTESIAN_POINT('Ctrl Pts',(1.78348897899994,5.2,4.12447004199999));
#335341=CARTESIAN_POINT('Ctrl Pts',(1.78348897899994,2.2,4.12447004199999));
#335342=CARTESIAN_POINT('Ctrl Pts',(1.78176520999994,12.2,4.12305591599999));
#335343=CARTESIAN_POINT('Ctrl Pts',(1.78176520999994,5.2,4.12305591599999));
#335344=CARTESIAN_POINT('Ctrl Pts',(1.78176520999994,2.2,4.12305591599999));
#335345=CARTESIAN_POINT('Ctrl Pts',(1.78004591999994,12.2,4.12164234599998));
#335346=CARTESIAN_POINT('Ctrl Pts',(1.78004591999994,5.2,4.12164234599998));
#335347=CARTESIAN_POINT('Ctrl Pts',(1.78004591999994,2.2,4.12164234599998));
#335348=CARTESIAN_POINT('Ctrl Pts',(1.77833111199994,12.2,4.12022934299999));
#335349=CARTESIAN_POINT('Ctrl Pts',(1.77833111199994,5.2,4.12022934299999));
#335350=CARTESIAN_POINT('Ctrl Pts',(1.77833111199994,2.2,4.12022934299999));
#335351=CARTESIAN_POINT('Ctrl Pts',(1.77662078699994,12.2,4.11881691399999));
#335352=CARTESIAN_POINT('Ctrl Pts',(1.77662078699994,5.2,4.11881691399999));
#335353=CARTESIAN_POINT('Ctrl Pts',(1.77662078699994,2.2,4.11881691399999));
#335354=CARTESIAN_POINT('Ctrl Pts',(1.77491494299994,12.2,4.11740507099999));
#335355=CARTESIAN_POINT('Ctrl Pts',(1.77491494299994,5.2,4.11740507099999));
#335356=CARTESIAN_POINT('Ctrl Pts',(1.77491494299994,2.2,4.11740507099999));
#335357=CARTESIAN_POINT('Ctrl Pts',(1.77321358199995,12.2,4.11599382299999));
#335358=CARTESIAN_POINT('Ctrl Pts',(1.77321358199995,5.2,4.11599382299999));
#335359=CARTESIAN_POINT('Ctrl Pts',(1.77321358199995,2.2,4.11599382299999));
#335360=CARTESIAN_POINT('Ctrl Pts',(1.77151670499994,12.2,4.11458318099999));
#335361=CARTESIAN_POINT('Ctrl Pts',(1.77151670499994,5.2,4.11458318099999));
#335362=CARTESIAN_POINT('Ctrl Pts',(1.77151670499994,2.2,4.11458318099999));
#335363=CARTESIAN_POINT('Ctrl Pts',(1.76982431199994,12.2,4.11317315499999));
#335364=CARTESIAN_POINT('Ctrl Pts',(1.76982431199994,5.2,4.11317315499999));
#335365=CARTESIAN_POINT('Ctrl Pts',(1.76982431199994,2.2,4.11317315499999));
#335366=CARTESIAN_POINT('Ctrl Pts',(1.76813640399994,12.2,4.11176375399998));
#335367=CARTESIAN_POINT('Ctrl Pts',(1.76813640399994,5.2,4.11176375399998));
#335368=CARTESIAN_POINT('Ctrl Pts',(1.76813640399994,2.2,4.11176375399998));
#335369=CARTESIAN_POINT('Ctrl Pts',(1.76645298099994,12.2,4.11035498799999));
#335370=CARTESIAN_POINT('Ctrl Pts',(1.76645298099994,5.2,4.11035498799999));
#335371=CARTESIAN_POINT('Ctrl Pts',(1.76645298099994,2.2,4.11035498799999));
#335372=CARTESIAN_POINT('Ctrl Pts',(1.76477404199994,12.2,4.10894686899999));
#335373=CARTESIAN_POINT('Ctrl Pts',(1.76477404199994,5.2,4.10894686899999));
#335374=CARTESIAN_POINT('Ctrl Pts',(1.76477404199994,2.2,4.10894686899999));
#335375=CARTESIAN_POINT('Ctrl Pts',(1.76309958999994,12.2,4.10753940599999));
#335376=CARTESIAN_POINT('Ctrl Pts',(1.76309958999994,5.2,4.10753940599999));
#335377=CARTESIAN_POINT('Ctrl Pts',(1.76309958999994,2.2,4.10753940599999));
#335378=CARTESIAN_POINT('Ctrl Pts',(1.76142962399994,12.2,4.10613260699999));
#335379=CARTESIAN_POINT('Ctrl Pts',(1.76142962399994,5.2,4.10613260699999));
#335380=CARTESIAN_POINT('Ctrl Pts',(1.76142962399994,2.2,4.10613260699999));
#335381=CARTESIAN_POINT('Ctrl Pts',(1.75976414499994,12.2,4.10472648599999));
#335382=CARTESIAN_POINT('Ctrl Pts',(1.75976414499994,5.2,4.10472648599999));
#335383=CARTESIAN_POINT('Ctrl Pts',(1.75976414499994,2.2,4.10472648599999));
#335384=CARTESIAN_POINT('Ctrl Pts',(1.75810315299994,12.2,4.10332105199998));
#335385=CARTESIAN_POINT('Ctrl Pts',(1.75810315299994,5.2,4.10332105199998));
#335386=CARTESIAN_POINT('Ctrl Pts',(1.75810315299994,2.2,4.10332105199998));
#335387=CARTESIAN_POINT('Ctrl Pts',(1.75644664999994,12.2,4.10191631299998));
#335388=CARTESIAN_POINT('Ctrl Pts',(1.75644664999994,5.2,4.10191631299998));
#335389=CARTESIAN_POINT('Ctrl Pts',(1.75644664999994,2.2,4.10191631299998));
#335390=CARTESIAN_POINT('Ctrl Pts',(1.75479463399994,12.2,4.10051228099999));
#335391=CARTESIAN_POINT('Ctrl Pts',(1.75479463399994,5.2,4.10051228099999));
#335392=CARTESIAN_POINT('Ctrl Pts',(1.75479463399994,2.2,4.10051228099999));
#335393=CARTESIAN_POINT('Ctrl Pts',(1.75314710699994,12.2,4.09910896499999));
#335394=CARTESIAN_POINT('Ctrl Pts',(1.75314710699994,5.2,4.09910896499999));
#335395=CARTESIAN_POINT('Ctrl Pts',(1.75314710699994,2.2,4.09910896499999));
#335396=CARTESIAN_POINT('Ctrl Pts',(1.75150406799994,12.2,4.09770637699998));
#335397=CARTESIAN_POINT('Ctrl Pts',(1.75150406799994,5.2,4.09770637699998));
#335398=CARTESIAN_POINT('Ctrl Pts',(1.75150406799994,2.2,4.09770637699998));
#335399=CARTESIAN_POINT('Ctrl Pts',(1.74986551799994,12.2,4.09630452599998));
#335400=CARTESIAN_POINT('Ctrl Pts',(1.74986551799994,5.2,4.09630452599998));
#335401=CARTESIAN_POINT('Ctrl Pts',(1.74986551799994,2.2,4.09630452599998));
#335402=CARTESIAN_POINT('Ctrl Pts',(1.74823145899994,12.2,4.09490342299998));
#335403=CARTESIAN_POINT('Ctrl Pts',(1.74823145899994,5.2,4.09490342299998));
#335404=CARTESIAN_POINT('Ctrl Pts',(1.74823145899994,2.2,4.09490342299998));
#335405=CARTESIAN_POINT('Ctrl Pts',(1.74660188899994,12.2,4.09350307699999));
#335406=CARTESIAN_POINT('Ctrl Pts',(1.74660188899994,5.2,4.09350307699999));
#335407=CARTESIAN_POINT('Ctrl Pts',(1.74660188899994,2.2,4.09350307699999));
#335408=CARTESIAN_POINT('Ctrl Pts',(1.74497680899994,12.2,4.09210349899999));
#335409=CARTESIAN_POINT('Ctrl Pts',(1.74497680899994,5.2,4.09210349899999));
#335410=CARTESIAN_POINT('Ctrl Pts',(1.74497680899994,2.2,4.09210349899999));
#335411=CARTESIAN_POINT('Ctrl Pts',(1.74335621999994,12.2,4.09070469999998));
#335412=CARTESIAN_POINT('Ctrl Pts',(1.74335621999994,5.2,4.09070469999998));
#335413=CARTESIAN_POINT('Ctrl Pts',(1.74335621999994,2.2,4.09070469999998));
#335414=CARTESIAN_POINT('Ctrl Pts',(1.74174012099995,12.2,4.08930668899998));
#335415=CARTESIAN_POINT('Ctrl Pts',(1.74174012099995,5.2,4.08930668899998));
#335416=CARTESIAN_POINT('Ctrl Pts',(1.74174012099995,2.2,4.08930668899998));
#335417=CARTESIAN_POINT('Ctrl Pts',(1.74012851399994,12.2,4.08790947699998));
#335418=CARTESIAN_POINT('Ctrl Pts',(1.74012851399994,5.2,4.08790947699998));
#335419=CARTESIAN_POINT('Ctrl Pts',(1.74012851399994,2.2,4.08790947699998));
#335420=CARTESIAN_POINT('Ctrl Pts',(1.73852139799994,12.2,4.08651307499999));
#335421=CARTESIAN_POINT('Ctrl Pts',(1.73852139799994,5.2,4.08651307499999));
#335422=CARTESIAN_POINT('Ctrl Pts',(1.73852139799994,2.2,4.08651307499999));
#335423=CARTESIAN_POINT('Ctrl Pts',(1.73691877299994,12.2,4.08511749099999));
#335424=CARTESIAN_POINT('Ctrl Pts',(1.73691877299994,5.2,4.08511749099999));
#335425=CARTESIAN_POINT('Ctrl Pts',(1.73691877299994,2.2,4.08511749099999));
#335426=CARTESIAN_POINT('Ctrl Pts',(1.73532063999994,12.2,4.08372273799999));
#335427=CARTESIAN_POINT('Ctrl Pts',(1.73532063999994,5.2,4.08372273799999));
#335428=CARTESIAN_POINT('Ctrl Pts',(1.73532063999994,2.2,4.08372273799999));
#335429=CARTESIAN_POINT('Ctrl Pts',(1.73372699999994,12.2,4.08232882499998));
#335430=CARTESIAN_POINT('Ctrl Pts',(1.73372699999994,5.2,4.08232882499998));
#335431=CARTESIAN_POINT('Ctrl Pts',(1.73372699999994,2.2,4.08232882499998));
#335432=CARTESIAN_POINT('Ctrl Pts',(1.73213785099994,12.2,4.08093576299999));
#335433=CARTESIAN_POINT('Ctrl Pts',(1.73213785099994,5.2,4.08093576299999));
#335434=CARTESIAN_POINT('Ctrl Pts',(1.73213785099994,2.2,4.08093576299999));
#335435=CARTESIAN_POINT('Ctrl Pts',(1.73055319499994,12.2,4.07954356199999));
#335436=CARTESIAN_POINT('Ctrl Pts',(1.73055319499994,5.2,4.07954356199999));
#335437=CARTESIAN_POINT('Ctrl Pts',(1.73055319499994,2.2,4.07954356199999));
#335438=CARTESIAN_POINT('Ctrl Pts',(1.72897303099994,12.2,4.07815223299998));
#335439=CARTESIAN_POINT('Ctrl Pts',(1.72897303099994,5.2,4.07815223299998));
#335440=CARTESIAN_POINT('Ctrl Pts',(1.72897303099994,2.2,4.07815223299998));
#335441=CARTESIAN_POINT('Ctrl Pts',(1.72739736099994,12.2,4.07676178499998));
#335442=CARTESIAN_POINT('Ctrl Pts',(1.72739736099994,5.2,4.07676178499998));
#335443=CARTESIAN_POINT('Ctrl Pts',(1.72739736099994,2.2,4.07676178499998));
#335444=CARTESIAN_POINT('Ctrl Pts',(1.72582618299994,12.2,4.07537222999999));
#335445=CARTESIAN_POINT('Ctrl Pts',(1.72582618299994,5.2,4.07537222999999));
#335446=CARTESIAN_POINT('Ctrl Pts',(1.72582618299994,2.2,4.07537222999999));
#335447=CARTESIAN_POINT('Ctrl Pts',(1.72425949799994,12.2,4.07398357899999));
#335448=CARTESIAN_POINT('Ctrl Pts',(1.72425949799994,5.2,4.07398357899999));
#335449=CARTESIAN_POINT('Ctrl Pts',(1.72425949799994,2.2,4.07398357899999));
#335450=CARTESIAN_POINT('Ctrl Pts',(1.72269730599994,12.2,4.07259584099998));
#335451=CARTESIAN_POINT('Ctrl Pts',(1.72269730599994,5.2,4.07259584099998));
#335452=CARTESIAN_POINT('Ctrl Pts',(1.72269730599994,2.2,4.07259584099998));
#335453=CARTESIAN_POINT('Ctrl Pts',(1.72113960799994,12.2,4.07120902699998));
#335454=CARTESIAN_POINT('Ctrl Pts',(1.72113960799994,5.2,4.07120902699998));
#335455=CARTESIAN_POINT('Ctrl Pts',(1.72113960799994,2.2,4.07120902699998));
#335456=CARTESIAN_POINT('Ctrl Pts',(1.71958640299994,12.2,4.06982314599999));
#335457=CARTESIAN_POINT('Ctrl Pts',(1.71958640299994,5.2,4.06982314599999));
#335458=CARTESIAN_POINT('Ctrl Pts',(1.71958640299994,2.2,4.06982314599999));
#335459=CARTESIAN_POINT('Ctrl Pts',(1.71803769099994,12.2,4.06843821099999));
#335460=CARTESIAN_POINT('Ctrl Pts',(1.71803769099994,5.2,4.06843821099999));
#335461=CARTESIAN_POINT('Ctrl Pts',(1.71803769099994,2.2,4.06843821099999));
#335462=CARTESIAN_POINT('Ctrl Pts',(1.71649347299994,12.2,4.06705423199998));
#335463=CARTESIAN_POINT('Ctrl Pts',(1.71649347299994,5.2,4.06705423199998));
#335464=CARTESIAN_POINT('Ctrl Pts',(1.71649347299994,2.2,4.06705423199998));
#335465=CARTESIAN_POINT('Ctrl Pts',(1.71495374999994,12.2,4.06567121899998));
#335466=CARTESIAN_POINT('Ctrl Pts',(1.71495374999994,5.2,4.06567121899998));
#335467=CARTESIAN_POINT('Ctrl Pts',(1.71495374999994,2.2,4.06567121899998));
#335468=CARTESIAN_POINT('Ctrl Pts',(1.71341851899994,12.2,4.06428918299999));
#335469=CARTESIAN_POINT('Ctrl Pts',(1.71341851899994,5.2,4.06428918299999));
#335470=CARTESIAN_POINT('Ctrl Pts',(1.71341851899994,2.2,4.06428918299999));
#335471=CARTESIAN_POINT('Ctrl Pts',(1.71188778099994,12.2,4.06290813299999));
#335472=CARTESIAN_POINT('Ctrl Pts',(1.71188778099994,5.2,4.06290813299999));
#335473=CARTESIAN_POINT('Ctrl Pts',(1.71188778099994,2.2,4.06290813299999));
#335474=CARTESIAN_POINT('Ctrl Pts',(1.71036153799994,12.2,4.06152808299999));
#335475=CARTESIAN_POINT('Ctrl Pts',(1.71036153799994,5.2,4.06152808299999));
#335476=CARTESIAN_POINT('Ctrl Pts',(1.71036153799994,2.2,4.06152808299999));
#335477=CARTESIAN_POINT('Ctrl Pts',(1.70883978799994,12.2,4.06014904099998));
#335478=CARTESIAN_POINT('Ctrl Pts',(1.70883978799994,5.2,4.06014904099998));
#335479=CARTESIAN_POINT('Ctrl Pts',(1.70883978799994,2.2,4.06014904099998));
#335480=CARTESIAN_POINT('Ctrl Pts',(1.70732253199994,12.2,4.05877101799998));
#335481=CARTESIAN_POINT('Ctrl Pts',(1.70732253199994,5.2,4.05877101799998));
#335482=CARTESIAN_POINT('Ctrl Pts',(1.70732253199994,2.2,4.05877101799998));
#335483=CARTESIAN_POINT('Ctrl Pts',(1.70580976999994,12.2,4.05739402399998));
#335484=CARTESIAN_POINT('Ctrl Pts',(1.70580976999994,5.2,4.05739402399998));
#335485=CARTESIAN_POINT('Ctrl Pts',(1.70580976999994,2.2,4.05739402399998));
#335486=CARTESIAN_POINT('Ctrl Pts',(1.70430150099994,12.2,4.05601807199999));
#335487=CARTESIAN_POINT('Ctrl Pts',(1.70430150099994,5.2,4.05601807199999));
#335488=CARTESIAN_POINT('Ctrl Pts',(1.70430150099994,2.2,4.05601807199999));
#335489=CARTESIAN_POINT('Ctrl Pts',(1.70279772599994,12.2,4.05464317099998));
#335490=CARTESIAN_POINT('Ctrl Pts',(1.70279772599994,5.2,4.05464317099998));
#335491=CARTESIAN_POINT('Ctrl Pts',(1.70279772599994,2.2,4.05464317099998));
#335492=CARTESIAN_POINT('Ctrl Pts',(1.70129844399994,12.2,4.05326933199999));
#335493=CARTESIAN_POINT('Ctrl Pts',(1.70129844399994,5.2,4.05326933199999));
#335494=CARTESIAN_POINT('Ctrl Pts',(1.70129844399994,2.2,4.05326933199999));
#335495=CARTESIAN_POINT('Ctrl Pts',(1.69980365399994,12.2,4.05189656599998));
#335496=CARTESIAN_POINT('Ctrl Pts',(1.69980365399994,5.2,4.05189656599998));
#335497=CARTESIAN_POINT('Ctrl Pts',(1.69980365399994,2.2,4.05189656599998));
#335498=CARTESIAN_POINT('Ctrl Pts',(1.69831335899994,12.2,4.05052488299999));
#335499=CARTESIAN_POINT('Ctrl Pts',(1.69831335899994,5.2,4.05052488299999));
#335500=CARTESIAN_POINT('Ctrl Pts',(1.69831335899994,2.2,4.05052488299999));
#335501=CARTESIAN_POINT('Ctrl Pts',(1.69682755599994,12.2,4.04915429499999));
#335502=CARTESIAN_POINT('Ctrl Pts',(1.69682755599994,5.2,4.04915429499999));
#335503=CARTESIAN_POINT('Ctrl Pts',(1.69682755599994,2.2,4.04915429499999));
#335504=CARTESIAN_POINT('Ctrl Pts',(1.69534624699994,12.2,4.04778481099999));
#335505=CARTESIAN_POINT('Ctrl Pts',(1.69534624699994,5.2,4.04778481099999));
#335506=CARTESIAN_POINT('Ctrl Pts',(1.69534624699994,2.2,4.04778481099999));
#335507=CARTESIAN_POINT('Ctrl Pts',(1.69386942999994,12.2,4.04641644499999));
#335508=CARTESIAN_POINT('Ctrl Pts',(1.69386942999994,5.2,4.04641644499999));
#335509=CARTESIAN_POINT('Ctrl Pts',(1.69386942999994,2.2,4.04641644499999));
#335510=CARTESIAN_POINT('Ctrl Pts',(1.69239710499994,12.2,4.04504920399999));
#335511=CARTESIAN_POINT('Ctrl Pts',(1.69239710499994,5.2,4.04504920399999));
#335512=CARTESIAN_POINT('Ctrl Pts',(1.69239710499994,2.2,4.04504920399999));
#335513=CARTESIAN_POINT('Ctrl Pts',(1.69092927299994,12.2,4.04368310099999));
#335514=CARTESIAN_POINT('Ctrl Pts',(1.69092927299994,5.2,4.04368310099999));
#335515=CARTESIAN_POINT('Ctrl Pts',(1.69092927299994,2.2,4.04368310099999));
#335516=CARTESIAN_POINT('Ctrl Pts',(1.68946593399994,12.2,4.04231814699998));
#335517=CARTESIAN_POINT('Ctrl Pts',(1.68946593399994,5.2,4.04231814699998));
#335518=CARTESIAN_POINT('Ctrl Pts',(1.68946593399994,2.2,4.04231814699998));
#335519=CARTESIAN_POINT('Ctrl Pts',(1.68800708599994,12.2,4.04095435199999));
#335520=CARTESIAN_POINT('Ctrl Pts',(1.68800708599994,5.2,4.04095435199999));
#335521=CARTESIAN_POINT('Ctrl Pts',(1.68800708599994,2.2,4.04095435199999));
#335522=CARTESIAN_POINT('Ctrl Pts',(1.68655272999994,12.2,4.03959172699999));
#335523=CARTESIAN_POINT('Ctrl Pts',(1.68655272999994,5.2,4.03959172699999));
#335524=CARTESIAN_POINT('Ctrl Pts',(1.68655272999994,2.2,4.03959172699999));
#335525=CARTESIAN_POINT('Ctrl Pts',(1.68510286499994,12.2,4.03823028399999));
#335526=CARTESIAN_POINT('Ctrl Pts',(1.68510286499994,5.2,4.03823028399999));
#335527=CARTESIAN_POINT('Ctrl Pts',(1.68510286499994,2.2,4.03823028399999));
#335528=CARTESIAN_POINT('Ctrl Pts',(1.68365749299994,12.2,4.03687003199998));
#335529=CARTESIAN_POINT('Ctrl Pts',(1.68365749299994,5.2,4.03687003199998));
#335530=CARTESIAN_POINT('Ctrl Pts',(1.68365749299994,2.2,4.03687003199998));
#335531=CARTESIAN_POINT('Ctrl Pts',(1.68221660999994,12.2,4.03551098399999));
#335532=CARTESIAN_POINT('Ctrl Pts',(1.68221660999994,5.2,4.03551098399999));
#335533=CARTESIAN_POINT('Ctrl Pts',(1.68221660999994,2.2,4.03551098399999));
#335534=CARTESIAN_POINT('Ctrl Pts',(1.68078021899994,12.2,4.03415314999998));
#335535=CARTESIAN_POINT('Ctrl Pts',(1.68078021899994,5.2,4.03415314999998));
#335536=CARTESIAN_POINT('Ctrl Pts',(1.68078021899994,2.2,4.03415314999998));
#335537=CARTESIAN_POINT('Ctrl Pts',(1.67934831799994,12.2,4.03279653999999));
#335538=CARTESIAN_POINT('Ctrl Pts',(1.67934831799994,5.2,4.03279653999999));
#335539=CARTESIAN_POINT('Ctrl Pts',(1.67934831799994,2.2,4.03279653999999));
#335540=CARTESIAN_POINT('Ctrl Pts',(1.67792090699994,12.2,4.03144116699998));
#335541=CARTESIAN_POINT('Ctrl Pts',(1.67792090699994,5.2,4.03144116699998));
#335542=CARTESIAN_POINT('Ctrl Pts',(1.67792090699994,2.2,4.03144116699998));
#335543=CARTESIAN_POINT('Ctrl Pts',(1.67649798599994,12.2,4.03008703999999));
#335544=CARTESIAN_POINT('Ctrl Pts',(1.67649798599994,5.2,4.03008703999999));
#335545=CARTESIAN_POINT('Ctrl Pts',(1.67649798599994,2.2,4.03008703999999));
#335546=CARTESIAN_POINT('Ctrl Pts',(1.67507955399994,12.2,4.02873417099999));
#335547=CARTESIAN_POINT('Ctrl Pts',(1.67507955399994,5.2,4.02873417099999));
#335548=CARTESIAN_POINT('Ctrl Pts',(1.67507955399994,2.2,4.02873417099999));
#335549=CARTESIAN_POINT('Ctrl Pts',(1.67366561099994,12.2,4.02738257199999));
#335550=CARTESIAN_POINT('Ctrl Pts',(1.67366561099994,5.2,4.02738257199999));
#335551=CARTESIAN_POINT('Ctrl Pts',(1.67366561099994,2.2,4.02738257199999));
#335552=CARTESIAN_POINT('Ctrl Pts',(1.67225615599994,12.2,4.02603225199999));
#335553=CARTESIAN_POINT('Ctrl Pts',(1.67225615599994,5.2,4.02603225199999));
#335554=CARTESIAN_POINT('Ctrl Pts',(1.67225615599994,2.2,4.02603225199999));
#335555=CARTESIAN_POINT('Ctrl Pts',(1.67085118999994,12.2,4.02468322399999));
#335556=CARTESIAN_POINT('Ctrl Pts',(1.67085118999994,5.2,4.02468322399999));
#335557=CARTESIAN_POINT('Ctrl Pts',(1.67085118999994,2.2,4.02468322399999));
#335558=CARTESIAN_POINT('Ctrl Pts',(1.66945071199994,12.2,4.02333549799998));
#335559=CARTESIAN_POINT('Ctrl Pts',(1.66945071199994,5.2,4.02333549799998));
#335560=CARTESIAN_POINT('Ctrl Pts',(1.66945071199994,2.2,4.02333549799998));
#335561=CARTESIAN_POINT('Ctrl Pts',(1.66805472199994,12.2,4.02198908599999));
#335562=CARTESIAN_POINT('Ctrl Pts',(1.66805472199994,5.2,4.02198908599999));
#335563=CARTESIAN_POINT('Ctrl Pts',(1.66805472199994,2.2,4.02198908599999));
#335564=CARTESIAN_POINT('Ctrl Pts',(1.66666321699994,12.2,4.02064399699999));
#335565=CARTESIAN_POINT('Ctrl Pts',(1.66666321699994,5.2,4.02064399699999));
#335566=CARTESIAN_POINT('Ctrl Pts',(1.66666321699994,2.2,4.02064399699999));
#335567=CARTESIAN_POINT('Ctrl Pts',(1.66527619999994,12.2,4.01930024499999));
#335568=CARTESIAN_POINT('Ctrl Pts',(1.66527619999994,5.2,4.01930024499999));
#335569=CARTESIAN_POINT('Ctrl Pts',(1.66527619999994,2.2,4.01930024499999));
#335570=CARTESIAN_POINT('Ctrl Pts',(1.66389366899994,12.2,4.01795783999999));
#335571=CARTESIAN_POINT('Ctrl Pts',(1.66389366899994,5.2,4.01795783999999));
#335572=CARTESIAN_POINT('Ctrl Pts',(1.66389366899994,2.2,4.01795783999999));
#335573=CARTESIAN_POINT('Ctrl Pts',(1.66251562299994,12.2,4.01661679299998));
#335574=CARTESIAN_POINT('Ctrl Pts',(1.66251562299994,5.2,4.01661679299998));
#335575=CARTESIAN_POINT('Ctrl Pts',(1.66251562299994,2.2,4.01661679299998));
#335576=CARTESIAN_POINT('Ctrl Pts',(1.66114206199994,12.2,4.01527711499998));
#335577=CARTESIAN_POINT('Ctrl Pts',(1.66114206199994,5.2,4.01527711499998));
#335578=CARTESIAN_POINT('Ctrl Pts',(1.66114206199994,2.2,4.01527711499998));
#335579=CARTESIAN_POINT('Ctrl Pts',(1.65977298499994,12.2,4.01393881699998));
#335580=CARTESIAN_POINT('Ctrl Pts',(1.65977298499994,5.2,4.01393881699998));
#335581=CARTESIAN_POINT('Ctrl Pts',(1.65977298499994,2.2,4.01393881699998));
#335582=CARTESIAN_POINT('Ctrl Pts',(1.65840839199994,12.2,4.01260191099999));
#335583=CARTESIAN_POINT('Ctrl Pts',(1.65840839199994,5.2,4.01260191099999));
#335584=CARTESIAN_POINT('Ctrl Pts',(1.65840839199994,2.2,4.01260191099999));
#335585=CARTESIAN_POINT('Ctrl Pts',(1.65704828299994,12.2,4.01126640799998));
#335586=CARTESIAN_POINT('Ctrl Pts',(1.65704828299994,5.2,4.01126640799998));
#335587=CARTESIAN_POINT('Ctrl Pts',(1.65704828299994,2.2,4.01126640799998));
#335588=CARTESIAN_POINT('Ctrl Pts',(1.65569265599994,12.2,4.00993231999998));
#335589=CARTESIAN_POINT('Ctrl Pts',(1.65569265599994,5.2,4.00993231999998));
#335590=CARTESIAN_POINT('Ctrl Pts',(1.65569265599994,2.2,4.00993231999998));
#335591=CARTESIAN_POINT('Ctrl Pts',(1.65434151199994,12.2,4.00859965599999));
#335592=CARTESIAN_POINT('Ctrl Pts',(1.65434151199994,5.2,4.00859965599999));
#335593=CARTESIAN_POINT('Ctrl Pts',(1.65434151199994,2.2,4.00859965599999));
#335594=CARTESIAN_POINT('Ctrl Pts',(1.65299484899994,12.2,4.00726843099999));
#335595=CARTESIAN_POINT('Ctrl Pts',(1.65299484899994,5.2,4.00726843099999));
#335596=CARTESIAN_POINT('Ctrl Pts',(1.65299484899994,2.2,4.00726843099999));
#335597=CARTESIAN_POINT('Ctrl Pts',(1.65165266699994,12.2,4.00593865299999));
#335598=CARTESIAN_POINT('Ctrl Pts',(1.65165266699994,5.2,4.00593865299999));
#335599=CARTESIAN_POINT('Ctrl Pts',(1.65165266699994,2.2,4.00593865299999));
#335600=CARTESIAN_POINT('Ctrl Pts',(1.65031496599994,12.2,4.00461033499998));
#335601=CARTESIAN_POINT('Ctrl Pts',(1.65031496599994,5.2,4.00461033499998));
#335602=CARTESIAN_POINT('Ctrl Pts',(1.65031496599994,2.2,4.00461033499998));
#335603=CARTESIAN_POINT('Ctrl Pts',(1.64898174299994,12.2,4.00328348699999));
#335604=CARTESIAN_POINT('Ctrl Pts',(1.64898174299994,5.2,4.00328348699999));
#335605=CARTESIAN_POINT('Ctrl Pts',(1.64898174299994,2.2,4.00328348699999));
#335606=CARTESIAN_POINT('Ctrl Pts',(1.64765300099994,12.2,4.00195812199998));
#335607=CARTESIAN_POINT('Ctrl Pts',(1.64765300099994,5.2,4.00195812199998));
#335608=CARTESIAN_POINT('Ctrl Pts',(1.64765300099994,2.2,4.00195812199998));
#335609=CARTESIAN_POINT('Ctrl Pts',(1.64632873599994,12.2,4.00063424999999));
#335610=CARTESIAN_POINT('Ctrl Pts',(1.64632873599994,5.2,4.00063424999999));
#335611=CARTESIAN_POINT('Ctrl Pts',(1.64632873599994,2.2,4.00063424999999));
#335612=CARTESIAN_POINT('Ctrl Pts',(1.64500894899994,12.2,3.99931188399999));
#335613=CARTESIAN_POINT('Ctrl Pts',(1.64500894899994,5.2,3.99931188399999));
#335614=CARTESIAN_POINT('Ctrl Pts',(1.64500894899994,2.2,3.99931188399999));
#335615=CARTESIAN_POINT('Ctrl Pts',(1.64369363799994,12.2,3.99799103399998));
#335616=CARTESIAN_POINT('Ctrl Pts',(1.64369363799994,5.2,3.99799103399998));
#335617=CARTESIAN_POINT('Ctrl Pts',(1.64369363799994,2.2,3.99799103399998));
#335618=CARTESIAN_POINT('Ctrl Pts',(1.64238280299994,12.2,3.99667171299999));
#335619=CARTESIAN_POINT('Ctrl Pts',(1.64238280299994,5.2,3.99667171299999));
#335620=CARTESIAN_POINT('Ctrl Pts',(1.64238280299994,2.2,3.99667171299999));
#335621=CARTESIAN_POINT('Ctrl Pts',(1.64107644399994,12.2,3.99535393099999));
#335622=CARTESIAN_POINT('Ctrl Pts',(1.64107644399994,5.2,3.99535393099999));
#335623=CARTESIAN_POINT('Ctrl Pts',(1.64107644399994,2.2,3.99535393099999));
#335624=CARTESIAN_POINT('Ctrl Pts',(1.63977455999994,12.2,3.99403769999999));
#335625=CARTESIAN_POINT('Ctrl Pts',(1.63977455999994,5.2,3.99403769999999));
#335626=CARTESIAN_POINT('Ctrl Pts',(1.63977455999994,2.2,3.99403769999999));
#335627=CARTESIAN_POINT('Ctrl Pts',(1.63847714899994,12.2,3.99272303099998));
#335628=CARTESIAN_POINT('Ctrl Pts',(1.63847714899994,5.2,3.99272303099998));
#335629=CARTESIAN_POINT('Ctrl Pts',(1.63847714899994,2.2,3.99272303099998));
#335630=CARTESIAN_POINT('Ctrl Pts',(1.63718421099994,12.2,3.99140993699999));
#335631=CARTESIAN_POINT('Ctrl Pts',(1.63718421099994,5.2,3.99140993699999));
#335632=CARTESIAN_POINT('Ctrl Pts',(1.63718421099994,2.2,3.99140993699999));
#335633=CARTESIAN_POINT('Ctrl Pts',(1.63589574499994,12.2,3.99009842799998));
#335634=CARTESIAN_POINT('Ctrl Pts',(1.63589574499994,5.2,3.99009842799998));
#335635=CARTESIAN_POINT('Ctrl Pts',(1.63589574499994,2.2,3.99009842799998));
#335636=CARTESIAN_POINT('Ctrl Pts',(1.63461175099994,12.2,3.98878851599999));
#335637=CARTESIAN_POINT('Ctrl Pts',(1.63461175099994,5.2,3.98878851599999));
#335638=CARTESIAN_POINT('Ctrl Pts',(1.63461175099994,2.2,3.98878851599999));
#335639=CARTESIAN_POINT('Ctrl Pts',(1.63333222699994,12.2,3.98748021299999));
#335640=CARTESIAN_POINT('Ctrl Pts',(1.63333222699994,5.2,3.98748021299999));
#335641=CARTESIAN_POINT('Ctrl Pts',(1.63333222699994,2.2,3.98748021299999));
#335642=CARTESIAN_POINT('Ctrl Pts',(1.63205717199994,12.2,3.98617353099999));
#335643=CARTESIAN_POINT('Ctrl Pts',(1.63205717199994,5.2,3.98617353099999));
#335644=CARTESIAN_POINT('Ctrl Pts',(1.63205717199994,2.2,3.98617353099999));
#335645=CARTESIAN_POINT('Ctrl Pts',(1.63078658599994,12.2,3.98486848099999));
#335646=CARTESIAN_POINT('Ctrl Pts',(1.63078658599994,5.2,3.98486848099999));
#335647=CARTESIAN_POINT('Ctrl Pts',(1.63078658599994,2.2,3.98486848099999));
#335648=CARTESIAN_POINT('Ctrl Pts',(1.62952046699994,12.2,3.98356507399999));
#335649=CARTESIAN_POINT('Ctrl Pts',(1.62952046699994,5.2,3.98356507399999));
#335650=CARTESIAN_POINT('Ctrl Pts',(1.62952046699994,2.2,3.98356507399999));
#335651=CARTESIAN_POINT('Ctrl Pts',(1.62825881599994,12.2,3.98226332299998));
#335652=CARTESIAN_POINT('Ctrl Pts',(1.62825881599994,5.2,3.98226332299998));
#335653=CARTESIAN_POINT('Ctrl Pts',(1.62825881599994,2.2,3.98226332299998));
#335654=CARTESIAN_POINT('Ctrl Pts',(1.62700162999994,12.2,3.98096323799999));
#335655=CARTESIAN_POINT('Ctrl Pts',(1.62700162999994,5.2,3.98096323799999));
#335656=CARTESIAN_POINT('Ctrl Pts',(1.62700162999994,2.2,3.98096323799999));
#335657=CARTESIAN_POINT('Ctrl Pts',(1.62574890899994,12.2,3.97966483299999));
#335658=CARTESIAN_POINT('Ctrl Pts',(1.62574890899994,5.2,3.97966483299999));
#335659=CARTESIAN_POINT('Ctrl Pts',(1.62574890899994,2.2,3.97966483299999));
#335660=CARTESIAN_POINT('Ctrl Pts',(1.62450065199994,12.2,3.97836811799999));
#335661=CARTESIAN_POINT('Ctrl Pts',(1.62450065199994,5.2,3.97836811799999));
#335662=CARTESIAN_POINT('Ctrl Pts',(1.62450065199994,2.2,3.97836811799999));
#335663=CARTESIAN_POINT('Ctrl Pts',(1.62325685899994,12.2,3.97707310499998));
#335664=CARTESIAN_POINT('Ctrl Pts',(1.62325685899994,5.2,3.97707310499998));
#335665=CARTESIAN_POINT('Ctrl Pts',(1.62325685899994,2.2,3.97707310499998));
#335666=CARTESIAN_POINT('Ctrl Pts',(1.62201752599994,12.2,3.97577980599999));
#335667=CARTESIAN_POINT('Ctrl Pts',(1.62201752599994,5.2,3.97577980599999));
#335668=CARTESIAN_POINT('Ctrl Pts',(1.62201752599994,2.2,3.97577980599999));
#335669=CARTESIAN_POINT('Ctrl Pts',(1.62078265399994,12.2,3.97448823299998));
#335670=CARTESIAN_POINT('Ctrl Pts',(1.62078265399994,5.2,3.97448823299998));
#335671=CARTESIAN_POINT('Ctrl Pts',(1.62078265399994,2.2,3.97448823299998));
#335672=CARTESIAN_POINT('Ctrl Pts',(1.61955224199994,12.2,3.97319839699998));
#335673=CARTESIAN_POINT('Ctrl Pts',(1.61955224199994,5.2,3.97319839699998));
#335674=CARTESIAN_POINT('Ctrl Pts',(1.61955224199994,2.2,3.97319839699998));
#335675=CARTESIAN_POINT('Ctrl Pts',(1.61832628899994,12.2,3.97191031099998));
#335676=CARTESIAN_POINT('Ctrl Pts',(1.61832628899994,5.2,3.97191031099998));
#335677=CARTESIAN_POINT('Ctrl Pts',(1.61832628899994,2.2,3.97191031099998));
#335678=CARTESIAN_POINT('Ctrl Pts',(1.61710479299994,12.2,3.97062398599999));
#335679=CARTESIAN_POINT('Ctrl Pts',(1.61710479299994,5.2,3.97062398599999));
#335680=CARTESIAN_POINT('Ctrl Pts',(1.61710479299994,2.2,3.97062398599999));
#335681=CARTESIAN_POINT('Ctrl Pts',(1.61588775399994,12.2,3.96933943399999));
#335682=CARTESIAN_POINT('Ctrl Pts',(1.61588775399994,5.2,3.96933943399999));
#335683=CARTESIAN_POINT('Ctrl Pts',(1.61588775399994,2.2,3.96933943399999));
#335684=CARTESIAN_POINT('Ctrl Pts',(1.61467517099994,12.2,3.96805666699999));
#335685=CARTESIAN_POINT('Ctrl Pts',(1.61467517099994,5.2,3.96805666699999));
#335686=CARTESIAN_POINT('Ctrl Pts',(1.61467517099994,2.2,3.96805666699999));
#335687=CARTESIAN_POINT('Ctrl Pts',(1.61346704099994,12.2,3.96677569699998));
#335688=CARTESIAN_POINT('Ctrl Pts',(1.61346704099994,5.2,3.96677569699998));
#335689=CARTESIAN_POINT('Ctrl Pts',(1.61346704099994,2.2,3.96677569699998));
#335690=CARTESIAN_POINT('Ctrl Pts',(1.61226336499994,12.2,3.96549653599998));
#335691=CARTESIAN_POINT('Ctrl Pts',(1.61226336499994,5.2,3.96549653599998));
#335692=CARTESIAN_POINT('Ctrl Pts',(1.61226336499994,2.2,3.96549653599998));
#335693=CARTESIAN_POINT('Ctrl Pts',(1.61106413999994,12.2,3.96421919499998));
#335694=CARTESIAN_POINT('Ctrl Pts',(1.61106413999994,5.2,3.96421919499998));
#335695=CARTESIAN_POINT('Ctrl Pts',(1.61106413999994,2.2,3.96421919499998));
#335696=CARTESIAN_POINT('Ctrl Pts',(1.60986936499994,12.2,3.96294368699999));
#335697=CARTESIAN_POINT('Ctrl Pts',(1.60986936499994,5.2,3.96294368699999));
#335698=CARTESIAN_POINT('Ctrl Pts',(1.60986936499994,2.2,3.96294368699999));
#335699=CARTESIAN_POINT('Ctrl Pts',(1.60867904099994,12.2,3.96167002399999));
#335700=CARTESIAN_POINT('Ctrl Pts',(1.60867904099994,5.2,3.96167002399999));
#335701=CARTESIAN_POINT('Ctrl Pts',(1.60867904099994,2.2,3.96167002399999));
#335702=CARTESIAN_POINT('Ctrl Pts',(1.60749316499994,12.2,3.96039821699999));
#335703=CARTESIAN_POINT('Ctrl Pts',(1.60749316499994,5.2,3.96039821699999));
#335704=CARTESIAN_POINT('Ctrl Pts',(1.60749316499994,2.2,3.96039821699999));
#335705=CARTESIAN_POINT('Ctrl Pts',(1.60631173599994,12.2,3.95912827899998));
#335706=CARTESIAN_POINT('Ctrl Pts',(1.60631173599994,5.2,3.95912827899998));
#335707=CARTESIAN_POINT('Ctrl Pts',(1.60631173599994,2.2,3.95912827899998));
#335708=CARTESIAN_POINT('Ctrl Pts',(1.60513475099994,12.2,3.95786022099998));
#335709=CARTESIAN_POINT('Ctrl Pts',(1.60513475099994,5.2,3.95786022099998));
#335710=CARTESIAN_POINT('Ctrl Pts',(1.60513475099994,2.2,3.95786022099998));
#335711=CARTESIAN_POINT('Ctrl Pts',(1.60396221199994,12.2,3.95659405699998));
#335712=CARTESIAN_POINT('Ctrl Pts',(1.60396221199994,5.2,3.95659405699998));
#335713=CARTESIAN_POINT('Ctrl Pts',(1.60396221199994,2.2,3.95659405699998));
#335714=CARTESIAN_POINT('Ctrl Pts',(1.60279411499994,12.2,3.95532979699999));
#335715=CARTESIAN_POINT('Ctrl Pts',(1.60279411499994,5.2,3.95532979699999));
#335716=CARTESIAN_POINT('Ctrl Pts',(1.60279411499994,2.2,3.95532979699999));
#335717=CARTESIAN_POINT('Ctrl Pts',(1.60163045999994,12.2,3.95406745399999));
#335718=CARTESIAN_POINT('Ctrl Pts',(1.60163045999994,5.2,3.95406745399999));
#335719=CARTESIAN_POINT('Ctrl Pts',(1.60163045999994,2.2,3.95406745399999));
#335720=CARTESIAN_POINT('Ctrl Pts',(1.60047124599994,12.2,3.95280703999998));
#335721=CARTESIAN_POINT('Ctrl Pts',(1.60047124599994,5.2,3.95280703999998));
#335722=CARTESIAN_POINT('Ctrl Pts',(1.60047124599994,2.2,3.95280703999998));
#335723=CARTESIAN_POINT('Ctrl Pts',(1.59931646999994,12.2,3.95154856899998));
#335724=CARTESIAN_POINT('Ctrl Pts',(1.59931646999994,5.2,3.95154856899998));
#335725=CARTESIAN_POINT('Ctrl Pts',(1.59931646999994,2.2,3.95154856899998));
#335726=CARTESIAN_POINT('Ctrl Pts',(1.59816613199994,12.2,3.95029204999998));
#335727=CARTESIAN_POINT('Ctrl Pts',(1.59816613199994,5.2,3.95029204999998));
#335728=CARTESIAN_POINT('Ctrl Pts',(1.59816613199994,2.2,3.95029204999998));
#335729=CARTESIAN_POINT('Ctrl Pts',(1.59702023099994,12.2,3.94903749599998));
#335730=CARTESIAN_POINT('Ctrl Pts',(1.59702023099994,5.2,3.94903749599998));
#335731=CARTESIAN_POINT('Ctrl Pts',(1.59702023099994,2.2,3.94903749599998));
#335732=CARTESIAN_POINT('Ctrl Pts',(1.59587876399994,12.2,3.94778491999999));
#335733=CARTESIAN_POINT('Ctrl Pts',(1.59587876399994,5.2,3.94778491999999));
#335734=CARTESIAN_POINT('Ctrl Pts',(1.59587876399994,2.2,3.94778491999999));
#335735=CARTESIAN_POINT('Ctrl Pts',(1.59474173099994,12.2,3.94653433399998));
#335736=CARTESIAN_POINT('Ctrl Pts',(1.59474173099994,5.2,3.94653433399998));
#335737=CARTESIAN_POINT('Ctrl Pts',(1.59474173099994,2.2,3.94653433399998));
#335738=CARTESIAN_POINT('Ctrl Pts',(1.59360912799994,12.2,3.94528574999998));
#335739=CARTESIAN_POINT('Ctrl Pts',(1.59360912799994,5.2,3.94528574999998));
#335740=CARTESIAN_POINT('Ctrl Pts',(1.59360912799994,2.2,3.94528574999998));
#335741=CARTESIAN_POINT('Ctrl Pts',(1.59248095699994,12.2,3.94403918099999));
#335742=CARTESIAN_POINT('Ctrl Pts',(1.59248095699994,5.2,3.94403918099999));
#335743=CARTESIAN_POINT('Ctrl Pts',(1.59248095699994,2.2,3.94403918099999));
#335744=CARTESIAN_POINT('Ctrl Pts',(1.59135721499994,12.2,3.94279463799998));
#335745=CARTESIAN_POINT('Ctrl Pts',(1.59135721499994,5.2,3.94279463799998));
#335746=CARTESIAN_POINT('Ctrl Pts',(1.59135721499994,2.2,3.94279463799998));
#335747=CARTESIAN_POINT('Ctrl Pts',(1.59023789999994,12.2,3.94155213499998));
#335748=CARTESIAN_POINT('Ctrl Pts',(1.59023789999994,5.2,3.94155213499998));
#335749=CARTESIAN_POINT('Ctrl Pts',(1.59023789999994,2.2,3.94155213499998));
#335750=CARTESIAN_POINT('Ctrl Pts',(1.58912301099994,12.2,3.94031168199999));
#335751=CARTESIAN_POINT('Ctrl Pts',(1.58912301099994,5.2,3.94031168199999));
#335752=CARTESIAN_POINT('Ctrl Pts',(1.58912301099994,2.2,3.94031168199999));
#335753=CARTESIAN_POINT('Ctrl Pts',(1.58801254499994,12.2,3.93907329399998));
#335754=CARTESIAN_POINT('Ctrl Pts',(1.58801254499994,5.2,3.93907329399998));
#335755=CARTESIAN_POINT('Ctrl Pts',(1.58801254499994,2.2,3.93907329399998));
#335756=CARTESIAN_POINT('Ctrl Pts',(1.58690650299994,12.2,3.93783698099998));
#335757=CARTESIAN_POINT('Ctrl Pts',(1.58690650299994,5.2,3.93783698099998));
#335758=CARTESIAN_POINT('Ctrl Pts',(1.58690650299994,2.2,3.93783698099998));
#335759=CARTESIAN_POINT('Ctrl Pts',(1.58580488199994,12.2,3.93660275799999));
#335760=CARTESIAN_POINT('Ctrl Pts',(1.58580488199994,5.2,3.93660275799999));
#335761=CARTESIAN_POINT('Ctrl Pts',(1.58580488199994,2.2,3.93660275799999));
#335762=CARTESIAN_POINT('Ctrl Pts',(1.58470767999994,12.2,3.93537063399998));
#335763=CARTESIAN_POINT('Ctrl Pts',(1.58470767999994,5.2,3.93537063399998));
#335764=CARTESIAN_POINT('Ctrl Pts',(1.58470767999994,2.2,3.93537063399998));
#335765=CARTESIAN_POINT('Ctrl Pts',(1.58361489599994,12.2,3.93414062499998));
#335766=CARTESIAN_POINT('Ctrl Pts',(1.58361489599994,5.2,3.93414062499998));
#335767=CARTESIAN_POINT('Ctrl Pts',(1.58361489599994,2.2,3.93414062499998));
#335768=CARTESIAN_POINT('Ctrl Pts',(1.58252652799994,12.2,3.93291274099998));
#335769=CARTESIAN_POINT('Ctrl Pts',(1.58252652799994,5.2,3.93291274099998));
#335770=CARTESIAN_POINT('Ctrl Pts',(1.58252652799994,2.2,3.93291274099998));
#335771=CARTESIAN_POINT('Ctrl Pts',(1.58144257399994,12.2,3.93168699499999));
#335772=CARTESIAN_POINT('Ctrl Pts',(1.58144257399994,5.2,3.93168699499999));
#335773=CARTESIAN_POINT('Ctrl Pts',(1.58144257399994,2.2,3.93168699499999));
#335774=CARTESIAN_POINT('Ctrl Pts',(1.58036303299994,12.2,3.93046339999999));
#335775=CARTESIAN_POINT('Ctrl Pts',(1.58036303299994,5.2,3.93046339999999));
#335776=CARTESIAN_POINT('Ctrl Pts',(1.58036303299994,2.2,3.93046339999999));
#335777=CARTESIAN_POINT('Ctrl Pts',(1.57928790399994,12.2,3.92924196799999));
#335778=CARTESIAN_POINT('Ctrl Pts',(1.57928790399994,5.2,3.92924196799999));
#335779=CARTESIAN_POINT('Ctrl Pts',(1.57928790399994,2.2,3.92924196799999));
#335780=CARTESIAN_POINT('Ctrl Pts',(1.57821718299994,12.2,3.92802271199999));
#335781=CARTESIAN_POINT('Ctrl Pts',(1.57821718299994,5.2,3.92802271199999));
#335782=CARTESIAN_POINT('Ctrl Pts',(1.57821718299994,2.2,3.92802271199999));
#335783=CARTESIAN_POINT('Ctrl Pts',(1.57715086999994,12.2,3.92680564399999));
#335784=CARTESIAN_POINT('Ctrl Pts',(1.57715086999994,5.2,3.92680564399999));
#335785=CARTESIAN_POINT('Ctrl Pts',(1.57715086999994,2.2,3.92680564399999));
#335786=CARTESIAN_POINT('Ctrl Pts',(1.57608896299994,12.2,3.92559077799999));
#335787=CARTESIAN_POINT('Ctrl Pts',(1.57608896299994,5.2,3.92559077799999));
#335788=CARTESIAN_POINT('Ctrl Pts',(1.57608896299994,2.2,3.92559077799999));
#335789=CARTESIAN_POINT('Ctrl Pts',(1.57503145999994,12.2,3.92437812499999));
#335790=CARTESIAN_POINT('Ctrl Pts',(1.57503145999994,5.2,3.92437812499999));
#335791=CARTESIAN_POINT('Ctrl Pts',(1.57503145999994,2.2,3.92437812499999));
#335792=CARTESIAN_POINT('Ctrl Pts',(1.57397835999994,12.2,3.92316769799999));
#335793=CARTESIAN_POINT('Ctrl Pts',(1.57397835999994,5.2,3.92316769799999));
#335794=CARTESIAN_POINT('Ctrl Pts',(1.57397835999994,2.2,3.92316769799999));
#335795=CARTESIAN_POINT('Ctrl Pts',(1.57292965799994,12.2,3.92195950899998));
#335796=CARTESIAN_POINT('Ctrl Pts',(1.57292965799994,5.2,3.92195950899998));
#335797=CARTESIAN_POINT('Ctrl Pts',(1.57292965799994,2.2,3.92195950899998));
#335798=CARTESIAN_POINT('Ctrl Pts',(1.57188535699994,12.2,3.92075357199998));
#335799=CARTESIAN_POINT('Ctrl Pts',(1.57188535699994,5.2,3.92075357199998));
#335800=CARTESIAN_POINT('Ctrl Pts',(1.57188535699994,2.2,3.92075357199998));
#335801=CARTESIAN_POINT('Ctrl Pts',(1.57084544999994,12.2,3.91954989899999));
#335802=CARTESIAN_POINT('Ctrl Pts',(1.57084544999994,5.2,3.91954989899999));
#335803=CARTESIAN_POINT('Ctrl Pts',(1.57084544999994,2.2,3.91954989899999));
#335804=CARTESIAN_POINT('Ctrl Pts',(1.56980993999994,12.2,3.91834850299999));
#335805=CARTESIAN_POINT('Ctrl Pts',(1.56980993999994,5.2,3.91834850299999));
#335806=CARTESIAN_POINT('Ctrl Pts',(1.56980993999994,2.2,3.91834850299999));
#335807=CARTESIAN_POINT('Ctrl Pts',(1.56877882099994,12.2,3.91714939699998));
#335808=CARTESIAN_POINT('Ctrl Pts',(1.56877882099994,5.2,3.91714939699998));
#335809=CARTESIAN_POINT('Ctrl Pts',(1.56877882099994,2.2,3.91714939699998));
#335810=CARTESIAN_POINT('Ctrl Pts',(1.56775209299994,12.2,3.91595259199998));
#335811=CARTESIAN_POINT('Ctrl Pts',(1.56775209299994,5.2,3.91595259199998));
#335812=CARTESIAN_POINT('Ctrl Pts',(1.56775209299994,2.2,3.91595259199998));
#335813=CARTESIAN_POINT('Ctrl Pts',(1.56672975399994,12.2,3.91475810299998));
#335814=CARTESIAN_POINT('Ctrl Pts',(1.56672975399994,5.2,3.91475810299998));
#335815=CARTESIAN_POINT('Ctrl Pts',(1.56672975399994,2.2,3.91475810299998));
#335816=CARTESIAN_POINT('Ctrl Pts',(1.56571180199994,12.2,3.91356594199999));
#335817=CARTESIAN_POINT('Ctrl Pts',(1.56571180199994,5.2,3.91356594199999));
#335818=CARTESIAN_POINT('Ctrl Pts',(1.56571180199994,2.2,3.91356594199999));
#335819=CARTESIAN_POINT('Ctrl Pts',(1.56469823499994,12.2,3.91237612099999));
#335820=CARTESIAN_POINT('Ctrl Pts',(1.56469823499994,5.2,3.91237612099999));
#335821=CARTESIAN_POINT('Ctrl Pts',(1.56469823499994,2.2,3.91237612099999));
#335822=CARTESIAN_POINT('Ctrl Pts',(1.56368904999994,12.2,3.91118865499998));
#335823=CARTESIAN_POINT('Ctrl Pts',(1.56368904999994,5.2,3.91118865499998));
#335824=CARTESIAN_POINT('Ctrl Pts',(1.56368904999994,2.2,3.91118865499998));
#335825=CARTESIAN_POINT('Ctrl Pts',(1.56268424599994,12.2,3.91000355399999));
#335826=CARTESIAN_POINT('Ctrl Pts',(1.56268424599994,5.2,3.91000355399999));
#335827=CARTESIAN_POINT('Ctrl Pts',(1.56268424599994,2.2,3.91000355399999));
#335828=CARTESIAN_POINT('Ctrl Pts',(1.56168382199994,12.2,3.90882083299999));
#335829=CARTESIAN_POINT('Ctrl Pts',(1.56168382199994,5.2,3.90882083299999));
#335830=CARTESIAN_POINT('Ctrl Pts',(1.56168382199994,2.2,3.90882083299999));
#335831=CARTESIAN_POINT('Ctrl Pts',(1.56068777299994,12.2,3.90764050399999));
#335832=CARTESIAN_POINT('Ctrl Pts',(1.56068777299994,5.2,3.90764050399999));
#335833=CARTESIAN_POINT('Ctrl Pts',(1.56068777299994,2.2,3.90764050399999));
#335834=CARTESIAN_POINT('Ctrl Pts',(1.55969609799994,12.2,3.90646258099999));
#335835=CARTESIAN_POINT('Ctrl Pts',(1.55969609799994,5.2,3.90646258099999));
#335836=CARTESIAN_POINT('Ctrl Pts',(1.55969609799994,2.2,3.90646258099999));
#335837=CARTESIAN_POINT('Ctrl Pts',(1.55870879599994,12.2,3.90528707499998));
#335838=CARTESIAN_POINT('Ctrl Pts',(1.55870879599994,5.2,3.90528707499998));
#335839=CARTESIAN_POINT('Ctrl Pts',(1.55870879599994,2.2,3.90528707499998));
#335840=CARTESIAN_POINT('Ctrl Pts',(1.55772586499994,12.2,3.90411400099998));
#335841=CARTESIAN_POINT('Ctrl Pts',(1.55772586499994,5.2,3.90411400099998));
#335842=CARTESIAN_POINT('Ctrl Pts',(1.55772586499994,2.2,3.90411400099998));
#335843=CARTESIAN_POINT('Ctrl Pts',(1.55674730099994,12.2,3.90294336899998));
#335844=CARTESIAN_POINT('Ctrl Pts',(1.55674730099994,5.2,3.90294336899998));
#335845=CARTESIAN_POINT('Ctrl Pts',(1.55674730099994,2.2,3.90294336899998));
#335846=CARTESIAN_POINT('Ctrl Pts',(1.55577310299994,12.2,3.90177519699999));
#335847=CARTESIAN_POINT('Ctrl Pts',(1.55577310299994,5.2,3.90177519699999));
#335848=CARTESIAN_POINT('Ctrl Pts',(1.55577310299994,2.2,3.90177519699999));
#335849=CARTESIAN_POINT('Ctrl Pts',(1.55480326799994,12.2,3.90060949299999));
#335850=CARTESIAN_POINT('Ctrl Pts',(1.55480326799994,5.2,3.90060949299999));
#335851=CARTESIAN_POINT('Ctrl Pts',(1.55480326799994,2.2,3.90060949299999));
#335852=CARTESIAN_POINT('Ctrl Pts',(1.55383779599994,12.2,3.89944627299998));
#335853=CARTESIAN_POINT('Ctrl Pts',(1.55383779599994,5.2,3.89944627299998));
#335854=CARTESIAN_POINT('Ctrl Pts',(1.55383779599994,2.2,3.89944627299998));
#335855=CARTESIAN_POINT('Ctrl Pts',(1.55287668099994,12.2,3.89828554999998));
#335856=CARTESIAN_POINT('Ctrl Pts',(1.55287668099994,5.2,3.89828554999998));
#335857=CARTESIAN_POINT('Ctrl Pts',(1.55287668099994,2.2,3.89828554999998));
#335858=CARTESIAN_POINT('Ctrl Pts',(1.55191992399994,12.2,3.89712733499999));
#335859=CARTESIAN_POINT('Ctrl Pts',(1.55191992399994,5.2,3.89712733499999));
#335860=CARTESIAN_POINT('Ctrl Pts',(1.55191992399994,2.2,3.89712733499999));
#335861=CARTESIAN_POINT('Ctrl Pts',(1.55096752099994,12.2,3.89597164399999));
#335862=CARTESIAN_POINT('Ctrl Pts',(1.55096752099994,5.2,3.89597164399999));
#335863=CARTESIAN_POINT('Ctrl Pts',(1.55096752099994,2.2,3.89597164399999));
#335864=CARTESIAN_POINT('Ctrl Pts',(1.55001946899994,12.2,3.89481848799999));
#335865=CARTESIAN_POINT('Ctrl Pts',(1.55001946899994,5.2,3.89481848799999));
#335866=CARTESIAN_POINT('Ctrl Pts',(1.55001946899994,2.2,3.89481848799999));
#335867=CARTESIAN_POINT('Ctrl Pts',(1.54907576899994,12.2,3.89366788099998));
#335868=CARTESIAN_POINT('Ctrl Pts',(1.54907576899994,5.2,3.89366788099998));
#335869=CARTESIAN_POINT('Ctrl Pts',(1.54907576899994,2.2,3.89366788099998));
#335870=CARTESIAN_POINT('Ctrl Pts',(1.54813641499994,12.2,3.89251983599999));
#335871=CARTESIAN_POINT('Ctrl Pts',(1.54813641499994,5.2,3.89251983599999));
#335872=CARTESIAN_POINT('Ctrl Pts',(1.54813641499994,2.2,3.89251983599999));
#335873=CARTESIAN_POINT('Ctrl Pts',(1.54720140599994,12.2,3.89137436699999));
#335874=CARTESIAN_POINT('Ctrl Pts',(1.54720140599994,5.2,3.89137436699999));
#335875=CARTESIAN_POINT('Ctrl Pts',(1.54720140599994,2.2,3.89137436699999));
#335876=CARTESIAN_POINT('Ctrl Pts',(1.54627073899994,12.2,3.89023148599998));
#335877=CARTESIAN_POINT('Ctrl Pts',(1.54627073899994,5.2,3.89023148599998));
#335878=CARTESIAN_POINT('Ctrl Pts',(1.54627073899994,2.2,3.89023148599998));
#335879=CARTESIAN_POINT('Ctrl Pts',(1.54534441299994,12.2,3.88909120699999));
#335880=CARTESIAN_POINT('Ctrl Pts',(1.54534441299994,5.2,3.88909120699999));
#335881=CARTESIAN_POINT('Ctrl Pts',(1.54534441299994,2.2,3.88909120699999));
#335882=CARTESIAN_POINT('Ctrl Pts',(1.54442242499994,12.2,3.88795354299998));
#335883=CARTESIAN_POINT('Ctrl Pts',(1.54442242499994,5.2,3.88795354299998));
#335884=CARTESIAN_POINT('Ctrl Pts',(1.54442242499994,2.2,3.88795354299998));
#335885=CARTESIAN_POINT('Ctrl Pts',(1.54350476999994,12.2,3.88681850799999));
#335886=CARTESIAN_POINT('Ctrl Pts',(1.54350476999994,5.2,3.88681850799999));
#335887=CARTESIAN_POINT('Ctrl Pts',(1.54350476999994,2.2,3.88681850799999));
#335888=CARTESIAN_POINT('Ctrl Pts',(1.54259144899994,12.2,3.88568611499998));
#335889=CARTESIAN_POINT('Ctrl Pts',(1.54259144899994,5.2,3.88568611499998));
#335890=CARTESIAN_POINT('Ctrl Pts',(1.54259144899994,2.2,3.88568611499998));
#335891=CARTESIAN_POINT('Ctrl Pts',(1.54168245899994,12.2,3.88455637699998));
#335892=CARTESIAN_POINT('Ctrl Pts',(1.54168245899994,5.2,3.88455637699998));
#335893=CARTESIAN_POINT('Ctrl Pts',(1.54168245899994,2.2,3.88455637699998));
#335894=CARTESIAN_POINT('Ctrl Pts',(1.54077779499994,12.2,3.88342930899999));
#335895=CARTESIAN_POINT('Ctrl Pts',(1.54077779499994,5.2,3.88342930899999));
#335896=CARTESIAN_POINT('Ctrl Pts',(1.54077779499994,2.2,3.88342930899999));
#335897=CARTESIAN_POINT('Ctrl Pts',(1.53987745599994,12.2,3.88230492199998));
#335898=CARTESIAN_POINT('Ctrl Pts',(1.53987745599994,5.2,3.88230492199998));
#335899=CARTESIAN_POINT('Ctrl Pts',(1.53987745599994,2.2,3.88230492199998));
#335900=CARTESIAN_POINT('Ctrl Pts',(1.53898143999994,12.2,3.88118322999999));
#335901=CARTESIAN_POINT('Ctrl Pts',(1.53898143999994,5.2,3.88118322999999));
#335902=CARTESIAN_POINT('Ctrl Pts',(1.53898143999994,2.2,3.88118322999999));
#335903=CARTESIAN_POINT('Ctrl Pts',(1.53808974299994,12.2,3.88006424799999));
#335904=CARTESIAN_POINT('Ctrl Pts',(1.53808974299994,5.2,3.88006424799999));
#335905=CARTESIAN_POINT('Ctrl Pts',(1.53808974299994,2.2,3.88006424799999));
#335906=CARTESIAN_POINT('Ctrl Pts',(1.53720236299994,12.2,3.87894798699998));
#335907=CARTESIAN_POINT('Ctrl Pts',(1.53720236299994,5.2,3.87894798699998));
#335908=CARTESIAN_POINT('Ctrl Pts',(1.53720236299994,2.2,3.87894798699998));
#335909=CARTESIAN_POINT('Ctrl Pts',(1.53631929799994,12.2,3.87783446399999));
#335910=CARTESIAN_POINT('Ctrl Pts',(1.53631929799994,5.2,3.87783446399999));
#335911=CARTESIAN_POINT('Ctrl Pts',(1.53631929799994,2.2,3.87783446399999));
#335912=CARTESIAN_POINT('Ctrl Pts',(1.53544054399994,12.2,3.87672368899998));
#335913=CARTESIAN_POINT('Ctrl Pts',(1.53544054399994,5.2,3.87672368899998));
#335914=CARTESIAN_POINT('Ctrl Pts',(1.53544054399994,2.2,3.87672368899998));
#335915=CARTESIAN_POINT('Ctrl Pts',(1.53456609999994,12.2,3.87561567799998));
#335916=CARTESIAN_POINT('Ctrl Pts',(1.53456609999994,5.2,3.87561567799998));
#335917=CARTESIAN_POINT('Ctrl Pts',(1.53456609999994,2.2,3.87561567799998));
#335918=CARTESIAN_POINT('Ctrl Pts',(1.53369595999994,12.2,3.87451044399998));
#335919=CARTESIAN_POINT('Ctrl Pts',(1.53369595999994,5.2,3.87451044399998));
#335920=CARTESIAN_POINT('Ctrl Pts',(1.53369595999994,2.2,3.87451044399998));
#335921=CARTESIAN_POINT('Ctrl Pts',(1.53283012499994,12.2,3.87340800099999));
#335922=CARTESIAN_POINT('Ctrl Pts',(1.53283012499994,5.2,3.87340800099999));
#335923=CARTESIAN_POINT('Ctrl Pts',(1.53283012499994,2.2,3.87340800099999));
#335924=CARTESIAN_POINT('Ctrl Pts',(1.53196858999994,12.2,3.87230836099998));
#335925=CARTESIAN_POINT('Ctrl Pts',(1.53196858999994,5.2,3.87230836099998));
#335926=CARTESIAN_POINT('Ctrl Pts',(1.53196858999994,2.2,3.87230836099998));
#335927=CARTESIAN_POINT('Ctrl Pts',(1.53111135299994,12.2,3.87121153899999));
#335928=CARTESIAN_POINT('Ctrl Pts',(1.53111135299994,5.2,3.87121153899999));
#335929=CARTESIAN_POINT('Ctrl Pts',(1.53111135299994,2.2,3.87121153899999));
#335930=CARTESIAN_POINT('Ctrl Pts',(1.53025841199994,12.2,3.87011754799998));
#335931=CARTESIAN_POINT('Ctrl Pts',(1.53025841199994,5.2,3.87011754799998));
#335932=CARTESIAN_POINT('Ctrl Pts',(1.53025841199994,2.2,3.87011754799998));
#335933=CARTESIAN_POINT('Ctrl Pts',(1.52940976199994,12.2,3.86902640299999));
#335934=CARTESIAN_POINT('Ctrl Pts',(1.52940976199994,5.2,3.86902640299999));
#335935=CARTESIAN_POINT('Ctrl Pts',(1.52940976199994,2.2,3.86902640299999));
#335936=CARTESIAN_POINT('Ctrl Pts',(1.52856539999994,12.2,3.86793811599999));
#335937=CARTESIAN_POINT('Ctrl Pts',(1.52856539999994,5.2,3.86793811599999));
#335938=CARTESIAN_POINT('Ctrl Pts',(1.52856539999994,2.2,3.86793811599999));
#335939=CARTESIAN_POINT('Ctrl Pts',(1.52772532599994,12.2,3.86685270299999));
#335940=CARTESIAN_POINT('Ctrl Pts',(1.52772532599994,5.2,3.86685270299999));
#335941=CARTESIAN_POINT('Ctrl Pts',(1.52772532599994,2.2,3.86685270299999));
#335942=CARTESIAN_POINT('Ctrl Pts',(1.52688953499994,12.2,3.86577017499998));
#335943=CARTESIAN_POINT('Ctrl Pts',(1.52688953499994,5.2,3.86577017499998));
#335944=CARTESIAN_POINT('Ctrl Pts',(1.52688953499994,2.2,3.86577017499998));
#335945=CARTESIAN_POINT('Ctrl Pts',(1.52605802399994,12.2,3.86469054799999));
#335946=CARTESIAN_POINT('Ctrl Pts',(1.52605802399994,5.2,3.86469054799999));
#335947=CARTESIAN_POINT('Ctrl Pts',(1.52605802399994,2.2,3.86469054799999));
#335948=CARTESIAN_POINT('Ctrl Pts',(1.52523078999994,12.2,3.86361383599999));
#335949=CARTESIAN_POINT('Ctrl Pts',(1.52523078999994,5.2,3.86361383599999));
#335950=CARTESIAN_POINT('Ctrl Pts',(1.52523078999994,2.2,3.86361383599999));
#335951=CARTESIAN_POINT('Ctrl Pts',(1.52440782999994,12.2,3.86254005099998));
#335952=CARTESIAN_POINT('Ctrl Pts',(1.52440782999994,5.2,3.86254005099998));
#335953=CARTESIAN_POINT('Ctrl Pts',(1.52440782999994,2.2,3.86254005099998));
#335954=CARTESIAN_POINT('Ctrl Pts',(1.52358914199994,12.2,3.86146920799998));
#335955=CARTESIAN_POINT('Ctrl Pts',(1.52358914199994,5.2,3.86146920799998));
#335956=CARTESIAN_POINT('Ctrl Pts',(1.52358914199994,2.2,3.86146920799998));
#335957=CARTESIAN_POINT('Ctrl Pts',(1.52277472299994,12.2,3.86040132099998));
#335958=CARTESIAN_POINT('Ctrl Pts',(1.52277472299994,5.2,3.86040132099998));
#335959=CARTESIAN_POINT('Ctrl Pts',(1.52277472299994,2.2,3.86040132099998));
#335960=CARTESIAN_POINT('Ctrl Pts',(1.52196456699994,12.2,3.85933640399998));
#335961=CARTESIAN_POINT('Ctrl Pts',(1.52196456699994,5.2,3.85933640399998));
#335962=CARTESIAN_POINT('Ctrl Pts',(1.52196456699994,2.2,3.85933640399998));
#335963=CARTESIAN_POINT('Ctrl Pts',(1.52115867499994,12.2,3.85827446999999));
#335964=CARTESIAN_POINT('Ctrl Pts',(1.52115867499994,5.2,3.85827446999999));
#335965=CARTESIAN_POINT('Ctrl Pts',(1.52115867499994,2.2,3.85827446999999));
#335966=CARTESIAN_POINT('Ctrl Pts',(1.52035704199994,12.2,3.85721553499998));
#335967=CARTESIAN_POINT('Ctrl Pts',(1.52035704199994,5.2,3.85721553499998));
#335968=CARTESIAN_POINT('Ctrl Pts',(1.52035704199994,2.2,3.85721553499998));
#335969=CARTESIAN_POINT('Ctrl Pts',(1.51955966299994,12.2,3.85615961099998));
#335970=CARTESIAN_POINT('Ctrl Pts',(1.51955966299994,5.2,3.85615961099998));
#335971=CARTESIAN_POINT('Ctrl Pts',(1.51955966299994,2.2,3.85615961099998));
#335972=CARTESIAN_POINT('Ctrl Pts',(1.51876653699994,12.2,3.85510671399998));
#335973=CARTESIAN_POINT('Ctrl Pts',(1.51876653699994,5.2,3.85510671399998));
#335974=CARTESIAN_POINT('Ctrl Pts',(1.51876653699994,2.2,3.85510671399998));
#335975=CARTESIAN_POINT('Ctrl Pts',(1.51797765999994,12.2,3.85405685599999));
#335976=CARTESIAN_POINT('Ctrl Pts',(1.51797765999994,5.2,3.85405685599999));
#335977=CARTESIAN_POINT('Ctrl Pts',(1.51797765999994,2.2,3.85405685599999));
#335978=CARTESIAN_POINT('Ctrl Pts',(1.51719302999994,12.2,3.85301005199998));
#335979=CARTESIAN_POINT('Ctrl Pts',(1.51719302999994,5.2,3.85301005199998));
#335980=CARTESIAN_POINT('Ctrl Pts',(1.51719302999994,2.2,3.85301005199998));
#335981=CARTESIAN_POINT('Ctrl Pts',(1.51641264299994,12.2,3.85196631599998));
#335982=CARTESIAN_POINT('Ctrl Pts',(1.51641264299994,5.2,3.85196631599998));
#335983=CARTESIAN_POINT('Ctrl Pts',(1.51641264299994,2.2,3.85196631599998));
#335984=CARTESIAN_POINT('Ctrl Pts',(1.51563649399994,12.2,3.85092566399998));
#335985=CARTESIAN_POINT('Ctrl Pts',(1.51563649399994,5.2,3.85092566399998));
#335986=CARTESIAN_POINT('Ctrl Pts',(1.51563649399994,2.2,3.85092566399998));
#335987=CARTESIAN_POINT('Ctrl Pts',(1.51486458299994,12.2,3.84988810699999));
#335988=CARTESIAN_POINT('Ctrl Pts',(1.51486458299994,5.2,3.84988810699999));
#335989=CARTESIAN_POINT('Ctrl Pts',(1.51486458299994,2.2,3.84988810699999));
#335990=CARTESIAN_POINT('Ctrl Pts',(1.51409690299994,12.2,3.84885366199998));
#335991=CARTESIAN_POINT('Ctrl Pts',(1.51409690299994,5.2,3.84885366199998));
#335992=CARTESIAN_POINT('Ctrl Pts',(1.51409690299994,2.2,3.84885366199998));
#335993=CARTESIAN_POINT('Ctrl Pts',(1.51333345399994,12.2,3.84782234099998));
#335994=CARTESIAN_POINT('Ctrl Pts',(1.51333345399994,5.2,3.84782234099998));
#335995=CARTESIAN_POINT('Ctrl Pts',(1.51333345399994,2.2,3.84782234099998));
#335996=CARTESIAN_POINT('Ctrl Pts',(1.51257422899994,12.2,3.84679415999998));
#335997=CARTESIAN_POINT('Ctrl Pts',(1.51257422899994,5.2,3.84679415999998));
#335998=CARTESIAN_POINT('Ctrl Pts',(1.51257422899994,2.2,3.84679415999998));
#335999=CARTESIAN_POINT('Ctrl Pts',(1.51181922799994,12.2,3.84576913299998));
#336000=CARTESIAN_POINT('Ctrl Pts',(1.51181922799994,5.2,3.84576913299998));
#336001=CARTESIAN_POINT('Ctrl Pts',(1.51181922799994,2.2,3.84576913299998));
#336002=CARTESIAN_POINT('Ctrl Pts',(1.51106844599994,12.2,3.84474727399999));
#336003=CARTESIAN_POINT('Ctrl Pts',(1.51106844599994,5.2,3.84474727399999));
#336004=CARTESIAN_POINT('Ctrl Pts',(1.51106844599994,2.2,3.84474727399999));
#336005=CARTESIAN_POINT('Ctrl Pts',(1.51032187999994,12.2,3.84372859599999));
#336006=CARTESIAN_POINT('Ctrl Pts',(1.51032187999994,5.2,3.84372859599999));
#336007=CARTESIAN_POINT('Ctrl Pts',(1.51032187999994,2.2,3.84372859599999));
#336008=CARTESIAN_POINT('Ctrl Pts',(1.50957952599994,12.2,3.84271311599999));
#336009=CARTESIAN_POINT('Ctrl Pts',(1.50957952599994,5.2,3.84271311599999));
#336010=CARTESIAN_POINT('Ctrl Pts',(1.50957952599994,2.2,3.84271311599999));
#336011=CARTESIAN_POINT('Ctrl Pts',(1.50884137999994,12.2,3.84170084599998));
#336012=CARTESIAN_POINT('Ctrl Pts',(1.50884137999994,5.2,3.84170084599998));
#336013=CARTESIAN_POINT('Ctrl Pts',(1.50884137999994,2.2,3.84170084599998));
#336014=CARTESIAN_POINT('Ctrl Pts',(1.50810743899994,12.2,3.84069180299999));
#336015=CARTESIAN_POINT('Ctrl Pts',(1.50810743899994,5.2,3.84069180299999));
#336016=CARTESIAN_POINT('Ctrl Pts',(1.50810743899994,2.2,3.84069180299999));
#336017=CARTESIAN_POINT('Ctrl Pts',(1.50737770099994,12.2,3.83968599899998));
#336018=CARTESIAN_POINT('Ctrl Pts',(1.50737770099994,5.2,3.83968599899998));
#336019=CARTESIAN_POINT('Ctrl Pts',(1.50737770099994,2.2,3.83968599899998));
#336020=CARTESIAN_POINT('Ctrl Pts',(1.50665215899994,12.2,3.83868344999998));
#336021=CARTESIAN_POINT('Ctrl Pts',(1.50665215899994,5.2,3.83868344999998));
#336022=CARTESIAN_POINT('Ctrl Pts',(1.50665215899994,2.2,3.83868344999998));
#336023=CARTESIAN_POINT('Ctrl Pts',(1.50593081299994,12.2,3.83768416999998));
#336024=CARTESIAN_POINT('Ctrl Pts',(1.50593081299994,5.2,3.83768416999998));
#336025=CARTESIAN_POINT('Ctrl Pts',(1.50593081299994,2.2,3.83768416999998));
#336026=CARTESIAN_POINT('Ctrl Pts',(1.50521365599994,12.2,3.83668817499998));
#336027=CARTESIAN_POINT('Ctrl Pts',(1.50521365599994,5.2,3.83668817499998));
#336028=CARTESIAN_POINT('Ctrl Pts',(1.50521365599994,2.2,3.83668817499998));
#336029=CARTESIAN_POINT('Ctrl Pts',(1.50450068699994,12.2,3.83569547699998));
#336030=CARTESIAN_POINT('Ctrl Pts',(1.50450068699994,5.2,3.83569547699998));
#336031=CARTESIAN_POINT('Ctrl Pts',(1.50450068699994,2.2,3.83569547699998));
#336032=CARTESIAN_POINT('Ctrl Pts',(1.50379189999994,12.2,3.83470609099999));
#336033=CARTESIAN_POINT('Ctrl Pts',(1.50379189999994,5.2,3.83470609099999));
#336034=CARTESIAN_POINT('Ctrl Pts',(1.50379189999994,2.2,3.83470609099999));
#336035=CARTESIAN_POINT('Ctrl Pts',(1.50308729399994,12.2,3.83372003399998));
#336036=CARTESIAN_POINT('Ctrl Pts',(1.50308729399994,5.2,3.83372003399998));
#336037=CARTESIAN_POINT('Ctrl Pts',(1.50308729399994,2.2,3.83372003399998));
#336038=CARTESIAN_POINT('Ctrl Pts',(1.50238686199994,12.2,3.83273731799999));
#336039=CARTESIAN_POINT('Ctrl Pts',(1.50238686199994,5.2,3.83273731799999));
#336040=CARTESIAN_POINT('Ctrl Pts',(1.50238686199994,2.2,3.83273731799999));
#336041=CARTESIAN_POINT('Ctrl Pts',(1.50169060299994,12.2,3.83175795899999));
#336042=CARTESIAN_POINT('Ctrl Pts',(1.50169060299994,5.2,3.83175795899999));
#336043=CARTESIAN_POINT('Ctrl Pts',(1.50169060299994,2.2,3.83175795899999));
#336044=CARTESIAN_POINT('Ctrl Pts',(1.50099851099994,12.2,3.83078197199998));
#336045=CARTESIAN_POINT('Ctrl Pts',(1.50099851099994,5.2,3.83078197199998));
#336046=CARTESIAN_POINT('Ctrl Pts',(1.50099851099994,2.2,3.83078197199998));
#336047=CARTESIAN_POINT('Ctrl Pts',(1.50031058399994,12.2,3.82980937199999));
#336048=CARTESIAN_POINT('Ctrl Pts',(1.50031058399994,5.2,3.82980937199999));
#336049=CARTESIAN_POINT('Ctrl Pts',(1.50031058399994,2.2,3.82980937199999));
#336050=CARTESIAN_POINT('Ctrl Pts',(1.49962681699994,12.2,3.82884017099999));
#336051=CARTESIAN_POINT('Ctrl Pts',(1.49962681699994,5.2,3.82884017099999));
#336052=CARTESIAN_POINT('Ctrl Pts',(1.49962681699994,2.2,3.82884017099999));
#336053=CARTESIAN_POINT('Ctrl Pts',(1.49894720599994,12.2,3.82787438799999));
#336054=CARTESIAN_POINT('Ctrl Pts',(1.49894720599994,5.2,3.82787438799999));
#336055=CARTESIAN_POINT('Ctrl Pts',(1.49894720599994,2.2,3.82787438799999));
#336056=CARTESIAN_POINT('Ctrl Pts',(1.49827174799994,12.2,3.82691203499999));
#336057=CARTESIAN_POINT('Ctrl Pts',(1.49827174799994,5.2,3.82691203499999));
#336058=CARTESIAN_POINT('Ctrl Pts',(1.49827174799994,2.2,3.82691203499999));
#336059=CARTESIAN_POINT('Ctrl Pts',(1.49760043799994,12.2,3.82595312699999));
#336060=CARTESIAN_POINT('Ctrl Pts',(1.49760043799994,5.2,3.82595312699999));
#336061=CARTESIAN_POINT('Ctrl Pts',(1.49760043799994,2.2,3.82595312699999));
#336062=CARTESIAN_POINT('Ctrl Pts',(1.49693327199994,12.2,3.82499767999998));
#336063=CARTESIAN_POINT('Ctrl Pts',(1.49693327199994,5.2,3.82499767999998));
#336064=CARTESIAN_POINT('Ctrl Pts',(1.49693327199994,2.2,3.82499767999998));
#336065=CARTESIAN_POINT('Ctrl Pts',(1.49627024699994,12.2,3.82404570799999));
#336066=CARTESIAN_POINT('Ctrl Pts',(1.49627024699994,5.2,3.82404570799999));
#336067=CARTESIAN_POINT('Ctrl Pts',(1.49627024699994,2.2,3.82404570799999));
#336068=CARTESIAN_POINT('Ctrl Pts',(1.49561135799994,12.2,3.82309722799998));
#336069=CARTESIAN_POINT('Ctrl Pts',(1.49561135799994,5.2,3.82309722799998));
#336070=CARTESIAN_POINT('Ctrl Pts',(1.49561135799994,2.2,3.82309722799998));
#336071=CARTESIAN_POINT('Ctrl Pts',(1.49495660099994,12.2,3.82215225199998));
#336072=CARTESIAN_POINT('Ctrl Pts',(1.49495660099994,5.2,3.82215225199998));
#336073=CARTESIAN_POINT('Ctrl Pts',(1.49495660099994,2.2,3.82215225199998));
#336074=CARTESIAN_POINT('Ctrl Pts',(1.49430597199994,12.2,3.82121079699999));
#336075=CARTESIAN_POINT('Ctrl Pts',(1.49430597199994,5.2,3.82121079699999));
#336076=CARTESIAN_POINT('Ctrl Pts',(1.49430597199994,2.2,3.82121079699999));
#336077=CARTESIAN_POINT('Ctrl Pts',(1.49365946699994,12.2,3.82027287699999));
#336078=CARTESIAN_POINT('Ctrl Pts',(1.49365946699994,5.2,3.82027287699999));
#336079=CARTESIAN_POINT('Ctrl Pts',(1.49365946699994,2.2,3.82027287699999));
#336080=CARTESIAN_POINT('Ctrl Pts',(1.49301708199994,12.2,3.81933850799999));
#336081=CARTESIAN_POINT('Ctrl Pts',(1.49301708199994,5.2,3.81933850799999));
#336082=CARTESIAN_POINT('Ctrl Pts',(1.49301708199994,2.2,3.81933850799999));
#336083=CARTESIAN_POINT('Ctrl Pts',(1.49237881299994,12.2,3.81840770299998));
#336084=CARTESIAN_POINT('Ctrl Pts',(1.49237881299994,5.2,3.81840770299998));
#336085=CARTESIAN_POINT('Ctrl Pts',(1.49237881299994,2.2,3.81840770299998));
#336086=CARTESIAN_POINT('Ctrl Pts',(1.49174465499994,12.2,3.81748048099999));
#336087=CARTESIAN_POINT('Ctrl Pts',(1.49174465499994,5.2,3.81748048099999));
#336088=CARTESIAN_POINT('Ctrl Pts',(1.49174465499994,2.2,3.81748048099999));
#336089=CARTESIAN_POINT('Ctrl Pts',(1.49111460299994,12.2,3.81655685399998));
#336090=CARTESIAN_POINT('Ctrl Pts',(1.49111460299994,5.2,3.81655685399998));
#336091=CARTESIAN_POINT('Ctrl Pts',(1.49111460299994,2.2,3.81655685399998));
#336092=CARTESIAN_POINT('Ctrl Pts',(1.49048865599994,12.2,3.81563683899999));
#336093=CARTESIAN_POINT('Ctrl Pts',(1.49048865599994,5.2,3.81563683899999));
#336094=CARTESIAN_POINT('Ctrl Pts',(1.49048865599994,2.2,3.81563683899999));
#336095=CARTESIAN_POINT('Ctrl Pts',(1.48986680499994,12.2,3.81472044999998));
#336096=CARTESIAN_POINT('Ctrl Pts',(1.48986680499994,5.2,3.81472044999998));
#336097=CARTESIAN_POINT('Ctrl Pts',(1.48986680499994,2.2,3.81472044999998));
#336098=CARTESIAN_POINT('Ctrl Pts',(1.48924904999994,12.2,3.81380770199998));
#336099=CARTESIAN_POINT('Ctrl Pts',(1.48924904999994,5.2,3.81380770199998));
#336100=CARTESIAN_POINT('Ctrl Pts',(1.48924904999994,2.2,3.81380770199998));
#336101=CARTESIAN_POINT('Ctrl Pts',(1.48863538399994,12.2,3.81289861099999));
#336102=CARTESIAN_POINT('Ctrl Pts',(1.48863538399994,5.2,3.81289861099999));
#336103=CARTESIAN_POINT('Ctrl Pts',(1.48863538399994,2.2,3.81289861099999));
#336104=CARTESIAN_POINT('Ctrl Pts',(1.48802580299994,12.2,3.81199319299999));
#336105=CARTESIAN_POINT('Ctrl Pts',(1.48802580299994,5.2,3.81199319299999));
#336106=CARTESIAN_POINT('Ctrl Pts',(1.48802580299994,2.2,3.81199319299999));
#336107=CARTESIAN_POINT('Ctrl Pts',(1.48742030299994,12.2,3.81109146299998));
#336108=CARTESIAN_POINT('Ctrl Pts',(1.48742030299994,5.2,3.81109146299998));
#336109=CARTESIAN_POINT('Ctrl Pts',(1.48742030299994,2.2,3.81109146299998));
#336110=CARTESIAN_POINT('Ctrl Pts',(1.48681887899994,12.2,3.81019343499998));
#336111=CARTESIAN_POINT('Ctrl Pts',(1.48681887899994,5.2,3.81019343499998));
#336112=CARTESIAN_POINT('Ctrl Pts',(1.48681887899994,2.2,3.81019343499998));
#336113=CARTESIAN_POINT('Ctrl Pts',(1.48622152799994,12.2,3.80929912599999));
#336114=CARTESIAN_POINT('Ctrl Pts',(1.48622152799994,5.2,3.80929912599999));
#336115=CARTESIAN_POINT('Ctrl Pts',(1.48622152799994,2.2,3.80929912599999));
#336116=CARTESIAN_POINT('Ctrl Pts',(1.48562824299994,12.2,3.80840855199998));
#336117=CARTESIAN_POINT('Ctrl Pts',(1.48562824299994,5.2,3.80840855199998));
#336118=CARTESIAN_POINT('Ctrl Pts',(1.48562824299994,2.2,3.80840855199998));
#336119=CARTESIAN_POINT('Ctrl Pts',(1.48503902099994,12.2,3.80752172599998));
#336120=CARTESIAN_POINT('Ctrl Pts',(1.48503902099994,5.2,3.80752172599998));
#336121=CARTESIAN_POINT('Ctrl Pts',(1.48503902099994,2.2,3.80752172599998));
#336122=CARTESIAN_POINT('Ctrl Pts',(1.48445385799994,12.2,3.80663866499999));
#336123=CARTESIAN_POINT('Ctrl Pts',(1.48445385799994,5.2,3.80663866499999));
#336124=CARTESIAN_POINT('Ctrl Pts',(1.48445385799994,2.2,3.80663866499999));
#336125=CARTESIAN_POINT('Ctrl Pts',(1.48387274799994,12.2,3.80575938499998));
#336126=CARTESIAN_POINT('Ctrl Pts',(1.48387274799994,5.2,3.80575938499998));
#336127=CARTESIAN_POINT('Ctrl Pts',(1.48387274799994,2.2,3.80575938499998));
#336128=CARTESIAN_POINT('Ctrl Pts',(1.48329568599994,12.2,3.80488390099998));
#336129=CARTESIAN_POINT('Ctrl Pts',(1.48329568599994,5.2,3.80488390099998));
#336130=CARTESIAN_POINT('Ctrl Pts',(1.48329568599994,2.2,3.80488390099998));
#336131=CARTESIAN_POINT('Ctrl Pts',(1.48272266999994,12.2,3.80401222799998));
#336132=CARTESIAN_POINT('Ctrl Pts',(1.48272266999994,5.2,3.80401222799998));
#336133=CARTESIAN_POINT('Ctrl Pts',(1.48272266999994,2.2,3.80401222799998));
#336134=CARTESIAN_POINT('Ctrl Pts',(1.48215369199994,12.2,3.80314438299998));
#336135=CARTESIAN_POINT('Ctrl Pts',(1.48215369199994,5.2,3.80314438299998));
#336136=CARTESIAN_POINT('Ctrl Pts',(1.48215369199994,2.2,3.80314438299998));
#336137=CARTESIAN_POINT('Ctrl Pts',(1.48158874799994,12.2,3.80228038099998));
#336138=CARTESIAN_POINT('Ctrl Pts',(1.48158874799994,5.2,3.80228038099998));
#336139=CARTESIAN_POINT('Ctrl Pts',(1.48158874799994,2.2,3.80228038099998));
#336140=CARTESIAN_POINT('Ctrl Pts',(1.48102783599994,12.2,3.80142023799999));
#336141=CARTESIAN_POINT('Ctrl Pts',(1.48102783599994,5.2,3.80142023799999));
#336142=CARTESIAN_POINT('Ctrl Pts',(1.48102783599994,2.2,3.80142023799999));
#336143=CARTESIAN_POINT('Ctrl Pts',(1.48047094699994,12.2,3.80056396999999));
#336144=CARTESIAN_POINT('Ctrl Pts',(1.48047094699994,5.2,3.80056396999999));
#336145=CARTESIAN_POINT('Ctrl Pts',(1.48047094699994,2.2,3.80056396999999));
#336146=CARTESIAN_POINT('Ctrl Pts',(1.47991807899994,12.2,3.79971159099998));
#336147=CARTESIAN_POINT('Ctrl Pts',(1.47991807899994,5.2,3.79971159099998));
#336148=CARTESIAN_POINT('Ctrl Pts',(1.47991807899994,2.2,3.79971159099998));
#336149=CARTESIAN_POINT('Ctrl Pts',(1.47936922699994,12.2,3.79886311799999));
#336150=CARTESIAN_POINT('Ctrl Pts',(1.47936922699994,5.2,3.79886311799999));
#336151=CARTESIAN_POINT('Ctrl Pts',(1.47936922699994,2.2,3.79886311799999));
#336152=CARTESIAN_POINT('Ctrl Pts',(1.47882438399994,12.2,3.79801856699999));
#336153=CARTESIAN_POINT('Ctrl Pts',(1.47882438399994,5.2,3.79801856699999));
#336154=CARTESIAN_POINT('Ctrl Pts',(1.47882438399994,2.2,3.79801856699999));
#336155=CARTESIAN_POINT('Ctrl Pts',(1.47828354699994,12.2,3.79717795399999));
#336156=CARTESIAN_POINT('Ctrl Pts',(1.47828354699994,5.2,3.79717795399999));
#336157=CARTESIAN_POINT('Ctrl Pts',(1.47828354699994,2.2,3.79717795399999));
#336158=CARTESIAN_POINT('Ctrl Pts',(1.47774671099994,12.2,3.79634129599999));
#336159=CARTESIAN_POINT('Ctrl Pts',(1.47774671099994,5.2,3.79634129599999));
#336160=CARTESIAN_POINT('Ctrl Pts',(1.47774671099994,2.2,3.79634129599999));
#336161=CARTESIAN_POINT('Ctrl Pts',(1.47721387099994,12.2,3.79550860599998));
#336162=CARTESIAN_POINT('Ctrl Pts',(1.47721387099994,5.2,3.79550860599998));
#336163=CARTESIAN_POINT('Ctrl Pts',(1.47721387099994,2.2,3.79550860599998));
#336164=CARTESIAN_POINT('Ctrl Pts',(1.47668501999994,12.2,3.79467990299998));
#336165=CARTESIAN_POINT('Ctrl Pts',(1.47668501999994,5.2,3.79467990299998));
#336166=CARTESIAN_POINT('Ctrl Pts',(1.47668501999994,2.2,3.79467990299998));
#336167=CARTESIAN_POINT('Ctrl Pts',(1.47616015499994,12.2,3.79385519999998));
#336168=CARTESIAN_POINT('Ctrl Pts',(1.47616015499994,5.2,3.79385519999998));
#336169=CARTESIAN_POINT('Ctrl Pts',(1.47616015499994,2.2,3.79385519999998));
#336170=CARTESIAN_POINT('Ctrl Pts',(1.47563926899994,12.2,3.79303451599998));
#336171=CARTESIAN_POINT('Ctrl Pts',(1.47563926899994,5.2,3.79303451599998));
#336172=CARTESIAN_POINT('Ctrl Pts',(1.47563926899994,2.2,3.79303451599998));
#336173=CARTESIAN_POINT('Ctrl Pts',(1.47512235999994,12.2,3.79221786499999));
#336174=CARTESIAN_POINT('Ctrl Pts',(1.47512235999994,5.2,3.79221786499999));
#336175=CARTESIAN_POINT('Ctrl Pts',(1.47512235999994,2.2,3.79221786499999));
#336176=CARTESIAN_POINT('Ctrl Pts',(1.47460941899994,12.2,3.79140526399999));
#336177=CARTESIAN_POINT('Ctrl Pts',(1.47460941899994,5.2,3.79140526399999));
#336178=CARTESIAN_POINT('Ctrl Pts',(1.47460941899994,2.2,3.79140526399999));
#336179=CARTESIAN_POINT('Ctrl Pts',(1.47410044399994,12.2,3.79059672899999));
#336180=CARTESIAN_POINT('Ctrl Pts',(1.47410044399994,5.2,3.79059672899999));
#336181=CARTESIAN_POINT('Ctrl Pts',(1.47410044399994,2.2,3.79059672899999));
#336182=CARTESIAN_POINT('Ctrl Pts',(1.47359542799994,12.2,3.78979227699999));
#336183=CARTESIAN_POINT('Ctrl Pts',(1.47359542799994,5.2,3.78979227699999));
#336184=CARTESIAN_POINT('Ctrl Pts',(1.47359542799994,2.2,3.78979227699999));
#336185=CARTESIAN_POINT('Ctrl Pts',(1.47309436599994,12.2,3.78899192199999));
#336186=CARTESIAN_POINT('Ctrl Pts',(1.47309436599994,5.2,3.78899192199999));
#336187=CARTESIAN_POINT('Ctrl Pts',(1.47309436599994,2.2,3.78899192199999));
#336188=CARTESIAN_POINT('Ctrl Pts',(1.47259725299994,12.2,3.78819568399998));
#336189=CARTESIAN_POINT('Ctrl Pts',(1.47259725299994,5.2,3.78819568399998));
#336190=CARTESIAN_POINT('Ctrl Pts',(1.47259725299994,2.2,3.78819568399998));
#336191=CARTESIAN_POINT('Ctrl Pts',(1.47210408299994,12.2,3.78740357599998));
#336192=CARTESIAN_POINT('Ctrl Pts',(1.47210408299994,5.2,3.78740357599998));
#336193=CARTESIAN_POINT('Ctrl Pts',(1.47210408299994,2.2,3.78740357599998));
#336194=CARTESIAN_POINT('Ctrl Pts',(1.47161485199994,12.2,3.78661561499998));
#336195=CARTESIAN_POINT('Ctrl Pts',(1.47161485199994,5.2,3.78661561499998));
#336196=CARTESIAN_POINT('Ctrl Pts',(1.47161485199994,2.2,3.78661561499998));
#336197=CARTESIAN_POINT('Ctrl Pts',(1.47112955299994,12.2,3.78583181699998));
#336198=CARTESIAN_POINT('Ctrl Pts',(1.47112955299994,5.2,3.78583181699998));
#336199=CARTESIAN_POINT('Ctrl Pts',(1.47112955299994,2.2,3.78583181699998));
#336200=CARTESIAN_POINT('Ctrl Pts',(1.47064817999994,12.2,3.78505219999998));
#336201=CARTESIAN_POINT('Ctrl Pts',(1.47064817999994,5.2,3.78505219999998));
#336202=CARTESIAN_POINT('Ctrl Pts',(1.47064817999994,2.2,3.78505219999998));
#336203=CARTESIAN_POINT('Ctrl Pts',(1.47017072999994,12.2,3.78427677899998));
#336204=CARTESIAN_POINT('Ctrl Pts',(1.47017072999994,5.2,3.78427677899998));
#336205=CARTESIAN_POINT('Ctrl Pts',(1.47017072999994,2.2,3.78427677899998));
#336206=CARTESIAN_POINT('Ctrl Pts',(1.46969719599994,12.2,3.78350557199998));
#336207=CARTESIAN_POINT('Ctrl Pts',(1.46969719599994,5.2,3.78350557199998));
#336208=CARTESIAN_POINT('Ctrl Pts',(1.46969719599994,2.2,3.78350557199998));
#336209=CARTESIAN_POINT('Ctrl Pts',(1.46922757299994,12.2,3.78273859399999));
#336210=CARTESIAN_POINT('Ctrl Pts',(1.46922757299994,5.2,3.78273859399999));
#336211=CARTESIAN_POINT('Ctrl Pts',(1.46922757299994,2.2,3.78273859399999));
#336212=CARTESIAN_POINT('Ctrl Pts',(1.46876185499994,12.2,3.78197586199998));
#336213=CARTESIAN_POINT('Ctrl Pts',(1.46876185499994,5.2,3.78197586199998));
#336214=CARTESIAN_POINT('Ctrl Pts',(1.46876185499994,2.2,3.78197586199998));
#336215=CARTESIAN_POINT('Ctrl Pts',(1.46830003499994,12.2,3.78121739299999));
#336216=CARTESIAN_POINT('Ctrl Pts',(1.46830003499994,5.2,3.78121739299999));
#336217=CARTESIAN_POINT('Ctrl Pts',(1.46830003499994,2.2,3.78121739299999));
#336218=CARTESIAN_POINT('Ctrl Pts',(1.46784210999995,12.2,3.78046320299998));
#336219=CARTESIAN_POINT('Ctrl Pts',(1.46784210999995,5.2,3.78046320299998));
#336220=CARTESIAN_POINT('Ctrl Pts',(1.46784210999995,2.2,3.78046320299998));
#336221=CARTESIAN_POINT('Ctrl Pts',(1.46738807199994,12.2,3.77971330899998));
#336222=CARTESIAN_POINT('Ctrl Pts',(1.46738807199994,5.2,3.77971330899998));
#336223=CARTESIAN_POINT('Ctrl Pts',(1.46738807199994,2.2,3.77971330899998));
#336224=CARTESIAN_POINT('Ctrl Pts',(1.46693791799994,12.2,3.77896772699999));
#336225=CARTESIAN_POINT('Ctrl Pts',(1.46693791799994,5.2,3.77896772699999));
#336226=CARTESIAN_POINT('Ctrl Pts',(1.46693791799994,2.2,3.77896772699999));
#336227=CARTESIAN_POINT('Ctrl Pts',(1.46649163899994,12.2,3.77822647599999));
#336228=CARTESIAN_POINT('Ctrl Pts',(1.46649163899994,5.2,3.77822647599999));
#336229=CARTESIAN_POINT('Ctrl Pts',(1.46649163899994,2.2,3.77822647599999));
#336230=CARTESIAN_POINT('Ctrl Pts',(1.46604923099994,12.2,3.77748956899998));
#336231=CARTESIAN_POINT('Ctrl Pts',(1.46604923099994,5.2,3.77748956899998));
#336232=CARTESIAN_POINT('Ctrl Pts',(1.46604923099994,2.2,3.77748956899998));
#336233=CARTESIAN_POINT('Ctrl Pts',(1.46561068799994,12.2,3.77675702699998));
#336234=CARTESIAN_POINT('Ctrl Pts',(1.46561068799994,5.2,3.77675702699998));
#336235=CARTESIAN_POINT('Ctrl Pts',(1.46561068799994,2.2,3.77675702699998));
#336236=CARTESIAN_POINT('Ctrl Pts',(1.46517600399994,12.2,3.77602886399998));
#336237=CARTESIAN_POINT('Ctrl Pts',(1.46517600399994,5.2,3.77602886399998));
#336238=CARTESIAN_POINT('Ctrl Pts',(1.46517600399994,2.2,3.77602886399998));
#336239=CARTESIAN_POINT('Ctrl Pts',(1.46474517199994,12.2,3.77530509699999));
#336240=CARTESIAN_POINT('Ctrl Pts',(1.46474517199994,5.2,3.77530509699999));
#336241=CARTESIAN_POINT('Ctrl Pts',(1.46474517199994,2.2,3.77530509699999));
#336242=CARTESIAN_POINT('Ctrl Pts',(1.46431818799994,12.2,3.77458574399999));
#336243=CARTESIAN_POINT('Ctrl Pts',(1.46431818799994,5.2,3.77458574399999));
#336244=CARTESIAN_POINT('Ctrl Pts',(1.46431818799994,2.2,3.77458574399999));
#336245=CARTESIAN_POINT('Ctrl Pts',(1.46389504399994,12.2,3.77387082099998));
#336246=CARTESIAN_POINT('Ctrl Pts',(1.46389504399994,5.2,3.77387082099998));
#336247=CARTESIAN_POINT('Ctrl Pts',(1.46389504399994,2.2,3.77387082099998));
#336248=CARTESIAN_POINT('Ctrl Pts',(1.46347573699994,12.2,3.77316034699999));
#336249=CARTESIAN_POINT('Ctrl Pts',(1.46347573699994,5.2,3.77316034699999));
#336250=CARTESIAN_POINT('Ctrl Pts',(1.46347573699994,2.2,3.77316034699999));
#336251=CARTESIAN_POINT('Ctrl Pts',(1.46306025699994,12.2,3.77245433599998));
#336252=CARTESIAN_POINT('Ctrl Pts',(1.46306025699994,5.2,3.77245433599998));
#336253=CARTESIAN_POINT('Ctrl Pts',(1.46306025699994,2.2,3.77245433599998));
#336254=CARTESIAN_POINT('Ctrl Pts',(1.46264860099994,12.2,3.77175280699999));
#336255=CARTESIAN_POINT('Ctrl Pts',(1.46264860099994,5.2,3.77175280699999));
#336256=CARTESIAN_POINT('Ctrl Pts',(1.46264860099994,2.2,3.77175280699999));
#336257=CARTESIAN_POINT('Ctrl Pts',(1.46224076099994,12.2,3.77105577799998));
#336258=CARTESIAN_POINT('Ctrl Pts',(1.46224076099994,5.2,3.77105577799998));
#336259=CARTESIAN_POINT('Ctrl Pts',(1.46224076099994,2.2,3.77105577799998));
#336260=CARTESIAN_POINT('Ctrl Pts',(1.46183673199994,12.2,3.77036326399999));
#336261=CARTESIAN_POINT('Ctrl Pts',(1.46183673199994,5.2,3.77036326399999));
#336262=CARTESIAN_POINT('Ctrl Pts',(1.46183673199994,2.2,3.77036326399999));
#336263=CARTESIAN_POINT('Ctrl Pts',(1.46143650699994,12.2,3.76967528299998));
#336264=CARTESIAN_POINT('Ctrl Pts',(1.46143650699994,5.2,3.76967528299998));
#336265=CARTESIAN_POINT('Ctrl Pts',(1.46143650699994,2.2,3.76967528299998));
#336266=CARTESIAN_POINT('Ctrl Pts',(1.46104007999994,12.2,3.76899185199999));
#336267=CARTESIAN_POINT('Ctrl Pts',(1.46104007999994,5.2,3.76899185199999));
#336268=CARTESIAN_POINT('Ctrl Pts',(1.46104007999994,2.2,3.76899185199999));
#336269=CARTESIAN_POINT('Ctrl Pts',(1.46064744499994,12.2,3.76831298899998));
#336270=CARTESIAN_POINT('Ctrl Pts',(1.46064744499994,5.2,3.76831298899998));
#336271=CARTESIAN_POINT('Ctrl Pts',(1.46064744499994,2.2,3.76831298899998));
#336272=CARTESIAN_POINT('Ctrl Pts',(1.46025859499994,12.2,3.76763871099998));
#336273=CARTESIAN_POINT('Ctrl Pts',(1.46025859499994,5.2,3.76763871099998));
#336274=CARTESIAN_POINT('Ctrl Pts',(1.46025859499994,2.2,3.76763871099998));
#336275=CARTESIAN_POINT('Ctrl Pts',(1.45987352399994,12.2,3.76696903499998));
#336276=CARTESIAN_POINT('Ctrl Pts',(1.45987352399994,5.2,3.76696903499998));
#336277=CARTESIAN_POINT('Ctrl Pts',(1.45987352399994,2.2,3.76696903499998));
#336278=CARTESIAN_POINT('Ctrl Pts',(1.45949222599994,12.2,3.76630397899999));
#336279=CARTESIAN_POINT('Ctrl Pts',(1.45949222599994,5.2,3.76630397899999));
#336280=CARTESIAN_POINT('Ctrl Pts',(1.45949222599994,2.2,3.76630397899999));
#336281=CARTESIAN_POINT('Ctrl Pts',(1.45911469399994,12.2,3.76564355999999));
#336282=CARTESIAN_POINT('Ctrl Pts',(1.45911469399994,5.2,3.76564355999999));
#336283=CARTESIAN_POINT('Ctrl Pts',(1.45911469399994,2.2,3.76564355999999));
#336284=CARTESIAN_POINT('Ctrl Pts',(1.45874092099994,12.2,3.76498779599999));
#336285=CARTESIAN_POINT('Ctrl Pts',(1.45874092099994,5.2,3.76498779599999));
#336286=CARTESIAN_POINT('Ctrl Pts',(1.45874092099994,2.2,3.76498779599999));
#336287=CARTESIAN_POINT('Ctrl Pts',(1.45837090199994,12.2,3.76433670299999));
#336288=CARTESIAN_POINT('Ctrl Pts',(1.45837090199994,5.2,3.76433670299999));
#336289=CARTESIAN_POINT('Ctrl Pts',(1.45837090199994,2.2,3.76433670299999));
#336290=CARTESIAN_POINT('Ctrl Pts',(1.45800462899994,12.2,3.76369030099998));
#336291=CARTESIAN_POINT('Ctrl Pts',(1.45800462899994,5.2,3.76369030099998));
#336292=CARTESIAN_POINT('Ctrl Pts',(1.45800462899994,2.2,3.76369030099998));
#336293=CARTESIAN_POINT('Ctrl Pts',(1.45764209599994,12.2,3.76304860499998));
#336294=CARTESIAN_POINT('Ctrl Pts',(1.45764209599994,5.2,3.76304860499998));
#336295=CARTESIAN_POINT('Ctrl Pts',(1.45764209599994,2.2,3.76304860499998));
#336296=CARTESIAN_POINT('Ctrl Pts',(1.45728329599994,12.2,3.76241163399998));
#336297=CARTESIAN_POINT('Ctrl Pts',(1.45728329599994,5.2,3.76241163399998));
#336298=CARTESIAN_POINT('Ctrl Pts',(1.45728329599994,2.2,3.76241163399998));
#336299=CARTESIAN_POINT('Ctrl Pts',(1.45692822299994,12.2,3.76177940599998));
#336300=CARTESIAN_POINT('Ctrl Pts',(1.45692822299994,5.2,3.76177940599998));
#336301=CARTESIAN_POINT('Ctrl Pts',(1.45692822299994,2.2,3.76177940599998));
#336302=CARTESIAN_POINT('Ctrl Pts',(1.45657686999994,12.2,3.76115193799999));
#336303=CARTESIAN_POINT('Ctrl Pts',(1.45657686999994,5.2,3.76115193799999));
#336304=CARTESIAN_POINT('Ctrl Pts',(1.45657686999994,2.2,3.76115193799999));
#336305=CARTESIAN_POINT('Ctrl Pts',(1.45622922999994,12.2,3.76052924899999));
#336306=CARTESIAN_POINT('Ctrl Pts',(1.45622922999994,5.2,3.76052924899999));
#336307=CARTESIAN_POINT('Ctrl Pts',(1.45622922999994,2.2,3.76052924899999));
#336308=CARTESIAN_POINT('Ctrl Pts',(1.45588529499994,12.2,3.75991135499999));
#336309=CARTESIAN_POINT('Ctrl Pts',(1.45588529499994,5.2,3.75991135499999));
#336310=CARTESIAN_POINT('Ctrl Pts',(1.45588529499994,2.2,3.75991135499999));
#336311=CARTESIAN_POINT('Ctrl Pts',(1.45554505999994,12.2,3.75929827399998));
#336312=CARTESIAN_POINT('Ctrl Pts',(1.45554505999994,5.2,3.75929827399998));
#336313=CARTESIAN_POINT('Ctrl Pts',(1.45554505999994,2.2,3.75929827399998));
#336314=CARTESIAN_POINT('Ctrl Pts',(1.45520851699994,12.2,3.75869002599998));
#336315=CARTESIAN_POINT('Ctrl Pts',(1.45520851699994,5.2,3.75869002599998));
#336316=CARTESIAN_POINT('Ctrl Pts',(1.45520851699994,2.2,3.75869002599998));
#336317=CARTESIAN_POINT('Ctrl Pts',(1.45487566099994,12.2,3.75808662699999));
#336318=CARTESIAN_POINT('Ctrl Pts',(1.45487566099994,5.2,3.75808662699999));
#336319=CARTESIAN_POINT('Ctrl Pts',(1.45487566099994,2.2,3.75808662699999));
#336320=CARTESIAN_POINT('Ctrl Pts',(1.45454648199994,12.2,3.75748809499999));
#336321=CARTESIAN_POINT('Ctrl Pts',(1.45454648199994,5.2,3.75748809499999));
#336322=CARTESIAN_POINT('Ctrl Pts',(1.45454648199994,2.2,3.75748809499999));
#336323=CARTESIAN_POINT('Ctrl Pts',(1.45422097599994,12.2,3.75689444899999));
#336324=CARTESIAN_POINT('Ctrl Pts',(1.45422097599994,5.2,3.75689444899999));
#336325=CARTESIAN_POINT('Ctrl Pts',(1.45422097599994,2.2,3.75689444899999));
#336326=CARTESIAN_POINT('Ctrl Pts',(1.45389913299994,12.2,3.75630570599998));
#336327=CARTESIAN_POINT('Ctrl Pts',(1.45389913299994,5.2,3.75630570599998));
#336328=CARTESIAN_POINT('Ctrl Pts',(1.45389913299994,2.2,3.75630570599998));
#336329=CARTESIAN_POINT('Ctrl Pts',(1.45358094899994,12.2,3.75572188599998));
#336330=CARTESIAN_POINT('Ctrl Pts',(1.45358094899994,5.2,3.75572188599998));
#336331=CARTESIAN_POINT('Ctrl Pts',(1.45358094899994,2.2,3.75572188599998));
#336332=CARTESIAN_POINT('Ctrl Pts',(1.45326641399994,12.2,3.75514300499999));
#336333=CARTESIAN_POINT('Ctrl Pts',(1.45326641399994,5.2,3.75514300499999));
#336334=CARTESIAN_POINT('Ctrl Pts',(1.45326641399994,2.2,3.75514300499999));
#336335=CARTESIAN_POINT('Ctrl Pts',(1.45295552199994,12.2,3.75456908199999));
#336336=CARTESIAN_POINT('Ctrl Pts',(1.45295552199994,5.2,3.75456908199999));
#336337=CARTESIAN_POINT('Ctrl Pts',(1.45295552199994,2.2,3.75456908199999));
#336338=CARTESIAN_POINT('Ctrl Pts',(1.45264826499994,12.2,3.75400013499998));
#336339=CARTESIAN_POINT('Ctrl Pts',(1.45264826499994,5.2,3.75400013499998));
#336340=CARTESIAN_POINT('Ctrl Pts',(1.45264826499994,2.2,3.75400013499998));
#336341=CARTESIAN_POINT('Ctrl Pts',(1.45234463799994,12.2,3.75343618299999));
#336342=CARTESIAN_POINT('Ctrl Pts',(1.45234463799994,5.2,3.75343618299999));
#336343=CARTESIAN_POINT('Ctrl Pts',(1.45234463799994,2.2,3.75343618299999));
#336344=CARTESIAN_POINT('Ctrl Pts',(1.45204463099994,12.2,3.75287724399998));
#336345=CARTESIAN_POINT('Ctrl Pts',(1.45204463099994,5.2,3.75287724399998));
#336346=CARTESIAN_POINT('Ctrl Pts',(1.45204463099994,2.2,3.75287724399998));
#336347=CARTESIAN_POINT('Ctrl Pts',(1.45174823799994,12.2,3.75232333599998));
#336348=CARTESIAN_POINT('Ctrl Pts',(1.45174823799994,5.2,3.75232333599998));
#336349=CARTESIAN_POINT('Ctrl Pts',(1.45174823799994,2.2,3.75232333599998));
#336350=CARTESIAN_POINT('Ctrl Pts',(1.45145545199994,12.2,3.75177447799998));
#336351=CARTESIAN_POINT('Ctrl Pts',(1.45145545199994,5.2,3.75177447799998));
#336352=CARTESIAN_POINT('Ctrl Pts',(1.45145545199994,2.2,3.75177447799998));
#336353=CARTESIAN_POINT('Ctrl Pts',(1.45116626499994,12.2,3.75123068799999));
#336354=CARTESIAN_POINT('Ctrl Pts',(1.45116626499994,5.2,3.75123068799999));
#336355=CARTESIAN_POINT('Ctrl Pts',(1.45116626499994,2.2,3.75123068799999));
#336356=CARTESIAN_POINT('Ctrl Pts',(1.45088066799994,12.2,3.75069198499999));
#336357=CARTESIAN_POINT('Ctrl Pts',(1.45088066799994,5.2,3.75069198499999));
#336358=CARTESIAN_POINT('Ctrl Pts',(1.45088066799994,2.2,3.75069198499999));
#336359=CARTESIAN_POINT('Ctrl Pts',(1.45059865499995,12.2,3.75015838699999));
#336360=CARTESIAN_POINT('Ctrl Pts',(1.45059865499995,5.2,3.75015838699999));
#336361=CARTESIAN_POINT('Ctrl Pts',(1.45059865499995,2.2,3.75015838699999));
#336362=CARTESIAN_POINT('Ctrl Pts',(1.45032021899994,12.2,3.74962991299999));
#336363=CARTESIAN_POINT('Ctrl Pts',(1.45032021899994,5.2,3.74962991299999));
#336364=CARTESIAN_POINT('Ctrl Pts',(1.45032021899994,2.2,3.74962991299999));
#336365=CARTESIAN_POINT('Ctrl Pts',(1.45004535099994,12.2,3.74910658199998));
#336366=CARTESIAN_POINT('Ctrl Pts',(1.45004535099994,5.2,3.74910658199998));
#336367=CARTESIAN_POINT('Ctrl Pts',(1.45004535099994,2.2,3.74910658199998));
#336368=CARTESIAN_POINT('Ctrl Pts',(1.44977404499994,12.2,3.74858841099999));
#336369=CARTESIAN_POINT('Ctrl Pts',(1.44977404499994,5.2,3.74858841099999));
#336370=CARTESIAN_POINT('Ctrl Pts',(1.44977404499994,2.2,3.74858841099999));
#336371=CARTESIAN_POINT('Ctrl Pts',(1.44950629199994,12.2,3.74807542099998));
#336372=CARTESIAN_POINT('Ctrl Pts',(1.44950629199994,5.2,3.74807542099998));
#336373=CARTESIAN_POINT('Ctrl Pts',(1.44950629199994,2.2,3.74807542099998));
#336374=CARTESIAN_POINT('Ctrl Pts',(1.44924208299994,12.2,3.74756762899998));
#336375=CARTESIAN_POINT('Ctrl Pts',(1.44924208299994,5.2,3.74756762899998));
#336376=CARTESIAN_POINT('Ctrl Pts',(1.44924208299994,2.2,3.74756762899998));
#336377=CARTESIAN_POINT('Ctrl Pts',(1.44898141299994,12.2,3.74706505499999));
#336378=CARTESIAN_POINT('Ctrl Pts',(1.44898141299994,5.2,3.74706505499999));
#336379=CARTESIAN_POINT('Ctrl Pts',(1.44898141299994,2.2,3.74706505499999));
#336380=CARTESIAN_POINT('Ctrl Pts',(1.44872427199994,12.2,3.74656771799999));
#336381=CARTESIAN_POINT('Ctrl Pts',(1.44872427199994,5.2,3.74656771799999));
#336382=CARTESIAN_POINT('Ctrl Pts',(1.44872427199994,2.2,3.74656771799999));
#336383=CARTESIAN_POINT('Ctrl Pts',(1.44847065299994,12.2,3.74607563599999));
#336384=CARTESIAN_POINT('Ctrl Pts',(1.44847065299994,5.2,3.74607563599999));
#336385=CARTESIAN_POINT('Ctrl Pts',(1.44847065299994,2.2,3.74607563599999));
#336386=CARTESIAN_POINT('Ctrl Pts',(1.44822054799994,12.2,3.74558882799998));
#336387=CARTESIAN_POINT('Ctrl Pts',(1.44822054799994,5.2,3.74558882799998));
#336388=CARTESIAN_POINT('Ctrl Pts',(1.44822054799994,2.2,3.74558882799998));
#336389=CARTESIAN_POINT('Ctrl Pts',(1.44797394999994,12.2,3.74510731399998));
#336390=CARTESIAN_POINT('Ctrl Pts',(1.44797394999994,5.2,3.74510731399998));
#336391=CARTESIAN_POINT('Ctrl Pts',(1.44797394999994,2.2,3.74510731399998));
#336392=CARTESIAN_POINT('Ctrl Pts',(1.44773084699994,12.2,3.74463111299999));
#336393=CARTESIAN_POINT('Ctrl Pts',(1.44773084699994,5.2,3.74463111299999));
#336394=CARTESIAN_POINT('Ctrl Pts',(1.44773084699994,2.2,3.74463111299999));
#336395=CARTESIAN_POINT('Ctrl Pts',(1.44749123599994,12.2,3.74416024299999));
#336396=CARTESIAN_POINT('Ctrl Pts',(1.44749123599994,5.2,3.74416024299999));
#336397=CARTESIAN_POINT('Ctrl Pts',(1.44749123599994,2.2,3.74416024299999));
#336398=CARTESIAN_POINT('Ctrl Pts',(1.44725510599994,12.2,3.74369472399999));
#336399=CARTESIAN_POINT('Ctrl Pts',(1.44725510599994,5.2,3.74369472399999));
#336400=CARTESIAN_POINT('Ctrl Pts',(1.44725510599994,2.2,3.74369472399999));
#336401=CARTESIAN_POINT('Ctrl Pts',(1.44702244999994,12.2,3.74323457499998));
#336402=CARTESIAN_POINT('Ctrl Pts',(1.44702244999994,5.2,3.74323457499998));
#336403=CARTESIAN_POINT('Ctrl Pts',(1.44702244999994,2.2,3.74323457499998));
#336404=CARTESIAN_POINT('Ctrl Pts',(1.44679325699994,12.2,3.74277981599998));
#336405=CARTESIAN_POINT('Ctrl Pts',(1.44679325699994,5.2,3.74277981599998));
#336406=CARTESIAN_POINT('Ctrl Pts',(1.44679325699994,2.2,3.74277981599998));
#336407=CARTESIAN_POINT('Ctrl Pts',(1.44656752299994,12.2,3.74233046599999));
#336408=CARTESIAN_POINT('Ctrl Pts',(1.44656752299994,5.2,3.74233046599999));
#336409=CARTESIAN_POINT('Ctrl Pts',(1.44656752299994,2.2,3.74233046599999));
#336410=CARTESIAN_POINT('Ctrl Pts',(1.44634523599994,12.2,3.74188654299999));
#336411=CARTESIAN_POINT('Ctrl Pts',(1.44634523599994,5.2,3.74188654299999));
#336412=CARTESIAN_POINT('Ctrl Pts',(1.44634523599994,2.2,3.74188654299999));
#336413=CARTESIAN_POINT('Ctrl Pts',(1.44612638999994,12.2,3.74144806799999));
#336414=CARTESIAN_POINT('Ctrl Pts',(1.44612638999994,5.2,3.74144806799999));
#336415=CARTESIAN_POINT('Ctrl Pts',(1.44612638999994,2.2,3.74144806799999));
#336416=CARTESIAN_POINT('Ctrl Pts',(1.44591097499994,12.2,3.74101505999998));
#336417=CARTESIAN_POINT('Ctrl Pts',(1.44591097499994,5.2,3.74101505999998));
#336418=CARTESIAN_POINT('Ctrl Pts',(1.44591097499994,2.2,3.74101505999998));
#336419=CARTESIAN_POINT('Ctrl Pts',(1.44569898399994,12.2,3.74058753799999));
#336420=CARTESIAN_POINT('Ctrl Pts',(1.44569898399994,5.2,3.74058753799999));
#336421=CARTESIAN_POINT('Ctrl Pts',(1.44569898399994,2.2,3.74058753799999));
#336422=CARTESIAN_POINT('Ctrl Pts',(1.44549040799994,12.2,3.74016552299998));
#336423=CARTESIAN_POINT('Ctrl Pts',(1.44549040799994,5.2,3.74016552299998));
#336424=CARTESIAN_POINT('Ctrl Pts',(1.44549040799994,2.2,3.74016552299998));
#336425=CARTESIAN_POINT('Ctrl Pts',(1.44528523599994,12.2,3.73974903399999));
#336426=CARTESIAN_POINT('Ctrl Pts',(1.44528523599994,5.2,3.73974903399999));
#336427=CARTESIAN_POINT('Ctrl Pts',(1.44528523599994,2.2,3.73974903399999));
#336428=CARTESIAN_POINT('Ctrl Pts',(1.44508346299994,12.2,3.73933809099999));
#336429=CARTESIAN_POINT('Ctrl Pts',(1.44508346299994,5.2,3.73933809099999));
#336430=CARTESIAN_POINT('Ctrl Pts',(1.44508346299994,2.2,3.73933809099999));
#336431=CARTESIAN_POINT('Ctrl Pts',(1.44488507799994,12.2,3.73893271199999));
#336432=CARTESIAN_POINT('Ctrl Pts',(1.44488507799994,5.2,3.73893271199999));
#336433=CARTESIAN_POINT('Ctrl Pts',(1.44488507799994,2.2,3.73893271199999));
#336434=CARTESIAN_POINT('Ctrl Pts',(1.44469007399994,12.2,3.73853291899999));
#336435=CARTESIAN_POINT('Ctrl Pts',(1.44469007399994,5.2,3.73853291899999));
#336436=CARTESIAN_POINT('Ctrl Pts',(1.44469007399994,2.2,3.73853291899999));
#336437=CARTESIAN_POINT('Ctrl Pts',(1.44449844099994,12.2,3.73813872999998));
#336438=CARTESIAN_POINT('Ctrl Pts',(1.44449844099994,5.2,3.73813872999998));
#336439=CARTESIAN_POINT('Ctrl Pts',(1.44449844099994,2.2,3.73813872999998));
#336440=CARTESIAN_POINT('Ctrl Pts',(1.44431016899994,12.2,3.73775016699998));
#336441=CARTESIAN_POINT('Ctrl Pts',(1.44431016899994,5.2,3.73775016699998));
#336442=CARTESIAN_POINT('Ctrl Pts',(1.44431016899994,2.2,3.73775016699998));
#336443=CARTESIAN_POINT('Ctrl Pts',(1.44412525099994,12.2,3.73736724799999));
#336444=CARTESIAN_POINT('Ctrl Pts',(1.44412525099994,5.2,3.73736724799999));
#336445=CARTESIAN_POINT('Ctrl Pts',(1.44412525099994,2.2,3.73736724799999));
#336446=CARTESIAN_POINT('Ctrl Pts',(1.44394367899994,12.2,3.73698999399998));
#336447=CARTESIAN_POINT('Ctrl Pts',(1.44394367899994,5.2,3.73698999399998));
#336448=CARTESIAN_POINT('Ctrl Pts',(1.44394367899994,2.2,3.73698999399998));
#336449=CARTESIAN_POINT('Ctrl Pts',(1.44376544099994,12.2,3.73661842499998));
#336450=CARTESIAN_POINT('Ctrl Pts',(1.44376544099994,5.2,3.73661842499998));
#336451=CARTESIAN_POINT('Ctrl Pts',(1.44376544099994,2.2,3.73661842499998));
#336452=CARTESIAN_POINT('Ctrl Pts',(1.44359052999994,12.2,3.73625256099999));
#336453=CARTESIAN_POINT('Ctrl Pts',(1.44359052999994,5.2,3.73625256099999));
#336454=CARTESIAN_POINT('Ctrl Pts',(1.44359052999994,2.2,3.73625256099999));
#336455=CARTESIAN_POINT('Ctrl Pts',(1.44341893599994,12.2,3.73589242199999));
#336456=CARTESIAN_POINT('Ctrl Pts',(1.44341893599994,5.2,3.73589242199999));
#336457=CARTESIAN_POINT('Ctrl Pts',(1.44341893599994,2.2,3.73589242199999));
#336458=CARTESIAN_POINT('Ctrl Pts',(1.44325064999994,12.2,3.73553802799999));
#336459=CARTESIAN_POINT('Ctrl Pts',(1.44325064999994,5.2,3.73553802799999));
#336460=CARTESIAN_POINT('Ctrl Pts',(1.44325064999994,2.2,3.73553802799999));
#336461=CARTESIAN_POINT('Ctrl Pts',(1.44308566399994,12.2,3.73518940099999));
#336462=CARTESIAN_POINT('Ctrl Pts',(1.44308566399994,5.2,3.73518940099999));
#336463=CARTESIAN_POINT('Ctrl Pts',(1.44308566399994,2.2,3.73518940099999));
#336464=CARTESIAN_POINT('Ctrl Pts',(1.44292396699994,12.2,3.73484655899999));
#336465=CARTESIAN_POINT('Ctrl Pts',(1.44292396699994,5.2,3.73484655899999));
#336466=CARTESIAN_POINT('Ctrl Pts',(1.44292396699994,2.2,3.73484655899999));
#336467=CARTESIAN_POINT('Ctrl Pts',(1.44276555099994,12.2,3.73450952399998));
#336468=CARTESIAN_POINT('Ctrl Pts',(1.44276555099994,5.2,3.73450952399998));
#336469=CARTESIAN_POINT('Ctrl Pts',(1.44276555099994,2.2,3.73450952399998));
#336470=CARTESIAN_POINT('Ctrl Pts',(1.44261040599994,12.2,3.73417831599999));
#336471=CARTESIAN_POINT('Ctrl Pts',(1.44261040599994,5.2,3.73417831599999));
#336472=CARTESIAN_POINT('Ctrl Pts',(1.44261040599994,2.2,3.73417831599999));
#336473=CARTESIAN_POINT('Ctrl Pts',(1.44245852199994,12.2,3.73385295499999));
#336474=CARTESIAN_POINT('Ctrl Pts',(1.44245852199994,5.2,3.73385295499999));
#336475=CARTESIAN_POINT('Ctrl Pts',(1.44245852199994,2.2,3.73385295499999));
#336476=CARTESIAN_POINT('Ctrl Pts',(1.44230989099994,12.2,3.73353346199998));
#336477=CARTESIAN_POINT('Ctrl Pts',(1.44230989099994,5.2,3.73353346199998));
#336478=CARTESIAN_POINT('Ctrl Pts',(1.44230989099994,2.2,3.73353346199998));
#336479=CARTESIAN_POINT('Ctrl Pts',(1.44216450299994,12.2,3.73321985799999));
#336480=CARTESIAN_POINT('Ctrl Pts',(1.44216450299994,5.2,3.73321985799999));
#336481=CARTESIAN_POINT('Ctrl Pts',(1.44216450299994,2.2,3.73321985799999));
#336482=CARTESIAN_POINT('Ctrl Pts',(1.44202234599994,12.2,3.73291216299998));
#336483=CARTESIAN_POINT('Ctrl Pts',(1.44202234599994,5.2,3.73291216299998));
#336484=CARTESIAN_POINT('Ctrl Pts',(1.44202234599994,2.2,3.73291216299998));
#336485=CARTESIAN_POINT('Ctrl Pts',(1.44188341399994,12.2,3.73261039799999));
#336486=CARTESIAN_POINT('Ctrl Pts',(1.44188341399994,5.2,3.73261039799999));
#336487=CARTESIAN_POINT('Ctrl Pts',(1.44188341399994,2.2,3.73261039799999));
#336488=CARTESIAN_POINT('Ctrl Pts',(1.44174769599994,12.2,3.73231458499999));
#336489=CARTESIAN_POINT('Ctrl Pts',(1.44174769599994,5.2,3.73231458499999));
#336490=CARTESIAN_POINT('Ctrl Pts',(1.44174769599994,2.2,3.73231458499999));
#336491=CARTESIAN_POINT('Ctrl Pts',(1.44161518099994,12.2,3.73202474299998));
#336492=CARTESIAN_POINT('Ctrl Pts',(1.44161518099994,5.2,3.73202474299998));
#336493=CARTESIAN_POINT('Ctrl Pts',(1.44161518099994,2.2,3.73202474299998));
#336494=CARTESIAN_POINT('Ctrl Pts',(1.44148585999994,12.2,3.73174089299999));
#336495=CARTESIAN_POINT('Ctrl Pts',(1.44148585999994,5.2,3.73174089299999));
#336496=CARTESIAN_POINT('Ctrl Pts',(1.44148585999994,2.2,3.73174089299999));
#336497=CARTESIAN_POINT('Ctrl Pts',(1.44135972499994,12.2,3.73146305799998));
#336498=CARTESIAN_POINT('Ctrl Pts',(1.44135972499994,5.2,3.73146305799998));
#336499=CARTESIAN_POINT('Ctrl Pts',(1.44135972499994,2.2,3.73146305799998));
#336500=CARTESIAN_POINT('Ctrl Pts',(1.44123676199994,12.2,3.73119125799998));
#336501=CARTESIAN_POINT('Ctrl Pts',(1.44123676199994,5.2,3.73119125799998));
#336502=CARTESIAN_POINT('Ctrl Pts',(1.44123676199994,2.2,3.73119125799998));
#336503=CARTESIAN_POINT('Ctrl Pts',(1.44111696499994,12.2,3.73092551199999));
#336504=CARTESIAN_POINT('Ctrl Pts',(1.44111696499994,5.2,3.73092551199999));
#336505=CARTESIAN_POINT('Ctrl Pts',(1.44111696499994,2.2,3.73092551199999));
#336506=CARTESIAN_POINT('Ctrl Pts',(1.44100032099994,12.2,3.73066584399999));
#336507=CARTESIAN_POINT('Ctrl Pts',(1.44100032099994,5.2,3.73066584399999));
#336508=CARTESIAN_POINT('Ctrl Pts',(1.44100032099994,2.2,3.73066584399999));
#336509=CARTESIAN_POINT('Ctrl Pts',(1.44088682199994,12.2,3.73041227499999));
#336510=CARTESIAN_POINT('Ctrl Pts',(1.44088682199994,5.2,3.73041227499999));
#336511=CARTESIAN_POINT('Ctrl Pts',(1.44088682199994,2.2,3.73041227499999));
#336512=CARTESIAN_POINT('Ctrl Pts',(1.44077645799994,12.2,3.73016482399999));
#336513=CARTESIAN_POINT('Ctrl Pts',(1.44077645799994,5.2,3.73016482399999));
#336514=CARTESIAN_POINT('Ctrl Pts',(1.44077645799994,2.2,3.73016482399999));
#336515=CARTESIAN_POINT('Ctrl Pts',(1.44066921699994,12.2,3.72992351399999));
#336516=CARTESIAN_POINT('Ctrl Pts',(1.44066921699994,5.2,3.72992351399999));
#336517=CARTESIAN_POINT('Ctrl Pts',(1.44066921699994,2.2,3.72992351399999));
#336518=CARTESIAN_POINT('Ctrl Pts',(1.44056508899994,12.2,3.72968836699999));
#336519=CARTESIAN_POINT('Ctrl Pts',(1.44056508899994,5.2,3.72968836699999));
#336520=CARTESIAN_POINT('Ctrl Pts',(1.44056508899994,2.2,3.72968836699999));
#336521=CARTESIAN_POINT('Ctrl Pts',(1.44046406499994,12.2,3.72945940399998));
#336522=CARTESIAN_POINT('Ctrl Pts',(1.44046406499994,5.2,3.72945940399998));
#336523=CARTESIAN_POINT('Ctrl Pts',(1.44046406499994,2.2,3.72945940399998));
#336524=CARTESIAN_POINT('Ctrl Pts',(1.44036613299994,12.2,3.72923664599998));
#336525=CARTESIAN_POINT('Ctrl Pts',(1.44036613299994,5.2,3.72923664599998));
#336526=CARTESIAN_POINT('Ctrl Pts',(1.44036613299994,2.2,3.72923664599998));
#336527=CARTESIAN_POINT('Ctrl Pts',(1.44027128399994,12.2,3.72902011499999));
#336528=CARTESIAN_POINT('Ctrl Pts',(1.44027128399994,5.2,3.72902011499999));
#336529=CARTESIAN_POINT('Ctrl Pts',(1.44027128399994,2.2,3.72902011499999));
#336530=CARTESIAN_POINT('Ctrl Pts',(1.44017950699994,12.2,3.72880983299999));
#336531=CARTESIAN_POINT('Ctrl Pts',(1.44017950699994,5.2,3.72880983299999));
#336532=CARTESIAN_POINT('Ctrl Pts',(1.44017950699994,2.2,3.72880983299999));
#336533=CARTESIAN_POINT('Ctrl Pts',(1.44009079099994,12.2,3.72860581999999));
#336534=CARTESIAN_POINT('Ctrl Pts',(1.44009079099994,5.2,3.72860581999999));
#336535=CARTESIAN_POINT('Ctrl Pts',(1.44009079099994,2.2,3.72860581999999));
#336536=CARTESIAN_POINT('Ctrl Pts',(1.44000512699994,12.2,3.72840809899999));
#336537=CARTESIAN_POINT('Ctrl Pts',(1.44000512699994,5.2,3.72840809899999));
#336538=CARTESIAN_POINT('Ctrl Pts',(1.44000512699994,2.2,3.72840809899999));
#336539=CARTESIAN_POINT('Ctrl Pts',(1.43992250199994,12.2,3.72821669299999));
#336540=CARTESIAN_POINT('Ctrl Pts',(1.43992250199994,5.2,3.72821669299999));
#336541=CARTESIAN_POINT('Ctrl Pts',(1.43992250199994,2.2,3.72821669299999));
#336542=CARTESIAN_POINT('Ctrl Pts',(1.43984290599994,12.2,3.72803162199999));
#336543=CARTESIAN_POINT('Ctrl Pts',(1.43984290599994,5.2,3.72803162199999));
#336544=CARTESIAN_POINT('Ctrl Pts',(1.43984290599994,2.2,3.72803162199999));
#336545=CARTESIAN_POINT('Ctrl Pts',(1.43976632799994,12.2,3.72785290999998));
#336546=CARTESIAN_POINT('Ctrl Pts',(1.43976632799994,5.2,3.72785290999998));
#336547=CARTESIAN_POINT('Ctrl Pts',(1.43976632799994,2.2,3.72785290999998));
#336548=CARTESIAN_POINT('Ctrl Pts',(1.43969275699994,12.2,3.72768057899999));
#336549=CARTESIAN_POINT('Ctrl Pts',(1.43969275699994,5.2,3.72768057899999));
#336550=CARTESIAN_POINT('Ctrl Pts',(1.43969275699994,2.2,3.72768057899999));
#336551=CARTESIAN_POINT('Ctrl Pts',(1.43962218299994,12.2,3.72751464899999));
#336552=CARTESIAN_POINT('Ctrl Pts',(1.43962218299994,5.2,3.72751464899999));
#336553=CARTESIAN_POINT('Ctrl Pts',(1.43962218299994,2.2,3.72751464899999));
#336554=CARTESIAN_POINT('Ctrl Pts',(1.43955459499994,12.2,3.72735514399999));
#336555=CARTESIAN_POINT('Ctrl Pts',(1.43955459499994,5.2,3.72735514399999));
#336556=CARTESIAN_POINT('Ctrl Pts',(1.43955459499994,2.2,3.72735514399999));
#336557=CARTESIAN_POINT('Ctrl Pts',(1.43948998199994,12.2,3.72720208399999));
#336558=CARTESIAN_POINT('Ctrl Pts',(1.43948998199994,5.2,3.72720208399999));
#336559=CARTESIAN_POINT('Ctrl Pts',(1.43948998199994,2.2,3.72720208399999));
#336560=CARTESIAN_POINT('Ctrl Pts',(1.43942833299994,12.2,3.72705549099998));
#336561=CARTESIAN_POINT('Ctrl Pts',(1.43942833299994,5.2,3.72705549099998));
#336562=CARTESIAN_POINT('Ctrl Pts',(1.43942833299994,2.2,3.72705549099998));
#336563=CARTESIAN_POINT('Ctrl Pts',(1.43936963499994,12.2,3.72691538999998));
#336564=CARTESIAN_POINT('Ctrl Pts',(1.43936963499994,5.2,3.72691538999998));
#336565=CARTESIAN_POINT('Ctrl Pts',(1.43936963499994,2.2,3.72691538999998));
#336566=CARTESIAN_POINT('Ctrl Pts',(1.43931387899994,12.2,3.72678180299998));
#336567=CARTESIAN_POINT('Ctrl Pts',(1.43931387899994,5.2,3.72678180299998));
#336568=CARTESIAN_POINT('Ctrl Pts',(1.43931387899994,2.2,3.72678180299998));
#336569=CARTESIAN_POINT('Ctrl Pts',(1.43926105099994,12.2,3.72665475399998));
#336570=CARTESIAN_POINT('Ctrl Pts',(1.43926105099994,5.2,3.72665475399998));
#336571=CARTESIAN_POINT('Ctrl Pts',(1.43926105099994,2.2,3.72665475399998));
#336572=CARTESIAN_POINT('Ctrl Pts',(1.43921114099994,12.2,3.72653426499999));
#336573=CARTESIAN_POINT('Ctrl Pts',(1.43921114099994,5.2,3.72653426499999));
#336574=CARTESIAN_POINT('Ctrl Pts',(1.43921114099994,2.2,3.72653426499999));
#336575=CARTESIAN_POINT('Ctrl Pts',(1.43916413499994,12.2,3.72642036099998));
#336576=CARTESIAN_POINT('Ctrl Pts',(1.43916413499994,5.2,3.72642036099998));
#336577=CARTESIAN_POINT('Ctrl Pts',(1.43916413499994,2.2,3.72642036099998));
#336578=CARTESIAN_POINT('Ctrl Pts',(1.43912002499994,12.2,3.72631305999998));
#336579=CARTESIAN_POINT('Ctrl Pts',(1.43912002499994,5.2,3.72631305999998));
#336580=CARTESIAN_POINT('Ctrl Pts',(1.43912002499994,2.2,3.72631305999998));
#336581=CARTESIAN_POINT('Ctrl Pts',(1.43907880099994,12.2,3.72621238199999));
#336582=CARTESIAN_POINT('Ctrl Pts',(1.43907880099994,5.2,3.72621238199999));
#336583=CARTESIAN_POINT('Ctrl Pts',(1.43907880099994,2.2,3.72621238199999));
#336584=CARTESIAN_POINT('Ctrl Pts',(1.43904044999994,12.2,3.72611834999999));
#336585=CARTESIAN_POINT('Ctrl Pts',(1.43904044999994,5.2,3.72611834999999));
#336586=CARTESIAN_POINT('Ctrl Pts',(1.43904044999994,2.2,3.72611834999999));
#336587=CARTESIAN_POINT('Ctrl Pts',(1.43900496299994,12.2,3.72603098699999));
#336588=CARTESIAN_POINT('Ctrl Pts',(1.43900496299994,5.2,3.72603098699999));
#336589=CARTESIAN_POINT('Ctrl Pts',(1.43900496299994,2.2,3.72603098699999));
#336590=CARTESIAN_POINT('Ctrl Pts',(1.43897232399994,12.2,3.72595031699999));
#336591=CARTESIAN_POINT('Ctrl Pts',(1.43897232399994,5.2,3.72595031699999));
#336592=CARTESIAN_POINT('Ctrl Pts',(1.43897232399994,2.2,3.72595031699999));
#336593=CARTESIAN_POINT('Ctrl Pts',(1.43894251899994,12.2,3.72587637199998));
#336594=CARTESIAN_POINT('Ctrl Pts',(1.43894251899994,5.2,3.72587637199998));
#336595=CARTESIAN_POINT('Ctrl Pts',(1.43894251899994,2.2,3.72587637199998));
#336596=CARTESIAN_POINT('Ctrl Pts',(1.43891553299994,12.2,3.72580917999999));
#336597=CARTESIAN_POINT('Ctrl Pts',(1.43891553299994,5.2,3.72580917999999));
#336598=CARTESIAN_POINT('Ctrl Pts',(1.43891553299994,2.2,3.72580917999999));
#336599=CARTESIAN_POINT('Ctrl Pts',(1.43889135199994,12.2,3.72574876699999));
#336600=CARTESIAN_POINT('Ctrl Pts',(1.43889135199994,5.2,3.72574876699999));
#336601=CARTESIAN_POINT('Ctrl Pts',(1.43889135199994,2.2,3.72574876699999));
#336602=CARTESIAN_POINT('Ctrl Pts',(1.43886996799994,12.2,3.72569515099999));
#336603=CARTESIAN_POINT('Ctrl Pts',(1.43886996799994,5.2,3.72569515099999));
#336604=CARTESIAN_POINT('Ctrl Pts',(1.43886996799994,2.2,3.72569515099999));
#336605=CARTESIAN_POINT('Ctrl Pts',(1.43884938350029,12.2,3.72564333328053));
#336606=CARTESIAN_POINT('Ctrl Pts',(1.43884938350029,5.2,3.72564333328053));
#336607=CARTESIAN_POINT('Ctrl Pts',(1.43884938350029,2.2,3.72564333328053));
#336608=CARTESIAN_POINT('Ctrl Pts',(1.43883538351011,12.2,3.72560788388561));
#336609=CARTESIAN_POINT('Ctrl Pts',(1.43883538351011,5.2,3.72560788388561));
#336610=CARTESIAN_POINT('Ctrl Pts',(1.43883538351011,2.2,3.72560788388561));
#336611=CARTESIAN_POINT('Ctrl Pts',(1.43882621103565,12.2,3.72558451224687));
#336612=CARTESIAN_POINT('Ctrl Pts',(1.43882621103565,5.2,3.72558451224687));
#336613=CARTESIAN_POINT('Ctrl Pts',(1.43882621103565,2.2,3.72558451224687));
#336614=CARTESIAN_POINT('Ctrl Pts',(1.43882053151532,12.2,3.72556994107896));
#336615=CARTESIAN_POINT('Ctrl Pts',(1.43882053151532,5.2,3.72556994107896));
#336616=CARTESIAN_POINT('Ctrl Pts',(1.43882053151532,2.2,3.72556994107896));
#336617=CARTESIAN_POINT('Ctrl Pts',(1.43881701799994,12.2,3.72556094399998));
#336618=CARTESIAN_POINT('Ctrl Pts',(1.43881701799994,5.2,3.72556094399998));
#336619=CARTESIAN_POINT('Ctrl Pts',(1.43881701799994,2.2,3.72556094399998));
#336620=CARTESIAN_POINT('',(2.02484994999994,12.2,4.29679911999998));
#336621=CARTESIAN_POINT('Origin',(-5.66300478732629E-14,15.2,-1.77635683940025E-14));
#336622=CARTESIAN_POINT('',(2.32438124199994,12.2,4.14243308299999));
#336623=CARTESIAN_POINT('Ctrl Pts',(2.19921389299994,12.2,3.33366470799999));
#336624=CARTESIAN_POINT('Ctrl Pts',(2.19921389299994,5.2,3.33366470799999));
#336625=CARTESIAN_POINT('Ctrl Pts',(2.19921389299994,2.2,3.33366470799999));
#336626=CARTESIAN_POINT('Ctrl Pts',(2.19921763978639,12.2,3.33367043367347));
#336627=CARTESIAN_POINT('Ctrl Pts',(2.19921763978639,5.2,3.33367043367347));
#336628=CARTESIAN_POINT('Ctrl Pts',(2.19921763978639,2.2,3.33367043367347));
#336629=CARTESIAN_POINT('Ctrl Pts',(2.19922488336832,12.2,3.3336815089074));
#336630=CARTESIAN_POINT('Ctrl Pts',(2.19922488336832,5.2,3.3336815089074));
#336631=CARTESIAN_POINT('Ctrl Pts',(2.19922488336832,2.2,3.3336815089074));
#336632=CARTESIAN_POINT('Ctrl Pts',(2.19923563657748,12.2,3.33369793329671));
#336633=CARTESIAN_POINT('Ctrl Pts',(2.19923563657748,5.19999999999999,3.33369793329671));
#336634=CARTESIAN_POINT('Ctrl Pts',(2.19923563657748,2.2,3.33369793329671));
#336635=CARTESIAN_POINT('Ctrl Pts',(2.19924982935574,12.2,3.3337196857409));
#336636=CARTESIAN_POINT('Ctrl Pts',(2.19924982935574,5.19999999999999,3.3337196857409));
#336637=CARTESIAN_POINT('Ctrl Pts',(2.19924982935574,2.2,3.3337196857409));
#336638=CARTESIAN_POINT('Ctrl Pts',(2.19927450199994,12.2,3.33375771899998));
#336639=CARTESIAN_POINT('Ctrl Pts',(2.19927450199994,5.2,3.33375771899998));
#336640=CARTESIAN_POINT('Ctrl Pts',(2.19927450199994,2.2,3.33375771899998));
#336641=CARTESIAN_POINT('Ctrl Pts',(2.19930183199994,12.2,3.33380002299998));
#336642=CARTESIAN_POINT('Ctrl Pts',(2.19930183199994,5.2,3.33380002299998));
#336643=CARTESIAN_POINT('Ctrl Pts',(2.19930183199994,2.2,3.33380002299998));
#336644=CARTESIAN_POINT('Ctrl Pts',(2.19933308799994,12.2,3.33384855099998));
#336645=CARTESIAN_POINT('Ctrl Pts',(2.19933308799994,5.2,3.33384855099998));
#336646=CARTESIAN_POINT('Ctrl Pts',(2.19933308799994,2.2,3.33384855099998));
#336647=CARTESIAN_POINT('Ctrl Pts',(2.19936825899994,12.2,3.33390330099999));
#336648=CARTESIAN_POINT('Ctrl Pts',(2.19936825899994,5.2,3.33390330099999));
#336649=CARTESIAN_POINT('Ctrl Pts',(2.19936825899994,2.2,3.33390330099999));
#336650=CARTESIAN_POINT('Ctrl Pts',(2.19940732099994,12.2,3.33396426999998));
#336651=CARTESIAN_POINT('Ctrl Pts',(2.19940732099994,5.2,3.33396426999998));
#336652=CARTESIAN_POINT('Ctrl Pts',(2.19940732099994,2.2,3.33396426999998));
#336653=CARTESIAN_POINT('Ctrl Pts',(2.19945024699994,12.2,3.33403145199998));
#336654=CARTESIAN_POINT('Ctrl Pts',(2.19945024699994,5.2,3.33403145199998));
#336655=CARTESIAN_POINT('Ctrl Pts',(2.19945024699994,2.2,3.33403145199998));
#336656=CARTESIAN_POINT('Ctrl Pts',(2.19949700499994,12.2,3.33410484499999));
#336657=CARTESIAN_POINT('Ctrl Pts',(2.19949700499994,5.2,3.33410484499999));
#336658=CARTESIAN_POINT('Ctrl Pts',(2.19949700499994,2.2,3.33410484499999));
#336659=CARTESIAN_POINT('Ctrl Pts',(2.19954756299995,12.2,3.33418444299999));
#336660=CARTESIAN_POINT('Ctrl Pts',(2.19954756299995,5.2,3.33418444299999));
#336661=CARTESIAN_POINT('Ctrl Pts',(2.19954756299995,2.2,3.33418444299999));
#336662=CARTESIAN_POINT('Ctrl Pts',(2.19960188999994,12.2,3.33427024099999));
#336663=CARTESIAN_POINT('Ctrl Pts',(2.19960188999994,5.2,3.33427024099999));
#336664=CARTESIAN_POINT('Ctrl Pts',(2.19960188999994,2.2,3.33427024099999));
#336665=CARTESIAN_POINT('Ctrl Pts',(2.19965995999994,12.2,3.33436223599998));
#336666=CARTESIAN_POINT('Ctrl Pts',(2.19965995999994,5.2,3.33436223599998));
#336667=CARTESIAN_POINT('Ctrl Pts',(2.19965995999994,2.2,3.33436223599998));
#336668=CARTESIAN_POINT('Ctrl Pts',(2.19972175099994,12.2,3.33446042499999));
#336669=CARTESIAN_POINT('Ctrl Pts',(2.19972175099994,5.2,3.33446042499999));
#336670=CARTESIAN_POINT('Ctrl Pts',(2.19972175099994,2.2,3.33446042499999));
#336671=CARTESIAN_POINT('Ctrl Pts',(2.19978724099994,12.2,3.33456480399998));
#336672=CARTESIAN_POINT('Ctrl Pts',(2.19978724099994,5.2,3.33456480399998));
#336673=CARTESIAN_POINT('Ctrl Pts',(2.19978724099994,2.2,3.33456480399998));
#336674=CARTESIAN_POINT('Ctrl Pts',(2.19985640599994,12.2,3.33467536999999));
#336675=CARTESIAN_POINT('Ctrl Pts',(2.19985640599994,5.2,3.33467536999999));
#336676=CARTESIAN_POINT('Ctrl Pts',(2.19985640599994,2.2,3.33467536999999));
#336677=CARTESIAN_POINT('Ctrl Pts',(2.19992921999994,12.2,3.33479211899999));
#336678=CARTESIAN_POINT('Ctrl Pts',(2.19992921999994,5.2,3.33479211899999));
#336679=CARTESIAN_POINT('Ctrl Pts',(2.19992921999994,2.2,3.33479211899999));
#336680=CARTESIAN_POINT('Ctrl Pts',(2.20000566099994,12.2,3.33491504499998));
#336681=CARTESIAN_POINT('Ctrl Pts',(2.20000566099994,5.2,3.33491504499998));
#336682=CARTESIAN_POINT('Ctrl Pts',(2.20000566099994,2.2,3.33491504499998));
#336683=CARTESIAN_POINT('Ctrl Pts',(2.20008569999994,12.2,3.33504414799998));
#336684=CARTESIAN_POINT('Ctrl Pts',(2.20008569999994,5.2,3.33504414799998));
#336685=CARTESIAN_POINT('Ctrl Pts',(2.20008569999994,2.2,3.33504414799998));
#336686=CARTESIAN_POINT('Ctrl Pts',(2.20016931299994,12.2,3.33517942099999));
#336687=CARTESIAN_POINT('Ctrl Pts',(2.20016931299994,5.2,3.33517942099999));
#336688=CARTESIAN_POINT('Ctrl Pts',(2.20016931299994,2.2,3.33517942099999));
#336689=CARTESIAN_POINT('Ctrl Pts',(2.20025647299994,12.2,3.33532086199998));
#336690=CARTESIAN_POINT('Ctrl Pts',(2.20025647299994,5.2,3.33532086199998));
#336691=CARTESIAN_POINT('Ctrl Pts',(2.20025647299994,2.2,3.33532086199998));
#336692=CARTESIAN_POINT('Ctrl Pts',(2.20034715699994,12.2,3.33546846599998));
#336693=CARTESIAN_POINT('Ctrl Pts',(2.20034715699994,5.2,3.33546846599998));
#336694=CARTESIAN_POINT('Ctrl Pts',(2.20034715699994,2.2,3.33546846599998));
#336695=CARTESIAN_POINT('Ctrl Pts',(2.20044133899994,12.2,3.33562222799999));
#336696=CARTESIAN_POINT('Ctrl Pts',(2.20044133899994,5.2,3.33562222799999));
#336697=CARTESIAN_POINT('Ctrl Pts',(2.20044133899994,2.2,3.33562222799999));
#336698=CARTESIAN_POINT('Ctrl Pts',(2.20053899599994,12.2,3.33578214599999));
#336699=CARTESIAN_POINT('Ctrl Pts',(2.20053899599994,5.2,3.33578214599999));
#336700=CARTESIAN_POINT('Ctrl Pts',(2.20053899599994,2.2,3.33578214599999));
#336701=CARTESIAN_POINT('Ctrl Pts',(2.20064010499994,12.2,3.33594821699998));
#336702=CARTESIAN_POINT('Ctrl Pts',(2.20064010499994,5.2,3.33594821699998));
#336703=CARTESIAN_POINT('Ctrl Pts',(2.20064010499994,2.2,3.33594821699998));
#336704=CARTESIAN_POINT('Ctrl Pts',(2.20074464099994,12.2,3.33612043399999));
#336705=CARTESIAN_POINT('Ctrl Pts',(2.20074464099994,5.2,3.33612043399999));
#336706=CARTESIAN_POINT('Ctrl Pts',(2.20074464099994,2.2,3.33612043399999));
#336707=CARTESIAN_POINT('Ctrl Pts',(2.20085257799994,12.2,3.33629879499998));
#336708=CARTESIAN_POINT('Ctrl Pts',(2.20085257799994,5.2,3.33629879499998));
#336709=CARTESIAN_POINT('Ctrl Pts',(2.20085257799994,2.2,3.33629879499998));
#336710=CARTESIAN_POINT('Ctrl Pts',(2.20096389399994,12.2,3.33648329599999));
#336711=CARTESIAN_POINT('Ctrl Pts',(2.20096389399994,5.2,3.33648329599999));
#336712=CARTESIAN_POINT('Ctrl Pts',(2.20096389399994,2.2,3.33648329599999));
#336713=CARTESIAN_POINT('Ctrl Pts',(2.20107856499994,12.2,3.33667393299999));
#336714=CARTESIAN_POINT('Ctrl Pts',(2.20107856499994,5.2,3.33667393299999));
#336715=CARTESIAN_POINT('Ctrl Pts',(2.20107856499994,2.2,3.33667393299999));
#336716=CARTESIAN_POINT('Ctrl Pts',(2.20119656499994,12.2,3.33687070099998));
#336717=CARTESIAN_POINT('Ctrl Pts',(2.20119656499994,5.2,3.33687070099998));
#336718=CARTESIAN_POINT('Ctrl Pts',(2.20119656499994,2.2,3.33687070099998));
#336719=CARTESIAN_POINT('Ctrl Pts',(2.20131787099994,12.2,3.33707359699999));
#336720=CARTESIAN_POINT('Ctrl Pts',(2.20131787099994,5.2,3.33707359699999));
#336721=CARTESIAN_POINT('Ctrl Pts',(2.20131787099994,2.2,3.33707359699999));
#336722=CARTESIAN_POINT('Ctrl Pts',(2.20144245999994,12.2,3.33728261799998));
#336723=CARTESIAN_POINT('Ctrl Pts',(2.20144245999994,5.2,3.33728261799998));
#336724=CARTESIAN_POINT('Ctrl Pts',(2.20144245999994,2.2,3.33728261799998));
#336725=CARTESIAN_POINT('Ctrl Pts',(2.20157030699994,12.2,3.33749775599999));
#336726=CARTESIAN_POINT('Ctrl Pts',(2.20157030699994,5.2,3.33749775599999));
#336727=CARTESIAN_POINT('Ctrl Pts',(2.20157030699994,2.2,3.33749775599999));
#336728=CARTESIAN_POINT('Ctrl Pts',(2.20170139099995,12.2,3.33771901199999));
#336729=CARTESIAN_POINT('Ctrl Pts',(2.20170139099995,5.2,3.33771901199999));
#336730=CARTESIAN_POINT('Ctrl Pts',(2.20170139099995,2.2,3.33771901199999));
#336731=CARTESIAN_POINT('Ctrl Pts',(2.20183568599994,12.2,3.33794637799999));
#336732=CARTESIAN_POINT('Ctrl Pts',(2.20183568599994,5.2,3.33794637799999));
#336733=CARTESIAN_POINT('Ctrl Pts',(2.20183568599994,2.2,3.33794637799999));
#336734=CARTESIAN_POINT('Ctrl Pts',(2.20197316999994,12.2,3.33817985299999));
#336735=CARTESIAN_POINT('Ctrl Pts',(2.20197316999994,5.2,3.33817985299999));
#336736=CARTESIAN_POINT('Ctrl Pts',(2.20197316999994,2.2,3.33817985299999));
#336737=CARTESIAN_POINT('Ctrl Pts',(2.20211381899994,12.2,3.33841942999998));
#336738=CARTESIAN_POINT('Ctrl Pts',(2.20211381899994,5.2,3.33841942999998));
#336739=CARTESIAN_POINT('Ctrl Pts',(2.20211381899994,2.2,3.33841942999998));
#336740=CARTESIAN_POINT('Ctrl Pts',(2.20225760999994,12.2,3.33866510799999));
#336741=CARTESIAN_POINT('Ctrl Pts',(2.20225760999994,5.2,3.33866510799999));
#336742=CARTESIAN_POINT('Ctrl Pts',(2.20225760999994,2.2,3.33866510799999));
#336743=CARTESIAN_POINT('Ctrl Pts',(2.20240451999994,12.2,3.33891687999999));
#336744=CARTESIAN_POINT('Ctrl Pts',(2.20240451999994,5.2,3.33891687999999));
#336745=CARTESIAN_POINT('Ctrl Pts',(2.20240451999994,2.2,3.33891687999999));
#336746=CARTESIAN_POINT('Ctrl Pts',(2.20255452499994,12.2,3.33917474399998));
#336747=CARTESIAN_POINT('Ctrl Pts',(2.20255452499994,5.2,3.33917474399998));
#336748=CARTESIAN_POINT('Ctrl Pts',(2.20255452499994,2.2,3.33917474399998));
#336749=CARTESIAN_POINT('Ctrl Pts',(2.20270760299994,12.2,3.33943869499999));
#336750=CARTESIAN_POINT('Ctrl Pts',(2.20270760299994,5.2,3.33943869499999));
#336751=CARTESIAN_POINT('Ctrl Pts',(2.20270760299994,2.2,3.33943869499999));
#336752=CARTESIAN_POINT('Ctrl Pts',(2.20286373099994,12.2,3.33970872899998));
#336753=CARTESIAN_POINT('Ctrl Pts',(2.20286373099994,5.2,3.33970872899998));
#336754=CARTESIAN_POINT('Ctrl Pts',(2.20286373099994,2.2,3.33970872899998));
#336755=CARTESIAN_POINT('Ctrl Pts',(2.20302288599994,12.2,3.33998484099999));
#336756=CARTESIAN_POINT('Ctrl Pts',(2.20302288599994,5.2,3.33998484099999));
#336757=CARTESIAN_POINT('Ctrl Pts',(2.20302288599994,2.2,3.33998484099999));
#336758=CARTESIAN_POINT('Ctrl Pts',(2.20318504499994,12.2,3.34026702899998));
#336759=CARTESIAN_POINT('Ctrl Pts',(2.20318504499994,5.2,3.34026702899998));
#336760=CARTESIAN_POINT('Ctrl Pts',(2.20318504499994,2.2,3.34026702899998));
#336761=CARTESIAN_POINT('Ctrl Pts',(2.20335018599994,12.2,3.34055528599999));
#336762=CARTESIAN_POINT('Ctrl Pts',(2.20335018599994,5.2,3.34055528599999));
#336763=CARTESIAN_POINT('Ctrl Pts',(2.20335018599994,2.2,3.34055528599999));
#336764=CARTESIAN_POINT('Ctrl Pts',(2.20351828599994,12.2,3.34084961099999));
#336765=CARTESIAN_POINT('Ctrl Pts',(2.20351828599994,5.2,3.34084961099999));
#336766=CARTESIAN_POINT('Ctrl Pts',(2.20351828599994,2.2,3.34084961099999));
#336767=CARTESIAN_POINT('Ctrl Pts',(2.20368932299994,12.2,3.34114999699998));
#336768=CARTESIAN_POINT('Ctrl Pts',(2.20368932299994,5.2,3.34114999699998));
#336769=CARTESIAN_POINT('Ctrl Pts',(2.20368932299994,2.2,3.34114999699998));
#336770=CARTESIAN_POINT('Ctrl Pts',(2.20386327299994,12.2,3.34145644199998));
#336771=CARTESIAN_POINT('Ctrl Pts',(2.20386327299994,5.2,3.34145644199998));
#336772=CARTESIAN_POINT('Ctrl Pts',(2.20386327299994,2.2,3.34145644199998));
#336773=CARTESIAN_POINT('Ctrl Pts',(2.20404011499994,12.2,3.34176893899999));
#336774=CARTESIAN_POINT('Ctrl Pts',(2.20404011499994,5.2,3.34176893899999));
#336775=CARTESIAN_POINT('Ctrl Pts',(2.20404011499994,2.2,3.34176893899999));
#336776=CARTESIAN_POINT('Ctrl Pts',(2.20421982799994,12.2,3.34208748699999));
#336777=CARTESIAN_POINT('Ctrl Pts',(2.20421982799994,5.2,3.34208748699999));
#336778=CARTESIAN_POINT('Ctrl Pts',(2.20421982799994,2.2,3.34208748699999));
#336779=CARTESIAN_POINT('Ctrl Pts',(2.20440238699994,12.2,3.34241207999998));
#336780=CARTESIAN_POINT('Ctrl Pts',(2.20440238699994,5.2,3.34241207999998));
#336781=CARTESIAN_POINT('Ctrl Pts',(2.20440238699994,2.2,3.34241207999998));
#336782=CARTESIAN_POINT('Ctrl Pts',(2.20458777199994,12.2,3.34274271399998));
#336783=CARTESIAN_POINT('Ctrl Pts',(2.20458777199994,5.2,3.34274271399998));
#336784=CARTESIAN_POINT('Ctrl Pts',(2.20458777199994,2.2,3.34274271399998));
#336785=CARTESIAN_POINT('Ctrl Pts',(2.20477595999994,12.2,3.34307938399999));
#336786=CARTESIAN_POINT('Ctrl Pts',(2.20477595999994,5.2,3.34307938399999));
#336787=CARTESIAN_POINT('Ctrl Pts',(2.20477595999994,2.2,3.34307938399999));
#336788=CARTESIAN_POINT('Ctrl Pts',(2.20496692899994,12.2,3.34342208699999));
#336789=CARTESIAN_POINT('Ctrl Pts',(2.20496692899994,5.2,3.34342208699999));
#336790=CARTESIAN_POINT('Ctrl Pts',(2.20496692899994,2.2,3.34342208699999));
#336791=CARTESIAN_POINT('Ctrl Pts',(2.20516065799994,12.2,3.34377081999998));
#336792=CARTESIAN_POINT('Ctrl Pts',(2.20516065799994,5.2,3.34377081999998));
#336793=CARTESIAN_POINT('Ctrl Pts',(2.20516065799994,2.2,3.34377081999998));
#336794=CARTESIAN_POINT('Ctrl Pts',(2.20535712399994,12.2,3.34412557399999));
#336795=CARTESIAN_POINT('Ctrl Pts',(2.20535712399994,5.2,3.34412557399999));
#336796=CARTESIAN_POINT('Ctrl Pts',(2.20535712399994,2.2,3.34412557399999));
#336797=CARTESIAN_POINT('Ctrl Pts',(2.20555630599994,12.2,3.34448634899999));
#336798=CARTESIAN_POINT('Ctrl Pts',(2.20555630599994,5.2,3.34448634899999));
#336799=CARTESIAN_POINT('Ctrl Pts',(2.20555630599994,2.2,3.34448634899999));
#336800=CARTESIAN_POINT('Ctrl Pts',(2.20575818299994,12.2,3.34485313999998));
#336801=CARTESIAN_POINT('Ctrl Pts',(2.20575818299994,5.2,3.34485313999998));
#336802=CARTESIAN_POINT('Ctrl Pts',(2.20575818299994,2.2,3.34485313999998));
#336803=CARTESIAN_POINT('Ctrl Pts',(2.20596273199994,12.2,3.34522594199999));
#336804=CARTESIAN_POINT('Ctrl Pts',(2.20596273199994,5.2,3.34522594199999));
#336805=CARTESIAN_POINT('Ctrl Pts',(2.20596273199994,2.2,3.34522594199999));
#336806=CARTESIAN_POINT('Ctrl Pts',(2.20616993299994,12.2,3.34560474899998));
#336807=CARTESIAN_POINT('Ctrl Pts',(2.20616993299994,5.2,3.34560474899998));
#336808=CARTESIAN_POINT('Ctrl Pts',(2.20616993299994,2.2,3.34560474899998));
#336809=CARTESIAN_POINT('Ctrl Pts',(2.20637976299995,12.2,3.34598955999999));
#336810=CARTESIAN_POINT('Ctrl Pts',(2.20637976299995,5.2,3.34598955999999));
#336811=CARTESIAN_POINT('Ctrl Pts',(2.20637976299995,2.2,3.34598955999999));
#336812=CARTESIAN_POINT('Ctrl Pts',(2.20659220199994,12.2,3.34638036899998));
#336813=CARTESIAN_POINT('Ctrl Pts',(2.20659220199994,5.2,3.34638036899998));
#336814=CARTESIAN_POINT('Ctrl Pts',(2.20659220199994,2.2,3.34638036899998));
#336815=CARTESIAN_POINT('Ctrl Pts',(2.20680722799994,12.2,3.34677717099999));
#336816=CARTESIAN_POINT('Ctrl Pts',(2.20680722799994,5.2,3.34677717099999));
#336817=CARTESIAN_POINT('Ctrl Pts',(2.20680722799994,2.2,3.34677717099999));
#336818=CARTESIAN_POINT('Ctrl Pts',(2.20702481999994,12.2,3.34717996199998));
#336819=CARTESIAN_POINT('Ctrl Pts',(2.20702481999994,5.2,3.34717996199998));
#336820=CARTESIAN_POINT('Ctrl Pts',(2.20702481999994,2.2,3.34717996199998));
#336821=CARTESIAN_POINT('Ctrl Pts',(2.20724495699994,12.2,3.34758873899998));
#336822=CARTESIAN_POINT('Ctrl Pts',(2.20724495699994,5.2,3.34758873899998));
#336823=CARTESIAN_POINT('Ctrl Pts',(2.20724495699994,2.2,3.34758873899998));
#336824=CARTESIAN_POINT('Ctrl Pts',(2.20746761799994,12.2,3.34800349499999));
#336825=CARTESIAN_POINT('Ctrl Pts',(2.20746761799994,5.2,3.34800349499999));
#336826=CARTESIAN_POINT('Ctrl Pts',(2.20746761799994,2.2,3.34800349499999));
#336827=CARTESIAN_POINT('Ctrl Pts',(2.20769278099994,12.2,3.34842422799999));
#336828=CARTESIAN_POINT('Ctrl Pts',(2.20769278099994,5.2,3.34842422799999));
#336829=CARTESIAN_POINT('Ctrl Pts',(2.20769278099994,2.2,3.34842422799999));
#336830=CARTESIAN_POINT('Ctrl Pts',(2.20792042699994,12.2,3.34885093299999));
#336831=CARTESIAN_POINT('Ctrl Pts',(2.20792042699994,5.2,3.34885093299999));
#336832=CARTESIAN_POINT('Ctrl Pts',(2.20792042699994,2.2,3.34885093299999));
#336833=CARTESIAN_POINT('Ctrl Pts',(2.20815053399994,12.2,3.34928360399999));
#336834=CARTESIAN_POINT('Ctrl Pts',(2.20815053399994,5.2,3.34928360399999));
#336835=CARTESIAN_POINT('Ctrl Pts',(2.20815053399994,2.2,3.34928360399999));
#336836=CARTESIAN_POINT('Ctrl Pts',(2.20838308099994,12.2,3.34972223899998));
#336837=CARTESIAN_POINT('Ctrl Pts',(2.20838308099994,5.2,3.34972223899998));
#336838=CARTESIAN_POINT('Ctrl Pts',(2.20838308099994,2.2,3.34972223899998));
#336839=CARTESIAN_POINT('Ctrl Pts',(2.20861804799994,12.2,3.35016683099998));
#336840=CARTESIAN_POINT('Ctrl Pts',(2.20861804799994,5.2,3.35016683099998));
#336841=CARTESIAN_POINT('Ctrl Pts',(2.20861804799994,2.2,3.35016683099998));
#336842=CARTESIAN_POINT('Ctrl Pts',(2.20885541299995,12.2,3.35061737799998));
#336843=CARTESIAN_POINT('Ctrl Pts',(2.20885541299995,5.2,3.35061737799998));
#336844=CARTESIAN_POINT('Ctrl Pts',(2.20885541299995,2.2,3.35061737799998));
#336845=CARTESIAN_POINT('Ctrl Pts',(2.20909515699994,12.2,3.35107387499999));
#336846=CARTESIAN_POINT('Ctrl Pts',(2.20909515699994,5.2,3.35107387499999));
#336847=CARTESIAN_POINT('Ctrl Pts',(2.20909515699994,2.2,3.35107387499999));
#336848=CARTESIAN_POINT('Ctrl Pts',(2.20933725999994,12.2,3.35153631599999));
#336849=CARTESIAN_POINT('Ctrl Pts',(2.20933725999994,5.2,3.35153631599999));
#336850=CARTESIAN_POINT('Ctrl Pts',(2.20933725999994,2.2,3.35153631599999));
#336851=CARTESIAN_POINT('Ctrl Pts',(2.20958169899994,12.2,3.35200469699998));
#336852=CARTESIAN_POINT('Ctrl Pts',(2.20958169899994,5.2,3.35200469699998));
#336853=CARTESIAN_POINT('Ctrl Pts',(2.20958169899994,2.2,3.35200469699998));
#336854=CARTESIAN_POINT('Ctrl Pts',(2.20982845599994,12.2,3.35247901499999));
#336855=CARTESIAN_POINT('Ctrl Pts',(2.20982845599994,5.2,3.35247901499999));
#336856=CARTESIAN_POINT('Ctrl Pts',(2.20982845599994,2.2,3.35247901499999));
#336857=CARTESIAN_POINT('Ctrl Pts',(2.21007750999994,12.2,3.35295926399999));
#336858=CARTESIAN_POINT('Ctrl Pts',(2.21007750999994,5.2,3.35295926399999));
#336859=CARTESIAN_POINT('Ctrl Pts',(2.21007750999994,2.2,3.35295926399999));
#336860=CARTESIAN_POINT('Ctrl Pts',(2.21032883999994,12.2,3.35344543999998));
#336861=CARTESIAN_POINT('Ctrl Pts',(2.21032883999994,5.2,3.35344543999998));
#336862=CARTESIAN_POINT('Ctrl Pts',(2.21032883999994,2.2,3.35344543999998));
#336863=CARTESIAN_POINT('Ctrl Pts',(2.21058242699994,12.2,3.35393753899999));
#336864=CARTESIAN_POINT('Ctrl Pts',(2.21058242699994,5.2,3.35393753899999));
#336865=CARTESIAN_POINT('Ctrl Pts',(2.21058242699994,2.2,3.35393753899999));
#336866=CARTESIAN_POINT('Ctrl Pts',(2.21083824999994,12.2,3.35443555499998));
#336867=CARTESIAN_POINT('Ctrl Pts',(2.21083824999994,5.2,3.35443555499998));
#336868=CARTESIAN_POINT('Ctrl Pts',(2.21083824999994,2.2,3.35443555499998));
#336869=CARTESIAN_POINT('Ctrl Pts',(2.21109629099994,12.2,3.35493948499998));
#336870=CARTESIAN_POINT('Ctrl Pts',(2.21109629099994,5.2,3.35493948499998));
#336871=CARTESIAN_POINT('Ctrl Pts',(2.21109629099994,2.2,3.35493948499998));
#336872=CARTESIAN_POINT('Ctrl Pts',(2.21135652699994,12.2,3.35544932399999));
#336873=CARTESIAN_POINT('Ctrl Pts',(2.21135652699994,5.2,3.35544932399999));
#336874=CARTESIAN_POINT('Ctrl Pts',(2.21135652699994,2.2,3.35544932399999));
#336875=CARTESIAN_POINT('Ctrl Pts',(2.21161893999994,12.2,3.35596506599998));
#336876=CARTESIAN_POINT('Ctrl Pts',(2.21161893999994,5.2,3.35596506599998));
#336877=CARTESIAN_POINT('Ctrl Pts',(2.21161893999994,2.2,3.35596506599998));
#336878=CARTESIAN_POINT('Ctrl Pts',(2.21188350999994,12.2,3.35648670799999));
#336879=CARTESIAN_POINT('Ctrl Pts',(2.21188350999994,5.2,3.35648670799999));
#336880=CARTESIAN_POINT('Ctrl Pts',(2.21188350999994,2.2,3.35648670799999));
#336881=CARTESIAN_POINT('Ctrl Pts',(2.21215021599994,12.2,3.35701424599999));
#336882=CARTESIAN_POINT('Ctrl Pts',(2.21215021599994,5.2,3.35701424599999));
#336883=CARTESIAN_POINT('Ctrl Pts',(2.21215021599994,2.2,3.35701424599999));
#336884=CARTESIAN_POINT('Ctrl Pts',(2.21241903999994,12.2,3.35754767399998));
#336885=CARTESIAN_POINT('Ctrl Pts',(2.21241903999994,5.2,3.35754767399998));
#336886=CARTESIAN_POINT('Ctrl Pts',(2.21241903999994,2.2,3.35754767399998));
#336887=CARTESIAN_POINT('Ctrl Pts',(2.21268996199994,12.2,3.35808698699999));
#336888=CARTESIAN_POINT('Ctrl Pts',(2.21268996199994,5.2,3.35808698699999));
#336889=CARTESIAN_POINT('Ctrl Pts',(2.21268996199994,2.2,3.35808698699999));
#336890=CARTESIAN_POINT('Ctrl Pts',(2.21296296199994,12.2,3.35863218199999));
#336891=CARTESIAN_POINT('Ctrl Pts',(2.21296296199994,5.2,3.35863218199999));
#336892=CARTESIAN_POINT('Ctrl Pts',(2.21296296199994,2.2,3.35863218199999));
#336893=CARTESIAN_POINT('Ctrl Pts',(2.21323802099994,12.2,3.35918325299998));
#336894=CARTESIAN_POINT('Ctrl Pts',(2.21323802099994,5.2,3.35918325299998));
#336895=CARTESIAN_POINT('Ctrl Pts',(2.21323802099994,2.2,3.35918325299998));
#336896=CARTESIAN_POINT('Ctrl Pts',(2.21351511799994,12.2,3.35974019599998));
#336897=CARTESIAN_POINT('Ctrl Pts',(2.21351511799994,5.2,3.35974019599998));
#336898=CARTESIAN_POINT('Ctrl Pts',(2.21351511799994,2.2,3.35974019599998));
#336899=CARTESIAN_POINT('Ctrl Pts',(2.21379423599994,12.2,3.36030300699999));
#336900=CARTESIAN_POINT('Ctrl Pts',(2.21379423599994,5.2,3.36030300699999));
#336901=CARTESIAN_POINT('Ctrl Pts',(2.21379423599994,2.2,3.36030300699999));
#336902=CARTESIAN_POINT('Ctrl Pts',(2.21407535399994,12.2,3.36087167999998));
#336903=CARTESIAN_POINT('Ctrl Pts',(2.21407535399994,5.2,3.36087167999998));
#336904=CARTESIAN_POINT('Ctrl Pts',(2.21407535399994,2.2,3.36087167999998));
#336905=CARTESIAN_POINT('Ctrl Pts',(2.21435845399994,12.2,3.36144621199999));
#336906=CARTESIAN_POINT('Ctrl Pts',(2.21435845399994,5.2,3.36144621199999));
#336907=CARTESIAN_POINT('Ctrl Pts',(2.21435845399994,2.2,3.36144621199999));
#336908=CARTESIAN_POINT('Ctrl Pts',(2.21464351599994,12.2,3.36202659699998));
#336909=CARTESIAN_POINT('Ctrl Pts',(2.21464351599994,5.2,3.36202659699998));
#336910=CARTESIAN_POINT('Ctrl Pts',(2.21464351599994,2.2,3.36202659699998));
#336911=CARTESIAN_POINT('Ctrl Pts',(2.21493052099994,12.2,3.36261282999998));
#336912=CARTESIAN_POINT('Ctrl Pts',(2.21493052099994,5.2,3.36261282999998));
#336913=CARTESIAN_POINT('Ctrl Pts',(2.21493052099994,2.2,3.36261282999998));
#336914=CARTESIAN_POINT('Ctrl Pts',(2.21521944899994,12.2,3.36320490799999));
#336915=CARTESIAN_POINT('Ctrl Pts',(2.21521944899994,5.2,3.36320490799999));
#336916=CARTESIAN_POINT('Ctrl Pts',(2.21521944899994,2.2,3.36320490799999));
#336917=CARTESIAN_POINT('Ctrl Pts',(2.21551028299994,12.2,3.36380282399999));
#336918=CARTESIAN_POINT('Ctrl Pts',(2.21551028299994,5.2,3.36380282399999));
#336919=CARTESIAN_POINT('Ctrl Pts',(2.21551028299994,2.2,3.36380282399999));
#336920=CARTESIAN_POINT('Ctrl Pts',(2.21580300199994,12.2,3.36440657499999));
#336921=CARTESIAN_POINT('Ctrl Pts',(2.21580300199994,5.2,3.36440657499999));
#336922=CARTESIAN_POINT('Ctrl Pts',(2.21580300199994,2.2,3.36440657499999));
#336923=CARTESIAN_POINT('Ctrl Pts',(2.21609758899994,12.2,3.36501615599998));
#336924=CARTESIAN_POINT('Ctrl Pts',(2.21609758899994,5.2,3.36501615599998));
#336925=CARTESIAN_POINT('Ctrl Pts',(2.21609758899994,2.2,3.36501615599998));
#336926=CARTESIAN_POINT('Ctrl Pts',(2.21639402399994,12.2,3.36563156199999));
#336927=CARTESIAN_POINT('Ctrl Pts',(2.21639402399994,5.2,3.36563156199999));
#336928=CARTESIAN_POINT('Ctrl Pts',(2.21639402399994,2.2,3.36563156199999));
#336929=CARTESIAN_POINT('Ctrl Pts',(2.21669228799994,12.2,3.36625278899999));
#336930=CARTESIAN_POINT('Ctrl Pts',(2.21669228799994,5.2,3.36625278899999));
#336931=CARTESIAN_POINT('Ctrl Pts',(2.21669228799994,2.2,3.36625278899999));
#336932=CARTESIAN_POINT('Ctrl Pts',(2.21699236399994,12.2,3.36687983099999));
#336933=CARTESIAN_POINT('Ctrl Pts',(2.21699236399994,5.2,3.36687983099999));
#336934=CARTESIAN_POINT('Ctrl Pts',(2.21699236399994,2.2,3.36687983099999));
#336935=CARTESIAN_POINT('Ctrl Pts',(2.21729423199994,12.2,3.36751268399999));
#336936=CARTESIAN_POINT('Ctrl Pts',(2.21729423199994,5.2,3.36751268399999));
#336937=CARTESIAN_POINT('Ctrl Pts',(2.21729423199994,2.2,3.36751268399999));
#336938=CARTESIAN_POINT('Ctrl Pts',(2.21759787299994,12.2,3.36815134299999));
#336939=CARTESIAN_POINT('Ctrl Pts',(2.21759787299994,5.2,3.36815134299999));
#336940=CARTESIAN_POINT('Ctrl Pts',(2.21759787299994,2.2,3.36815134299999));
#336941=CARTESIAN_POINT('Ctrl Pts',(2.21790326999994,12.2,3.36879580399999));
#336942=CARTESIAN_POINT('Ctrl Pts',(2.21790326999994,5.2,3.36879580399999));
#336943=CARTESIAN_POINT('Ctrl Pts',(2.21790326999994,2.2,3.36879580399999));
#336944=CARTESIAN_POINT('Ctrl Pts',(2.21821040299994,12.2,3.36944606099999));
#336945=CARTESIAN_POINT('Ctrl Pts',(2.21821040299994,5.2,3.36944606099999));
#336946=CARTESIAN_POINT('Ctrl Pts',(2.21821040299994,2.2,3.36944606099999));
#336947=CARTESIAN_POINT('Ctrl Pts',(2.21851925399994,12.2,3.37010210999999));
#336948=CARTESIAN_POINT('Ctrl Pts',(2.21851925399994,5.2,3.37010210999999));
#336949=CARTESIAN_POINT('Ctrl Pts',(2.21851925399994,2.2,3.37010210999999));
#336950=CARTESIAN_POINT('Ctrl Pts',(2.21882980499994,12.2,3.37076394599999));
#336951=CARTESIAN_POINT('Ctrl Pts',(2.21882980499994,5.2,3.37076394599999));
#336952=CARTESIAN_POINT('Ctrl Pts',(2.21882980499994,2.2,3.37076394599999));
#336953=CARTESIAN_POINT('Ctrl Pts',(2.21914203899995,12.2,3.37143156299998));
#336954=CARTESIAN_POINT('Ctrl Pts',(2.21914203899995,5.2,3.37143156299998));
#336955=CARTESIAN_POINT('Ctrl Pts',(2.21914203899995,2.2,3.37143156299998));
#336956=CARTESIAN_POINT('Ctrl Pts',(2.21945593499994,12.2,3.37210495899999));
#336957=CARTESIAN_POINT('Ctrl Pts',(2.21945593499994,5.2,3.37210495899999));
#336958=CARTESIAN_POINT('Ctrl Pts',(2.21945593499994,2.2,3.37210495899999));
#336959=CARTESIAN_POINT('Ctrl Pts',(2.21977147599994,12.2,3.37278412699998));
#336960=CARTESIAN_POINT('Ctrl Pts',(2.21977147599994,5.2,3.37278412699998));
#336961=CARTESIAN_POINT('Ctrl Pts',(2.21977147599994,2.2,3.37278412699998));
#336962=CARTESIAN_POINT('Ctrl Pts',(2.22008864599994,12.2,3.37346906199999));
#336963=CARTESIAN_POINT('Ctrl Pts',(2.22008864599994,5.2,3.37346906199999));
#336964=CARTESIAN_POINT('Ctrl Pts',(2.22008864599994,2.2,3.37346906199999));
#336965=CARTESIAN_POINT('Ctrl Pts',(2.22040742299995,12.2,3.37415976099999));
#336966=CARTESIAN_POINT('Ctrl Pts',(2.22040742299995,5.2,3.37415976099999));
#336967=CARTESIAN_POINT('Ctrl Pts',(2.22040742299995,2.2,3.37415976099999));
#336968=CARTESIAN_POINT('Ctrl Pts',(2.22072779299994,12.2,3.37485621799999));
#336969=CARTESIAN_POINT('Ctrl Pts',(2.22072779299994,5.2,3.37485621799999));
#336970=CARTESIAN_POINT('Ctrl Pts',(2.22072779299994,2.2,3.37485621799999));
#336971=CARTESIAN_POINT('Ctrl Pts',(2.22104973399994,12.2,3.37555842699999));
#336972=CARTESIAN_POINT('Ctrl Pts',(2.22104973399994,5.2,3.37555842699999));
#336973=CARTESIAN_POINT('Ctrl Pts',(2.22104973399994,2.2,3.37555842699999));
#336974=CARTESIAN_POINT('Ctrl Pts',(2.22137323299994,12.2,3.37626638599998));
#336975=CARTESIAN_POINT('Ctrl Pts',(2.22137323299994,5.2,3.37626638599998));
#336976=CARTESIAN_POINT('Ctrl Pts',(2.22137323299994,2.2,3.37626638599998));
#336977=CARTESIAN_POINT('Ctrl Pts',(2.22169826699994,12.2,3.37698008699999));
#336978=CARTESIAN_POINT('Ctrl Pts',(2.22169826699994,5.2,3.37698008699999));
#336979=CARTESIAN_POINT('Ctrl Pts',(2.22169826699994,2.2,3.37698008699999));
#336980=CARTESIAN_POINT('Ctrl Pts',(2.22202482099994,12.2,3.37769952699999));
#336981=CARTESIAN_POINT('Ctrl Pts',(2.22202482099994,5.2,3.37769952699999));
#336982=CARTESIAN_POINT('Ctrl Pts',(2.22202482099994,2.2,3.37769952699999));
#336983=CARTESIAN_POINT('Ctrl Pts',(2.22235287899994,12.2,3.37842469999998));
#336984=CARTESIAN_POINT('Ctrl Pts',(2.22235287899994,5.2,3.37842469999998));
#336985=CARTESIAN_POINT('Ctrl Pts',(2.22235287899994,2.2,3.37842469999998));
#336986=CARTESIAN_POINT('Ctrl Pts',(2.22268241899994,12.2,3.37915560199999));
#336987=CARTESIAN_POINT('Ctrl Pts',(2.22268241899994,5.2,3.37915560199999));
#336988=CARTESIAN_POINT('Ctrl Pts',(2.22268241899994,2.2,3.37915560199999));
#336989=CARTESIAN_POINT('Ctrl Pts',(2.22301342599994,12.2,3.37989222799998));
#336990=CARTESIAN_POINT('Ctrl Pts',(2.22301342599994,5.2,3.37989222799998));
#336991=CARTESIAN_POINT('Ctrl Pts',(2.22301342599994,2.2,3.37989222799998));
#336992=CARTESIAN_POINT('Ctrl Pts',(2.22334588299994,12.2,3.38063457399999));
#336993=CARTESIAN_POINT('Ctrl Pts',(2.22334588299994,5.2,3.38063457399999));
#336994=CARTESIAN_POINT('Ctrl Pts',(2.22334588299994,2.2,3.38063457399999));
#336995=CARTESIAN_POINT('Ctrl Pts',(2.22367976999994,12.2,3.38138263299999));
#336996=CARTESIAN_POINT('Ctrl Pts',(2.22367976999994,5.2,3.38138263299999));
#336997=CARTESIAN_POINT('Ctrl Pts',(2.22367976999994,2.2,3.38138263299999));
#336998=CARTESIAN_POINT('Ctrl Pts',(2.22401507299994,12.2,3.38213640099998));
#336999=CARTESIAN_POINT('Ctrl Pts',(2.22401507299994,5.2,3.38213640099998));
#337000=CARTESIAN_POINT('Ctrl Pts',(2.22401507299994,2.2,3.38213640099998));
#337001=CARTESIAN_POINT('Ctrl Pts',(2.22435177099995,12.2,3.38289587299998));
#337002=CARTESIAN_POINT('Ctrl Pts',(2.22435177099995,5.2,3.38289587299998));
#337003=CARTESIAN_POINT('Ctrl Pts',(2.22435177099995,2.2,3.38289587299998));
#337004=CARTESIAN_POINT('Ctrl Pts',(2.22468984999994,12.2,3.38366104499999));
#337005=CARTESIAN_POINT('Ctrl Pts',(2.22468984999994,5.2,3.38366104499999));
#337006=CARTESIAN_POINT('Ctrl Pts',(2.22468984999994,2.2,3.38366104499999));
#337007=CARTESIAN_POINT('Ctrl Pts',(2.22502928999994,12.2,3.38443191099999));
#337008=CARTESIAN_POINT('Ctrl Pts',(2.22502928999994,5.2,3.38443191099999));
#337009=CARTESIAN_POINT('Ctrl Pts',(2.22502928999994,2.2,3.38443191099999));
#337010=CARTESIAN_POINT('Ctrl Pts',(2.22537007499994,12.2,3.38520846499998));
#337011=CARTESIAN_POINT('Ctrl Pts',(2.22537007499994,5.2,3.38520846499998));
#337012=CARTESIAN_POINT('Ctrl Pts',(2.22537007499994,2.2,3.38520846499998));
#337013=CARTESIAN_POINT('Ctrl Pts',(2.22571218799994,12.2,3.38599070399999));
#337014=CARTESIAN_POINT('Ctrl Pts',(2.22571218799994,5.2,3.38599070399999));
#337015=CARTESIAN_POINT('Ctrl Pts',(2.22571218799994,2.2,3.38599070399999));
#337016=CARTESIAN_POINT('Ctrl Pts',(2.22605561199994,12.2,3.38677862399998));
#337017=CARTESIAN_POINT('Ctrl Pts',(2.22605561199994,5.2,3.38677862399998));
#337018=CARTESIAN_POINT('Ctrl Pts',(2.22605561199994,2.2,3.38677862399998));
#337019=CARTESIAN_POINT('Ctrl Pts',(2.22640032799994,12.2,3.38757221599998));
#337020=CARTESIAN_POINT('Ctrl Pts',(2.22640032799994,5.2,3.38757221599998));
#337021=CARTESIAN_POINT('Ctrl Pts',(2.22640032799994,2.2,3.38757221599998));
#337022=CARTESIAN_POINT('Ctrl Pts',(2.22674632099995,12.2,3.38837147799998));
#337023=CARTESIAN_POINT('Ctrl Pts',(2.22674632099995,5.2,3.38837147799998));
#337024=CARTESIAN_POINT('Ctrl Pts',(2.22674632099995,2.2,3.38837147799998));
#337025=CARTESIAN_POINT('Ctrl Pts',(2.22709357399994,12.2,3.38917640399998));
#337026=CARTESIAN_POINT('Ctrl Pts',(2.22709357399994,5.2,3.38917640399998));
#337027=CARTESIAN_POINT('Ctrl Pts',(2.22709357399994,2.2,3.38917640399998));
#337028=CARTESIAN_POINT('Ctrl Pts',(2.22744206899994,12.2,3.38998698999998));
#337029=CARTESIAN_POINT('Ctrl Pts',(2.22744206899994,5.2,3.38998698999998));
#337030=CARTESIAN_POINT('Ctrl Pts',(2.22744206899994,2.2,3.38998698999998));
#337031=CARTESIAN_POINT('Ctrl Pts',(2.22779178999994,12.2,3.39080322999998));
#337032=CARTESIAN_POINT('Ctrl Pts',(2.22779178999994,5.2,3.39080322999998));
#337033=CARTESIAN_POINT('Ctrl Pts',(2.22779178999994,2.2,3.39080322999998));
#337034=CARTESIAN_POINT('Ctrl Pts',(2.22814272099995,12.2,3.39162511899998));
#337035=CARTESIAN_POINT('Ctrl Pts',(2.22814272099995,5.2,3.39162511899998));
#337036=CARTESIAN_POINT('Ctrl Pts',(2.22814272099995,2.2,3.39162511899998));
#337037=CARTESIAN_POINT('Ctrl Pts',(2.22849484199994,12.2,3.39245265299999));
#337038=CARTESIAN_POINT('Ctrl Pts',(2.22849484199994,5.2,3.39245265299999));
#337039=CARTESIAN_POINT('Ctrl Pts',(2.22849484199994,2.2,3.39245265299999));
#337040=CARTESIAN_POINT('Ctrl Pts',(2.22884813899995,12.2,3.39328582599999));
#337041=CARTESIAN_POINT('Ctrl Pts',(2.22884813899995,5.2,3.39328582599999));
#337042=CARTESIAN_POINT('Ctrl Pts',(2.22884813899995,2.2,3.39328582599999));
#337043=CARTESIAN_POINT('Ctrl Pts',(2.22920259499995,12.2,3.39412463199999));
#337044=CARTESIAN_POINT('Ctrl Pts',(2.22920259499995,5.2,3.39412463199999));
#337045=CARTESIAN_POINT('Ctrl Pts',(2.22920259499995,2.2,3.39412463199999));
#337046=CARTESIAN_POINT('Ctrl Pts',(2.22955819299994,12.2,3.39496906799998));
#337047=CARTESIAN_POINT('Ctrl Pts',(2.22955819299994,5.2,3.39496906799998));
#337048=CARTESIAN_POINT('Ctrl Pts',(2.22955819299994,2.2,3.39496906799998));
#337049=CARTESIAN_POINT('Ctrl Pts',(2.22991491599994,12.2,3.39581912699998));
#337050=CARTESIAN_POINT('Ctrl Pts',(2.22991491599994,5.2,3.39581912699998));
#337051=CARTESIAN_POINT('Ctrl Pts',(2.22991491599994,2.2,3.39581912699998));
#337052=CARTESIAN_POINT('Ctrl Pts',(2.23027274799994,12.2,3.39667480699998));
#337053=CARTESIAN_POINT('Ctrl Pts',(2.23027274799994,5.2,3.39667480699998));
#337054=CARTESIAN_POINT('Ctrl Pts',(2.23027274799994,2.2,3.39667480699998));
#337055=CARTESIAN_POINT('Ctrl Pts',(2.23063167299994,12.2,3.39753609899999));
#337056=CARTESIAN_POINT('Ctrl Pts',(2.23063167299994,5.2,3.39753609899999));
#337057=CARTESIAN_POINT('Ctrl Pts',(2.23063167299994,2.2,3.39753609899999));
#337058=CARTESIAN_POINT('Ctrl Pts',(2.23099167299994,12.2,3.39840300099999));
#337059=CARTESIAN_POINT('Ctrl Pts',(2.23099167299994,5.2,3.39840300099999));
#337060=CARTESIAN_POINT('Ctrl Pts',(2.23099167299994,2.2,3.39840300099999));
#337061=CARTESIAN_POINT('Ctrl Pts',(2.23135273399994,12.2,3.39927550499999));
#337062=CARTESIAN_POINT('Ctrl Pts',(2.23135273399994,5.2,3.39927550499999));
#337063=CARTESIAN_POINT('Ctrl Pts',(2.23135273399994,2.2,3.39927550499999));
#337064=CARTESIAN_POINT('Ctrl Pts',(2.23171483799994,12.2,3.40015360899999));
#337065=CARTESIAN_POINT('Ctrl Pts',(2.23171483799994,5.2,3.40015360899999));
#337066=CARTESIAN_POINT('Ctrl Pts',(2.23171483799994,2.2,3.40015360899999));
#337067=CARTESIAN_POINT('Ctrl Pts',(2.23207796799994,12.2,3.40103730699998));
#337068=CARTESIAN_POINT('Ctrl Pts',(2.23207796799994,5.2,3.40103730699998));
#337069=CARTESIAN_POINT('Ctrl Pts',(2.23207796799994,2.2,3.40103730699998));
#337070=CARTESIAN_POINT('Ctrl Pts',(2.23244210999994,12.2,3.40192659199998));
#337071=CARTESIAN_POINT('Ctrl Pts',(2.23244210999994,5.2,3.40192659199998));
#337072=CARTESIAN_POINT('Ctrl Pts',(2.23244210999994,2.2,3.40192659199998));
#337073=CARTESIAN_POINT('Ctrl Pts',(2.23280724699995,12.2,3.40282145999999));
#337074=CARTESIAN_POINT('Ctrl Pts',(2.23280724699995,5.2,3.40282145999999));
#337075=CARTESIAN_POINT('Ctrl Pts',(2.23280724699995,2.2,3.40282145999999));
#337076=CARTESIAN_POINT('Ctrl Pts',(2.23317336099994,12.2,3.40372190699998));
#337077=CARTESIAN_POINT('Ctrl Pts',(2.23317336099994,5.2,3.40372190699998));
#337078=CARTESIAN_POINT('Ctrl Pts',(2.23317336099994,2.2,3.40372190699998));
#337079=CARTESIAN_POINT('Ctrl Pts',(2.23354043899994,12.2,3.40462792699999));
#337080=CARTESIAN_POINT('Ctrl Pts',(2.23354043899994,5.2,3.40462792699999));
#337081=CARTESIAN_POINT('Ctrl Pts',(2.23354043899994,2.2,3.40462792699999));
#337082=CARTESIAN_POINT('Ctrl Pts',(2.23390846199994,12.2,3.40553951399999));
#337083=CARTESIAN_POINT('Ctrl Pts',(2.23390846199994,5.2,3.40553951399999));
#337084=CARTESIAN_POINT('Ctrl Pts',(2.23390846199994,2.2,3.40553951399999));
#337085=CARTESIAN_POINT('Ctrl Pts',(2.23427741599994,12.2,3.40645666299999));
#337086=CARTESIAN_POINT('Ctrl Pts',(2.23427741599994,5.2,3.40645666299999));
#337087=CARTESIAN_POINT('Ctrl Pts',(2.23427741599994,2.2,3.40645666299999));
#337088=CARTESIAN_POINT('Ctrl Pts',(2.23464728399994,12.2,3.40737937099998));
#337089=CARTESIAN_POINT('Ctrl Pts',(2.23464728399994,5.2,3.40737937099998));
#337090=CARTESIAN_POINT('Ctrl Pts',(2.23464728399994,2.2,3.40737937099998));
#337091=CARTESIAN_POINT('Ctrl Pts',(2.23501805199994,12.2,3.40830763099999));
#337092=CARTESIAN_POINT('Ctrl Pts',(2.23501805199994,5.2,3.40830763099999));
#337093=CARTESIAN_POINT('Ctrl Pts',(2.23501805199994,2.2,3.40830763099999));
#337094=CARTESIAN_POINT('Ctrl Pts',(2.23538970099994,12.2,3.40924143799998));
#337095=CARTESIAN_POINT('Ctrl Pts',(2.23538970099994,5.2,3.40924143799998));
#337096=CARTESIAN_POINT('Ctrl Pts',(2.23538970099994,2.2,3.40924143799998));
#337097=CARTESIAN_POINT('Ctrl Pts',(2.23576221699994,12.2,3.41018078599999));
#337098=CARTESIAN_POINT('Ctrl Pts',(2.23576221699994,5.2,3.41018078599999));
#337099=CARTESIAN_POINT('Ctrl Pts',(2.23576221699994,2.2,3.41018078599999));
#337100=CARTESIAN_POINT('Ctrl Pts',(2.23613558499994,12.2,3.41112567199998));
#337101=CARTESIAN_POINT('Ctrl Pts',(2.23613558499994,5.2,3.41112567199998));
#337102=CARTESIAN_POINT('Ctrl Pts',(2.23613558499994,2.2,3.41112567199998));
#337103=CARTESIAN_POINT('Ctrl Pts',(2.23650978899994,12.2,3.41207608999999));
#337104=CARTESIAN_POINT('Ctrl Pts',(2.23650978899994,5.2,3.41207608999999));
#337105=CARTESIAN_POINT('Ctrl Pts',(2.23650978899994,2.2,3.41207608999999));
#337106=CARTESIAN_POINT('Ctrl Pts',(2.23688481099994,12.2,3.41303203299999));
#337107=CARTESIAN_POINT('Ctrl Pts',(2.23688481099994,5.2,3.41303203299999));
#337108=CARTESIAN_POINT('Ctrl Pts',(2.23688481099994,2.2,3.41303203299999));
#337109=CARTESIAN_POINT('Ctrl Pts',(2.23726063799994,12.2,3.41399349799998));
#337110=CARTESIAN_POINT('Ctrl Pts',(2.23726063799994,5.2,3.41399349799998));
#337111=CARTESIAN_POINT('Ctrl Pts',(2.23726063799994,2.2,3.41399349799998));
#337112=CARTESIAN_POINT('Ctrl Pts',(2.23763725399994,12.2,3.41496047799998));
#337113=CARTESIAN_POINT('Ctrl Pts',(2.23763725399994,5.2,3.41496047799998));
#337114=CARTESIAN_POINT('Ctrl Pts',(2.23763725399994,2.2,3.41496047799998));
#337115=CARTESIAN_POINT('Ctrl Pts',(2.23801464299994,12.2,3.41593296899998));
#337116=CARTESIAN_POINT('Ctrl Pts',(2.23801464299994,5.2,3.41593296899998));
#337117=CARTESIAN_POINT('Ctrl Pts',(2.23801464299994,2.2,3.41593296899998));
#337118=CARTESIAN_POINT('Ctrl Pts',(2.23839278799994,12.2,3.41691096599998));
#337119=CARTESIAN_POINT('Ctrl Pts',(2.23839278799994,5.2,3.41691096599998));
#337120=CARTESIAN_POINT('Ctrl Pts',(2.23839278799994,2.2,3.41691096599998));
#337121=CARTESIAN_POINT('Ctrl Pts',(2.23877167599994,12.2,3.41789446399999));
#337122=CARTESIAN_POINT('Ctrl Pts',(2.23877167599994,5.2,3.41789446399999));
#337123=CARTESIAN_POINT('Ctrl Pts',(2.23877167599994,2.2,3.41789446399999));
#337124=CARTESIAN_POINT('Ctrl Pts',(2.23915129199994,12.2,3.41888345499999));
#337125=CARTESIAN_POINT('Ctrl Pts',(2.23915129199994,5.2,3.41888345499999));
#337126=CARTESIAN_POINT('Ctrl Pts',(2.23915129199994,2.2,3.41888345499999));
#337127=CARTESIAN_POINT('Ctrl Pts',(2.23953161699994,12.2,3.41987793699998));
#337128=CARTESIAN_POINT('Ctrl Pts',(2.23953161699994,5.2,3.41987793699998));
#337129=CARTESIAN_POINT('Ctrl Pts',(2.23953161699994,2.2,3.41987793699998));
#337130=CARTESIAN_POINT('Ctrl Pts',(2.23991263999994,12.2,3.42087790399999));
#337131=CARTESIAN_POINT('Ctrl Pts',(2.23991263999994,5.2,3.42087790399999));
#337132=CARTESIAN_POINT('Ctrl Pts',(2.23991263999994,2.2,3.42087790399999));
#337133=CARTESIAN_POINT('Ctrl Pts',(2.24029434299994,12.2,3.42188334899999));
#337134=CARTESIAN_POINT('Ctrl Pts',(2.24029434299994,5.2,3.42188334899999));
#337135=CARTESIAN_POINT('Ctrl Pts',(2.24029434299994,2.2,3.42188334899999));
#337136=CARTESIAN_POINT('Ctrl Pts',(2.24067671199994,12.2,3.42289426799999));
#337137=CARTESIAN_POINT('Ctrl Pts',(2.24067671199994,5.2,3.42289426799999));
#337138=CARTESIAN_POINT('Ctrl Pts',(2.24067671199994,2.2,3.42289426799999));
#337139=CARTESIAN_POINT('Ctrl Pts',(2.24105973099994,12.2,3.42391065599998));
#337140=CARTESIAN_POINT('Ctrl Pts',(2.24105973099994,5.2,3.42391065599998));
#337141=CARTESIAN_POINT('Ctrl Pts',(2.24105973099994,2.2,3.42391065599998));
#337142=CARTESIAN_POINT('Ctrl Pts',(2.24144338499995,12.2,3.42493250799999));
#337143=CARTESIAN_POINT('Ctrl Pts',(2.24144338499995,5.2,3.42493250799999));
#337144=CARTESIAN_POINT('Ctrl Pts',(2.24144338499995,2.2,3.42493250799999));
#337145=CARTESIAN_POINT('Ctrl Pts',(2.24182765899994,12.2,3.42595981699999));
#337146=CARTESIAN_POINT('Ctrl Pts',(2.24182765899994,5.2,3.42595981699999));
#337147=CARTESIAN_POINT('Ctrl Pts',(2.24182765899994,2.2,3.42595981699999));
#337148=CARTESIAN_POINT('Ctrl Pts',(2.24221253899994,12.2,3.42699257899999));
#337149=CARTESIAN_POINT('Ctrl Pts',(2.24221253899994,5.2,3.42699257899999));
#337150=CARTESIAN_POINT('Ctrl Pts',(2.24221253899994,2.2,3.42699257899999));
#337151=CARTESIAN_POINT('Ctrl Pts',(2.24259800899994,12.2,3.42803078999999));
#337152=CARTESIAN_POINT('Ctrl Pts',(2.24259800899994,5.2,3.42803078999999));
#337153=CARTESIAN_POINT('Ctrl Pts',(2.24259800899994,2.2,3.42803078999999));
#337154=CARTESIAN_POINT('Ctrl Pts',(2.24298405299994,12.2,3.42907444099998));
#337155=CARTESIAN_POINT('Ctrl Pts',(2.24298405299994,5.2,3.42907444099998));
#337156=CARTESIAN_POINT('Ctrl Pts',(2.24298405299994,2.2,3.42907444099998));
#337157=CARTESIAN_POINT('Ctrl Pts',(2.24337065799994,12.2,3.43012352999998));
#337158=CARTESIAN_POINT('Ctrl Pts',(2.24337065799994,5.2,3.43012352999998));
#337159=CARTESIAN_POINT('Ctrl Pts',(2.24337065799994,2.2,3.43012352999998));
#337160=CARTESIAN_POINT('Ctrl Pts',(2.24375780799994,12.2,3.43117804999999));
#337161=CARTESIAN_POINT('Ctrl Pts',(2.24375780799994,5.2,3.43117804999999));
#337162=CARTESIAN_POINT('Ctrl Pts',(2.24375780799994,2.2,3.43117804999999));
#337163=CARTESIAN_POINT('Ctrl Pts',(2.24414548899994,12.2,3.43223799699999));
#337164=CARTESIAN_POINT('Ctrl Pts',(2.24414548899994,5.2,3.43223799699999));
#337165=CARTESIAN_POINT('Ctrl Pts',(2.24414548899994,2.2,3.43223799699999));
#337166=CARTESIAN_POINT('Ctrl Pts',(2.24453368499994,12.2,3.43330336399998));
#337167=CARTESIAN_POINT('Ctrl Pts',(2.24453368499994,5.2,3.43330336399998));
#337168=CARTESIAN_POINT('Ctrl Pts',(2.24453368499994,2.2,3.43330336399998));
#337169=CARTESIAN_POINT('Ctrl Pts',(2.24492238299994,12.2,3.43437414699999));
#337170=CARTESIAN_POINT('Ctrl Pts',(2.24492238299994,5.2,3.43437414699999));
#337171=CARTESIAN_POINT('Ctrl Pts',(2.24492238299994,2.2,3.43437414699999));
#337172=CARTESIAN_POINT('Ctrl Pts',(2.24531156699994,12.2,3.43545033999998));
#337173=CARTESIAN_POINT('Ctrl Pts',(2.24531156699994,5.2,3.43545033999998));
#337174=CARTESIAN_POINT('Ctrl Pts',(2.24531156699994,2.2,3.43545033999998));
#337175=CARTESIAN_POINT('Ctrl Pts',(2.24570122199994,12.2,3.43653193799998));
#337176=CARTESIAN_POINT('Ctrl Pts',(2.24570122199994,5.2,3.43653193799998));
#337177=CARTESIAN_POINT('Ctrl Pts',(2.24570122199994,2.2,3.43653193799998));
#337178=CARTESIAN_POINT('Ctrl Pts',(2.24609133499994,12.2,3.43761893499998));
#337179=CARTESIAN_POINT('Ctrl Pts',(2.24609133499994,5.2,3.43761893499998));
#337180=CARTESIAN_POINT('Ctrl Pts',(2.24609133499994,2.2,3.43761893499998));
#337181=CARTESIAN_POINT('Ctrl Pts',(2.24648188999994,12.2,3.43871132799999));
#337182=CARTESIAN_POINT('Ctrl Pts',(2.24648188999994,5.2,3.43871132799999));
#337183=CARTESIAN_POINT('Ctrl Pts',(2.24648188999994,2.2,3.43871132799999));
#337184=CARTESIAN_POINT('Ctrl Pts',(2.24687287199994,12.2,3.43980910799999));
#337185=CARTESIAN_POINT('Ctrl Pts',(2.24687287199994,5.2,3.43980910799999));
#337186=CARTESIAN_POINT('Ctrl Pts',(2.24687287199994,2.2,3.43980910799999));
#337187=CARTESIAN_POINT('Ctrl Pts',(2.24726426799994,12.2,3.44091227099998));
#337188=CARTESIAN_POINT('Ctrl Pts',(2.24726426799994,5.2,3.44091227099998));
#337189=CARTESIAN_POINT('Ctrl Pts',(2.24726426799994,2.2,3.44091227099998));
#337190=CARTESIAN_POINT('Ctrl Pts',(2.24765606399994,12.2,3.44202081299999));
#337191=CARTESIAN_POINT('Ctrl Pts',(2.24765606399994,5.2,3.44202081299999));
#337192=CARTESIAN_POINT('Ctrl Pts',(2.24765606399994,2.2,3.44202081299999));
#337193=CARTESIAN_POINT('Ctrl Pts',(2.24804824299994,12.2,3.44313472599998));
#337194=CARTESIAN_POINT('Ctrl Pts',(2.24804824299994,5.2,3.44313472599998));
#337195=CARTESIAN_POINT('Ctrl Pts',(2.24804824299994,2.2,3.44313472599998));
#337196=CARTESIAN_POINT('Ctrl Pts',(2.24844079299995,12.2,3.44425400799998));
#337197=CARTESIAN_POINT('Ctrl Pts',(2.24844079299995,5.2,3.44425400799998));
#337198=CARTESIAN_POINT('Ctrl Pts',(2.24844079299995,2.2,3.44425400799998));
#337199=CARTESIAN_POINT('Ctrl Pts',(2.24883369799994,12.2,3.44537865099999));
#337200=CARTESIAN_POINT('Ctrl Pts',(2.24883369799994,5.2,3.44537865099999));
#337201=CARTESIAN_POINT('Ctrl Pts',(2.24883369799994,2.2,3.44537865099999));
#337202=CARTESIAN_POINT('Ctrl Pts',(2.24922694499994,12.2,3.44650864999998));
#337203=CARTESIAN_POINT('Ctrl Pts',(2.24922694499994,5.2,3.44650864999998));
#337204=CARTESIAN_POINT('Ctrl Pts',(2.24922694499994,2.2,3.44650864999998));
#337205=CARTESIAN_POINT('Ctrl Pts',(2.24962051999994,12.2,3.44764399999999));
#337206=CARTESIAN_POINT('Ctrl Pts',(2.24962051999994,5.2,3.44764399999999));
#337207=CARTESIAN_POINT('Ctrl Pts',(2.24962051999994,2.2,3.44764399999999));
#337208=CARTESIAN_POINT('Ctrl Pts',(2.25001440599994,12.2,3.44878469599998));
#337209=CARTESIAN_POINT('Ctrl Pts',(2.25001440599994,5.2,3.44878469599998));
#337210=CARTESIAN_POINT('Ctrl Pts',(2.25001440599994,2.2,3.44878469599998));
#337211=CARTESIAN_POINT('Ctrl Pts',(2.25040859199995,12.2,3.44993073199999));
#337212=CARTESIAN_POINT('Ctrl Pts',(2.25040859199995,5.2,3.44993073199999));
#337213=CARTESIAN_POINT('Ctrl Pts',(2.25040859199995,2.2,3.44993073199999));
#337214=CARTESIAN_POINT('Ctrl Pts',(2.25080306199994,12.2,3.45108210299998));
#337215=CARTESIAN_POINT('Ctrl Pts',(2.25080306199994,5.2,3.45108210299998));
#337216=CARTESIAN_POINT('Ctrl Pts',(2.25080306199994,2.2,3.45108210299998));
#337217=CARTESIAN_POINT('Ctrl Pts',(2.25119780399994,12.2,3.45223880199999));
#337218=CARTESIAN_POINT('Ctrl Pts',(2.25119780399994,5.2,3.45223880199999));
#337219=CARTESIAN_POINT('Ctrl Pts',(2.25119780399994,2.2,3.45223880199999));
#337220=CARTESIAN_POINT('Ctrl Pts',(2.25159280199994,12.2,3.45340082499998));
#337221=CARTESIAN_POINT('Ctrl Pts',(2.25159280199994,5.2,3.45340082499998));
#337222=CARTESIAN_POINT('Ctrl Pts',(2.25159280199994,2.2,3.45340082499998));
#337223=CARTESIAN_POINT('Ctrl Pts',(2.25198804199994,12.2,3.45456816699999));
#337224=CARTESIAN_POINT('Ctrl Pts',(2.25198804199994,5.2,3.45456816699999));
#337225=CARTESIAN_POINT('Ctrl Pts',(2.25198804199994,2.2,3.45456816699999));
#337226=CARTESIAN_POINT('Ctrl Pts',(2.25238351099994,12.2,3.45574082199998));
#337227=CARTESIAN_POINT('Ctrl Pts',(2.25238351099994,5.2,3.45574082199998));
#337228=CARTESIAN_POINT('Ctrl Pts',(2.25238351099994,2.2,3.45574082199998));
#337229=CARTESIAN_POINT('Ctrl Pts',(2.25277919399994,12.2,3.45691878299998));
#337230=CARTESIAN_POINT('Ctrl Pts',(2.25277919399994,5.2,3.45691878299998));
#337231=CARTESIAN_POINT('Ctrl Pts',(2.25277919399994,2.2,3.45691878299998));
#337232=CARTESIAN_POINT('Ctrl Pts',(2.25317507799994,12.2,3.45810204699998));
#337233=CARTESIAN_POINT('Ctrl Pts',(2.25317507799994,5.2,3.45810204699998));
#337234=CARTESIAN_POINT('Ctrl Pts',(2.25317507799994,2.2,3.45810204699998));
#337235=CARTESIAN_POINT('Ctrl Pts',(2.25357114899994,12.2,3.45929060799998));
#337236=CARTESIAN_POINT('Ctrl Pts',(2.25357114899994,5.2,3.45929060799998));
#337237=CARTESIAN_POINT('Ctrl Pts',(2.25357114899994,2.2,3.45929060799998));
#337238=CARTESIAN_POINT('Ctrl Pts',(2.25396739399994,12.2,3.46048445899999));
#337239=CARTESIAN_POINT('Ctrl Pts',(2.25396739399994,5.2,3.46048445899999));
#337240=CARTESIAN_POINT('Ctrl Pts',(2.25396739399994,2.2,3.46048445899999));
#337241=CARTESIAN_POINT('Ctrl Pts',(2.25436379699994,12.2,3.46168359599999));
#337242=CARTESIAN_POINT('Ctrl Pts',(2.25436379699994,5.2,3.46168359599999));
#337243=CARTESIAN_POINT('Ctrl Pts',(2.25436379699994,2.2,3.46168359599999));
#337244=CARTESIAN_POINT('Ctrl Pts',(2.25476034499994,12.2,3.46288801199999));
#337245=CARTESIAN_POINT('Ctrl Pts',(2.25476034499994,5.2,3.46288801199999));
#337246=CARTESIAN_POINT('Ctrl Pts',(2.25476034499994,2.2,3.46288801199999));
#337247=CARTESIAN_POINT('Ctrl Pts',(2.25515702499994,12.2,3.46409770399998));
#337248=CARTESIAN_POINT('Ctrl Pts',(2.25515702499994,5.2,3.46409770399998));
#337249=CARTESIAN_POINT('Ctrl Pts',(2.25515702499994,2.2,3.46409770399998));
#337250=CARTESIAN_POINT('Ctrl Pts',(2.25555382399994,12.2,3.46531266399998));
#337251=CARTESIAN_POINT('Ctrl Pts',(2.25555382399994,5.2,3.46531266399998));
#337252=CARTESIAN_POINT('Ctrl Pts',(2.25555382399994,2.2,3.46531266399998));
#337253=CARTESIAN_POINT('Ctrl Pts',(2.25595072699994,12.2,3.46653288799998));
#337254=CARTESIAN_POINT('Ctrl Pts',(2.25595072699994,5.2,3.46653288799998));
#337255=CARTESIAN_POINT('Ctrl Pts',(2.25595072699994,2.2,3.46653288799998));
#337256=CARTESIAN_POINT('Ctrl Pts',(2.25634771999994,12.2,3.46775836899998));
#337257=CARTESIAN_POINT('Ctrl Pts',(2.25634771999994,5.2,3.46775836899998));
#337258=CARTESIAN_POINT('Ctrl Pts',(2.25634771999994,2.2,3.46775836899998));
#337259=CARTESIAN_POINT('Ctrl Pts',(2.25674479099994,12.2,3.46898910299998));
#337260=CARTESIAN_POINT('Ctrl Pts',(2.25674479099994,5.2,3.46898910299998));
#337261=CARTESIAN_POINT('Ctrl Pts',(2.25674479099994,2.2,3.46898910299998));
#337262=CARTESIAN_POINT('Ctrl Pts',(2.25714192599995,12.2,3.47022508299998));
#337263=CARTESIAN_POINT('Ctrl Pts',(2.25714192599995,5.2,3.47022508299998));
#337264=CARTESIAN_POINT('Ctrl Pts',(2.25714192599995,2.2,3.47022508299998));
#337265=CARTESIAN_POINT('Ctrl Pts',(2.25753911099994,12.2,3.47146630599998));
#337266=CARTESIAN_POINT('Ctrl Pts',(2.25753911099994,5.2,3.47146630599998));
#337267=CARTESIAN_POINT('Ctrl Pts',(2.25753911099994,2.2,3.47146630599998));
#337268=CARTESIAN_POINT('Ctrl Pts',(2.25793633199994,12.2,3.47271276399999));
#337269=CARTESIAN_POINT('Ctrl Pts',(2.25793633199994,5.2,3.47271276399999));
#337270=CARTESIAN_POINT('Ctrl Pts',(2.25793633199994,2.2,3.47271276399999));
#337271=CARTESIAN_POINT('Ctrl Pts',(2.25833357799994,12.2,3.47396445199998));
#337272=CARTESIAN_POINT('Ctrl Pts',(2.25833357799994,5.2,3.47396445199998));
#337273=CARTESIAN_POINT('Ctrl Pts',(2.25833357799994,2.2,3.47396445199998));
#337274=CARTESIAN_POINT('Ctrl Pts',(2.25873083299994,12.2,3.47522136599999));
#337275=CARTESIAN_POINT('Ctrl Pts',(2.25873083299994,5.2,3.47522136599999));
#337276=CARTESIAN_POINT('Ctrl Pts',(2.25873083299994,2.2,3.47522136599999));
#337277=CARTESIAN_POINT('Ctrl Pts',(2.25912808499994,12.2,3.47648349699998));
#337278=CARTESIAN_POINT('Ctrl Pts',(2.25912808499994,5.2,3.47648349699998));
#337279=CARTESIAN_POINT('Ctrl Pts',(2.25912808499994,2.2,3.47648349699998));
#337280=CARTESIAN_POINT('Ctrl Pts',(2.25952531999994,12.2,3.47775084299998));
#337281=CARTESIAN_POINT('Ctrl Pts',(2.25952531999994,5.2,3.47775084299998));
#337282=CARTESIAN_POINT('Ctrl Pts',(2.25952531999994,2.2,3.47775084299998));
#337283=CARTESIAN_POINT('Ctrl Pts',(2.25992252599994,12.2,3.47902339799998));
#337284=CARTESIAN_POINT('Ctrl Pts',(2.25992252599994,5.2,3.47902339799998));
#337285=CARTESIAN_POINT('Ctrl Pts',(2.25992252599994,2.2,3.47902339799998));
#337286=CARTESIAN_POINT('Ctrl Pts',(2.26031968799994,12.2,3.48030115399999));
#337287=CARTESIAN_POINT('Ctrl Pts',(2.26031968799994,5.2,3.48030115399999));
#337288=CARTESIAN_POINT('Ctrl Pts',(2.26031968799994,2.2,3.48030115399999));
#337289=CARTESIAN_POINT('Ctrl Pts',(2.26071679399994,12.2,3.48158410699998));
#337290=CARTESIAN_POINT('Ctrl Pts',(2.26071679399994,5.2,3.48158410699998));
#337291=CARTESIAN_POINT('Ctrl Pts',(2.26071679399994,2.2,3.48158410699998));
#337292=CARTESIAN_POINT('Ctrl Pts',(2.26111382999994,12.2,3.48287225199999));
#337293=CARTESIAN_POINT('Ctrl Pts',(2.26111382999994,5.2,3.48287225199999));
#337294=CARTESIAN_POINT('Ctrl Pts',(2.26111382999994,2.2,3.48287225199999));
#337295=CARTESIAN_POINT('Ctrl Pts',(2.26151078499994,12.2,3.48416558199999));
#337296=CARTESIAN_POINT('Ctrl Pts',(2.26151078499994,5.2,3.48416558199999));
#337297=CARTESIAN_POINT('Ctrl Pts',(2.26151078499994,2.2,3.48416558199999));
#337298=CARTESIAN_POINT('Ctrl Pts',(2.26190764199994,12.2,3.48546409299999));
#337299=CARTESIAN_POINT('Ctrl Pts',(2.26190764199994,5.2,3.48546409299999));
#337300=CARTESIAN_POINT('Ctrl Pts',(2.26190764199994,2.2,3.48546409299999));
#337301=CARTESIAN_POINT('Ctrl Pts',(2.26230439099994,12.2,3.48676777799999));
#337302=CARTESIAN_POINT('Ctrl Pts',(2.26230439099994,5.2,3.48676777799999));
#337303=CARTESIAN_POINT('Ctrl Pts',(2.26230439099994,2.2,3.48676777799999));
#337304=CARTESIAN_POINT('Ctrl Pts',(2.26270101999994,12.2,3.48807663199998));
#337305=CARTESIAN_POINT('Ctrl Pts',(2.26270101999994,5.2,3.48807663199998));
#337306=CARTESIAN_POINT('Ctrl Pts',(2.26270101999994,2.2,3.48807663199998));
#337307=CARTESIAN_POINT('Ctrl Pts',(2.26309751299994,12.2,3.48939064899999));
#337308=CARTESIAN_POINT('Ctrl Pts',(2.26309751299994,5.2,3.48939064899999));
#337309=CARTESIAN_POINT('Ctrl Pts',(2.26309751299994,2.2,3.48939064899999));
#337310=CARTESIAN_POINT('Ctrl Pts',(2.26349385799994,12.2,3.49070982399999));
#337311=CARTESIAN_POINT('Ctrl Pts',(2.26349385799994,5.2,3.49070982399999));
#337312=CARTESIAN_POINT('Ctrl Pts',(2.26349385799994,2.2,3.49070982399999));
#337313=CARTESIAN_POINT('Ctrl Pts',(2.26389004199994,12.2,3.49203415199998));
#337314=CARTESIAN_POINT('Ctrl Pts',(2.26389004199994,5.2,3.49203415199998));
#337315=CARTESIAN_POINT('Ctrl Pts',(2.26389004199994,2.2,3.49203415199998));
#337316=CARTESIAN_POINT('Ctrl Pts',(2.26428605399994,12.2,3.49336362599999));
#337317=CARTESIAN_POINT('Ctrl Pts',(2.26428605399994,5.2,3.49336362599999));
#337318=CARTESIAN_POINT('Ctrl Pts',(2.26428605399994,2.2,3.49336362599999));
#337319=CARTESIAN_POINT('Ctrl Pts',(2.26468187899994,12.2,3.49469823999998));
#337320=CARTESIAN_POINT('Ctrl Pts',(2.26468187899994,5.2,3.49469823999998));
#337321=CARTESIAN_POINT('Ctrl Pts',(2.26468187899994,2.2,3.49469823999998));
#337322=CARTESIAN_POINT('Ctrl Pts',(2.26507750499994,12.2,3.49603798999999));
#337323=CARTESIAN_POINT('Ctrl Pts',(2.26507750499994,5.2,3.49603798999999));
#337324=CARTESIAN_POINT('Ctrl Pts',(2.26507750499994,2.2,3.49603798999999));
#337325=CARTESIAN_POINT('Ctrl Pts',(2.26547291799994,12.2,3.49738286999998));
#337326=CARTESIAN_POINT('Ctrl Pts',(2.26547291799994,5.2,3.49738286999998));
#337327=CARTESIAN_POINT('Ctrl Pts',(2.26547291799994,2.2,3.49738286999998));
#337328=CARTESIAN_POINT('Ctrl Pts',(2.26586810699994,12.2,3.49873287299998));
#337329=CARTESIAN_POINT('Ctrl Pts',(2.26586810699994,5.2,3.49873287299998));
#337330=CARTESIAN_POINT('Ctrl Pts',(2.26586810699994,2.2,3.49873287299998));
#337331=CARTESIAN_POINT('Ctrl Pts',(2.26626305999994,12.2,3.50008799499999));
#337332=CARTESIAN_POINT('Ctrl Pts',(2.26626305999994,5.2,3.50008799499999));
#337333=CARTESIAN_POINT('Ctrl Pts',(2.26626305999994,2.2,3.50008799499999));
#337334=CARTESIAN_POINT('Ctrl Pts',(2.26665776199994,12.2,3.50144822999999));
#337335=CARTESIAN_POINT('Ctrl Pts',(2.26665776199994,5.2,3.50144822999999));
#337336=CARTESIAN_POINT('Ctrl Pts',(2.26665776199994,2.2,3.50144822999999));
#337337=CARTESIAN_POINT('Ctrl Pts',(2.26705220099995,12.2,3.50281357199999));
#337338=CARTESIAN_POINT('Ctrl Pts',(2.26705220099995,5.2,3.50281357199999));
#337339=CARTESIAN_POINT('Ctrl Pts',(2.26705220099995,2.2,3.50281357199999));
#337340=CARTESIAN_POINT('Ctrl Pts',(2.26744636499994,12.2,3.50418401399998));
#337341=CARTESIAN_POINT('Ctrl Pts',(2.26744636499994,5.2,3.50418401399998));
#337342=CARTESIAN_POINT('Ctrl Pts',(2.26744636499994,2.2,3.50418401399998));
#337343=CARTESIAN_POINT('Ctrl Pts',(2.26784024099994,12.2,3.50555955299999));
#337344=CARTESIAN_POINT('Ctrl Pts',(2.26784024099994,5.2,3.50555955299999));
#337345=CARTESIAN_POINT('Ctrl Pts',(2.26784024099994,2.2,3.50555955299999));
#337346=CARTESIAN_POINT('Ctrl Pts',(2.26823381699994,12.2,3.50694018099999));
#337347=CARTESIAN_POINT('Ctrl Pts',(2.26823381699994,5.2,3.50694018099999));
#337348=CARTESIAN_POINT('Ctrl Pts',(2.26823381699994,2.2,3.50694018099999));
#337349=CARTESIAN_POINT('Ctrl Pts',(2.26862707899994,12.2,3.50832589399998));
#337350=CARTESIAN_POINT('Ctrl Pts',(2.26862707899994,5.2,3.50832589399998));
#337351=CARTESIAN_POINT('Ctrl Pts',(2.26862707899994,2.2,3.50832589399998));
#337352=CARTESIAN_POINT('Ctrl Pts',(2.26902001799994,12.2,3.50971668499999));
#337353=CARTESIAN_POINT('Ctrl Pts',(2.26902001799994,5.2,3.50971668499999));
#337354=CARTESIAN_POINT('Ctrl Pts',(2.26902001799994,2.2,3.50971668499999));
#337355=CARTESIAN_POINT('Ctrl Pts',(2.26941261799994,12.2,3.51111254999999));
#337356=CARTESIAN_POINT('Ctrl Pts',(2.26941261799994,5.2,3.51111254999999));
#337357=CARTESIAN_POINT('Ctrl Pts',(2.26941261799994,2.2,3.51111254999999));
#337358=CARTESIAN_POINT('Ctrl Pts',(2.26980486699994,12.2,3.51251348199998));
#337359=CARTESIAN_POINT('Ctrl Pts',(2.26980486699994,5.2,3.51251348199998));
#337360=CARTESIAN_POINT('Ctrl Pts',(2.26980486699994,2.2,3.51251348199998));
#337361=CARTESIAN_POINT('Ctrl Pts',(2.27019675399994,12.2,3.51391947499998));
#337362=CARTESIAN_POINT('Ctrl Pts',(2.27019675399994,5.2,3.51391947499998));
#337363=CARTESIAN_POINT('Ctrl Pts',(2.27019675399994,2.2,3.51391947499998));
#337364=CARTESIAN_POINT('Ctrl Pts',(2.27058826699994,12.2,3.51533052499998));
#337365=CARTESIAN_POINT('Ctrl Pts',(2.27058826699994,5.2,3.51533052499998));
#337366=CARTESIAN_POINT('Ctrl Pts',(2.27058826699994,2.2,3.51533052499998));
#337367=CARTESIAN_POINT('Ctrl Pts',(2.27097939199994,12.2,3.51674662399999));
#337368=CARTESIAN_POINT('Ctrl Pts',(2.27097939199994,5.2,3.51674662399999));
#337369=CARTESIAN_POINT('Ctrl Pts',(2.27097939199994,2.2,3.51674662399999));
#337370=CARTESIAN_POINT('Ctrl Pts',(2.27137011799994,12.2,3.51816776699999));
#337371=CARTESIAN_POINT('Ctrl Pts',(2.27137011799994,5.2,3.51816776699999));
#337372=CARTESIAN_POINT('Ctrl Pts',(2.27137011799994,2.2,3.51816776699999));
#337373=CARTESIAN_POINT('Ctrl Pts',(2.27176043199994,12.2,3.51959394999999));
#337374=CARTESIAN_POINT('Ctrl Pts',(2.27176043199994,5.2,3.51959394999999));
#337375=CARTESIAN_POINT('Ctrl Pts',(2.27176043199994,2.2,3.51959394999999));
#337376=CARTESIAN_POINT('Ctrl Pts',(2.27215032199994,12.2,3.52102516599999));
#337377=CARTESIAN_POINT('Ctrl Pts',(2.27215032199994,5.2,3.52102516599999));
#337378=CARTESIAN_POINT('Ctrl Pts',(2.27215032199994,2.2,3.52102516599999));
#337379=CARTESIAN_POINT('Ctrl Pts',(2.27253977599994,12.2,3.52246140899998));
#337380=CARTESIAN_POINT('Ctrl Pts',(2.27253977599994,5.2,3.52246140899998));
#337381=CARTESIAN_POINT('Ctrl Pts',(2.27253977599994,2.2,3.52246140899998));
#337382=CARTESIAN_POINT('Ctrl Pts',(2.27292878199994,12.2,3.52390267299998));
#337383=CARTESIAN_POINT('Ctrl Pts',(2.27292878199994,5.2,3.52390267299998));
#337384=CARTESIAN_POINT('Ctrl Pts',(2.27292878199994,2.2,3.52390267299998));
#337385=CARTESIAN_POINT('Ctrl Pts',(2.27331732799994,12.2,3.52534895399998));
#337386=CARTESIAN_POINT('Ctrl Pts',(2.27331732799994,5.2,3.52534895399998));
#337387=CARTESIAN_POINT('Ctrl Pts',(2.27331732799994,2.2,3.52534895399998));
#337388=CARTESIAN_POINT('Ctrl Pts',(2.27370540099994,12.2,3.52680024399999));
#337389=CARTESIAN_POINT('Ctrl Pts',(2.27370540099994,5.2,3.52680024399999));
#337390=CARTESIAN_POINT('Ctrl Pts',(2.27370540099994,2.2,3.52680024399999));
#337391=CARTESIAN_POINT('Ctrl Pts',(2.27409298999994,12.2,3.52825653899998));
#337392=CARTESIAN_POINT('Ctrl Pts',(2.27409298999994,5.2,3.52825653899998));
#337393=CARTESIAN_POINT('Ctrl Pts',(2.27409298999994,2.2,3.52825653899998));
#337394=CARTESIAN_POINT('Ctrl Pts',(2.27448008299994,12.2,3.52971783199998));
#337395=CARTESIAN_POINT('Ctrl Pts',(2.27448008299994,5.2,3.52971783199998));
#337396=CARTESIAN_POINT('Ctrl Pts',(2.27448008299994,2.2,3.52971783199998));
#337397=CARTESIAN_POINT('Ctrl Pts',(2.27486666599995,12.2,3.53118411799999));
#337398=CARTESIAN_POINT('Ctrl Pts',(2.27486666599995,5.2,3.53118411799999));
#337399=CARTESIAN_POINT('Ctrl Pts',(2.27486666599995,2.2,3.53118411799999));
#337400=CARTESIAN_POINT('Ctrl Pts',(2.27525272999994,12.2,3.53265539299999));
#337401=CARTESIAN_POINT('Ctrl Pts',(2.27525272999994,5.2,3.53265539299999));
#337402=CARTESIAN_POINT('Ctrl Pts',(2.27525272999994,2.2,3.53265539299999));
#337403=CARTESIAN_POINT('Ctrl Pts',(2.27563826199995,12.2,3.53413164699998));
#337404=CARTESIAN_POINT('Ctrl Pts',(2.27563826199995,5.2,3.53413164699998));
#337405=CARTESIAN_POINT('Ctrl Pts',(2.27563826199995,2.2,3.53413164699998));
#337406=CARTESIAN_POINT('Ctrl Pts',(2.27602324899994,12.2,3.53561287799998));
#337407=CARTESIAN_POINT('Ctrl Pts',(2.27602324899994,5.2,3.53561287799998));
#337408=CARTESIAN_POINT('Ctrl Pts',(2.27602324899994,2.2,3.53561287799998));
#337409=CARTESIAN_POINT('Ctrl Pts',(2.27640768099994,12.2,3.53709907799999));
#337410=CARTESIAN_POINT('Ctrl Pts',(2.27640768099994,5.2,3.53709907799999));
#337411=CARTESIAN_POINT('Ctrl Pts',(2.27640768099994,2.2,3.53709907799999));
#337412=CARTESIAN_POINT('Ctrl Pts',(2.27679154299994,12.2,3.53859024199998));
#337413=CARTESIAN_POINT('Ctrl Pts',(2.27679154299994,5.2,3.53859024199998));
#337414=CARTESIAN_POINT('Ctrl Pts',(2.27679154299994,2.2,3.53859024199998));
#337415=CARTESIAN_POINT('Ctrl Pts',(2.27717482699994,12.2,3.54008636499999));
#337416=CARTESIAN_POINT('Ctrl Pts',(2.27717482699994,5.2,3.54008636499999));
#337417=CARTESIAN_POINT('Ctrl Pts',(2.27717482699994,2.2,3.54008636499999));
#337418=CARTESIAN_POINT('Ctrl Pts',(2.27755751999994,12.2,3.54158743999999));
#337419=CARTESIAN_POINT('Ctrl Pts',(2.27755751999994,5.2,3.54158743999999));
#337420=CARTESIAN_POINT('Ctrl Pts',(2.27755751999994,2.2,3.54158743999999));
#337421=CARTESIAN_POINT('Ctrl Pts',(2.27793960899994,12.2,3.54309346199998));
#337422=CARTESIAN_POINT('Ctrl Pts',(2.27793960899994,5.2,3.54309346199998));
#337423=CARTESIAN_POINT('Ctrl Pts',(2.27793960899994,2.2,3.54309346199998));
#337424=CARTESIAN_POINT('Ctrl Pts',(2.27832108299994,12.2,3.54460442399999));
#337425=CARTESIAN_POINT('Ctrl Pts',(2.27832108299994,5.2,3.54460442399999));
#337426=CARTESIAN_POINT('Ctrl Pts',(2.27832108299994,2.2,3.54460442399999));
#337427=CARTESIAN_POINT('Ctrl Pts',(2.27870193199994,12.2,3.54612032199999));
#337428=CARTESIAN_POINT('Ctrl Pts',(2.27870193199994,5.2,3.54612032199999));
#337429=CARTESIAN_POINT('Ctrl Pts',(2.27870193199994,2.2,3.54612032199999));
#337430=CARTESIAN_POINT('Ctrl Pts',(2.27908214199994,12.2,3.54764114899999));
#337431=CARTESIAN_POINT('Ctrl Pts',(2.27908214199994,5.2,3.54764114899999));
#337432=CARTESIAN_POINT('Ctrl Pts',(2.27908214199994,2.2,3.54764114899999));
#337433=CARTESIAN_POINT('Ctrl Pts',(2.27946170199994,12.2,3.54916689899999));
#337434=CARTESIAN_POINT('Ctrl Pts',(2.27946170199994,5.2,3.54916689899999));
#337435=CARTESIAN_POINT('Ctrl Pts',(2.27946170199994,2.2,3.54916689899999));
#337436=CARTESIAN_POINT('Ctrl Pts',(2.27984059999994,12.2,3.55069756799999));
#337437=CARTESIAN_POINT('Ctrl Pts',(2.27984059999994,5.2,3.55069756799999));
#337438=CARTESIAN_POINT('Ctrl Pts',(2.27984059999994,2.2,3.55069756799999));
#337439=CARTESIAN_POINT('Ctrl Pts',(2.28021882599994,12.2,3.55223314899998));
#337440=CARTESIAN_POINT('Ctrl Pts',(2.28021882599994,5.2,3.55223314899998));
#337441=CARTESIAN_POINT('Ctrl Pts',(2.28021882599994,2.2,3.55223314899998));
#337442=CARTESIAN_POINT('Ctrl Pts',(2.28059636799994,12.2,3.55377363399998));
#337443=CARTESIAN_POINT('Ctrl Pts',(2.28059636799994,5.2,3.55377363399998));
#337444=CARTESIAN_POINT('Ctrl Pts',(2.28059636799994,2.2,3.55377363399998));
#337445=CARTESIAN_POINT('Ctrl Pts',(2.28097321299995,12.2,3.55531902099998));
#337446=CARTESIAN_POINT('Ctrl Pts',(2.28097321299995,5.2,3.55531902099998));
#337447=CARTESIAN_POINT('Ctrl Pts',(2.28097321299995,2.2,3.55531902099998));
#337448=CARTESIAN_POINT('Ctrl Pts',(2.28134935199995,12.2,3.55686930299999));
#337449=CARTESIAN_POINT('Ctrl Pts',(2.28134935199995,5.2,3.55686930299999));
#337450=CARTESIAN_POINT('Ctrl Pts',(2.28134935199995,2.2,3.55686930299999));
#337451=CARTESIAN_POINT('Ctrl Pts',(2.28172477199994,12.2,3.55842447199999));
#337452=CARTESIAN_POINT('Ctrl Pts',(2.28172477199994,5.2,3.55842447199999));
#337453=CARTESIAN_POINT('Ctrl Pts',(2.28172477199994,2.2,3.55842447199999));
#337454=CARTESIAN_POINT('Ctrl Pts',(2.28209946099994,12.2,3.55998452399999));
#337455=CARTESIAN_POINT('Ctrl Pts',(2.28209946099994,5.2,3.55998452399999));
#337456=CARTESIAN_POINT('Ctrl Pts',(2.28209946099994,2.2,3.55998452399999));
#337457=CARTESIAN_POINT('Ctrl Pts',(2.28247340999994,12.2,3.56154945399999));
#337458=CARTESIAN_POINT('Ctrl Pts',(2.28247340999994,5.2,3.56154945399999));
#337459=CARTESIAN_POINT('Ctrl Pts',(2.28247340999994,2.2,3.56154945399999));
#337460=CARTESIAN_POINT('Ctrl Pts',(2.28284660499994,12.2,3.56311925399999));
#337461=CARTESIAN_POINT('Ctrl Pts',(2.28284660499994,5.2,3.56311925399999));
#337462=CARTESIAN_POINT('Ctrl Pts',(2.28284660499994,2.2,3.56311925399999));
#337463=CARTESIAN_POINT('Ctrl Pts',(2.28321903599995,12.2,3.56469391999998));
#337464=CARTESIAN_POINT('Ctrl Pts',(2.28321903599995,5.2,3.56469391999998));
#337465=CARTESIAN_POINT('Ctrl Pts',(2.28321903599995,2.2,3.56469391999998));
#337466=CARTESIAN_POINT('Ctrl Pts',(2.28359069099994,12.2,3.56627344499999));
#337467=CARTESIAN_POINT('Ctrl Pts',(2.28359069099994,5.2,3.56627344499999));
#337468=CARTESIAN_POINT('Ctrl Pts',(2.28359069099994,2.2,3.56627344499999));
#337469=CARTESIAN_POINT('Ctrl Pts',(2.28396156099994,12.2,3.56785782399999));
#337470=CARTESIAN_POINT('Ctrl Pts',(2.28396156099994,5.2,3.56785782399999));
#337471=CARTESIAN_POINT('Ctrl Pts',(2.28396156099994,2.2,3.56785782399999));
#337472=CARTESIAN_POINT('Ctrl Pts',(2.28433163099994,12.2,3.56944704999999));
#337473=CARTESIAN_POINT('Ctrl Pts',(2.28433163099994,5.2,3.56944704999999));
#337474=CARTESIAN_POINT('Ctrl Pts',(2.28433163099994,2.2,3.56944704999999));
#337475=CARTESIAN_POINT('Ctrl Pts',(2.28470089299994,12.2,3.57104111799998));
#337476=CARTESIAN_POINT('Ctrl Pts',(2.28470089299994,5.2,3.57104111799998));
#337477=CARTESIAN_POINT('Ctrl Pts',(2.28470089299994,2.2,3.57104111799998));
#337478=CARTESIAN_POINT('Ctrl Pts',(2.28506933499994,12.2,3.57264002299999));
#337479=CARTESIAN_POINT('Ctrl Pts',(2.28506933499994,5.2,3.57264002299999));
#337480=CARTESIAN_POINT('Ctrl Pts',(2.28506933499994,2.2,3.57264002299999));
#337481=CARTESIAN_POINT('Ctrl Pts',(2.28543694599994,12.2,3.57424375699999));
#337482=CARTESIAN_POINT('Ctrl Pts',(2.28543694599994,5.2,3.57424375699999));
#337483=CARTESIAN_POINT('Ctrl Pts',(2.28543694599994,2.2,3.57424375699999));
#337484=CARTESIAN_POINT('Ctrl Pts',(2.28580371299994,12.2,3.57585231599998));
#337485=CARTESIAN_POINT('Ctrl Pts',(2.28580371299994,5.2,3.57585231599998));
#337486=CARTESIAN_POINT('Ctrl Pts',(2.28580371299994,2.2,3.57585231599998));
#337487=CARTESIAN_POINT('Ctrl Pts',(2.28616962799994,12.2,3.57746569199998));
#337488=CARTESIAN_POINT('Ctrl Pts',(2.28616962799994,5.2,3.57746569199998));
#337489=CARTESIAN_POINT('Ctrl Pts',(2.28616962799994,2.2,3.57746569199998));
#337490=CARTESIAN_POINT('Ctrl Pts',(2.28653467799994,12.2,3.57908388199998));
#337491=CARTESIAN_POINT('Ctrl Pts',(2.28653467799994,5.2,3.57908388199998));
#337492=CARTESIAN_POINT('Ctrl Pts',(2.28653467799994,2.2,3.57908388199998));
#337493=CARTESIAN_POINT('Ctrl Pts',(2.28689885199994,12.2,3.58070687699998));
#337494=CARTESIAN_POINT('Ctrl Pts',(2.28689885199994,5.2,3.58070687699998));
#337495=CARTESIAN_POINT('Ctrl Pts',(2.28689885199994,2.2,3.58070687699998));
#337496=CARTESIAN_POINT('Ctrl Pts',(2.28726213899995,12.2,3.58233467399998));
#337497=CARTESIAN_POINT('Ctrl Pts',(2.28726213899995,5.2,3.58233467399998));
#337498=CARTESIAN_POINT('Ctrl Pts',(2.28726213899995,2.2,3.58233467399998));
#337499=CARTESIAN_POINT('Ctrl Pts',(2.28762452899994,12.2,3.58396726599998));
#337500=CARTESIAN_POINT('Ctrl Pts',(2.28762452899994,5.2,3.58396726599998));
#337501=CARTESIAN_POINT('Ctrl Pts',(2.28762452899994,2.2,3.58396726599998));
#337502=CARTESIAN_POINT('Ctrl Pts',(2.28798600999994,12.2,3.58560464599999));
#337503=CARTESIAN_POINT('Ctrl Pts',(2.28798600999994,5.2,3.58560464599999));
#337504=CARTESIAN_POINT('Ctrl Pts',(2.28798600999994,2.2,3.58560464599999));
#337505=CARTESIAN_POINT('Ctrl Pts',(2.28834657299994,12.2,3.58724680899999));
#337506=CARTESIAN_POINT('Ctrl Pts',(2.28834657299994,5.2,3.58724680899999));
#337507=CARTESIAN_POINT('Ctrl Pts',(2.28834657299994,2.2,3.58724680899999));
#337508=CARTESIAN_POINT('Ctrl Pts',(2.28870620399994,12.2,3.58889374999999));
#337509=CARTESIAN_POINT('Ctrl Pts',(2.28870620399994,5.2,3.58889374999999));
#337510=CARTESIAN_POINT('Ctrl Pts',(2.28870620399994,2.2,3.58889374999999));
#337511=CARTESIAN_POINT('Ctrl Pts',(2.28906489399994,12.2,3.59054546099999));
#337512=CARTESIAN_POINT('Ctrl Pts',(2.28906489399994,5.2,3.59054546099999));
#337513=CARTESIAN_POINT('Ctrl Pts',(2.28906489399994,2.2,3.59054546099999));
#337514=CARTESIAN_POINT('Ctrl Pts',(2.28942263299994,12.2,3.59220193799998));
#337515=CARTESIAN_POINT('Ctrl Pts',(2.28942263299994,5.2,3.59220193799998));
#337516=CARTESIAN_POINT('Ctrl Pts',(2.28942263299994,2.2,3.59220193799998));
#337517=CARTESIAN_POINT('Ctrl Pts',(2.28977940899994,12.2,3.59386317399998));
#337518=CARTESIAN_POINT('Ctrl Pts',(2.28977940899994,5.2,3.59386317399998));
#337519=CARTESIAN_POINT('Ctrl Pts',(2.28977940899994,2.2,3.59386317399998));
#337520=CARTESIAN_POINT('Ctrl Pts',(2.29013521099994,12.2,3.59552916399998));
#337521=CARTESIAN_POINT('Ctrl Pts',(2.29013521099994,5.2,3.59552916399998));
#337522=CARTESIAN_POINT('Ctrl Pts',(2.29013521099994,2.2,3.59552916399998));
#337523=CARTESIAN_POINT('Ctrl Pts',(2.29049002999994,12.2,3.59719990199999));
#337524=CARTESIAN_POINT('Ctrl Pts',(2.29049002999994,5.2,3.59719990199999));
#337525=CARTESIAN_POINT('Ctrl Pts',(2.29049002999994,2.2,3.59719990199999));
#337526=CARTESIAN_POINT('Ctrl Pts',(2.29084385299994,12.2,3.59887538099999));
#337527=CARTESIAN_POINT('Ctrl Pts',(2.29084385299994,5.2,3.59887538099999));
#337528=CARTESIAN_POINT('Ctrl Pts',(2.29084385299994,2.2,3.59887538099999));
#337529=CARTESIAN_POINT('Ctrl Pts',(2.29119666999994,12.2,3.60055559599999));
#337530=CARTESIAN_POINT('Ctrl Pts',(2.29119666999994,5.2,3.60055559599999));
#337531=CARTESIAN_POINT('Ctrl Pts',(2.29119666999994,2.2,3.60055559599999));
#337532=CARTESIAN_POINT('Ctrl Pts',(2.29154847199994,12.2,3.60224053999998));
#337533=CARTESIAN_POINT('Ctrl Pts',(2.29154847199994,5.2,3.60224053999998));
#337534=CARTESIAN_POINT('Ctrl Pts',(2.29154847199994,2.2,3.60224053999998));
#337535=CARTESIAN_POINT('Ctrl Pts',(2.29189924599994,12.2,3.60393020899998));
#337536=CARTESIAN_POINT('Ctrl Pts',(2.29189924599994,5.2,3.60393020899998));
#337537=CARTESIAN_POINT('Ctrl Pts',(2.29189924599994,2.2,3.60393020899998));
#337538=CARTESIAN_POINT('Ctrl Pts',(2.29224898299994,12.2,3.60562459499998));
#337539=CARTESIAN_POINT('Ctrl Pts',(2.29224898299994,5.2,3.60562459499998));
#337540=CARTESIAN_POINT('Ctrl Pts',(2.29224898299994,2.2,3.60562459499998));
#337541=CARTESIAN_POINT('Ctrl Pts',(2.29259767199994,12.2,3.60732369299999));
#337542=CARTESIAN_POINT('Ctrl Pts',(2.29259767199994,5.2,3.60732369299999));
#337543=CARTESIAN_POINT('Ctrl Pts',(2.29259767199994,2.2,3.60732369299999));
#337544=CARTESIAN_POINT('Ctrl Pts',(2.29294530199994,12.2,3.60902749699999));
#337545=CARTESIAN_POINT('Ctrl Pts',(2.29294530199994,5.2,3.60902749699999));
#337546=CARTESIAN_POINT('Ctrl Pts',(2.29294530199994,2.2,3.60902749699999));
#337547=CARTESIAN_POINT('Ctrl Pts',(2.29329186299994,12.2,3.61073600099999));
#337548=CARTESIAN_POINT('Ctrl Pts',(2.29329186299994,5.2,3.61073600099999));
#337549=CARTESIAN_POINT('Ctrl Pts',(2.29329186299994,2.2,3.61073600099999));
#337550=CARTESIAN_POINT('Ctrl Pts',(2.29363734499994,12.2,3.61244919999999));
#337551=CARTESIAN_POINT('Ctrl Pts',(2.29363734499994,5.2,3.61244919999999));
#337552=CARTESIAN_POINT('Ctrl Pts',(2.29363734499994,2.2,3.61244919999999));
#337553=CARTESIAN_POINT('Ctrl Pts',(2.29398173699995,12.2,3.61416708599998));
#337554=CARTESIAN_POINT('Ctrl Pts',(2.29398173699995,5.2,3.61416708599998));
#337555=CARTESIAN_POINT('Ctrl Pts',(2.29398173699995,2.2,3.61416708599998));
#337556=CARTESIAN_POINT('Ctrl Pts',(2.29432502699995,12.2,3.61588965499998));
#337557=CARTESIAN_POINT('Ctrl Pts',(2.29432502699995,5.2,3.61588965499998));
#337558=CARTESIAN_POINT('Ctrl Pts',(2.29432502699995,2.2,3.61588965499998));
#337559=CARTESIAN_POINT('Ctrl Pts',(2.29466720699994,12.2,3.61761689899998));
#337560=CARTESIAN_POINT('Ctrl Pts',(2.29466720699994,5.2,3.61761689899998));
#337561=CARTESIAN_POINT('Ctrl Pts',(2.29466720699994,2.2,3.61761689899998));
#337562=CARTESIAN_POINT('Ctrl Pts',(2.29500826599994,12.2,3.61934881399999));
#337563=CARTESIAN_POINT('Ctrl Pts',(2.29500826599994,5.2,3.61934881399999));
#337564=CARTESIAN_POINT('Ctrl Pts',(2.29500826599994,2.2,3.61934881399999));
#337565=CARTESIAN_POINT('Ctrl Pts',(2.29534819299994,12.2,3.62108539299999));
#337566=CARTESIAN_POINT('Ctrl Pts',(2.29534819299994,5.2,3.62108539299999));
#337567=CARTESIAN_POINT('Ctrl Pts',(2.29534819299994,2.2,3.62108539299999));
#337568=CARTESIAN_POINT('Ctrl Pts',(2.29568697699994,12.2,3.62282663099998));
#337569=CARTESIAN_POINT('Ctrl Pts',(2.29568697699994,5.2,3.62282663099998));
#337570=CARTESIAN_POINT('Ctrl Pts',(2.29568697699994,2.2,3.62282663099998));
#337571=CARTESIAN_POINT('Ctrl Pts',(2.29602460999994,12.2,3.62457252099999));
#337572=CARTESIAN_POINT('Ctrl Pts',(2.29602460999994,5.2,3.62457252099999));
#337573=CARTESIAN_POINT('Ctrl Pts',(2.29602460999994,2.2,3.62457252099999));
#337574=CARTESIAN_POINT('Ctrl Pts',(2.29636107999994,12.2,3.62632305699999));
#337575=CARTESIAN_POINT('Ctrl Pts',(2.29636107999994,5.2,3.62632305699999));
#337576=CARTESIAN_POINT('Ctrl Pts',(2.29636107999994,2.2,3.62632305699999));
#337577=CARTESIAN_POINT('Ctrl Pts',(2.29669637699994,12.2,3.62807823299998));
#337578=CARTESIAN_POINT('Ctrl Pts',(2.29669637699994,5.2,3.62807823299998));
#337579=CARTESIAN_POINT('Ctrl Pts',(2.29669637699994,2.2,3.62807823299998));
#337580=CARTESIAN_POINT('Ctrl Pts',(2.29703049199994,12.2,3.62983804499999));
#337581=CARTESIAN_POINT('Ctrl Pts',(2.29703049199994,5.2,3.62983804499999));
#337582=CARTESIAN_POINT('Ctrl Pts',(2.29703049199994,2.2,3.62983804499999));
#337583=CARTESIAN_POINT('Ctrl Pts',(2.29736341199994,12.2,3.63160248399998));
#337584=CARTESIAN_POINT('Ctrl Pts',(2.29736341199994,5.2,3.63160248399998));
#337585=CARTESIAN_POINT('Ctrl Pts',(2.29736341199994,2.2,3.63160248399998));
#337586=CARTESIAN_POINT('Ctrl Pts',(2.29769512999995,12.2,3.63337154599999));
#337587=CARTESIAN_POINT('Ctrl Pts',(2.29769512999995,5.2,3.63337154599999));
#337588=CARTESIAN_POINT('Ctrl Pts',(2.29769512999995,2.2,3.63337154599999));
#337589=CARTESIAN_POINT('Ctrl Pts',(2.29802563399994,12.2,3.63514522399999));
#337590=CARTESIAN_POINT('Ctrl Pts',(2.29802563399994,5.2,3.63514522399999));
#337591=CARTESIAN_POINT('Ctrl Pts',(2.29802563399994,2.2,3.63514522399999));
#337592=CARTESIAN_POINT('Ctrl Pts',(2.29835491399994,12.2,3.63692351199998));
#337593=CARTESIAN_POINT('Ctrl Pts',(2.29835491399994,5.2,3.63692351199998));
#337594=CARTESIAN_POINT('Ctrl Pts',(2.29835491399994,2.2,3.63692351199998));
#337595=CARTESIAN_POINT('Ctrl Pts',(2.29868296099994,12.2,3.63870640499999));
#337596=CARTESIAN_POINT('Ctrl Pts',(2.29868296099994,5.2,3.63870640499999));
#337597=CARTESIAN_POINT('Ctrl Pts',(2.29868296099994,2.2,3.63870640499999));
#337598=CARTESIAN_POINT('Ctrl Pts',(2.29900976199994,12.2,3.64049389599998));
#337599=CARTESIAN_POINT('Ctrl Pts',(2.29900976199994,5.2,3.64049389599998));
#337600=CARTESIAN_POINT('Ctrl Pts',(2.29900976199994,2.2,3.64049389599998));
#337601=CARTESIAN_POINT('Ctrl Pts',(2.29933531199995,12.2,3.64228597899999));
#337602=CARTESIAN_POINT('Ctrl Pts',(2.29933531199995,5.2,3.64228597899999));
#337603=CARTESIAN_POINT('Ctrl Pts',(2.29933531199995,2.2,3.64228597899999));
#337604=CARTESIAN_POINT('Ctrl Pts',(2.29965959599994,12.2,3.64408264899998));
#337605=CARTESIAN_POINT('Ctrl Pts',(2.29965959599994,5.2,3.64408264899998));
#337606=CARTESIAN_POINT('Ctrl Pts',(2.29965959599994,2.2,3.64408264899998));
#337607=CARTESIAN_POINT('Ctrl Pts',(2.29998260699994,12.2,3.64588389899998));
#337608=CARTESIAN_POINT('Ctrl Pts',(2.29998260699994,5.2,3.64588389899998));
#337609=CARTESIAN_POINT('Ctrl Pts',(2.29998260699994,2.2,3.64588389899998));
#337610=CARTESIAN_POINT('Ctrl Pts',(2.30030433499994,12.2,3.64768972399999));
#337611=CARTESIAN_POINT('Ctrl Pts',(2.30030433499994,5.2,3.64768972399999));
#337612=CARTESIAN_POINT('Ctrl Pts',(2.30030433499994,2.2,3.64768972399999));
#337613=CARTESIAN_POINT('Ctrl Pts',(2.30062476699994,12.2,3.64950011699998));
#337614=CARTESIAN_POINT('Ctrl Pts',(2.30062476699994,5.2,3.64950011699998));
#337615=CARTESIAN_POINT('Ctrl Pts',(2.30062476699994,2.2,3.64950011699998));
#337616=CARTESIAN_POINT('Ctrl Pts',(2.30094389699994,12.2,3.65131507199998));
#337617=CARTESIAN_POINT('Ctrl Pts',(2.30094389699994,5.2,3.65131507199998));
#337618=CARTESIAN_POINT('Ctrl Pts',(2.30094389699994,2.2,3.65131507199998));
#337619=CARTESIAN_POINT('Ctrl Pts',(2.30126171299994,12.2,3.65313458299998));
#337620=CARTESIAN_POINT('Ctrl Pts',(2.30126171299994,5.2,3.65313458299998));
#337621=CARTESIAN_POINT('Ctrl Pts',(2.30126171299994,2.2,3.65313458299998));
#337622=CARTESIAN_POINT('Ctrl Pts',(2.30157820499994,12.2,3.65495864499999));
#337623=CARTESIAN_POINT('Ctrl Pts',(2.30157820499994,5.2,3.65495864499999));
#337624=CARTESIAN_POINT('Ctrl Pts',(2.30157820499994,2.2,3.65495864499999));
#337625=CARTESIAN_POINT('Ctrl Pts',(2.30189336399994,12.2,3.65678724999999));
#337626=CARTESIAN_POINT('Ctrl Pts',(2.30189336399994,5.2,3.65678724999999));
#337627=CARTESIAN_POINT('Ctrl Pts',(2.30189336399994,2.2,3.65678724999999));
#337628=CARTESIAN_POINT('Ctrl Pts',(2.30220717999994,12.2,3.65862039399998));
#337629=CARTESIAN_POINT('Ctrl Pts',(2.30220717999994,5.2,3.65862039399998));
#337630=CARTESIAN_POINT('Ctrl Pts',(2.30220717999994,2.2,3.65862039399998));
#337631=CARTESIAN_POINT('Ctrl Pts',(2.30251964299994,12.2,3.66045806999999));
#337632=CARTESIAN_POINT('Ctrl Pts',(2.30251964299994,5.2,3.66045806999999));
#337633=CARTESIAN_POINT('Ctrl Pts',(2.30251964299994,2.2,3.66045806999999));
#337634=CARTESIAN_POINT('Ctrl Pts',(2.30283074299994,12.2,3.66230027199999));
#337635=CARTESIAN_POINT('Ctrl Pts',(2.30283074299994,5.2,3.66230027199999));
#337636=CARTESIAN_POINT('Ctrl Pts',(2.30283074299994,2.2,3.66230027199999));
#337637=CARTESIAN_POINT('Ctrl Pts',(2.30314047099994,12.2,3.66414699399999));
#337638=CARTESIAN_POINT('Ctrl Pts',(2.30314047099994,5.2,3.66414699399999));
#337639=CARTESIAN_POINT('Ctrl Pts',(2.30314047099994,2.2,3.66414699399999));
#337640=CARTESIAN_POINT('Ctrl Pts',(2.30344881599994,12.2,3.66599822899998));
#337641=CARTESIAN_POINT('Ctrl Pts',(2.30344881599994,5.2,3.66599822899998));
#337642=CARTESIAN_POINT('Ctrl Pts',(2.30344881599994,2.2,3.66599822899998));
#337643=CARTESIAN_POINT('Ctrl Pts',(2.30375576999994,12.2,3.66785397299999));
#337644=CARTESIAN_POINT('Ctrl Pts',(2.30375576999994,5.2,3.66785397299999));
#337645=CARTESIAN_POINT('Ctrl Pts',(2.30375576999994,2.2,3.66785397299999));
#337646=CARTESIAN_POINT('Ctrl Pts',(2.30406132199994,12.2,3.66971421799998));
#337647=CARTESIAN_POINT('Ctrl Pts',(2.30406132199994,5.2,3.66971421799998));
#337648=CARTESIAN_POINT('Ctrl Pts',(2.30406132199994,2.2,3.66971421799998));
#337649=CARTESIAN_POINT('Ctrl Pts',(2.30436546299994,12.2,3.67157895999998));
#337650=CARTESIAN_POINT('Ctrl Pts',(2.30436546299994,5.2,3.67157895999998));
#337651=CARTESIAN_POINT('Ctrl Pts',(2.30436546299994,2.2,3.67157895999998));
#337652=CARTESIAN_POINT('Ctrl Pts',(2.30466818299994,12.2,3.67344819099999));
#337653=CARTESIAN_POINT('Ctrl Pts',(2.30466818299994,5.2,3.67344819099999));
#337654=CARTESIAN_POINT('Ctrl Pts',(2.30466818299994,2.2,3.67344819099999));
#337655=CARTESIAN_POINT('Ctrl Pts',(2.30496947299994,12.2,3.67532190499999));
#337656=CARTESIAN_POINT('Ctrl Pts',(2.30496947299994,5.2,3.67532190499999));
#337657=CARTESIAN_POINT('Ctrl Pts',(2.30496947299994,2.2,3.67532190499999));
#337658=CARTESIAN_POINT('Ctrl Pts',(2.30526932399994,12.2,3.67720009799999));
#337659=CARTESIAN_POINT('Ctrl Pts',(2.30526932399994,5.2,3.67720009799999));
#337660=CARTESIAN_POINT('Ctrl Pts',(2.30526932399994,2.2,3.67720009799999));
#337661=CARTESIAN_POINT('Ctrl Pts',(2.30556772399995,12.2,3.67908276099998));
#337662=CARTESIAN_POINT('Ctrl Pts',(2.30556772399995,5.2,3.67908276099998));
#337663=CARTESIAN_POINT('Ctrl Pts',(2.30556772399995,2.2,3.67908276099998));
#337664=CARTESIAN_POINT('Ctrl Pts',(2.30586466499994,12.2,3.68096988999999));
#337665=CARTESIAN_POINT('Ctrl Pts',(2.30586466499994,5.2,3.68096988999999));
#337666=CARTESIAN_POINT('Ctrl Pts',(2.30586466499994,2.2,3.68096988999999));
#337667=CARTESIAN_POINT('Ctrl Pts',(2.30616013899994,12.2,3.68286147899998));
#337668=CARTESIAN_POINT('Ctrl Pts',(2.30616013899994,5.2,3.68286147899998));
#337669=CARTESIAN_POINT('Ctrl Pts',(2.30616013899994,2.2,3.68286147899998));
#337670=CARTESIAN_POINT('Ctrl Pts',(2.30645413399994,12.2,3.68475751999998));
#337671=CARTESIAN_POINT('Ctrl Pts',(2.30645413399994,5.2,3.68475751999998));
#337672=CARTESIAN_POINT('Ctrl Pts',(2.30645413399994,2.2,3.68475751999998));
#337673=CARTESIAN_POINT('Ctrl Pts',(2.30674664199995,12.2,3.68665800899999));
#337674=CARTESIAN_POINT('Ctrl Pts',(2.30674664199995,5.2,3.68665800899999));
#337675=CARTESIAN_POINT('Ctrl Pts',(2.30674664199995,2.2,3.68665800899999));
#337676=CARTESIAN_POINT('Ctrl Pts',(2.30703765199994,12.2,3.68856293899999));
#337677=CARTESIAN_POINT('Ctrl Pts',(2.30703765199994,5.2,3.68856293899999));
#337678=CARTESIAN_POINT('Ctrl Pts',(2.30703765199994,2.2,3.68856293899999));
#337679=CARTESIAN_POINT('Ctrl Pts',(2.30732715699994,12.2,3.69047230399998));
#337680=CARTESIAN_POINT('Ctrl Pts',(2.30732715699994,5.2,3.69047230399998));
#337681=CARTESIAN_POINT('Ctrl Pts',(2.30732715699994,2.2,3.69047230399998));
#337682=CARTESIAN_POINT('Ctrl Pts',(2.30761514599994,12.2,3.69238609799999));
#337683=CARTESIAN_POINT('Ctrl Pts',(2.30761514599994,5.2,3.69238609799999));
#337684=CARTESIAN_POINT('Ctrl Pts',(2.30761514599994,2.2,3.69238609799999));
#337685=CARTESIAN_POINT('Ctrl Pts',(2.30790160999994,12.2,3.69430431499998));
#337686=CARTESIAN_POINT('Ctrl Pts',(2.30790160999994,5.2,3.69430431499998));
#337687=CARTESIAN_POINT('Ctrl Pts',(2.30790160999994,2.2,3.69430431499998));
#337688=CARTESIAN_POINT('Ctrl Pts',(2.30818653999994,12.2,3.69622694799999));
#337689=CARTESIAN_POINT('Ctrl Pts',(2.30818653999994,5.2,3.69622694799999));
#337690=CARTESIAN_POINT('Ctrl Pts',(2.30818653999994,2.2,3.69622694799999));
#337691=CARTESIAN_POINT('Ctrl Pts',(2.30846992599994,12.2,3.69815399199998));
#337692=CARTESIAN_POINT('Ctrl Pts',(2.30846992599994,5.2,3.69815399199998));
#337693=CARTESIAN_POINT('Ctrl Pts',(2.30846992599994,2.2,3.69815399199998));
#337694=CARTESIAN_POINT('Ctrl Pts',(2.30875175899994,12.2,3.70008544099999));
#337695=CARTESIAN_POINT('Ctrl Pts',(2.30875175899994,5.2,3.70008544099999));
#337696=CARTESIAN_POINT('Ctrl Pts',(2.30875175899994,2.2,3.70008544099999));
#337697=CARTESIAN_POINT('Ctrl Pts',(2.30903203099994,12.2,3.70202128799999));
#337698=CARTESIAN_POINT('Ctrl Pts',(2.30903203099994,5.2,3.70202128799999));
#337699=CARTESIAN_POINT('Ctrl Pts',(2.30903203099994,2.2,3.70202128799999));
#337700=CARTESIAN_POINT('Ctrl Pts',(2.30931073099994,12.2,3.70396152699998));
#337701=CARTESIAN_POINT('Ctrl Pts',(2.30931073099994,5.2,3.70396152699998));
#337702=CARTESIAN_POINT('Ctrl Pts',(2.30931073099994,2.2,3.70396152699998));
#337703=CARTESIAN_POINT('Ctrl Pts',(2.30958784999994,12.2,3.70590615299999));
#337704=CARTESIAN_POINT('Ctrl Pts',(2.30958784999994,5.2,3.70590615299999));
#337705=CARTESIAN_POINT('Ctrl Pts',(2.30958784999994,2.2,3.70590615299999));
#337706=CARTESIAN_POINT('Ctrl Pts',(2.30986337899994,12.2,3.70785515799999));
#337707=CARTESIAN_POINT('Ctrl Pts',(2.30986337899994,5.2,3.70785515799999));
#337708=CARTESIAN_POINT('Ctrl Pts',(2.30986337899994,2.2,3.70785515799999));
#337709=CARTESIAN_POINT('Ctrl Pts',(2.31013730899994,12.2,3.70980853799999));
#337710=CARTESIAN_POINT('Ctrl Pts',(2.31013730899994,5.2,3.70980853799999));
#337711=CARTESIAN_POINT('Ctrl Pts',(2.31013730899994,2.2,3.70980853799999));
#337712=CARTESIAN_POINT('Ctrl Pts',(2.31040963199994,12.2,3.71176628599999));
#337713=CARTESIAN_POINT('Ctrl Pts',(2.31040963199994,5.2,3.71176628599999));
#337714=CARTESIAN_POINT('Ctrl Pts',(2.31040963199994,2.2,3.71176628599999));
#337715=CARTESIAN_POINT('Ctrl Pts',(2.31068033599994,12.2,3.71372839499998));
#337716=CARTESIAN_POINT('Ctrl Pts',(2.31068033599994,5.2,3.71372839499998));
#337717=CARTESIAN_POINT('Ctrl Pts',(2.31068033599994,2.2,3.71372839499998));
#337718=CARTESIAN_POINT('Ctrl Pts',(2.31094941499994,12.2,3.71569485999999));
#337719=CARTESIAN_POINT('Ctrl Pts',(2.31094941499994,5.2,3.71569485999999));
#337720=CARTESIAN_POINT('Ctrl Pts',(2.31094941499994,2.2,3.71569485999999));
#337721=CARTESIAN_POINT('Ctrl Pts',(2.31121685899994,12.2,3.71766567399998));
#337722=CARTESIAN_POINT('Ctrl Pts',(2.31121685899994,5.2,3.71766567399998));
#337723=CARTESIAN_POINT('Ctrl Pts',(2.31121685899994,2.2,3.71766567399998));
#337724=CARTESIAN_POINT('Ctrl Pts',(2.31148265799995,12.2,3.71964083199998));
#337725=CARTESIAN_POINT('Ctrl Pts',(2.31148265799995,5.2,3.71964083199998));
#337726=CARTESIAN_POINT('Ctrl Pts',(2.31148265799995,2.2,3.71964083199998));
#337727=CARTESIAN_POINT('Ctrl Pts',(2.31174680299994,12.2,3.72162032699999));
#337728=CARTESIAN_POINT('Ctrl Pts',(2.31174680299994,5.2,3.72162032699999));
#337729=CARTESIAN_POINT('Ctrl Pts',(2.31174680299994,2.2,3.72162032699999));
#337730=CARTESIAN_POINT('Ctrl Pts',(2.31200928699994,12.2,3.72360415299998));
#337731=CARTESIAN_POINT('Ctrl Pts',(2.31200928699994,5.2,3.72360415299998));
#337732=CARTESIAN_POINT('Ctrl Pts',(2.31200928699994,2.2,3.72360415299998));
#337733=CARTESIAN_POINT('Ctrl Pts',(2.31227009899994,12.2,3.72559230399998));
#337734=CARTESIAN_POINT('Ctrl Pts',(2.31227009899994,5.2,3.72559230399998));
#337735=CARTESIAN_POINT('Ctrl Pts',(2.31227009899994,2.2,3.72559230399998));
#337736=CARTESIAN_POINT('Ctrl Pts',(2.31252923099994,12.2,3.72758477399999));
#337737=CARTESIAN_POINT('Ctrl Pts',(2.31252923099994,5.2,3.72758477399999));
#337738=CARTESIAN_POINT('Ctrl Pts',(2.31252923099994,2.2,3.72758477399999));
#337739=CARTESIAN_POINT('Ctrl Pts',(2.31278667299994,12.2,3.72958155599999));
#337740=CARTESIAN_POINT('Ctrl Pts',(2.31278667299994,5.2,3.72958155599999));
#337741=CARTESIAN_POINT('Ctrl Pts',(2.31278667299994,2.2,3.72958155599999));
#337742=CARTESIAN_POINT('Ctrl Pts',(2.31304241599994,12.2,3.73158264599999));
#337743=CARTESIAN_POINT('Ctrl Pts',(2.31304241599994,5.2,3.73158264599999));
#337744=CARTESIAN_POINT('Ctrl Pts',(2.31304241599994,2.2,3.73158264599999));
#337745=CARTESIAN_POINT('Ctrl Pts',(2.31329645199994,12.2,3.73358803499999));
#337746=CARTESIAN_POINT('Ctrl Pts',(2.31329645199994,5.2,3.73358803499999));
#337747=CARTESIAN_POINT('Ctrl Pts',(2.31329645199994,2.2,3.73358803499999));
#337748=CARTESIAN_POINT('Ctrl Pts',(2.31354877299994,12.2,3.73559771899998));
#337749=CARTESIAN_POINT('Ctrl Pts',(2.31354877299994,5.2,3.73559771899998));
#337750=CARTESIAN_POINT('Ctrl Pts',(2.31354877299994,2.2,3.73559771899998));
#337751=CARTESIAN_POINT('Ctrl Pts',(2.31379936899994,12.2,3.73761168999999));
#337752=CARTESIAN_POINT('Ctrl Pts',(2.31379936899994,5.2,3.73761168999999));
#337753=CARTESIAN_POINT('Ctrl Pts',(2.31379936899994,2.2,3.73761168999999));
#337754=CARTESIAN_POINT('Ctrl Pts',(2.31404823199994,12.2,3.73962994399999));
#337755=CARTESIAN_POINT('Ctrl Pts',(2.31404823199994,5.2,3.73962994399999));
#337756=CARTESIAN_POINT('Ctrl Pts',(2.31404823199994,2.2,3.73962994399999));
#337757=CARTESIAN_POINT('Ctrl Pts',(2.31429535099994,12.2,3.74165247399999));
#337758=CARTESIAN_POINT('Ctrl Pts',(2.31429535099994,5.2,3.74165247399999));
#337759=CARTESIAN_POINT('Ctrl Pts',(2.31429535099994,2.2,3.74165247399999));
#337760=CARTESIAN_POINT('Ctrl Pts',(2.31454071899994,12.2,3.74367927299998));
#337761=CARTESIAN_POINT('Ctrl Pts',(2.31454071899994,5.2,3.74367927299998));
#337762=CARTESIAN_POINT('Ctrl Pts',(2.31454071899994,2.2,3.74367927299998));
#337763=CARTESIAN_POINT('Ctrl Pts',(2.31478432699994,12.2,3.74571033499999));
#337764=CARTESIAN_POINT('Ctrl Pts',(2.31478432699994,5.2,3.74571033499999));
#337765=CARTESIAN_POINT('Ctrl Pts',(2.31478432699994,2.2,3.74571033499999));
#337766=CARTESIAN_POINT('Ctrl Pts',(2.31502616799994,12.2,3.74774565599999));
#337767=CARTESIAN_POINT('Ctrl Pts',(2.31502616799994,5.2,3.74774565599999));
#337768=CARTESIAN_POINT('Ctrl Pts',(2.31502616799994,2.2,3.74774565599999));
#337769=CARTESIAN_POINT('Ctrl Pts',(2.31526622999994,12.2,3.74978522699998));
#337770=CARTESIAN_POINT('Ctrl Pts',(2.31526622999994,5.2,3.74978522699998));
#337771=CARTESIAN_POINT('Ctrl Pts',(2.31526622999994,2.2,3.74978522699998));
#337772=CARTESIAN_POINT('Ctrl Pts',(2.31550450599994,12.2,3.75182904199999));
#337773=CARTESIAN_POINT('Ctrl Pts',(2.31550450599994,5.2,3.75182904199999));
#337774=CARTESIAN_POINT('Ctrl Pts',(2.31550450599994,2.2,3.75182904199999));
#337775=CARTESIAN_POINT('Ctrl Pts',(2.31574098699994,12.2,3.75387709699999));
#337776=CARTESIAN_POINT('Ctrl Pts',(2.31574098699994,5.2,3.75387709699999));
#337777=CARTESIAN_POINT('Ctrl Pts',(2.31574098699994,2.2,3.75387709699999));
#337778=CARTESIAN_POINT('Ctrl Pts',(2.31597566499994,12.2,3.75592938499998));
#337779=CARTESIAN_POINT('Ctrl Pts',(2.31597566499994,5.2,3.75592938499998));
#337780=CARTESIAN_POINT('Ctrl Pts',(2.31597566499994,2.2,3.75592938499998));
#337781=CARTESIAN_POINT('Ctrl Pts',(2.31620852999994,12.2,3.75798589899999));
#337782=CARTESIAN_POINT('Ctrl Pts',(2.31620852999994,5.2,3.75798589899999));
#337783=CARTESIAN_POINT('Ctrl Pts',(2.31620852999994,2.2,3.75798589899999));
#337784=CARTESIAN_POINT('Ctrl Pts',(2.31643957499994,12.2,3.76004663299998));
#337785=CARTESIAN_POINT('Ctrl Pts',(2.31643957499994,5.2,3.76004663299998));
#337786=CARTESIAN_POINT('Ctrl Pts',(2.31643957499994,2.2,3.76004663299998));
#337787=CARTESIAN_POINT('Ctrl Pts',(2.31666879099994,12.2,3.76211158199999));
#337788=CARTESIAN_POINT('Ctrl Pts',(2.31666879099994,5.2,3.76211158199999));
#337789=CARTESIAN_POINT('Ctrl Pts',(2.31666879099994,2.2,3.76211158199999));
#337790=CARTESIAN_POINT('Ctrl Pts',(2.31689616899994,12.2,3.76418073899998));
#337791=CARTESIAN_POINT('Ctrl Pts',(2.31689616899994,5.2,3.76418073899998));
#337792=CARTESIAN_POINT('Ctrl Pts',(2.31689616899994,2.2,3.76418073899998));
#337793=CARTESIAN_POINT('Ctrl Pts',(2.31712169999994,12.2,3.76625409599999));
#337794=CARTESIAN_POINT('Ctrl Pts',(2.31712169999994,5.2,3.76625409599999));
#337795=CARTESIAN_POINT('Ctrl Pts',(2.31712169999994,2.2,3.76625409599999));
#337796=CARTESIAN_POINT('Ctrl Pts',(2.31734537599994,12.2,3.76833164999999));
#337797=CARTESIAN_POINT('Ctrl Pts',(2.31734537599994,5.2,3.76833164999999));
#337798=CARTESIAN_POINT('Ctrl Pts',(2.31734537599994,2.2,3.76833164999999));
#337799=CARTESIAN_POINT('Ctrl Pts',(2.31756718999994,12.2,3.77041339299999));
#337800=CARTESIAN_POINT('Ctrl Pts',(2.31756718999994,5.2,3.77041339299999));
#337801=CARTESIAN_POINT('Ctrl Pts',(2.31756718999994,2.2,3.77041339299999));
#337802=CARTESIAN_POINT('Ctrl Pts',(2.31778713099994,12.2,3.77249931899998));
#337803=CARTESIAN_POINT('Ctrl Pts',(2.31778713099994,5.2,3.77249931899998));
#337804=CARTESIAN_POINT('Ctrl Pts',(2.31778713099994,2.2,3.77249931899998));
#337805=CARTESIAN_POINT('Ctrl Pts',(2.31800519199994,12.2,3.77458942199999));
#337806=CARTESIAN_POINT('Ctrl Pts',(2.31800519199994,5.2,3.77458942199999));
#337807=CARTESIAN_POINT('Ctrl Pts',(2.31800519199994,2.2,3.77458942199999));
#337808=CARTESIAN_POINT('Ctrl Pts',(2.31822136499995,12.2,3.77668369599998));
#337809=CARTESIAN_POINT('Ctrl Pts',(2.31822136499995,5.2,3.77668369599998));
#337810=CARTESIAN_POINT('Ctrl Pts',(2.31822136499995,2.2,3.77668369599998));
#337811=CARTESIAN_POINT('Ctrl Pts',(2.31843563999994,12.2,3.77878213499999));
#337812=CARTESIAN_POINT('Ctrl Pts',(2.31843563999994,5.2,3.77878213499999));
#337813=CARTESIAN_POINT('Ctrl Pts',(2.31843563999994,2.2,3.77878213499999));
#337814=CARTESIAN_POINT('Ctrl Pts',(2.31864800899995,12.2,3.78088473199998));
#337815=CARTESIAN_POINT('Ctrl Pts',(2.31864800899995,5.2,3.78088473199998));
#337816=CARTESIAN_POINT('Ctrl Pts',(2.31864800899995,2.2,3.78088473199998));
#337817=CARTESIAN_POINT('Ctrl Pts',(2.31885846499994,12.2,3.78299148099998));
#337818=CARTESIAN_POINT('Ctrl Pts',(2.31885846499994,5.2,3.78299148099998));
#337819=CARTESIAN_POINT('Ctrl Pts',(2.31885846499994,2.2,3.78299148099998));
#337820=CARTESIAN_POINT('Ctrl Pts',(2.31906699899994,12.2,3.78510237599999));
#337821=CARTESIAN_POINT('Ctrl Pts',(2.31906699899994,5.2,3.78510237599999));
#337822=CARTESIAN_POINT('Ctrl Pts',(2.31906699899994,2.2,3.78510237599999));
#337823=CARTESIAN_POINT('Ctrl Pts',(2.31927360099994,12.2,3.78721741099999));
#337824=CARTESIAN_POINT('Ctrl Pts',(2.31927360099994,5.2,3.78721741099999));
#337825=CARTESIAN_POINT('Ctrl Pts',(2.31927360099994,2.2,3.78721741099999));
#337826=CARTESIAN_POINT('Ctrl Pts',(2.31947826499994,12.2,3.78933657999998));
#337827=CARTESIAN_POINT('Ctrl Pts',(2.31947826499994,5.2,3.78933657999998));
#337828=CARTESIAN_POINT('Ctrl Pts',(2.31947826499994,2.2,3.78933657999998));
#337829=CARTESIAN_POINT('Ctrl Pts',(2.31968098099994,12.2,3.79145987599999));
#337830=CARTESIAN_POINT('Ctrl Pts',(2.31968098099994,5.2,3.79145987599999));
#337831=CARTESIAN_POINT('Ctrl Pts',(2.31968098099994,2.2,3.79145987599999));
#337832=CARTESIAN_POINT('Ctrl Pts',(2.31988174199994,12.2,3.79358729299998));
#337833=CARTESIAN_POINT('Ctrl Pts',(2.31988174199994,5.2,3.79358729299998));
#337834=CARTESIAN_POINT('Ctrl Pts',(2.31988174199994,2.2,3.79358729299998));
#337835=CARTESIAN_POINT('Ctrl Pts',(2.32008053999994,12.2,3.79571882499998));
#337836=CARTESIAN_POINT('Ctrl Pts',(2.32008053999994,5.2,3.79571882499998));
#337837=CARTESIAN_POINT('Ctrl Pts',(2.32008053999994,2.2,3.79571882499998));
#337838=CARTESIAN_POINT('Ctrl Pts',(2.32027736599994,12.2,3.79785446599998));
#337839=CARTESIAN_POINT('Ctrl Pts',(2.32027736599994,5.2,3.79785446599998));
#337840=CARTESIAN_POINT('Ctrl Pts',(2.32027736599994,2.2,3.79785446599998));
#337841=CARTESIAN_POINT('Ctrl Pts',(2.32047221099994,12.2,3.79999420999999));
#337842=CARTESIAN_POINT('Ctrl Pts',(2.32047221099994,5.2,3.79999420999999));
#337843=CARTESIAN_POINT('Ctrl Pts',(2.32047221099994,2.2,3.79999420999999));
#337844=CARTESIAN_POINT('Ctrl Pts',(2.32066506899994,12.2,3.80213804899999));
#337845=CARTESIAN_POINT('Ctrl Pts',(2.32066506899994,5.2,3.80213804899999));
#337846=CARTESIAN_POINT('Ctrl Pts',(2.32066506899994,2.2,3.80213804899999));
#337847=CARTESIAN_POINT('Ctrl Pts',(2.32085592999994,12.2,3.80428597799998));
#337848=CARTESIAN_POINT('Ctrl Pts',(2.32085592999994,5.2,3.80428597799998));
#337849=CARTESIAN_POINT('Ctrl Pts',(2.32085592999994,2.2,3.80428597799998));
#337850=CARTESIAN_POINT('Ctrl Pts',(2.32104478499994,12.2,3.80643799199999));
#337851=CARTESIAN_POINT('Ctrl Pts',(2.32104478499994,5.2,3.80643799199999));
#337852=CARTESIAN_POINT('Ctrl Pts',(2.32104478499994,2.2,3.80643799199999));
#337853=CARTESIAN_POINT('Ctrl Pts',(2.32123162999994,12.2,3.80859408399999));
#337854=CARTESIAN_POINT('Ctrl Pts',(2.32123162999994,5.2,3.80859408399999));
#337855=CARTESIAN_POINT('Ctrl Pts',(2.32123162999994,2.2,3.80859408399999));
#337856=CARTESIAN_POINT('Ctrl Pts',(2.32141645199994,12.2,3.81075424599998));
#337857=CARTESIAN_POINT('Ctrl Pts',(2.32141645199994,5.2,3.81075424599998));
#337858=CARTESIAN_POINT('Ctrl Pts',(2.32141645199994,2.2,3.81075424599998));
#337859=CARTESIAN_POINT('Ctrl Pts',(2.32159924599994,12.2,3.81291847499998));
#337860=CARTESIAN_POINT('Ctrl Pts',(2.32159924599994,5.2,3.81291847499998));
#337861=CARTESIAN_POINT('Ctrl Pts',(2.32159924599994,2.2,3.81291847499998));
#337862=CARTESIAN_POINT('Ctrl Pts',(2.32178000199994,12.2,3.81508676099998));
#337863=CARTESIAN_POINT('Ctrl Pts',(2.32178000199994,5.2,3.81508676099998));
#337864=CARTESIAN_POINT('Ctrl Pts',(2.32178000199994,2.2,3.81508676099998));
#337865=CARTESIAN_POINT('Ctrl Pts',(2.32195871499994,12.2,3.81725910099998));
#337866=CARTESIAN_POINT('Ctrl Pts',(2.32195871499994,5.2,3.81725910099998));
#337867=CARTESIAN_POINT('Ctrl Pts',(2.32195871499994,2.2,3.81725910099998));
#337868=CARTESIAN_POINT('Ctrl Pts',(2.32213537299994,12.2,3.81943548699999));
#337869=CARTESIAN_POINT('Ctrl Pts',(2.32213537299994,5.2,3.81943548699999));
#337870=CARTESIAN_POINT('Ctrl Pts',(2.32213537299994,2.2,3.81943548699999));
#337871=CARTESIAN_POINT('Ctrl Pts',(2.32230997199994,12.2,3.82161591299998));
#337872=CARTESIAN_POINT('Ctrl Pts',(2.32230997199994,5.2,3.82161591299998));
#337873=CARTESIAN_POINT('Ctrl Pts',(2.32230997199994,2.2,3.82161591299998));
#337874=CARTESIAN_POINT('Ctrl Pts',(2.32248249999994,12.2,3.82380037299999));
#337875=CARTESIAN_POINT('Ctrl Pts',(2.32248249999994,5.2,3.82380037299999));
#337876=CARTESIAN_POINT('Ctrl Pts',(2.32248249999994,2.2,3.82380037299999));
#337877=CARTESIAN_POINT('Ctrl Pts',(2.32265295199995,12.2,3.82598886199998));
#337878=CARTESIAN_POINT('Ctrl Pts',(2.32265295199995,5.2,3.82598886199998));
#337879=CARTESIAN_POINT('Ctrl Pts',(2.32265295199995,2.2,3.82598886199998));
#337880=CARTESIAN_POINT('Ctrl Pts',(2.32282131999995,12.2,3.82818137199998));
#337881=CARTESIAN_POINT('Ctrl Pts',(2.32282131999995,5.2,3.82818137199998));
#337882=CARTESIAN_POINT('Ctrl Pts',(2.32282131999995,2.2,3.82818137199998));
#337883=CARTESIAN_POINT('Ctrl Pts',(2.32298759399994,12.2,3.83037789599998));
#337884=CARTESIAN_POINT('Ctrl Pts',(2.32298759399994,5.2,3.83037789599998));
#337885=CARTESIAN_POINT('Ctrl Pts',(2.32298759399994,2.2,3.83037789599998));
#337886=CARTESIAN_POINT('Ctrl Pts',(2.32315176699994,12.2,3.83257843099998));
#337887=CARTESIAN_POINT('Ctrl Pts',(2.32315176699994,5.2,3.83257843099998));
#337888=CARTESIAN_POINT('Ctrl Pts',(2.32315176699994,2.2,3.83257843099998));
#337889=CARTESIAN_POINT('Ctrl Pts',(2.32331383199994,12.2,3.83478296699998));
#337890=CARTESIAN_POINT('Ctrl Pts',(2.32331383199994,5.2,3.83478296699998));
#337891=CARTESIAN_POINT('Ctrl Pts',(2.32331383199994,2.2,3.83478296699998));
#337892=CARTESIAN_POINT('Ctrl Pts',(2.32347378099994,12.2,3.83699150099999));
#337893=CARTESIAN_POINT('Ctrl Pts',(2.32347378099994,5.2,3.83699150099999));
#337894=CARTESIAN_POINT('Ctrl Pts',(2.32347378099994,2.2,3.83699150099999));
#337895=CARTESIAN_POINT('Ctrl Pts',(2.32363160599994,12.2,3.83920402399998));
#337896=CARTESIAN_POINT('Ctrl Pts',(2.32363160599994,5.2,3.83920402399998));
#337897=CARTESIAN_POINT('Ctrl Pts',(2.32363160599994,2.2,3.83920402399998));
#337898=CARTESIAN_POINT('Ctrl Pts',(2.32378729899994,12.2,3.84142053199999));
#337899=CARTESIAN_POINT('Ctrl Pts',(2.32378729899994,5.2,3.84142053199999));
#337900=CARTESIAN_POINT('Ctrl Pts',(2.32378729899994,2.2,3.84142053199999));
#337901=CARTESIAN_POINT('Ctrl Pts',(2.32394085099994,12.2,3.84364101799999));
#337902=CARTESIAN_POINT('Ctrl Pts',(2.32394085099994,5.2,3.84364101799999));
#337903=CARTESIAN_POINT('Ctrl Pts',(2.32394085099994,2.2,3.84364101799999));
#337904=CARTESIAN_POINT('Ctrl Pts',(2.32409225599994,12.2,3.84586547499998));
#337905=CARTESIAN_POINT('Ctrl Pts',(2.32409225599994,5.2,3.84586547499998));
#337906=CARTESIAN_POINT('Ctrl Pts',(2.32409225599994,2.2,3.84586547499998));
#337907=CARTESIAN_POINT('Ctrl Pts',(2.32424150599994,12.2,3.84809389699999));
#337908=CARTESIAN_POINT('Ctrl Pts',(2.32424150599994,5.2,3.84809389699999));
#337909=CARTESIAN_POINT('Ctrl Pts',(2.32424150599994,2.2,3.84809389699999));
#337910=CARTESIAN_POINT('Ctrl Pts',(2.32438859199994,12.2,3.85032627899999));
#337911=CARTESIAN_POINT('Ctrl Pts',(2.32438859199994,5.2,3.85032627899999));
#337912=CARTESIAN_POINT('Ctrl Pts',(2.32438859199994,2.2,3.85032627899999));
#337913=CARTESIAN_POINT('Ctrl Pts',(2.32453350799994,12.2,3.85256261199999));
#337914=CARTESIAN_POINT('Ctrl Pts',(2.32453350799994,5.2,3.85256261199999));
#337915=CARTESIAN_POINT('Ctrl Pts',(2.32453350799994,2.2,3.85256261199999));
#337916=CARTESIAN_POINT('Ctrl Pts',(2.32467624499994,12.2,3.85480289399998));
#337917=CARTESIAN_POINT('Ctrl Pts',(2.32467624499994,5.2,3.85480289399998));
#337918=CARTESIAN_POINT('Ctrl Pts',(2.32467624499994,2.2,3.85480289399998));
#337919=CARTESIAN_POINT('Ctrl Pts',(2.32481679599994,12.2,3.85704711399999));
#337920=CARTESIAN_POINT('Ctrl Pts',(2.32481679599994,5.2,3.85704711399999));
#337921=CARTESIAN_POINT('Ctrl Pts',(2.32481679599994,2.2,3.85704711399999));
#337922=CARTESIAN_POINT('Ctrl Pts',(2.32495515299994,12.2,3.85929526899999));
#337923=CARTESIAN_POINT('Ctrl Pts',(2.32495515299994,5.2,3.85929526899999));
#337924=CARTESIAN_POINT('Ctrl Pts',(2.32495515299994,2.2,3.85929526899999));
#337925=CARTESIAN_POINT('Ctrl Pts',(2.32509130799994,12.2,3.86154735199998));
#337926=CARTESIAN_POINT('Ctrl Pts',(2.32509130799994,5.2,3.86154735199998));
#337927=CARTESIAN_POINT('Ctrl Pts',(2.32509130799994,2.2,3.86154735199998));
#337928=CARTESIAN_POINT('Ctrl Pts',(2.32522525399994,12.2,3.86380335599998));
#337929=CARTESIAN_POINT('Ctrl Pts',(2.32522525399994,5.2,3.86380335599998));
#337930=CARTESIAN_POINT('Ctrl Pts',(2.32522525399994,2.2,3.86380335599998));
#337931=CARTESIAN_POINT('Ctrl Pts',(2.32535698399994,12.2,3.86606327499998));
#337932=CARTESIAN_POINT('Ctrl Pts',(2.32535698399994,5.2,3.86606327499998));
#337933=CARTESIAN_POINT('Ctrl Pts',(2.32535698399994,2.2,3.86606327499998));
#337934=CARTESIAN_POINT('Ctrl Pts',(2.32548648899995,12.2,3.86832710299998));
#337935=CARTESIAN_POINT('Ctrl Pts',(2.32548648899995,5.2,3.86832710299998));
#337936=CARTESIAN_POINT('Ctrl Pts',(2.32548648899995,2.2,3.86832710299998));
#337937=CARTESIAN_POINT('Ctrl Pts',(2.32561376299994,12.2,3.87059483399998));
#337938=CARTESIAN_POINT('Ctrl Pts',(2.32561376299994,5.2,3.87059483399998));
#337939=CARTESIAN_POINT('Ctrl Pts',(2.32561376299994,2.2,3.87059483399998));
#337940=CARTESIAN_POINT('Ctrl Pts',(2.32573879599994,12.2,3.87286646099999));
#337941=CARTESIAN_POINT('Ctrl Pts',(2.32573879599994,5.2,3.87286646099999));
#337942=CARTESIAN_POINT('Ctrl Pts',(2.32573879599994,2.2,3.87286646099999));
#337943=CARTESIAN_POINT('Ctrl Pts',(2.32586158399994,12.2,3.87514197799998));
#337944=CARTESIAN_POINT('Ctrl Pts',(2.32586158399994,5.2,3.87514197799998));
#337945=CARTESIAN_POINT('Ctrl Pts',(2.32586158399994,2.2,3.87514197799998));
#337946=CARTESIAN_POINT('Ctrl Pts',(2.32598211699994,12.2,3.87742137899998));
#337947=CARTESIAN_POINT('Ctrl Pts',(2.32598211699994,5.2,3.87742137899998));
#337948=CARTESIAN_POINT('Ctrl Pts',(2.32598211699994,2.2,3.87742137899998));
#337949=CARTESIAN_POINT('Ctrl Pts',(2.32610038699994,12.2,3.87970465699999));
#337950=CARTESIAN_POINT('Ctrl Pts',(2.32610038699994,5.2,3.87970465699999));
#337951=CARTESIAN_POINT('Ctrl Pts',(2.32610038699994,2.2,3.87970465699999));
#337952=CARTESIAN_POINT('Ctrl Pts',(2.32621638899994,12.2,3.88199180699999));
#337953=CARTESIAN_POINT('Ctrl Pts',(2.32621638899994,5.2,3.88199180699999));
#337954=CARTESIAN_POINT('Ctrl Pts',(2.32621638899994,2.2,3.88199180699999));
#337955=CARTESIAN_POINT('Ctrl Pts',(2.32633011299994,12.2,3.88428282199998));
#337956=CARTESIAN_POINT('Ctrl Pts',(2.32633011299994,5.2,3.88428282199998));
#337957=CARTESIAN_POINT('Ctrl Pts',(2.32633011299994,2.2,3.88428282199998));
#337958=CARTESIAN_POINT('Ctrl Pts',(2.32644155199994,12.2,3.88657769599998));
#337959=CARTESIAN_POINT('Ctrl Pts',(2.32644155199994,5.2,3.88657769599998));
#337960=CARTESIAN_POINT('Ctrl Pts',(2.32644155199994,2.2,3.88657769599998));
#337961=CARTESIAN_POINT('Ctrl Pts',(2.32655070199994,12.2,3.88887642099998));
#337962=CARTESIAN_POINT('Ctrl Pts',(2.32655070199994,5.2,3.88887642099998));
#337963=CARTESIAN_POINT('Ctrl Pts',(2.32655070199994,2.2,3.88887642099998));
#337964=CARTESIAN_POINT('Ctrl Pts',(2.32665754999994,12.2,3.89117899199999));
#337965=CARTESIAN_POINT('Ctrl Pts',(2.32665754999994,5.2,3.89117899199999));
#337966=CARTESIAN_POINT('Ctrl Pts',(2.32665754999994,2.2,3.89117899199999));
#337967=CARTESIAN_POINT('Ctrl Pts',(2.32676209299994,12.2,3.89348540499999));
#337968=CARTESIAN_POINT('Ctrl Pts',(2.32676209299994,5.2,3.89348540499999));
#337969=CARTESIAN_POINT('Ctrl Pts',(2.32676209299994,2.2,3.89348540499999));
#337970=CARTESIAN_POINT('Ctrl Pts',(2.32686432199994,12.2,3.89579564899999));
#337971=CARTESIAN_POINT('Ctrl Pts',(2.32686432199994,5.2,3.89579564899999));
#337972=CARTESIAN_POINT('Ctrl Pts',(2.32686432199994,2.2,3.89579564899999));
#337973=CARTESIAN_POINT('Ctrl Pts',(2.32696422899994,12.2,3.89810972199999));
#337974=CARTESIAN_POINT('Ctrl Pts',(2.32696422899994,5.2,3.89810972199999));
#337975=CARTESIAN_POINT('Ctrl Pts',(2.32696422899994,2.2,3.89810972199999));
#337976=CARTESIAN_POINT('Ctrl Pts',(2.32706180899994,12.2,3.90042761499998));
#337977=CARTESIAN_POINT('Ctrl Pts',(2.32706180899994,5.2,3.90042761499998));
#337978=CARTESIAN_POINT('Ctrl Pts',(2.32706180899994,2.2,3.90042761499998));
#337979=CARTESIAN_POINT('Ctrl Pts',(2.32715705299994,12.2,3.90274932299998));
#337980=CARTESIAN_POINT('Ctrl Pts',(2.32715705299994,5.2,3.90274932299998));
#337981=CARTESIAN_POINT('Ctrl Pts',(2.32715705299994,2.2,3.90274932299998));
#337982=CARTESIAN_POINT('Ctrl Pts',(2.32724995299994,12.2,3.90507483899999));
#337983=CARTESIAN_POINT('Ctrl Pts',(2.32724995299994,5.2,3.90507483899999));
#337984=CARTESIAN_POINT('Ctrl Pts',(2.32724995299994,2.2,3.90507483899999));
#337985=CARTESIAN_POINT('Ctrl Pts',(2.32734050299995,12.2,3.90740415699998));
#337986=CARTESIAN_POINT('Ctrl Pts',(2.32734050299995,5.2,3.90740415699998));
#337987=CARTESIAN_POINT('Ctrl Pts',(2.32734050299995,2.2,3.90740415699998));
#337988=CARTESIAN_POINT('Ctrl Pts',(2.32742869599994,12.2,3.90973727099999));
#337989=CARTESIAN_POINT('Ctrl Pts',(2.32742869599994,5.2,3.90973727099999));
#337990=CARTESIAN_POINT('Ctrl Pts',(2.32742869599994,2.2,3.90973727099999));
#337991=CARTESIAN_POINT('Ctrl Pts',(2.32751452399994,12.2,3.91207417399999));
#337992=CARTESIAN_POINT('Ctrl Pts',(2.32751452399994,5.2,3.91207417399999));
#337993=CARTESIAN_POINT('Ctrl Pts',(2.32751452399994,2.2,3.91207417399999));
#337994=CARTESIAN_POINT('Ctrl Pts',(2.32759797899994,12.2,3.91441486099998));
#337995=CARTESIAN_POINT('Ctrl Pts',(2.32759797899994,5.2,3.91441486099998));
#337996=CARTESIAN_POINT('Ctrl Pts',(2.32759797899994,2.2,3.91441486099998));
#337997=CARTESIAN_POINT('Ctrl Pts',(2.32767905599994,12.2,3.91675932499999));
#337998=CARTESIAN_POINT('Ctrl Pts',(2.32767905599994,5.2,3.91675932499999));
#337999=CARTESIAN_POINT('Ctrl Pts',(2.32767905599994,2.2,3.91675932499999));
#338000=CARTESIAN_POINT('Ctrl Pts',(2.32775774599994,12.2,3.91910755799999));
#338001=CARTESIAN_POINT('Ctrl Pts',(2.32775774599994,5.2,3.91910755799999));
#338002=CARTESIAN_POINT('Ctrl Pts',(2.32775774599994,2.2,3.91910755799999));
#338003=CARTESIAN_POINT('Ctrl Pts',(2.32783404299994,12.2,3.92145955599998));
#338004=CARTESIAN_POINT('Ctrl Pts',(2.32783404299994,5.2,3.92145955599998));
#338005=CARTESIAN_POINT('Ctrl Pts',(2.32783404299994,2.2,3.92145955599998));
#338006=CARTESIAN_POINT('Ctrl Pts',(2.32790793899994,12.2,3.92381531299999));
#338007=CARTESIAN_POINT('Ctrl Pts',(2.32790793899994,5.2,3.92381531299999));
#338008=CARTESIAN_POINT('Ctrl Pts',(2.32790793899994,2.2,3.92381531299999));
#338009=CARTESIAN_POINT('Ctrl Pts',(2.32797942799994,12.2,3.92617481999999));
#338010=CARTESIAN_POINT('Ctrl Pts',(2.32797942799994,5.2,3.92617481999999));
#338011=CARTESIAN_POINT('Ctrl Pts',(2.32797942799994,2.2,3.92617481999999));
#338012=CARTESIAN_POINT('Ctrl Pts',(2.32804850099994,12.2,3.92853807299999));
#338013=CARTESIAN_POINT('Ctrl Pts',(2.32804850099994,5.2,3.92853807299999));
#338014=CARTESIAN_POINT('Ctrl Pts',(2.32804850099994,2.2,3.92853807299999));
#338015=CARTESIAN_POINT('Ctrl Pts',(2.32811515299994,12.2,3.93090506499998));
#338016=CARTESIAN_POINT('Ctrl Pts',(2.32811515299994,5.2,3.93090506499998));
#338017=CARTESIAN_POINT('Ctrl Pts',(2.32811515299994,2.2,3.93090506499998));
#338018=CARTESIAN_POINT('Ctrl Pts',(2.32817937599994,12.2,3.93327578999998));
#338019=CARTESIAN_POINT('Ctrl Pts',(2.32817937599994,5.2,3.93327578999998));
#338020=CARTESIAN_POINT('Ctrl Pts',(2.32817937599994,2.2,3.93327578999998));
#338021=CARTESIAN_POINT('Ctrl Pts',(2.32824116199994,12.2,3.93565023999999));
#338022=CARTESIAN_POINT('Ctrl Pts',(2.32824116199994,5.2,3.93565023999999));
#338023=CARTESIAN_POINT('Ctrl Pts',(2.32824116199994,2.2,3.93565023999999));
#338024=CARTESIAN_POINT('Ctrl Pts',(2.32830050599994,12.2,3.93802841199999));
#338025=CARTESIAN_POINT('Ctrl Pts',(2.32830050599994,5.2,3.93802841199999));
#338026=CARTESIAN_POINT('Ctrl Pts',(2.32830050599994,2.2,3.93802841199999));
#338027=CARTESIAN_POINT('Ctrl Pts',(2.32835739899994,12.2,3.94041029599999));
#338028=CARTESIAN_POINT('Ctrl Pts',(2.32835739899994,5.2,3.94041029599999));
#338029=CARTESIAN_POINT('Ctrl Pts',(2.32835739899994,2.2,3.94041029599999));
#338030=CARTESIAN_POINT('Ctrl Pts',(2.32841183599994,12.2,3.94279588799999));
#338031=CARTESIAN_POINT('Ctrl Pts',(2.32841183599994,5.2,3.94279588799999));
#338032=CARTESIAN_POINT('Ctrl Pts',(2.32841183599994,2.2,3.94279588799999));
#338033=CARTESIAN_POINT('Ctrl Pts',(2.32846380899994,12.2,3.94518518199998));
#338034=CARTESIAN_POINT('Ctrl Pts',(2.32846380899994,5.2,3.94518518199998));
#338035=CARTESIAN_POINT('Ctrl Pts',(2.32846380899994,2.2,3.94518518199998));
#338036=CARTESIAN_POINT('Ctrl Pts',(2.32851330999994,12.2,3.94757816999999));
#338037=CARTESIAN_POINT('Ctrl Pts',(2.32851330999994,5.2,3.94757816999999));
#338038=CARTESIAN_POINT('Ctrl Pts',(2.32851330999994,2.2,3.94757816999999));
#338039=CARTESIAN_POINT('Ctrl Pts',(2.32856033299994,12.2,3.94997484599998));
#338040=CARTESIAN_POINT('Ctrl Pts',(2.32856033299994,5.2,3.94997484599998));
#338041=CARTESIAN_POINT('Ctrl Pts',(2.32856033299994,2.2,3.94997484599998));
#338042=CARTESIAN_POINT('Ctrl Pts',(2.32860487199994,12.2,3.95237520499998));
#338043=CARTESIAN_POINT('Ctrl Pts',(2.32860487199994,5.2,3.95237520499998));
#338044=CARTESIAN_POINT('Ctrl Pts',(2.32860487199994,2.2,3.95237520499998));
#338045=CARTESIAN_POINT('Ctrl Pts',(2.32864691899994,12.2,3.95477923899998));
#338046=CARTESIAN_POINT('Ctrl Pts',(2.32864691899994,5.2,3.95477923899998));
#338047=CARTESIAN_POINT('Ctrl Pts',(2.32864691899994,2.2,3.95477923899998));
#338048=CARTESIAN_POINT('Ctrl Pts',(2.32868646699994,12.2,3.95718694299998));
#338049=CARTESIAN_POINT('Ctrl Pts',(2.32868646699994,5.2,3.95718694299998));
#338050=CARTESIAN_POINT('Ctrl Pts',(2.32868646699994,2.2,3.95718694299998));
#338051=CARTESIAN_POINT('Ctrl Pts',(2.32872350999994,12.2,3.95959830999999));
#338052=CARTESIAN_POINT('Ctrl Pts',(2.32872350999994,5.2,3.95959830999999));
#338053=CARTESIAN_POINT('Ctrl Pts',(2.32872350999994,2.2,3.95959830999999));
#338054=CARTESIAN_POINT('Ctrl Pts',(2.32875804099994,12.2,3.96201333399999));
#338055=CARTESIAN_POINT('Ctrl Pts',(2.32875804099994,5.2,3.96201333399999));
#338056=CARTESIAN_POINT('Ctrl Pts',(2.32875804099994,2.2,3.96201333399999));
#338057=CARTESIAN_POINT('Ctrl Pts',(2.32879005199994,12.2,3.96443200799999));
#338058=CARTESIAN_POINT('Ctrl Pts',(2.32879005199994,5.2,3.96443200799999));
#338059=CARTESIAN_POINT('Ctrl Pts',(2.32879005199994,2.2,3.96443200799999));
#338060=CARTESIAN_POINT('Ctrl Pts',(2.32881953799994,12.2,3.96685432699999));
#338061=CARTESIAN_POINT('Ctrl Pts',(2.32881953799994,5.2,3.96685432699999));
#338062=CARTESIAN_POINT('Ctrl Pts',(2.32881953799994,2.2,3.96685432699999));
#338063=CARTESIAN_POINT('Ctrl Pts',(2.32884649099994,12.2,3.96928028299998));
#338064=CARTESIAN_POINT('Ctrl Pts',(2.32884649099994,5.2,3.96928028299998));
#338065=CARTESIAN_POINT('Ctrl Pts',(2.32884649099994,2.2,3.96928028299998));
#338066=CARTESIAN_POINT('Ctrl Pts',(2.32887090299994,12.2,3.97170987099998));
#338067=CARTESIAN_POINT('Ctrl Pts',(2.32887090299994,5.2,3.97170987099998));
#338068=CARTESIAN_POINT('Ctrl Pts',(2.32887090299994,2.2,3.97170987099998));
#338069=CARTESIAN_POINT('Ctrl Pts',(2.32889277099994,12.2,3.97414308499999));
#338070=CARTESIAN_POINT('Ctrl Pts',(2.32889277099994,5.2,3.97414308499999));
#338071=CARTESIAN_POINT('Ctrl Pts',(2.32889277099994,2.2,3.97414308499999));
#338072=CARTESIAN_POINT('Ctrl Pts',(2.32891208399994,12.2,3.97657991599999));
#338073=CARTESIAN_POINT('Ctrl Pts',(2.32891208399994,5.2,3.97657991599999));
#338074=CARTESIAN_POINT('Ctrl Pts',(2.32891208399994,2.2,3.97657991599999));
#338075=CARTESIAN_POINT('Ctrl Pts',(2.32892883899994,12.2,3.97902035999999));
#338076=CARTESIAN_POINT('Ctrl Pts',(2.32892883899994,5.2,3.97902035999999));
#338077=CARTESIAN_POINT('Ctrl Pts',(2.32892883899994,2.2,3.97902035999999));
#338078=CARTESIAN_POINT('Ctrl Pts',(2.32894302699994,12.2,3.98146441099998));
#338079=CARTESIAN_POINT('Ctrl Pts',(2.32894302699994,5.2,3.98146441099998));
#338080=CARTESIAN_POINT('Ctrl Pts',(2.32894302699994,2.2,3.98146441099998));
#338081=CARTESIAN_POINT('Ctrl Pts',(2.32895464099994,12.2,3.98391206199998));
#338082=CARTESIAN_POINT('Ctrl Pts',(2.32895464099994,5.2,3.98391206199998));
#338083=CARTESIAN_POINT('Ctrl Pts',(2.32895464099994,2.2,3.98391206199998));
#338084=CARTESIAN_POINT('Ctrl Pts',(2.32896367499994,12.2,3.98636330599999));
#338085=CARTESIAN_POINT('Ctrl Pts',(2.32896367499994,5.2,3.98636330599999));
#338086=CARTESIAN_POINT('Ctrl Pts',(2.32896367499994,2.2,3.98636330599999));
#338087=CARTESIAN_POINT('Ctrl Pts',(2.32897012299994,12.2,3.98881813699998));
#338088=CARTESIAN_POINT('Ctrl Pts',(2.32897012299994,5.2,3.98881813699998));
#338089=CARTESIAN_POINT('Ctrl Pts',(2.32897012299994,2.2,3.98881813699998));
#338090=CARTESIAN_POINT('Ctrl Pts',(2.32897397899994,12.2,3.99127654899999));
#338091=CARTESIAN_POINT('Ctrl Pts',(2.32897397899994,5.2,3.99127654899999));
#338092=CARTESIAN_POINT('Ctrl Pts',(2.32897397899994,2.2,3.99127654899999));
#338093=CARTESIAN_POINT('Ctrl Pts',(2.32897523399994,12.2,3.99373853499998));
#338094=CARTESIAN_POINT('Ctrl Pts',(2.32897523399994,5.2,3.99373853499998));
#338095=CARTESIAN_POINT('Ctrl Pts',(2.32897523399994,2.2,3.99373853499998));
#338096=CARTESIAN_POINT('Ctrl Pts',(2.32897388199994,12.2,3.99620408999999));
#338097=CARTESIAN_POINT('Ctrl Pts',(2.32897388199994,5.2,3.99620408999999));
#338098=CARTESIAN_POINT('Ctrl Pts',(2.32897388199994,2.2,3.99620408999999));
#338099=CARTESIAN_POINT('Ctrl Pts',(2.32896991899994,12.2,3.99867320599999));
#338100=CARTESIAN_POINT('Ctrl Pts',(2.32896991899994,5.2,3.99867320599999));
#338101=CARTESIAN_POINT('Ctrl Pts',(2.32896991899994,2.2,3.99867320599999));
#338102=CARTESIAN_POINT('Ctrl Pts',(2.32896333499994,12.2,4.00114587899999));
#338103=CARTESIAN_POINT('Ctrl Pts',(2.32896333499994,5.2,4.00114587899999));
#338104=CARTESIAN_POINT('Ctrl Pts',(2.32896333499994,2.2,4.00114587899999));
#338105=CARTESIAN_POINT('Ctrl Pts',(2.32895412499994,12.2,4.00362209899999));
#338106=CARTESIAN_POINT('Ctrl Pts',(2.32895412499994,5.2,4.00362209899999));
#338107=CARTESIAN_POINT('Ctrl Pts',(2.32895412499994,2.2,4.00362209899999));
#338108=CARTESIAN_POINT('Ctrl Pts',(2.32894228399994,12.2,4.00610186299998));
#338109=CARTESIAN_POINT('Ctrl Pts',(2.32894228399994,5.2,4.00610186299998));
#338110=CARTESIAN_POINT('Ctrl Pts',(2.32894228399994,2.2,4.00610186299998));
#338111=CARTESIAN_POINT('Ctrl Pts',(2.32892780199994,12.2,4.00858516399998));
#338112=CARTESIAN_POINT('Ctrl Pts',(2.32892780199994,5.2,4.00858516399998));
#338113=CARTESIAN_POINT('Ctrl Pts',(2.32892780199994,2.2,4.00858516399998));
#338114=CARTESIAN_POINT('Ctrl Pts',(2.32891067499994,12.2,4.01107199399998));
#338115=CARTESIAN_POINT('Ctrl Pts',(2.32891067499994,5.2,4.01107199399998));
#338116=CARTESIAN_POINT('Ctrl Pts',(2.32891067499994,2.2,4.01107199399998));
#338117=CARTESIAN_POINT('Ctrl Pts',(2.32889089599994,12.2,4.01356234799999));
#338118=CARTESIAN_POINT('Ctrl Pts',(2.32889089599994,5.2,4.01356234799999));
#338119=CARTESIAN_POINT('Ctrl Pts',(2.32889089599994,2.2,4.01356234799999));
#338120=CARTESIAN_POINT('Ctrl Pts',(2.32886845899994,12.2,4.01605621899999));
#338121=CARTESIAN_POINT('Ctrl Pts',(2.32886845899994,5.2,4.01605621899999));
#338122=CARTESIAN_POINT('Ctrl Pts',(2.32886845899994,2.2,4.01605621899999));
#338123=CARTESIAN_POINT('Ctrl Pts',(2.32884335599994,12.2,4.01855360199999));
#338124=CARTESIAN_POINT('Ctrl Pts',(2.32884335599994,5.2,4.01855360199999));
#338125=CARTESIAN_POINT('Ctrl Pts',(2.32884335599994,2.2,4.01855360199999));
#338126=CARTESIAN_POINT('Ctrl Pts',(2.32881558199994,12.2,4.02105448799999));
#338127=CARTESIAN_POINT('Ctrl Pts',(2.32881558199994,5.2,4.02105448799999));
#338128=CARTESIAN_POINT('Ctrl Pts',(2.32881558199994,2.2,4.02105448799999));
#338129=CARTESIAN_POINT('Ctrl Pts',(2.32878512999994,12.2,4.02355887399998));
#338130=CARTESIAN_POINT('Ctrl Pts',(2.32878512999994,5.2,4.02355887399998));
#338131=CARTESIAN_POINT('Ctrl Pts',(2.32878512999994,2.2,4.02355887399998));
#338132=CARTESIAN_POINT('Ctrl Pts',(2.32875199399994,12.2,4.02606675199999));
#338133=CARTESIAN_POINT('Ctrl Pts',(2.32875199399994,5.2,4.02606675199999));
#338134=CARTESIAN_POINT('Ctrl Pts',(2.32875199399994,2.2,4.02606675199999));
#338135=CARTESIAN_POINT('Ctrl Pts',(2.32871616699994,12.2,4.02857811499998));
#338136=CARTESIAN_POINT('Ctrl Pts',(2.32871616699994,5.2,4.02857811499998));
#338137=CARTESIAN_POINT('Ctrl Pts',(2.32871616699994,2.2,4.02857811499998));
#338138=CARTESIAN_POINT('Ctrl Pts',(2.32867764299994,12.2,4.03109295699998));
#338139=CARTESIAN_POINT('Ctrl Pts',(2.32867764299994,5.2,4.03109295699998));
#338140=CARTESIAN_POINT('Ctrl Pts',(2.32867764299994,2.2,4.03109295699998));
#338141=CARTESIAN_POINT('Ctrl Pts',(2.32863641599994,12.2,4.03361127299998));
#338142=CARTESIAN_POINT('Ctrl Pts',(2.32863641599994,5.2,4.03361127299998));
#338143=CARTESIAN_POINT('Ctrl Pts',(2.32863641599994,2.2,4.03361127299998));
#338144=CARTESIAN_POINT('Ctrl Pts',(2.32859247799994,12.2,4.03613305399999));
#338145=CARTESIAN_POINT('Ctrl Pts',(2.32859247799994,5.2,4.03613305399999));
#338146=CARTESIAN_POINT('Ctrl Pts',(2.32859247799994,2.2,4.03613305399999));
#338147=CARTESIAN_POINT('Ctrl Pts',(2.32854582499994,12.2,4.03865829699999));
#338148=CARTESIAN_POINT('Ctrl Pts',(2.32854582499994,5.2,4.03865829699999));
#338149=CARTESIAN_POINT('Ctrl Pts',(2.32854582499994,2.2,4.03865829699999));
#338150=CARTESIAN_POINT('Ctrl Pts',(2.32849644899995,12.2,4.04118699199999));
#338151=CARTESIAN_POINT('Ctrl Pts',(2.32849644899995,5.2,4.04118699199999));
#338152=CARTESIAN_POINT('Ctrl Pts',(2.32849644899995,2.2,4.04118699199999));
#338153=CARTESIAN_POINT('Ctrl Pts',(2.32844434499994,12.2,4.04371913499999));
#338154=CARTESIAN_POINT('Ctrl Pts',(2.32844434499994,5.2,4.04371913499999));
#338155=CARTESIAN_POINT('Ctrl Pts',(2.32844434499994,2.2,4.04371913499999));
#338156=CARTESIAN_POINT('Ctrl Pts',(2.32838950599994,12.2,4.04625471999999));
#338157=CARTESIAN_POINT('Ctrl Pts',(2.32838950599994,5.2,4.04625471999999));
#338158=CARTESIAN_POINT('Ctrl Pts',(2.32838950599994,2.2,4.04625471999999));
#338159=CARTESIAN_POINT('Ctrl Pts',(2.32833192599994,12.2,4.04879373899998));
#338160=CARTESIAN_POINT('Ctrl Pts',(2.32833192599994,5.2,4.04879373899998));
#338161=CARTESIAN_POINT('Ctrl Pts',(2.32833192599994,2.2,4.04879373899998));
#338162=CARTESIAN_POINT('Ctrl Pts',(2.32827159799994,12.2,4.05133618699999));
#338163=CARTESIAN_POINT('Ctrl Pts',(2.32827159799994,5.2,4.05133618699999));
#338164=CARTESIAN_POINT('Ctrl Pts',(2.32827159799994,2.2,4.05133618699999));
#338165=CARTESIAN_POINT('Ctrl Pts',(2.32820851699994,12.2,4.05388205699998));
#338166=CARTESIAN_POINT('Ctrl Pts',(2.32820851699994,5.2,4.05388205699998));
#338167=CARTESIAN_POINT('Ctrl Pts',(2.32820851699994,2.2,4.05388205699998));
#338168=CARTESIAN_POINT('Ctrl Pts',(2.32814267599994,12.2,4.05643134199998));
#338169=CARTESIAN_POINT('Ctrl Pts',(2.32814267599994,5.2,4.05643134199998));
#338170=CARTESIAN_POINT('Ctrl Pts',(2.32814267599994,2.2,4.05643134199998));
#338171=CARTESIAN_POINT('Ctrl Pts',(2.32807406899994,12.2,4.05898403699998));
#338172=CARTESIAN_POINT('Ctrl Pts',(2.32807406899994,5.2,4.05898403699998));
#338173=CARTESIAN_POINT('Ctrl Pts',(2.32807406899994,2.2,4.05898403699998));
#338174=CARTESIAN_POINT('Ctrl Pts',(2.32800268999994,12.2,4.06154013499999));
#338175=CARTESIAN_POINT('Ctrl Pts',(2.32800268999994,5.2,4.06154013499999));
#338176=CARTESIAN_POINT('Ctrl Pts',(2.32800268999994,2.2,4.06154013499999));
#338177=CARTESIAN_POINT('Ctrl Pts',(2.32792853199994,12.2,4.06409962899998));
#338178=CARTESIAN_POINT('Ctrl Pts',(2.32792853199994,5.2,4.06409962899998));
#338179=CARTESIAN_POINT('Ctrl Pts',(2.32792853199994,2.2,4.06409962899998));
#338180=CARTESIAN_POINT('Ctrl Pts',(2.32785158999994,12.2,4.06666251299999));
#338181=CARTESIAN_POINT('Ctrl Pts',(2.32785158999994,5.2,4.06666251299999));
#338182=CARTESIAN_POINT('Ctrl Pts',(2.32785158999994,2.2,4.06666251299999));
#338183=CARTESIAN_POINT('Ctrl Pts',(2.32777185699994,12.2,4.06922878199998));
#338184=CARTESIAN_POINT('Ctrl Pts',(2.32777185699994,5.2,4.06922878199998));
#338185=CARTESIAN_POINT('Ctrl Pts',(2.32777185699994,2.2,4.06922878199998));
#338186=CARTESIAN_POINT('Ctrl Pts',(2.32768932599994,12.2,4.07179842699998));
#338187=CARTESIAN_POINT('Ctrl Pts',(2.32768932599994,5.2,4.07179842699998));
#338188=CARTESIAN_POINT('Ctrl Pts',(2.32768932599994,2.2,4.07179842699998));
#338189=CARTESIAN_POINT('Ctrl Pts',(2.32760399399994,12.2,4.07437144399999));
#338190=CARTESIAN_POINT('Ctrl Pts',(2.32760399399994,5.2,4.07437144399999));
#338191=CARTESIAN_POINT('Ctrl Pts',(2.32760399399994,2.2,4.07437144399999));
#338192=CARTESIAN_POINT('Ctrl Pts',(2.32751585199995,12.2,4.07694782499998));
#338193=CARTESIAN_POINT('Ctrl Pts',(2.32751585199995,5.2,4.07694782499998));
#338194=CARTESIAN_POINT('Ctrl Pts',(2.32751585199995,2.2,4.07694782499998));
#338195=CARTESIAN_POINT('Ctrl Pts',(2.32742489599994,12.2,4.07952756599999));
#338196=CARTESIAN_POINT('Ctrl Pts',(2.32742489599994,5.2,4.07952756599999));
#338197=CARTESIAN_POINT('Ctrl Pts',(2.32742489599994,2.2,4.07952756599999));
#338198=CARTESIAN_POINT('Ctrl Pts',(2.32733111999994,12.2,4.08211065799998));
#338199=CARTESIAN_POINT('Ctrl Pts',(2.32733111999994,5.2,4.08211065799998));
#338200=CARTESIAN_POINT('Ctrl Pts',(2.32733111999994,2.2,4.08211065799998));
#338201=CARTESIAN_POINT('Ctrl Pts',(2.32723451599994,12.2,4.08469709699999));
#338202=CARTESIAN_POINT('Ctrl Pts',(2.32723451599994,5.2,4.08469709699999));
#338203=CARTESIAN_POINT('Ctrl Pts',(2.32723451599994,2.2,4.08469709699999));
#338204=CARTESIAN_POINT('Ctrl Pts',(2.32713507999994,12.2,4.08728687499998));
#338205=CARTESIAN_POINT('Ctrl Pts',(2.32713507999994,5.2,4.08728687499998));
#338206=CARTESIAN_POINT('Ctrl Pts',(2.32713507999994,2.2,4.08728687499998));
#338207=CARTESIAN_POINT('Ctrl Pts',(2.32703280399994,12.2,4.08987998599999));
#338208=CARTESIAN_POINT('Ctrl Pts',(2.32703280399994,5.2,4.08987998599999));
#338209=CARTESIAN_POINT('Ctrl Pts',(2.32703280399994,2.2,4.08987998599999));
#338210=CARTESIAN_POINT('Ctrl Pts',(2.32692768299994,12.2,4.09247642199999));
#338211=CARTESIAN_POINT('Ctrl Pts',(2.32692768299994,5.2,4.09247642199999));
#338212=CARTESIAN_POINT('Ctrl Pts',(2.32692768299994,2.2,4.09247642199999));
#338213=CARTESIAN_POINT('Ctrl Pts',(2.32681970999994,12.2,4.09507617799999));
#338214=CARTESIAN_POINT('Ctrl Pts',(2.32681970999994,5.2,4.09507617799999));
#338215=CARTESIAN_POINT('Ctrl Pts',(2.32681970999994,2.2,4.09507617799999));
#338216=CARTESIAN_POINT('Ctrl Pts',(2.32670887999994,12.2,4.09767924799999));
#338217=CARTESIAN_POINT('Ctrl Pts',(2.32670887999994,5.2,4.09767924799999));
#338218=CARTESIAN_POINT('Ctrl Pts',(2.32670887999994,2.2,4.09767924799999));
#338219=CARTESIAN_POINT('Ctrl Pts',(2.32659518599994,12.2,4.10028562499999));
#338220=CARTESIAN_POINT('Ctrl Pts',(2.32659518599994,5.2,4.10028562499999));
#338221=CARTESIAN_POINT('Ctrl Pts',(2.32659518599994,2.2,4.10028562499999));
#338222=CARTESIAN_POINT('Ctrl Pts',(2.32647862299994,12.2,4.10289530199999));
#338223=CARTESIAN_POINT('Ctrl Pts',(2.32647862299994,5.2,4.10289530199999));
#338224=CARTESIAN_POINT('Ctrl Pts',(2.32647862299994,2.2,4.10289530199999));
#338225=CARTESIAN_POINT('Ctrl Pts',(2.32635918599994,12.2,4.10550827399998));
#338226=CARTESIAN_POINT('Ctrl Pts',(2.32635918599994,5.2,4.10550827399998));
#338227=CARTESIAN_POINT('Ctrl Pts',(2.32635918599994,2.2,4.10550827399998));
#338228=CARTESIAN_POINT('Ctrl Pts',(2.32623686999994,12.2,4.10812453699998));
#338229=CARTESIAN_POINT('Ctrl Pts',(2.32623686999994,5.2,4.10812453699998));
#338230=CARTESIAN_POINT('Ctrl Pts',(2.32623686999994,2.2,4.10812453699998));
#338231=CARTESIAN_POINT('Ctrl Pts',(2.32611166899995,12.2,4.11074408199998));
#338232=CARTESIAN_POINT('Ctrl Pts',(2.32611166899995,5.2,4.11074408199998));
#338233=CARTESIAN_POINT('Ctrl Pts',(2.32611166899995,2.2,4.11074408199998));
#338234=CARTESIAN_POINT('Ctrl Pts',(2.32598357799994,12.2,4.11336690499999));
#338235=CARTESIAN_POINT('Ctrl Pts',(2.32598357799994,5.2,4.11336690499999));
#338236=CARTESIAN_POINT('Ctrl Pts',(2.32598357799994,2.2,4.11336690499999));
#338237=CARTESIAN_POINT('Ctrl Pts',(2.32585258899995,12.2,4.11599299899999));
#338238=CARTESIAN_POINT('Ctrl Pts',(2.32585258899995,5.2,4.11599299899999));
#338239=CARTESIAN_POINT('Ctrl Pts',(2.32585258899995,2.2,4.11599299899999));
#338240=CARTESIAN_POINT('Ctrl Pts',(2.32571869499994,12.2,4.11862235399998));
#338241=CARTESIAN_POINT('Ctrl Pts',(2.32571869499994,5.2,4.11862235399998));
#338242=CARTESIAN_POINT('Ctrl Pts',(2.32571869499994,2.2,4.11862235399998));
#338243=CARTESIAN_POINT('Ctrl Pts',(2.32558188999994,12.2,4.12125496399998));
#338244=CARTESIAN_POINT('Ctrl Pts',(2.32558188999994,5.2,4.12125496399998));
#338245=CARTESIAN_POINT('Ctrl Pts',(2.32558188999994,2.2,4.12125496399998));
#338246=CARTESIAN_POINT('Ctrl Pts',(2.32544216699994,12.2,4.12389081999999));
#338247=CARTESIAN_POINT('Ctrl Pts',(2.32544216699994,5.2,4.12389081999999));
#338248=CARTESIAN_POINT('Ctrl Pts',(2.32544216699994,2.2,4.12389081999999));
#338249=CARTESIAN_POINT('Ctrl Pts',(2.32529951799994,12.2,4.12652991599998));
#338250=CARTESIAN_POINT('Ctrl Pts',(2.32529951799994,5.2,4.12652991599998));
#338251=CARTESIAN_POINT('Ctrl Pts',(2.32529951799994,2.2,4.12652991599998));
#338252=CARTESIAN_POINT('Ctrl Pts',(2.32515393799994,12.2,4.12917224599998));
#338253=CARTESIAN_POINT('Ctrl Pts',(2.32515393799994,5.2,4.12917224599998));
#338254=CARTESIAN_POINT('Ctrl Pts',(2.32515393799994,2.2,4.12917224599998));
#338255=CARTESIAN_POINT('Ctrl Pts',(2.32500542299994,12.2,4.13181780399999));
#338256=CARTESIAN_POINT('Ctrl Pts',(2.32500542299994,5.2,4.13181780399999));
#338257=CARTESIAN_POINT('Ctrl Pts',(2.32500542299994,2.2,4.13181780399999));
#338258=CARTESIAN_POINT('Ctrl Pts',(2.32485396999994,12.2,4.13446658699999));
#338259=CARTESIAN_POINT('Ctrl Pts',(2.32485396999994,5.2,4.13446658699999));
#338260=CARTESIAN_POINT('Ctrl Pts',(2.32485396999994,2.2,4.13446658699999));
#338261=CARTESIAN_POINT('Ctrl Pts',(2.3246995789955,12.2,4.1371185950763));
#338262=CARTESIAN_POINT('Ctrl Pts',(2.3246995789955,5.2,4.1371185950763));
#338263=CARTESIAN_POINT('Ctrl Pts',(2.3246995789955,2.2,4.1371185950763));
#338264=CARTESIAN_POINT('Ctrl Pts',(2.32457371399089,12.2,4.1392427791528));
#338265=CARTESIAN_POINT('Ctrl Pts',(2.32457371399089,5.2,4.1392427791528));
#338266=CARTESIAN_POINT('Ctrl Pts',(2.32457371399089,2.2,4.1392427791528));
#338267=CARTESIAN_POINT('Ctrl Pts',(2.32447799198617,12.2,4.14083736722942));
#338268=CARTESIAN_POINT('Ctrl Pts',(2.32447799198617,5.2,4.14083736722942));
#338269=CARTESIAN_POINT('Ctrl Pts',(2.32447799198617,2.2,4.14083736722942));
#338270=CARTESIAN_POINT('Ctrl Pts',(2.32441358898141,12.2,4.14190107030607));
#338271=CARTESIAN_POINT('Ctrl Pts',(2.32441358898141,5.2,4.14190107030607));
#338272=CARTESIAN_POINT('Ctrl Pts',(2.32441358898141,2.2,4.14190107030607));
#338273=CARTESIAN_POINT('Ctrl Pts',(2.32438124099994,12.2,4.14243308299999));
#338274=CARTESIAN_POINT('Ctrl Pts',(2.32438124099994,5.2,4.14243308299999));
#338275=CARTESIAN_POINT('Ctrl Pts',(2.32438124099994,2.2,4.14243308299999));
#338276=CARTESIAN_POINT('Origin',(2.68745007499994,15.2,2.95418363899999));
#338277=CARTESIAN_POINT('',(2.43934748299994,2.2,2.68145648099999));
#338278=CARTESIAN_POINT('',(2.68748460699994,12.2,2.95422159799998));
#338279=CARTESIAN_POINT('Origin',(-5.66300478732629E-14,15.2,-1.77635683940025E-14));
#338280=CARTESIAN_POINT('',(3.25496455399994,12.2,2.31410196199999));
#338281=CARTESIAN_POINT('',(2.95444430699995,12.2,2.10044848399999));
#338282=CARTESIAN_POINT('Ctrl Pts',(3.44029922199995,12.2,3.27518568399999));
#338283=CARTESIAN_POINT('Ctrl Pts',(3.44029922199995,5.2,3.27518568399999));
#338284=CARTESIAN_POINT('Ctrl Pts',(3.44029922199995,2.2,3.27518568399999));
#338285=CARTESIAN_POINT('Ctrl Pts',(3.43977569199994,12.2,3.27508567799998));
#338286=CARTESIAN_POINT('Ctrl Pts',(3.43977569199994,5.2,3.27508567799998));
#338287=CARTESIAN_POINT('Ctrl Pts',(3.43977569199994,2.2,3.27508567799998));
#338288=CARTESIAN_POINT('Ctrl Pts',(3.43872901899994,12.2,3.27488545899998));
#338289=CARTESIAN_POINT('Ctrl Pts',(3.43872901899994,5.2,3.27488545899998));
#338290=CARTESIAN_POINT('Ctrl Pts',(3.43872901899994,2.2,3.27488545899998));
#338291=CARTESIAN_POINT('Ctrl Pts',(3.43716016399994,12.2,3.27458451299999));
#338292=CARTESIAN_POINT('Ctrl Pts',(3.43716016399994,5.2,3.27458451299999));
#338293=CARTESIAN_POINT('Ctrl Pts',(3.43716016399994,2.2,3.27458451299999));
#338294=CARTESIAN_POINT('Ctrl Pts',(3.43507066699994,12.2,3.27418202199999));
#338295=CARTESIAN_POINT('Ctrl Pts',(3.43507066699994,5.2,3.27418202199999));
#338296=CARTESIAN_POINT('Ctrl Pts',(3.43507066699994,2.2,3.27418202199999));
#338297=CARTESIAN_POINT('Ctrl Pts',(3.43246264299994,12.2,3.27367685499999));
#338298=CARTESIAN_POINT('Ctrl Pts',(3.43246264299994,5.2,3.27367685499999));
#338299=CARTESIAN_POINT('Ctrl Pts',(3.43246264299994,2.2,3.27367685499999));
#338300=CARTESIAN_POINT('Ctrl Pts',(3.42985846999994,12.2,3.27316963499998));
#338301=CARTESIAN_POINT('Ctrl Pts',(3.42985846999994,5.2,3.27316963499998));
#338302=CARTESIAN_POINT('Ctrl Pts',(3.42985846999994,2.2,3.27316963499998));
#338303=CARTESIAN_POINT('Ctrl Pts',(3.42725814699994,12.2,3.27266036499999));
#338304=CARTESIAN_POINT('Ctrl Pts',(3.42725814699994,5.2,3.27266036499999));
#338305=CARTESIAN_POINT('Ctrl Pts',(3.42725814699994,2.2,3.27266036499999));
#338306=CARTESIAN_POINT('Ctrl Pts',(3.42466167799994,12.2,3.27214904799998));
#338307=CARTESIAN_POINT('Ctrl Pts',(3.42466167799994,5.2,3.27214904799998));
#338308=CARTESIAN_POINT('Ctrl Pts',(3.42466167799994,2.2,3.27214904799998));
#338309=CARTESIAN_POINT('Ctrl Pts',(3.42206906499994,12.2,3.27163568999998));
#338310=CARTESIAN_POINT('Ctrl Pts',(3.42206906499994,5.2,3.27163568999998));
#338311=CARTESIAN_POINT('Ctrl Pts',(3.42206906499994,2.2,3.27163568999998));
#338312=CARTESIAN_POINT('Ctrl Pts',(3.41948031499994,12.2,3.27112029599999));
#338313=CARTESIAN_POINT('Ctrl Pts',(3.41948031499994,5.2,3.27112029599999));
#338314=CARTESIAN_POINT('Ctrl Pts',(3.41948031499994,2.2,3.27112029599999));
#338315=CARTESIAN_POINT('Ctrl Pts',(3.41689542999994,12.2,3.27060287499998));
#338316=CARTESIAN_POINT('Ctrl Pts',(3.41689542999994,5.2,3.27060287499998));
#338317=CARTESIAN_POINT('Ctrl Pts',(3.41689542999994,2.2,3.27060287499998));
#338318=CARTESIAN_POINT('Ctrl Pts',(3.41431441799994,12.2,3.27008343699998));
#338319=CARTESIAN_POINT('Ctrl Pts',(3.41431441799994,5.2,3.27008343699998));
#338320=CARTESIAN_POINT('Ctrl Pts',(3.41431441799994,2.2,3.27008343699998));
#338321=CARTESIAN_POINT('Ctrl Pts',(3.41173728499994,12.2,3.26956198899998));
#338322=CARTESIAN_POINT('Ctrl Pts',(3.41173728499994,5.2,3.26956198899998));
#338323=CARTESIAN_POINT('Ctrl Pts',(3.41173728499994,2.2,3.26956198899998));
#338324=CARTESIAN_POINT('Ctrl Pts',(3.40916403599994,12.2,3.26903854199998));
#338325=CARTESIAN_POINT('Ctrl Pts',(3.40916403599994,5.2,3.26903854199998));
#338326=CARTESIAN_POINT('Ctrl Pts',(3.40916403599994,2.2,3.26903854199998));
#338327=CARTESIAN_POINT('Ctrl Pts',(3.40659467599994,12.2,3.26851310199999));
#338328=CARTESIAN_POINT('Ctrl Pts',(3.40659467599994,5.2,3.26851310199999));
#338329=CARTESIAN_POINT('Ctrl Pts',(3.40659467599994,2.2,3.26851310199999));
#338330=CARTESIAN_POINT('Ctrl Pts',(3.40402921099995,12.2,3.26798567699999));
#338331=CARTESIAN_POINT('Ctrl Pts',(3.40402921099995,5.2,3.26798567699999));
#338332=CARTESIAN_POINT('Ctrl Pts',(3.40402921099995,2.2,3.26798567699999));
#338333=CARTESIAN_POINT('Ctrl Pts',(3.40146764399994,12.2,3.26745627399998));
#338334=CARTESIAN_POINT('Ctrl Pts',(3.40146764399994,5.2,3.26745627399998));
#338335=CARTESIAN_POINT('Ctrl Pts',(3.40146764399994,2.2,3.26745627399998));
#338336=CARTESIAN_POINT('Ctrl Pts',(3.39890997999994,12.2,3.26692490099998));
#338337=CARTESIAN_POINT('Ctrl Pts',(3.39890997999994,5.2,3.26692490099998));
#338338=CARTESIAN_POINT('Ctrl Pts',(3.39890997999994,2.2,3.26692490099998));
#338339=CARTESIAN_POINT('Ctrl Pts',(3.39635622399994,12.2,3.26639156099999));
#338340=CARTESIAN_POINT('Ctrl Pts',(3.39635622399994,5.2,3.26639156099999));
#338341=CARTESIAN_POINT('Ctrl Pts',(3.39635622399994,2.2,3.26639156099999));
#338342=CARTESIAN_POINT('Ctrl Pts',(3.39380637899994,12.2,3.26585626399999));
#338343=CARTESIAN_POINT('Ctrl Pts',(3.39380637899994,5.2,3.26585626399999));
#338344=CARTESIAN_POINT('Ctrl Pts',(3.39380637899994,2.2,3.26585626399999));
#338345=CARTESIAN_POINT('Ctrl Pts',(3.39126044899994,12.2,3.26531901499998));
#338346=CARTESIAN_POINT('Ctrl Pts',(3.39126044899994,5.2,3.26531901499998));
#338347=CARTESIAN_POINT('Ctrl Pts',(3.39126044899994,2.2,3.26531901499998));
#338348=CARTESIAN_POINT('Ctrl Pts',(3.38871844099994,12.2,3.26477982299998));
#338349=CARTESIAN_POINT('Ctrl Pts',(3.38871844099994,5.2,3.26477982299998));
#338350=CARTESIAN_POINT('Ctrl Pts',(3.38871844099994,2.2,3.26477982299998));
#338351=CARTESIAN_POINT('Ctrl Pts',(3.38618035899994,12.2,3.26423869499998));
#338352=CARTESIAN_POINT('Ctrl Pts',(3.38618035899994,5.2,3.26423869499998));
#338353=CARTESIAN_POINT('Ctrl Pts',(3.38618035899994,2.2,3.26423869499998));
#338354=CARTESIAN_POINT('Ctrl Pts',(3.38364620599994,12.2,3.26369563699998));
#338355=CARTESIAN_POINT('Ctrl Pts',(3.38364620599994,5.2,3.26369563699998));
#338356=CARTESIAN_POINT('Ctrl Pts',(3.38364620599994,2.2,3.26369563699998));
#338357=CARTESIAN_POINT('Ctrl Pts',(3.38111598999994,12.2,3.26315065999999));
#338358=CARTESIAN_POINT('Ctrl Pts',(3.38111598999994,5.2,3.26315065999999));
#338359=CARTESIAN_POINT('Ctrl Pts',(3.38111598999994,2.2,3.26315065999999));
#338360=CARTESIAN_POINT('Ctrl Pts',(3.37858971299994,12.2,3.26260376899998));
#338361=CARTESIAN_POINT('Ctrl Pts',(3.37858971299994,5.2,3.26260376899998));
#338362=CARTESIAN_POINT('Ctrl Pts',(3.37858971299994,2.2,3.26260376899998));
#338363=CARTESIAN_POINT('Ctrl Pts',(3.37606738299994,12.2,3.26205497299998));
#338364=CARTESIAN_POINT('Ctrl Pts',(3.37606738299994,5.2,3.26205497299998));
#338365=CARTESIAN_POINT('Ctrl Pts',(3.37606738299994,2.2,3.26205497299998));
#338366=CARTESIAN_POINT('Ctrl Pts',(3.37354899999994,12.2,3.26150427799998));
#338367=CARTESIAN_POINT('Ctrl Pts',(3.37354899999994,5.2,3.26150427799998));
#338368=CARTESIAN_POINT('Ctrl Pts',(3.37354899999994,2.2,3.26150427799998));
#338369=CARTESIAN_POINT('Ctrl Pts',(3.37103457299994,12.2,3.26095169299998));
#338370=CARTESIAN_POINT('Ctrl Pts',(3.37103457299994,5.2,3.26095169299998));
#338371=CARTESIAN_POINT('Ctrl Pts',(3.37103457299994,2.2,3.26095169299998));
#338372=CARTESIAN_POINT('Ctrl Pts',(3.36852410399994,12.2,3.26039722299999));
#338373=CARTESIAN_POINT('Ctrl Pts',(3.36852410399994,5.2,3.26039722299999));
#338374=CARTESIAN_POINT('Ctrl Pts',(3.36852410399994,2.2,3.26039722299999));
#338375=CARTESIAN_POINT('Ctrl Pts',(3.36601759899994,12.2,3.25984087699998));
#338376=CARTESIAN_POINT('Ctrl Pts',(3.36601759899994,5.2,3.25984087699998));
#338377=CARTESIAN_POINT('Ctrl Pts',(3.36601759899994,2.2,3.25984087699998));
#338378=CARTESIAN_POINT('Ctrl Pts',(3.36351506199994,12.2,3.25928266199998));
#338379=CARTESIAN_POINT('Ctrl Pts',(3.36351506199994,5.2,3.25928266199998));
#338380=CARTESIAN_POINT('Ctrl Pts',(3.36351506199994,2.2,3.25928266199998));
#338381=CARTESIAN_POINT('Ctrl Pts',(3.36101649699994,12.2,3.25872258599999));
#338382=CARTESIAN_POINT('Ctrl Pts',(3.36101649699994,5.2,3.25872258599999));
#338383=CARTESIAN_POINT('Ctrl Pts',(3.36101649699994,2.2,3.25872258599999));
#338384=CARTESIAN_POINT('Ctrl Pts',(3.35852190999995,12.2,3.25816065699998));
#338385=CARTESIAN_POINT('Ctrl Pts',(3.35852190999995,5.2,3.25816065699998));
#338386=CARTESIAN_POINT('Ctrl Pts',(3.35852190999995,2.2,3.25816065699998));
#338387=CARTESIAN_POINT('Ctrl Pts',(3.35603130399994,12.2,3.25759688099998));
#338388=CARTESIAN_POINT('Ctrl Pts',(3.35603130399994,5.2,3.25759688099998));
#338389=CARTESIAN_POINT('Ctrl Pts',(3.35603130399994,2.2,3.25759688099998));
#338390=CARTESIAN_POINT('Ctrl Pts',(3.35354468599995,12.2,3.25703126499998));
#338391=CARTESIAN_POINT('Ctrl Pts',(3.35354468599995,5.2,3.25703126499998));
#338392=CARTESIAN_POINT('Ctrl Pts',(3.35354468599995,2.2,3.25703126499998));
#338393=CARTESIAN_POINT('Ctrl Pts',(3.35106205899995,12.2,3.25646381999999));
#338394=CARTESIAN_POINT('Ctrl Pts',(3.35106205899995,5.2,3.25646381999999));
#338395=CARTESIAN_POINT('Ctrl Pts',(3.35106205899995,2.2,3.25646381999999));
#338396=CARTESIAN_POINT('Ctrl Pts',(3.34858342799994,12.2,3.25589455099998));
#338397=CARTESIAN_POINT('Ctrl Pts',(3.34858342799994,5.2,3.25589455099998));
#338398=CARTESIAN_POINT('Ctrl Pts',(3.34858342799994,2.2,3.25589455099998));
#338399=CARTESIAN_POINT('Ctrl Pts',(3.34610879699994,12.2,3.25532346499998));
#338400=CARTESIAN_POINT('Ctrl Pts',(3.34610879699994,5.2,3.25532346499998));
#338401=CARTESIAN_POINT('Ctrl Pts',(3.34610879699994,2.2,3.25532346499998));
#338402=CARTESIAN_POINT('Ctrl Pts',(3.34363817199994,12.2,3.25475057199998));
#338403=CARTESIAN_POINT('Ctrl Pts',(3.34363817199994,5.2,3.25475057199998));
#338404=CARTESIAN_POINT('Ctrl Pts',(3.34363817199994,2.2,3.25475057199998));
#338405=CARTESIAN_POINT('Ctrl Pts',(3.34117155699994,12.2,3.25417587899998));
#338406=CARTESIAN_POINT('Ctrl Pts',(3.34117155699994,5.2,3.25417587899998));
#338407=CARTESIAN_POINT('Ctrl Pts',(3.34117155699994,2.2,3.25417587899998));
#338408=CARTESIAN_POINT('Ctrl Pts',(3.33870895599994,12.2,3.25359939099998));
#338409=CARTESIAN_POINT('Ctrl Pts',(3.33870895599994,5.2,3.25359939099998));
#338410=CARTESIAN_POINT('Ctrl Pts',(3.33870895599994,2.2,3.25359939099998));
#338411=CARTESIAN_POINT('Ctrl Pts',(3.33625037399994,12.2,3.25302111999999));
#338412=CARTESIAN_POINT('Ctrl Pts',(3.33625037399994,5.2,3.25302111999999));
#338413=CARTESIAN_POINT('Ctrl Pts',(3.33625037399994,2.2,3.25302111999999));
#338414=CARTESIAN_POINT('Ctrl Pts',(3.33379581499994,12.2,3.25244106999998));
#338415=CARTESIAN_POINT('Ctrl Pts',(3.33379581499994,5.2,3.25244106999998));
#338416=CARTESIAN_POINT('Ctrl Pts',(3.33379581499994,2.2,3.25244106999998));
#338417=CARTESIAN_POINT('Ctrl Pts',(3.33134528499994,12.2,3.25185924999998));
#338418=CARTESIAN_POINT('Ctrl Pts',(3.33134528499994,5.2,3.25185924999998));
#338419=CARTESIAN_POINT('Ctrl Pts',(3.33134528499994,2.2,3.25185924999998));
#338420=CARTESIAN_POINT('Ctrl Pts',(3.32889878899994,12.2,3.25127566799999));
#338421=CARTESIAN_POINT('Ctrl Pts',(3.32889878899994,5.2,3.25127566799999));
#338422=CARTESIAN_POINT('Ctrl Pts',(3.32889878899994,2.2,3.25127566799999));
#338423=CARTESIAN_POINT('Ctrl Pts',(3.32645632899994,12.2,3.25069033099999));
#338424=CARTESIAN_POINT('Ctrl Pts',(3.32645632899994,5.2,3.25069033099999));
#338425=CARTESIAN_POINT('Ctrl Pts',(3.32645632899994,2.2,3.25069033099999));
#338426=CARTESIAN_POINT('Ctrl Pts',(3.32401791099994,12.2,3.25010324799998));
#338427=CARTESIAN_POINT('Ctrl Pts',(3.32401791099994,5.2,3.25010324799998));
#338428=CARTESIAN_POINT('Ctrl Pts',(3.32401791099994,2.2,3.25010324799998));
#338429=CARTESIAN_POINT('Ctrl Pts',(3.32158353999994,12.2,3.24951442599998));
#338430=CARTESIAN_POINT('Ctrl Pts',(3.32158353999994,5.2,3.24951442599998));
#338431=CARTESIAN_POINT('Ctrl Pts',(3.32158353999994,2.2,3.24951442599998));
#338432=CARTESIAN_POINT('Ctrl Pts',(3.31915322099994,12.2,3.24892387199998));
#338433=CARTESIAN_POINT('Ctrl Pts',(3.31915322099994,5.2,3.24892387199998));
#338434=CARTESIAN_POINT('Ctrl Pts',(3.31915322099994,2.2,3.24892387199998));
#338435=CARTESIAN_POINT('Ctrl Pts',(3.31672695699994,12.2,3.24833159499998));
#338436=CARTESIAN_POINT('Ctrl Pts',(3.31672695699994,5.2,3.24833159499998));
#338437=CARTESIAN_POINT('Ctrl Pts',(3.31672695699994,2.2,3.24833159499998));
#338438=CARTESIAN_POINT('Ctrl Pts',(3.31430475199994,12.2,3.24773760199999));
#338439=CARTESIAN_POINT('Ctrl Pts',(3.31430475199994,5.2,3.24773760199999));
#338440=CARTESIAN_POINT('Ctrl Pts',(3.31430475199994,2.2,3.24773760199999));
#338441=CARTESIAN_POINT('Ctrl Pts',(3.31188661399994,12.2,3.24714190199998));
#338442=CARTESIAN_POINT('Ctrl Pts',(3.31188661399994,5.2,3.24714190199998));
#338443=CARTESIAN_POINT('Ctrl Pts',(3.31188661399994,2.2,3.24714190199998));
#338444=CARTESIAN_POINT('Ctrl Pts',(3.30947254399995,12.2,3.24654450099998));
#338445=CARTESIAN_POINT('Ctrl Pts',(3.30947254399995,5.2,3.24654450099998));
#338446=CARTESIAN_POINT('Ctrl Pts',(3.30947254399995,2.2,3.24654450099998));
#338447=CARTESIAN_POINT('Ctrl Pts',(3.30706254899995,12.2,3.24594540799998));
#338448=CARTESIAN_POINT('Ctrl Pts',(3.30706254899995,5.2,3.24594540799998));
#338449=CARTESIAN_POINT('Ctrl Pts',(3.30706254899995,2.2,3.24594540799998));
#338450=CARTESIAN_POINT('Ctrl Pts',(3.30465663199994,12.2,3.24534463199999));
#338451=CARTESIAN_POINT('Ctrl Pts',(3.30465663199994,5.2,3.24534463199999));
#338452=CARTESIAN_POINT('Ctrl Pts',(3.30465663199994,2.2,3.24534463199999));
#338453=CARTESIAN_POINT('Ctrl Pts',(3.30225479899994,12.2,3.24474217799998));
#338454=CARTESIAN_POINT('Ctrl Pts',(3.30225479899994,5.2,3.24474217799998));
#338455=CARTESIAN_POINT('Ctrl Pts',(3.30225479899994,2.2,3.24474217799998));
#338456=CARTESIAN_POINT('Ctrl Pts',(3.29985705299995,12.2,3.24413805699999));
#338457=CARTESIAN_POINT('Ctrl Pts',(3.29985705299995,5.2,3.24413805699999));
#338458=CARTESIAN_POINT('Ctrl Pts',(3.29985705299995,2.2,3.24413805699999));
#338459=CARTESIAN_POINT('Ctrl Pts',(3.29746339799994,12.2,3.24353227399998));
#338460=CARTESIAN_POINT('Ctrl Pts',(3.29746339799994,5.2,3.24353227399998));
#338461=CARTESIAN_POINT('Ctrl Pts',(3.29746339799994,2.2,3.24353227399998));
#338462=CARTESIAN_POINT('Ctrl Pts',(3.29507384099994,12.2,3.24292483899999));
#338463=CARTESIAN_POINT('Ctrl Pts',(3.29507384099994,5.2,3.24292483899999));
#338464=CARTESIAN_POINT('Ctrl Pts',(3.29507384099994,2.2,3.24292483899999));
#338465=CARTESIAN_POINT('Ctrl Pts',(3.29268838499994,12.2,3.24231575899999));
#338466=CARTESIAN_POINT('Ctrl Pts',(3.29268838499994,5.2,3.24231575899999));
#338467=CARTESIAN_POINT('Ctrl Pts',(3.29268838499994,2.2,3.24231575899999));
#338468=CARTESIAN_POINT('Ctrl Pts',(3.29030703499994,12.2,3.24170504199999));
#338469=CARTESIAN_POINT('Ctrl Pts',(3.29030703499994,5.2,3.24170504199999));
#338470=CARTESIAN_POINT('Ctrl Pts',(3.29030703499994,2.2,3.24170504199999));
#338471=CARTESIAN_POINT('Ctrl Pts',(3.28792979399994,12.2,3.24109269699999));
#338472=CARTESIAN_POINT('Ctrl Pts',(3.28792979399994,5.2,3.24109269699999));
#338473=CARTESIAN_POINT('Ctrl Pts',(3.28792979399994,2.2,3.24109269699999));
#338474=CARTESIAN_POINT('Ctrl Pts',(3.28555666899994,12.2,3.24047873199999));
#338475=CARTESIAN_POINT('Ctrl Pts',(3.28555666899994,5.2,3.24047873199999));
#338476=CARTESIAN_POINT('Ctrl Pts',(3.28555666899994,2.2,3.24047873199999));
#338477=CARTESIAN_POINT('Ctrl Pts',(3.28318766199994,12.2,3.23986315299998));
#338478=CARTESIAN_POINT('Ctrl Pts',(3.28318766199994,5.2,3.23986315299998));
#338479=CARTESIAN_POINT('Ctrl Pts',(3.28318766199994,2.2,3.23986315299998));
#338480=CARTESIAN_POINT('Ctrl Pts',(3.28082277999994,12.2,3.23924596999999));
#338481=CARTESIAN_POINT('Ctrl Pts',(3.28082277999994,5.2,3.23924596999999));
#338482=CARTESIAN_POINT('Ctrl Pts',(3.28082277999994,2.2,3.23924596999999));
#338483=CARTESIAN_POINT('Ctrl Pts',(3.27846202599994,12.2,3.23862718999998));
#338484=CARTESIAN_POINT('Ctrl Pts',(3.27846202599994,5.2,3.23862718999998));
#338485=CARTESIAN_POINT('Ctrl Pts',(3.27846202599994,2.2,3.23862718999998));
#338486=CARTESIAN_POINT('Ctrl Pts',(3.27610540399994,12.2,3.23800682099999));
#338487=CARTESIAN_POINT('Ctrl Pts',(3.27610540399994,5.2,3.23800682099999));
#338488=CARTESIAN_POINT('Ctrl Pts',(3.27610540399994,2.2,3.23800682099999));
#338489=CARTESIAN_POINT('Ctrl Pts',(3.27375291999994,12.2,3.23738487199999));
#338490=CARTESIAN_POINT('Ctrl Pts',(3.27375291999994,5.2,3.23738487199999));
#338491=CARTESIAN_POINT('Ctrl Pts',(3.27375291999994,2.2,3.23738487199999));
#338492=CARTESIAN_POINT('Ctrl Pts',(3.27140457599994,12.2,3.23676135099999));
#338493=CARTESIAN_POINT('Ctrl Pts',(3.27140457599994,5.2,3.23676135099999));
#338494=CARTESIAN_POINT('Ctrl Pts',(3.27140457599994,2.2,3.23676135099999));
#338495=CARTESIAN_POINT('Ctrl Pts',(3.26906037999994,12.2,3.23613626499998));
#338496=CARTESIAN_POINT('Ctrl Pts',(3.26906037999994,5.2,3.23613626499998));
#338497=CARTESIAN_POINT('Ctrl Pts',(3.26906037999994,2.2,3.23613626499998));
#338498=CARTESIAN_POINT('Ctrl Pts',(3.26672033299995,12.2,3.23550962299999));
#338499=CARTESIAN_POINT('Ctrl Pts',(3.26672033299995,5.2,3.23550962299999));
#338500=CARTESIAN_POINT('Ctrl Pts',(3.26672033299995,2.2,3.23550962299999));
#338501=CARTESIAN_POINT('Ctrl Pts',(3.26438444199994,12.2,3.23488143299999));
#338502=CARTESIAN_POINT('Ctrl Pts',(3.26438444199994,5.2,3.23488143299999));
#338503=CARTESIAN_POINT('Ctrl Pts',(3.26438444199994,2.2,3.23488143299999));
#338504=CARTESIAN_POINT('Ctrl Pts',(3.26205271099994,12.2,3.23425170299998));
#338505=CARTESIAN_POINT('Ctrl Pts',(3.26205271099994,5.2,3.23425170299998));
#338506=CARTESIAN_POINT('Ctrl Pts',(3.26205271099994,2.2,3.23425170299998));
#338507=CARTESIAN_POINT('Ctrl Pts',(3.25972514299994,12.2,3.23362044099999));
#338508=CARTESIAN_POINT('Ctrl Pts',(3.25972514299994,5.2,3.23362044099999));
#338509=CARTESIAN_POINT('Ctrl Pts',(3.25972514299994,2.2,3.23362044099999));
#338510=CARTESIAN_POINT('Ctrl Pts',(3.25740174399994,12.2,3.23298765599999));
#338511=CARTESIAN_POINT('Ctrl Pts',(3.25740174399994,5.2,3.23298765599999));
#338512=CARTESIAN_POINT('Ctrl Pts',(3.25740174399994,2.2,3.23298765599999));
#338513=CARTESIAN_POINT('Ctrl Pts',(3.25508251599994,12.2,3.23235335699999));
#338514=CARTESIAN_POINT('Ctrl Pts',(3.25508251599994,5.2,3.23235335699999));
#338515=CARTESIAN_POINT('Ctrl Pts',(3.25508251599994,2.2,3.23235335699999));
#338516=CARTESIAN_POINT('Ctrl Pts',(3.25276746699994,12.2,3.23171754899998));
#338517=CARTESIAN_POINT('Ctrl Pts',(3.25276746699994,5.2,3.23171754899998));
#338518=CARTESIAN_POINT('Ctrl Pts',(3.25276746699994,2.2,3.23171754899998));
#338519=CARTESIAN_POINT('Ctrl Pts',(3.25045659899994,12.2,3.23108024299999));
#338520=CARTESIAN_POINT('Ctrl Pts',(3.25045659899994,5.2,3.23108024299999));
#338521=CARTESIAN_POINT('Ctrl Pts',(3.25045659899994,2.2,3.23108024299999));
#338522=CARTESIAN_POINT('Ctrl Pts',(3.24814991699995,12.2,3.23044144699999));
#338523=CARTESIAN_POINT('Ctrl Pts',(3.24814991699995,5.2,3.23044144699999));
#338524=CARTESIAN_POINT('Ctrl Pts',(3.24814991699995,2.2,3.23044144699999));
#338525=CARTESIAN_POINT('Ctrl Pts',(3.24584742499994,12.2,3.22980116799998));
#338526=CARTESIAN_POINT('Ctrl Pts',(3.24584742499994,5.2,3.22980116799998));
#338527=CARTESIAN_POINT('Ctrl Pts',(3.24584742499994,2.2,3.22980116799998));
#338528=CARTESIAN_POINT('Ctrl Pts',(3.24354912899994,12.2,3.22915941499998));
#338529=CARTESIAN_POINT('Ctrl Pts',(3.24354912899994,5.2,3.22915941499998));
#338530=CARTESIAN_POINT('Ctrl Pts',(3.24354912899994,2.2,3.22915941499998));
#338531=CARTESIAN_POINT('Ctrl Pts',(3.24125503199994,12.2,3.22851619699998));
#338532=CARTESIAN_POINT('Ctrl Pts',(3.24125503199994,5.2,3.22851619699998));
#338533=CARTESIAN_POINT('Ctrl Pts',(3.24125503199994,2.2,3.22851619699998));
#338534=CARTESIAN_POINT('Ctrl Pts',(3.23896513799995,12.2,3.22787152099998));
#338535=CARTESIAN_POINT('Ctrl Pts',(3.23896513799995,5.2,3.22787152099998));
#338536=CARTESIAN_POINT('Ctrl Pts',(3.23896513799995,2.2,3.22787152099998));
#338537=CARTESIAN_POINT('Ctrl Pts',(3.23667945299994,12.2,3.22722539699999));
#338538=CARTESIAN_POINT('Ctrl Pts',(3.23667945299994,5.2,3.22722539699999));
#338539=CARTESIAN_POINT('Ctrl Pts',(3.23667945299994,2.2,3.22722539699999));
#338540=CARTESIAN_POINT('Ctrl Pts',(3.23439797999994,12.2,3.22657783099999));
#338541=CARTESIAN_POINT('Ctrl Pts',(3.23439797999994,5.2,3.22657783099999));
#338542=CARTESIAN_POINT('Ctrl Pts',(3.23439797999994,2.2,3.22657783099999));
#338543=CARTESIAN_POINT('Ctrl Pts',(3.23212072399994,12.2,3.22592883399999));
#338544=CARTESIAN_POINT('Ctrl Pts',(3.23212072399994,5.2,3.22592883399999));
#338545=CARTESIAN_POINT('Ctrl Pts',(3.23212072399994,2.2,3.22592883399999));
#338546=CARTESIAN_POINT('Ctrl Pts',(3.22984768899994,12.2,3.22527841199998));
#338547=CARTESIAN_POINT('Ctrl Pts',(3.22984768899994,5.2,3.22527841199998));
#338548=CARTESIAN_POINT('Ctrl Pts',(3.22984768899994,2.2,3.22527841199998));
#338549=CARTESIAN_POINT('Ctrl Pts',(3.22757887999995,12.2,3.22462657599999));
#338550=CARTESIAN_POINT('Ctrl Pts',(3.22757887999995,5.2,3.22462657599999));
#338551=CARTESIAN_POINT('Ctrl Pts',(3.22757887999995,2.2,3.22462657599999));
#338552=CARTESIAN_POINT('Ctrl Pts',(3.22531429999994,12.2,3.22397333299998));
#338553=CARTESIAN_POINT('Ctrl Pts',(3.22531429999994,5.2,3.22397333299998));
#338554=CARTESIAN_POINT('Ctrl Pts',(3.22531429999994,2.2,3.22397333299998));
#338555=CARTESIAN_POINT('Ctrl Pts',(3.22305395499995,12.2,3.22331869099998));
#338556=CARTESIAN_POINT('Ctrl Pts',(3.22305395499995,5.2,3.22331869099998));
#338557=CARTESIAN_POINT('Ctrl Pts',(3.22305395499995,2.2,3.22331869099998));
#338558=CARTESIAN_POINT('Ctrl Pts',(3.22079784899994,12.2,3.22266265899999));
#338559=CARTESIAN_POINT('Ctrl Pts',(3.22079784899994,5.2,3.22266265899999));
#338560=CARTESIAN_POINT('Ctrl Pts',(3.22079784899994,2.2,3.22266265899999));
#338561=CARTESIAN_POINT('Ctrl Pts',(3.21854598499994,12.2,3.22200524599998));
#338562=CARTESIAN_POINT('Ctrl Pts',(3.21854598499994,5.2,3.22200524599998));
#338563=CARTESIAN_POINT('Ctrl Pts',(3.21854598499994,2.2,3.22200524599998));
#338564=CARTESIAN_POINT('Ctrl Pts',(3.21629836899994,12.2,3.22134645899999));
#338565=CARTESIAN_POINT('Ctrl Pts',(3.21629836899994,5.2,3.22134645899999));
#338566=CARTESIAN_POINT('Ctrl Pts',(3.21629836899994,2.2,3.22134645899999));
#338567=CARTESIAN_POINT('Ctrl Pts',(3.21405500399994,12.2,3.22068630799999));
#338568=CARTESIAN_POINT('Ctrl Pts',(3.21405500399994,5.2,3.22068630799999));
#338569=CARTESIAN_POINT('Ctrl Pts',(3.21405500399994,2.2,3.22068630799999));
#338570=CARTESIAN_POINT('Ctrl Pts',(3.21181589499994,12.2,3.22002480099999));
#338571=CARTESIAN_POINT('Ctrl Pts',(3.21181589499994,5.2,3.22002480099999));
#338572=CARTESIAN_POINT('Ctrl Pts',(3.21181589499994,2.2,3.22002480099999));
#338573=CARTESIAN_POINT('Ctrl Pts',(3.20958104699994,12.2,3.21936194599999));
#338574=CARTESIAN_POINT('Ctrl Pts',(3.20958104699994,5.2,3.21936194599999));
#338575=CARTESIAN_POINT('Ctrl Pts',(3.20958104699994,2.2,3.21936194599999));
#338576=CARTESIAN_POINT('Ctrl Pts',(3.20735046399995,12.2,3.21869775299999));
#338577=CARTESIAN_POINT('Ctrl Pts',(3.20735046399995,5.2,3.21869775299999));
#338578=CARTESIAN_POINT('Ctrl Pts',(3.20735046399995,2.2,3.21869775299999));
#338579=CARTESIAN_POINT('Ctrl Pts',(3.20512414899994,12.2,3.21803222899998));
#338580=CARTESIAN_POINT('Ctrl Pts',(3.20512414899994,5.2,3.21803222899998));
#338581=CARTESIAN_POINT('Ctrl Pts',(3.20512414899994,2.2,3.21803222899998));
#338582=CARTESIAN_POINT('Ctrl Pts',(3.20290210799994,12.2,3.21736538499999));
#338583=CARTESIAN_POINT('Ctrl Pts',(3.20290210799994,5.2,3.21736538499999));
#338584=CARTESIAN_POINT('Ctrl Pts',(3.20290210799994,2.2,3.21736538499999));
#338585=CARTESIAN_POINT('Ctrl Pts',(3.20068434399994,12.2,3.21669722699998));
#338586=CARTESIAN_POINT('Ctrl Pts',(3.20068434399994,5.2,3.21669722699998));
#338587=CARTESIAN_POINT('Ctrl Pts',(3.20068434399994,2.2,3.21669722699998));
#338588=CARTESIAN_POINT('Ctrl Pts',(3.19847086099994,12.2,3.21602776399998));
#338589=CARTESIAN_POINT('Ctrl Pts',(3.19847086099994,5.2,3.21602776399998));
#338590=CARTESIAN_POINT('Ctrl Pts',(3.19847086099994,2.2,3.21602776399998));
#338591=CARTESIAN_POINT('Ctrl Pts',(3.19626166499994,12.2,3.21535700599998));
#338592=CARTESIAN_POINT('Ctrl Pts',(3.19626166499994,5.2,3.21535700599998));
#338593=CARTESIAN_POINT('Ctrl Pts',(3.19626166499994,2.2,3.21535700599998));
#338594=CARTESIAN_POINT('Ctrl Pts',(3.19405675999994,12.2,3.21468495999999));
#338595=CARTESIAN_POINT('Ctrl Pts',(3.19405675999994,5.2,3.21468495999999));
#338596=CARTESIAN_POINT('Ctrl Pts',(3.19405675999994,2.2,3.21468495999999));
#338597=CARTESIAN_POINT('Ctrl Pts',(3.19185614899994,12.2,3.21401163799998));
#338598=CARTESIAN_POINT('Ctrl Pts',(3.19185614899994,5.2,3.21401163799998));
#338599=CARTESIAN_POINT('Ctrl Pts',(3.19185614899994,2.2,3.21401163799998));
#338600=CARTESIAN_POINT('Ctrl Pts',(3.18965983699994,12.2,3.21333704399999));
#338601=CARTESIAN_POINT('Ctrl Pts',(3.18965983699994,5.2,3.21333704399999));
#338602=CARTESIAN_POINT('Ctrl Pts',(3.18965983699994,2.2,3.21333704399999));
#338603=CARTESIAN_POINT('Ctrl Pts',(3.18746782799994,12.2,3.21266118999999));
#338604=CARTESIAN_POINT('Ctrl Pts',(3.18746782799994,5.2,3.21266118999999));
#338605=CARTESIAN_POINT('Ctrl Pts',(3.18746782799994,2.2,3.21266118999999));
#338606=CARTESIAN_POINT('Ctrl Pts',(3.18528012699994,12.2,3.21198408399999));
#338607=CARTESIAN_POINT('Ctrl Pts',(3.18528012699994,5.2,3.21198408399999));
#338608=CARTESIAN_POINT('Ctrl Pts',(3.18528012699994,2.2,3.21198408399999));
#338609=CARTESIAN_POINT('Ctrl Pts',(3.18309673699994,12.2,3.21130573399999));
#338610=CARTESIAN_POINT('Ctrl Pts',(3.18309673699994,5.2,3.21130573399999));
#338611=CARTESIAN_POINT('Ctrl Pts',(3.18309673699994,2.2,3.21130573399999));
#338612=CARTESIAN_POINT('Ctrl Pts',(3.18091766399994,12.2,3.21062614999998));
#338613=CARTESIAN_POINT('Ctrl Pts',(3.18091766399994,5.2,3.21062614999998));
#338614=CARTESIAN_POINT('Ctrl Pts',(3.18091766399994,2.2,3.21062614999998));
#338615=CARTESIAN_POINT('Ctrl Pts',(3.17874290899995,12.2,3.20994534099999));
#338616=CARTESIAN_POINT('Ctrl Pts',(3.17874290899995,5.2,3.20994534099999));
#338617=CARTESIAN_POINT('Ctrl Pts',(3.17874290899995,2.2,3.20994534099999));
#338618=CARTESIAN_POINT('Ctrl Pts',(3.17657247999994,12.2,3.20926331399999));
#338619=CARTESIAN_POINT('Ctrl Pts',(3.17657247999994,5.2,3.20926331399999));
#338620=CARTESIAN_POINT('Ctrl Pts',(3.17657247999994,2.2,3.20926331399999));
#338621=CARTESIAN_POINT('Ctrl Pts',(3.17440637999994,12.2,3.20858007899999));
#338622=CARTESIAN_POINT('Ctrl Pts',(3.17440637999994,5.2,3.20858007899999));
#338623=CARTESIAN_POINT('Ctrl Pts',(3.17440637999994,2.2,3.20858007899999));
#338624=CARTESIAN_POINT('Ctrl Pts',(3.17224461299995,12.2,3.20789564499999));
#338625=CARTESIAN_POINT('Ctrl Pts',(3.17224461299995,5.2,3.20789564499999));
#338626=CARTESIAN_POINT('Ctrl Pts',(3.17224461299995,2.2,3.20789564499999));
#338627=CARTESIAN_POINT('Ctrl Pts',(3.17008718199994,12.2,3.20721002099998));
#338628=CARTESIAN_POINT('Ctrl Pts',(3.17008718199994,5.2,3.20721002099998));
#338629=CARTESIAN_POINT('Ctrl Pts',(3.17008718199994,2.2,3.20721002099998));
#338630=CARTESIAN_POINT('Ctrl Pts',(3.16793409199994,12.2,3.20652321499999));
#338631=CARTESIAN_POINT('Ctrl Pts',(3.16793409199994,5.2,3.20652321499999));
#338632=CARTESIAN_POINT('Ctrl Pts',(3.16793409199994,2.2,3.20652321499999));
#338633=CARTESIAN_POINT('Ctrl Pts',(3.16578534799994,12.2,3.20583523599999));
#338634=CARTESIAN_POINT('Ctrl Pts',(3.16578534799994,5.2,3.20583523599999));
#338635=CARTESIAN_POINT('Ctrl Pts',(3.16578534799994,2.2,3.20583523599999));
#338636=CARTESIAN_POINT('Ctrl Pts',(3.16364095399994,12.2,3.20514609399999));
#338637=CARTESIAN_POINT('Ctrl Pts',(3.16364095399994,5.2,3.20514609399999));
#338638=CARTESIAN_POINT('Ctrl Pts',(3.16364095399994,2.2,3.20514609399999));
#338639=CARTESIAN_POINT('Ctrl Pts',(3.16150091399995,12.2,3.20445579799999));
#338640=CARTESIAN_POINT('Ctrl Pts',(3.16150091399995,5.2,3.20445579799999));
#338641=CARTESIAN_POINT('Ctrl Pts',(3.16150091399995,2.2,3.20445579799999));
#338642=CARTESIAN_POINT('Ctrl Pts',(3.15936523199994,12.2,3.20376435599999));
#338643=CARTESIAN_POINT('Ctrl Pts',(3.15936523199994,5.2,3.20376435599999));
#338644=CARTESIAN_POINT('Ctrl Pts',(3.15936523199994,2.2,3.20376435599999));
#338645=CARTESIAN_POINT('Ctrl Pts',(3.15723391199994,12.2,3.20307177699998));
#338646=CARTESIAN_POINT('Ctrl Pts',(3.15723391199994,5.2,3.20307177699998));
#338647=CARTESIAN_POINT('Ctrl Pts',(3.15723391199994,2.2,3.20307177699998));
#338648=CARTESIAN_POINT('Ctrl Pts',(3.15510695899994,12.2,3.20237806899998));
#338649=CARTESIAN_POINT('Ctrl Pts',(3.15510695899994,5.2,3.20237806899998));
#338650=CARTESIAN_POINT('Ctrl Pts',(3.15510695899994,2.2,3.20237806899998));
#338651=CARTESIAN_POINT('Ctrl Pts',(3.15298437499994,12.2,3.20168324399998));
#338652=CARTESIAN_POINT('Ctrl Pts',(3.15298437499994,5.2,3.20168324399998));
#338653=CARTESIAN_POINT('Ctrl Pts',(3.15298437499994,2.2,3.20168324399998));
#338654=CARTESIAN_POINT('Ctrl Pts',(3.15086616699995,12.2,3.20098730899999));
#338655=CARTESIAN_POINT('Ctrl Pts',(3.15086616699995,5.2,3.20098730899999));
#338656=CARTESIAN_POINT('Ctrl Pts',(3.15086616699995,2.2,3.20098730899999));
#338657=CARTESIAN_POINT('Ctrl Pts',(3.14875233699994,12.2,3.20029027299999));
#338658=CARTESIAN_POINT('Ctrl Pts',(3.14875233699994,5.2,3.20029027299999));
#338659=CARTESIAN_POINT('Ctrl Pts',(3.14875233699994,2.2,3.20029027299999));
#338660=CARTESIAN_POINT('Ctrl Pts',(3.14664288999994,12.2,3.19959214699999));
#338661=CARTESIAN_POINT('Ctrl Pts',(3.14664288999994,5.2,3.19959214699999));
#338662=CARTESIAN_POINT('Ctrl Pts',(3.14664288999994,2.2,3.19959214699999));
#338663=CARTESIAN_POINT('Ctrl Pts',(3.14453782999994,12.2,3.19889293699998));
#338664=CARTESIAN_POINT('Ctrl Pts',(3.14453782999994,5.2,3.19889293699998));
#338665=CARTESIAN_POINT('Ctrl Pts',(3.14453782999994,2.2,3.19889293699998));
#338666=CARTESIAN_POINT('Ctrl Pts',(3.14243716299994,12.2,3.19819265399998));
#338667=CARTESIAN_POINT('Ctrl Pts',(3.14243716299994,5.2,3.19819265399998));
#338668=CARTESIAN_POINT('Ctrl Pts',(3.14243716299994,2.2,3.19819265399998));
#338669=CARTESIAN_POINT('Ctrl Pts',(3.14034088999994,12.2,3.19749130699999));
#338670=CARTESIAN_POINT('Ctrl Pts',(3.14034088999994,5.2,3.19749130699999));
#338671=CARTESIAN_POINT('Ctrl Pts',(3.14034088999994,2.2,3.19749130699999));
#338672=CARTESIAN_POINT('Ctrl Pts',(3.13824901599994,12.2,3.19678890499999));
#338673=CARTESIAN_POINT('Ctrl Pts',(3.13824901599994,5.2,3.19678890499999));
#338674=CARTESIAN_POINT('Ctrl Pts',(3.13824901599994,2.2,3.19678890499999));
#338675=CARTESIAN_POINT('Ctrl Pts',(3.13616154599994,12.2,3.19608545799999));
#338676=CARTESIAN_POINT('Ctrl Pts',(3.13616154599994,5.2,3.19608545799999));
#338677=CARTESIAN_POINT('Ctrl Pts',(3.13616154599994,2.2,3.19608545799999));
#338678=CARTESIAN_POINT('Ctrl Pts',(3.13407848399994,12.2,3.19538097399998));
#338679=CARTESIAN_POINT('Ctrl Pts',(3.13407848399994,5.2,3.19538097399998));
#338680=CARTESIAN_POINT('Ctrl Pts',(3.13407848399994,2.2,3.19538097399998));
#338681=CARTESIAN_POINT('Ctrl Pts',(3.13199983299994,12.2,3.19467546199999));
#338682=CARTESIAN_POINT('Ctrl Pts',(3.13199983299994,5.2,3.19467546199999));
#338683=CARTESIAN_POINT('Ctrl Pts',(3.13199983299994,2.2,3.19467546199999));
#338684=CARTESIAN_POINT('Ctrl Pts',(3.12992559899994,12.2,3.19396893199999));
#338685=CARTESIAN_POINT('Ctrl Pts',(3.12992559899994,5.2,3.19396893199999));
#338686=CARTESIAN_POINT('Ctrl Pts',(3.12992559899994,2.2,3.19396893199999));
#338687=CARTESIAN_POINT('Ctrl Pts',(3.12785578499994,12.2,3.19326139299999));
#338688=CARTESIAN_POINT('Ctrl Pts',(3.12785578499994,5.2,3.19326139299999));
#338689=CARTESIAN_POINT('Ctrl Pts',(3.12785578499994,2.2,3.19326139299999));
#338690=CARTESIAN_POINT('Ctrl Pts',(3.12579039399994,12.2,3.19255285499998));
#338691=CARTESIAN_POINT('Ctrl Pts',(3.12579039399994,5.2,3.19255285499998));
#338692=CARTESIAN_POINT('Ctrl Pts',(3.12579039399994,2.2,3.19255285499998));
#338693=CARTESIAN_POINT('Ctrl Pts',(3.12372943099994,12.2,3.19184332599999));
#338694=CARTESIAN_POINT('Ctrl Pts',(3.12372943099994,5.2,3.19184332599999));
#338695=CARTESIAN_POINT('Ctrl Pts',(3.12372943099994,2.2,3.19184332599999));
#338696=CARTESIAN_POINT('Ctrl Pts',(3.12167290099994,12.2,3.19113281599999));
#338697=CARTESIAN_POINT('Ctrl Pts',(3.12167290099994,5.2,3.19113281599999));
#338698=CARTESIAN_POINT('Ctrl Pts',(3.12167290099994,2.2,3.19113281599999));
#338699=CARTESIAN_POINT('Ctrl Pts',(3.11962080699994,12.2,3.19042133399999));
#338700=CARTESIAN_POINT('Ctrl Pts',(3.11962080699994,5.2,3.19042133399999));
#338701=CARTESIAN_POINT('Ctrl Pts',(3.11962080699994,2.2,3.19042133399999));
#338702=CARTESIAN_POINT('Ctrl Pts',(3.11757315299994,12.2,3.18970889099998));
#338703=CARTESIAN_POINT('Ctrl Pts',(3.11757315299994,5.2,3.18970889099998));
#338704=CARTESIAN_POINT('Ctrl Pts',(3.11757315299994,2.2,3.18970889099998));
#338705=CARTESIAN_POINT('Ctrl Pts',(3.11552994399994,12.2,3.18899549399998));
#338706=CARTESIAN_POINT('Ctrl Pts',(3.11552994399994,5.2,3.18899549399998));
#338707=CARTESIAN_POINT('Ctrl Pts',(3.11552994399994,2.2,3.18899549399998));
#338708=CARTESIAN_POINT('Ctrl Pts',(3.11349118199994,12.2,3.18828115299999));
#338709=CARTESIAN_POINT('Ctrl Pts',(3.11349118199994,5.2,3.18828115299999));
#338710=CARTESIAN_POINT('Ctrl Pts',(3.11349118199994,2.2,3.18828115299999));
#338711=CARTESIAN_POINT('Ctrl Pts',(3.11145687399994,12.2,3.18756587899999));
#338712=CARTESIAN_POINT('Ctrl Pts',(3.11145687399994,5.2,3.18756587899999));
#338713=CARTESIAN_POINT('Ctrl Pts',(3.11145687399994,2.2,3.18756587899999));
#338714=CARTESIAN_POINT('Ctrl Pts',(3.10942702099994,12.2,3.18684967899999));
#338715=CARTESIAN_POINT('Ctrl Pts',(3.10942702099994,5.2,3.18684967899999));
#338716=CARTESIAN_POINT('Ctrl Pts',(3.10942702099994,2.2,3.18684967899999));
#338717=CARTESIAN_POINT('Ctrl Pts',(3.10740162899994,12.2,3.18613256399999));
#338718=CARTESIAN_POINT('Ctrl Pts',(3.10740162899994,5.2,3.18613256399999));
#338719=CARTESIAN_POINT('Ctrl Pts',(3.10740162899994,2.2,3.18613256399999));
#338720=CARTESIAN_POINT('Ctrl Pts',(3.10538070199994,12.2,3.18541454299999));
#338721=CARTESIAN_POINT('Ctrl Pts',(3.10538070199994,5.2,3.18541454299999));
#338722=CARTESIAN_POINT('Ctrl Pts',(3.10538070199994,2.2,3.18541454299999));
#338723=CARTESIAN_POINT('Ctrl Pts',(3.10336424299994,12.2,3.18469562499998));
#338724=CARTESIAN_POINT('Ctrl Pts',(3.10336424299994,5.2,3.18469562499998));
#338725=CARTESIAN_POINT('Ctrl Pts',(3.10336424299994,2.2,3.18469562499998));
#338726=CARTESIAN_POINT('Ctrl Pts',(3.10135225599995,12.2,3.18397582199999));
#338727=CARTESIAN_POINT('Ctrl Pts',(3.10135225599995,5.2,3.18397582199999));
#338728=CARTESIAN_POINT('Ctrl Pts',(3.10135225599995,2.2,3.18397582199999));
#338729=CARTESIAN_POINT('Ctrl Pts',(3.09934474499994,12.2,3.18325513999999));
#338730=CARTESIAN_POINT('Ctrl Pts',(3.09934474499994,5.2,3.18325513999999));
#338731=CARTESIAN_POINT('Ctrl Pts',(3.09934474499994,2.2,3.18325513999999));
#338732=CARTESIAN_POINT('Ctrl Pts',(3.09734171599994,12.2,3.18253358999999));
#338733=CARTESIAN_POINT('Ctrl Pts',(3.09734171599994,5.2,3.18253358999999));
#338734=CARTESIAN_POINT('Ctrl Pts',(3.09734171599994,2.2,3.18253358999999));
#338735=CARTESIAN_POINT('Ctrl Pts',(3.09534316999994,12.2,3.18181118299999));
#338736=CARTESIAN_POINT('Ctrl Pts',(3.09534316999994,5.2,3.18181118299999));
#338737=CARTESIAN_POINT('Ctrl Pts',(3.09534316999994,2.2,3.18181118299999));
#338738=CARTESIAN_POINT('Ctrl Pts',(3.09334911199994,12.2,3.18108792599999));
#338739=CARTESIAN_POINT('Ctrl Pts',(3.09334911199994,5.2,3.18108792599999));
#338740=CARTESIAN_POINT('Ctrl Pts',(3.09334911199994,2.2,3.18108792599999));
#338741=CARTESIAN_POINT('Ctrl Pts',(3.09135954699994,12.2,3.18036382999999));
#338742=CARTESIAN_POINT('Ctrl Pts',(3.09135954699994,5.2,3.18036382999999));
#338743=CARTESIAN_POINT('Ctrl Pts',(3.09135954699994,2.2,3.18036382999999));
#338744=CARTESIAN_POINT('Ctrl Pts',(3.08937447799994,12.2,3.17963890499998));
#338745=CARTESIAN_POINT('Ctrl Pts',(3.08937447799994,5.2,3.17963890499998));
#338746=CARTESIAN_POINT('Ctrl Pts',(3.08937447799994,2.2,3.17963890499998));
#338747=CARTESIAN_POINT('Ctrl Pts',(3.08739390899994,12.2,3.17891316099999));
#338748=CARTESIAN_POINT('Ctrl Pts',(3.08739390899994,5.2,3.17891316099999));
#338749=CARTESIAN_POINT('Ctrl Pts',(3.08739390899994,2.2,3.17891316099999));
#338750=CARTESIAN_POINT('Ctrl Pts',(3.08541784499994,12.2,3.17818660599999));
#338751=CARTESIAN_POINT('Ctrl Pts',(3.08541784499994,5.2,3.17818660599999));
#338752=CARTESIAN_POINT('Ctrl Pts',(3.08541784499994,2.2,3.17818660599999));
#338753=CARTESIAN_POINT('Ctrl Pts',(3.08344628799994,12.2,3.17745925099998));
#338754=CARTESIAN_POINT('Ctrl Pts',(3.08344628799994,5.2,3.17745925099998));
#338755=CARTESIAN_POINT('Ctrl Pts',(3.08344628799994,2.2,3.17745925099998));
#338756=CARTESIAN_POINT('Ctrl Pts',(3.08147924299994,12.2,3.17673110399999));
#338757=CARTESIAN_POINT('Ctrl Pts',(3.08147924299994,5.2,3.17673110399999));
#338758=CARTESIAN_POINT('Ctrl Pts',(3.08147924299994,2.2,3.17673110399999));
#338759=CARTESIAN_POINT('Ctrl Pts',(3.07951671499994,12.2,3.17600217599999));
#338760=CARTESIAN_POINT('Ctrl Pts',(3.07951671499994,5.2,3.17600217599999));
#338761=CARTESIAN_POINT('Ctrl Pts',(3.07951671499994,2.2,3.17600217599999));
#338762=CARTESIAN_POINT('Ctrl Pts',(3.07755870499994,12.2,3.17527247699999));
#338763=CARTESIAN_POINT('Ctrl Pts',(3.07755870499994,5.2,3.17527247699999));
#338764=CARTESIAN_POINT('Ctrl Pts',(3.07755870499994,2.2,3.17527247699999));
#338765=CARTESIAN_POINT('Ctrl Pts',(3.07560521899994,12.2,3.17454201799999));
#338766=CARTESIAN_POINT('Ctrl Pts',(3.07560521899994,5.2,3.17454201799999));
#338767=CARTESIAN_POINT('Ctrl Pts',(3.07560521899994,2.2,3.17454201799999));
#338768=CARTESIAN_POINT('Ctrl Pts',(3.07365626099994,12.2,3.17381080499998));
#338769=CARTESIAN_POINT('Ctrl Pts',(3.07365626099994,5.2,3.17381080499998));
#338770=CARTESIAN_POINT('Ctrl Pts',(3.07365626099994,2.2,3.17381080499998));
#338771=CARTESIAN_POINT('Ctrl Pts',(3.07171183499995,12.2,3.17307885099999));
#338772=CARTESIAN_POINT('Ctrl Pts',(3.07171183499995,5.2,3.17307885099999));
#338773=CARTESIAN_POINT('Ctrl Pts',(3.07171183499995,2.2,3.17307885099999));
#338774=CARTESIAN_POINT('Ctrl Pts',(3.06977194399995,12.2,3.17234616499999));
#338775=CARTESIAN_POINT('Ctrl Pts',(3.06977194399995,5.2,3.17234616499999));
#338776=CARTESIAN_POINT('Ctrl Pts',(3.06977194399995,2.2,3.17234616499999));
#338777=CARTESIAN_POINT('Ctrl Pts',(3.06783659099994,12.2,3.17161275499998));
#338778=CARTESIAN_POINT('Ctrl Pts',(3.06783659099994,5.2,3.17161275499998));
#338779=CARTESIAN_POINT('Ctrl Pts',(3.06783659099994,2.2,3.17161275499998));
#338780=CARTESIAN_POINT('Ctrl Pts',(3.06590578199994,12.2,3.17087863499999));
#338781=CARTESIAN_POINT('Ctrl Pts',(3.06590578199994,5.2,3.17087863499999));
#338782=CARTESIAN_POINT('Ctrl Pts',(3.06590578199994,2.2,3.17087863499999));
#338783=CARTESIAN_POINT('Ctrl Pts',(3.06397951999994,12.2,3.17014381099998));
#338784=CARTESIAN_POINT('Ctrl Pts',(3.06397951999994,5.2,3.17014381099998));
#338785=CARTESIAN_POINT('Ctrl Pts',(3.06397951999994,2.2,3.17014381099998));
#338786=CARTESIAN_POINT('Ctrl Pts',(3.06205780799994,12.2,3.16940829399999));
#338787=CARTESIAN_POINT('Ctrl Pts',(3.06205780799994,5.2,3.16940829399999));
#338788=CARTESIAN_POINT('Ctrl Pts',(3.06205780799994,2.2,3.16940829399999));
#338789=CARTESIAN_POINT('Ctrl Pts',(3.06014065099995,12.2,3.16867209499998));
#338790=CARTESIAN_POINT('Ctrl Pts',(3.06014065099995,5.2,3.16867209499998));
#338791=CARTESIAN_POINT('Ctrl Pts',(3.06014065099995,2.2,3.16867209499998));
#338792=CARTESIAN_POINT('Ctrl Pts',(3.05822805299994,12.2,3.16793522299999));
#338793=CARTESIAN_POINT('Ctrl Pts',(3.05822805299994,5.2,3.16793522299999));
#338794=CARTESIAN_POINT('Ctrl Pts',(3.05822805299994,2.2,3.16793522299999));
#338795=CARTESIAN_POINT('Ctrl Pts',(3.05632001699994,12.2,3.16719768799998));
#338796=CARTESIAN_POINT('Ctrl Pts',(3.05632001699994,5.2,3.16719768799998));
#338797=CARTESIAN_POINT('Ctrl Pts',(3.05632001699994,2.2,3.16719768799998));
#338798=CARTESIAN_POINT('Ctrl Pts',(3.05441654599994,12.2,3.16645949999998));
#338799=CARTESIAN_POINT('Ctrl Pts',(3.05441654599994,5.2,3.16645949999998));
#338800=CARTESIAN_POINT('Ctrl Pts',(3.05441654599994,2.2,3.16645949999998));
#338801=CARTESIAN_POINT('Ctrl Pts',(3.05251764599995,12.2,3.16572066899998));
#338802=CARTESIAN_POINT('Ctrl Pts',(3.05251764599995,5.2,3.16572066899998));
#338803=CARTESIAN_POINT('Ctrl Pts',(3.05251764599995,2.2,3.16572066899998));
#338804=CARTESIAN_POINT('Ctrl Pts',(3.05062331899994,12.2,3.16498120599999));
#338805=CARTESIAN_POINT('Ctrl Pts',(3.05062331899994,5.2,3.16498120599999));
#338806=CARTESIAN_POINT('Ctrl Pts',(3.05062331899994,2.2,3.16498120599999));
#338807=CARTESIAN_POINT('Ctrl Pts',(3.04873356899994,12.2,3.16424111899998));
#338808=CARTESIAN_POINT('Ctrl Pts',(3.04873356899994,5.2,3.16424111899998));
#338809=CARTESIAN_POINT('Ctrl Pts',(3.04873356899994,2.2,3.16424111899998));
#338810=CARTESIAN_POINT('Ctrl Pts',(3.04684840199994,12.2,3.16350042099998));
#338811=CARTESIAN_POINT('Ctrl Pts',(3.04684840199994,5.2,3.16350042099998));
#338812=CARTESIAN_POINT('Ctrl Pts',(3.04684840199994,2.2,3.16350042099998));
#338813=CARTESIAN_POINT('Ctrl Pts',(3.04496781799994,12.2,3.16275911799998));
#338814=CARTESIAN_POINT('Ctrl Pts',(3.04496781799994,5.2,3.16275911799998));
#338815=CARTESIAN_POINT('Ctrl Pts',(3.04496781799994,2.2,3.16275911799998));
#338816=CARTESIAN_POINT('Ctrl Pts',(3.04309182299995,12.2,3.16201722499999));
#338817=CARTESIAN_POINT('Ctrl Pts',(3.04309182299995,5.2,3.16201722499999));
#338818=CARTESIAN_POINT('Ctrl Pts',(3.04309182299995,2.2,3.16201722499999));
#338819=CARTESIAN_POINT('Ctrl Pts',(3.04122042199995,12.2,3.16127474799998));
#338820=CARTESIAN_POINT('Ctrl Pts',(3.04122042199995,5.2,3.16127474799998));
#338821=CARTESIAN_POINT('Ctrl Pts',(3.04122042199995,2.2,3.16127474799998));
#338822=CARTESIAN_POINT('Ctrl Pts',(3.03935361599994,12.2,3.16053169999999));
#338823=CARTESIAN_POINT('Ctrl Pts',(3.03935361599994,5.2,3.16053169999999));
#338824=CARTESIAN_POINT('Ctrl Pts',(3.03935361599994,2.2,3.16053169999999));
#338825=CARTESIAN_POINT('Ctrl Pts',(3.03749140999995,12.2,3.15978808799999));
#338826=CARTESIAN_POINT('Ctrl Pts',(3.03749140999995,5.2,3.15978808799999));
#338827=CARTESIAN_POINT('Ctrl Pts',(3.03749140999995,2.2,3.15978808799999));
#338828=CARTESIAN_POINT('Ctrl Pts',(3.03563380799994,12.2,3.15904392599998));
#338829=CARTESIAN_POINT('Ctrl Pts',(3.03563380799994,5.2,3.15904392599998));
#338830=CARTESIAN_POINT('Ctrl Pts',(3.03563380799994,2.2,3.15904392599998));
#338831=CARTESIAN_POINT('Ctrl Pts',(3.03378081399994,12.2,3.15829922099999));
#338832=CARTESIAN_POINT('Ctrl Pts',(3.03378081399994,5.2,3.15829922099999));
#338833=CARTESIAN_POINT('Ctrl Pts',(3.03378081399994,2.2,3.15829922099999));
#338834=CARTESIAN_POINT('Ctrl Pts',(3.03193242999994,12.2,3.15755398499999));
#338835=CARTESIAN_POINT('Ctrl Pts',(3.03193242999994,5.2,3.15755398499999));
#338836=CARTESIAN_POINT('Ctrl Pts',(3.03193242999994,2.2,3.15755398499999));
#338837=CARTESIAN_POINT('Ctrl Pts',(3.03008866199994,12.2,3.15680822899999));
#338838=CARTESIAN_POINT('Ctrl Pts',(3.03008866199994,5.2,3.15680822899999));
#338839=CARTESIAN_POINT('Ctrl Pts',(3.03008866199994,2.2,3.15680822899999));
#338840=CARTESIAN_POINT('Ctrl Pts',(3.02824951199994,12.2,3.15606196099999));
#338841=CARTESIAN_POINT('Ctrl Pts',(3.02824951199994,5.2,3.15606196099999));
#338842=CARTESIAN_POINT('Ctrl Pts',(3.02824951199994,2.2,3.15606196099999));
#338843=CARTESIAN_POINT('Ctrl Pts',(3.02641498399994,12.2,3.15531519299999));
#338844=CARTESIAN_POINT('Ctrl Pts',(3.02641498399994,5.2,3.15531519299999));
#338845=CARTESIAN_POINT('Ctrl Pts',(3.02641498399994,2.2,3.15531519299999));
#338846=CARTESIAN_POINT('Ctrl Pts',(3.02458508299994,12.2,3.15456793499998));
#338847=CARTESIAN_POINT('Ctrl Pts',(3.02458508299994,5.2,3.15456793499998));
#338848=CARTESIAN_POINT('Ctrl Pts',(3.02458508299994,2.2,3.15456793499998));
#338849=CARTESIAN_POINT('Ctrl Pts',(3.02275981199994,12.2,3.15382019599999));
#338850=CARTESIAN_POINT('Ctrl Pts',(3.02275981199994,5.2,3.15382019599999));
#338851=CARTESIAN_POINT('Ctrl Pts',(3.02275981199994,2.2,3.15382019599999));
#338852=CARTESIAN_POINT('Ctrl Pts',(3.02093917299994,12.2,3.15307198799999));
#338853=CARTESIAN_POINT('Ctrl Pts',(3.02093917299994,5.2,3.15307198799999));
#338854=CARTESIAN_POINT('Ctrl Pts',(3.02093917299994,2.2,3.15307198799999));
#338855=CARTESIAN_POINT('Ctrl Pts',(3.01912317099994,12.2,3.15232332099999));
#338856=CARTESIAN_POINT('Ctrl Pts',(3.01912317099994,5.2,3.15232332099999));
#338857=CARTESIAN_POINT('Ctrl Pts',(3.01912317099994,2.2,3.15232332099999));
#338858=CARTESIAN_POINT('Ctrl Pts',(3.01731180999994,12.2,3.15157420499999));
#338859=CARTESIAN_POINT('Ctrl Pts',(3.01731180999994,5.2,3.15157420499999));
#338860=CARTESIAN_POINT('Ctrl Pts',(3.01731180999994,2.2,3.15157420499999));
#338861=CARTESIAN_POINT('Ctrl Pts',(3.01550509399994,12.2,3.15082465099999));
#338862=CARTESIAN_POINT('Ctrl Pts',(3.01550509399994,5.2,3.15082465099999));
#338863=CARTESIAN_POINT('Ctrl Pts',(3.01550509399994,2.2,3.15082465099999));
#338864=CARTESIAN_POINT('Ctrl Pts',(3.01370302499994,12.2,3.15007466999998));
#338865=CARTESIAN_POINT('Ctrl Pts',(3.01370302499994,5.2,3.15007466999998));
#338866=CARTESIAN_POINT('Ctrl Pts',(3.01370302499994,2.2,3.15007466999998));
#338867=CARTESIAN_POINT('Ctrl Pts',(3.01190560799995,12.2,3.14932426999999));
#338868=CARTESIAN_POINT('Ctrl Pts',(3.01190560799995,5.2,3.14932426999999));
#338869=CARTESIAN_POINT('Ctrl Pts',(3.01190560799995,2.2,3.14932426999999));
#338870=CARTESIAN_POINT('Ctrl Pts',(3.01011284599995,12.2,3.14857346399998));
#338871=CARTESIAN_POINT('Ctrl Pts',(3.01011284599995,5.2,3.14857346399998));
#338872=CARTESIAN_POINT('Ctrl Pts',(3.01011284599995,2.2,3.14857346399998));
#338873=CARTESIAN_POINT('Ctrl Pts',(3.00832474399995,12.2,3.14782226199998));
#338874=CARTESIAN_POINT('Ctrl Pts',(3.00832474399995,5.2,3.14782226199998));
#338875=CARTESIAN_POINT('Ctrl Pts',(3.00832474399995,2.2,3.14782226199998));
#338876=CARTESIAN_POINT('Ctrl Pts',(3.00654130299994,12.2,3.14707067499998));
#338877=CARTESIAN_POINT('Ctrl Pts',(3.00654130299994,5.2,3.14707067499998));
#338878=CARTESIAN_POINT('Ctrl Pts',(3.00654130299994,2.2,3.14707067499998));
#338879=CARTESIAN_POINT('Ctrl Pts',(3.00476252899994,12.2,3.14631871099999));
#338880=CARTESIAN_POINT('Ctrl Pts',(3.00476252899994,5.2,3.14631871099999));
#338881=CARTESIAN_POINT('Ctrl Pts',(3.00476252899994,2.2,3.14631871099999));
#338882=CARTESIAN_POINT('Ctrl Pts',(3.00298842299994,12.2,3.14556638299998));
#338883=CARTESIAN_POINT('Ctrl Pts',(3.00298842299994,5.2,3.14556638299998));
#338884=CARTESIAN_POINT('Ctrl Pts',(3.00298842299994,2.2,3.14556638299998));
#338885=CARTESIAN_POINT('Ctrl Pts',(3.00121899199994,12.2,3.14481370199999));
#338886=CARTESIAN_POINT('Ctrl Pts',(3.00121899199994,5.2,3.14481370199999));
#338887=CARTESIAN_POINT('Ctrl Pts',(3.00121899199994,2.2,3.14481370199999));
#338888=CARTESIAN_POINT('Ctrl Pts',(2.99945423699994,12.2,3.14406067699998));
#338889=CARTESIAN_POINT('Ctrl Pts',(2.99945423699994,5.2,3.14406067699998));
#338890=CARTESIAN_POINT('Ctrl Pts',(2.99945423699994,2.2,3.14406067699998));
#338891=CARTESIAN_POINT('Ctrl Pts',(2.99769416199994,12.2,3.14330731899998));
#338892=CARTESIAN_POINT('Ctrl Pts',(2.99769416199994,5.2,3.14330731899998));
#338893=CARTESIAN_POINT('Ctrl Pts',(2.99769416199994,2.2,3.14330731899998));
#338894=CARTESIAN_POINT('Ctrl Pts',(2.99593877199994,12.2,3.14255363899999));
#338895=CARTESIAN_POINT('Ctrl Pts',(2.99593877199994,5.2,3.14255363899999));
#338896=CARTESIAN_POINT('Ctrl Pts',(2.99593877199994,2.2,3.14255363899999));
#338897=CARTESIAN_POINT('Ctrl Pts',(2.99418806799994,12.2,3.14179964699999));
#338898=CARTESIAN_POINT('Ctrl Pts',(2.99418806799994,5.2,3.14179964699999));
#338899=CARTESIAN_POINT('Ctrl Pts',(2.99418806799994,2.2,3.14179964699999));
#338900=CARTESIAN_POINT('Ctrl Pts',(2.99244205499994,12.2,3.14104535499999));
#338901=CARTESIAN_POINT('Ctrl Pts',(2.99244205499994,5.2,3.14104535499999));
#338902=CARTESIAN_POINT('Ctrl Pts',(2.99244205499994,2.2,3.14104535499999));
#338903=CARTESIAN_POINT('Ctrl Pts',(2.99070073699994,12.2,3.14029077499999));
#338904=CARTESIAN_POINT('Ctrl Pts',(2.99070073699994,5.2,3.14029077499999));
#338905=CARTESIAN_POINT('Ctrl Pts',(2.99070073699994,2.2,3.14029077499999));
#338906=CARTESIAN_POINT('Ctrl Pts',(2.98896411699995,12.2,3.13953591399999));
#338907=CARTESIAN_POINT('Ctrl Pts',(2.98896411699995,5.2,3.13953591399999));
#338908=CARTESIAN_POINT('Ctrl Pts',(2.98896411699995,2.2,3.13953591399999));
#338909=CARTESIAN_POINT('Ctrl Pts',(2.98723219799994,12.2,3.13878078399998));
#338910=CARTESIAN_POINT('Ctrl Pts',(2.98723219799994,5.2,3.13878078399998));
#338911=CARTESIAN_POINT('Ctrl Pts',(2.98723219799994,2.2,3.13878078399998));
#338912=CARTESIAN_POINT('Ctrl Pts',(2.98550498499994,12.2,3.13802539799998));
#338913=CARTESIAN_POINT('Ctrl Pts',(2.98550498499994,5.2,3.13802539799998));
#338914=CARTESIAN_POINT('Ctrl Pts',(2.98550498499994,2.2,3.13802539799998));
#338915=CARTESIAN_POINT('Ctrl Pts',(2.98378247999994,12.2,3.13726976499999));
#338916=CARTESIAN_POINT('Ctrl Pts',(2.98378247999994,5.2,3.13726976499999));
#338917=CARTESIAN_POINT('Ctrl Pts',(2.98378247999994,2.2,3.13726976499999));
#338918=CARTESIAN_POINT('Ctrl Pts',(2.98206468699994,12.2,3.13651389599999));
#338919=CARTESIAN_POINT('Ctrl Pts',(2.98206468699994,5.2,3.13651389599999));
#338920=CARTESIAN_POINT('Ctrl Pts',(2.98206468699994,2.2,3.13651389599999));
#338921=CARTESIAN_POINT('Ctrl Pts',(2.98035160799994,12.2,3.13575780299999));
#338922=CARTESIAN_POINT('Ctrl Pts',(2.98035160799994,5.2,3.13575780299999));
#338923=CARTESIAN_POINT('Ctrl Pts',(2.98035160799994,2.2,3.13575780299999));
#338924=CARTESIAN_POINT('Ctrl Pts',(2.97864324999995,12.2,3.13500149499998));
#338925=CARTESIAN_POINT('Ctrl Pts',(2.97864324999995,5.2,3.13500149499998));
#338926=CARTESIAN_POINT('Ctrl Pts',(2.97864324999995,2.2,3.13500149499998));
#338927=CARTESIAN_POINT('Ctrl Pts',(2.97693961299994,12.2,3.13424498399999));
#338928=CARTESIAN_POINT('Ctrl Pts',(2.97693961299994,5.2,3.13424498399999));
#338929=CARTESIAN_POINT('Ctrl Pts',(2.97693961299994,2.2,3.13424498399999));
#338930=CARTESIAN_POINT('Ctrl Pts',(2.97524070299994,12.2,3.13348828099999));
#338931=CARTESIAN_POINT('Ctrl Pts',(2.97524070299994,5.2,3.13348828099999));
#338932=CARTESIAN_POINT('Ctrl Pts',(2.97524070299994,2.2,3.13348828099999));
#338933=CARTESIAN_POINT('Ctrl Pts',(2.97354652199994,12.2,3.13273139699999));
#338934=CARTESIAN_POINT('Ctrl Pts',(2.97354652199994,5.2,3.13273139699999));
#338935=CARTESIAN_POINT('Ctrl Pts',(2.97354652199994,2.2,3.13273139699999));
#338936=CARTESIAN_POINT('Ctrl Pts',(2.97185707199994,12.2,3.13197434399999));
#338937=CARTESIAN_POINT('Ctrl Pts',(2.97185707199994,5.2,3.13197434399999));
#338938=CARTESIAN_POINT('Ctrl Pts',(2.97185707199994,2.2,3.13197434399999));
#338939=CARTESIAN_POINT('Ctrl Pts',(2.97017235999995,12.2,3.13121713099999));
#338940=CARTESIAN_POINT('Ctrl Pts',(2.97017235999995,5.2,3.13121713099999));
#338941=CARTESIAN_POINT('Ctrl Pts',(2.97017235999995,2.2,3.13121713099999));
#338942=CARTESIAN_POINT('Ctrl Pts',(2.96849238699994,12.2,3.13045976999998));
#338943=CARTESIAN_POINT('Ctrl Pts',(2.96849238699994,5.2,3.13045976999998));
#338944=CARTESIAN_POINT('Ctrl Pts',(2.96849238699994,2.2,3.13045976999998));
#338945=CARTESIAN_POINT('Ctrl Pts',(2.96681715699994,12.2,3.12970227099999));
#338946=CARTESIAN_POINT('Ctrl Pts',(2.96681715699994,5.2,3.12970227099999));
#338947=CARTESIAN_POINT('Ctrl Pts',(2.96681715699994,2.2,3.12970227099999));
#338948=CARTESIAN_POINT('Ctrl Pts',(2.96514667299994,12.2,3.12894464799999));
#338949=CARTESIAN_POINT('Ctrl Pts',(2.96514667299994,5.2,3.12894464799999));
#338950=CARTESIAN_POINT('Ctrl Pts',(2.96514667299994,2.2,3.12894464799999));
#338951=CARTESIAN_POINT('Ctrl Pts',(2.96348093899995,12.2,3.12818690899999));
#338952=CARTESIAN_POINT('Ctrl Pts',(2.96348093899995,5.2,3.12818690899999));
#338953=CARTESIAN_POINT('Ctrl Pts',(2.96348093899995,2.2,3.12818690899999));
#338954=CARTESIAN_POINT('Ctrl Pts',(2.96181995799994,12.2,3.12742906699999));
#338955=CARTESIAN_POINT('Ctrl Pts',(2.96181995799994,5.2,3.12742906699999));
#338956=CARTESIAN_POINT('Ctrl Pts',(2.96181995799994,2.2,3.12742906699999));
#338957=CARTESIAN_POINT('Ctrl Pts',(2.96016373299994,12.2,3.12667113199999));
#338958=CARTESIAN_POINT('Ctrl Pts',(2.96016373299994,5.2,3.12667113199999));
#338959=CARTESIAN_POINT('Ctrl Pts',(2.96016373299994,2.2,3.12667113199999));
#338960=CARTESIAN_POINT('Ctrl Pts',(2.95851226799994,12.2,3.12591311699999));
#338961=CARTESIAN_POINT('Ctrl Pts',(2.95851226799994,5.2,3.12591311699999));
#338962=CARTESIAN_POINT('Ctrl Pts',(2.95851226799994,2.2,3.12591311699999));
#338963=CARTESIAN_POINT('Ctrl Pts',(2.95686556599994,12.2,3.12515503099998));
#338964=CARTESIAN_POINT('Ctrl Pts',(2.95686556599994,5.2,3.12515503099998));
#338965=CARTESIAN_POINT('Ctrl Pts',(2.95686556599994,2.2,3.12515503099998));
#338966=CARTESIAN_POINT('Ctrl Pts',(2.95522362999994,12.2,3.12439688599999));
#338967=CARTESIAN_POINT('Ctrl Pts',(2.95522362999994,5.2,3.12439688599999));
#338968=CARTESIAN_POINT('Ctrl Pts',(2.95522362999994,2.2,3.12439688599999));
#338969=CARTESIAN_POINT('Ctrl Pts',(2.95358646499994,12.2,3.12363869399999));
#338970=CARTESIAN_POINT('Ctrl Pts',(2.95358646499994,5.2,3.12363869399999));
#338971=CARTESIAN_POINT('Ctrl Pts',(2.95358646499994,2.2,3.12363869399999));
#338972=CARTESIAN_POINT('Ctrl Pts',(2.95195407199994,12.2,3.12288046599999));
#338973=CARTESIAN_POINT('Ctrl Pts',(2.95195407199994,5.2,3.12288046599999));
#338974=CARTESIAN_POINT('Ctrl Pts',(2.95195407199994,2.2,3.12288046599999));
#338975=CARTESIAN_POINT('Ctrl Pts',(2.95032645599994,12.2,3.12212221199999));
#338976=CARTESIAN_POINT('Ctrl Pts',(2.95032645599994,5.2,3.12212221199999));
#338977=CARTESIAN_POINT('Ctrl Pts',(2.95032645599994,2.2,3.12212221199999));
#338978=CARTESIAN_POINT('Ctrl Pts',(2.94870361999994,12.2,3.12136394499999));
#338979=CARTESIAN_POINT('Ctrl Pts',(2.94870361999994,5.2,3.12136394499999));
#338980=CARTESIAN_POINT('Ctrl Pts',(2.94870361999994,2.2,3.12136394499999));
#338981=CARTESIAN_POINT('Ctrl Pts',(2.94708556599995,12.2,3.12060567599998));
#338982=CARTESIAN_POINT('Ctrl Pts',(2.94708556599995,5.2,3.12060567599998));
#338983=CARTESIAN_POINT('Ctrl Pts',(2.94708556599995,2.2,3.12060567599998));
#338984=CARTESIAN_POINT('Ctrl Pts',(2.94547229899994,12.2,3.11984741699998));
#338985=CARTESIAN_POINT('Ctrl Pts',(2.94547229899994,5.2,3.11984741699998));
#338986=CARTESIAN_POINT('Ctrl Pts',(2.94547229899994,2.2,3.11984741699998));
#338987=CARTESIAN_POINT('Ctrl Pts',(2.94386382099994,12.2,3.11908917699999));
#338988=CARTESIAN_POINT('Ctrl Pts',(2.94386382099994,5.2,3.11908917699999));
#338989=CARTESIAN_POINT('Ctrl Pts',(2.94386382099994,2.2,3.11908917699999));
#338990=CARTESIAN_POINT('Ctrl Pts',(2.94226013599994,12.2,3.11833096999998));
#338991=CARTESIAN_POINT('Ctrl Pts',(2.94226013599994,5.2,3.11833096999998));
#338992=CARTESIAN_POINT('Ctrl Pts',(2.94226013599994,2.2,3.11833096999998));
#338993=CARTESIAN_POINT('Ctrl Pts',(2.94066124799994,12.2,3.11757280599998));
#338994=CARTESIAN_POINT('Ctrl Pts',(2.94066124799994,5.2,3.11757280599998));
#338995=CARTESIAN_POINT('Ctrl Pts',(2.94066124799994,2.2,3.11757280599998));
#338996=CARTESIAN_POINT('Ctrl Pts',(2.93906715799995,12.2,3.11681469799999));
#338997=CARTESIAN_POINT('Ctrl Pts',(2.93906715799995,5.2,3.11681469799999));
#338998=CARTESIAN_POINT('Ctrl Pts',(2.93906715799995,2.2,3.11681469799999));
#338999=CARTESIAN_POINT('Ctrl Pts',(2.93747787099994,12.2,3.11605665499999));
#339000=CARTESIAN_POINT('Ctrl Pts',(2.93747787099994,5.2,3.11605665499999));
#339001=CARTESIAN_POINT('Ctrl Pts',(2.93747787099994,2.2,3.11605665499999));
#339002=CARTESIAN_POINT('Ctrl Pts',(2.93589338999994,12.2,3.11529869099999));
#339003=CARTESIAN_POINT('Ctrl Pts',(2.93589338999994,5.2,3.11529869099999));
#339004=CARTESIAN_POINT('Ctrl Pts',(2.93589338999994,2.2,3.11529869099999));
#339005=CARTESIAN_POINT('Ctrl Pts',(2.93431371699994,12.2,3.11454081699999));
#339006=CARTESIAN_POINT('Ctrl Pts',(2.93431371699994,5.2,3.11454081699999));
#339007=CARTESIAN_POINT('Ctrl Pts',(2.93431371699994,2.2,3.11454081699999));
#339008=CARTESIAN_POINT('Ctrl Pts',(2.93273885699994,12.2,3.11378304199999));
#339009=CARTESIAN_POINT('Ctrl Pts',(2.93273885699994,5.2,3.11378304199999));
#339010=CARTESIAN_POINT('Ctrl Pts',(2.93273885699994,2.2,3.11378304199999));
#339011=CARTESIAN_POINT('Ctrl Pts',(2.93116881199994,12.2,3.11302538199998));
#339012=CARTESIAN_POINT('Ctrl Pts',(2.93116881199994,5.2,3.11302538199998));
#339013=CARTESIAN_POINT('Ctrl Pts',(2.93116881199994,2.2,3.11302538199998));
#339014=CARTESIAN_POINT('Ctrl Pts',(2.92960358599994,12.2,3.11226784599998));
#339015=CARTESIAN_POINT('Ctrl Pts',(2.92960358599994,5.2,3.11226784599998));
#339016=CARTESIAN_POINT('Ctrl Pts',(2.92960358599994,2.2,3.11226784599998));
#339017=CARTESIAN_POINT('Ctrl Pts',(2.92804318099994,12.2,3.11151044499999));
#339018=CARTESIAN_POINT('Ctrl Pts',(2.92804318099994,5.2,3.11151044499999));
#339019=CARTESIAN_POINT('Ctrl Pts',(2.92804318099994,2.2,3.11151044499999));
#339020=CARTESIAN_POINT('Ctrl Pts',(2.92648760099994,12.2,3.11075319299999));
#339021=CARTESIAN_POINT('Ctrl Pts',(2.92648760099994,5.2,3.11075319299999));
#339022=CARTESIAN_POINT('Ctrl Pts',(2.92648760099994,2.2,3.11075319299999));
#339023=CARTESIAN_POINT('Ctrl Pts',(2.92493684899994,12.2,3.10999609999998));
#339024=CARTESIAN_POINT('Ctrl Pts',(2.92493684899994,5.2,3.10999609999998));
#339025=CARTESIAN_POINT('Ctrl Pts',(2.92493684899994,2.2,3.10999609999998));
#339026=CARTESIAN_POINT('Ctrl Pts',(2.92339092799994,12.2,3.10923917799999));
#339027=CARTESIAN_POINT('Ctrl Pts',(2.92339092799994,5.2,3.10923917799999));
#339028=CARTESIAN_POINT('Ctrl Pts',(2.92339092799994,2.2,3.10923917799999));
#339029=CARTESIAN_POINT('Ctrl Pts',(2.92184984099995,12.2,3.10848243799998));
#339030=CARTESIAN_POINT('Ctrl Pts',(2.92184984099995,5.2,3.10848243799998));
#339031=CARTESIAN_POINT('Ctrl Pts',(2.92184984099995,2.2,3.10848243799998));
#339032=CARTESIAN_POINT('Ctrl Pts',(2.92031359299994,12.2,3.10772589399999));
#339033=CARTESIAN_POINT('Ctrl Pts',(2.92031359299994,5.2,3.10772589399999));
#339034=CARTESIAN_POINT('Ctrl Pts',(2.92031359299994,2.2,3.10772589399999));
#339035=CARTESIAN_POINT('Ctrl Pts',(2.91878218399995,12.2,3.10696955699999));
#339036=CARTESIAN_POINT('Ctrl Pts',(2.91878218399995,5.2,3.10696955699999));
#339037=CARTESIAN_POINT('Ctrl Pts',(2.91878218399995,2.2,3.10696955699999));
#339038=CARTESIAN_POINT('Ctrl Pts',(2.91725561899994,12.2,3.10621343799999));
#339039=CARTESIAN_POINT('Ctrl Pts',(2.91725561899994,5.2,3.10621343799999));
#339040=CARTESIAN_POINT('Ctrl Pts',(2.91725561899994,2.2,3.10621343799999));
#339041=CARTESIAN_POINT('Ctrl Pts',(2.91573389999995,12.2,3.10545754899999));
#339042=CARTESIAN_POINT('Ctrl Pts',(2.91573389999995,5.2,3.10545754899999));
#339043=CARTESIAN_POINT('Ctrl Pts',(2.91573389999995,2.2,3.10545754899999));
#339044=CARTESIAN_POINT('Ctrl Pts',(2.91421703099994,12.2,3.10470190199998));
#339045=CARTESIAN_POINT('Ctrl Pts',(2.91421703099994,5.2,3.10470190199998));
#339046=CARTESIAN_POINT('Ctrl Pts',(2.91421703099994,2.2,3.10470190199998));
#339047=CARTESIAN_POINT('Ctrl Pts',(2.91270501499994,12.2,3.10394650799999));
#339048=CARTESIAN_POINT('Ctrl Pts',(2.91270501499994,5.2,3.10394650799999));
#339049=CARTESIAN_POINT('Ctrl Pts',(2.91270501499994,2.2,3.10394650799999));
#339050=CARTESIAN_POINT('Ctrl Pts',(2.91119785499995,12.2,3.10319138199999));
#339051=CARTESIAN_POINT('Ctrl Pts',(2.91119785499995,5.2,3.10319138199999));
#339052=CARTESIAN_POINT('Ctrl Pts',(2.91119785499995,2.2,3.10319138199999));
#339053=CARTESIAN_POINT('Ctrl Pts',(2.90969555299994,12.2,3.10243653299998));
#339054=CARTESIAN_POINT('Ctrl Pts',(2.90969555299994,5.2,3.10243653299998));
#339055=CARTESIAN_POINT('Ctrl Pts',(2.90969555299994,2.2,3.10243653299998));
#339056=CARTESIAN_POINT('Ctrl Pts',(2.90819811399994,12.2,3.10168197399998));
#339057=CARTESIAN_POINT('Ctrl Pts',(2.90819811399994,5.2,3.10168197399998));
#339058=CARTESIAN_POINT('Ctrl Pts',(2.90819811399994,2.2,3.10168197399998));
#339059=CARTESIAN_POINT('Ctrl Pts',(2.90670553999994,12.2,3.10092771799999));
#339060=CARTESIAN_POINT('Ctrl Pts',(2.90670553999994,5.2,3.10092771799999));
#339061=CARTESIAN_POINT('Ctrl Pts',(2.90670553999994,2.2,3.10092771799999));
#339062=CARTESIAN_POINT('Ctrl Pts',(2.90521783399994,12.2,3.10017377499998));
#339063=CARTESIAN_POINT('Ctrl Pts',(2.90521783399994,5.2,3.10017377499998));
#339064=CARTESIAN_POINT('Ctrl Pts',(2.90521783399994,2.2,3.10017377499998));
#339065=CARTESIAN_POINT('Ctrl Pts',(2.90373499899995,12.2,3.09942015899999));
#339066=CARTESIAN_POINT('Ctrl Pts',(2.90373499899995,5.2,3.09942015899999));
#339067=CARTESIAN_POINT('Ctrl Pts',(2.90373499899995,2.2,3.09942015899999));
#339068=CARTESIAN_POINT('Ctrl Pts',(2.90225703699994,12.2,3.09866687999998));
#339069=CARTESIAN_POINT('Ctrl Pts',(2.90225703699994,5.2,3.09866687999998));
#339070=CARTESIAN_POINT('Ctrl Pts',(2.90225703699994,2.2,3.09866687999998));
#339071=CARTESIAN_POINT('Ctrl Pts',(2.90078395299994,12.2,3.09791395199999));
#339072=CARTESIAN_POINT('Ctrl Pts',(2.90078395299994,5.2,3.09791395199999));
#339073=CARTESIAN_POINT('Ctrl Pts',(2.90078395299994,2.2,3.09791395199999));
#339074=CARTESIAN_POINT('Ctrl Pts',(2.89931574799994,12.2,3.09716138599998));
#339075=CARTESIAN_POINT('Ctrl Pts',(2.89931574799994,5.2,3.09716138599998));
#339076=CARTESIAN_POINT('Ctrl Pts',(2.89931574799994,2.2,3.09716138599998));
#339077=CARTESIAN_POINT('Ctrl Pts',(2.89785242599994,12.2,3.09640919499999));
#339078=CARTESIAN_POINT('Ctrl Pts',(2.89785242599994,5.2,3.09640919499999));
#339079=CARTESIAN_POINT('Ctrl Pts',(2.89785242599994,2.2,3.09640919499999));
#339080=CARTESIAN_POINT('Ctrl Pts',(2.89639399099994,12.2,3.09565739199999));
#339081=CARTESIAN_POINT('Ctrl Pts',(2.89639399099994,5.2,3.09565739199999));
#339082=CARTESIAN_POINT('Ctrl Pts',(2.89639399099994,2.2,3.09565739199999));
#339083=CARTESIAN_POINT('Ctrl Pts',(2.89494044399994,12.2,3.09490598699998));
#339084=CARTESIAN_POINT('Ctrl Pts',(2.89494044399994,5.2,3.09490598699998));
#339085=CARTESIAN_POINT('Ctrl Pts',(2.89494044399994,2.2,3.09490598699998));
#339086=CARTESIAN_POINT('Ctrl Pts',(2.89349178899994,12.2,3.09415499399999));
#339087=CARTESIAN_POINT('Ctrl Pts',(2.89349178899994,5.2,3.09415499399999));
#339088=CARTESIAN_POINT('Ctrl Pts',(2.89349178899994,2.2,3.09415499399999));
#339089=CARTESIAN_POINT('Ctrl Pts',(2.89204802899994,12.2,3.09340442399999));
#339090=CARTESIAN_POINT('Ctrl Pts',(2.89204802899994,5.2,3.09340442399999));
#339091=CARTESIAN_POINT('Ctrl Pts',(2.89204802899994,2.2,3.09340442399999));
#339092=CARTESIAN_POINT('Ctrl Pts',(2.89060916499994,12.2,3.09265429099998));
#339093=CARTESIAN_POINT('Ctrl Pts',(2.89060916499994,5.2,3.09265429099998));
#339094=CARTESIAN_POINT('Ctrl Pts',(2.89060916499994,2.2,3.09265429099998));
#339095=CARTESIAN_POINT('Ctrl Pts',(2.88917520199994,12.2,3.09190460599999));
#339096=CARTESIAN_POINT('Ctrl Pts',(2.88917520199994,5.2,3.09190460599999));
#339097=CARTESIAN_POINT('Ctrl Pts',(2.88917520199994,2.2,3.09190460599999));
#339098=CARTESIAN_POINT('Ctrl Pts',(2.88774614299995,12.2,3.09115538099999));
#339099=CARTESIAN_POINT('Ctrl Pts',(2.88774614299995,5.2,3.09115538099999));
#339100=CARTESIAN_POINT('Ctrl Pts',(2.88774614299995,2.2,3.09115538099999));
#339101=CARTESIAN_POINT('Ctrl Pts',(2.88632198899994,12.2,3.09040662899999));
#339102=CARTESIAN_POINT('Ctrl Pts',(2.88632198899994,5.2,3.09040662899999));
#339103=CARTESIAN_POINT('Ctrl Pts',(2.88632198899994,2.2,3.09040662899999));
#339104=CARTESIAN_POINT('Ctrl Pts',(2.88490274499994,12.2,3.08965836399998));
#339105=CARTESIAN_POINT('Ctrl Pts',(2.88490274499994,5.2,3.08965836399998));
#339106=CARTESIAN_POINT('Ctrl Pts',(2.88490274499994,2.2,3.08965836399998));
#339107=CARTESIAN_POINT('Ctrl Pts',(2.88348841299995,12.2,3.08891059699998));
#339108=CARTESIAN_POINT('Ctrl Pts',(2.88348841299995,5.2,3.08891059699998));
#339109=CARTESIAN_POINT('Ctrl Pts',(2.88348841299995,2.2,3.08891059699998));
#339110=CARTESIAN_POINT('Ctrl Pts',(2.88207899499994,12.2,3.08816333899999));
#339111=CARTESIAN_POINT('Ctrl Pts',(2.88207899499994,5.2,3.08816333899999));
#339112=CARTESIAN_POINT('Ctrl Pts',(2.88207899499994,2.2,3.08816333899999));
#339113=CARTESIAN_POINT('Ctrl Pts',(2.88067449499994,12.2,3.08741660499999));
#339114=CARTESIAN_POINT('Ctrl Pts',(2.88067449499994,5.2,3.08741660499999));
#339115=CARTESIAN_POINT('Ctrl Pts',(2.88067449499994,2.2,3.08741660499999));
#339116=CARTESIAN_POINT('Ctrl Pts',(2.87927491499994,12.2,3.08667040599998));
#339117=CARTESIAN_POINT('Ctrl Pts',(2.87927491499994,5.2,3.08667040599998));
#339118=CARTESIAN_POINT('Ctrl Pts',(2.87927491499994,2.2,3.08667040599998));
#339119=CARTESIAN_POINT('Ctrl Pts',(2.87788025899995,12.2,3.08592475599998));
#339120=CARTESIAN_POINT('Ctrl Pts',(2.87788025899995,5.2,3.08592475599998));
#339121=CARTESIAN_POINT('Ctrl Pts',(2.87788025899995,2.2,3.08592475599998));
#339122=CARTESIAN_POINT('Ctrl Pts',(2.87649052899994,12.2,3.08517966499998));
#339123=CARTESIAN_POINT('Ctrl Pts',(2.87649052899994,5.2,3.08517966499998));
#339124=CARTESIAN_POINT('Ctrl Pts',(2.87649052899994,2.2,3.08517966499998));
#339125=CARTESIAN_POINT('Ctrl Pts',(2.87510572599994,12.2,3.08443514899999));
#339126=CARTESIAN_POINT('Ctrl Pts',(2.87510572599994,5.2,3.08443514899999));
#339127=CARTESIAN_POINT('Ctrl Pts',(2.87510572599994,2.2,3.08443514899999));
#339128=CARTESIAN_POINT('Ctrl Pts',(2.87372585599994,12.2,3.08369121799998));
#339129=CARTESIAN_POINT('Ctrl Pts',(2.87372585599994,5.2,3.08369121799998));
#339130=CARTESIAN_POINT('Ctrl Pts',(2.87372585599994,2.2,3.08369121799998));
#339131=CARTESIAN_POINT('Ctrl Pts',(2.87235091999994,12.2,3.08294788699998));
#339132=CARTESIAN_POINT('Ctrl Pts',(2.87235091999994,5.2,3.08294788699998));
#339133=CARTESIAN_POINT('Ctrl Pts',(2.87235091999994,2.2,3.08294788699998));
#339134=CARTESIAN_POINT('Ctrl Pts',(2.87098092099995,12.2,3.08220516599999));
#339135=CARTESIAN_POINT('Ctrl Pts',(2.87098092099995,5.2,3.08220516599999));
#339136=CARTESIAN_POINT('Ctrl Pts',(2.87098092099995,2.2,3.08220516599999));
#339137=CARTESIAN_POINT('Ctrl Pts',(2.86961586199994,12.2,3.08146307099998));
#339138=CARTESIAN_POINT('Ctrl Pts',(2.86961586199994,5.2,3.08146307099998));
#339139=CARTESIAN_POINT('Ctrl Pts',(2.86961586199994,2.2,3.08146307099998));
#339140=CARTESIAN_POINT('Ctrl Pts',(2.86825574499994,12.2,3.08072161099999));
#339141=CARTESIAN_POINT('Ctrl Pts',(2.86825574499994,5.2,3.08072161099999));
#339142=CARTESIAN_POINT('Ctrl Pts',(2.86825574499994,2.2,3.08072161099999));
#339143=CARTESIAN_POINT('Ctrl Pts',(2.86690057399994,12.2,3.07998080199999));
#339144=CARTESIAN_POINT('Ctrl Pts',(2.86690057399994,5.2,3.07998080199999));
#339145=CARTESIAN_POINT('Ctrl Pts',(2.86690057399994,2.2,3.07998080199999));
#339146=CARTESIAN_POINT('Ctrl Pts',(2.86555034999994,12.2,3.07924065399998));
#339147=CARTESIAN_POINT('Ctrl Pts',(2.86555034999994,5.2,3.07924065399998));
#339148=CARTESIAN_POINT('Ctrl Pts',(2.86555034999994,2.2,3.07924065399998));
#339149=CARTESIAN_POINT('Ctrl Pts',(2.86420507699995,12.2,3.07850118299999));
#339150=CARTESIAN_POINT('Ctrl Pts',(2.86420507699995,5.2,3.07850118299999));
#339151=CARTESIAN_POINT('Ctrl Pts',(2.86420507699995,2.2,3.07850118299999));
#339152=CARTESIAN_POINT('Ctrl Pts',(2.86286475699994,12.2,3.07776239899999));
#339153=CARTESIAN_POINT('Ctrl Pts',(2.86286475699994,5.2,3.07776239899999));
#339154=CARTESIAN_POINT('Ctrl Pts',(2.86286475699994,2.2,3.07776239899999));
#339155=CARTESIAN_POINT('Ctrl Pts',(2.86152939299994,12.2,3.07702431599999));
#339156=CARTESIAN_POINT('Ctrl Pts',(2.86152939299994,5.2,3.07702431599999));
#339157=CARTESIAN_POINT('Ctrl Pts',(2.86152939299994,2.2,3.07702431599999));
#339158=CARTESIAN_POINT('Ctrl Pts',(2.86019898699994,12.2,3.07628694799998));
#339159=CARTESIAN_POINT('Ctrl Pts',(2.86019898699994,5.2,3.07628694799998));
#339160=CARTESIAN_POINT('Ctrl Pts',(2.86019898699994,2.2,3.07628694799998));
#339161=CARTESIAN_POINT('Ctrl Pts',(2.85887354299994,12.2,3.07555030699999));
#339162=CARTESIAN_POINT('Ctrl Pts',(2.85887354299994,5.2,3.07555030699999));
#339163=CARTESIAN_POINT('Ctrl Pts',(2.85887354299994,2.2,3.07555030699999));
#339164=CARTESIAN_POINT('Ctrl Pts',(2.85755306199994,12.2,3.07481440599998));
#339165=CARTESIAN_POINT('Ctrl Pts',(2.85755306199994,5.2,3.07481440599998));
#339166=CARTESIAN_POINT('Ctrl Pts',(2.85755306199994,2.2,3.07481440599998));
#339167=CARTESIAN_POINT('Ctrl Pts',(2.85623754899994,12.2,3.07407925799998));
#339168=CARTESIAN_POINT('Ctrl Pts',(2.85623754899994,5.2,3.07407925799998));
#339169=CARTESIAN_POINT('Ctrl Pts',(2.85623754899994,2.2,3.07407925799998));
#339170=CARTESIAN_POINT('Ctrl Pts',(2.85492700399995,12.2,3.07334487499999));
#339171=CARTESIAN_POINT('Ctrl Pts',(2.85492700399995,5.2,3.07334487499999));
#339172=CARTESIAN_POINT('Ctrl Pts',(2.85492700399995,2.2,3.07334487499999));
#339173=CARTESIAN_POINT('Ctrl Pts',(2.85362142999994,12.2,3.07261127299999));
#339174=CARTESIAN_POINT('Ctrl Pts',(2.85362142999994,5.2,3.07261127299999));
#339175=CARTESIAN_POINT('Ctrl Pts',(2.85362142999994,2.2,3.07261127299999));
#339176=CARTESIAN_POINT('Ctrl Pts',(2.85232083099995,12.2,3.07187846199999));
#339177=CARTESIAN_POINT('Ctrl Pts',(2.85232083099995,5.2,3.07187846199999));
#339178=CARTESIAN_POINT('Ctrl Pts',(2.85232083099995,2.2,3.07187846199999));
#339179=CARTESIAN_POINT('Ctrl Pts',(2.85102520899994,12.2,3.07114645799999));
#339180=CARTESIAN_POINT('Ctrl Pts',(2.85102520899994,5.2,3.07114645799999));
#339181=CARTESIAN_POINT('Ctrl Pts',(2.85102520899994,2.2,3.07114645799999));
#339182=CARTESIAN_POINT('Ctrl Pts',(2.84973456599994,12.2,3.07041527099998));
#339183=CARTESIAN_POINT('Ctrl Pts',(2.84973456599994,5.2,3.07041527099998));
#339184=CARTESIAN_POINT('Ctrl Pts',(2.84973456599994,2.2,3.07041527099998));
#339185=CARTESIAN_POINT('Ctrl Pts',(2.84844890399994,12.2,3.06968491699998));
#339186=CARTESIAN_POINT('Ctrl Pts',(2.84844890399994,5.2,3.06968491699998));
#339187=CARTESIAN_POINT('Ctrl Pts',(2.84844890399994,2.2,3.06968491699998));
#339188=CARTESIAN_POINT('Ctrl Pts',(2.84716822699994,12.2,3.06895540799999));
#339189=CARTESIAN_POINT('Ctrl Pts',(2.84716822699994,5.2,3.06895540799999));
#339190=CARTESIAN_POINT('Ctrl Pts',(2.84716822699994,2.2,3.06895540799999));
#339191=CARTESIAN_POINT('Ctrl Pts',(2.84589253799994,12.2,3.06822675799998));
#339192=CARTESIAN_POINT('Ctrl Pts',(2.84589253799994,5.2,3.06822675799998));
#339193=CARTESIAN_POINT('Ctrl Pts',(2.84589253799994,2.2,3.06822675799998));
#339194=CARTESIAN_POINT('Ctrl Pts',(2.84462183699994,12.2,3.06749897899999));
#339195=CARTESIAN_POINT('Ctrl Pts',(2.84462183699994,5.2,3.06749897899999));
#339196=CARTESIAN_POINT('Ctrl Pts',(2.84462183699994,2.2,3.06749897899999));
#339197=CARTESIAN_POINT('Ctrl Pts',(2.84335612799994,12.2,3.06677208499998));
#339198=CARTESIAN_POINT('Ctrl Pts',(2.84335612799994,5.2,3.06677208499998));
#339199=CARTESIAN_POINT('Ctrl Pts',(2.84335612799994,2.2,3.06677208499998));
#339200=CARTESIAN_POINT('Ctrl Pts',(2.84209541399994,12.2,3.06604608899999));
#339201=CARTESIAN_POINT('Ctrl Pts',(2.84209541399994,5.2,3.06604608899999));
#339202=CARTESIAN_POINT('Ctrl Pts',(2.84209541399994,2.2,3.06604608899999));
#339203=CARTESIAN_POINT('Ctrl Pts',(2.84083969699994,12.2,3.06532100499999));
#339204=CARTESIAN_POINT('Ctrl Pts',(2.84083969699994,5.2,3.06532100499999));
#339205=CARTESIAN_POINT('Ctrl Pts',(2.84083969699994,2.2,3.06532100499999));
#339206=CARTESIAN_POINT('Ctrl Pts',(2.83958897899995,12.2,3.06459684699998));
#339207=CARTESIAN_POINT('Ctrl Pts',(2.83958897899995,5.2,3.06459684699998));
#339208=CARTESIAN_POINT('Ctrl Pts',(2.83958897899995,2.2,3.06459684699998));
#339209=CARTESIAN_POINT('Ctrl Pts',(2.83834326299994,12.2,3.06387362699999));
#339210=CARTESIAN_POINT('Ctrl Pts',(2.83834326299994,5.2,3.06387362699999));
#339211=CARTESIAN_POINT('Ctrl Pts',(2.83834326299994,2.2,3.06387362699999));
#339212=CARTESIAN_POINT('Ctrl Pts',(2.83710254999994,12.2,3.06315135899998));
#339213=CARTESIAN_POINT('Ctrl Pts',(2.83710254999994,5.2,3.06315135899998));
#339214=CARTESIAN_POINT('Ctrl Pts',(2.83710254999994,2.2,3.06315135899998));
#339215=CARTESIAN_POINT('Ctrl Pts',(2.83586684499994,12.2,3.06243005699999));
#339216=CARTESIAN_POINT('Ctrl Pts',(2.83586684499994,5.2,3.06243005699999));
#339217=CARTESIAN_POINT('Ctrl Pts',(2.83586684499994,2.2,3.06243005699999));
#339218=CARTESIAN_POINT('Ctrl Pts',(2.83463614899994,12.2,3.06170973399999));
#339219=CARTESIAN_POINT('Ctrl Pts',(2.83463614899994,5.2,3.06170973399999));
#339220=CARTESIAN_POINT('Ctrl Pts',(2.83463614899994,2.2,3.06170973399999));
#339221=CARTESIAN_POINT('Ctrl Pts',(2.83341046299994,12.2,3.06099040399998));
#339222=CARTESIAN_POINT('Ctrl Pts',(2.83341046299994,5.2,3.06099040399998));
#339223=CARTESIAN_POINT('Ctrl Pts',(2.83341046299994,2.2,3.06099040399998));
#339224=CARTESIAN_POINT('Ctrl Pts',(2.83218979199995,12.2,3.06027208099999));
#339225=CARTESIAN_POINT('Ctrl Pts',(2.83218979199995,5.2,3.06027208099999));
#339226=CARTESIAN_POINT('Ctrl Pts',(2.83218979199995,2.2,3.06027208099999));
#339227=CARTESIAN_POINT('Ctrl Pts',(2.83097413699994,12.2,3.05955477799999));
#339228=CARTESIAN_POINT('Ctrl Pts',(2.83097413699994,5.2,3.05955477799999));
#339229=CARTESIAN_POINT('Ctrl Pts',(2.83097413699994,2.2,3.05955477799999));
#339230=CARTESIAN_POINT('Ctrl Pts',(2.82976349999994,12.2,3.05883850699999));
#339231=CARTESIAN_POINT('Ctrl Pts',(2.82976349999994,5.2,3.05883850699999));
#339232=CARTESIAN_POINT('Ctrl Pts',(2.82976349999994,2.2,3.05883850699999));
#339233=CARTESIAN_POINT('Ctrl Pts',(2.82855788499994,12.2,3.05812328499999));
#339234=CARTESIAN_POINT('Ctrl Pts',(2.82855788499994,5.2,3.05812328499999));
#339235=CARTESIAN_POINT('Ctrl Pts',(2.82855788499994,2.2,3.05812328499999));
#339236=CARTESIAN_POINT('Ctrl Pts',(2.82735729199994,12.2,3.05740912399998));
#339237=CARTESIAN_POINT('Ctrl Pts',(2.82735729199994,5.2,3.05740912399998));
#339238=CARTESIAN_POINT('Ctrl Pts',(2.82735729199994,2.2,3.05740912399998));
#339239=CARTESIAN_POINT('Ctrl Pts',(2.82616172399994,12.2,3.05669603699998));
#339240=CARTESIAN_POINT('Ctrl Pts',(2.82616172399994,5.2,3.05669603699998));
#339241=CARTESIAN_POINT('Ctrl Pts',(2.82616172399994,2.2,3.05669603699998));
#339242=CARTESIAN_POINT('Ctrl Pts',(2.82497118399994,12.2,3.05598403999999));
#339243=CARTESIAN_POINT('Ctrl Pts',(2.82497118399994,5.2,3.05598403999999));
#339244=CARTESIAN_POINT('Ctrl Pts',(2.82497118399994,2.2,3.05598403999999));
#339245=CARTESIAN_POINT('Ctrl Pts',(2.82378567499994,12.2,3.05527314499999));
#339246=CARTESIAN_POINT('Ctrl Pts',(2.82378567499994,5.2,3.05527314499999));
#339247=CARTESIAN_POINT('Ctrl Pts',(2.82378567499994,2.2,3.05527314499999));
#339248=CARTESIAN_POINT('Ctrl Pts',(2.82260519599994,12.2,3.05456336699999));
#339249=CARTESIAN_POINT('Ctrl Pts',(2.82260519599994,5.2,3.05456336699999));
#339250=CARTESIAN_POINT('Ctrl Pts',(2.82260519599994,2.2,3.05456336699999));
#339251=CARTESIAN_POINT('Ctrl Pts',(2.82142975399994,12.2,3.05385471799998));
#339252=CARTESIAN_POINT('Ctrl Pts',(2.82142975399994,5.2,3.05385471799998));
#339253=CARTESIAN_POINT('Ctrl Pts',(2.82142975399994,2.2,3.05385471799998));
#339254=CARTESIAN_POINT('Ctrl Pts',(2.82025934699994,12.2,3.05314721399998));
#339255=CARTESIAN_POINT('Ctrl Pts',(2.82025934699994,5.2,3.05314721399998));
#339256=CARTESIAN_POINT('Ctrl Pts',(2.82025934699994,2.2,3.05314721399998));
#339257=CARTESIAN_POINT('Ctrl Pts',(2.81909397999994,12.2,3.05244086899998));
#339258=CARTESIAN_POINT('Ctrl Pts',(2.81909397999994,5.2,3.05244086899998));
#339259=CARTESIAN_POINT('Ctrl Pts',(2.81909397999994,2.2,3.05244086899998));
#339260=CARTESIAN_POINT('Ctrl Pts',(2.81793365499994,12.2,3.05173569499999));
#339261=CARTESIAN_POINT('Ctrl Pts',(2.81793365499994,5.2,3.05173569499999));
#339262=CARTESIAN_POINT('Ctrl Pts',(2.81793365499994,2.2,3.05173569499999));
#339263=CARTESIAN_POINT('Ctrl Pts',(2.81677837199994,12.2,3.05103170699999));
#339264=CARTESIAN_POINT('Ctrl Pts',(2.81677837199994,5.2,3.05103170699999));
#339265=CARTESIAN_POINT('Ctrl Pts',(2.81677837199994,2.2,3.05103170699999));
#339266=CARTESIAN_POINT('Ctrl Pts',(2.81562813499994,12.2,3.05032892099998));
#339267=CARTESIAN_POINT('Ctrl Pts',(2.81562813499994,5.2,3.05032892099998));
#339268=CARTESIAN_POINT('Ctrl Pts',(2.81562813499994,2.2,3.05032892099998));
#339269=CARTESIAN_POINT('Ctrl Pts',(2.81448294599994,12.2,3.04962734799999));
#339270=CARTESIAN_POINT('Ctrl Pts',(2.81448294599994,5.2,3.04962734799999));
#339271=CARTESIAN_POINT('Ctrl Pts',(2.81448294599994,2.2,3.04962734799999));
#339272=CARTESIAN_POINT('Ctrl Pts',(2.81334280599994,12.2,3.04892700399999));
#339273=CARTESIAN_POINT('Ctrl Pts',(2.81334280599994,5.2,3.04892700399999));
#339274=CARTESIAN_POINT('Ctrl Pts',(2.81334280599994,2.2,3.04892700399999));
#339275=CARTESIAN_POINT('Ctrl Pts',(2.81220771899994,12.2,3.04822790299998));
#339276=CARTESIAN_POINT('Ctrl Pts',(2.81220771899994,5.2,3.04822790299998));
#339277=CARTESIAN_POINT('Ctrl Pts',(2.81220771899994,2.2,3.04822790299998));
#339278=CARTESIAN_POINT('Ctrl Pts',(2.81107768699994,12.2,3.04753005899999));
#339279=CARTESIAN_POINT('Ctrl Pts',(2.81107768699994,5.2,3.04753005899999));
#339280=CARTESIAN_POINT('Ctrl Pts',(2.81107768699994,2.2,3.04753005899999));
#339281=CARTESIAN_POINT('Ctrl Pts',(2.80995270899994,12.2,3.04683348499999));
#339282=CARTESIAN_POINT('Ctrl Pts',(2.80995270899994,5.2,3.04683348499999));
#339283=CARTESIAN_POINT('Ctrl Pts',(2.80995270899994,2.2,3.04683348499999));
#339284=CARTESIAN_POINT('Ctrl Pts',(2.80883279199994,12.2,3.04613819699998));
#339285=CARTESIAN_POINT('Ctrl Pts',(2.80883279199994,5.2,3.04613819699998));
#339286=CARTESIAN_POINT('Ctrl Pts',(2.80883279199994,2.2,3.04613819699998));
#339287=CARTESIAN_POINT('Ctrl Pts',(2.80771793299994,12.2,3.04544420899998));
#339288=CARTESIAN_POINT('Ctrl Pts',(2.80771793299994,5.2,3.04544420899998));
#339289=CARTESIAN_POINT('Ctrl Pts',(2.80771793299994,2.2,3.04544420899998));
#339290=CARTESIAN_POINT('Ctrl Pts',(2.80660813799994,12.2,3.04475153399999));
#339291=CARTESIAN_POINT('Ctrl Pts',(2.80660813799994,5.2,3.04475153399999));
#339292=CARTESIAN_POINT('Ctrl Pts',(2.80660813799994,2.2,3.04475153399999));
#339293=CARTESIAN_POINT('Ctrl Pts',(2.80550340799994,12.2,3.04406018899999));
#339294=CARTESIAN_POINT('Ctrl Pts',(2.80550340799994,5.2,3.04406018899999));
#339295=CARTESIAN_POINT('Ctrl Pts',(2.80550340799994,2.2,3.04406018899999));
#339296=CARTESIAN_POINT('Ctrl Pts',(2.80440374399994,12.2,3.04337018599998));
#339297=CARTESIAN_POINT('Ctrl Pts',(2.80440374399994,5.2,3.04337018599998));
#339298=CARTESIAN_POINT('Ctrl Pts',(2.80440374399994,2.2,3.04337018599998));
#339299=CARTESIAN_POINT('Ctrl Pts',(2.80330914799995,12.2,3.04268154099999));
#339300=CARTESIAN_POINT('Ctrl Pts',(2.80330914799995,5.2,3.04268154099999));
#339301=CARTESIAN_POINT('Ctrl Pts',(2.80330914799995,2.2,3.04268154099999));
#339302=CARTESIAN_POINT('Ctrl Pts',(2.80221962399994,12.2,3.04199426699999));
#339303=CARTESIAN_POINT('Ctrl Pts',(2.80221962399994,5.2,3.04199426699999));
#339304=CARTESIAN_POINT('Ctrl Pts',(2.80221962399994,2.2,3.04199426699999));
#339305=CARTESIAN_POINT('Ctrl Pts',(2.80113517299994,12.2,3.04130837799998));
#339306=CARTESIAN_POINT('Ctrl Pts',(2.80113517299994,5.2,3.04130837799998));
#339307=CARTESIAN_POINT('Ctrl Pts',(2.80113517299994,2.2,3.04130837799998));
#339308=CARTESIAN_POINT('Ctrl Pts',(2.80005579499994,12.2,3.04062389199999));
#339309=CARTESIAN_POINT('Ctrl Pts',(2.80005579499994,5.2,3.04062389199999));
#339310=CARTESIAN_POINT('Ctrl Pts',(2.80005579499994,2.2,3.04062389199999));
#339311=CARTESIAN_POINT('Ctrl Pts',(2.79898149599994,12.2,3.03994081999999));
#339312=CARTESIAN_POINT('Ctrl Pts',(2.79898149599994,5.2,3.03994081999999));
#339313=CARTESIAN_POINT('Ctrl Pts',(2.79898149599994,2.2,3.03994081999999));
#339314=CARTESIAN_POINT('Ctrl Pts',(2.79791227399994,12.2,3.03925917799998));
#339315=CARTESIAN_POINT('Ctrl Pts',(2.79791227399994,5.2,3.03925917799998));
#339316=CARTESIAN_POINT('Ctrl Pts',(2.79791227399994,2.2,3.03925917799998));
#339317=CARTESIAN_POINT('Ctrl Pts',(2.79684813299995,12.2,3.03857898099999));
#339318=CARTESIAN_POINT('Ctrl Pts',(2.79684813299995,5.2,3.03857898099999));
#339319=CARTESIAN_POINT('Ctrl Pts',(2.79684813299995,2.2,3.03857898099999));
#339320=CARTESIAN_POINT('Ctrl Pts',(2.79578907399994,12.2,3.03790024299998));
#339321=CARTESIAN_POINT('Ctrl Pts',(2.79578907399994,5.2,3.03790024299998));
#339322=CARTESIAN_POINT('Ctrl Pts',(2.79578907399994,2.2,3.03790024299998));
#339323=CARTESIAN_POINT('Ctrl Pts',(2.79473510099994,12.2,3.03722297899998));
#339324=CARTESIAN_POINT('Ctrl Pts',(2.79473510099994,5.2,3.03722297899998));
#339325=CARTESIAN_POINT('Ctrl Pts',(2.79473510099994,2.2,3.03722297899998));
#339326=CARTESIAN_POINT('Ctrl Pts',(2.79368621299994,12.2,3.03654720399999));
#339327=CARTESIAN_POINT('Ctrl Pts',(2.79368621299994,5.2,3.03654720399999));
#339328=CARTESIAN_POINT('Ctrl Pts',(2.79368621299994,2.2,3.03654720399999));
#339329=CARTESIAN_POINT('Ctrl Pts',(2.79264241399994,12.2,3.03587293199998));
#339330=CARTESIAN_POINT('Ctrl Pts',(2.79264241399994,5.2,3.03587293199998));
#339331=CARTESIAN_POINT('Ctrl Pts',(2.79264241399994,2.2,3.03587293199998));
#339332=CARTESIAN_POINT('Ctrl Pts',(2.79160370399994,12.2,3.03520017899999));
#339333=CARTESIAN_POINT('Ctrl Pts',(2.79160370399994,5.2,3.03520017899999));
#339334=CARTESIAN_POINT('Ctrl Pts',(2.79160370399994,2.2,3.03520017899999));
#339335=CARTESIAN_POINT('Ctrl Pts',(2.79057008599994,12.2,3.03452895899999));
#339336=CARTESIAN_POINT('Ctrl Pts',(2.79057008599994,5.2,3.03452895899999));
#339337=CARTESIAN_POINT('Ctrl Pts',(2.79057008599994,2.2,3.03452895899999));
#339338=CARTESIAN_POINT('Ctrl Pts',(2.78954156299994,12.2,3.03385928599998));
#339339=CARTESIAN_POINT('Ctrl Pts',(2.78954156299994,5.2,3.03385928599998));
#339340=CARTESIAN_POINT('Ctrl Pts',(2.78954156299994,2.2,3.03385928599998));
#339341=CARTESIAN_POINT('Ctrl Pts',(2.78851813399994,12.2,3.03319117699999));
#339342=CARTESIAN_POINT('Ctrl Pts',(2.78851813399994,5.2,3.03319117699999));
#339343=CARTESIAN_POINT('Ctrl Pts',(2.78851813399994,2.2,3.03319117699999));
#339344=CARTESIAN_POINT('Ctrl Pts',(2.78749980299994,12.2,3.03252464699998));
#339345=CARTESIAN_POINT('Ctrl Pts',(2.78749980299994,5.2,3.03252464699998));
#339346=CARTESIAN_POINT('Ctrl Pts',(2.78749980299994,2.2,3.03252464699998));
#339347=CARTESIAN_POINT('Ctrl Pts',(2.78648657199994,12.2,3.03185970799999));
#339348=CARTESIAN_POINT('Ctrl Pts',(2.78648657199994,5.2,3.03185970799999));
#339349=CARTESIAN_POINT('Ctrl Pts',(2.78648657199994,2.2,3.03185970799999));
#339350=CARTESIAN_POINT('Ctrl Pts',(2.78547844199994,12.2,3.03119637799998));
#339351=CARTESIAN_POINT('Ctrl Pts',(2.78547844199994,5.2,3.03119637799998));
#339352=CARTESIAN_POINT('Ctrl Pts',(2.78547844199994,2.2,3.03119637799998));
#339353=CARTESIAN_POINT('Ctrl Pts',(2.78447541399995,12.2,3.03053467099998));
#339354=CARTESIAN_POINT('Ctrl Pts',(2.78447541399995,5.2,3.03053467099998));
#339355=CARTESIAN_POINT('Ctrl Pts',(2.78447541399995,2.2,3.03053467099998));
#339356=CARTESIAN_POINT('Ctrl Pts',(2.78347749099995,12.2,3.02987460199999));
#339357=CARTESIAN_POINT('Ctrl Pts',(2.78347749099995,5.2,3.02987460199999));
#339358=CARTESIAN_POINT('Ctrl Pts',(2.78347749099995,2.2,3.02987460199999));
#339359=CARTESIAN_POINT('Ctrl Pts',(2.78248467399994,12.2,3.02921618799999));
#339360=CARTESIAN_POINT('Ctrl Pts',(2.78248467399994,5.2,3.02921618799999));
#339361=CARTESIAN_POINT('Ctrl Pts',(2.78248467399994,2.2,3.02921618799999));
#339362=CARTESIAN_POINT('Ctrl Pts',(2.78149696399994,12.2,3.02855943999998));
#339363=CARTESIAN_POINT('Ctrl Pts',(2.78149696399994,5.2,3.02855943999998));
#339364=CARTESIAN_POINT('Ctrl Pts',(2.78149696399994,2.2,3.02855943999998));
#339365=CARTESIAN_POINT('Ctrl Pts',(2.78051436499994,12.2,3.02790437799998));
#339366=CARTESIAN_POINT('Ctrl Pts',(2.78051436499994,5.2,3.02790437799998));
#339367=CARTESIAN_POINT('Ctrl Pts',(2.78051436499994,2.2,3.02790437799998));
#339368=CARTESIAN_POINT('Ctrl Pts',(2.77953687699994,12.2,3.02725101399999));
#339369=CARTESIAN_POINT('Ctrl Pts',(2.77953687699994,5.2,3.02725101399999));
#339370=CARTESIAN_POINT('Ctrl Pts',(2.77953687699994,2.2,3.02725101399999));
#339371=CARTESIAN_POINT('Ctrl Pts',(2.77856450199994,12.2,3.02659936399999));
#339372=CARTESIAN_POINT('Ctrl Pts',(2.77856450199994,5.2,3.02659936399999));
#339373=CARTESIAN_POINT('Ctrl Pts',(2.77856450199994,2.2,3.02659936399999));
#339374=CARTESIAN_POINT('Ctrl Pts',(2.77759723999994,12.2,3.02594944399999));
#339375=CARTESIAN_POINT('Ctrl Pts',(2.77759723999994,5.2,3.02594944399999));
#339376=CARTESIAN_POINT('Ctrl Pts',(2.77759723999994,2.2,3.02594944399999));
#339377=CARTESIAN_POINT('Ctrl Pts',(2.77663509599994,12.2,3.02530126999999));
#339378=CARTESIAN_POINT('Ctrl Pts',(2.77663509599994,5.2,3.02530126999999));
#339379=CARTESIAN_POINT('Ctrl Pts',(2.77663509599994,2.2,3.02530126999999));
#339380=CARTESIAN_POINT('Ctrl Pts',(2.77567806899994,12.2,3.02465485599999));
#339381=CARTESIAN_POINT('Ctrl Pts',(2.77567806899994,5.2,3.02465485599999));
#339382=CARTESIAN_POINT('Ctrl Pts',(2.77567806899994,2.2,3.02465485599999));
#339383=CARTESIAN_POINT('Ctrl Pts',(2.77472616299994,12.2,3.02401021799999));
#339384=CARTESIAN_POINT('Ctrl Pts',(2.77472616299994,5.2,3.02401021799999));
#339385=CARTESIAN_POINT('Ctrl Pts',(2.77472616299994,2.2,3.02401021799999));
#339386=CARTESIAN_POINT('Ctrl Pts',(2.77377937599995,12.2,3.02336737099999));
#339387=CARTESIAN_POINT('Ctrl Pts',(2.77377937599995,5.2,3.02336737099999));
#339388=CARTESIAN_POINT('Ctrl Pts',(2.77377937599995,2.2,3.02336737099999));
#339389=CARTESIAN_POINT('Ctrl Pts',(2.77283771299994,12.2,3.02272633199999));
#339390=CARTESIAN_POINT('Ctrl Pts',(2.77283771299994,5.2,3.02272633199999));
#339391=CARTESIAN_POINT('Ctrl Pts',(2.77283771299994,2.2,3.02272633199999));
#339392=CARTESIAN_POINT('Ctrl Pts',(2.77190117299994,12.2,3.02208711399999));
#339393=CARTESIAN_POINT('Ctrl Pts',(2.77190117299994,5.2,3.02208711399999));
#339394=CARTESIAN_POINT('Ctrl Pts',(2.77190117299994,2.2,3.02208711399999));
#339395=CARTESIAN_POINT('Ctrl Pts',(2.77096975999994,12.2,3.02144973499999));
#339396=CARTESIAN_POINT('Ctrl Pts',(2.77096975999994,5.2,3.02144973499999));
#339397=CARTESIAN_POINT('Ctrl Pts',(2.77096975999994,2.2,3.02144973499999));
#339398=CARTESIAN_POINT('Ctrl Pts',(2.77004347399994,12.2,3.02081421099999));
#339399=CARTESIAN_POINT('Ctrl Pts',(2.77004347399994,5.2,3.02081421099999));
#339400=CARTESIAN_POINT('Ctrl Pts',(2.77004347399994,2.2,3.02081421099999));
#339401=CARTESIAN_POINT('Ctrl Pts',(2.76912231599994,12.2,3.02018055499998));
#339402=CARTESIAN_POINT('Ctrl Pts',(2.76912231599994,5.2,3.02018055499998));
#339403=CARTESIAN_POINT('Ctrl Pts',(2.76912231599994,2.2,3.02018055499998));
#339404=CARTESIAN_POINT('Ctrl Pts',(2.76820628899995,12.2,3.01954878399999));
#339405=CARTESIAN_POINT('Ctrl Pts',(2.76820628899995,5.2,3.01954878399999));
#339406=CARTESIAN_POINT('Ctrl Pts',(2.76820628899995,2.2,3.01954878399999));
#339407=CARTESIAN_POINT('Ctrl Pts',(2.76729539299994,12.2,3.01891891499999));
#339408=CARTESIAN_POINT('Ctrl Pts',(2.76729539299994,5.2,3.01891891499999));
#339409=CARTESIAN_POINT('Ctrl Pts',(2.76729539299994,2.2,3.01891891499999));
#339410=CARTESIAN_POINT('Ctrl Pts',(2.76638963099994,12.2,3.01829096199998));
#339411=CARTESIAN_POINT('Ctrl Pts',(2.76638963099994,5.2,3.01829096199998));
#339412=CARTESIAN_POINT('Ctrl Pts',(2.76638963099994,2.2,3.01829096199998));
#339413=CARTESIAN_POINT('Ctrl Pts',(2.76548900299994,12.2,3.01766494299999));
#339414=CARTESIAN_POINT('Ctrl Pts',(2.76548900299994,5.2,3.01766494299999));
#339415=CARTESIAN_POINT('Ctrl Pts',(2.76548900299994,2.2,3.01766494299999));
#339416=CARTESIAN_POINT('Ctrl Pts',(2.76459351099994,12.2,3.01704087099999));
#339417=CARTESIAN_POINT('Ctrl Pts',(2.76459351099994,5.2,3.01704087099999));
#339418=CARTESIAN_POINT('Ctrl Pts',(2.76459351099994,2.2,3.01704087099999));
#339419=CARTESIAN_POINT('Ctrl Pts',(2.76370315599994,12.2,3.01641876399999));
#339420=CARTESIAN_POINT('Ctrl Pts',(2.76370315599994,5.2,3.01641876399999));
#339421=CARTESIAN_POINT('Ctrl Pts',(2.76370315599994,2.2,3.01641876399999));
#339422=CARTESIAN_POINT('Ctrl Pts',(2.76281793999994,12.2,3.01579863699998));
#339423=CARTESIAN_POINT('Ctrl Pts',(2.76281793999994,5.2,3.01579863699998));
#339424=CARTESIAN_POINT('Ctrl Pts',(2.76281793999994,2.2,3.01579863699998));
#339425=CARTESIAN_POINT('Ctrl Pts',(2.76193786499995,12.2,3.01518050799999));
#339426=CARTESIAN_POINT('Ctrl Pts',(2.76193786499995,5.2,3.01518050799999));
#339427=CARTESIAN_POINT('Ctrl Pts',(2.76193786499995,2.2,3.01518050799999));
#339428=CARTESIAN_POINT('Ctrl Pts',(2.76106292999994,12.2,3.01456438999999));
#339429=CARTESIAN_POINT('Ctrl Pts',(2.76106292999994,5.2,3.01456438999999));
#339430=CARTESIAN_POINT('Ctrl Pts',(2.76106292999994,2.2,3.01456438999999));
#339431=CARTESIAN_POINT('Ctrl Pts',(2.76019313899994,12.2,3.01395030099999));
#339432=CARTESIAN_POINT('Ctrl Pts',(2.76019313899994,5.2,3.01395030099999));
#339433=CARTESIAN_POINT('Ctrl Pts',(2.76019313899994,2.2,3.01395030099999));
#339434=CARTESIAN_POINT('Ctrl Pts',(2.75932849199994,12.2,3.01333825799999));
#339435=CARTESIAN_POINT('Ctrl Pts',(2.75932849199994,5.2,3.01333825799999));
#339436=CARTESIAN_POINT('Ctrl Pts',(2.75932849199994,2.2,3.01333825799999));
#339437=CARTESIAN_POINT('Ctrl Pts',(2.75846898999994,12.2,3.01272827399998));
#339438=CARTESIAN_POINT('Ctrl Pts',(2.75846898999994,5.2,3.01272827399998));
#339439=CARTESIAN_POINT('Ctrl Pts',(2.75846898999994,2.2,3.01272827399998));
#339440=CARTESIAN_POINT('Ctrl Pts',(2.75761463499994,12.2,3.01212036899998));
#339441=CARTESIAN_POINT('Ctrl Pts',(2.75761463499994,5.2,3.01212036899998));
#339442=CARTESIAN_POINT('Ctrl Pts',(2.75761463499994,2.2,3.01212036899998));
#339443=CARTESIAN_POINT('Ctrl Pts',(2.75676542799994,12.2,3.01151455599998));
#339444=CARTESIAN_POINT('Ctrl Pts',(2.75676542799994,5.2,3.01151455599998));
#339445=CARTESIAN_POINT('Ctrl Pts',(2.75676542799994,2.2,3.01151455599998));
#339446=CARTESIAN_POINT('Ctrl Pts',(2.75592137099995,12.2,3.01091085199998));
#339447=CARTESIAN_POINT('Ctrl Pts',(2.75592137099995,5.2,3.01091085199998));
#339448=CARTESIAN_POINT('Ctrl Pts',(2.75592137099995,2.2,3.01091085199998));
#339449=CARTESIAN_POINT('Ctrl Pts',(2.75508246399994,12.2,3.01030927599999));
#339450=CARTESIAN_POINT('Ctrl Pts',(2.75508246399994,5.2,3.01030927599999));
#339451=CARTESIAN_POINT('Ctrl Pts',(2.75508246399994,2.2,3.01030927599999));
#339452=CARTESIAN_POINT('Ctrl Pts',(2.75424870799994,12.2,3.00970984099998));
#339453=CARTESIAN_POINT('Ctrl Pts',(2.75424870799994,5.2,3.00970984099998));
#339454=CARTESIAN_POINT('Ctrl Pts',(2.75424870799994,2.2,3.00970984099998));
#339455=CARTESIAN_POINT('Ctrl Pts',(2.75342010599994,12.2,3.00911256499998));
#339456=CARTESIAN_POINT('Ctrl Pts',(2.75342010599994,5.2,3.00911256499998));
#339457=CARTESIAN_POINT('Ctrl Pts',(2.75342010599994,2.2,3.00911256499998));
#339458=CARTESIAN_POINT('Ctrl Pts',(2.75259665699994,12.2,3.00851746499998));
#339459=CARTESIAN_POINT('Ctrl Pts',(2.75259665699994,5.2,3.00851746499998));
#339460=CARTESIAN_POINT('Ctrl Pts',(2.75259665699994,2.2,3.00851746499998));
#339461=CARTESIAN_POINT('Ctrl Pts',(2.75177836299994,12.2,3.00792455699998));
#339462=CARTESIAN_POINT('Ctrl Pts',(2.75177836299994,5.2,3.00792455699998));
#339463=CARTESIAN_POINT('Ctrl Pts',(2.75177836299994,2.2,3.00792455699998));
#339464=CARTESIAN_POINT('Ctrl Pts',(2.75096522599994,12.2,3.00733385699999));
#339465=CARTESIAN_POINT('Ctrl Pts',(2.75096522599994,5.2,3.00733385699999));
#339466=CARTESIAN_POINT('Ctrl Pts',(2.75096522599994,2.2,3.00733385699999));
#339467=CARTESIAN_POINT('Ctrl Pts',(2.75015724699994,12.2,3.00674538099998));
#339468=CARTESIAN_POINT('Ctrl Pts',(2.75015724699994,5.2,3.00674538099998));
#339469=CARTESIAN_POINT('Ctrl Pts',(2.75015724699994,2.2,3.00674538099998));
#339470=CARTESIAN_POINT('Ctrl Pts',(2.74935442599994,12.2,3.00615914699998));
#339471=CARTESIAN_POINT('Ctrl Pts',(2.74935442599994,5.2,3.00615914699998));
#339472=CARTESIAN_POINT('Ctrl Pts',(2.74935442599994,2.2,3.00615914699998));
#339473=CARTESIAN_POINT('Ctrl Pts',(2.74855676399994,12.2,3.00557517099998));
#339474=CARTESIAN_POINT('Ctrl Pts',(2.74855676399994,5.2,3.00557517099998));
#339475=CARTESIAN_POINT('Ctrl Pts',(2.74855676399994,2.2,3.00557517099998));
#339476=CARTESIAN_POINT('Ctrl Pts',(2.74776426299994,12.2,3.00499347099999));
#339477=CARTESIAN_POINT('Ctrl Pts',(2.74776426299994,5.2,3.00499347099999));
#339478=CARTESIAN_POINT('Ctrl Pts',(2.74776426299994,2.2,3.00499347099999));
#339479=CARTESIAN_POINT('Ctrl Pts',(2.74697692399994,12.2,3.00441406299999));
#339480=CARTESIAN_POINT('Ctrl Pts',(2.74697692399994,5.2,3.00441406299999));
#339481=CARTESIAN_POINT('Ctrl Pts',(2.74697692399994,2.2,3.00441406299999));
#339482=CARTESIAN_POINT('Ctrl Pts',(2.74619474799994,12.2,3.00383696199999));
#339483=CARTESIAN_POINT('Ctrl Pts',(2.74619474799994,5.2,3.00383696199999));
#339484=CARTESIAN_POINT('Ctrl Pts',(2.74619474799994,2.2,3.00383696199999));
#339485=CARTESIAN_POINT('Ctrl Pts',(2.74541773599994,12.2,3.00326218699999));
#339486=CARTESIAN_POINT('Ctrl Pts',(2.74541773599994,5.2,3.00326218699999));
#339487=CARTESIAN_POINT('Ctrl Pts',(2.74541773599994,2.2,3.00326218699999));
#339488=CARTESIAN_POINT('Ctrl Pts',(2.74464588799994,12.2,3.00268975499999));
#339489=CARTESIAN_POINT('Ctrl Pts',(2.74464588799994,5.2,3.00268975499999));
#339490=CARTESIAN_POINT('Ctrl Pts',(2.74464588799994,2.2,3.00268975499999));
#339491=CARTESIAN_POINT('Ctrl Pts',(2.74387920599994,12.2,3.00211968199999));
#339492=CARTESIAN_POINT('Ctrl Pts',(2.74387920599994,5.2,3.00211968199999));
#339493=CARTESIAN_POINT('Ctrl Pts',(2.74387920599994,2.2,3.00211968199999));
#339494=CARTESIAN_POINT('Ctrl Pts',(2.74311768999994,12.2,3.00155198599998));
#339495=CARTESIAN_POINT('Ctrl Pts',(2.74311768999994,5.2,3.00155198599998));
#339496=CARTESIAN_POINT('Ctrl Pts',(2.74311768999994,2.2,3.00155198599998));
#339497=CARTESIAN_POINT('Ctrl Pts',(2.74236134299994,12.2,3.00098668199999));
#339498=CARTESIAN_POINT('Ctrl Pts',(2.74236134299994,5.2,3.00098668199999));
#339499=CARTESIAN_POINT('Ctrl Pts',(2.74236134299994,2.2,3.00098668199999));
#339500=CARTESIAN_POINT('Ctrl Pts',(2.74161016399994,12.2,3.00042378899998));
#339501=CARTESIAN_POINT('Ctrl Pts',(2.74161016399994,5.2,3.00042378899998));
#339502=CARTESIAN_POINT('Ctrl Pts',(2.74161016399994,2.2,3.00042378899998));
#339503=CARTESIAN_POINT('Ctrl Pts',(2.74086415499994,12.2,2.99986332399998));
#339504=CARTESIAN_POINT('Ctrl Pts',(2.74086415499994,5.2,2.99986332399998));
#339505=CARTESIAN_POINT('Ctrl Pts',(2.74086415499994,2.2,2.99986332399998));
#339506=CARTESIAN_POINT('Ctrl Pts',(2.74012331499994,12.2,2.99930530299999));
#339507=CARTESIAN_POINT('Ctrl Pts',(2.74012331499994,5.2,2.99930530299999));
#339508=CARTESIAN_POINT('Ctrl Pts',(2.74012331499994,2.2,2.99930530299999));
#339509=CARTESIAN_POINT('Ctrl Pts',(2.73938764699994,12.2,2.99874974399999));
#339510=CARTESIAN_POINT('Ctrl Pts',(2.73938764699994,5.2,2.99874974399999));
#339511=CARTESIAN_POINT('Ctrl Pts',(2.73938764699994,2.2,2.99874974399999));
#339512=CARTESIAN_POINT('Ctrl Pts',(2.73865715199994,12.2,2.99819666399999));
#339513=CARTESIAN_POINT('Ctrl Pts',(2.73865715199994,5.2,2.99819666399999));
#339514=CARTESIAN_POINT('Ctrl Pts',(2.73865715199994,2.2,2.99819666399999));
#339515=CARTESIAN_POINT('Ctrl Pts',(2.73793182799994,12.2,2.99764608099998));
#339516=CARTESIAN_POINT('Ctrl Pts',(2.73793182799994,5.2,2.99764608099998));
#339517=CARTESIAN_POINT('Ctrl Pts',(2.73793182799994,2.2,2.99764608099998));
#339518=CARTESIAN_POINT('Ctrl Pts',(2.73721167799994,12.2,2.99709801099999));
#339519=CARTESIAN_POINT('Ctrl Pts',(2.73721167799994,5.2,2.99709801099999));
#339520=CARTESIAN_POINT('Ctrl Pts',(2.73721167799994,2.2,2.99709801099999));
#339521=CARTESIAN_POINT('Ctrl Pts',(2.73649670299994,12.2,2.99655247299999));
#339522=CARTESIAN_POINT('Ctrl Pts',(2.73649670299994,5.2,2.99655247299999));
#339523=CARTESIAN_POINT('Ctrl Pts',(2.73649670299994,2.2,2.99655247299999));
#339524=CARTESIAN_POINT('Ctrl Pts',(2.73578690299995,12.2,2.99600948399998));
#339525=CARTESIAN_POINT('Ctrl Pts',(2.73578690299995,5.2,2.99600948399998));
#339526=CARTESIAN_POINT('Ctrl Pts',(2.73578690299995,2.2,2.99600948399998));
#339527=CARTESIAN_POINT('Ctrl Pts',(2.73508227899995,12.2,2.99546906099999));
#339528=CARTESIAN_POINT('Ctrl Pts',(2.73508227899995,5.2,2.99546906099999));
#339529=CARTESIAN_POINT('Ctrl Pts',(2.73508227899995,2.2,2.99546906099999));
#339530=CARTESIAN_POINT('Ctrl Pts',(2.73438283199994,12.2,2.99493122099998));
#339531=CARTESIAN_POINT('Ctrl Pts',(2.73438283199994,5.2,2.99493122099998));
#339532=CARTESIAN_POINT('Ctrl Pts',(2.73438283199994,2.2,2.99493122099998));
#339533=CARTESIAN_POINT('Ctrl Pts',(2.73368856099995,12.2,2.99439598299998));
#339534=CARTESIAN_POINT('Ctrl Pts',(2.73368856099995,5.2,2.99439598299998));
#339535=CARTESIAN_POINT('Ctrl Pts',(2.73368856099995,2.2,2.99439598299998));
#339536=CARTESIAN_POINT('Ctrl Pts',(2.73299946899995,12.2,2.99386336399999));
#339537=CARTESIAN_POINT('Ctrl Pts',(2.73299946899995,5.2,2.99386336399999));
#339538=CARTESIAN_POINT('Ctrl Pts',(2.73299946899995,2.2,2.99386336399999));
#339539=CARTESIAN_POINT('Ctrl Pts',(2.73231555499994,12.2,2.99333338199999));
#339540=CARTESIAN_POINT('Ctrl Pts',(2.73231555499994,5.2,2.99333338199999));
#339541=CARTESIAN_POINT('Ctrl Pts',(2.73231555499994,2.2,2.99333338199999));
#339542=CARTESIAN_POINT('Ctrl Pts',(2.73163682099994,12.2,2.99280605399999));
#339543=CARTESIAN_POINT('Ctrl Pts',(2.73163682099994,5.2,2.99280605399999));
#339544=CARTESIAN_POINT('Ctrl Pts',(2.73163682099994,2.2,2.99280605399999));
#339545=CARTESIAN_POINT('Ctrl Pts',(2.73096326699994,12.2,2.99228139699999));
#339546=CARTESIAN_POINT('Ctrl Pts',(2.73096326699994,5.2,2.99228139699999));
#339547=CARTESIAN_POINT('Ctrl Pts',(2.73096326699994,2.2,2.99228139699999));
#339548=CARTESIAN_POINT('Ctrl Pts',(2.73029489299994,12.2,2.99175943199998));
#339549=CARTESIAN_POINT('Ctrl Pts',(2.73029489299994,5.2,2.99175943199998));
#339550=CARTESIAN_POINT('Ctrl Pts',(2.73029489299994,2.2,2.99175943199998));
#339551=CARTESIAN_POINT('Ctrl Pts',(2.72963169999994,12.2,2.99124017399999));
#339552=CARTESIAN_POINT('Ctrl Pts',(2.72963169999994,5.2,2.99124017399999));
#339553=CARTESIAN_POINT('Ctrl Pts',(2.72963169999994,2.2,2.99124017399999));
#339554=CARTESIAN_POINT('Ctrl Pts',(2.72897368899994,12.2,2.99072364099998));
#339555=CARTESIAN_POINT('Ctrl Pts',(2.72897368899994,5.2,2.99072364099998));
#339556=CARTESIAN_POINT('Ctrl Pts',(2.72897368899994,2.2,2.99072364099998));
#339557=CARTESIAN_POINT('Ctrl Pts',(2.72832085899994,12.2,2.99020985299999));
#339558=CARTESIAN_POINT('Ctrl Pts',(2.72832085899994,5.2,2.99020985299999));
#339559=CARTESIAN_POINT('Ctrl Pts',(2.72832085899994,2.2,2.99020985299999));
#339560=CARTESIAN_POINT('Ctrl Pts',(2.72767321299995,12.2,2.98969882599998));
#339561=CARTESIAN_POINT('Ctrl Pts',(2.72767321299995,5.2,2.98969882599998));
#339562=CARTESIAN_POINT('Ctrl Pts',(2.72767321299995,2.2,2.98969882599998));
#339563=CARTESIAN_POINT('Ctrl Pts',(2.72703074999994,12.2,2.98919057999999));
#339564=CARTESIAN_POINT('Ctrl Pts',(2.72703074999994,5.2,2.98919057999999));
#339565=CARTESIAN_POINT('Ctrl Pts',(2.72703074999994,2.2,2.98919057999999));
#339566=CARTESIAN_POINT('Ctrl Pts',(2.72639347099994,12.2,2.98868513199999));
#339567=CARTESIAN_POINT('Ctrl Pts',(2.72639347099994,5.2,2.98868513199999));
#339568=CARTESIAN_POINT('Ctrl Pts',(2.72639347099994,2.2,2.98868513199999));
#339569=CARTESIAN_POINT('Ctrl Pts',(2.72576137499994,12.2,2.98818249999999));
#339570=CARTESIAN_POINT('Ctrl Pts',(2.72576137499994,5.2,2.98818249999999));
#339571=CARTESIAN_POINT('Ctrl Pts',(2.72576137499994,2.2,2.98818249999999));
#339572=CARTESIAN_POINT('Ctrl Pts',(2.72513446399994,12.2,2.98768270099998));
#339573=CARTESIAN_POINT('Ctrl Pts',(2.72513446399994,5.2,2.98768270099998));
#339574=CARTESIAN_POINT('Ctrl Pts',(2.72513446399994,2.2,2.98768270099998));
#339575=CARTESIAN_POINT('Ctrl Pts',(2.72451273799994,12.2,2.98718575599998));
#339576=CARTESIAN_POINT('Ctrl Pts',(2.72451273799994,5.2,2.98718575599998));
#339577=CARTESIAN_POINT('Ctrl Pts',(2.72451273799994,2.2,2.98718575599998));
#339578=CARTESIAN_POINT('Ctrl Pts',(2.72389619799994,12.2,2.98669168199999));
#339579=CARTESIAN_POINT('Ctrl Pts',(2.72389619799994,5.2,2.98669168199999));
#339580=CARTESIAN_POINT('Ctrl Pts',(2.72389619799994,2.2,2.98669168199999));
#339581=CARTESIAN_POINT('Ctrl Pts',(2.72328484299994,12.2,2.98620049699998));
#339582=CARTESIAN_POINT('Ctrl Pts',(2.72328484299994,5.2,2.98620049699998));
#339583=CARTESIAN_POINT('Ctrl Pts',(2.72328484299994,2.2,2.98620049699998));
#339584=CARTESIAN_POINT('Ctrl Pts',(2.72267867399994,12.2,2.98571222099999));
#339585=CARTESIAN_POINT('Ctrl Pts',(2.72267867399994,5.2,2.98571222099999));
#339586=CARTESIAN_POINT('Ctrl Pts',(2.72267867399994,2.2,2.98571222099999));
#339587=CARTESIAN_POINT('Ctrl Pts',(2.72207768999994,12.2,2.98522686999998));
#339588=CARTESIAN_POINT('Ctrl Pts',(2.72207768999994,5.2,2.98522686999998));
#339589=CARTESIAN_POINT('Ctrl Pts',(2.72207768999994,2.2,2.98522686999998));
#339590=CARTESIAN_POINT('Ctrl Pts',(2.72148189399994,12.2,2.98474446399998));
#339591=CARTESIAN_POINT('Ctrl Pts',(2.72148189399994,5.2,2.98474446399998));
#339592=CARTESIAN_POINT('Ctrl Pts',(2.72148189399994,2.2,2.98474446399998));
#339593=CARTESIAN_POINT('Ctrl Pts',(2.72089128599994,12.2,2.98426502199998));
#339594=CARTESIAN_POINT('Ctrl Pts',(2.72089128599994,5.2,2.98426502199998));
#339595=CARTESIAN_POINT('Ctrl Pts',(2.72089128599994,2.2,2.98426502199998));
#339596=CARTESIAN_POINT('Ctrl Pts',(2.72030586299994,12.2,2.98378856299998));
#339597=CARTESIAN_POINT('Ctrl Pts',(2.72030586299994,5.2,2.98378856299998));
#339598=CARTESIAN_POINT('Ctrl Pts',(2.72030586299994,2.2,2.98378856299998));
#339599=CARTESIAN_POINT('Ctrl Pts',(2.71972562899994,12.2,2.98331510299998));
#339600=CARTESIAN_POINT('Ctrl Pts',(2.71972562899994,5.2,2.98331510299998));
#339601=CARTESIAN_POINT('Ctrl Pts',(2.71972562899994,2.2,2.98331510299998));
#339602=CARTESIAN_POINT('Ctrl Pts',(2.71915058199995,12.2,2.98284466299998));
#339603=CARTESIAN_POINT('Ctrl Pts',(2.71915058199995,5.2,2.98284466299998));
#339604=CARTESIAN_POINT('Ctrl Pts',(2.71915058199995,2.2,2.98284466299998));
#339605=CARTESIAN_POINT('Ctrl Pts',(2.71858072299994,12.2,2.98237726199999));
#339606=CARTESIAN_POINT('Ctrl Pts',(2.71858072299994,5.2,2.98237726199999));
#339607=CARTESIAN_POINT('Ctrl Pts',(2.71858072299994,2.2,2.98237726199999));
#339608=CARTESIAN_POINT('Ctrl Pts',(2.71801605199995,12.2,2.98191291799998));
#339609=CARTESIAN_POINT('Ctrl Pts',(2.71801605199995,5.2,2.98191291799998));
#339610=CARTESIAN_POINT('Ctrl Pts',(2.71801605199995,2.2,2.98191291799998));
#339611=CARTESIAN_POINT('Ctrl Pts',(2.71745656899995,12.2,2.98145165099999));
#339612=CARTESIAN_POINT('Ctrl Pts',(2.71745656899995,5.2,2.98145165099999));
#339613=CARTESIAN_POINT('Ctrl Pts',(2.71745656899995,2.2,2.98145165099999));
#339614=CARTESIAN_POINT('Ctrl Pts',(2.71690227399994,12.2,2.98099347799998));
#339615=CARTESIAN_POINT('Ctrl Pts',(2.71690227399994,5.2,2.98099347799998));
#339616=CARTESIAN_POINT('Ctrl Pts',(2.71690227399994,2.2,2.98099347799998));
#339617=CARTESIAN_POINT('Ctrl Pts',(2.71635316699995,12.2,2.98053841899999));
#339618=CARTESIAN_POINT('Ctrl Pts',(2.71635316699995,5.2,2.98053841899999));
#339619=CARTESIAN_POINT('Ctrl Pts',(2.71635316699995,2.2,2.98053841899999));
#339620=CARTESIAN_POINT('Ctrl Pts',(2.71580924999994,12.2,2.98008649399998));
#339621=CARTESIAN_POINT('Ctrl Pts',(2.71580924999994,5.2,2.98008649399998));
#339622=CARTESIAN_POINT('Ctrl Pts',(2.71580924999994,2.2,2.98008649399998));
#339623=CARTESIAN_POINT('Ctrl Pts',(2.71527051999994,12.2,2.97963772099998));
#339624=CARTESIAN_POINT('Ctrl Pts',(2.71527051999994,5.2,2.97963772099998));
#339625=CARTESIAN_POINT('Ctrl Pts',(2.71527051999994,2.2,2.97963772099998));
#339626=CARTESIAN_POINT('Ctrl Pts',(2.71473697799994,12.2,2.97919211899998));
#339627=CARTESIAN_POINT('Ctrl Pts',(2.71473697799994,5.2,2.97919211899998));
#339628=CARTESIAN_POINT('Ctrl Pts',(2.71473697799994,2.2,2.97919211899998));
#339629=CARTESIAN_POINT('Ctrl Pts',(2.71420862599994,12.2,2.97874970699999));
#339630=CARTESIAN_POINT('Ctrl Pts',(2.71420862599994,5.2,2.97874970699999));
#339631=CARTESIAN_POINT('Ctrl Pts',(2.71420862599994,2.2,2.97874970699999));
#339632=CARTESIAN_POINT('Ctrl Pts',(2.71368546199994,12.2,2.97831050599999));
#339633=CARTESIAN_POINT('Ctrl Pts',(2.71368546199994,5.2,2.97831050599999));
#339634=CARTESIAN_POINT('Ctrl Pts',(2.71368546199994,2.2,2.97831050599999));
#339635=CARTESIAN_POINT('Ctrl Pts',(2.71316748599994,12.2,2.97787453299998));
#339636=CARTESIAN_POINT('Ctrl Pts',(2.71316748599994,5.2,2.97787453299998));
#339637=CARTESIAN_POINT('Ctrl Pts',(2.71316748599994,2.2,2.97787453299998));
#339638=CARTESIAN_POINT('Ctrl Pts',(2.71265469899994,12.2,2.97744181099999));
#339639=CARTESIAN_POINT('Ctrl Pts',(2.71265469899994,5.2,2.97744181099999));
#339640=CARTESIAN_POINT('Ctrl Pts',(2.71265469899994,2.2,2.97744181099999));
#339641=CARTESIAN_POINT('Ctrl Pts',(2.71214709999994,12.2,2.97701235599998));
#339642=CARTESIAN_POINT('Ctrl Pts',(2.71214709999994,5.2,2.97701235599998));
#339643=CARTESIAN_POINT('Ctrl Pts',(2.71214709999994,2.2,2.97701235599998));
#339644=CARTESIAN_POINT('Ctrl Pts',(2.71164468899994,12.2,2.97658618899998));
#339645=CARTESIAN_POINT('Ctrl Pts',(2.71164468899994,5.2,2.97658618899998));
#339646=CARTESIAN_POINT('Ctrl Pts',(2.71164468899994,2.2,2.97658618899998));
#339647=CARTESIAN_POINT('Ctrl Pts',(2.71114746499994,12.2,2.97616332799999));
#339648=CARTESIAN_POINT('Ctrl Pts',(2.71114746499994,5.2,2.97616332799999));
#339649=CARTESIAN_POINT('Ctrl Pts',(2.71114746499994,2.2,2.97616332799999));
#339650=CARTESIAN_POINT('Ctrl Pts',(2.71065543099994,12.2,2.97574379499999));
#339651=CARTESIAN_POINT('Ctrl Pts',(2.71065543099994,5.2,2.97574379499999));
#339652=CARTESIAN_POINT('Ctrl Pts',(2.71065543099994,2.2,2.97574379499999));
#339653=CARTESIAN_POINT('Ctrl Pts',(2.71016858299994,12.2,2.97532760899998));
#339654=CARTESIAN_POINT('Ctrl Pts',(2.71016858299994,5.2,2.97532760899998));
#339655=CARTESIAN_POINT('Ctrl Pts',(2.71016858299994,2.2,2.97532760899998));
#339656=CARTESIAN_POINT('Ctrl Pts',(2.70968692299994,12.2,2.97491478899998));
#339657=CARTESIAN_POINT('Ctrl Pts',(2.70968692299994,5.2,2.97491478899998));
#339658=CARTESIAN_POINT('Ctrl Pts',(2.70968692299994,2.2,2.97491478899998));
#339659=CARTESIAN_POINT('Ctrl Pts',(2.70921044999994,12.2,2.97450535399998));
#339660=CARTESIAN_POINT('Ctrl Pts',(2.70921044999994,5.2,2.97450535399998));
#339661=CARTESIAN_POINT('Ctrl Pts',(2.70921044999994,2.2,2.97450535399998));
#339662=CARTESIAN_POINT('Ctrl Pts',(2.70873916399994,12.2,2.97409932599999));
#339663=CARTESIAN_POINT('Ctrl Pts',(2.70873916399994,5.2,2.97409932599999));
#339664=CARTESIAN_POINT('Ctrl Pts',(2.70873916399994,2.2,2.97409932599999));
#339665=CARTESIAN_POINT('Ctrl Pts',(2.70827306599994,12.2,2.97369672399999));
#339666=CARTESIAN_POINT('Ctrl Pts',(2.70827306599994,5.2,2.97369672399999));
#339667=CARTESIAN_POINT('Ctrl Pts',(2.70827306599994,2.2,2.97369672399999));
#339668=CARTESIAN_POINT('Ctrl Pts',(2.70781215299994,12.2,2.97329756699998));
#339669=CARTESIAN_POINT('Ctrl Pts',(2.70781215299994,5.2,2.97329756699998));
#339670=CARTESIAN_POINT('Ctrl Pts',(2.70781215299994,2.2,2.97329756699998));
#339671=CARTESIAN_POINT('Ctrl Pts',(2.70735642699994,12.2,2.97290187599998));
#339672=CARTESIAN_POINT('Ctrl Pts',(2.70735642699994,5.2,2.97290187599998));
#339673=CARTESIAN_POINT('Ctrl Pts',(2.70735642699994,2.2,2.97290187599998));
#339674=CARTESIAN_POINT('Ctrl Pts',(2.70690588599994,12.2,2.97250967099998));
#339675=CARTESIAN_POINT('Ctrl Pts',(2.70690588599994,5.2,2.97250967099998));
#339676=CARTESIAN_POINT('Ctrl Pts',(2.70690588599994,2.2,2.97250967099998));
#339677=CARTESIAN_POINT('Ctrl Pts',(2.70646052999994,12.2,2.97212097299998));
#339678=CARTESIAN_POINT('Ctrl Pts',(2.70646052999994,5.2,2.97212097299998));
#339679=CARTESIAN_POINT('Ctrl Pts',(2.70646052999994,2.2,2.97212097299998));
#339680=CARTESIAN_POINT('Ctrl Pts',(2.70602035899994,12.2,2.97173580099999));
#339681=CARTESIAN_POINT('Ctrl Pts',(2.70602035899994,5.2,2.97173580099999));
#339682=CARTESIAN_POINT('Ctrl Pts',(2.70602035899994,2.2,2.97173580099999));
#339683=CARTESIAN_POINT('Ctrl Pts',(2.70558537299994,12.2,2.97135417599999));
#339684=CARTESIAN_POINT('Ctrl Pts',(2.70558537299994,5.2,2.97135417599999));
#339685=CARTESIAN_POINT('Ctrl Pts',(2.70558537299994,2.2,2.97135417599999));
#339686=CARTESIAN_POINT('Ctrl Pts',(2.70515557099994,12.2,2.97097611699999));
#339687=CARTESIAN_POINT('Ctrl Pts',(2.70515557099994,5.2,2.97097611699999));
#339688=CARTESIAN_POINT('Ctrl Pts',(2.70515557099994,2.2,2.97097611699999));
#339689=CARTESIAN_POINT('Ctrl Pts',(2.70473095299995,12.2,2.97060164499998));
#339690=CARTESIAN_POINT('Ctrl Pts',(2.70473095299995,5.2,2.97060164499998));
#339691=CARTESIAN_POINT('Ctrl Pts',(2.70473095299995,2.2,2.97060164499998));
#339692=CARTESIAN_POINT('Ctrl Pts',(2.70431151699994,12.2,2.97023078199998));
#339693=CARTESIAN_POINT('Ctrl Pts',(2.70431151699994,5.2,2.97023078199998));
#339694=CARTESIAN_POINT('Ctrl Pts',(2.70431151699994,2.2,2.97023078199998));
#339695=CARTESIAN_POINT('Ctrl Pts',(2.70389726299994,12.2,2.96986354699998));
#339696=CARTESIAN_POINT('Ctrl Pts',(2.70389726299994,5.2,2.96986354699998));
#339697=CARTESIAN_POINT('Ctrl Pts',(2.70389726299994,2.2,2.96986354699998));
#339698=CARTESIAN_POINT('Ctrl Pts',(2.70348819199994,12.2,2.96949996099999));
#339699=CARTESIAN_POINT('Ctrl Pts',(2.70348819199994,5.2,2.96949996099999));
#339700=CARTESIAN_POINT('Ctrl Pts',(2.70348819199994,2.2,2.96949996099999));
#339701=CARTESIAN_POINT('Ctrl Pts',(2.70308430199994,12.2,2.96914004499998));
#339702=CARTESIAN_POINT('Ctrl Pts',(2.70308430199994,5.2,2.96914004499998));
#339703=CARTESIAN_POINT('Ctrl Pts',(2.70308430199994,2.2,2.96914004499998));
#339704=CARTESIAN_POINT('Ctrl Pts',(2.70268559399995,12.2,2.96878381799999));
#339705=CARTESIAN_POINT('Ctrl Pts',(2.70268559399995,5.2,2.96878381799999));
#339706=CARTESIAN_POINT('Ctrl Pts',(2.70268559399995,2.2,2.96878381799999));
#339707=CARTESIAN_POINT('Ctrl Pts',(2.70229206499994,12.2,2.96843130299998));
#339708=CARTESIAN_POINT('Ctrl Pts',(2.70229206499994,5.2,2.96843130299998));
#339709=CARTESIAN_POINT('Ctrl Pts',(2.70229206499994,2.2,2.96843130299998));
#339710=CARTESIAN_POINT('Ctrl Pts',(2.70190371499994,12.2,2.96808251899999));
#339711=CARTESIAN_POINT('Ctrl Pts',(2.70190371499994,5.2,2.96808251899999));
#339712=CARTESIAN_POINT('Ctrl Pts',(2.70190371499994,2.2,2.96808251899999));
#339713=CARTESIAN_POINT('Ctrl Pts',(2.70152054299994,12.2,2.96773748899999));
#339714=CARTESIAN_POINT('Ctrl Pts',(2.70152054299994,5.2,2.96773748899999));
#339715=CARTESIAN_POINT('Ctrl Pts',(2.70152054299994,2.2,2.96773748899999));
#339716=CARTESIAN_POINT('Ctrl Pts',(2.70114255199994,12.2,2.96739623199999));
#339717=CARTESIAN_POINT('Ctrl Pts',(2.70114255199994,5.2,2.96739623199999));
#339718=CARTESIAN_POINT('Ctrl Pts',(2.70114255199994,2.2,2.96739623199999));
#339719=CARTESIAN_POINT('Ctrl Pts',(2.70076973599994,12.2,2.96705876999999));
#339720=CARTESIAN_POINT('Ctrl Pts',(2.70076973599994,5.2,2.96705876999999));
#339721=CARTESIAN_POINT('Ctrl Pts',(2.70076973599994,2.2,2.96705876999999));
#339722=CARTESIAN_POINT('Ctrl Pts',(2.70040209599994,12.2,2.96672512299998));
#339723=CARTESIAN_POINT('Ctrl Pts',(2.70040209599994,5.2,2.96672512299998));
#339724=CARTESIAN_POINT('Ctrl Pts',(2.70040209599994,2.2,2.96672512299998));
#339725=CARTESIAN_POINT('Ctrl Pts',(2.70003963199994,12.2,2.96639531499999));
#339726=CARTESIAN_POINT('Ctrl Pts',(2.70003963199994,5.2,2.96639531499999));
#339727=CARTESIAN_POINT('Ctrl Pts',(2.70003963199994,2.2,2.96639531499999));
#339728=CARTESIAN_POINT('Ctrl Pts',(2.69968234399995,12.2,2.96606936399999));
#339729=CARTESIAN_POINT('Ctrl Pts',(2.69968234399995,5.2,2.96606936399999));
#339730=CARTESIAN_POINT('Ctrl Pts',(2.69968234399995,2.2,2.96606936399999));
#339731=CARTESIAN_POINT('Ctrl Pts',(2.69933022999994,12.2,2.96574729199998));
#339732=CARTESIAN_POINT('Ctrl Pts',(2.69933022999994,5.2,2.96574729199998));
#339733=CARTESIAN_POINT('Ctrl Pts',(2.69933022999994,2.2,2.96574729199998));
#339734=CARTESIAN_POINT('Ctrl Pts',(2.69898328799994,12.2,2.96542912099999));
#339735=CARTESIAN_POINT('Ctrl Pts',(2.69898328799994,5.2,2.96542912099999));
#339736=CARTESIAN_POINT('Ctrl Pts',(2.69898328799994,2.2,2.96542912099999));
#339737=CARTESIAN_POINT('Ctrl Pts',(2.69864151899994,12.2,2.96511487199999));
#339738=CARTESIAN_POINT('Ctrl Pts',(2.69864151899994,5.2,2.96511487199999));
#339739=CARTESIAN_POINT('Ctrl Pts',(2.69864151899994,2.2,2.96511487199999));
#339740=CARTESIAN_POINT('Ctrl Pts',(2.69830492099994,12.2,2.96480456799999));
#339741=CARTESIAN_POINT('Ctrl Pts',(2.69830492099994,5.2,2.96480456799999));
#339742=CARTESIAN_POINT('Ctrl Pts',(2.69830492099994,2.2,2.96480456799999));
#339743=CARTESIAN_POINT('Ctrl Pts',(2.69797349399994,12.2,2.96449822799998));
#339744=CARTESIAN_POINT('Ctrl Pts',(2.69797349399994,5.2,2.96449822799998));
#339745=CARTESIAN_POINT('Ctrl Pts',(2.69797349399994,2.2,2.96449822799998));
#339746=CARTESIAN_POINT('Ctrl Pts',(2.69764723399994,12.2,2.96419587599999));
#339747=CARTESIAN_POINT('Ctrl Pts',(2.69764723399994,5.2,2.96419587599999));
#339748=CARTESIAN_POINT('Ctrl Pts',(2.69764723399994,2.2,2.96419587599999));
#339749=CARTESIAN_POINT('Ctrl Pts',(2.69732614499994,12.2,2.96389753299999));
#339750=CARTESIAN_POINT('Ctrl Pts',(2.69732614499994,5.2,2.96389753299999));
#339751=CARTESIAN_POINT('Ctrl Pts',(2.69732614499994,2.2,2.96389753299999));
#339752=CARTESIAN_POINT('Ctrl Pts',(2.69701022099994,12.2,2.96360321899999));
#339753=CARTESIAN_POINT('Ctrl Pts',(2.69701022099994,5.2,2.96360321899999));
#339754=CARTESIAN_POINT('Ctrl Pts',(2.69701022099994,2.2,2.96360321899999));
#339755=CARTESIAN_POINT('Ctrl Pts',(2.69669946499994,12.2,2.96331295699999));
#339756=CARTESIAN_POINT('Ctrl Pts',(2.69669946499994,5.2,2.96331295699999));
#339757=CARTESIAN_POINT('Ctrl Pts',(2.69669946499994,2.2,2.96331295699999));
#339758=CARTESIAN_POINT('Ctrl Pts',(2.69639387299994,12.2,2.96302676999999));
#339759=CARTESIAN_POINT('Ctrl Pts',(2.69639387299994,5.2,2.96302676999999));
#339760=CARTESIAN_POINT('Ctrl Pts',(2.69639387299994,2.2,2.96302676999999));
#339761=CARTESIAN_POINT('Ctrl Pts',(2.69609344499994,12.2,2.96274467999999));
#339762=CARTESIAN_POINT('Ctrl Pts',(2.69609344499994,5.2,2.96274467999999));
#339763=CARTESIAN_POINT('Ctrl Pts',(2.69609344499994,2.2,2.96274467999999));
#339764=CARTESIAN_POINT('Ctrl Pts',(2.69579818099994,12.2,2.96246670699999));
#339765=CARTESIAN_POINT('Ctrl Pts',(2.69579818099994,5.2,2.96246670699999));
#339766=CARTESIAN_POINT('Ctrl Pts',(2.69579818099994,2.2,2.96246670699999));
#339767=CARTESIAN_POINT('Ctrl Pts',(2.69550807599995,12.2,2.96219287399998));
#339768=CARTESIAN_POINT('Ctrl Pts',(2.69550807599995,5.2,2.96219287399998));
#339769=CARTESIAN_POINT('Ctrl Pts',(2.69550807599995,2.2,2.96219287399998));
#339770=CARTESIAN_POINT('Ctrl Pts',(2.69522313299994,12.2,2.96192320399999));
#339771=CARTESIAN_POINT('Ctrl Pts',(2.69522313299994,5.2,2.96192320399999));
#339772=CARTESIAN_POINT('Ctrl Pts',(2.69522313299994,2.2,2.96192320399999));
#339773=CARTESIAN_POINT('Ctrl Pts',(2.69494334899994,12.2,2.96165771799998));
#339774=CARTESIAN_POINT('Ctrl Pts',(2.69494334899994,5.2,2.96165771799998));
#339775=CARTESIAN_POINT('Ctrl Pts',(2.69494334899994,2.2,2.96165771799998));
#339776=CARTESIAN_POINT('Ctrl Pts',(2.69466872299994,12.2,2.96139643899998));
#339777=CARTESIAN_POINT('Ctrl Pts',(2.69466872299994,5.2,2.96139643899998));
#339778=CARTESIAN_POINT('Ctrl Pts',(2.69466872299994,2.2,2.96139643899998));
#339779=CARTESIAN_POINT('Ctrl Pts',(2.69439925299995,12.2,2.96113938999999));
#339780=CARTESIAN_POINT('Ctrl Pts',(2.69439925299995,5.2,2.96113938999999));
#339781=CARTESIAN_POINT('Ctrl Pts',(2.69439925299995,2.2,2.96113938999999));
#339782=CARTESIAN_POINT('Ctrl Pts',(2.69413493799994,12.2,2.96088659199999));
#339783=CARTESIAN_POINT('Ctrl Pts',(2.69413493799994,5.2,2.96088659199999));
#339784=CARTESIAN_POINT('Ctrl Pts',(2.69413493799994,2.2,2.96088659199999));
#339785=CARTESIAN_POINT('Ctrl Pts',(2.69387577699994,12.2,2.96063806999998));
#339786=CARTESIAN_POINT('Ctrl Pts',(2.69387577699994,5.2,2.96063806999998));
#339787=CARTESIAN_POINT('Ctrl Pts',(2.69387577699994,2.2,2.96063806999998));
#339788=CARTESIAN_POINT('Ctrl Pts',(2.69362176799994,12.2,2.96039384299998));
#339789=CARTESIAN_POINT('Ctrl Pts',(2.69362176799994,5.2,2.96039384299998));
#339790=CARTESIAN_POINT('Ctrl Pts',(2.69362176799994,2.2,2.96039384299998));
#339791=CARTESIAN_POINT('Ctrl Pts',(2.69337290999994,12.2,2.96015393599999));
#339792=CARTESIAN_POINT('Ctrl Pts',(2.69337290999994,5.2,2.96015393599999));
#339793=CARTESIAN_POINT('Ctrl Pts',(2.69337290999994,2.2,2.96015393599999));
#339794=CARTESIAN_POINT('Ctrl Pts',(2.69312920199994,12.2,2.95991837199999));
#339795=CARTESIAN_POINT('Ctrl Pts',(2.69312920199994,5.2,2.95991837199999));
#339796=CARTESIAN_POINT('Ctrl Pts',(2.69312920199994,2.2,2.95991837199999));
#339797=CARTESIAN_POINT('Ctrl Pts',(2.69289064099994,12.2,2.95968717299999));
#339798=CARTESIAN_POINT('Ctrl Pts',(2.69289064099994,5.2,2.95968717299999));
#339799=CARTESIAN_POINT('Ctrl Pts',(2.69289064099994,2.2,2.95968717299999));
#339800=CARTESIAN_POINT('Ctrl Pts',(2.69265722699994,12.2,2.95946036199998));
#339801=CARTESIAN_POINT('Ctrl Pts',(2.69265722699994,5.2,2.95946036199998));
#339802=CARTESIAN_POINT('Ctrl Pts',(2.69265722699994,2.2,2.95946036199998));
#339803=CARTESIAN_POINT('Ctrl Pts',(2.69242895799994,12.2,2.95923796299999));
#339804=CARTESIAN_POINT('Ctrl Pts',(2.69242895799994,5.2,2.95923796299999));
#339805=CARTESIAN_POINT('Ctrl Pts',(2.69242895799994,2.2,2.95923796299999));
#339806=CARTESIAN_POINT('Ctrl Pts',(2.69220583199994,12.2,2.95901999699999));
#339807=CARTESIAN_POINT('Ctrl Pts',(2.69220583199994,5.2,2.95901999699999));
#339808=CARTESIAN_POINT('Ctrl Pts',(2.69220583199994,2.2,2.95901999699999));
#339809=CARTESIAN_POINT('Ctrl Pts',(2.69198784799995,12.2,2.95880648799999));
#339810=CARTESIAN_POINT('Ctrl Pts',(2.69198784799995,5.2,2.95880648799999));
#339811=CARTESIAN_POINT('Ctrl Pts',(2.69198784799995,2.2,2.95880648799999));
#339812=CARTESIAN_POINT('Ctrl Pts',(2.69177500299994,12.2,2.95859746099998));
#339813=CARTESIAN_POINT('Ctrl Pts',(2.69177500299994,5.2,2.95859746099998));
#339814=CARTESIAN_POINT('Ctrl Pts',(2.69177500299994,2.2,2.95859746099998));
#339815=CARTESIAN_POINT('Ctrl Pts',(2.69156729699994,12.2,2.95839293699999));
#339816=CARTESIAN_POINT('Ctrl Pts',(2.69156729699994,5.2,2.95839293699999));
#339817=CARTESIAN_POINT('Ctrl Pts',(2.69156729699994,2.2,2.95839293699999));
#339818=CARTESIAN_POINT('Ctrl Pts',(2.69136472799994,12.2,2.95819293999998));
#339819=CARTESIAN_POINT('Ctrl Pts',(2.69136472799994,5.2,2.95819293999998));
#339820=CARTESIAN_POINT('Ctrl Pts',(2.69136472799994,2.2,2.95819293999998));
#339821=CARTESIAN_POINT('Ctrl Pts',(2.69116729299994,12.2,2.95799749299999));
#339822=CARTESIAN_POINT('Ctrl Pts',(2.69116729299994,5.2,2.95799749299999));
#339823=CARTESIAN_POINT('Ctrl Pts',(2.69116729299994,2.2,2.95799749299999));
#339824=CARTESIAN_POINT('Ctrl Pts',(2.69097499199995,12.2,2.95780662099999));
#339825=CARTESIAN_POINT('Ctrl Pts',(2.69097499199995,5.2,2.95780662099999));
#339826=CARTESIAN_POINT('Ctrl Pts',(2.69097499199995,2.2,2.95780662099999));
#339827=CARTESIAN_POINT('Ctrl Pts',(2.69078782199994,12.2,2.95762034699998));
#339828=CARTESIAN_POINT('Ctrl Pts',(2.69078782199994,5.2,2.95762034699998));
#339829=CARTESIAN_POINT('Ctrl Pts',(2.69078782199994,2.2,2.95762034699998));
#339830=CARTESIAN_POINT('Ctrl Pts',(2.69060577999995,12.2,2.95743869399999));
#339831=CARTESIAN_POINT('Ctrl Pts',(2.69060577999995,5.2,2.95743869399999));
#339832=CARTESIAN_POINT('Ctrl Pts',(2.69060577999995,2.2,2.95743869399999));
#339833=CARTESIAN_POINT('Ctrl Pts',(2.69042886699994,12.2,2.95726168599998));
#339834=CARTESIAN_POINT('Ctrl Pts',(2.69042886699994,5.2,2.95726168599998));
#339835=CARTESIAN_POINT('Ctrl Pts',(2.69042886699994,2.2,2.95726168599998));
#339836=CARTESIAN_POINT('Ctrl Pts',(2.69025707999994,12.2,2.95708934699999));
#339837=CARTESIAN_POINT('Ctrl Pts',(2.69025707999994,5.2,2.95708934699999));
#339838=CARTESIAN_POINT('Ctrl Pts',(2.69025707999994,2.2,2.95708934699999));
#339839=CARTESIAN_POINT('Ctrl Pts',(2.69009041599995,12.2,2.95692170099999));
#339840=CARTESIAN_POINT('Ctrl Pts',(2.69009041599995,5.2,2.95692170099999));
#339841=CARTESIAN_POINT('Ctrl Pts',(2.69009041599995,2.2,2.95692170099999));
#339842=CARTESIAN_POINT('Ctrl Pts',(2.68992887199994,12.2,2.95675877199999));
#339843=CARTESIAN_POINT('Ctrl Pts',(2.68992887199994,5.2,2.95675877199999));
#339844=CARTESIAN_POINT('Ctrl Pts',(2.68992887199994,2.2,2.95675877199999));
#339845=CARTESIAN_POINT('Ctrl Pts',(2.68977244999994,12.2,2.95660058499998));
#339846=CARTESIAN_POINT('Ctrl Pts',(2.68977244999994,5.2,2.95660058499998));
#339847=CARTESIAN_POINT('Ctrl Pts',(2.68977244999994,2.2,2.95660058499998));
#339848=CARTESIAN_POINT('Ctrl Pts',(2.68962114499995,12.2,2.95644716099999));
#339849=CARTESIAN_POINT('Ctrl Pts',(2.68962114499995,5.2,2.95644716099999));
#339850=CARTESIAN_POINT('Ctrl Pts',(2.68962114499995,2.2,2.95644716099999));
#339851=CARTESIAN_POINT('Ctrl Pts',(2.68947495599994,12.2,2.95629852799999));
#339852=CARTESIAN_POINT('Ctrl Pts',(2.68947495599994,5.2,2.95629852799999));
#339853=CARTESIAN_POINT('Ctrl Pts',(2.68947495599994,2.2,2.95629852799999));
#339854=CARTESIAN_POINT('Ctrl Pts',(2.68933387899994,12.2,2.95615470799999));
#339855=CARTESIAN_POINT('Ctrl Pts',(2.68933387899994,5.2,2.95615470799999));
#339856=CARTESIAN_POINT('Ctrl Pts',(2.68933387899994,2.2,2.95615470799999));
#339857=CARTESIAN_POINT('Ctrl Pts',(2.68919791499994,12.2,2.95601572699999));
#339858=CARTESIAN_POINT('Ctrl Pts',(2.68919791499994,5.2,2.95601572699999));
#339859=CARTESIAN_POINT('Ctrl Pts',(2.68919791499994,2.2,2.95601572699999));
#339860=CARTESIAN_POINT('Ctrl Pts',(2.68906705899994,12.2,2.95588160999999));
#339861=CARTESIAN_POINT('Ctrl Pts',(2.68906705899994,5.2,2.95588160999999));
#339862=CARTESIAN_POINT('Ctrl Pts',(2.68906705899994,2.2,2.95588160999999));
#339863=CARTESIAN_POINT('Ctrl Pts',(2.68894130999994,12.2,2.95575237899998));
#339864=CARTESIAN_POINT('Ctrl Pts',(2.68894130999994,5.2,2.95575237899998));
#339865=CARTESIAN_POINT('Ctrl Pts',(2.68894130999994,2.2,2.95575237899998));
#339866=CARTESIAN_POINT('Ctrl Pts',(2.68882066599994,12.2,2.95562805999998));
#339867=CARTESIAN_POINT('Ctrl Pts',(2.68882066599994,5.2,2.95562805999998));
#339868=CARTESIAN_POINT('Ctrl Pts',(2.68882066599994,2.2,2.95562805999998));
#339869=CARTESIAN_POINT('Ctrl Pts',(2.68870512299995,12.2,2.95550867699998));
#339870=CARTESIAN_POINT('Ctrl Pts',(2.68870512299995,5.2,2.95550867699998));
#339871=CARTESIAN_POINT('Ctrl Pts',(2.68870512299995,2.2,2.95550867699998));
#339872=CARTESIAN_POINT('Ctrl Pts',(2.68859468199994,12.2,2.95539425399999));
#339873=CARTESIAN_POINT('Ctrl Pts',(2.68859468199994,5.2,2.95539425399999));
#339874=CARTESIAN_POINT('Ctrl Pts',(2.68859468199994,2.2,2.95539425399999));
#339875=CARTESIAN_POINT('Ctrl Pts',(2.68848933799994,12.2,2.95528481599998));
#339876=CARTESIAN_POINT('Ctrl Pts',(2.68848933799994,5.2,2.95528481599998));
#339877=CARTESIAN_POINT('Ctrl Pts',(2.68848933799994,2.2,2.95528481599998));
#339878=CARTESIAN_POINT('Ctrl Pts',(2.68838908999995,12.2,2.95518039199998));
#339879=CARTESIAN_POINT('Ctrl Pts',(2.68838908999995,5.2,2.95518039199998));
#339880=CARTESIAN_POINT('Ctrl Pts',(2.68838908999995,2.2,2.95518039199998));
#339881=CARTESIAN_POINT('Ctrl Pts',(2.68829393399994,12.2,2.95508100599999));
#339882=CARTESIAN_POINT('Ctrl Pts',(2.68829393399994,5.2,2.95508100599999));
#339883=CARTESIAN_POINT('Ctrl Pts',(2.68829393399994,2.2,2.95508100599999));
#339884=CARTESIAN_POINT('Ctrl Pts',(2.68820386799994,12.2,2.95498668399999));
#339885=CARTESIAN_POINT('Ctrl Pts',(2.68820386799994,5.2,2.95498668399999));
#339886=CARTESIAN_POINT('Ctrl Pts',(2.68820386799994,2.2,2.95498668399999));
#339887=CARTESIAN_POINT('Ctrl Pts',(2.68811888899994,12.2,2.95489745099999));
#339888=CARTESIAN_POINT('Ctrl Pts',(2.68811888899994,5.2,2.95489745099999));
#339889=CARTESIAN_POINT('Ctrl Pts',(2.68811888899994,2.2,2.95489745099999));
#339890=CARTESIAN_POINT('Ctrl Pts',(2.68803899599994,12.2,2.95481332999999));
#339891=CARTESIAN_POINT('Ctrl Pts',(2.68803899599994,5.2,2.95481332999999));
#339892=CARTESIAN_POINT('Ctrl Pts',(2.68803899599994,2.2,2.95481332999999));
#339893=CARTESIAN_POINT('Ctrl Pts',(2.68796418699994,12.2,2.95473434299999));
#339894=CARTESIAN_POINT('Ctrl Pts',(2.68796418699994,5.2,2.95473434299999));
#339895=CARTESIAN_POINT('Ctrl Pts',(2.68796418699994,2.2,2.95473434299999));
#339896=CARTESIAN_POINT('Ctrl Pts',(2.68789445799994,12.2,2.95466051499999));
#339897=CARTESIAN_POINT('Ctrl Pts',(2.68789445799994,5.2,2.95466051499999));
#339898=CARTESIAN_POINT('Ctrl Pts',(2.68789445799994,2.2,2.95466051499999));
#339899=CARTESIAN_POINT('Ctrl Pts',(2.68782980799994,12.2,2.95459186999998));
#339900=CARTESIAN_POINT('Ctrl Pts',(2.68782980799994,5.2,2.95459186999998));
#339901=CARTESIAN_POINT('Ctrl Pts',(2.68782980799994,2.2,2.95459186999998));
#339902=CARTESIAN_POINT('Ctrl Pts',(2.68777023099994,12.2,2.95452843899999));
#339903=CARTESIAN_POINT('Ctrl Pts',(2.68777023099994,5.2,2.95452843899999));
#339904=CARTESIAN_POINT('Ctrl Pts',(2.68777023099994,2.2,2.95452843899999));
#339905=CARTESIAN_POINT('Ctrl Pts',(2.68771572699994,12.2,2.95447025399999));
#339906=CARTESIAN_POINT('Ctrl Pts',(2.68771572699994,5.2,2.95447025399999));
#339907=CARTESIAN_POINT('Ctrl Pts',(2.68771572699994,2.2,2.95447025399999));
#339908=CARTESIAN_POINT('Ctrl Pts',(2.68766629099995,12.2,2.95441734799999));
#339909=CARTESIAN_POINT('Ctrl Pts',(2.68766629099995,5.2,2.95441734799999));
#339910=CARTESIAN_POINT('Ctrl Pts',(2.68766629099995,2.2,2.95441734799999));
#339911=CARTESIAN_POINT('Ctrl Pts',(2.68762191999994,12.2,2.95436974999999));
#339912=CARTESIAN_POINT('Ctrl Pts',(2.68762191999994,5.2,2.95436974999999));
#339913=CARTESIAN_POINT('Ctrl Pts',(2.68762191999994,2.2,2.95436974999999));
#339914=CARTESIAN_POINT('Ctrl Pts',(2.68758261099994,12.2,2.95432747899999));
#339915=CARTESIAN_POINT('Ctrl Pts',(2.68758261099994,5.2,2.95432747899999));
#339916=CARTESIAN_POINT('Ctrl Pts',(2.68758261099994,2.2,2.95432747899999));
#339917=CARTESIAN_POINT('Ctrl Pts',(2.68754469767605,12.2,2.95428659655369));
#339918=CARTESIAN_POINT('Ctrl Pts',(2.68754469767605,5.2,2.95428659655369));
#339919=CARTESIAN_POINT('Ctrl Pts',(2.68754469767605,2.2,2.95428659655369));
#339920=CARTESIAN_POINT('Ctrl Pts',(2.68751883712808,12.2,2.9542585984447));
#339921=CARTESIAN_POINT('Ctrl Pts',(2.68751883712808,5.2,2.9542585984447));
#339922=CARTESIAN_POINT('Ctrl Pts',(2.68751883712808,2.2,2.9542585984447));
#339923=CARTESIAN_POINT('Ctrl Pts',(2.68750184158111,12.2,2.95424011739526));
#339924=CARTESIAN_POINT('Ctrl Pts',(2.68750184158111,5.2,2.95424011739526));
#339925=CARTESIAN_POINT('Ctrl Pts',(2.68750184158111,2.2,2.95424011739526));
#339926=CARTESIAN_POINT('Ctrl Pts',(2.68749128112236,12.2,2.95422858071313));
#339927=CARTESIAN_POINT('Ctrl Pts',(2.68749128112236,5.2,2.95422858071313));
#339928=CARTESIAN_POINT('Ctrl Pts',(2.68749128112236,2.2,2.95422858071313));
#339929=CARTESIAN_POINT('Ctrl Pts',(2.68748475499994,12.2,2.95422146199999));
#339930=CARTESIAN_POINT('Ctrl Pts',(2.68748475499994,5.2,2.95422146199999));
#339931=CARTESIAN_POINT('Ctrl Pts',(2.68748475499994,2.2,2.95422146199999));
#339932=CARTESIAN_POINT('',(3.44029922199995,12.2,3.27518568399999));
#339933=CARTESIAN_POINT('Origin',(-5.66300478732629E-14,15.2,-1.77635683940025E-14));
#339934=CARTESIAN_POINT('',(3.66384038699994,12.2,3.02304045899999));
#339935=CARTESIAN_POINT('Ctrl Pts',(3.25496447599994,12.2,2.31410207099998));
#339936=CARTESIAN_POINT('Ctrl Pts',(3.25496447599994,5.2,2.31410207099998));
#339937=CARTESIAN_POINT('Ctrl Pts',(3.25496447599994,2.2,2.31410207099998));
#339938=CARTESIAN_POINT('Ctrl Pts',(3.25497003667146,12.2,2.31410605776463));
#339939=CARTESIAN_POINT('Ctrl Pts',(3.25497003667146,5.2,2.31410605776463));
#339940=CARTESIAN_POINT('Ctrl Pts',(3.25497003667146,2.2,2.31410605776463));
#339941=CARTESIAN_POINT('Ctrl Pts',(3.25498079470201,12.2,2.31411376555869));
#339942=CARTESIAN_POINT('Ctrl Pts',(3.25498079470201,5.2,2.31411376555869));
#339943=CARTESIAN_POINT('Ctrl Pts',(3.25498079470201,2.2,2.31411376555869));
#339944=CARTESIAN_POINT('Ctrl Pts',(3.25499674313561,12.2,2.31412520718679));
#339945=CARTESIAN_POINT('Ctrl Pts',(3.25499674313561,5.19999999999999,2.31412520718679));
#339946=CARTESIAN_POINT('Ctrl Pts',(3.25499674313561,2.2,2.31412520718679));
#339947=CARTESIAN_POINT('Ctrl Pts',(3.25501789589991,12.2,2.31414031259025));
#339948=CARTESIAN_POINT('Ctrl Pts',(3.25501789589991,5.19999999999999,2.31414031259025));
#339949=CARTESIAN_POINT('Ctrl Pts',(3.25501789589991,2.2,2.31414031259025));
#339950=CARTESIAN_POINT('Ctrl Pts',(3.25505458999995,12.2,2.31416690699998));
#339951=CARTESIAN_POINT('Ctrl Pts',(3.25505458999995,5.2,2.31416690699998));
#339952=CARTESIAN_POINT('Ctrl Pts',(3.25505458999995,2.2,2.31416690699998));
#339953=CARTESIAN_POINT('Ctrl Pts',(3.25509535799994,12.2,2.31419648199998));
#339954=CARTESIAN_POINT('Ctrl Pts',(3.25509535799994,5.2,2.31419648199998));
#339955=CARTESIAN_POINT('Ctrl Pts',(3.25509535799994,2.2,2.31419648199998));
#339956=CARTESIAN_POINT('Ctrl Pts',(3.25514203299994,12.2,2.31423044199999));
#339957=CARTESIAN_POINT('Ctrl Pts',(3.25514203299994,5.2,2.31423044199999));
#339958=CARTESIAN_POINT('Ctrl Pts',(3.25514203299994,2.2,2.31423044199999));
#339959=CARTESIAN_POINT('Ctrl Pts',(3.25519460599994,12.2,2.31426878999998));
#339960=CARTESIAN_POINT('Ctrl Pts',(3.25519460599994,5.2,2.31426878999998));
#339961=CARTESIAN_POINT('Ctrl Pts',(3.25519460599994,2.2,2.31426878999998));
#339962=CARTESIAN_POINT('Ctrl Pts',(3.25525305499994,12.2,2.31431152999999));
#339963=CARTESIAN_POINT('Ctrl Pts',(3.25525305499994,5.2,2.31431152999999));
#339964=CARTESIAN_POINT('Ctrl Pts',(3.25525305499994,2.2,2.31431152999999));
#339965=CARTESIAN_POINT('Ctrl Pts',(3.25531735199994,12.2,2.31435866999998));
#339966=CARTESIAN_POINT('Ctrl Pts',(3.25531735199994,5.2,2.31435866999998));
#339967=CARTESIAN_POINT('Ctrl Pts',(3.25531735199994,2.2,2.31435866999998));
#339968=CARTESIAN_POINT('Ctrl Pts',(3.25538746499995,12.2,2.31441021399998));
#339969=CARTESIAN_POINT('Ctrl Pts',(3.25538746499995,5.2,2.31441021399998));
#339970=CARTESIAN_POINT('Ctrl Pts',(3.25538746499995,2.2,2.31441021399998));
#339971=CARTESIAN_POINT('Ctrl Pts',(3.25546336299994,12.2,2.31446617399999));
#339972=CARTESIAN_POINT('Ctrl Pts',(3.25546336299994,5.2,2.31446617399999));
#339973=CARTESIAN_POINT('Ctrl Pts',(3.25546336299994,2.2,2.31446617399999));
#339974=CARTESIAN_POINT('Ctrl Pts',(3.25554501499994,12.2,2.31452655399998));
#339975=CARTESIAN_POINT('Ctrl Pts',(3.25554501499994,5.2,2.31452655399998));
#339976=CARTESIAN_POINT('Ctrl Pts',(3.25554501499994,2.2,2.31452655399998));
#339977=CARTESIAN_POINT('Ctrl Pts',(3.25563239699994,12.2,2.31459135899998));
#339978=CARTESIAN_POINT('Ctrl Pts',(3.25563239699994,5.2,2.31459135899998));
#339979=CARTESIAN_POINT('Ctrl Pts',(3.25563239699994,2.2,2.31459135899998));
#339980=CARTESIAN_POINT('Ctrl Pts',(3.25572548599995,12.2,2.31466059599999));
#339981=CARTESIAN_POINT('Ctrl Pts',(3.25572548599995,5.2,2.31466059599999));
#339982=CARTESIAN_POINT('Ctrl Pts',(3.25572548599995,2.2,2.31466059599999));
#339983=CARTESIAN_POINT('Ctrl Pts',(3.25582425799994,12.2,2.31473426899999));
#339984=CARTESIAN_POINT('Ctrl Pts',(3.25582425799994,5.2,2.31473426899999));
#339985=CARTESIAN_POINT('Ctrl Pts',(3.25582425799994,2.2,2.31473426899999));
#339986=CARTESIAN_POINT('Ctrl Pts',(3.25592869299994,12.2,2.31481238299999));
#339987=CARTESIAN_POINT('Ctrl Pts',(3.25592869299994,5.2,2.31481238299999));
#339988=CARTESIAN_POINT('Ctrl Pts',(3.25592869299994,2.2,2.31481238299999));
#339989=CARTESIAN_POINT('Ctrl Pts',(3.25603876599994,12.2,2.31489494399999));
#339990=CARTESIAN_POINT('Ctrl Pts',(3.25603876599994,5.2,2.31489494399999));
#339991=CARTESIAN_POINT('Ctrl Pts',(3.25603876599994,2.2,2.31489494399999));
#339992=CARTESIAN_POINT('Ctrl Pts',(3.25615445099994,12.2,2.31498195699999));
#339993=CARTESIAN_POINT('Ctrl Pts',(3.25615445099994,5.2,2.31498195699999));
#339994=CARTESIAN_POINT('Ctrl Pts',(3.25615445099994,2.2,2.31498195699999));
#339995=CARTESIAN_POINT('Ctrl Pts',(3.25627572299994,12.2,2.31507342799999));
#339996=CARTESIAN_POINT('Ctrl Pts',(3.25627572299994,5.2,2.31507342799999));
#339997=CARTESIAN_POINT('Ctrl Pts',(3.25627572299994,2.2,2.31507342799999));
#339998=CARTESIAN_POINT('Ctrl Pts',(3.25640255599994,12.2,2.31516936199998));
#339999=CARTESIAN_POINT('Ctrl Pts',(3.25640255599994,5.2,2.31516936199998));
#340000=CARTESIAN_POINT('Ctrl Pts',(3.25640255599994,2.2,2.31516936199998));
#340001=CARTESIAN_POINT('Ctrl Pts',(3.25653492399995,12.2,2.31526976599998));
#340002=CARTESIAN_POINT('Ctrl Pts',(3.25653492399995,5.2,2.31526976599998));
#340003=CARTESIAN_POINT('Ctrl Pts',(3.25653492399995,2.2,2.31526976599998));
#340004=CARTESIAN_POINT('Ctrl Pts',(3.25667280399994,12.2,2.31537464299999));
#340005=CARTESIAN_POINT('Ctrl Pts',(3.25667280399994,5.2,2.31537464299999));
#340006=CARTESIAN_POINT('Ctrl Pts',(3.25667280399994,2.2,2.31537464299999));
#340007=CARTESIAN_POINT('Ctrl Pts',(3.25681617199994,12.2,2.31548399999999));
#340008=CARTESIAN_POINT('Ctrl Pts',(3.25681617199994,5.2,2.31548399999999));
#340009=CARTESIAN_POINT('Ctrl Pts',(3.25681617199994,2.2,2.31548399999999));
#340010=CARTESIAN_POINT('Ctrl Pts',(3.25696500399994,12.2,2.31559784099999));
#340011=CARTESIAN_POINT('Ctrl Pts',(3.25696500399994,5.2,2.31559784099999));
#340012=CARTESIAN_POINT('Ctrl Pts',(3.25696500399994,2.2,2.31559784099999));
#340013=CARTESIAN_POINT('Ctrl Pts',(3.25711927599994,12.2,2.31571617199998));
#340014=CARTESIAN_POINT('Ctrl Pts',(3.25711927599994,5.2,2.31571617199998));
#340015=CARTESIAN_POINT('Ctrl Pts',(3.25711927599994,2.2,2.31571617199998));
#340016=CARTESIAN_POINT('Ctrl Pts',(3.25727896499994,12.2,2.31583899699999));
#340017=CARTESIAN_POINT('Ctrl Pts',(3.25727896499994,5.2,2.31583899699999));
#340018=CARTESIAN_POINT('Ctrl Pts',(3.25727896499994,2.2,2.31583899699999));
#340019=CARTESIAN_POINT('Ctrl Pts',(3.25744404599994,12.2,2.31596632299999));
#340020=CARTESIAN_POINT('Ctrl Pts',(3.25744404599994,5.2,2.31596632299999));
#340021=CARTESIAN_POINT('Ctrl Pts',(3.25744404599994,2.2,2.31596632299999));
#340022=CARTESIAN_POINT('Ctrl Pts',(3.25761449399995,12.2,2.31609815299999));
#340023=CARTESIAN_POINT('Ctrl Pts',(3.25761449399995,5.2,2.31609815299999));
#340024=CARTESIAN_POINT('Ctrl Pts',(3.25761449399995,2.2,2.31609815299999));
#340025=CARTESIAN_POINT('Ctrl Pts',(3.25779028699994,12.2,2.31623449299999));
#340026=CARTESIAN_POINT('Ctrl Pts',(3.25779028699994,5.2,2.31623449299999));
#340027=CARTESIAN_POINT('Ctrl Pts',(3.25779028699994,2.2,2.31623449299999));
#340028=CARTESIAN_POINT('Ctrl Pts',(3.25797139899994,12.2,2.31637534699999));
#340029=CARTESIAN_POINT('Ctrl Pts',(3.25797139899994,5.2,2.31637534699999));
#340030=CARTESIAN_POINT('Ctrl Pts',(3.25797139899994,2.2,2.31637534699999));
#340031=CARTESIAN_POINT('Ctrl Pts',(3.25815780899994,12.2,2.31652072099998));
#340032=CARTESIAN_POINT('Ctrl Pts',(3.25815780899994,5.2,2.31652072099998));
#340033=CARTESIAN_POINT('Ctrl Pts',(3.25815780899994,2.2,2.31652072099998));
#340034=CARTESIAN_POINT('Ctrl Pts',(3.25834949099994,12.2,2.31667061999998));
#340035=CARTESIAN_POINT('Ctrl Pts',(3.25834949099994,5.2,2.31667061999998));
#340036=CARTESIAN_POINT('Ctrl Pts',(3.25834949099994,2.2,2.31667061999998));
#340037=CARTESIAN_POINT('Ctrl Pts',(3.25854642299995,12.2,2.31682504699998));
#340038=CARTESIAN_POINT('Ctrl Pts',(3.25854642299995,5.2,2.31682504699998));
#340039=CARTESIAN_POINT('Ctrl Pts',(3.25854642299995,2.2,2.31682504699998));
#340040=CARTESIAN_POINT('Ctrl Pts',(3.25874858199994,12.2,2.31698400899999));
#340041=CARTESIAN_POINT('Ctrl Pts',(3.25874858199994,5.2,2.31698400899999));
#340042=CARTESIAN_POINT('Ctrl Pts',(3.25874858199994,2.2,2.31698400899999));
#340043=CARTESIAN_POINT('Ctrl Pts',(3.25895594299995,12.2,2.31714750899998));
#340044=CARTESIAN_POINT('Ctrl Pts',(3.25895594299995,5.2,2.31714750899998));
#340045=CARTESIAN_POINT('Ctrl Pts',(3.25895594299995,2.2,2.31714750899998));
#340046=CARTESIAN_POINT('Ctrl Pts',(3.25916848299994,12.2,2.31731555299998));
#340047=CARTESIAN_POINT('Ctrl Pts',(3.25916848299994,5.2,2.31731555299998));
#340048=CARTESIAN_POINT('Ctrl Pts',(3.25916848299994,2.2,2.31731555299998));
#340049=CARTESIAN_POINT('Ctrl Pts',(3.25938617999994,12.2,2.31748814399999));
#340050=CARTESIAN_POINT('Ctrl Pts',(3.25938617999994,5.2,2.31748814399999));
#340051=CARTESIAN_POINT('Ctrl Pts',(3.25938617999994,2.2,2.31748814399999));
#340052=CARTESIAN_POINT('Ctrl Pts',(3.25960900999994,12.2,2.31766528799998));
#340053=CARTESIAN_POINT('Ctrl Pts',(3.25960900999994,5.2,2.31766528799998));
#340054=CARTESIAN_POINT('Ctrl Pts',(3.25960900999994,2.2,2.31766528799998));
#340055=CARTESIAN_POINT('Ctrl Pts',(3.25983694999994,12.2,2.31784698899999));
#340056=CARTESIAN_POINT('Ctrl Pts',(3.25983694999994,5.2,2.31784698899999));
#340057=CARTESIAN_POINT('Ctrl Pts',(3.25983694999994,2.2,2.31784698899999));
#340058=CARTESIAN_POINT('Ctrl Pts',(3.26006997599994,12.2,2.31803325099999));
#340059=CARTESIAN_POINT('Ctrl Pts',(3.26006997599994,5.2,2.31803325099999));
#340060=CARTESIAN_POINT('Ctrl Pts',(3.26006997599994,2.2,2.31803325099999));
#340061=CARTESIAN_POINT('Ctrl Pts',(3.26030806799994,12.2,2.31822407999998));
#340062=CARTESIAN_POINT('Ctrl Pts',(3.26030806799994,5.2,2.31822407999998));
#340063=CARTESIAN_POINT('Ctrl Pts',(3.26030806799994,2.2,2.31822407999998));
#340064=CARTESIAN_POINT('Ctrl Pts',(3.26055119999995,12.2,2.31841947899999));
#340065=CARTESIAN_POINT('Ctrl Pts',(3.26055119999995,5.2,2.31841947899999));
#340066=CARTESIAN_POINT('Ctrl Pts',(3.26055119999995,2.2,2.31841947899999));
#340067=CARTESIAN_POINT('Ctrl Pts',(3.26079935099994,12.2,2.31861945399999));
#340068=CARTESIAN_POINT('Ctrl Pts',(3.26079935099994,5.2,2.31861945399999));
#340069=CARTESIAN_POINT('Ctrl Pts',(3.26079935099994,2.2,2.31861945399999));
#340070=CARTESIAN_POINT('Ctrl Pts',(3.26105249699994,12.2,2.31882400699998));
#340071=CARTESIAN_POINT('Ctrl Pts',(3.26105249699994,5.2,2.31882400699998));
#340072=CARTESIAN_POINT('Ctrl Pts',(3.26105249699994,2.2,2.31882400699998));
#340073=CARTESIAN_POINT('Ctrl Pts',(3.26131061799994,12.2,2.31903314399998));
#340074=CARTESIAN_POINT('Ctrl Pts',(3.26131061799994,5.2,2.31903314399998));
#340075=CARTESIAN_POINT('Ctrl Pts',(3.26131061799994,2.2,2.31903314399998));
#340076=CARTESIAN_POINT('Ctrl Pts',(3.26157368799994,12.2,2.31924686699998));
#340077=CARTESIAN_POINT('Ctrl Pts',(3.26157368799994,5.2,2.31924686699998));
#340078=CARTESIAN_POINT('Ctrl Pts',(3.26157368799994,2.2,2.31924686699998));
#340079=CARTESIAN_POINT('Ctrl Pts',(3.26184168799994,12.2,2.31946518399999));
#340080=CARTESIAN_POINT('Ctrl Pts',(3.26184168799994,5.2,2.31946518399999));
#340081=CARTESIAN_POINT('Ctrl Pts',(3.26184168799994,2.2,2.31946518399999));
#340082=CARTESIAN_POINT('Ctrl Pts',(3.26211459199994,12.2,2.31968809699998));
#340083=CARTESIAN_POINT('Ctrl Pts',(3.26211459199994,5.2,2.31968809699998));
#340084=CARTESIAN_POINT('Ctrl Pts',(3.26211459199994,2.2,2.31968809699998));
#340085=CARTESIAN_POINT('Ctrl Pts',(3.26239237999994,12.2,2.31991560899999));
#340086=CARTESIAN_POINT('Ctrl Pts',(3.26239237999994,5.2,2.31991560899999));
#340087=CARTESIAN_POINT('Ctrl Pts',(3.26239237999994,2.2,2.31991560899999));
#340088=CARTESIAN_POINT('Ctrl Pts',(3.26267502899994,12.2,2.32014772599999));
#340089=CARTESIAN_POINT('Ctrl Pts',(3.26267502899994,5.2,2.32014772599999));
#340090=CARTESIAN_POINT('Ctrl Pts',(3.26267502899994,2.2,2.32014772599999));
#340091=CARTESIAN_POINT('Ctrl Pts',(3.26296251699994,12.2,2.32038445199999));
#340092=CARTESIAN_POINT('Ctrl Pts',(3.26296251699994,5.2,2.32038445199999));
#340093=CARTESIAN_POINT('Ctrl Pts',(3.26296251699994,2.2,2.32038445199999));
#340094=CARTESIAN_POINT('Ctrl Pts',(3.26325482199994,12.2,2.32062579099999));
#340095=CARTESIAN_POINT('Ctrl Pts',(3.26325482199994,5.2,2.32062579099999));
#340096=CARTESIAN_POINT('Ctrl Pts',(3.26325482199994,2.2,2.32062579099999));
#340097=CARTESIAN_POINT('Ctrl Pts',(3.26355192099994,12.2,2.32087174499998));
#340098=CARTESIAN_POINT('Ctrl Pts',(3.26355192099994,5.2,2.32087174499998));
#340099=CARTESIAN_POINT('Ctrl Pts',(3.26355192099994,2.2,2.32087174499998));
#340100=CARTESIAN_POINT('Ctrl Pts',(3.26385379399994,12.2,2.32112232099999));
#340101=CARTESIAN_POINT('Ctrl Pts',(3.26385379399994,5.2,2.32112232099999));
#340102=CARTESIAN_POINT('Ctrl Pts',(3.26385379399994,2.2,2.32112232099999));
#340103=CARTESIAN_POINT('Ctrl Pts',(3.26416041699995,12.2,2.32137751999999));
#340104=CARTESIAN_POINT('Ctrl Pts',(3.26416041699995,5.2,2.32137751999999));
#340105=CARTESIAN_POINT('Ctrl Pts',(3.26416041699995,2.2,2.32137751999999));
#340106=CARTESIAN_POINT('Ctrl Pts',(3.26447176799994,12.2,2.32163734799999));
#340107=CARTESIAN_POINT('Ctrl Pts',(3.26447176799994,5.2,2.32163734799999));
#340108=CARTESIAN_POINT('Ctrl Pts',(3.26447176799994,2.2,2.32163734799999));
#340109=CARTESIAN_POINT('Ctrl Pts',(3.26478782799994,12.2,2.32190180699998));
#340110=CARTESIAN_POINT('Ctrl Pts',(3.26478782799994,5.2,2.32190180699998));
#340111=CARTESIAN_POINT('Ctrl Pts',(3.26478782799994,2.2,2.32190180699998));
#340112=CARTESIAN_POINT('Ctrl Pts',(3.26510857199994,12.2,2.32217090299998));
#340113=CARTESIAN_POINT('Ctrl Pts',(3.26510857199994,5.2,2.32217090299998));
#340114=CARTESIAN_POINT('Ctrl Pts',(3.26510857199994,2.2,2.32217090299998));
#340115=CARTESIAN_POINT('Ctrl Pts',(3.26543397999994,12.2,2.32244463899999));
#340116=CARTESIAN_POINT('Ctrl Pts',(3.26543397999994,5.2,2.32244463899999));
#340117=CARTESIAN_POINT('Ctrl Pts',(3.26543397999994,2.2,2.32244463899999));
#340118=CARTESIAN_POINT('Ctrl Pts',(3.26576402999994,12.2,2.32272301699998));
#340119=CARTESIAN_POINT('Ctrl Pts',(3.26576402999994,5.2,2.32272301699998));
#340120=CARTESIAN_POINT('Ctrl Pts',(3.26576402999994,2.2,2.32272301699998));
#340121=CARTESIAN_POINT('Ctrl Pts',(3.26609869999994,12.2,2.32300604199999));
#340122=CARTESIAN_POINT('Ctrl Pts',(3.26609869999994,5.2,2.32300604199999));
#340123=CARTESIAN_POINT('Ctrl Pts',(3.26609869999994,2.2,2.32300604199999));
#340124=CARTESIAN_POINT('Ctrl Pts',(3.26643796999994,12.2,2.32329371799999));
#340125=CARTESIAN_POINT('Ctrl Pts',(3.26643796999994,5.2,2.32329371799999));
#340126=CARTESIAN_POINT('Ctrl Pts',(3.26643796999994,2.2,2.32329371799999));
#340127=CARTESIAN_POINT('Ctrl Pts',(3.26678181699994,12.2,2.32358604899999));
#340128=CARTESIAN_POINT('Ctrl Pts',(3.26678181699994,5.2,2.32358604899999));
#340129=CARTESIAN_POINT('Ctrl Pts',(3.26678181699994,2.2,2.32358604899999));
#340130=CARTESIAN_POINT('Ctrl Pts',(3.26713022099994,12.2,2.32388303699999));
#340131=CARTESIAN_POINT('Ctrl Pts',(3.26713022099994,5.2,2.32388303699999));
#340132=CARTESIAN_POINT('Ctrl Pts',(3.26713022099994,2.2,2.32388303699999));
#340133=CARTESIAN_POINT('Ctrl Pts',(3.26748315999994,12.2,2.32418468699999));
#340134=CARTESIAN_POINT('Ctrl Pts',(3.26748315999994,5.2,2.32418468699999));
#340135=CARTESIAN_POINT('Ctrl Pts',(3.26748315999994,2.2,2.32418468699999));
#340136=CARTESIAN_POINT('Ctrl Pts',(3.26784061199994,12.2,2.32449100199998));
#340137=CARTESIAN_POINT('Ctrl Pts',(3.26784061199994,5.2,2.32449100199998));
#340138=CARTESIAN_POINT('Ctrl Pts',(3.26784061199994,2.2,2.32449100199998));
#340139=CARTESIAN_POINT('Ctrl Pts',(3.26820255799994,12.2,2.32480198599998));
#340140=CARTESIAN_POINT('Ctrl Pts',(3.26820255799994,5.2,2.32480198599998));
#340141=CARTESIAN_POINT('Ctrl Pts',(3.26820255799994,2.2,2.32480198599998));
#340142=CARTESIAN_POINT('Ctrl Pts',(3.26856897399994,12.2,2.32511764099999));
#340143=CARTESIAN_POINT('Ctrl Pts',(3.26856897399994,5.2,2.32511764099999));
#340144=CARTESIAN_POINT('Ctrl Pts',(3.26856897399994,2.2,2.32511764099999));
#340145=CARTESIAN_POINT('Ctrl Pts',(3.26893984099994,12.2,2.32543797099999));
#340146=CARTESIAN_POINT('Ctrl Pts',(3.26893984099994,5.2,2.32543797099999));
#340147=CARTESIAN_POINT('Ctrl Pts',(3.26893984099994,2.2,2.32543797099999));
#340148=CARTESIAN_POINT('Ctrl Pts',(3.26931513799994,12.2,2.32576297999998));
#340149=CARTESIAN_POINT('Ctrl Pts',(3.26931513799994,5.2,2.32576297999998));
#340150=CARTESIAN_POINT('Ctrl Pts',(3.26931513799994,2.2,2.32576297999998));
#340151=CARTESIAN_POINT('Ctrl Pts',(3.26969484299994,12.2,2.32609266999999));
#340152=CARTESIAN_POINT('Ctrl Pts',(3.26969484299994,5.2,2.32609266999999));
#340153=CARTESIAN_POINT('Ctrl Pts',(3.26969484299994,2.2,2.32609266999999));
#340154=CARTESIAN_POINT('Ctrl Pts',(3.27007893599994,12.2,2.32642704699999));
#340155=CARTESIAN_POINT('Ctrl Pts',(3.27007893599994,5.2,2.32642704699999));
#340156=CARTESIAN_POINT('Ctrl Pts',(3.27007893599994,2.2,2.32642704699999));
#340157=CARTESIAN_POINT('Ctrl Pts',(3.27046739699994,12.2,2.32676611099999));
#340158=CARTESIAN_POINT('Ctrl Pts',(3.27046739699994,5.2,2.32676611099999));
#340159=CARTESIAN_POINT('Ctrl Pts',(3.27046739699994,2.2,2.32676611099999));
#340160=CARTESIAN_POINT('Ctrl Pts',(3.27086020299994,12.2,2.32710986699999));
#340161=CARTESIAN_POINT('Ctrl Pts',(3.27086020299994,5.2,2.32710986699999));
#340162=CARTESIAN_POINT('Ctrl Pts',(3.27086020299994,2.2,2.32710986699999));
#340163=CARTESIAN_POINT('Ctrl Pts',(3.27125733499994,12.2,2.32745831799999));
#340164=CARTESIAN_POINT('Ctrl Pts',(3.27125733499994,5.2,2.32745831799999));
#340165=CARTESIAN_POINT('Ctrl Pts',(3.27125733499994,2.2,2.32745831799999));
#340166=CARTESIAN_POINT('Ctrl Pts',(3.27165877199994,12.2,2.32781146799999));
#340167=CARTESIAN_POINT('Ctrl Pts',(3.27165877199994,5.2,2.32781146799999));
#340168=CARTESIAN_POINT('Ctrl Pts',(3.27165877199994,2.2,2.32781146799999));
#340169=CARTESIAN_POINT('Ctrl Pts',(3.27206449399994,12.2,2.32816931799999));
#340170=CARTESIAN_POINT('Ctrl Pts',(3.27206449399994,5.2,2.32816931799999));
#340171=CARTESIAN_POINT('Ctrl Pts',(3.27206449399994,2.2,2.32816931799999));
#340172=CARTESIAN_POINT('Ctrl Pts',(3.27247447999994,12.2,2.32853187299999));
#340173=CARTESIAN_POINT('Ctrl Pts',(3.27247447999994,5.2,2.32853187299999));
#340174=CARTESIAN_POINT('Ctrl Pts',(3.27247447999994,2.2,2.32853187299999));
#340175=CARTESIAN_POINT('Ctrl Pts',(3.27288870899994,12.2,2.32889913399998));
#340176=CARTESIAN_POINT('Ctrl Pts',(3.27288870899994,5.2,2.32889913399998));
#340177=CARTESIAN_POINT('Ctrl Pts',(3.27288870899994,2.2,2.32889913399998));
#340178=CARTESIAN_POINT('Ctrl Pts',(3.27330716099994,12.2,2.32927110699999));
#340179=CARTESIAN_POINT('Ctrl Pts',(3.27330716099994,5.2,2.32927110699999));
#340180=CARTESIAN_POINT('Ctrl Pts',(3.27330716099994,2.2,2.32927110699999));
#340181=CARTESIAN_POINT('Ctrl Pts',(3.27372981699994,12.2,2.32964779199999));
#340182=CARTESIAN_POINT('Ctrl Pts',(3.27372981699994,5.2,2.32964779199999));
#340183=CARTESIAN_POINT('Ctrl Pts',(3.27372981699994,2.2,2.32964779199999));
#340184=CARTESIAN_POINT('Ctrl Pts',(3.27415665499994,12.2,2.33002919399999));
#340185=CARTESIAN_POINT('Ctrl Pts',(3.27415665499994,5.2,2.33002919399999));
#340186=CARTESIAN_POINT('Ctrl Pts',(3.27415665499994,2.2,2.33002919399999));
#340187=CARTESIAN_POINT('Ctrl Pts',(3.27458765499994,12.2,2.33041531599998));
#340188=CARTESIAN_POINT('Ctrl Pts',(3.27458765499994,5.2,2.33041531599998));
#340189=CARTESIAN_POINT('Ctrl Pts',(3.27458765499994,2.2,2.33041531599998));
#340190=CARTESIAN_POINT('Ctrl Pts',(3.27502279799994,12.2,2.33080615899999));
#340191=CARTESIAN_POINT('Ctrl Pts',(3.27502279799994,5.2,2.33080615899999));
#340192=CARTESIAN_POINT('Ctrl Pts',(3.27502279799994,2.2,2.33080615899999));
#340193=CARTESIAN_POINT('Ctrl Pts',(3.27546206299994,12.2,2.33120172699998));
#340194=CARTESIAN_POINT('Ctrl Pts',(3.27546206299994,5.2,2.33120172699998));
#340195=CARTESIAN_POINT('Ctrl Pts',(3.27546206299994,2.2,2.33120172699998));
#340196=CARTESIAN_POINT('Ctrl Pts',(3.27590543099994,12.2,2.33160202399999));
#340197=CARTESIAN_POINT('Ctrl Pts',(3.27590543099994,5.2,2.33160202399999));
#340198=CARTESIAN_POINT('Ctrl Pts',(3.27590543099994,2.2,2.33160202399999));
#340199=CARTESIAN_POINT('Ctrl Pts',(3.27635287999994,12.2,2.33200705099998));
#340200=CARTESIAN_POINT('Ctrl Pts',(3.27635287999994,5.2,2.33200705099998));
#340201=CARTESIAN_POINT('Ctrl Pts',(3.27635287999994,2.2,2.33200705099998));
#340202=CARTESIAN_POINT('Ctrl Pts',(3.27680439199994,12.2,2.33241680999999));
#340203=CARTESIAN_POINT('Ctrl Pts',(3.27680439199994,5.2,2.33241680999999));
#340204=CARTESIAN_POINT('Ctrl Pts',(3.27680439199994,2.2,2.33241680999999));
#340205=CARTESIAN_POINT('Ctrl Pts',(3.27725994699994,12.2,2.33283130599999));
#340206=CARTESIAN_POINT('Ctrl Pts',(3.27725994699994,5.2,2.33283130599999));
#340207=CARTESIAN_POINT('Ctrl Pts',(3.27725994699994,2.2,2.33283130599999));
#340208=CARTESIAN_POINT('Ctrl Pts',(3.27771952399994,12.2,2.33325054099998));
#340209=CARTESIAN_POINT('Ctrl Pts',(3.27771952399994,5.2,2.33325054099998));
#340210=CARTESIAN_POINT('Ctrl Pts',(3.27771952399994,2.2,2.33325054099998));
#340211=CARTESIAN_POINT('Ctrl Pts',(3.27818310399994,12.2,2.33367451799999));
#340212=CARTESIAN_POINT('Ctrl Pts',(3.27818310399994,5.2,2.33367451799999));
#340213=CARTESIAN_POINT('Ctrl Pts',(3.27818310399994,2.2,2.33367451799999));
#340214=CARTESIAN_POINT('Ctrl Pts',(3.27865066799994,12.2,2.33410323899998));
#340215=CARTESIAN_POINT('Ctrl Pts',(3.27865066799994,5.2,2.33410323899998));
#340216=CARTESIAN_POINT('Ctrl Pts',(3.27865066799994,2.2,2.33410323899998));
#340217=CARTESIAN_POINT('Ctrl Pts',(3.27912219499995,12.2,2.33453670599999));
#340218=CARTESIAN_POINT('Ctrl Pts',(3.27912219499995,5.2,2.33453670599999));
#340219=CARTESIAN_POINT('Ctrl Pts',(3.27912219499995,2.2,2.33453670599999));
#340220=CARTESIAN_POINT('Ctrl Pts',(3.27959766499994,12.2,2.33497492199998));
#340221=CARTESIAN_POINT('Ctrl Pts',(3.27959766499994,5.2,2.33497492199998));
#340222=CARTESIAN_POINT('Ctrl Pts',(3.27959766499994,2.2,2.33497492199998));
#340223=CARTESIAN_POINT('Ctrl Pts',(3.28007706199994,12.2,2.33541788999998));
#340224=CARTESIAN_POINT('Ctrl Pts',(3.28007706199994,5.2,2.33541788999998));
#340225=CARTESIAN_POINT('Ctrl Pts',(3.28007706199994,2.2,2.33541788999998));
#340226=CARTESIAN_POINT('Ctrl Pts',(3.28056036299994,12.2,2.33586561299999));
#340227=CARTESIAN_POINT('Ctrl Pts',(3.28056036299994,5.2,2.33586561299999));
#340228=CARTESIAN_POINT('Ctrl Pts',(3.28056036299994,2.2,2.33586561299999));
#340229=CARTESIAN_POINT('Ctrl Pts',(3.28104754899994,12.2,2.33631809299998));
#340230=CARTESIAN_POINT('Ctrl Pts',(3.28104754899994,5.2,2.33631809299998));
#340231=CARTESIAN_POINT('Ctrl Pts',(3.28104754899994,2.2,2.33631809299998));
#340232=CARTESIAN_POINT('Ctrl Pts',(3.28153860199994,12.2,2.33677533199999));
#340233=CARTESIAN_POINT('Ctrl Pts',(3.28153860199994,5.2,2.33677533199999));
#340234=CARTESIAN_POINT('Ctrl Pts',(3.28153860199994,2.2,2.33677533199999));
#340235=CARTESIAN_POINT('Ctrl Pts',(3.28203350199994,12.2,2.33723733099998));
#340236=CARTESIAN_POINT('Ctrl Pts',(3.28203350199994,5.2,2.33723733099998));
#340237=CARTESIAN_POINT('Ctrl Pts',(3.28203350199994,2.2,2.33723733099998));
#340238=CARTESIAN_POINT('Ctrl Pts',(3.28253222999995,12.2,2.33770409699999));
#340239=CARTESIAN_POINT('Ctrl Pts',(3.28253222999995,5.2,2.33770409699999));
#340240=CARTESIAN_POINT('Ctrl Pts',(3.28253222999995,2.2,2.33770409699999));
#340241=CARTESIAN_POINT('Ctrl Pts',(3.28303476599995,12.2,2.33817562699999));
#340242=CARTESIAN_POINT('Ctrl Pts',(3.28303476599995,5.2,2.33817562699999));
#340243=CARTESIAN_POINT('Ctrl Pts',(3.28303476599995,2.2,2.33817562699999));
#340244=CARTESIAN_POINT('Ctrl Pts',(3.28354109199994,12.2,2.33865192699998));
#340245=CARTESIAN_POINT('Ctrl Pts',(3.28354109199994,5.2,2.33865192699998));
#340246=CARTESIAN_POINT('Ctrl Pts',(3.28354109199994,2.2,2.33865192699998));
#340247=CARTESIAN_POINT('Ctrl Pts',(3.28405118799994,12.2,2.33913299699998));
#340248=CARTESIAN_POINT('Ctrl Pts',(3.28405118799994,5.2,2.33913299699998));
#340249=CARTESIAN_POINT('Ctrl Pts',(3.28405118799994,2.2,2.33913299699998));
#340250=CARTESIAN_POINT('Ctrl Pts',(3.28456503599994,12.2,2.33961884099998));
#340251=CARTESIAN_POINT('Ctrl Pts',(3.28456503599994,5.2,2.33961884099998));
#340252=CARTESIAN_POINT('Ctrl Pts',(3.28456503599994,2.2,2.33961884099998));
#340253=CARTESIAN_POINT('Ctrl Pts',(3.28508261599994,12.2,2.34010946099998));
#340254=CARTESIAN_POINT('Ctrl Pts',(3.28508261599994,5.2,2.34010946099998));
#340255=CARTESIAN_POINT('Ctrl Pts',(3.28508261599994,2.2,2.34010946099998));
#340256=CARTESIAN_POINT('Ctrl Pts',(3.28560390899994,12.2,2.34060485799999));
#340257=CARTESIAN_POINT('Ctrl Pts',(3.28560390899994,5.2,2.34060485799999));
#340258=CARTESIAN_POINT('Ctrl Pts',(3.28560390899994,2.2,2.34060485799999));
#340259=CARTESIAN_POINT('Ctrl Pts',(3.28612889699994,12.2,2.34110503599998));
#340260=CARTESIAN_POINT('Ctrl Pts',(3.28612889699994,5.2,2.34110503599998));
#340261=CARTESIAN_POINT('Ctrl Pts',(3.28612889699994,2.2,2.34110503599998));
#340262=CARTESIAN_POINT('Ctrl Pts',(3.28665755999995,12.2,2.34160999499998));
#340263=CARTESIAN_POINT('Ctrl Pts',(3.28665755999995,5.2,2.34160999499998));
#340264=CARTESIAN_POINT('Ctrl Pts',(3.28665755999995,2.2,2.34160999499998));
#340265=CARTESIAN_POINT('Ctrl Pts',(3.28718987999994,12.2,2.34211973899999));
#340266=CARTESIAN_POINT('Ctrl Pts',(3.28718987999994,5.2,2.34211973899999));
#340267=CARTESIAN_POINT('Ctrl Pts',(3.28718987999994,2.2,2.34211973899999));
#340268=CARTESIAN_POINT('Ctrl Pts',(3.28772583699994,12.2,2.34263426899998));
#340269=CARTESIAN_POINT('Ctrl Pts',(3.28772583699994,5.2,2.34263426899998));
#340270=CARTESIAN_POINT('Ctrl Pts',(3.28772583699994,2.2,2.34263426899998));
#340271=CARTESIAN_POINT('Ctrl Pts',(3.28826541599994,12.2,2.34315358699998));
#340272=CARTESIAN_POINT('Ctrl Pts',(3.28826541599994,5.2,2.34315358699998));
#340273=CARTESIAN_POINT('Ctrl Pts',(3.28826541599994,2.2,2.34315358699998));
#340274=CARTESIAN_POINT('Ctrl Pts',(3.28880859399994,12.2,2.34367769699999));
#340275=CARTESIAN_POINT('Ctrl Pts',(3.28880859399994,5.2,2.34367769699999));
#340276=CARTESIAN_POINT('Ctrl Pts',(3.28880859399994,2.2,2.34367769699999));
#340277=CARTESIAN_POINT('Ctrl Pts',(3.28935535399994,12.2,2.34420659699999));
#340278=CARTESIAN_POINT('Ctrl Pts',(3.28935535399994,5.2,2.34420659699999));
#340279=CARTESIAN_POINT('Ctrl Pts',(3.28935535399994,2.2,2.34420659699999));
#340280=CARTESIAN_POINT('Ctrl Pts',(3.28990567899994,12.2,2.34474029299998));
#340281=CARTESIAN_POINT('Ctrl Pts',(3.28990567899994,5.2,2.34474029299998));
#340282=CARTESIAN_POINT('Ctrl Pts',(3.28990567899994,2.2,2.34474029299998));
#340283=CARTESIAN_POINT('Ctrl Pts',(3.29045954899994,12.2,2.34527878499998));
#340284=CARTESIAN_POINT('Ctrl Pts',(3.29045954899994,5.2,2.34527878499998));
#340285=CARTESIAN_POINT('Ctrl Pts',(3.29045954899994,2.2,2.34527878499998));
#340286=CARTESIAN_POINT('Ctrl Pts',(3.29101694499994,12.2,2.34582207599999));
#340287=CARTESIAN_POINT('Ctrl Pts',(3.29101694499994,5.2,2.34582207599999));
#340288=CARTESIAN_POINT('Ctrl Pts',(3.29101694499994,2.2,2.34582207599999));
#340289=CARTESIAN_POINT('Ctrl Pts',(3.29157784999994,12.2,2.34637016699998));
#340290=CARTESIAN_POINT('Ctrl Pts',(3.29157784999994,5.2,2.34637016699998));
#340291=CARTESIAN_POINT('Ctrl Pts',(3.29157784999994,2.2,2.34637016699998));
#340292=CARTESIAN_POINT('Ctrl Pts',(3.29214224399994,12.2,2.34692305899999));
#340293=CARTESIAN_POINT('Ctrl Pts',(3.29214224399994,5.2,2.34692305899999));
#340294=CARTESIAN_POINT('Ctrl Pts',(3.29214224399994,2.2,2.34692305899999));
#340295=CARTESIAN_POINT('Ctrl Pts',(3.29271011099994,12.2,2.34748075599999));
#340296=CARTESIAN_POINT('Ctrl Pts',(3.29271011099994,5.2,2.34748075599999));
#340297=CARTESIAN_POINT('Ctrl Pts',(3.29271011099994,2.2,2.34748075599999));
#340298=CARTESIAN_POINT('Ctrl Pts',(3.29328143099994,12.2,2.34804325699999));
#340299=CARTESIAN_POINT('Ctrl Pts',(3.29328143099994,5.2,2.34804325699999));
#340300=CARTESIAN_POINT('Ctrl Pts',(3.29328143099994,2.2,2.34804325699999));
#340301=CARTESIAN_POINT('Ctrl Pts',(3.29385618599995,12.2,2.34861056699998));
#340302=CARTESIAN_POINT('Ctrl Pts',(3.29385618599995,5.2,2.34861056699998));
#340303=CARTESIAN_POINT('Ctrl Pts',(3.29385618599995,2.2,2.34861056699998));
#340304=CARTESIAN_POINT('Ctrl Pts',(3.29443435799994,12.2,2.34918268699998));
#340305=CARTESIAN_POINT('Ctrl Pts',(3.29443435799994,5.2,2.34918268699998));
#340306=CARTESIAN_POINT('Ctrl Pts',(3.29443435799994,2.2,2.34918268699998));
#340307=CARTESIAN_POINT('Ctrl Pts',(3.29501592899994,12.2,2.34975961699998));
#340308=CARTESIAN_POINT('Ctrl Pts',(3.29501592899994,5.2,2.34975961699998));
#340309=CARTESIAN_POINT('Ctrl Pts',(3.29501592899994,2.2,2.34975961699998));
#340310=CARTESIAN_POINT('Ctrl Pts',(3.29560088099994,12.2,2.35034135999998));
#340311=CARTESIAN_POINT('Ctrl Pts',(3.29560088099994,5.2,2.35034135999998));
#340312=CARTESIAN_POINT('Ctrl Pts',(3.29560088099994,2.2,2.35034135999998));
#340313=CARTESIAN_POINT('Ctrl Pts',(3.29618919699994,12.2,2.35092791599998));
#340314=CARTESIAN_POINT('Ctrl Pts',(3.29618919699994,5.2,2.35092791599998));
#340315=CARTESIAN_POINT('Ctrl Pts',(3.29618919699994,2.2,2.35092791599998));
#340316=CARTESIAN_POINT('Ctrl Pts',(3.29678085799994,12.2,2.35151928999999));
#340317=CARTESIAN_POINT('Ctrl Pts',(3.29678085799994,5.2,2.35151928999999));
#340318=CARTESIAN_POINT('Ctrl Pts',(3.29678085799994,2.2,2.35151928999999));
#340319=CARTESIAN_POINT('Ctrl Pts',(3.29737584499994,12.2,2.35211548099999));
#340320=CARTESIAN_POINT('Ctrl Pts',(3.29737584499994,5.2,2.35211548099999));
#340321=CARTESIAN_POINT('Ctrl Pts',(3.29737584499994,2.2,2.35211548099999));
#340322=CARTESIAN_POINT('Ctrl Pts',(3.29797414199994,12.2,2.35271649099998));
#340323=CARTESIAN_POINT('Ctrl Pts',(3.29797414199994,5.2,2.35271649099998));
#340324=CARTESIAN_POINT('Ctrl Pts',(3.29797414199994,2.2,2.35271649099998));
#340325=CARTESIAN_POINT('Ctrl Pts',(3.29857572899994,12.2,2.35332232199998));
#340326=CARTESIAN_POINT('Ctrl Pts',(3.29857572899994,5.2,2.35332232199998));
#340327=CARTESIAN_POINT('Ctrl Pts',(3.29857572899994,2.2,2.35332232199998));
#340328=CARTESIAN_POINT('Ctrl Pts',(3.29918059199994,12.2,2.35393297499999));
#340329=CARTESIAN_POINT('Ctrl Pts',(3.29918059199994,5.2,2.35393297499999));
#340330=CARTESIAN_POINT('Ctrl Pts',(3.29918059199994,2.2,2.35393297499999));
#340331=CARTESIAN_POINT('Ctrl Pts',(3.29978870899994,12.2,2.35454845199998));
#340332=CARTESIAN_POINT('Ctrl Pts',(3.29978870899994,5.2,2.35454845199998));
#340333=CARTESIAN_POINT('Ctrl Pts',(3.29978870899994,2.2,2.35454845199998));
#340334=CARTESIAN_POINT('Ctrl Pts',(3.30040006499994,12.2,2.35516875499999));
#340335=CARTESIAN_POINT('Ctrl Pts',(3.30040006499994,5.2,2.35516875499999));
#340336=CARTESIAN_POINT('Ctrl Pts',(3.30040006499994,2.2,2.35516875499999));
#340337=CARTESIAN_POINT('Ctrl Pts',(3.30101464199994,12.2,2.35579388399999));
#340338=CARTESIAN_POINT('Ctrl Pts',(3.30101464199994,5.2,2.35579388399999));
#340339=CARTESIAN_POINT('Ctrl Pts',(3.30101464199994,2.2,2.35579388399999));
#340340=CARTESIAN_POINT('Ctrl Pts',(3.30163242099994,12.2,2.35642384199998));
#340341=CARTESIAN_POINT('Ctrl Pts',(3.30163242099994,5.2,2.35642384199998));
#340342=CARTESIAN_POINT('Ctrl Pts',(3.30163242099994,2.2,2.35642384199998));
#340343=CARTESIAN_POINT('Ctrl Pts',(3.30225338599994,12.2,2.35705862899999));
#340344=CARTESIAN_POINT('Ctrl Pts',(3.30225338599994,5.2,2.35705862899999));
#340345=CARTESIAN_POINT('Ctrl Pts',(3.30225338599994,2.2,2.35705862899999));
#340346=CARTESIAN_POINT('Ctrl Pts',(3.30287751899994,12.2,2.35769824699998));
#340347=CARTESIAN_POINT('Ctrl Pts',(3.30287751899994,5.2,2.35769824699998));
#340348=CARTESIAN_POINT('Ctrl Pts',(3.30287751899994,2.2,2.35769824699998));
#340349=CARTESIAN_POINT('Ctrl Pts',(3.30350480199994,12.2,2.35834269899998));
#340350=CARTESIAN_POINT('Ctrl Pts',(3.30350480199994,5.2,2.35834269899998));
#340351=CARTESIAN_POINT('Ctrl Pts',(3.30350480199994,2.2,2.35834269899998));
#340352=CARTESIAN_POINT('Ctrl Pts',(3.30413521799994,12.2,2.35899198299999));
#340353=CARTESIAN_POINT('Ctrl Pts',(3.30413521799994,5.2,2.35899198299999));
#340354=CARTESIAN_POINT('Ctrl Pts',(3.30413521799994,2.2,2.35899198299999));
#340355=CARTESIAN_POINT('Ctrl Pts',(3.30476875099994,12.2,2.35964610299998));
#340356=CARTESIAN_POINT('Ctrl Pts',(3.30476875099994,5.2,2.35964610299998));
#340357=CARTESIAN_POINT('Ctrl Pts',(3.30476875099994,2.2,2.35964610299998));
#340358=CARTESIAN_POINT('Ctrl Pts',(3.30540538099994,12.2,2.36030505899999));
#340359=CARTESIAN_POINT('Ctrl Pts',(3.30540538099994,5.2,2.36030505899999));
#340360=CARTESIAN_POINT('Ctrl Pts',(3.30540538099994,2.2,2.36030505899999));
#340361=CARTESIAN_POINT('Ctrl Pts',(3.30604509299994,12.2,2.36096885299999));
#340362=CARTESIAN_POINT('Ctrl Pts',(3.30604509299994,5.2,2.36096885299999));
#340363=CARTESIAN_POINT('Ctrl Pts',(3.30604509299994,2.2,2.36096885299999));
#340364=CARTESIAN_POINT('Ctrl Pts',(3.30668786899994,12.2,2.36163748599999));
#340365=CARTESIAN_POINT('Ctrl Pts',(3.30668786899994,5.2,2.36163748599999));
#340366=CARTESIAN_POINT('Ctrl Pts',(3.30668786899994,2.2,2.36163748599999));
#340367=CARTESIAN_POINT('Ctrl Pts',(3.30733368999995,12.2,2.36231095899999));
#340368=CARTESIAN_POINT('Ctrl Pts',(3.30733368999995,5.2,2.36231095899999));
#340369=CARTESIAN_POINT('Ctrl Pts',(3.30733368999995,2.2,2.36231095899999));
#340370=CARTESIAN_POINT('Ctrl Pts',(3.30798254199994,12.2,2.36298927299998));
#340371=CARTESIAN_POINT('Ctrl Pts',(3.30798254199994,5.2,2.36298927299998));
#340372=CARTESIAN_POINT('Ctrl Pts',(3.30798254199994,2.2,2.36298927299998));
#340373=CARTESIAN_POINT('Ctrl Pts',(3.30863440599994,12.2,2.36367242999999));
#340374=CARTESIAN_POINT('Ctrl Pts',(3.30863440599994,5.2,2.36367242999999));
#340375=CARTESIAN_POINT('Ctrl Pts',(3.30863440599994,2.2,2.36367242999999));
#340376=CARTESIAN_POINT('Ctrl Pts',(3.30928926599994,12.2,2.36436042899999));
#340377=CARTESIAN_POINT('Ctrl Pts',(3.30928926599994,5.2,2.36436042899999));
#340378=CARTESIAN_POINT('Ctrl Pts',(3.30928926599994,2.2,2.36436042899999));
#340379=CARTESIAN_POINT('Ctrl Pts',(3.30994710299994,12.2,2.36505327499999));
#340380=CARTESIAN_POINT('Ctrl Pts',(3.30994710299994,5.2,2.36505327499999));
#340381=CARTESIAN_POINT('Ctrl Pts',(3.30994710299994,2.2,2.36505327499999));
#340382=CARTESIAN_POINT('Ctrl Pts',(3.31060790199994,12.2,2.36575096499998));
#340383=CARTESIAN_POINT('Ctrl Pts',(3.31060790199994,5.2,2.36575096499998));
#340384=CARTESIAN_POINT('Ctrl Pts',(3.31060790199994,2.2,2.36575096499998));
#340385=CARTESIAN_POINT('Ctrl Pts',(3.31127164499994,12.2,2.36645350299998));
#340386=CARTESIAN_POINT('Ctrl Pts',(3.31127164499994,5.2,2.36645350299998));
#340387=CARTESIAN_POINT('Ctrl Pts',(3.31127164499994,2.2,2.36645350299998));
#340388=CARTESIAN_POINT('Ctrl Pts',(3.31193831499994,12.2,2.36716088899998));
#340389=CARTESIAN_POINT('Ctrl Pts',(3.31193831499994,5.2,2.36716088899998));
#340390=CARTESIAN_POINT('Ctrl Pts',(3.31193831499994,2.2,2.36716088899998));
#340391=CARTESIAN_POINT('Ctrl Pts',(3.31260789699994,12.2,2.36787312299998));
#340392=CARTESIAN_POINT('Ctrl Pts',(3.31260789699994,5.2,2.36787312299998));
#340393=CARTESIAN_POINT('Ctrl Pts',(3.31260789699994,2.2,2.36787312299998));
#340394=CARTESIAN_POINT('Ctrl Pts',(3.31328037199994,12.2,2.36859020799999));
#340395=CARTESIAN_POINT('Ctrl Pts',(3.31328037199994,5.2,2.36859020799999));
#340396=CARTESIAN_POINT('Ctrl Pts',(3.31328037199994,2.2,2.36859020799999));
#340397=CARTESIAN_POINT('Ctrl Pts',(3.31395572399994,12.2,2.36931214299998));
#340398=CARTESIAN_POINT('Ctrl Pts',(3.31395572399994,5.2,2.36931214299998));
#340399=CARTESIAN_POINT('Ctrl Pts',(3.31395572399994,2.2,2.36931214299998));
#340400=CARTESIAN_POINT('Ctrl Pts',(3.31463393699994,12.2,2.37003892999999));
#340401=CARTESIAN_POINT('Ctrl Pts',(3.31463393699994,5.2,2.37003892999999));
#340402=CARTESIAN_POINT('Ctrl Pts',(3.31463393699994,2.2,2.37003892999999));
#340403=CARTESIAN_POINT('Ctrl Pts',(3.31531499199994,12.2,2.37077056999999));
#340404=CARTESIAN_POINT('Ctrl Pts',(3.31531499199994,5.2,2.37077056999999));
#340405=CARTESIAN_POINT('Ctrl Pts',(3.31531499199994,2.2,2.37077056999999));
#340406=CARTESIAN_POINT('Ctrl Pts',(3.31599887599995,12.2,2.37150706399999));
#340407=CARTESIAN_POINT('Ctrl Pts',(3.31599887599995,5.2,2.37150706399999));
#340408=CARTESIAN_POINT('Ctrl Pts',(3.31599887599995,2.2,2.37150706399999));
#340409=CARTESIAN_POINT('Ctrl Pts',(3.31668556899994,12.2,2.37224841199998));
#340410=CARTESIAN_POINT('Ctrl Pts',(3.31668556899994,5.2,2.37224841199998));
#340411=CARTESIAN_POINT('Ctrl Pts',(3.31668556899994,2.2,2.37224841199998));
#340412=CARTESIAN_POINT('Ctrl Pts',(3.31737505599994,12.2,2.37299461599999));
#340413=CARTESIAN_POINT('Ctrl Pts',(3.31737505599994,5.2,2.37299461599999));
#340414=CARTESIAN_POINT('Ctrl Pts',(3.31737505599994,2.2,2.37299461599999));
#340415=CARTESIAN_POINT('Ctrl Pts',(3.31806731999994,12.2,2.37374567499998));
#340416=CARTESIAN_POINT('Ctrl Pts',(3.31806731999994,5.2,2.37374567499998));
#340417=CARTESIAN_POINT('Ctrl Pts',(3.31806731999994,2.2,2.37374567499998));
#340418=CARTESIAN_POINT('Ctrl Pts',(3.31876234499994,12.2,2.37450159199999));
#340419=CARTESIAN_POINT('Ctrl Pts',(3.31876234499994,5.2,2.37450159199999));
#340420=CARTESIAN_POINT('Ctrl Pts',(3.31876234499994,2.2,2.37450159199999));
#340421=CARTESIAN_POINT('Ctrl Pts',(3.31946011499994,12.2,2.37526236699999));
#340422=CARTESIAN_POINT('Ctrl Pts',(3.31946011499994,5.2,2.37526236699999));
#340423=CARTESIAN_POINT('Ctrl Pts',(3.31946011499994,2.2,2.37526236699999));
#340424=CARTESIAN_POINT('Ctrl Pts',(3.32016061199994,12.2,2.37602799999999));
#340425=CARTESIAN_POINT('Ctrl Pts',(3.32016061199994,5.2,2.37602799999999));
#340426=CARTESIAN_POINT('Ctrl Pts',(3.32016061199994,2.2,2.37602799999999));
#340427=CARTESIAN_POINT('Ctrl Pts',(3.32086381999994,12.2,2.37679849299998));
#340428=CARTESIAN_POINT('Ctrl Pts',(3.32086381999994,5.2,2.37679849299998));
#340429=CARTESIAN_POINT('Ctrl Pts',(3.32086381999994,2.2,2.37679849299998));
#340430=CARTESIAN_POINT('Ctrl Pts',(3.32156972399994,12.2,2.37757384599998));
#340431=CARTESIAN_POINT('Ctrl Pts',(3.32156972399994,5.2,2.37757384599998));
#340432=CARTESIAN_POINT('Ctrl Pts',(3.32156972399994,2.2,2.37757384599998));
#340433=CARTESIAN_POINT('Ctrl Pts',(3.32227830699994,12.2,2.37835405899999));
#340434=CARTESIAN_POINT('Ctrl Pts',(3.32227830699994,5.2,2.37835405899999));
#340435=CARTESIAN_POINT('Ctrl Pts',(3.32227830699994,2.2,2.37835405899999));
#340436=CARTESIAN_POINT('Ctrl Pts',(3.32298955199994,12.2,2.37913913399999));
#340437=CARTESIAN_POINT('Ctrl Pts',(3.32298955199994,5.2,2.37913913399999));
#340438=CARTESIAN_POINT('Ctrl Pts',(3.32298955199994,2.2,2.37913913399999));
#340439=CARTESIAN_POINT('Ctrl Pts',(3.32370344499994,12.2,2.37992907099999));
#340440=CARTESIAN_POINT('Ctrl Pts',(3.32370344499994,5.2,2.37992907099999));
#340441=CARTESIAN_POINT('Ctrl Pts',(3.32370344499994,2.2,2.37992907099999));
#340442=CARTESIAN_POINT('Ctrl Pts',(3.32441996699994,12.2,2.38072386999999));
#340443=CARTESIAN_POINT('Ctrl Pts',(3.32441996699994,5.2,2.38072386999999));
#340444=CARTESIAN_POINT('Ctrl Pts',(3.32441996699994,2.2,2.38072386999999));
#340445=CARTESIAN_POINT('Ctrl Pts',(3.32513910199994,12.2,2.38152353399999));
#340446=CARTESIAN_POINT('Ctrl Pts',(3.32513910199994,5.2,2.38152353399999));
#340447=CARTESIAN_POINT('Ctrl Pts',(3.32513910199994,2.2,2.38152353399999));
#340448=CARTESIAN_POINT('Ctrl Pts',(3.32586083699994,12.2,2.38232805999999));
#340449=CARTESIAN_POINT('Ctrl Pts',(3.32586083699994,5.2,2.38232805999999));
#340450=CARTESIAN_POINT('Ctrl Pts',(3.32586083699994,2.2,2.38232805999999));
#340451=CARTESIAN_POINT('Ctrl Pts',(3.32658515399994,12.2,2.38313745099998));
#340452=CARTESIAN_POINT('Ctrl Pts',(3.32658515399994,5.2,2.38313745099998));
#340453=CARTESIAN_POINT('Ctrl Pts',(3.32658515399994,2.2,2.38313745099998));
#340454=CARTESIAN_POINT('Ctrl Pts',(3.32731203599994,12.2,2.38395170799999));
#340455=CARTESIAN_POINT('Ctrl Pts',(3.32731203599994,5.2,2.38395170799999));
#340456=CARTESIAN_POINT('Ctrl Pts',(3.32731203599994,2.2,2.38395170799999));
#340457=CARTESIAN_POINT('Ctrl Pts',(3.32804146799994,12.2,2.38477082899998));
#340458=CARTESIAN_POINT('Ctrl Pts',(3.32804146799994,5.2,2.38477082899998));
#340459=CARTESIAN_POINT('Ctrl Pts',(3.32804146799994,2.2,2.38477082899998));
#340460=CARTESIAN_POINT('Ctrl Pts',(3.32877343399994,12.2,2.38559481699999));
#340461=CARTESIAN_POINT('Ctrl Pts',(3.32877343399994,5.2,2.38559481699999));
#340462=CARTESIAN_POINT('Ctrl Pts',(3.32877343399994,2.2,2.38559481699999));
#340463=CARTESIAN_POINT('Ctrl Pts',(3.32950791799994,12.2,2.38642367099998));
#340464=CARTESIAN_POINT('Ctrl Pts',(3.32950791799994,5.2,2.38642367099998));
#340465=CARTESIAN_POINT('Ctrl Pts',(3.32950791799994,2.2,2.38642367099998));
#340466=CARTESIAN_POINT('Ctrl Pts',(3.33024490499994,12.2,2.38725739199998));
#340467=CARTESIAN_POINT('Ctrl Pts',(3.33024490499994,5.2,2.38725739199998));
#340468=CARTESIAN_POINT('Ctrl Pts',(3.33024490499994,2.2,2.38725739199998));
#340469=CARTESIAN_POINT('Ctrl Pts',(3.33098437699994,12.2,2.38809598099999));
#340470=CARTESIAN_POINT('Ctrl Pts',(3.33098437699994,5.2,2.38809598099999));
#340471=CARTESIAN_POINT('Ctrl Pts',(3.33098437699994,2.2,2.38809598099999));
#340472=CARTESIAN_POINT('Ctrl Pts',(3.33172632099994,12.2,2.38893943699999));
#340473=CARTESIAN_POINT('Ctrl Pts',(3.33172632099994,5.2,2.38893943699999));
#340474=CARTESIAN_POINT('Ctrl Pts',(3.33172632099994,2.2,2.38893943699999));
#340475=CARTESIAN_POINT('Ctrl Pts',(3.33247071999994,12.2,2.38978775999998));
#340476=CARTESIAN_POINT('Ctrl Pts',(3.33247071999994,5.2,2.38978775999998));
#340477=CARTESIAN_POINT('Ctrl Pts',(3.33247071999994,2.2,2.38978775999998));
#340478=CARTESIAN_POINT('Ctrl Pts',(3.33321755799994,12.2,2.39064095399999));
#340479=CARTESIAN_POINT('Ctrl Pts',(3.33321755799994,5.2,2.39064095399999));
#340480=CARTESIAN_POINT('Ctrl Pts',(3.33321755799994,2.2,2.39064095399999));
#340481=CARTESIAN_POINT('Ctrl Pts',(3.33396681799994,12.2,2.39149901499999));
#340482=CARTESIAN_POINT('Ctrl Pts',(3.33396681799994,5.2,2.39149901499999));
#340483=CARTESIAN_POINT('Ctrl Pts',(3.33396681799994,2.2,2.39149901499999));
#340484=CARTESIAN_POINT('Ctrl Pts',(3.33471848799994,12.2,2.39236194599999));
#340485=CARTESIAN_POINT('Ctrl Pts',(3.33471848799994,5.2,2.39236194599999));
#340486=CARTESIAN_POINT('Ctrl Pts',(3.33471848799994,2.2,2.39236194599999));
#340487=CARTESIAN_POINT('Ctrl Pts',(3.33547254899994,12.2,2.39322974699999));
#340488=CARTESIAN_POINT('Ctrl Pts',(3.33547254899994,5.2,2.39322974699999));
#340489=CARTESIAN_POINT('Ctrl Pts',(3.33547254899994,2.2,2.39322974699999));
#340490=CARTESIAN_POINT('Ctrl Pts',(3.33622898699995,12.2,2.39410241599998));
#340491=CARTESIAN_POINT('Ctrl Pts',(3.33622898699995,5.2,2.39410241599998));
#340492=CARTESIAN_POINT('Ctrl Pts',(3.33622898699995,2.2,2.39410241599998));
#340493=CARTESIAN_POINT('Ctrl Pts',(3.33698778599994,12.2,2.39497995699999));
#340494=CARTESIAN_POINT('Ctrl Pts',(3.33698778599994,5.2,2.39497995699999));
#340495=CARTESIAN_POINT('Ctrl Pts',(3.33698778599994,2.2,2.39497995699999));
#340496=CARTESIAN_POINT('Ctrl Pts',(3.33774892999994,12.2,2.39586236699999));
#340497=CARTESIAN_POINT('Ctrl Pts',(3.33774892999994,5.2,2.39586236699999));
#340498=CARTESIAN_POINT('Ctrl Pts',(3.33774892999994,2.2,2.39586236699999));
#340499=CARTESIAN_POINT('Ctrl Pts',(3.33851240499994,12.2,2.39674964699999));
#340500=CARTESIAN_POINT('Ctrl Pts',(3.33851240499994,5.2,2.39674964699999));
#340501=CARTESIAN_POINT('Ctrl Pts',(3.33851240499994,2.2,2.39674964699999));
#340502=CARTESIAN_POINT('Ctrl Pts',(3.33927819399995,12.2,2.39764179899999));
#340503=CARTESIAN_POINT('Ctrl Pts',(3.33927819399995,5.2,2.39764179899999));
#340504=CARTESIAN_POINT('Ctrl Pts',(3.33927819399995,2.2,2.39764179899999));
#340505=CARTESIAN_POINT('Ctrl Pts',(3.34004628199994,12.2,2.39853882099998));
#340506=CARTESIAN_POINT('Ctrl Pts',(3.34004628199994,5.2,2.39853882099998));
#340507=CARTESIAN_POINT('Ctrl Pts',(3.34004628199994,2.2,2.39853882099998));
#340508=CARTESIAN_POINT('Ctrl Pts',(3.34081665599995,12.2,2.39944071499998));
#340509=CARTESIAN_POINT('Ctrl Pts',(3.34081665599995,5.2,2.39944071499998));
#340510=CARTESIAN_POINT('Ctrl Pts',(3.34081665599995,2.2,2.39944071499998));
#340511=CARTESIAN_POINT('Ctrl Pts',(3.34158929699994,12.2,2.40034747899998));
#340512=CARTESIAN_POINT('Ctrl Pts',(3.34158929699994,5.2,2.40034747899998));
#340513=CARTESIAN_POINT('Ctrl Pts',(3.34158929699994,2.2,2.40034747899998));
#340514=CARTESIAN_POINT('Ctrl Pts',(3.34236419099994,12.2,2.40125911499998));
#340515=CARTESIAN_POINT('Ctrl Pts',(3.34236419099994,5.2,2.40125911499998));
#340516=CARTESIAN_POINT('Ctrl Pts',(3.34236419099994,2.2,2.40125911499998));
#340517=CARTESIAN_POINT('Ctrl Pts',(3.34314132399995,12.2,2.40217562199999));
#340518=CARTESIAN_POINT('Ctrl Pts',(3.34314132399995,5.2,2.40217562199999));
#340519=CARTESIAN_POINT('Ctrl Pts',(3.34314132399995,2.2,2.40217562199999));
#340520=CARTESIAN_POINT('Ctrl Pts',(3.34392067899994,12.2,2.40309700199998));
#340521=CARTESIAN_POINT('Ctrl Pts',(3.34392067899994,5.2,2.40309700199998));
#340522=CARTESIAN_POINT('Ctrl Pts',(3.34392067899994,2.2,2.40309700199998));
#340523=CARTESIAN_POINT('Ctrl Pts',(3.34470224199995,12.2,2.40402325199998));
#340524=CARTESIAN_POINT('Ctrl Pts',(3.34470224199995,5.2,2.40402325199998));
#340525=CARTESIAN_POINT('Ctrl Pts',(3.34470224199995,2.2,2.40402325199998));
#340526=CARTESIAN_POINT('Ctrl Pts',(3.34548599799994,12.2,2.40495437299998));
#340527=CARTESIAN_POINT('Ctrl Pts',(3.34548599799994,5.2,2.40495437299998));
#340528=CARTESIAN_POINT('Ctrl Pts',(3.34548599799994,2.2,2.40495437299998));
#340529=CARTESIAN_POINT('Ctrl Pts',(3.34627193199994,12.2,2.40589036699999));
#340530=CARTESIAN_POINT('Ctrl Pts',(3.34627193199994,5.2,2.40589036699999));
#340531=CARTESIAN_POINT('Ctrl Pts',(3.34627193199994,2.2,2.40589036699999));
#340532=CARTESIAN_POINT('Ctrl Pts',(3.34706002699994,12.2,2.40683123199998));
#340533=CARTESIAN_POINT('Ctrl Pts',(3.34706002699994,5.2,2.40683123199998));
#340534=CARTESIAN_POINT('Ctrl Pts',(3.34706002699994,2.2,2.40683123199998));
#340535=CARTESIAN_POINT('Ctrl Pts',(3.34785027099994,12.2,2.40777696799999));
#340536=CARTESIAN_POINT('Ctrl Pts',(3.34785027099994,5.2,2.40777696799999));
#340537=CARTESIAN_POINT('Ctrl Pts',(3.34785027099994,2.2,2.40777696799999));
#340538=CARTESIAN_POINT('Ctrl Pts',(3.34864264599994,12.2,2.40872757599998));
#340539=CARTESIAN_POINT('Ctrl Pts',(3.34864264599994,5.2,2.40872757599998));
#340540=CARTESIAN_POINT('Ctrl Pts',(3.34864264599994,2.2,2.40872757599998));
#340541=CARTESIAN_POINT('Ctrl Pts',(3.34943713899994,12.2,2.40968305499998));
#340542=CARTESIAN_POINT('Ctrl Pts',(3.34943713899994,5.2,2.40968305499998));
#340543=CARTESIAN_POINT('Ctrl Pts',(3.34943713899994,2.2,2.40968305499998));
#340544=CARTESIAN_POINT('Ctrl Pts',(3.35023373399994,12.2,2.41064340599999));
#340545=CARTESIAN_POINT('Ctrl Pts',(3.35023373399994,5.2,2.41064340599999));
#340546=CARTESIAN_POINT('Ctrl Pts',(3.35023373399994,2.2,2.41064340599999));
#340547=CARTESIAN_POINT('Ctrl Pts',(3.35103241699994,12.2,2.41160862899999));
#340548=CARTESIAN_POINT('Ctrl Pts',(3.35103241699994,5.2,2.41160862899999));
#340549=CARTESIAN_POINT('Ctrl Pts',(3.35103241699994,2.2,2.41160862899999));
#340550=CARTESIAN_POINT('Ctrl Pts',(3.35183317199995,12.2,2.41257872199999));
#340551=CARTESIAN_POINT('Ctrl Pts',(3.35183317199995,5.2,2.41257872199999));
#340552=CARTESIAN_POINT('Ctrl Pts',(3.35183317199995,2.2,2.41257872199999));
#340553=CARTESIAN_POINT('Ctrl Pts',(3.35263598499994,12.2,2.41355368599999));
#340554=CARTESIAN_POINT('Ctrl Pts',(3.35263598499994,5.2,2.41355368599999));
#340555=CARTESIAN_POINT('Ctrl Pts',(3.35263598499994,2.2,2.41355368599999));
#340556=CARTESIAN_POINT('Ctrl Pts',(3.35344084099995,12.2,2.41453352099998));
#340557=CARTESIAN_POINT('Ctrl Pts',(3.35344084099995,5.2,2.41453352099998));
#340558=CARTESIAN_POINT('Ctrl Pts',(3.35344084099995,2.2,2.41453352099998));
#340559=CARTESIAN_POINT('Ctrl Pts',(3.35424772499994,12.2,2.41551822699999));
#340560=CARTESIAN_POINT('Ctrl Pts',(3.35424772499994,5.2,2.41551822699999));
#340561=CARTESIAN_POINT('Ctrl Pts',(3.35424772499994,2.2,2.41551822699999));
#340562=CARTESIAN_POINT('Ctrl Pts',(3.35505662299994,12.2,2.41650780399999));
#340563=CARTESIAN_POINT('Ctrl Pts',(3.35505662299994,5.2,2.41650780399999));
#340564=CARTESIAN_POINT('Ctrl Pts',(3.35505662299994,2.2,2.41650780399999));
#340565=CARTESIAN_POINT('Ctrl Pts',(3.35586751999994,12.2,2.41750225099998));
#340566=CARTESIAN_POINT('Ctrl Pts',(3.35586751999994,5.2,2.41750225099998));
#340567=CARTESIAN_POINT('Ctrl Pts',(3.35586751999994,2.2,2.41750225099998));
#340568=CARTESIAN_POINT('Ctrl Pts',(3.35668039999995,12.2,2.41850156699999));
#340569=CARTESIAN_POINT('Ctrl Pts',(3.35668039999995,5.2,2.41850156699999));
#340570=CARTESIAN_POINT('Ctrl Pts',(3.35668039999995,2.2,2.41850156699999));
#340571=CARTESIAN_POINT('Ctrl Pts',(3.35749524999994,12.2,2.41950575399999));
#340572=CARTESIAN_POINT('Ctrl Pts',(3.35749524999994,5.2,2.41950575399999));
#340573=CARTESIAN_POINT('Ctrl Pts',(3.35749524999994,2.2,2.41950575399999));
#340574=CARTESIAN_POINT('Ctrl Pts',(3.35831205499994,12.2,2.42051480999999));
#340575=CARTESIAN_POINT('Ctrl Pts',(3.35831205499994,5.2,2.42051480999999));
#340576=CARTESIAN_POINT('Ctrl Pts',(3.35831205499994,2.2,2.42051480999999));
#340577=CARTESIAN_POINT('Ctrl Pts',(3.35913079999994,12.2,2.42152873599998));
#340578=CARTESIAN_POINT('Ctrl Pts',(3.35913079999994,5.2,2.42152873599998));
#340579=CARTESIAN_POINT('Ctrl Pts',(3.35913079999994,2.2,2.42152873599998));
#340580=CARTESIAN_POINT('Ctrl Pts',(3.35995147099994,12.2,2.42254753099999));
#340581=CARTESIAN_POINT('Ctrl Pts',(3.35995147099994,5.2,2.42254753099999));
#340582=CARTESIAN_POINT('Ctrl Pts',(3.35995147099994,2.2,2.42254753099999));
#340583=CARTESIAN_POINT('Ctrl Pts',(3.36077405299994,12.2,2.42357119399998));
#340584=CARTESIAN_POINT('Ctrl Pts',(3.36077405299994,5.2,2.42357119399998));
#340585=CARTESIAN_POINT('Ctrl Pts',(3.36077405299994,2.2,2.42357119399998));
#340586=CARTESIAN_POINT('Ctrl Pts',(3.36159853199994,12.2,2.42459972499999));
#340587=CARTESIAN_POINT('Ctrl Pts',(3.36159853199994,5.2,2.42459972499999));
#340588=CARTESIAN_POINT('Ctrl Pts',(3.36159853199994,2.2,2.42459972499999));
#340589=CARTESIAN_POINT('Ctrl Pts',(3.36242489299994,12.2,2.42563312399999));
#340590=CARTESIAN_POINT('Ctrl Pts',(3.36242489299994,5.2,2.42563312399999));
#340591=CARTESIAN_POINT('Ctrl Pts',(3.36242489299994,2.2,2.42563312399999));
#340592=CARTESIAN_POINT('Ctrl Pts',(3.36325312199994,12.2,2.42667139099999));
#340593=CARTESIAN_POINT('Ctrl Pts',(3.36325312199994,5.2,2.42667139099999));
#340594=CARTESIAN_POINT('Ctrl Pts',(3.36325312199994,2.2,2.42667139099999));
#340595=CARTESIAN_POINT('Ctrl Pts',(3.36408320499994,12.2,2.42771452499999));
#340596=CARTESIAN_POINT('Ctrl Pts',(3.36408320499994,5.2,2.42771452499999));
#340597=CARTESIAN_POINT('Ctrl Pts',(3.36408320499994,2.2,2.42771452499999));
#340598=CARTESIAN_POINT('Ctrl Pts',(3.36491512599994,12.2,2.42876252599999));
#340599=CARTESIAN_POINT('Ctrl Pts',(3.36491512599994,5.2,2.42876252599999));
#340600=CARTESIAN_POINT('Ctrl Pts',(3.36491512599994,2.2,2.42876252599999));
#340601=CARTESIAN_POINT('Ctrl Pts',(3.36574887299995,12.2,2.42981539299999));
#340602=CARTESIAN_POINT('Ctrl Pts',(3.36574887299995,5.2,2.42981539299999));
#340603=CARTESIAN_POINT('Ctrl Pts',(3.36574887299995,2.2,2.42981539299999));
#340604=CARTESIAN_POINT('Ctrl Pts',(3.36658442999994,12.2,2.43087312599998));
#340605=CARTESIAN_POINT('Ctrl Pts',(3.36658442999994,5.2,2.43087312599998));
#340606=CARTESIAN_POINT('Ctrl Pts',(3.36658442999994,2.2,2.43087312599998));
#340607=CARTESIAN_POINT('Ctrl Pts',(3.36742178299994,12.2,2.43193572399999));
#340608=CARTESIAN_POINT('Ctrl Pts',(3.36742178299994,5.2,2.43193572399999));
#340609=CARTESIAN_POINT('Ctrl Pts',(3.36742178299994,2.2,2.43193572399999));
#340610=CARTESIAN_POINT('Ctrl Pts',(3.36826091899994,12.2,2.43300318699998));
#340611=CARTESIAN_POINT('Ctrl Pts',(3.36826091899994,5.2,2.43300318699998));
#340612=CARTESIAN_POINT('Ctrl Pts',(3.36826091899994,2.2,2.43300318699998));
#340613=CARTESIAN_POINT('Ctrl Pts',(3.36910182099994,12.2,2.43407551499998));
#340614=CARTESIAN_POINT('Ctrl Pts',(3.36910182099994,5.2,2.43407551499998));
#340615=CARTESIAN_POINT('Ctrl Pts',(3.36910182099994,2.2,2.43407551499998));
#340616=CARTESIAN_POINT('Ctrl Pts',(3.36994447899994,12.2,2.43515270699999));
#340617=CARTESIAN_POINT('Ctrl Pts',(3.36994447899994,5.2,2.43515270699999));
#340618=CARTESIAN_POINT('Ctrl Pts',(3.36994447899994,2.2,2.43515270699999));
#340619=CARTESIAN_POINT('Ctrl Pts',(3.37078887499994,12.2,2.43623476199998));
#340620=CARTESIAN_POINT('Ctrl Pts',(3.37078887499994,5.2,2.43623476199998));
#340621=CARTESIAN_POINT('Ctrl Pts',(3.37078887499994,2.2,2.43623476199998));
#340622=CARTESIAN_POINT('Ctrl Pts',(3.37163499699995,12.2,2.43732167999998));
#340623=CARTESIAN_POINT('Ctrl Pts',(3.37163499699995,5.2,2.43732167999998));
#340624=CARTESIAN_POINT('Ctrl Pts',(3.37163499699995,2.2,2.43732167999998));
#340625=CARTESIAN_POINT('Ctrl Pts',(3.37248283099994,12.2,2.43841345999999));
#340626=CARTESIAN_POINT('Ctrl Pts',(3.37248283099994,5.2,2.43841345999999));
#340627=CARTESIAN_POINT('Ctrl Pts',(3.37248283099994,2.2,2.43841345999999));
#340628=CARTESIAN_POINT('Ctrl Pts',(3.37333236099994,12.2,2.43951010199999));
#340629=CARTESIAN_POINT('Ctrl Pts',(3.37333236099994,5.2,2.43951010199999));
#340630=CARTESIAN_POINT('Ctrl Pts',(3.37333236099994,2.2,2.43951010199999));
#340631=CARTESIAN_POINT('Ctrl Pts',(3.37418357599995,12.2,2.44061160399998));
#340632=CARTESIAN_POINT('Ctrl Pts',(3.37418357599995,5.2,2.44061160399998));
#340633=CARTESIAN_POINT('Ctrl Pts',(3.37418357599995,2.2,2.44061160399998));
#340634=CARTESIAN_POINT('Ctrl Pts',(3.37503645899994,12.2,2.44171796699998));
#340635=CARTESIAN_POINT('Ctrl Pts',(3.37503645899994,5.2,2.44171796699998));
#340636=CARTESIAN_POINT('Ctrl Pts',(3.37503645899994,2.2,2.44171796699998));
#340637=CARTESIAN_POINT('Ctrl Pts',(3.37589099799994,12.2,2.44282918999998));
#340638=CARTESIAN_POINT('Ctrl Pts',(3.37589099799994,5.2,2.44282918999998));
#340639=CARTESIAN_POINT('Ctrl Pts',(3.37589099799994,2.2,2.44282918999998));
#340640=CARTESIAN_POINT('Ctrl Pts',(3.37674717799994,12.2,2.44394527199999));
#340641=CARTESIAN_POINT('Ctrl Pts',(3.37674717799994,5.2,2.44394527199999));
#340642=CARTESIAN_POINT('Ctrl Pts',(3.37674717799994,2.2,2.44394527199999));
#340643=CARTESIAN_POINT('Ctrl Pts',(3.37760498599994,12.2,2.44506621199999));
#340644=CARTESIAN_POINT('Ctrl Pts',(3.37760498599994,5.2,2.44506621199999));
#340645=CARTESIAN_POINT('Ctrl Pts',(3.37760498599994,2.2,2.44506621199999));
#340646=CARTESIAN_POINT('Ctrl Pts',(3.37846440799995,12.2,2.44619201099999));
#340647=CARTESIAN_POINT('Ctrl Pts',(3.37846440799995,5.2,2.44619201099999));
#340648=CARTESIAN_POINT('Ctrl Pts',(3.37846440799995,2.2,2.44619201099999));
#340649=CARTESIAN_POINT('Ctrl Pts',(3.37932542999994,12.2,2.44732266599998));
#340650=CARTESIAN_POINT('Ctrl Pts',(3.37932542999994,5.2,2.44732266599998));
#340651=CARTESIAN_POINT('Ctrl Pts',(3.37932542999994,2.2,2.44732266599998));
#340652=CARTESIAN_POINT('Ctrl Pts',(3.38018803799994,12.2,2.44845817699999));
#340653=CARTESIAN_POINT('Ctrl Pts',(3.38018803799994,5.2,2.44845817699999));
#340654=CARTESIAN_POINT('Ctrl Pts',(3.38018803799994,2.2,2.44845817699999));
#340655=CARTESIAN_POINT('Ctrl Pts',(3.38105221899994,12.2,2.44959854399998));
#340656=CARTESIAN_POINT('Ctrl Pts',(3.38105221899994,5.2,2.44959854399998));
#340657=CARTESIAN_POINT('Ctrl Pts',(3.38105221899994,2.2,2.44959854399998));
#340658=CARTESIAN_POINT('Ctrl Pts',(3.38191795799994,12.2,2.45074376599998));
#340659=CARTESIAN_POINT('Ctrl Pts',(3.38191795799994,5.2,2.45074376599998));
#340660=CARTESIAN_POINT('Ctrl Pts',(3.38191795799994,2.2,2.45074376599998));
#340661=CARTESIAN_POINT('Ctrl Pts',(3.38278524199994,12.2,2.45189384199998));
#340662=CARTESIAN_POINT('Ctrl Pts',(3.38278524199994,5.2,2.45189384199998));
#340663=CARTESIAN_POINT('Ctrl Pts',(3.38278524199994,2.2,2.45189384199998));
#340664=CARTESIAN_POINT('Ctrl Pts',(3.38365405699995,12.2,2.45304877099999));
#340665=CARTESIAN_POINT('Ctrl Pts',(3.38365405699995,5.2,2.45304877099999));
#340666=CARTESIAN_POINT('Ctrl Pts',(3.38365405699995,2.2,2.45304877099999));
#340667=CARTESIAN_POINT('Ctrl Pts',(3.38452438999994,12.2,2.45420855199999));
#340668=CARTESIAN_POINT('Ctrl Pts',(3.38452438999994,5.2,2.45420855199999));
#340669=CARTESIAN_POINT('Ctrl Pts',(3.38452438999994,2.2,2.45420855199999));
#340670=CARTESIAN_POINT('Ctrl Pts',(3.38539622699995,12.2,2.45537318499998));
#340671=CARTESIAN_POINT('Ctrl Pts',(3.38539622699995,5.2,2.45537318499998));
#340672=CARTESIAN_POINT('Ctrl Pts',(3.38539622699995,2.2,2.45537318499998));
#340673=CARTESIAN_POINT('Ctrl Pts',(3.38626955399994,12.2,2.45654266899999));
#340674=CARTESIAN_POINT('Ctrl Pts',(3.38626955399994,5.2,2.45654266899999));
#340675=CARTESIAN_POINT('Ctrl Pts',(3.38626955399994,2.2,2.45654266899999));
#340676=CARTESIAN_POINT('Ctrl Pts',(3.38714435899994,12.2,2.45771700299999));
#340677=CARTESIAN_POINT('Ctrl Pts',(3.38714435899994,5.2,2.45771700299999));
#340678=CARTESIAN_POINT('Ctrl Pts',(3.38714435899994,2.2,2.45771700299999));
#340679=CARTESIAN_POINT('Ctrl Pts',(3.38802062599994,12.2,2.45889618499999));
#340680=CARTESIAN_POINT('Ctrl Pts',(3.38802062599994,5.2,2.45889618499999));
#340681=CARTESIAN_POINT('Ctrl Pts',(3.38802062599994,2.2,2.45889618499999));
#340682=CARTESIAN_POINT('Ctrl Pts',(3.38889834299994,12.2,2.46008021599998));
#340683=CARTESIAN_POINT('Ctrl Pts',(3.38889834299994,5.2,2.46008021599998));
#340684=CARTESIAN_POINT('Ctrl Pts',(3.38889834299994,2.2,2.46008021599998));
#340685=CARTESIAN_POINT('Ctrl Pts',(3.38977749699994,12.2,2.46126909299999));
#340686=CARTESIAN_POINT('Ctrl Pts',(3.38977749699994,5.2,2.46126909299999));
#340687=CARTESIAN_POINT('Ctrl Pts',(3.38977749699994,2.2,2.46126909299999));
#340688=CARTESIAN_POINT('Ctrl Pts',(3.39065807299994,12.2,2.46246281799999));
#340689=CARTESIAN_POINT('Ctrl Pts',(3.39065807299994,5.2,2.46246281799999));
#340690=CARTESIAN_POINT('Ctrl Pts',(3.39065807299994,2.2,2.46246281799999));
#340691=CARTESIAN_POINT('Ctrl Pts',(3.39154005999994,12.2,2.46366138699998));
#340692=CARTESIAN_POINT('Ctrl Pts',(3.39154005999994,5.2,2.46366138699998));
#340693=CARTESIAN_POINT('Ctrl Pts',(3.39154005999994,2.2,2.46366138699998));
#340694=CARTESIAN_POINT('Ctrl Pts',(3.39242344199994,12.2,2.46486480199999));
#340695=CARTESIAN_POINT('Ctrl Pts',(3.39242344199994,5.2,2.46486480199999));
#340696=CARTESIAN_POINT('Ctrl Pts',(3.39242344199994,2.2,2.46486480199999));
#340697=CARTESIAN_POINT('Ctrl Pts',(3.39330820699994,12.2,2.46607305899998));
#340698=CARTESIAN_POINT('Ctrl Pts',(3.39330820699994,5.2,2.46607305899998));
#340699=CARTESIAN_POINT('Ctrl Pts',(3.39330820699994,2.2,2.46607305899998));
#340700=CARTESIAN_POINT('Ctrl Pts',(3.39419434099994,12.2,2.46728615799999));
#340701=CARTESIAN_POINT('Ctrl Pts',(3.39419434099994,5.2,2.46728615799999));
#340702=CARTESIAN_POINT('Ctrl Pts',(3.39419434099994,2.2,2.46728615799999));
#340703=CARTESIAN_POINT('Ctrl Pts',(3.39508183099994,12.2,2.46850409999999));
#340704=CARTESIAN_POINT('Ctrl Pts',(3.39508183099994,5.2,2.46850409999999));
#340705=CARTESIAN_POINT('Ctrl Pts',(3.39508183099994,2.2,2.46850409999999));
#340706=CARTESIAN_POINT('Ctrl Pts',(3.39597066499994,12.2,2.46972688099999));
#340707=CARTESIAN_POINT('Ctrl Pts',(3.39597066499994,5.2,2.46972688099999));
#340708=CARTESIAN_POINT('Ctrl Pts',(3.39597066499994,2.2,2.46972688099999));
#340709=CARTESIAN_POINT('Ctrl Pts',(3.39686082699994,12.2,2.47095450299998));
#340710=CARTESIAN_POINT('Ctrl Pts',(3.39686082699994,5.2,2.47095450299998));
#340711=CARTESIAN_POINT('Ctrl Pts',(3.39686082699994,2.2,2.47095450299998));
#340712=CARTESIAN_POINT('Ctrl Pts',(3.39775230599995,12.2,2.47218696199998));
#340713=CARTESIAN_POINT('Ctrl Pts',(3.39775230599995,5.2,2.47218696199998));
#340714=CARTESIAN_POINT('Ctrl Pts',(3.39775230599995,2.2,2.47218696199998));
#340715=CARTESIAN_POINT('Ctrl Pts',(3.39864508699995,12.2,2.47342425899999));
#340716=CARTESIAN_POINT('Ctrl Pts',(3.39864508699995,5.2,2.47342425899999));
#340717=CARTESIAN_POINT('Ctrl Pts',(3.39864508699995,2.2,2.47342425899999));
#340718=CARTESIAN_POINT('Ctrl Pts',(3.39953915999994,12.2,2.47466639199998));
#340719=CARTESIAN_POINT('Ctrl Pts',(3.39953915999994,5.2,2.47466639199998));
#340720=CARTESIAN_POINT('Ctrl Pts',(3.39953915999994,2.2,2.47466639199998));
#340721=CARTESIAN_POINT('Ctrl Pts',(3.40043450899994,12.2,2.47591335999999));
#340722=CARTESIAN_POINT('Ctrl Pts',(3.40043450899994,5.2,2.47591335999999));
#340723=CARTESIAN_POINT('Ctrl Pts',(3.40043450899994,2.2,2.47591335999999));
#340724=CARTESIAN_POINT('Ctrl Pts',(3.40133112099994,12.2,2.47716516099998));
#340725=CARTESIAN_POINT('Ctrl Pts',(3.40133112099994,5.2,2.47716516099998));
#340726=CARTESIAN_POINT('Ctrl Pts',(3.40133112099994,2.2,2.47716516099998));
#340727=CARTESIAN_POINT('Ctrl Pts',(3.40222898499994,12.2,2.47842179599999));
#340728=CARTESIAN_POINT('Ctrl Pts',(3.40222898499994,5.2,2.47842179599999));
#340729=CARTESIAN_POINT('Ctrl Pts',(3.40222898499994,2.2,2.47842179599999));
#340730=CARTESIAN_POINT('Ctrl Pts',(3.40312808599994,12.2,2.47968326199998));
#340731=CARTESIAN_POINT('Ctrl Pts',(3.40312808599994,5.2,2.47968326199998));
#340732=CARTESIAN_POINT('Ctrl Pts',(3.40312808599994,2.2,2.47968326199998));
#340733=CARTESIAN_POINT('Ctrl Pts',(3.40402841099994,12.2,2.48094955899998));
#340734=CARTESIAN_POINT('Ctrl Pts',(3.40402841099994,5.2,2.48094955899998));
#340735=CARTESIAN_POINT('Ctrl Pts',(3.40402841099994,2.2,2.48094955899998));
#340736=CARTESIAN_POINT('Ctrl Pts',(3.40492994799994,12.2,2.48222068499998));
#340737=CARTESIAN_POINT('Ctrl Pts',(3.40492994799994,5.2,2.48222068499998));
#340738=CARTESIAN_POINT('Ctrl Pts',(3.40492994799994,2.2,2.48222068499998));
#340739=CARTESIAN_POINT('Ctrl Pts',(3.40583268299994,12.2,2.48349663999999));
#340740=CARTESIAN_POINT('Ctrl Pts',(3.40583268299994,5.2,2.48349663999999));
#340741=CARTESIAN_POINT('Ctrl Pts',(3.40583268299994,2.2,2.48349663999999));
#340742=CARTESIAN_POINT('Ctrl Pts',(3.40673660499994,12.2,2.48477742199999));
#340743=CARTESIAN_POINT('Ctrl Pts',(3.40673660499994,5.2,2.48477742199999));
#340744=CARTESIAN_POINT('Ctrl Pts',(3.40673660499994,2.2,2.48477742199999));
#340745=CARTESIAN_POINT('Ctrl Pts',(3.40764169899994,12.2,2.48606302799999));
#340746=CARTESIAN_POINT('Ctrl Pts',(3.40764169899994,5.2,2.48606302799999));
#340747=CARTESIAN_POINT('Ctrl Pts',(3.40764169899994,2.2,2.48606302799999));
#340748=CARTESIAN_POINT('Ctrl Pts',(3.40854795299995,12.2,2.48735345999999));
#340749=CARTESIAN_POINT('Ctrl Pts',(3.40854795299995,5.2,2.48735345999999));
#340750=CARTESIAN_POINT('Ctrl Pts',(3.40854795299995,2.2,2.48735345999999));
#340751=CARTESIAN_POINT('Ctrl Pts',(3.40945535399995,12.2,2.48864871499999));
#340752=CARTESIAN_POINT('Ctrl Pts',(3.40945535399995,5.2,2.48864871499999));
#340753=CARTESIAN_POINT('Ctrl Pts',(3.40945535399995,2.2,2.48864871499999));
#340754=CARTESIAN_POINT('Ctrl Pts',(3.41036388799994,12.2,2.48994879199999));
#340755=CARTESIAN_POINT('Ctrl Pts',(3.41036388799994,5.2,2.48994879199999));
#340756=CARTESIAN_POINT('Ctrl Pts',(3.41036388799994,2.2,2.48994879199999));
#340757=CARTESIAN_POINT('Ctrl Pts',(3.41127354499994,12.2,2.49125368899998));
#340758=CARTESIAN_POINT('Ctrl Pts',(3.41127354499994,5.2,2.49125368899998));
#340759=CARTESIAN_POINT('Ctrl Pts',(3.41127354499994,2.2,2.49125368899998));
#340760=CARTESIAN_POINT('Ctrl Pts',(3.41218430899994,12.2,2.49256340699999));
#340761=CARTESIAN_POINT('Ctrl Pts',(3.41218430899994,5.2,2.49256340699999));
#340762=CARTESIAN_POINT('Ctrl Pts',(3.41218430899994,2.2,2.49256340699999));
#340763=CARTESIAN_POINT('Ctrl Pts',(3.41309616999995,12.2,2.49387794199999));
#340764=CARTESIAN_POINT('Ctrl Pts',(3.41309616999995,5.2,2.49387794199999));
#340765=CARTESIAN_POINT('Ctrl Pts',(3.41309616999995,2.2,2.49387794199999));
#340766=CARTESIAN_POINT('Ctrl Pts',(3.41400911399994,12.2,2.49519729399999));
#340767=CARTESIAN_POINT('Ctrl Pts',(3.41400911399994,5.2,2.49519729399999));
#340768=CARTESIAN_POINT('Ctrl Pts',(3.41400911399994,2.2,2.49519729399999));
#340769=CARTESIAN_POINT('Ctrl Pts',(3.41492312799994,12.2,2.49652146199999));
#340770=CARTESIAN_POINT('Ctrl Pts',(3.41492312799994,5.2,2.49652146199999));
#340771=CARTESIAN_POINT('Ctrl Pts',(3.41492312799994,2.2,2.49652146199999));
#340772=CARTESIAN_POINT('Ctrl Pts',(3.41583819899994,12.2,2.49785044399999));
#340773=CARTESIAN_POINT('Ctrl Pts',(3.41583819899994,5.2,2.49785044399999));
#340774=CARTESIAN_POINT('Ctrl Pts',(3.41583819899994,2.2,2.49785044399999));
#340775=CARTESIAN_POINT('Ctrl Pts',(3.41675431499994,12.2,2.49918423799999));
#340776=CARTESIAN_POINT('Ctrl Pts',(3.41675431499994,5.2,2.49918423799999));
#340777=CARTESIAN_POINT('Ctrl Pts',(3.41675431499994,2.2,2.49918423799999));
#340778=CARTESIAN_POINT('Ctrl Pts',(3.41767146399994,12.2,2.50052284399998));
#340779=CARTESIAN_POINT('Ctrl Pts',(3.41767146399994,5.2,2.50052284399998));
#340780=CARTESIAN_POINT('Ctrl Pts',(3.41767146399994,2.2,2.50052284399998));
#340781=CARTESIAN_POINT('Ctrl Pts',(3.41858963299994,12.2,2.50186625899998));
#340782=CARTESIAN_POINT('Ctrl Pts',(3.41858963299994,5.2,2.50186625899998));
#340783=CARTESIAN_POINT('Ctrl Pts',(3.41858963299994,2.2,2.50186625899998));
#340784=CARTESIAN_POINT('Ctrl Pts',(3.41950880899994,12.2,2.50321448399998));
#340785=CARTESIAN_POINT('Ctrl Pts',(3.41950880899994,5.2,2.50321448399998));
#340786=CARTESIAN_POINT('Ctrl Pts',(3.41950880899994,2.2,2.50321448399998));
#340787=CARTESIAN_POINT('Ctrl Pts',(3.42042897899994,12.2,2.50456751499998));
#340788=CARTESIAN_POINT('Ctrl Pts',(3.42042897899994,5.2,2.50456751499998));
#340789=CARTESIAN_POINT('Ctrl Pts',(3.42042897899994,2.2,2.50456751499998));
#340790=CARTESIAN_POINT('Ctrl Pts',(3.42135013199994,12.2,2.50592535199999));
#340791=CARTESIAN_POINT('Ctrl Pts',(3.42135013199994,5.2,2.50592535199999));
#340792=CARTESIAN_POINT('Ctrl Pts',(3.42135013199994,2.2,2.50592535199999));
#340793=CARTESIAN_POINT('Ctrl Pts',(3.42227225299994,12.2,2.50728799399998));
#340794=CARTESIAN_POINT('Ctrl Pts',(3.42227225299994,5.2,2.50728799399998));
#340795=CARTESIAN_POINT('Ctrl Pts',(3.42227225299994,2.2,2.50728799399998));
#340796=CARTESIAN_POINT('Ctrl Pts',(3.42319533199994,12.2,2.50865543899998));
#340797=CARTESIAN_POINT('Ctrl Pts',(3.42319533199994,5.2,2.50865543899998));
#340798=CARTESIAN_POINT('Ctrl Pts',(3.42319533199994,2.2,2.50865543899998));
#340799=CARTESIAN_POINT('Ctrl Pts',(3.42411935599995,12.2,2.51002768399999));
#340800=CARTESIAN_POINT('Ctrl Pts',(3.42411935599995,5.2,2.51002768399999));
#340801=CARTESIAN_POINT('Ctrl Pts',(3.42411935599995,2.2,2.51002768399999));
#340802=CARTESIAN_POINT('Ctrl Pts',(3.42504431299994,12.2,2.51140472999998));
#340803=CARTESIAN_POINT('Ctrl Pts',(3.42504431299994,5.2,2.51140472999998));
#340804=CARTESIAN_POINT('Ctrl Pts',(3.42504431299994,2.2,2.51140472999998));
#340805=CARTESIAN_POINT('Ctrl Pts',(3.42597018799994,12.2,2.51278657299999));
#340806=CARTESIAN_POINT('Ctrl Pts',(3.42597018799994,5.2,2.51278657299999));
#340807=CARTESIAN_POINT('Ctrl Pts',(3.42597018799994,2.2,2.51278657299999));
#340808=CARTESIAN_POINT('Ctrl Pts',(3.42689697199994,12.2,2.51417321299999));
#340809=CARTESIAN_POINT('Ctrl Pts',(3.42689697199994,5.2,2.51417321299999));
#340810=CARTESIAN_POINT('Ctrl Pts',(3.42689697199994,2.2,2.51417321299999));
#340811=CARTESIAN_POINT('Ctrl Pts',(3.42782465099994,12.2,2.51556464999998));
#340812=CARTESIAN_POINT('Ctrl Pts',(3.42782465099994,5.2,2.51556464999998));
#340813=CARTESIAN_POINT('Ctrl Pts',(3.42782465099994,2.2,2.51556464999998));
#340814=CARTESIAN_POINT('Ctrl Pts',(3.42875321299994,12.2,2.51696087899998));
#340815=CARTESIAN_POINT('Ctrl Pts',(3.42875321299994,5.2,2.51696087899998));
#340816=CARTESIAN_POINT('Ctrl Pts',(3.42875321299994,2.2,2.51696087899998));
#340817=CARTESIAN_POINT('Ctrl Pts',(3.42968264399994,12.2,2.51836190099999));
#340818=CARTESIAN_POINT('Ctrl Pts',(3.42968264399994,5.2,2.51836190099999));
#340819=CARTESIAN_POINT('Ctrl Pts',(3.42968264399994,2.2,2.51836190099999));
#340820=CARTESIAN_POINT('Ctrl Pts',(3.43061293499995,12.2,2.51976771299999));
#340821=CARTESIAN_POINT('Ctrl Pts',(3.43061293499995,5.2,2.51976771299999));
#340822=CARTESIAN_POINT('Ctrl Pts',(3.43061293499995,2.2,2.51976771299999));
#340823=CARTESIAN_POINT('Ctrl Pts',(3.43154406999994,12.2,2.52117831499999));
#340824=CARTESIAN_POINT('Ctrl Pts',(3.43154406999994,5.2,2.52117831499999));
#340825=CARTESIAN_POINT('Ctrl Pts',(3.43154406999994,2.2,2.52117831499999));
#340826=CARTESIAN_POINT('Ctrl Pts',(3.43247603999994,12.2,2.52259370399998));
#340827=CARTESIAN_POINT('Ctrl Pts',(3.43247603999994,5.2,2.52259370399998));
#340828=CARTESIAN_POINT('Ctrl Pts',(3.43247603999994,2.2,2.52259370399998));
#340829=CARTESIAN_POINT('Ctrl Pts',(3.43340883199994,12.2,2.52401387799999));
#340830=CARTESIAN_POINT('Ctrl Pts',(3.43340883199994,5.2,2.52401387799999));
#340831=CARTESIAN_POINT('Ctrl Pts',(3.43340883199994,2.2,2.52401387799999));
#340832=CARTESIAN_POINT('Ctrl Pts',(3.43434243299995,12.2,2.52543883599999));
#340833=CARTESIAN_POINT('Ctrl Pts',(3.43434243299995,5.2,2.52543883599999));
#340834=CARTESIAN_POINT('Ctrl Pts',(3.43434243299995,2.2,2.52543883599999));
#340835=CARTESIAN_POINT('Ctrl Pts',(3.43527682999994,12.2,2.52686857799999));
#340836=CARTESIAN_POINT('Ctrl Pts',(3.43527682999994,5.2,2.52686857799999));
#340837=CARTESIAN_POINT('Ctrl Pts',(3.43527682999994,2.2,2.52686857799999));
#340838=CARTESIAN_POINT('Ctrl Pts',(3.43621201299994,12.2,2.52830309999998));
#340839=CARTESIAN_POINT('Ctrl Pts',(3.43621201299994,5.2,2.52830309999998));
#340840=CARTESIAN_POINT('Ctrl Pts',(3.43621201299994,2.2,2.52830309999998));
#340841=CARTESIAN_POINT('Ctrl Pts',(3.43714796899994,12.2,2.52974240099999));
#340842=CARTESIAN_POINT('Ctrl Pts',(3.43714796899994,5.2,2.52974240099999));
#340843=CARTESIAN_POINT('Ctrl Pts',(3.43714796899994,2.2,2.52974240099999));
#340844=CARTESIAN_POINT('Ctrl Pts',(3.43808468699994,12.2,2.53118647999998));
#340845=CARTESIAN_POINT('Ctrl Pts',(3.43808468699994,5.2,2.53118647999998));
#340846=CARTESIAN_POINT('Ctrl Pts',(3.43808468699994,2.2,2.53118647999998));
#340847=CARTESIAN_POINT('Ctrl Pts',(3.43902215299994,12.2,2.53263533399998));
#340848=CARTESIAN_POINT('Ctrl Pts',(3.43902215299994,5.2,2.53263533399998));
#340849=CARTESIAN_POINT('Ctrl Pts',(3.43902215299994,2.2,2.53263533399998));
#340850=CARTESIAN_POINT('Ctrl Pts',(3.43996035499994,12.2,2.53408896199999));
#340851=CARTESIAN_POINT('Ctrl Pts',(3.43996035499994,5.2,2.53408896199999));
#340852=CARTESIAN_POINT('Ctrl Pts',(3.43996035499994,2.2,2.53408896199999));
#340853=CARTESIAN_POINT('Ctrl Pts',(3.44089928299995,12.2,2.53554736299999));
#340854=CARTESIAN_POINT('Ctrl Pts',(3.44089928299995,5.2,2.53554736299999));
#340855=CARTESIAN_POINT('Ctrl Pts',(3.44089928299995,2.2,2.53554736299999));
#340856=CARTESIAN_POINT('Ctrl Pts',(3.44183892399994,12.2,2.53701053499999));
#340857=CARTESIAN_POINT('Ctrl Pts',(3.44183892399994,5.2,2.53701053499999));
#340858=CARTESIAN_POINT('Ctrl Pts',(3.44183892399994,2.2,2.53701053499999));
#340859=CARTESIAN_POINT('Ctrl Pts',(3.44277926599994,12.2,2.53847847499999));
#340860=CARTESIAN_POINT('Ctrl Pts',(3.44277926599994,5.2,2.53847847499999));
#340861=CARTESIAN_POINT('Ctrl Pts',(3.44277926599994,2.2,2.53847847499999));
#340862=CARTESIAN_POINT('Ctrl Pts',(3.44372029599994,12.2,2.53995118299999));
#340863=CARTESIAN_POINT('Ctrl Pts',(3.44372029599994,5.2,2.53995118299999));
#340864=CARTESIAN_POINT('Ctrl Pts',(3.44372029599994,2.2,2.53995118299999));
#340865=CARTESIAN_POINT('Ctrl Pts',(3.44466200399994,12.2,2.54142865499999));
#340866=CARTESIAN_POINT('Ctrl Pts',(3.44466200399994,5.2,2.54142865499999));
#340867=CARTESIAN_POINT('Ctrl Pts',(3.44466200399994,2.2,2.54142865499999));
#340868=CARTESIAN_POINT('Ctrl Pts',(3.44560437599994,12.2,2.54291089099999));
#340869=CARTESIAN_POINT('Ctrl Pts',(3.44560437599994,5.2,2.54291089099999));
#340870=CARTESIAN_POINT('Ctrl Pts',(3.44560437599994,2.2,2.54291089099999));
#340871=CARTESIAN_POINT('Ctrl Pts',(3.44654740199994,12.2,2.54439788899998));
#340872=CARTESIAN_POINT('Ctrl Pts',(3.44654740199994,5.2,2.54439788899998));
#340873=CARTESIAN_POINT('Ctrl Pts',(3.44654740199994,2.2,2.54439788899998));
#340874=CARTESIAN_POINT('Ctrl Pts',(3.44749106999994,12.2,2.54588964799999));
#340875=CARTESIAN_POINT('Ctrl Pts',(3.44749106999994,5.2,2.54588964799999));
#340876=CARTESIAN_POINT('Ctrl Pts',(3.44749106999994,2.2,2.54588964799999));
#340877=CARTESIAN_POINT('Ctrl Pts',(3.44843536699994,12.2,2.54738616399998));
#340878=CARTESIAN_POINT('Ctrl Pts',(3.44843536699994,5.2,2.54738616399998));
#340879=CARTESIAN_POINT('Ctrl Pts',(3.44843536699994,2.2,2.54738616399998));
#340880=CARTESIAN_POINT('Ctrl Pts',(3.44938028199994,12.2,2.54888743599999));
#340881=CARTESIAN_POINT('Ctrl Pts',(3.44938028199994,5.2,2.54888743599999));
#340882=CARTESIAN_POINT('Ctrl Pts',(3.44938028199994,2.2,2.54888743599999));
#340883=CARTESIAN_POINT('Ctrl Pts',(3.45032580399995,12.2,2.55039346299998));
#340884=CARTESIAN_POINT('Ctrl Pts',(3.45032580399995,5.2,2.55039346299998));
#340885=CARTESIAN_POINT('Ctrl Pts',(3.45032580399995,2.2,2.55039346299998));
#340886=CARTESIAN_POINT('Ctrl Pts',(3.45127191899994,12.2,2.55190424299998));
#340887=CARTESIAN_POINT('Ctrl Pts',(3.45127191899994,5.2,2.55190424299998));
#340888=CARTESIAN_POINT('Ctrl Pts',(3.45127191899994,2.2,2.55190424299998));
#340889=CARTESIAN_POINT('Ctrl Pts',(3.45221861799994,12.2,2.55341977199999));
#340890=CARTESIAN_POINT('Ctrl Pts',(3.45221861799994,5.2,2.55341977199999));
#340891=CARTESIAN_POINT('Ctrl Pts',(3.45221861799994,2.2,2.55341977199999));
#340892=CARTESIAN_POINT('Ctrl Pts',(3.45316588699994,12.2,2.55494005199999));
#340893=CARTESIAN_POINT('Ctrl Pts',(3.45316588699994,5.2,2.55494005199999));
#340894=CARTESIAN_POINT('Ctrl Pts',(3.45316588699994,2.2,2.55494005199999));
#340895=CARTESIAN_POINT('Ctrl Pts',(3.45411371499994,12.2,2.55646507699999));
#340896=CARTESIAN_POINT('Ctrl Pts',(3.45411371499994,5.2,2.55646507699999));
#340897=CARTESIAN_POINT('Ctrl Pts',(3.45411371499994,2.2,2.55646507699999));
#340898=CARTESIAN_POINT('Ctrl Pts',(3.45506209099995,12.2,2.55799484799999));
#340899=CARTESIAN_POINT('Ctrl Pts',(3.45506209099995,5.2,2.55799484799999));
#340900=CARTESIAN_POINT('Ctrl Pts',(3.45506209099995,2.2,2.55799484799999));
#340901=CARTESIAN_POINT('Ctrl Pts',(3.45601100299994,12.2,2.55952936199999));
#340902=CARTESIAN_POINT('Ctrl Pts',(3.45601100299994,5.2,2.55952936199999));
#340903=CARTESIAN_POINT('Ctrl Pts',(3.45601100299994,2.2,2.55952936199999));
#340904=CARTESIAN_POINT('Ctrl Pts',(3.45696043999994,12.2,2.56106861699998));
#340905=CARTESIAN_POINT('Ctrl Pts',(3.45696043999994,5.2,2.56106861699998));
#340906=CARTESIAN_POINT('Ctrl Pts',(3.45696043999994,2.2,2.56106861699998));
#340907=CARTESIAN_POINT('Ctrl Pts',(3.45791038899995,12.2,2.56261261099999));
#340908=CARTESIAN_POINT('Ctrl Pts',(3.45791038899995,5.2,2.56261261099999));
#340909=CARTESIAN_POINT('Ctrl Pts',(3.45791038899995,2.2,2.56261261099999));
#340910=CARTESIAN_POINT('Ctrl Pts',(3.45886083999994,12.2,2.56416134199998));
#340911=CARTESIAN_POINT('Ctrl Pts',(3.45886083999994,5.2,2.56416134199998));
#340912=CARTESIAN_POINT('Ctrl Pts',(3.45886083999994,2.2,2.56416134199998));
#340913=CARTESIAN_POINT('Ctrl Pts',(3.45981177999994,12.2,2.56571480799998));
#340914=CARTESIAN_POINT('Ctrl Pts',(3.45981177999994,5.2,2.56571480799998));
#340915=CARTESIAN_POINT('Ctrl Pts',(3.45981177999994,2.2,2.56571480799998));
#340916=CARTESIAN_POINT('Ctrl Pts',(3.46076319899994,12.2,2.56727300699998));
#340917=CARTESIAN_POINT('Ctrl Pts',(3.46076319899994,5.2,2.56727300699998));
#340918=CARTESIAN_POINT('Ctrl Pts',(3.46076319899994,2.2,2.56727300699998));
#340919=CARTESIAN_POINT('Ctrl Pts',(3.46171508399994,12.2,2.56883593899998));
#340920=CARTESIAN_POINT('Ctrl Pts',(3.46171508399994,5.2,2.56883593899998));
#340921=CARTESIAN_POINT('Ctrl Pts',(3.46171508399994,2.2,2.56883593899998));
#340922=CARTESIAN_POINT('Ctrl Pts',(3.46266742399994,12.2,2.57040359899998));
#340923=CARTESIAN_POINT('Ctrl Pts',(3.46266742399994,5.2,2.57040359899998));
#340924=CARTESIAN_POINT('Ctrl Pts',(3.46266742399994,2.2,2.57040359899998));
#340925=CARTESIAN_POINT('Ctrl Pts',(3.46362020899994,12.2,2.57197598599999));
#340926=CARTESIAN_POINT('Ctrl Pts',(3.46362020899994,5.2,2.57197598599999));
#340927=CARTESIAN_POINT('Ctrl Pts',(3.46362020899994,2.2,2.57197598599999));
#340928=CARTESIAN_POINT('Ctrl Pts',(3.46457342599995,12.2,2.57355309899998));
#340929=CARTESIAN_POINT('Ctrl Pts',(3.46457342599995,5.2,2.57355309899998));
#340930=CARTESIAN_POINT('Ctrl Pts',(3.46457342599995,2.2,2.57355309899998));
#340931=CARTESIAN_POINT('Ctrl Pts',(3.46552706299994,12.2,2.57513493299999));
#340932=CARTESIAN_POINT('Ctrl Pts',(3.46552706299994,5.2,2.57513493299999));
#340933=CARTESIAN_POINT('Ctrl Pts',(3.46552706299994,2.2,2.57513493299999));
#340934=CARTESIAN_POINT('Ctrl Pts',(3.46648111099995,12.2,2.57672148999998));
#340935=CARTESIAN_POINT('Ctrl Pts',(3.46648111099995,5.2,2.57672148999998));
#340936=CARTESIAN_POINT('Ctrl Pts',(3.46648111099995,2.2,2.57672148999998));
#340937=CARTESIAN_POINT('Ctrl Pts',(3.46743555599994,12.2,2.57831276599998));
#340938=CARTESIAN_POINT('Ctrl Pts',(3.46743555599994,5.2,2.57831276599998));
#340939=CARTESIAN_POINT('Ctrl Pts',(3.46743555599994,2.2,2.57831276599998));
#340940=CARTESIAN_POINT('Ctrl Pts',(3.46839038799994,12.2,2.57990875799998));
#340941=CARTESIAN_POINT('Ctrl Pts',(3.46839038799994,5.2,2.57990875799998));
#340942=CARTESIAN_POINT('Ctrl Pts',(3.46839038799994,2.2,2.57990875799998));
#340943=CARTESIAN_POINT('Ctrl Pts',(3.46934559599994,12.2,2.58150946499998));
#340944=CARTESIAN_POINT('Ctrl Pts',(3.46934559599994,5.2,2.58150946499998));
#340945=CARTESIAN_POINT('Ctrl Pts',(3.46934559599994,2.2,2.58150946499998));
#340946=CARTESIAN_POINT('Ctrl Pts',(3.47030116899994,12.2,2.58311488399999));
#340947=CARTESIAN_POINT('Ctrl Pts',(3.47030116899994,5.2,2.58311488399999));
#340948=CARTESIAN_POINT('Ctrl Pts',(3.47030116899994,2.2,2.58311488399999));
#340949=CARTESIAN_POINT('Ctrl Pts',(3.47125709399994,12.2,2.58472501499998));
#340950=CARTESIAN_POINT('Ctrl Pts',(3.47125709399994,5.2,2.58472501499998));
#340951=CARTESIAN_POINT('Ctrl Pts',(3.47125709399994,2.2,2.58472501499998));
#340952=CARTESIAN_POINT('Ctrl Pts',(3.47221336199994,12.2,2.58633985299999));
#340953=CARTESIAN_POINT('Ctrl Pts',(3.47221336199994,5.2,2.58633985299999));
#340954=CARTESIAN_POINT('Ctrl Pts',(3.47221336199994,2.2,2.58633985299999));
#340955=CARTESIAN_POINT('Ctrl Pts',(3.47316995899994,12.2,2.58795939899999));
#340956=CARTESIAN_POINT('Ctrl Pts',(3.47316995899994,5.2,2.58795939899999));
#340957=CARTESIAN_POINT('Ctrl Pts',(3.47316995899994,2.2,2.58795939899999));
#340958=CARTESIAN_POINT('Ctrl Pts',(3.47412687699994,12.2,2.58958364799999));
#340959=CARTESIAN_POINT('Ctrl Pts',(3.47412687699994,5.2,2.58958364799999));
#340960=CARTESIAN_POINT('Ctrl Pts',(3.47412687699994,2.2,2.58958364799999));
#340961=CARTESIAN_POINT('Ctrl Pts',(3.47508410099994,12.2,2.59121259899998));
#340962=CARTESIAN_POINT('Ctrl Pts',(3.47508410099994,5.2,2.59121259899998));
#340963=CARTESIAN_POINT('Ctrl Pts',(3.47508410099994,2.2,2.59121259899998));
#340964=CARTESIAN_POINT('Ctrl Pts',(3.47604162499994,12.2,2.59284624899998));
#340965=CARTESIAN_POINT('Ctrl Pts',(3.47604162499994,5.2,2.59284624899998));
#340966=CARTESIAN_POINT('Ctrl Pts',(3.47604162499994,2.2,2.59284624899998));
#340967=CARTESIAN_POINT('Ctrl Pts',(3.47699943199994,12.2,2.59448459699998));
#340968=CARTESIAN_POINT('Ctrl Pts',(3.47699943199994,5.2,2.59448459699998));
#340969=CARTESIAN_POINT('Ctrl Pts',(3.47699943199994,2.2,2.59448459699998));
#340970=CARTESIAN_POINT('Ctrl Pts',(3.47795751599994,12.2,2.59612764199999));
#340971=CARTESIAN_POINT('Ctrl Pts',(3.47795751599994,5.2,2.59612764199999));
#340972=CARTESIAN_POINT('Ctrl Pts',(3.47795751599994,2.2,2.59612764199999));
#340973=CARTESIAN_POINT('Ctrl Pts',(3.47891586199994,12.2,2.59777537799999));
#340974=CARTESIAN_POINT('Ctrl Pts',(3.47891586199994,5.2,2.59777537799999));
#340975=CARTESIAN_POINT('Ctrl Pts',(3.47891586199994,2.2,2.59777537799999));
#340976=CARTESIAN_POINT('Ctrl Pts',(3.47987446199994,12.2,2.59942780599999));
#340977=CARTESIAN_POINT('Ctrl Pts',(3.47987446199994,5.2,2.59942780599999));
#340978=CARTESIAN_POINT('Ctrl Pts',(3.47987446199994,2.2,2.59942780599999));
#340979=CARTESIAN_POINT('Ctrl Pts',(3.48083330299994,12.2,2.60108492199999));
#340980=CARTESIAN_POINT('Ctrl Pts',(3.48083330299994,5.2,2.60108492199999));
#340981=CARTESIAN_POINT('Ctrl Pts',(3.48083330299994,2.2,2.60108492199999));
#340982=CARTESIAN_POINT('Ctrl Pts',(3.48179237399994,12.2,2.60274672499998));
#340983=CARTESIAN_POINT('Ctrl Pts',(3.48179237399994,5.2,2.60274672499998));
#340984=CARTESIAN_POINT('Ctrl Pts',(3.48179237399994,2.2,2.60274672499998));
#340985=CARTESIAN_POINT('Ctrl Pts',(3.48275166499994,12.2,2.60441321199998));
#340986=CARTESIAN_POINT('Ctrl Pts',(3.48275166499994,5.2,2.60441321199998));
#340987=CARTESIAN_POINT('Ctrl Pts',(3.48275166499994,2.2,2.60441321199998));
#340988=CARTESIAN_POINT('Ctrl Pts',(3.48371116499994,12.2,2.60608438099998));
#340989=CARTESIAN_POINT('Ctrl Pts',(3.48371116499994,5.2,2.60608438099998));
#340990=CARTESIAN_POINT('Ctrl Pts',(3.48371116499994,2.2,2.60608438099998));
#340991=CARTESIAN_POINT('Ctrl Pts',(3.48467086199994,12.2,2.60776022999998));
#340992=CARTESIAN_POINT('Ctrl Pts',(3.48467086199994,5.2,2.60776022999998));
#340993=CARTESIAN_POINT('Ctrl Pts',(3.48467086199994,2.2,2.60776022999998));
#340994=CARTESIAN_POINT('Ctrl Pts',(3.48563074599994,12.2,2.60944075599999));
#340995=CARTESIAN_POINT('Ctrl Pts',(3.48563074599994,5.2,2.60944075599999));
#340996=CARTESIAN_POINT('Ctrl Pts',(3.48563074599994,2.2,2.60944075599999));
#340997=CARTESIAN_POINT('Ctrl Pts',(3.48659080599994,12.2,2.61112595699998));
#340998=CARTESIAN_POINT('Ctrl Pts',(3.48659080599994,5.2,2.61112595699998));
#340999=CARTESIAN_POINT('Ctrl Pts',(3.48659080599994,2.2,2.61112595699998));
#341000=CARTESIAN_POINT('Ctrl Pts',(3.48755102999994,12.2,2.61281583099999));
#341001=CARTESIAN_POINT('Ctrl Pts',(3.48755102999994,5.2,2.61281583099999));
#341002=CARTESIAN_POINT('Ctrl Pts',(3.48755102999994,2.2,2.61281583099999));
#341003=CARTESIAN_POINT('Ctrl Pts',(3.48851140799994,12.2,2.61451037499998));
#341004=CARTESIAN_POINT('Ctrl Pts',(3.48851140799994,5.2,2.61451037499998));
#341005=CARTESIAN_POINT('Ctrl Pts',(3.48851140799994,2.2,2.61451037499998));
#341006=CARTESIAN_POINT('Ctrl Pts',(3.48947192999994,12.2,2.61620958799998));
#341007=CARTESIAN_POINT('Ctrl Pts',(3.48947192999994,5.2,2.61620958799998));
#341008=CARTESIAN_POINT('Ctrl Pts',(3.48947192999994,2.2,2.61620958799998));
#341009=CARTESIAN_POINT('Ctrl Pts',(3.49043258299994,12.2,2.61791346599999));
#341010=CARTESIAN_POINT('Ctrl Pts',(3.49043258299994,5.2,2.61791346599999));
#341011=CARTESIAN_POINT('Ctrl Pts',(3.49043258299994,2.2,2.61791346599999));
#341012=CARTESIAN_POINT('Ctrl Pts',(3.49139335899994,12.2,2.61962200699998));
#341013=CARTESIAN_POINT('Ctrl Pts',(3.49139335899994,5.2,2.61962200699998));
#341014=CARTESIAN_POINT('Ctrl Pts',(3.49139335899994,2.2,2.61962200699998));
#341015=CARTESIAN_POINT('Ctrl Pts',(3.49235424499994,12.2,2.62133520899998));
#341016=CARTESIAN_POINT('Ctrl Pts',(3.49235424499994,5.2,2.62133520899998));
#341017=CARTESIAN_POINT('Ctrl Pts',(3.49235424499994,2.2,2.62133520899998));
#341018=CARTESIAN_POINT('Ctrl Pts',(3.49331522999994,12.2,2.62305306999998));
#341019=CARTESIAN_POINT('Ctrl Pts',(3.49331522999994,5.2,2.62305306999998));
#341020=CARTESIAN_POINT('Ctrl Pts',(3.49331522999994,2.2,2.62305306999998));
#341021=CARTESIAN_POINT('Ctrl Pts',(3.49427630399994,12.2,2.62477558799999));
#341022=CARTESIAN_POINT('Ctrl Pts',(3.49427630399994,5.2,2.62477558799999));
#341023=CARTESIAN_POINT('Ctrl Pts',(3.49427630399994,2.2,2.62477558799999));
#341024=CARTESIAN_POINT('Ctrl Pts',(3.49523745799994,12.2,2.62650275899999));
#341025=CARTESIAN_POINT('Ctrl Pts',(3.49523745799994,5.2,2.62650275899999));
#341026=CARTESIAN_POINT('Ctrl Pts',(3.49523745799994,2.2,2.62650275899999));
#341027=CARTESIAN_POINT('Ctrl Pts',(3.49619867799994,12.2,2.62823458099999));
#341028=CARTESIAN_POINT('Ctrl Pts',(3.49619867799994,5.2,2.62823458099999));
#341029=CARTESIAN_POINT('Ctrl Pts',(3.49619867799994,2.2,2.62823458099999));
#341030=CARTESIAN_POINT('Ctrl Pts',(3.49715995499994,12.2,2.62997105199998));
#341031=CARTESIAN_POINT('Ctrl Pts',(3.49715995499994,5.2,2.62997105199998));
#341032=CARTESIAN_POINT('Ctrl Pts',(3.49715995499994,2.2,2.62997105199998));
#341033=CARTESIAN_POINT('Ctrl Pts',(3.49812127999995,12.2,2.63171216999999));
#341034=CARTESIAN_POINT('Ctrl Pts',(3.49812127999995,5.2,2.63171216999999));
#341035=CARTESIAN_POINT('Ctrl Pts',(3.49812127999995,2.2,2.63171216999999));
#341036=CARTESIAN_POINT('Ctrl Pts',(3.49908263899994,12.2,2.63345793199999));
#341037=CARTESIAN_POINT('Ctrl Pts',(3.49908263899994,5.2,2.63345793199999));
#341038=CARTESIAN_POINT('Ctrl Pts',(3.49908263899994,2.2,2.63345793199999));
#341039=CARTESIAN_POINT('Ctrl Pts',(3.50004402399994,12.2,2.63520833499998));
#341040=CARTESIAN_POINT('Ctrl Pts',(3.50004402399994,5.2,2.63520833499998));
#341041=CARTESIAN_POINT('Ctrl Pts',(3.50004402399994,2.2,2.63520833499998));
#341042=CARTESIAN_POINT('Ctrl Pts',(3.50100542299994,12.2,2.63696337799999));
#341043=CARTESIAN_POINT('Ctrl Pts',(3.50100542299994,5.2,2.63696337799999));
#341044=CARTESIAN_POINT('Ctrl Pts',(3.50100542299994,2.2,2.63696337799999));
#341045=CARTESIAN_POINT('Ctrl Pts',(3.50196682599994,12.2,2.63872305799998));
#341046=CARTESIAN_POINT('Ctrl Pts',(3.50196682599994,5.2,2.63872305799998));
#341047=CARTESIAN_POINT('Ctrl Pts',(3.50196682599994,2.2,2.63872305799998));
#341048=CARTESIAN_POINT('Ctrl Pts',(3.50292822099994,12.2,2.64048737199998));
#341049=CARTESIAN_POINT('Ctrl Pts',(3.50292822099994,5.2,2.64048737199998));
#341050=CARTESIAN_POINT('Ctrl Pts',(3.50292822099994,2.2,2.64048737199998));
#341051=CARTESIAN_POINT('Ctrl Pts',(3.50388959899994,12.2,2.64225631699999));
#341052=CARTESIAN_POINT('Ctrl Pts',(3.50388959899994,5.2,2.64225631699999));
#341053=CARTESIAN_POINT('Ctrl Pts',(3.50388959899994,2.2,2.64225631699999));
#341054=CARTESIAN_POINT('Ctrl Pts',(3.50485095099994,12.2,2.64402989199999));
#341055=CARTESIAN_POINT('Ctrl Pts',(3.50485095099994,5.2,2.64402989199999));
#341056=CARTESIAN_POINT('Ctrl Pts',(3.50485095099994,2.2,2.64402989199999));
#341057=CARTESIAN_POINT('Ctrl Pts',(3.50581226299994,12.2,2.64580809299999));
#341058=CARTESIAN_POINT('Ctrl Pts',(3.50581226299994,5.2,2.64580809299999));
#341059=CARTESIAN_POINT('Ctrl Pts',(3.50581226299994,2.2,2.64580809299999));
#341060=CARTESIAN_POINT('Ctrl Pts',(3.50677352599994,12.2,2.64759091899998));
#341061=CARTESIAN_POINT('Ctrl Pts',(3.50677352599994,5.2,2.64759091899998));
#341062=CARTESIAN_POINT('Ctrl Pts',(3.50677352599994,2.2,2.64759091899998));
#341063=CARTESIAN_POINT('Ctrl Pts',(3.50773473099994,12.2,2.64937836699998));
#341064=CARTESIAN_POINT('Ctrl Pts',(3.50773473099994,5.2,2.64937836699998));
#341065=CARTESIAN_POINT('Ctrl Pts',(3.50773473099994,2.2,2.64937836699998));
#341066=CARTESIAN_POINT('Ctrl Pts',(3.50869586499994,12.2,2.65117043299998));
#341067=CARTESIAN_POINT('Ctrl Pts',(3.50869586499994,5.2,2.65117043299998));
#341068=CARTESIAN_POINT('Ctrl Pts',(3.50869586499994,2.2,2.65117043299998));
#341069=CARTESIAN_POINT('Ctrl Pts',(3.50965691899995,12.2,2.65296711499998));
#341070=CARTESIAN_POINT('Ctrl Pts',(3.50965691899995,5.2,2.65296711499998));
#341071=CARTESIAN_POINT('Ctrl Pts',(3.50965691899995,2.2,2.65296711499998));
#341072=CARTESIAN_POINT('Ctrl Pts',(3.51061788199994,12.2,2.65476841099999));
#341073=CARTESIAN_POINT('Ctrl Pts',(3.51061788199994,5.2,2.65476841099999));
#341074=CARTESIAN_POINT('Ctrl Pts',(3.51061788199994,2.2,2.65476841099999));
#341075=CARTESIAN_POINT('Ctrl Pts',(3.51157874499994,12.2,2.65657431999998));
#341076=CARTESIAN_POINT('Ctrl Pts',(3.51157874499994,5.2,2.65657431999998));
#341077=CARTESIAN_POINT('Ctrl Pts',(3.51157874499994,2.2,2.65657431999998));
#341078=CARTESIAN_POINT('Ctrl Pts',(3.51253949599994,12.2,2.65838483699999));
#341079=CARTESIAN_POINT('Ctrl Pts',(3.51253949599994,5.2,2.65838483699999));
#341080=CARTESIAN_POINT('Ctrl Pts',(3.51253949599994,2.2,2.65838483699999));
#341081=CARTESIAN_POINT('Ctrl Pts',(3.51350012599994,12.2,2.66019995999999));
#341082=CARTESIAN_POINT('Ctrl Pts',(3.51350012599994,5.2,2.66019995999999));
#341083=CARTESIAN_POINT('Ctrl Pts',(3.51350012599994,2.2,2.66019995999999));
#341084=CARTESIAN_POINT('Ctrl Pts',(3.51446062299994,12.2,2.66201968599999));
#341085=CARTESIAN_POINT('Ctrl Pts',(3.51446062299994,5.2,2.66201968599999));
#341086=CARTESIAN_POINT('Ctrl Pts',(3.51446062299994,2.2,2.66201968599999));
#341087=CARTESIAN_POINT('Ctrl Pts',(3.51542097799994,12.2,2.66384401299998));
#341088=CARTESIAN_POINT('Ctrl Pts',(3.51542097799994,5.2,2.66384401299998));
#341089=CARTESIAN_POINT('Ctrl Pts',(3.51542097799994,2.2,2.66384401299998));
#341090=CARTESIAN_POINT('Ctrl Pts',(3.51638117999994,12.2,2.66567293999999));
#341091=CARTESIAN_POINT('Ctrl Pts',(3.51638117999994,5.2,2.66567293999999));
#341092=CARTESIAN_POINT('Ctrl Pts',(3.51638117999994,2.2,2.66567293999999));
#341093=CARTESIAN_POINT('Ctrl Pts',(3.51734121999994,12.2,2.66750645999998));
#341094=CARTESIAN_POINT('Ctrl Pts',(3.51734121999994,5.2,2.66750645999998));
#341095=CARTESIAN_POINT('Ctrl Pts',(3.51734121999994,2.2,2.66750645999998));
#341096=CARTESIAN_POINT('Ctrl Pts',(3.51830108599994,12.2,2.66934457499998));
#341097=CARTESIAN_POINT('Ctrl Pts',(3.51830108599994,5.2,2.66934457499998));
#341098=CARTESIAN_POINT('Ctrl Pts',(3.51830108599994,2.2,2.66934457499998));
#341099=CARTESIAN_POINT('Ctrl Pts',(3.51926076799994,12.2,2.67118727999998));
#341100=CARTESIAN_POINT('Ctrl Pts',(3.51926076799994,5.2,2.67118727999998));
#341101=CARTESIAN_POINT('Ctrl Pts',(3.51926076799994,2.2,2.67118727999998));
#341102=CARTESIAN_POINT('Ctrl Pts',(3.52022025699994,12.2,2.67303457199999));
#341103=CARTESIAN_POINT('Ctrl Pts',(3.52022025699994,5.2,2.67303457199999));
#341104=CARTESIAN_POINT('Ctrl Pts',(3.52022025699994,2.2,2.67303457199999));
#341105=CARTESIAN_POINT('Ctrl Pts',(3.52117954299994,12.2,2.67488644999998));
#341106=CARTESIAN_POINT('Ctrl Pts',(3.52117954299994,5.2,2.67488644999998));
#341107=CARTESIAN_POINT('Ctrl Pts',(3.52117954299994,2.2,2.67488644999998));
#341108=CARTESIAN_POINT('Ctrl Pts',(3.52213861299994,12.2,2.67674290999998));
#341109=CARTESIAN_POINT('Ctrl Pts',(3.52213861299994,5.2,2.67674290999998));
#341110=CARTESIAN_POINT('Ctrl Pts',(3.52213861299994,2.2,2.67674290999998));
#341111=CARTESIAN_POINT('Ctrl Pts',(3.52309746099994,12.2,2.67860394899999));
#341112=CARTESIAN_POINT('Ctrl Pts',(3.52309746099994,5.2,2.67860394899999));
#341113=CARTESIAN_POINT('Ctrl Pts',(3.52309746099994,2.2,2.67860394899999));
#341114=CARTESIAN_POINT('Ctrl Pts',(3.52405607299994,12.2,2.68046956499998));
#341115=CARTESIAN_POINT('Ctrl Pts',(3.52405607299994,5.2,2.68046956499998));
#341116=CARTESIAN_POINT('Ctrl Pts',(3.52405607299994,2.2,2.68046956499998));
#341117=CARTESIAN_POINT('Ctrl Pts',(3.52501444199994,12.2,2.68233975599999));
#341118=CARTESIAN_POINT('Ctrl Pts',(3.52501444199994,5.2,2.68233975599999));
#341119=CARTESIAN_POINT('Ctrl Pts',(3.52501444199994,2.2,2.68233975599999));
#341120=CARTESIAN_POINT('Ctrl Pts',(3.52597255499994,12.2,2.68421451799998));
#341121=CARTESIAN_POINT('Ctrl Pts',(3.52597255499994,5.2,2.68421451799998));
#341122=CARTESIAN_POINT('Ctrl Pts',(3.52597255499994,2.2,2.68421451799998));
#341123=CARTESIAN_POINT('Ctrl Pts',(3.52693040399994,12.2,2.68609384799999));
#341124=CARTESIAN_POINT('Ctrl Pts',(3.52693040399994,5.2,2.68609384799999));
#341125=CARTESIAN_POINT('Ctrl Pts',(3.52693040399994,2.2,2.68609384799999));
#341126=CARTESIAN_POINT('Ctrl Pts',(3.52788797899994,12.2,2.68797774499999));
#341127=CARTESIAN_POINT('Ctrl Pts',(3.52788797899994,5.2,2.68797774499999));
#341128=CARTESIAN_POINT('Ctrl Pts',(3.52788797899994,2.2,2.68797774499999));
#341129=CARTESIAN_POINT('Ctrl Pts',(3.52884526799994,12.2,2.68986620399998));
#341130=CARTESIAN_POINT('Ctrl Pts',(3.52884526799994,5.2,2.68986620399998));
#341131=CARTESIAN_POINT('Ctrl Pts',(3.52884526799994,2.2,2.68986620399998));
#341132=CARTESIAN_POINT('Ctrl Pts',(3.52980226299994,12.2,2.69175922499999));
#341133=CARTESIAN_POINT('Ctrl Pts',(3.52980226299994,5.2,2.69175922499999));
#341134=CARTESIAN_POINT('Ctrl Pts',(3.52980226299994,2.2,2.69175922499999));
#341135=CARTESIAN_POINT('Ctrl Pts',(3.53075895299995,12.2,2.69365680299998));
#341136=CARTESIAN_POINT('Ctrl Pts',(3.53075895299995,5.2,2.69365680299998));
#341137=CARTESIAN_POINT('Ctrl Pts',(3.53075895299995,2.2,2.69365680299998));
#341138=CARTESIAN_POINT('Ctrl Pts',(3.53171532799994,12.2,2.69555893499999));
#341139=CARTESIAN_POINT('Ctrl Pts',(3.53171532799994,5.2,2.69555893499999));
#341140=CARTESIAN_POINT('Ctrl Pts',(3.53171532799994,2.2,2.69555893499999));
#341141=CARTESIAN_POINT('Ctrl Pts',(3.53267137899994,12.2,2.69746561999998));
#341142=CARTESIAN_POINT('Ctrl Pts',(3.53267137899994,5.2,2.69746561999998));
#341143=CARTESIAN_POINT('Ctrl Pts',(3.53267137899994,2.2,2.69746561999998));
#341144=CARTESIAN_POINT('Ctrl Pts',(3.53362709499994,12.2,2.69937685399999));
#341145=CARTESIAN_POINT('Ctrl Pts',(3.53362709499994,5.2,2.69937685399999));
#341146=CARTESIAN_POINT('Ctrl Pts',(3.53362709499994,2.2,2.69937685399999));
#341147=CARTESIAN_POINT('Ctrl Pts',(3.53458246599994,12.2,2.70129263399999));
#341148=CARTESIAN_POINT('Ctrl Pts',(3.53458246599994,5.2,2.70129263399999));
#341149=CARTESIAN_POINT('Ctrl Pts',(3.53458246599994,2.2,2.70129263399999));
#341150=CARTESIAN_POINT('Ctrl Pts',(3.53553748299994,12.2,2.70321295899999));
#341151=CARTESIAN_POINT('Ctrl Pts',(3.53553748299994,5.2,2.70321295899999));
#341152=CARTESIAN_POINT('Ctrl Pts',(3.53553748299994,2.2,2.70321295899999));
#341153=CARTESIAN_POINT('Ctrl Pts',(3.53649213599994,12.2,2.70513782399998));
#341154=CARTESIAN_POINT('Ctrl Pts',(3.53649213599994,5.2,2.70513782399998));
#341155=CARTESIAN_POINT('Ctrl Pts',(3.53649213599994,2.2,2.70513782399998));
#341156=CARTESIAN_POINT('Ctrl Pts',(3.53744641399994,12.2,2.70706722699998));
#341157=CARTESIAN_POINT('Ctrl Pts',(3.53744641399994,5.2,2.70706722699998));
#341158=CARTESIAN_POINT('Ctrl Pts',(3.53744641399994,2.2,2.70706722699998));
#341159=CARTESIAN_POINT('Ctrl Pts',(3.53840030899994,12.2,2.70900116499998));
#341160=CARTESIAN_POINT('Ctrl Pts',(3.53840030899994,5.2,2.70900116499998));
#341161=CARTESIAN_POINT('Ctrl Pts',(3.53840030899994,2.2,2.70900116499998));
#341162=CARTESIAN_POINT('Ctrl Pts',(3.53935380899994,12.2,2.71093963499998));
#341163=CARTESIAN_POINT('Ctrl Pts',(3.53935380899994,5.2,2.71093963499998));
#341164=CARTESIAN_POINT('Ctrl Pts',(3.53935380899994,2.2,2.71093963499998));
#341165=CARTESIAN_POINT('Ctrl Pts',(3.54030690499994,12.2,2.71288263399998));
#341166=CARTESIAN_POINT('Ctrl Pts',(3.54030690499994,5.2,2.71288263399998));
#341167=CARTESIAN_POINT('Ctrl Pts',(3.54030690499994,2.2,2.71288263399998));
#341168=CARTESIAN_POINT('Ctrl Pts',(3.54125958799994,12.2,2.71483016099998));
#341169=CARTESIAN_POINT('Ctrl Pts',(3.54125958799994,5.2,2.71483016099998));
#341170=CARTESIAN_POINT('Ctrl Pts',(3.54125958799994,2.2,2.71483016099998));
#341171=CARTESIAN_POINT('Ctrl Pts',(3.54221184699994,12.2,2.71678220999998));
#341172=CARTESIAN_POINT('Ctrl Pts',(3.54221184699994,5.2,2.71678220999998));
#341173=CARTESIAN_POINT('Ctrl Pts',(3.54221184699994,2.2,2.71678220999998));
#341174=CARTESIAN_POINT('Ctrl Pts',(3.54316367399994,12.2,2.71873878099999));
#341175=CARTESIAN_POINT('Ctrl Pts',(3.54316367399994,5.2,2.71873878099999));
#341176=CARTESIAN_POINT('Ctrl Pts',(3.54316367399994,2.2,2.71873878099999));
#341177=CARTESIAN_POINT('Ctrl Pts',(3.54411505699994,12.2,2.72069986899999));
#341178=CARTESIAN_POINT('Ctrl Pts',(3.54411505699994,5.2,2.72069986899999));
#341179=CARTESIAN_POINT('Ctrl Pts',(3.54411505699994,2.2,2.72069986899999));
#341180=CARTESIAN_POINT('Ctrl Pts',(3.54506598799994,12.2,2.72266547199998));
#341181=CARTESIAN_POINT('Ctrl Pts',(3.54506598799994,5.2,2.72266547199998));
#341182=CARTESIAN_POINT('Ctrl Pts',(3.54506598799994,2.2,2.72266547199998));
#341183=CARTESIAN_POINT('Ctrl Pts',(3.54601645599994,12.2,2.72463558699998));
#341184=CARTESIAN_POINT('Ctrl Pts',(3.54601645599994,5.2,2.72463558699998));
#341185=CARTESIAN_POINT('Ctrl Pts',(3.54601645599994,2.2,2.72463558699998));
#341186=CARTESIAN_POINT('Ctrl Pts',(3.54696645299994,12.2,2.72661021099999));
#341187=CARTESIAN_POINT('Ctrl Pts',(3.54696645299994,5.2,2.72661021099999));
#341188=CARTESIAN_POINT('Ctrl Pts',(3.54696645299994,2.2,2.72661021099999));
#341189=CARTESIAN_POINT('Ctrl Pts',(3.54791596799994,12.2,2.72858934099999));
#341190=CARTESIAN_POINT('Ctrl Pts',(3.54791596799994,5.2,2.72858934099999));
#341191=CARTESIAN_POINT('Ctrl Pts',(3.54791596799994,2.2,2.72858934099999));
#341192=CARTESIAN_POINT('Ctrl Pts',(3.54886499099994,12.2,2.73057297399999));
#341193=CARTESIAN_POINT('Ctrl Pts',(3.54886499099994,5.2,2.73057297399999));
#341194=CARTESIAN_POINT('Ctrl Pts',(3.54886499099994,2.2,2.73057297399999));
#341195=CARTESIAN_POINT('Ctrl Pts',(3.54981351399994,12.2,2.73256110699998));
#341196=CARTESIAN_POINT('Ctrl Pts',(3.54981351399994,5.2,2.73256110699998));
#341197=CARTESIAN_POINT('Ctrl Pts',(3.54981351399994,2.2,2.73256110699998));
#341198=CARTESIAN_POINT('Ctrl Pts',(3.55076152599994,12.2,2.73455373799998));
#341199=CARTESIAN_POINT('Ctrl Pts',(3.55076152599994,5.2,2.73455373799998));
#341200=CARTESIAN_POINT('Ctrl Pts',(3.55076152599994,2.2,2.73455373799998));
#341201=CARTESIAN_POINT('Ctrl Pts',(3.55170901699994,12.2,2.73655086199999));
#341202=CARTESIAN_POINT('Ctrl Pts',(3.55170901699994,5.2,2.73655086199999));
#341203=CARTESIAN_POINT('Ctrl Pts',(3.55170901699994,2.2,2.73655086199999));
#341204=CARTESIAN_POINT('Ctrl Pts',(3.55265597999994,12.2,2.73855247899998));
#341205=CARTESIAN_POINT('Ctrl Pts',(3.55265597999994,5.2,2.73855247899998));
#341206=CARTESIAN_POINT('Ctrl Pts',(3.55265597999994,2.2,2.73855247899998));
#341207=CARTESIAN_POINT('Ctrl Pts',(3.55360240199994,12.2,2.74055858299998));
#341208=CARTESIAN_POINT('Ctrl Pts',(3.55360240199994,5.2,2.74055858299998));
#341209=CARTESIAN_POINT('Ctrl Pts',(3.55360240199994,2.2,2.74055858299998));
#341210=CARTESIAN_POINT('Ctrl Pts',(3.55454827599994,12.2,2.74256917199998));
#341211=CARTESIAN_POINT('Ctrl Pts',(3.55454827599994,5.2,2.74256917199998));
#341212=CARTESIAN_POINT('Ctrl Pts',(3.55454827599994,2.2,2.74256917199998));
#341213=CARTESIAN_POINT('Ctrl Pts',(3.55549359199994,12.2,2.74458424399998));
#341214=CARTESIAN_POINT('Ctrl Pts',(3.55549359199994,5.2,2.74458424399998));
#341215=CARTESIAN_POINT('Ctrl Pts',(3.55549359199994,2.2,2.74458424399998));
#341216=CARTESIAN_POINT('Ctrl Pts',(3.55643833899994,12.2,2.74660379399998));
#341217=CARTESIAN_POINT('Ctrl Pts',(3.55643833899994,5.2,2.74660379399998));
#341218=CARTESIAN_POINT('Ctrl Pts',(3.55643833899994,2.2,2.74660379399998));
#341219=CARTESIAN_POINT('Ctrl Pts',(3.55738250899994,12.2,2.74862782199998));
#341220=CARTESIAN_POINT('Ctrl Pts',(3.55738250899994,5.2,2.74862782199998));
#341221=CARTESIAN_POINT('Ctrl Pts',(3.55738250899994,2.2,2.74862782199998));
#341222=CARTESIAN_POINT('Ctrl Pts',(3.55832609299994,12.2,2.75065632199999));
#341223=CARTESIAN_POINT('Ctrl Pts',(3.55832609299994,5.2,2.75065632199999));
#341224=CARTESIAN_POINT('Ctrl Pts',(3.55832609299994,2.2,2.75065632199999));
#341225=CARTESIAN_POINT('Ctrl Pts',(3.55926907899994,12.2,2.75268929099998));
#341226=CARTESIAN_POINT('Ctrl Pts',(3.55926907899994,5.2,2.75268929099998));
#341227=CARTESIAN_POINT('Ctrl Pts',(3.55926907899994,2.2,2.75268929099998));
#341228=CARTESIAN_POINT('Ctrl Pts',(3.56021145999994,12.2,2.75472672799999));
#341229=CARTESIAN_POINT('Ctrl Pts',(3.56021145999994,5.2,2.75472672799999));
#341230=CARTESIAN_POINT('Ctrl Pts',(3.56021145999994,2.2,2.75472672799999));
#341231=CARTESIAN_POINT('Ctrl Pts',(3.56115322699994,12.2,2.75676862799998));
#341232=CARTESIAN_POINT('Ctrl Pts',(3.56115322699994,5.2,2.75676862799998));
#341233=CARTESIAN_POINT('Ctrl Pts',(3.56115322699994,2.2,2.75676862799998));
#341234=CARTESIAN_POINT('Ctrl Pts',(3.56209436799994,12.2,2.75881499099999));
#341235=CARTESIAN_POINT('Ctrl Pts',(3.56209436799994,5.2,2.75881499099999));
#341236=CARTESIAN_POINT('Ctrl Pts',(3.56209436799994,2.2,2.75881499099999));
#341237=CARTESIAN_POINT('Ctrl Pts',(3.56303487499994,12.2,2.76086580999999));
#341238=CARTESIAN_POINT('Ctrl Pts',(3.56303487499994,5.2,2.76086580999999));
#341239=CARTESIAN_POINT('Ctrl Pts',(3.56303487499994,2.2,2.76086580999999));
#341240=CARTESIAN_POINT('Ctrl Pts',(3.56397473899994,12.2,2.76292108399999));
#341241=CARTESIAN_POINT('Ctrl Pts',(3.56397473899994,5.2,2.76292108399999));
#341242=CARTESIAN_POINT('Ctrl Pts',(3.56397473899994,2.2,2.76292108399999));
#341243=CARTESIAN_POINT('Ctrl Pts',(3.56491394999995,12.2,2.76498080999998));
#341244=CARTESIAN_POINT('Ctrl Pts',(3.56491394999995,5.2,2.76498080999998));
#341245=CARTESIAN_POINT('Ctrl Pts',(3.56491394999995,2.2,2.76498080999998));
#341246=CARTESIAN_POINT('Ctrl Pts',(3.56585249999994,12.2,2.76704498399998));
#341247=CARTESIAN_POINT('Ctrl Pts',(3.56585249999994,5.2,2.76704498399998));
#341248=CARTESIAN_POINT('Ctrl Pts',(3.56585249999994,2.2,2.76704498399998));
#341249=CARTESIAN_POINT('Ctrl Pts',(3.56679037699994,12.2,2.76911360399998));
#341250=CARTESIAN_POINT('Ctrl Pts',(3.56679037699994,5.2,2.76911360399998));
#341251=CARTESIAN_POINT('Ctrl Pts',(3.56679037699994,2.2,2.76911360399998));
#341252=CARTESIAN_POINT('Ctrl Pts',(3.56772757399995,12.2,2.77118666499998));
#341253=CARTESIAN_POINT('Ctrl Pts',(3.56772757399995,5.2,2.77118666499998));
#341254=CARTESIAN_POINT('Ctrl Pts',(3.56772757399995,2.2,2.77118666499998));
#341255=CARTESIAN_POINT('Ctrl Pts',(3.56866408199994,12.2,2.77326416599998));
#341256=CARTESIAN_POINT('Ctrl Pts',(3.56866408199994,5.2,2.77326416599998));
#341257=CARTESIAN_POINT('Ctrl Pts',(3.56866408199994,2.2,2.77326416599998));
#341258=CARTESIAN_POINT('Ctrl Pts',(3.56959988899994,12.2,2.77534610199999));
#341259=CARTESIAN_POINT('Ctrl Pts',(3.56959988899994,5.2,2.77534610199999));
#341260=CARTESIAN_POINT('Ctrl Pts',(3.56959988899994,2.2,2.77534610199999));
#341261=CARTESIAN_POINT('Ctrl Pts',(3.57053498799994,12.2,2.77743247199999));
#341262=CARTESIAN_POINT('Ctrl Pts',(3.57053498799994,5.2,2.77743247199999));
#341263=CARTESIAN_POINT('Ctrl Pts',(3.57053498799994,2.2,2.77743247199999));
#341264=CARTESIAN_POINT('Ctrl Pts',(3.57146936999994,12.2,2.77952327099998));
#341265=CARTESIAN_POINT('Ctrl Pts',(3.57146936999994,5.2,2.77952327099998));
#341266=CARTESIAN_POINT('Ctrl Pts',(3.57146936999994,2.2,2.77952327099998));
#341267=CARTESIAN_POINT('Ctrl Pts',(3.57240302499994,12.2,2.78161849699998));
#341268=CARTESIAN_POINT('Ctrl Pts',(3.57240302499994,5.2,2.78161849699998));
#341269=CARTESIAN_POINT('Ctrl Pts',(3.57240302499994,2.2,2.78161849699998));
#341270=CARTESIAN_POINT('Ctrl Pts',(3.57333594399994,12.2,2.78371814599998));
#341271=CARTESIAN_POINT('Ctrl Pts',(3.57333594399994,5.2,2.78371814599998));
#341272=CARTESIAN_POINT('Ctrl Pts',(3.57333594399994,2.2,2.78371814599998));
#341273=CARTESIAN_POINT('Ctrl Pts',(3.57426811699994,12.2,2.78582221499998));
#341274=CARTESIAN_POINT('Ctrl Pts',(3.57426811699994,5.2,2.78582221499998));
#341275=CARTESIAN_POINT('Ctrl Pts',(3.57426811699994,2.2,2.78582221499998));
#341276=CARTESIAN_POINT('Ctrl Pts',(3.57519953599994,12.2,2.78793069999999));
#341277=CARTESIAN_POINT('Ctrl Pts',(3.57519953599994,5.2,2.78793069999999));
#341278=CARTESIAN_POINT('Ctrl Pts',(3.57519953599994,2.2,2.78793069999999));
#341279=CARTESIAN_POINT('Ctrl Pts',(3.57613019099994,12.2,2.79004359899999));
#341280=CARTESIAN_POINT('Ctrl Pts',(3.57613019099994,5.2,2.79004359899999));
#341281=CARTESIAN_POINT('Ctrl Pts',(3.57613019099994,2.2,2.79004359899999));
#341282=CARTESIAN_POINT('Ctrl Pts',(3.57706007399994,12.2,2.79216090999999));
#341283=CARTESIAN_POINT('Ctrl Pts',(3.57706007399994,5.2,2.79216090999999));
#341284=CARTESIAN_POINT('Ctrl Pts',(3.57706007399994,2.2,2.79216090999999));
#341285=CARTESIAN_POINT('Ctrl Pts',(3.57798917399994,12.2,2.79428262799998));
#341286=CARTESIAN_POINT('Ctrl Pts',(3.57798917399994,5.2,2.79428262799998));
#341287=CARTESIAN_POINT('Ctrl Pts',(3.57798917399994,2.2,2.79428262799998));
#341288=CARTESIAN_POINT('Ctrl Pts',(3.57891748399994,12.2,2.79640874799998));
#341289=CARTESIAN_POINT('Ctrl Pts',(3.57891748399994,5.2,2.79640874799998));
#341290=CARTESIAN_POINT('Ctrl Pts',(3.57891748399994,2.2,2.79640874799998));
#341291=CARTESIAN_POINT('Ctrl Pts',(3.57984499299994,12.2,2.79853926999999));
#341292=CARTESIAN_POINT('Ctrl Pts',(3.57984499299994,5.2,2.79853926999999));
#341293=CARTESIAN_POINT('Ctrl Pts',(3.57984499299994,2.2,2.79853926999999));
#341294=CARTESIAN_POINT('Ctrl Pts',(3.58077169299994,12.2,2.80067419099999));
#341295=CARTESIAN_POINT('Ctrl Pts',(3.58077169299994,5.2,2.80067419099999));
#341296=CARTESIAN_POINT('Ctrl Pts',(3.58077169299994,2.2,2.80067419099999));
#341297=CARTESIAN_POINT('Ctrl Pts',(3.58169757499994,12.2,2.80281350399999));
#341298=CARTESIAN_POINT('Ctrl Pts',(3.58169757499994,5.2,2.80281350399999));
#341299=CARTESIAN_POINT('Ctrl Pts',(3.58169757499994,2.2,2.80281350399999));
#341300=CARTESIAN_POINT('Ctrl Pts',(3.58262263099994,12.2,2.80495720899999));
#341301=CARTESIAN_POINT('Ctrl Pts',(3.58262263099994,5.2,2.80495720899999));
#341302=CARTESIAN_POINT('Ctrl Pts',(3.58262263099994,2.2,2.80495720899999));
#341303=CARTESIAN_POINT('Ctrl Pts',(3.58354684999994,12.2,2.80710530299999));
#341304=CARTESIAN_POINT('Ctrl Pts',(3.58354684999994,5.2,2.80710530299999));
#341305=CARTESIAN_POINT('Ctrl Pts',(3.58354684999994,2.2,2.80710530299999));
#341306=CARTESIAN_POINT('Ctrl Pts',(3.58447022299994,12.2,2.80925777999999));
#341307=CARTESIAN_POINT('Ctrl Pts',(3.58447022299994,5.2,2.80925777999999));
#341308=CARTESIAN_POINT('Ctrl Pts',(3.58447022299994,2.2,2.80925777999999));
#341309=CARTESIAN_POINT('Ctrl Pts',(3.58539274299994,12.2,2.81141463799998));
#341310=CARTESIAN_POINT('Ctrl Pts',(3.58539274299994,5.2,2.81141463799998));
#341311=CARTESIAN_POINT('Ctrl Pts',(3.58539274299994,2.2,2.81141463799998));
#341312=CARTESIAN_POINT('Ctrl Pts',(3.58631439899994,12.2,2.81357587599998));
#341313=CARTESIAN_POINT('Ctrl Pts',(3.58631439899994,5.2,2.81357587599998));
#341314=CARTESIAN_POINT('Ctrl Pts',(3.58631439899994,2.2,2.81357587599998));
#341315=CARTESIAN_POINT('Ctrl Pts',(3.58723518399994,12.2,2.81574148699999));
#341316=CARTESIAN_POINT('Ctrl Pts',(3.58723518399994,5.2,2.81574148699999));
#341317=CARTESIAN_POINT('Ctrl Pts',(3.58723518399994,2.2,2.81574148699999));
#341318=CARTESIAN_POINT('Ctrl Pts',(3.58815508699994,12.2,2.81791146899998));
#341319=CARTESIAN_POINT('Ctrl Pts',(3.58815508699994,5.2,2.81791146899998));
#341320=CARTESIAN_POINT('Ctrl Pts',(3.58815508699994,2.2,2.81791146899998));
#341321=CARTESIAN_POINT('Ctrl Pts',(3.58907410099994,12.2,2.82008581999998));
#341322=CARTESIAN_POINT('Ctrl Pts',(3.58907410099994,5.2,2.82008581999998));
#341323=CARTESIAN_POINT('Ctrl Pts',(3.58907410099994,2.2,2.82008581999998));
#341324=CARTESIAN_POINT('Ctrl Pts',(3.58999221499994,12.2,2.82226453499998));
#341325=CARTESIAN_POINT('Ctrl Pts',(3.58999221499994,5.2,2.82226453499998));
#341326=CARTESIAN_POINT('Ctrl Pts',(3.58999221499994,2.2,2.82226453499998));
#341327=CARTESIAN_POINT('Ctrl Pts',(3.59090942199995,12.2,2.82444761199999));
#341328=CARTESIAN_POINT('Ctrl Pts',(3.59090942199995,5.2,2.82444761199999));
#341329=CARTESIAN_POINT('Ctrl Pts',(3.59090942199995,2.2,2.82444761199999));
#341330=CARTESIAN_POINT('Ctrl Pts',(3.59182571199994,12.2,2.82663504699999));
#341331=CARTESIAN_POINT('Ctrl Pts',(3.59182571199994,5.2,2.82663504699999));
#341332=CARTESIAN_POINT('Ctrl Pts',(3.59182571199994,2.2,2.82663504699999));
#341333=CARTESIAN_POINT('Ctrl Pts',(3.59274107699994,12.2,2.82882683699999));
#341334=CARTESIAN_POINT('Ctrl Pts',(3.59274107699994,5.2,2.82882683699999));
#341335=CARTESIAN_POINT('Ctrl Pts',(3.59274107699994,2.2,2.82882683699999));
#341336=CARTESIAN_POINT('Ctrl Pts',(3.59365550899994,12.2,2.83102297799999));
#341337=CARTESIAN_POINT('Ctrl Pts',(3.59365550899994,5.2,2.83102297799999));
#341338=CARTESIAN_POINT('Ctrl Pts',(3.59365550899994,2.2,2.83102297799999));
#341339=CARTESIAN_POINT('Ctrl Pts',(3.59456899599994,12.2,2.83322346799999));
#341340=CARTESIAN_POINT('Ctrl Pts',(3.59456899599994,5.2,2.83322346799999));
#341341=CARTESIAN_POINT('Ctrl Pts',(3.59456899599994,2.2,2.83322346799999));
#341342=CARTESIAN_POINT('Ctrl Pts',(3.59548153099994,12.2,2.83542830099999));
#341343=CARTESIAN_POINT('Ctrl Pts',(3.59548153099994,5.2,2.83542830099999));
#341344=CARTESIAN_POINT('Ctrl Pts',(3.59548153099994,2.2,2.83542830099999));
#341345=CARTESIAN_POINT('Ctrl Pts',(3.59639310699994,12.2,2.83763747599998));
#341346=CARTESIAN_POINT('Ctrl Pts',(3.59639310699994,5.2,2.83763747599998));
#341347=CARTESIAN_POINT('Ctrl Pts',(3.59639310699994,2.2,2.83763747599998));
#341348=CARTESIAN_POINT('Ctrl Pts',(3.59730371299994,12.2,2.83985098799998));
#341349=CARTESIAN_POINT('Ctrl Pts',(3.59730371299994,5.2,2.83985098799998));
#341350=CARTESIAN_POINT('Ctrl Pts',(3.59730371299994,2.2,2.83985098799998));
#341351=CARTESIAN_POINT('Ctrl Pts',(3.59821333999994,12.2,2.84206883599998));
#341352=CARTESIAN_POINT('Ctrl Pts',(3.59821333999994,5.2,2.84206883599998));
#341353=CARTESIAN_POINT('Ctrl Pts',(3.59821333999994,2.2,2.84206883599998));
#341354=CARTESIAN_POINT('Ctrl Pts',(3.59912197999994,12.2,2.84429101499998));
#341355=CARTESIAN_POINT('Ctrl Pts',(3.59912197999994,5.2,2.84429101499998));
#341356=CARTESIAN_POINT('Ctrl Pts',(3.59912197999994,2.2,2.84429101499998));
#341357=CARTESIAN_POINT('Ctrl Pts',(3.60002962499994,12.2,2.84651751999998));
#341358=CARTESIAN_POINT('Ctrl Pts',(3.60002962499994,5.2,2.84651751999998));
#341359=CARTESIAN_POINT('Ctrl Pts',(3.60002962499994,2.2,2.84651751999998));
#341360=CARTESIAN_POINT('Ctrl Pts',(3.60093626599994,12.2,2.84874835199999));
#341361=CARTESIAN_POINT('Ctrl Pts',(3.60093626599994,5.2,2.84874835199999));
#341362=CARTESIAN_POINT('Ctrl Pts',(3.60093626599994,2.2,2.84874835199999));
#341363=CARTESIAN_POINT('Ctrl Pts',(3.60184189399994,12.2,2.85098350199998));
#341364=CARTESIAN_POINT('Ctrl Pts',(3.60184189399994,5.2,2.85098350199998));
#341365=CARTESIAN_POINT('Ctrl Pts',(3.60184189399994,2.2,2.85098350199998));
#341366=CARTESIAN_POINT('Ctrl Pts',(3.60274650099994,12.2,2.85322297199999));
#341367=CARTESIAN_POINT('Ctrl Pts',(3.60274650099994,5.2,2.85322297199999));
#341368=CARTESIAN_POINT('Ctrl Pts',(3.60274650099994,2.2,2.85322297199999));
#341369=CARTESIAN_POINT('Ctrl Pts',(3.60365007599994,12.2,2.85546675399999));
#341370=CARTESIAN_POINT('Ctrl Pts',(3.60365007599994,5.2,2.85546675399999));
#341371=CARTESIAN_POINT('Ctrl Pts',(3.60365007599994,2.2,2.85546675399999));
#341372=CARTESIAN_POINT('Ctrl Pts',(3.60455261199994,12.2,2.85771484799999));
#341373=CARTESIAN_POINT('Ctrl Pts',(3.60455261199994,5.2,2.85771484799999));
#341374=CARTESIAN_POINT('Ctrl Pts',(3.60455261199994,2.2,2.85771484799999));
#341375=CARTESIAN_POINT('Ctrl Pts',(3.60545410099994,12.2,2.85996724799999));
#341376=CARTESIAN_POINT('Ctrl Pts',(3.60545410099994,5.2,2.85996724799999));
#341377=CARTESIAN_POINT('Ctrl Pts',(3.60545410099994,2.2,2.85996724799999));
#341378=CARTESIAN_POINT('Ctrl Pts',(3.60635453499994,12.2,2.86222395299998));
#341379=CARTESIAN_POINT('Ctrl Pts',(3.60635453499994,5.2,2.86222395299998));
#341380=CARTESIAN_POINT('Ctrl Pts',(3.60635453499994,2.2,2.86222395299998));
#341381=CARTESIAN_POINT('Ctrl Pts',(3.60725390299994,12.2,2.86448495699998));
#341382=CARTESIAN_POINT('Ctrl Pts',(3.60725390299994,5.2,2.86448495699998));
#341383=CARTESIAN_POINT('Ctrl Pts',(3.60725390299994,2.2,2.86448495699998));
#341384=CARTESIAN_POINT('Ctrl Pts',(3.60815219799994,12.2,2.86675025799998));
#341385=CARTESIAN_POINT('Ctrl Pts',(3.60815219799994,5.2,2.86675025799998));
#341386=CARTESIAN_POINT('Ctrl Pts',(3.60815219799994,2.2,2.86675025799998));
#341387=CARTESIAN_POINT('Ctrl Pts',(3.60904941099994,12.2,2.86901985299998));
#341388=CARTESIAN_POINT('Ctrl Pts',(3.60904941099994,5.2,2.86901985299998));
#341389=CARTESIAN_POINT('Ctrl Pts',(3.60904941099994,2.2,2.86901985299998));
#341390=CARTESIAN_POINT('Ctrl Pts',(3.60994553399994,12.2,2.87129373699998));
#341391=CARTESIAN_POINT('Ctrl Pts',(3.60994553399994,5.2,2.87129373699998));
#341392=CARTESIAN_POINT('Ctrl Pts',(3.60994553399994,2.2,2.87129373699998));
#341393=CARTESIAN_POINT('Ctrl Pts',(3.61084055699994,12.2,2.87357190699999));
#341394=CARTESIAN_POINT('Ctrl Pts',(3.61084055699994,5.2,2.87357190699999));
#341395=CARTESIAN_POINT('Ctrl Pts',(3.61084055699994,2.2,2.87357190699999));
#341396=CARTESIAN_POINT('Ctrl Pts',(3.61173447299994,12.2,2.87585435999999));
#341397=CARTESIAN_POINT('Ctrl Pts',(3.61173447299994,5.2,2.87585435999999));
#341398=CARTESIAN_POINT('Ctrl Pts',(3.61173447299994,2.2,2.87585435999999));
#341399=CARTESIAN_POINT('Ctrl Pts',(3.61262727299994,12.2,2.87814109199999));
#341400=CARTESIAN_POINT('Ctrl Pts',(3.61262727299994,5.2,2.87814109199999));
#341401=CARTESIAN_POINT('Ctrl Pts',(3.61262727299994,2.2,2.87814109199999));
#341402=CARTESIAN_POINT('Ctrl Pts',(3.61351894799994,12.2,2.88043210099998));
#341403=CARTESIAN_POINT('Ctrl Pts',(3.61351894799994,5.2,2.88043210099998));
#341404=CARTESIAN_POINT('Ctrl Pts',(3.61351894799994,2.2,2.88043210099998));
#341405=CARTESIAN_POINT('Ctrl Pts',(3.61440949099994,12.2,2.88272738199999));
#341406=CARTESIAN_POINT('Ctrl Pts',(3.61440949099994,5.2,2.88272738199999));
#341407=CARTESIAN_POINT('Ctrl Pts',(3.61440949099994,2.2,2.88272738199999));
#341408=CARTESIAN_POINT('Ctrl Pts',(3.61529889299994,12.2,2.88502693099999));
#341409=CARTESIAN_POINT('Ctrl Pts',(3.61529889299994,5.2,2.88502693099999));
#341410=CARTESIAN_POINT('Ctrl Pts',(3.61529889299994,2.2,2.88502693099999));
#341411=CARTESIAN_POINT('Ctrl Pts',(3.61618714399994,12.2,2.88733074599998));
#341412=CARTESIAN_POINT('Ctrl Pts',(3.61618714399994,5.2,2.88733074599998));
#341413=CARTESIAN_POINT('Ctrl Pts',(3.61618714399994,2.2,2.88733074599998));
#341414=CARTESIAN_POINT('Ctrl Pts',(3.61707423799994,12.2,2.88963882199998));
#341415=CARTESIAN_POINT('Ctrl Pts',(3.61707423799994,5.2,2.88963882199998));
#341416=CARTESIAN_POINT('Ctrl Pts',(3.61707423799994,2.2,2.88963882199998));
#341417=CARTESIAN_POINT('Ctrl Pts',(3.61796016399994,12.2,2.89195115599998));
#341418=CARTESIAN_POINT('Ctrl Pts',(3.61796016399994,5.2,2.89195115599998));
#341419=CARTESIAN_POINT('Ctrl Pts',(3.61796016399994,2.2,2.89195115599998));
#341420=CARTESIAN_POINT('Ctrl Pts',(3.61884491599994,12.2,2.89426774499999));
#341421=CARTESIAN_POINT('Ctrl Pts',(3.61884491599994,5.2,2.89426774499999));
#341422=CARTESIAN_POINT('Ctrl Pts',(3.61884491599994,2.2,2.89426774499999));
#341423=CARTESIAN_POINT('Ctrl Pts',(3.61972848299994,12.2,2.89658858399999));
#341424=CARTESIAN_POINT('Ctrl Pts',(3.61972848299994,5.2,2.89658858399999));
#341425=CARTESIAN_POINT('Ctrl Pts',(3.61972848299994,2.2,2.89658858399999));
#341426=CARTESIAN_POINT('Ctrl Pts',(3.62061085999994,12.2,2.89891367199999));
#341427=CARTESIAN_POINT('Ctrl Pts',(3.62061085999994,5.2,2.89891367199999));
#341428=CARTESIAN_POINT('Ctrl Pts',(3.62061085999994,2.2,2.89891367199999));
#341429=CARTESIAN_POINT('Ctrl Pts',(3.62149203599994,12.2,2.90124300299999));
#341430=CARTESIAN_POINT('Ctrl Pts',(3.62149203599994,5.2,2.90124300299999));
#341431=CARTESIAN_POINT('Ctrl Pts',(3.62149203599994,2.2,2.90124300299999));
#341432=CARTESIAN_POINT('Ctrl Pts',(3.62237200399994,12.2,2.90357657399999));
#341433=CARTESIAN_POINT('Ctrl Pts',(3.62237200399994,5.2,2.90357657399999));
#341434=CARTESIAN_POINT('Ctrl Pts',(3.62237200399994,2.2,2.90357657399999));
#341435=CARTESIAN_POINT('Ctrl Pts',(3.62325075499994,12.2,2.90591438199999));
#341436=CARTESIAN_POINT('Ctrl Pts',(3.62325075499994,5.2,2.90591438199999));
#341437=CARTESIAN_POINT('Ctrl Pts',(3.62325075499994,2.2,2.90591438199999));
#341438=CARTESIAN_POINT('Ctrl Pts',(3.62412828099994,12.2,2.90825642199999));
#341439=CARTESIAN_POINT('Ctrl Pts',(3.62412828099994,5.2,2.90825642199999));
#341440=CARTESIAN_POINT('Ctrl Pts',(3.62412828099994,2.2,2.90825642199999));
#341441=CARTESIAN_POINT('Ctrl Pts',(3.62500457299994,12.2,2.91060269299999));
#341442=CARTESIAN_POINT('Ctrl Pts',(3.62500457299994,5.2,2.91060269299999));
#341443=CARTESIAN_POINT('Ctrl Pts',(3.62500457299994,2.2,2.91060269299999));
#341444=CARTESIAN_POINT('Ctrl Pts',(3.62587962499994,12.2,2.91295318899999));
#341445=CARTESIAN_POINT('Ctrl Pts',(3.62587962499994,5.2,2.91295318899999));
#341446=CARTESIAN_POINT('Ctrl Pts',(3.62587962499994,2.2,2.91295318899999));
#341447=CARTESIAN_POINT('Ctrl Pts',(3.62675342599994,12.2,2.91530790699999));
#341448=CARTESIAN_POINT('Ctrl Pts',(3.62675342599994,5.2,2.91530790699999));
#341449=CARTESIAN_POINT('Ctrl Pts',(3.62675342599994,2.2,2.91530790699999));
#341450=CARTESIAN_POINT('Ctrl Pts',(3.62762596899994,12.2,2.91766684499999));
#341451=CARTESIAN_POINT('Ctrl Pts',(3.62762596899994,5.2,2.91766684499999));
#341452=CARTESIAN_POINT('Ctrl Pts',(3.62762596899994,2.2,2.91766684499999));
#341453=CARTESIAN_POINT('Ctrl Pts',(3.62849724599994,12.2,2.92002999699999));
#341454=CARTESIAN_POINT('Ctrl Pts',(3.62849724599994,5.2,2.92002999699999));
#341455=CARTESIAN_POINT('Ctrl Pts',(3.62849724599994,2.2,2.92002999699999));
#341456=CARTESIAN_POINT('Ctrl Pts',(3.62936724899994,12.2,2.92239736099998));
#341457=CARTESIAN_POINT('Ctrl Pts',(3.62936724899994,5.2,2.92239736099998));
#341458=CARTESIAN_POINT('Ctrl Pts',(3.62936724899994,2.2,2.92239736099998));
#341459=CARTESIAN_POINT('Ctrl Pts',(3.63023596899994,12.2,2.92476893199999));
#341460=CARTESIAN_POINT('Ctrl Pts',(3.63023596899994,5.2,2.92476893199999));
#341461=CARTESIAN_POINT('Ctrl Pts',(3.63023596899994,2.2,2.92476893199999));
#341462=CARTESIAN_POINT('Ctrl Pts',(3.63110339699994,12.2,2.92714470699998));
#341463=CARTESIAN_POINT('Ctrl Pts',(3.63110339699994,5.2,2.92714470699998));
#341464=CARTESIAN_POINT('Ctrl Pts',(3.63110339699994,2.2,2.92714470699998));
#341465=CARTESIAN_POINT('Ctrl Pts',(3.63196952799994,12.2,2.92952468299998));
#341466=CARTESIAN_POINT('Ctrl Pts',(3.63196952799994,5.2,2.92952468299998));
#341467=CARTESIAN_POINT('Ctrl Pts',(3.63196952799994,2.2,2.92952468299998));
#341468=CARTESIAN_POINT('Ctrl Pts',(3.63283434999994,12.2,2.93190885499998));
#341469=CARTESIAN_POINT('Ctrl Pts',(3.63283434999994,5.2,2.93190885499998));
#341470=CARTESIAN_POINT('Ctrl Pts',(3.63283434999994,2.2,2.93190885499998));
#341471=CARTESIAN_POINT('Ctrl Pts',(3.63369785799994,12.2,2.93429721999999));
#341472=CARTESIAN_POINT('Ctrl Pts',(3.63369785799994,5.2,2.93429721999999));
#341473=CARTESIAN_POINT('Ctrl Pts',(3.63369785799994,2.2,2.93429721999999));
#341474=CARTESIAN_POINT('Ctrl Pts',(3.63456004199994,12.2,2.93668977499999));
#341475=CARTESIAN_POINT('Ctrl Pts',(3.63456004199994,5.2,2.93668977499999));
#341476=CARTESIAN_POINT('Ctrl Pts',(3.63456004199994,2.2,2.93668977499999));
#341477=CARTESIAN_POINT('Ctrl Pts',(3.63542089399994,12.2,2.93908651499999));
#341478=CARTESIAN_POINT('Ctrl Pts',(3.63542089399994,5.2,2.93908651499999));
#341479=CARTESIAN_POINT('Ctrl Pts',(3.63542089399994,2.2,2.93908651499999));
#341480=CARTESIAN_POINT('Ctrl Pts',(3.63628040899994,12.2,2.94148743699999));
#341481=CARTESIAN_POINT('Ctrl Pts',(3.63628040899994,5.2,2.94148743699999));
#341482=CARTESIAN_POINT('Ctrl Pts',(3.63628040899994,2.2,2.94148743699999));
#341483=CARTESIAN_POINT('Ctrl Pts',(3.63713857299994,12.2,2.94389253799999));
#341484=CARTESIAN_POINT('Ctrl Pts',(3.63713857299994,5.2,2.94389253799999));
#341485=CARTESIAN_POINT('Ctrl Pts',(3.63713857299994,2.2,2.94389253799999));
#341486=CARTESIAN_POINT('Ctrl Pts',(3.63799538399994,12.2,2.94630181399998));
#341487=CARTESIAN_POINT('Ctrl Pts',(3.63799538399994,5.2,2.94630181399998));
#341488=CARTESIAN_POINT('Ctrl Pts',(3.63799538399994,2.2,2.94630181399998));
#341489=CARTESIAN_POINT('Ctrl Pts',(3.63885082999994,12.2,2.94871525999999));
#341490=CARTESIAN_POINT('Ctrl Pts',(3.63885082999994,5.2,2.94871525999999));
#341491=CARTESIAN_POINT('Ctrl Pts',(3.63885082999994,2.2,2.94871525999999));
#341492=CARTESIAN_POINT('Ctrl Pts',(3.63970490299994,12.2,2.95113287299999));
#341493=CARTESIAN_POINT('Ctrl Pts',(3.63970490299994,5.2,2.95113287299999));
#341494=CARTESIAN_POINT('Ctrl Pts',(3.63970490299994,2.2,2.95113287299999));
#341495=CARTESIAN_POINT('Ctrl Pts',(3.64055759799994,12.2,2.95355464999999));
#341496=CARTESIAN_POINT('Ctrl Pts',(3.64055759799994,5.2,2.95355464999999));
#341497=CARTESIAN_POINT('Ctrl Pts',(3.64055759799994,2.2,2.95355464999999));
#341498=CARTESIAN_POINT('Ctrl Pts',(3.64140890399994,12.2,2.95598058599998));
#341499=CARTESIAN_POINT('Ctrl Pts',(3.64140890399994,5.2,2.95598058599998));
#341500=CARTESIAN_POINT('Ctrl Pts',(3.64140890399994,2.2,2.95598058599998));
#341501=CARTESIAN_POINT('Ctrl Pts',(3.64225881399994,12.2,2.95841067899998));
#341502=CARTESIAN_POINT('Ctrl Pts',(3.64225881399994,5.2,2.95841067899998));
#341503=CARTESIAN_POINT('Ctrl Pts',(3.64225881399994,2.2,2.95841067899998));
#341504=CARTESIAN_POINT('Ctrl Pts',(3.64310732199994,12.2,2.96084492299999));
#341505=CARTESIAN_POINT('Ctrl Pts',(3.64310732199994,5.2,2.96084492299999));
#341506=CARTESIAN_POINT('Ctrl Pts',(3.64310732199994,2.2,2.96084492299999));
#341507=CARTESIAN_POINT('Ctrl Pts',(3.64395441699994,12.2,2.96328331599998));
#341508=CARTESIAN_POINT('Ctrl Pts',(3.64395441699994,5.2,2.96328331599998));
#341509=CARTESIAN_POINT('Ctrl Pts',(3.64395441699994,2.2,2.96328331599998));
#341510=CARTESIAN_POINT('Ctrl Pts',(3.64480009299994,12.2,2.96572585499998));
#341511=CARTESIAN_POINT('Ctrl Pts',(3.64480009299994,5.2,2.96572585499998));
#341512=CARTESIAN_POINT('Ctrl Pts',(3.64480009299994,2.2,2.96572585499998));
#341513=CARTESIAN_POINT('Ctrl Pts',(3.64564434199994,12.2,2.96817253399999));
#341514=CARTESIAN_POINT('Ctrl Pts',(3.64564434199994,5.2,2.96817253399999));
#341515=CARTESIAN_POINT('Ctrl Pts',(3.64564434199994,2.2,2.96817253399999));
#341516=CARTESIAN_POINT('Ctrl Pts',(3.64648715699994,12.2,2.97062334999998));
#341517=CARTESIAN_POINT('Ctrl Pts',(3.64648715699994,5.2,2.97062334999998));
#341518=CARTESIAN_POINT('Ctrl Pts',(3.64648715699994,2.2,2.97062334999998));
#341519=CARTESIAN_POINT('Ctrl Pts',(3.64732852699994,12.2,2.97307830099999));
#341520=CARTESIAN_POINT('Ctrl Pts',(3.64732852699994,5.2,2.97307830099999));
#341521=CARTESIAN_POINT('Ctrl Pts',(3.64732852699994,2.2,2.97307830099999));
#341522=CARTESIAN_POINT('Ctrl Pts',(3.64816844599994,12.2,2.97553737999999));
#341523=CARTESIAN_POINT('Ctrl Pts',(3.64816844599994,5.2,2.97553737999999));
#341524=CARTESIAN_POINT('Ctrl Pts',(3.64816844599994,2.2,2.97553737999999));
#341525=CARTESIAN_POINT('Ctrl Pts',(3.64900690399994,12.2,2.97800058399999));
#341526=CARTESIAN_POINT('Ctrl Pts',(3.64900690399994,5.2,2.97800058399999));
#341527=CARTESIAN_POINT('Ctrl Pts',(3.64900690399994,2.2,2.97800058399999));
#341528=CARTESIAN_POINT('Ctrl Pts',(3.64984389599994,12.2,2.98046791099999));
#341529=CARTESIAN_POINT('Ctrl Pts',(3.64984389599994,5.2,2.98046791099999));
#341530=CARTESIAN_POINT('Ctrl Pts',(3.64984389599994,2.2,2.98046791099999));
#341531=CARTESIAN_POINT('Ctrl Pts',(3.65067941099994,12.2,2.98293935599999));
#341532=CARTESIAN_POINT('Ctrl Pts',(3.65067941099994,5.2,2.98293935599999));
#341533=CARTESIAN_POINT('Ctrl Pts',(3.65067941099994,2.2,2.98293935599999));
#341534=CARTESIAN_POINT('Ctrl Pts',(3.65151344299994,12.2,2.98541491399998));
#341535=CARTESIAN_POINT('Ctrl Pts',(3.65151344299994,5.2,2.98541491399998));
#341536=CARTESIAN_POINT('Ctrl Pts',(3.65151344299994,2.2,2.98541491399998));
#341537=CARTESIAN_POINT('Ctrl Pts',(3.65234598699994,12.2,2.98789458399998));
#341538=CARTESIAN_POINT('Ctrl Pts',(3.65234598699994,5.2,2.98789458399998));
#341539=CARTESIAN_POINT('Ctrl Pts',(3.65234598699994,2.2,2.98789458399998));
#341540=CARTESIAN_POINT('Ctrl Pts',(3.65317703299994,12.2,2.99037836199999));
#341541=CARTESIAN_POINT('Ctrl Pts',(3.65317703299994,5.2,2.99037836199999));
#341542=CARTESIAN_POINT('Ctrl Pts',(3.65317703299994,2.2,2.99037836199999));
#341543=CARTESIAN_POINT('Ctrl Pts',(3.65400657599994,12.2,2.99286624399999));
#341544=CARTESIAN_POINT('Ctrl Pts',(3.65400657599994,5.2,2.99286624399999));
#341545=CARTESIAN_POINT('Ctrl Pts',(3.65400657599994,2.2,2.99286624399999));
#341546=CARTESIAN_POINT('Ctrl Pts',(3.65483460699994,12.2,2.99535822499998));
#341547=CARTESIAN_POINT('Ctrl Pts',(3.65483460699994,5.2,2.99535822499998));
#341548=CARTESIAN_POINT('Ctrl Pts',(3.65483460699994,2.2,2.99535822499998));
#341549=CARTESIAN_POINT('Ctrl Pts',(3.65566111799994,12.2,2.99785430299998));
#341550=CARTESIAN_POINT('Ctrl Pts',(3.65566111799994,5.2,2.99785430299998));
#341551=CARTESIAN_POINT('Ctrl Pts',(3.65566111799994,2.2,2.99785430299998));
#341552=CARTESIAN_POINT('Ctrl Pts',(3.65648609799994,12.2,3.00035447199999));
#341553=CARTESIAN_POINT('Ctrl Pts',(3.65648609799994,5.2,3.00035447199999));
#341554=CARTESIAN_POINT('Ctrl Pts',(3.65648609799994,2.2,3.00035447199999));
#341555=CARTESIAN_POINT('Ctrl Pts',(3.65730953999994,12.2,3.00285872699998));
#341556=CARTESIAN_POINT('Ctrl Pts',(3.65730953999994,5.2,3.00285872699998));
#341557=CARTESIAN_POINT('Ctrl Pts',(3.65730953999994,2.2,3.00285872699998));
#341558=CARTESIAN_POINT('Ctrl Pts',(3.65813143199994,12.2,3.00536706399999));
#341559=CARTESIAN_POINT('Ctrl Pts',(3.65813143199994,5.2,3.00536706399999));
#341560=CARTESIAN_POINT('Ctrl Pts',(3.65813143199994,2.2,3.00536706399999));
#341561=CARTESIAN_POINT('Ctrl Pts',(3.65895176799994,12.2,3.00787947899998));
#341562=CARTESIAN_POINT('Ctrl Pts',(3.65895176799994,5.2,3.00787947899998));
#341563=CARTESIAN_POINT('Ctrl Pts',(3.65895176799994,2.2,3.00787947899998));
#341564=CARTESIAN_POINT('Ctrl Pts',(3.65977053899994,12.2,3.01039596699999));
#341565=CARTESIAN_POINT('Ctrl Pts',(3.65977053899994,5.2,3.01039596699999));
#341566=CARTESIAN_POINT('Ctrl Pts',(3.65977053899994,2.2,3.01039596699999));
#341567=CARTESIAN_POINT('Ctrl Pts',(3.66058773799994,12.2,3.01291652599998));
#341568=CARTESIAN_POINT('Ctrl Pts',(3.66058773799994,5.2,3.01291652599998));
#341569=CARTESIAN_POINT('Ctrl Pts',(3.66058773799994,2.2,3.01291652599998));
#341570=CARTESIAN_POINT('Ctrl Pts',(3.66140336299994,12.2,3.01544115399999));
#341571=CARTESIAN_POINT('Ctrl Pts',(3.66140336299994,5.2,3.01544115399999));
#341572=CARTESIAN_POINT('Ctrl Pts',(3.66140336299994,2.2,3.01544115399999));
#341573=CARTESIAN_POINT('Ctrl Pts',(3.66221741303907,12.2,3.01796985012154));
#341574=CARTESIAN_POINT('Ctrl Pts',(3.66221741303907,5.2,3.01796985012154));
#341575=CARTESIAN_POINT('Ctrl Pts',(3.66221741303907,2.2,3.01796985012154));
#341576=CARTESIAN_POINT('Ctrl Pts',(3.66286739107805,12.2,3.01999606024348));
#341577=CARTESIAN_POINT('Ctrl Pts',(3.66286739107805,5.2,3.01999606024348));
#341578=CARTESIAN_POINT('Ctrl Pts',(3.66286739107805,2.2,3.01999606024348));
#341579=CARTESIAN_POINT('Ctrl Pts',(3.66335416511694,12.2,3.02151754936566));
#341580=CARTESIAN_POINT('Ctrl Pts',(3.66335416511694,5.2,3.02151754936566));
#341581=CARTESIAN_POINT('Ctrl Pts',(3.66335416511694,2.2,3.02151754936566));
#341582=CARTESIAN_POINT('Ctrl Pts',(3.66367836615578,12.2,3.02253268748795));
#341583=CARTESIAN_POINT('Ctrl Pts',(3.66367836615578,5.2,3.02253268748795));
#341584=CARTESIAN_POINT('Ctrl Pts',(3.66367836615578,2.2,3.02253268748795));
#341585=CARTESIAN_POINT('Ctrl Pts',(3.66384038699994,12.2,3.02304045999998));
#341586=CARTESIAN_POINT('Ctrl Pts',(3.66384038699994,5.2,3.02304045999998));
#341587=CARTESIAN_POINT('Ctrl Pts',(3.66384038699994,2.2,3.02304045999998));
#341588=CARTESIAN_POINT('Origin',(-5.66300478732629E-14,15.2,-1.77635683940025E-14));
#341589=CARTESIAN_POINT('',(3.24327759199994,2.2,1.61918975399999));
#341590=CARTESIAN_POINT('Origin',(3.57314678299994,15.2,1.78387526099999));
#341591=CARTESIAN_POINT('',(3.57319269599994,12.2,1.78389818299999));
#341592=CARTESIAN_POINT('Ctrl Pts',(4.39111701799995,12.2,1.81124027399999));
#341593=CARTESIAN_POINT('Ctrl Pts',(4.39111701799995,5.2,1.81124027399999));
#341594=CARTESIAN_POINT('Ctrl Pts',(4.39111701799995,2.2,1.81124027399999));
#341595=CARTESIAN_POINT('Ctrl Pts',(4.39059271499994,12.2,1.81133614099998));
#341596=CARTESIAN_POINT('Ctrl Pts',(4.39059271499994,5.2,1.81133614099998));
#341597=CARTESIAN_POINT('Ctrl Pts',(4.39059271499994,2.2,1.81133614099998));
#341598=CARTESIAN_POINT('Ctrl Pts',(4.38954439399994,12.2,1.81152754399998));
#341599=CARTESIAN_POINT('Ctrl Pts',(4.38954439399994,5.2,1.81152754399998));
#341600=CARTESIAN_POINT('Ctrl Pts',(4.38954439399994,2.2,1.81152754399998));
#341601=CARTESIAN_POINT('Ctrl Pts',(4.38797276699994,12.2,1.81181365699999));
#341602=CARTESIAN_POINT('Ctrl Pts',(4.38797276699994,5.2,1.81181365699999));
#341603=CARTESIAN_POINT('Ctrl Pts',(4.38797276699994,2.2,1.81181365699999));
#341604=CARTESIAN_POINT('Ctrl Pts',(4.38587897099994,12.2,1.81219315899999));
#341605=CARTESIAN_POINT('Ctrl Pts',(4.38587897099994,5.2,1.81219315899999));
#341606=CARTESIAN_POINT('Ctrl Pts',(4.38587897099994,2.2,1.81219315899999));
#341607=CARTESIAN_POINT('Ctrl Pts',(4.38326457499994,12.2,1.81266423099999));
#341608=CARTESIAN_POINT('Ctrl Pts',(4.38326457499994,5.2,1.81266423099999));
#341609=CARTESIAN_POINT('Ctrl Pts',(4.38326457499994,2.2,1.81266423099999));
#341610=CARTESIAN_POINT('Ctrl Pts',(4.38065302599994,12.2,1.81313199799999));
#341611=CARTESIAN_POINT('Ctrl Pts',(4.38065302599994,5.2,1.81313199799999));
#341612=CARTESIAN_POINT('Ctrl Pts',(4.38065302599994,2.2,1.81313199799999));
#341613=CARTESIAN_POINT('Ctrl Pts',(4.37804432799994,12.2,1.81359646299999));
#341614=CARTESIAN_POINT('Ctrl Pts',(4.37804432799994,5.2,1.81359646299999));
#341615=CARTESIAN_POINT('Ctrl Pts',(4.37804432799994,2.2,1.81359646299999));
#341616=CARTESIAN_POINT('Ctrl Pts',(4.37543848299994,12.2,1.81405762699999));
#341617=CARTESIAN_POINT('Ctrl Pts',(4.37543848299994,5.2,1.81405762699999));
#341618=CARTESIAN_POINT('Ctrl Pts',(4.37543848299994,2.2,1.81405762699999));
#341619=CARTESIAN_POINT('Ctrl Pts',(4.37283549799994,12.2,1.81451549399998));
#341620=CARTESIAN_POINT('Ctrl Pts',(4.37283549799994,5.2,1.81451549399998));
#341621=CARTESIAN_POINT('Ctrl Pts',(4.37283549799994,2.2,1.81451549399998));
#341622=CARTESIAN_POINT('Ctrl Pts',(4.37023537799995,12.2,1.81497006899999));
#341623=CARTESIAN_POINT('Ctrl Pts',(4.37023537799995,5.2,1.81497006899999));
#341624=CARTESIAN_POINT('Ctrl Pts',(4.37023537799995,2.2,1.81497006899999));
#341625=CARTESIAN_POINT('Ctrl Pts',(4.36763813199994,12.2,1.81542135599999));
#341626=CARTESIAN_POINT('Ctrl Pts',(4.36763813199994,5.2,1.81542135599999));
#341627=CARTESIAN_POINT('Ctrl Pts',(4.36763813199994,2.2,1.81542135599999));
#341628=CARTESIAN_POINT('Ctrl Pts',(4.36504376699994,12.2,1.81586936299999));
#341629=CARTESIAN_POINT('Ctrl Pts',(4.36504376699994,5.2,1.81586936299999));
#341630=CARTESIAN_POINT('Ctrl Pts',(4.36504376699994,2.2,1.81586936299999));
#341631=CARTESIAN_POINT('Ctrl Pts',(4.36245229199994,12.2,1.81631409599999));
#341632=CARTESIAN_POINT('Ctrl Pts',(4.36245229199994,5.2,1.81631409599999));
#341633=CARTESIAN_POINT('Ctrl Pts',(4.36245229199994,2.2,1.81631409599999));
#341634=CARTESIAN_POINT('Ctrl Pts',(4.35986371899994,12.2,1.81675555999998));
#341635=CARTESIAN_POINT('Ctrl Pts',(4.35986371899994,5.2,1.81675555999998));
#341636=CARTESIAN_POINT('Ctrl Pts',(4.35986371899994,2.2,1.81675555999998));
#341637=CARTESIAN_POINT('Ctrl Pts',(4.35727805099994,12.2,1.81719376199998));
#341638=CARTESIAN_POINT('Ctrl Pts',(4.35727805099994,5.2,1.81719376199998));
#341639=CARTESIAN_POINT('Ctrl Pts',(4.35727805099994,2.2,1.81719376199998));
#341640=CARTESIAN_POINT('Ctrl Pts',(4.35469529799995,12.2,1.81762870599998));
#341641=CARTESIAN_POINT('Ctrl Pts',(4.35469529799995,5.2,1.81762870599998));
#341642=CARTESIAN_POINT('Ctrl Pts',(4.35469529799995,2.2,1.81762870599998));
#341643=CARTESIAN_POINT('Ctrl Pts',(4.35211546599994,12.2,1.81806039799998));
#341644=CARTESIAN_POINT('Ctrl Pts',(4.35211546599994,5.2,1.81806039799998));
#341645=CARTESIAN_POINT('Ctrl Pts',(4.35211546599994,2.2,1.81806039799998));
#341646=CARTESIAN_POINT('Ctrl Pts',(4.34953856099995,12.2,1.81848884099999));
#341647=CARTESIAN_POINT('Ctrl Pts',(4.34953856099995,5.2,1.81848884099999));
#341648=CARTESIAN_POINT('Ctrl Pts',(4.34953856099995,2.2,1.81848884099999));
#341649=CARTESIAN_POINT('Ctrl Pts',(4.34696458899994,12.2,1.81891403999999));
#341650=CARTESIAN_POINT('Ctrl Pts',(4.34696458899994,5.2,1.81891403999999));
#341651=CARTESIAN_POINT('Ctrl Pts',(4.34696458899994,2.2,1.81891403999999));
#341652=CARTESIAN_POINT('Ctrl Pts',(4.34439355799995,12.2,1.81933599999998));
#341653=CARTESIAN_POINT('Ctrl Pts',(4.34439355799995,5.2,1.81933599999998));
#341654=CARTESIAN_POINT('Ctrl Pts',(4.34439355799995,2.2,1.81933599999998));
#341655=CARTESIAN_POINT('Ctrl Pts',(4.34182547399994,12.2,1.81975472699999));
#341656=CARTESIAN_POINT('Ctrl Pts',(4.34182547399994,5.2,1.81975472699999));
#341657=CARTESIAN_POINT('Ctrl Pts',(4.34182547399994,2.2,1.81975472699999));
#341658=CARTESIAN_POINT('Ctrl Pts',(4.33926034299995,12.2,1.82017022399998));
#341659=CARTESIAN_POINT('Ctrl Pts',(4.33926034299995,5.2,1.82017022399998));
#341660=CARTESIAN_POINT('Ctrl Pts',(4.33926034299995,2.2,1.82017022399998));
#341661=CARTESIAN_POINT('Ctrl Pts',(4.33669817299995,12.2,1.82058249799999));
#341662=CARTESIAN_POINT('Ctrl Pts',(4.33669817299995,5.2,1.82058249799999));
#341663=CARTESIAN_POINT('Ctrl Pts',(4.33669817299995,2.2,1.82058249799999));
#341664=CARTESIAN_POINT('Ctrl Pts',(4.33413897099994,12.2,1.82099155399999));
#341665=CARTESIAN_POINT('Ctrl Pts',(4.33413897099994,5.2,1.82099155399999));
#341666=CARTESIAN_POINT('Ctrl Pts',(4.33413897099994,2.2,1.82099155399999));
#341667=CARTESIAN_POINT('Ctrl Pts',(4.33158274699994,12.2,1.82139739699998));
#341668=CARTESIAN_POINT('Ctrl Pts',(4.33158274699994,5.2,1.82139739699998));
#341669=CARTESIAN_POINT('Ctrl Pts',(4.33158274699994,2.2,1.82139739699998));
#341670=CARTESIAN_POINT('Ctrl Pts',(4.32902950299995,12.2,1.82180003299999));
#341671=CARTESIAN_POINT('Ctrl Pts',(4.32902950299995,5.2,1.82180003299999));
#341672=CARTESIAN_POINT('Ctrl Pts',(4.32902950299995,2.2,1.82180003299999));
#341673=CARTESIAN_POINT('Ctrl Pts',(4.32647925199994,12.2,1.82219946699998));
#341674=CARTESIAN_POINT('Ctrl Pts',(4.32647925199994,5.2,1.82219946699998));
#341675=CARTESIAN_POINT('Ctrl Pts',(4.32647925199994,2.2,1.82219946699998));
#341676=CARTESIAN_POINT('Ctrl Pts',(4.32393199699994,12.2,1.82259570299999));
#341677=CARTESIAN_POINT('Ctrl Pts',(4.32393199699994,5.2,1.82259570299999));
#341678=CARTESIAN_POINT('Ctrl Pts',(4.32393199699994,2.2,1.82259570299999));
#341679=CARTESIAN_POINT('Ctrl Pts',(4.32138774599994,12.2,1.82298874899999));
#341680=CARTESIAN_POINT('Ctrl Pts',(4.32138774599994,5.2,1.82298874899999));
#341681=CARTESIAN_POINT('Ctrl Pts',(4.32138774599994,2.2,1.82298874899999));
#341682=CARTESIAN_POINT('Ctrl Pts',(4.31884650699994,12.2,1.82337860699999));
#341683=CARTESIAN_POINT('Ctrl Pts',(4.31884650699994,5.2,1.82337860699999));
#341684=CARTESIAN_POINT('Ctrl Pts',(4.31884650699994,2.2,1.82337860699999));
#341685=CARTESIAN_POINT('Ctrl Pts',(4.31630828499994,12.2,1.82376528399999));
#341686=CARTESIAN_POINT('Ctrl Pts',(4.31630828499994,5.2,1.82376528399999));
#341687=CARTESIAN_POINT('Ctrl Pts',(4.31630828499994,2.2,1.82376528399999));
#341688=CARTESIAN_POINT('Ctrl Pts',(4.31377308699994,12.2,1.82414878599999));
#341689=CARTESIAN_POINT('Ctrl Pts',(4.31377308699994,5.2,1.82414878599999));
#341690=CARTESIAN_POINT('Ctrl Pts',(4.31377308699994,2.2,1.82414878599999));
#341691=CARTESIAN_POINT('Ctrl Pts',(4.31124092199994,12.2,1.82452911599999));
#341692=CARTESIAN_POINT('Ctrl Pts',(4.31124092199994,5.2,1.82452911599999));
#341693=CARTESIAN_POINT('Ctrl Pts',(4.31124092199994,2.2,1.82452911599999));
#341694=CARTESIAN_POINT('Ctrl Pts',(4.30871179599994,12.2,1.82490628099998));
#341695=CARTESIAN_POINT('Ctrl Pts',(4.30871179599994,5.2,1.82490628099998));
#341696=CARTESIAN_POINT('Ctrl Pts',(4.30871179599994,2.2,1.82490628099998));
#341697=CARTESIAN_POINT('Ctrl Pts',(4.30618571699994,12.2,1.82528028499998));
#341698=CARTESIAN_POINT('Ctrl Pts',(4.30618571699994,5.2,1.82528028499998));
#341699=CARTESIAN_POINT('Ctrl Pts',(4.30618571699994,2.2,1.82528028499998));
#341700=CARTESIAN_POINT('Ctrl Pts',(4.30366269099994,12.2,1.82565113499999));
#341701=CARTESIAN_POINT('Ctrl Pts',(4.30366269099994,5.2,1.82565113499999));
#341702=CARTESIAN_POINT('Ctrl Pts',(4.30366269099994,2.2,1.82565113499999));
#341703=CARTESIAN_POINT('Ctrl Pts',(4.30114272499994,12.2,1.82601883599999));
#341704=CARTESIAN_POINT('Ctrl Pts',(4.30114272499994,5.2,1.82601883599999));
#341705=CARTESIAN_POINT('Ctrl Pts',(4.30114272499994,2.2,1.82601883599999));
#341706=CARTESIAN_POINT('Ctrl Pts',(4.29862582699994,12.2,1.82638339399999));
#341707=CARTESIAN_POINT('Ctrl Pts',(4.29862582699994,5.2,1.82638339399999));
#341708=CARTESIAN_POINT('Ctrl Pts',(4.29862582699994,2.2,1.82638339399999));
#341709=CARTESIAN_POINT('Ctrl Pts',(4.29611200199994,12.2,1.82674481199999));
#341710=CARTESIAN_POINT('Ctrl Pts',(4.29611200199994,5.2,1.82674481199999));
#341711=CARTESIAN_POINT('Ctrl Pts',(4.29611200199994,2.2,1.82674481199999));
#341712=CARTESIAN_POINT('Ctrl Pts',(4.29360125999994,12.2,1.82710309799999));
#341713=CARTESIAN_POINT('Ctrl Pts',(4.29360125999994,5.2,1.82710309799999));
#341714=CARTESIAN_POINT('Ctrl Pts',(4.29360125999994,2.2,1.82710309799999));
#341715=CARTESIAN_POINT('Ctrl Pts',(4.29109360699994,12.2,1.82745825599998));
#341716=CARTESIAN_POINT('Ctrl Pts',(4.29109360699994,5.2,1.82745825599998));
#341717=CARTESIAN_POINT('Ctrl Pts',(4.29109360699994,2.2,1.82745825599998));
#341718=CARTESIAN_POINT('Ctrl Pts',(4.28858904899994,12.2,1.82781029199999));
#341719=CARTESIAN_POINT('Ctrl Pts',(4.28858904899994,5.2,1.82781029199999));
#341720=CARTESIAN_POINT('Ctrl Pts',(4.28858904899994,2.2,1.82781029199999));
#341721=CARTESIAN_POINT('Ctrl Pts',(4.28608759299994,12.2,1.82815921199999));
#341722=CARTESIAN_POINT('Ctrl Pts',(4.28608759299994,5.2,1.82815921199999));
#341723=CARTESIAN_POINT('Ctrl Pts',(4.28608759299994,2.2,1.82815921199999));
#341724=CARTESIAN_POINT('Ctrl Pts',(4.28358924799995,12.2,1.82850502099999));
#341725=CARTESIAN_POINT('Ctrl Pts',(4.28358924799995,5.2,1.82850502099999));
#341726=CARTESIAN_POINT('Ctrl Pts',(4.28358924799995,2.2,1.82850502099999));
#341727=CARTESIAN_POINT('Ctrl Pts',(4.28109401899994,12.2,1.82884772299999));
#341728=CARTESIAN_POINT('Ctrl Pts',(4.28109401899994,5.2,1.82884772299999));
#341729=CARTESIAN_POINT('Ctrl Pts',(4.28109401899994,2.2,1.82884772299999));
#341730=CARTESIAN_POINT('Ctrl Pts',(4.27860191399995,12.2,1.82918732499999));
#341731=CARTESIAN_POINT('Ctrl Pts',(4.27860191399995,5.2,1.82918732499999));
#341732=CARTESIAN_POINT('Ctrl Pts',(4.27860191399995,2.2,1.82918732499999));
#341733=CARTESIAN_POINT('Ctrl Pts',(4.27611294099994,12.2,1.82952383399998));
#341734=CARTESIAN_POINT('Ctrl Pts',(4.27611294099994,5.2,1.82952383399998));
#341735=CARTESIAN_POINT('Ctrl Pts',(4.27611294099994,2.2,1.82952383399998));
#341736=CARTESIAN_POINT('Ctrl Pts',(4.27362710499995,12.2,1.82985725299998));
#341737=CARTESIAN_POINT('Ctrl Pts',(4.27362710499995,5.2,1.82985725299998));
#341738=CARTESIAN_POINT('Ctrl Pts',(4.27362710499995,2.2,1.82985725299998));
#341739=CARTESIAN_POINT('Ctrl Pts',(4.27114441499994,12.2,1.83018758799999));
#341740=CARTESIAN_POINT('Ctrl Pts',(4.27114441499994,5.2,1.83018758799999));
#341741=CARTESIAN_POINT('Ctrl Pts',(4.27114441499994,2.2,1.83018758799999));
#341742=CARTESIAN_POINT('Ctrl Pts',(4.26866487599994,12.2,1.83051484599998));
#341743=CARTESIAN_POINT('Ctrl Pts',(4.26866487599994,5.2,1.83051484599998));
#341744=CARTESIAN_POINT('Ctrl Pts',(4.26866487599994,2.2,1.83051484599998));
#341745=CARTESIAN_POINT('Ctrl Pts',(4.26618849699994,12.2,1.83083903299998));
#341746=CARTESIAN_POINT('Ctrl Pts',(4.26618849699994,5.2,1.83083903299998));
#341747=CARTESIAN_POINT('Ctrl Pts',(4.26618849699994,2.2,1.83083903299998));
#341748=CARTESIAN_POINT('Ctrl Pts',(4.26371528399994,12.2,1.83116015199999));
#341749=CARTESIAN_POINT('Ctrl Pts',(4.26371528399994,5.2,1.83116015199999));
#341750=CARTESIAN_POINT('Ctrl Pts',(4.26371528399994,2.2,1.83116015199999));
#341751=CARTESIAN_POINT('Ctrl Pts',(4.26124524499994,12.2,1.83147820999999));
#341752=CARTESIAN_POINT('Ctrl Pts',(4.26124524499994,5.2,1.83147820999999));
#341753=CARTESIAN_POINT('Ctrl Pts',(4.26124524499994,2.2,1.83147820999999));
#341754=CARTESIAN_POINT('Ctrl Pts',(4.25877838699994,12.2,1.83179321299999));
#341755=CARTESIAN_POINT('Ctrl Pts',(4.25877838699994,5.2,1.83179321299999));
#341756=CARTESIAN_POINT('Ctrl Pts',(4.25877838699994,2.2,1.83179321299999));
#341757=CARTESIAN_POINT('Ctrl Pts',(4.25631471599995,12.2,1.83210516699999));
#341758=CARTESIAN_POINT('Ctrl Pts',(4.25631471599995,5.2,1.83210516699999));
#341759=CARTESIAN_POINT('Ctrl Pts',(4.25631471599995,2.2,1.83210516699999));
#341760=CARTESIAN_POINT('Ctrl Pts',(4.25385423899994,12.2,1.83241407499999));
#341761=CARTESIAN_POINT('Ctrl Pts',(4.25385423899994,5.2,1.83241407499999));
#341762=CARTESIAN_POINT('Ctrl Pts',(4.25385423899994,2.2,1.83241407499999));
#341763=CARTESIAN_POINT('Ctrl Pts',(4.25139696499994,12.2,1.83271994799998));
#341764=CARTESIAN_POINT('Ctrl Pts',(4.25139696499994,5.2,1.83271994799998));
#341765=CARTESIAN_POINT('Ctrl Pts',(4.25139696499994,2.2,1.83271994799998));
#341766=CARTESIAN_POINT('Ctrl Pts',(4.24894289999994,12.2,1.83302278599998));
#341767=CARTESIAN_POINT('Ctrl Pts',(4.24894289999994,5.2,1.83302278599998));
#341768=CARTESIAN_POINT('Ctrl Pts',(4.24894289999994,2.2,1.83302278599998));
#341769=CARTESIAN_POINT('Ctrl Pts',(4.24649204999994,12.2,1.83332259799998));
#341770=CARTESIAN_POINT('Ctrl Pts',(4.24649204999994,5.2,1.83332259799998));
#341771=CARTESIAN_POINT('Ctrl Pts',(4.24649204999994,2.2,1.83332259799998));
#341772=CARTESIAN_POINT('Ctrl Pts',(4.24404442299994,12.2,1.83361938999999));
#341773=CARTESIAN_POINT('Ctrl Pts',(4.24404442299994,5.2,1.83361938999999));
#341774=CARTESIAN_POINT('Ctrl Pts',(4.24404442299994,2.2,1.83361938999999));
#341775=CARTESIAN_POINT('Ctrl Pts',(4.24160002599994,12.2,1.83391316599999));
#341776=CARTESIAN_POINT('Ctrl Pts',(4.24160002599994,5.2,1.83391316599999));
#341777=CARTESIAN_POINT('Ctrl Pts',(4.24160002599994,2.2,1.83391316599999));
#341778=CARTESIAN_POINT('Ctrl Pts',(4.23915886699994,12.2,1.83420393299999));
#341779=CARTESIAN_POINT('Ctrl Pts',(4.23915886699994,5.2,1.83420393299999));
#341780=CARTESIAN_POINT('Ctrl Pts',(4.23915886699994,2.2,1.83420393299999));
#341781=CARTESIAN_POINT('Ctrl Pts',(4.23672095199994,12.2,1.83449169599998));
#341782=CARTESIAN_POINT('Ctrl Pts',(4.23672095199994,5.2,1.83449169599998));
#341783=CARTESIAN_POINT('Ctrl Pts',(4.23672095199994,2.2,1.83449169599998));
#341784=CARTESIAN_POINT('Ctrl Pts',(4.23428628799994,12.2,1.83477646199998));
#341785=CARTESIAN_POINT('Ctrl Pts',(4.23428628799994,5.2,1.83477646199998));
#341786=CARTESIAN_POINT('Ctrl Pts',(4.23428628799994,2.2,1.83477646199998));
#341787=CARTESIAN_POINT('Ctrl Pts',(4.23185488199994,12.2,1.83505823599999));
#341788=CARTESIAN_POINT('Ctrl Pts',(4.23185488199994,5.2,1.83505823599999));
#341789=CARTESIAN_POINT('Ctrl Pts',(4.23185488199994,2.2,1.83505823599999));
#341790=CARTESIAN_POINT('Ctrl Pts',(4.22942674399994,12.2,1.83533702299998));
#341791=CARTESIAN_POINT('Ctrl Pts',(4.22942674399994,5.2,1.83533702299998));
#341792=CARTESIAN_POINT('Ctrl Pts',(4.22942674399994,2.2,1.83533702299998));
#341793=CARTESIAN_POINT('Ctrl Pts',(4.22700187599994,12.2,1.83561283099999));
#341794=CARTESIAN_POINT('Ctrl Pts',(4.22700187599994,5.2,1.83561283099999));
#341795=CARTESIAN_POINT('Ctrl Pts',(4.22700187599994,2.2,1.83561283099999));
#341796=CARTESIAN_POINT('Ctrl Pts',(4.22458028899994,12.2,1.83588566399999));
#341797=CARTESIAN_POINT('Ctrl Pts',(4.22458028899994,5.2,1.83588566399999));
#341798=CARTESIAN_POINT('Ctrl Pts',(4.22458028899994,2.2,1.83588566399999));
#341799=CARTESIAN_POINT('Ctrl Pts',(4.22216198899994,12.2,1.83615552999999));
#341800=CARTESIAN_POINT('Ctrl Pts',(4.22216198899994,5.2,1.83615552999999));
#341801=CARTESIAN_POINT('Ctrl Pts',(4.22216198899994,2.2,1.83615552999999));
#341802=CARTESIAN_POINT('Ctrl Pts',(4.21974698199994,12.2,1.83642243199999));
#341803=CARTESIAN_POINT('Ctrl Pts',(4.21974698199994,5.2,1.83642243199999));
#341804=CARTESIAN_POINT('Ctrl Pts',(4.21974698199994,2.2,1.83642243199999));
#341805=CARTESIAN_POINT('Ctrl Pts',(4.21733527599994,12.2,1.83668637899999));
#341806=CARTESIAN_POINT('Ctrl Pts',(4.21733527599994,5.2,1.83668637899999));
#341807=CARTESIAN_POINT('Ctrl Pts',(4.21733527599994,2.2,1.83668637899999));
#341808=CARTESIAN_POINT('Ctrl Pts',(4.21492687899994,12.2,1.83694737499998));
#341809=CARTESIAN_POINT('Ctrl Pts',(4.21492687899994,5.2,1.83694737499998));
#341810=CARTESIAN_POINT('Ctrl Pts',(4.21492687899994,2.2,1.83694737499998));
#341811=CARTESIAN_POINT('Ctrl Pts',(4.21252179699994,12.2,1.83720542699998));
#341812=CARTESIAN_POINT('Ctrl Pts',(4.21252179699994,5.2,1.83720542699998));
#341813=CARTESIAN_POINT('Ctrl Pts',(4.21252179699994,2.2,1.83720542699998));
#341814=CARTESIAN_POINT('Ctrl Pts',(4.21012003699994,12.2,1.83746053999998));
#341815=CARTESIAN_POINT('Ctrl Pts',(4.21012003699994,5.2,1.83746053999998));
#341816=CARTESIAN_POINT('Ctrl Pts',(4.21012003699994,2.2,1.83746053999998));
#341817=CARTESIAN_POINT('Ctrl Pts',(4.20772160699994,12.2,1.83771271999999));
#341818=CARTESIAN_POINT('Ctrl Pts',(4.20772160699994,5.2,1.83771271999999));
#341819=CARTESIAN_POINT('Ctrl Pts',(4.20772160699994,2.2,1.83771271999999));
#341820=CARTESIAN_POINT('Ctrl Pts',(4.20532651299994,12.2,1.83796197499999));
#341821=CARTESIAN_POINT('Ctrl Pts',(4.20532651299994,5.2,1.83796197499999));
#341822=CARTESIAN_POINT('Ctrl Pts',(4.20532651299994,2.2,1.83796197499999));
#341823=CARTESIAN_POINT('Ctrl Pts',(4.20293476299994,12.2,1.83820830899998));
#341824=CARTESIAN_POINT('Ctrl Pts',(4.20293476299994,5.2,1.83820830899998));
#341825=CARTESIAN_POINT('Ctrl Pts',(4.20293476299994,2.2,1.83820830899998));
#341826=CARTESIAN_POINT('Ctrl Pts',(4.20054636399994,12.2,1.83845172799999));
#341827=CARTESIAN_POINT('Ctrl Pts',(4.20054636399994,5.2,1.83845172799999));
#341828=CARTESIAN_POINT('Ctrl Pts',(4.20054636399994,2.2,1.83845172799999));
#341829=CARTESIAN_POINT('Ctrl Pts',(4.19816132099994,12.2,1.83869223899999));
#341830=CARTESIAN_POINT('Ctrl Pts',(4.19816132099994,5.2,1.83869223899999));
#341831=CARTESIAN_POINT('Ctrl Pts',(4.19816132099994,2.2,1.83869223899999));
#341832=CARTESIAN_POINT('Ctrl Pts',(4.19577964499994,12.2,1.83892984999999));
#341833=CARTESIAN_POINT('Ctrl Pts',(4.19577964499994,5.2,1.83892984999999));
#341834=CARTESIAN_POINT('Ctrl Pts',(4.19577964499994,2.2,1.83892984999999));
#341835=CARTESIAN_POINT('Ctrl Pts',(4.19340133999994,12.2,1.83916456299999));
#341836=CARTESIAN_POINT('Ctrl Pts',(4.19340133999994,5.2,1.83916456299999));
#341837=CARTESIAN_POINT('Ctrl Pts',(4.19340133999994,2.2,1.83916456299999));
#341838=CARTESIAN_POINT('Ctrl Pts',(4.19102641499994,12.2,1.83939638699998));
#341839=CARTESIAN_POINT('Ctrl Pts',(4.19102641499994,5.2,1.83939638699998));
#341840=CARTESIAN_POINT('Ctrl Pts',(4.19102641499994,2.2,1.83939638699998));
#341841=CARTESIAN_POINT('Ctrl Pts',(4.18865487599995,12.2,1.83962532699999));
#341842=CARTESIAN_POINT('Ctrl Pts',(4.18865487599995,5.2,1.83962532699999));
#341843=CARTESIAN_POINT('Ctrl Pts',(4.18865487599995,2.2,1.83962532699999));
#341844=CARTESIAN_POINT('Ctrl Pts',(4.18628672999994,12.2,1.83985138999998));
#341845=CARTESIAN_POINT('Ctrl Pts',(4.18628672999994,5.2,1.83985138999998));
#341846=CARTESIAN_POINT('Ctrl Pts',(4.18628672999994,2.2,1.83985138999998));
#341847=CARTESIAN_POINT('Ctrl Pts',(4.18392198399994,12.2,1.84007458199998));
#341848=CARTESIAN_POINT('Ctrl Pts',(4.18392198399994,5.2,1.84007458199998));
#341849=CARTESIAN_POINT('Ctrl Pts',(4.18392198399994,2.2,1.84007458199998));
#341850=CARTESIAN_POINT('Ctrl Pts',(4.18156064699994,12.2,1.84029490799999));
#341851=CARTESIAN_POINT('Ctrl Pts',(4.18156064699994,5.2,1.84029490799999));
#341852=CARTESIAN_POINT('Ctrl Pts',(4.18156064699994,2.2,1.84029490799999));
#341853=CARTESIAN_POINT('Ctrl Pts',(4.17920272399994,12.2,1.84051237599999));
#341854=CARTESIAN_POINT('Ctrl Pts',(4.17920272399994,5.2,1.84051237599999));
#341855=CARTESIAN_POINT('Ctrl Pts',(4.17920272399994,2.2,1.84051237599999));
#341856=CARTESIAN_POINT('Ctrl Pts',(4.17684822299994,12.2,1.84072699099998));
#341857=CARTESIAN_POINT('Ctrl Pts',(4.17684822299994,5.2,1.84072699099998));
#341858=CARTESIAN_POINT('Ctrl Pts',(4.17684822299994,2.2,1.84072699099998));
#341859=CARTESIAN_POINT('Ctrl Pts',(4.17449715099994,12.2,1.84093875999999));
#341860=CARTESIAN_POINT('Ctrl Pts',(4.17449715099994,5.2,1.84093875999999));
#341861=CARTESIAN_POINT('Ctrl Pts',(4.17449715099994,2.2,1.84093875999999));
#341862=CARTESIAN_POINT('Ctrl Pts',(4.17214951399994,12.2,1.84114768899999));
#341863=CARTESIAN_POINT('Ctrl Pts',(4.17214951399994,5.2,1.84114768899999));
#341864=CARTESIAN_POINT('Ctrl Pts',(4.17214951399994,2.2,1.84114768899999));
#341865=CARTESIAN_POINT('Ctrl Pts',(4.16980532099995,12.2,1.84135378499999));
#341866=CARTESIAN_POINT('Ctrl Pts',(4.16980532099995,5.2,1.84135378499999));
#341867=CARTESIAN_POINT('Ctrl Pts',(4.16980532099995,2.2,1.84135378499999));
#341868=CARTESIAN_POINT('Ctrl Pts',(4.16746457899994,12.2,1.84155705199998));
#341869=CARTESIAN_POINT('Ctrl Pts',(4.16746457899994,5.2,1.84155705199998));
#341870=CARTESIAN_POINT('Ctrl Pts',(4.16746457899994,2.2,1.84155705199998));
#341871=CARTESIAN_POINT('Ctrl Pts',(4.16512729299995,12.2,1.84175749999998));
#341872=CARTESIAN_POINT('Ctrl Pts',(4.16512729299995,5.2,1.84175749999998));
#341873=CARTESIAN_POINT('Ctrl Pts',(4.16512729299995,2.2,1.84175749999998));
#341874=CARTESIAN_POINT('Ctrl Pts',(4.16279347199994,12.2,1.84195513199999));
#341875=CARTESIAN_POINT('Ctrl Pts',(4.16279347199994,5.2,1.84195513199999));
#341876=CARTESIAN_POINT('Ctrl Pts',(4.16279347199994,2.2,1.84195513199999));
#341877=CARTESIAN_POINT('Ctrl Pts',(4.16046312299994,12.2,1.84214995599998));
#341878=CARTESIAN_POINT('Ctrl Pts',(4.16046312299994,5.2,1.84214995599998));
#341879=CARTESIAN_POINT('Ctrl Pts',(4.16046312299994,2.2,1.84214995599998));
#341880=CARTESIAN_POINT('Ctrl Pts',(4.15813625299995,12.2,1.84234197899999));
#341881=CARTESIAN_POINT('Ctrl Pts',(4.15813625299995,5.2,1.84234197899999));
#341882=CARTESIAN_POINT('Ctrl Pts',(4.15813625299995,2.2,1.84234197899999));
#341883=CARTESIAN_POINT('Ctrl Pts',(4.15581286799994,12.2,1.84253120599998));
#341884=CARTESIAN_POINT('Ctrl Pts',(4.15581286799994,5.2,1.84253120599998));
#341885=CARTESIAN_POINT('Ctrl Pts',(4.15581286799994,2.2,1.84253120599998));
#341886=CARTESIAN_POINT('Ctrl Pts',(4.15349297599994,12.2,1.84271764399998));
#341887=CARTESIAN_POINT('Ctrl Pts',(4.15349297599994,5.2,1.84271764399998));
#341888=CARTESIAN_POINT('Ctrl Pts',(4.15349297599994,2.2,1.84271764399998));
#341889=CARTESIAN_POINT('Ctrl Pts',(4.15117658499994,12.2,1.84290129899999));
#341890=CARTESIAN_POINT('Ctrl Pts',(4.15117658499994,5.2,1.84290129899999));
#341891=CARTESIAN_POINT('Ctrl Pts',(4.15117658499994,2.2,1.84290129899999));
#341892=CARTESIAN_POINT('Ctrl Pts',(4.14886370099994,12.2,1.84308217899999));
#341893=CARTESIAN_POINT('Ctrl Pts',(4.14886370099994,5.2,1.84308217899999));
#341894=CARTESIAN_POINT('Ctrl Pts',(4.14886370099994,2.2,1.84308217899999));
#341895=CARTESIAN_POINT('Ctrl Pts',(4.14655433099994,12.2,1.84326028799998));
#341896=CARTESIAN_POINT('Ctrl Pts',(4.14655433099994,5.2,1.84326028799998));
#341897=CARTESIAN_POINT('Ctrl Pts',(4.14655433099994,2.2,1.84326028799998));
#341898=CARTESIAN_POINT('Ctrl Pts',(4.14424848299995,12.2,1.84343563499999));
#341899=CARTESIAN_POINT('Ctrl Pts',(4.14424848299995,5.2,1.84343563499999));
#341900=CARTESIAN_POINT('Ctrl Pts',(4.14424848299995,2.2,1.84343563499999));
#341901=CARTESIAN_POINT('Ctrl Pts',(4.14194616299994,12.2,1.84360822599999));
#341902=CARTESIAN_POINT('Ctrl Pts',(4.14194616299994,5.2,1.84360822599999));
#341903=CARTESIAN_POINT('Ctrl Pts',(4.14194616299994,2.2,1.84360822599999));
#341904=CARTESIAN_POINT('Ctrl Pts',(4.13964737899994,12.2,1.84377806599999));
#341905=CARTESIAN_POINT('Ctrl Pts',(4.13964737899994,5.2,1.84377806599999));
#341906=CARTESIAN_POINT('Ctrl Pts',(4.13964737899994,2.2,1.84377806599999));
#341907=CARTESIAN_POINT('Ctrl Pts',(4.13735213799994,12.2,1.84394516299998));
#341908=CARTESIAN_POINT('Ctrl Pts',(4.13735213799994,5.2,1.84394516299998));
#341909=CARTESIAN_POINT('Ctrl Pts',(4.13735213799994,2.2,1.84394516299998));
#341910=CARTESIAN_POINT('Ctrl Pts',(4.13506044699994,12.2,1.84410952299999));
#341911=CARTESIAN_POINT('Ctrl Pts',(4.13506044699994,5.2,1.84410952299999));
#341912=CARTESIAN_POINT('Ctrl Pts',(4.13506044699994,2.2,1.84410952299999));
#341913=CARTESIAN_POINT('Ctrl Pts',(4.13277231299995,12.2,1.84427115299998));
#341914=CARTESIAN_POINT('Ctrl Pts',(4.13277231299995,5.2,1.84427115299998));
#341915=CARTESIAN_POINT('Ctrl Pts',(4.13277231299995,2.2,1.84427115299998));
#341916=CARTESIAN_POINT('Ctrl Pts',(4.13048774299994,12.2,1.84443005899999));
#341917=CARTESIAN_POINT('Ctrl Pts',(4.13048774299994,5.2,1.84443005899999));
#341918=CARTESIAN_POINT('Ctrl Pts',(4.13048774299994,2.2,1.84443005899999));
#341919=CARTESIAN_POINT('Ctrl Pts',(4.12820674499994,12.2,1.84458624799999));
#341920=CARTESIAN_POINT('Ctrl Pts',(4.12820674499994,5.2,1.84458624799999));
#341921=CARTESIAN_POINT('Ctrl Pts',(4.12820674499994,2.2,1.84458624799999));
#341922=CARTESIAN_POINT('Ctrl Pts',(4.12592932499994,12.2,1.84473972799998));
#341923=CARTESIAN_POINT('Ctrl Pts',(4.12592932499994,5.2,1.84473972799998));
#341924=CARTESIAN_POINT('Ctrl Pts',(4.12592932499994,2.2,1.84473972799998));
#341925=CARTESIAN_POINT('Ctrl Pts',(4.12365549099994,12.2,1.84489050299999));
#341926=CARTESIAN_POINT('Ctrl Pts',(4.12365549099994,5.2,1.84489050299999));
#341927=CARTESIAN_POINT('Ctrl Pts',(4.12365549099994,2.2,1.84489050299999));
#341928=CARTESIAN_POINT('Ctrl Pts',(4.12138524999994,12.2,1.84503858199998));
#341929=CARTESIAN_POINT('Ctrl Pts',(4.12138524999994,5.2,1.84503858199998));
#341930=CARTESIAN_POINT('Ctrl Pts',(4.12138524999994,2.2,1.84503858199998));
#341931=CARTESIAN_POINT('Ctrl Pts',(4.11911860799994,12.2,1.84518396999998));
#341932=CARTESIAN_POINT('Ctrl Pts',(4.11911860799994,5.2,1.84518396999998));
#341933=CARTESIAN_POINT('Ctrl Pts',(4.11911860799994,2.2,1.84518396999998));
#341934=CARTESIAN_POINT('Ctrl Pts',(4.11685557399994,12.2,1.84532667399999));
#341935=CARTESIAN_POINT('Ctrl Pts',(4.11685557399994,5.2,1.84532667399999));
#341936=CARTESIAN_POINT('Ctrl Pts',(4.11685557399994,2.2,1.84532667399999));
#341937=CARTESIAN_POINT('Ctrl Pts',(4.11459615299994,12.2,1.84546670299999));
#341938=CARTESIAN_POINT('Ctrl Pts',(4.11459615299994,5.2,1.84546670299999));
#341939=CARTESIAN_POINT('Ctrl Pts',(4.11459615299994,2.2,1.84546670299999));
#341940=CARTESIAN_POINT('Ctrl Pts',(4.11234035499994,12.2,1.84560406099999));
#341941=CARTESIAN_POINT('Ctrl Pts',(4.11234035499994,5.2,1.84560406099999));
#341942=CARTESIAN_POINT('Ctrl Pts',(4.11234035499994,2.2,1.84560406099999));
#341943=CARTESIAN_POINT('Ctrl Pts',(4.11008818399995,12.2,1.84573875499999));
#341944=CARTESIAN_POINT('Ctrl Pts',(4.11008818399995,5.2,1.84573875499999));
#341945=CARTESIAN_POINT('Ctrl Pts',(4.11008818399995,2.2,1.84573875499999));
#341946=CARTESIAN_POINT('Ctrl Pts',(4.10783964999994,12.2,1.84587079399999));
#341947=CARTESIAN_POINT('Ctrl Pts',(4.10783964999994,5.2,1.84587079399999));
#341948=CARTESIAN_POINT('Ctrl Pts',(4.10783964999994,2.2,1.84587079399999));
#341949=CARTESIAN_POINT('Ctrl Pts',(4.10559475699994,12.2,1.84600018399999));
#341950=CARTESIAN_POINT('Ctrl Pts',(4.10559475699994,5.2,1.84600018399999));
#341951=CARTESIAN_POINT('Ctrl Pts',(4.10559475699994,2.2,1.84600018399999));
#341952=CARTESIAN_POINT('Ctrl Pts',(4.10335351499994,12.2,1.84612693099998));
#341953=CARTESIAN_POINT('Ctrl Pts',(4.10335351499994,5.2,1.84612693099998));
#341954=CARTESIAN_POINT('Ctrl Pts',(4.10335351499994,2.2,1.84612693099998));
#341955=CARTESIAN_POINT('Ctrl Pts',(4.10111592999994,12.2,1.84625104099998));
#341956=CARTESIAN_POINT('Ctrl Pts',(4.10111592999994,5.2,1.84625104099998));
#341957=CARTESIAN_POINT('Ctrl Pts',(4.10111592999994,2.2,1.84625104099998));
#341958=CARTESIAN_POINT('Ctrl Pts',(4.09888200799994,12.2,1.84637252299999));
#341959=CARTESIAN_POINT('Ctrl Pts',(4.09888200799994,5.2,1.84637252299999));
#341960=CARTESIAN_POINT('Ctrl Pts',(4.09888200799994,2.2,1.84637252299999));
#341961=CARTESIAN_POINT('Ctrl Pts',(4.09665175899994,12.2,1.84649138299998));
#341962=CARTESIAN_POINT('Ctrl Pts',(4.09665175899994,5.2,1.84649138299998));
#341963=CARTESIAN_POINT('Ctrl Pts',(4.09665175899994,2.2,1.84649138299998));
#341964=CARTESIAN_POINT('Ctrl Pts',(4.09442518799994,12.2,1.84660762799998));
#341965=CARTESIAN_POINT('Ctrl Pts',(4.09442518799994,5.2,1.84660762799998));
#341966=CARTESIAN_POINT('Ctrl Pts',(4.09442518799994,2.2,1.84660762799998));
#341967=CARTESIAN_POINT('Ctrl Pts',(4.09220230199994,12.2,1.84672126599999));
#341968=CARTESIAN_POINT('Ctrl Pts',(4.09220230199994,5.2,1.84672126599999));
#341969=CARTESIAN_POINT('Ctrl Pts',(4.09220230199994,2.2,1.84672126599999));
#341970=CARTESIAN_POINT('Ctrl Pts',(4.08998310899995,12.2,1.84683230099999));
#341971=CARTESIAN_POINT('Ctrl Pts',(4.08998310899995,5.2,1.84683230099999));
#341972=CARTESIAN_POINT('Ctrl Pts',(4.08998310899995,2.2,1.84683230099999));
#341973=CARTESIAN_POINT('Ctrl Pts',(4.08776761599994,12.2,1.84694074299999));
#341974=CARTESIAN_POINT('Ctrl Pts',(4.08776761599994,5.2,1.84694074299999));
#341975=CARTESIAN_POINT('Ctrl Pts',(4.08776761599994,2.2,1.84694074299999));
#341976=CARTESIAN_POINT('Ctrl Pts',(4.08555582999994,12.2,1.84704659699999));
#341977=CARTESIAN_POINT('Ctrl Pts',(4.08555582999994,5.2,1.84704659699999));
#341978=CARTESIAN_POINT('Ctrl Pts',(4.08555582999994,2.2,1.84704659699999));
#341979=CARTESIAN_POINT('Ctrl Pts',(4.08334775699995,12.2,1.84714987299999));
#341980=CARTESIAN_POINT('Ctrl Pts',(4.08334775699995,5.2,1.84714987299999));
#341981=CARTESIAN_POINT('Ctrl Pts',(4.08334775699995,2.2,1.84714987299999));
#341982=CARTESIAN_POINT('Ctrl Pts',(4.08114340699994,12.2,1.84725057399998));
#341983=CARTESIAN_POINT('Ctrl Pts',(4.08114340699994,5.2,1.84725057399998));
#341984=CARTESIAN_POINT('Ctrl Pts',(4.08114340699994,2.2,1.84725057399998));
#341985=CARTESIAN_POINT('Ctrl Pts',(4.07894278499994,12.2,1.84734870999999));
#341986=CARTESIAN_POINT('Ctrl Pts',(4.07894278499994,5.2,1.84734870999999));
#341987=CARTESIAN_POINT('Ctrl Pts',(4.07894278499994,2.2,1.84734870999999));
#341988=CARTESIAN_POINT('Ctrl Pts',(4.07674589799994,12.2,1.84744428699998));
#341989=CARTESIAN_POINT('Ctrl Pts',(4.07674589799994,5.2,1.84744428699998));
#341990=CARTESIAN_POINT('Ctrl Pts',(4.07674589799994,2.2,1.84744428699998));
#341991=CARTESIAN_POINT('Ctrl Pts',(4.07455275399994,12.2,1.84753731199998));
#341992=CARTESIAN_POINT('Ctrl Pts',(4.07455275399994,5.2,1.84753731199998));
#341993=CARTESIAN_POINT('Ctrl Pts',(4.07455275399994,2.2,1.84753731199998));
#341994=CARTESIAN_POINT('Ctrl Pts',(4.07236335899994,12.2,1.84762779199998));
#341995=CARTESIAN_POINT('Ctrl Pts',(4.07236335899994,5.2,1.84762779199998));
#341996=CARTESIAN_POINT('Ctrl Pts',(4.07236335899994,2.2,1.84762779199998));
#341997=CARTESIAN_POINT('Ctrl Pts',(4.07017772299994,12.2,1.84771573499999));
#341998=CARTESIAN_POINT('Ctrl Pts',(4.07017772299994,5.2,1.84771573499999));
#341999=CARTESIAN_POINT('Ctrl Pts',(4.07017772299994,2.2,1.84771573499999));
#342000=CARTESIAN_POINT('Ctrl Pts',(4.06799584999994,12.2,1.84780114799999));
#342001=CARTESIAN_POINT('Ctrl Pts',(4.06799584999994,5.2,1.84780114799999));
#342002=CARTESIAN_POINT('Ctrl Pts',(4.06799584999994,2.2,1.84780114799999));
#342003=CARTESIAN_POINT('Ctrl Pts',(4.06581774699994,12.2,1.84788403799999));
#342004=CARTESIAN_POINT('Ctrl Pts',(4.06581774699994,5.2,1.84788403799999));
#342005=CARTESIAN_POINT('Ctrl Pts',(4.06581774699994,2.2,1.84788403799999));
#342006=CARTESIAN_POINT('Ctrl Pts',(4.06364342499994,12.2,1.84796441199999));
#342007=CARTESIAN_POINT('Ctrl Pts',(4.06364342499994,5.2,1.84796441199999));
#342008=CARTESIAN_POINT('Ctrl Pts',(4.06364342499994,2.2,1.84796441199999));
#342009=CARTESIAN_POINT('Ctrl Pts',(4.06147288699994,12.2,1.84804227599999));
#342010=CARTESIAN_POINT('Ctrl Pts',(4.06147288699994,5.2,1.84804227599999));
#342011=CARTESIAN_POINT('Ctrl Pts',(4.06147288699994,2.2,1.84804227599999));
#342012=CARTESIAN_POINT('Ctrl Pts',(4.05930614299994,12.2,1.84811763999999));
#342013=CARTESIAN_POINT('Ctrl Pts',(4.05930614299994,5.2,1.84811763999999));
#342014=CARTESIAN_POINT('Ctrl Pts',(4.05930614299994,2.2,1.84811763999999));
#342015=CARTESIAN_POINT('Ctrl Pts',(4.05714319699995,12.2,1.84819050899999));
#342016=CARTESIAN_POINT('Ctrl Pts',(4.05714319699995,5.2,1.84819050899999));
#342017=CARTESIAN_POINT('Ctrl Pts',(4.05714319699995,2.2,1.84819050899999));
#342018=CARTESIAN_POINT('Ctrl Pts',(4.05498405999994,12.2,1.84826089199999));
#342019=CARTESIAN_POINT('Ctrl Pts',(4.05498405999994,5.2,1.84826089199999));
#342020=CARTESIAN_POINT('Ctrl Pts',(4.05498405999994,2.2,1.84826089199999));
#342021=CARTESIAN_POINT('Ctrl Pts',(4.05282873699994,12.2,1.84832879599998));
#342022=CARTESIAN_POINT('Ctrl Pts',(4.05282873699994,5.2,1.84832879599998));
#342023=CARTESIAN_POINT('Ctrl Pts',(4.05282873699994,2.2,1.84832879599998));
#342024=CARTESIAN_POINT('Ctrl Pts',(4.05067723499995,12.2,1.84839422599998));
#342025=CARTESIAN_POINT('Ctrl Pts',(4.05067723499995,5.2,1.84839422599998));
#342026=CARTESIAN_POINT('Ctrl Pts',(4.05067723499995,2.2,1.84839422599998));
#342027=CARTESIAN_POINT('Ctrl Pts',(4.04852955999994,12.2,1.84845719299998));
#342028=CARTESIAN_POINT('Ctrl Pts',(4.04852955999994,5.2,1.84845719299998));
#342029=CARTESIAN_POINT('Ctrl Pts',(4.04852955999994,2.2,1.84845719299998));
#342030=CARTESIAN_POINT('Ctrl Pts',(4.04638572299994,12.2,1.84851770099999));
#342031=CARTESIAN_POINT('Ctrl Pts',(4.04638572299994,5.2,1.84851770099999));
#342032=CARTESIAN_POINT('Ctrl Pts',(4.04638572299994,2.2,1.84851770099999));
#342033=CARTESIAN_POINT('Ctrl Pts',(4.04424572799994,12.2,1.84857575999999));
#342034=CARTESIAN_POINT('Ctrl Pts',(4.04424572799994,5.2,1.84857575999999));
#342035=CARTESIAN_POINT('Ctrl Pts',(4.04424572799994,2.2,1.84857575999999));
#342036=CARTESIAN_POINT('Ctrl Pts',(4.04210958299995,12.2,1.84863137599999));
#342037=CARTESIAN_POINT('Ctrl Pts',(4.04210958299995,5.2,1.84863137599999));
#342038=CARTESIAN_POINT('Ctrl Pts',(4.04210958299995,2.2,1.84863137599999));
#342039=CARTESIAN_POINT('Ctrl Pts',(4.03997729399994,12.2,1.84868455699998));
#342040=CARTESIAN_POINT('Ctrl Pts',(4.03997729399994,5.2,1.84868455699998));
#342041=CARTESIAN_POINT('Ctrl Pts',(4.03997729399994,2.2,1.84868455699998));
#342042=CARTESIAN_POINT('Ctrl Pts',(4.03784887099994,12.2,1.84873531099999));
#342043=CARTESIAN_POINT('Ctrl Pts',(4.03784887099994,5.2,1.84873531099999));
#342044=CARTESIAN_POINT('Ctrl Pts',(4.03784887099994,2.2,1.84873531099999));
#342045=CARTESIAN_POINT('Ctrl Pts',(4.03572431899994,12.2,1.84878364299998));
#342046=CARTESIAN_POINT('Ctrl Pts',(4.03572431899994,5.2,1.84878364299998));
#342047=CARTESIAN_POINT('Ctrl Pts',(4.03572431899994,2.2,1.84878364299998));
#342048=CARTESIAN_POINT('Ctrl Pts',(4.03360364499994,12.2,1.84882956299999));
#342049=CARTESIAN_POINT('Ctrl Pts',(4.03360364499994,5.2,1.84882956299999));
#342050=CARTESIAN_POINT('Ctrl Pts',(4.03360364499994,2.2,1.84882956299999));
#342051=CARTESIAN_POINT('Ctrl Pts',(4.03148685699994,12.2,1.84887307799999));
#342052=CARTESIAN_POINT('Ctrl Pts',(4.03148685699994,5.2,1.84887307799999));
#342053=CARTESIAN_POINT('Ctrl Pts',(4.03148685699994,2.2,1.84887307799999));
#342054=CARTESIAN_POINT('Ctrl Pts',(4.02937396299994,12.2,1.84891419499999));
#342055=CARTESIAN_POINT('Ctrl Pts',(4.02937396299994,5.2,1.84891419499999));
#342056=CARTESIAN_POINT('Ctrl Pts',(4.02937396299994,2.2,1.84891419499999));
#342057=CARTESIAN_POINT('Ctrl Pts',(4.02726496799994,12.2,1.84895292199998));
#342058=CARTESIAN_POINT('Ctrl Pts',(4.02726496799994,5.2,1.84895292199998));
#342059=CARTESIAN_POINT('Ctrl Pts',(4.02726496799994,2.2,1.84895292199998));
#342060=CARTESIAN_POINT('Ctrl Pts',(4.02515988099994,12.2,1.84898926699999));
#342061=CARTESIAN_POINT('Ctrl Pts',(4.02515988099994,5.2,1.84898926699999));
#342062=CARTESIAN_POINT('Ctrl Pts',(4.02515988099994,2.2,1.84898926699999));
#342063=CARTESIAN_POINT('Ctrl Pts',(4.02305870799994,12.2,1.84902323599998));
#342064=CARTESIAN_POINT('Ctrl Pts',(4.02305870799994,5.2,1.84902323599998));
#342065=CARTESIAN_POINT('Ctrl Pts',(4.02305870799994,2.2,1.84902323599998));
#342066=CARTESIAN_POINT('Ctrl Pts',(4.02096145599994,12.2,1.84905483799998));
#342067=CARTESIAN_POINT('Ctrl Pts',(4.02096145599994,5.2,1.84905483799998));
#342068=CARTESIAN_POINT('Ctrl Pts',(4.02096145599994,2.2,1.84905483799998));
#342069=CARTESIAN_POINT('Ctrl Pts',(4.01886813399994,12.2,1.84908408199998));
#342070=CARTESIAN_POINT('Ctrl Pts',(4.01886813399994,5.2,1.84908408199998));
#342071=CARTESIAN_POINT('Ctrl Pts',(4.01886813399994,2.2,1.84908408199998));
#342072=CARTESIAN_POINT('Ctrl Pts',(4.01677874699994,12.2,1.84911097199999));
#342073=CARTESIAN_POINT('Ctrl Pts',(4.01677874699994,5.2,1.84911097199999));
#342074=CARTESIAN_POINT('Ctrl Pts',(4.01677874699994,2.2,1.84911097199999));
#342075=CARTESIAN_POINT('Ctrl Pts',(4.01469330299994,12.2,1.84913551799998));
#342076=CARTESIAN_POINT('Ctrl Pts',(4.01469330299994,5.2,1.84913551799998));
#342077=CARTESIAN_POINT('Ctrl Pts',(4.01469330299994,2.2,1.84913551799998));
#342078=CARTESIAN_POINT('Ctrl Pts',(4.01261180999995,12.2,1.84915772799998));
#342079=CARTESIAN_POINT('Ctrl Pts',(4.01261180999995,5.2,1.84915772799998));
#342080=CARTESIAN_POINT('Ctrl Pts',(4.01261180999995,2.2,1.84915772799998));
#342081=CARTESIAN_POINT('Ctrl Pts',(4.01053427299995,12.2,1.84917760899999));
#342082=CARTESIAN_POINT('Ctrl Pts',(4.01053427299995,5.2,1.84917760899999));
#342083=CARTESIAN_POINT('Ctrl Pts',(4.01053427299995,2.2,1.84917760899999));
#342084=CARTESIAN_POINT('Ctrl Pts',(4.00846070199994,12.2,1.84919516899999));
#342085=CARTESIAN_POINT('Ctrl Pts',(4.00846070199994,5.2,1.84919516899999));
#342086=CARTESIAN_POINT('Ctrl Pts',(4.00846070199994,2.2,1.84919516899999));
#342087=CARTESIAN_POINT('Ctrl Pts',(4.00639110199995,12.2,1.84921041499999));
#342088=CARTESIAN_POINT('Ctrl Pts',(4.00639110199995,5.2,1.84921041499999));
#342089=CARTESIAN_POINT('Ctrl Pts',(4.00639110199995,2.2,1.84921041499999));
#342090=CARTESIAN_POINT('Ctrl Pts',(4.00432548099994,12.2,1.84922335699999));
#342091=CARTESIAN_POINT('Ctrl Pts',(4.00432548099994,5.2,1.84922335699999));
#342092=CARTESIAN_POINT('Ctrl Pts',(4.00432548099994,2.2,1.84922335699999));
#342093=CARTESIAN_POINT('Ctrl Pts',(4.00226384599994,12.2,1.84923399999999));
#342094=CARTESIAN_POINT('Ctrl Pts',(4.00226384599994,5.2,1.84923399999999));
#342095=CARTESIAN_POINT('Ctrl Pts',(4.00226384599994,2.2,1.84923399999999));
#342096=CARTESIAN_POINT('Ctrl Pts',(4.00020620399994,12.2,1.84924235299999));
#342097=CARTESIAN_POINT('Ctrl Pts',(4.00020620399994,5.2,1.84924235299999));
#342098=CARTESIAN_POINT('Ctrl Pts',(4.00020620399994,2.2,1.84924235299999));
#342099=CARTESIAN_POINT('Ctrl Pts',(3.99815256199994,12.2,1.84924842499999));
#342100=CARTESIAN_POINT('Ctrl Pts',(3.99815256199994,5.2,1.84924842499999));
#342101=CARTESIAN_POINT('Ctrl Pts',(3.99815256199994,2.2,1.84924842499999));
#342102=CARTESIAN_POINT('Ctrl Pts',(3.99610292899994,12.2,1.84925222199999));
#342103=CARTESIAN_POINT('Ctrl Pts',(3.99610292899994,5.2,1.84925222199999));
#342104=CARTESIAN_POINT('Ctrl Pts',(3.99610292899994,2.2,1.84925222199999));
#342105=CARTESIAN_POINT('Ctrl Pts',(3.99405730999994,12.2,1.84925375299999));
#342106=CARTESIAN_POINT('Ctrl Pts',(3.99405730999994,5.2,1.84925375299999));
#342107=CARTESIAN_POINT('Ctrl Pts',(3.99405730999994,2.2,1.84925375299999));
#342108=CARTESIAN_POINT('Ctrl Pts',(3.99201571199994,12.2,1.84925302699999));
#342109=CARTESIAN_POINT('Ctrl Pts',(3.99201571199994,5.2,1.84925302699999));
#342110=CARTESIAN_POINT('Ctrl Pts',(3.99201571199994,2.2,1.84925302699999));
#342111=CARTESIAN_POINT('Ctrl Pts',(3.98997814399995,12.2,1.84925004999998));
#342112=CARTESIAN_POINT('Ctrl Pts',(3.98997814399995,5.2,1.84925004999998));
#342113=CARTESIAN_POINT('Ctrl Pts',(3.98997814399995,2.2,1.84925004999998));
#342114=CARTESIAN_POINT('Ctrl Pts',(3.98794461099994,12.2,1.84924482999998));
#342115=CARTESIAN_POINT('Ctrl Pts',(3.98794461099994,5.2,1.84924482999998));
#342116=CARTESIAN_POINT('Ctrl Pts',(3.98794461099994,2.2,1.84924482999998));
#342117=CARTESIAN_POINT('Ctrl Pts',(3.98591512199994,12.2,1.84923737699998));
#342118=CARTESIAN_POINT('Ctrl Pts',(3.98591512199994,5.2,1.84923737699998));
#342119=CARTESIAN_POINT('Ctrl Pts',(3.98591512199994,2.2,1.84923737699998));
#342120=CARTESIAN_POINT('Ctrl Pts',(3.98388968399995,12.2,1.84922769599998));
#342121=CARTESIAN_POINT('Ctrl Pts',(3.98388968399995,5.2,1.84922769599998));
#342122=CARTESIAN_POINT('Ctrl Pts',(3.98388968399995,2.2,1.84922769599998));
#342123=CARTESIAN_POINT('Ctrl Pts',(3.98186830299994,12.2,1.84921579899999));
#342124=CARTESIAN_POINT('Ctrl Pts',(3.98186830299994,5.2,1.84921579899999));
#342125=CARTESIAN_POINT('Ctrl Pts',(3.98186830299994,2.2,1.84921579899999));
#342126=CARTESIAN_POINT('Ctrl Pts',(3.97985098799994,12.2,1.84920168999998));
#342127=CARTESIAN_POINT('Ctrl Pts',(3.97985098799994,5.2,1.84920168999998));
#342128=CARTESIAN_POINT('Ctrl Pts',(3.97985098799994,2.2,1.84920168999998));
#342129=CARTESIAN_POINT('Ctrl Pts',(3.97783774399994,12.2,1.84918537999998));
#342130=CARTESIAN_POINT('Ctrl Pts',(3.97783774399994,5.2,1.84918537999998));
#342131=CARTESIAN_POINT('Ctrl Pts',(3.97783774399994,2.2,1.84918537999998));
#342132=CARTESIAN_POINT('Ctrl Pts',(3.97582857899994,12.2,1.84916687499999));
#342133=CARTESIAN_POINT('Ctrl Pts',(3.97582857899994,5.2,1.84916687499999));
#342134=CARTESIAN_POINT('Ctrl Pts',(3.97582857899994,2.2,1.84916687499999));
#342135=CARTESIAN_POINT('Ctrl Pts',(3.97382350099994,12.2,1.84914618499999));
#342136=CARTESIAN_POINT('Ctrl Pts',(3.97382350099994,5.2,1.84914618499999));
#342137=CARTESIAN_POINT('Ctrl Pts',(3.97382350099994,2.2,1.84914618499999));
#342138=CARTESIAN_POINT('Ctrl Pts',(3.97182251499994,12.2,1.84912331799998));
#342139=CARTESIAN_POINT('Ctrl Pts',(3.97182251499994,5.2,1.84912331799998));
#342140=CARTESIAN_POINT('Ctrl Pts',(3.97182251499994,2.2,1.84912331799998));
#342141=CARTESIAN_POINT('Ctrl Pts',(3.96982563199994,12.2,1.84909827999999));
#342142=CARTESIAN_POINT('Ctrl Pts',(3.96982563199994,5.2,1.84909827999999));
#342143=CARTESIAN_POINT('Ctrl Pts',(3.96982563199994,2.2,1.84909827999999));
#342144=CARTESIAN_POINT('Ctrl Pts',(3.96783285499994,12.2,1.84907108099999));
#342145=CARTESIAN_POINT('Ctrl Pts',(3.96783285499994,5.2,1.84907108099999));
#342146=CARTESIAN_POINT('Ctrl Pts',(3.96783285499994,2.2,1.84907108099999));
#342147=CARTESIAN_POINT('Ctrl Pts',(3.96584419399994,12.2,1.84904172999998));
#342148=CARTESIAN_POINT('Ctrl Pts',(3.96584419399994,5.2,1.84904172999998));
#342149=CARTESIAN_POINT('Ctrl Pts',(3.96584419399994,2.2,1.84904172999998));
#342150=CARTESIAN_POINT('Ctrl Pts',(3.96385965499995,12.2,1.84901023299998));
#342151=CARTESIAN_POINT('Ctrl Pts',(3.96385965499995,5.2,1.84901023299998));
#342152=CARTESIAN_POINT('Ctrl Pts',(3.96385965499995,2.2,1.84901023299998));
#342153=CARTESIAN_POINT('Ctrl Pts',(3.96187924499994,12.2,1.84897660099999));
#342154=CARTESIAN_POINT('Ctrl Pts',(3.96187924499994,5.2,1.84897660099999));
#342155=CARTESIAN_POINT('Ctrl Pts',(3.96187924499994,2.2,1.84897660099999));
#342156=CARTESIAN_POINT('Ctrl Pts',(3.95990297199994,12.2,1.84894083999998));
#342157=CARTESIAN_POINT('Ctrl Pts',(3.95990297199994,5.2,1.84894083999998));
#342158=CARTESIAN_POINT('Ctrl Pts',(3.95990297199994,2.2,1.84894083999998));
#342159=CARTESIAN_POINT('Ctrl Pts',(3.95793084199994,12.2,1.84890295799998));
#342160=CARTESIAN_POINT('Ctrl Pts',(3.95793084199994,5.2,1.84890295799998));
#342161=CARTESIAN_POINT('Ctrl Pts',(3.95793084199994,2.2,1.84890295799998));
#342162=CARTESIAN_POINT('Ctrl Pts',(3.95596286399994,12.2,1.84886296599998));
#342163=CARTESIAN_POINT('Ctrl Pts',(3.95596286399994,5.2,1.84886296599998));
#342164=CARTESIAN_POINT('Ctrl Pts',(3.95596286399994,2.2,1.84886296599998));
#342165=CARTESIAN_POINT('Ctrl Pts',(3.95399904299994,12.2,1.84882086999998));
#342166=CARTESIAN_POINT('Ctrl Pts',(3.95399904299994,5.2,1.84882086999998));
#342167=CARTESIAN_POINT('Ctrl Pts',(3.95399904299994,2.2,1.84882086999998));
#342168=CARTESIAN_POINT('Ctrl Pts',(3.95203938799995,12.2,1.84877667999999));
#342169=CARTESIAN_POINT('Ctrl Pts',(3.95203938799995,5.2,1.84877667999999));
#342170=CARTESIAN_POINT('Ctrl Pts',(3.95203938799995,2.2,1.84877667999999));
#342171=CARTESIAN_POINT('Ctrl Pts',(3.95008390499994,12.2,1.84873040199999));
#342172=CARTESIAN_POINT('Ctrl Pts',(3.95008390499994,5.2,1.84873040199999));
#342173=CARTESIAN_POINT('Ctrl Pts',(3.95008390499994,2.2,1.84873040199999));
#342174=CARTESIAN_POINT('Ctrl Pts',(3.94813260099994,12.2,1.84868204799999));
#342175=CARTESIAN_POINT('Ctrl Pts',(3.94813260099994,5.2,1.84868204799999));
#342176=CARTESIAN_POINT('Ctrl Pts',(3.94813260099994,2.2,1.84868204799999));
#342177=CARTESIAN_POINT('Ctrl Pts',(3.94618548399994,12.2,1.84863162399999));
#342178=CARTESIAN_POINT('Ctrl Pts',(3.94618548399994,5.2,1.84863162399999));
#342179=CARTESIAN_POINT('Ctrl Pts',(3.94618548399994,2.2,1.84863162399999));
#342180=CARTESIAN_POINT('Ctrl Pts',(3.94424256099994,12.2,1.84857913799998));
#342181=CARTESIAN_POINT('Ctrl Pts',(3.94424256099994,5.2,1.84857913799998));
#342182=CARTESIAN_POINT('Ctrl Pts',(3.94424256099994,2.2,1.84857913799998));
#342183=CARTESIAN_POINT('Ctrl Pts',(3.94230383899994,12.2,1.84852459999998));
#342184=CARTESIAN_POINT('Ctrl Pts',(3.94230383899994,5.2,1.84852459999998));
#342185=CARTESIAN_POINT('Ctrl Pts',(3.94230383899994,2.2,1.84852459999998));
#342186=CARTESIAN_POINT('Ctrl Pts',(3.94036932599994,12.2,1.84846801799999));
#342187=CARTESIAN_POINT('Ctrl Pts',(3.94036932599994,5.2,1.84846801799999));
#342188=CARTESIAN_POINT('Ctrl Pts',(3.94036932599994,2.2,1.84846801799999));
#342189=CARTESIAN_POINT('Ctrl Pts',(3.93843902799994,12.2,1.84840940099999));
#342190=CARTESIAN_POINT('Ctrl Pts',(3.93843902799994,5.2,1.84840940099999));
#342191=CARTESIAN_POINT('Ctrl Pts',(3.93843902799994,2.2,1.84840940099999));
#342192=CARTESIAN_POINT('Ctrl Pts',(3.93651295199994,12.2,1.84834875699998));
#342193=CARTESIAN_POINT('Ctrl Pts',(3.93651295199994,5.2,1.84834875699998));
#342194=CARTESIAN_POINT('Ctrl Pts',(3.93651295199994,2.2,1.84834875699998));
#342195=CARTESIAN_POINT('Ctrl Pts',(3.93459110599994,12.2,1.84828609399998));
#342196=CARTESIAN_POINT('Ctrl Pts',(3.93459110599994,5.2,1.84828609399998));
#342197=CARTESIAN_POINT('Ctrl Pts',(3.93459110599994,2.2,1.84828609399998));
#342198=CARTESIAN_POINT('Ctrl Pts',(3.93267349599994,12.2,1.84822142199998));
#342199=CARTESIAN_POINT('Ctrl Pts',(3.93267349599994,5.2,1.84822142199998));
#342200=CARTESIAN_POINT('Ctrl Pts',(3.93267349599994,2.2,1.84822142199998));
#342201=CARTESIAN_POINT('Ctrl Pts',(3.93076013199994,12.2,1.84815474899999));
#342202=CARTESIAN_POINT('Ctrl Pts',(3.93076013199994,5.2,1.84815474899999));
#342203=CARTESIAN_POINT('Ctrl Pts',(3.93076013199994,2.2,1.84815474899999));
#342204=CARTESIAN_POINT('Ctrl Pts',(3.92885101799994,12.2,1.84808608399999));
#342205=CARTESIAN_POINT('Ctrl Pts',(3.92885101799994,5.2,1.84808608399999));
#342206=CARTESIAN_POINT('Ctrl Pts',(3.92885101799994,2.2,1.84808608399999));
#342207=CARTESIAN_POINT('Ctrl Pts',(3.92694616199994,12.2,1.84801543499999));
#342208=CARTESIAN_POINT('Ctrl Pts',(3.92694616199994,5.2,1.84801543499999));
#342209=CARTESIAN_POINT('Ctrl Pts',(3.92694616199994,2.2,1.84801543499999));
#342210=CARTESIAN_POINT('Ctrl Pts',(3.92504557199994,12.2,1.84794281199999));
#342211=CARTESIAN_POINT('Ctrl Pts',(3.92504557199994,5.2,1.84794281199999));
#342212=CARTESIAN_POINT('Ctrl Pts',(3.92504557199994,2.2,1.84794281199999));
#342213=CARTESIAN_POINT('Ctrl Pts',(3.92314925599994,12.2,1.84786822199999));
#342214=CARTESIAN_POINT('Ctrl Pts',(3.92314925599994,5.2,1.84786822199999));
#342215=CARTESIAN_POINT('Ctrl Pts',(3.92314925599994,2.2,1.84786822199999));
#342216=CARTESIAN_POINT('Ctrl Pts',(3.92125721899994,12.2,1.84779167499999));
#342217=CARTESIAN_POINT('Ctrl Pts',(3.92125721899994,5.2,1.84779167499999));
#342218=CARTESIAN_POINT('Ctrl Pts',(3.92125721899994,2.2,1.84779167499999));
#342219=CARTESIAN_POINT('Ctrl Pts',(3.91936946799994,12.2,1.84771317899999));
#342220=CARTESIAN_POINT('Ctrl Pts',(3.91936946799994,5.2,1.84771317899999));
#342221=CARTESIAN_POINT('Ctrl Pts',(3.91936946799994,2.2,1.84771317899999));
#342222=CARTESIAN_POINT('Ctrl Pts',(3.91748601299994,12.2,1.84763274399999));
#342223=CARTESIAN_POINT('Ctrl Pts',(3.91748601299994,5.2,1.84763274399999));
#342224=CARTESIAN_POINT('Ctrl Pts',(3.91748601299994,2.2,1.84763274399999));
#342225=CARTESIAN_POINT('Ctrl Pts',(3.91560685799994,12.2,1.84755037699999));
#342226=CARTESIAN_POINT('Ctrl Pts',(3.91560685799994,5.2,1.84755037699999));
#342227=CARTESIAN_POINT('Ctrl Pts',(3.91560685799994,2.2,1.84755037699999));
#342228=CARTESIAN_POINT('Ctrl Pts',(3.91373201199994,12.2,1.84746608899998));
#342229=CARTESIAN_POINT('Ctrl Pts',(3.91373201199994,5.2,1.84746608899998));
#342230=CARTESIAN_POINT('Ctrl Pts',(3.91373201199994,2.2,1.84746608899998));
#342231=CARTESIAN_POINT('Ctrl Pts',(3.91186148299994,12.2,1.84737988799998));
#342232=CARTESIAN_POINT('Ctrl Pts',(3.91186148299994,5.2,1.84737988799998));
#342233=CARTESIAN_POINT('Ctrl Pts',(3.91186148299994,2.2,1.84737988799998));
#342234=CARTESIAN_POINT('Ctrl Pts',(3.90999527499994,12.2,1.84729178299999));
#342235=CARTESIAN_POINT('Ctrl Pts',(3.90999527499994,5.2,1.84729178299999));
#342236=CARTESIAN_POINT('Ctrl Pts',(3.90999527499994,2.2,1.84729178299999));
#342237=CARTESIAN_POINT('Ctrl Pts',(3.90813339899994,12.2,1.84720178199999));
#342238=CARTESIAN_POINT('Ctrl Pts',(3.90813339899994,5.2,1.84720178199999));
#342239=CARTESIAN_POINT('Ctrl Pts',(3.90813339899994,2.2,1.84720178199999));
#342240=CARTESIAN_POINT('Ctrl Pts',(3.90627585999994,12.2,1.84710989499999));
#342241=CARTESIAN_POINT('Ctrl Pts',(3.90627585999994,5.2,1.84710989499999));
#342242=CARTESIAN_POINT('Ctrl Pts',(3.90627585999994,2.2,1.84710989499999));
#342243=CARTESIAN_POINT('Ctrl Pts',(3.90442266399994,12.2,1.84701613099998));
#342244=CARTESIAN_POINT('Ctrl Pts',(3.90442266399994,5.2,1.84701613099998));
#342245=CARTESIAN_POINT('Ctrl Pts',(3.90442266399994,2.2,1.84701613099998));
#342246=CARTESIAN_POINT('Ctrl Pts',(3.90257382099994,12.2,1.84692049799999));
#342247=CARTESIAN_POINT('Ctrl Pts',(3.90257382099994,5.2,1.84692049799999));
#342248=CARTESIAN_POINT('Ctrl Pts',(3.90257382099994,2.2,1.84692049799999));
#342249=CARTESIAN_POINT('Ctrl Pts',(3.90072933599994,12.2,1.84682300599999));
#342250=CARTESIAN_POINT('Ctrl Pts',(3.90072933599994,5.2,1.84682300599999));
#342251=CARTESIAN_POINT('Ctrl Pts',(3.90072933599994,2.2,1.84682300599999));
#342252=CARTESIAN_POINT('Ctrl Pts',(3.89888921699994,12.2,1.84672366499999));
#342253=CARTESIAN_POINT('Ctrl Pts',(3.89888921699994,5.2,1.84672366499999));
#342254=CARTESIAN_POINT('Ctrl Pts',(3.89888921699994,2.2,1.84672366499999));
#342255=CARTESIAN_POINT('Ctrl Pts',(3.89705347199994,12.2,1.84662248199999));
#342256=CARTESIAN_POINT('Ctrl Pts',(3.89705347199994,5.2,1.84662248199999));
#342257=CARTESIAN_POINT('Ctrl Pts',(3.89705347199994,2.2,1.84662248199999));
#342258=CARTESIAN_POINT('Ctrl Pts',(3.89522210699994,12.2,1.84651946599999));
#342259=CARTESIAN_POINT('Ctrl Pts',(3.89522210699994,5.2,1.84651946599999));
#342260=CARTESIAN_POINT('Ctrl Pts',(3.89522210699994,2.2,1.84651946599999));
#342261=CARTESIAN_POINT('Ctrl Pts',(3.89339512899994,12.2,1.84641462899998));
#342262=CARTESIAN_POINT('Ctrl Pts',(3.89339512899994,5.2,1.84641462899998));
#342263=CARTESIAN_POINT('Ctrl Pts',(3.89339512899994,2.2,1.84641462899998));
#342264=CARTESIAN_POINT('Ctrl Pts',(3.89157254599994,12.2,1.84630797799999));
#342265=CARTESIAN_POINT('Ctrl Pts',(3.89157254599994,5.2,1.84630797799999));
#342266=CARTESIAN_POINT('Ctrl Pts',(3.89157254599994,2.2,1.84630797799999));
#342267=CARTESIAN_POINT('Ctrl Pts',(3.88975436499994,12.2,1.84619952299999));
#342268=CARTESIAN_POINT('Ctrl Pts',(3.88975436499994,5.2,1.84619952299999));
#342269=CARTESIAN_POINT('Ctrl Pts',(3.88975436499994,2.2,1.84619952299999));
#342270=CARTESIAN_POINT('Ctrl Pts',(3.88794059199994,12.2,1.84608927199998));
#342271=CARTESIAN_POINT('Ctrl Pts',(3.88794059199994,5.2,1.84608927199998));
#342272=CARTESIAN_POINT('Ctrl Pts',(3.88794059199994,2.2,1.84608927199998));
#342273=CARTESIAN_POINT('Ctrl Pts',(3.88613123699994,12.2,1.84597723499999));
#342274=CARTESIAN_POINT('Ctrl Pts',(3.88613123699994,5.2,1.84597723499999));
#342275=CARTESIAN_POINT('Ctrl Pts',(3.88613123699994,2.2,1.84597723499999));
#342276=CARTESIAN_POINT('Ctrl Pts',(3.88432630399994,12.2,1.84586342199998));
#342277=CARTESIAN_POINT('Ctrl Pts',(3.88432630399994,5.2,1.84586342199998));
#342278=CARTESIAN_POINT('Ctrl Pts',(3.88432630399994,2.2,1.84586342199998));
#342279=CARTESIAN_POINT('Ctrl Pts',(3.88252580199994,12.2,1.84574784099999));
#342280=CARTESIAN_POINT('Ctrl Pts',(3.88252580199994,5.2,1.84574784099999));
#342281=CARTESIAN_POINT('Ctrl Pts',(3.88252580199994,2.2,1.84574784099999));
#342282=CARTESIAN_POINT('Ctrl Pts',(3.88072973799995,12.2,1.84563050199999));
#342283=CARTESIAN_POINT('Ctrl Pts',(3.88072973799995,5.2,1.84563050199999));
#342284=CARTESIAN_POINT('Ctrl Pts',(3.88072973799995,2.2,1.84563050199999));
#342285=CARTESIAN_POINT('Ctrl Pts',(3.87893811799994,12.2,1.84551141499998));
#342286=CARTESIAN_POINT('Ctrl Pts',(3.87893811799994,5.2,1.84551141499998));
#342287=CARTESIAN_POINT('Ctrl Pts',(3.87893811799994,2.2,1.84551141499998));
#342288=CARTESIAN_POINT('Ctrl Pts',(3.87715095099994,12.2,1.84539058799999));
#342289=CARTESIAN_POINT('Ctrl Pts',(3.87715095099994,5.2,1.84539058799999));
#342290=CARTESIAN_POINT('Ctrl Pts',(3.87715095099994,2.2,1.84539058799999));
#342291=CARTESIAN_POINT('Ctrl Pts',(3.87536824199994,12.2,1.84526803199998));
#342292=CARTESIAN_POINT('Ctrl Pts',(3.87536824199994,5.2,1.84526803199998));
#342293=CARTESIAN_POINT('Ctrl Pts',(3.87536824199994,2.2,1.84526803199998));
#342294=CARTESIAN_POINT('Ctrl Pts',(3.87359000099994,12.2,1.84514375499999));
#342295=CARTESIAN_POINT('Ctrl Pts',(3.87359000099994,5.2,1.84514375499999));
#342296=CARTESIAN_POINT('Ctrl Pts',(3.87359000099994,2.2,1.84514375499999));
#342297=CARTESIAN_POINT('Ctrl Pts',(3.87181623199994,12.2,1.84501776699999));
#342298=CARTESIAN_POINT('Ctrl Pts',(3.87181623199994,5.2,1.84501776699999));
#342299=CARTESIAN_POINT('Ctrl Pts',(3.87181623199994,2.2,1.84501776699999));
#342300=CARTESIAN_POINT('Ctrl Pts',(3.87004694499994,12.2,1.84489007799999));
#342301=CARTESIAN_POINT('Ctrl Pts',(3.87004694499994,5.2,1.84489007799999));
#342302=CARTESIAN_POINT('Ctrl Pts',(3.87004694499994,2.2,1.84489007799999));
#342303=CARTESIAN_POINT('Ctrl Pts',(3.86828214499995,12.2,1.84476069599999));
#342304=CARTESIAN_POINT('Ctrl Pts',(3.86828214499995,5.2,1.84476069599999));
#342305=CARTESIAN_POINT('Ctrl Pts',(3.86828214499995,2.2,1.84476069599999));
#342306=CARTESIAN_POINT('Ctrl Pts',(3.86652183999994,12.2,1.84462963199998));
#342307=CARTESIAN_POINT('Ctrl Pts',(3.86652183999994,5.2,1.84462963199998));
#342308=CARTESIAN_POINT('Ctrl Pts',(3.86652183999994,2.2,1.84462963199998));
#342309=CARTESIAN_POINT('Ctrl Pts',(3.86476603699994,12.2,1.84449689599999));
#342310=CARTESIAN_POINT('Ctrl Pts',(3.86476603699994,5.2,1.84449689599999));
#342311=CARTESIAN_POINT('Ctrl Pts',(3.86476603699994,2.2,1.84449689599999));
#342312=CARTESIAN_POINT('Ctrl Pts',(3.86301474399994,12.2,1.84436249499999));
#342313=CARTESIAN_POINT('Ctrl Pts',(3.86301474399994,5.2,1.84436249499999));
#342314=CARTESIAN_POINT('Ctrl Pts',(3.86301474399994,2.2,1.84436249499999));
#342315=CARTESIAN_POINT('Ctrl Pts',(3.86126796699994,12.2,1.84422644199998));
#342316=CARTESIAN_POINT('Ctrl Pts',(3.86126796699994,5.2,1.84422644199998));
#342317=CARTESIAN_POINT('Ctrl Pts',(3.86126796699994,2.2,1.84422644199998));
#342318=CARTESIAN_POINT('Ctrl Pts',(3.85952571499994,12.2,1.84408874499999));
#342319=CARTESIAN_POINT('Ctrl Pts',(3.85952571499994,5.2,1.84408874499999));
#342320=CARTESIAN_POINT('Ctrl Pts',(3.85952571499994,2.2,1.84408874499999));
#342321=CARTESIAN_POINT('Ctrl Pts',(3.85778799299994,12.2,1.84394941199999));
#342322=CARTESIAN_POINT('Ctrl Pts',(3.85778799299994,5.2,1.84394941199999));
#342323=CARTESIAN_POINT('Ctrl Pts',(3.85778799299994,2.2,1.84394941199999));
#342324=CARTESIAN_POINT('Ctrl Pts',(3.85605480899994,12.2,1.84380845599998));
#342325=CARTESIAN_POINT('Ctrl Pts',(3.85605480899994,5.2,1.84380845599998));
#342326=CARTESIAN_POINT('Ctrl Pts',(3.85605480899994,2.2,1.84380845599998));
#342327=CARTESIAN_POINT('Ctrl Pts',(3.85432616999994,12.2,1.84366588399998));
#342328=CARTESIAN_POINT('Ctrl Pts',(3.85432616999994,5.2,1.84366588399998));
#342329=CARTESIAN_POINT('Ctrl Pts',(3.85432616999994,2.2,1.84366588399998));
#342330=CARTESIAN_POINT('Ctrl Pts',(3.85260208399994,12.2,1.84352170699999));
#342331=CARTESIAN_POINT('Ctrl Pts',(3.85260208399994,5.2,1.84352170699999));
#342332=CARTESIAN_POINT('Ctrl Pts',(3.85260208399994,2.2,1.84352170699999));
#342333=CARTESIAN_POINT('Ctrl Pts',(3.85088255699995,12.2,1.84337593499999));
#342334=CARTESIAN_POINT('Ctrl Pts',(3.85088255699995,5.2,1.84337593499999));
#342335=CARTESIAN_POINT('Ctrl Pts',(3.85088255699995,2.2,1.84337593499999));
#342336=CARTESIAN_POINT('Ctrl Pts',(3.84916759799994,12.2,1.84322857799998));
#342337=CARTESIAN_POINT('Ctrl Pts',(3.84916759799994,5.2,1.84322857799998));
#342338=CARTESIAN_POINT('Ctrl Pts',(3.84916759799994,2.2,1.84322857799998));
#342339=CARTESIAN_POINT('Ctrl Pts',(3.84745721099994,12.2,1.84307964399999));
#342340=CARTESIAN_POINT('Ctrl Pts',(3.84745721099994,5.2,1.84307964399999));
#342341=CARTESIAN_POINT('Ctrl Pts',(3.84745721099994,2.2,1.84307964399999));
#342342=CARTESIAN_POINT('Ctrl Pts',(3.84575140599994,12.2,1.84292914499999));
#342343=CARTESIAN_POINT('Ctrl Pts',(3.84575140599994,5.2,1.84292914499999));
#342344=CARTESIAN_POINT('Ctrl Pts',(3.84575140599994,2.2,1.84292914499999));
#342345=CARTESIAN_POINT('Ctrl Pts',(3.84405018899994,12.2,1.84277708999999));
#342346=CARTESIAN_POINT('Ctrl Pts',(3.84405018899994,5.2,1.84277708999999));
#342347=CARTESIAN_POINT('Ctrl Pts',(3.84405018899994,2.2,1.84277708999999));
#342348=CARTESIAN_POINT('Ctrl Pts',(3.84235356799994,12.2,1.84262348899999));
#342349=CARTESIAN_POINT('Ctrl Pts',(3.84235356799994,5.2,1.84262348899999));
#342350=CARTESIAN_POINT('Ctrl Pts',(3.84235356799994,2.2,1.84262348899999));
#342351=CARTESIAN_POINT('Ctrl Pts',(3.84066154899994,12.2,1.84246835099998));
#342352=CARTESIAN_POINT('Ctrl Pts',(3.84066154899994,5.2,1.84246835099998));
#342353=CARTESIAN_POINT('Ctrl Pts',(3.84066154899994,2.2,1.84246835099998));
#342354=CARTESIAN_POINT('Ctrl Pts',(3.83897413999994,12.2,1.84231168799998));
#342355=CARTESIAN_POINT('Ctrl Pts',(3.83897413999994,5.2,1.84231168799998));
#342356=CARTESIAN_POINT('Ctrl Pts',(3.83897413999994,2.2,1.84231168799998));
#342357=CARTESIAN_POINT('Ctrl Pts',(3.83729134699994,12.2,1.84215350799999));
#342358=CARTESIAN_POINT('Ctrl Pts',(3.83729134699994,5.2,1.84215350799999));
#342359=CARTESIAN_POINT('Ctrl Pts',(3.83729134699994,2.2,1.84215350799999));
#342360=CARTESIAN_POINT('Ctrl Pts',(3.83561317899995,12.2,1.84199382299999));
#342361=CARTESIAN_POINT('Ctrl Pts',(3.83561317899995,5.2,1.84199382299999));
#342362=CARTESIAN_POINT('Ctrl Pts',(3.83561317899995,2.2,1.84199382299999));
#342363=CARTESIAN_POINT('Ctrl Pts',(3.83393964199994,12.2,1.84183264099998));
#342364=CARTESIAN_POINT('Ctrl Pts',(3.83393964199994,5.2,1.84183264099998));
#342365=CARTESIAN_POINT('Ctrl Pts',(3.83393964199994,2.2,1.84183264099998));
#342366=CARTESIAN_POINT('Ctrl Pts',(3.83227074399994,12.2,1.84166997299998));
#342367=CARTESIAN_POINT('Ctrl Pts',(3.83227074399994,5.2,1.84166997299998));
#342368=CARTESIAN_POINT('Ctrl Pts',(3.83227074399994,2.2,1.84166997299998));
#342369=CARTESIAN_POINT('Ctrl Pts',(3.83060648999995,12.2,1.84150582999999));
#342370=CARTESIAN_POINT('Ctrl Pts',(3.83060648999995,5.2,1.84150582999999));
#342371=CARTESIAN_POINT('Ctrl Pts',(3.83060648999995,2.2,1.84150582999999));
#342372=CARTESIAN_POINT('Ctrl Pts',(3.82894688999994,12.2,1.84134021999999));
#342373=CARTESIAN_POINT('Ctrl Pts',(3.82894688999994,5.2,1.84134021999999));
#342374=CARTESIAN_POINT('Ctrl Pts',(3.82894688999994,2.2,1.84134021999999));
#342375=CARTESIAN_POINT('Ctrl Pts',(3.82729194999994,12.2,1.84117315599998));
#342376=CARTESIAN_POINT('Ctrl Pts',(3.82729194999994,5.2,1.84117315599998));
#342377=CARTESIAN_POINT('Ctrl Pts',(3.82729194999994,2.2,1.84117315599998));
#342378=CARTESIAN_POINT('Ctrl Pts',(3.82564167599994,12.2,1.84100464599998));
#342379=CARTESIAN_POINT('Ctrl Pts',(3.82564167599994,5.2,1.84100464599998));
#342380=CARTESIAN_POINT('Ctrl Pts',(3.82564167599994,2.2,1.84100464599998));
#342381=CARTESIAN_POINT('Ctrl Pts',(3.82399607699994,12.2,1.84083470099999));
#342382=CARTESIAN_POINT('Ctrl Pts',(3.82399607699994,5.2,1.84083470099999));
#342383=CARTESIAN_POINT('Ctrl Pts',(3.82399607699994,2.2,1.84083470099999));
#342384=CARTESIAN_POINT('Ctrl Pts',(3.82235515999994,12.2,1.84066333199999));
#342385=CARTESIAN_POINT('Ctrl Pts',(3.82235515999994,5.2,1.84066333199999));
#342386=CARTESIAN_POINT('Ctrl Pts',(3.82235515999994,2.2,1.84066333199999));
#342387=CARTESIAN_POINT('Ctrl Pts',(3.82071892999994,12.2,1.84049054699999));
#342388=CARTESIAN_POINT('Ctrl Pts',(3.82071892999994,5.2,1.84049054699999));
#342389=CARTESIAN_POINT('Ctrl Pts',(3.82071892999994,2.2,1.84049054699999));
#342390=CARTESIAN_POINT('Ctrl Pts',(3.81908739599994,12.2,1.84031635899998));
#342391=CARTESIAN_POINT('Ctrl Pts',(3.81908739599994,5.2,1.84031635899998));
#342392=CARTESIAN_POINT('Ctrl Pts',(3.81908739599994,2.2,1.84031635899998));
#342393=CARTESIAN_POINT('Ctrl Pts',(3.81746056499995,12.2,1.84014077599999));
#342394=CARTESIAN_POINT('Ctrl Pts',(3.81746056499995,5.2,1.84014077599999));
#342395=CARTESIAN_POINT('Ctrl Pts',(3.81746056499995,2.2,1.84014077599999));
#342396=CARTESIAN_POINT('Ctrl Pts',(3.81583844399994,12.2,1.83996380999998));
#342397=CARTESIAN_POINT('Ctrl Pts',(3.81583844399994,5.2,1.83996380999998));
#342398=CARTESIAN_POINT('Ctrl Pts',(3.81583844399994,2.2,1.83996380999998));
#342399=CARTESIAN_POINT('Ctrl Pts',(3.81422104099994,12.2,1.83978547199999));
#342400=CARTESIAN_POINT('Ctrl Pts',(3.81422104099994,5.2,1.83978547199999));
#342401=CARTESIAN_POINT('Ctrl Pts',(3.81422104099994,2.2,1.83978547199999));
#342402=CARTESIAN_POINT('Ctrl Pts',(3.81260836099994,12.2,1.83960576999999));
#342403=CARTESIAN_POINT('Ctrl Pts',(3.81260836099994,5.2,1.83960576999999));
#342404=CARTESIAN_POINT('Ctrl Pts',(3.81260836099994,2.2,1.83960576999999));
#342405=CARTESIAN_POINT('Ctrl Pts',(3.81100041299994,12.2,1.83942471699998));
#342406=CARTESIAN_POINT('Ctrl Pts',(3.81100041299994,5.2,1.83942471699998));
#342407=CARTESIAN_POINT('Ctrl Pts',(3.81100041299994,2.2,1.83942471699998));
#342408=CARTESIAN_POINT('Ctrl Pts',(3.80939720399994,12.2,1.83924232099999));
#342409=CARTESIAN_POINT('Ctrl Pts',(3.80939720399994,5.2,1.83924232099999));
#342410=CARTESIAN_POINT('Ctrl Pts',(3.80939720399994,2.2,1.83924232099999));
#342411=CARTESIAN_POINT('Ctrl Pts',(3.80779873999994,12.2,1.83905859499998));
#342412=CARTESIAN_POINT('Ctrl Pts',(3.80779873999994,5.2,1.83905859499998));
#342413=CARTESIAN_POINT('Ctrl Pts',(3.80779873999994,2.2,1.83905859499998));
#342414=CARTESIAN_POINT('Ctrl Pts',(3.80620502999994,12.2,1.83887354799999));
#342415=CARTESIAN_POINT('Ctrl Pts',(3.80620502999994,5.2,1.83887354799999));
#342416=CARTESIAN_POINT('Ctrl Pts',(3.80620502999994,2.2,1.83887354799999));
#342417=CARTESIAN_POINT('Ctrl Pts',(3.80461607899994,12.2,1.83868719099999));
#342418=CARTESIAN_POINT('Ctrl Pts',(3.80461607899994,5.2,1.83868719099999));
#342419=CARTESIAN_POINT('Ctrl Pts',(3.80461607899994,2.2,1.83868719099999));
#342420=CARTESIAN_POINT('Ctrl Pts',(3.80303189599994,12.2,1.83849953499998));
#342421=CARTESIAN_POINT('Ctrl Pts',(3.80303189599994,5.2,1.83849953499998));
#342422=CARTESIAN_POINT('Ctrl Pts',(3.80303189599994,2.2,1.83849953499998));
#342423=CARTESIAN_POINT('Ctrl Pts',(3.80145248699994,12.2,1.83831058999999));
#342424=CARTESIAN_POINT('Ctrl Pts',(3.80145248699994,5.2,1.83831058999999));
#342425=CARTESIAN_POINT('Ctrl Pts',(3.80145248699994,2.2,1.83831058999999));
#342426=CARTESIAN_POINT('Ctrl Pts',(3.79987785999994,12.2,1.83812036699999));
#342427=CARTESIAN_POINT('Ctrl Pts',(3.79987785999994,5.2,1.83812036699999));
#342428=CARTESIAN_POINT('Ctrl Pts',(3.79987785999994,2.2,1.83812036699999));
#342429=CARTESIAN_POINT('Ctrl Pts',(3.79830802199994,12.2,1.83792887599999));
#342430=CARTESIAN_POINT('Ctrl Pts',(3.79830802199994,5.2,1.83792887599999));
#342431=CARTESIAN_POINT('Ctrl Pts',(3.79830802199994,2.2,1.83792887599999));
#342432=CARTESIAN_POINT('Ctrl Pts',(3.79674297899994,12.2,1.83773612999999));
#342433=CARTESIAN_POINT('Ctrl Pts',(3.79674297899994,5.2,1.83773612999999));
#342434=CARTESIAN_POINT('Ctrl Pts',(3.79674297899994,2.2,1.83773612999999));
#342435=CARTESIAN_POINT('Ctrl Pts',(3.79518273999994,12.2,1.83754213599999));
#342436=CARTESIAN_POINT('Ctrl Pts',(3.79518273999994,5.2,1.83754213599999));
#342437=CARTESIAN_POINT('Ctrl Pts',(3.79518273999994,2.2,1.83754213599999));
#342438=CARTESIAN_POINT('Ctrl Pts',(3.79362730999994,12.2,1.83734690799998));
#342439=CARTESIAN_POINT('Ctrl Pts',(3.79362730999994,5.2,1.83734690799998));
#342440=CARTESIAN_POINT('Ctrl Pts',(3.79362730999994,2.2,1.83734690799998));
#342441=CARTESIAN_POINT('Ctrl Pts',(3.79207669799994,12.2,1.83715045699998));
#342442=CARTESIAN_POINT('Ctrl Pts',(3.79207669799994,5.2,1.83715045699998));
#342443=CARTESIAN_POINT('Ctrl Pts',(3.79207669799994,2.2,1.83715045699998));
#342444=CARTESIAN_POINT('Ctrl Pts',(3.79053090999994,12.2,1.83695279099998));
#342445=CARTESIAN_POINT('Ctrl Pts',(3.79053090999994,5.2,1.83695279099998));
#342446=CARTESIAN_POINT('Ctrl Pts',(3.79053090999994,2.2,1.83695279099998));
#342447=CARTESIAN_POINT('Ctrl Pts',(3.78898995399994,12.2,1.83675392399998));
#342448=CARTESIAN_POINT('Ctrl Pts',(3.78898995399994,5.2,1.83675392399998));
#342449=CARTESIAN_POINT('Ctrl Pts',(3.78898995399994,2.2,1.83675392399998));
#342450=CARTESIAN_POINT('Ctrl Pts',(3.78745383699994,12.2,1.83655386399999));
#342451=CARTESIAN_POINT('Ctrl Pts',(3.78745383699994,5.2,1.83655386399999));
#342452=CARTESIAN_POINT('Ctrl Pts',(3.78745383699994,2.2,1.83655386399999));
#342453=CARTESIAN_POINT('Ctrl Pts',(3.78592256599994,12.2,1.83635262399998));
#342454=CARTESIAN_POINT('Ctrl Pts',(3.78592256599994,5.2,1.83635262399998));
#342455=CARTESIAN_POINT('Ctrl Pts',(3.78592256599994,2.2,1.83635262399998));
#342456=CARTESIAN_POINT('Ctrl Pts',(3.78439614799994,12.2,1.83615021499998));
#342457=CARTESIAN_POINT('Ctrl Pts',(3.78439614799994,5.2,1.83615021499998));
#342458=CARTESIAN_POINT('Ctrl Pts',(3.78439614799994,2.2,1.83615021499998));
#342459=CARTESIAN_POINT('Ctrl Pts',(3.78287458899994,12.2,1.83594664599998));
#342460=CARTESIAN_POINT('Ctrl Pts',(3.78287458899994,5.2,1.83594664599998));
#342461=CARTESIAN_POINT('Ctrl Pts',(3.78287458899994,2.2,1.83594664599998));
#342462=CARTESIAN_POINT('Ctrl Pts',(3.78135789899994,12.2,1.83574193099998));
#342463=CARTESIAN_POINT('Ctrl Pts',(3.78135789899994,5.2,1.83574193099998));
#342464=CARTESIAN_POINT('Ctrl Pts',(3.78135789899994,2.2,1.83574193099998));
#342465=CARTESIAN_POINT('Ctrl Pts',(3.77984608399994,12.2,1.83553607799999));
#342466=CARTESIAN_POINT('Ctrl Pts',(3.77984608399994,5.2,1.83553607799999));
#342467=CARTESIAN_POINT('Ctrl Pts',(3.77984608399994,2.2,1.83553607799999));
#342468=CARTESIAN_POINT('Ctrl Pts',(3.77833914899994,12.2,1.83532910099999));
#342469=CARTESIAN_POINT('Ctrl Pts',(3.77833914899994,5.2,1.83532910099999));
#342470=CARTESIAN_POINT('Ctrl Pts',(3.77833914899994,2.2,1.83532910099999));
#342471=CARTESIAN_POINT('Ctrl Pts',(3.77683710299995,12.2,1.83512100899998));
#342472=CARTESIAN_POINT('Ctrl Pts',(3.77683710299995,5.2,1.83512100899998));
#342473=CARTESIAN_POINT('Ctrl Pts',(3.77683710299995,2.2,1.83512100899998));
#342474=CARTESIAN_POINT('Ctrl Pts',(3.77533995399994,12.2,1.83491181399999));
#342475=CARTESIAN_POINT('Ctrl Pts',(3.77533995399994,5.2,1.83491181399999));
#342476=CARTESIAN_POINT('Ctrl Pts',(3.77533995399994,2.2,1.83491181399999));
#342477=CARTESIAN_POINT('Ctrl Pts',(3.77384770799994,12.2,1.83470152699998));
#342478=CARTESIAN_POINT('Ctrl Pts',(3.77384770799994,5.2,1.83470152699998));
#342479=CARTESIAN_POINT('Ctrl Pts',(3.77384770799994,2.2,1.83470152699998));
#342480=CARTESIAN_POINT('Ctrl Pts',(3.77236037099994,12.2,1.83449015999999));
#342481=CARTESIAN_POINT('Ctrl Pts',(3.77236037099994,5.2,1.83449015999999));
#342482=CARTESIAN_POINT('Ctrl Pts',(3.77236037099994,2.2,1.83449015999999));
#342483=CARTESIAN_POINT('Ctrl Pts',(3.77087795299994,12.2,1.83427772399999));
#342484=CARTESIAN_POINT('Ctrl Pts',(3.77087795299994,5.2,1.83427772399999));
#342485=CARTESIAN_POINT('Ctrl Pts',(3.77087795299994,2.2,1.83427772399999));
#342486=CARTESIAN_POINT('Ctrl Pts',(3.76940045799994,12.2,1.83406422899999));
#342487=CARTESIAN_POINT('Ctrl Pts',(3.76940045799994,5.2,1.83406422899999));
#342488=CARTESIAN_POINT('Ctrl Pts',(3.76940045799994,2.2,1.83406422899999));
#342489=CARTESIAN_POINT('Ctrl Pts',(3.76792789499994,12.2,1.83384968799999));
#342490=CARTESIAN_POINT('Ctrl Pts',(3.76792789499994,5.2,1.83384968799999));
#342491=CARTESIAN_POINT('Ctrl Pts',(3.76792789499994,2.2,1.83384968799999));
#342492=CARTESIAN_POINT('Ctrl Pts',(3.76646027099994,12.2,1.83363411099998));
#342493=CARTESIAN_POINT('Ctrl Pts',(3.76646027099994,5.2,1.83363411099998));
#342494=CARTESIAN_POINT('Ctrl Pts',(3.76646027099994,2.2,1.83363411099998));
#342495=CARTESIAN_POINT('Ctrl Pts',(3.76499759399994,12.2,1.83341750999999));
#342496=CARTESIAN_POINT('Ctrl Pts',(3.76499759399994,5.2,1.83341750999999));
#342497=CARTESIAN_POINT('Ctrl Pts',(3.76499759399994,2.2,1.83341750999999));
#342498=CARTESIAN_POINT('Ctrl Pts',(3.76353986899994,12.2,1.83319989699998));
#342499=CARTESIAN_POINT('Ctrl Pts',(3.76353986899994,5.2,1.83319989699998));
#342500=CARTESIAN_POINT('Ctrl Pts',(3.76353986899994,2.2,1.83319989699998));
#342501=CARTESIAN_POINT('Ctrl Pts',(3.76208710599994,12.2,1.83298128299999));
#342502=CARTESIAN_POINT('Ctrl Pts',(3.76208710599994,5.2,1.83298128299999));
#342503=CARTESIAN_POINT('Ctrl Pts',(3.76208710599994,2.2,1.83298128299999));
#342504=CARTESIAN_POINT('Ctrl Pts',(3.76063930899994,12.2,1.83276167899999));
#342505=CARTESIAN_POINT('Ctrl Pts',(3.76063930899994,5.2,1.83276167899999));
#342506=CARTESIAN_POINT('Ctrl Pts',(3.76063930899994,2.2,1.83276167899999));
#342507=CARTESIAN_POINT('Ctrl Pts',(3.75919648599994,12.2,1.83254109699998));
#342508=CARTESIAN_POINT('Ctrl Pts',(3.75919648599994,5.2,1.83254109699998));
#342509=CARTESIAN_POINT('Ctrl Pts',(3.75919648599994,2.2,1.83254109699998));
#342510=CARTESIAN_POINT('Ctrl Pts',(3.75775864499994,12.2,1.83231954999998));
#342511=CARTESIAN_POINT('Ctrl Pts',(3.75775864499994,5.2,1.83231954999998));
#342512=CARTESIAN_POINT('Ctrl Pts',(3.75775864499994,2.2,1.83231954999998));
#342513=CARTESIAN_POINT('Ctrl Pts',(3.75632579299995,12.2,1.83209704599999));
#342514=CARTESIAN_POINT('Ctrl Pts',(3.75632579299995,5.2,1.83209704599999));
#342515=CARTESIAN_POINT('Ctrl Pts',(3.75632579299995,2.2,1.83209704599999));
#342516=CARTESIAN_POINT('Ctrl Pts',(3.75489793799994,12.2,1.83187359999998));
#342517=CARTESIAN_POINT('Ctrl Pts',(3.75489793799994,5.2,1.83187359999998));
#342518=CARTESIAN_POINT('Ctrl Pts',(3.75489793799994,2.2,1.83187359999998));
#342519=CARTESIAN_POINT('Ctrl Pts',(3.75347508399994,12.2,1.83164922199999));
#342520=CARTESIAN_POINT('Ctrl Pts',(3.75347508399994,5.2,1.83164922199999));
#342521=CARTESIAN_POINT('Ctrl Pts',(3.75347508399994,2.2,1.83164922199999));
#342522=CARTESIAN_POINT('Ctrl Pts',(3.75205724199994,12.2,1.83142392399999));
#342523=CARTESIAN_POINT('Ctrl Pts',(3.75205724199994,5.2,1.83142392399999));
#342524=CARTESIAN_POINT('Ctrl Pts',(3.75205724199994,2.2,1.83142392399999));
#342525=CARTESIAN_POINT('Ctrl Pts',(3.75064441599994,12.2,1.83119771799999));
#342526=CARTESIAN_POINT('Ctrl Pts',(3.75064441599994,5.2,1.83119771799999));
#342527=CARTESIAN_POINT('Ctrl Pts',(3.75064441599994,2.2,1.83119771799999));
#342528=CARTESIAN_POINT('Ctrl Pts',(3.74923661499994,12.2,1.83097061599999));
#342529=CARTESIAN_POINT('Ctrl Pts',(3.74923661499994,5.2,1.83097061599999));
#342530=CARTESIAN_POINT('Ctrl Pts',(3.74923661499994,2.2,1.83097061599999));
#342531=CARTESIAN_POINT('Ctrl Pts',(3.74783384499994,12.2,1.83074262899999));
#342532=CARTESIAN_POINT('Ctrl Pts',(3.74783384499994,5.2,1.83074262899999));
#342533=CARTESIAN_POINT('Ctrl Pts',(3.74783384499994,2.2,1.83074262899999));
#342534=CARTESIAN_POINT('Ctrl Pts',(3.74643611499994,12.2,1.83051377099999));
#342535=CARTESIAN_POINT('Ctrl Pts',(3.74643611499994,5.2,1.83051377099999));
#342536=CARTESIAN_POINT('Ctrl Pts',(3.74643611499994,2.2,1.83051377099999));
#342537=CARTESIAN_POINT('Ctrl Pts',(3.74504342999994,12.2,1.83028404999999));
#342538=CARTESIAN_POINT('Ctrl Pts',(3.74504342999994,5.2,1.83028404999999));
#342539=CARTESIAN_POINT('Ctrl Pts',(3.74504342999994,2.2,1.83028404999999));
#342540=CARTESIAN_POINT('Ctrl Pts',(3.74365579899994,12.2,1.83005348099998));
#342541=CARTESIAN_POINT('Ctrl Pts',(3.74365579899994,5.2,1.83005348099998));
#342542=CARTESIAN_POINT('Ctrl Pts',(3.74365579899994,2.2,1.83005348099998));
#342543=CARTESIAN_POINT('Ctrl Pts',(3.74227322699995,12.2,1.82982207499998));
#342544=CARTESIAN_POINT('Ctrl Pts',(3.74227322699995,5.2,1.82982207499998));
#342545=CARTESIAN_POINT('Ctrl Pts',(3.74227322699995,2.2,1.82982207499998));
#342546=CARTESIAN_POINT('Ctrl Pts',(3.74089572299994,12.2,1.82958984299999));
#342547=CARTESIAN_POINT('Ctrl Pts',(3.74089572299994,5.2,1.82958984299999));
#342548=CARTESIAN_POINT('Ctrl Pts',(3.74089572299994,2.2,1.82958984299999));
#342549=CARTESIAN_POINT('Ctrl Pts',(3.73952329299994,12.2,1.82935679899999));
#342550=CARTESIAN_POINT('Ctrl Pts',(3.73952329299994,5.2,1.82935679899999));
#342551=CARTESIAN_POINT('Ctrl Pts',(3.73952329299994,2.2,1.82935679899999));
#342552=CARTESIAN_POINT('Ctrl Pts',(3.73815594499994,12.2,1.82912295299999));
#342553=CARTESIAN_POINT('Ctrl Pts',(3.73815594499994,5.2,1.82912295299999));
#342554=CARTESIAN_POINT('Ctrl Pts',(3.73815594499994,2.2,1.82912295299999));
#342555=CARTESIAN_POINT('Ctrl Pts',(3.73679368499995,12.2,1.82888831899998));
#342556=CARTESIAN_POINT('Ctrl Pts',(3.73679368499995,5.2,1.82888831899998));
#342557=CARTESIAN_POINT('Ctrl Pts',(3.73679368499995,2.2,1.82888831899998));
#342558=CARTESIAN_POINT('Ctrl Pts',(3.73543651999994,12.2,1.82865290799999));
#342559=CARTESIAN_POINT('Ctrl Pts',(3.73543651999994,5.2,1.82865290799999));
#342560=CARTESIAN_POINT('Ctrl Pts',(3.73543651999994,2.2,1.82865290799999));
#342561=CARTESIAN_POINT('Ctrl Pts',(3.73408445899994,12.2,1.82841673099999));
#342562=CARTESIAN_POINT('Ctrl Pts',(3.73408445899994,5.2,1.82841673099999));
#342563=CARTESIAN_POINT('Ctrl Pts',(3.73408445899994,2.2,1.82841673099999));
#342564=CARTESIAN_POINT('Ctrl Pts',(3.73273750799994,12.2,1.82817980399999));
#342565=CARTESIAN_POINT('Ctrl Pts',(3.73273750799994,5.2,1.82817980399999));
#342566=CARTESIAN_POINT('Ctrl Pts',(3.73273750799994,2.2,1.82817980399999));
#342567=CARTESIAN_POINT('Ctrl Pts',(3.73139567399994,12.2,1.82794213499998));
#342568=CARTESIAN_POINT('Ctrl Pts',(3.73139567399994,5.2,1.82794213499998));
#342569=CARTESIAN_POINT('Ctrl Pts',(3.73139567399994,2.2,1.82794213499998));
#342570=CARTESIAN_POINT('Ctrl Pts',(3.73005896399994,12.2,1.82770373799999));
#342571=CARTESIAN_POINT('Ctrl Pts',(3.73005896399994,5.2,1.82770373799999));
#342572=CARTESIAN_POINT('Ctrl Pts',(3.73005896399994,2.2,1.82770373799999));
#342573=CARTESIAN_POINT('Ctrl Pts',(3.72872738599995,12.2,1.82746462599999));
#342574=CARTESIAN_POINT('Ctrl Pts',(3.72872738599995,5.2,1.82746462599999));
#342575=CARTESIAN_POINT('Ctrl Pts',(3.72872738599995,2.2,1.82746462599999));
#342576=CARTESIAN_POINT('Ctrl Pts',(3.72740094599994,12.2,1.82722480999999));
#342577=CARTESIAN_POINT('Ctrl Pts',(3.72740094599994,5.2,1.82722480999999));
#342578=CARTESIAN_POINT('Ctrl Pts',(3.72740094599994,2.2,1.82722480999999));
#342579=CARTESIAN_POINT('Ctrl Pts',(3.72607965099994,12.2,1.82698430299999));
#342580=CARTESIAN_POINT('Ctrl Pts',(3.72607965099994,5.2,1.82698430299999));
#342581=CARTESIAN_POINT('Ctrl Pts',(3.72607965099994,2.2,1.82698430299999));
#342582=CARTESIAN_POINT('Ctrl Pts',(3.72476350899994,12.2,1.82674311799999));
#342583=CARTESIAN_POINT('Ctrl Pts',(3.72476350899994,5.2,1.82674311799999));
#342584=CARTESIAN_POINT('Ctrl Pts',(3.72476350899994,2.2,1.82674311799999));
#342585=CARTESIAN_POINT('Ctrl Pts',(3.72345252799994,12.2,1.82650126599999));
#342586=CARTESIAN_POINT('Ctrl Pts',(3.72345252799994,5.2,1.82650126599999));
#342587=CARTESIAN_POINT('Ctrl Pts',(3.72345252799994,2.2,1.82650126599999));
#342588=CARTESIAN_POINT('Ctrl Pts',(3.72214671299994,12.2,1.82625875999999));
#342589=CARTESIAN_POINT('Ctrl Pts',(3.72214671299994,5.2,1.82625875999999));
#342590=CARTESIAN_POINT('Ctrl Pts',(3.72214671299994,2.2,1.82625875999999));
#342591=CARTESIAN_POINT('Ctrl Pts',(3.72084607199994,12.2,1.82601561299998));
#342592=CARTESIAN_POINT('Ctrl Pts',(3.72084607199994,5.2,1.82601561299998));
#342593=CARTESIAN_POINT('Ctrl Pts',(3.72084607199994,2.2,1.82601561299998));
#342594=CARTESIAN_POINT('Ctrl Pts',(3.71955061299994,12.2,1.82577183799999));
#342595=CARTESIAN_POINT('Ctrl Pts',(3.71955061299994,5.2,1.82577183799999));
#342596=CARTESIAN_POINT('Ctrl Pts',(3.71955061299994,2.2,1.82577183799999));
#342597=CARTESIAN_POINT('Ctrl Pts',(3.71826034199994,12.2,1.82552744599999));
#342598=CARTESIAN_POINT('Ctrl Pts',(3.71826034199994,5.2,1.82552744599999));
#342599=CARTESIAN_POINT('Ctrl Pts',(3.71826034199994,2.2,1.82552744599999));
#342600=CARTESIAN_POINT('Ctrl Pts',(3.71697526499994,12.2,1.82528245099999));
#342601=CARTESIAN_POINT('Ctrl Pts',(3.71697526499994,5.2,1.82528245099999));
#342602=CARTESIAN_POINT('Ctrl Pts',(3.71697526499994,2.2,1.82528245099999));
#342603=CARTESIAN_POINT('Ctrl Pts',(3.71569539199994,12.2,1.82503686499999));
#342604=CARTESIAN_POINT('Ctrl Pts',(3.71569539199994,5.2,1.82503686499999));
#342605=CARTESIAN_POINT('Ctrl Pts',(3.71569539199994,2.2,1.82503686499999));
#342606=CARTESIAN_POINT('Ctrl Pts',(3.71442072799994,12.2,1.82479070099999));
#342607=CARTESIAN_POINT('Ctrl Pts',(3.71442072799994,5.2,1.82479070099999));
#342608=CARTESIAN_POINT('Ctrl Pts',(3.71442072799994,2.2,1.82479070099999));
#342609=CARTESIAN_POINT('Ctrl Pts',(3.71315128099994,12.2,1.82454397199999));
#342610=CARTESIAN_POINT('Ctrl Pts',(3.71315128099994,5.2,1.82454397199999));
#342611=CARTESIAN_POINT('Ctrl Pts',(3.71315128099994,2.2,1.82454397199999));
#342612=CARTESIAN_POINT('Ctrl Pts',(3.71188705699994,12.2,1.82429668899998));
#342613=CARTESIAN_POINT('Ctrl Pts',(3.71188705699994,5.2,1.82429668899998));
#342614=CARTESIAN_POINT('Ctrl Pts',(3.71188705699994,2.2,1.82429668899998));
#342615=CARTESIAN_POINT('Ctrl Pts',(3.71062806599994,12.2,1.82404886699999));
#342616=CARTESIAN_POINT('Ctrl Pts',(3.71062806599994,5.2,1.82404886699999));
#342617=CARTESIAN_POINT('Ctrl Pts',(3.71062806599994,2.2,1.82404886699999));
#342618=CARTESIAN_POINT('Ctrl Pts',(3.70937431099994,12.2,1.82380051699999));
#342619=CARTESIAN_POINT('Ctrl Pts',(3.70937431099994,5.2,1.82380051699999));
#342620=CARTESIAN_POINT('Ctrl Pts',(3.70937431099994,2.2,1.82380051699999));
#342621=CARTESIAN_POINT('Ctrl Pts',(3.70812580199994,12.2,1.82355165499999));
#342622=CARTESIAN_POINT('Ctrl Pts',(3.70812580199994,5.2,1.82355165499999));
#342623=CARTESIAN_POINT('Ctrl Pts',(3.70812580199994,2.2,1.82355165499999));
#342624=CARTESIAN_POINT('Ctrl Pts',(3.70688254499994,12.2,1.82330228899998));
#342625=CARTESIAN_POINT('Ctrl Pts',(3.70688254499994,5.2,1.82330228899998));
#342626=CARTESIAN_POINT('Ctrl Pts',(3.70688254499994,2.2,1.82330228899998));
#342627=CARTESIAN_POINT('Ctrl Pts',(3.70564454699994,12.2,1.82305243699998));
#342628=CARTESIAN_POINT('Ctrl Pts',(3.70564454699994,5.2,1.82305243699998));
#342629=CARTESIAN_POINT('Ctrl Pts',(3.70564454699994,2.2,1.82305243699998));
#342630=CARTESIAN_POINT('Ctrl Pts',(3.70441181699994,12.2,1.82280210899998));
#342631=CARTESIAN_POINT('Ctrl Pts',(3.70441181699994,5.2,1.82280210899998));
#342632=CARTESIAN_POINT('Ctrl Pts',(3.70441181699994,2.2,1.82280210899998));
#342633=CARTESIAN_POINT('Ctrl Pts',(3.70318435899994,12.2,1.82255131799999));
#342634=CARTESIAN_POINT('Ctrl Pts',(3.70318435899994,5.2,1.82255131799999));
#342635=CARTESIAN_POINT('Ctrl Pts',(3.70318435899994,2.2,1.82255131799999));
#342636=CARTESIAN_POINT('Ctrl Pts',(3.70196218199994,12.2,1.82230007799999));
#342637=CARTESIAN_POINT('Ctrl Pts',(3.70196218199994,5.2,1.82230007799999));
#342638=CARTESIAN_POINT('Ctrl Pts',(3.70196218199994,2.2,1.82230007799999));
#342639=CARTESIAN_POINT('Ctrl Pts',(3.70074529299994,12.2,1.82204840299999));
#342640=CARTESIAN_POINT('Ctrl Pts',(3.70074529299994,5.2,1.82204840299999));
#342641=CARTESIAN_POINT('Ctrl Pts',(3.70074529299994,2.2,1.82204840299999));
#342642=CARTESIAN_POINT('Ctrl Pts',(3.69953369899994,12.2,1.82179630399999));
#342643=CARTESIAN_POINT('Ctrl Pts',(3.69953369899994,5.2,1.82179630399999));
#342644=CARTESIAN_POINT('Ctrl Pts',(3.69953369899994,2.2,1.82179630399999));
#342645=CARTESIAN_POINT('Ctrl Pts',(3.69832740599994,12.2,1.82154379499998));
#342646=CARTESIAN_POINT('Ctrl Pts',(3.69832740599994,5.2,1.82154379499998));
#342647=CARTESIAN_POINT('Ctrl Pts',(3.69832740599994,2.2,1.82154379499998));
#342648=CARTESIAN_POINT('Ctrl Pts',(3.69712642399994,12.2,1.82129088999998));
#342649=CARTESIAN_POINT('Ctrl Pts',(3.69712642399994,5.2,1.82129088999998));
#342650=CARTESIAN_POINT('Ctrl Pts',(3.69712642399994,2.2,1.82129088999998));
#342651=CARTESIAN_POINT('Ctrl Pts',(3.69593075599994,12.2,1.82103760199999));
#342652=CARTESIAN_POINT('Ctrl Pts',(3.69593075599994,5.2,1.82103760199999));
#342653=CARTESIAN_POINT('Ctrl Pts',(3.69593075599994,2.2,1.82103760199999));
#342654=CARTESIAN_POINT('Ctrl Pts',(3.69474041299994,12.2,1.82078394399999));
#342655=CARTESIAN_POINT('Ctrl Pts',(3.69474041299994,5.2,1.82078394399999));
#342656=CARTESIAN_POINT('Ctrl Pts',(3.69474041299994,2.2,1.82078394399999));
#342657=CARTESIAN_POINT('Ctrl Pts',(3.69355539899995,12.2,1.82052992899999));
#342658=CARTESIAN_POINT('Ctrl Pts',(3.69355539899995,5.2,1.82052992899999));
#342659=CARTESIAN_POINT('Ctrl Pts',(3.69355539899995,2.2,1.82052992899999));
#342660=CARTESIAN_POINT('Ctrl Pts',(3.69237572299994,12.2,1.82027557199998));
#342661=CARTESIAN_POINT('Ctrl Pts',(3.69237572299994,5.2,1.82027557199998));
#342662=CARTESIAN_POINT('Ctrl Pts',(3.69237572299994,2.2,1.82027557199998));
#342663=CARTESIAN_POINT('Ctrl Pts',(3.69120139099994,12.2,1.82002088299999));
#342664=CARTESIAN_POINT('Ctrl Pts',(3.69120139099994,5.2,1.82002088299999));
#342665=CARTESIAN_POINT('Ctrl Pts',(3.69120139099994,2.2,1.82002088299999));
#342666=CARTESIAN_POINT('Ctrl Pts',(3.69003241099994,12.2,1.81976587899999));
#342667=CARTESIAN_POINT('Ctrl Pts',(3.69003241099994,5.2,1.81976587899999));
#342668=CARTESIAN_POINT('Ctrl Pts',(3.69003241099994,2.2,1.81976587899999));
#342669=CARTESIAN_POINT('Ctrl Pts',(3.68886878899994,12.2,1.81951057199999));
#342670=CARTESIAN_POINT('Ctrl Pts',(3.68886878899994,5.2,1.81951057199999));
#342671=CARTESIAN_POINT('Ctrl Pts',(3.68886878899994,2.2,1.81951057199999));
#342672=CARTESIAN_POINT('Ctrl Pts',(3.68771053399994,12.2,1.81925497599998));
#342673=CARTESIAN_POINT('Ctrl Pts',(3.68771053399994,5.2,1.81925497599998));
#342674=CARTESIAN_POINT('Ctrl Pts',(3.68771053399994,2.2,1.81925497599998));
#342675=CARTESIAN_POINT('Ctrl Pts',(3.68655765099994,12.2,1.81899910299999));
#342676=CARTESIAN_POINT('Ctrl Pts',(3.68655765099994,5.2,1.81899910299999));
#342677=CARTESIAN_POINT('Ctrl Pts',(3.68655765099994,2.2,1.81899910299999));
#342678=CARTESIAN_POINT('Ctrl Pts',(3.68541014799994,12.2,1.81874296999998));
#342679=CARTESIAN_POINT('Ctrl Pts',(3.68541014799994,5.2,1.81874296999998));
#342680=CARTESIAN_POINT('Ctrl Pts',(3.68541014799994,2.2,1.81874296999998));
#342681=CARTESIAN_POINT('Ctrl Pts',(3.68426803199994,12.2,1.81848658699999));
#342682=CARTESIAN_POINT('Ctrl Pts',(3.68426803199994,5.2,1.81848658699999));
#342683=CARTESIAN_POINT('Ctrl Pts',(3.68426803199994,2.2,1.81848658699999));
#342684=CARTESIAN_POINT('Ctrl Pts',(3.68313131099994,12.2,1.81822996999998));
#342685=CARTESIAN_POINT('Ctrl Pts',(3.68313131099994,5.2,1.81822996999998));
#342686=CARTESIAN_POINT('Ctrl Pts',(3.68313131099994,2.2,1.81822996999998));
#342687=CARTESIAN_POINT('Ctrl Pts',(3.68199998999994,12.2,1.81797313199999));
#342688=CARTESIAN_POINT('Ctrl Pts',(3.68199998999994,5.2,1.81797313199999));
#342689=CARTESIAN_POINT('Ctrl Pts',(3.68199998999994,2.2,1.81797313199999));
#342690=CARTESIAN_POINT('Ctrl Pts',(3.68087407699994,12.2,1.81771608599998));
#342691=CARTESIAN_POINT('Ctrl Pts',(3.68087407699994,5.2,1.81771608599998));
#342692=CARTESIAN_POINT('Ctrl Pts',(3.68087407699994,2.2,1.81771608599998));
#342693=CARTESIAN_POINT('Ctrl Pts',(3.67975357999994,12.2,1.81745884699998));
#342694=CARTESIAN_POINT('Ctrl Pts',(3.67975357999994,5.2,1.81745884699998));
#342695=CARTESIAN_POINT('Ctrl Pts',(3.67975357999994,2.2,1.81745884699998));
#342696=CARTESIAN_POINT('Ctrl Pts',(3.67863850499994,12.2,1.81720142899998));
#342697=CARTESIAN_POINT('Ctrl Pts',(3.67863850499994,5.2,1.81720142899998));
#342698=CARTESIAN_POINT('Ctrl Pts',(3.67863850499994,2.2,1.81720142899998));
#342699=CARTESIAN_POINT('Ctrl Pts',(3.67752885999994,12.2,1.81694384599998));
#342700=CARTESIAN_POINT('Ctrl Pts',(3.67752885999994,5.2,1.81694384599998));
#342701=CARTESIAN_POINT('Ctrl Pts',(3.67752885999994,2.2,1.81694384599998));
#342702=CARTESIAN_POINT('Ctrl Pts',(3.67642465199994,12.2,1.81668610999999));
#342703=CARTESIAN_POINT('Ctrl Pts',(3.67642465199994,5.2,1.81668610999999));
#342704=CARTESIAN_POINT('Ctrl Pts',(3.67642465199994,2.2,1.81668610999999));
#342705=CARTESIAN_POINT('Ctrl Pts',(3.67532588699994,12.2,1.81642823799999));
#342706=CARTESIAN_POINT('Ctrl Pts',(3.67532588699994,5.2,1.81642823799999));
#342707=CARTESIAN_POINT('Ctrl Pts',(3.67532588699994,2.2,1.81642823799999));
#342708=CARTESIAN_POINT('Ctrl Pts',(3.67423257199994,12.2,1.81617024099999));
#342709=CARTESIAN_POINT('Ctrl Pts',(3.67423257199994,5.2,1.81617024099999));
#342710=CARTESIAN_POINT('Ctrl Pts',(3.67423257199994,2.2,1.81617024099999));
#342711=CARTESIAN_POINT('Ctrl Pts',(3.67314471499994,12.2,1.81591213499999));
#342712=CARTESIAN_POINT('Ctrl Pts',(3.67314471499994,5.2,1.81591213499999));
#342713=CARTESIAN_POINT('Ctrl Pts',(3.67314471499994,2.2,1.81591213499999));
#342714=CARTESIAN_POINT('Ctrl Pts',(3.67206232299994,12.2,1.81565393399998));
#342715=CARTESIAN_POINT('Ctrl Pts',(3.67206232299994,5.2,1.81565393399998));
#342716=CARTESIAN_POINT('Ctrl Pts',(3.67206232299994,2.2,1.81565393399998));
#342717=CARTESIAN_POINT('Ctrl Pts',(3.67098540399994,12.2,1.81539565199999));
#342718=CARTESIAN_POINT('Ctrl Pts',(3.67098540399994,5.2,1.81539565199999));
#342719=CARTESIAN_POINT('Ctrl Pts',(3.67098540399994,2.2,1.81539565199999));
#342720=CARTESIAN_POINT('Ctrl Pts',(3.66991396299994,12.2,1.81513730299999));
#342721=CARTESIAN_POINT('Ctrl Pts',(3.66991396299994,5.2,1.81513730299999));
#342722=CARTESIAN_POINT('Ctrl Pts',(3.66991396299994,2.2,1.81513730299999));
#342723=CARTESIAN_POINT('Ctrl Pts',(3.66884800699994,12.2,1.81487890099998));
#342724=CARTESIAN_POINT('Ctrl Pts',(3.66884800699994,5.2,1.81487890099998));
#342725=CARTESIAN_POINT('Ctrl Pts',(3.66884800699994,2.2,1.81487890099998));
#342726=CARTESIAN_POINT('Ctrl Pts',(3.66778754499994,12.2,1.81462046099998));
#342727=CARTESIAN_POINT('Ctrl Pts',(3.66778754499994,5.2,1.81462046099998));
#342728=CARTESIAN_POINT('Ctrl Pts',(3.66778754499994,2.2,1.81462046099998));
#342729=CARTESIAN_POINT('Ctrl Pts',(3.66673258299994,12.2,1.81436199699998));
#342730=CARTESIAN_POINT('Ctrl Pts',(3.66673258299994,5.2,1.81436199699998));
#342731=CARTESIAN_POINT('Ctrl Pts',(3.66673258299994,2.2,1.81436199699998));
#342732=CARTESIAN_POINT('Ctrl Pts',(3.66568312899994,12.2,1.81410352299999));
#342733=CARTESIAN_POINT('Ctrl Pts',(3.66568312899994,5.2,1.81410352299999));
#342734=CARTESIAN_POINT('Ctrl Pts',(3.66568312899994,2.2,1.81410352299999));
#342735=CARTESIAN_POINT('Ctrl Pts',(3.66463918899994,12.2,1.81384505499999));
#342736=CARTESIAN_POINT('Ctrl Pts',(3.66463918899994,5.2,1.81384505499999));
#342737=CARTESIAN_POINT('Ctrl Pts',(3.66463918899994,2.2,1.81384505499999));
#342738=CARTESIAN_POINT('Ctrl Pts',(3.66360076999994,12.2,1.81358660399999));
#342739=CARTESIAN_POINT('Ctrl Pts',(3.66360076999994,5.2,1.81358660399999));
#342740=CARTESIAN_POINT('Ctrl Pts',(3.66360076999994,2.2,1.81358660399999));
#342741=CARTESIAN_POINT('Ctrl Pts',(3.66256787899994,12.2,1.81332818799998));
#342742=CARTESIAN_POINT('Ctrl Pts',(3.66256787899994,5.2,1.81332818799998));
#342743=CARTESIAN_POINT('Ctrl Pts',(3.66256787899994,2.2,1.81332818799998));
#342744=CARTESIAN_POINT('Ctrl Pts',(3.66154052399994,12.2,1.81306981999999));
#342745=CARTESIAN_POINT('Ctrl Pts',(3.66154052399994,5.2,1.81306981999999));
#342746=CARTESIAN_POINT('Ctrl Pts',(3.66154052399994,2.2,1.81306981999999));
#342747=CARTESIAN_POINT('Ctrl Pts',(3.66051871099994,12.2,1.81281151599999));
#342748=CARTESIAN_POINT('Ctrl Pts',(3.66051871099994,5.2,1.81281151599999));
#342749=CARTESIAN_POINT('Ctrl Pts',(3.66051871099994,2.2,1.81281151599999));
#342750=CARTESIAN_POINT('Ctrl Pts',(3.65950244799994,12.2,1.81255328999999));
#342751=CARTESIAN_POINT('Ctrl Pts',(3.65950244799994,5.2,1.81255328999999));
#342752=CARTESIAN_POINT('Ctrl Pts',(3.65950244799994,2.2,1.81255328999999));
#342753=CARTESIAN_POINT('Ctrl Pts',(3.65849174099994,12.2,1.81229515499998));
#342754=CARTESIAN_POINT('Ctrl Pts',(3.65849174099994,5.2,1.81229515499998));
#342755=CARTESIAN_POINT('Ctrl Pts',(3.65849174099994,2.2,1.81229515499998));
#342756=CARTESIAN_POINT('Ctrl Pts',(3.65748659799995,12.2,1.81203712699999));
#342757=CARTESIAN_POINT('Ctrl Pts',(3.65748659799995,5.2,1.81203712699999));
#342758=CARTESIAN_POINT('Ctrl Pts',(3.65748659799995,2.2,1.81203712699999));
#342759=CARTESIAN_POINT('Ctrl Pts',(3.65648702599994,12.2,1.81177922199999));
#342760=CARTESIAN_POINT('Ctrl Pts',(3.65648702599994,5.2,1.81177922199999));
#342761=CARTESIAN_POINT('Ctrl Pts',(3.65648702599994,2.2,1.81177922199999));
#342762=CARTESIAN_POINT('Ctrl Pts',(3.65549302999994,12.2,1.81152145299999));
#342763=CARTESIAN_POINT('Ctrl Pts',(3.65549302999994,5.2,1.81152145299999));
#342764=CARTESIAN_POINT('Ctrl Pts',(3.65549302999994,2.2,1.81152145299999));
#342765=CARTESIAN_POINT('Ctrl Pts',(3.65450462099994,12.2,1.81126383599999));
#342766=CARTESIAN_POINT('Ctrl Pts',(3.65450462099994,5.2,1.81126383599999));
#342767=CARTESIAN_POINT('Ctrl Pts',(3.65450462099994,2.2,1.81126383599999));
#342768=CARTESIAN_POINT('Ctrl Pts',(3.65352180299995,12.2,1.81100638499998));
#342769=CARTESIAN_POINT('Ctrl Pts',(3.65352180299995,5.2,1.81100638499998));
#342770=CARTESIAN_POINT('Ctrl Pts',(3.65352180299995,2.2,1.81100638499998));
#342771=CARTESIAN_POINT('Ctrl Pts',(3.65254458399995,12.2,1.81074911599998));
#342772=CARTESIAN_POINT('Ctrl Pts',(3.65254458399995,5.2,1.81074911599998));
#342773=CARTESIAN_POINT('Ctrl Pts',(3.65254458399995,2.2,1.81074911599998));
#342774=CARTESIAN_POINT('Ctrl Pts',(3.65157297099994,12.2,1.81049204299998));
#342775=CARTESIAN_POINT('Ctrl Pts',(3.65157297099994,5.2,1.81049204299998));
#342776=CARTESIAN_POINT('Ctrl Pts',(3.65157297099994,2.2,1.81049204299998));
#342777=CARTESIAN_POINT('Ctrl Pts',(3.65060696999994,12.2,1.81023518199999));
#342778=CARTESIAN_POINT('Ctrl Pts',(3.65060696999994,5.2,1.81023518199999));
#342779=CARTESIAN_POINT('Ctrl Pts',(3.65060696999994,2.2,1.81023518199999));
#342780=CARTESIAN_POINT('Ctrl Pts',(3.64964658899994,12.2,1.80997854799998));
#342781=CARTESIAN_POINT('Ctrl Pts',(3.64964658899994,5.2,1.80997854799998));
#342782=CARTESIAN_POINT('Ctrl Pts',(3.64964658899994,2.2,1.80997854799998));
#342783=CARTESIAN_POINT('Ctrl Pts',(3.64869183599994,12.2,1.80972215599999));
#342784=CARTESIAN_POINT('Ctrl Pts',(3.64869183599994,5.2,1.80972215599999));
#342785=CARTESIAN_POINT('Ctrl Pts',(3.64869183599994,2.2,1.80972215599999));
#342786=CARTESIAN_POINT('Ctrl Pts',(3.64774271599994,12.2,1.80946602099999));
#342787=CARTESIAN_POINT('Ctrl Pts',(3.64774271599994,5.2,1.80946602099999));
#342788=CARTESIAN_POINT('Ctrl Pts',(3.64774271599994,2.2,1.80946602099999));
#342789=CARTESIAN_POINT('Ctrl Pts',(3.64679923799994,12.2,1.80921015799999));
#342790=CARTESIAN_POINT('Ctrl Pts',(3.64679923799994,5.2,1.80921015799999));
#342791=CARTESIAN_POINT('Ctrl Pts',(3.64679923799994,2.2,1.80921015799999));
#342792=CARTESIAN_POINT('Ctrl Pts',(3.64586140799994,12.2,1.80895458299998));
#342793=CARTESIAN_POINT('Ctrl Pts',(3.64586140799994,5.2,1.80895458299998));
#342794=CARTESIAN_POINT('Ctrl Pts',(3.64586140799994,2.2,1.80895458299998));
#342795=CARTESIAN_POINT('Ctrl Pts',(3.64492923299994,12.2,1.80869930999998));
#342796=CARTESIAN_POINT('Ctrl Pts',(3.64492923299994,5.2,1.80869930999998));
#342797=CARTESIAN_POINT('Ctrl Pts',(3.64492923299994,2.2,1.80869930999998));
#342798=CARTESIAN_POINT('Ctrl Pts',(3.64400271999994,12.2,1.80844435699999));
#342799=CARTESIAN_POINT('Ctrl Pts',(3.64400271999994,5.2,1.80844435699999));
#342800=CARTESIAN_POINT('Ctrl Pts',(3.64400271999994,2.2,1.80844435699999));
#342801=CARTESIAN_POINT('Ctrl Pts',(3.64308187599994,12.2,1.80818973699999));
#342802=CARTESIAN_POINT('Ctrl Pts',(3.64308187599994,5.2,1.80818973699999));
#342803=CARTESIAN_POINT('Ctrl Pts',(3.64308187599994,2.2,1.80818973699999));
#342804=CARTESIAN_POINT('Ctrl Pts',(3.64216670899994,12.2,1.80793546599999));
#342805=CARTESIAN_POINT('Ctrl Pts',(3.64216670899994,5.2,1.80793546599999));
#342806=CARTESIAN_POINT('Ctrl Pts',(3.64216670899994,2.2,1.80793546599999));
#342807=CARTESIAN_POINT('Ctrl Pts',(3.64125722499994,12.2,1.80768156099999));
#342808=CARTESIAN_POINT('Ctrl Pts',(3.64125722499994,5.2,1.80768156099999));
#342809=CARTESIAN_POINT('Ctrl Pts',(3.64125722499994,2.2,1.80768156099999));
#342810=CARTESIAN_POINT('Ctrl Pts',(3.64035343099994,12.2,1.80742803599999));
#342811=CARTESIAN_POINT('Ctrl Pts',(3.64035343099994,5.2,1.80742803599999));
#342812=CARTESIAN_POINT('Ctrl Pts',(3.64035343099994,2.2,1.80742803599999));
#342813=CARTESIAN_POINT('Ctrl Pts',(3.63945533399994,12.2,1.80717490699998));
#342814=CARTESIAN_POINT('Ctrl Pts',(3.63945533399994,5.2,1.80717490699998));
#342815=CARTESIAN_POINT('Ctrl Pts',(3.63945533399994,2.2,1.80717490699998));
#342816=CARTESIAN_POINT('Ctrl Pts',(3.63856294199994,12.2,1.80692218999999));
#342817=CARTESIAN_POINT('Ctrl Pts',(3.63856294199994,5.2,1.80692218999999));
#342818=CARTESIAN_POINT('Ctrl Pts',(3.63856294199994,2.2,1.80692218999999));
#342819=CARTESIAN_POINT('Ctrl Pts',(3.63767625999994,12.2,1.80666990099999));
#342820=CARTESIAN_POINT('Ctrl Pts',(3.63767625999994,5.2,1.80666990099999));
#342821=CARTESIAN_POINT('Ctrl Pts',(3.63767625999994,2.2,1.80666990099999));
#342822=CARTESIAN_POINT('Ctrl Pts',(3.63679529799994,12.2,1.80641805499999));
#342823=CARTESIAN_POINT('Ctrl Pts',(3.63679529799994,5.2,1.80641805499999));
#342824=CARTESIAN_POINT('Ctrl Pts',(3.63679529799994,2.2,1.80641805499999));
#342825=CARTESIAN_POINT('Ctrl Pts',(3.63592005999994,12.2,1.80616666899999));
#342826=CARTESIAN_POINT('Ctrl Pts',(3.63592005999994,5.2,1.80616666899999));
#342827=CARTESIAN_POINT('Ctrl Pts',(3.63592005999994,2.2,1.80616666899999));
#342828=CARTESIAN_POINT('Ctrl Pts',(3.63505055499994,12.2,1.80591575699999));
#342829=CARTESIAN_POINT('Ctrl Pts',(3.63505055499994,5.2,1.80591575699999));
#342830=CARTESIAN_POINT('Ctrl Pts',(3.63505055499994,2.2,1.80591575699999));
#342831=CARTESIAN_POINT('Ctrl Pts',(3.63418678899994,12.2,1.80566533699999));
#342832=CARTESIAN_POINT('Ctrl Pts',(3.63418678899994,5.2,1.80566533699999));
#342833=CARTESIAN_POINT('Ctrl Pts',(3.63418678899994,2.2,1.80566533699999));
#342834=CARTESIAN_POINT('Ctrl Pts',(3.63332876999995,12.2,1.80541542399999));
#342835=CARTESIAN_POINT('Ctrl Pts',(3.63332876999995,5.2,1.80541542399999));
#342836=CARTESIAN_POINT('Ctrl Pts',(3.63332876999995,2.2,1.80541542399999));
#342837=CARTESIAN_POINT('Ctrl Pts',(3.63247650399994,12.2,1.80516603399999));
#342838=CARTESIAN_POINT('Ctrl Pts',(3.63247650399994,5.2,1.80516603399999));
#342839=CARTESIAN_POINT('Ctrl Pts',(3.63247650399994,2.2,1.80516603399999));
#342840=CARTESIAN_POINT('Ctrl Pts',(3.63162999899994,12.2,1.80491718299999));
#342841=CARTESIAN_POINT('Ctrl Pts',(3.63162999899994,5.2,1.80491718299999));
#342842=CARTESIAN_POINT('Ctrl Pts',(3.63162999899994,2.2,1.80491718299999));
#342843=CARTESIAN_POINT('Ctrl Pts',(3.63078926099994,12.2,1.80466888799999));
#342844=CARTESIAN_POINT('Ctrl Pts',(3.63078926099994,5.2,1.80466888799999));
#342845=CARTESIAN_POINT('Ctrl Pts',(3.63078926099994,2.2,1.80466888799999));
#342846=CARTESIAN_POINT('Ctrl Pts',(3.62995429699994,12.2,1.80442116399998));
#342847=CARTESIAN_POINT('Ctrl Pts',(3.62995429699994,5.2,1.80442116399998));
#342848=CARTESIAN_POINT('Ctrl Pts',(3.62995429699994,2.2,1.80442116399998));
#342849=CARTESIAN_POINT('Ctrl Pts',(3.62912511499994,12.2,1.80417402799999));
#342850=CARTESIAN_POINT('Ctrl Pts',(3.62912511499994,5.2,1.80417402799999));
#342851=CARTESIAN_POINT('Ctrl Pts',(3.62912511499994,2.2,1.80417402799999));
#342852=CARTESIAN_POINT('Ctrl Pts',(3.62830172199994,12.2,1.80392749599998));
#342853=CARTESIAN_POINT('Ctrl Pts',(3.62830172199994,5.2,1.80392749599998));
#342854=CARTESIAN_POINT('Ctrl Pts',(3.62830172199994,2.2,1.80392749599998));
#342855=CARTESIAN_POINT('Ctrl Pts',(3.62748412299994,12.2,1.80368158599999));
#342856=CARTESIAN_POINT('Ctrl Pts',(3.62748412299994,5.2,1.80368158599999));
#342857=CARTESIAN_POINT('Ctrl Pts',(3.62748412299994,2.2,1.80368158599999));
#342858=CARTESIAN_POINT('Ctrl Pts',(3.62667232799994,12.2,1.80343631099999));
#342859=CARTESIAN_POINT('Ctrl Pts',(3.62667232799994,5.2,1.80343631099999));
#342860=CARTESIAN_POINT('Ctrl Pts',(3.62667232799994,2.2,1.80343631099999));
#342861=CARTESIAN_POINT('Ctrl Pts',(3.62586634099994,12.2,1.80319168999999));
#342862=CARTESIAN_POINT('Ctrl Pts',(3.62586634099994,5.2,1.80319168999999));
#342863=CARTESIAN_POINT('Ctrl Pts',(3.62586634099994,2.2,1.80319168999999));
#342864=CARTESIAN_POINT('Ctrl Pts',(3.62506617099994,12.2,1.80294773999998));
#342865=CARTESIAN_POINT('Ctrl Pts',(3.62506617099994,5.2,1.80294773999998));
#342866=CARTESIAN_POINT('Ctrl Pts',(3.62506617099994,2.2,1.80294773999998));
#342867=CARTESIAN_POINT('Ctrl Pts',(3.62427182399994,12.2,1.80270447599999));
#342868=CARTESIAN_POINT('Ctrl Pts',(3.62427182399994,5.2,1.80270447599999));
#342869=CARTESIAN_POINT('Ctrl Pts',(3.62427182399994,2.2,1.80270447599999));
#342870=CARTESIAN_POINT('Ctrl Pts',(3.62348330799994,12.2,1.80246191399998));
#342871=CARTESIAN_POINT('Ctrl Pts',(3.62348330799994,5.2,1.80246191399998));
#342872=CARTESIAN_POINT('Ctrl Pts',(3.62348330799994,2.2,1.80246191399998));
#342873=CARTESIAN_POINT('Ctrl Pts',(3.62270062899994,12.2,1.80222007199998));
#342874=CARTESIAN_POINT('Ctrl Pts',(3.62270062899994,5.2,1.80222007199998));
#342875=CARTESIAN_POINT('Ctrl Pts',(3.62270062899994,2.2,1.80222007199998));
#342876=CARTESIAN_POINT('Ctrl Pts',(3.62192379399994,12.2,1.80197896699998));
#342877=CARTESIAN_POINT('Ctrl Pts',(3.62192379399994,5.2,1.80197896699998));
#342878=CARTESIAN_POINT('Ctrl Pts',(3.62192379399994,2.2,1.80197896699998));
#342879=CARTESIAN_POINT('Ctrl Pts',(3.62115281099994,12.2,1.80173861599998));
#342880=CARTESIAN_POINT('Ctrl Pts',(3.62115281099994,5.2,1.80173861599998));
#342881=CARTESIAN_POINT('Ctrl Pts',(3.62115281099994,2.2,1.80173861599998));
#342882=CARTESIAN_POINT('Ctrl Pts',(3.62038768599994,12.2,1.80149903499998));
#342883=CARTESIAN_POINT('Ctrl Pts',(3.62038768599994,5.2,1.80149903499998));
#342884=CARTESIAN_POINT('Ctrl Pts',(3.62038768599994,2.2,1.80149903499998));
#342885=CARTESIAN_POINT('Ctrl Pts',(3.61962842599994,12.2,1.80126024099998));
#342886=CARTESIAN_POINT('Ctrl Pts',(3.61962842599994,5.2,1.80126024099998));
#342887=CARTESIAN_POINT('Ctrl Pts',(3.61962842599994,2.2,1.80126024099998));
#342888=CARTESIAN_POINT('Ctrl Pts',(3.61887503899994,12.2,1.80102225099999));
#342889=CARTESIAN_POINT('Ctrl Pts',(3.61887503899994,5.2,1.80102225099999));
#342890=CARTESIAN_POINT('Ctrl Pts',(3.61887503899994,2.2,1.80102225099999));
#342891=CARTESIAN_POINT('Ctrl Pts',(3.61812753099994,12.2,1.80078508099998));
#342892=CARTESIAN_POINT('Ctrl Pts',(3.61812753099994,5.2,1.80078508099998));
#342893=CARTESIAN_POINT('Ctrl Pts',(3.61812753099994,2.2,1.80078508099998));
#342894=CARTESIAN_POINT('Ctrl Pts',(3.61738590899995,12.2,1.80054874999998));
#342895=CARTESIAN_POINT('Ctrl Pts',(3.61738590899995,5.2,1.80054874999998));
#342896=CARTESIAN_POINT('Ctrl Pts',(3.61738590899995,2.2,1.80054874999998));
#342897=CARTESIAN_POINT('Ctrl Pts',(3.61665018099994,12.2,1.80031327399998));
#342898=CARTESIAN_POINT('Ctrl Pts',(3.61665018099994,5.2,1.80031327399998));
#342899=CARTESIAN_POINT('Ctrl Pts',(3.61665018099994,2.2,1.80031327399998));
#342900=CARTESIAN_POINT('Ctrl Pts',(3.61592035299994,12.2,1.80007867099999));
#342901=CARTESIAN_POINT('Ctrl Pts',(3.61592035299994,5.2,1.80007867099999));
#342902=CARTESIAN_POINT('Ctrl Pts',(3.61592035299994,2.2,1.80007867099999));
#342903=CARTESIAN_POINT('Ctrl Pts',(3.61519643199994,12.2,1.79984495799999));
#342904=CARTESIAN_POINT('Ctrl Pts',(3.61519643199994,5.2,1.79984495799999));
#342905=CARTESIAN_POINT('Ctrl Pts',(3.61519643199994,2.2,1.79984495799999));
#342906=CARTESIAN_POINT('Ctrl Pts',(3.61447842499994,12.2,1.79961215099999));
#342907=CARTESIAN_POINT('Ctrl Pts',(3.61447842499994,5.2,1.79961215099999));
#342908=CARTESIAN_POINT('Ctrl Pts',(3.61447842499994,2.2,1.79961215099999));
#342909=CARTESIAN_POINT('Ctrl Pts',(3.61376633899994,12.2,1.79938026799999));
#342910=CARTESIAN_POINT('Ctrl Pts',(3.61376633899994,5.2,1.79938026799999));
#342911=CARTESIAN_POINT('Ctrl Pts',(3.61376633899994,2.2,1.79938026799999));
#342912=CARTESIAN_POINT('Ctrl Pts',(3.61306018199994,12.2,1.79914932599999));
#342913=CARTESIAN_POINT('Ctrl Pts',(3.61306018199994,5.2,1.79914932599999));
#342914=CARTESIAN_POINT('Ctrl Pts',(3.61306018199994,2.2,1.79914932599999));
#342915=CARTESIAN_POINT('Ctrl Pts',(3.61235995899994,12.2,1.79891934399999));
#342916=CARTESIAN_POINT('Ctrl Pts',(3.61235995899994,5.2,1.79891934399999));
#342917=CARTESIAN_POINT('Ctrl Pts',(3.61235995899994,2.2,1.79891934399999));
#342918=CARTESIAN_POINT('Ctrl Pts',(3.61166567899994,12.2,1.79869033999998));
#342919=CARTESIAN_POINT('Ctrl Pts',(3.61166567899994,5.2,1.79869033999998));
#342920=CARTESIAN_POINT('Ctrl Pts',(3.61166567899994,2.2,1.79869033999998));
#342921=CARTESIAN_POINT('Ctrl Pts',(3.61097734699994,12.2,1.79846232899999));
#342922=CARTESIAN_POINT('Ctrl Pts',(3.61097734699994,5.2,1.79846232899999));
#342923=CARTESIAN_POINT('Ctrl Pts',(3.61097734699994,2.2,1.79846232899999));
#342924=CARTESIAN_POINT('Ctrl Pts',(3.61029497199994,12.2,1.79823532999999));
#342925=CARTESIAN_POINT('Ctrl Pts',(3.61029497199994,5.2,1.79823532999999));
#342926=CARTESIAN_POINT('Ctrl Pts',(3.61029497199994,2.2,1.79823532999999));
#342927=CARTESIAN_POINT('Ctrl Pts',(3.60961855799994,12.2,1.79800935999999));
#342928=CARTESIAN_POINT('Ctrl Pts',(3.60961855799994,5.2,1.79800935999999));
#342929=CARTESIAN_POINT('Ctrl Pts',(3.60961855799994,2.2,1.79800935999999));
#342930=CARTESIAN_POINT('Ctrl Pts',(3.60894811499994,12.2,1.79778443799998));
#342931=CARTESIAN_POINT('Ctrl Pts',(3.60894811499994,5.2,1.79778443799998));
#342932=CARTESIAN_POINT('Ctrl Pts',(3.60894811499994,2.2,1.79778443799998));
#342933=CARTESIAN_POINT('Ctrl Pts',(3.60828364999994,12.2,1.79756058099999));
#342934=CARTESIAN_POINT('Ctrl Pts',(3.60828364999994,5.2,1.79756058099999));
#342935=CARTESIAN_POINT('Ctrl Pts',(3.60828364999994,2.2,1.79756058099999));
#342936=CARTESIAN_POINT('Ctrl Pts',(3.60762516799995,12.2,1.79733780699999));
#342937=CARTESIAN_POINT('Ctrl Pts',(3.60762516799995,5.2,1.79733780699999));
#342938=CARTESIAN_POINT('Ctrl Pts',(3.60762516799995,2.2,1.79733780699999));
#342939=CARTESIAN_POINT('Ctrl Pts',(3.60697267599994,12.2,1.79711613399999));
#342940=CARTESIAN_POINT('Ctrl Pts',(3.60697267599994,5.2,1.79711613399999));
#342941=CARTESIAN_POINT('Ctrl Pts',(3.60697267599994,2.2,1.79711613399999));
#342942=CARTESIAN_POINT('Ctrl Pts',(3.60632618199995,12.2,1.79689557899998));
#342943=CARTESIAN_POINT('Ctrl Pts',(3.60632618199995,5.2,1.79689557899998));
#342944=CARTESIAN_POINT('Ctrl Pts',(3.60632618199995,2.2,1.79689557899998));
#342945=CARTESIAN_POINT('Ctrl Pts',(3.60568569299994,12.2,1.79667616299998));
#342946=CARTESIAN_POINT('Ctrl Pts',(3.60568569299994,5.2,1.79667616299998));
#342947=CARTESIAN_POINT('Ctrl Pts',(3.60568569299994,2.2,1.79667616299998));
#342948=CARTESIAN_POINT('Ctrl Pts',(3.60505121499994,12.2,1.79645790099999));
#342949=CARTESIAN_POINT('Ctrl Pts',(3.60505121499994,5.2,1.79645790099999));
#342950=CARTESIAN_POINT('Ctrl Pts',(3.60505121499994,2.2,1.79645790099999));
#342951=CARTESIAN_POINT('Ctrl Pts',(3.60442275599994,12.2,1.79624081099998));
#342952=CARTESIAN_POINT('Ctrl Pts',(3.60442275599994,5.2,1.79624081099998));
#342953=CARTESIAN_POINT('Ctrl Pts',(3.60442275599994,2.2,1.79624081099998));
#342954=CARTESIAN_POINT('Ctrl Pts',(3.60380032199994,12.2,1.79602491399999));
#342955=CARTESIAN_POINT('Ctrl Pts',(3.60380032199994,5.2,1.79602491399999));
#342956=CARTESIAN_POINT('Ctrl Pts',(3.60380032199994,2.2,1.79602491399999));
#342957=CARTESIAN_POINT('Ctrl Pts',(3.60318392099995,12.2,1.79581022599999));
#342958=CARTESIAN_POINT('Ctrl Pts',(3.60318392099995,5.2,1.79581022599999));
#342959=CARTESIAN_POINT('Ctrl Pts',(3.60318392099995,2.2,1.79581022599999));
#342960=CARTESIAN_POINT('Ctrl Pts',(3.60257355899994,12.2,1.79559676699999));
#342961=CARTESIAN_POINT('Ctrl Pts',(3.60257355899994,5.2,1.79559676699999));
#342962=CARTESIAN_POINT('Ctrl Pts',(3.60257355899994,2.2,1.79559676699999));
#342963=CARTESIAN_POINT('Ctrl Pts',(3.60196924399994,12.2,1.79538455399999));
#342964=CARTESIAN_POINT('Ctrl Pts',(3.60196924399994,5.2,1.79538455399999));
#342965=CARTESIAN_POINT('Ctrl Pts',(3.60196924399994,2.2,1.79538455399999));
#342966=CARTESIAN_POINT('Ctrl Pts',(3.60137098099994,12.2,1.79517360599998));
#342967=CARTESIAN_POINT('Ctrl Pts',(3.60137098099994,5.2,1.79517360599998));
#342968=CARTESIAN_POINT('Ctrl Pts',(3.60137098099994,2.2,1.79517360599998));
#342969=CARTESIAN_POINT('Ctrl Pts',(3.60077877899994,12.2,1.79496394199999));
#342970=CARTESIAN_POINT('Ctrl Pts',(3.60077877899994,5.2,1.79496394199999));
#342971=CARTESIAN_POINT('Ctrl Pts',(3.60077877899994,2.2,1.79496394199999));
#342972=CARTESIAN_POINT('Ctrl Pts',(3.60019264299994,12.2,1.79475557999998));
#342973=CARTESIAN_POINT('Ctrl Pts',(3.60019264299994,5.2,1.79475557999998));
#342974=CARTESIAN_POINT('Ctrl Pts',(3.60019264299994,2.2,1.79475557999998));
#342975=CARTESIAN_POINT('Ctrl Pts',(3.59961258299994,12.2,1.79454853799998));
#342976=CARTESIAN_POINT('Ctrl Pts',(3.59961258299994,5.2,1.79454853799998));
#342977=CARTESIAN_POINT('Ctrl Pts',(3.59961258299994,2.2,1.79454853799998));
#342978=CARTESIAN_POINT('Ctrl Pts',(3.59903860199994,12.2,1.79434283699999));
#342979=CARTESIAN_POINT('Ctrl Pts',(3.59903860199994,5.2,1.79434283699999));
#342980=CARTESIAN_POINT('Ctrl Pts',(3.59903860199994,2.2,1.79434283699999));
#342981=CARTESIAN_POINT('Ctrl Pts',(3.59847070999994,12.2,1.79413849399999));
#342982=CARTESIAN_POINT('Ctrl Pts',(3.59847070999994,5.2,1.79413849399999));
#342983=CARTESIAN_POINT('Ctrl Pts',(3.59847070999994,2.2,1.79413849399999));
#342984=CARTESIAN_POINT('Ctrl Pts',(3.59790891199994,12.2,1.79393552899999));
#342985=CARTESIAN_POINT('Ctrl Pts',(3.59790891199994,5.2,1.79393552899999));
#342986=CARTESIAN_POINT('Ctrl Pts',(3.59790891199994,2.2,1.79393552899999));
#342987=CARTESIAN_POINT('Ctrl Pts',(3.59735321699994,12.2,1.79373395799999));
#342988=CARTESIAN_POINT('Ctrl Pts',(3.59735321699994,5.2,1.79373395799999));
#342989=CARTESIAN_POINT('Ctrl Pts',(3.59735321699994,2.2,1.79373395799999));
#342990=CARTESIAN_POINT('Ctrl Pts',(3.59680362899994,12.2,1.79353380499998));
#342991=CARTESIAN_POINT('Ctrl Pts',(3.59680362899994,5.2,1.79353380499998));
#342992=CARTESIAN_POINT('Ctrl Pts',(3.59680362899994,2.2,1.79353380499998));
#342993=CARTESIAN_POINT('Ctrl Pts',(3.59626015799994,12.2,1.79333508399999));
#342994=CARTESIAN_POINT('Ctrl Pts',(3.59626015799994,5.2,1.79333508399999));
#342995=CARTESIAN_POINT('Ctrl Pts',(3.59626015799994,2.2,1.79333508399999));
#342996=CARTESIAN_POINT('Ctrl Pts',(3.59572280899994,12.2,1.79313781699999));
#342997=CARTESIAN_POINT('Ctrl Pts',(3.59572280899994,5.2,1.79313781699999));
#342998=CARTESIAN_POINT('Ctrl Pts',(3.59572280899994,2.2,1.79313781699999));
#342999=CARTESIAN_POINT('Ctrl Pts',(3.59519158999994,12.2,1.79294202399999));
#343000=CARTESIAN_POINT('Ctrl Pts',(3.59519158999994,5.2,1.79294202399999));
#343001=CARTESIAN_POINT('Ctrl Pts',(3.59519158999994,2.2,1.79294202399999));
#343002=CARTESIAN_POINT('Ctrl Pts',(3.59466650499995,12.2,1.79274772199999));
#343003=CARTESIAN_POINT('Ctrl Pts',(3.59466650499995,5.2,1.79274772199999));
#343004=CARTESIAN_POINT('Ctrl Pts',(3.59466650499995,2.2,1.79274772199999));
#343005=CARTESIAN_POINT('Ctrl Pts',(3.59414756599994,12.2,1.79255492999999));
#343006=CARTESIAN_POINT('Ctrl Pts',(3.59414756599994,5.2,1.79255492999999));
#343007=CARTESIAN_POINT('Ctrl Pts',(3.59414756599994,2.2,1.79255492999999));
#343008=CARTESIAN_POINT('Ctrl Pts',(3.59363477599994,12.2,1.79236366999998));
#343009=CARTESIAN_POINT('Ctrl Pts',(3.59363477599994,5.2,1.79236366999998));
#343010=CARTESIAN_POINT('Ctrl Pts',(3.59363477599994,2.2,1.79236366999998));
#343011=CARTESIAN_POINT('Ctrl Pts',(3.59312814299994,12.2,1.79217395899999));
#343012=CARTESIAN_POINT('Ctrl Pts',(3.59312814299994,5.2,1.79217395899999));
#343013=CARTESIAN_POINT('Ctrl Pts',(3.59312814299994,2.2,1.79217395899999));
#343014=CARTESIAN_POINT('Ctrl Pts',(3.59262767399994,12.2,1.79198581899998));
#343015=CARTESIAN_POINT('Ctrl Pts',(3.59262767399994,5.2,1.79198581899998));
#343016=CARTESIAN_POINT('Ctrl Pts',(3.59262767399994,2.2,1.79198581899998));
#343017=CARTESIAN_POINT('Ctrl Pts',(3.59213337499994,12.2,1.79179926699998));
#343018=CARTESIAN_POINT('Ctrl Pts',(3.59213337499994,5.2,1.79179926699998));
#343019=CARTESIAN_POINT('Ctrl Pts',(3.59213337499994,2.2,1.79179926699998));
#343020=CARTESIAN_POINT('Ctrl Pts',(3.59164525599994,12.2,1.79161432399999));
#343021=CARTESIAN_POINT('Ctrl Pts',(3.59164525599994,5.2,1.79161432399999));
#343022=CARTESIAN_POINT('Ctrl Pts',(3.59164525599994,2.2,1.79161432399999));
#343023=CARTESIAN_POINT('Ctrl Pts',(3.59116331899994,12.2,1.79143100999998));
#343024=CARTESIAN_POINT('Ctrl Pts',(3.59116331899994,5.2,1.79143100999998));
#343025=CARTESIAN_POINT('Ctrl Pts',(3.59116331899994,2.2,1.79143100999998));
#343026=CARTESIAN_POINT('Ctrl Pts',(3.59068757599994,12.2,1.79124934399999));
#343027=CARTESIAN_POINT('Ctrl Pts',(3.59068757599994,5.2,1.79124934399999));
#343028=CARTESIAN_POINT('Ctrl Pts',(3.59068757599994,2.2,1.79124934399999));
#343029=CARTESIAN_POINT('Ctrl Pts',(3.59021802899994,12.2,1.79106934699998));
#343030=CARTESIAN_POINT('Ctrl Pts',(3.59021802899994,5.2,1.79106934699998));
#343031=CARTESIAN_POINT('Ctrl Pts',(3.59021802899994,2.2,1.79106934699998));
#343032=CARTESIAN_POINT('Ctrl Pts',(3.58975468999994,12.2,1.79089103799999));
#343033=CARTESIAN_POINT('Ctrl Pts',(3.58975468999994,5.2,1.79089103799999));
#343034=CARTESIAN_POINT('Ctrl Pts',(3.58975468999994,2.2,1.79089103799999));
#343035=CARTESIAN_POINT('Ctrl Pts',(3.58929756199994,12.2,1.79071443699999));
#343036=CARTESIAN_POINT('Ctrl Pts',(3.58929756199994,5.2,1.79071443699999));
#343037=CARTESIAN_POINT('Ctrl Pts',(3.58929756199994,2.2,1.79071443699999));
#343038=CARTESIAN_POINT('Ctrl Pts',(3.58884665299994,12.2,1.79053956299999));
#343039=CARTESIAN_POINT('Ctrl Pts',(3.58884665299994,5.2,1.79053956299999));
#343040=CARTESIAN_POINT('Ctrl Pts',(3.58884665299994,2.2,1.79053956299999));
#343041=CARTESIAN_POINT('Ctrl Pts',(3.58840196999994,12.2,1.79036643899999));
#343042=CARTESIAN_POINT('Ctrl Pts',(3.58840196999994,5.2,1.79036643899999));
#343043=CARTESIAN_POINT('Ctrl Pts',(3.58840196999994,2.2,1.79036643899999));
#343044=CARTESIAN_POINT('Ctrl Pts',(3.58796351999994,12.2,1.79019508399998));
#343045=CARTESIAN_POINT('Ctrl Pts',(3.58796351999994,5.2,1.79019508399998));
#343046=CARTESIAN_POINT('Ctrl Pts',(3.58796351999994,2.2,1.79019508399998));
#343047=CARTESIAN_POINT('Ctrl Pts',(3.58753130999994,12.2,1.79002551699998));
#343048=CARTESIAN_POINT('Ctrl Pts',(3.58753130999994,5.2,1.79002551699998));
#343049=CARTESIAN_POINT('Ctrl Pts',(3.58753130999994,2.2,1.79002551699998));
#343050=CARTESIAN_POINT('Ctrl Pts',(3.58710534699994,12.2,1.78985775999998));
#343051=CARTESIAN_POINT('Ctrl Pts',(3.58710534699994,5.2,1.78985775999998));
#343052=CARTESIAN_POINT('Ctrl Pts',(3.58710534699994,2.2,1.78985775999998));
#343053=CARTESIAN_POINT('Ctrl Pts',(3.58668563699994,12.2,1.78969183199999));
#343054=CARTESIAN_POINT('Ctrl Pts',(3.58668563699994,5.2,1.78969183199999));
#343055=CARTESIAN_POINT('Ctrl Pts',(3.58668563699994,2.2,1.78969183199999));
#343056=CARTESIAN_POINT('Ctrl Pts',(3.58627218799994,12.2,1.78952775499999));
#343057=CARTESIAN_POINT('Ctrl Pts',(3.58627218799994,5.2,1.78952775499999));
#343058=CARTESIAN_POINT('Ctrl Pts',(3.58627218799994,2.2,1.78952775499999));
#343059=CARTESIAN_POINT('Ctrl Pts',(3.58586500599994,12.2,1.78936554899999));
#343060=CARTESIAN_POINT('Ctrl Pts',(3.58586500599994,5.2,1.78936554899999));
#343061=CARTESIAN_POINT('Ctrl Pts',(3.58586500599994,2.2,1.78936554899999));
#343062=CARTESIAN_POINT('Ctrl Pts',(3.58546409799994,12.2,1.78920523399999));
#343063=CARTESIAN_POINT('Ctrl Pts',(3.58546409799994,5.2,1.78920523399999));
#343064=CARTESIAN_POINT('Ctrl Pts',(3.58546409799994,2.2,1.78920523399999));
#343065=CARTESIAN_POINT('Ctrl Pts',(3.58506947199994,12.2,1.78904683199999));
#343066=CARTESIAN_POINT('Ctrl Pts',(3.58506947199994,5.2,1.78904683199999));
#343067=CARTESIAN_POINT('Ctrl Pts',(3.58506947199994,2.2,1.78904683199999));
#343068=CARTESIAN_POINT('Ctrl Pts',(3.58468113399994,12.2,1.78889036299998));
#343069=CARTESIAN_POINT('Ctrl Pts',(3.58468113399994,5.2,1.78889036299998));
#343070=CARTESIAN_POINT('Ctrl Pts',(3.58468113399994,2.2,1.78889036299998));
#343071=CARTESIAN_POINT('Ctrl Pts',(3.58429908999994,12.2,1.78873584799998));
#343072=CARTESIAN_POINT('Ctrl Pts',(3.58429908999994,5.2,1.78873584799998));
#343073=CARTESIAN_POINT('Ctrl Pts',(3.58429908999994,2.2,1.78873584799998));
#343074=CARTESIAN_POINT('Ctrl Pts',(3.58392334799994,12.2,1.78858330799998));
#343075=CARTESIAN_POINT('Ctrl Pts',(3.58392334799994,5.2,1.78858330799998));
#343076=CARTESIAN_POINT('Ctrl Pts',(3.58392334799994,2.2,1.78858330799998));
#343077=CARTESIAN_POINT('Ctrl Pts',(3.58355391499994,12.2,1.78843276399999));
#343078=CARTESIAN_POINT('Ctrl Pts',(3.58355391499994,5.2,1.78843276399999));
#343079=CARTESIAN_POINT('Ctrl Pts',(3.58355391499994,2.2,1.78843276399999));
#343080=CARTESIAN_POINT('Ctrl Pts',(3.58319079699994,12.2,1.78828423699999));
#343081=CARTESIAN_POINT('Ctrl Pts',(3.58319079699994,5.2,1.78828423699999));
#343082=CARTESIAN_POINT('Ctrl Pts',(3.58319079699994,2.2,1.78828423699999));
#343083=CARTESIAN_POINT('Ctrl Pts',(3.58283400099995,12.2,1.78813774899998));
#343084=CARTESIAN_POINT('Ctrl Pts',(3.58283400099995,5.2,1.78813774899998));
#343085=CARTESIAN_POINT('Ctrl Pts',(3.58283400099995,2.2,1.78813774899998));
#343086=CARTESIAN_POINT('Ctrl Pts',(3.58248353499994,12.2,1.78799332099999));
#343087=CARTESIAN_POINT('Ctrl Pts',(3.58248353499994,5.2,1.78799332099999));
#343088=CARTESIAN_POINT('Ctrl Pts',(3.58248353499994,2.2,1.78799332099999));
#343089=CARTESIAN_POINT('Ctrl Pts',(3.58213940499994,12.2,1.78785097299999));
#343090=CARTESIAN_POINT('Ctrl Pts',(3.58213940499994,5.2,1.78785097299999));
#343091=CARTESIAN_POINT('Ctrl Pts',(3.58213940499994,2.2,1.78785097299999));
#343092=CARTESIAN_POINT('Ctrl Pts',(3.58180161799994,12.2,1.78771072799998));
#343093=CARTESIAN_POINT('Ctrl Pts',(3.58180161799994,5.2,1.78771072799998));
#343094=CARTESIAN_POINT('Ctrl Pts',(3.58180161799994,2.2,1.78771072799998));
#343095=CARTESIAN_POINT('Ctrl Pts',(3.58147017999995,12.2,1.78757260699999));
#343096=CARTESIAN_POINT('Ctrl Pts',(3.58147017999995,5.2,1.78757260699999));
#343097=CARTESIAN_POINT('Ctrl Pts',(3.58147017999995,2.2,1.78757260699999));
#343098=CARTESIAN_POINT('Ctrl Pts',(3.58114509999994,12.2,1.78743663099999));
#343099=CARTESIAN_POINT('Ctrl Pts',(3.58114509999994,5.2,1.78743663099999));
#343100=CARTESIAN_POINT('Ctrl Pts',(3.58114509999994,2.2,1.78743663099999));
#343101=CARTESIAN_POINT('Ctrl Pts',(3.58082638199994,12.2,1.78730282199998));
#343102=CARTESIAN_POINT('Ctrl Pts',(3.58082638199994,5.2,1.78730282199998));
#343103=CARTESIAN_POINT('Ctrl Pts',(3.58082638199994,2.2,1.78730282199998));
#343104=CARTESIAN_POINT('Ctrl Pts',(3.58051403599994,12.2,1.78717120299998));
#343105=CARTESIAN_POINT('Ctrl Pts',(3.58051403599994,5.2,1.78717120299998));
#343106=CARTESIAN_POINT('Ctrl Pts',(3.58051403599994,2.2,1.78717120299998));
#343107=CARTESIAN_POINT('Ctrl Pts',(3.58020806599994,12.2,1.78704179399999));
#343108=CARTESIAN_POINT('Ctrl Pts',(3.58020806599994,5.2,1.78704179399999));
#343109=CARTESIAN_POINT('Ctrl Pts',(3.58020806599994,2.2,1.78704179399999));
#343110=CARTESIAN_POINT('Ctrl Pts',(3.57990847899994,12.2,1.78691461799998));
#343111=CARTESIAN_POINT('Ctrl Pts',(3.57990847899994,5.2,1.78691461799998));
#343112=CARTESIAN_POINT('Ctrl Pts',(3.57990847899994,2.2,1.78691461799998));
#343113=CARTESIAN_POINT('Ctrl Pts',(3.57961528499994,12.2,1.78678969699999));
#343114=CARTESIAN_POINT('Ctrl Pts',(3.57961528499994,5.2,1.78678969699999));
#343115=CARTESIAN_POINT('Ctrl Pts',(3.57961528499994,2.2,1.78678969699999));
#343116=CARTESIAN_POINT('Ctrl Pts',(3.57932848799994,12.2,1.78666705199999));
#343117=CARTESIAN_POINT('Ctrl Pts',(3.57932848799994,5.2,1.78666705199999));
#343118=CARTESIAN_POINT('Ctrl Pts',(3.57932848799994,2.2,1.78666705199999));
#343119=CARTESIAN_POINT('Ctrl Pts',(3.57904809599995,12.2,1.78654670699999));
#343120=CARTESIAN_POINT('Ctrl Pts',(3.57904809599995,5.2,1.78654670699999));
#343121=CARTESIAN_POINT('Ctrl Pts',(3.57904809599995,2.2,1.78654670699999));
#343122=CARTESIAN_POINT('Ctrl Pts',(3.57877411399994,12.2,1.78642868299999));
#343123=CARTESIAN_POINT('Ctrl Pts',(3.57877411399994,5.2,1.78642868299999));
#343124=CARTESIAN_POINT('Ctrl Pts',(3.57877411399994,2.2,1.78642868299999));
#343125=CARTESIAN_POINT('Ctrl Pts',(3.57850655199994,12.2,1.78631300199998));
#343126=CARTESIAN_POINT('Ctrl Pts',(3.57850655199994,5.2,1.78631300199998));
#343127=CARTESIAN_POINT('Ctrl Pts',(3.57850655199994,2.2,1.78631300199998));
#343128=CARTESIAN_POINT('Ctrl Pts',(3.57824541399994,12.2,1.78619968699998));
#343129=CARTESIAN_POINT('Ctrl Pts',(3.57824541399994,5.2,1.78619968699998));
#343130=CARTESIAN_POINT('Ctrl Pts',(3.57824541399994,2.2,1.78619968699998));
#343131=CARTESIAN_POINT('Ctrl Pts',(3.57799070899994,12.2,1.78608875999998));
#343132=CARTESIAN_POINT('Ctrl Pts',(3.57799070899994,5.2,1.78608875999998));
#343133=CARTESIAN_POINT('Ctrl Pts',(3.57799070899994,2.2,1.78608875999998));
#343134=CARTESIAN_POINT('Ctrl Pts',(3.57774244199994,12.2,1.78598024399999));
#343135=CARTESIAN_POINT('Ctrl Pts',(3.57774244199994,5.2,1.78598024399999));
#343136=CARTESIAN_POINT('Ctrl Pts',(3.57774244199994,2.2,1.78598024399999));
#343137=CARTESIAN_POINT('Ctrl Pts',(3.57750061999994,12.2,1.78587416299999));
#343138=CARTESIAN_POINT('Ctrl Pts',(3.57750061999994,5.2,1.78587416299999));
#343139=CARTESIAN_POINT('Ctrl Pts',(3.57750061999994,2.2,1.78587416299999));
#343140=CARTESIAN_POINT('Ctrl Pts',(3.57726525199995,12.2,1.78577053699998));
#343141=CARTESIAN_POINT('Ctrl Pts',(3.57726525199995,5.2,1.78577053699998));
#343142=CARTESIAN_POINT('Ctrl Pts',(3.57726525199995,2.2,1.78577053699998));
#343143=CARTESIAN_POINT('Ctrl Pts',(3.57703634199994,12.2,1.78566938999999));
#343144=CARTESIAN_POINT('Ctrl Pts',(3.57703634199994,5.2,1.78566938999999));
#343145=CARTESIAN_POINT('Ctrl Pts',(3.57703634199994,2.2,1.78566938999999));
#343146=CARTESIAN_POINT('Ctrl Pts',(3.57681389999994,12.2,1.78557074599999));
#343147=CARTESIAN_POINT('Ctrl Pts',(3.57681389999994,5.2,1.78557074599999));
#343148=CARTESIAN_POINT('Ctrl Pts',(3.57681389999994,2.2,1.78557074599999));
#343149=CARTESIAN_POINT('Ctrl Pts',(3.57659792899994,12.2,1.78547462699999));
#343150=CARTESIAN_POINT('Ctrl Pts',(3.57659792899994,5.2,1.78547462699999));
#343151=CARTESIAN_POINT('Ctrl Pts',(3.57659792899994,2.2,1.78547462699999));
#343152=CARTESIAN_POINT('Ctrl Pts',(3.57638843899994,12.2,1.78538105599999));
#343153=CARTESIAN_POINT('Ctrl Pts',(3.57638843899994,5.2,1.78538105599999));
#343154=CARTESIAN_POINT('Ctrl Pts',(3.57638843899994,2.2,1.78538105599999));
#343155=CARTESIAN_POINT('Ctrl Pts',(3.57618543499994,12.2,1.78529005699998));
#343156=CARTESIAN_POINT('Ctrl Pts',(3.57618543499994,5.2,1.78529005699998));
#343157=CARTESIAN_POINT('Ctrl Pts',(3.57618543499994,2.2,1.78529005699998));
#343158=CARTESIAN_POINT('Ctrl Pts',(3.57598892399994,12.2,1.78520165199998));
#343159=CARTESIAN_POINT('Ctrl Pts',(3.57598892399994,5.2,1.78520165199998));
#343160=CARTESIAN_POINT('Ctrl Pts',(3.57598892399994,2.2,1.78520165199998));
#343161=CARTESIAN_POINT('Ctrl Pts',(3.57579891299994,12.2,1.78511586499999));
#343162=CARTESIAN_POINT('Ctrl Pts',(3.57579891299994,5.2,1.78511586499999));
#343163=CARTESIAN_POINT('Ctrl Pts',(3.57579891299994,2.2,1.78511586499999));
#343164=CARTESIAN_POINT('Ctrl Pts',(3.57561540999995,12.2,1.78503271999999));
#343165=CARTESIAN_POINT('Ctrl Pts',(3.57561540999995,5.2,1.78503271999999));
#343166=CARTESIAN_POINT('Ctrl Pts',(3.57561540999995,2.2,1.78503271999999));
#343167=CARTESIAN_POINT('Ctrl Pts',(3.57543842099994,12.2,1.78495223999999));
#343168=CARTESIAN_POINT('Ctrl Pts',(3.57543842099994,5.2,1.78495223999999));
#343169=CARTESIAN_POINT('Ctrl Pts',(3.57543842099994,2.2,1.78495223999999));
#343170=CARTESIAN_POINT('Ctrl Pts',(3.57526795299994,12.2,1.78487444899998));
#343171=CARTESIAN_POINT('Ctrl Pts',(3.57526795299994,5.2,1.78487444899998));
#343172=CARTESIAN_POINT('Ctrl Pts',(3.57526795299994,2.2,1.78487444899998));
#343173=CARTESIAN_POINT('Ctrl Pts',(3.57510401099994,12.2,1.78479937099999));
#343174=CARTESIAN_POINT('Ctrl Pts',(3.57510401099994,5.2,1.78479937099999));
#343175=CARTESIAN_POINT('Ctrl Pts',(3.57510401099994,2.2,1.78479937099999));
#343176=CARTESIAN_POINT('Ctrl Pts',(3.57494660499994,12.2,1.78472702899999));
#343177=CARTESIAN_POINT('Ctrl Pts',(3.57494660499994,5.2,1.78472702899999));
#343178=CARTESIAN_POINT('Ctrl Pts',(3.57494660499994,2.2,1.78472702899999));
#343179=CARTESIAN_POINT('Ctrl Pts',(3.57479573999994,12.2,1.78465744599999));
#343180=CARTESIAN_POINT('Ctrl Pts',(3.57479573999994,5.2,1.78465744599999));
#343181=CARTESIAN_POINT('Ctrl Pts',(3.57479573999994,2.2,1.78465744599999));
#343182=CARTESIAN_POINT('Ctrl Pts',(3.57465142099994,12.2,1.78459064599998));
#343183=CARTESIAN_POINT('Ctrl Pts',(3.57465142099994,5.2,1.78459064599998));
#343184=CARTESIAN_POINT('Ctrl Pts',(3.57465142099994,2.2,1.78459064599998));
#343185=CARTESIAN_POINT('Ctrl Pts',(3.57451365799994,12.2,1.78452665399998));
#343186=CARTESIAN_POINT('Ctrl Pts',(3.57451365799994,5.2,1.78452665399998));
#343187=CARTESIAN_POINT('Ctrl Pts',(3.57451365799994,2.2,1.78452665399998));
#343188=CARTESIAN_POINT('Ctrl Pts',(3.57438245599994,12.2,1.78446549499998));
#343189=CARTESIAN_POINT('Ctrl Pts',(3.57438245599994,5.2,1.78446549499998));
#343190=CARTESIAN_POINT('Ctrl Pts',(3.57438245599994,2.2,1.78446549499998));
#343191=CARTESIAN_POINT('Ctrl Pts',(3.57425782399994,12.2,1.78440719399998));
#343192=CARTESIAN_POINT('Ctrl Pts',(3.57425782399994,5.2,1.78440719399998));
#343193=CARTESIAN_POINT('Ctrl Pts',(3.57425782399994,2.2,1.78440719399998));
#343194=CARTESIAN_POINT('Ctrl Pts',(3.57413976699994,12.2,1.78435177699999));
#343195=CARTESIAN_POINT('Ctrl Pts',(3.57413976699994,5.2,1.78435177699999));
#343196=CARTESIAN_POINT('Ctrl Pts',(3.57413976699994,2.2,1.78435177699999));
#343197=CARTESIAN_POINT('Ctrl Pts',(3.57402829299994,12.2,1.78429926699998));
#343198=CARTESIAN_POINT('Ctrl Pts',(3.57402829299994,5.2,1.78429926699998));
#343199=CARTESIAN_POINT('Ctrl Pts',(3.57402829299994,2.2,1.78429926699998));
#343200=CARTESIAN_POINT('Ctrl Pts',(3.57392340599994,12.2,1.78424968799999));
#343201=CARTESIAN_POINT('Ctrl Pts',(3.57392340599994,5.2,1.78424968799999));
#343202=CARTESIAN_POINT('Ctrl Pts',(3.57392340599994,2.2,1.78424968799999));
#343203=CARTESIAN_POINT('Ctrl Pts',(3.57382511499994,12.2,1.78420305899999));
#343204=CARTESIAN_POINT('Ctrl Pts',(3.57382511499994,5.2,1.78420305899999));
#343205=CARTESIAN_POINT('Ctrl Pts',(3.57382511499994,2.2,1.78420305899999));
#343206=CARTESIAN_POINT('Ctrl Pts',(3.57373342599994,12.2,1.78415940499999));
#343207=CARTESIAN_POINT('Ctrl Pts',(3.57373342599994,5.2,1.78415940499999));
#343208=CARTESIAN_POINT('Ctrl Pts',(3.57373342599994,2.2,1.78415940499999));
#343209=CARTESIAN_POINT('Ctrl Pts',(3.57364834299994,12.2,1.78411874999998));
#343210=CARTESIAN_POINT('Ctrl Pts',(3.57364834299994,5.2,1.78411874999998));
#343211=CARTESIAN_POINT('Ctrl Pts',(3.57364834299994,2.2,1.78411874999998));
#343212=CARTESIAN_POINT('Ctrl Pts',(3.57356987599994,12.2,1.78408112399998));
#343213=CARTESIAN_POINT('Ctrl Pts',(3.57356987599994,5.2,1.78408112399998));
#343214=CARTESIAN_POINT('Ctrl Pts',(3.57356987599994,2.2,1.78408112399998));
#343215=CARTESIAN_POINT('Ctrl Pts',(3.57349803399994,12.2,1.78404655699998));
#343216=CARTESIAN_POINT('Ctrl Pts',(3.57349803399994,5.2,1.78404655699998));
#343217=CARTESIAN_POINT('Ctrl Pts',(3.57349803399994,2.2,1.78404655699998));
#343218=CARTESIAN_POINT('Ctrl Pts',(3.57343282299994,12.2,1.78401508199999));
#343219=CARTESIAN_POINT('Ctrl Pts',(3.57343282299994,5.2,1.78401508199999));
#343220=CARTESIAN_POINT('Ctrl Pts',(3.57343282299994,2.2,1.78401508199999));
#343221=CARTESIAN_POINT('Ctrl Pts',(3.57337425399994,12.2,1.78398672599998));
#343222=CARTESIAN_POINT('Ctrl Pts',(3.57337425399994,5.2,1.78398672599998));
#343223=CARTESIAN_POINT('Ctrl Pts',(3.57337425399994,2.2,1.78398672599998));
#343224=CARTESIAN_POINT('Ctrl Pts',(3.57332232999994,12.2,1.78396150999999));
#343225=CARTESIAN_POINT('Ctrl Pts',(3.57332232999994,5.2,1.78396150999999));
#343226=CARTESIAN_POINT('Ctrl Pts',(3.57332232999994,2.2,1.78396150999999));
#343227=CARTESIAN_POINT('Ctrl Pts',(3.57327705499995,12.2,1.78393944699998));
#343228=CARTESIAN_POINT('Ctrl Pts',(3.57327705499995,5.2,1.78393944699998));
#343229=CARTESIAN_POINT('Ctrl Pts',(3.57327705499995,2.2,1.78393944699998));
#343230=CARTESIAN_POINT('Ctrl Pts',(3.57324615599994,12.2,1.78392432099999));
#343231=CARTESIAN_POINT('Ctrl Pts',(3.57324615599994,5.2,1.78392432099999));
#343232=CARTESIAN_POINT('Ctrl Pts',(3.57324615599994,2.2,1.78392432099999));
#343233=CARTESIAN_POINT('Ctrl Pts',(3.57322597299994,12.2,1.78391439999999));
#343234=CARTESIAN_POINT('Ctrl Pts',(3.57322597299994,5.2,1.78391439999999));
#343235=CARTESIAN_POINT('Ctrl Pts',(3.57322597299994,2.2,1.78391439999999));
#343236=CARTESIAN_POINT('Ctrl Pts',(3.57321384899994,12.2,1.78390841799999));
#343237=CARTESIAN_POINT('Ctrl Pts',(3.57321384899994,5.2,1.78390841799999));
#343238=CARTESIAN_POINT('Ctrl Pts',(3.57321384899994,2.2,1.78390841799999));
#343239=CARTESIAN_POINT('Ctrl Pts',(3.57320811899994,12.2,1.78390558399999));
#343240=CARTESIAN_POINT('Ctrl Pts',(3.57320811899994,5.2,1.78390558399999));
#343241=CARTESIAN_POINT('Ctrl Pts',(3.57320811899994,2.2,1.78390558399999));
#343242=CARTESIAN_POINT('',(4.39111701799995,12.2,1.81124027399999));
#343243=CARTESIAN_POINT('Origin',(-5.66300478732629E-14,15.2,-1.77635683940025E-14));
#343244=CARTESIAN_POINT('',(4.50847758599994,12.2,1.49536946999998));
#343245=CARTESIAN_POINT('Ctrl Pts',(3.87111406899994,12.2,0.982007125999989));
#343246=CARTESIAN_POINT('Ctrl Pts',(3.87111406899994,5.2,0.982007125999989));
#343247=CARTESIAN_POINT('Ctrl Pts',(3.87111406899994,2.2,0.982007125999989));
#343248=CARTESIAN_POINT('Ctrl Pts',(3.87112069459513,12.2,0.98200883489564));
#343249=CARTESIAN_POINT('Ctrl Pts',(3.87112069459513,5.2,0.98200883489564));
#343250=CARTESIAN_POINT('Ctrl Pts',(3.87112069459513,2.2,0.98200883489564));
#343251=CARTESIAN_POINT('Ctrl Pts',(3.87113351057882,12.2,0.982012138502726));
#343252=CARTESIAN_POINT('Ctrl Pts',(3.87113351057882,5.2,0.982012138502726));
#343253=CARTESIAN_POINT('Ctrl Pts',(3.87113351057882,2.2,0.982012138502726));
#343254=CARTESIAN_POINT('Ctrl Pts',(3.8711525108998,12.2,0.982017032143299));
#343255=CARTESIAN_POINT('Ctrl Pts',(3.8711525108998,5.2,0.982017032143299));
#343256=CARTESIAN_POINT('Ctrl Pts',(3.8711525108998,2.2,0.982017032143299));
#343257=CARTESIAN_POINT('Ctrl Pts',(3.87117775167996,12.2,0.982023550844282));
#343258=CARTESIAN_POINT('Ctrl Pts',(3.87117775167996,5.2,0.982023550844282));
#343259=CARTESIAN_POINT('Ctrl Pts',(3.87117775167996,2.2,0.982023550844282));
#343260=CARTESIAN_POINT('Ctrl Pts',(3.87122151999994,12.2,0.982035030999988));
#343261=CARTESIAN_POINT('Ctrl Pts',(3.87122151999994,5.2,0.982035030999988));
#343262=CARTESIAN_POINT('Ctrl Pts',(3.87122151999994,2.2,0.982035030999988));
#343263=CARTESIAN_POINT('Ctrl Pts',(3.87127021899994,12.2,0.982047882999986));
#343264=CARTESIAN_POINT('Ctrl Pts',(3.87127021899994,5.2,0.982047882999986));
#343265=CARTESIAN_POINT('Ctrl Pts',(3.87127021899994,2.2,0.982047882999986));
#343266=CARTESIAN_POINT('Ctrl Pts',(3.87132600999994,12.2,0.982062687999985));
#343267=CARTESIAN_POINT('Ctrl Pts',(3.87132600999994,5.2,0.982062687999985));
#343268=CARTESIAN_POINT('Ctrl Pts',(3.87132600999994,2.2,0.982062687999985));
#343269=CARTESIAN_POINT('Ctrl Pts',(3.87138888599994,12.2,0.982079453999987));
#343270=CARTESIAN_POINT('Ctrl Pts',(3.87138888599994,5.2,0.982079453999987));
#343271=CARTESIAN_POINT('Ctrl Pts',(3.87138888599994,2.2,0.982079453999987));
#343272=CARTESIAN_POINT('Ctrl Pts',(3.87145882699994,12.2,0.982098194999987));
#343273=CARTESIAN_POINT('Ctrl Pts',(3.87145882699994,5.2,0.982098194999987));
#343274=CARTESIAN_POINT('Ctrl Pts',(3.87145882699994,2.2,0.982098194999987));
#343275=CARTESIAN_POINT('Ctrl Pts',(3.87153580999994,12.2,0.982118923999984));
#343276=CARTESIAN_POINT('Ctrl Pts',(3.87153580999994,5.2,0.982118923999984));
#343277=CARTESIAN_POINT('Ctrl Pts',(3.87153580999994,2.2,0.982118923999984));
#343278=CARTESIAN_POINT('Ctrl Pts',(3.87161980999994,12.2,0.982141659999982));
#343279=CARTESIAN_POINT('Ctrl Pts',(3.87161980999994,5.2,0.982141659999982));
#343280=CARTESIAN_POINT('Ctrl Pts',(3.87161980999994,2.2,0.982141659999982));
#343281=CARTESIAN_POINT('Ctrl Pts',(3.87171079599994,12.2,0.982166423999988));
#343282=CARTESIAN_POINT('Ctrl Pts',(3.87171079599994,5.2,0.982166423999988));
#343283=CARTESIAN_POINT('Ctrl Pts',(3.87171079599994,2.2,0.982166423999988));
#343284=CARTESIAN_POINT('Ctrl Pts',(3.87180874699994,12.2,0.982193229999986));
#343285=CARTESIAN_POINT('Ctrl Pts',(3.87180874699994,5.2,0.982193229999986));
#343286=CARTESIAN_POINT('Ctrl Pts',(3.87180874699994,2.2,0.982193229999986));
#343287=CARTESIAN_POINT('Ctrl Pts',(3.87191363799994,12.2,0.982222092999985));
#343288=CARTESIAN_POINT('Ctrl Pts',(3.87191363799994,5.2,0.982222092999985));
#343289=CARTESIAN_POINT('Ctrl Pts',(3.87191363799994,2.2,0.982222092999985));
#343290=CARTESIAN_POINT('Ctrl Pts',(3.87202545199994,12.2,0.982253026999986));
#343291=CARTESIAN_POINT('Ctrl Pts',(3.87202545199994,5.2,0.982253026999986));
#343292=CARTESIAN_POINT('Ctrl Pts',(3.87202545199994,2.2,0.982253026999986));
#343293=CARTESIAN_POINT('Ctrl Pts',(3.87214416899994,12.2,0.982286043999987));
#343294=CARTESIAN_POINT('Ctrl Pts',(3.87214416899994,5.2,0.982286043999987));
#343295=CARTESIAN_POINT('Ctrl Pts',(3.87214416899994,2.2,0.982286043999987));
#343296=CARTESIAN_POINT('Ctrl Pts',(3.87226976899994,12.2,0.982321156999983));
#343297=CARTESIAN_POINT('Ctrl Pts',(3.87226976899994,5.2,0.982321156999983));
#343298=CARTESIAN_POINT('Ctrl Pts',(3.87226976899994,2.2,0.982321156999983));
#343299=CARTESIAN_POINT('Ctrl Pts',(3.87240223399994,12.2,0.982358379999986));
#343300=CARTESIAN_POINT('Ctrl Pts',(3.87240223399994,5.2,0.982358379999986));
#343301=CARTESIAN_POINT('Ctrl Pts',(3.87240223399994,2.2,0.982358379999986));
#343302=CARTESIAN_POINT('Ctrl Pts',(3.87254153999994,12.2,0.982397726999986));
#343303=CARTESIAN_POINT('Ctrl Pts',(3.87254153999994,5.2,0.982397726999986));
#343304=CARTESIAN_POINT('Ctrl Pts',(3.87254153999994,2.2,0.982397726999986));
#343305=CARTESIAN_POINT('Ctrl Pts',(3.87268766499994,12.2,0.982439212999986));
#343306=CARTESIAN_POINT('Ctrl Pts',(3.87268766499994,5.2,0.982439212999986));
#343307=CARTESIAN_POINT('Ctrl Pts',(3.87268766499994,2.2,0.982439212999986));
#343308=CARTESIAN_POINT('Ctrl Pts',(3.87284058799994,12.2,0.982482850999986));
#343309=CARTESIAN_POINT('Ctrl Pts',(3.87284058799994,5.2,0.982482850999986));
#343310=CARTESIAN_POINT('Ctrl Pts',(3.87284058799994,2.2,0.982482850999986));
#343311=CARTESIAN_POINT('Ctrl Pts',(3.87300028899995,12.2,0.982528657999988));
#343312=CARTESIAN_POINT('Ctrl Pts',(3.87300028899995,5.2,0.982528657999988));
#343313=CARTESIAN_POINT('Ctrl Pts',(3.87300028899995,2.2,0.982528657999988));
#343314=CARTESIAN_POINT('Ctrl Pts',(3.87316674399994,12.2,0.982576645999984));
#343315=CARTESIAN_POINT('Ctrl Pts',(3.87316674399994,5.2,0.982576645999984));
#343316=CARTESIAN_POINT('Ctrl Pts',(3.87316674399994,2.2,0.982576645999984));
#343317=CARTESIAN_POINT('Ctrl Pts',(3.87333993499994,12.2,0.982626826999984));
#343318=CARTESIAN_POINT('Ctrl Pts',(3.87333993499994,5.2,0.982626826999984));
#343319=CARTESIAN_POINT('Ctrl Pts',(3.87333993499994,2.2,0.982626826999984));
#343320=CARTESIAN_POINT('Ctrl Pts',(3.87351984099995,12.2,0.982679216999984));
#343321=CARTESIAN_POINT('Ctrl Pts',(3.87351984099995,5.2,0.982679216999984));
#343322=CARTESIAN_POINT('Ctrl Pts',(3.87351984099995,2.2,0.982679216999984));
#343323=CARTESIAN_POINT('Ctrl Pts',(3.87370644199994,12.2,0.982733826999986));
#343324=CARTESIAN_POINT('Ctrl Pts',(3.87370644199994,5.2,0.982733826999986));
#343325=CARTESIAN_POINT('Ctrl Pts',(3.87370644199994,2.2,0.982733826999986));
#343326=CARTESIAN_POINT('Ctrl Pts',(3.87389971699994,12.2,0.982790672999982));
#343327=CARTESIAN_POINT('Ctrl Pts',(3.87389971699994,5.2,0.982790672999982));
#343328=CARTESIAN_POINT('Ctrl Pts',(3.87389971699994,2.2,0.982790672999982));
#343329=CARTESIAN_POINT('Ctrl Pts',(3.87409964499994,12.2,0.982849765999987));
#343330=CARTESIAN_POINT('Ctrl Pts',(3.87409964499994,5.2,0.982849765999987));
#343331=CARTESIAN_POINT('Ctrl Pts',(3.87409964499994,2.2,0.982849765999987));
#343332=CARTESIAN_POINT('Ctrl Pts',(3.87430620599994,12.2,0.982911120999983));
#343333=CARTESIAN_POINT('Ctrl Pts',(3.87430620599994,5.2,0.982911120999983));
#343334=CARTESIAN_POINT('Ctrl Pts',(3.87430620599994,2.2,0.982911120999983));
#343335=CARTESIAN_POINT('Ctrl Pts',(3.87451937999994,12.2,0.982974749999985));
#343336=CARTESIAN_POINT('Ctrl Pts',(3.87451937999994,5.2,0.982974749999985));
#343337=CARTESIAN_POINT('Ctrl Pts',(3.87451937999994,2.2,0.982974749999985));
#343338=CARTESIAN_POINT('Ctrl Pts',(3.87473914399994,12.2,0.983040666999986));
#343339=CARTESIAN_POINT('Ctrl Pts',(3.87473914399994,5.2,0.983040666999986));
#343340=CARTESIAN_POINT('Ctrl Pts',(3.87473914399994,2.2,0.983040666999986));
#343341=CARTESIAN_POINT('Ctrl Pts',(3.87496548099994,12.2,0.983108885999986));
#343342=CARTESIAN_POINT('Ctrl Pts',(3.87496548099994,5.2,0.983108885999986));
#343343=CARTESIAN_POINT('Ctrl Pts',(3.87496548099994,2.2,0.983108885999986));
#343344=CARTESIAN_POINT('Ctrl Pts',(3.87519836899994,12.2,0.983179417999986));
#343345=CARTESIAN_POINT('Ctrl Pts',(3.87519836899994,5.2,0.983179417999986));
#343346=CARTESIAN_POINT('Ctrl Pts',(3.87519836899994,2.2,0.983179417999986));
#343347=CARTESIAN_POINT('Ctrl Pts',(3.87543778799994,12.2,0.983252276999984));
#343348=CARTESIAN_POINT('Ctrl Pts',(3.87543778799994,5.2,0.983252276999984));
#343349=CARTESIAN_POINT('Ctrl Pts',(3.87543778799994,2.2,0.983252276999984));
#343350=CARTESIAN_POINT('Ctrl Pts',(3.87568371899994,12.2,0.983327476999989));
#343351=CARTESIAN_POINT('Ctrl Pts',(3.87568371899994,5.2,0.983327476999989));
#343352=CARTESIAN_POINT('Ctrl Pts',(3.87568371899994,2.2,0.983327476999989));
#343353=CARTESIAN_POINT('Ctrl Pts',(3.87593613999994,12.2,0.983405027999984));
#343354=CARTESIAN_POINT('Ctrl Pts',(3.87593613999994,5.2,0.983405027999984));
#343355=CARTESIAN_POINT('Ctrl Pts',(3.87593613999994,2.2,0.983405027999984));
#343356=CARTESIAN_POINT('Ctrl Pts',(3.87619503199994,12.2,0.983484946999984));
#343357=CARTESIAN_POINT('Ctrl Pts',(3.87619503199994,5.2,0.983484946999984));
#343358=CARTESIAN_POINT('Ctrl Pts',(3.87619503199994,2.2,0.983484946999984));
#343359=CARTESIAN_POINT('Ctrl Pts',(3.87646037599994,12.2,0.983567240999985));
#343360=CARTESIAN_POINT('Ctrl Pts',(3.87646037599994,5.2,0.983567240999985));
#343361=CARTESIAN_POINT('Ctrl Pts',(3.87646037599994,2.2,0.983567240999985));
#343362=CARTESIAN_POINT('Ctrl Pts',(3.87673214999994,12.2,0.983651927999984));
#343363=CARTESIAN_POINT('Ctrl Pts',(3.87673214999994,5.2,0.983651927999984));
#343364=CARTESIAN_POINT('Ctrl Pts',(3.87673214999994,2.2,0.983651927999984));
#343365=CARTESIAN_POINT('Ctrl Pts',(3.87701033499994,12.2,0.983739017999987));
#343366=CARTESIAN_POINT('Ctrl Pts',(3.87701033499994,5.2,0.983739017999987));
#343367=CARTESIAN_POINT('Ctrl Pts',(3.87701033499994,2.2,0.983739017999987));
#343368=CARTESIAN_POINT('Ctrl Pts',(3.87729491299994,12.2,0.983828522999985));
#343369=CARTESIAN_POINT('Ctrl Pts',(3.87729491299994,5.2,0.983828522999985));
#343370=CARTESIAN_POINT('Ctrl Pts',(3.87729491299994,2.2,0.983828522999985));
#343371=CARTESIAN_POINT('Ctrl Pts',(3.87758586199995,12.2,0.983920457999985));
#343372=CARTESIAN_POINT('Ctrl Pts',(3.87758586199995,5.2,0.983920457999985));
#343373=CARTESIAN_POINT('Ctrl Pts',(3.87758586199995,2.2,0.983920457999985));
#343374=CARTESIAN_POINT('Ctrl Pts',(3.87788316199994,12.2,0.984014831999982));
#343375=CARTESIAN_POINT('Ctrl Pts',(3.87788316199994,5.2,0.984014831999982));
#343376=CARTESIAN_POINT('Ctrl Pts',(3.87788316199994,2.2,0.984014831999982));
#343377=CARTESIAN_POINT('Ctrl Pts',(3.87818679499994,12.2,0.984111659999982));
#343378=CARTESIAN_POINT('Ctrl Pts',(3.87818679499994,5.2,0.984111659999982));
#343379=CARTESIAN_POINT('Ctrl Pts',(3.87818679499994,2.2,0.984111659999982));
#343380=CARTESIAN_POINT('Ctrl Pts',(3.87849674099995,12.2,0.984210952999987));
#343381=CARTESIAN_POINT('Ctrl Pts',(3.87849674099995,5.2,0.984210952999987));
#343382=CARTESIAN_POINT('Ctrl Pts',(3.87849674099995,2.2,0.984210952999987));
#343383=CARTESIAN_POINT('Ctrl Pts',(3.87881297899995,12.2,0.984312722999987));
#343384=CARTESIAN_POINT('Ctrl Pts',(3.87881297899995,5.2,0.984312722999987));
#343385=CARTESIAN_POINT('Ctrl Pts',(3.87881297899995,2.2,0.984312722999987));
#343386=CARTESIAN_POINT('Ctrl Pts',(3.87913549099994,12.2,0.984416982999985));
#343387=CARTESIAN_POINT('Ctrl Pts',(3.87913549099994,5.2,0.984416982999985));
#343388=CARTESIAN_POINT('Ctrl Pts',(3.87913549099994,2.2,0.984416982999985));
#343389=CARTESIAN_POINT('Ctrl Pts',(3.87946425799994,12.2,0.984523744999986));
#343390=CARTESIAN_POINT('Ctrl Pts',(3.87946425799994,5.2,0.984523744999986));
#343391=CARTESIAN_POINT('Ctrl Pts',(3.87946425799994,2.2,0.984523744999986));
#343392=CARTESIAN_POINT('Ctrl Pts',(3.87979925899994,12.2,0.984633019999985));
#343393=CARTESIAN_POINT('Ctrl Pts',(3.87979925899994,5.2,0.984633019999985));
#343394=CARTESIAN_POINT('Ctrl Pts',(3.87979925899994,2.2,0.984633019999985));
#343395=CARTESIAN_POINT('Ctrl Pts',(3.88014047599994,12.2,0.984744821999985));
#343396=CARTESIAN_POINT('Ctrl Pts',(3.88014047599994,5.2,0.984744821999985));
#343397=CARTESIAN_POINT('Ctrl Pts',(3.88014047599994,2.2,0.984744821999985));
#343398=CARTESIAN_POINT('Ctrl Pts',(3.88048788899995,12.2,0.984859158999987));
#343399=CARTESIAN_POINT('Ctrl Pts',(3.88048788899995,5.2,0.984859158999987));
#343400=CARTESIAN_POINT('Ctrl Pts',(3.88048788899995,2.2,0.984859158999987));
#343401=CARTESIAN_POINT('Ctrl Pts',(3.88084147899994,12.2,0.984976046999986));
#343402=CARTESIAN_POINT('Ctrl Pts',(3.88084147899994,5.2,0.984976046999986));
#343403=CARTESIAN_POINT('Ctrl Pts',(3.88084147899994,2.2,0.984976046999986));
#343404=CARTESIAN_POINT('Ctrl Pts',(3.88120122599994,12.2,0.985095495999988));
#343405=CARTESIAN_POINT('Ctrl Pts',(3.88120122599994,5.2,0.985095495999988));
#343406=CARTESIAN_POINT('Ctrl Pts',(3.88120122599994,2.2,0.985095495999988));
#343407=CARTESIAN_POINT('Ctrl Pts',(3.88156711199994,12.2,0.985217516999985));
#343408=CARTESIAN_POINT('Ctrl Pts',(3.88156711199994,5.2,0.985217516999985));
#343409=CARTESIAN_POINT('Ctrl Pts',(3.88156711199994,2.2,0.985217516999985));
#343410=CARTESIAN_POINT('Ctrl Pts',(3.88193911799994,12.2,0.985342121999988));
#343411=CARTESIAN_POINT('Ctrl Pts',(3.88193911799994,5.2,0.985342121999988));
#343412=CARTESIAN_POINT('Ctrl Pts',(3.88193911799994,2.2,0.985342121999988));
#343413=CARTESIAN_POINT('Ctrl Pts',(3.88231722399994,12.2,0.985469323999983));
#343414=CARTESIAN_POINT('Ctrl Pts',(3.88231722399994,5.2,0.985469323999983));
#343415=CARTESIAN_POINT('Ctrl Pts',(3.88231722399994,2.2,0.985469323999983));
#343416=CARTESIAN_POINT('Ctrl Pts',(3.88270141199994,12.2,0.985599131999986));
#343417=CARTESIAN_POINT('Ctrl Pts',(3.88270141199994,5.2,0.985599131999986));
#343418=CARTESIAN_POINT('Ctrl Pts',(3.88270141199994,2.2,0.985599131999986));
#343419=CARTESIAN_POINT('Ctrl Pts',(3.88309166199994,12.2,0.985731559999987));
#343420=CARTESIAN_POINT('Ctrl Pts',(3.88309166199994,5.2,0.985731559999987));
#343421=CARTESIAN_POINT('Ctrl Pts',(3.88309166199994,2.2,0.985731559999987));
#343422=CARTESIAN_POINT('Ctrl Pts',(3.88348795599994,12.2,0.985866618999989));
#343423=CARTESIAN_POINT('Ctrl Pts',(3.88348795599994,5.2,0.985866618999989));
#343424=CARTESIAN_POINT('Ctrl Pts',(3.88348795599994,2.2,0.985866618999989));
#343425=CARTESIAN_POINT('Ctrl Pts',(3.88389027299994,12.2,0.986004317999987));
#343426=CARTESIAN_POINT('Ctrl Pts',(3.88389027299994,5.2,0.986004317999987));
#343427=CARTESIAN_POINT('Ctrl Pts',(3.88389027299994,2.2,0.986004317999987));
#343428=CARTESIAN_POINT('Ctrl Pts',(3.88429859799994,12.2,0.986144669999987));
#343429=CARTESIAN_POINT('Ctrl Pts',(3.88429859799994,5.2,0.986144669999987));
#343430=CARTESIAN_POINT('Ctrl Pts',(3.88429859799994,2.2,0.986144669999987));
#343431=CARTESIAN_POINT('Ctrl Pts',(3.88471290899994,12.2,0.986287686999985));
#343432=CARTESIAN_POINT('Ctrl Pts',(3.88471290899994,5.2,0.986287686999985));
#343433=CARTESIAN_POINT('Ctrl Pts',(3.88471290899994,2.2,0.986287686999985));
#343434=CARTESIAN_POINT('Ctrl Pts',(3.88513318999994,12.2,0.986433378999987));
#343435=CARTESIAN_POINT('Ctrl Pts',(3.88513318999994,5.2,0.986433378999987));
#343436=CARTESIAN_POINT('Ctrl Pts',(3.88513318999994,2.2,0.986433378999987));
#343437=CARTESIAN_POINT('Ctrl Pts',(3.88555942099994,12.2,0.986581756999985));
#343438=CARTESIAN_POINT('Ctrl Pts',(3.88555942099994,5.2,0.986581756999985));
#343439=CARTESIAN_POINT('Ctrl Pts',(3.88555942099994,2.2,0.986581756999985));
#343440=CARTESIAN_POINT('Ctrl Pts',(3.88599158099994,12.2,0.986732831999984));
#343441=CARTESIAN_POINT('Ctrl Pts',(3.88599158099994,5.2,0.986732831999984));
#343442=CARTESIAN_POINT('Ctrl Pts',(3.88599158099994,2.2,0.986732831999984));
#343443=CARTESIAN_POINT('Ctrl Pts',(3.88642965499994,12.2,0.986886615999989));
#343444=CARTESIAN_POINT('Ctrl Pts',(3.88642965499994,5.2,0.986886615999989));
#343445=CARTESIAN_POINT('Ctrl Pts',(3.88642965499994,2.2,0.986886615999989));
#343446=CARTESIAN_POINT('Ctrl Pts',(3.88687362299994,12.2,0.987043119999989));
#343447=CARTESIAN_POINT('Ctrl Pts',(3.88687362299994,5.2,0.987043119999989));
#343448=CARTESIAN_POINT('Ctrl Pts',(3.88687362299994,2.2,0.987043119999989));
#343449=CARTESIAN_POINT('Ctrl Pts',(3.88732346699994,12.2,0.987202352999983));
#343450=CARTESIAN_POINT('Ctrl Pts',(3.88732346699994,5.2,0.987202352999983));
#343451=CARTESIAN_POINT('Ctrl Pts',(3.88732346699994,2.2,0.987202352999983));
#343452=CARTESIAN_POINT('Ctrl Pts',(3.88777916899994,12.2,0.987364327999987));
#343453=CARTESIAN_POINT('Ctrl Pts',(3.88777916899994,5.2,0.987364327999987));
#343454=CARTESIAN_POINT('Ctrl Pts',(3.88777916899994,2.2,0.987364327999987));
#343455=CARTESIAN_POINT('Ctrl Pts',(3.88824070799994,12.2,0.987529053999987));
#343456=CARTESIAN_POINT('Ctrl Pts',(3.88824070799994,5.2,0.987529053999987));
#343457=CARTESIAN_POINT('Ctrl Pts',(3.88824070799994,2.2,0.987529053999987));
#343458=CARTESIAN_POINT('Ctrl Pts',(3.88870806899994,12.2,0.987696542999985));
#343459=CARTESIAN_POINT('Ctrl Pts',(3.88870806899994,5.2,0.987696542999985));
#343460=CARTESIAN_POINT('Ctrl Pts',(3.88870806899994,2.2,0.987696542999985));
#343461=CARTESIAN_POINT('Ctrl Pts',(3.88918123199994,12.2,0.987866804999986));
#343462=CARTESIAN_POINT('Ctrl Pts',(3.88918123199994,5.2,0.987866804999986));
#343463=CARTESIAN_POINT('Ctrl Pts',(3.88918123199994,2.2,0.987866804999986));
#343464=CARTESIAN_POINT('Ctrl Pts',(3.88966017899994,12.2,0.988039850999982));
#343465=CARTESIAN_POINT('Ctrl Pts',(3.88966017899994,5.2,0.988039850999982));
#343466=CARTESIAN_POINT('Ctrl Pts',(3.88966017899994,2.2,0.988039850999982));
#343467=CARTESIAN_POINT('Ctrl Pts',(3.89014489099994,12.2,0.988215690999983));
#343468=CARTESIAN_POINT('Ctrl Pts',(3.89014489099994,5.2,0.988215690999983));
#343469=CARTESIAN_POINT('Ctrl Pts',(3.89014489099994,2.2,0.988215690999983));
#343470=CARTESIAN_POINT('Ctrl Pts',(3.89063535099994,12.2,0.988394335999985));
#343471=CARTESIAN_POINT('Ctrl Pts',(3.89063535099994,5.2,0.988394335999985));
#343472=CARTESIAN_POINT('Ctrl Pts',(3.89063535099994,2.2,0.988394335999985));
#343473=CARTESIAN_POINT('Ctrl Pts',(3.89113154099994,12.2,0.988575795999989));
#343474=CARTESIAN_POINT('Ctrl Pts',(3.89113154099994,5.2,0.988575795999989));
#343475=CARTESIAN_POINT('Ctrl Pts',(3.89113154099994,2.2,0.988575795999989));
#343476=CARTESIAN_POINT('Ctrl Pts',(3.89163344299994,12.2,0.988760082999987));
#343477=CARTESIAN_POINT('Ctrl Pts',(3.89163344299994,5.2,0.988760082999987));
#343478=CARTESIAN_POINT('Ctrl Pts',(3.89163344299994,2.2,0.988760082999987));
#343479=CARTESIAN_POINT('Ctrl Pts',(3.89214103699994,12.2,0.988947204999988));
#343480=CARTESIAN_POINT('Ctrl Pts',(3.89214103699994,5.2,0.988947204999988));
#343481=CARTESIAN_POINT('Ctrl Pts',(3.89214103699994,2.2,0.988947204999988));
#343482=CARTESIAN_POINT('Ctrl Pts',(3.89265430699994,12.2,0.989137172999985));
#343483=CARTESIAN_POINT('Ctrl Pts',(3.89265430699994,5.2,0.989137172999985));
#343484=CARTESIAN_POINT('Ctrl Pts',(3.89265430699994,2.2,0.989137172999985));
#343485=CARTESIAN_POINT('Ctrl Pts',(3.89317323499994,12.2,0.989329997999988));
#343486=CARTESIAN_POINT('Ctrl Pts',(3.89317323499994,5.2,0.989329997999988));
#343487=CARTESIAN_POINT('Ctrl Pts',(3.89317323499994,2.2,0.989329997999988));
#343488=CARTESIAN_POINT('Ctrl Pts',(3.89369780199994,12.2,0.989525688999984));
#343489=CARTESIAN_POINT('Ctrl Pts',(3.89369780199994,5.2,0.989525688999984));
#343490=CARTESIAN_POINT('Ctrl Pts',(3.89369780199994,2.2,0.989525688999984));
#343491=CARTESIAN_POINT('Ctrl Pts',(3.89422799099994,12.2,0.989724256999986));
#343492=CARTESIAN_POINT('Ctrl Pts',(3.89422799099994,5.2,0.989724256999986));
#343493=CARTESIAN_POINT('Ctrl Pts',(3.89422799099994,2.2,0.989724256999986));
#343494=CARTESIAN_POINT('Ctrl Pts',(3.89476378299995,12.2,0.989925711999984));
#343495=CARTESIAN_POINT('Ctrl Pts',(3.89476378299995,5.2,0.989925711999984));
#343496=CARTESIAN_POINT('Ctrl Pts',(3.89476378299995,2.2,0.989925711999984));
#343497=CARTESIAN_POINT('Ctrl Pts',(3.89530516299994,12.2,0.990130063999985));
#343498=CARTESIAN_POINT('Ctrl Pts',(3.89530516299994,5.2,0.990130063999985));
#343499=CARTESIAN_POINT('Ctrl Pts',(3.89530516299994,2.2,0.990130063999985));
#343500=CARTESIAN_POINT('Ctrl Pts',(3.89585210999994,12.2,0.990337322999988));
#343501=CARTESIAN_POINT('Ctrl Pts',(3.89585210999994,5.2,0.990337322999988));
#343502=CARTESIAN_POINT('Ctrl Pts',(3.89585210999994,2.2,0.990337322999988));
#343503=CARTESIAN_POINT('Ctrl Pts',(3.89640460899995,12.2,0.990547498999987));
#343504=CARTESIAN_POINT('Ctrl Pts',(3.89640460899995,5.2,0.990547498999987));
#343505=CARTESIAN_POINT('Ctrl Pts',(3.89640460899995,2.2,0.990547498999987));
#343506=CARTESIAN_POINT('Ctrl Pts',(3.89696263999994,12.2,0.990760599999985));
#343507=CARTESIAN_POINT('Ctrl Pts',(3.89696263999994,5.2,0.990760599999985));
#343508=CARTESIAN_POINT('Ctrl Pts',(3.89696263999994,2.2,0.990760599999985));
#343509=CARTESIAN_POINT('Ctrl Pts',(3.89752618599994,12.2,0.990976638999985));
#343510=CARTESIAN_POINT('Ctrl Pts',(3.89752618599994,5.2,0.990976638999985));
#343511=CARTESIAN_POINT('Ctrl Pts',(3.89752618599994,2.2,0.990976638999985));
#343512=CARTESIAN_POINT('Ctrl Pts',(3.89809523199994,12.2,0.991195624999985));
#343513=CARTESIAN_POINT('Ctrl Pts',(3.89809523199994,5.2,0.991195624999985));
#343514=CARTESIAN_POINT('Ctrl Pts',(3.89809523199994,2.2,0.991195624999985));
#343515=CARTESIAN_POINT('Ctrl Pts',(3.89866975699994,12.2,0.991417564999986));
#343516=CARTESIAN_POINT('Ctrl Pts',(3.89866975699994,5.2,0.991417564999986));
#343517=CARTESIAN_POINT('Ctrl Pts',(3.89866975699994,2.2,0.991417564999986));
#343518=CARTESIAN_POINT('Ctrl Pts',(3.89924974499994,12.2,0.991642471999987));
#343519=CARTESIAN_POINT('Ctrl Pts',(3.89924974499994,5.2,0.991642471999987));
#343520=CARTESIAN_POINT('Ctrl Pts',(3.89924974499994,2.2,0.991642471999987));
#343521=CARTESIAN_POINT('Ctrl Pts',(3.89983517799994,12.2,0.991870353999986));
#343522=CARTESIAN_POINT('Ctrl Pts',(3.89983517799994,5.2,0.991870353999986));
#343523=CARTESIAN_POINT('Ctrl Pts',(3.89983517799994,2.2,0.991870353999986));
#343524=CARTESIAN_POINT('Ctrl Pts',(3.90042604099994,12.2,0.992101219999988));
#343525=CARTESIAN_POINT('Ctrl Pts',(3.90042604099994,5.2,0.992101219999988));
#343526=CARTESIAN_POINT('Ctrl Pts',(3.90042604099994,2.2,0.992101219999988));
#343527=CARTESIAN_POINT('Ctrl Pts',(3.90102231199994,12.2,0.992335080999984));
#343528=CARTESIAN_POINT('Ctrl Pts',(3.90102231199994,5.2,0.992335080999984));
#343529=CARTESIAN_POINT('Ctrl Pts',(3.90102231199994,2.2,0.992335080999984));
#343530=CARTESIAN_POINT('Ctrl Pts',(3.90162397899994,12.2,0.992571945999985));
#343531=CARTESIAN_POINT('Ctrl Pts',(3.90162397899994,5.2,0.992571945999985));
#343532=CARTESIAN_POINT('Ctrl Pts',(3.90162397899994,2.2,0.992571945999985));
#343533=CARTESIAN_POINT('Ctrl Pts',(3.90223102099994,12.2,0.992811823999986));
#343534=CARTESIAN_POINT('Ctrl Pts',(3.90223102099994,5.2,0.992811823999986));
#343535=CARTESIAN_POINT('Ctrl Pts',(3.90223102099994,2.2,0.992811823999986));
#343536=CARTESIAN_POINT('Ctrl Pts',(3.90284342099994,12.2,0.993054724999984));
#343537=CARTESIAN_POINT('Ctrl Pts',(3.90284342099994,5.2,0.993054724999984));
#343538=CARTESIAN_POINT('Ctrl Pts',(3.90284342099994,2.2,0.993054724999984));
#343539=CARTESIAN_POINT('Ctrl Pts',(3.90346116399995,12.2,0.993300655999985));
#343540=CARTESIAN_POINT('Ctrl Pts',(3.90346116399995,5.2,0.993300655999985));
#343541=CARTESIAN_POINT('Ctrl Pts',(3.90346116399995,2.2,0.993300655999985));
#343542=CARTESIAN_POINT('Ctrl Pts',(3.90408422999994,12.2,0.993549630999984));
#343543=CARTESIAN_POINT('Ctrl Pts',(3.90408422999994,5.2,0.993549630999984));
#343544=CARTESIAN_POINT('Ctrl Pts',(3.90408422999994,2.2,0.993549630999984));
#343545=CARTESIAN_POINT('Ctrl Pts',(3.90471260399994,12.2,0.993801653999986));
#343546=CARTESIAN_POINT('Ctrl Pts',(3.90471260399994,5.2,0.993801653999986));
#343547=CARTESIAN_POINT('Ctrl Pts',(3.90471260399994,2.2,0.993801653999986));
#343548=CARTESIAN_POINT('Ctrl Pts',(3.90534626899994,12.2,0.994056737999984));
#343549=CARTESIAN_POINT('Ctrl Pts',(3.90534626899994,5.2,0.994056737999984));
#343550=CARTESIAN_POINT('Ctrl Pts',(3.90534626899994,2.2,0.994056737999984));
#343551=CARTESIAN_POINT('Ctrl Pts',(3.90598520699994,12.2,0.994314889999988));
#343552=CARTESIAN_POINT('Ctrl Pts',(3.90598520699994,5.2,0.994314889999988));
#343553=CARTESIAN_POINT('Ctrl Pts',(3.90598520699994,2.2,0.994314889999988));
#343554=CARTESIAN_POINT('Ctrl Pts',(3.90662940099994,12.2,0.994576120999984));
#343555=CARTESIAN_POINT('Ctrl Pts',(3.90662940099994,5.2,0.994576120999984));
#343556=CARTESIAN_POINT('Ctrl Pts',(3.90662940099994,2.2,0.994576120999984));
#343557=CARTESIAN_POINT('Ctrl Pts',(3.90727883399994,12.2,0.994840437999986));
#343558=CARTESIAN_POINT('Ctrl Pts',(3.90727883399994,5.2,0.994840437999986));
#343559=CARTESIAN_POINT('Ctrl Pts',(3.90727883399994,2.2,0.994840437999986));
#343560=CARTESIAN_POINT('Ctrl Pts',(3.90793348999994,12.2,0.995107849999983));
#343561=CARTESIAN_POINT('Ctrl Pts',(3.90793348999994,5.2,0.995107849999983));
#343562=CARTESIAN_POINT('Ctrl Pts',(3.90793348999994,2.2,0.995107849999983));
#343563=CARTESIAN_POINT('Ctrl Pts',(3.90859335099994,12.2,0.995378367999984));
#343564=CARTESIAN_POINT('Ctrl Pts',(3.90859335099994,5.2,0.995378367999984));
#343565=CARTESIAN_POINT('Ctrl Pts',(3.90859335099994,2.2,0.995378367999984));
#343566=CARTESIAN_POINT('Ctrl Pts',(3.90925840099994,12.2,0.995651999999985));
#343567=CARTESIAN_POINT('Ctrl Pts',(3.90925840099994,5.2,0.995651999999985));
#343568=CARTESIAN_POINT('Ctrl Pts',(3.90925840099994,2.2,0.995651999999985));
#343569=CARTESIAN_POINT('Ctrl Pts',(3.90992862199994,12.2,0.995928753999986));
#343570=CARTESIAN_POINT('Ctrl Pts',(3.90992862199994,5.2,0.995928753999986));
#343571=CARTESIAN_POINT('Ctrl Pts',(3.90992862199994,2.2,0.995928753999986));
#343572=CARTESIAN_POINT('Ctrl Pts',(3.91060399799994,12.2,0.996208638999985));
#343573=CARTESIAN_POINT('Ctrl Pts',(3.91060399799994,5.2,0.996208638999985));
#343574=CARTESIAN_POINT('Ctrl Pts',(3.91060399799994,2.2,0.996208638999985));
#343575=CARTESIAN_POINT('Ctrl Pts',(3.91128451199994,12.2,0.996491665999986));
#343576=CARTESIAN_POINT('Ctrl Pts',(3.91128451199994,5.2,0.996491665999986));
#343577=CARTESIAN_POINT('Ctrl Pts',(3.91128451199994,2.2,0.996491665999986));
#343578=CARTESIAN_POINT('Ctrl Pts',(3.91197014899994,12.2,0.996777839999985));
#343579=CARTESIAN_POINT('Ctrl Pts',(3.91197014899994,5.2,0.996777839999985));
#343580=CARTESIAN_POINT('Ctrl Pts',(3.91197014899994,2.2,0.996777839999985));
#343581=CARTESIAN_POINT('Ctrl Pts',(3.91266088899994,12.2,0.997067171999984));
#343582=CARTESIAN_POINT('Ctrl Pts',(3.91266088899994,5.2,0.997067171999984));
#343583=CARTESIAN_POINT('Ctrl Pts',(3.91266088899994,2.2,0.997067171999984));
#343584=CARTESIAN_POINT('Ctrl Pts',(3.91335671699994,12.2,0.997359669999986));
#343585=CARTESIAN_POINT('Ctrl Pts',(3.91335671699994,5.2,0.997359669999986));
#343586=CARTESIAN_POINT('Ctrl Pts',(3.91335671699994,2.2,0.997359669999986));
#343587=CARTESIAN_POINT('Ctrl Pts',(3.91405761799994,12.2,0.997655342999986));
#343588=CARTESIAN_POINT('Ctrl Pts',(3.91405761799994,5.2,0.997655342999986));
#343589=CARTESIAN_POINT('Ctrl Pts',(3.91405761799994,2.2,0.997655342999986));
#343590=CARTESIAN_POINT('Ctrl Pts',(3.91476357299994,12.2,0.997954198999986));
#343591=CARTESIAN_POINT('Ctrl Pts',(3.91476357299994,5.2,0.997954198999986));
#343592=CARTESIAN_POINT('Ctrl Pts',(3.91476357299994,2.2,0.997954198999986));
#343593=CARTESIAN_POINT('Ctrl Pts',(3.91547456599994,12.2,0.998256247999985));
#343594=CARTESIAN_POINT('Ctrl Pts',(3.91547456599994,5.2,0.998256247999985));
#343595=CARTESIAN_POINT('Ctrl Pts',(3.91547456599994,2.2,0.998256247999985));
#343596=CARTESIAN_POINT('Ctrl Pts',(3.91619058299994,12.2,0.998561495999986));
#343597=CARTESIAN_POINT('Ctrl Pts',(3.91619058299994,5.2,0.998561495999986));
#343598=CARTESIAN_POINT('Ctrl Pts',(3.91619058299994,2.2,0.998561495999986));
#343599=CARTESIAN_POINT('Ctrl Pts',(3.91691160399994,12.2,0.998869953999986));
#343600=CARTESIAN_POINT('Ctrl Pts',(3.91691160399994,5.2,0.998869953999986));
#343601=CARTESIAN_POINT('Ctrl Pts',(3.91691160399994,2.2,0.998869953999986));
#343602=CARTESIAN_POINT('Ctrl Pts',(3.91763761399994,12.2,0.999181626999985));
#343603=CARTESIAN_POINT('Ctrl Pts',(3.91763761399994,5.2,0.999181626999985));
#343604=CARTESIAN_POINT('Ctrl Pts',(3.91763761399994,2.2,0.999181626999985));
#343605=CARTESIAN_POINT('Ctrl Pts',(3.91836859699994,12.2,0.999496526999986));
#343606=CARTESIAN_POINT('Ctrl Pts',(3.91836859699994,5.2,0.999496526999986));
#343607=CARTESIAN_POINT('Ctrl Pts',(3.91836859699994,2.2,0.999496526999986));
#343608=CARTESIAN_POINT('Ctrl Pts',(3.91910453599994,12.2,0.999814659999987));
#343609=CARTESIAN_POINT('Ctrl Pts',(3.91910453599994,5.2,0.999814659999987));
#343610=CARTESIAN_POINT('Ctrl Pts',(3.91910453599994,2.2,0.999814659999987));
#343611=CARTESIAN_POINT('Ctrl Pts',(3.91984541599994,12.2,1.00013603499999));
#343612=CARTESIAN_POINT('Ctrl Pts',(3.91984541599994,5.2,1.00013603499999));
#343613=CARTESIAN_POINT('Ctrl Pts',(3.91984541599994,2.2,1.00013603499999));
#343614=CARTESIAN_POINT('Ctrl Pts',(3.92059121899994,12.2,1.00046065999999));
#343615=CARTESIAN_POINT('Ctrl Pts',(3.92059121899994,5.2,1.00046065999999));
#343616=CARTESIAN_POINT('Ctrl Pts',(3.92059121899994,2.2,1.00046065999999));
#343617=CARTESIAN_POINT('Ctrl Pts',(3.92134192799994,12.2,1.00078854399999));
#343618=CARTESIAN_POINT('Ctrl Pts',(3.92134192799994,5.2,1.00078854399999));
#343619=CARTESIAN_POINT('Ctrl Pts',(3.92134192799994,2.2,1.00078854399999));
#343620=CARTESIAN_POINT('Ctrl Pts',(3.92209752999995,12.2,1.00111969399999));
#343621=CARTESIAN_POINT('Ctrl Pts',(3.92209752999995,5.2,1.00111969399999));
#343622=CARTESIAN_POINT('Ctrl Pts',(3.92209752999995,2.2,1.00111969399999));
#343623=CARTESIAN_POINT('Ctrl Pts',(3.92285800599994,12.2,1.00145411799998));
#343624=CARTESIAN_POINT('Ctrl Pts',(3.92285800599994,5.2,1.00145411799998));
#343625=CARTESIAN_POINT('Ctrl Pts',(3.92285800599994,2.2,1.00145411799998));
#343626=CARTESIAN_POINT('Ctrl Pts',(3.92362334199994,12.2,1.00179182499998));
#343627=CARTESIAN_POINT('Ctrl Pts',(3.92362334199994,5.2,1.00179182499998));
#343628=CARTESIAN_POINT('Ctrl Pts',(3.92362334199994,2.2,1.00179182499998));
#343629=CARTESIAN_POINT('Ctrl Pts',(3.92439352099994,12.2,1.00213282199999));
#343630=CARTESIAN_POINT('Ctrl Pts',(3.92439352099994,5.2,1.00213282199999));
#343631=CARTESIAN_POINT('Ctrl Pts',(3.92439352099994,2.2,1.00213282199999));
#343632=CARTESIAN_POINT('Ctrl Pts',(3.92516852499994,12.2,1.00247711799998));
#343633=CARTESIAN_POINT('Ctrl Pts',(3.92516852499994,5.2,1.00247711799998));
#343634=CARTESIAN_POINT('Ctrl Pts',(3.92516852499994,2.2,1.00247711799998));
#343635=CARTESIAN_POINT('Ctrl Pts',(3.92594834099994,12.2,1.00282471899999));
#343636=CARTESIAN_POINT('Ctrl Pts',(3.92594834099994,5.2,1.00282471899999));
#343637=CARTESIAN_POINT('Ctrl Pts',(3.92594834099994,2.2,1.00282471899999));
#343638=CARTESIAN_POINT('Ctrl Pts',(3.92673295199994,12.2,1.00317563499999));
#343639=CARTESIAN_POINT('Ctrl Pts',(3.92673295199994,5.2,1.00317563499999));
#343640=CARTESIAN_POINT('Ctrl Pts',(3.92673295199994,2.2,1.00317563499999));
#343641=CARTESIAN_POINT('Ctrl Pts',(3.92752233999994,12.2,1.00352987299999));
#343642=CARTESIAN_POINT('Ctrl Pts',(3.92752233999994,5.2,1.00352987299999));
#343643=CARTESIAN_POINT('Ctrl Pts',(3.92752233999994,2.2,1.00352987299999));
#343644=CARTESIAN_POINT('Ctrl Pts',(3.92831649199994,12.2,1.00388744099998));
#343645=CARTESIAN_POINT('Ctrl Pts',(3.92831649199994,5.2,1.00388744099998));
#343646=CARTESIAN_POINT('Ctrl Pts',(3.92831649199994,2.2,1.00388744099998));
#343647=CARTESIAN_POINT('Ctrl Pts',(3.92911538899994,12.2,1.00424834599998));
#343648=CARTESIAN_POINT('Ctrl Pts',(3.92911538899994,5.2,1.00424834599998));
#343649=CARTESIAN_POINT('Ctrl Pts',(3.92911538899994,2.2,1.00424834599998));
#343650=CARTESIAN_POINT('Ctrl Pts',(3.92991901899994,12.2,1.00461259699999));
#343651=CARTESIAN_POINT('Ctrl Pts',(3.92991901899994,5.2,1.00461259699999));
#343652=CARTESIAN_POINT('Ctrl Pts',(3.92991901899994,2.2,1.00461259699999));
#343653=CARTESIAN_POINT('Ctrl Pts',(3.93072736299994,12.2,1.00498019899999));
#343654=CARTESIAN_POINT('Ctrl Pts',(3.93072736299994,5.2,1.00498019899999));
#343655=CARTESIAN_POINT('Ctrl Pts',(3.93072736299994,2.2,1.00498019899999));
#343656=CARTESIAN_POINT('Ctrl Pts',(3.93154040599994,12.2,1.00535116299998));
#343657=CARTESIAN_POINT('Ctrl Pts',(3.93154040599994,5.2,1.00535116299998));
#343658=CARTESIAN_POINT('Ctrl Pts',(3.93154040599994,2.2,1.00535116299998));
#343659=CARTESIAN_POINT('Ctrl Pts',(3.93235813299994,12.2,1.00572549499998));
#343660=CARTESIAN_POINT('Ctrl Pts',(3.93235813299994,5.2,1.00572549499998));
#343661=CARTESIAN_POINT('Ctrl Pts',(3.93235813299994,2.2,1.00572549499998));
#343662=CARTESIAN_POINT('Ctrl Pts',(3.93318052799994,12.2,1.00610320199999));
#343663=CARTESIAN_POINT('Ctrl Pts',(3.93318052799994,5.2,1.00610320199999));
#343664=CARTESIAN_POINT('Ctrl Pts',(3.93318052799994,2.2,1.00610320199999));
#343665=CARTESIAN_POINT('Ctrl Pts',(3.93400757499994,12.2,1.00648429199999));
#343666=CARTESIAN_POINT('Ctrl Pts',(3.93400757499994,5.2,1.00648429199999));
#343667=CARTESIAN_POINT('Ctrl Pts',(3.93400757499994,2.2,1.00648429199999));
#343668=CARTESIAN_POINT('Ctrl Pts',(3.93483925699994,12.2,1.00686877299998));
#343669=CARTESIAN_POINT('Ctrl Pts',(3.93483925699994,5.2,1.00686877299998));
#343670=CARTESIAN_POINT('Ctrl Pts',(3.93483925699994,2.2,1.00686877299998));
#343671=CARTESIAN_POINT('Ctrl Pts',(3.93567556099994,12.2,1.00725665199999));
#343672=CARTESIAN_POINT('Ctrl Pts',(3.93567556099994,5.2,1.00725665199999));
#343673=CARTESIAN_POINT('Ctrl Pts',(3.93567556099994,2.2,1.00725665199999));
#343674=CARTESIAN_POINT('Ctrl Pts',(3.93651646899994,12.2,1.00764793699998));
#343675=CARTESIAN_POINT('Ctrl Pts',(3.93651646899994,5.2,1.00764793699998));
#343676=CARTESIAN_POINT('Ctrl Pts',(3.93651646899994,2.2,1.00764793699998));
#343677=CARTESIAN_POINT('Ctrl Pts',(3.93736196599995,12.2,1.00804263299999));
#343678=CARTESIAN_POINT('Ctrl Pts',(3.93736196599995,5.2,1.00804263299999));
#343679=CARTESIAN_POINT('Ctrl Pts',(3.93736196599995,2.2,1.00804263299999));
#343680=CARTESIAN_POINT('Ctrl Pts',(3.93821203799994,12.2,1.00844074999999));
#343681=CARTESIAN_POINT('Ctrl Pts',(3.93821203799994,5.2,1.00844074999999));
#343682=CARTESIAN_POINT('Ctrl Pts',(3.93821203799994,2.2,1.00844074999999));
#343683=CARTESIAN_POINT('Ctrl Pts',(3.93906666699994,12.2,1.00884229399998));
#343684=CARTESIAN_POINT('Ctrl Pts',(3.93906666699994,5.2,1.00884229399998));
#343685=CARTESIAN_POINT('Ctrl Pts',(3.93906666699994,2.2,1.00884229399998));
#343686=CARTESIAN_POINT('Ctrl Pts',(3.93992583999994,12.2,1.00924727299998));
#343687=CARTESIAN_POINT('Ctrl Pts',(3.93992583999994,5.2,1.00924727299998));
#343688=CARTESIAN_POINT('Ctrl Pts',(3.93992583999994,2.2,1.00924727299998));
#343689=CARTESIAN_POINT('Ctrl Pts',(3.94078953999994,12.2,1.00965569399999));
#343690=CARTESIAN_POINT('Ctrl Pts',(3.94078953999994,5.2,1.00965569399999));
#343691=CARTESIAN_POINT('Ctrl Pts',(3.94078953999994,2.2,1.00965569399999));
#343692=CARTESIAN_POINT('Ctrl Pts',(3.94165775099994,12.2,1.01006756199999));
#343693=CARTESIAN_POINT('Ctrl Pts',(3.94165775099994,5.2,1.01006756199999));
#343694=CARTESIAN_POINT('Ctrl Pts',(3.94165775099994,2.2,1.01006756199999));
#343695=CARTESIAN_POINT('Ctrl Pts',(3.94253045899994,12.2,1.01048288799999));
#343696=CARTESIAN_POINT('Ctrl Pts',(3.94253045899994,5.2,1.01048288799999));
#343697=CARTESIAN_POINT('Ctrl Pts',(3.94253045899994,2.2,1.01048288799999));
#343698=CARTESIAN_POINT('Ctrl Pts',(3.94340764899995,12.2,1.01090167499999));
#343699=CARTESIAN_POINT('Ctrl Pts',(3.94340764899995,5.2,1.01090167499999));
#343700=CARTESIAN_POINT('Ctrl Pts',(3.94340764899995,2.2,1.01090167499999));
#343701=CARTESIAN_POINT('Ctrl Pts',(3.94428930299994,12.2,1.01132393399999));
#343702=CARTESIAN_POINT('Ctrl Pts',(3.94428930299994,5.2,1.01132393399999));
#343703=CARTESIAN_POINT('Ctrl Pts',(3.94428930299994,2.2,1.01132393399999));
#343704=CARTESIAN_POINT('Ctrl Pts',(3.94517540899994,12.2,1.01174966899999));
#343705=CARTESIAN_POINT('Ctrl Pts',(3.94517540899994,5.2,1.01174966899999));
#343706=CARTESIAN_POINT('Ctrl Pts',(3.94517540899994,2.2,1.01174966899999));
#343707=CARTESIAN_POINT('Ctrl Pts',(3.94606594899995,12.2,1.01217888899999));
#343708=CARTESIAN_POINT('Ctrl Pts',(3.94606594899995,5.2,1.01217888899999));
#343709=CARTESIAN_POINT('Ctrl Pts',(3.94606594899995,2.2,1.01217888899999));
#343710=CARTESIAN_POINT('Ctrl Pts',(3.94696090899994,12.2,1.01261159899999));
#343711=CARTESIAN_POINT('Ctrl Pts',(3.94696090899994,5.2,1.01261159899999));
#343712=CARTESIAN_POINT('Ctrl Pts',(3.94696090899994,2.2,1.01261159899999));
#343713=CARTESIAN_POINT('Ctrl Pts',(3.94786027299994,12.2,1.01304780699999));
#343714=CARTESIAN_POINT('Ctrl Pts',(3.94786027299994,5.2,1.01304780699999));
#343715=CARTESIAN_POINT('Ctrl Pts',(3.94786027299994,2.2,1.01304780699999));
#343716=CARTESIAN_POINT('Ctrl Pts',(3.94876402799994,12.2,1.01348751999998));
#343717=CARTESIAN_POINT('Ctrl Pts',(3.94876402799994,5.2,1.01348751999998));
#343718=CARTESIAN_POINT('Ctrl Pts',(3.94876402799994,2.2,1.01348751999998));
#343719=CARTESIAN_POINT('Ctrl Pts',(3.94967215599995,12.2,1.01393074399999));
#343720=CARTESIAN_POINT('Ctrl Pts',(3.94967215599995,5.2,1.01393074399999));
#343721=CARTESIAN_POINT('Ctrl Pts',(3.94967215599995,2.2,1.01393074399999));
#343722=CARTESIAN_POINT('Ctrl Pts',(3.95058464299994,12.2,1.01437748699999));
#343723=CARTESIAN_POINT('Ctrl Pts',(3.95058464299994,5.2,1.01437748699999));
#343724=CARTESIAN_POINT('Ctrl Pts',(3.95058464299994,2.2,1.01437748699999));
#343725=CARTESIAN_POINT('Ctrl Pts',(3.95150147499994,12.2,1.01482775399999));
#343726=CARTESIAN_POINT('Ctrl Pts',(3.95150147499994,5.2,1.01482775399999));
#343727=CARTESIAN_POINT('Ctrl Pts',(3.95150147499994,2.2,1.01482775399999));
#343728=CARTESIAN_POINT('Ctrl Pts',(3.95242263499994,12.2,1.01528155399999));
#343729=CARTESIAN_POINT('Ctrl Pts',(3.95242263499994,5.2,1.01528155399999));
#343730=CARTESIAN_POINT('Ctrl Pts',(3.95242263499994,2.2,1.01528155399999));
#343731=CARTESIAN_POINT('Ctrl Pts',(3.95334810899994,12.2,1.01573889199999));
#343732=CARTESIAN_POINT('Ctrl Pts',(3.95334810899994,5.2,1.01573889199999));
#343733=CARTESIAN_POINT('Ctrl Pts',(3.95334810899994,2.2,1.01573889199999));
#343734=CARTESIAN_POINT('Ctrl Pts',(3.95427788199994,12.2,1.01619977599999));
#343735=CARTESIAN_POINT('Ctrl Pts',(3.95427788199994,5.2,1.01619977599999));
#343736=CARTESIAN_POINT('Ctrl Pts',(3.95427788199994,2.2,1.01619977599999));
#343737=CARTESIAN_POINT('Ctrl Pts',(3.95521193899994,12.2,1.01666420999999));
#343738=CARTESIAN_POINT('Ctrl Pts',(3.95521193899994,5.2,1.01666420999999));
#343739=CARTESIAN_POINT('Ctrl Pts',(3.95521193899994,2.2,1.01666420999999));
#343740=CARTESIAN_POINT('Ctrl Pts',(3.95615026299994,12.2,1.01713220299999));
#343741=CARTESIAN_POINT('Ctrl Pts',(3.95615026299994,5.2,1.01713220299999));
#343742=CARTESIAN_POINT('Ctrl Pts',(3.95615026299994,2.2,1.01713220299999));
#343743=CARTESIAN_POINT('Ctrl Pts',(3.95709284299994,12.2,1.01760375999998));
#343744=CARTESIAN_POINT('Ctrl Pts',(3.95709284299994,5.2,1.01760375999998));
#343745=CARTESIAN_POINT('Ctrl Pts',(3.95709284299994,2.2,1.01760375999998));
#343746=CARTESIAN_POINT('Ctrl Pts',(3.95803966099994,12.2,1.01807888899998));
#343747=CARTESIAN_POINT('Ctrl Pts',(3.95803966099994,5.2,1.01807888899998));
#343748=CARTESIAN_POINT('Ctrl Pts',(3.95803966099994,2.2,1.01807888899998));
#343749=CARTESIAN_POINT('Ctrl Pts',(3.95899070299994,12.2,1.01855759699998));
#343750=CARTESIAN_POINT('Ctrl Pts',(3.95899070299994,5.2,1.01855759699998));
#343751=CARTESIAN_POINT('Ctrl Pts',(3.95899070299994,2.2,1.01855759699998));
#343752=CARTESIAN_POINT('Ctrl Pts',(3.95994595499995,12.2,1.01903988699998));
#343753=CARTESIAN_POINT('Ctrl Pts',(3.95994595499995,5.2,1.01903988699998));
#343754=CARTESIAN_POINT('Ctrl Pts',(3.95994595499995,2.2,1.01903988699998));
#343755=CARTESIAN_POINT('Ctrl Pts',(3.96090540099994,12.2,1.01952576899999));
#343756=CARTESIAN_POINT('Ctrl Pts',(3.96090540099994,5.2,1.01952576899999));
#343757=CARTESIAN_POINT('Ctrl Pts',(3.96090540099994,2.2,1.01952576899999));
#343758=CARTESIAN_POINT('Ctrl Pts',(3.96186902799994,12.2,1.02001524699999));
#343759=CARTESIAN_POINT('Ctrl Pts',(3.96186902799994,5.2,1.02001524699999));
#343760=CARTESIAN_POINT('Ctrl Pts',(3.96186902799994,2.2,1.02001524699999));
#343761=CARTESIAN_POINT('Ctrl Pts',(3.96283681799994,12.2,1.02050832899999));
#343762=CARTESIAN_POINT('Ctrl Pts',(3.96283681799994,5.2,1.02050832899999));
#343763=CARTESIAN_POINT('Ctrl Pts',(3.96283681799994,2.2,1.02050832899999));
#343764=CARTESIAN_POINT('Ctrl Pts',(3.96380875899994,12.2,1.02100501999999));
#343765=CARTESIAN_POINT('Ctrl Pts',(3.96380875899994,5.2,1.02100501999999));
#343766=CARTESIAN_POINT('Ctrl Pts',(3.96380875899994,2.2,1.02100501999999));
#343767=CARTESIAN_POINT('Ctrl Pts',(3.96478483499994,12.2,1.02150532699998));
#343768=CARTESIAN_POINT('Ctrl Pts',(3.96478483499994,5.2,1.02150532699998));
#343769=CARTESIAN_POINT('Ctrl Pts',(3.96478483499994,2.2,1.02150532699998));
#343770=CARTESIAN_POINT('Ctrl Pts',(3.96576503099995,12.2,1.02200925599998));
#343771=CARTESIAN_POINT('Ctrl Pts',(3.96576503099995,5.2,1.02200925599998));
#343772=CARTESIAN_POINT('Ctrl Pts',(3.96576503099995,2.2,1.02200925599998));
#343773=CARTESIAN_POINT('Ctrl Pts',(3.96674933499995,12.2,1.02251681299999));
#343774=CARTESIAN_POINT('Ctrl Pts',(3.96674933499995,5.2,1.02251681299999));
#343775=CARTESIAN_POINT('Ctrl Pts',(3.96674933499995,2.2,1.02251681299999));
#343776=CARTESIAN_POINT('Ctrl Pts',(3.96773772899994,12.2,1.02302800399999));
#343777=CARTESIAN_POINT('Ctrl Pts',(3.96773772899994,5.2,1.02302800399999));
#343778=CARTESIAN_POINT('Ctrl Pts',(3.96773772899994,2.2,1.02302800399999));
#343779=CARTESIAN_POINT('Ctrl Pts',(3.96873019999994,12.2,1.02354283599999));
#343780=CARTESIAN_POINT('Ctrl Pts',(3.96873019999994,5.2,1.02354283599999));
#343781=CARTESIAN_POINT('Ctrl Pts',(3.96873019999994,2.2,1.02354283599999));
#343782=CARTESIAN_POINT('Ctrl Pts',(3.96972673299994,12.2,1.02406131499999));
#343783=CARTESIAN_POINT('Ctrl Pts',(3.96972673299994,5.2,1.02406131499999));
#343784=CARTESIAN_POINT('Ctrl Pts',(3.96972673299994,2.2,1.02406131499999));
#343785=CARTESIAN_POINT('Ctrl Pts',(3.97072731399994,12.2,1.02458344599999));
#343786=CARTESIAN_POINT('Ctrl Pts',(3.97072731399994,5.2,1.02458344599999));
#343787=CARTESIAN_POINT('Ctrl Pts',(3.97072731399994,2.2,1.02458344599999));
#343788=CARTESIAN_POINT('Ctrl Pts',(3.97173192799994,12.2,1.02510923499999));
#343789=CARTESIAN_POINT('Ctrl Pts',(3.97173192799994,5.2,1.02510923499999));
#343790=CARTESIAN_POINT('Ctrl Pts',(3.97173192799994,2.2,1.02510923499999));
#343791=CARTESIAN_POINT('Ctrl Pts',(3.97274056099994,12.2,1.02563868999999));
#343792=CARTESIAN_POINT('Ctrl Pts',(3.97274056099994,5.2,1.02563868999999));
#343793=CARTESIAN_POINT('Ctrl Pts',(3.97274056099994,2.2,1.02563868999999));
#343794=CARTESIAN_POINT('Ctrl Pts',(3.97375319799994,12.2,1.02617181399999));
#343795=CARTESIAN_POINT('Ctrl Pts',(3.97375319799994,5.2,1.02617181399999));
#343796=CARTESIAN_POINT('Ctrl Pts',(3.97375319799994,2.2,1.02617181399999));
#343797=CARTESIAN_POINT('Ctrl Pts',(3.97476982499994,12.2,1.02670861599998));
#343798=CARTESIAN_POINT('Ctrl Pts',(3.97476982499994,5.2,1.02670861599998));
#343799=CARTESIAN_POINT('Ctrl Pts',(3.97476982499994,2.2,1.02670861599998));
#343800=CARTESIAN_POINT('Ctrl Pts',(3.97579042599994,12.2,1.02724909999999));
#343801=CARTESIAN_POINT('Ctrl Pts',(3.97579042599994,5.2,1.02724909999999));
#343802=CARTESIAN_POINT('Ctrl Pts',(3.97579042599994,2.2,1.02724909999999));
#343803=CARTESIAN_POINT('Ctrl Pts',(3.97681498899995,12.2,1.02779327199999));
#343804=CARTESIAN_POINT('Ctrl Pts',(3.97681498899995,5.2,1.02779327199999));
#343805=CARTESIAN_POINT('Ctrl Pts',(3.97681498899995,2.2,1.02779327199999));
#343806=CARTESIAN_POINT('Ctrl Pts',(3.97784349899994,12.2,1.02834113799998));
#343807=CARTESIAN_POINT('Ctrl Pts',(3.97784349899994,5.2,1.02834113799998));
#343808=CARTESIAN_POINT('Ctrl Pts',(3.97784349899994,2.2,1.02834113799998));
#343809=CARTESIAN_POINT('Ctrl Pts',(3.97887594099994,12.2,1.02889270399999));
#343810=CARTESIAN_POINT('Ctrl Pts',(3.97887594099994,5.2,1.02889270399999));
#343811=CARTESIAN_POINT('Ctrl Pts',(3.97887594099994,2.2,1.02889270399999));
#343812=CARTESIAN_POINT('Ctrl Pts',(3.97991229999994,12.2,1.02944797499998));
#343813=CARTESIAN_POINT('Ctrl Pts',(3.97991229999994,5.2,1.02944797499998));
#343814=CARTESIAN_POINT('Ctrl Pts',(3.97991229999994,2.2,1.02944797499998));
#343815=CARTESIAN_POINT('Ctrl Pts',(3.98095256299994,12.2,1.03000695799999));
#343816=CARTESIAN_POINT('Ctrl Pts',(3.98095256299994,5.2,1.03000695799999));
#343817=CARTESIAN_POINT('Ctrl Pts',(3.98095256299994,2.2,1.03000695799999));
#343818=CARTESIAN_POINT('Ctrl Pts',(3.98199671599994,12.2,1.03056965699999));
#343819=CARTESIAN_POINT('Ctrl Pts',(3.98199671599994,5.2,1.03056965699999));
#343820=CARTESIAN_POINT('Ctrl Pts',(3.98199671599994,2.2,1.03056965699999));
#343821=CARTESIAN_POINT('Ctrl Pts',(3.98304474399994,12.2,1.03113607999999));
#343822=CARTESIAN_POINT('Ctrl Pts',(3.98304474399994,5.2,1.03113607999999));
#343823=CARTESIAN_POINT('Ctrl Pts',(3.98304474399994,2.2,1.03113607999999));
#343824=CARTESIAN_POINT('Ctrl Pts',(3.98409663299994,12.2,1.03170623099999));
#343825=CARTESIAN_POINT('Ctrl Pts',(3.98409663299994,5.2,1.03170623099999));
#343826=CARTESIAN_POINT('Ctrl Pts',(3.98409663299994,2.2,1.03170623099999));
#343827=CARTESIAN_POINT('Ctrl Pts',(3.98515236799994,12.2,1.03228011599999));
#343828=CARTESIAN_POINT('Ctrl Pts',(3.98515236799994,5.2,1.03228011599999));
#343829=CARTESIAN_POINT('Ctrl Pts',(3.98515236799994,2.2,1.03228011599999));
#343830=CARTESIAN_POINT('Ctrl Pts',(3.98621193499994,12.2,1.03285773999998));
#343831=CARTESIAN_POINT('Ctrl Pts',(3.98621193499994,5.2,1.03285773999998));
#343832=CARTESIAN_POINT('Ctrl Pts',(3.98621193499994,2.2,1.03285773999998));
#343833=CARTESIAN_POINT('Ctrl Pts',(3.98727532099994,12.2,1.03343910999998));
#343834=CARTESIAN_POINT('Ctrl Pts',(3.98727532099994,5.2,1.03343910999998));
#343835=CARTESIAN_POINT('Ctrl Pts',(3.98727532099994,2.2,1.03343910999998));
#343836=CARTESIAN_POINT('Ctrl Pts',(3.98834251199994,12.2,1.03402422899999));
#343837=CARTESIAN_POINT('Ctrl Pts',(3.98834251199994,5.2,1.03402422899999));
#343838=CARTESIAN_POINT('Ctrl Pts',(3.98834251199994,2.2,1.03402422899999));
#343839=CARTESIAN_POINT('Ctrl Pts',(3.98941349399994,12.2,1.03461310499998));
#343840=CARTESIAN_POINT('Ctrl Pts',(3.98941349399994,5.2,1.03461310499998));
#343841=CARTESIAN_POINT('Ctrl Pts',(3.98941349399994,2.2,1.03461310499998));
#343842=CARTESIAN_POINT('Ctrl Pts',(3.99048824999995,12.2,1.03520574299999));
#343843=CARTESIAN_POINT('Ctrl Pts',(3.99048824999995,5.2,1.03520574299999));
#343844=CARTESIAN_POINT('Ctrl Pts',(3.99048824999995,2.2,1.03520574299999));
#343845=CARTESIAN_POINT('Ctrl Pts',(3.99156676899994,12.2,1.03580214699999));
#343846=CARTESIAN_POINT('Ctrl Pts',(3.99156676899994,5.2,1.03580214699999));
#343847=CARTESIAN_POINT('Ctrl Pts',(3.99156676899994,2.2,1.03580214699999));
#343848=CARTESIAN_POINT('Ctrl Pts',(3.99264903699994,12.2,1.03640232399998));
#343849=CARTESIAN_POINT('Ctrl Pts',(3.99264903699994,5.2,1.03640232399998));
#343850=CARTESIAN_POINT('Ctrl Pts',(3.99264903699994,2.2,1.03640232399998));
#343851=CARTESIAN_POINT('Ctrl Pts',(3.99373503799994,12.2,1.03700627899999));
#343852=CARTESIAN_POINT('Ctrl Pts',(3.99373503799994,5.2,1.03700627899999));
#343853=CARTESIAN_POINT('Ctrl Pts',(3.99373503799994,2.2,1.03700627899999));
#343854=CARTESIAN_POINT('Ctrl Pts',(3.99482475899994,12.2,1.03761401499999));
#343855=CARTESIAN_POINT('Ctrl Pts',(3.99482475899994,5.2,1.03761401499999));
#343856=CARTESIAN_POINT('Ctrl Pts',(3.99482475899994,2.2,1.03761401499999));
#343857=CARTESIAN_POINT('Ctrl Pts',(3.99591818699994,12.2,1.03822554099999));
#343858=CARTESIAN_POINT('Ctrl Pts',(3.99591818699994,5.2,1.03822554099999));
#343859=CARTESIAN_POINT('Ctrl Pts',(3.99591818699994,2.2,1.03822554099999));
#343860=CARTESIAN_POINT('Ctrl Pts',(3.99701530699994,12.2,1.03884085899999));
#343861=CARTESIAN_POINT('Ctrl Pts',(3.99701530699994,5.2,1.03884085899999));
#343862=CARTESIAN_POINT('Ctrl Pts',(3.99701530699994,2.2,1.03884085899999));
#343863=CARTESIAN_POINT('Ctrl Pts',(3.99811610699994,12.2,1.03945997699999));
#343864=CARTESIAN_POINT('Ctrl Pts',(3.99811610699994,5.2,1.03945997699999));
#343865=CARTESIAN_POINT('Ctrl Pts',(3.99811610699994,2.2,1.03945997699999));
#343866=CARTESIAN_POINT('Ctrl Pts',(3.99922056899995,12.2,1.04008289899999));
#343867=CARTESIAN_POINT('Ctrl Pts',(3.99922056899995,5.2,1.04008289899999));
#343868=CARTESIAN_POINT('Ctrl Pts',(3.99922056899995,2.2,1.04008289899999));
#343869=CARTESIAN_POINT('Ctrl Pts',(4.00032868299994,12.2,1.04070962899999));
#343870=CARTESIAN_POINT('Ctrl Pts',(4.00032868299994,5.2,1.04070962899999));
#343871=CARTESIAN_POINT('Ctrl Pts',(4.00032868299994,2.2,1.04070962899999));
#343872=CARTESIAN_POINT('Ctrl Pts',(4.00144043399994,12.2,1.04134017399999));
#343873=CARTESIAN_POINT('Ctrl Pts',(4.00144043399994,5.2,1.04134017399999));
#343874=CARTESIAN_POINT('Ctrl Pts',(4.00144043399994,2.2,1.04134017399999));
#343875=CARTESIAN_POINT('Ctrl Pts',(4.00255580899994,12.2,1.04197453899999));
#343876=CARTESIAN_POINT('Ctrl Pts',(4.00255580899994,5.2,1.04197453899999));
#343877=CARTESIAN_POINT('Ctrl Pts',(4.00255580899994,2.2,1.04197453899999));
#343878=CARTESIAN_POINT('Ctrl Pts',(4.00367479199994,12.2,1.04261272799999));
#343879=CARTESIAN_POINT('Ctrl Pts',(4.00367479199994,5.2,1.04261272799999));
#343880=CARTESIAN_POINT('Ctrl Pts',(4.00367479199994,2.2,1.04261272799999));
#343881=CARTESIAN_POINT('Ctrl Pts',(4.00479737099994,12.2,1.04325474599999));
#343882=CARTESIAN_POINT('Ctrl Pts',(4.00479737099994,5.2,1.04325474599999));
#343883=CARTESIAN_POINT('Ctrl Pts',(4.00479737099994,2.2,1.04325474599999));
#343884=CARTESIAN_POINT('Ctrl Pts',(4.00592353199994,12.2,1.04390059899998));
#343885=CARTESIAN_POINT('Ctrl Pts',(4.00592353199994,5.2,1.04390059899998));
#343886=CARTESIAN_POINT('Ctrl Pts',(4.00592353199994,2.2,1.04390059899998));
#343887=CARTESIAN_POINT('Ctrl Pts',(4.00705326099995,12.2,1.04455029199999));
#343888=CARTESIAN_POINT('Ctrl Pts',(4.00705326099995,5.2,1.04455029199999));
#343889=CARTESIAN_POINT('Ctrl Pts',(4.00705326099995,2.2,1.04455029199999));
#343890=CARTESIAN_POINT('Ctrl Pts',(4.00818654499994,12.2,1.04520382899999));
#343891=CARTESIAN_POINT('Ctrl Pts',(4.00818654499994,5.2,1.04520382899999));
#343892=CARTESIAN_POINT('Ctrl Pts',(4.00818654499994,2.2,1.04520382899999));
#343893=CARTESIAN_POINT('Ctrl Pts',(4.00932336999994,12.2,1.04586121499999));
#343894=CARTESIAN_POINT('Ctrl Pts',(4.00932336999994,5.2,1.04586121499999));
#343895=CARTESIAN_POINT('Ctrl Pts',(4.00932336999994,2.2,1.04586121499999));
#343896=CARTESIAN_POINT('Ctrl Pts',(4.01046372199994,12.2,1.04652245599999));
#343897=CARTESIAN_POINT('Ctrl Pts',(4.01046372199994,5.2,1.04652245599999));
#343898=CARTESIAN_POINT('Ctrl Pts',(4.01046372199994,2.2,1.04652245599999));
#343899=CARTESIAN_POINT('Ctrl Pts',(4.01160758699994,12.2,1.04718755599999));
#343900=CARTESIAN_POINT('Ctrl Pts',(4.01160758699994,5.2,1.04718755599999));
#343901=CARTESIAN_POINT('Ctrl Pts',(4.01160758699994,2.2,1.04718755599999));
#343902=CARTESIAN_POINT('Ctrl Pts',(4.01275495299994,12.2,1.04785651999999));
#343903=CARTESIAN_POINT('Ctrl Pts',(4.01275495299994,5.2,1.04785651999999));
#343904=CARTESIAN_POINT('Ctrl Pts',(4.01275495299994,2.2,1.04785651999999));
#343905=CARTESIAN_POINT('Ctrl Pts',(4.01390580599994,12.2,1.04852935399999));
#343906=CARTESIAN_POINT('Ctrl Pts',(4.01390580599994,5.2,1.04852935399999));
#343907=CARTESIAN_POINT('Ctrl Pts',(4.01390580599994,2.2,1.04852935399999));
#343908=CARTESIAN_POINT('Ctrl Pts',(4.01506013099994,12.2,1.04920606099999));
#343909=CARTESIAN_POINT('Ctrl Pts',(4.01506013099994,5.2,1.04920606099999));
#343910=CARTESIAN_POINT('Ctrl Pts',(4.01506013099994,2.2,1.04920606099999));
#343911=CARTESIAN_POINT('Ctrl Pts',(4.01621791599994,12.2,1.04988664599999));
#343912=CARTESIAN_POINT('Ctrl Pts',(4.01621791599994,5.2,1.04988664599999));
#343913=CARTESIAN_POINT('Ctrl Pts',(4.01621791599994,2.2,1.04988664599999));
#343914=CARTESIAN_POINT('Ctrl Pts',(4.01737914599994,12.2,1.05057111399999));
#343915=CARTESIAN_POINT('Ctrl Pts',(4.01737914599994,5.2,1.05057111399999));
#343916=CARTESIAN_POINT('Ctrl Pts',(4.01737914599994,2.2,1.05057111399999));
#343917=CARTESIAN_POINT('Ctrl Pts',(4.01854380999994,12.2,1.05125947099999));
#343918=CARTESIAN_POINT('Ctrl Pts',(4.01854380999994,5.2,1.05125947099999));
#343919=CARTESIAN_POINT('Ctrl Pts',(4.01854380999994,2.2,1.05125947099999));
#343920=CARTESIAN_POINT('Ctrl Pts',(4.01971189299995,12.2,1.05195172099998));
#343921=CARTESIAN_POINT('Ctrl Pts',(4.01971189299995,5.2,1.05195172099998));
#343922=CARTESIAN_POINT('Ctrl Pts',(4.01971189299995,2.2,1.05195172099998));
#343923=CARTESIAN_POINT('Ctrl Pts',(4.02088338099994,12.2,1.05264786699999));
#343924=CARTESIAN_POINT('Ctrl Pts',(4.02088338099994,5.2,1.05264786699999));
#343925=CARTESIAN_POINT('Ctrl Pts',(4.02088338099994,2.2,1.05264786699999));
#343926=CARTESIAN_POINT('Ctrl Pts',(4.02205826199994,12.2,1.05334791499998));
#343927=CARTESIAN_POINT('Ctrl Pts',(4.02205826199994,5.2,1.05334791499998));
#343928=CARTESIAN_POINT('Ctrl Pts',(4.02205826199994,2.2,1.05334791499998));
#343929=CARTESIAN_POINT('Ctrl Pts',(4.02323652199994,12.2,1.05405186999999));
#343930=CARTESIAN_POINT('Ctrl Pts',(4.02323652199994,5.2,1.05405186999999));
#343931=CARTESIAN_POINT('Ctrl Pts',(4.02323652199994,2.2,1.05405186999999));
#343932=CARTESIAN_POINT('Ctrl Pts',(4.02441814699994,12.2,1.05475973599999));
#343933=CARTESIAN_POINT('Ctrl Pts',(4.02441814699994,5.2,1.05475973599999));
#343934=CARTESIAN_POINT('Ctrl Pts',(4.02441814699994,2.2,1.05475973599999));
#343935=CARTESIAN_POINT('Ctrl Pts',(4.02560312399994,12.2,1.05547151799998));
#343936=CARTESIAN_POINT('Ctrl Pts',(4.02560312399994,5.2,1.05547151799998));
#343937=CARTESIAN_POINT('Ctrl Pts',(4.02560312399994,2.2,1.05547151799998));
#343938=CARTESIAN_POINT('Ctrl Pts',(4.02679144099995,12.2,1.05618721999999));
#343939=CARTESIAN_POINT('Ctrl Pts',(4.02679144099995,5.2,1.05618721999999));
#343940=CARTESIAN_POINT('Ctrl Pts',(4.02679144099995,2.2,1.05618721999999));
#343941=CARTESIAN_POINT('Ctrl Pts',(4.02798308299994,12.2,1.05690684699999));
#343942=CARTESIAN_POINT('Ctrl Pts',(4.02798308299994,5.2,1.05690684699999));
#343943=CARTESIAN_POINT('Ctrl Pts',(4.02798308299994,2.2,1.05690684699999));
#343944=CARTESIAN_POINT('Ctrl Pts',(4.02917803799994,12.2,1.05763040199998));
#343945=CARTESIAN_POINT('Ctrl Pts',(4.02917803799994,5.2,1.05763040199998));
#343946=CARTESIAN_POINT('Ctrl Pts',(4.02917803799994,2.2,1.05763040199998));
#343947=CARTESIAN_POINT('Ctrl Pts',(4.03037629099994,12.2,1.05835789199999));
#343948=CARTESIAN_POINT('Ctrl Pts',(4.03037629099994,5.2,1.05835789199999));
#343949=CARTESIAN_POINT('Ctrl Pts',(4.03037629099994,2.2,1.05835789199999));
#343950=CARTESIAN_POINT('Ctrl Pts',(4.03157783099994,12.2,1.05908931899998));
#343951=CARTESIAN_POINT('Ctrl Pts',(4.03157783099994,5.2,1.05908931899998));
#343952=CARTESIAN_POINT('Ctrl Pts',(4.03157783099994,2.2,1.05908931899998));
#343953=CARTESIAN_POINT('Ctrl Pts',(4.03278264399995,12.2,1.05982468899999));
#343954=CARTESIAN_POINT('Ctrl Pts',(4.03278264399995,5.2,1.05982468899999));
#343955=CARTESIAN_POINT('Ctrl Pts',(4.03278264399995,2.2,1.05982468899999));
#343956=CARTESIAN_POINT('Ctrl Pts',(4.03399071699994,12.2,1.06056400499998));
#343957=CARTESIAN_POINT('Ctrl Pts',(4.03399071699994,5.2,1.06056400499998));
#343958=CARTESIAN_POINT('Ctrl Pts',(4.03399071699994,2.2,1.06056400499998));
#343959=CARTESIAN_POINT('Ctrl Pts',(4.03520203599994,12.2,1.06130727299998));
#343960=CARTESIAN_POINT('Ctrl Pts',(4.03520203599994,5.2,1.06130727299998));
#343961=CARTESIAN_POINT('Ctrl Pts',(4.03520203599994,2.2,1.06130727299998));
#343962=CARTESIAN_POINT('Ctrl Pts',(4.03641658799994,12.2,1.06205449599999));
#343963=CARTESIAN_POINT('Ctrl Pts',(4.03641658799994,5.2,1.06205449599999));
#343964=CARTESIAN_POINT('Ctrl Pts',(4.03641658799994,2.2,1.06205449599999));
#343965=CARTESIAN_POINT('Ctrl Pts',(4.03763435999995,12.2,1.06280567799999));
#343966=CARTESIAN_POINT('Ctrl Pts',(4.03763435999995,5.2,1.06280567799999));
#343967=CARTESIAN_POINT('Ctrl Pts',(4.03763435999995,2.2,1.06280567799999));
#343968=CARTESIAN_POINT('Ctrl Pts',(4.03885533999994,12.2,1.06356082499998));
#343969=CARTESIAN_POINT('Ctrl Pts',(4.03885533999994,5.2,1.06356082499998));
#343970=CARTESIAN_POINT('Ctrl Pts',(4.03885533999994,2.2,1.06356082499998));
#343971=CARTESIAN_POINT('Ctrl Pts',(4.04007951299994,12.2,1.06431993999998));
#343972=CARTESIAN_POINT('Ctrl Pts',(4.04007951299994,5.2,1.06431993999998));
#343973=CARTESIAN_POINT('Ctrl Pts',(4.04007951299994,2.2,1.06431993999998));
#343974=CARTESIAN_POINT('Ctrl Pts',(4.04130686699994,12.2,1.06508302599998));
#343975=CARTESIAN_POINT('Ctrl Pts',(4.04130686699994,5.2,1.06508302599998));
#343976=CARTESIAN_POINT('Ctrl Pts',(4.04130686699994,2.2,1.06508302599998));
#343977=CARTESIAN_POINT('Ctrl Pts',(4.04253738999994,12.2,1.06585008899998));
#343978=CARTESIAN_POINT('Ctrl Pts',(4.04253738999994,5.2,1.06585008899998));
#343979=CARTESIAN_POINT('Ctrl Pts',(4.04253738999994,2.2,1.06585008899998));
#343980=CARTESIAN_POINT('Ctrl Pts',(4.04377106799994,12.2,1.06662113399999));
#343981=CARTESIAN_POINT('Ctrl Pts',(4.04377106799994,5.2,1.06662113399999));
#343982=CARTESIAN_POINT('Ctrl Pts',(4.04377106799994,2.2,1.06662113399999));
#343983=CARTESIAN_POINT('Ctrl Pts',(4.04500788799994,12.2,1.06739616299999));
#343984=CARTESIAN_POINT('Ctrl Pts',(4.04500788799994,5.2,1.06739616299999));
#343985=CARTESIAN_POINT('Ctrl Pts',(4.04500788799994,2.2,1.06739616299999));
#343986=CARTESIAN_POINT('Ctrl Pts',(4.04624783599994,12.2,1.06817518099998));
#343987=CARTESIAN_POINT('Ctrl Pts',(4.04624783599994,5.2,1.06817518099998));
#343988=CARTESIAN_POINT('Ctrl Pts',(4.04624783599994,2.2,1.06817518099998));
#343989=CARTESIAN_POINT('Ctrl Pts',(4.04749090199994,12.2,1.06895819199998));
#343990=CARTESIAN_POINT('Ctrl Pts',(4.04749090199994,5.2,1.06895819199998));
#343991=CARTESIAN_POINT('Ctrl Pts',(4.04749090199994,2.2,1.06895819199998));
#343992=CARTESIAN_POINT('Ctrl Pts',(4.04873706999994,12.2,1.06974519899998));
#343993=CARTESIAN_POINT('Ctrl Pts',(4.04873706999994,5.2,1.06974519899998));
#343994=CARTESIAN_POINT('Ctrl Pts',(4.04873706999994,2.2,1.06974519899998));
#343995=CARTESIAN_POINT('Ctrl Pts',(4.04998632799995,12.2,1.07053620799999));
#343996=CARTESIAN_POINT('Ctrl Pts',(4.04998632799995,5.2,1.07053620799999));
#343997=CARTESIAN_POINT('Ctrl Pts',(4.04998632799995,2.2,1.07053620799999));
#343998=CARTESIAN_POINT('Ctrl Pts',(4.05123866399994,12.2,1.07133122099999));
#343999=CARTESIAN_POINT('Ctrl Pts',(4.05123866399994,5.2,1.07133122099999));
#344000=CARTESIAN_POINT('Ctrl Pts',(4.05123866399994,2.2,1.07133122099999));
#344001=CARTESIAN_POINT('Ctrl Pts',(4.05249406499994,12.2,1.07213024499998));
#344002=CARTESIAN_POINT('Ctrl Pts',(4.05249406499994,5.2,1.07213024499998));
#344003=CARTESIAN_POINT('Ctrl Pts',(4.05249406499994,2.2,1.07213024499998));
#344004=CARTESIAN_POINT('Ctrl Pts',(4.05375251799994,12.2,1.07293327999999));
#344005=CARTESIAN_POINT('Ctrl Pts',(4.05375251799994,5.2,1.07293327999999));
#344006=CARTESIAN_POINT('Ctrl Pts',(4.05375251799994,2.2,1.07293327999999));
#344007=CARTESIAN_POINT('Ctrl Pts',(4.05501400899994,12.2,1.07374033199998));
#344008=CARTESIAN_POINT('Ctrl Pts',(4.05501400899994,5.2,1.07374033199998));
#344009=CARTESIAN_POINT('Ctrl Pts',(4.05501400899994,2.2,1.07374033199998));
#344010=CARTESIAN_POINT('Ctrl Pts',(4.05627852699994,12.2,1.07455140599999));
#344011=CARTESIAN_POINT('Ctrl Pts',(4.05627852699994,5.2,1.07455140599999));
#344012=CARTESIAN_POINT('Ctrl Pts',(4.05627852699994,2.2,1.07455140599999));
#344013=CARTESIAN_POINT('Ctrl Pts',(4.05754605799994,12.2,1.07536650399998));
#344014=CARTESIAN_POINT('Ctrl Pts',(4.05754605799994,5.2,1.07536650399998));
#344015=CARTESIAN_POINT('Ctrl Pts',(4.05754605799994,2.2,1.07536650399998));
#344016=CARTESIAN_POINT('Ctrl Pts',(4.05881658999994,12.2,1.07618562999999));
#344017=CARTESIAN_POINT('Ctrl Pts',(4.05881658999994,5.2,1.07618562999999));
#344018=CARTESIAN_POINT('Ctrl Pts',(4.05881658999994,2.2,1.07618562999999));
#344019=CARTESIAN_POINT('Ctrl Pts',(4.06009010899994,12.2,1.07700878899998));
#344020=CARTESIAN_POINT('Ctrl Pts',(4.06009010899994,5.2,1.07700878899998));
#344021=CARTESIAN_POINT('Ctrl Pts',(4.06009010899994,2.2,1.07700878899998));
#344022=CARTESIAN_POINT('Ctrl Pts',(4.06136660399994,12.2,1.07783598399998));
#344023=CARTESIAN_POINT('Ctrl Pts',(4.06136660399994,5.2,1.07783598399998));
#344024=CARTESIAN_POINT('Ctrl Pts',(4.06136660399994,2.2,1.07783598399998));
#344025=CARTESIAN_POINT('Ctrl Pts',(4.06264606199994,12.2,1.07866721799999));
#344026=CARTESIAN_POINT('Ctrl Pts',(4.06264606199994,5.2,1.07866721799999));
#344027=CARTESIAN_POINT('Ctrl Pts',(4.06264606199994,2.2,1.07866721799999));
#344028=CARTESIAN_POINT('Ctrl Pts',(4.06392846999994,12.2,1.07950249699998));
#344029=CARTESIAN_POINT('Ctrl Pts',(4.06392846999994,5.2,1.07950249699998));
#344030=CARTESIAN_POINT('Ctrl Pts',(4.06392846999994,2.2,1.07950249699998));
#344031=CARTESIAN_POINT('Ctrl Pts',(4.06521381399994,12.2,1.08034182199999));
#344032=CARTESIAN_POINT('Ctrl Pts',(4.06521381399994,5.2,1.08034182199999));
#344033=CARTESIAN_POINT('Ctrl Pts',(4.06521381399994,2.2,1.08034182199999));
#344034=CARTESIAN_POINT('Ctrl Pts',(4.06650208399994,12.2,1.08118519899998));
#344035=CARTESIAN_POINT('Ctrl Pts',(4.06650208399994,5.2,1.08118519899998));
#344036=CARTESIAN_POINT('Ctrl Pts',(4.06650208399994,2.2,1.08118519899998));
#344037=CARTESIAN_POINT('Ctrl Pts',(4.06779326599994,12.2,1.08203262999998));
#344038=CARTESIAN_POINT('Ctrl Pts',(4.06779326599994,5.2,1.08203262999998));
#344039=CARTESIAN_POINT('Ctrl Pts',(4.06779326599994,2.2,1.08203262999998));
#344040=CARTESIAN_POINT('Ctrl Pts',(4.06908734599994,12.2,1.08288411999999));
#344041=CARTESIAN_POINT('Ctrl Pts',(4.06908734599994,5.2,1.08288411999999));
#344042=CARTESIAN_POINT('Ctrl Pts',(4.06908734599994,2.2,1.08288411999999));
#344043=CARTESIAN_POINT('Ctrl Pts',(4.07038431399994,12.2,1.08373967099999));
#344044=CARTESIAN_POINT('Ctrl Pts',(4.07038431399994,5.2,1.08373967099999));
#344045=CARTESIAN_POINT('Ctrl Pts',(4.07038431399994,2.2,1.08373967099999));
#344046=CARTESIAN_POINT('Ctrl Pts',(4.07168415599994,12.2,1.08459928899999));
#344047=CARTESIAN_POINT('Ctrl Pts',(4.07168415599994,5.2,1.08459928899999));
#344048=CARTESIAN_POINT('Ctrl Pts',(4.07168415599994,2.2,1.08459928899999));
#344049=CARTESIAN_POINT('Ctrl Pts',(4.07298685999994,12.2,1.08546297499998));
#344050=CARTESIAN_POINT('Ctrl Pts',(4.07298685999994,5.2,1.08546297499998));
#344051=CARTESIAN_POINT('Ctrl Pts',(4.07298685999994,2.2,1.08546297499998));
#344052=CARTESIAN_POINT('Ctrl Pts',(4.07429241299995,12.2,1.08633073399998));
#344053=CARTESIAN_POINT('Ctrl Pts',(4.07429241299995,5.2,1.08633073399998));
#344054=CARTESIAN_POINT('Ctrl Pts',(4.07429241299995,2.2,1.08633073399998));
#344055=CARTESIAN_POINT('Ctrl Pts',(4.07560080199994,12.2,1.08720256999999));
#344056=CARTESIAN_POINT('Ctrl Pts',(4.07560080199994,5.2,1.08720256999999));
#344057=CARTESIAN_POINT('Ctrl Pts',(4.07560080199994,2.2,1.08720256999999));
#344058=CARTESIAN_POINT('Ctrl Pts',(4.07691201699994,12.2,1.08807848499998));
#344059=CARTESIAN_POINT('Ctrl Pts',(4.07691201699994,5.2,1.08807848499998));
#344060=CARTESIAN_POINT('Ctrl Pts',(4.07691201699994,2.2,1.08807848499998));
#344061=CARTESIAN_POINT('Ctrl Pts',(4.07822604299994,12.2,1.08895848199999));
#344062=CARTESIAN_POINT('Ctrl Pts',(4.07822604299994,5.2,1.08895848199999));
#344063=CARTESIAN_POINT('Ctrl Pts',(4.07822604299994,2.2,1.08895848199999));
#344064=CARTESIAN_POINT('Ctrl Pts',(4.07954286799994,12.2,1.08984256799999));
#344065=CARTESIAN_POINT('Ctrl Pts',(4.07954286799994,5.2,1.08984256799999));
#344066=CARTESIAN_POINT('Ctrl Pts',(4.07954286799994,2.2,1.08984256799999));
#344067=CARTESIAN_POINT('Ctrl Pts',(4.08086248099994,12.2,1.09073074299999));
#344068=CARTESIAN_POINT('Ctrl Pts',(4.08086248099994,5.2,1.09073074299999));
#344069=CARTESIAN_POINT('Ctrl Pts',(4.08086248099994,2.2,1.09073074299999));
#344070=CARTESIAN_POINT('Ctrl Pts',(4.08218486799994,12.2,1.09162301099999));
#344071=CARTESIAN_POINT('Ctrl Pts',(4.08218486799994,5.2,1.09162301099999));
#344072=CARTESIAN_POINT('Ctrl Pts',(4.08218486799994,2.2,1.09162301099999));
#344073=CARTESIAN_POINT('Ctrl Pts',(4.08351001799994,12.2,1.09251937699999));
#344074=CARTESIAN_POINT('Ctrl Pts',(4.08351001799994,5.2,1.09251937699999));
#344075=CARTESIAN_POINT('Ctrl Pts',(4.08351001799994,2.2,1.09251937699999));
#344076=CARTESIAN_POINT('Ctrl Pts',(4.08483791699994,12.2,1.09341984299999));
#344077=CARTESIAN_POINT('Ctrl Pts',(4.08483791699994,5.2,1.09341984299999));
#344078=CARTESIAN_POINT('Ctrl Pts',(4.08483791699994,2.2,1.09341984299999));
#344079=CARTESIAN_POINT('Ctrl Pts',(4.08616855399995,12.2,1.09432441199999));
#344080=CARTESIAN_POINT('Ctrl Pts',(4.08616855399995,5.2,1.09432441199999));
#344081=CARTESIAN_POINT('Ctrl Pts',(4.08616855399995,2.2,1.09432441199999));
#344082=CARTESIAN_POINT('Ctrl Pts',(4.08750191699994,12.2,1.09523308899998));
#344083=CARTESIAN_POINT('Ctrl Pts',(4.08750191699994,5.2,1.09523308899998));
#344084=CARTESIAN_POINT('Ctrl Pts',(4.08750191699994,2.2,1.09523308899998));
#344085=CARTESIAN_POINT('Ctrl Pts',(4.08883799199994,12.2,1.09614587499999));
#344086=CARTESIAN_POINT('Ctrl Pts',(4.08883799199994,5.2,1.09614587499999));
#344087=CARTESIAN_POINT('Ctrl Pts',(4.08883799199994,2.2,1.09614587499999));
#344088=CARTESIAN_POINT('Ctrl Pts',(4.09017676799994,12.2,1.09706277699999));
#344089=CARTESIAN_POINT('Ctrl Pts',(4.09017676799994,5.2,1.09706277699999));
#344090=CARTESIAN_POINT('Ctrl Pts',(4.09017676799994,2.2,1.09706277699999));
#344091=CARTESIAN_POINT('Ctrl Pts',(4.09151823199995,12.2,1.09798379399999));
#344092=CARTESIAN_POINT('Ctrl Pts',(4.09151823199995,5.2,1.09798379399999));
#344093=CARTESIAN_POINT('Ctrl Pts',(4.09151823199995,2.2,1.09798379399999));
#344094=CARTESIAN_POINT('Ctrl Pts',(4.09286237299994,12.2,1.09890893099998));
#344095=CARTESIAN_POINT('Ctrl Pts',(4.09286237299994,5.2,1.09890893099998));
#344096=CARTESIAN_POINT('Ctrl Pts',(4.09286237299994,2.2,1.09890893099998));
#344097=CARTESIAN_POINT('Ctrl Pts',(4.09420917799994,12.2,1.09983819099998));
#344098=CARTESIAN_POINT('Ctrl Pts',(4.09420917799994,5.2,1.09983819099998));
#344099=CARTESIAN_POINT('Ctrl Pts',(4.09420917799994,2.2,1.09983819099998));
#344100=CARTESIAN_POINT('Ctrl Pts',(4.09555863499994,12.2,1.10077157799998));
#344101=CARTESIAN_POINT('Ctrl Pts',(4.09555863499994,5.2,1.10077157799998));
#344102=CARTESIAN_POINT('Ctrl Pts',(4.09555863499994,2.2,1.10077157799998));
#344103=CARTESIAN_POINT('Ctrl Pts',(4.09691072999994,12.2,1.10170909499999));
#344104=CARTESIAN_POINT('Ctrl Pts',(4.09691072999994,5.2,1.10170909499999));
#344105=CARTESIAN_POINT('Ctrl Pts',(4.09691072999994,2.2,1.10170909499999));
#344106=CARTESIAN_POINT('Ctrl Pts',(4.09826545399994,12.2,1.10265074399999));
#344107=CARTESIAN_POINT('Ctrl Pts',(4.09826545399994,5.2,1.10265074399999));
#344108=CARTESIAN_POINT('Ctrl Pts',(4.09826545399994,2.2,1.10265074399999));
#344109=CARTESIAN_POINT('Ctrl Pts',(4.09962279199994,12.2,1.10359652899998));
#344110=CARTESIAN_POINT('Ctrl Pts',(4.09962279199994,5.2,1.10359652899998));
#344111=CARTESIAN_POINT('Ctrl Pts',(4.09962279199994,2.2,1.10359652899998));
#344112=CARTESIAN_POINT('Ctrl Pts',(4.10098273499994,12.2,1.10454645299999));
#344113=CARTESIAN_POINT('Ctrl Pts',(4.10098273499994,5.2,1.10454645299999));
#344114=CARTESIAN_POINT('Ctrl Pts',(4.10098273499994,2.2,1.10454645299999));
#344115=CARTESIAN_POINT('Ctrl Pts',(4.10234526799994,12.2,1.10550051799999));
#344116=CARTESIAN_POINT('Ctrl Pts',(4.10234526799994,5.2,1.10550051799999));
#344117=CARTESIAN_POINT('Ctrl Pts',(4.10234526799994,2.2,1.10550051799999));
#344118=CARTESIAN_POINT('Ctrl Pts',(4.10371038099994,12.2,1.10645872899998));
#344119=CARTESIAN_POINT('Ctrl Pts',(4.10371038099994,5.2,1.10645872899998));
#344120=CARTESIAN_POINT('Ctrl Pts',(4.10371038099994,2.2,1.10645872899998));
#344121=CARTESIAN_POINT('Ctrl Pts',(4.10507805999995,12.2,1.10742108799998));
#344122=CARTESIAN_POINT('Ctrl Pts',(4.10507805999995,5.2,1.10742108799998));
#344123=CARTESIAN_POINT('Ctrl Pts',(4.10507805999995,2.2,1.10742108799998));
#344124=CARTESIAN_POINT('Ctrl Pts',(4.10644829399994,12.2,1.10838759899998));
#344125=CARTESIAN_POINT('Ctrl Pts',(4.10644829399994,5.2,1.10838759899998));
#344126=CARTESIAN_POINT('Ctrl Pts',(4.10644829399994,2.2,1.10838759899998));
#344127=CARTESIAN_POINT('Ctrl Pts',(4.10782107099994,12.2,1.10935826299999));
#344128=CARTESIAN_POINT('Ctrl Pts',(4.10782107099994,5.2,1.10935826299999));
#344129=CARTESIAN_POINT('Ctrl Pts',(4.10782107099994,2.2,1.10935826299999));
#344130=CARTESIAN_POINT('Ctrl Pts',(4.10919637799994,12.2,1.11033308499998));
#344131=CARTESIAN_POINT('Ctrl Pts',(4.10919637799994,5.2,1.11033308499998));
#344132=CARTESIAN_POINT('Ctrl Pts',(4.10919637799994,2.2,1.11033308499998));
#344133=CARTESIAN_POINT('Ctrl Pts',(4.11057420499994,12.2,1.11131206599998));
#344134=CARTESIAN_POINT('Ctrl Pts',(4.11057420499994,5.2,1.11131206599998));
#344135=CARTESIAN_POINT('Ctrl Pts',(4.11057420499994,2.2,1.11131206599998));
#344136=CARTESIAN_POINT('Ctrl Pts',(4.11195453799994,12.2,1.11229520999998));
#344137=CARTESIAN_POINT('Ctrl Pts',(4.11195453799994,5.2,1.11229520999998));
#344138=CARTESIAN_POINT('Ctrl Pts',(4.11195453799994,2.2,1.11229520999998));
#344139=CARTESIAN_POINT('Ctrl Pts',(4.11333736599994,12.2,1.11328251999999));
#344140=CARTESIAN_POINT('Ctrl Pts',(4.11333736599994,5.2,1.11328251999999));
#344141=CARTESIAN_POINT('Ctrl Pts',(4.11333736599994,2.2,1.11328251999999));
#344142=CARTESIAN_POINT('Ctrl Pts',(4.11472267799994,12.2,1.11427399899998));
#344143=CARTESIAN_POINT('Ctrl Pts',(4.11472267799994,5.2,1.11427399899998));
#344144=CARTESIAN_POINT('Ctrl Pts',(4.11472267799994,2.2,1.11427399899998));
#344145=CARTESIAN_POINT('Ctrl Pts',(4.11611045999994,12.2,1.11526964999999));
#344146=CARTESIAN_POINT('Ctrl Pts',(4.11611045999994,5.2,1.11526964999999));
#344147=CARTESIAN_POINT('Ctrl Pts',(4.11611045999994,2.2,1.11526964999999));
#344148=CARTESIAN_POINT('Ctrl Pts',(4.11750070199994,12.2,1.11626947399999));
#344149=CARTESIAN_POINT('Ctrl Pts',(4.11750070199994,5.2,1.11626947399999));
#344150=CARTESIAN_POINT('Ctrl Pts',(4.11750070199994,2.2,1.11626947399999));
#344151=CARTESIAN_POINT('Ctrl Pts',(4.11889338999995,12.2,1.11727347599999));
#344152=CARTESIAN_POINT('Ctrl Pts',(4.11889338999995,5.2,1.11727347599999));
#344153=CARTESIAN_POINT('Ctrl Pts',(4.11889338999995,2.2,1.11727347599999));
#344154=CARTESIAN_POINT('Ctrl Pts',(4.12028851399994,12.2,1.11828165799999));
#344155=CARTESIAN_POINT('Ctrl Pts',(4.12028851399994,5.2,1.11828165799999));
#344156=CARTESIAN_POINT('Ctrl Pts',(4.12028851399994,2.2,1.11828165799999));
#344157=CARTESIAN_POINT('Ctrl Pts',(4.12168606199994,12.2,1.11929402299999));
#344158=CARTESIAN_POINT('Ctrl Pts',(4.12168606199994,5.2,1.11929402299999));
#344159=CARTESIAN_POINT('Ctrl Pts',(4.12168606199994,2.2,1.11929402299999));
#344160=CARTESIAN_POINT('Ctrl Pts',(4.12308602099994,12.2,1.12031057299999));
#344161=CARTESIAN_POINT('Ctrl Pts',(4.12308602099994,5.2,1.12031057299999));
#344162=CARTESIAN_POINT('Ctrl Pts',(4.12308602099994,2.2,1.12031057299999));
#344163=CARTESIAN_POINT('Ctrl Pts',(4.12448838099994,12.2,1.12133131199998));
#344164=CARTESIAN_POINT('Ctrl Pts',(4.12448838099994,5.2,1.12133131199998));
#344165=CARTESIAN_POINT('Ctrl Pts',(4.12448838099994,2.2,1.12133131199998));
#344166=CARTESIAN_POINT('Ctrl Pts',(4.12589312799994,12.2,1.12235624199998));
#344167=CARTESIAN_POINT('Ctrl Pts',(4.12589312799994,5.2,1.12235624199998));
#344168=CARTESIAN_POINT('Ctrl Pts',(4.12589312799994,2.2,1.12235624199998));
#344169=CARTESIAN_POINT('Ctrl Pts',(4.12730025099994,12.2,1.12338536399998));
#344170=CARTESIAN_POINT('Ctrl Pts',(4.12730025099994,5.2,1.12338536399998));
#344171=CARTESIAN_POINT('Ctrl Pts',(4.12730025099994,2.2,1.12338536399998));
#344172=CARTESIAN_POINT('Ctrl Pts',(4.12870973899994,12.2,1.12441868399999));
#344173=CARTESIAN_POINT('Ctrl Pts',(4.12870973899994,5.2,1.12441868399999));
#344174=CARTESIAN_POINT('Ctrl Pts',(4.12870973899994,2.2,1.12441868399999));
#344175=CARTESIAN_POINT('Ctrl Pts',(4.13012157999994,12.2,1.12545620199999));
#344176=CARTESIAN_POINT('Ctrl Pts',(4.13012157999994,5.2,1.12545620199999));
#344177=CARTESIAN_POINT('Ctrl Pts',(4.13012157999994,2.2,1.12545620199999));
#344178=CARTESIAN_POINT('Ctrl Pts',(4.13153576199994,12.2,1.12649792199999));
#344179=CARTESIAN_POINT('Ctrl Pts',(4.13153576199994,5.2,1.12649792199999));
#344180=CARTESIAN_POINT('Ctrl Pts',(4.13153576199994,2.2,1.12649792199999));
#344181=CARTESIAN_POINT('Ctrl Pts',(4.13295227299994,12.2,1.12754384699999));
#344182=CARTESIAN_POINT('Ctrl Pts',(4.13295227299994,5.2,1.12754384699999));
#344183=CARTESIAN_POINT('Ctrl Pts',(4.13295227299994,2.2,1.12754384699999));
#344184=CARTESIAN_POINT('Ctrl Pts',(4.13437110199994,12.2,1.12859397699999));
#344185=CARTESIAN_POINT('Ctrl Pts',(4.13437110199994,5.2,1.12859397699999));
#344186=CARTESIAN_POINT('Ctrl Pts',(4.13437110199994,2.2,1.12859397699999));
#344187=CARTESIAN_POINT('Ctrl Pts',(4.13579223699994,12.2,1.12964831799998));
#344188=CARTESIAN_POINT('Ctrl Pts',(4.13579223699994,5.2,1.12964831799998));
#344189=CARTESIAN_POINT('Ctrl Pts',(4.13579223699994,2.2,1.12964831799998));
#344190=CARTESIAN_POINT('Ctrl Pts',(4.13721566599994,12.2,1.13070686999999));
#344191=CARTESIAN_POINT('Ctrl Pts',(4.13721566599994,5.2,1.13070686999999));
#344192=CARTESIAN_POINT('Ctrl Pts',(4.13721566599994,2.2,1.13070686999999));
#344193=CARTESIAN_POINT('Ctrl Pts',(4.13864137799994,12.2,1.13176963599999));
#344194=CARTESIAN_POINT('Ctrl Pts',(4.13864137799994,5.2,1.13176963599999));
#344195=CARTESIAN_POINT('Ctrl Pts',(4.13864137799994,2.2,1.13176963599999));
#344196=CARTESIAN_POINT('Ctrl Pts',(4.14006936099994,12.2,1.13283661899999));
#344197=CARTESIAN_POINT('Ctrl Pts',(4.14006936099994,5.2,1.13283661899999));
#344198=CARTESIAN_POINT('Ctrl Pts',(4.14006936099994,2.2,1.13283661899999));
#344199=CARTESIAN_POINT('Ctrl Pts',(4.14149960399994,12.2,1.13390782299998));
#344200=CARTESIAN_POINT('Ctrl Pts',(4.14149960399994,5.2,1.13390782299998));
#344201=CARTESIAN_POINT('Ctrl Pts',(4.14149960399994,2.2,1.13390782299998));
#344202=CARTESIAN_POINT('Ctrl Pts',(4.14293209399994,12.2,1.13498324699998));
#344203=CARTESIAN_POINT('Ctrl Pts',(4.14293209399994,5.2,1.13498324699998));
#344204=CARTESIAN_POINT('Ctrl Pts',(4.14293209399994,2.2,1.13498324699998));
#344205=CARTESIAN_POINT('Ctrl Pts',(4.14436682099994,12.2,1.13606289599999));
#344206=CARTESIAN_POINT('Ctrl Pts',(4.14436682099994,5.2,1.13606289599999));
#344207=CARTESIAN_POINT('Ctrl Pts',(4.14436682099994,2.2,1.13606289599999));
#344208=CARTESIAN_POINT('Ctrl Pts',(4.14580377199994,12.2,1.13714677199999));
#344209=CARTESIAN_POINT('Ctrl Pts',(4.14580377199994,5.2,1.13714677199999));
#344210=CARTESIAN_POINT('Ctrl Pts',(4.14580377199994,2.2,1.13714677199999));
#344211=CARTESIAN_POINT('Ctrl Pts',(4.14724293699994,12.2,1.13823487699999));
#344212=CARTESIAN_POINT('Ctrl Pts',(4.14724293699994,5.2,1.13823487699999));
#344213=CARTESIAN_POINT('Ctrl Pts',(4.14724293699994,2.2,1.13823487699999));
#344214=CARTESIAN_POINT('Ctrl Pts',(4.14868430299994,12.2,1.13932721399999));
#344215=CARTESIAN_POINT('Ctrl Pts',(4.14868430299994,5.2,1.13932721399999));
#344216=CARTESIAN_POINT('Ctrl Pts',(4.14868430299994,2.2,1.13932721399999));
#344217=CARTESIAN_POINT('Ctrl Pts',(4.15012785899994,12.2,1.14042378299999));
#344218=CARTESIAN_POINT('Ctrl Pts',(4.15012785899994,5.2,1.14042378299999));
#344219=CARTESIAN_POINT('Ctrl Pts',(4.15012785899994,2.2,1.14042378299999));
#344220=CARTESIAN_POINT('Ctrl Pts',(4.15157359399995,12.2,1.14152458999999));
#344221=CARTESIAN_POINT('Ctrl Pts',(4.15157359399995,5.2,1.14152458999999));
#344222=CARTESIAN_POINT('Ctrl Pts',(4.15157359399995,2.2,1.14152458999999));
#344223=CARTESIAN_POINT('Ctrl Pts',(4.15302149599994,12.2,1.14262963499999));
#344224=CARTESIAN_POINT('Ctrl Pts',(4.15302149599994,5.2,1.14262963499999));
#344225=CARTESIAN_POINT('Ctrl Pts',(4.15302149599994,2.2,1.14262963499999));
#344226=CARTESIAN_POINT('Ctrl Pts',(4.15447155399994,12.2,1.14373892099998));
#344227=CARTESIAN_POINT('Ctrl Pts',(4.15447155399994,5.2,1.14373892099998));
#344228=CARTESIAN_POINT('Ctrl Pts',(4.15447155399994,2.2,1.14373892099998));
#344229=CARTESIAN_POINT('Ctrl Pts',(4.15592375599994,12.2,1.14485244999999));
#344230=CARTESIAN_POINT('Ctrl Pts',(4.15592375599994,5.2,1.14485244999999));
#344231=CARTESIAN_POINT('Ctrl Pts',(4.15592375599994,2.2,1.14485244999999));
#344232=CARTESIAN_POINT('Ctrl Pts',(4.15737809199995,12.2,1.14597022399999));
#344233=CARTESIAN_POINT('Ctrl Pts',(4.15737809199995,5.2,1.14597022399999));
#344234=CARTESIAN_POINT('Ctrl Pts',(4.15737809199995,2.2,1.14597022399999));
#344235=CARTESIAN_POINT('Ctrl Pts',(4.15883454899994,12.2,1.14709224599999));
#344236=CARTESIAN_POINT('Ctrl Pts',(4.15883454899994,5.2,1.14709224599999));
#344237=CARTESIAN_POINT('Ctrl Pts',(4.15883454899994,2.2,1.14709224599999));
#344238=CARTESIAN_POINT('Ctrl Pts',(4.16029311599995,12.2,1.14821851799999));
#344239=CARTESIAN_POINT('Ctrl Pts',(4.16029311599995,5.2,1.14821851799999));
#344240=CARTESIAN_POINT('Ctrl Pts',(4.16029311599995,2.2,1.14821851799999));
#344241=CARTESIAN_POINT('Ctrl Pts',(4.16175377999994,12.2,1.14934904099998));
#344242=CARTESIAN_POINT('Ctrl Pts',(4.16175377999994,5.2,1.14934904099998));
#344243=CARTESIAN_POINT('Ctrl Pts',(4.16175377999994,2.2,1.14934904099998));
#344244=CARTESIAN_POINT('Ctrl Pts',(4.16321653299994,12.2,1.15048381999999));
#344245=CARTESIAN_POINT('Ctrl Pts',(4.16321653299994,5.2,1.15048381999999));
#344246=CARTESIAN_POINT('Ctrl Pts',(4.16321653299994,2.2,1.15048381999999));
#344247=CARTESIAN_POINT('Ctrl Pts',(4.16468136199994,12.2,1.15162285499999));
#344248=CARTESIAN_POINT('Ctrl Pts',(4.16468136199994,5.2,1.15162285499999));
#344249=CARTESIAN_POINT('Ctrl Pts',(4.16468136199994,2.2,1.15162285499999));
#344250=CARTESIAN_POINT('Ctrl Pts',(4.16614825599994,12.2,1.15276614799999));
#344251=CARTESIAN_POINT('Ctrl Pts',(4.16614825599994,5.2,1.15276614799999));
#344252=CARTESIAN_POINT('Ctrl Pts',(4.16614825599994,2.2,1.15276614799999));
#344253=CARTESIAN_POINT('Ctrl Pts',(4.16761720299994,12.2,1.15391370199998));
#344254=CARTESIAN_POINT('Ctrl Pts',(4.16761720299994,5.2,1.15391370199998));
#344255=CARTESIAN_POINT('Ctrl Pts',(4.16761720299994,2.2,1.15391370199998));
#344256=CARTESIAN_POINT('Ctrl Pts',(4.16908819199994,12.2,1.15506551899998));
#344257=CARTESIAN_POINT('Ctrl Pts',(4.16908819199994,5.2,1.15506551899998));
#344258=CARTESIAN_POINT('Ctrl Pts',(4.16908819199994,2.2,1.15506551899998));
#344259=CARTESIAN_POINT('Ctrl Pts',(4.17056121199994,12.2,1.15622159999999));
#344260=CARTESIAN_POINT('Ctrl Pts',(4.17056121199994,5.2,1.15622159999999));
#344261=CARTESIAN_POINT('Ctrl Pts',(4.17056121199994,2.2,1.15622159999999));
#344262=CARTESIAN_POINT('Ctrl Pts',(4.17203625199994,12.2,1.15738194899999));
#344263=CARTESIAN_POINT('Ctrl Pts',(4.17203625199994,5.2,1.15738194899999));
#344264=CARTESIAN_POINT('Ctrl Pts',(4.17203625199994,2.2,1.15738194899999));
#344265=CARTESIAN_POINT('Ctrl Pts',(4.17351329999994,12.2,1.15854656699999));
#344266=CARTESIAN_POINT('Ctrl Pts',(4.17351329999994,5.2,1.15854656699999));
#344267=CARTESIAN_POINT('Ctrl Pts',(4.17351329999994,2.2,1.15854656699999));
#344268=CARTESIAN_POINT('Ctrl Pts',(4.17499234499994,12.2,1.15971545599999));
#344269=CARTESIAN_POINT('Ctrl Pts',(4.17499234499994,5.2,1.15971545599999));
#344270=CARTESIAN_POINT('Ctrl Pts',(4.17499234499994,2.2,1.15971545599999));
#344271=CARTESIAN_POINT('Ctrl Pts',(4.17647337599994,12.2,1.16088861699998));
#344272=CARTESIAN_POINT('Ctrl Pts',(4.17647337599994,5.2,1.16088861699998));
#344273=CARTESIAN_POINT('Ctrl Pts',(4.17647337599994,2.2,1.16088861699998));
#344274=CARTESIAN_POINT('Ctrl Pts',(4.17795638199994,12.2,1.16206605399999));
#344275=CARTESIAN_POINT('Ctrl Pts',(4.17795638199994,5.2,1.16206605399999));
#344276=CARTESIAN_POINT('Ctrl Pts',(4.17795638199994,2.2,1.16206605399999));
#344277=CARTESIAN_POINT('Ctrl Pts',(4.17944135099994,12.2,1.16324776899999));
#344278=CARTESIAN_POINT('Ctrl Pts',(4.17944135099994,5.2,1.16324776899999));
#344279=CARTESIAN_POINT('Ctrl Pts',(4.17944135099994,2.2,1.16324776899999));
#344280=CARTESIAN_POINT('Ctrl Pts',(4.18092827299995,12.2,1.16443376099999));
#344281=CARTESIAN_POINT('Ctrl Pts',(4.18092827299995,5.2,1.16443376099999));
#344282=CARTESIAN_POINT('Ctrl Pts',(4.18092827299995,2.2,1.16443376099999));
#344283=CARTESIAN_POINT('Ctrl Pts',(4.18241713599994,12.2,1.16562403599998));
#344284=CARTESIAN_POINT('Ctrl Pts',(4.18241713599994,5.2,1.16562403599998));
#344285=CARTESIAN_POINT('Ctrl Pts',(4.18241713599994,2.2,1.16562403599998));
#344286=CARTESIAN_POINT('Ctrl Pts',(4.18390792899995,12.2,1.16681859199999));
#344287=CARTESIAN_POINT('Ctrl Pts',(4.18390792899995,5.2,1.16681859199999));
#344288=CARTESIAN_POINT('Ctrl Pts',(4.18390792899995,2.2,1.16681859199999));
#344289=CARTESIAN_POINT('Ctrl Pts',(4.18540064099994,12.2,1.16801743399999));
#344290=CARTESIAN_POINT('Ctrl Pts',(4.18540064099994,5.2,1.16801743399999));
#344291=CARTESIAN_POINT('Ctrl Pts',(4.18540064099994,2.2,1.16801743399999));
#344292=CARTESIAN_POINT('Ctrl Pts',(4.18689526199994,12.2,1.16922056299999));
#344293=CARTESIAN_POINT('Ctrl Pts',(4.18689526199994,5.2,1.16922056299999));
#344294=CARTESIAN_POINT('Ctrl Pts',(4.18689526199994,2.2,1.16922056299999));
#344295=CARTESIAN_POINT('Ctrl Pts',(4.18839177799994,12.2,1.17042797999999));
#344296=CARTESIAN_POINT('Ctrl Pts',(4.18839177799994,5.2,1.17042797999999));
#344297=CARTESIAN_POINT('Ctrl Pts',(4.18839177799994,2.2,1.17042797999999));
#344298=CARTESIAN_POINT('Ctrl Pts',(4.18989018099994,12.2,1.17163968799999));
#344299=CARTESIAN_POINT('Ctrl Pts',(4.18989018099994,5.2,1.17163968799999));
#344300=CARTESIAN_POINT('Ctrl Pts',(4.18989018099994,2.2,1.17163968799999));
#344301=CARTESIAN_POINT('Ctrl Pts',(4.19139045799994,12.2,1.17285568699999));
#344302=CARTESIAN_POINT('Ctrl Pts',(4.19139045799994,5.2,1.17285568699999));
#344303=CARTESIAN_POINT('Ctrl Pts',(4.19139045799994,2.2,1.17285568699999));
#344304=CARTESIAN_POINT('Ctrl Pts',(4.19289259999994,12.2,1.17407598099998));
#344305=CARTESIAN_POINT('Ctrl Pts',(4.19289259999994,5.2,1.17407598099998));
#344306=CARTESIAN_POINT('Ctrl Pts',(4.19289259999994,2.2,1.17407598099998));
#344307=CARTESIAN_POINT('Ctrl Pts',(4.19439659299994,12.2,1.17530057099998));
#344308=CARTESIAN_POINT('Ctrl Pts',(4.19439659299994,5.2,1.17530057099998));
#344309=CARTESIAN_POINT('Ctrl Pts',(4.19439659299994,2.2,1.17530057099998));
#344310=CARTESIAN_POINT('Ctrl Pts',(4.19590242799995,12.2,1.17652945699998));
#344311=CARTESIAN_POINT('Ctrl Pts',(4.19590242799995,5.2,1.17652945699998));
#344312=CARTESIAN_POINT('Ctrl Pts',(4.19590242799995,2.2,1.17652945699998));
#344313=CARTESIAN_POINT('Ctrl Pts',(4.19741009499994,12.2,1.17776264499998));
#344314=CARTESIAN_POINT('Ctrl Pts',(4.19741009499994,5.2,1.17776264499998));
#344315=CARTESIAN_POINT('Ctrl Pts',(4.19741009499994,2.2,1.17776264499998));
#344316=CARTESIAN_POINT('Ctrl Pts',(4.19891957999995,12.2,1.17900013199999));
#344317=CARTESIAN_POINT('Ctrl Pts',(4.19891957999995,5.2,1.17900013199999));
#344318=CARTESIAN_POINT('Ctrl Pts',(4.19891957999995,2.2,1.17900013199999));
#344319=CARTESIAN_POINT('Ctrl Pts',(4.20043087499994,12.2,1.18024192399998));
#344320=CARTESIAN_POINT('Ctrl Pts',(4.20043087499994,5.2,1.18024192399998));
#344321=CARTESIAN_POINT('Ctrl Pts',(4.20043087499994,2.2,1.18024192399998));
#344322=CARTESIAN_POINT('Ctrl Pts',(4.20194396799995,12.2,1.18148801899999));
#344323=CARTESIAN_POINT('Ctrl Pts',(4.20194396799995,5.2,1.18148801899999));
#344324=CARTESIAN_POINT('Ctrl Pts',(4.20194396799995,2.2,1.18148801899999));
#344325=CARTESIAN_POINT('Ctrl Pts',(4.20345884699994,12.2,1.18273841999998));
#344326=CARTESIAN_POINT('Ctrl Pts',(4.20345884699994,5.2,1.18273841999998));
#344327=CARTESIAN_POINT('Ctrl Pts',(4.20345884699994,2.2,1.18273841999998));
#344328=CARTESIAN_POINT('Ctrl Pts',(4.20497550199994,12.2,1.18399312999999));
#344329=CARTESIAN_POINT('Ctrl Pts',(4.20497550199994,5.2,1.18399312999999));
#344330=CARTESIAN_POINT('Ctrl Pts',(4.20497550199994,2.2,1.18399312999999));
#344331=CARTESIAN_POINT('Ctrl Pts',(4.20649392199994,12.2,1.18525214899998));
#344332=CARTESIAN_POINT('Ctrl Pts',(4.20649392199994,5.2,1.18525214899998));
#344333=CARTESIAN_POINT('Ctrl Pts',(4.20649392199994,2.2,1.18525214899998));
#344334=CARTESIAN_POINT('Ctrl Pts',(4.20801409699994,12.2,1.18651547999999));
#344335=CARTESIAN_POINT('Ctrl Pts',(4.20801409699994,5.2,1.18651547999999));
#344336=CARTESIAN_POINT('Ctrl Pts',(4.20801409699994,2.2,1.18651547999999));
#344337=CARTESIAN_POINT('Ctrl Pts',(4.20953601499995,12.2,1.18778312299999));
#344338=CARTESIAN_POINT('Ctrl Pts',(4.20953601499995,5.2,1.18778312299999));
#344339=CARTESIAN_POINT('Ctrl Pts',(4.20953601499995,2.2,1.18778312299999));
#344340=CARTESIAN_POINT('Ctrl Pts',(4.21105966599994,12.2,1.18905508099999));
#344341=CARTESIAN_POINT('Ctrl Pts',(4.21105966599994,5.2,1.18905508099999));
#344342=CARTESIAN_POINT('Ctrl Pts',(4.21105966599994,2.2,1.18905508099999));
#344343=CARTESIAN_POINT('Ctrl Pts',(4.21258503799994,12.2,1.19033135499999));
#344344=CARTESIAN_POINT('Ctrl Pts',(4.21258503799994,5.2,1.19033135499999));
#344345=CARTESIAN_POINT('Ctrl Pts',(4.21258503799994,2.2,1.19033135499999));
#344346=CARTESIAN_POINT('Ctrl Pts',(4.21411212099995,12.2,1.19161194699998));
#344347=CARTESIAN_POINT('Ctrl Pts',(4.21411212099995,5.2,1.19161194699998));
#344348=CARTESIAN_POINT('Ctrl Pts',(4.21411212099995,2.2,1.19161194699998));
#344349=CARTESIAN_POINT('Ctrl Pts',(4.21564090399994,12.2,1.19289685699998));
#344350=CARTESIAN_POINT('Ctrl Pts',(4.21564090399994,5.2,1.19289685699998));
#344351=CARTESIAN_POINT('Ctrl Pts',(4.21564090399994,2.2,1.19289685699998));
#344352=CARTESIAN_POINT('Ctrl Pts',(4.21717137599994,12.2,1.19418608799998));
#344353=CARTESIAN_POINT('Ctrl Pts',(4.21717137599994,5.2,1.19418608799998));
#344354=CARTESIAN_POINT('Ctrl Pts',(4.21717137599994,2.2,1.19418608799998));
#344355=CARTESIAN_POINT('Ctrl Pts',(4.21870352699994,12.2,1.19547964099999));
#344356=CARTESIAN_POINT('Ctrl Pts',(4.21870352699994,5.2,1.19547964099999));
#344357=CARTESIAN_POINT('Ctrl Pts',(4.21870352699994,2.2,1.19547964099999));
#344358=CARTESIAN_POINT('Ctrl Pts',(4.22023734499995,12.2,1.19677751899999));
#344359=CARTESIAN_POINT('Ctrl Pts',(4.22023734499995,5.2,1.19677751899999));
#344360=CARTESIAN_POINT('Ctrl Pts',(4.22023734499995,2.2,1.19677751899999));
#344361=CARTESIAN_POINT('Ctrl Pts',(4.22177282099994,12.2,1.19807972199999));
#344362=CARTESIAN_POINT('Ctrl Pts',(4.22177282099994,5.2,1.19807972199999));
#344363=CARTESIAN_POINT('Ctrl Pts',(4.22177282099994,2.2,1.19807972199999));
#344364=CARTESIAN_POINT('Ctrl Pts',(4.22330994299995,12.2,1.19938625099998));
#344365=CARTESIAN_POINT('Ctrl Pts',(4.22330994299995,5.2,1.19938625099998));
#344366=CARTESIAN_POINT('Ctrl Pts',(4.22330994299995,2.2,1.19938625099998));
#344367=CARTESIAN_POINT('Ctrl Pts',(4.22484870099994,12.2,1.20069710799998));
#344368=CARTESIAN_POINT('Ctrl Pts',(4.22484870099994,5.2,1.20069710799998));
#344369=CARTESIAN_POINT('Ctrl Pts',(4.22484870099994,2.2,1.20069710799998));
#344370=CARTESIAN_POINT('Ctrl Pts',(4.22638908299994,12.2,1.20201229499999));
#344371=CARTESIAN_POINT('Ctrl Pts',(4.22638908299994,5.2,1.20201229499999));
#344372=CARTESIAN_POINT('Ctrl Pts',(4.22638908299994,2.2,1.20201229499999));
#344373=CARTESIAN_POINT('Ctrl Pts',(4.22793107999994,12.2,1.20333181299999));
#344374=CARTESIAN_POINT('Ctrl Pts',(4.22793107999994,5.2,1.20333181299999));
#344375=CARTESIAN_POINT('Ctrl Pts',(4.22793107999994,2.2,1.20333181299999));
#344376=CARTESIAN_POINT('Ctrl Pts',(4.22947467999994,12.2,1.20465566299998));
#344377=CARTESIAN_POINT('Ctrl Pts',(4.22947467999994,5.2,1.20465566299998));
#344378=CARTESIAN_POINT('Ctrl Pts',(4.22947467999994,2.2,1.20465566299998));
#344379=CARTESIAN_POINT('Ctrl Pts',(4.23101987299995,12.2,1.20598384699999));
#344380=CARTESIAN_POINT('Ctrl Pts',(4.23101987299995,5.2,1.20598384699999));
#344381=CARTESIAN_POINT('Ctrl Pts',(4.23101987299995,2.2,1.20598384699999));
#344382=CARTESIAN_POINT('Ctrl Pts',(4.23256664799994,12.2,1.20731636599999));
#344383=CARTESIAN_POINT('Ctrl Pts',(4.23256664799994,5.2,1.20731636599999));
#344384=CARTESIAN_POINT('Ctrl Pts',(4.23256664799994,2.2,1.20731636599999));
#344385=CARTESIAN_POINT('Ctrl Pts',(4.23411499399994,12.2,1.20865322199998));
#344386=CARTESIAN_POINT('Ctrl Pts',(4.23411499399994,5.2,1.20865322199998));
#344387=CARTESIAN_POINT('Ctrl Pts',(4.23411499399994,2.2,1.20865322199998));
#344388=CARTESIAN_POINT('Ctrl Pts',(4.23566490199994,12.2,1.20999441399999));
#344389=CARTESIAN_POINT('Ctrl Pts',(4.23566490199994,5.2,1.20999441399999));
#344390=CARTESIAN_POINT('Ctrl Pts',(4.23566490199994,2.2,1.20999441399999));
#344391=CARTESIAN_POINT('Ctrl Pts',(4.23721636099994,12.2,1.21133994699999));
#344392=CARTESIAN_POINT('Ctrl Pts',(4.23721636099994,5.2,1.21133994699999));
#344393=CARTESIAN_POINT('Ctrl Pts',(4.23721636099994,2.2,1.21133994699999));
#344394=CARTESIAN_POINT('Ctrl Pts',(4.23876935899994,12.2,1.21268981999998));
#344395=CARTESIAN_POINT('Ctrl Pts',(4.23876935899994,5.2,1.21268981999998));
#344396=CARTESIAN_POINT('Ctrl Pts',(4.23876935899994,2.2,1.21268981999998));
#344397=CARTESIAN_POINT('Ctrl Pts',(4.24032388699994,12.2,1.21404403499998));
#344398=CARTESIAN_POINT('Ctrl Pts',(4.24032388699994,5.2,1.21404403499998));
#344399=CARTESIAN_POINT('Ctrl Pts',(4.24032388699994,2.2,1.21404403499998));
#344400=CARTESIAN_POINT('Ctrl Pts',(4.24187993299994,12.2,1.21540259199998));
#344401=CARTESIAN_POINT('Ctrl Pts',(4.24187993299994,5.2,1.21540259199998));
#344402=CARTESIAN_POINT('Ctrl Pts',(4.24187993299994,2.2,1.21540259199998));
#344403=CARTESIAN_POINT('Ctrl Pts',(4.24343748699994,12.2,1.21676549299998));
#344404=CARTESIAN_POINT('Ctrl Pts',(4.24343748699994,5.2,1.21676549299998));
#344405=CARTESIAN_POINT('Ctrl Pts',(4.24343748699994,2.2,1.21676549299998));
#344406=CARTESIAN_POINT('Ctrl Pts',(4.24499653899994,12.2,1.21813273999999));
#344407=CARTESIAN_POINT('Ctrl Pts',(4.24499653899994,5.2,1.21813273999999));
#344408=CARTESIAN_POINT('Ctrl Pts',(4.24499653899994,2.2,1.21813273999999));
#344409=CARTESIAN_POINT('Ctrl Pts',(4.24655707799994,12.2,1.21950433399999));
#344410=CARTESIAN_POINT('Ctrl Pts',(4.24655707799994,5.2,1.21950433399999));
#344411=CARTESIAN_POINT('Ctrl Pts',(4.24655707799994,2.2,1.21950433399999));
#344412=CARTESIAN_POINT('Ctrl Pts',(4.24811909399994,12.2,1.22088027599998));
#344413=CARTESIAN_POINT('Ctrl Pts',(4.24811909399994,5.2,1.22088027599998));
#344414=CARTESIAN_POINT('Ctrl Pts',(4.24811909399994,2.2,1.22088027599998));
#344415=CARTESIAN_POINT('Ctrl Pts',(4.24968257599994,12.2,1.22226056599999));
#344416=CARTESIAN_POINT('Ctrl Pts',(4.24968257599994,5.2,1.22226056599999));
#344417=CARTESIAN_POINT('Ctrl Pts',(4.24968257599994,2.2,1.22226056599999));
#344418=CARTESIAN_POINT('Ctrl Pts',(4.25124751399994,12.2,1.22364520699998));
#344419=CARTESIAN_POINT('Ctrl Pts',(4.25124751399994,5.2,1.22364520699998));
#344420=CARTESIAN_POINT('Ctrl Pts',(4.25124751399994,2.2,1.22364520699998));
#344421=CARTESIAN_POINT('Ctrl Pts',(4.25281389699994,12.2,1.22503419899999));
#344422=CARTESIAN_POINT('Ctrl Pts',(4.25281389699994,5.2,1.22503419899999));
#344423=CARTESIAN_POINT('Ctrl Pts',(4.25281389699994,2.2,1.22503419899999));
#344424=CARTESIAN_POINT('Ctrl Pts',(4.25438171499994,12.2,1.22642754299998));
#344425=CARTESIAN_POINT('Ctrl Pts',(4.25438171499994,5.2,1.22642754299998));
#344426=CARTESIAN_POINT('Ctrl Pts',(4.25438171499994,2.2,1.22642754299998));
#344427=CARTESIAN_POINT('Ctrl Pts',(4.25595095699994,12.2,1.22782524099998));
#344428=CARTESIAN_POINT('Ctrl Pts',(4.25595095699994,5.2,1.22782524099998));
#344429=CARTESIAN_POINT('Ctrl Pts',(4.25595095699994,2.2,1.22782524099998));
#344430=CARTESIAN_POINT('Ctrl Pts',(4.25752161399994,12.2,1.22922729499999));
#344431=CARTESIAN_POINT('Ctrl Pts',(4.25752161399994,5.2,1.22922729499999));
#344432=CARTESIAN_POINT('Ctrl Pts',(4.25752161399994,2.2,1.22922729499999));
#344433=CARTESIAN_POINT('Ctrl Pts',(4.25909367399994,12.2,1.23063370299999));
#344434=CARTESIAN_POINT('Ctrl Pts',(4.25909367399994,5.2,1.23063370299999));
#344435=CARTESIAN_POINT('Ctrl Pts',(4.25909367399994,2.2,1.23063370299999));
#344436=CARTESIAN_POINT('Ctrl Pts',(4.26066712699994,12.2,1.23204446899999));
#344437=CARTESIAN_POINT('Ctrl Pts',(4.26066712699994,5.2,1.23204446899999));
#344438=CARTESIAN_POINT('Ctrl Pts',(4.26066712699994,2.2,1.23204446899999));
#344439=CARTESIAN_POINT('Ctrl Pts',(4.26224196399995,12.2,1.23345959199999));
#344440=CARTESIAN_POINT('Ctrl Pts',(4.26224196399995,5.2,1.23345959199999));
#344441=CARTESIAN_POINT('Ctrl Pts',(4.26224196399995,2.2,1.23345959199999));
#344442=CARTESIAN_POINT('Ctrl Pts',(4.26381817199994,12.2,1.23487907399999));
#344443=CARTESIAN_POINT('Ctrl Pts',(4.26381817199994,5.2,1.23487907399999));
#344444=CARTESIAN_POINT('Ctrl Pts',(4.26381817199994,2.2,1.23487907399999));
#344445=CARTESIAN_POINT('Ctrl Pts',(4.26539574399994,12.2,1.23630291699998));
#344446=CARTESIAN_POINT('Ctrl Pts',(4.26539574399994,5.2,1.23630291699998));
#344447=CARTESIAN_POINT('Ctrl Pts',(4.26539574399994,2.2,1.23630291699998));
#344448=CARTESIAN_POINT('Ctrl Pts',(4.26697466699994,12.2,1.23773111999999));
#344449=CARTESIAN_POINT('Ctrl Pts',(4.26697466699994,5.2,1.23773111999999));
#344450=CARTESIAN_POINT('Ctrl Pts',(4.26697466699994,2.2,1.23773111999999));
#344451=CARTESIAN_POINT('Ctrl Pts',(4.26855493199994,12.2,1.23916368499998));
#344452=CARTESIAN_POINT('Ctrl Pts',(4.26855493199994,5.2,1.23916368499998));
#344453=CARTESIAN_POINT('Ctrl Pts',(4.26855493199994,2.2,1.23916368499998));
#344454=CARTESIAN_POINT('Ctrl Pts',(4.27013652799995,12.2,1.24060061399998));
#344455=CARTESIAN_POINT('Ctrl Pts',(4.27013652799995,5.2,1.24060061399998));
#344456=CARTESIAN_POINT('Ctrl Pts',(4.27013652799995,2.2,1.24060061399998));
#344457=CARTESIAN_POINT('Ctrl Pts',(4.27171944499994,12.2,1.24204190499999));
#344458=CARTESIAN_POINT('Ctrl Pts',(4.27171944499994,5.2,1.24204190499999));
#344459=CARTESIAN_POINT('Ctrl Pts',(4.27171944499994,2.2,1.24204190499999));
#344460=CARTESIAN_POINT('Ctrl Pts',(4.27330367199994,12.2,1.24348756299999));
#344461=CARTESIAN_POINT('Ctrl Pts',(4.27330367199994,5.2,1.24348756299999));
#344462=CARTESIAN_POINT('Ctrl Pts',(4.27330367199994,2.2,1.24348756299999));
#344463=CARTESIAN_POINT('Ctrl Pts',(4.27488920099994,12.2,1.24493758599999));
#344464=CARTESIAN_POINT('Ctrl Pts',(4.27488920099994,5.2,1.24493758599999));
#344465=CARTESIAN_POINT('Ctrl Pts',(4.27488920099994,2.2,1.24493758599999));
#344466=CARTESIAN_POINT('Ctrl Pts',(4.27647601999994,12.2,1.24639197499999));
#344467=CARTESIAN_POINT('Ctrl Pts',(4.27647601999994,5.2,1.24639197499999));
#344468=CARTESIAN_POINT('Ctrl Pts',(4.27647601999994,2.2,1.24639197499999));
#344469=CARTESIAN_POINT('Ctrl Pts',(4.27806411899994,12.2,1.24785073299998));
#344470=CARTESIAN_POINT('Ctrl Pts',(4.27806411899994,5.2,1.24785073299998));
#344471=CARTESIAN_POINT('Ctrl Pts',(4.27806411899994,2.2,1.24785073299998));
#344472=CARTESIAN_POINT('Ctrl Pts',(4.27965348699994,12.2,1.24931385799998));
#344473=CARTESIAN_POINT('Ctrl Pts',(4.27965348699994,5.2,1.24931385799998));
#344474=CARTESIAN_POINT('Ctrl Pts',(4.27965348699994,2.2,1.24931385799998));
#344475=CARTESIAN_POINT('Ctrl Pts',(4.28124411599994,12.2,1.25078135299999));
#344476=CARTESIAN_POINT('Ctrl Pts',(4.28124411599994,5.2,1.25078135299999));
#344477=CARTESIAN_POINT('Ctrl Pts',(4.28124411599994,2.2,1.25078135299999));
#344478=CARTESIAN_POINT('Ctrl Pts',(4.28283599299994,12.2,1.25225321799999));
#344479=CARTESIAN_POINT('Ctrl Pts',(4.28283599299994,5.2,1.25225321799999));
#344480=CARTESIAN_POINT('Ctrl Pts',(4.28283599299994,2.2,1.25225321799999));
#344481=CARTESIAN_POINT('Ctrl Pts',(4.28442910999994,12.2,1.25372945399999));
#344482=CARTESIAN_POINT('Ctrl Pts',(4.28442910999994,5.2,1.25372945399999));
#344483=CARTESIAN_POINT('Ctrl Pts',(4.28442910999994,2.2,1.25372945399999));
#344484=CARTESIAN_POINT('Ctrl Pts',(4.28602345699994,12.2,1.25521006299998));
#344485=CARTESIAN_POINT('Ctrl Pts',(4.28602345699994,5.2,1.25521006299998));
#344486=CARTESIAN_POINT('Ctrl Pts',(4.28602345699994,2.2,1.25521006299998));
#344487=CARTESIAN_POINT('Ctrl Pts',(4.28761902199995,12.2,1.25669504399998));
#344488=CARTESIAN_POINT('Ctrl Pts',(4.28761902199995,5.2,1.25669504399998));
#344489=CARTESIAN_POINT('Ctrl Pts',(4.28761902199995,2.2,1.25669504399998));
#344490=CARTESIAN_POINT('Ctrl Pts',(4.28921579599994,12.2,1.25818439799998));
#344491=CARTESIAN_POINT('Ctrl Pts',(4.28921579599994,5.2,1.25818439799998));
#344492=CARTESIAN_POINT('Ctrl Pts',(4.28921579599994,2.2,1.25818439799998));
#344493=CARTESIAN_POINT('Ctrl Pts',(4.29081376899994,12.2,1.25967812699999));
#344494=CARTESIAN_POINT('Ctrl Pts',(4.29081376899994,5.2,1.25967812699999));
#344495=CARTESIAN_POINT('Ctrl Pts',(4.29081376899994,2.2,1.25967812699999));
#344496=CARTESIAN_POINT('Ctrl Pts',(4.29241293099994,12.2,1.26117623099999));
#344497=CARTESIAN_POINT('Ctrl Pts',(4.29241293099994,5.2,1.26117623099999));
#344498=CARTESIAN_POINT('Ctrl Pts',(4.29241293099994,2.2,1.26117623099999));
#344499=CARTESIAN_POINT('Ctrl Pts',(4.29401327199994,12.2,1.26267870999999));
#344500=CARTESIAN_POINT('Ctrl Pts',(4.29401327199994,5.2,1.26267870999999));
#344501=CARTESIAN_POINT('Ctrl Pts',(4.29401327199994,2.2,1.26267870999999));
#344502=CARTESIAN_POINT('Ctrl Pts',(4.29561478099994,12.2,1.26418556599999));
#344503=CARTESIAN_POINT('Ctrl Pts',(4.29561478099994,5.2,1.26418556599999));
#344504=CARTESIAN_POINT('Ctrl Pts',(4.29561478099994,2.2,1.26418556599999));
#344505=CARTESIAN_POINT('Ctrl Pts',(4.29721744799994,12.2,1.26569679999998));
#344506=CARTESIAN_POINT('Ctrl Pts',(4.29721744799994,5.2,1.26569679999998));
#344507=CARTESIAN_POINT('Ctrl Pts',(4.29721744799994,2.2,1.26569679999998));
#344508=CARTESIAN_POINT('Ctrl Pts',(4.29882126499994,12.2,1.26721241099998));
#344509=CARTESIAN_POINT('Ctrl Pts',(4.29882126499994,5.2,1.26721241099998));
#344510=CARTESIAN_POINT('Ctrl Pts',(4.29882126499994,2.2,1.26721241099998));
#344511=CARTESIAN_POINT('Ctrl Pts',(4.30042621899995,12.2,1.26873239999998));
#344512=CARTESIAN_POINT('Ctrl Pts',(4.30042621899995,5.2,1.26873239999998));
#344513=CARTESIAN_POINT('Ctrl Pts',(4.30042621899995,2.2,1.26873239999998));
#344514=CARTESIAN_POINT('Ctrl Pts',(4.30203230199994,12.2,1.27025676999999));
#344515=CARTESIAN_POINT('Ctrl Pts',(4.30203230199994,5.2,1.27025676999999));
#344516=CARTESIAN_POINT('Ctrl Pts',(4.30203230199994,2.2,1.27025676999999));
#344517=CARTESIAN_POINT('Ctrl Pts',(4.30363950299994,12.2,1.27178551899998));
#344518=CARTESIAN_POINT('Ctrl Pts',(4.30363950299994,5.2,1.27178551899998));
#344519=CARTESIAN_POINT('Ctrl Pts',(4.30363950299994,2.2,1.27178551899998));
#344520=CARTESIAN_POINT('Ctrl Pts',(4.30524781299995,12.2,1.27331864799999));
#344521=CARTESIAN_POINT('Ctrl Pts',(4.30524781299995,5.2,1.27331864799999));
#344522=CARTESIAN_POINT('Ctrl Pts',(4.30524781299995,2.2,1.27331864799999));
#344523=CARTESIAN_POINT('Ctrl Pts',(4.30685722099994,12.2,1.27485615899999));
#344524=CARTESIAN_POINT('Ctrl Pts',(4.30685722099994,5.2,1.27485615899999));
#344525=CARTESIAN_POINT('Ctrl Pts',(4.30685722099994,2.2,1.27485615899999));
#344526=CARTESIAN_POINT('Ctrl Pts',(4.30846771799995,12.2,1.27639805199999));
#344527=CARTESIAN_POINT('Ctrl Pts',(4.30846771799995,5.2,1.27639805199999));
#344528=CARTESIAN_POINT('Ctrl Pts',(4.30846771799995,2.2,1.27639805199999));
#344529=CARTESIAN_POINT('Ctrl Pts',(4.31007929299995,12.2,1.27794432699998));
#344530=CARTESIAN_POINT('Ctrl Pts',(4.31007929299995,5.2,1.27794432699998));
#344531=CARTESIAN_POINT('Ctrl Pts',(4.31007929299995,2.2,1.27794432699998));
#344532=CARTESIAN_POINT('Ctrl Pts',(4.31169193699994,12.2,1.27949498499999));
#344533=CARTESIAN_POINT('Ctrl Pts',(4.31169193699994,5.2,1.27949498499999));
#344534=CARTESIAN_POINT('Ctrl Pts',(4.31169193699994,2.2,1.27949498499999));
#344535=CARTESIAN_POINT('Ctrl Pts',(4.31330563999994,12.2,1.28105002699999));
#344536=CARTESIAN_POINT('Ctrl Pts',(4.31330563999994,5.2,1.28105002699999));
#344537=CARTESIAN_POINT('Ctrl Pts',(4.31330563999994,2.2,1.28105002699999));
#344538=CARTESIAN_POINT('Ctrl Pts',(4.31492039099994,12.2,1.28260945399999));
#344539=CARTESIAN_POINT('Ctrl Pts',(4.31492039099994,5.2,1.28260945399999));
#344540=CARTESIAN_POINT('Ctrl Pts',(4.31492039099994,2.2,1.28260945399999));
#344541=CARTESIAN_POINT('Ctrl Pts',(4.31653618199995,12.2,1.28417326399999));
#344542=CARTESIAN_POINT('Ctrl Pts',(4.31653618199995,5.2,1.28417326399999));
#344543=CARTESIAN_POINT('Ctrl Pts',(4.31653618199995,2.2,1.28417326399999));
#344544=CARTESIAN_POINT('Ctrl Pts',(4.31815299999994,12.2,1.28574145999998));
#344545=CARTESIAN_POINT('Ctrl Pts',(4.31815299999994,5.2,1.28574145999998));
#344546=CARTESIAN_POINT('Ctrl Pts',(4.31815299999994,2.2,1.28574145999998));
#344547=CARTESIAN_POINT('Ctrl Pts',(4.31977083899994,12.2,1.28731404199999));
#344548=CARTESIAN_POINT('Ctrl Pts',(4.31977083899994,5.2,1.28731404199999));
#344549=CARTESIAN_POINT('Ctrl Pts',(4.31977083899994,2.2,1.28731404199999));
#344550=CARTESIAN_POINT('Ctrl Pts',(4.32138968599994,12.2,1.28889100999999));
#344551=CARTESIAN_POINT('Ctrl Pts',(4.32138968599994,5.2,1.28889100999999));
#344552=CARTESIAN_POINT('Ctrl Pts',(4.32138968599994,2.2,1.28889100999999));
#344553=CARTESIAN_POINT('Ctrl Pts',(4.32300953299994,12.2,1.29047236499999));
#344554=CARTESIAN_POINT('Ctrl Pts',(4.32300953299994,5.2,1.29047236499999));
#344555=CARTESIAN_POINT('Ctrl Pts',(4.32300953299994,2.2,1.29047236499999));
#344556=CARTESIAN_POINT('Ctrl Pts',(4.32463036999994,12.2,1.29205810699998));
#344557=CARTESIAN_POINT('Ctrl Pts',(4.32463036999994,5.2,1.29205810699998));
#344558=CARTESIAN_POINT('Ctrl Pts',(4.32463036999994,2.2,1.29205810699998));
#344559=CARTESIAN_POINT('Ctrl Pts',(4.32625218699994,12.2,1.29364823599999));
#344560=CARTESIAN_POINT('Ctrl Pts',(4.32625218699994,5.2,1.29364823599999));
#344561=CARTESIAN_POINT('Ctrl Pts',(4.32625218699994,2.2,1.29364823599999));
#344562=CARTESIAN_POINT('Ctrl Pts',(4.32787497299994,12.2,1.29524275399998));
#344563=CARTESIAN_POINT('Ctrl Pts',(4.32787497299994,5.2,1.29524275399998));
#344564=CARTESIAN_POINT('Ctrl Pts',(4.32787497299994,2.2,1.29524275399998));
#344565=CARTESIAN_POINT('Ctrl Pts',(4.32949871899994,12.2,1.29684166099999));
#344566=CARTESIAN_POINT('Ctrl Pts',(4.32949871899994,5.2,1.29684166099999));
#344567=CARTESIAN_POINT('Ctrl Pts',(4.32949871899994,2.2,1.29684166099999));
#344568=CARTESIAN_POINT('Ctrl Pts',(4.33112341699994,12.2,1.29844495599999));
#344569=CARTESIAN_POINT('Ctrl Pts',(4.33112341699994,5.2,1.29844495599999));
#344570=CARTESIAN_POINT('Ctrl Pts',(4.33112341699994,2.2,1.29844495599999));
#344571=CARTESIAN_POINT('Ctrl Pts',(4.33274905499994,12.2,1.30005264099998));
#344572=CARTESIAN_POINT('Ctrl Pts',(4.33274905499994,5.2,1.30005264099998));
#344573=CARTESIAN_POINT('Ctrl Pts',(4.33274905499994,2.2,1.30005264099998));
#344574=CARTESIAN_POINT('Ctrl Pts',(4.33437562399994,12.2,1.30166471499999));
#344575=CARTESIAN_POINT('Ctrl Pts',(4.33437562399994,5.2,1.30166471499999));
#344576=CARTESIAN_POINT('Ctrl Pts',(4.33437562399994,2.2,1.30166471499999));
#344577=CARTESIAN_POINT('Ctrl Pts',(4.33600311299995,12.2,1.30328117999999));
#344578=CARTESIAN_POINT('Ctrl Pts',(4.33600311299995,5.2,1.30328117999999));
#344579=CARTESIAN_POINT('Ctrl Pts',(4.33600311299995,2.2,1.30328117999999));
#344580=CARTESIAN_POINT('Ctrl Pts',(4.33763151499994,12.2,1.30490203499999));
#344581=CARTESIAN_POINT('Ctrl Pts',(4.33763151499994,5.2,1.30490203499999));
#344582=CARTESIAN_POINT('Ctrl Pts',(4.33763151499994,2.2,1.30490203499999));
#344583=CARTESIAN_POINT('Ctrl Pts',(4.33926081799994,12.2,1.30652727999998));
#344584=CARTESIAN_POINT('Ctrl Pts',(4.33926081799994,5.2,1.30652727999998));
#344585=CARTESIAN_POINT('Ctrl Pts',(4.33926081799994,2.2,1.30652727999998));
#344586=CARTESIAN_POINT('Ctrl Pts',(4.34089101299994,12.2,1.30815691799999));
#344587=CARTESIAN_POINT('Ctrl Pts',(4.34089101299994,5.2,1.30815691799999));
#344588=CARTESIAN_POINT('Ctrl Pts',(4.34089101299994,2.2,1.30815691799999));
#344589=CARTESIAN_POINT('Ctrl Pts',(4.34252208999994,12.2,1.30979094599999));
#344590=CARTESIAN_POINT('Ctrl Pts',(4.34252208999994,5.2,1.30979094599999));
#344591=CARTESIAN_POINT('Ctrl Pts',(4.34252208999994,2.2,1.30979094599999));
#344592=CARTESIAN_POINT('Ctrl Pts',(4.34415404099994,12.2,1.31142936699999));
#344593=CARTESIAN_POINT('Ctrl Pts',(4.34415404099994,5.2,1.31142936699999));
#344594=CARTESIAN_POINT('Ctrl Pts',(4.34415404099994,2.2,1.31142936699999));
#344595=CARTESIAN_POINT('Ctrl Pts',(4.34578685399994,12.2,1.31307217999999));
#344596=CARTESIAN_POINT('Ctrl Pts',(4.34578685399994,5.2,1.31307217999999));
#344597=CARTESIAN_POINT('Ctrl Pts',(4.34578685399994,2.2,1.31307217999999));
#344598=CARTESIAN_POINT('Ctrl Pts',(4.34742051999994,12.2,1.31471938499998));
#344599=CARTESIAN_POINT('Ctrl Pts',(4.34742051999994,5.2,1.31471938499998));
#344600=CARTESIAN_POINT('Ctrl Pts',(4.34742051999994,2.2,1.31471938499998));
#344601=CARTESIAN_POINT('Ctrl Pts',(4.34905503099994,12.2,1.31637098199999));
#344602=CARTESIAN_POINT('Ctrl Pts',(4.34905503099994,5.2,1.31637098199999));
#344603=CARTESIAN_POINT('Ctrl Pts',(4.34905503099994,2.2,1.31637098199999));
#344604=CARTESIAN_POINT('Ctrl Pts',(4.35069037499995,12.2,1.31802697399999));
#344605=CARTESIAN_POINT('Ctrl Pts',(4.35069037499995,5.2,1.31802697399999));
#344606=CARTESIAN_POINT('Ctrl Pts',(4.35069037499995,2.2,1.31802697399999));
#344607=CARTESIAN_POINT('Ctrl Pts',(4.35232654399995,12.2,1.31968735699999));
#344608=CARTESIAN_POINT('Ctrl Pts',(4.35232654399995,5.2,1.31968735699999));
#344609=CARTESIAN_POINT('Ctrl Pts',(4.35232654399995,2.2,1.31968735699999));
#344610=CARTESIAN_POINT('Ctrl Pts',(4.35396352699995,12.2,1.32135213299998));
#344611=CARTESIAN_POINT('Ctrl Pts',(4.35396352699995,5.2,1.32135213299998));
#344612=CARTESIAN_POINT('Ctrl Pts',(4.35396352699995,2.2,1.32135213299998));
#344613=CARTESIAN_POINT('Ctrl Pts',(4.35560131699994,12.2,1.32302130499999));
#344614=CARTESIAN_POINT('Ctrl Pts',(4.35560131699994,5.2,1.32302130499999));
#344615=CARTESIAN_POINT('Ctrl Pts',(4.35560131699994,2.2,1.32302130499999));
#344616=CARTESIAN_POINT('Ctrl Pts',(4.35723990199994,12.2,1.32469486899998));
#344617=CARTESIAN_POINT('Ctrl Pts',(4.35723990199994,5.2,1.32469486899998));
#344618=CARTESIAN_POINT('Ctrl Pts',(4.35723990199994,2.2,1.32469486899998));
#344619=CARTESIAN_POINT('Ctrl Pts',(4.35887927299994,12.2,1.32637282699998));
#344620=CARTESIAN_POINT('Ctrl Pts',(4.35887927299994,5.2,1.32637282699998));
#344621=CARTESIAN_POINT('Ctrl Pts',(4.35887927299994,2.2,1.32637282699998));
#344622=CARTESIAN_POINT('Ctrl Pts',(4.36051941999995,12.2,1.32805517999998));
#344623=CARTESIAN_POINT('Ctrl Pts',(4.36051941999995,5.2,1.32805517999998));
#344624=CARTESIAN_POINT('Ctrl Pts',(4.36051941999995,2.2,1.32805517999998));
#344625=CARTESIAN_POINT('Ctrl Pts',(4.36216033499994,12.2,1.32974192599999));
#344626=CARTESIAN_POINT('Ctrl Pts',(4.36216033499994,5.2,1.32974192599999));
#344627=CARTESIAN_POINT('Ctrl Pts',(4.36216033499994,2.2,1.32974192599999));
#344628=CARTESIAN_POINT('Ctrl Pts',(4.36380200799994,12.2,1.33143306799999));
#344629=CARTESIAN_POINT('Ctrl Pts',(4.36380200799994,5.2,1.33143306799999));
#344630=CARTESIAN_POINT('Ctrl Pts',(4.36380200799994,2.2,1.33143306799999));
#344631=CARTESIAN_POINT('Ctrl Pts',(4.36544442799994,12.2,1.33312860399998));
#344632=CARTESIAN_POINT('Ctrl Pts',(4.36544442799994,5.2,1.33312860399998));
#344633=CARTESIAN_POINT('Ctrl Pts',(4.36544442799994,2.2,1.33312860399998));
#344634=CARTESIAN_POINT('Ctrl Pts',(4.36708758799994,12.2,1.33482853399999));
#344635=CARTESIAN_POINT('Ctrl Pts',(4.36708758799994,5.2,1.33482853399999));
#344636=CARTESIAN_POINT('Ctrl Pts',(4.36708758799994,2.2,1.33482853399999));
#344637=CARTESIAN_POINT('Ctrl Pts',(4.36873147599994,12.2,1.33653285899999));
#344638=CARTESIAN_POINT('Ctrl Pts',(4.36873147599994,5.2,1.33653285899999));
#344639=CARTESIAN_POINT('Ctrl Pts',(4.36873147599994,2.2,1.33653285899999));
#344640=CARTESIAN_POINT('Ctrl Pts',(4.37037608399994,12.2,1.33824157899999));
#344641=CARTESIAN_POINT('Ctrl Pts',(4.37037608399994,5.2,1.33824157899999));
#344642=CARTESIAN_POINT('Ctrl Pts',(4.37037608399994,2.2,1.33824157899999));
#344643=CARTESIAN_POINT('Ctrl Pts',(4.37202140199994,12.2,1.33995469399999));
#344644=CARTESIAN_POINT('Ctrl Pts',(4.37202140199994,5.2,1.33995469399999));
#344645=CARTESIAN_POINT('Ctrl Pts',(4.37202140199994,2.2,1.33995469399999));
#344646=CARTESIAN_POINT('Ctrl Pts',(4.37366742099994,12.2,1.34167220399998));
#344647=CARTESIAN_POINT('Ctrl Pts',(4.37366742099994,5.2,1.34167220399998));
#344648=CARTESIAN_POINT('Ctrl Pts',(4.37366742099994,2.2,1.34167220399998));
#344649=CARTESIAN_POINT('Ctrl Pts',(4.37531413099994,12.2,1.34339410999999));
#344650=CARTESIAN_POINT('Ctrl Pts',(4.37531413099994,5.2,1.34339410999999));
#344651=CARTESIAN_POINT('Ctrl Pts',(4.37531413099994,2.2,1.34339410999999));
#344652=CARTESIAN_POINT('Ctrl Pts',(4.37696152299995,12.2,1.34512040999998));
#344653=CARTESIAN_POINT('Ctrl Pts',(4.37696152299995,5.2,1.34512040999998));
#344654=CARTESIAN_POINT('Ctrl Pts',(4.37696152299995,2.2,1.34512040999998));
#344655=CARTESIAN_POINT('Ctrl Pts',(4.37860958799994,12.2,1.34685110599999));
#344656=CARTESIAN_POINT('Ctrl Pts',(4.37860958799994,5.2,1.34685110599999));
#344657=CARTESIAN_POINT('Ctrl Pts',(4.37860958799994,2.2,1.34685110599999));
#344658=CARTESIAN_POINT('Ctrl Pts',(4.38025831499994,12.2,1.34858619499999));
#344659=CARTESIAN_POINT('Ctrl Pts',(4.38025831499994,5.2,1.34858619499999));
#344660=CARTESIAN_POINT('Ctrl Pts',(4.38025831499994,2.2,1.34858619499999));
#344661=CARTESIAN_POINT('Ctrl Pts',(4.38190769699994,12.2,1.35032568199998));
#344662=CARTESIAN_POINT('Ctrl Pts',(4.38190769699994,5.2,1.35032568199998));
#344663=CARTESIAN_POINT('Ctrl Pts',(4.38190769699994,2.2,1.35032568199998));
#344664=CARTESIAN_POINT('Ctrl Pts',(4.38355772299994,12.2,1.35206956199998));
#344665=CARTESIAN_POINT('Ctrl Pts',(4.38355772299994,5.2,1.35206956199998));
#344666=CARTESIAN_POINT('Ctrl Pts',(4.38355772299994,2.2,1.35206956199998));
#344667=CARTESIAN_POINT('Ctrl Pts',(4.38520838299994,12.2,1.35381783799998));
#344668=CARTESIAN_POINT('Ctrl Pts',(4.38520838299994,5.2,1.35381783799998));
#344669=CARTESIAN_POINT('Ctrl Pts',(4.38520838299994,2.2,1.35381783799998));
#344670=CARTESIAN_POINT('Ctrl Pts',(4.38685966999994,12.2,1.35557050899999));
#344671=CARTESIAN_POINT('Ctrl Pts',(4.38685966999994,5.2,1.35557050899999));
#344672=CARTESIAN_POINT('Ctrl Pts',(4.38685966999994,2.2,1.35557050899999));
#344673=CARTESIAN_POINT('Ctrl Pts',(4.38851157199994,12.2,1.35732757499999));
#344674=CARTESIAN_POINT('Ctrl Pts',(4.38851157199994,5.2,1.35732757499999));
#344675=CARTESIAN_POINT('Ctrl Pts',(4.38851157199994,2.2,1.35732757499999));
#344676=CARTESIAN_POINT('Ctrl Pts',(4.39016408099994,12.2,1.35908903699999));
#344677=CARTESIAN_POINT('Ctrl Pts',(4.39016408099994,5.2,1.35908903699999));
#344678=CARTESIAN_POINT('Ctrl Pts',(4.39016408099994,2.2,1.35908903699999));
#344679=CARTESIAN_POINT('Ctrl Pts',(4.39181718799994,12.2,1.36085489299999));
#344680=CARTESIAN_POINT('Ctrl Pts',(4.39181718799994,5.2,1.36085489299999));
#344681=CARTESIAN_POINT('Ctrl Pts',(4.39181718799994,2.2,1.36085489299999));
#344682=CARTESIAN_POINT('Ctrl Pts',(4.39347088399995,12.2,1.36262514299998));
#344683=CARTESIAN_POINT('Ctrl Pts',(4.39347088399995,5.2,1.36262514299998));
#344684=CARTESIAN_POINT('Ctrl Pts',(4.39347088399995,2.2,1.36262514299998));
#344685=CARTESIAN_POINT('Ctrl Pts',(4.39512515799994,12.2,1.36439978799999));
#344686=CARTESIAN_POINT('Ctrl Pts',(4.39512515799994,5.2,1.36439978799999));
#344687=CARTESIAN_POINT('Ctrl Pts',(4.39512515799994,2.2,1.36439978799999));
#344688=CARTESIAN_POINT('Ctrl Pts',(4.39678000299994,12.2,1.36617882899999));
#344689=CARTESIAN_POINT('Ctrl Pts',(4.39678000299994,5.2,1.36617882899999));
#344690=CARTESIAN_POINT('Ctrl Pts',(4.39678000299994,2.2,1.36617882899999));
#344691=CARTESIAN_POINT('Ctrl Pts',(4.39843540799994,12.2,1.36796226299999));
#344692=CARTESIAN_POINT('Ctrl Pts',(4.39843540799994,5.2,1.36796226299999));
#344693=CARTESIAN_POINT('Ctrl Pts',(4.39843540799994,2.2,1.36796226299999));
#344694=CARTESIAN_POINT('Ctrl Pts',(4.40009136299994,12.2,1.36975009199999));
#344695=CARTESIAN_POINT('Ctrl Pts',(4.40009136299994,5.2,1.36975009199999));
#344696=CARTESIAN_POINT('Ctrl Pts',(4.40009136299994,2.2,1.36975009199999));
#344697=CARTESIAN_POINT('Ctrl Pts',(4.40174786199994,12.2,1.37154231599999));
#344698=CARTESIAN_POINT('Ctrl Pts',(4.40174786199994,5.2,1.37154231599999));
#344699=CARTESIAN_POINT('Ctrl Pts',(4.40174786199994,2.2,1.37154231599999));
#344700=CARTESIAN_POINT('Ctrl Pts',(4.40340489299994,12.2,1.37333893199999));
#344701=CARTESIAN_POINT('Ctrl Pts',(4.40340489299994,5.2,1.37333893199999));
#344702=CARTESIAN_POINT('Ctrl Pts',(4.40340489299994,2.2,1.37333893199999));
#344703=CARTESIAN_POINT('Ctrl Pts',(4.40506244799994,12.2,1.37513994299999));
#344704=CARTESIAN_POINT('Ctrl Pts',(4.40506244799994,5.2,1.37513994299999));
#344705=CARTESIAN_POINT('Ctrl Pts',(4.40506244799994,2.2,1.37513994299999));
#344706=CARTESIAN_POINT('Ctrl Pts',(4.40672051699995,12.2,1.37694534799999));
#344707=CARTESIAN_POINT('Ctrl Pts',(4.40672051699995,5.2,1.37694534799999));
#344708=CARTESIAN_POINT('Ctrl Pts',(4.40672051699995,2.2,1.37694534799999));
#344709=CARTESIAN_POINT('Ctrl Pts',(4.40837909099994,12.2,1.37875514499999));
#344710=CARTESIAN_POINT('Ctrl Pts',(4.40837909099994,5.2,1.37875514499999));
#344711=CARTESIAN_POINT('Ctrl Pts',(4.40837909099994,2.2,1.37875514499999));
#344712=CARTESIAN_POINT('Ctrl Pts',(4.41003816199994,12.2,1.38056933699998));
#344713=CARTESIAN_POINT('Ctrl Pts',(4.41003816199994,5.2,1.38056933699998));
#344714=CARTESIAN_POINT('Ctrl Pts',(4.41003816199994,2.2,1.38056933699998));
#344715=CARTESIAN_POINT('Ctrl Pts',(4.41169771899994,12.2,1.38238792099999));
#344716=CARTESIAN_POINT('Ctrl Pts',(4.41169771899994,5.2,1.38238792099999));
#344717=CARTESIAN_POINT('Ctrl Pts',(4.41169771899994,2.2,1.38238792099999));
#344718=CARTESIAN_POINT('Ctrl Pts',(4.41335775399994,12.2,1.38421089799999));
#344719=CARTESIAN_POINT('Ctrl Pts',(4.41335775399994,5.2,1.38421089799999));
#344720=CARTESIAN_POINT('Ctrl Pts',(4.41335775399994,2.2,1.38421089799999));
#344721=CARTESIAN_POINT('Ctrl Pts',(4.41501825699994,12.2,1.38603826799998));
#344722=CARTESIAN_POINT('Ctrl Pts',(4.41501825699994,5.2,1.38603826799998));
#344723=CARTESIAN_POINT('Ctrl Pts',(4.41501825699994,2.2,1.38603826799998));
#344724=CARTESIAN_POINT('Ctrl Pts',(4.41667922099994,12.2,1.38787002999999));
#344725=CARTESIAN_POINT('Ctrl Pts',(4.41667922099994,5.2,1.38787002999999));
#344726=CARTESIAN_POINT('Ctrl Pts',(4.41667922099994,2.2,1.38787002999999));
#344727=CARTESIAN_POINT('Ctrl Pts',(4.41834063399994,12.2,1.38970618399998));
#344728=CARTESIAN_POINT('Ctrl Pts',(4.41834063399994,5.2,1.38970618399998));
#344729=CARTESIAN_POINT('Ctrl Pts',(4.41834063399994,2.2,1.38970618399998));
#344730=CARTESIAN_POINT('Ctrl Pts',(4.42000248799994,12.2,1.39154672899998));
#344731=CARTESIAN_POINT('Ctrl Pts',(4.42000248799994,5.2,1.39154672899998));
#344732=CARTESIAN_POINT('Ctrl Pts',(4.42000248799994,2.2,1.39154672899998));
#344733=CARTESIAN_POINT('Ctrl Pts',(4.42166477499994,12.2,1.39339166599999));
#344734=CARTESIAN_POINT('Ctrl Pts',(4.42166477499994,5.2,1.39339166599999));
#344735=CARTESIAN_POINT('Ctrl Pts',(4.42166477499994,2.2,1.39339166599999));
#344736=CARTESIAN_POINT('Ctrl Pts',(4.42332748499994,12.2,1.39524099499999));
#344737=CARTESIAN_POINT('Ctrl Pts',(4.42332748499994,5.2,1.39524099499999));
#344738=CARTESIAN_POINT('Ctrl Pts',(4.42332748499994,2.2,1.39524099499999));
#344739=CARTESIAN_POINT('Ctrl Pts',(4.42499060899994,12.2,1.39709471299998));
#344740=CARTESIAN_POINT('Ctrl Pts',(4.42499060899994,5.2,1.39709471299998));
#344741=CARTESIAN_POINT('Ctrl Pts',(4.42499060899994,2.2,1.39709471299998));
#344742=CARTESIAN_POINT('Ctrl Pts',(4.42665413799994,12.2,1.39895282199999));
#344743=CARTESIAN_POINT('Ctrl Pts',(4.42665413799994,5.2,1.39895282199999));
#344744=CARTESIAN_POINT('Ctrl Pts',(4.42665413799994,2.2,1.39895282199999));
#344745=CARTESIAN_POINT('Ctrl Pts',(4.42831806199994,12.2,1.40081532299998));
#344746=CARTESIAN_POINT('Ctrl Pts',(4.42831806199994,5.2,1.40081532299998));
#344747=CARTESIAN_POINT('Ctrl Pts',(4.42831806199994,2.2,1.40081532299998));
#344748=CARTESIAN_POINT('Ctrl Pts',(4.42998237399994,12.2,1.40268221199999));
#344749=CARTESIAN_POINT('Ctrl Pts',(4.42998237399994,5.2,1.40268221199999));
#344750=CARTESIAN_POINT('Ctrl Pts',(4.42998237399994,2.2,1.40268221199999));
#344751=CARTESIAN_POINT('Ctrl Pts',(4.43164706299994,12.2,1.40455348999998));
#344752=CARTESIAN_POINT('Ctrl Pts',(4.43164706299994,5.2,1.40455348999998));
#344753=CARTESIAN_POINT('Ctrl Pts',(4.43164706299994,2.2,1.40455348999998));
#344754=CARTESIAN_POINT('Ctrl Pts',(4.43331212099995,12.2,1.40642915799999));
#344755=CARTESIAN_POINT('Ctrl Pts',(4.43331212099995,5.2,1.40642915799999));
#344756=CARTESIAN_POINT('Ctrl Pts',(4.43331212099995,2.2,1.40642915799999));
#344757=CARTESIAN_POINT('Ctrl Pts',(4.43497753899995,12.2,1.40830921399999));
#344758=CARTESIAN_POINT('Ctrl Pts',(4.43497753899995,5.2,1.40830921399999));
#344759=CARTESIAN_POINT('Ctrl Pts',(4.43497753899995,2.2,1.40830921399999));
#344760=CARTESIAN_POINT('Ctrl Pts',(4.43664330699994,12.2,1.41019365799998));
#344761=CARTESIAN_POINT('Ctrl Pts',(4.43664330699994,5.2,1.41019365799998));
#344762=CARTESIAN_POINT('Ctrl Pts',(4.43664330699994,2.2,1.41019365799998));
#344763=CARTESIAN_POINT('Ctrl Pts',(4.43830941799995,12.2,1.41208248999999));
#344764=CARTESIAN_POINT('Ctrl Pts',(4.43830941799995,5.2,1.41208248999999));
#344765=CARTESIAN_POINT('Ctrl Pts',(4.43830941799995,2.2,1.41208248999999));
#344766=CARTESIAN_POINT('Ctrl Pts',(4.43997586199994,12.2,1.41397570899999));
#344767=CARTESIAN_POINT('Ctrl Pts',(4.43997586199994,5.2,1.41397570899999));
#344768=CARTESIAN_POINT('Ctrl Pts',(4.43997586199994,2.2,1.41397570899999));
#344769=CARTESIAN_POINT('Ctrl Pts',(4.44164262899994,12.2,1.41587331599998));
#344770=CARTESIAN_POINT('Ctrl Pts',(4.44164262899994,5.2,1.41587331599998));
#344771=CARTESIAN_POINT('Ctrl Pts',(4.44164262899994,2.2,1.41587331599998));
#344772=CARTESIAN_POINT('Ctrl Pts',(4.44330971099994,12.2,1.41777530899999));
#344773=CARTESIAN_POINT('Ctrl Pts',(4.44330971099994,5.2,1.41777530899999));
#344774=CARTESIAN_POINT('Ctrl Pts',(4.44330971099994,2.2,1.41777530899999));
#344775=CARTESIAN_POINT('Ctrl Pts',(4.44497709999994,12.2,1.41968168799998));
#344776=CARTESIAN_POINT('Ctrl Pts',(4.44497709999994,5.2,1.41968168799998));
#344777=CARTESIAN_POINT('Ctrl Pts',(4.44497709999994,2.2,1.41968168799998));
#344778=CARTESIAN_POINT('Ctrl Pts',(4.44664478499995,12.2,1.42159245199998));
#344779=CARTESIAN_POINT('Ctrl Pts',(4.44664478499995,5.2,1.42159245199998));
#344780=CARTESIAN_POINT('Ctrl Pts',(4.44664478499995,2.2,1.42159245199998));
#344781=CARTESIAN_POINT('Ctrl Pts',(4.44831275899995,12.2,1.42350760199998));
#344782=CARTESIAN_POINT('Ctrl Pts',(4.44831275899995,5.2,1.42350760199998));
#344783=CARTESIAN_POINT('Ctrl Pts',(4.44831275899995,2.2,1.42350760199998));
#344784=CARTESIAN_POINT('Ctrl Pts',(4.44998101199995,12.2,1.42542713599998));
#344785=CARTESIAN_POINT('Ctrl Pts',(4.44998101199995,5.2,1.42542713599998));
#344786=CARTESIAN_POINT('Ctrl Pts',(4.44998101199995,2.2,1.42542713599998));
#344787=CARTESIAN_POINT('Ctrl Pts',(4.45164953699994,12.2,1.42735105399999));
#344788=CARTESIAN_POINT('Ctrl Pts',(4.45164953699994,5.2,1.42735105399999));
#344789=CARTESIAN_POINT('Ctrl Pts',(4.45164953699994,2.2,1.42735105399999));
#344790=CARTESIAN_POINT('Ctrl Pts',(4.45331832199995,12.2,1.42927935499999));
#344791=CARTESIAN_POINT('Ctrl Pts',(4.45331832199995,5.2,1.42927935499999));
#344792=CARTESIAN_POINT('Ctrl Pts',(4.45331832199995,2.2,1.42927935499999));
#344793=CARTESIAN_POINT('Ctrl Pts',(4.45498735999994,12.2,1.43121203999999));
#344794=CARTESIAN_POINT('Ctrl Pts',(4.45498735999994,5.2,1.43121203999999));
#344795=CARTESIAN_POINT('Ctrl Pts',(4.45498735999994,2.2,1.43121203999999));
#344796=CARTESIAN_POINT('Ctrl Pts',(4.45665664199994,12.2,1.43314910699999));
#344797=CARTESIAN_POINT('Ctrl Pts',(4.45665664199994,5.2,1.43314910699999));
#344798=CARTESIAN_POINT('Ctrl Pts',(4.45665664199994,2.2,1.43314910699999));
#344799=CARTESIAN_POINT('Ctrl Pts',(4.45832615899994,12.2,1.43509055599999));
#344800=CARTESIAN_POINT('Ctrl Pts',(4.45832615899994,5.2,1.43509055599999));
#344801=CARTESIAN_POINT('Ctrl Pts',(4.45832615899994,2.2,1.43509055599999));
#344802=CARTESIAN_POINT('Ctrl Pts',(4.45999590199994,12.2,1.43703638499999));
#344803=CARTESIAN_POINT('Ctrl Pts',(4.45999590199994,5.2,1.43703638499999));
#344804=CARTESIAN_POINT('Ctrl Pts',(4.45999590199994,2.2,1.43703638499999));
#344805=CARTESIAN_POINT('Ctrl Pts',(4.46166586199995,12.2,1.43898659599999));
#344806=CARTESIAN_POINT('Ctrl Pts',(4.46166586199995,5.2,1.43898659599999));
#344807=CARTESIAN_POINT('Ctrl Pts',(4.46166586199995,2.2,1.43898659599999));
#344808=CARTESIAN_POINT('Ctrl Pts',(4.46333603099994,12.2,1.44094118699998));
#344809=CARTESIAN_POINT('Ctrl Pts',(4.46333603099994,5.2,1.44094118699998));
#344810=CARTESIAN_POINT('Ctrl Pts',(4.46333603099994,2.2,1.44094118699998));
#344811=CARTESIAN_POINT('Ctrl Pts',(4.46500639899994,12.2,1.44290015799998));
#344812=CARTESIAN_POINT('Ctrl Pts',(4.46500639899994,5.2,1.44290015799998));
#344813=CARTESIAN_POINT('Ctrl Pts',(4.46500639899994,2.2,1.44290015799998));
#344814=CARTESIAN_POINT('Ctrl Pts',(4.46667695899994,12.2,1.44486350799998));
#344815=CARTESIAN_POINT('Ctrl Pts',(4.46667695899994,5.2,1.44486350799998));
#344816=CARTESIAN_POINT('Ctrl Pts',(4.46667695899994,2.2,1.44486350799998));
#344817=CARTESIAN_POINT('Ctrl Pts',(4.46834770199994,12.2,1.44683123499998));
#344818=CARTESIAN_POINT('Ctrl Pts',(4.46834770199994,5.2,1.44683123499998));
#344819=CARTESIAN_POINT('Ctrl Pts',(4.46834770199994,2.2,1.44683123499998));
#344820=CARTESIAN_POINT('Ctrl Pts',(4.47001861799994,12.2,1.44880333999998));
#344821=CARTESIAN_POINT('Ctrl Pts',(4.47001861799994,5.2,1.44880333999998));
#344822=CARTESIAN_POINT('Ctrl Pts',(4.47001861799994,2.2,1.44880333999998));
#344823=CARTESIAN_POINT('Ctrl Pts',(4.47168969899994,12.2,1.45077982299998));
#344824=CARTESIAN_POINT('Ctrl Pts',(4.47168969899994,5.2,1.45077982299998));
#344825=CARTESIAN_POINT('Ctrl Pts',(4.47168969899994,2.2,1.45077982299998));
#344826=CARTESIAN_POINT('Ctrl Pts',(4.47336093799994,12.2,1.45276068199998));
#344827=CARTESIAN_POINT('Ctrl Pts',(4.47336093799994,5.2,1.45276068199998));
#344828=CARTESIAN_POINT('Ctrl Pts',(4.47336093799994,2.2,1.45276068199998));
#344829=CARTESIAN_POINT('Ctrl Pts',(4.47503232199994,12.2,1.45474591699998));
#344830=CARTESIAN_POINT('Ctrl Pts',(4.47503232199994,5.2,1.45474591699998));
#344831=CARTESIAN_POINT('Ctrl Pts',(4.47503232199994,2.2,1.45474591699998));
#344832=CARTESIAN_POINT('Ctrl Pts',(4.47670384499994,12.2,1.45673552699999));
#344833=CARTESIAN_POINT('Ctrl Pts',(4.47670384499994,5.2,1.45673552699999));
#344834=CARTESIAN_POINT('Ctrl Pts',(4.47670384499994,2.2,1.45673552699999));
#344835=CARTESIAN_POINT('Ctrl Pts',(4.47837549599994,12.2,1.45872950999999));
#344836=CARTESIAN_POINT('Ctrl Pts',(4.47837549599994,5.2,1.45872950999999));
#344837=CARTESIAN_POINT('Ctrl Pts',(4.47837549599994,2.2,1.45872950999999));
#344838=CARTESIAN_POINT('Ctrl Pts',(4.48004726799994,12.2,1.46072786799999));
#344839=CARTESIAN_POINT('Ctrl Pts',(4.48004726799994,5.2,1.46072786799999));
#344840=CARTESIAN_POINT('Ctrl Pts',(4.48004726799994,2.2,1.46072786799999));
#344841=CARTESIAN_POINT('Ctrl Pts',(4.48171915199994,12.2,1.46273059799999));
#344842=CARTESIAN_POINT('Ctrl Pts',(4.48171915199994,5.2,1.46273059799999));
#344843=CARTESIAN_POINT('Ctrl Pts',(4.48171915199994,2.2,1.46273059799999));
#344844=CARTESIAN_POINT('Ctrl Pts',(4.48339113899995,12.2,1.46473769999998));
#344845=CARTESIAN_POINT('Ctrl Pts',(4.48339113899995,5.2,1.46473769999998));
#344846=CARTESIAN_POINT('Ctrl Pts',(4.48339113899995,2.2,1.46473769999998));
#344847=CARTESIAN_POINT('Ctrl Pts',(4.48506322299994,12.2,1.46674917399999));
#344848=CARTESIAN_POINT('Ctrl Pts',(4.48506322299994,5.2,1.46674917399999));
#344849=CARTESIAN_POINT('Ctrl Pts',(4.48506322299994,2.2,1.46674917399999));
#344850=CARTESIAN_POINT('Ctrl Pts',(4.48673539399994,12.2,1.46876501899999));
#344851=CARTESIAN_POINT('Ctrl Pts',(4.48673539399994,5.2,1.46876501899999));
#344852=CARTESIAN_POINT('Ctrl Pts',(4.48673539399994,2.2,1.46876501899999));
#344853=CARTESIAN_POINT('Ctrl Pts',(4.48840764599994,12.2,1.47078523499999));
#344854=CARTESIAN_POINT('Ctrl Pts',(4.48840764599994,5.2,1.47078523499999));
#344855=CARTESIAN_POINT('Ctrl Pts',(4.48840764599994,2.2,1.47078523499999));
#344856=CARTESIAN_POINT('Ctrl Pts',(4.49007996999994,12.2,1.47280981899998));
#344857=CARTESIAN_POINT('Ctrl Pts',(4.49007996999994,5.2,1.47280981899998));
#344858=CARTESIAN_POINT('Ctrl Pts',(4.49007996999994,2.2,1.47280981899998));
#344859=CARTESIAN_POINT('Ctrl Pts',(4.49175235499994,12.2,1.47483877199999));
#344860=CARTESIAN_POINT('Ctrl Pts',(4.49175235499994,5.2,1.47483877199999));
#344861=CARTESIAN_POINT('Ctrl Pts',(4.49175235499994,2.2,1.47483877199999));
#344862=CARTESIAN_POINT('Ctrl Pts',(4.49342479299994,12.2,1.47687209299999));
#344863=CARTESIAN_POINT('Ctrl Pts',(4.49342479299994,5.2,1.47687209299999));
#344864=CARTESIAN_POINT('Ctrl Pts',(4.49342479299994,2.2,1.47687209299999));
#344865=CARTESIAN_POINT('Ctrl Pts',(4.49509727099994,12.2,1.47890977999999));
#344866=CARTESIAN_POINT('Ctrl Pts',(4.49509727099994,5.2,1.47890977999999));
#344867=CARTESIAN_POINT('Ctrl Pts',(4.49509727099994,2.2,1.47890977999999));
#344868=CARTESIAN_POINT('Ctrl Pts',(4.49676977799994,12.2,1.48095183199999));
#344869=CARTESIAN_POINT('Ctrl Pts',(4.49676977799994,5.2,1.48095183199999));
#344870=CARTESIAN_POINT('Ctrl Pts',(4.49676977799994,2.2,1.48095183199999));
#344871=CARTESIAN_POINT('Ctrl Pts',(4.49844230699994,12.2,1.48299824999999));
#344872=CARTESIAN_POINT('Ctrl Pts',(4.49844230699994,5.2,1.48299824999999));
#344873=CARTESIAN_POINT('Ctrl Pts',(4.49844230699994,2.2,1.48299824999999));
#344874=CARTESIAN_POINT('Ctrl Pts',(4.50011484799994,12.2,1.48504903199999));
#344875=CARTESIAN_POINT('Ctrl Pts',(4.50011484799994,5.2,1.48504903199999));
#344876=CARTESIAN_POINT('Ctrl Pts',(4.50011484799994,2.2,1.48504903199999));
#344877=CARTESIAN_POINT('Ctrl Pts',(4.50178739499994,12.2,1.48710417599998));
#344878=CARTESIAN_POINT('Ctrl Pts',(4.50178739499994,5.2,1.48710417599998));
#344879=CARTESIAN_POINT('Ctrl Pts',(4.50178739499994,2.2,1.48710417599998));
#344880=CARTESIAN_POINT('Ctrl Pts',(4.50345994399994,12.2,1.48916368399998));
#344881=CARTESIAN_POINT('Ctrl Pts',(4.50345994399994,5.2,1.48916368399998));
#344882=CARTESIAN_POINT('Ctrl Pts',(4.50345994399994,2.2,1.48916368399998));
#344883=CARTESIAN_POINT('Ctrl Pts',(4.5051324930519,12.2,1.4912275540641));
#344884=CARTESIAN_POINT('Ctrl Pts',(4.5051324930519,5.2,1.4912275540641));
#344885=CARTESIAN_POINT('Ctrl Pts',(4.5051324930519,2.2,1.4912275540641));
#344886=CARTESIAN_POINT('Ctrl Pts',(4.50647053110386,12.2,1.49288214012849));
#344887=CARTESIAN_POINT('Ctrl Pts',(4.50647053110386,5.2,1.49288214012849));
#344888=CARTESIAN_POINT('Ctrl Pts',(4.50647053110386,2.2,1.49288214012849));
#344889=CARTESIAN_POINT('Ctrl Pts',(4.50747405915582,12.2,1.49412504219303));
#344890=CARTESIAN_POINT('Ctrl Pts',(4.50747405915582,5.2,1.49412504219303));
#344891=CARTESIAN_POINT('Ctrl Pts',(4.50747405915582,2.2,1.49412504219303));
#344892=CARTESIAN_POINT('Ctrl Pts',(4.50814307720777,12.2,1.49495451625766));
#344893=CARTESIAN_POINT('Ctrl Pts',(4.50814307720777,5.2,1.49495451625766));
#344894=CARTESIAN_POINT('Ctrl Pts',(4.50814307720777,2.2,1.49495451625766));
#344895=CARTESIAN_POINT('Ctrl Pts',(4.50847758599994,12.2,1.49536947099998));
#344896=CARTESIAN_POINT('Ctrl Pts',(4.50847758599994,5.2,1.49536947099998));
#344897=CARTESIAN_POINT('Ctrl Pts',(4.50847758599994,2.2,1.49536947099998));
#344898=CARTESIAN_POINT('',(3.87111410199994,12.2,0.982006995999987));
#344899=CARTESIAN_POINT('Origin',(-5.66300478732629E-14,15.2,-1.77635683940025E-14));
#344900=CARTESIAN_POINT('',(3.51370677999994,12.2,0.891341496999987));
#344901=CARTESIAN_POINT('Origin',(-5.66300478732629E-14,15.2,-1.77635683940025E-14));
#344902=CARTESIAN_POINT('Origin',(-5.66300478732629E-14,15.2,-1.77635683940025E-14));
#344903=CARTESIAN_POINT('',(3.60918509199994,2.2,0.338242477999984));
#344904=CARTESIAN_POINT('Origin',(-5.66300478732629E-14,15.2,-1.77635683940025E-14));
#344905=CARTESIAN_POINT('',(3.96444824099994,12.2,-0.482713455000017));
#344906=CARTESIAN_POINT('',(3.59842368199994,12.2,-0.438146099000014));
#344907=CARTESIAN_POINT('Origin',(3.97627021699994,15.2,0.372644643999984));
#344908=CARTESIAN_POINT('',(3.97632130999995,12.2,0.372649431999985));
#344909=CARTESIAN_POINT('Ctrl Pts',(4.74889012999994,12.2,0.102676827999986));
#344910=CARTESIAN_POINT('Ctrl Pts',(4.74889012999994,5.2,0.102676827999986));
#344911=CARTESIAN_POINT('Ctrl Pts',(4.74889012999994,2.2,0.102676827999986));
#344912=CARTESIAN_POINT('Ctrl Pts',(4.74843586199994,12.2,0.102955621999987));
#344913=CARTESIAN_POINT('Ctrl Pts',(4.74843586199994,5.2,0.102955621999987));
#344914=CARTESIAN_POINT('Ctrl Pts',(4.74843586199994,2.2,0.102955621999987));
#344915=CARTESIAN_POINT('Ctrl Pts',(4.74752747599994,12.2,0.103512796999983));
#344916=CARTESIAN_POINT('Ctrl Pts',(4.74752747599994,5.2,0.103512796999983));
#344917=CARTESIAN_POINT('Ctrl Pts',(4.74752747599994,2.2,0.103512796999983));
#344918=CARTESIAN_POINT('Ctrl Pts',(4.74616533299994,12.2,0.104347326999985));
#344919=CARTESIAN_POINT('Ctrl Pts',(4.74616533299994,5.2,0.104347326999985));
#344920=CARTESIAN_POINT('Ctrl Pts',(4.74616533299994,2.2,0.104347326999985));
#344921=CARTESIAN_POINT('Ctrl Pts',(4.74435001799994,12.2,0.105457566999987));
#344922=CARTESIAN_POINT('Ctrl Pts',(4.74435001799994,5.2,0.105457566999987));
#344923=CARTESIAN_POINT('Ctrl Pts',(4.74435001799994,2.2,0.105457566999987));
#344924=CARTESIAN_POINT('Ctrl Pts',(4.74208233599994,12.2,0.106841257999988));
#344925=CARTESIAN_POINT('Ctrl Pts',(4.74208233599994,5.2,0.106841257999988));
#344926=CARTESIAN_POINT('Ctrl Pts',(4.74208233599994,2.2,0.106841257999988));
#344927=CARTESIAN_POINT('Ctrl Pts',(4.73981611699994,12.2,0.108220837999986));
#344928=CARTESIAN_POINT('Ctrl Pts',(4.73981611699994,5.2,0.108220837999986));
#344929=CARTESIAN_POINT('Ctrl Pts',(4.73981611699994,2.2,0.108220837999986));
#344930=CARTESIAN_POINT('Ctrl Pts',(4.73755136299994,12.2,0.109596309999986));
#344931=CARTESIAN_POINT('Ctrl Pts',(4.73755136299994,5.2,0.109596309999986));
#344932=CARTESIAN_POINT('Ctrl Pts',(4.73755136299994,2.2,0.109596309999986));
#344933=CARTESIAN_POINT('Ctrl Pts',(4.73528807699994,12.2,0.110967671999984));
#344934=CARTESIAN_POINT('Ctrl Pts',(4.73528807699994,5.2,0.110967671999984));
#344935=CARTESIAN_POINT('Ctrl Pts',(4.73528807699994,2.2,0.110967671999984));
#344936=CARTESIAN_POINT('Ctrl Pts',(4.73302626599994,12.2,0.112334925999988));
#344937=CARTESIAN_POINT('Ctrl Pts',(4.73302626599994,5.2,0.112334925999988));
#344938=CARTESIAN_POINT('Ctrl Pts',(4.73302626599994,2.2,0.112334925999988));
#344939=CARTESIAN_POINT('Ctrl Pts',(4.73076593799994,12.2,0.113698076999986));
#344940=CARTESIAN_POINT('Ctrl Pts',(4.73076593799994,5.2,0.113698076999986));
#344941=CARTESIAN_POINT('Ctrl Pts',(4.73076593799994,2.2,0.113698076999986));
#344942=CARTESIAN_POINT('Ctrl Pts',(4.72850710099994,12.2,0.115057122999982));
#344943=CARTESIAN_POINT('Ctrl Pts',(4.72850710099994,5.2,0.115057122999982));
#344944=CARTESIAN_POINT('Ctrl Pts',(4.72850710099994,2.2,0.115057122999982));
#344945=CARTESIAN_POINT('Ctrl Pts',(4.72624976699994,12.2,0.116412069999985));
#344946=CARTESIAN_POINT('Ctrl Pts',(4.72624976699994,5.2,0.116412069999985));
#344947=CARTESIAN_POINT('Ctrl Pts',(4.72624976699994,2.2,0.116412069999985));
#344948=CARTESIAN_POINT('Ctrl Pts',(4.72399394499994,12.2,0.117762919999986));
#344949=CARTESIAN_POINT('Ctrl Pts',(4.72399394499994,5.2,0.117762919999986));
#344950=CARTESIAN_POINT('Ctrl Pts',(4.72399394499994,2.2,0.117762919999986));
#344951=CARTESIAN_POINT('Ctrl Pts',(4.72173964699994,12.2,0.119109672999986));
#344952=CARTESIAN_POINT('Ctrl Pts',(4.72173964699994,5.2,0.119109672999986));
#344953=CARTESIAN_POINT('Ctrl Pts',(4.72173964699994,2.2,0.119109672999986));
#344954=CARTESIAN_POINT('Ctrl Pts',(4.71948688099994,12.2,0.120452335999985));
#344955=CARTESIAN_POINT('Ctrl Pts',(4.71948688099994,5.2,0.120452335999985));
#344956=CARTESIAN_POINT('Ctrl Pts',(4.71948688099994,2.2,0.120452335999985));
#344957=CARTESIAN_POINT('Ctrl Pts',(4.71723565499994,12.2,0.121790906999983));
#344958=CARTESIAN_POINT('Ctrl Pts',(4.71723565499994,5.2,0.121790906999983));
#344959=CARTESIAN_POINT('Ctrl Pts',(4.71723565499994,2.2,0.121790906999983));
#344960=CARTESIAN_POINT('Ctrl Pts',(4.71498597799994,12.2,0.123125388999985));
#344961=CARTESIAN_POINT('Ctrl Pts',(4.71498597799994,5.2,0.123125388999985));
#344962=CARTESIAN_POINT('Ctrl Pts',(4.71498597799994,2.2,0.123125388999985));
#344963=CARTESIAN_POINT('Ctrl Pts',(4.71273785699994,12.2,0.124455785999986));
#344964=CARTESIAN_POINT('Ctrl Pts',(4.71273785699994,5.2,0.124455785999986));
#344965=CARTESIAN_POINT('Ctrl Pts',(4.71273785699994,2.2,0.124455785999986));
#344966=CARTESIAN_POINT('Ctrl Pts',(4.71049130099994,12.2,0.125782098999987));
#344967=CARTESIAN_POINT('Ctrl Pts',(4.71049130099994,5.2,0.125782098999987));
#344968=CARTESIAN_POINT('Ctrl Pts',(4.71049130099994,2.2,0.125782098999987));
#344969=CARTESIAN_POINT('Ctrl Pts',(4.70824631499994,12.2,0.127104328999987));
#344970=CARTESIAN_POINT('Ctrl Pts',(4.70824631499994,5.2,0.127104328999987));
#344971=CARTESIAN_POINT('Ctrl Pts',(4.70824631499994,2.2,0.127104328999987));
#344972=CARTESIAN_POINT('Ctrl Pts',(4.70600290799994,12.2,0.128422478999983));
#344973=CARTESIAN_POINT('Ctrl Pts',(4.70600290799994,5.2,0.128422478999983));
#344974=CARTESIAN_POINT('Ctrl Pts',(4.70600290799994,2.2,0.128422478999983));
#344975=CARTESIAN_POINT('Ctrl Pts',(4.70376108999994,12.2,0.129736550999984));
#344976=CARTESIAN_POINT('Ctrl Pts',(4.70376108999994,5.2,0.129736550999984));
#344977=CARTESIAN_POINT('Ctrl Pts',(4.70376108999994,2.2,0.129736550999984));
#344978=CARTESIAN_POINT('Ctrl Pts',(4.70152086799994,12.2,0.131046545999984));
#344979=CARTESIAN_POINT('Ctrl Pts',(4.70152086799994,5.2,0.131046545999984));
#344980=CARTESIAN_POINT('Ctrl Pts',(4.70152086799994,2.2,0.131046545999984));
#344981=CARTESIAN_POINT('Ctrl Pts',(4.69928225199994,12.2,0.132352469999986));
#344982=CARTESIAN_POINT('Ctrl Pts',(4.69928225199994,5.2,0.132352469999986));
#344983=CARTESIAN_POINT('Ctrl Pts',(4.69928225199994,2.2,0.132352469999986));
#344984=CARTESIAN_POINT('Ctrl Pts',(4.69704524999994,12.2,0.133654322999988));
#344985=CARTESIAN_POINT('Ctrl Pts',(4.69704524999994,5.2,0.133654322999988));
#344986=CARTESIAN_POINT('Ctrl Pts',(4.69704524999994,2.2,0.133654322999988));
#344987=CARTESIAN_POINT('Ctrl Pts',(4.69480987199994,12.2,0.134952106999986));
#344988=CARTESIAN_POINT('Ctrl Pts',(4.69480987199994,5.2,0.134952106999986));
#344989=CARTESIAN_POINT('Ctrl Pts',(4.69480987199994,2.2,0.134952106999986));
#344990=CARTESIAN_POINT('Ctrl Pts',(4.69257612499994,12.2,0.136245824999985));
#344991=CARTESIAN_POINT('Ctrl Pts',(4.69257612499994,5.2,0.136245824999985));
#344992=CARTESIAN_POINT('Ctrl Pts',(4.69257612499994,2.2,0.136245824999985));
#344993=CARTESIAN_POINT('Ctrl Pts',(4.69034401799994,12.2,0.137535479999986));
#344994=CARTESIAN_POINT('Ctrl Pts',(4.69034401799994,5.2,0.137535479999986));
#344995=CARTESIAN_POINT('Ctrl Pts',(4.69034401799994,2.2,0.137535479999986));
#344996=CARTESIAN_POINT('Ctrl Pts',(4.68811355899994,12.2,0.138821072999988));
#344997=CARTESIAN_POINT('Ctrl Pts',(4.68811355899994,5.2,0.138821072999988));
#344998=CARTESIAN_POINT('Ctrl Pts',(4.68811355899994,2.2,0.138821072999988));
#344999=CARTESIAN_POINT('Ctrl Pts',(4.68588475599994,12.2,0.140102605999988));
#345000=CARTESIAN_POINT('Ctrl Pts',(4.68588475599994,5.2,0.140102605999988));
#345001=CARTESIAN_POINT('Ctrl Pts',(4.68588475599994,2.2,0.140102605999988));
#345002=CARTESIAN_POINT('Ctrl Pts',(4.68365761899994,12.2,0.141380083999985));
#345003=CARTESIAN_POINT('Ctrl Pts',(4.68365761899994,5.2,0.141380083999985));
#345004=CARTESIAN_POINT('Ctrl Pts',(4.68365761899994,2.2,0.141380083999985));
#345005=CARTESIAN_POINT('Ctrl Pts',(4.68143215399994,12.2,0.142653506999988));
#345006=CARTESIAN_POINT('Ctrl Pts',(4.68143215399994,5.2,0.142653506999988));
#345007=CARTESIAN_POINT('Ctrl Pts',(4.68143215399994,2.2,0.142653506999988));
#345008=CARTESIAN_POINT('Ctrl Pts',(4.67920837299994,12.2,0.143922876999985));
#345009=CARTESIAN_POINT('Ctrl Pts',(4.67920837299994,5.2,0.143922876999985));
#345010=CARTESIAN_POINT('Ctrl Pts',(4.67920837299994,2.2,0.143922876999985));
#345011=CARTESIAN_POINT('Ctrl Pts',(4.67698627999994,12.2,0.145188198999988));
#345012=CARTESIAN_POINT('Ctrl Pts',(4.67698627999994,5.2,0.145188198999988));
#345013=CARTESIAN_POINT('Ctrl Pts',(4.67698627999994,2.2,0.145188198999988));
#345014=CARTESIAN_POINT('Ctrl Pts',(4.67476588699994,12.2,0.146449472999985));
#345015=CARTESIAN_POINT('Ctrl Pts',(4.67476588699994,5.2,0.146449472999985));
#345016=CARTESIAN_POINT('Ctrl Pts',(4.67476588699994,2.2,0.146449472999985));
#345017=CARTESIAN_POINT('Ctrl Pts',(4.67254720199994,12.2,0.147706702999986));
#345018=CARTESIAN_POINT('Ctrl Pts',(4.67254720199994,5.2,0.147706702999986));
#345019=CARTESIAN_POINT('Ctrl Pts',(4.67254720199994,2.2,0.147706702999986));
#345020=CARTESIAN_POINT('Ctrl Pts',(4.67033023199994,12.2,0.148959889999984));
#345021=CARTESIAN_POINT('Ctrl Pts',(4.67033023199994,5.2,0.148959889999984));
#345022=CARTESIAN_POINT('Ctrl Pts',(4.67033023199994,2.2,0.148959889999984));
#345023=CARTESIAN_POINT('Ctrl Pts',(4.66811498799994,12.2,0.150209038999982));
#345024=CARTESIAN_POINT('Ctrl Pts',(4.66811498799994,5.2,0.150209038999982));
#345025=CARTESIAN_POINT('Ctrl Pts',(4.66811498799994,2.2,0.150209038999982));
#345026=CARTESIAN_POINT('Ctrl Pts',(4.66590147699994,12.2,0.151454149999988));
#345027=CARTESIAN_POINT('Ctrl Pts',(4.66590147699994,5.2,0.151454149999988));
#345028=CARTESIAN_POINT('Ctrl Pts',(4.66590147699994,2.2,0.151454149999988));
#345029=CARTESIAN_POINT('Ctrl Pts',(4.66368970599994,12.2,0.152695225999988));
#345030=CARTESIAN_POINT('Ctrl Pts',(4.66368970599994,5.2,0.152695225999988));
#345031=CARTESIAN_POINT('Ctrl Pts',(4.66368970599994,2.2,0.152695225999988));
#345032=CARTESIAN_POINT('Ctrl Pts',(4.66147968699994,12.2,0.153932269999988));
#345033=CARTESIAN_POINT('Ctrl Pts',(4.66147968699994,5.2,0.153932269999988));
#345034=CARTESIAN_POINT('Ctrl Pts',(4.66147968699994,2.2,0.153932269999988));
#345035=CARTESIAN_POINT('Ctrl Pts',(4.65927142699994,12.2,0.155165283999987));
#345036=CARTESIAN_POINT('Ctrl Pts',(4.65927142699994,5.2,0.155165283999987));
#345037=CARTESIAN_POINT('Ctrl Pts',(4.65927142699994,2.2,0.155165283999987));
#345038=CARTESIAN_POINT('Ctrl Pts',(4.65706493399995,12.2,0.156394271999982));
#345039=CARTESIAN_POINT('Ctrl Pts',(4.65706493399995,5.2,0.156394271999982));
#345040=CARTESIAN_POINT('Ctrl Pts',(4.65706493399995,2.2,0.156394271999982));
#345041=CARTESIAN_POINT('Ctrl Pts',(4.65486021599994,12.2,0.157619235999986));
#345042=CARTESIAN_POINT('Ctrl Pts',(4.65486021599994,5.2,0.157619235999986));
#345043=CARTESIAN_POINT('Ctrl Pts',(4.65486021599994,2.2,0.157619235999986));
#345044=CARTESIAN_POINT('Ctrl Pts',(4.65265728299994,12.2,0.158840176999986));
#345045=CARTESIAN_POINT('Ctrl Pts',(4.65265728299994,5.2,0.158840176999986));
#345046=CARTESIAN_POINT('Ctrl Pts',(4.65265728299994,2.2,0.158840176999986));
#345047=CARTESIAN_POINT('Ctrl Pts',(4.65045614299994,12.2,0.160057098999986));
#345048=CARTESIAN_POINT('Ctrl Pts',(4.65045614299994,5.2,0.160057098999986));
#345049=CARTESIAN_POINT('Ctrl Pts',(4.65045614299994,2.2,0.160057098999986));
#345050=CARTESIAN_POINT('Ctrl Pts',(4.64825680499994,12.2,0.161270003999987));
#345051=CARTESIAN_POINT('Ctrl Pts',(4.64825680499994,5.2,0.161270003999987));
#345052=CARTESIAN_POINT('Ctrl Pts',(4.64825680499994,2.2,0.161270003999987));
#345053=CARTESIAN_POINT('Ctrl Pts',(4.64605927599994,12.2,0.162478894999989));
#345054=CARTESIAN_POINT('Ctrl Pts',(4.64605927599994,5.2,0.162478894999989));
#345055=CARTESIAN_POINT('Ctrl Pts',(4.64605927599994,2.2,0.162478894999989));
#345056=CARTESIAN_POINT('Ctrl Pts',(4.64386356799994,12.2,0.163683775999988));
#345057=CARTESIAN_POINT('Ctrl Pts',(4.64386356799994,5.2,0.163683775999988));
#345058=CARTESIAN_POINT('Ctrl Pts',(4.64386356799994,2.2,0.163683775999988));
#345059=CARTESIAN_POINT('Ctrl Pts',(4.64166968599994,12.2,0.164884647999983));
#345060=CARTESIAN_POINT('Ctrl Pts',(4.64166968599994,5.2,0.164884647999983));
#345061=CARTESIAN_POINT('Ctrl Pts',(4.64166968599994,2.2,0.164884647999983));
#345062=CARTESIAN_POINT('Ctrl Pts',(4.63947764099994,12.2,0.166081512999985));
#345063=CARTESIAN_POINT('Ctrl Pts',(4.63947764099994,5.2,0.166081512999985));
#345064=CARTESIAN_POINT('Ctrl Pts',(4.63947764099994,2.2,0.166081512999985));
#345065=CARTESIAN_POINT('Ctrl Pts',(4.63728744099994,12.2,0.167274374999984));
#345066=CARTESIAN_POINT('Ctrl Pts',(4.63728744099994,5.2,0.167274374999984));
#345067=CARTESIAN_POINT('Ctrl Pts',(4.63728744099994,2.2,0.167274374999984));
#345068=CARTESIAN_POINT('Ctrl Pts',(4.63509909399995,12.2,0.168463236999985));
#345069=CARTESIAN_POINT('Ctrl Pts',(4.63509909399995,5.2,0.168463236999985));
#345070=CARTESIAN_POINT('Ctrl Pts',(4.63509909399995,2.2,0.168463236999985));
#345071=CARTESIAN_POINT('Ctrl Pts',(4.63291260899994,12.2,0.169648099999984));
#345072=CARTESIAN_POINT('Ctrl Pts',(4.63291260899994,5.2,0.169648099999984));
#345073=CARTESIAN_POINT('Ctrl Pts',(4.63291260899994,2.2,0.169648099999984));
#345074=CARTESIAN_POINT('Ctrl Pts',(4.63072799499994,12.2,0.170828968999985));
#345075=CARTESIAN_POINT('Ctrl Pts',(4.63072799499994,5.2,0.170828968999985));
#345076=CARTESIAN_POINT('Ctrl Pts',(4.63072799499994,2.2,0.170828968999985));
#345077=CARTESIAN_POINT('Ctrl Pts',(4.62854525999994,12.2,0.172005844999985));
#345078=CARTESIAN_POINT('Ctrl Pts',(4.62854525999994,5.2,0.172005844999985));
#345079=CARTESIAN_POINT('Ctrl Pts',(4.62854525999994,2.2,0.172005844999985));
#345080=CARTESIAN_POINT('Ctrl Pts',(4.62636441299995,12.2,0.173178731999983));
#345081=CARTESIAN_POINT('Ctrl Pts',(4.62636441299995,5.2,0.173178731999983));
#345082=CARTESIAN_POINT('Ctrl Pts',(4.62636441299995,2.2,0.173178731999983));
#345083=CARTESIAN_POINT('Ctrl Pts',(4.62418546299994,12.2,0.174347630999985));
#345084=CARTESIAN_POINT('Ctrl Pts',(4.62418546299994,5.2,0.174347630999985));
#345085=CARTESIAN_POINT('Ctrl Pts',(4.62418546299994,2.2,0.174347630999985));
#345086=CARTESIAN_POINT('Ctrl Pts',(4.62200841899994,12.2,0.175512546999985));
#345087=CARTESIAN_POINT('Ctrl Pts',(4.62200841899994,5.2,0.175512546999985));
#345088=CARTESIAN_POINT('Ctrl Pts',(4.62200841899994,2.2,0.175512546999985));
#345089=CARTESIAN_POINT('Ctrl Pts',(4.61983328799994,12.2,0.176673481999985));
#345090=CARTESIAN_POINT('Ctrl Pts',(4.61983328799994,5.2,0.176673481999985));
#345091=CARTESIAN_POINT('Ctrl Pts',(4.61983328799994,2.2,0.176673481999985));
#345092=CARTESIAN_POINT('Ctrl Pts',(4.61766008099994,12.2,0.177830437999984));
#345093=CARTESIAN_POINT('Ctrl Pts',(4.61766008099994,5.2,0.177830437999984));
#345094=CARTESIAN_POINT('Ctrl Pts',(4.61766008099994,2.2,0.177830437999984));
#345095=CARTESIAN_POINT('Ctrl Pts',(4.61548880399994,12.2,0.178983417999987));
#345096=CARTESIAN_POINT('Ctrl Pts',(4.61548880399994,5.2,0.178983417999987));
#345097=CARTESIAN_POINT('Ctrl Pts',(4.61548880399994,2.2,0.178983417999987));
#345098=CARTESIAN_POINT('Ctrl Pts',(4.61331946799994,12.2,0.180132425999986));
#345099=CARTESIAN_POINT('Ctrl Pts',(4.61331946799994,5.2,0.180132425999986));
#345100=CARTESIAN_POINT('Ctrl Pts',(4.61331946799994,2.2,0.180132425999986));
#345101=CARTESIAN_POINT('Ctrl Pts',(4.61115208099994,12.2,0.181277463999985));
#345102=CARTESIAN_POINT('Ctrl Pts',(4.61115208099994,5.2,0.181277463999985));
#345103=CARTESIAN_POINT('Ctrl Pts',(4.61115208099994,2.2,0.181277463999985));
#345104=CARTESIAN_POINT('Ctrl Pts',(4.60898665099994,12.2,0.182418534999984));
#345105=CARTESIAN_POINT('Ctrl Pts',(4.60898665099994,5.2,0.182418534999984));
#345106=CARTESIAN_POINT('Ctrl Pts',(4.60898665099994,2.2,0.182418534999984));
#345107=CARTESIAN_POINT('Ctrl Pts',(4.60682318899994,12.2,0.183555642999984));
#345108=CARTESIAN_POINT('Ctrl Pts',(4.60682318899994,5.2,0.183555642999984));
#345109=CARTESIAN_POINT('Ctrl Pts',(4.60682318899994,2.2,0.183555642999984));
#345110=CARTESIAN_POINT('Ctrl Pts',(4.60466170099994,12.2,0.184688787999985));
#345111=CARTESIAN_POINT('Ctrl Pts',(4.60466170099994,5.2,0.184688787999985));
#345112=CARTESIAN_POINT('Ctrl Pts',(4.60466170099994,2.2,0.184688787999985));
#345113=CARTESIAN_POINT('Ctrl Pts',(4.60250219699994,12.2,0.185817975999987));
#345114=CARTESIAN_POINT('Ctrl Pts',(4.60250219699994,5.2,0.185817975999987));
#345115=CARTESIAN_POINT('Ctrl Pts',(4.60250219699994,2.2,0.185817975999987));
#345116=CARTESIAN_POINT('Ctrl Pts',(4.60034468499994,12.2,0.186943208999986));
#345117=CARTESIAN_POINT('Ctrl Pts',(4.60034468499994,5.2,0.186943208999986));
#345118=CARTESIAN_POINT('Ctrl Pts',(4.60034468499994,2.2,0.186943208999986));
#345119=CARTESIAN_POINT('Ctrl Pts',(4.59818917499994,12.2,0.188064488999986));
#345120=CARTESIAN_POINT('Ctrl Pts',(4.59818917499994,5.2,0.188064488999986));
#345121=CARTESIAN_POINT('Ctrl Pts',(4.59818917499994,2.2,0.188064488999986));
#345122=CARTESIAN_POINT('Ctrl Pts',(4.59603567499994,12.2,0.189181820999984));
#345123=CARTESIAN_POINT('Ctrl Pts',(4.59603567499994,5.2,0.189181820999984));
#345124=CARTESIAN_POINT('Ctrl Pts',(4.59603567499994,2.2,0.189181820999984));
#345125=CARTESIAN_POINT('Ctrl Pts',(4.59388419399994,12.2,0.190295204999984));
#345126=CARTESIAN_POINT('Ctrl Pts',(4.59388419399994,5.2,0.190295204999984));
#345127=CARTESIAN_POINT('Ctrl Pts',(4.59388419399994,2.2,0.190295204999984));
#345128=CARTESIAN_POINT('Ctrl Pts',(4.59173473999994,12.2,0.191404646999986));
#345129=CARTESIAN_POINT('Ctrl Pts',(4.59173473999994,5.2,0.191404646999986));
#345130=CARTESIAN_POINT('Ctrl Pts',(4.59173473999994,2.2,0.191404646999986));
#345131=CARTESIAN_POINT('Ctrl Pts',(4.58958732499995,12.2,0.192510148999983));
#345132=CARTESIAN_POINT('Ctrl Pts',(4.58958732499995,5.2,0.192510148999983));
#345133=CARTESIAN_POINT('Ctrl Pts',(4.58958732499995,2.2,0.192510148999983));
#345134=CARTESIAN_POINT('Ctrl Pts',(4.58744195199994,12.2,0.193611713999986));
#345135=CARTESIAN_POINT('Ctrl Pts',(4.58744195199994,5.2,0.193611713999986));
#345136=CARTESIAN_POINT('Ctrl Pts',(4.58744195199994,2.2,0.193611713999986));
#345137=CARTESIAN_POINT('Ctrl Pts',(4.58529863499994,12.2,0.194709342999988));
#345138=CARTESIAN_POINT('Ctrl Pts',(4.58529863499994,5.2,0.194709342999988));
#345139=CARTESIAN_POINT('Ctrl Pts',(4.58529863499994,2.2,0.194709342999988));
#345140=CARTESIAN_POINT('Ctrl Pts',(4.58315737999994,12.2,0.195803042999985));
#345141=CARTESIAN_POINT('Ctrl Pts',(4.58315737999994,5.2,0.195803042999985));
#345142=CARTESIAN_POINT('Ctrl Pts',(4.58315737999994,2.2,0.195803042999985));
#345143=CARTESIAN_POINT('Ctrl Pts',(4.58101819799994,12.2,0.196892814999985));
#345144=CARTESIAN_POINT('Ctrl Pts',(4.58101819799994,5.2,0.196892814999985));
#345145=CARTESIAN_POINT('Ctrl Pts',(4.58101819799994,2.2,0.196892814999985));
#345146=CARTESIAN_POINT('Ctrl Pts',(4.57888109499994,12.2,0.197978660999985));
#345147=CARTESIAN_POINT('Ctrl Pts',(4.57888109499994,5.2,0.197978660999985));
#345148=CARTESIAN_POINT('Ctrl Pts',(4.57888109499994,2.2,0.197978660999985));
#345149=CARTESIAN_POINT('Ctrl Pts',(4.57674608199994,12.2,0.199060585999984));
#345150=CARTESIAN_POINT('Ctrl Pts',(4.57674608199994,5.2,0.199060585999984));
#345151=CARTESIAN_POINT('Ctrl Pts',(4.57674608199994,2.2,0.199060585999984));
#345152=CARTESIAN_POINT('Ctrl Pts',(4.57461316799994,12.2,0.200138592999988));
#345153=CARTESIAN_POINT('Ctrl Pts',(4.57461316799994,5.2,0.200138592999988));
#345154=CARTESIAN_POINT('Ctrl Pts',(4.57461316799994,2.2,0.200138592999988));
#345155=CARTESIAN_POINT('Ctrl Pts',(4.57248235999994,12.2,0.201212683999987));
#345156=CARTESIAN_POINT('Ctrl Pts',(4.57248235999994,5.2,0.201212683999987));
#345157=CARTESIAN_POINT('Ctrl Pts',(4.57248235999994,2.2,0.201212683999987));
#345158=CARTESIAN_POINT('Ctrl Pts',(4.57035366899994,12.2,0.202282863999983));
#345159=CARTESIAN_POINT('Ctrl Pts',(4.57035366899994,5.2,0.202282863999983));
#345160=CARTESIAN_POINT('Ctrl Pts',(4.57035366899994,2.2,0.202282863999983));
#345161=CARTESIAN_POINT('Ctrl Pts',(4.56822710199994,12.2,0.203349133999984));
#345162=CARTESIAN_POINT('Ctrl Pts',(4.56822710199994,5.2,0.203349133999984));
#345163=CARTESIAN_POINT('Ctrl Pts',(4.56822710199994,2.2,0.203349133999984));
#345164=CARTESIAN_POINT('Ctrl Pts',(4.56610266799994,12.2,0.204411497999986));
#345165=CARTESIAN_POINT('Ctrl Pts',(4.56610266799994,5.2,0.204411497999986));
#345166=CARTESIAN_POINT('Ctrl Pts',(4.56610266799994,2.2,0.204411497999986));
#345167=CARTESIAN_POINT('Ctrl Pts',(4.56398037799994,12.2,0.205469959999984));
#345168=CARTESIAN_POINT('Ctrl Pts',(4.56398037799994,5.2,0.205469959999984));
#345169=CARTESIAN_POINT('Ctrl Pts',(4.56398037799994,2.2,0.205469959999984));
#345170=CARTESIAN_POINT('Ctrl Pts',(4.56186023799994,12.2,0.206524522999985));
#345171=CARTESIAN_POINT('Ctrl Pts',(4.56186023799994,5.2,0.206524522999985));
#345172=CARTESIAN_POINT('Ctrl Pts',(4.56186023799994,2.2,0.206524522999985));
#345173=CARTESIAN_POINT('Ctrl Pts',(4.55974225999994,12.2,0.207575188999982));
#345174=CARTESIAN_POINT('Ctrl Pts',(4.55974225999994,5.2,0.207575188999982));
#345175=CARTESIAN_POINT('Ctrl Pts',(4.55974225999994,2.2,0.207575188999982));
#345176=CARTESIAN_POINT('Ctrl Pts',(4.55762644999994,12.2,0.208621963999986));
#345177=CARTESIAN_POINT('Ctrl Pts',(4.55762644999994,5.2,0.208621963999986));
#345178=CARTESIAN_POINT('Ctrl Pts',(4.55762644999994,2.2,0.208621963999986));
#345179=CARTESIAN_POINT('Ctrl Pts',(4.55551281799994,12.2,0.209664847999989));
#345180=CARTESIAN_POINT('Ctrl Pts',(4.55551281799994,5.2,0.209664847999989));
#345181=CARTESIAN_POINT('Ctrl Pts',(4.55551281799994,2.2,0.209664847999989));
#345182=CARTESIAN_POINT('Ctrl Pts',(4.55340137299994,12.2,0.210703846999984));
#345183=CARTESIAN_POINT('Ctrl Pts',(4.55340137299994,5.2,0.210703846999984));
#345184=CARTESIAN_POINT('Ctrl Pts',(4.55340137299994,2.2,0.210703846999984));
#345185=CARTESIAN_POINT('Ctrl Pts',(4.55129212499994,12.2,0.211738961999988));
#345186=CARTESIAN_POINT('Ctrl Pts',(4.55129212499994,5.2,0.211738961999988));
#345187=CARTESIAN_POINT('Ctrl Pts',(4.55129212499994,2.2,0.211738961999988));
#345188=CARTESIAN_POINT('Ctrl Pts',(4.54918508099994,12.2,0.212770198999985));
#345189=CARTESIAN_POINT('Ctrl Pts',(4.54918508099994,5.2,0.212770198999985));
#345190=CARTESIAN_POINT('Ctrl Pts',(4.54918508099994,2.2,0.212770198999985));
#345191=CARTESIAN_POINT('Ctrl Pts',(4.54708025099994,12.2,0.213797558999986));
#345192=CARTESIAN_POINT('Ctrl Pts',(4.54708025099994,5.2,0.213797558999986));
#345193=CARTESIAN_POINT('Ctrl Pts',(4.54708025099994,2.2,0.213797558999986));
#345194=CARTESIAN_POINT('Ctrl Pts',(4.54497764299994,12.2,0.214821045999987));
#345195=CARTESIAN_POINT('Ctrl Pts',(4.54497764299994,5.2,0.214821045999987));
#345196=CARTESIAN_POINT('Ctrl Pts',(4.54497764299994,2.2,0.214821045999987));
#345197=CARTESIAN_POINT('Ctrl Pts',(4.54287726799994,12.2,0.215840664999987));
#345198=CARTESIAN_POINT('Ctrl Pts',(4.54287726799994,5.2,0.215840664999987));
#345199=CARTESIAN_POINT('Ctrl Pts',(4.54287726799994,2.2,0.215840664999987));
#345200=CARTESIAN_POINT('Ctrl Pts',(4.54077913299994,12.2,0.216856416999986));
#345201=CARTESIAN_POINT('Ctrl Pts',(4.54077913299994,5.2,0.216856416999986));
#345202=CARTESIAN_POINT('Ctrl Pts',(4.54077913299994,2.2,0.216856416999986));
#345203=CARTESIAN_POINT('Ctrl Pts',(4.53868324699994,12.2,0.217868305999982));
#345204=CARTESIAN_POINT('Ctrl Pts',(4.53868324699994,5.2,0.217868305999982));
#345205=CARTESIAN_POINT('Ctrl Pts',(4.53868324699994,2.2,0.217868305999982));
#345206=CARTESIAN_POINT('Ctrl Pts',(4.53658962099994,12.2,0.218876336999987));
#345207=CARTESIAN_POINT('Ctrl Pts',(4.53658962099994,5.2,0.218876336999987));
#345208=CARTESIAN_POINT('Ctrl Pts',(4.53658962099994,2.2,0.218876336999987));
#345209=CARTESIAN_POINT('Ctrl Pts',(4.53449826199994,12.2,0.219880511999988));
#345210=CARTESIAN_POINT('Ctrl Pts',(4.53449826199994,5.2,0.219880511999988));
#345211=CARTESIAN_POINT('Ctrl Pts',(4.53449826199994,2.2,0.219880511999988));
#345212=CARTESIAN_POINT('Ctrl Pts',(4.53240917899994,12.2,0.220880834999986));
#345213=CARTESIAN_POINT('Ctrl Pts',(4.53240917899994,5.2,0.220880834999986));
#345214=CARTESIAN_POINT('Ctrl Pts',(4.53240917899994,2.2,0.220880834999986));
#345215=CARTESIAN_POINT('Ctrl Pts',(4.53032238199994,12.2,0.221877309999985));
#345216=CARTESIAN_POINT('Ctrl Pts',(4.53032238199994,5.2,0.221877309999985));
#345217=CARTESIAN_POINT('Ctrl Pts',(4.53032238199994,2.2,0.221877309999985));
#345218=CARTESIAN_POINT('Ctrl Pts',(4.52823787999994,12.2,0.222869938999986));
#345219=CARTESIAN_POINT('Ctrl Pts',(4.52823787999994,5.2,0.222869938999986));
#345220=CARTESIAN_POINT('Ctrl Pts',(4.52823787999994,2.2,0.222869938999986));
#345221=CARTESIAN_POINT('Ctrl Pts',(4.52615568099994,12.2,0.223858726999988));
#345222=CARTESIAN_POINT('Ctrl Pts',(4.52615568099994,5.2,0.223858726999988));
#345223=CARTESIAN_POINT('Ctrl Pts',(4.52615568099994,2.2,0.223858726999988));
#345224=CARTESIAN_POINT('Ctrl Pts',(4.52407579499994,12.2,0.224843676999988));
#345225=CARTESIAN_POINT('Ctrl Pts',(4.52407579499994,5.2,0.224843676999988));
#345226=CARTESIAN_POINT('Ctrl Pts',(4.52407579499994,2.2,0.224843676999988));
#345227=CARTESIAN_POINT('Ctrl Pts',(4.52199822999994,12.2,0.225824792999987));
#345228=CARTESIAN_POINT('Ctrl Pts',(4.52199822999994,5.2,0.225824792999987));
#345229=CARTESIAN_POINT('Ctrl Pts',(4.52199822999994,2.2,0.225824792999987));
#345230=CARTESIAN_POINT('Ctrl Pts',(4.51992299599994,12.2,0.226802076999988));
#345231=CARTESIAN_POINT('Ctrl Pts',(4.51992299599994,5.2,0.226802076999988));
#345232=CARTESIAN_POINT('Ctrl Pts',(4.51992299599994,2.2,0.226802076999988));
#345233=CARTESIAN_POINT('Ctrl Pts',(4.51785010199994,12.2,0.227775534999988));
#345234=CARTESIAN_POINT('Ctrl Pts',(4.51785010199994,5.2,0.227775534999988));
#345235=CARTESIAN_POINT('Ctrl Pts',(4.51785010199994,2.2,0.227775534999988));
#345236=CARTESIAN_POINT('Ctrl Pts',(4.51577955699995,12.2,0.228745167999986));
#345237=CARTESIAN_POINT('Ctrl Pts',(4.51577955699995,5.2,0.228745167999986));
#345238=CARTESIAN_POINT('Ctrl Pts',(4.51577955699995,2.2,0.228745167999986));
#345239=CARTESIAN_POINT('Ctrl Pts',(4.51371136899994,12.2,0.229710981999984));
#345240=CARTESIAN_POINT('Ctrl Pts',(4.51371136899994,5.2,0.229710981999984));
#345241=CARTESIAN_POINT('Ctrl Pts',(4.51371136899994,2.2,0.229710981999984));
#345242=CARTESIAN_POINT('Ctrl Pts',(4.51164554799994,12.2,0.230672978999986));
#345243=CARTESIAN_POINT('Ctrl Pts',(4.51164554799994,5.2,0.230672978999986));
#345244=CARTESIAN_POINT('Ctrl Pts',(4.51164554799994,2.2,0.230672978999986));
#345245=CARTESIAN_POINT('Ctrl Pts',(4.50958210299994,12.2,0.231631163999988));
#345246=CARTESIAN_POINT('Ctrl Pts',(4.50958210299994,5.2,0.231631163999988));
#345247=CARTESIAN_POINT('Ctrl Pts',(4.50958210299994,2.2,0.231631163999988));
#345248=CARTESIAN_POINT('Ctrl Pts',(4.50752104299994,12.2,0.232585539999985));
#345249=CARTESIAN_POINT('Ctrl Pts',(4.50752104299994,5.2,0.232585539999985));
#345250=CARTESIAN_POINT('Ctrl Pts',(4.50752104299994,2.2,0.232585539999985));
#345251=CARTESIAN_POINT('Ctrl Pts',(4.50546237799994,12.2,0.233536110999988));
#345252=CARTESIAN_POINT('Ctrl Pts',(4.50546237799994,5.2,0.233536110999988));
#345253=CARTESIAN_POINT('Ctrl Pts',(4.50546237799994,2.2,0.233536110999988));
#345254=CARTESIAN_POINT('Ctrl Pts',(4.50340611499994,12.2,0.234482879999987));
#345255=CARTESIAN_POINT('Ctrl Pts',(4.50340611499994,5.2,0.234482879999987));
#345256=CARTESIAN_POINT('Ctrl Pts',(4.50340611499994,2.2,0.234482879999987));
#345257=CARTESIAN_POINT('Ctrl Pts',(4.50135226499994,12.2,0.235425850999986));
#345258=CARTESIAN_POINT('Ctrl Pts',(4.50135226499994,5.2,0.235425850999986));
#345259=CARTESIAN_POINT('Ctrl Pts',(4.50135226499994,2.2,0.235425850999986));
#345260=CARTESIAN_POINT('Ctrl Pts',(4.49930083599994,12.2,0.236365028999987));
#345261=CARTESIAN_POINT('Ctrl Pts',(4.49930083599994,5.2,0.236365028999987));
#345262=CARTESIAN_POINT('Ctrl Pts',(4.49930083599994,2.2,0.236365028999987));
#345263=CARTESIAN_POINT('Ctrl Pts',(4.49725183699995,12.2,0.237300414999986));
#345264=CARTESIAN_POINT('Ctrl Pts',(4.49725183699995,5.2,0.237300414999986));
#345265=CARTESIAN_POINT('Ctrl Pts',(4.49725183699995,2.2,0.237300414999986));
#345266=CARTESIAN_POINT('Ctrl Pts',(4.49520527799994,12.2,0.238232014999986));
#345267=CARTESIAN_POINT('Ctrl Pts',(4.49520527799994,5.2,0.238232014999986));
#345268=CARTESIAN_POINT('Ctrl Pts',(4.49520527799994,2.2,0.238232014999986));
#345269=CARTESIAN_POINT('Ctrl Pts',(4.49316116899994,12.2,0.239159833999985));
#345270=CARTESIAN_POINT('Ctrl Pts',(4.49316116899994,5.2,0.239159833999985));
#345271=CARTESIAN_POINT('Ctrl Pts',(4.49316116899994,2.2,0.239159833999985));
#345272=CARTESIAN_POINT('Ctrl Pts',(4.49111951599994,12.2,0.240083871999985));
#345273=CARTESIAN_POINT('Ctrl Pts',(4.49111951599994,5.2,0.240083871999985));
#345274=CARTESIAN_POINT('Ctrl Pts',(4.49111951599994,2.2,0.240083871999985));
#345275=CARTESIAN_POINT('Ctrl Pts',(4.48908033099995,12.2,0.241004136999985));
#345276=CARTESIAN_POINT('Ctrl Pts',(4.48908033099995,5.2,0.241004136999985));
#345277=CARTESIAN_POINT('Ctrl Pts',(4.48908033099995,2.2,0.241004136999985));
#345278=CARTESIAN_POINT('Ctrl Pts',(4.48704362299994,12.2,0.241920629999988));
#345279=CARTESIAN_POINT('Ctrl Pts',(4.48704362299994,5.2,0.241920629999988));
#345280=CARTESIAN_POINT('Ctrl Pts',(4.48704362299994,2.2,0.241920629999988));
#345281=CARTESIAN_POINT('Ctrl Pts',(4.48500939999994,12.2,0.242833354999985));
#345282=CARTESIAN_POINT('Ctrl Pts',(4.48500939999994,5.2,0.242833354999985));
#345283=CARTESIAN_POINT('Ctrl Pts',(4.48500939999994,2.2,0.242833354999985));
#345284=CARTESIAN_POINT('Ctrl Pts',(4.48297766999994,12.2,0.243742316999986));
#345285=CARTESIAN_POINT('Ctrl Pts',(4.48297766999994,5.2,0.243742316999986));
#345286=CARTESIAN_POINT('Ctrl Pts',(4.48297766999994,2.2,0.243742316999986));
#345287=CARTESIAN_POINT('Ctrl Pts',(4.48094844499995,12.2,0.244647520999983));
#345288=CARTESIAN_POINT('Ctrl Pts',(4.48094844499995,5.2,0.244647520999983));
#345289=CARTESIAN_POINT('Ctrl Pts',(4.48094844499995,2.2,0.244647520999983));
#345290=CARTESIAN_POINT('Ctrl Pts',(4.47892173299994,12.2,0.245548966999984));
#345291=CARTESIAN_POINT('Ctrl Pts',(4.47892173299994,5.2,0.245548966999984));
#345292=CARTESIAN_POINT('Ctrl Pts',(4.47892173299994,2.2,0.245548966999984));
#345293=CARTESIAN_POINT('Ctrl Pts',(4.47689754399994,12.2,0.246446662999986));
#345294=CARTESIAN_POINT('Ctrl Pts',(4.47689754399994,5.2,0.246446662999986));
#345295=CARTESIAN_POINT('Ctrl Pts',(4.47689754399994,2.2,0.246446662999986));
#345296=CARTESIAN_POINT('Ctrl Pts',(4.47487588399994,12.2,0.247340611999984));
#345297=CARTESIAN_POINT('Ctrl Pts',(4.47487588399994,5.2,0.247340611999984));
#345298=CARTESIAN_POINT('Ctrl Pts',(4.47487588399994,2.2,0.247340611999984));
#345299=CARTESIAN_POINT('Ctrl Pts',(4.47285676699994,12.2,0.248230816999988));
#345300=CARTESIAN_POINT('Ctrl Pts',(4.47285676699994,5.2,0.248230816999988));
#345301=CARTESIAN_POINT('Ctrl Pts',(4.47285676699994,2.2,0.248230816999988));
#345302=CARTESIAN_POINT('Ctrl Pts',(4.47084019799994,12.2,0.249117281999984));
#345303=CARTESIAN_POINT('Ctrl Pts',(4.47084019799994,5.2,0.249117281999984));
#345304=CARTESIAN_POINT('Ctrl Pts',(4.47084019799994,2.2,0.249117281999984));
#345305=CARTESIAN_POINT('Ctrl Pts',(4.46882618799994,12.2,0.250000010999987));
#345306=CARTESIAN_POINT('Ctrl Pts',(4.46882618799994,5.2,0.250000010999987));
#345307=CARTESIAN_POINT('Ctrl Pts',(4.46882618799994,2.2,0.250000010999987));
#345308=CARTESIAN_POINT('Ctrl Pts',(4.46681474699994,12.2,0.250879009999987));
#345309=CARTESIAN_POINT('Ctrl Pts',(4.46681474699994,5.2,0.250879009999987));
#345310=CARTESIAN_POINT('Ctrl Pts',(4.46681474699994,2.2,0.250879009999987));
#345311=CARTESIAN_POINT('Ctrl Pts',(4.46480588299994,12.2,0.251754280999985));
#345312=CARTESIAN_POINT('Ctrl Pts',(4.46480588299994,5.2,0.251754280999985));
#345313=CARTESIAN_POINT('Ctrl Pts',(4.46480588299994,2.2,0.251754280999985));
#345314=CARTESIAN_POINT('Ctrl Pts',(4.46279960599994,12.2,0.252625828999986));
#345315=CARTESIAN_POINT('Ctrl Pts',(4.46279960599994,5.2,0.252625828999986));
#345316=CARTESIAN_POINT('Ctrl Pts',(4.46279960599994,2.2,0.252625828999986));
#345317=CARTESIAN_POINT('Ctrl Pts',(4.46079592399994,12.2,0.253493656999986));
#345318=CARTESIAN_POINT('Ctrl Pts',(4.46079592399994,5.2,0.253493656999986));
#345319=CARTESIAN_POINT('Ctrl Pts',(4.46079592399994,2.2,0.253493656999986));
#345320=CARTESIAN_POINT('Ctrl Pts',(4.45879484899994,12.2,0.254357769999984));
#345321=CARTESIAN_POINT('Ctrl Pts',(4.45879484899994,5.2,0.254357769999984));
#345322=CARTESIAN_POINT('Ctrl Pts',(4.45879484899994,2.2,0.254357769999984));
#345323=CARTESIAN_POINT('Ctrl Pts',(4.45679638699994,12.2,0.255218172999987));
#345324=CARTESIAN_POINT('Ctrl Pts',(4.45679638699994,5.2,0.255218172999987));
#345325=CARTESIAN_POINT('Ctrl Pts',(4.45679638699994,2.2,0.255218172999987));
#345326=CARTESIAN_POINT('Ctrl Pts',(4.45480054899994,12.2,0.256074867999985));
#345327=CARTESIAN_POINT('Ctrl Pts',(4.45480054899994,5.2,0.256074867999985));
#345328=CARTESIAN_POINT('Ctrl Pts',(4.45480054899994,2.2,0.256074867999985));
#345329=CARTESIAN_POINT('Ctrl Pts',(4.45280734399994,12.2,0.256927860999987));
#345330=CARTESIAN_POINT('Ctrl Pts',(4.45280734399994,5.2,0.256927860999987));
#345331=CARTESIAN_POINT('Ctrl Pts',(4.45280734399994,2.2,0.256927860999987));
#345332=CARTESIAN_POINT('Ctrl Pts',(4.45081678199994,12.2,0.257777155999985));
#345333=CARTESIAN_POINT('Ctrl Pts',(4.45081678199994,5.2,0.257777155999985));
#345334=CARTESIAN_POINT('Ctrl Pts',(4.45081678199994,2.2,0.257777155999985));
#345335=CARTESIAN_POINT('Ctrl Pts',(4.44882887099994,12.2,0.258622755999984));
#345336=CARTESIAN_POINT('Ctrl Pts',(4.44882887099994,5.2,0.258622755999984));
#345337=CARTESIAN_POINT('Ctrl Pts',(4.44882887099994,2.2,0.258622755999984));
#345338=CARTESIAN_POINT('Ctrl Pts',(4.44684362099994,12.2,0.259464666999989));
#345339=CARTESIAN_POINT('Ctrl Pts',(4.44684362099994,5.2,0.259464666999989));
#345340=CARTESIAN_POINT('Ctrl Pts',(4.44684362099994,2.2,0.259464666999989));
#345341=CARTESIAN_POINT('Ctrl Pts',(4.44486104099994,12.2,0.260302891999986));
#345342=CARTESIAN_POINT('Ctrl Pts',(4.44486104099994,5.2,0.260302891999986));
#345343=CARTESIAN_POINT('Ctrl Pts',(4.44486104099994,2.2,0.260302891999986));
#345344=CARTESIAN_POINT('Ctrl Pts',(4.44288114199994,12.2,0.261137435999985));
#345345=CARTESIAN_POINT('Ctrl Pts',(4.44288114199994,5.2,0.261137435999985));
#345346=CARTESIAN_POINT('Ctrl Pts',(4.44288114199994,2.2,0.261137435999985));
#345347=CARTESIAN_POINT('Ctrl Pts',(4.44090392999995,12.2,0.261968301999986));
#345348=CARTESIAN_POINT('Ctrl Pts',(4.44090392999995,5.2,0.261968301999986));
#345349=CARTESIAN_POINT('Ctrl Pts',(4.44090392999995,2.2,0.261968301999986));
#345350=CARTESIAN_POINT('Ctrl Pts',(4.43892941799994,12.2,0.262795494999986));
#345351=CARTESIAN_POINT('Ctrl Pts',(4.43892941799994,5.2,0.262795494999986));
#345352=CARTESIAN_POINT('Ctrl Pts',(4.43892941799994,2.2,0.262795494999986));
#345353=CARTESIAN_POINT('Ctrl Pts',(4.43695761199994,12.2,0.263619019999983));
#345354=CARTESIAN_POINT('Ctrl Pts',(4.43695761199994,5.2,0.263619019999983));
#345355=CARTESIAN_POINT('Ctrl Pts',(4.43695761199994,2.2,0.263619019999983));
#345356=CARTESIAN_POINT('Ctrl Pts',(4.43498852499994,12.2,0.264438880999984));
#345357=CARTESIAN_POINT('Ctrl Pts',(4.43498852499994,5.2,0.264438880999984));
#345358=CARTESIAN_POINT('Ctrl Pts',(4.43498852499994,2.2,0.264438880999984));
#345359=CARTESIAN_POINT('Ctrl Pts',(4.43302216299994,12.2,0.265255081999989));
#345360=CARTESIAN_POINT('Ctrl Pts',(4.43302216299994,5.2,0.265255081999989));
#345361=CARTESIAN_POINT('Ctrl Pts',(4.43302216299994,2.2,0.265255081999989));
#345362=CARTESIAN_POINT('Ctrl Pts',(4.43105853599994,12.2,0.266067626999984));
#345363=CARTESIAN_POINT('Ctrl Pts',(4.43105853599994,5.2,0.266067626999984));
#345364=CARTESIAN_POINT('Ctrl Pts',(4.43105853599994,2.2,0.266067626999984));
#345365=CARTESIAN_POINT('Ctrl Pts',(4.42909765599994,12.2,0.266876522999984));
#345366=CARTESIAN_POINT('Ctrl Pts',(4.42909765599994,5.2,0.266876522999984));
#345367=CARTESIAN_POINT('Ctrl Pts',(4.42909765599994,2.2,0.266876522999984));
#345368=CARTESIAN_POINT('Ctrl Pts',(4.42713952999994,12.2,0.267681770999988));
#345369=CARTESIAN_POINT('Ctrl Pts',(4.42713952999994,5.2,0.267681770999988));
#345370=CARTESIAN_POINT('Ctrl Pts',(4.42713952999994,2.2,0.267681770999988));
#345371=CARTESIAN_POINT('Ctrl Pts',(4.42518416699994,12.2,0.268483376999988));
#345372=CARTESIAN_POINT('Ctrl Pts',(4.42518416699994,5.2,0.268483376999988));
#345373=CARTESIAN_POINT('Ctrl Pts',(4.42518416699994,2.2,0.268483376999988));
#345374=CARTESIAN_POINT('Ctrl Pts',(4.42323157799995,12.2,0.269281345999985));
#345375=CARTESIAN_POINT('Ctrl Pts',(4.42323157799995,5.2,0.269281345999985));
#345376=CARTESIAN_POINT('Ctrl Pts',(4.42323157799995,2.2,0.269281345999985));
#345377=CARTESIAN_POINT('Ctrl Pts',(4.42128177099994,12.2,0.270075680999984));
#345378=CARTESIAN_POINT('Ctrl Pts',(4.42128177099994,5.2,0.270075680999984));
#345379=CARTESIAN_POINT('Ctrl Pts',(4.42128177099994,2.2,0.270075680999984));
#345380=CARTESIAN_POINT('Ctrl Pts',(4.41933475699994,12.2,0.270866387999984));
#345381=CARTESIAN_POINT('Ctrl Pts',(4.41933475699994,5.2,0.270866387999984));
#345382=CARTESIAN_POINT('Ctrl Pts',(4.41933475699994,2.2,0.270866387999984));
#345383=CARTESIAN_POINT('Ctrl Pts',(4.41739054399994,12.2,0.271653470999986));
#345384=CARTESIAN_POINT('Ctrl Pts',(4.41739054399994,5.2,0.271653470999986));
#345385=CARTESIAN_POINT('Ctrl Pts',(4.41739054399994,2.2,0.271653470999986));
#345386=CARTESIAN_POINT('Ctrl Pts',(4.41544914199994,12.2,0.272436934999987));
#345387=CARTESIAN_POINT('Ctrl Pts',(4.41544914199994,5.2,0.272436934999987));
#345388=CARTESIAN_POINT('Ctrl Pts',(4.41544914199994,2.2,0.272436934999987));
#345389=CARTESIAN_POINT('Ctrl Pts',(4.41351056199994,12.2,0.273216782999985));
#345390=CARTESIAN_POINT('Ctrl Pts',(4.41351056199994,5.2,0.273216782999985));
#345391=CARTESIAN_POINT('Ctrl Pts',(4.41351056199994,2.2,0.273216782999985));
#345392=CARTESIAN_POINT('Ctrl Pts',(4.41157481099994,12.2,0.273993020999987));
#345393=CARTESIAN_POINT('Ctrl Pts',(4.41157481099994,5.2,0.273993020999987));
#345394=CARTESIAN_POINT('Ctrl Pts',(4.41157481099994,2.2,0.273993020999987));
#345395=CARTESIAN_POINT('Ctrl Pts',(4.40964189899994,12.2,0.274765652999989));
#345396=CARTESIAN_POINT('Ctrl Pts',(4.40964189899994,5.2,0.274765652999989));
#345397=CARTESIAN_POINT('Ctrl Pts',(4.40964189899994,2.2,0.274765652999989));
#345398=CARTESIAN_POINT('Ctrl Pts',(4.40771183599994,12.2,0.275534683999985));
#345399=CARTESIAN_POINT('Ctrl Pts',(4.40771183599994,5.2,0.275534683999985));
#345400=CARTESIAN_POINT('Ctrl Pts',(4.40771183599994,2.2,0.275534683999985));
#345401=CARTESIAN_POINT('Ctrl Pts',(4.40578463099994,12.2,0.276300118999986));
#345402=CARTESIAN_POINT('Ctrl Pts',(4.40578463099994,5.2,0.276300118999986));
#345403=CARTESIAN_POINT('Ctrl Pts',(4.40578463099994,2.2,0.276300118999986));
#345404=CARTESIAN_POINT('Ctrl Pts',(4.40386029399995,12.2,0.277061960999987));
#345405=CARTESIAN_POINT('Ctrl Pts',(4.40386029399995,5.2,0.277061960999987));
#345406=CARTESIAN_POINT('Ctrl Pts',(4.40386029399995,2.2,0.277061960999987));
#345407=CARTESIAN_POINT('Ctrl Pts',(4.40193883499994,12.2,0.277820216999984));
#345408=CARTESIAN_POINT('Ctrl Pts',(4.40193883499994,5.2,0.277820216999984));
#345409=CARTESIAN_POINT('Ctrl Pts',(4.40193883499994,2.2,0.277820216999984));
#345410=CARTESIAN_POINT('Ctrl Pts',(4.40002026299994,12.2,0.278574889999987));
#345411=CARTESIAN_POINT('Ctrl Pts',(4.40002026299994,5.2,0.278574889999987));
#345412=CARTESIAN_POINT('Ctrl Pts',(4.40002026299994,2.2,0.278574889999987));
#345413=CARTESIAN_POINT('Ctrl Pts',(4.39810458599994,12.2,0.279325985999983));
#345414=CARTESIAN_POINT('Ctrl Pts',(4.39810458599994,5.2,0.279325985999983));
#345415=CARTESIAN_POINT('Ctrl Pts',(4.39810458599994,2.2,0.279325985999983));
#345416=CARTESIAN_POINT('Ctrl Pts',(4.39619181599994,12.2,0.280073507999985));
#345417=CARTESIAN_POINT('Ctrl Pts',(4.39619181599994,5.2,0.280073507999985));
#345418=CARTESIAN_POINT('Ctrl Pts',(4.39619181599994,2.2,0.280073507999985));
#345419=CARTESIAN_POINT('Ctrl Pts',(4.39428196099994,12.2,0.280817461999985));
#345420=CARTESIAN_POINT('Ctrl Pts',(4.39428196099994,5.2,0.280817461999985));
#345421=CARTESIAN_POINT('Ctrl Pts',(4.39428196099994,2.2,0.280817461999985));
#345422=CARTESIAN_POINT('Ctrl Pts',(4.39237503099995,12.2,0.281557852999987));
#345423=CARTESIAN_POINT('Ctrl Pts',(4.39237503099995,5.2,0.281557852999987));
#345424=CARTESIAN_POINT('Ctrl Pts',(4.39237503099995,2.2,0.281557852999987));
#345425=CARTESIAN_POINT('Ctrl Pts',(4.39047103599994,12.2,0.282294684999984));
#345426=CARTESIAN_POINT('Ctrl Pts',(4.39047103599994,5.2,0.282294684999984));
#345427=CARTESIAN_POINT('Ctrl Pts',(4.39047103599994,2.2,0.282294684999984));
#345428=CARTESIAN_POINT('Ctrl Pts',(4.38856998399995,12.2,0.283027963999984));
#345429=CARTESIAN_POINT('Ctrl Pts',(4.38856998399995,5.2,0.283027963999984));
#345430=CARTESIAN_POINT('Ctrl Pts',(4.38856998399995,2.2,0.283027963999984));
#345431=CARTESIAN_POINT('Ctrl Pts',(4.38667188599995,12.2,0.283757692999984));
#345432=CARTESIAN_POINT('Ctrl Pts',(4.38667188599995,5.2,0.283757692999984));
#345433=CARTESIAN_POINT('Ctrl Pts',(4.38667188599995,2.2,0.283757692999984));
#345434=CARTESIAN_POINT('Ctrl Pts',(4.38477675099994,12.2,0.284483878999984));
#345435=CARTESIAN_POINT('Ctrl Pts',(4.38477675099994,5.2,0.284483878999984));
#345436=CARTESIAN_POINT('Ctrl Pts',(4.38477675099994,2.2,0.284483878999984));
#345437=CARTESIAN_POINT('Ctrl Pts',(4.38288458899994,12.2,0.285206524999988));
#345438=CARTESIAN_POINT('Ctrl Pts',(4.38288458899994,5.2,0.285206524999988));
#345439=CARTESIAN_POINT('Ctrl Pts',(4.38288458899994,2.2,0.285206524999988));
#345440=CARTESIAN_POINT('Ctrl Pts',(4.38099540999994,12.2,0.285925636999984));
#345441=CARTESIAN_POINT('Ctrl Pts',(4.38099540999994,5.2,0.285925636999984));
#345442=CARTESIAN_POINT('Ctrl Pts',(4.38099540999994,2.2,0.285925636999984));
#345443=CARTESIAN_POINT('Ctrl Pts',(4.37910922299994,12.2,0.286641219999986));
#345444=CARTESIAN_POINT('Ctrl Pts',(4.37910922299994,5.2,0.286641219999986));
#345445=CARTESIAN_POINT('Ctrl Pts',(4.37910922299994,2.2,0.286641219999986));
#345446=CARTESIAN_POINT('Ctrl Pts',(4.37722603699994,12.2,0.287353278999984));
#345447=CARTESIAN_POINT('Ctrl Pts',(4.37722603699994,5.2,0.287353278999984));
#345448=CARTESIAN_POINT('Ctrl Pts',(4.37722603699994,2.2,0.287353278999984));
#345449=CARTESIAN_POINT('Ctrl Pts',(4.37534586199994,12.2,0.288061817999985));
#345450=CARTESIAN_POINT('Ctrl Pts',(4.37534586199994,5.2,0.288061817999985));
#345451=CARTESIAN_POINT('Ctrl Pts',(4.37534586199994,2.2,0.288061817999985));
#345452=CARTESIAN_POINT('Ctrl Pts',(4.37346870799994,12.2,0.288766842999983));
#345453=CARTESIAN_POINT('Ctrl Pts',(4.37346870799994,5.2,0.288766842999983));
#345454=CARTESIAN_POINT('Ctrl Pts',(4.37346870799994,2.2,0.288766842999983));
#345455=CARTESIAN_POINT('Ctrl Pts',(4.37159458399995,12.2,0.289468358999985));
#345456=CARTESIAN_POINT('Ctrl Pts',(4.37159458399995,5.2,0.289468358999985));
#345457=CARTESIAN_POINT('Ctrl Pts',(4.37159458399995,2.2,0.289468358999985));
#345458=CARTESIAN_POINT('Ctrl Pts',(4.36972350099994,12.2,0.290166369999985));
#345459=CARTESIAN_POINT('Ctrl Pts',(4.36972350099994,5.2,0.290166369999985));
#345460=CARTESIAN_POINT('Ctrl Pts',(4.36972350099994,2.2,0.290166369999985));
#345461=CARTESIAN_POINT('Ctrl Pts',(4.36785546599994,12.2,0.290860881999984));
#345462=CARTESIAN_POINT('Ctrl Pts',(4.36785546599994,5.2,0.290860881999984));
#345463=CARTESIAN_POINT('Ctrl Pts',(4.36785546599994,2.2,0.290860881999984));
#345464=CARTESIAN_POINT('Ctrl Pts',(4.36599049299994,12.2,0.291551899999987));
#345465=CARTESIAN_POINT('Ctrl Pts',(4.36599049299994,5.2,0.291551899999987));
#345466=CARTESIAN_POINT('Ctrl Pts',(4.36599049299994,2.2,0.291551899999987));
#345467=CARTESIAN_POINT('Ctrl Pts',(4.36412858699994,12.2,0.292239427999985));
#345468=CARTESIAN_POINT('Ctrl Pts',(4.36412858699994,5.2,0.292239427999985));
#345469=CARTESIAN_POINT('Ctrl Pts',(4.36412858699994,2.2,0.292239427999985));
#345470=CARTESIAN_POINT('Ctrl Pts',(4.36226975999995,12.2,0.292923472999984));
#345471=CARTESIAN_POINT('Ctrl Pts',(4.36226975999995,5.2,0.292923472999984));
#345472=CARTESIAN_POINT('Ctrl Pts',(4.36226975999995,2.2,0.292923472999984));
#345473=CARTESIAN_POINT('Ctrl Pts',(4.36041402199994,12.2,0.293604038999984));
#345474=CARTESIAN_POINT('Ctrl Pts',(4.36041402199994,5.2,0.293604038999984));
#345475=CARTESIAN_POINT('Ctrl Pts',(4.36041402199994,2.2,0.293604038999984));
#345476=CARTESIAN_POINT('Ctrl Pts',(4.35856138199994,12.2,0.294281131999985));
#345477=CARTESIAN_POINT('Ctrl Pts',(4.35856138199994,5.2,0.294281131999985));
#345478=CARTESIAN_POINT('Ctrl Pts',(4.35856138199994,2.2,0.294281131999985));
#345479=CARTESIAN_POINT('Ctrl Pts',(4.35671184899994,12.2,0.294954754999988));
#345480=CARTESIAN_POINT('Ctrl Pts',(4.35671184899994,5.2,0.294954754999988));
#345481=CARTESIAN_POINT('Ctrl Pts',(4.35671184899994,2.2,0.294954754999988));
#345482=CARTESIAN_POINT('Ctrl Pts',(4.35486543399994,12.2,0.295624915999984));
#345483=CARTESIAN_POINT('Ctrl Pts',(4.35486543399994,5.2,0.295624915999984));
#345484=CARTESIAN_POINT('Ctrl Pts',(4.35486543399994,2.2,0.295624915999984));
#345485=CARTESIAN_POINT('Ctrl Pts',(4.35302214599994,12.2,0.296291618999986));
#345486=CARTESIAN_POINT('Ctrl Pts',(4.35302214599994,5.2,0.296291618999986));
#345487=CARTESIAN_POINT('Ctrl Pts',(4.35302214599994,2.2,0.296291618999986));
#345488=CARTESIAN_POINT('Ctrl Pts',(4.35118199599995,12.2,0.296954867999983));
#345489=CARTESIAN_POINT('Ctrl Pts',(4.35118199599995,5.2,0.296954867999983));
#345490=CARTESIAN_POINT('Ctrl Pts',(4.35118199599995,2.2,0.296954867999983));
#345491=CARTESIAN_POINT('Ctrl Pts',(4.34934499099994,12.2,0.297614670999984));
#345492=CARTESIAN_POINT('Ctrl Pts',(4.34934499099994,5.2,0.297614670999984));
#345493=CARTESIAN_POINT('Ctrl Pts',(4.34934499099994,2.2,0.297614670999984));
#345494=CARTESIAN_POINT('Ctrl Pts',(4.34751114399995,12.2,0.298271030999988));
#345495=CARTESIAN_POINT('Ctrl Pts',(4.34751114399995,5.2,0.298271030999988));
#345496=CARTESIAN_POINT('Ctrl Pts',(4.34751114399995,2.2,0.298271030999988));
#345497=CARTESIAN_POINT('Ctrl Pts',(4.34568046199994,12.2,0.298923954999988));
#345498=CARTESIAN_POINT('Ctrl Pts',(4.34568046199994,5.2,0.298923954999988));
#345499=CARTESIAN_POINT('Ctrl Pts',(4.34568046199994,2.2,0.298923954999988));
#345500=CARTESIAN_POINT('Ctrl Pts',(4.34385295599994,12.2,0.299573446999983));
#345501=CARTESIAN_POINT('Ctrl Pts',(4.34385295599994,5.2,0.299573446999983));
#345502=CARTESIAN_POINT('Ctrl Pts',(4.34385295599994,2.2,0.299573446999983));
#345503=CARTESIAN_POINT('Ctrl Pts',(4.34202863699995,12.2,0.300219512999984));
#345504=CARTESIAN_POINT('Ctrl Pts',(4.34202863699995,5.2,0.300219512999984));
#345505=CARTESIAN_POINT('Ctrl Pts',(4.34202863699995,2.2,0.300219512999984));
#345506=CARTESIAN_POINT('Ctrl Pts',(4.34020751199994,12.2,0.300862157999986));
#345507=CARTESIAN_POINT('Ctrl Pts',(4.34020751199994,5.2,0.300862157999986));
#345508=CARTESIAN_POINT('Ctrl Pts',(4.34020751199994,2.2,0.300862157999986));
#345509=CARTESIAN_POINT('Ctrl Pts',(4.33838959199994,12.2,0.301501387999985));
#345510=CARTESIAN_POINT('Ctrl Pts',(4.33838959199994,5.2,0.301501387999985));
#345511=CARTESIAN_POINT('Ctrl Pts',(4.33838959199994,2.2,0.301501387999985));
#345512=CARTESIAN_POINT('Ctrl Pts',(4.33657488799994,12.2,0.302137207999986));
#345513=CARTESIAN_POINT('Ctrl Pts',(4.33657488799994,5.2,0.302137207999986));
#345514=CARTESIAN_POINT('Ctrl Pts',(4.33657488799994,2.2,0.302137207999986));
#345515=CARTESIAN_POINT('Ctrl Pts',(4.33476340899994,12.2,0.302769622999985));
#345516=CARTESIAN_POINT('Ctrl Pts',(4.33476340899994,5.2,0.302769622999985));
#345517=CARTESIAN_POINT('Ctrl Pts',(4.33476340899994,2.2,0.302769622999985));
#345518=CARTESIAN_POINT('Ctrl Pts',(4.33295516399994,12.2,0.303398639999983));
#345519=CARTESIAN_POINT('Ctrl Pts',(4.33295516399994,5.2,0.303398639999983));
#345520=CARTESIAN_POINT('Ctrl Pts',(4.33295516399994,2.2,0.303398639999983));
#345521=CARTESIAN_POINT('Ctrl Pts',(4.33115016299995,12.2,0.304024262999985));
#345522=CARTESIAN_POINT('Ctrl Pts',(4.33115016299995,5.2,0.304024262999985));
#345523=CARTESIAN_POINT('Ctrl Pts',(4.33115016299995,2.2,0.304024262999985));
#345524=CARTESIAN_POINT('Ctrl Pts',(4.32934841799994,12.2,0.304646498999985));
#345525=CARTESIAN_POINT('Ctrl Pts',(4.32934841799994,5.2,0.304646498999985));
#345526=CARTESIAN_POINT('Ctrl Pts',(4.32934841799994,2.2,0.304646498999985));
#345527=CARTESIAN_POINT('Ctrl Pts',(4.32754993599994,12.2,0.305265350999986));
#345528=CARTESIAN_POINT('Ctrl Pts',(4.32754993599994,5.2,0.305265350999986));
#345529=CARTESIAN_POINT('Ctrl Pts',(4.32754993599994,2.2,0.305265350999986));
#345530=CARTESIAN_POINT('Ctrl Pts',(4.32575472799994,12.2,0.305880825999987));
#345531=CARTESIAN_POINT('Ctrl Pts',(4.32575472799994,5.2,0.305880825999987));
#345532=CARTESIAN_POINT('Ctrl Pts',(4.32575472799994,2.2,0.305880825999987));
#345533=CARTESIAN_POINT('Ctrl Pts',(4.32396280299994,12.2,0.306492931999984));
#345534=CARTESIAN_POINT('Ctrl Pts',(4.32396280299994,5.2,0.306492931999984));
#345535=CARTESIAN_POINT('Ctrl Pts',(4.32396280299994,2.2,0.306492931999984));
#345536=CARTESIAN_POINT('Ctrl Pts',(4.32217417299994,12.2,0.307101670999987));
#345537=CARTESIAN_POINT('Ctrl Pts',(4.32217417299994,5.2,0.307101670999987));
#345538=CARTESIAN_POINT('Ctrl Pts',(4.32217417299994,2.2,0.307101670999987));
#345539=CARTESIAN_POINT('Ctrl Pts',(4.32038884599994,12.2,0.307707049999983));
#345540=CARTESIAN_POINT('Ctrl Pts',(4.32038884599994,5.2,0.307707049999983));
#345541=CARTESIAN_POINT('Ctrl Pts',(4.32038884599994,2.2,0.307707049999983));
#345542=CARTESIAN_POINT('Ctrl Pts',(4.31860683299994,12.2,0.308309073999986));
#345543=CARTESIAN_POINT('Ctrl Pts',(4.31860683299994,5.2,0.308309073999986));
#345544=CARTESIAN_POINT('Ctrl Pts',(4.31860683299994,2.2,0.308309073999986));
#345545=CARTESIAN_POINT('Ctrl Pts',(4.31682814299994,12.2,0.308907748999987));
#345546=CARTESIAN_POINT('Ctrl Pts',(4.31682814299994,5.2,0.308907748999987));
#345547=CARTESIAN_POINT('Ctrl Pts',(4.31682814299994,2.2,0.308907748999987));
#345548=CARTESIAN_POINT('Ctrl Pts',(4.31505278699994,12.2,0.309503082999987));
#345549=CARTESIAN_POINT('Ctrl Pts',(4.31505278699994,5.2,0.309503082999987));
#345550=CARTESIAN_POINT('Ctrl Pts',(4.31505278699994,2.2,0.309503082999987));
#345551=CARTESIAN_POINT('Ctrl Pts',(4.31328077299994,12.2,0.310095078999986));
#345552=CARTESIAN_POINT('Ctrl Pts',(4.31328077299994,5.2,0.310095078999986));
#345553=CARTESIAN_POINT('Ctrl Pts',(4.31328077299994,2.2,0.310095078999986));
#345554=CARTESIAN_POINT('Ctrl Pts',(4.31151211199994,12.2,0.310683742999984));
#345555=CARTESIAN_POINT('Ctrl Pts',(4.31151211199994,5.2,0.310683742999984));
#345556=CARTESIAN_POINT('Ctrl Pts',(4.31151211199994,2.2,0.310683742999984));
#345557=CARTESIAN_POINT('Ctrl Pts',(4.30974681499994,12.2,0.311269080999987));
#345558=CARTESIAN_POINT('Ctrl Pts',(4.30974681499994,5.2,0.311269080999987));
#345559=CARTESIAN_POINT('Ctrl Pts',(4.30974681499994,2.2,0.311269080999987));
#345560=CARTESIAN_POINT('Ctrl Pts',(4.30798488999994,12.2,0.311851100999987));
#345561=CARTESIAN_POINT('Ctrl Pts',(4.30798488999994,5.2,0.311851100999987));
#345562=CARTESIAN_POINT('Ctrl Pts',(4.30798488999994,2.2,0.311851100999987));
#345563=CARTESIAN_POINT('Ctrl Pts',(4.30622634899995,12.2,0.312429804999983));
#345564=CARTESIAN_POINT('Ctrl Pts',(4.30622634899995,5.2,0.312429804999983));
#345565=CARTESIAN_POINT('Ctrl Pts',(4.30622634899995,2.2,0.312429804999983));
#345566=CARTESIAN_POINT('Ctrl Pts',(4.30447119999994,12.2,0.313005201999985));
#345567=CARTESIAN_POINT('Ctrl Pts',(4.30447119999994,5.2,0.313005201999985));
#345568=CARTESIAN_POINT('Ctrl Pts',(4.30447119999994,2.2,0.313005201999985));
#345569=CARTESIAN_POINT('Ctrl Pts',(4.30271945399994,12.2,0.313577295999985));
#345570=CARTESIAN_POINT('Ctrl Pts',(4.30271945399994,5.2,0.313577295999985));
#345571=CARTESIAN_POINT('Ctrl Pts',(4.30271945399994,2.2,0.313577295999985));
#345572=CARTESIAN_POINT('Ctrl Pts',(4.30097112099994,12.2,0.314146092999987));
#345573=CARTESIAN_POINT('Ctrl Pts',(4.30097112099994,5.2,0.314146092999987));
#345574=CARTESIAN_POINT('Ctrl Pts',(4.30097112099994,2.2,0.314146092999987));
#345575=CARTESIAN_POINT('Ctrl Pts',(4.29922621099994,12.2,0.314711599999988));
#345576=CARTESIAN_POINT('Ctrl Pts',(4.29922621099994,5.2,0.314711599999988));
#345577=CARTESIAN_POINT('Ctrl Pts',(4.29922621099994,2.2,0.314711599999988));
#345578=CARTESIAN_POINT('Ctrl Pts',(4.29748473299994,12.2,0.315273821999984));
#345579=CARTESIAN_POINT('Ctrl Pts',(4.29748473299994,5.2,0.315273821999984));
#345580=CARTESIAN_POINT('Ctrl Pts',(4.29748473299994,2.2,0.315273821999984));
#345581=CARTESIAN_POINT('Ctrl Pts',(4.29574669799995,12.2,0.315832764999988));
#345582=CARTESIAN_POINT('Ctrl Pts',(4.29574669799995,5.2,0.315832764999988));
#345583=CARTESIAN_POINT('Ctrl Pts',(4.29574669799995,2.2,0.315832764999988));
#345584=CARTESIAN_POINT('Ctrl Pts',(4.29401211599994,12.2,0.316388435999984));
#345585=CARTESIAN_POINT('Ctrl Pts',(4.29401211599994,5.2,0.316388435999984));
#345586=CARTESIAN_POINT('Ctrl Pts',(4.29401211599994,2.2,0.316388435999984));
#345587=CARTESIAN_POINT('Ctrl Pts',(4.29228099699994,12.2,0.316940840999984));
#345588=CARTESIAN_POINT('Ctrl Pts',(4.29228099699994,5.2,0.316940840999984));
#345589=CARTESIAN_POINT('Ctrl Pts',(4.29228099699994,2.2,0.316940840999984));
#345590=CARTESIAN_POINT('Ctrl Pts',(4.29055334999994,12.2,0.317489983999986));
#345591=CARTESIAN_POINT('Ctrl Pts',(4.29055334999994,5.2,0.317489983999986));
#345592=CARTESIAN_POINT('Ctrl Pts',(4.29055334999994,2.2,0.317489983999986));
#345593=CARTESIAN_POINT('Ctrl Pts',(4.28882918699994,12.2,0.318035873999989));
#345594=CARTESIAN_POINT('Ctrl Pts',(4.28882918699994,5.2,0.318035873999989));
#345595=CARTESIAN_POINT('Ctrl Pts',(4.28882918699994,2.2,0.318035873999989));
#345596=CARTESIAN_POINT('Ctrl Pts',(4.28710851599994,12.2,0.318578514999985));
#345597=CARTESIAN_POINT('Ctrl Pts',(4.28710851599994,5.2,0.318578514999985));
#345598=CARTESIAN_POINT('Ctrl Pts',(4.28710851599994,2.2,0.318578514999985));
#345599=CARTESIAN_POINT('Ctrl Pts',(4.28539134799994,12.2,0.319117911999989));
#345600=CARTESIAN_POINT('Ctrl Pts',(4.28539134799994,5.2,0.319117911999989));
#345601=CARTESIAN_POINT('Ctrl Pts',(4.28539134799994,2.2,0.319117911999989));
#345602=CARTESIAN_POINT('Ctrl Pts',(4.28367769399994,12.2,0.319654074999987));
#345603=CARTESIAN_POINT('Ctrl Pts',(4.28367769399994,5.2,0.319654074999987));
#345604=CARTESIAN_POINT('Ctrl Pts',(4.28367769399994,2.2,0.319654074999987));
#345605=CARTESIAN_POINT('Ctrl Pts',(4.28196756099995,12.2,0.320187006999983));
#345606=CARTESIAN_POINT('Ctrl Pts',(4.28196756099995,5.2,0.320187006999983));
#345607=CARTESIAN_POINT('Ctrl Pts',(4.28196756099995,2.2,0.320187006999983));
#345608=CARTESIAN_POINT('Ctrl Pts',(4.28026096299994,12.2,0.320716713999989));
#345609=CARTESIAN_POINT('Ctrl Pts',(4.28026096299994,5.2,0.320716713999989));
#345610=CARTESIAN_POINT('Ctrl Pts',(4.28026096299994,2.2,0.320716713999989));
#345611=CARTESIAN_POINT('Ctrl Pts',(4.27855790799994,12.2,0.321243204999986));
#345612=CARTESIAN_POINT('Ctrl Pts',(4.27855790799994,5.2,0.321243204999986));
#345613=CARTESIAN_POINT('Ctrl Pts',(4.27855790799994,2.2,0.321243204999986));
#345614=CARTESIAN_POINT('Ctrl Pts',(4.27685840599994,12.2,0.321766483999983));
#345615=CARTESIAN_POINT('Ctrl Pts',(4.27685840599994,5.2,0.321766483999983));
#345616=CARTESIAN_POINT('Ctrl Pts',(4.27685840599994,2.2,0.321766483999983));
#345617=CARTESIAN_POINT('Ctrl Pts',(4.27516246799994,12.2,0.322286556999987));
#345618=CARTESIAN_POINT('Ctrl Pts',(4.27516246799994,5.2,0.322286556999987));
#345619=CARTESIAN_POINT('Ctrl Pts',(4.27516246799994,2.2,0.322286556999987));
#345620=CARTESIAN_POINT('Ctrl Pts',(4.27347010299994,12.2,0.322803431999983));
#345621=CARTESIAN_POINT('Ctrl Pts',(4.27347010299994,5.2,0.322803431999983));
#345622=CARTESIAN_POINT('Ctrl Pts',(4.27347010299994,2.2,0.322803431999983));
#345623=CARTESIAN_POINT('Ctrl Pts',(4.27178132099994,12.2,0.323317113999986));
#345624=CARTESIAN_POINT('Ctrl Pts',(4.27178132099994,5.2,0.323317113999986));
#345625=CARTESIAN_POINT('Ctrl Pts',(4.27178132099994,2.2,0.323317113999986));
#345626=CARTESIAN_POINT('Ctrl Pts',(4.27009613399994,12.2,0.323827609999987));
#345627=CARTESIAN_POINT('Ctrl Pts',(4.27009613399994,5.2,0.323827609999987));
#345628=CARTESIAN_POINT('Ctrl Pts',(4.27009613399994,2.2,0.323827609999987));
#345629=CARTESIAN_POINT('Ctrl Pts',(4.26841455099995,12.2,0.324334924999987));
#345630=CARTESIAN_POINT('Ctrl Pts',(4.26841455099995,5.2,0.324334924999987));
#345631=CARTESIAN_POINT('Ctrl Pts',(4.26841455099995,2.2,0.324334924999987));
#345632=CARTESIAN_POINT('Ctrl Pts',(4.26673658299995,12.2,0.324839067999987));
#345633=CARTESIAN_POINT('Ctrl Pts',(4.26673658299995,5.2,0.324839067999987));
#345634=CARTESIAN_POINT('Ctrl Pts',(4.26673658299995,2.2,0.324839067999987));
#345635=CARTESIAN_POINT('Ctrl Pts',(4.26506223899994,12.2,0.325340042999986));
#345636=CARTESIAN_POINT('Ctrl Pts',(4.26506223899994,5.2,0.325340042999986));
#345637=CARTESIAN_POINT('Ctrl Pts',(4.26506223899994,2.2,0.325340042999986));
#345638=CARTESIAN_POINT('Ctrl Pts',(4.26339152799994,12.2,0.325837856999982));
#345639=CARTESIAN_POINT('Ctrl Pts',(4.26339152799994,5.2,0.325837856999982));
#345640=CARTESIAN_POINT('Ctrl Pts',(4.26339152799994,2.2,0.325837856999982));
#345641=CARTESIAN_POINT('Ctrl Pts',(4.26172446299994,12.2,0.326332516999983));
#345642=CARTESIAN_POINT('Ctrl Pts',(4.26172446299994,5.2,0.326332516999983));
#345643=CARTESIAN_POINT('Ctrl Pts',(4.26172446299994,2.2,0.326332516999983));
#345644=CARTESIAN_POINT('Ctrl Pts',(4.26006105299995,12.2,0.326824029999986));
#345645=CARTESIAN_POINT('Ctrl Pts',(4.26006105299995,5.2,0.326824029999986));
#345646=CARTESIAN_POINT('Ctrl Pts',(4.26006105299995,2.2,0.326824029999986));
#345647=CARTESIAN_POINT('Ctrl Pts',(4.25840130699994,12.2,0.327312400999986));
#345648=CARTESIAN_POINT('Ctrl Pts',(4.25840130699994,5.2,0.327312400999986));
#345649=CARTESIAN_POINT('Ctrl Pts',(4.25840130699994,2.2,0.327312400999986));
#345650=CARTESIAN_POINT('Ctrl Pts',(4.25674523699994,12.2,0.327797636999985));
#345651=CARTESIAN_POINT('Ctrl Pts',(4.25674523699994,5.2,0.327797636999985));
#345652=CARTESIAN_POINT('Ctrl Pts',(4.25674523699994,2.2,0.327797636999985));
#345653=CARTESIAN_POINT('Ctrl Pts',(4.25509285299994,12.2,0.328279744999986));
#345654=CARTESIAN_POINT('Ctrl Pts',(4.25509285299994,5.2,0.328279744999986));
#345655=CARTESIAN_POINT('Ctrl Pts',(4.25509285299994,2.2,0.328279744999986));
#345656=CARTESIAN_POINT('Ctrl Pts',(4.25344416499995,12.2,0.328758731999983));
#345657=CARTESIAN_POINT('Ctrl Pts',(4.25344416499995,5.2,0.328758731999983));
#345658=CARTESIAN_POINT('Ctrl Pts',(4.25344416499995,2.2,0.328758731999983));
#345659=CARTESIAN_POINT('Ctrl Pts',(4.25179918199994,12.2,0.329234602999984));
#345660=CARTESIAN_POINT('Ctrl Pts',(4.25179918199994,5.2,0.329234602999984));
#345661=CARTESIAN_POINT('Ctrl Pts',(4.25179918199994,2.2,0.329234602999984));
#345662=CARTESIAN_POINT('Ctrl Pts',(4.25015791599994,12.2,0.329707365999985));
#345663=CARTESIAN_POINT('Ctrl Pts',(4.25015791599994,5.2,0.329707365999985));
#345664=CARTESIAN_POINT('Ctrl Pts',(4.25015791599994,2.2,0.329707365999985));
#345665=CARTESIAN_POINT('Ctrl Pts',(4.24852037599995,12.2,0.330177027999987));
#345666=CARTESIAN_POINT('Ctrl Pts',(4.24852037599995,5.2,0.330177027999987));
#345667=CARTESIAN_POINT('Ctrl Pts',(4.24852037599995,2.2,0.330177027999987));
#345668=CARTESIAN_POINT('Ctrl Pts',(4.24688657399994,12.2,0.330643593999986));
#345669=CARTESIAN_POINT('Ctrl Pts',(4.24688657399994,5.2,0.330643593999986));
#345670=CARTESIAN_POINT('Ctrl Pts',(4.24688657399994,2.2,0.330643593999986));
#345671=CARTESIAN_POINT('Ctrl Pts',(4.24525651799994,12.2,0.331107071999988));
#345672=CARTESIAN_POINT('Ctrl Pts',(4.24525651799994,5.2,0.331107071999988));
#345673=CARTESIAN_POINT('Ctrl Pts',(4.24525651799994,2.2,0.331107071999988));
#345674=CARTESIAN_POINT('Ctrl Pts',(4.24363022099994,12.2,0.331567468999987));
#345675=CARTESIAN_POINT('Ctrl Pts',(4.24363022099994,5.2,0.331567468999987));
#345676=CARTESIAN_POINT('Ctrl Pts',(4.24363022099994,2.2,0.331567468999987));
#345677=CARTESIAN_POINT('Ctrl Pts',(4.24200768999994,12.2,0.332024789999985));
#345678=CARTESIAN_POINT('Ctrl Pts',(4.24200768999994,5.2,0.332024789999985));
#345679=CARTESIAN_POINT('Ctrl Pts',(4.24200768999994,2.2,0.332024789999985));
#345680=CARTESIAN_POINT('Ctrl Pts',(4.24038893699994,12.2,0.332479043999987));
#345681=CARTESIAN_POINT('Ctrl Pts',(4.24038893699994,5.2,0.332479043999987));
#345682=CARTESIAN_POINT('Ctrl Pts',(4.24038893699994,2.2,0.332479043999987));
#345683=CARTESIAN_POINT('Ctrl Pts',(4.23877397399994,12.2,0.332930236999989));
#345684=CARTESIAN_POINT('Ctrl Pts',(4.23877397399994,5.2,0.332930236999989));
#345685=CARTESIAN_POINT('Ctrl Pts',(4.23877397399994,2.2,0.332930236999989));
#345686=CARTESIAN_POINT('Ctrl Pts',(4.23716280899994,12.2,0.333378374999986));
#345687=CARTESIAN_POINT('Ctrl Pts',(4.23716280899994,5.2,0.333378374999986));
#345688=CARTESIAN_POINT('Ctrl Pts',(4.23716280899994,2.2,0.333378374999986));
#345689=CARTESIAN_POINT('Ctrl Pts',(4.23555545199994,12.2,0.333823465999985));
#345690=CARTESIAN_POINT('Ctrl Pts',(4.23555545199994,5.2,0.333823465999985));
#345691=CARTESIAN_POINT('Ctrl Pts',(4.23555545199994,2.2,0.333823465999985));
#345692=CARTESIAN_POINT('Ctrl Pts',(4.23395191599994,12.2,0.334265516999985));
#345693=CARTESIAN_POINT('Ctrl Pts',(4.23395191599994,5.2,0.334265516999985));
#345694=CARTESIAN_POINT('Ctrl Pts',(4.23395191599994,2.2,0.334265516999985));
#345695=CARTESIAN_POINT('Ctrl Pts',(4.23235220799994,12.2,0.334704532999983));
#345696=CARTESIAN_POINT('Ctrl Pts',(4.23235220799994,5.2,0.334704532999983));
#345697=CARTESIAN_POINT('Ctrl Pts',(4.23235220799994,2.2,0.334704532999983));
#345698=CARTESIAN_POINT('Ctrl Pts',(4.23075634099995,12.2,0.335140522999984));
#345699=CARTESIAN_POINT('Ctrl Pts',(4.23075634099995,5.2,0.335140522999984));
#345700=CARTESIAN_POINT('Ctrl Pts',(4.23075634099995,2.2,0.335140522999984));
#345701=CARTESIAN_POINT('Ctrl Pts',(4.22916432499994,12.2,0.335573492999988));
#345702=CARTESIAN_POINT('Ctrl Pts',(4.22916432499994,5.2,0.335573492999988));
#345703=CARTESIAN_POINT('Ctrl Pts',(4.22916432499994,2.2,0.335573492999988));
#345704=CARTESIAN_POINT('Ctrl Pts',(4.22757616999994,12.2,0.336003450999982));
#345705=CARTESIAN_POINT('Ctrl Pts',(4.22757616999994,5.2,0.336003450999982));
#345706=CARTESIAN_POINT('Ctrl Pts',(4.22757616999994,2.2,0.336003450999982));
#345707=CARTESIAN_POINT('Ctrl Pts',(4.22599188699994,12.2,0.336430402999985));
#345708=CARTESIAN_POINT('Ctrl Pts',(4.22599188699994,5.2,0.336430402999985));
#345709=CARTESIAN_POINT('Ctrl Pts',(4.22599188699994,2.2,0.336430402999985));
#345710=CARTESIAN_POINT('Ctrl Pts',(4.22441148399994,12.2,0.336854356999985));
#345711=CARTESIAN_POINT('Ctrl Pts',(4.22441148399994,5.2,0.336854356999985));
#345712=CARTESIAN_POINT('Ctrl Pts',(4.22441148399994,2.2,0.336854356999985));
#345713=CARTESIAN_POINT('Ctrl Pts',(4.22283497399994,12.2,0.337275318999986));
#345714=CARTESIAN_POINT('Ctrl Pts',(4.22283497399994,5.2,0.337275318999986));
#345715=CARTESIAN_POINT('Ctrl Pts',(4.22283497399994,2.2,0.337275318999986));
#345716=CARTESIAN_POINT('Ctrl Pts',(4.22126236599994,12.2,0.337693296999984));
#345717=CARTESIAN_POINT('Ctrl Pts',(4.22126236599994,5.2,0.337693296999984));
#345718=CARTESIAN_POINT('Ctrl Pts',(4.22126236599994,2.2,0.337693296999984));
#345719=CARTESIAN_POINT('Ctrl Pts',(4.21969367199994,12.2,0.338108296999984));
#345720=CARTESIAN_POINT('Ctrl Pts',(4.21969367199994,5.2,0.338108296999984));
#345721=CARTESIAN_POINT('Ctrl Pts',(4.21969367199994,2.2,0.338108296999984));
#345722=CARTESIAN_POINT('Ctrl Pts',(4.21812890099994,12.2,0.338520327999987));
#345723=CARTESIAN_POINT('Ctrl Pts',(4.21812890099994,5.2,0.338520327999987));
#345724=CARTESIAN_POINT('Ctrl Pts',(4.21812890099994,2.2,0.338520327999987));
#345725=CARTESIAN_POINT('Ctrl Pts',(4.21656806399994,12.2,0.338929394999985));
#345726=CARTESIAN_POINT('Ctrl Pts',(4.21656806399994,5.2,0.338929394999985));
#345727=CARTESIAN_POINT('Ctrl Pts',(4.21656806399994,2.2,0.338929394999985));
#345728=CARTESIAN_POINT('Ctrl Pts',(4.21501117099994,12.2,0.339335506999987));
#345729=CARTESIAN_POINT('Ctrl Pts',(4.21501117099994,5.2,0.339335506999987));
#345730=CARTESIAN_POINT('Ctrl Pts',(4.21501117099994,2.2,0.339335506999987));
#345731=CARTESIAN_POINT('Ctrl Pts',(4.21345823399994,12.2,0.339738669999985));
#345732=CARTESIAN_POINT('Ctrl Pts',(4.21345823399994,5.2,0.339738669999985));
#345733=CARTESIAN_POINT('Ctrl Pts',(4.21345823399994,2.2,0.339738669999985));
#345734=CARTESIAN_POINT('Ctrl Pts',(4.21190926199994,12.2,0.340138891999988));
#345735=CARTESIAN_POINT('Ctrl Pts',(4.21190926199994,5.2,0.340138891999988));
#345736=CARTESIAN_POINT('Ctrl Pts',(4.21190926199994,2.2,0.340138891999988));
#345737=CARTESIAN_POINT('Ctrl Pts',(4.21036426599994,12.2,0.340536181999984));
#345738=CARTESIAN_POINT('Ctrl Pts',(4.21036426599994,5.2,0.340536181999984));
#345739=CARTESIAN_POINT('Ctrl Pts',(4.21036426599994,2.2,0.340536181999984));
#345740=CARTESIAN_POINT('Ctrl Pts',(4.20882325699994,12.2,0.340930543999987));
#345741=CARTESIAN_POINT('Ctrl Pts',(4.20882325699994,5.2,0.340930543999987));
#345742=CARTESIAN_POINT('Ctrl Pts',(4.20882325699994,2.2,0.340930543999987));
#345743=CARTESIAN_POINT('Ctrl Pts',(4.20728624399994,12.2,0.341321986999983));
#345744=CARTESIAN_POINT('Ctrl Pts',(4.20728624399994,5.2,0.341321986999983));
#345745=CARTESIAN_POINT('Ctrl Pts',(4.20728624399994,2.2,0.341321986999983));
#345746=CARTESIAN_POINT('Ctrl Pts',(4.20575323899994,12.2,0.341710518999987));
#345747=CARTESIAN_POINT('Ctrl Pts',(4.20575323899994,5.2,0.341710518999987));
#345748=CARTESIAN_POINT('Ctrl Pts',(4.20575323899994,2.2,0.341710518999987));
#345749=CARTESIAN_POINT('Ctrl Pts',(4.20422425099995,12.2,0.342096144999986));
#345750=CARTESIAN_POINT('Ctrl Pts',(4.20422425099995,5.2,0.342096144999986));
#345751=CARTESIAN_POINT('Ctrl Pts',(4.20422425099995,2.2,0.342096144999986));
#345752=CARTESIAN_POINT('Ctrl Pts',(4.20269929299994,12.2,0.342478876999985));
#345753=CARTESIAN_POINT('Ctrl Pts',(4.20269929299994,5.2,0.342478876999985));
#345754=CARTESIAN_POINT('Ctrl Pts',(4.20269929299994,2.2,0.342478876999985));
#345755=CARTESIAN_POINT('Ctrl Pts',(4.20117837399994,12.2,0.342858717999985));
#345756=CARTESIAN_POINT('Ctrl Pts',(4.20117837399994,5.2,0.342858717999985));
#345757=CARTESIAN_POINT('Ctrl Pts',(4.20117837399994,2.2,0.342858717999985));
#345758=CARTESIAN_POINT('Ctrl Pts',(4.19966150399994,12.2,0.343235676999987));
#345759=CARTESIAN_POINT('Ctrl Pts',(4.19966150399994,5.2,0.343235676999987));
#345760=CARTESIAN_POINT('Ctrl Pts',(4.19966150399994,2.2,0.343235676999987));
#345761=CARTESIAN_POINT('Ctrl Pts',(4.19814869599994,12.2,0.343609762999986));
#345762=CARTESIAN_POINT('Ctrl Pts',(4.19814869599994,5.2,0.343609762999986));
#345763=CARTESIAN_POINT('Ctrl Pts',(4.19814869599994,2.2,0.343609762999986));
#345764=CARTESIAN_POINT('Ctrl Pts',(4.19663995799994,12.2,0.343980981999987));
#345765=CARTESIAN_POINT('Ctrl Pts',(4.19663995799994,5.2,0.343980981999987));
#345766=CARTESIAN_POINT('Ctrl Pts',(4.19663995799994,2.2,0.343980981999987));
#345767=CARTESIAN_POINT('Ctrl Pts',(4.19513530099994,12.2,0.344349341999983));
#345768=CARTESIAN_POINT('Ctrl Pts',(4.19513530099994,5.2,0.344349341999983));
#345769=CARTESIAN_POINT('Ctrl Pts',(4.19513530099994,2.2,0.344349341999983));
#345770=CARTESIAN_POINT('Ctrl Pts',(4.19363473699994,12.2,0.344714848999987));
#345771=CARTESIAN_POINT('Ctrl Pts',(4.19363473699994,5.2,0.344714848999987));
#345772=CARTESIAN_POINT('Ctrl Pts',(4.19363473699994,2.2,0.344714848999987));
#345773=CARTESIAN_POINT('Ctrl Pts',(4.19213827599994,12.2,0.345077513999983));
#345774=CARTESIAN_POINT('Ctrl Pts',(4.19213827599994,5.2,0.345077513999983));
#345775=CARTESIAN_POINT('Ctrl Pts',(4.19213827599994,2.2,0.345077513999983));
#345776=CARTESIAN_POINT('Ctrl Pts',(4.19064592699994,12.2,0.345437342999984));
#345777=CARTESIAN_POINT('Ctrl Pts',(4.19064592699994,5.2,0.345437342999984));
#345778=CARTESIAN_POINT('Ctrl Pts',(4.19064592699994,2.2,0.345437342999984));
#345779=CARTESIAN_POINT('Ctrl Pts',(4.18915770399995,12.2,0.345794341999985));
#345780=CARTESIAN_POINT('Ctrl Pts',(4.18915770399995,5.2,0.345794341999985));
#345781=CARTESIAN_POINT('Ctrl Pts',(4.18915770399995,2.2,0.345794341999985));
#345782=CARTESIAN_POINT('Ctrl Pts',(4.18767361599994,12.2,0.346148521999985));
#345783=CARTESIAN_POINT('Ctrl Pts',(4.18767361599994,5.2,0.346148521999985));
#345784=CARTESIAN_POINT('Ctrl Pts',(4.18767361599994,2.2,0.346148521999985));
#345785=CARTESIAN_POINT('Ctrl Pts',(4.18619367199994,12.2,0.346499887999983));
#345786=CARTESIAN_POINT('Ctrl Pts',(4.18619367199994,5.2,0.346499887999983));
#345787=CARTESIAN_POINT('Ctrl Pts',(4.18619367199994,2.2,0.346499887999983));
#345788=CARTESIAN_POINT('Ctrl Pts',(4.18471788499994,12.2,0.346848449999988));
#345789=CARTESIAN_POINT('Ctrl Pts',(4.18471788499994,5.2,0.346848449999988));
#345790=CARTESIAN_POINT('Ctrl Pts',(4.18471788499994,2.2,0.346848449999988));
#345791=CARTESIAN_POINT('Ctrl Pts',(4.18324626499994,12.2,0.347194214999984));
#345792=CARTESIAN_POINT('Ctrl Pts',(4.18324626499994,5.2,0.347194214999984));
#345793=CARTESIAN_POINT('Ctrl Pts',(4.18324626499994,2.2,0.347194214999984));
#345794=CARTESIAN_POINT('Ctrl Pts',(4.18177882199994,12.2,0.347537189999985));
#345795=CARTESIAN_POINT('Ctrl Pts',(4.18177882199994,5.2,0.347537189999985));
#345796=CARTESIAN_POINT('Ctrl Pts',(4.18177882199994,2.2,0.347537189999985));
#345797=CARTESIAN_POINT('Ctrl Pts',(4.18031556799995,12.2,0.347877382999986));
#345798=CARTESIAN_POINT('Ctrl Pts',(4.18031556799995,5.2,0.347877382999986));
#345799=CARTESIAN_POINT('Ctrl Pts',(4.18031556799995,2.2,0.347877382999986));
#345800=CARTESIAN_POINT('Ctrl Pts',(4.17885651199995,12.2,0.348214803999984));
#345801=CARTESIAN_POINT('Ctrl Pts',(4.17885651199995,5.2,0.348214803999984));
#345802=CARTESIAN_POINT('Ctrl Pts',(4.17885651199995,2.2,0.348214803999984));
#345803=CARTESIAN_POINT('Ctrl Pts',(4.17740166699994,12.2,0.348549458999985));
#345804=CARTESIAN_POINT('Ctrl Pts',(4.17740166699994,5.2,0.348549458999985));
#345805=CARTESIAN_POINT('Ctrl Pts',(4.17740166699994,2.2,0.348549458999985));
#345806=CARTESIAN_POINT('Ctrl Pts',(4.17595104199994,12.2,0.348881354999988));
#345807=CARTESIAN_POINT('Ctrl Pts',(4.17595104199994,5.2,0.348881354999988));
#345808=CARTESIAN_POINT('Ctrl Pts',(4.17595104199994,2.2,0.348881354999988));
#345809=CARTESIAN_POINT('Ctrl Pts',(4.17450464799995,12.2,0.349210502999986));
#345810=CARTESIAN_POINT('Ctrl Pts',(4.17450464799995,5.2,0.349210502999986));
#345811=CARTESIAN_POINT('Ctrl Pts',(4.17450464799995,2.2,0.349210502999986));
#345812=CARTESIAN_POINT('Ctrl Pts',(4.17306249699995,12.2,0.349536908999983));
#345813=CARTESIAN_POINT('Ctrl Pts',(4.17306249699995,5.2,0.349536908999983));
#345814=CARTESIAN_POINT('Ctrl Pts',(4.17306249699995,2.2,0.349536908999983));
#345815=CARTESIAN_POINT('Ctrl Pts',(4.17162459799994,12.2,0.349860581999986));
#345816=CARTESIAN_POINT('Ctrl Pts',(4.17162459799994,5.2,0.349860581999986));
#345817=CARTESIAN_POINT('Ctrl Pts',(4.17162459799994,2.2,0.349860581999986));
#345818=CARTESIAN_POINT('Ctrl Pts',(4.17019096299994,12.2,0.350181528999984));
#345819=CARTESIAN_POINT('Ctrl Pts',(4.17019096299994,5.2,0.350181528999984));
#345820=CARTESIAN_POINT('Ctrl Pts',(4.17019096299994,2.2,0.350181528999984));
#345821=CARTESIAN_POINT('Ctrl Pts',(4.16876160299995,12.2,0.350499758999985));
#345822=CARTESIAN_POINT('Ctrl Pts',(4.16876160299995,5.2,0.350499758999985));
#345823=CARTESIAN_POINT('Ctrl Pts',(4.16876160299995,2.2,0.350499758999985));
#345824=CARTESIAN_POINT('Ctrl Pts',(4.16733652799994,12.2,0.350815279999988));
#345825=CARTESIAN_POINT('Ctrl Pts',(4.16733652799994,5.2,0.350815279999988));
#345826=CARTESIAN_POINT('Ctrl Pts',(4.16733652799994,2.2,0.350815279999988));
#345827=CARTESIAN_POINT('Ctrl Pts',(4.16591574799994,12.2,0.351128100999984));
#345828=CARTESIAN_POINT('Ctrl Pts',(4.16591574799994,5.2,0.351128100999984));
#345829=CARTESIAN_POINT('Ctrl Pts',(4.16591574799994,2.2,0.351128100999984));
#345830=CARTESIAN_POINT('Ctrl Pts',(4.16449927599994,12.2,0.351438228999985));
#345831=CARTESIAN_POINT('Ctrl Pts',(4.16449927599994,5.2,0.351438228999985));
#345832=CARTESIAN_POINT('Ctrl Pts',(4.16449927599994,2.2,0.351438228999985));
#345833=CARTESIAN_POINT('Ctrl Pts',(4.16308712199995,12.2,0.351745671999986));
#345834=CARTESIAN_POINT('Ctrl Pts',(4.16308712199995,5.2,0.351745671999986));
#345835=CARTESIAN_POINT('Ctrl Pts',(4.16308712199995,2.2,0.351745671999986));
#345836=CARTESIAN_POINT('Ctrl Pts',(4.16167929599994,12.2,0.352050439999987));
#345837=CARTESIAN_POINT('Ctrl Pts',(4.16167929599994,5.2,0.352050439999987));
#345838=CARTESIAN_POINT('Ctrl Pts',(4.16167929599994,2.2,0.352050439999987));
#345839=CARTESIAN_POINT('Ctrl Pts',(4.16027580999994,12.2,0.352352540999985));
#345840=CARTESIAN_POINT('Ctrl Pts',(4.16027580999994,5.2,0.352352540999985));
#345841=CARTESIAN_POINT('Ctrl Pts',(4.16027580999994,2.2,0.352352540999985));
#345842=CARTESIAN_POINT('Ctrl Pts',(4.15887667599994,12.2,0.352651980999985));
#345843=CARTESIAN_POINT('Ctrl Pts',(4.15887667599994,5.2,0.352651980999985));
#345844=CARTESIAN_POINT('Ctrl Pts',(4.15887667599994,2.2,0.352651980999985));
#345845=CARTESIAN_POINT('Ctrl Pts',(4.15748190099994,12.2,0.352948770999983));
#345846=CARTESIAN_POINT('Ctrl Pts',(4.15748190099994,5.2,0.352948770999983));
#345847=CARTESIAN_POINT('Ctrl Pts',(4.15748190099994,2.2,0.352948770999983));
#345848=CARTESIAN_POINT('Ctrl Pts',(4.15609149899994,12.2,0.353242917999985));
#345849=CARTESIAN_POINT('Ctrl Pts',(4.15609149899994,5.2,0.353242917999985));
#345850=CARTESIAN_POINT('Ctrl Pts',(4.15609149899994,2.2,0.353242917999985));
#345851=CARTESIAN_POINT('Ctrl Pts',(4.15470548099994,12.2,0.353534431999982));
#345852=CARTESIAN_POINT('Ctrl Pts',(4.15470548099994,5.2,0.353534431999982));
#345853=CARTESIAN_POINT('Ctrl Pts',(4.15470548099994,2.2,0.353534431999982));
#345854=CARTESIAN_POINT('Ctrl Pts',(4.15332385599995,12.2,0.353823319999984));
#345855=CARTESIAN_POINT('Ctrl Pts',(4.15332385599995,5.2,0.353823319999984));
#345856=CARTESIAN_POINT('Ctrl Pts',(4.15332385599995,2.2,0.353823319999984));
#345857=CARTESIAN_POINT('Ctrl Pts',(4.15194663699994,12.2,0.354109590999983));
#345858=CARTESIAN_POINT('Ctrl Pts',(4.15194663699994,5.2,0.354109590999983));
#345859=CARTESIAN_POINT('Ctrl Pts',(4.15194663699994,2.2,0.354109590999983));
#345860=CARTESIAN_POINT('Ctrl Pts',(4.15057383399995,12.2,0.354393252999987));
#345861=CARTESIAN_POINT('Ctrl Pts',(4.15057383399995,5.2,0.354393252999987));
#345862=CARTESIAN_POINT('Ctrl Pts',(4.15057383399995,2.2,0.354393252999987));
#345863=CARTESIAN_POINT('Ctrl Pts',(4.14920545699994,12.2,0.354674315999985));
#345864=CARTESIAN_POINT('Ctrl Pts',(4.14920545699994,5.2,0.354674315999985));
#345865=CARTESIAN_POINT('Ctrl Pts',(4.14920545699994,2.2,0.354674315999985));
#345866=CARTESIAN_POINT('Ctrl Pts',(4.14784151899994,12.2,0.354952786999987));
#345867=CARTESIAN_POINT('Ctrl Pts',(4.14784151899994,5.2,0.354952786999987));
#345868=CARTESIAN_POINT('Ctrl Pts',(4.14784151899994,2.2,0.354952786999987));
#345869=CARTESIAN_POINT('Ctrl Pts',(4.14648202999994,12.2,0.355228675999988));
#345870=CARTESIAN_POINT('Ctrl Pts',(4.14648202999994,5.2,0.355228675999988));
#345871=CARTESIAN_POINT('Ctrl Pts',(4.14648202999994,2.2,0.355228675999988));
#345872=CARTESIAN_POINT('Ctrl Pts',(4.14512700099994,12.2,0.355501990999985));
#345873=CARTESIAN_POINT('Ctrl Pts',(4.14512700099994,5.2,0.355501990999985));
#345874=CARTESIAN_POINT('Ctrl Pts',(4.14512700099994,2.2,0.355501990999985));
#345875=CARTESIAN_POINT('Ctrl Pts',(4.14377644299995,12.2,0.355772740999987));
#345876=CARTESIAN_POINT('Ctrl Pts',(4.14377644299995,5.2,0.355772740999987));
#345877=CARTESIAN_POINT('Ctrl Pts',(4.14377644299995,2.2,0.355772740999987));
#345878=CARTESIAN_POINT('Ctrl Pts',(4.14243036799994,12.2,0.356040933999986));
#345879=CARTESIAN_POINT('Ctrl Pts',(4.14243036799994,5.2,0.356040933999986));
#345880=CARTESIAN_POINT('Ctrl Pts',(4.14243036799994,2.2,0.356040933999986));
#345881=CARTESIAN_POINT('Ctrl Pts',(4.14108878399994,12.2,0.356306579999988));
#345882=CARTESIAN_POINT('Ctrl Pts',(4.14108878399994,5.2,0.356306579999988));
#345883=CARTESIAN_POINT('Ctrl Pts',(4.14108878399994,2.2,0.356306579999988));
#345884=CARTESIAN_POINT('Ctrl Pts',(4.13975170499994,12.2,0.356569686999983));
#345885=CARTESIAN_POINT('Ctrl Pts',(4.13975170499994,5.2,0.356569686999983));
#345886=CARTESIAN_POINT('Ctrl Pts',(4.13975170499994,2.2,0.356569686999983));
#345887=CARTESIAN_POINT('Ctrl Pts',(4.13841914099994,12.2,0.356830263999988));
#345888=CARTESIAN_POINT('Ctrl Pts',(4.13841914099994,5.2,0.356830263999988));
#345889=CARTESIAN_POINT('Ctrl Pts',(4.13841914099994,2.2,0.356830263999988));
#345890=CARTESIAN_POINT('Ctrl Pts',(4.13709110399994,12.2,0.357088320999988));
#345891=CARTESIAN_POINT('Ctrl Pts',(4.13709110399994,5.2,0.357088320999988));
#345892=CARTESIAN_POINT('Ctrl Pts',(4.13709110399994,2.2,0.357088320999988));
#345893=CARTESIAN_POINT('Ctrl Pts',(4.13576760499994,12.2,0.357343863999984));
#345894=CARTESIAN_POINT('Ctrl Pts',(4.13576760499994,5.2,0.357343863999984));
#345895=CARTESIAN_POINT('Ctrl Pts',(4.13576760499994,2.2,0.357343863999984));
#345896=CARTESIAN_POINT('Ctrl Pts',(4.13444865299994,12.2,0.357596904999986));
#345897=CARTESIAN_POINT('Ctrl Pts',(4.13444865299994,5.2,0.357596904999986));
#345898=CARTESIAN_POINT('Ctrl Pts',(4.13444865299994,2.2,0.357596904999986));
#345899=CARTESIAN_POINT('Ctrl Pts',(4.13313426199994,12.2,0.357847450999986));
#345900=CARTESIAN_POINT('Ctrl Pts',(4.13313426199994,5.2,0.357847450999986));
#345901=CARTESIAN_POINT('Ctrl Pts',(4.13313426199994,2.2,0.357847450999986));
#345902=CARTESIAN_POINT('Ctrl Pts',(4.13182443999994,12.2,0.358095511999985));
#345903=CARTESIAN_POINT('Ctrl Pts',(4.13182443999994,5.2,0.358095511999985));
#345904=CARTESIAN_POINT('Ctrl Pts',(4.13182443999994,2.2,0.358095511999985));
#345905=CARTESIAN_POINT('Ctrl Pts',(4.13051920099995,12.2,0.358341096999983));
#345906=CARTESIAN_POINT('Ctrl Pts',(4.13051920099995,5.2,0.358341096999983));
#345907=CARTESIAN_POINT('Ctrl Pts',(4.13051920099995,2.2,0.358341096999983));
#345908=CARTESIAN_POINT('Ctrl Pts',(4.12921855399994,12.2,0.358584215999986));
#345909=CARTESIAN_POINT('Ctrl Pts',(4.12921855399994,5.2,0.358584215999986));
#345910=CARTESIAN_POINT('Ctrl Pts',(4.12921855399994,2.2,0.358584215999986));
#345911=CARTESIAN_POINT('Ctrl Pts',(4.12792251299994,12.2,0.358824875999986));
#345912=CARTESIAN_POINT('Ctrl Pts',(4.12792251299994,5.2,0.358824875999986));
#345913=CARTESIAN_POINT('Ctrl Pts',(4.12792251299994,2.2,0.358824875999986));
#345914=CARTESIAN_POINT('Ctrl Pts',(4.12663108599994,12.2,0.359063086999987));
#345915=CARTESIAN_POINT('Ctrl Pts',(4.12663108599994,5.2,0.359063086999987));
#345916=CARTESIAN_POINT('Ctrl Pts',(4.12663108599994,2.2,0.359063086999987));
#345917=CARTESIAN_POINT('Ctrl Pts',(4.12534428599994,12.2,0.359298858999986));
#345918=CARTESIAN_POINT('Ctrl Pts',(4.12534428599994,5.2,0.359298858999986));
#345919=CARTESIAN_POINT('Ctrl Pts',(4.12534428599994,2.2,0.359298858999986));
#345920=CARTESIAN_POINT('Ctrl Pts',(4.12406212399994,12.2,0.359532199999983));
#345921=CARTESIAN_POINT('Ctrl Pts',(4.12406212399994,5.2,0.359532199999983));
#345922=CARTESIAN_POINT('Ctrl Pts',(4.12406212399994,2.2,0.359532199999983));
#345923=CARTESIAN_POINT('Ctrl Pts',(4.12278461099994,12.2,0.359763120999985));
#345924=CARTESIAN_POINT('Ctrl Pts',(4.12278461099994,5.2,0.359763120999985));
#345925=CARTESIAN_POINT('Ctrl Pts',(4.12278461099994,2.2,0.359763120999985));
#345926=CARTESIAN_POINT('Ctrl Pts',(4.12151175799994,12.2,0.359991628999987));
#345927=CARTESIAN_POINT('Ctrl Pts',(4.12151175799994,5.2,0.359991628999987));
#345928=CARTESIAN_POINT('Ctrl Pts',(4.12151175799994,2.2,0.359991628999987));
#345929=CARTESIAN_POINT('Ctrl Pts',(4.12024357499994,12.2,0.360217734999986));
#345930=CARTESIAN_POINT('Ctrl Pts',(4.12024357499994,5.2,0.360217734999986));
#345931=CARTESIAN_POINT('Ctrl Pts',(4.12024357499994,2.2,0.360217734999986));
#345932=CARTESIAN_POINT('Ctrl Pts',(4.11898007599994,12.2,0.360441448999986));
#345933=CARTESIAN_POINT('Ctrl Pts',(4.11898007599994,5.2,0.360441448999986));
#345934=CARTESIAN_POINT('Ctrl Pts',(4.11898007599994,2.2,0.360441448999986));
#345935=CARTESIAN_POINT('Ctrl Pts',(4.11772127099994,12.2,0.360662777999985));
#345936=CARTESIAN_POINT('Ctrl Pts',(4.11772127099994,5.2,0.360662777999985));
#345937=CARTESIAN_POINT('Ctrl Pts',(4.11772127099994,2.2,0.360662777999985));
#345938=CARTESIAN_POINT('Ctrl Pts',(4.11646717199995,12.2,0.360881732999987));
#345939=CARTESIAN_POINT('Ctrl Pts',(4.11646717199995,5.2,0.360881732999987));
#345940=CARTESIAN_POINT('Ctrl Pts',(4.11646717199995,2.2,0.360881732999987));
#345941=CARTESIAN_POINT('Ctrl Pts',(4.11521778799994,12.2,0.361098323999984));
#345942=CARTESIAN_POINT('Ctrl Pts',(4.11521778799994,5.2,0.361098323999984));
#345943=CARTESIAN_POINT('Ctrl Pts',(4.11521778799994,2.2,0.361098323999984));
#345944=CARTESIAN_POINT('Ctrl Pts',(4.11397313199994,12.2,0.361312558999987));
#345945=CARTESIAN_POINT('Ctrl Pts',(4.11397313199994,5.2,0.361312558999987));
#345946=CARTESIAN_POINT('Ctrl Pts',(4.11397313199994,2.2,0.361312558999987));
#345947=CARTESIAN_POINT('Ctrl Pts',(4.11273321599994,12.2,0.361524448999986));
#345948=CARTESIAN_POINT('Ctrl Pts',(4.11273321599994,5.2,0.361524448999986));
#345949=CARTESIAN_POINT('Ctrl Pts',(4.11273321599994,2.2,0.361524448999986));
#345950=CARTESIAN_POINT('Ctrl Pts',(4.11149805099994,12.2,0.361734002999987));
#345951=CARTESIAN_POINT('Ctrl Pts',(4.11149805099994,5.2,0.361734002999987));
#345952=CARTESIAN_POINT('Ctrl Pts',(4.11149805099994,2.2,0.361734002999987));
#345953=CARTESIAN_POINT('Ctrl Pts',(4.11026764599994,12.2,0.361941229999987));
#345954=CARTESIAN_POINT('Ctrl Pts',(4.11026764599994,5.2,0.361941229999987));
#345955=CARTESIAN_POINT('Ctrl Pts',(4.11026764599994,2.2,0.361941229999987));
#345956=CARTESIAN_POINT('Ctrl Pts',(4.10904201499994,12.2,0.362146139999986));
#345957=CARTESIAN_POINT('Ctrl Pts',(4.10904201499994,5.2,0.362146139999986));
#345958=CARTESIAN_POINT('Ctrl Pts',(4.10904201499994,2.2,0.362146139999986));
#345959=CARTESIAN_POINT('Ctrl Pts',(4.10782116899994,12.2,0.362348742999985));
#345960=CARTESIAN_POINT('Ctrl Pts',(4.10782116899994,5.2,0.362348742999985));
#345961=CARTESIAN_POINT('Ctrl Pts',(4.10782116899994,2.2,0.362348742999985));
#345962=CARTESIAN_POINT('Ctrl Pts',(4.10660511699994,12.2,0.362549048999985));
#345963=CARTESIAN_POINT('Ctrl Pts',(4.10660511699994,5.2,0.362549048999985));
#345964=CARTESIAN_POINT('Ctrl Pts',(4.10660511699994,2.2,0.362549048999985));
#345965=CARTESIAN_POINT('Ctrl Pts',(4.10539387399994,12.2,0.362747067999987));
#345966=CARTESIAN_POINT('Ctrl Pts',(4.10539387399994,5.2,0.362747067999987));
#345967=CARTESIAN_POINT('Ctrl Pts',(4.10539387399994,2.2,0.362747067999987));
#345968=CARTESIAN_POINT('Ctrl Pts',(4.10418744999994,12.2,0.362942807999986));
#345969=CARTESIAN_POINT('Ctrl Pts',(4.10418744999994,5.2,0.362942807999986));
#345970=CARTESIAN_POINT('Ctrl Pts',(4.10418744999994,2.2,0.362942807999986));
#345971=CARTESIAN_POINT('Ctrl Pts',(4.10298585499994,12.2,0.363136280999985));
#345972=CARTESIAN_POINT('Ctrl Pts',(4.10298585499994,5.2,0.363136280999985));
#345973=CARTESIAN_POINT('Ctrl Pts',(4.10298585499994,2.2,0.363136280999985));
#345974=CARTESIAN_POINT('Ctrl Pts',(4.10178910199994,12.2,0.363327494999983));
#345975=CARTESIAN_POINT('Ctrl Pts',(4.10178910199994,5.2,0.363327494999983));
#345976=CARTESIAN_POINT('Ctrl Pts',(4.10178910199994,2.2,0.363327494999983));
#345977=CARTESIAN_POINT('Ctrl Pts',(4.10059720199994,12.2,0.363516460999986));
#345978=CARTESIAN_POINT('Ctrl Pts',(4.10059720199994,5.2,0.363516460999986));
#345979=CARTESIAN_POINT('Ctrl Pts',(4.10059720199994,2.2,0.363516460999986));
#345980=CARTESIAN_POINT('Ctrl Pts',(4.09941016599995,12.2,0.363703188999986));
#345981=CARTESIAN_POINT('Ctrl Pts',(4.09941016599995,5.2,0.363703188999986));
#345982=CARTESIAN_POINT('Ctrl Pts',(4.09941016599995,2.2,0.363703188999986));
#345983=CARTESIAN_POINT('Ctrl Pts',(4.09822800699995,12.2,0.363887689999984));
#345984=CARTESIAN_POINT('Ctrl Pts',(4.09822800699995,5.2,0.363887689999984));
#345985=CARTESIAN_POINT('Ctrl Pts',(4.09822800699995,2.2,0.363887689999984));
#345986=CARTESIAN_POINT('Ctrl Pts',(4.09705073399994,12.2,0.364069971999985));
#345987=CARTESIAN_POINT('Ctrl Pts',(4.09705073399994,5.2,0.364069971999985));
#345988=CARTESIAN_POINT('Ctrl Pts',(4.09705073399994,2.2,0.364069971999985));
#345989=CARTESIAN_POINT('Ctrl Pts',(4.09587836199994,12.2,0.364250044999985));
#345990=CARTESIAN_POINT('Ctrl Pts',(4.09587836199994,5.2,0.364250044999985));
#345991=CARTESIAN_POINT('Ctrl Pts',(4.09587836199994,2.2,0.364250044999985));
#345992=CARTESIAN_POINT('Ctrl Pts',(4.09471089799994,12.2,0.364427920999986));
#345993=CARTESIAN_POINT('Ctrl Pts',(4.09471089799994,5.2,0.364427920999986));
#345994=CARTESIAN_POINT('Ctrl Pts',(4.09471089799994,2.2,0.364427920999986));
#345995=CARTESIAN_POINT('Ctrl Pts',(4.09354835799994,12.2,0.364603608999987));
#345996=CARTESIAN_POINT('Ctrl Pts',(4.09354835799994,5.2,0.364603608999987));
#345997=CARTESIAN_POINT('Ctrl Pts',(4.09354835799994,2.2,0.364603608999987));
#345998=CARTESIAN_POINT('Ctrl Pts',(4.09239074999994,12.2,0.364777118999986));
#345999=CARTESIAN_POINT('Ctrl Pts',(4.09239074999994,5.2,0.364777118999986));
#346000=CARTESIAN_POINT('Ctrl Pts',(4.09239074999994,2.2,0.364777118999986));
#346001=CARTESIAN_POINT('Ctrl Pts',(4.09123808799994,12.2,0.364948461999983));
#346002=CARTESIAN_POINT('Ctrl Pts',(4.09123808799994,5.2,0.364948461999983));
#346003=CARTESIAN_POINT('Ctrl Pts',(4.09123808799994,2.2,0.364948461999983));
#346004=CARTESIAN_POINT('Ctrl Pts',(4.09009038199994,12.2,0.365117647999984));
#346005=CARTESIAN_POINT('Ctrl Pts',(4.09009038199994,5.2,0.365117647999984));
#346006=CARTESIAN_POINT('Ctrl Pts',(4.09009038199994,2.2,0.365117647999984));
#346007=CARTESIAN_POINT('Ctrl Pts',(4.08894764399994,12.2,0.365284685999985));
#346008=CARTESIAN_POINT('Ctrl Pts',(4.08894764399994,5.2,0.365284685999985));
#346009=CARTESIAN_POINT('Ctrl Pts',(4.08894764399994,2.2,0.365284685999985));
#346010=CARTESIAN_POINT('Ctrl Pts',(4.08780988599994,12.2,0.365449588999986));
#346011=CARTESIAN_POINT('Ctrl Pts',(4.08780988599994,5.2,0.365449588999986));
#346012=CARTESIAN_POINT('Ctrl Pts',(4.08780988599994,2.2,0.365449588999986));
#346013=CARTESIAN_POINT('Ctrl Pts',(4.08667711999994,12.2,0.365612363999985));
#346014=CARTESIAN_POINT('Ctrl Pts',(4.08667711999994,5.2,0.365612363999985));
#346015=CARTESIAN_POINT('Ctrl Pts',(4.08667711999994,2.2,0.365612363999985));
#346016=CARTESIAN_POINT('Ctrl Pts',(4.08554935699994,12.2,0.365773025999987));
#346017=CARTESIAN_POINT('Ctrl Pts',(4.08554935699994,5.2,0.365773025999987));
#346018=CARTESIAN_POINT('Ctrl Pts',(4.08554935699994,2.2,0.365773025999987));
#346019=CARTESIAN_POINT('Ctrl Pts',(4.08442660799994,12.2,0.365931580999987));
#346020=CARTESIAN_POINT('Ctrl Pts',(4.08442660799994,5.2,0.365931580999987));
#346021=CARTESIAN_POINT('Ctrl Pts',(4.08442660799994,2.2,0.365931580999987));
#346022=CARTESIAN_POINT('Ctrl Pts',(4.08330888599994,12.2,0.366088040999983));
#346023=CARTESIAN_POINT('Ctrl Pts',(4.08330888599994,5.2,0.366088040999983));
#346024=CARTESIAN_POINT('Ctrl Pts',(4.08330888599994,2.2,0.366088040999983));
#346025=CARTESIAN_POINT('Ctrl Pts',(4.08219620099994,12.2,0.366242417999985));
#346026=CARTESIAN_POINT('Ctrl Pts',(4.08219620099994,5.2,0.366242417999985));
#346027=CARTESIAN_POINT('Ctrl Pts',(4.08219620099994,2.2,0.366242417999985));
#346028=CARTESIAN_POINT('Ctrl Pts',(4.08108856699995,12.2,0.366394719999987));
#346029=CARTESIAN_POINT('Ctrl Pts',(4.08108856699995,5.2,0.366394719999987));
#346030=CARTESIAN_POINT('Ctrl Pts',(4.08108856699995,2.2,0.366394719999987));
#346031=CARTESIAN_POINT('Ctrl Pts',(4.07998599399995,12.2,0.366544959999988));
#346032=CARTESIAN_POINT('Ctrl Pts',(4.07998599399995,5.2,0.366544959999988));
#346033=CARTESIAN_POINT('Ctrl Pts',(4.07998599399995,2.2,0.366544959999988));
#346034=CARTESIAN_POINT('Ctrl Pts',(4.07888849299994,12.2,0.366693146999988));
#346035=CARTESIAN_POINT('Ctrl Pts',(4.07888849299994,5.2,0.366693146999988));
#346036=CARTESIAN_POINT('Ctrl Pts',(4.07888849299994,2.2,0.366693146999988));
#346037=CARTESIAN_POINT('Ctrl Pts',(4.07779607799994,12.2,0.366839292999988));
#346038=CARTESIAN_POINT('Ctrl Pts',(4.07779607799994,5.2,0.366839292999988));
#346039=CARTESIAN_POINT('Ctrl Pts',(4.07779607799994,2.2,0.366839292999988));
#346040=CARTESIAN_POINT('Ctrl Pts',(4.07670875899994,12.2,0.366983407999988));
#346041=CARTESIAN_POINT('Ctrl Pts',(4.07670875899994,5.2,0.366983407999988));
#346042=CARTESIAN_POINT('Ctrl Pts',(4.07670875899994,2.2,0.366983407999988));
#346043=CARTESIAN_POINT('Ctrl Pts',(4.07562654799994,12.2,0.367125501999985));
#346044=CARTESIAN_POINT('Ctrl Pts',(4.07562654799994,5.2,0.367125501999985));
#346045=CARTESIAN_POINT('Ctrl Pts',(4.07562654799994,2.2,0.367125501999985));
#346046=CARTESIAN_POINT('Ctrl Pts',(4.07454945699994,12.2,0.367265587999985));
#346047=CARTESIAN_POINT('Ctrl Pts',(4.07454945699994,5.2,0.367265587999985));
#346048=CARTESIAN_POINT('Ctrl Pts',(4.07454945699994,2.2,0.367265587999985));
#346049=CARTESIAN_POINT('Ctrl Pts',(4.07347749899994,12.2,0.367403674999984));
#346050=CARTESIAN_POINT('Ctrl Pts',(4.07347749899994,5.2,0.367403674999984));
#346051=CARTESIAN_POINT('Ctrl Pts',(4.07347749899994,2.2,0.367403674999984));
#346052=CARTESIAN_POINT('Ctrl Pts',(4.07241068399994,12.2,0.367539774999983));
#346053=CARTESIAN_POINT('Ctrl Pts',(4.07241068399994,5.2,0.367539774999983));
#346054=CARTESIAN_POINT('Ctrl Pts',(4.07241068399994,2.2,0.367539774999983));
#346055=CARTESIAN_POINT('Ctrl Pts',(4.07134902399994,12.2,0.367673896999987));
#346056=CARTESIAN_POINT('Ctrl Pts',(4.07134902399994,5.2,0.367673896999987));
#346057=CARTESIAN_POINT('Ctrl Pts',(4.07134902399994,2.2,0.367673896999987));
#346058=CARTESIAN_POINT('Ctrl Pts',(4.07029253099994,12.2,0.367806055999989));
#346059=CARTESIAN_POINT('Ctrl Pts',(4.07029253099994,5.2,0.367806055999989));
#346060=CARTESIAN_POINT('Ctrl Pts',(4.07029253099994,2.2,0.367806055999989));
#346061=CARTESIAN_POINT('Ctrl Pts',(4.06924121799995,12.2,0.367936258999984));
#346062=CARTESIAN_POINT('Ctrl Pts',(4.06924121799995,5.2,0.367936258999984));
#346063=CARTESIAN_POINT('Ctrl Pts',(4.06924121799995,2.2,0.367936258999984));
#346064=CARTESIAN_POINT('Ctrl Pts',(4.06819509499995,12.2,0.368064516999986));
#346065=CARTESIAN_POINT('Ctrl Pts',(4.06819509499995,5.2,0.368064516999986));
#346066=CARTESIAN_POINT('Ctrl Pts',(4.06819509499995,2.2,0.368064516999986));
#346067=CARTESIAN_POINT('Ctrl Pts',(4.06715417699994,12.2,0.368190844999985));
#346068=CARTESIAN_POINT('Ctrl Pts',(4.06715417699994,5.2,0.368190844999985));
#346069=CARTESIAN_POINT('Ctrl Pts',(4.06715417699994,2.2,0.368190844999985));
#346070=CARTESIAN_POINT('Ctrl Pts',(4.06611847099995,12.2,0.368315250999984));
#346071=CARTESIAN_POINT('Ctrl Pts',(4.06611847099995,5.2,0.368315250999984));
#346072=CARTESIAN_POINT('Ctrl Pts',(4.06611847099995,2.2,0.368315250999984));
#346073=CARTESIAN_POINT('Ctrl Pts',(4.06508799299994,12.2,0.368437746999986));
#346074=CARTESIAN_POINT('Ctrl Pts',(4.06508799299994,5.2,0.368437746999986));
#346075=CARTESIAN_POINT('Ctrl Pts',(4.06508799299994,2.2,0.368437746999986));
#346076=CARTESIAN_POINT('Ctrl Pts',(4.06406275399994,12.2,0.368558344999985));
#346077=CARTESIAN_POINT('Ctrl Pts',(4.06406275399994,5.2,0.368558344999985));
#346078=CARTESIAN_POINT('Ctrl Pts',(4.06406275399994,2.2,0.368558344999985));
#346079=CARTESIAN_POINT('Ctrl Pts',(4.06304276399994,12.2,0.368677054999988));
#346080=CARTESIAN_POINT('Ctrl Pts',(4.06304276399994,5.2,0.368677054999988));
#346081=CARTESIAN_POINT('Ctrl Pts',(4.06304276399994,2.2,0.368677054999988));
#346082=CARTESIAN_POINT('Ctrl Pts',(4.06202803699994,12.2,0.368793888999988));
#346083=CARTESIAN_POINT('Ctrl Pts',(4.06202803699994,5.2,0.368793888999988));
#346084=CARTESIAN_POINT('Ctrl Pts',(4.06202803699994,2.2,0.368793888999988));
#346085=CARTESIAN_POINT('Ctrl Pts',(4.06101858399994,12.2,0.368908857999983));
#346086=CARTESIAN_POINT('Ctrl Pts',(4.06101858399994,5.2,0.368908857999983));
#346087=CARTESIAN_POINT('Ctrl Pts',(4.06101858399994,2.2,0.368908857999983));
#346088=CARTESIAN_POINT('Ctrl Pts',(4.06001441899994,12.2,0.369021973999986));
#346089=CARTESIAN_POINT('Ctrl Pts',(4.06001441899994,5.2,0.369021973999986));
#346090=CARTESIAN_POINT('Ctrl Pts',(4.06001441899994,2.2,0.369021973999986));
#346091=CARTESIAN_POINT('Ctrl Pts',(4.05901555099994,12.2,0.369133247999986));
#346092=CARTESIAN_POINT('Ctrl Pts',(4.05901555099994,5.2,0.369133247999986));
#346093=CARTESIAN_POINT('Ctrl Pts',(4.05901555099994,2.2,0.369133247999986));
#346094=CARTESIAN_POINT('Ctrl Pts',(4.05802199399994,12.2,0.369242691999982));
#346095=CARTESIAN_POINT('Ctrl Pts',(4.05802199399994,5.2,0.369242691999982));
#346096=CARTESIAN_POINT('Ctrl Pts',(4.05802199399994,2.2,0.369242691999982));
#346097=CARTESIAN_POINT('Ctrl Pts',(4.05703375799995,12.2,0.369350315999988));
#346098=CARTESIAN_POINT('Ctrl Pts',(4.05703375799995,5.2,0.369350315999988));
#346099=CARTESIAN_POINT('Ctrl Pts',(4.05703375799995,2.2,0.369350315999988));
#346100=CARTESIAN_POINT('Ctrl Pts',(4.05605085799994,12.2,0.369456134999986));
#346101=CARTESIAN_POINT('Ctrl Pts',(4.05605085799994,5.2,0.369456134999986));
#346102=CARTESIAN_POINT('Ctrl Pts',(4.05605085799994,2.2,0.369456134999986));
#346103=CARTESIAN_POINT('Ctrl Pts',(4.05507330299994,12.2,0.369560156999986));
#346104=CARTESIAN_POINT('Ctrl Pts',(4.05507330299994,5.2,0.369560156999986));
#346105=CARTESIAN_POINT('Ctrl Pts',(4.05507330299994,2.2,0.369560156999986));
#346106=CARTESIAN_POINT('Ctrl Pts',(4.05410110799994,12.2,0.369662395999986));
#346107=CARTESIAN_POINT('Ctrl Pts',(4.05410110799994,5.2,0.369662395999986));
#346108=CARTESIAN_POINT('Ctrl Pts',(4.05410110799994,2.2,0.369662395999986));
#346109=CARTESIAN_POINT('Ctrl Pts',(4.05313428299995,12.2,0.369762862999985));
#346110=CARTESIAN_POINT('Ctrl Pts',(4.05313428299995,5.2,0.369762862999985));
#346111=CARTESIAN_POINT('Ctrl Pts',(4.05313428299995,2.2,0.369762862999985));
#346112=CARTESIAN_POINT('Ctrl Pts',(4.05217283999994,12.2,0.369861568999985));
#346113=CARTESIAN_POINT('Ctrl Pts',(4.05217283999994,5.2,0.369861568999985));
#346114=CARTESIAN_POINT('Ctrl Pts',(4.05217283999994,2.2,0.369861568999985));
#346115=CARTESIAN_POINT('Ctrl Pts',(4.05121679299994,12.2,0.369958526999987));
#346116=CARTESIAN_POINT('Ctrl Pts',(4.05121679299994,5.2,0.369958526999987));
#346117=CARTESIAN_POINT('Ctrl Pts',(4.05121679299994,2.2,0.369958526999987));
#346118=CARTESIAN_POINT('Ctrl Pts',(4.05026615299994,12.2,0.370053747999983));
#346119=CARTESIAN_POINT('Ctrl Pts',(4.05026615299994,5.2,0.370053747999983));
#346120=CARTESIAN_POINT('Ctrl Pts',(4.05026615299994,2.2,0.370053747999983));
#346121=CARTESIAN_POINT('Ctrl Pts',(4.04932093099994,12.2,0.370147244999988));
#346122=CARTESIAN_POINT('Ctrl Pts',(4.04932093099994,5.2,0.370147244999988));
#346123=CARTESIAN_POINT('Ctrl Pts',(4.04932093099994,2.2,0.370147244999988));
#346124=CARTESIAN_POINT('Ctrl Pts',(4.04838114099995,12.2,0.370239027999983));
#346125=CARTESIAN_POINT('Ctrl Pts',(4.04838114099995,5.2,0.370239027999983));
#346126=CARTESIAN_POINT('Ctrl Pts',(4.04838114099995,2.2,0.370239027999983));
#346127=CARTESIAN_POINT('Ctrl Pts',(4.04744679499994,12.2,0.370329110999985));
#346128=CARTESIAN_POINT('Ctrl Pts',(4.04744679499994,5.2,0.370329110999985));
#346129=CARTESIAN_POINT('Ctrl Pts',(4.04744679499994,2.2,0.370329110999985));
#346130=CARTESIAN_POINT('Ctrl Pts',(4.04651790299994,12.2,0.370417505999985));
#346131=CARTESIAN_POINT('Ctrl Pts',(4.04651790299994,5.2,0.370417505999985));
#346132=CARTESIAN_POINT('Ctrl Pts',(4.04651790299994,2.2,0.370417505999985));
#346133=CARTESIAN_POINT('Ctrl Pts',(4.04559448099994,12.2,0.370504222999983));
#346134=CARTESIAN_POINT('Ctrl Pts',(4.04559448099994,5.2,0.370504222999983));
#346135=CARTESIAN_POINT('Ctrl Pts',(4.04559448099994,2.2,0.370504222999983));
#346136=CARTESIAN_POINT('Ctrl Pts',(4.04467653799994,12.2,0.370589276999986));
#346137=CARTESIAN_POINT('Ctrl Pts',(4.04467653799994,5.2,0.370589276999986));
#346138=CARTESIAN_POINT('Ctrl Pts',(4.04467653799994,2.2,0.370589276999986));
#346139=CARTESIAN_POINT('Ctrl Pts',(4.04376408699994,12.2,0.370672677999986));
#346140=CARTESIAN_POINT('Ctrl Pts',(4.04376408699994,5.2,0.370672677999986));
#346141=CARTESIAN_POINT('Ctrl Pts',(4.04376408699994,2.2,0.370672677999986));
#346142=CARTESIAN_POINT('Ctrl Pts',(4.04285714099994,12.2,0.370754438999987));
#346143=CARTESIAN_POINT('Ctrl Pts',(4.04285714099994,5.2,0.370754438999987));
#346144=CARTESIAN_POINT('Ctrl Pts',(4.04285714099994,2.2,0.370754438999987));
#346145=CARTESIAN_POINT('Ctrl Pts',(4.04195571199994,12.2,0.370834572999983));
#346146=CARTESIAN_POINT('Ctrl Pts',(4.04195571199994,5.2,0.370834572999983));
#346147=CARTESIAN_POINT('Ctrl Pts',(4.04195571199994,2.2,0.370834572999983));
#346148=CARTESIAN_POINT('Ctrl Pts',(4.04105981299994,12.2,0.370913090999987));
#346149=CARTESIAN_POINT('Ctrl Pts',(4.04105981299994,5.2,0.370913090999987));
#346150=CARTESIAN_POINT('Ctrl Pts',(4.04105981299994,2.2,0.370913090999987));
#346151=CARTESIAN_POINT('Ctrl Pts',(4.04016945399994,12.2,0.370990005999987));
#346152=CARTESIAN_POINT('Ctrl Pts',(4.04016945399994,5.2,0.370990005999987));
#346153=CARTESIAN_POINT('Ctrl Pts',(4.04016945399994,2.2,0.370990005999987));
#346154=CARTESIAN_POINT('Ctrl Pts',(4.03928464999994,12.2,0.371065330999985));
#346155=CARTESIAN_POINT('Ctrl Pts',(4.03928464999994,5.2,0.371065330999985));
#346156=CARTESIAN_POINT('Ctrl Pts',(4.03928464999994,2.2,0.371065330999985));
#346157=CARTESIAN_POINT('Ctrl Pts',(4.03840541199994,12.2,0.371139076999984));
#346158=CARTESIAN_POINT('Ctrl Pts',(4.03840541199994,5.2,0.371139076999984));
#346159=CARTESIAN_POINT('Ctrl Pts',(4.03840541199994,2.2,0.371139076999984));
#346160=CARTESIAN_POINT('Ctrl Pts',(4.03753175299994,12.2,0.371211257999988));
#346161=CARTESIAN_POINT('Ctrl Pts',(4.03753175299994,5.2,0.371211257999988));
#346162=CARTESIAN_POINT('Ctrl Pts',(4.03753175299994,2.2,0.371211257999988));
#346163=CARTESIAN_POINT('Ctrl Pts',(4.03666368399994,12.2,0.371281886999988));
#346164=CARTESIAN_POINT('Ctrl Pts',(4.03666368399994,5.2,0.371281886999988));
#346165=CARTESIAN_POINT('Ctrl Pts',(4.03666368399994,2.2,0.371281886999988));
#346166=CARTESIAN_POINT('Ctrl Pts',(4.03580121899994,12.2,0.371350974999984));
#346167=CARTESIAN_POINT('Ctrl Pts',(4.03580121899994,5.2,0.371350974999984));
#346168=CARTESIAN_POINT('Ctrl Pts',(4.03580121899994,2.2,0.371350974999984));
#346169=CARTESIAN_POINT('Ctrl Pts',(4.03494436999994,12.2,0.371418534999983));
#346170=CARTESIAN_POINT('Ctrl Pts',(4.03494436999994,5.2,0.371418534999983));
#346171=CARTESIAN_POINT('Ctrl Pts',(4.03494436999994,2.2,0.371418534999983));
#346172=CARTESIAN_POINT('Ctrl Pts',(4.03409314899995,12.2,0.371484579999986));
#346173=CARTESIAN_POINT('Ctrl Pts',(4.03409314899995,5.2,0.371484579999986));
#346174=CARTESIAN_POINT('Ctrl Pts',(4.03409314899995,2.2,0.371484579999986));
#346175=CARTESIAN_POINT('Ctrl Pts',(4.03324756799995,12.2,0.371549123999984));
#346176=CARTESIAN_POINT('Ctrl Pts',(4.03324756799995,5.2,0.371549123999984));
#346177=CARTESIAN_POINT('Ctrl Pts',(4.03324756799995,2.2,0.371549123999984));
#346178=CARTESIAN_POINT('Ctrl Pts',(4.03240764099994,12.2,0.371612176999987));
#346179=CARTESIAN_POINT('Ctrl Pts',(4.03240764099994,5.2,0.371612176999987));
#346180=CARTESIAN_POINT('Ctrl Pts',(4.03240764099994,2.2,0.371612176999987));
#346181=CARTESIAN_POINT('Ctrl Pts',(4.03157337899995,12.2,0.371673753999988));
#346182=CARTESIAN_POINT('Ctrl Pts',(4.03157337899995,5.2,0.371673753999988));
#346183=CARTESIAN_POINT('Ctrl Pts',(4.03157337899995,2.2,0.371673753999988));
#346184=CARTESIAN_POINT('Ctrl Pts',(4.03074479599994,12.2,0.371733868999984));
#346185=CARTESIAN_POINT('Ctrl Pts',(4.03074479599994,5.2,0.371733868999984));
#346186=CARTESIAN_POINT('Ctrl Pts',(4.03074479599994,2.2,0.371733868999984));
#346187=CARTESIAN_POINT('Ctrl Pts',(4.02992190299994,12.2,0.371792531999984));
#346188=CARTESIAN_POINT('Ctrl Pts',(4.02992190299994,5.2,0.371792531999984));
#346189=CARTESIAN_POINT('Ctrl Pts',(4.02992190299994,2.2,0.371792531999984));
#346190=CARTESIAN_POINT('Ctrl Pts',(4.02910471299994,12.2,0.371849756999989));
#346191=CARTESIAN_POINT('Ctrl Pts',(4.02910471299994,5.2,0.371849756999989));
#346192=CARTESIAN_POINT('Ctrl Pts',(4.02910471299994,2.2,0.371849756999989));
#346193=CARTESIAN_POINT('Ctrl Pts',(4.02829323899994,12.2,0.371905558999988));
#346194=CARTESIAN_POINT('Ctrl Pts',(4.02829323899994,5.2,0.371905558999988));
#346195=CARTESIAN_POINT('Ctrl Pts',(4.02829323899994,2.2,0.371905558999988));
#346196=CARTESIAN_POINT('Ctrl Pts',(4.02748749399994,12.2,0.371959948999985));
#346197=CARTESIAN_POINT('Ctrl Pts',(4.02748749399994,5.2,0.371959948999985));
#346198=CARTESIAN_POINT('Ctrl Pts',(4.02748749399994,2.2,0.371959948999985));
#346199=CARTESIAN_POINT('Ctrl Pts',(4.02668748999994,12.2,0.372012940999986));
#346200=CARTESIAN_POINT('Ctrl Pts',(4.02668748999994,5.2,0.372012940999986));
#346201=CARTESIAN_POINT('Ctrl Pts',(4.02668748999994,2.2,0.372012940999986));
#346202=CARTESIAN_POINT('Ctrl Pts',(4.02589323899995,12.2,0.372064548999984));
#346203=CARTESIAN_POINT('Ctrl Pts',(4.02589323899995,5.2,0.372064548999984));
#346204=CARTESIAN_POINT('Ctrl Pts',(4.02589323899995,2.2,0.372064548999984));
#346205=CARTESIAN_POINT('Ctrl Pts',(4.02510475399994,12.2,0.372114783999984));
#346206=CARTESIAN_POINT('Ctrl Pts',(4.02510475399994,5.2,0.372114783999984));
#346207=CARTESIAN_POINT('Ctrl Pts',(4.02510475399994,2.2,0.372114783999984));
#346208=CARTESIAN_POINT('Ctrl Pts',(4.02432204899995,12.2,0.372163661999987));
#346209=CARTESIAN_POINT('Ctrl Pts',(4.02432204899995,5.2,0.372163661999987));
#346210=CARTESIAN_POINT('Ctrl Pts',(4.02432204899995,2.2,0.372163661999987));
#346211=CARTESIAN_POINT('Ctrl Pts',(4.02354513399994,12.2,0.372211193999985));
#346212=CARTESIAN_POINT('Ctrl Pts',(4.02354513399994,5.2,0.372211193999985));
#346213=CARTESIAN_POINT('Ctrl Pts',(4.02354513399994,2.2,0.372211193999985));
#346214=CARTESIAN_POINT('Ctrl Pts',(4.02277402399995,12.2,0.372257394999984));
#346215=CARTESIAN_POINT('Ctrl Pts',(4.02277402399995,5.2,0.372257394999984));
#346216=CARTESIAN_POINT('Ctrl Pts',(4.02277402399995,2.2,0.372257394999984));
#346217=CARTESIAN_POINT('Ctrl Pts',(4.02200873099994,12.2,0.372302277999985));
#346218=CARTESIAN_POINT('Ctrl Pts',(4.02200873099994,5.2,0.372302277999985));
#346219=CARTESIAN_POINT('Ctrl Pts',(4.02200873099994,2.2,0.372302277999985));
#346220=CARTESIAN_POINT('Ctrl Pts',(4.02124926799994,12.2,0.372345856999985));
#346221=CARTESIAN_POINT('Ctrl Pts',(4.02124926799994,5.2,0.372345856999985));
#346222=CARTESIAN_POINT('Ctrl Pts',(4.02124926799994,2.2,0.372345856999985));
#346223=CARTESIAN_POINT('Ctrl Pts',(4.02049564699994,12.2,0.372388144999984));
#346224=CARTESIAN_POINT('Ctrl Pts',(4.02049564699994,5.2,0.372388144999984));
#346225=CARTESIAN_POINT('Ctrl Pts',(4.02049564699994,2.2,0.372388144999984));
#346226=CARTESIAN_POINT('Ctrl Pts',(4.01974787999994,12.2,0.372429155999985));
#346227=CARTESIAN_POINT('Ctrl Pts',(4.01974787999994,5.2,0.372429155999985));
#346228=CARTESIAN_POINT('Ctrl Pts',(4.01974787999994,2.2,0.372429155999985));
#346229=CARTESIAN_POINT('Ctrl Pts',(4.01900598299994,12.2,0.372468902999987));
#346230=CARTESIAN_POINT('Ctrl Pts',(4.01900598299994,5.2,0.372468902999987));
#346231=CARTESIAN_POINT('Ctrl Pts',(4.01900598299994,2.2,0.372468902999987));
#346232=CARTESIAN_POINT('Ctrl Pts',(4.01826996599994,12.2,0.372507400999984));
#346233=CARTESIAN_POINT('Ctrl Pts',(4.01826996599994,5.2,0.372507400999984));
#346234=CARTESIAN_POINT('Ctrl Pts',(4.01826996599994,2.2,0.372507400999984));
#346235=CARTESIAN_POINT('Ctrl Pts',(4.01753984299994,12.2,0.372544663999985));
#346236=CARTESIAN_POINT('Ctrl Pts',(4.01753984299994,5.2,0.372544663999985));
#346237=CARTESIAN_POINT('Ctrl Pts',(4.01753984299994,2.2,0.372544663999985));
#346238=CARTESIAN_POINT('Ctrl Pts',(4.01681562499994,12.2,0.372580703999983));
#346239=CARTESIAN_POINT('Ctrl Pts',(4.01681562499994,5.2,0.372580703999983));
#346240=CARTESIAN_POINT('Ctrl Pts',(4.01681562499994,2.2,0.372580703999983));
#346241=CARTESIAN_POINT('Ctrl Pts',(4.01609732699994,12.2,0.372615535999987));
#346242=CARTESIAN_POINT('Ctrl Pts',(4.01609732699994,5.2,0.372615535999987));
#346243=CARTESIAN_POINT('Ctrl Pts',(4.01609732699994,2.2,0.372615535999987));
#346244=CARTESIAN_POINT('Ctrl Pts',(4.01538496099994,12.2,0.372649174999986));
#346245=CARTESIAN_POINT('Ctrl Pts',(4.01538496099994,5.2,0.372649174999986));
#346246=CARTESIAN_POINT('Ctrl Pts',(4.01538496099994,2.2,0.372649174999986));
#346247=CARTESIAN_POINT('Ctrl Pts',(4.01467854099994,12.2,0.372681631999985));
#346248=CARTESIAN_POINT('Ctrl Pts',(4.01467854099994,5.2,0.372681631999985));
#346249=CARTESIAN_POINT('Ctrl Pts',(4.01467854099994,2.2,0.372681631999985));
#346250=CARTESIAN_POINT('Ctrl Pts',(4.01397807799994,12.2,0.372712924999985));
#346251=CARTESIAN_POINT('Ctrl Pts',(4.01397807799994,5.2,0.372712924999985));
#346252=CARTESIAN_POINT('Ctrl Pts',(4.01397807799994,2.2,0.372712924999985));
#346253=CARTESIAN_POINT('Ctrl Pts',(4.01328358599994,12.2,0.372743064999987));
#346254=CARTESIAN_POINT('Ctrl Pts',(4.01328358599994,5.2,0.372743064999987));
#346255=CARTESIAN_POINT('Ctrl Pts',(4.01328358599994,2.2,0.372743064999987));
#346256=CARTESIAN_POINT('Ctrl Pts',(4.01259507899994,12.2,0.372772067999985));
#346257=CARTESIAN_POINT('Ctrl Pts',(4.01259507899994,5.2,0.372772067999985));
#346258=CARTESIAN_POINT('Ctrl Pts',(4.01259507899994,2.2,0.372772067999985));
#346259=CARTESIAN_POINT('Ctrl Pts',(4.01191256799994,12.2,0.372799947999987));
#346260=CARTESIAN_POINT('Ctrl Pts',(4.01191256799994,5.2,0.372799947999987));
#346261=CARTESIAN_POINT('Ctrl Pts',(4.01191256799994,2.2,0.372799947999987));
#346262=CARTESIAN_POINT('Ctrl Pts',(4.01123606699994,12.2,0.372826718999986));
#346263=CARTESIAN_POINT('Ctrl Pts',(4.01123606699994,5.2,0.372826718999986));
#346264=CARTESIAN_POINT('Ctrl Pts',(4.01123606699994,2.2,0.372826718999986));
#346265=CARTESIAN_POINT('Ctrl Pts',(4.01056558899994,12.2,0.372852395999987));
#346266=CARTESIAN_POINT('Ctrl Pts',(4.01056558899994,5.2,0.372852395999987));
#346267=CARTESIAN_POINT('Ctrl Pts',(4.01056558899994,2.2,0.372852395999987));
#346268=CARTESIAN_POINT('Ctrl Pts',(4.00990114699994,12.2,0.372876991999984));
#346269=CARTESIAN_POINT('Ctrl Pts',(4.00990114699994,5.2,0.372876991999984));
#346270=CARTESIAN_POINT('Ctrl Pts',(4.00990114699994,2.2,0.372876991999984));
#346271=CARTESIAN_POINT('Ctrl Pts',(4.00924275299994,12.2,0.372900522999986));
#346272=CARTESIAN_POINT('Ctrl Pts',(4.00924275299994,5.2,0.372900522999986));
#346273=CARTESIAN_POINT('Ctrl Pts',(4.00924275299994,2.2,0.372900522999986));
#346274=CARTESIAN_POINT('Ctrl Pts',(4.00859042199994,12.2,0.372923001999985));
#346275=CARTESIAN_POINT('Ctrl Pts',(4.00859042199994,5.2,0.372923001999985));
#346276=CARTESIAN_POINT('Ctrl Pts',(4.00859042199994,2.2,0.372923001999985));
#346277=CARTESIAN_POINT('Ctrl Pts',(4.00794416599994,12.2,0.372944444999987));
#346278=CARTESIAN_POINT('Ctrl Pts',(4.00794416599994,5.2,0.372944444999987));
#346279=CARTESIAN_POINT('Ctrl Pts',(4.00794416599994,2.2,0.372944444999987));
#346280=CARTESIAN_POINT('Ctrl Pts',(4.00730399899994,12.2,0.372964865999985));
#346281=CARTESIAN_POINT('Ctrl Pts',(4.00730399899994,5.2,0.372964865999985));
#346282=CARTESIAN_POINT('Ctrl Pts',(4.00730399899994,2.2,0.372964865999985));
#346283=CARTESIAN_POINT('Ctrl Pts',(4.00666993199995,12.2,0.372984279999984));
#346284=CARTESIAN_POINT('Ctrl Pts',(4.00666993199995,5.2,0.372984279999984));
#346285=CARTESIAN_POINT('Ctrl Pts',(4.00666993199995,2.2,0.372984279999984));
#346286=CARTESIAN_POINT('Ctrl Pts',(4.00604197999994,12.2,0.373002701999985));
#346287=CARTESIAN_POINT('Ctrl Pts',(4.00604197999994,5.2,0.373002701999985));
#346288=CARTESIAN_POINT('Ctrl Pts',(4.00604197999994,2.2,0.373002701999985));
#346289=CARTESIAN_POINT('Ctrl Pts',(4.00542015699994,12.2,0.373020146999985));
#346290=CARTESIAN_POINT('Ctrl Pts',(4.00542015699994,5.2,0.373020146999985));
#346291=CARTESIAN_POINT('Ctrl Pts',(4.00542015699994,2.2,0.373020146999985));
#346292=CARTESIAN_POINT('Ctrl Pts',(4.00480447399994,12.2,0.373036628999985));
#346293=CARTESIAN_POINT('Ctrl Pts',(4.00480447399994,5.2,0.373036628999985));
#346294=CARTESIAN_POINT('Ctrl Pts',(4.00480447399994,2.2,0.373036628999985));
#346295=CARTESIAN_POINT('Ctrl Pts',(4.00419494499994,12.2,0.373052163999983));
#346296=CARTESIAN_POINT('Ctrl Pts',(4.00419494499994,5.2,0.373052163999983));
#346297=CARTESIAN_POINT('Ctrl Pts',(4.00419494499994,2.2,0.373052163999983));
#346298=CARTESIAN_POINT('Ctrl Pts',(4.00359158399994,12.2,0.373066765999983));
#346299=CARTESIAN_POINT('Ctrl Pts',(4.00359158399994,5.2,0.373066765999983));
#346300=CARTESIAN_POINT('Ctrl Pts',(4.00359158399994,2.2,0.373066765999983));
#346301=CARTESIAN_POINT('Ctrl Pts',(4.00299440399994,12.2,0.373080450999983));
#346302=CARTESIAN_POINT('Ctrl Pts',(4.00299440399994,5.2,0.373080450999983));
#346303=CARTESIAN_POINT('Ctrl Pts',(4.00299440399994,2.2,0.373080450999983));
#346304=CARTESIAN_POINT('Ctrl Pts',(4.00240341799995,12.2,0.373093232999988));
#346305=CARTESIAN_POINT('Ctrl Pts',(4.00240341799995,5.2,0.373093232999988));
#346306=CARTESIAN_POINT('Ctrl Pts',(4.00240341799995,2.2,0.373093232999988));
#346307=CARTESIAN_POINT('Ctrl Pts',(4.00181863899994,12.2,0.373105127999986));
#346308=CARTESIAN_POINT('Ctrl Pts',(4.00181863899994,5.2,0.373105127999986));
#346309=CARTESIAN_POINT('Ctrl Pts',(4.00181863899994,2.2,0.373105127999986));
#346310=CARTESIAN_POINT('Ctrl Pts',(4.00124008099994,12.2,0.373116152999984));
#346311=CARTESIAN_POINT('Ctrl Pts',(4.00124008099994,5.2,0.373116152999984));
#346312=CARTESIAN_POINT('Ctrl Pts',(4.00124008099994,2.2,0.373116152999984));
#346313=CARTESIAN_POINT('Ctrl Pts',(4.00066775699994,12.2,0.373126319999986));
#346314=CARTESIAN_POINT('Ctrl Pts',(4.00066775699994,5.2,0.373126319999986));
#346315=CARTESIAN_POINT('Ctrl Pts',(4.00066775699994,2.2,0.373126319999986));
#346316=CARTESIAN_POINT('Ctrl Pts',(4.00010167999994,12.2,0.373135644999985));
#346317=CARTESIAN_POINT('Ctrl Pts',(4.00010167999994,5.2,0.373135644999985));
#346318=CARTESIAN_POINT('Ctrl Pts',(4.00010167999994,2.2,0.373135644999985));
#346319=CARTESIAN_POINT('Ctrl Pts',(3.99954186399994,12.2,0.373144146999986));
#346320=CARTESIAN_POINT('Ctrl Pts',(3.99954186399994,5.2,0.373144146999986));
#346321=CARTESIAN_POINT('Ctrl Pts',(3.99954186399994,2.2,0.373144146999986));
#346322=CARTESIAN_POINT('Ctrl Pts',(3.99898832299994,12.2,0.373151836999988));
#346323=CARTESIAN_POINT('Ctrl Pts',(3.99898832299994,5.2,0.373151836999988));
#346324=CARTESIAN_POINT('Ctrl Pts',(3.99898832299994,2.2,0.373151836999988));
#346325=CARTESIAN_POINT('Ctrl Pts',(3.99844106899994,12.2,0.373158732999985));
#346326=CARTESIAN_POINT('Ctrl Pts',(3.99844106899994,5.2,0.373158732999985));
#346327=CARTESIAN_POINT('Ctrl Pts',(3.99844106899994,2.2,0.373158732999985));
#346328=CARTESIAN_POINT('Ctrl Pts',(3.99790011699994,12.2,0.373164850999985));
#346329=CARTESIAN_POINT('Ctrl Pts',(3.99790011699994,5.2,0.373164850999985));
#346330=CARTESIAN_POINT('Ctrl Pts',(3.99790011699994,2.2,0.373164850999985));
#346331=CARTESIAN_POINT('Ctrl Pts',(3.99736547899994,12.2,0.373170204999984));
#346332=CARTESIAN_POINT('Ctrl Pts',(3.99736547899994,5.2,0.373170204999984));
#346333=CARTESIAN_POINT('Ctrl Pts',(3.99736547899994,2.2,0.373170204999984));
#346334=CARTESIAN_POINT('Ctrl Pts',(3.99683716899994,12.2,0.373174810999988));
#346335=CARTESIAN_POINT('Ctrl Pts',(3.99683716899994,5.2,0.373174810999988));
#346336=CARTESIAN_POINT('Ctrl Pts',(3.99683716899994,2.2,0.373174810999988));
#346337=CARTESIAN_POINT('Ctrl Pts',(3.99631520299994,12.2,0.373178685999989));
#346338=CARTESIAN_POINT('Ctrl Pts',(3.99631520299994,5.2,0.373178685999989));
#346339=CARTESIAN_POINT('Ctrl Pts',(3.99631520299994,2.2,0.373178685999989));
#346340=CARTESIAN_POINT('Ctrl Pts',(3.99579958899994,12.2,0.373181846999984));
#346341=CARTESIAN_POINT('Ctrl Pts',(3.99579958899994,5.2,0.373181846999984));
#346342=CARTESIAN_POINT('Ctrl Pts',(3.99579958899994,2.2,0.373181846999984));
#346343=CARTESIAN_POINT('Ctrl Pts',(3.99529034599994,12.2,0.373184306999987));
#346344=CARTESIAN_POINT('Ctrl Pts',(3.99529034599994,5.2,0.373184306999987));
#346345=CARTESIAN_POINT('Ctrl Pts',(3.99529034599994,2.2,0.373184306999987));
#346346=CARTESIAN_POINT('Ctrl Pts',(3.99478748599994,12.2,0.373186083999983));
#346347=CARTESIAN_POINT('Ctrl Pts',(3.99478748599994,5.2,0.373186083999983));
#346348=CARTESIAN_POINT('Ctrl Pts',(3.99478748599994,2.2,0.373186083999983));
#346349=CARTESIAN_POINT('Ctrl Pts',(3.99429102099994,12.2,0.373187192999982));
#346350=CARTESIAN_POINT('Ctrl Pts',(3.99429102099994,5.2,0.373187192999982));
#346351=CARTESIAN_POINT('Ctrl Pts',(3.99429102099994,2.2,0.373187192999982));
#346352=CARTESIAN_POINT('Ctrl Pts',(3.99380096699994,12.2,0.373187650999984));
#346353=CARTESIAN_POINT('Ctrl Pts',(3.99380096699994,5.2,0.373187650999984));
#346354=CARTESIAN_POINT('Ctrl Pts',(3.99380096699994,2.2,0.373187650999984));
#346355=CARTESIAN_POINT('Ctrl Pts',(3.99331733399995,12.2,0.373187473999987));
#346356=CARTESIAN_POINT('Ctrl Pts',(3.99331733399995,5.2,0.373187473999987));
#346357=CARTESIAN_POINT('Ctrl Pts',(3.99331733399995,2.2,0.373187473999987));
#346358=CARTESIAN_POINT('Ctrl Pts',(3.99284013999994,12.2,0.373186677999984));
#346359=CARTESIAN_POINT('Ctrl Pts',(3.99284013999994,5.2,0.373186677999984));
#346360=CARTESIAN_POINT('Ctrl Pts',(3.99284013999994,2.2,0.373186677999984));
#346361=CARTESIAN_POINT('Ctrl Pts',(3.99236939699994,12.2,0.373185279999984));
#346362=CARTESIAN_POINT('Ctrl Pts',(3.99236939699994,5.2,0.373185279999984));
#346363=CARTESIAN_POINT('Ctrl Pts',(3.99236939699994,2.2,0.373185279999984));
#346364=CARTESIAN_POINT('Ctrl Pts',(3.99190511899994,12.2,0.373183295999984));
#346365=CARTESIAN_POINT('Ctrl Pts',(3.99190511899994,5.2,0.373183295999984));
#346366=CARTESIAN_POINT('Ctrl Pts',(3.99190511899994,2.2,0.373183295999984));
#346367=CARTESIAN_POINT('Ctrl Pts',(3.99144731899994,12.2,0.373180742999986));
#346368=CARTESIAN_POINT('Ctrl Pts',(3.99144731899994,5.2,0.373180742999986));
#346369=CARTESIAN_POINT('Ctrl Pts',(3.99144731899994,2.2,0.373180742999986));
#346370=CARTESIAN_POINT('Ctrl Pts',(3.99099601199994,12.2,0.373177636999986));
#346371=CARTESIAN_POINT('Ctrl Pts',(3.99099601199994,5.2,0.373177636999986));
#346372=CARTESIAN_POINT('Ctrl Pts',(3.99099601199994,2.2,0.373177636999986));
#346373=CARTESIAN_POINT('Ctrl Pts',(3.99055120999994,12.2,0.373173994999987));
#346374=CARTESIAN_POINT('Ctrl Pts',(3.99055120999994,5.2,0.373173994999987));
#346375=CARTESIAN_POINT('Ctrl Pts',(3.99055120999994,2.2,0.373173994999987));
#346376=CARTESIAN_POINT('Ctrl Pts',(3.99011292899994,12.2,0.373169832999984));
#346377=CARTESIAN_POINT('Ctrl Pts',(3.99011292899994,5.2,0.373169832999984));
#346378=CARTESIAN_POINT('Ctrl Pts',(3.99011292899994,2.2,0.373169832999984));
#346379=CARTESIAN_POINT('Ctrl Pts',(3.98968118199994,12.2,0.373165167999985));
#346380=CARTESIAN_POINT('Ctrl Pts',(3.98968118199994,5.2,0.373165167999985));
#346381=CARTESIAN_POINT('Ctrl Pts',(3.98968118199994,2.2,0.373165167999985));
#346382=CARTESIAN_POINT('Ctrl Pts',(3.98925598199994,12.2,0.373160018999985));
#346383=CARTESIAN_POINT('Ctrl Pts',(3.98925598199994,5.2,0.373160018999985));
#346384=CARTESIAN_POINT('Ctrl Pts',(3.98925598199994,2.2,0.373160018999985));
#346385=CARTESIAN_POINT('Ctrl Pts',(3.98883734399994,12.2,0.373154398999986));
#346386=CARTESIAN_POINT('Ctrl Pts',(3.98883734399994,5.2,0.373154398999986));
#346387=CARTESIAN_POINT('Ctrl Pts',(3.98883734399994,2.2,0.373154398999986));
#346388=CARTESIAN_POINT('Ctrl Pts',(3.98842528099994,12.2,0.373148327999986));
#346389=CARTESIAN_POINT('Ctrl Pts',(3.98842528099994,5.2,0.373148327999986));
#346390=CARTESIAN_POINT('Ctrl Pts',(3.98842528099994,2.2,0.373148327999986));
#346391=CARTESIAN_POINT('Ctrl Pts',(3.98801980899994,12.2,0.373141822999985));
#346392=CARTESIAN_POINT('Ctrl Pts',(3.98801980899994,5.2,0.373141822999985));
#346393=CARTESIAN_POINT('Ctrl Pts',(3.98801980899994,2.2,0.373141822999985));
#346394=CARTESIAN_POINT('Ctrl Pts',(3.98762093899994,12.2,0.373134899999985));
#346395=CARTESIAN_POINT('Ctrl Pts',(3.98762093899994,5.2,0.373134899999985));
#346396=CARTESIAN_POINT('Ctrl Pts',(3.98762093899994,2.2,0.373134899999985));
#346397=CARTESIAN_POINT('Ctrl Pts',(3.98722868799994,12.2,0.373127575999987));
#346398=CARTESIAN_POINT('Ctrl Pts',(3.98722868799994,5.2,0.373127575999987));
#346399=CARTESIAN_POINT('Ctrl Pts',(3.98722868799994,2.2,0.373127575999987));
#346400=CARTESIAN_POINT('Ctrl Pts',(3.98684306899994,12.2,0.373119868999985));
#346401=CARTESIAN_POINT('Ctrl Pts',(3.98684306899994,5.2,0.373119868999985));
#346402=CARTESIAN_POINT('Ctrl Pts',(3.98684306899994,2.2,0.373119868999985));
#346403=CARTESIAN_POINT('Ctrl Pts',(3.98646409499994,12.2,0.373111795999983));
#346404=CARTESIAN_POINT('Ctrl Pts',(3.98646409499994,5.2,0.373111795999983));
#346405=CARTESIAN_POINT('Ctrl Pts',(3.98646409499994,2.2,0.373111795999983));
#346406=CARTESIAN_POINT('Ctrl Pts',(3.98609178199994,12.2,0.373103375999988));
#346407=CARTESIAN_POINT('Ctrl Pts',(3.98609178199994,5.2,0.373103375999988));
#346408=CARTESIAN_POINT('Ctrl Pts',(3.98609178199994,2.2,0.373103375999988));
#346409=CARTESIAN_POINT('Ctrl Pts',(3.98572614199994,12.2,0.373094623999983));
#346410=CARTESIAN_POINT('Ctrl Pts',(3.98572614199994,5.2,0.373094623999983));
#346411=CARTESIAN_POINT('Ctrl Pts',(3.98572614199994,2.2,0.373094623999983));
#346412=CARTESIAN_POINT('Ctrl Pts',(3.98536718999994,12.2,0.373085557999988));
#346413=CARTESIAN_POINT('Ctrl Pts',(3.98536718999994,5.2,0.373085557999988));
#346414=CARTESIAN_POINT('Ctrl Pts',(3.98536718999994,2.2,0.373085557999988));
#346415=CARTESIAN_POINT('Ctrl Pts',(3.98501494199994,12.2,0.373076197999986));
#346416=CARTESIAN_POINT('Ctrl Pts',(3.98501494199994,5.2,0.373076197999986));
#346417=CARTESIAN_POINT('Ctrl Pts',(3.98501494199994,2.2,0.373076197999986));
#346418=CARTESIAN_POINT('Ctrl Pts',(3.98466940899994,12.2,0.373066557999984));
#346419=CARTESIAN_POINT('Ctrl Pts',(3.98466940899994,5.2,0.373066557999984));
#346420=CARTESIAN_POINT('Ctrl Pts',(3.98466940899994,2.2,0.373066557999984));
#346421=CARTESIAN_POINT('Ctrl Pts',(3.98433060799994,12.2,0.373056658999986));
#346422=CARTESIAN_POINT('Ctrl Pts',(3.98433060799994,5.2,0.373056658999986));
#346423=CARTESIAN_POINT('Ctrl Pts',(3.98433060799994,2.2,0.373056658999986));
#346424=CARTESIAN_POINT('Ctrl Pts',(3.98399855199994,12.2,0.373046518999987));
#346425=CARTESIAN_POINT('Ctrl Pts',(3.98399855199994,5.2,0.373046518999987));
#346426=CARTESIAN_POINT('Ctrl Pts',(3.98399855199994,2.2,0.373046518999987));
#346427=CARTESIAN_POINT('Ctrl Pts',(3.98367325499994,12.2,0.373036153999986));
#346428=CARTESIAN_POINT('Ctrl Pts',(3.98367325499994,5.2,0.373036153999986));
#346429=CARTESIAN_POINT('Ctrl Pts',(3.98367325499994,2.2,0.373036153999986));
#346430=CARTESIAN_POINT('Ctrl Pts',(3.98335473199994,12.2,0.373025581999986));
#346431=CARTESIAN_POINT('Ctrl Pts',(3.98335473199994,5.2,0.373025581999986));
#346432=CARTESIAN_POINT('Ctrl Pts',(3.98335473199994,2.2,0.373025581999986));
#346433=CARTESIAN_POINT('Ctrl Pts',(3.98304299799995,12.2,0.373014822999984));
#346434=CARTESIAN_POINT('Ctrl Pts',(3.98304299799995,5.2,0.373014822999984));
#346435=CARTESIAN_POINT('Ctrl Pts',(3.98304299799995,2.2,0.373014822999984));
#346436=CARTESIAN_POINT('Ctrl Pts',(3.98273806599994,12.2,0.373003892999986));
#346437=CARTESIAN_POINT('Ctrl Pts',(3.98273806599994,5.2,0.373003892999986));
#346438=CARTESIAN_POINT('Ctrl Pts',(3.98273806599994,2.2,0.373003892999986));
#346439=CARTESIAN_POINT('Ctrl Pts',(3.98243995099994,12.2,0.372992811999988));
#346440=CARTESIAN_POINT('Ctrl Pts',(3.98243995099994,5.2,0.372992811999988));
#346441=CARTESIAN_POINT('Ctrl Pts',(3.98243995099994,2.2,0.372992811999988));
#346442=CARTESIAN_POINT('Ctrl Pts',(3.98214866699994,12.2,0.372981597999988));
#346443=CARTESIAN_POINT('Ctrl Pts',(3.98214866699994,5.2,0.372981597999988));
#346444=CARTESIAN_POINT('Ctrl Pts',(3.98214866699994,2.2,0.372981597999988));
#346445=CARTESIAN_POINT('Ctrl Pts',(3.98186422899994,12.2,0.372970267999988));
#346446=CARTESIAN_POINT('Ctrl Pts',(3.98186422899994,5.2,0.372970267999988));
#346447=CARTESIAN_POINT('Ctrl Pts',(3.98186422899994,2.2,0.372970267999988));
#346448=CARTESIAN_POINT('Ctrl Pts',(3.98158665199994,12.2,0.372958841999989));
#346449=CARTESIAN_POINT('Ctrl Pts',(3.98158665199994,5.2,0.372958841999989));
#346450=CARTESIAN_POINT('Ctrl Pts',(3.98158665199994,2.2,0.372958841999989));
#346451=CARTESIAN_POINT('Ctrl Pts',(3.98131594999994,12.2,0.372947338999987));
#346452=CARTESIAN_POINT('Ctrl Pts',(3.98131594999994,5.2,0.372947338999987));
#346453=CARTESIAN_POINT('Ctrl Pts',(3.98131594999994,2.2,0.372947338999987));
#346454=CARTESIAN_POINT('Ctrl Pts',(3.98105213699994,12.2,0.372935775999985));
#346455=CARTESIAN_POINT('Ctrl Pts',(3.98105213699994,5.2,0.372935775999985));
#346456=CARTESIAN_POINT('Ctrl Pts',(3.98105213699994,2.2,0.372935775999985));
#346457=CARTESIAN_POINT('Ctrl Pts',(3.98079522899994,12.2,0.372924173999984));
#346458=CARTESIAN_POINT('Ctrl Pts',(3.98079522899994,5.2,0.372924173999984));
#346459=CARTESIAN_POINT('Ctrl Pts',(3.98079522899994,2.2,0.372924173999984));
#346460=CARTESIAN_POINT('Ctrl Pts',(3.98054523899994,12.2,0.372912548999986));
#346461=CARTESIAN_POINT('Ctrl Pts',(3.98054523899994,5.2,0.372912548999986));
#346462=CARTESIAN_POINT('Ctrl Pts',(3.98054523899994,2.2,0.372912548999986));
#346463=CARTESIAN_POINT('Ctrl Pts',(3.98030218199994,12.2,0.372900921999988));
#346464=CARTESIAN_POINT('Ctrl Pts',(3.98030218199994,5.2,0.372900921999988));
#346465=CARTESIAN_POINT('Ctrl Pts',(3.98030218199994,2.2,0.372900921999988));
#346466=CARTESIAN_POINT('Ctrl Pts',(3.98006607399994,12.2,0.372889311999987));
#346467=CARTESIAN_POINT('Ctrl Pts',(3.98006607399994,5.2,0.372889311999987));
#346468=CARTESIAN_POINT('Ctrl Pts',(3.98006607399994,2.2,0.372889311999987));
#346469=CARTESIAN_POINT('Ctrl Pts',(3.97983692799994,12.2,0.372877735999988));
#346470=CARTESIAN_POINT('Ctrl Pts',(3.97983692799994,5.2,0.372877735999988));
#346471=CARTESIAN_POINT('Ctrl Pts',(3.97983692799994,2.2,0.372877735999988));
#346472=CARTESIAN_POINT('Ctrl Pts',(3.97961475899994,12.2,0.372866213999985));
#346473=CARTESIAN_POINT('Ctrl Pts',(3.97961475899994,5.2,0.372866213999985));
#346474=CARTESIAN_POINT('Ctrl Pts',(3.97961475899994,2.2,0.372866213999985));
#346475=CARTESIAN_POINT('Ctrl Pts',(3.97939958299994,12.2,0.372854766999984));
#346476=CARTESIAN_POINT('Ctrl Pts',(3.97939958299994,5.2,0.372854766999984));
#346477=CARTESIAN_POINT('Ctrl Pts',(3.97939958299994,2.2,0.372854766999984));
#346478=CARTESIAN_POINT('Ctrl Pts',(3.97919141399994,12.2,0.372843411999986));
#346479=CARTESIAN_POINT('Ctrl Pts',(3.97919141399994,5.2,0.372843411999986));
#346480=CARTESIAN_POINT('Ctrl Pts',(3.97919141399994,2.2,0.372843411999986));
#346481=CARTESIAN_POINT('Ctrl Pts',(3.97899026699994,12.2,0.372832170999988));
#346482=CARTESIAN_POINT('Ctrl Pts',(3.97899026699994,5.2,0.372832170999988));
#346483=CARTESIAN_POINT('Ctrl Pts',(3.97899026699994,2.2,0.372832170999988));
#346484=CARTESIAN_POINT('Ctrl Pts',(3.97879615699994,12.2,0.372821060999984));
#346485=CARTESIAN_POINT('Ctrl Pts',(3.97879615699994,5.2,0.372821060999984));
#346486=CARTESIAN_POINT('Ctrl Pts',(3.97879615699994,2.2,0.372821060999984));
#346487=CARTESIAN_POINT('Ctrl Pts',(3.97860909799994,12.2,0.372810104999988));
#346488=CARTESIAN_POINT('Ctrl Pts',(3.97860909799994,5.2,0.372810104999988));
#346489=CARTESIAN_POINT('Ctrl Pts',(3.97860909799994,2.2,0.372810104999988));
#346490=CARTESIAN_POINT('Ctrl Pts',(3.97842910699994,12.2,0.372799318999988));
#346491=CARTESIAN_POINT('Ctrl Pts',(3.97842910699994,5.2,0.372799318999988));
#346492=CARTESIAN_POINT('Ctrl Pts',(3.97842910699994,2.2,0.372799318999988));
#346493=CARTESIAN_POINT('Ctrl Pts',(3.97825619699994,12.2,0.372788722999986));
#346494=CARTESIAN_POINT('Ctrl Pts',(3.97825619699994,5.2,0.372788722999986));
#346495=CARTESIAN_POINT('Ctrl Pts',(3.97825619699994,2.2,0.372788722999986));
#346496=CARTESIAN_POINT('Ctrl Pts',(3.97809038299994,12.2,0.372778337999984));
#346497=CARTESIAN_POINT('Ctrl Pts',(3.97809038299994,5.2,0.372778337999984));
#346498=CARTESIAN_POINT('Ctrl Pts',(3.97809038299994,2.2,0.372778337999984));
#346499=CARTESIAN_POINT('Ctrl Pts',(3.97793167899994,12.2,0.372768182999987));
#346500=CARTESIAN_POINT('Ctrl Pts',(3.97793167899994,5.2,0.372768182999987));
#346501=CARTESIAN_POINT('Ctrl Pts',(3.97793167899994,2.2,0.372768182999987));
#346502=CARTESIAN_POINT('Ctrl Pts',(3.97778010099994,12.2,0.372758277999985));
#346503=CARTESIAN_POINT('Ctrl Pts',(3.97778010099994,5.2,0.372758277999985));
#346504=CARTESIAN_POINT('Ctrl Pts',(3.97778010099994,2.2,0.372758277999985));
#346505=CARTESIAN_POINT('Ctrl Pts',(3.97763566599994,12.2,0.372748643999987));
#346506=CARTESIAN_POINT('Ctrl Pts',(3.97763566599994,5.2,0.372748643999987));
#346507=CARTESIAN_POINT('Ctrl Pts',(3.97763566599994,2.2,0.372748643999987));
#346508=CARTESIAN_POINT('Ctrl Pts',(3.97749838899994,12.2,0.372739301999987));
#346509=CARTESIAN_POINT('Ctrl Pts',(3.97749838899994,5.2,0.372739301999987));
#346510=CARTESIAN_POINT('Ctrl Pts',(3.97749838899994,2.2,0.372739301999987));
#346511=CARTESIAN_POINT('Ctrl Pts',(3.97736828499994,12.2,0.372730274999986));
#346512=CARTESIAN_POINT('Ctrl Pts',(3.97736828499994,5.2,0.372730274999986));
#346513=CARTESIAN_POINT('Ctrl Pts',(3.97736828499994,2.2,0.372730274999986));
#346514=CARTESIAN_POINT('Ctrl Pts',(3.97724536999994,12.2,0.372721580999986));
#346515=CARTESIAN_POINT('Ctrl Pts',(3.97724536999994,5.2,0.372721580999986));
#346516=CARTESIAN_POINT('Ctrl Pts',(3.97724536999994,2.2,0.372721580999986));
#346517=CARTESIAN_POINT('Ctrl Pts',(3.97712965699994,12.2,0.372713236999989));
#346518=CARTESIAN_POINT('Ctrl Pts',(3.97712965699994,5.2,0.372713236999989));
#346519=CARTESIAN_POINT('Ctrl Pts',(3.97712965699994,2.2,0.372713236999989));
#346520=CARTESIAN_POINT('Ctrl Pts',(3.97702115899994,12.2,0.372705264999986));
#346521=CARTESIAN_POINT('Ctrl Pts',(3.97702115899994,5.2,0.372705264999986));
#346522=CARTESIAN_POINT('Ctrl Pts',(3.97702115899994,2.2,0.372705264999986));
#346523=CARTESIAN_POINT('Ctrl Pts',(3.97691989099994,12.2,0.372697680999985));
#346524=CARTESIAN_POINT('Ctrl Pts',(3.97691989099994,5.2,0.372697680999985));
#346525=CARTESIAN_POINT('Ctrl Pts',(3.97691989099994,2.2,0.372697680999985));
#346526=CARTESIAN_POINT('Ctrl Pts',(3.97682586699994,12.2,0.372690505999986));
#346527=CARTESIAN_POINT('Ctrl Pts',(3.97682586699994,5.2,0.372690505999986));
#346528=CARTESIAN_POINT('Ctrl Pts',(3.97682586699994,2.2,0.372690505999986));
#346529=CARTESIAN_POINT('Ctrl Pts',(3.97673910699994,12.2,0.372683765999984));
#346530=CARTESIAN_POINT('Ctrl Pts',(3.97673910699994,5.2,0.372683765999984));
#346531=CARTESIAN_POINT('Ctrl Pts',(3.97673910699994,2.2,0.372683765999984));
#346532=CARTESIAN_POINT('Ctrl Pts',(3.97665962899994,12.2,0.372677485999984));
#346533=CARTESIAN_POINT('Ctrl Pts',(3.97665962899994,5.2,0.372677485999984));
#346534=CARTESIAN_POINT('Ctrl Pts',(3.97665962899994,2.2,0.372677485999984));
#346535=CARTESIAN_POINT('Ctrl Pts',(3.97658745199994,12.2,0.372671693999984));
#346536=CARTESIAN_POINT('Ctrl Pts',(3.97658745199994,5.2,0.372671693999984));
#346537=CARTESIAN_POINT('Ctrl Pts',(3.97658745199994,2.2,0.372671693999984));
#346538=CARTESIAN_POINT('Ctrl Pts',(3.97652259499994,12.2,0.372666410999987));
#346539=CARTESIAN_POINT('Ctrl Pts',(3.97652259499994,5.2,0.372666410999987));
#346540=CARTESIAN_POINT('Ctrl Pts',(3.97652259499994,2.2,0.372666410999987));
#346541=CARTESIAN_POINT('Ctrl Pts',(3.97646506799994,12.2,0.372661654999984));
#346542=CARTESIAN_POINT('Ctrl Pts',(3.97646506799994,5.2,0.372661654999984));
#346543=CARTESIAN_POINT('Ctrl Pts',(3.97646506799994,2.2,0.372661654999984));
#346544=CARTESIAN_POINT('Ctrl Pts',(3.97640950604921,12.2,0.372656984337683));
#346545=CARTESIAN_POINT('Ctrl Pts',(3.97640950604921,5.2,0.372656984337683));
#346546=CARTESIAN_POINT('Ctrl Pts',(3.97640950604921,2.2,0.372656984337683));
#346547=CARTESIAN_POINT('Ctrl Pts',(3.97637153472191,12.2,0.372653714372708));
#346548=CARTESIAN_POINT('Ctrl Pts',(3.97637153472191,5.2,0.372653714372708));
#346549=CARTESIAN_POINT('Ctrl Pts',(3.97637153472191,2.2,0.372653714372708));
#346550=CARTESIAN_POINT('Ctrl Pts',(3.97634652385127,12.2,0.372651508425408));
#346551=CARTESIAN_POINT('Ctrl Pts',(3.97634652385127,5.2,0.372651508425408));
#346552=CARTESIAN_POINT('Ctrl Pts',(3.97634652385127,2.2,0.372651508425408));
#346553=CARTESIAN_POINT('Ctrl Pts',(3.97633094703549,12.2,0.372650094949822));
#346554=CARTESIAN_POINT('Ctrl Pts',(3.97633094703549,5.2,0.372650094949822));
#346555=CARTESIAN_POINT('Ctrl Pts',(3.97633094703549,2.2,0.372650094949822));
#346556=CARTESIAN_POINT('Ctrl Pts',(3.97632132799994,12.2,0.372649231999986));
#346557=CARTESIAN_POINT('Ctrl Pts',(3.97632132799994,5.2,0.372649231999986));
#346558=CARTESIAN_POINT('Ctrl Pts',(3.97632132799994,2.2,0.372649231999986));
#346559=CARTESIAN_POINT('',(4.74889012999994,12.2,0.102676828999986));
#346560=CARTESIAN_POINT('Origin',(-5.66300478732629E-14,15.2,-1.77635683940025E-14));
#346561=CARTESIAN_POINT('',(4.74421990499994,12.2,-0.234259451000014));
#346562=CARTESIAN_POINT('Ctrl Pts',(3.96444825599994,12.2,-0.482713322000015));
#346563=CARTESIAN_POINT('Ctrl Pts',(3.96444825599994,5.2,-0.482713322000015));
#346564=CARTESIAN_POINT('Ctrl Pts',(3.96444825599994,2.2,-0.482713322000015));
#346565=CARTESIAN_POINT('Ctrl Pts',(3.9644550525987,12.2,-0.482714122952763));
#346566=CARTESIAN_POINT('Ctrl Pts',(3.9644550525987,5.2,-0.482714122952763));
#346567=CARTESIAN_POINT('Ctrl Pts',(3.9644550525987,2.2,-0.482714122952763));
#346568=CARTESIAN_POINT('Ctrl Pts',(3.96446819348808,12.2,-0.482715670305005));
#346569=CARTESIAN_POINT('Ctrl Pts',(3.96446819348808,5.2,-0.482715670305005));
#346570=CARTESIAN_POINT('Ctrl Pts',(3.96446819348808,2.2,-0.482715670305005));
#346571=CARTESIAN_POINT('Ctrl Pts',(3.9644876922665,12.2,-0.482717970545998));
#346572=CARTESIAN_POINT('Ctrl Pts',(3.9644876922665,5.2,-0.482717970545998));
#346573=CARTESIAN_POINT('Ctrl Pts',(3.9644876922665,2.2,-0.482717970545998));
#346574=CARTESIAN_POINT('Ctrl Pts',(3.96451349997268,12.2,-0.482721030842654));
#346575=CARTESIAN_POINT('Ctrl Pts',(3.96451349997268,5.2,-0.482721030842654));
#346576=CARTESIAN_POINT('Ctrl Pts',(3.96451349997268,2.2,-0.482721030842654));
#346577=CARTESIAN_POINT('Ctrl Pts',(3.96455853299994,12.2,-0.482726117000016));
#346578=CARTESIAN_POINT('Ctrl Pts',(3.96455853299994,5.2,-0.482726117000016));
#346579=CARTESIAN_POINT('Ctrl Pts',(3.96455853299994,2.2,-0.482726117000016));
#346580=CARTESIAN_POINT('Ctrl Pts',(3.96460858399994,12.2,-0.482731726000014));
#346581=CARTESIAN_POINT('Ctrl Pts',(3.96460858399994,5.2,-0.482731726000014));
#346582=CARTESIAN_POINT('Ctrl Pts',(3.96460858399994,2.2,-0.482731726000014));
#346583=CARTESIAN_POINT('Ctrl Pts',(3.96466595699994,12.2,-0.482738075000011));
#346584=CARTESIAN_POINT('Ctrl Pts',(3.96466595699994,5.2,-0.482738075000011));
#346585=CARTESIAN_POINT('Ctrl Pts',(3.96466595699994,2.2,-0.482738075000011));
#346586=CARTESIAN_POINT('Ctrl Pts',(3.96473064299994,12.2,-0.482745154000015));
#346587=CARTESIAN_POINT('Ctrl Pts',(3.96473064299994,5.2,-0.482745154000015));
#346588=CARTESIAN_POINT('Ctrl Pts',(3.96473064299994,2.2,-0.482745154000015));
#346589=CARTESIAN_POINT('Ctrl Pts',(3.96480263099994,12.2,-0.482752944000016));
#346590=CARTESIAN_POINT('Ctrl Pts',(3.96480263099994,5.2,-0.482752944000016));
#346591=CARTESIAN_POINT('Ctrl Pts',(3.96480263099994,2.2,-0.482752944000016));
#346592=CARTESIAN_POINT('Ctrl Pts',(3.96488190499994,12.2,-0.482761424000016));
#346593=CARTESIAN_POINT('Ctrl Pts',(3.96488190499994,5.2,-0.482761424000016));
#346594=CARTESIAN_POINT('Ctrl Pts',(3.96488190499994,2.2,-0.482761424000016));
#346595=CARTESIAN_POINT('Ctrl Pts',(3.96496844499994,12.2,-0.482770567000017));
#346596=CARTESIAN_POINT('Ctrl Pts',(3.96496844499994,5.2,-0.482770567000017));
#346597=CARTESIAN_POINT('Ctrl Pts',(3.96496844499994,2.2,-0.482770567000017));
#346598=CARTESIAN_POINT('Ctrl Pts',(3.96506223299994,12.2,-0.482780345000013));
#346599=CARTESIAN_POINT('Ctrl Pts',(3.96506223299994,5.2,-0.482780345000013));
#346600=CARTESIAN_POINT('Ctrl Pts',(3.96506223299994,2.2,-0.482780345000013));
#346601=CARTESIAN_POINT('Ctrl Pts',(3.96516325199994,12.2,-0.482790732000016));
#346602=CARTESIAN_POINT('Ctrl Pts',(3.96516325199994,5.2,-0.482790732000016));
#346603=CARTESIAN_POINT('Ctrl Pts',(3.96516325199994,2.2,-0.482790732000016));
#346604=CARTESIAN_POINT('Ctrl Pts',(3.96527148799994,12.2,-0.482801710000014));
#346605=CARTESIAN_POINT('Ctrl Pts',(3.96527148799994,5.2,-0.482801710000014));
#346606=CARTESIAN_POINT('Ctrl Pts',(3.96527148799994,2.2,-0.482801710000014));
#346607=CARTESIAN_POINT('Ctrl Pts',(3.96538692599994,12.2,-0.482813256000014));
#346608=CARTESIAN_POINT('Ctrl Pts',(3.96538692599994,5.2,-0.482813256000014));
#346609=CARTESIAN_POINT('Ctrl Pts',(3.96538692599994,2.2,-0.482813256000014));
#346610=CARTESIAN_POINT('Ctrl Pts',(3.96550955299994,12.2,-0.482825354000016));
#346611=CARTESIAN_POINT('Ctrl Pts',(3.96550955299994,5.2,-0.482825354000016));
#346612=CARTESIAN_POINT('Ctrl Pts',(3.96550955299994,2.2,-0.482825354000016));
#346613=CARTESIAN_POINT('Ctrl Pts',(3.96563935599994,12.2,-0.482837984000017));
#346614=CARTESIAN_POINT('Ctrl Pts',(3.96563935599994,5.2,-0.482837984000017));
#346615=CARTESIAN_POINT('Ctrl Pts',(3.96563935599994,2.2,-0.482837984000017));
#346616=CARTESIAN_POINT('Ctrl Pts',(3.96577632199994,12.2,-0.482851127000017));
#346617=CARTESIAN_POINT('Ctrl Pts',(3.96577632199994,5.2,-0.482851127000017));
#346618=CARTESIAN_POINT('Ctrl Pts',(3.96577632199994,2.2,-0.482851127000017));
#346619=CARTESIAN_POINT('Ctrl Pts',(3.96592043499994,12.2,-0.482864759000012));
#346620=CARTESIAN_POINT('Ctrl Pts',(3.96592043499994,5.2,-0.482864759000012));
#346621=CARTESIAN_POINT('Ctrl Pts',(3.96592043499994,2.2,-0.482864759000012));
#346622=CARTESIAN_POINT('Ctrl Pts',(3.96607167899994,12.2,-0.482878862000016));
#346623=CARTESIAN_POINT('Ctrl Pts',(3.96607167899994,5.2,-0.482878862000016));
#346624=CARTESIAN_POINT('Ctrl Pts',(3.96607167899994,2.2,-0.482878862000016));
#346625=CARTESIAN_POINT('Ctrl Pts',(3.96623003999994,12.2,-0.482893412000016));
#346626=CARTESIAN_POINT('Ctrl Pts',(3.96623003999994,5.2,-0.482893412000016));
#346627=CARTESIAN_POINT('Ctrl Pts',(3.96623003999994,2.2,-0.482893412000016));
#346628=CARTESIAN_POINT('Ctrl Pts',(3.96639550299994,12.2,-0.482908389000016));
#346629=CARTESIAN_POINT('Ctrl Pts',(3.96639550299994,5.2,-0.482908389000016));
#346630=CARTESIAN_POINT('Ctrl Pts',(3.96639550299994,2.2,-0.482908389000016));
#346631=CARTESIAN_POINT('Ctrl Pts',(3.96656805299994,12.2,-0.482923774000015));
#346632=CARTESIAN_POINT('Ctrl Pts',(3.96656805299994,5.2,-0.482923774000015));
#346633=CARTESIAN_POINT('Ctrl Pts',(3.96656805299994,2.2,-0.482923774000015));
#346634=CARTESIAN_POINT('Ctrl Pts',(3.96674767599994,12.2,-0.482939544000014));
#346635=CARTESIAN_POINT('Ctrl Pts',(3.96674767599994,5.2,-0.482939544000014));
#346636=CARTESIAN_POINT('Ctrl Pts',(3.96674767599994,2.2,-0.482939544000014));
#346637=CARTESIAN_POINT('Ctrl Pts',(3.96693435899994,12.2,-0.482955682000017));
#346638=CARTESIAN_POINT('Ctrl Pts',(3.96693435899994,5.2,-0.482955682000017));
#346639=CARTESIAN_POINT('Ctrl Pts',(3.96693435899994,2.2,-0.482955682000017));
#346640=CARTESIAN_POINT('Ctrl Pts',(3.96712808699994,12.2,-0.482972166000017));
#346641=CARTESIAN_POINT('Ctrl Pts',(3.96712808699994,5.2,-0.482972166000017));
#346642=CARTESIAN_POINT('Ctrl Pts',(3.96712808699994,2.2,-0.482972166000017));
#346643=CARTESIAN_POINT('Ctrl Pts',(3.96732884499994,12.2,-0.482988979000014));
#346644=CARTESIAN_POINT('Ctrl Pts',(3.96732884499994,5.2,-0.482988979000014));
#346645=CARTESIAN_POINT('Ctrl Pts',(3.96732884499994,2.2,-0.482988979000014));
#346646=CARTESIAN_POINT('Ctrl Pts',(3.96753661899994,12.2,-0.483006098000014));
#346647=CARTESIAN_POINT('Ctrl Pts',(3.96753661899994,5.2,-0.483006098000014));
#346648=CARTESIAN_POINT('Ctrl Pts',(3.96753661899994,2.2,-0.483006098000014));
#346649=CARTESIAN_POINT('Ctrl Pts',(3.96775139599994,12.2,-0.483023505000015));
#346650=CARTESIAN_POINT('Ctrl Pts',(3.96775139599994,5.2,-0.483023505000015));
#346651=CARTESIAN_POINT('Ctrl Pts',(3.96775139599994,2.2,-0.483023505000015));
#346652=CARTESIAN_POINT('Ctrl Pts',(3.96797315999994,12.2,-0.483041180000012));
#346653=CARTESIAN_POINT('Ctrl Pts',(3.96797315999994,5.2,-0.483041180000012));
#346654=CARTESIAN_POINT('Ctrl Pts',(3.96797315999994,2.2,-0.483041180000012));
#346655=CARTESIAN_POINT('Ctrl Pts',(3.96820189699994,12.2,-0.483059102000016));
#346656=CARTESIAN_POINT('Ctrl Pts',(3.96820189699994,5.2,-0.483059102000016));
#346657=CARTESIAN_POINT('Ctrl Pts',(3.96820189699994,2.2,-0.483059102000016));
#346658=CARTESIAN_POINT('Ctrl Pts',(3.96843759299994,12.2,-0.483077252000013));
#346659=CARTESIAN_POINT('Ctrl Pts',(3.96843759299994,5.2,-0.483077252000013));
#346660=CARTESIAN_POINT('Ctrl Pts',(3.96843759299994,2.2,-0.483077252000013));
#346661=CARTESIAN_POINT('Ctrl Pts',(3.96868023399994,12.2,-0.483095611000017));
#346662=CARTESIAN_POINT('Ctrl Pts',(3.96868023399994,5.2,-0.483095611000017));
#346663=CARTESIAN_POINT('Ctrl Pts',(3.96868023399994,2.2,-0.483095611000017));
#346664=CARTESIAN_POINT('Ctrl Pts',(3.96892980499994,12.2,-0.483114161000016));
#346665=CARTESIAN_POINT('Ctrl Pts',(3.96892980499994,5.2,-0.483114161000016));
#346666=CARTESIAN_POINT('Ctrl Pts',(3.96892980499994,2.2,-0.483114161000016));
#346667=CARTESIAN_POINT('Ctrl Pts',(3.96918629399994,12.2,-0.483132879000014));
#346668=CARTESIAN_POINT('Ctrl Pts',(3.96918629399994,5.2,-0.483132879000014));
#346669=CARTESIAN_POINT('Ctrl Pts',(3.96918629399994,2.2,-0.483132879000014));
#346670=CARTESIAN_POINT('Ctrl Pts',(3.96944968499994,12.2,-0.483151750000013));
#346671=CARTESIAN_POINT('Ctrl Pts',(3.96944968499994,5.2,-0.483151750000013));
#346672=CARTESIAN_POINT('Ctrl Pts',(3.96944968499994,2.2,-0.483151750000013));
#346673=CARTESIAN_POINT('Ctrl Pts',(3.96971996399994,12.2,-0.483170752000017));
#346674=CARTESIAN_POINT('Ctrl Pts',(3.96971996399994,5.2,-0.483170752000017));
#346675=CARTESIAN_POINT('Ctrl Pts',(3.96971996399994,2.2,-0.483170752000017));
#346676=CARTESIAN_POINT('Ctrl Pts',(3.96999711799995,12.2,-0.483189867000018));
#346677=CARTESIAN_POINT('Ctrl Pts',(3.96999711799995,5.2,-0.483189867000018));
#346678=CARTESIAN_POINT('Ctrl Pts',(3.96999711799995,2.2,-0.483189867000018));
#346679=CARTESIAN_POINT('Ctrl Pts',(3.97028113299994,12.2,-0.483209075000013));
#346680=CARTESIAN_POINT('Ctrl Pts',(3.97028113299994,5.2,-0.483209075000013));
#346681=CARTESIAN_POINT('Ctrl Pts',(3.97028113299994,2.2,-0.483209075000013));
#346682=CARTESIAN_POINT('Ctrl Pts',(3.97057199299994,12.2,-0.483228358000014));
#346683=CARTESIAN_POINT('Ctrl Pts',(3.97057199299994,5.2,-0.483228358000014));
#346684=CARTESIAN_POINT('Ctrl Pts',(3.97057199299994,2.2,-0.483228358000014));
#346685=CARTESIAN_POINT('Ctrl Pts',(3.97086968699994,12.2,-0.483247698000016));
#346686=CARTESIAN_POINT('Ctrl Pts',(3.97086968699994,5.2,-0.483247698000016));
#346687=CARTESIAN_POINT('Ctrl Pts',(3.97086968699994,2.2,-0.483247698000016));
#346688=CARTESIAN_POINT('Ctrl Pts',(3.97117419799994,12.2,-0.483267075000011));
#346689=CARTESIAN_POINT('Ctrl Pts',(3.97117419799994,5.2,-0.483267075000011));
#346690=CARTESIAN_POINT('Ctrl Pts',(3.97117419799994,2.2,-0.483267075000011));
#346691=CARTESIAN_POINT('Ctrl Pts',(3.97148551499994,12.2,-0.483286471000017));
#346692=CARTESIAN_POINT('Ctrl Pts',(3.97148551499994,5.2,-0.483286471000017));
#346693=CARTESIAN_POINT('Ctrl Pts',(3.97148551499994,2.2,-0.483286471000017));
#346694=CARTESIAN_POINT('Ctrl Pts',(3.97180362299994,12.2,-0.483305866000014));
#346695=CARTESIAN_POINT('Ctrl Pts',(3.97180362299994,5.2,-0.483305866000014));
#346696=CARTESIAN_POINT('Ctrl Pts',(3.97180362299994,2.2,-0.483305866000014));
#346697=CARTESIAN_POINT('Ctrl Pts',(3.97212850699994,12.2,-0.483325243000015));
#346698=CARTESIAN_POINT('Ctrl Pts',(3.97212850699994,5.2,-0.483325243000015));
#346699=CARTESIAN_POINT('Ctrl Pts',(3.97212850699994,2.2,-0.483325243000015));
#346700=CARTESIAN_POINT('Ctrl Pts',(3.97246015499995,12.2,-0.483344584000012));
#346701=CARTESIAN_POINT('Ctrl Pts',(3.97246015499995,5.2,-0.483344584000012));
#346702=CARTESIAN_POINT('Ctrl Pts',(3.97246015499995,2.2,-0.483344584000012));
#346703=CARTESIAN_POINT('Ctrl Pts',(3.97279855099994,12.2,-0.483363869000013));
#346704=CARTESIAN_POINT('Ctrl Pts',(3.97279855099994,5.2,-0.483363869000013));
#346705=CARTESIAN_POINT('Ctrl Pts',(3.97279855099994,2.2,-0.483363869000013));
#346706=CARTESIAN_POINT('Ctrl Pts',(3.97314368299994,12.2,-0.483383081000017));
#346707=CARTESIAN_POINT('Ctrl Pts',(3.97314368299994,5.2,-0.483383081000017));
#346708=CARTESIAN_POINT('Ctrl Pts',(3.97314368299994,2.2,-0.483383081000017));
#346709=CARTESIAN_POINT('Ctrl Pts',(3.97349553699994,12.2,-0.483402201000014));
#346710=CARTESIAN_POINT('Ctrl Pts',(3.97349553699994,5.2,-0.483402201000014));
#346711=CARTESIAN_POINT('Ctrl Pts',(3.97349553699994,2.2,-0.483402201000014));
#346712=CARTESIAN_POINT('Ctrl Pts',(3.97385409999994,12.2,-0.483421212000015));
#346713=CARTESIAN_POINT('Ctrl Pts',(3.97385409999994,5.2,-0.483421212000015));
#346714=CARTESIAN_POINT('Ctrl Pts',(3.97385409999994,2.2,-0.483421212000015));
#346715=CARTESIAN_POINT('Ctrl Pts',(3.97421935599994,12.2,-0.483440095000014));
#346716=CARTESIAN_POINT('Ctrl Pts',(3.97421935599994,5.2,-0.483440095000014));
#346717=CARTESIAN_POINT('Ctrl Pts',(3.97421935599994,2.2,-0.483440095000014));
#346718=CARTESIAN_POINT('Ctrl Pts',(3.97459129399994,12.2,-0.483458832000014));
#346719=CARTESIAN_POINT('Ctrl Pts',(3.97459129399994,5.2,-0.483458832000014));
#346720=CARTESIAN_POINT('Ctrl Pts',(3.97459129399994,2.2,-0.483458832000014));
#346721=CARTESIAN_POINT('Ctrl Pts',(3.97496989799994,12.2,-0.483477405000015));
#346722=CARTESIAN_POINT('Ctrl Pts',(3.97496989799994,5.2,-0.483477405000015));
#346723=CARTESIAN_POINT('Ctrl Pts',(3.97496989799994,2.2,-0.483477405000015));
#346724=CARTESIAN_POINT('Ctrl Pts',(3.97535515599994,12.2,-0.483495797000018));
#346725=CARTESIAN_POINT('Ctrl Pts',(3.97535515599994,5.2,-0.483495797000018));
#346726=CARTESIAN_POINT('Ctrl Pts',(3.97535515599994,2.2,-0.483495797000018));
#346727=CARTESIAN_POINT('Ctrl Pts',(3.97574705299994,12.2,-0.483513990000013));
#346728=CARTESIAN_POINT('Ctrl Pts',(3.97574705299994,5.2,-0.483513990000013));
#346729=CARTESIAN_POINT('Ctrl Pts',(3.97574705299994,2.2,-0.483513990000013));
#346730=CARTESIAN_POINT('Ctrl Pts',(3.97614557699994,12.2,-0.483531966000013));
#346731=CARTESIAN_POINT('Ctrl Pts',(3.97614557699994,5.2,-0.483531966000013));
#346732=CARTESIAN_POINT('Ctrl Pts',(3.97614557699994,2.2,-0.483531966000013));
#346733=CARTESIAN_POINT('Ctrl Pts',(3.97655071399994,12.2,-0.483549707000015));
#346734=CARTESIAN_POINT('Ctrl Pts',(3.97655071399994,5.2,-0.483549707000015));
#346735=CARTESIAN_POINT('Ctrl Pts',(3.97655071399994,2.2,-0.483549707000015));
#346736=CARTESIAN_POINT('Ctrl Pts',(3.97696244899994,12.2,-0.483567197000014));
#346737=CARTESIAN_POINT('Ctrl Pts',(3.97696244899994,5.2,-0.483567197000014));
#346738=CARTESIAN_POINT('Ctrl Pts',(3.97696244899994,2.2,-0.483567197000014));
#346739=CARTESIAN_POINT('Ctrl Pts',(3.97738077099994,12.2,-0.483584416000014));
#346740=CARTESIAN_POINT('Ctrl Pts',(3.97738077099994,5.2,-0.483584416000014));
#346741=CARTESIAN_POINT('Ctrl Pts',(3.97738077099994,2.2,-0.483584416000014));
#346742=CARTESIAN_POINT('Ctrl Pts',(3.97780566499994,12.2,-0.483601350000011));
#346743=CARTESIAN_POINT('Ctrl Pts',(3.97780566499994,5.2,-0.483601350000011));
#346744=CARTESIAN_POINT('Ctrl Pts',(3.97780566499994,2.2,-0.483601350000011));
#346745=CARTESIAN_POINT('Ctrl Pts',(3.97823711799994,12.2,-0.483617978000015));
#346746=CARTESIAN_POINT('Ctrl Pts',(3.97823711799994,5.2,-0.483617978000015));
#346747=CARTESIAN_POINT('Ctrl Pts',(3.97823711799994,2.2,-0.483617978000015));
#346748=CARTESIAN_POINT('Ctrl Pts',(3.97867511499994,12.2,-0.483634286000014));
#346749=CARTESIAN_POINT('Ctrl Pts',(3.97867511499994,5.2,-0.483634286000014));
#346750=CARTESIAN_POINT('Ctrl Pts',(3.97867511499994,2.2,-0.483634286000014));
#346751=CARTESIAN_POINT('Ctrl Pts',(3.97911964499994,12.2,-0.483650256000012));
#346752=CARTESIAN_POINT('Ctrl Pts',(3.97911964499994,5.2,-0.483650256000012));
#346753=CARTESIAN_POINT('Ctrl Pts',(3.97911964499994,2.2,-0.483650256000012));
#346754=CARTESIAN_POINT('Ctrl Pts',(3.97957069299994,12.2,-0.483665869000016));
#346755=CARTESIAN_POINT('Ctrl Pts',(3.97957069299994,5.2,-0.483665869000016));
#346756=CARTESIAN_POINT('Ctrl Pts',(3.97957069299994,2.2,-0.483665869000016));
#346757=CARTESIAN_POINT('Ctrl Pts',(3.98002824599994,12.2,-0.483681109000016));
#346758=CARTESIAN_POINT('Ctrl Pts',(3.98002824599994,5.2,-0.483681109000016));
#346759=CARTESIAN_POINT('Ctrl Pts',(3.98002824599994,2.2,-0.483681109000016));
#346760=CARTESIAN_POINT('Ctrl Pts',(3.98049229099994,12.2,-0.483695961000015));
#346761=CARTESIAN_POINT('Ctrl Pts',(3.98049229099994,5.2,-0.483695961000015));
#346762=CARTESIAN_POINT('Ctrl Pts',(3.98049229099994,2.2,-0.483695961000015));
#346763=CARTESIAN_POINT('Ctrl Pts',(3.98096281399994,12.2,-0.483710406000015));
#346764=CARTESIAN_POINT('Ctrl Pts',(3.98096281399994,5.2,-0.483710406000015));
#346765=CARTESIAN_POINT('Ctrl Pts',(3.98096281399994,2.2,-0.483710406000015));
#346766=CARTESIAN_POINT('Ctrl Pts',(3.98143980299994,12.2,-0.483724427000016));
#346767=CARTESIAN_POINT('Ctrl Pts',(3.98143980299994,5.2,-0.483724427000016));
#346768=CARTESIAN_POINT('Ctrl Pts',(3.98143980299994,2.2,-0.483724427000016));
#346769=CARTESIAN_POINT('Ctrl Pts',(3.98192324299994,12.2,-0.483738009000017));
#346770=CARTESIAN_POINT('Ctrl Pts',(3.98192324299994,5.2,-0.483738009000017));
#346771=CARTESIAN_POINT('Ctrl Pts',(3.98192324299994,2.2,-0.483738009000017));
#346772=CARTESIAN_POINT('Ctrl Pts',(3.98241312199994,12.2,-0.483751134000014));
#346773=CARTESIAN_POINT('Ctrl Pts',(3.98241312199994,5.2,-0.483751134000014));
#346774=CARTESIAN_POINT('Ctrl Pts',(3.98241312199994,2.2,-0.483751134000014));
#346775=CARTESIAN_POINT('Ctrl Pts',(3.98290942699994,12.2,-0.483763784000013));
#346776=CARTESIAN_POINT('Ctrl Pts',(3.98290942699994,5.2,-0.483763784000013));
#346777=CARTESIAN_POINT('Ctrl Pts',(3.98290942699994,2.2,-0.483763784000013));
#346778=CARTESIAN_POINT('Ctrl Pts',(3.98341214399994,12.2,-0.483775947000016));
#346779=CARTESIAN_POINT('Ctrl Pts',(3.98341214399994,5.2,-0.483775947000016));
#346780=CARTESIAN_POINT('Ctrl Pts',(3.98341214399994,2.2,-0.483775947000016));
#346781=CARTESIAN_POINT('Ctrl Pts',(3.98392125999994,12.2,-0.483787602000016));
#346782=CARTESIAN_POINT('Ctrl Pts',(3.98392125999994,5.2,-0.483787602000016));
#346783=CARTESIAN_POINT('Ctrl Pts',(3.98392125999994,2.2,-0.483787602000016));
#346784=CARTESIAN_POINT('Ctrl Pts',(3.98443676199994,12.2,-0.483798734000014));
#346785=CARTESIAN_POINT('Ctrl Pts',(3.98443676199994,5.2,-0.483798734000014));
#346786=CARTESIAN_POINT('Ctrl Pts',(3.98443676199994,2.2,-0.483798734000014));
#346787=CARTESIAN_POINT('Ctrl Pts',(3.98495863699994,12.2,-0.483809327000015));
#346788=CARTESIAN_POINT('Ctrl Pts',(3.98495863699994,5.2,-0.483809327000015));
#346789=CARTESIAN_POINT('Ctrl Pts',(3.98495863699994,2.2,-0.483809327000015));
#346790=CARTESIAN_POINT('Ctrl Pts',(3.98548687099994,12.2,-0.483819364000015));
#346791=CARTESIAN_POINT('Ctrl Pts',(3.98548687099994,5.2,-0.483819364000015));
#346792=CARTESIAN_POINT('Ctrl Pts',(3.98548687099994,2.2,-0.483819364000015));
#346793=CARTESIAN_POINT('Ctrl Pts',(3.98602145199995,12.2,-0.483828830000017));
#346794=CARTESIAN_POINT('Ctrl Pts',(3.98602145199995,5.2,-0.483828830000017));
#346795=CARTESIAN_POINT('Ctrl Pts',(3.98602145199995,2.2,-0.483828830000017));
#346796=CARTESIAN_POINT('Ctrl Pts',(3.98656236599995,12.2,-0.483837709000015));
#346797=CARTESIAN_POINT('Ctrl Pts',(3.98656236599995,5.2,-0.483837709000015));
#346798=CARTESIAN_POINT('Ctrl Pts',(3.98656236599995,2.2,-0.483837709000015));
#346799=CARTESIAN_POINT('Ctrl Pts',(3.98710959999994,12.2,-0.483845983000015));
#346800=CARTESIAN_POINT('Ctrl Pts',(3.98710959999994,5.2,-0.483845983000015));
#346801=CARTESIAN_POINT('Ctrl Pts',(3.98710959999994,2.2,-0.483845983000015));
#346802=CARTESIAN_POINT('Ctrl Pts',(3.98766314199994,12.2,-0.483853638000014));
#346803=CARTESIAN_POINT('Ctrl Pts',(3.98766314199994,5.2,-0.483853638000014));
#346804=CARTESIAN_POINT('Ctrl Pts',(3.98766314199994,2.2,-0.483853638000014));
#346805=CARTESIAN_POINT('Ctrl Pts',(3.98822297899994,12.2,-0.483860657000013));
#346806=CARTESIAN_POINT('Ctrl Pts',(3.98822297899994,5.2,-0.483860657000013));
#346807=CARTESIAN_POINT('Ctrl Pts',(3.98822297899994,2.2,-0.483860657000013));
#346808=CARTESIAN_POINT('Ctrl Pts',(3.98878909599994,12.2,-0.483867023000015));
#346809=CARTESIAN_POINT('Ctrl Pts',(3.98878909599994,5.2,-0.483867023000015));
#346810=CARTESIAN_POINT('Ctrl Pts',(3.98878909599994,2.2,-0.483867023000015));
#346811=CARTESIAN_POINT('Ctrl Pts',(3.98936148199994,12.2,-0.483872724000012));
#346812=CARTESIAN_POINT('Ctrl Pts',(3.98936148199994,5.2,-0.483872724000012));
#346813=CARTESIAN_POINT('Ctrl Pts',(3.98936148199994,2.2,-0.483872724000012));
#346814=CARTESIAN_POINT('Ctrl Pts',(3.98994012399994,12.2,-0.483877739000014));
#346815=CARTESIAN_POINT('Ctrl Pts',(3.98994012399994,5.2,-0.483877739000014));
#346816=CARTESIAN_POINT('Ctrl Pts',(3.98994012399994,2.2,-0.483877739000014));
#346817=CARTESIAN_POINT('Ctrl Pts',(3.99052500699994,12.2,-0.483882056000016));
#346818=CARTESIAN_POINT('Ctrl Pts',(3.99052500699994,5.2,-0.483882056000016));
#346819=CARTESIAN_POINT('Ctrl Pts',(3.99052500699994,2.2,-0.483882056000016));
#346820=CARTESIAN_POINT('Ctrl Pts',(3.99111612099994,12.2,-0.483885659000016));
#346821=CARTESIAN_POINT('Ctrl Pts',(3.99111612099994,5.2,-0.483885659000016));
#346822=CARTESIAN_POINT('Ctrl Pts',(3.99111612099994,2.2,-0.483885659000016));
#346823=CARTESIAN_POINT('Ctrl Pts',(3.99171345099994,12.2,-0.483888531000014));
#346824=CARTESIAN_POINT('Ctrl Pts',(3.99171345099994,5.2,-0.483888531000014));
#346825=CARTESIAN_POINT('Ctrl Pts',(3.99171345099994,2.2,-0.483888531000014));
#346826=CARTESIAN_POINT('Ctrl Pts',(3.99231698499994,12.2,-0.483890657000017));
#346827=CARTESIAN_POINT('Ctrl Pts',(3.99231698499994,5.2,-0.483890657000017));
#346828=CARTESIAN_POINT('Ctrl Pts',(3.99231698499994,2.2,-0.483890657000017));
#346829=CARTESIAN_POINT('Ctrl Pts',(3.99292670999994,12.2,-0.483892023000014));
#346830=CARTESIAN_POINT('Ctrl Pts',(3.99292670999994,5.2,-0.483892023000014));
#346831=CARTESIAN_POINT('Ctrl Pts',(3.99292670999994,2.2,-0.483892023000014));
#346832=CARTESIAN_POINT('Ctrl Pts',(3.99354261299994,12.2,-0.483892612000014));
#346833=CARTESIAN_POINT('Ctrl Pts',(3.99354261299994,5.2,-0.483892612000014));
#346834=CARTESIAN_POINT('Ctrl Pts',(3.99354261299994,2.2,-0.483892612000014));
#346835=CARTESIAN_POINT('Ctrl Pts',(3.99416468199994,12.2,-0.483892409000015));
#346836=CARTESIAN_POINT('Ctrl Pts',(3.99416468199994,5.2,-0.483892409000015));
#346837=CARTESIAN_POINT('Ctrl Pts',(3.99416468199994,2.2,-0.483892409000015));
#346838=CARTESIAN_POINT('Ctrl Pts',(3.99479290299994,12.2,-0.483891397000011));
#346839=CARTESIAN_POINT('Ctrl Pts',(3.99479290299994,5.2,-0.483891397000011));
#346840=CARTESIAN_POINT('Ctrl Pts',(3.99479290299994,2.2,-0.483891397000011));
#346841=CARTESIAN_POINT('Ctrl Pts',(3.99542726299994,12.2,-0.483889565000015));
#346842=CARTESIAN_POINT('Ctrl Pts',(3.99542726299994,5.2,-0.483889565000015));
#346843=CARTESIAN_POINT('Ctrl Pts',(3.99542726299994,2.2,-0.483889565000015));
#346844=CARTESIAN_POINT('Ctrl Pts',(3.99606775099994,12.2,-0.483886895000012));
#346845=CARTESIAN_POINT('Ctrl Pts',(3.99606775099994,5.2,-0.483886895000012));
#346846=CARTESIAN_POINT('Ctrl Pts',(3.99606775099994,2.2,-0.483886895000012));
#346847=CARTESIAN_POINT('Ctrl Pts',(3.99671435299994,12.2,-0.483883372000014));
#346848=CARTESIAN_POINT('Ctrl Pts',(3.99671435299994,5.2,-0.483883372000014));
#346849=CARTESIAN_POINT('Ctrl Pts',(3.99671435299994,2.2,-0.483883372000014));
#346850=CARTESIAN_POINT('Ctrl Pts',(3.99736705599994,12.2,-0.483878981000014));
#346851=CARTESIAN_POINT('Ctrl Pts',(3.99736705599994,5.2,-0.483878981000014));
#346852=CARTESIAN_POINT('Ctrl Pts',(3.99736705599994,2.2,-0.483878981000014));
#346853=CARTESIAN_POINT('Ctrl Pts',(3.99802584899994,12.2,-0.483873708000013));
#346854=CARTESIAN_POINT('Ctrl Pts',(3.99802584899994,5.2,-0.483873708000013));
#346855=CARTESIAN_POINT('Ctrl Pts',(3.99802584899994,2.2,-0.483873708000013));
#346856=CARTESIAN_POINT('Ctrl Pts',(3.99869071799994,12.2,-0.483867537000013));
#346857=CARTESIAN_POINT('Ctrl Pts',(3.99869071799994,5.2,-0.483867537000013));
#346858=CARTESIAN_POINT('Ctrl Pts',(3.99869071799994,2.2,-0.483867537000013));
#346859=CARTESIAN_POINT('Ctrl Pts',(3.99936164999994,12.2,-0.483860454000014));
#346860=CARTESIAN_POINT('Ctrl Pts',(3.99936164999994,5.2,-0.483860454000014));
#346861=CARTESIAN_POINT('Ctrl Pts',(3.99936164999994,2.2,-0.483860454000014));
#346862=CARTESIAN_POINT('Ctrl Pts',(4.00003863299994,12.2,-0.483852443000017));
#346863=CARTESIAN_POINT('Ctrl Pts',(4.00003863299994,5.2,-0.483852443000017));
#346864=CARTESIAN_POINT('Ctrl Pts',(4.00003863299994,2.2,-0.483852443000017));
#346865=CARTESIAN_POINT('Ctrl Pts',(4.00072165499994,12.2,-0.483843491000013));
#346866=CARTESIAN_POINT('Ctrl Pts',(4.00072165499994,5.2,-0.483843491000013));
#346867=CARTESIAN_POINT('Ctrl Pts',(4.00072165499994,2.2,-0.483843491000013));
#346868=CARTESIAN_POINT('Ctrl Pts',(4.00141070199994,12.2,-0.483833582000015));
#346869=CARTESIAN_POINT('Ctrl Pts',(4.00141070199994,5.2,-0.483833582000015));
#346870=CARTESIAN_POINT('Ctrl Pts',(4.00141070199994,2.2,-0.483833582000015));
#346871=CARTESIAN_POINT('Ctrl Pts',(4.00210576199994,12.2,-0.483822701000012));
#346872=CARTESIAN_POINT('Ctrl Pts',(4.00210576199994,5.2,-0.483822701000012));
#346873=CARTESIAN_POINT('Ctrl Pts',(4.00210576199994,2.2,-0.483822701000012));
#346874=CARTESIAN_POINT('Ctrl Pts',(4.00280682299995,12.2,-0.483810836000016));
#346875=CARTESIAN_POINT('Ctrl Pts',(4.00280682299995,5.2,-0.483810836000016));
#346876=CARTESIAN_POINT('Ctrl Pts',(4.00280682299995,2.2,-0.483810836000016));
#346877=CARTESIAN_POINT('Ctrl Pts',(4.00351387199995,12.2,-0.483797969000013));
#346878=CARTESIAN_POINT('Ctrl Pts',(4.00351387199995,5.2,-0.483797969000013));
#346879=CARTESIAN_POINT('Ctrl Pts',(4.00351387199995,2.2,-0.483797969000013));
#346880=CARTESIAN_POINT('Ctrl Pts',(4.00422689599994,12.2,-0.483784088000014));
#346881=CARTESIAN_POINT('Ctrl Pts',(4.00422689599994,5.2,-0.483784088000014));
#346882=CARTESIAN_POINT('Ctrl Pts',(4.00422689599994,2.2,-0.483784088000014));
#346883=CARTESIAN_POINT('Ctrl Pts',(4.00494588399994,12.2,-0.483769178000015));
#346884=CARTESIAN_POINT('Ctrl Pts',(4.00494588399994,5.2,-0.483769178000015));
#346885=CARTESIAN_POINT('Ctrl Pts',(4.00494588399994,2.2,-0.483769178000015));
#346886=CARTESIAN_POINT('Ctrl Pts',(4.00567082099994,12.2,-0.483753224000014));
#346887=CARTESIAN_POINT('Ctrl Pts',(4.00567082099994,5.2,-0.483753224000014));
#346888=CARTESIAN_POINT('Ctrl Pts',(4.00567082099994,2.2,-0.483753224000014));
#346889=CARTESIAN_POINT('Ctrl Pts',(4.00640169699995,12.2,-0.483736213000014));
#346890=CARTESIAN_POINT('Ctrl Pts',(4.00640169699995,5.2,-0.483736213000014));
#346891=CARTESIAN_POINT('Ctrl Pts',(4.00640169699995,2.2,-0.483736213000014));
#346892=CARTESIAN_POINT('Ctrl Pts',(4.00713849899994,12.2,-0.483718129000015));
#346893=CARTESIAN_POINT('Ctrl Pts',(4.00713849899994,5.2,-0.483718129000015));
#346894=CARTESIAN_POINT('Ctrl Pts',(4.00713849899994,2.2,-0.483718129000015));
#346895=CARTESIAN_POINT('Ctrl Pts',(4.00788121299995,12.2,-0.483698960000014));
#346896=CARTESIAN_POINT('Ctrl Pts',(4.00788121299995,5.2,-0.483698960000014));
#346897=CARTESIAN_POINT('Ctrl Pts',(4.00788121299995,2.2,-0.483698960000014));
#346898=CARTESIAN_POINT('Ctrl Pts',(4.00862982799994,12.2,-0.483678690000016));
#346899=CARTESIAN_POINT('Ctrl Pts',(4.00862982799994,5.2,-0.483678690000016));
#346900=CARTESIAN_POINT('Ctrl Pts',(4.00862982799994,2.2,-0.483678690000016));
#346901=CARTESIAN_POINT('Ctrl Pts',(4.00938433099994,12.2,-0.483657306000014));
#346902=CARTESIAN_POINT('Ctrl Pts',(4.00938433099994,5.2,-0.483657306000014));
#346903=CARTESIAN_POINT('Ctrl Pts',(4.00938433099994,2.2,-0.483657306000014));
#346904=CARTESIAN_POINT('Ctrl Pts',(4.01014471099994,12.2,-0.483634794000012));
#346905=CARTESIAN_POINT('Ctrl Pts',(4.01014471099994,5.2,-0.483634794000012));
#346906=CARTESIAN_POINT('Ctrl Pts',(4.01014471099994,2.2,-0.483634794000012));
#346907=CARTESIAN_POINT('Ctrl Pts',(4.01091095499994,12.2,-0.483611138000013));
#346908=CARTESIAN_POINT('Ctrl Pts',(4.01091095499994,5.2,-0.483611138000013));
#346909=CARTESIAN_POINT('Ctrl Pts',(4.01091095499994,2.2,-0.483611138000013));
#346910=CARTESIAN_POINT('Ctrl Pts',(4.01168304899994,12.2,-0.483586328000012));
#346911=CARTESIAN_POINT('Ctrl Pts',(4.01168304899994,5.2,-0.483586328000012));
#346912=CARTESIAN_POINT('Ctrl Pts',(4.01168304899994,2.2,-0.483586328000012));
#346913=CARTESIAN_POINT('Ctrl Pts',(4.01246098199994,12.2,-0.483560347000012));
#346914=CARTESIAN_POINT('Ctrl Pts',(4.01246098199994,5.2,-0.483560347000012));
#346915=CARTESIAN_POINT('Ctrl Pts',(4.01246098199994,2.2,-0.483560347000012));
#346916=CARTESIAN_POINT('Ctrl Pts',(4.01324474199994,12.2,-0.483533182000015));
#346917=CARTESIAN_POINT('Ctrl Pts',(4.01324474199994,5.2,-0.483533182000015));
#346918=CARTESIAN_POINT('Ctrl Pts',(4.01324474199994,2.2,-0.483533182000015));
#346919=CARTESIAN_POINT('Ctrl Pts',(4.01403431599994,12.2,-0.483504820000018));
#346920=CARTESIAN_POINT('Ctrl Pts',(4.01403431599994,5.2,-0.483504820000018));
#346921=CARTESIAN_POINT('Ctrl Pts',(4.01403431599994,2.2,-0.483504820000018));
#346922=CARTESIAN_POINT('Ctrl Pts',(4.01482969199995,12.2,-0.483475246000014));
#346923=CARTESIAN_POINT('Ctrl Pts',(4.01482969199995,5.2,-0.483475246000014));
#346924=CARTESIAN_POINT('Ctrl Pts',(4.01482969199995,2.2,-0.483475246000014));
#346925=CARTESIAN_POINT('Ctrl Pts',(4.01563085799994,12.2,-0.483444448000014));
#346926=CARTESIAN_POINT('Ctrl Pts',(4.01563085799994,5.2,-0.483444448000014));
#346927=CARTESIAN_POINT('Ctrl Pts',(4.01563085799994,2.2,-0.483444448000014));
#346928=CARTESIAN_POINT('Ctrl Pts',(4.01643780099994,12.2,-0.483412411000015));
#346929=CARTESIAN_POINT('Ctrl Pts',(4.01643780099994,5.2,-0.483412411000015));
#346930=CARTESIAN_POINT('Ctrl Pts',(4.01643780099994,2.2,-0.483412411000015));
#346931=CARTESIAN_POINT('Ctrl Pts',(4.01725050999994,12.2,-0.483379121000014));
#346932=CARTESIAN_POINT('Ctrl Pts',(4.01725050999994,5.2,-0.483379121000014));
#346933=CARTESIAN_POINT('Ctrl Pts',(4.01725050999994,2.2,-0.483379121000014));
#346934=CARTESIAN_POINT('Ctrl Pts',(4.01806897099994,12.2,-0.483344567000015));
#346935=CARTESIAN_POINT('Ctrl Pts',(4.01806897099994,5.2,-0.483344567000015));
#346936=CARTESIAN_POINT('Ctrl Pts',(4.01806897099994,2.2,-0.483344567000015));
#346937=CARTESIAN_POINT('Ctrl Pts',(4.01889317399994,12.2,-0.483308734000012));
#346938=CARTESIAN_POINT('Ctrl Pts',(4.01889317399994,5.2,-0.483308734000012));
#346939=CARTESIAN_POINT('Ctrl Pts',(4.01889317399994,2.2,-0.483308734000012));
#346940=CARTESIAN_POINT('Ctrl Pts',(4.01972310599994,12.2,-0.483271609000013));
#346941=CARTESIAN_POINT('Ctrl Pts',(4.01972310599994,5.2,-0.483271609000013));
#346942=CARTESIAN_POINT('Ctrl Pts',(4.01972310599994,2.2,-0.483271609000013));
#346943=CARTESIAN_POINT('Ctrl Pts',(4.02055875299994,12.2,-0.483233178000013));
#346944=CARTESIAN_POINT('Ctrl Pts',(4.02055875299994,5.2,-0.483233178000013));
#346945=CARTESIAN_POINT('Ctrl Pts',(4.02055875299994,2.2,-0.483233178000013));
#346946=CARTESIAN_POINT('Ctrl Pts',(4.02140010499994,12.2,-0.483193427000015));
#346947=CARTESIAN_POINT('Ctrl Pts',(4.02140010499994,5.2,-0.483193427000015));
#346948=CARTESIAN_POINT('Ctrl Pts',(4.02140010499994,2.2,-0.483193427000015));
#346949=CARTESIAN_POINT('Ctrl Pts',(4.02224714999995,12.2,-0.483152346000013));
#346950=CARTESIAN_POINT('Ctrl Pts',(4.02224714999995,5.2,-0.483152346000013));
#346951=CARTESIAN_POINT('Ctrl Pts',(4.02224714999995,2.2,-0.483152346000013));
#346952=CARTESIAN_POINT('Ctrl Pts',(4.02309987399994,12.2,-0.483109919000011));
#346953=CARTESIAN_POINT('Ctrl Pts',(4.02309987399994,5.2,-0.483109919000011));
#346954=CARTESIAN_POINT('Ctrl Pts',(4.02309987399994,2.2,-0.483109919000011));
#346955=CARTESIAN_POINT('Ctrl Pts',(4.02395826699994,12.2,-0.483066133000012));
#346956=CARTESIAN_POINT('Ctrl Pts',(4.02395826699994,5.2,-0.483066133000012));
#346957=CARTESIAN_POINT('Ctrl Pts',(4.02395826699994,2.2,-0.483066133000012));
#346958=CARTESIAN_POINT('Ctrl Pts',(4.02482231599994,12.2,-0.483020976000015));
#346959=CARTESIAN_POINT('Ctrl Pts',(4.02482231599994,5.2,-0.483020976000015));
#346960=CARTESIAN_POINT('Ctrl Pts',(4.02482231599994,2.2,-0.483020976000015));
#346961=CARTESIAN_POINT('Ctrl Pts',(4.02569200799994,12.2,-0.482974435000014));
#346962=CARTESIAN_POINT('Ctrl Pts',(4.02569200799994,5.2,-0.482974435000014));
#346963=CARTESIAN_POINT('Ctrl Pts',(4.02569200799994,2.2,-0.482974435000014));
#346964=CARTESIAN_POINT('Ctrl Pts',(4.02656733299994,12.2,-0.482926497000014));
#346965=CARTESIAN_POINT('Ctrl Pts',(4.02656733299994,5.2,-0.482926497000014));
#346966=CARTESIAN_POINT('Ctrl Pts',(4.02656733299994,2.2,-0.482926497000014));
#346967=CARTESIAN_POINT('Ctrl Pts',(4.02744827799994,12.2,-0.482877148000016));
#346968=CARTESIAN_POINT('Ctrl Pts',(4.02744827799994,5.2,-0.482877148000016));
#346969=CARTESIAN_POINT('Ctrl Pts',(4.02744827799994,2.2,-0.482877148000016));
#346970=CARTESIAN_POINT('Ctrl Pts',(4.02833482899995,12.2,-0.482826375000016));
#346971=CARTESIAN_POINT('Ctrl Pts',(4.02833482899995,5.2,-0.482826375000016));
#346972=CARTESIAN_POINT('Ctrl Pts',(4.02833482899995,2.2,-0.482826375000016));
#346973=CARTESIAN_POINT('Ctrl Pts',(4.02922697699994,12.2,-0.482774167000013));
#346974=CARTESIAN_POINT('Ctrl Pts',(4.02922697699994,5.2,-0.482774167000013));
#346975=CARTESIAN_POINT('Ctrl Pts',(4.02922697699994,2.2,-0.482774167000013));
#346976=CARTESIAN_POINT('Ctrl Pts',(4.03012470899994,12.2,-0.482720510000014));
#346977=CARTESIAN_POINT('Ctrl Pts',(4.03012470899994,5.2,-0.482720510000014));
#346978=CARTESIAN_POINT('Ctrl Pts',(4.03012470899994,2.2,-0.482720510000014));
#346979=CARTESIAN_POINT('Ctrl Pts',(4.03102801199995,12.2,-0.482665392000015));
#346980=CARTESIAN_POINT('Ctrl Pts',(4.03102801199995,5.2,-0.482665392000015));
#346981=CARTESIAN_POINT('Ctrl Pts',(4.03102801199995,2.2,-0.482665392000015));
#346982=CARTESIAN_POINT('Ctrl Pts',(4.03193687599994,12.2,-0.482608799000013));
#346983=CARTESIAN_POINT('Ctrl Pts',(4.03193687599994,5.2,-0.482608799000013));
#346984=CARTESIAN_POINT('Ctrl Pts',(4.03193687599994,2.2,-0.482608799000013));
#346985=CARTESIAN_POINT('Ctrl Pts',(4.03285128799994,12.2,-0.482550720000017));
#346986=CARTESIAN_POINT('Ctrl Pts',(4.03285128799994,5.2,-0.482550720000017));
#346987=CARTESIAN_POINT('Ctrl Pts',(4.03285128799994,2.2,-0.482550720000017));
#346988=CARTESIAN_POINT('Ctrl Pts',(4.03377123599994,12.2,-0.482491142000012));
#346989=CARTESIAN_POINT('Ctrl Pts',(4.03377123599994,5.2,-0.482491142000012));
#346990=CARTESIAN_POINT('Ctrl Pts',(4.03377123599994,2.2,-0.482491142000012));
#346991=CARTESIAN_POINT('Ctrl Pts',(4.03469670699994,12.2,-0.482430050000016));
#346992=CARTESIAN_POINT('Ctrl Pts',(4.03469670699994,5.2,-0.482430050000016));
#346993=CARTESIAN_POINT('Ctrl Pts',(4.03469670699994,2.2,-0.482430050000016));
#346994=CARTESIAN_POINT('Ctrl Pts',(4.03562769099994,12.2,-0.482367436000013));
#346995=CARTESIAN_POINT('Ctrl Pts',(4.03562769099994,5.2,-0.482367436000013));
#346996=CARTESIAN_POINT('Ctrl Pts',(4.03562769099994,2.2,-0.482367436000013));
#346997=CARTESIAN_POINT('Ctrl Pts',(4.03656417599994,12.2,-0.482303284000012));
#346998=CARTESIAN_POINT('Ctrl Pts',(4.03656417599994,5.2,-0.482303284000012));
#346999=CARTESIAN_POINT('Ctrl Pts',(4.03656417599994,2.2,-0.482303284000012));
#347000=CARTESIAN_POINT('Ctrl Pts',(4.03750614799994,12.2,-0.482237583000016));
#347001=CARTESIAN_POINT('Ctrl Pts',(4.03750614799994,5.2,-0.482237583000016));
#347002=CARTESIAN_POINT('Ctrl Pts',(4.03750614799994,2.2,-0.482237583000016));
#347003=CARTESIAN_POINT('Ctrl Pts',(4.03845359799995,12.2,-0.482170321000015));
#347004=CARTESIAN_POINT('Ctrl Pts',(4.03845359799995,5.2,-0.482170321000015));
#347005=CARTESIAN_POINT('Ctrl Pts',(4.03845359799995,2.2,-0.482170321000015));
#347006=CARTESIAN_POINT('Ctrl Pts',(4.03940651299994,12.2,-0.482101484000013));
#347007=CARTESIAN_POINT('Ctrl Pts',(4.03940651299994,5.2,-0.482101484000013));
#347008=CARTESIAN_POINT('Ctrl Pts',(4.03940651299994,2.2,-0.482101484000013));
#347009=CARTESIAN_POINT('Ctrl Pts',(4.04036487999995,12.2,-0.482031062000012));
#347010=CARTESIAN_POINT('Ctrl Pts',(4.04036487999995,5.2,-0.482031062000012));
#347011=CARTESIAN_POINT('Ctrl Pts',(4.04036487999995,2.2,-0.482031062000012));
#347012=CARTESIAN_POINT('Ctrl Pts',(4.04132868899994,12.2,-0.481959041000017));
#347013=CARTESIAN_POINT('Ctrl Pts',(4.04132868899994,5.2,-0.481959041000017));
#347014=CARTESIAN_POINT('Ctrl Pts',(4.04132868899994,2.2,-0.481959041000017));
#347015=CARTESIAN_POINT('Ctrl Pts',(4.04229792699994,12.2,-0.481885410000018));
#347016=CARTESIAN_POINT('Ctrl Pts',(4.04229792699994,5.2,-0.481885410000018));
#347017=CARTESIAN_POINT('Ctrl Pts',(4.04229792699994,2.2,-0.481885410000018));
#347018=CARTESIAN_POINT('Ctrl Pts',(4.04327258299995,12.2,-0.481810156000013));
#347019=CARTESIAN_POINT('Ctrl Pts',(4.04327258299995,5.2,-0.481810156000013));
#347020=CARTESIAN_POINT('Ctrl Pts',(4.04327258299995,2.2,-0.481810156000013));
#347021=CARTESIAN_POINT('Ctrl Pts',(4.04425264399995,12.2,-0.481733268000015));
#347022=CARTESIAN_POINT('Ctrl Pts',(4.04425264399995,5.2,-0.481733268000015));
#347023=CARTESIAN_POINT('Ctrl Pts',(4.04425264399995,2.2,-0.481733268000015));
#347024=CARTESIAN_POINT('Ctrl Pts',(4.04523810099994,12.2,-0.481654733000014));
#347025=CARTESIAN_POINT('Ctrl Pts',(4.04523810099994,5.2,-0.481654733000014));
#347026=CARTESIAN_POINT('Ctrl Pts',(4.04523810099994,2.2,-0.481654733000014));
#347027=CARTESIAN_POINT('Ctrl Pts',(4.04622893899994,12.2,-0.481574540000014));
#347028=CARTESIAN_POINT('Ctrl Pts',(4.04622893899994,5.2,-0.481574540000014));
#347029=CARTESIAN_POINT('Ctrl Pts',(4.04622893899994,2.2,-0.481574540000014));
#347030=CARTESIAN_POINT('Ctrl Pts',(4.04722514799994,12.2,-0.481492676000013));
#347031=CARTESIAN_POINT('Ctrl Pts',(4.04722514799994,5.2,-0.481492676000013));
#347032=CARTESIAN_POINT('Ctrl Pts',(4.04722514799994,2.2,-0.481492676000013));
#347033=CARTESIAN_POINT('Ctrl Pts',(4.04822671599994,12.2,-0.481409130000015));
#347034=CARTESIAN_POINT('Ctrl Pts',(4.04822671599994,5.2,-0.481409130000015));
#347035=CARTESIAN_POINT('Ctrl Pts',(4.04822671599994,2.2,-0.481409130000015));
#347036=CARTESIAN_POINT('Ctrl Pts',(4.04923363199994,12.2,-0.481323889000014));
#347037=CARTESIAN_POINT('Ctrl Pts',(4.04923363199994,5.2,-0.481323889000014));
#347038=CARTESIAN_POINT('Ctrl Pts',(4.04923363199994,2.2,-0.481323889000014));
#347039=CARTESIAN_POINT('Ctrl Pts',(4.05024588299994,12.2,-0.481236942000014));
#347040=CARTESIAN_POINT('Ctrl Pts',(4.05024588299994,5.2,-0.481236942000014));
#347041=CARTESIAN_POINT('Ctrl Pts',(4.05024588299994,2.2,-0.481236942000014));
#347042=CARTESIAN_POINT('Ctrl Pts',(4.05126345799994,12.2,-0.481148277000014));
#347043=CARTESIAN_POINT('Ctrl Pts',(4.05126345799994,5.2,-0.481148277000014));
#347044=CARTESIAN_POINT('Ctrl Pts',(4.05126345799994,2.2,-0.481148277000014));
#347045=CARTESIAN_POINT('Ctrl Pts',(4.05228634599994,12.2,-0.481057884000013));
#347046=CARTESIAN_POINT('Ctrl Pts',(4.05228634599994,5.2,-0.481057884000013));
#347047=CARTESIAN_POINT('Ctrl Pts',(4.05228634599994,2.2,-0.481057884000013));
#347048=CARTESIAN_POINT('Ctrl Pts',(4.05331453399994,12.2,-0.480965749000015));
#347049=CARTESIAN_POINT('Ctrl Pts',(4.05331453399994,5.2,-0.480965749000015));
#347050=CARTESIAN_POINT('Ctrl Pts',(4.05331453399994,2.2,-0.480965749000015));
#347051=CARTESIAN_POINT('Ctrl Pts',(4.05434801099995,12.2,-0.480871860000014));
#347052=CARTESIAN_POINT('Ctrl Pts',(4.05434801099995,5.2,-0.480871860000014));
#347053=CARTESIAN_POINT('Ctrl Pts',(4.05434801099995,2.2,-0.480871860000014));
#347054=CARTESIAN_POINT('Ctrl Pts',(4.05538676699994,12.2,-0.480776208000013));
#347055=CARTESIAN_POINT('Ctrl Pts',(4.05538676699994,5.2,-0.480776208000013));
#347056=CARTESIAN_POINT('Ctrl Pts',(4.05538676699994,2.2,-0.480776208000013));
#347057=CARTESIAN_POINT('Ctrl Pts',(4.05643078799994,12.2,-0.480678780000012));
#347058=CARTESIAN_POINT('Ctrl Pts',(4.05643078799994,5.2,-0.480678780000012));
#347059=CARTESIAN_POINT('Ctrl Pts',(4.05643078799994,2.2,-0.480678780000012));
#347060=CARTESIAN_POINT('Ctrl Pts',(4.05748006299994,12.2,-0.480579565000014));
#347061=CARTESIAN_POINT('Ctrl Pts',(4.05748006299994,5.2,-0.480579565000014));
#347062=CARTESIAN_POINT('Ctrl Pts',(4.05748006299994,2.2,-0.480579565000014));
#347063=CARTESIAN_POINT('Ctrl Pts',(4.05853458199994,12.2,-0.480478550000014));
#347064=CARTESIAN_POINT('Ctrl Pts',(4.05853458199994,5.2,-0.480478550000014));
#347065=CARTESIAN_POINT('Ctrl Pts',(4.05853458199994,2.2,-0.480478550000014));
#347066=CARTESIAN_POINT('Ctrl Pts',(4.05959433099994,12.2,-0.480375726000015));
#347067=CARTESIAN_POINT('Ctrl Pts',(4.05959433099994,5.2,-0.480375726000015));
#347068=CARTESIAN_POINT('Ctrl Pts',(4.05959433099994,2.2,-0.480375726000015));
#347069=CARTESIAN_POINT('Ctrl Pts',(4.06065929999994,12.2,-0.480271080000012));
#347070=CARTESIAN_POINT('Ctrl Pts',(4.06065929999994,5.2,-0.480271080000012));
#347071=CARTESIAN_POINT('Ctrl Pts',(4.06065929999994,2.2,-0.480271080000012));
#347072=CARTESIAN_POINT('Ctrl Pts',(4.06172947699995,12.2,-0.480164600000013));
#347073=CARTESIAN_POINT('Ctrl Pts',(4.06172947699995,5.2,-0.480164600000013));
#347074=CARTESIAN_POINT('Ctrl Pts',(4.06172947699995,2.2,-0.480164600000013));
#347075=CARTESIAN_POINT('Ctrl Pts',(4.06280485199995,12.2,-0.480056278000016));
#347076=CARTESIAN_POINT('Ctrl Pts',(4.06280485199995,5.2,-0.480056278000016));
#347077=CARTESIAN_POINT('Ctrl Pts',(4.06280485199995,2.2,-0.480056278000016));
#347078=CARTESIAN_POINT('Ctrl Pts',(4.06388541099994,12.2,-0.479946099000017));
#347079=CARTESIAN_POINT('Ctrl Pts',(4.06388541099994,5.2,-0.479946099000017));
#347080=CARTESIAN_POINT('Ctrl Pts',(4.06388541099994,2.2,-0.479946099000017));
#347081=CARTESIAN_POINT('Ctrl Pts',(4.06497114499994,12.2,-0.479834053000014));
#347082=CARTESIAN_POINT('Ctrl Pts',(4.06497114499994,5.2,-0.479834053000014));
#347083=CARTESIAN_POINT('Ctrl Pts',(4.06497114499994,2.2,-0.479834053000014));
#347084=CARTESIAN_POINT('Ctrl Pts',(4.06606203999995,12.2,-0.479720131000012));
#347085=CARTESIAN_POINT('Ctrl Pts',(4.06606203999995,5.2,-0.479720131000012));
#347086=CARTESIAN_POINT('Ctrl Pts',(4.06606203999995,2.2,-0.479720131000012));
#347087=CARTESIAN_POINT('Ctrl Pts',(4.06715808699994,12.2,-0.479604318000018));
#347088=CARTESIAN_POINT('Ctrl Pts',(4.06715808699994,5.2,-0.479604318000018));
#347089=CARTESIAN_POINT('Ctrl Pts',(4.06715808699994,2.2,-0.479604318000018));
#347090=CARTESIAN_POINT('Ctrl Pts',(4.06825927299994,12.2,-0.479486607000013));
#347091=CARTESIAN_POINT('Ctrl Pts',(4.06825927299994,5.2,-0.479486607000013));
#347092=CARTESIAN_POINT('Ctrl Pts',(4.06825927299994,2.2,-0.479486607000013));
#347093=CARTESIAN_POINT('Ctrl Pts',(4.06936558599994,12.2,-0.479366984000014));
#347094=CARTESIAN_POINT('Ctrl Pts',(4.06936558599994,5.2,-0.479366984000014));
#347095=CARTESIAN_POINT('Ctrl Pts',(4.06936558599994,2.2,-0.479366984000014));
#347096=CARTESIAN_POINT('Ctrl Pts',(4.07047701699994,12.2,-0.479245440000016));
#347097=CARTESIAN_POINT('Ctrl Pts',(4.07047701699994,5.2,-0.479245440000016));
#347098=CARTESIAN_POINT('Ctrl Pts',(4.07047701699994,2.2,-0.479245440000016));
#347099=CARTESIAN_POINT('Ctrl Pts',(4.07159355199994,12.2,-0.479121962000013));
#347100=CARTESIAN_POINT('Ctrl Pts',(4.07159355199994,5.2,-0.479121962000013));
#347101=CARTESIAN_POINT('Ctrl Pts',(4.07159355199994,2.2,-0.479121962000013));
#347102=CARTESIAN_POINT('Ctrl Pts',(4.07271518199994,12.2,-0.478996541000014));
#347103=CARTESIAN_POINT('Ctrl Pts',(4.07271518199994,5.2,-0.478996541000014));
#347104=CARTESIAN_POINT('Ctrl Pts',(4.07271518199994,2.2,-0.478996541000014));
#347105=CARTESIAN_POINT('Ctrl Pts',(4.07384189399994,12.2,-0.478869166000013));
#347106=CARTESIAN_POINT('Ctrl Pts',(4.07384189399994,5.2,-0.478869166000013));
#347107=CARTESIAN_POINT('Ctrl Pts',(4.07384189399994,2.2,-0.478869166000013));
#347108=CARTESIAN_POINT('Ctrl Pts',(4.07497367699994,12.2,-0.478739825000014));
#347109=CARTESIAN_POINT('Ctrl Pts',(4.07497367699994,5.2,-0.478739825000014));
#347110=CARTESIAN_POINT('Ctrl Pts',(4.07497367699994,2.2,-0.478739825000014));
#347111=CARTESIAN_POINT('Ctrl Pts',(4.07611051999995,12.2,-0.478608507000011));
#347112=CARTESIAN_POINT('Ctrl Pts',(4.07611051999995,5.2,-0.478608507000011));
#347113=CARTESIAN_POINT('Ctrl Pts',(4.07611051999995,2.2,-0.478608507000011));
#347114=CARTESIAN_POINT('Ctrl Pts',(4.07725240999994,12.2,-0.478475202000013));
#347115=CARTESIAN_POINT('Ctrl Pts',(4.07725240999994,5.2,-0.478475202000013));
#347116=CARTESIAN_POINT('Ctrl Pts',(4.07725240999994,2.2,-0.478475202000013));
#347117=CARTESIAN_POINT('Ctrl Pts',(4.07839933899994,12.2,-0.478339900000013));
#347118=CARTESIAN_POINT('Ctrl Pts',(4.07839933899994,5.2,-0.478339900000013));
#347119=CARTESIAN_POINT('Ctrl Pts',(4.07839933899994,2.2,-0.478339900000013));
#347120=CARTESIAN_POINT('Ctrl Pts',(4.07955129299994,12.2,-0.478202590000016));
#347121=CARTESIAN_POINT('Ctrl Pts',(4.07955129299994,5.2,-0.478202590000016));
#347122=CARTESIAN_POINT('Ctrl Pts',(4.07955129299994,2.2,-0.478202590000016));
#347123=CARTESIAN_POINT('Ctrl Pts',(4.08070826099994,12.2,-0.478063260000017));
#347124=CARTESIAN_POINT('Ctrl Pts',(4.08070826099994,5.2,-0.478063260000017));
#347125=CARTESIAN_POINT('Ctrl Pts',(4.08070826099994,2.2,-0.478063260000017));
#347126=CARTESIAN_POINT('Ctrl Pts',(4.08187023299995,12.2,-0.477921902000014));
#347127=CARTESIAN_POINT('Ctrl Pts',(4.08187023299995,5.2,-0.477921902000014));
#347128=CARTESIAN_POINT('Ctrl Pts',(4.08187023299995,2.2,-0.477921902000014));
#347129=CARTESIAN_POINT('Ctrl Pts',(4.08303719699994,12.2,-0.477778502000015));
#347130=CARTESIAN_POINT('Ctrl Pts',(4.08303719699994,5.2,-0.477778502000015));
#347131=CARTESIAN_POINT('Ctrl Pts',(4.08303719699994,2.2,-0.477778502000015));
#347132=CARTESIAN_POINT('Ctrl Pts',(4.08420914199994,12.2,-0.477633053000015));
#347133=CARTESIAN_POINT('Ctrl Pts',(4.08420914199994,5.2,-0.477633053000015));
#347134=CARTESIAN_POINT('Ctrl Pts',(4.08420914199994,2.2,-0.477633053000015));
#347135=CARTESIAN_POINT('Ctrl Pts',(4.08538605599994,12.2,-0.477485542000018));
#347136=CARTESIAN_POINT('Ctrl Pts',(4.08538605599994,5.2,-0.477485542000018));
#347137=CARTESIAN_POINT('Ctrl Pts',(4.08538605599994,2.2,-0.477485542000018));
#347138=CARTESIAN_POINT('Ctrl Pts',(4.08656792799994,12.2,-0.477335960000014));
#347139=CARTESIAN_POINT('Ctrl Pts',(4.08656792799994,5.2,-0.477335960000014));
#347140=CARTESIAN_POINT('Ctrl Pts',(4.08656792799994,2.2,-0.477335960000014));
#347141=CARTESIAN_POINT('Ctrl Pts',(4.08775474699994,12.2,-0.477184296000015));
#347142=CARTESIAN_POINT('Ctrl Pts',(4.08775474699994,5.2,-0.477184296000015));
#347143=CARTESIAN_POINT('Ctrl Pts',(4.08775474699994,2.2,-0.477184296000015));
#347144=CARTESIAN_POINT('Ctrl Pts',(4.08894650199994,12.2,-0.477030541000012));
#347145=CARTESIAN_POINT('Ctrl Pts',(4.08894650199994,5.2,-0.477030541000012));
#347146=CARTESIAN_POINT('Ctrl Pts',(4.08894650199994,2.2,-0.477030541000012));
#347147=CARTESIAN_POINT('Ctrl Pts',(4.09014318199994,12.2,-0.476874682000012));
#347148=CARTESIAN_POINT('Ctrl Pts',(4.09014318199994,5.2,-0.476874682000012));
#347149=CARTESIAN_POINT('Ctrl Pts',(4.09014318199994,2.2,-0.476874682000012));
#347150=CARTESIAN_POINT('Ctrl Pts',(4.09134477499994,12.2,-0.476716711000016));
#347151=CARTESIAN_POINT('Ctrl Pts',(4.09134477499994,5.2,-0.476716711000016));
#347152=CARTESIAN_POINT('Ctrl Pts',(4.09134477499994,2.2,-0.476716711000016));
#347153=CARTESIAN_POINT('Ctrl Pts',(4.09255126999994,12.2,-0.476556616000017));
#347154=CARTESIAN_POINT('Ctrl Pts',(4.09255126999994,5.2,-0.476556616000017));
#347155=CARTESIAN_POINT('Ctrl Pts',(4.09255126999994,2.2,-0.476556616000017));
#347156=CARTESIAN_POINT('Ctrl Pts',(4.09376265599994,12.2,-0.476394388000014));
#347157=CARTESIAN_POINT('Ctrl Pts',(4.09376265599994,5.2,-0.476394388000014));
#347158=CARTESIAN_POINT('Ctrl Pts',(4.09376265599994,2.2,-0.476394388000014));
#347159=CARTESIAN_POINT('Ctrl Pts',(4.09497892299994,12.2,-0.476230018000017));
#347160=CARTESIAN_POINT('Ctrl Pts',(4.09497892299994,5.2,-0.476230018000017));
#347161=CARTESIAN_POINT('Ctrl Pts',(4.09497892299994,2.2,-0.476230018000017));
#347162=CARTESIAN_POINT('Ctrl Pts',(4.09620005699994,12.2,-0.476063493000014));
#347163=CARTESIAN_POINT('Ctrl Pts',(4.09620005699994,5.2,-0.476063493000014));
#347164=CARTESIAN_POINT('Ctrl Pts',(4.09620005699994,2.2,-0.476063493000014));
#347165=CARTESIAN_POINT('Ctrl Pts',(4.09742605099995,12.2,-0.475894805000014));
#347166=CARTESIAN_POINT('Ctrl Pts',(4.09742605099995,5.2,-0.475894805000014));
#347167=CARTESIAN_POINT('Ctrl Pts',(4.09742605099995,2.2,-0.475894805000014));
#347168=CARTESIAN_POINT('Ctrl Pts',(4.09865689099994,12.2,-0.475723944000013));
#347169=CARTESIAN_POINT('Ctrl Pts',(4.09865689099994,5.2,-0.475723944000013));
#347170=CARTESIAN_POINT('Ctrl Pts',(4.09865689099994,2.2,-0.475723944000013));
#347171=CARTESIAN_POINT('Ctrl Pts',(4.09989256499994,12.2,-0.475550898000012));
#347172=CARTESIAN_POINT('Ctrl Pts',(4.09989256499994,5.2,-0.475550898000012));
#347173=CARTESIAN_POINT('Ctrl Pts',(4.09989256499994,2.2,-0.475550898000012));
#347174=CARTESIAN_POINT('Ctrl Pts',(4.10113306499994,12.2,-0.475375660000013));
#347175=CARTESIAN_POINT('Ctrl Pts',(4.10113306499994,5.2,-0.475375660000013));
#347176=CARTESIAN_POINT('Ctrl Pts',(4.10113306499994,2.2,-0.475375660000013));
#347177=CARTESIAN_POINT('Ctrl Pts',(4.10237837799994,12.2,-0.475198217000017));
#347178=CARTESIAN_POINT('Ctrl Pts',(4.10237837799994,5.2,-0.475198217000017));
#347179=CARTESIAN_POINT('Ctrl Pts',(4.10237837799994,2.2,-0.475198217000017));
#347180=CARTESIAN_POINT('Ctrl Pts',(4.10362849299994,12.2,-0.475018562000016));
#347181=CARTESIAN_POINT('Ctrl Pts',(4.10362849299994,5.2,-0.475018562000016));
#347182=CARTESIAN_POINT('Ctrl Pts',(4.10362849299994,2.2,-0.475018562000016));
#347183=CARTESIAN_POINT('Ctrl Pts',(4.10488339999994,12.2,-0.474836683000017));
#347184=CARTESIAN_POINT('Ctrl Pts',(4.10488339999994,5.2,-0.474836683000017));
#347185=CARTESIAN_POINT('Ctrl Pts',(4.10488339999994,2.2,-0.474836683000017));
#347186=CARTESIAN_POINT('Ctrl Pts',(4.10614308599994,12.2,-0.474652570000016));
#347187=CARTESIAN_POINT('Ctrl Pts',(4.10614308599994,5.2,-0.474652570000016));
#347188=CARTESIAN_POINT('Ctrl Pts',(4.10614308599994,2.2,-0.474652570000016));
#347189=CARTESIAN_POINT('Ctrl Pts',(4.10740754199994,12.2,-0.474466215000016));
#347190=CARTESIAN_POINT('Ctrl Pts',(4.10740754199994,5.2,-0.474466215000016));
#347191=CARTESIAN_POINT('Ctrl Pts',(4.10740754199994,2.2,-0.474466215000016));
#347192=CARTESIAN_POINT('Ctrl Pts',(4.10867675699994,12.2,-0.474277608000016));
#347193=CARTESIAN_POINT('Ctrl Pts',(4.10867675699994,5.2,-0.474277608000016));
#347194=CARTESIAN_POINT('Ctrl Pts',(4.10867675699994,2.2,-0.474277608000016));
#347195=CARTESIAN_POINT('Ctrl Pts',(4.10995071699995,12.2,-0.474086738000015));
#347196=CARTESIAN_POINT('Ctrl Pts',(4.10995071699995,5.2,-0.474086738000015));
#347197=CARTESIAN_POINT('Ctrl Pts',(4.10995071699995,2.2,-0.474086738000015));
#347198=CARTESIAN_POINT('Ctrl Pts',(4.11122941499994,12.2,-0.473893597000017));
#347199=CARTESIAN_POINT('Ctrl Pts',(4.11122941499994,5.2,-0.473893597000017));
#347200=CARTESIAN_POINT('Ctrl Pts',(4.11122941499994,2.2,-0.473893597000017));
#347201=CARTESIAN_POINT('Ctrl Pts',(4.11251283799994,12.2,-0.473698173000017));
#347202=CARTESIAN_POINT('Ctrl Pts',(4.11251283799994,5.2,-0.473698173000017));
#347203=CARTESIAN_POINT('Ctrl Pts',(4.11251283799994,2.2,-0.473698173000017));
#347204=CARTESIAN_POINT('Ctrl Pts',(4.11380097599995,12.2,-0.473500458000018));
#347205=CARTESIAN_POINT('Ctrl Pts',(4.11380097599995,5.2,-0.473500458000018));
#347206=CARTESIAN_POINT('Ctrl Pts',(4.11380097599995,2.2,-0.473500458000018));
#347207=CARTESIAN_POINT('Ctrl Pts',(4.11509381599994,12.2,-0.473300442000015));
#347208=CARTESIAN_POINT('Ctrl Pts',(4.11509381599994,5.2,-0.473300442000015));
#347209=CARTESIAN_POINT('Ctrl Pts',(4.11509381599994,2.2,-0.473300442000015));
#347210=CARTESIAN_POINT('Ctrl Pts',(4.11639134899994,12.2,-0.473098116000017));
#347211=CARTESIAN_POINT('Ctrl Pts',(4.11639134899994,5.2,-0.473098116000017));
#347212=CARTESIAN_POINT('Ctrl Pts',(4.11639134899994,2.2,-0.473098116000017));
#347213=CARTESIAN_POINT('Ctrl Pts',(4.11769356299994,12.2,-0.472893470000013));
#347214=CARTESIAN_POINT('Ctrl Pts',(4.11769356299994,5.2,-0.472893470000013));
#347215=CARTESIAN_POINT('Ctrl Pts',(4.11769356299994,2.2,-0.472893470000013));
#347216=CARTESIAN_POINT('Ctrl Pts',(4.11900044799994,12.2,-0.472686494000012));
#347217=CARTESIAN_POINT('Ctrl Pts',(4.11900044799994,5.2,-0.472686494000012));
#347218=CARTESIAN_POINT('Ctrl Pts',(4.11900044799994,2.2,-0.472686494000012));
#347219=CARTESIAN_POINT('Ctrl Pts',(4.12031199199994,12.2,-0.472477180000013));
#347220=CARTESIAN_POINT('Ctrl Pts',(4.12031199199994,5.2,-0.472477180000013));
#347221=CARTESIAN_POINT('Ctrl Pts',(4.12031199199994,2.2,-0.472477180000013));
#347222=CARTESIAN_POINT('Ctrl Pts',(4.12162818599994,12.2,-0.472265517000015));
#347223=CARTESIAN_POINT('Ctrl Pts',(4.12162818599994,5.2,-0.472265517000015));
#347224=CARTESIAN_POINT('Ctrl Pts',(4.12162818599994,2.2,-0.472265517000015));
#347225=CARTESIAN_POINT('Ctrl Pts',(4.12294901699994,12.2,-0.472051498000017));
#347226=CARTESIAN_POINT('Ctrl Pts',(4.12294901699994,5.2,-0.472051498000017));
#347227=CARTESIAN_POINT('Ctrl Pts',(4.12294901699994,2.2,-0.472051498000017));
#347228=CARTESIAN_POINT('Ctrl Pts',(4.12427447499994,12.2,-0.471835110000014));
#347229=CARTESIAN_POINT('Ctrl Pts',(4.12427447499994,5.2,-0.471835110000014));
#347230=CARTESIAN_POINT('Ctrl Pts',(4.12427447499994,2.2,-0.471835110000014));
#347231=CARTESIAN_POINT('Ctrl Pts',(4.12560454899995,12.2,-0.471616347000015));
#347232=CARTESIAN_POINT('Ctrl Pts',(4.12560454899995,5.2,-0.471616347000015));
#347233=CARTESIAN_POINT('Ctrl Pts',(4.12560454899995,2.2,-0.471616347000015));
#347234=CARTESIAN_POINT('Ctrl Pts',(4.12693922899994,12.2,-0.471395199000018));
#347235=CARTESIAN_POINT('Ctrl Pts',(4.12693922899994,5.2,-0.471395199000018));
#347236=CARTESIAN_POINT('Ctrl Pts',(4.12693922899994,2.2,-0.471395199000018));
#347237=CARTESIAN_POINT('Ctrl Pts',(4.12827850199994,12.2,-0.471171656000013));
#347238=CARTESIAN_POINT('Ctrl Pts',(4.12827850199994,5.2,-0.471171656000013));
#347239=CARTESIAN_POINT('Ctrl Pts',(4.12827850199994,2.2,-0.471171656000013));
#347240=CARTESIAN_POINT('Ctrl Pts',(4.12962235999994,12.2,-0.470945710000015));
#347241=CARTESIAN_POINT('Ctrl Pts',(4.12962235999994,5.2,-0.470945710000015));
#347242=CARTESIAN_POINT('Ctrl Pts',(4.12962235999994,2.2,-0.470945710000015));
#347243=CARTESIAN_POINT('Ctrl Pts',(4.13097078999995,12.2,-0.470717349000012));
#347244=CARTESIAN_POINT('Ctrl Pts',(4.13097078999995,5.2,-0.470717349000012));
#347245=CARTESIAN_POINT('Ctrl Pts',(4.13097078999995,2.2,-0.470717349000012));
#347246=CARTESIAN_POINT('Ctrl Pts',(4.13232378199995,12.2,-0.470486567000012));
#347247=CARTESIAN_POINT('Ctrl Pts',(4.13232378199995,5.2,-0.470486567000012));
#347248=CARTESIAN_POINT('Ctrl Pts',(4.13232378199995,2.2,-0.470486567000012));
#347249=CARTESIAN_POINT('Ctrl Pts',(4.13368132599994,12.2,-0.470253354000012));
#347250=CARTESIAN_POINT('Ctrl Pts',(4.13368132599994,5.2,-0.470253354000012));
#347251=CARTESIAN_POINT('Ctrl Pts',(4.13368132599994,2.2,-0.470253354000012));
#347252=CARTESIAN_POINT('Ctrl Pts',(4.13504340999994,12.2,-0.470017700000014));
#347253=CARTESIAN_POINT('Ctrl Pts',(4.13504340999994,5.2,-0.470017700000014));
#347254=CARTESIAN_POINT('Ctrl Pts',(4.13504340999994,2.2,-0.470017700000014));
#347255=CARTESIAN_POINT('Ctrl Pts',(4.13641002299994,12.2,-0.469779598000013));
#347256=CARTESIAN_POINT('Ctrl Pts',(4.13641002299994,5.2,-0.469779598000013));
#347257=CARTESIAN_POINT('Ctrl Pts',(4.13641002299994,2.2,-0.469779598000013));
#347258=CARTESIAN_POINT('Ctrl Pts',(4.13778115599994,12.2,-0.469539037000013));
#347259=CARTESIAN_POINT('Ctrl Pts',(4.13778115599994,5.2,-0.469539037000013));
#347260=CARTESIAN_POINT('Ctrl Pts',(4.13778115599994,2.2,-0.469539037000013));
#347261=CARTESIAN_POINT('Ctrl Pts',(4.13915679599994,12.2,-0.469296008000013));
#347262=CARTESIAN_POINT('Ctrl Pts',(4.13915679599994,5.2,-0.469296008000013));
#347263=CARTESIAN_POINT('Ctrl Pts',(4.13915679599994,2.2,-0.469296008000013));
#347264=CARTESIAN_POINT('Ctrl Pts',(4.14053693499994,12.2,-0.469050504000013));
#347265=CARTESIAN_POINT('Ctrl Pts',(4.14053693499994,5.2,-0.469050504000013));
#347266=CARTESIAN_POINT('Ctrl Pts',(4.14053693499994,2.2,-0.469050504000013));
#347267=CARTESIAN_POINT('Ctrl Pts',(4.14192155899994,12.2,-0.468802514000015));
#347268=CARTESIAN_POINT('Ctrl Pts',(4.14192155899994,5.2,-0.468802514000015));
#347269=CARTESIAN_POINT('Ctrl Pts',(4.14192155899994,2.2,-0.468802514000015));
#347270=CARTESIAN_POINT('Ctrl Pts',(4.14331065899994,12.2,-0.468552031000016));
#347271=CARTESIAN_POINT('Ctrl Pts',(4.14331065899994,5.2,-0.468552031000016));
#347272=CARTESIAN_POINT('Ctrl Pts',(4.14331065899994,2.2,-0.468552031000016));
#347273=CARTESIAN_POINT('Ctrl Pts',(4.14470422499994,12.2,-0.468299046000014));
#347274=CARTESIAN_POINT('Ctrl Pts',(4.14470422499994,5.2,-0.468299046000014));
#347275=CARTESIAN_POINT('Ctrl Pts',(4.14470422499994,2.2,-0.468299046000014));
#347276=CARTESIAN_POINT('Ctrl Pts',(4.14610224599994,12.2,-0.468043548000012));
#347277=CARTESIAN_POINT('Ctrl Pts',(4.14610224599994,5.2,-0.468043548000012));
#347278=CARTESIAN_POINT('Ctrl Pts',(4.14610224599994,2.2,-0.468043548000012));
#347279=CARTESIAN_POINT('Ctrl Pts',(4.14750470899994,12.2,-0.467785530000011));
#347280=CARTESIAN_POINT('Ctrl Pts',(4.14750470899994,5.2,-0.467785530000011));
#347281=CARTESIAN_POINT('Ctrl Pts',(4.14750470899994,2.2,-0.467785530000011));
#347282=CARTESIAN_POINT('Ctrl Pts',(4.14891160699994,12.2,-0.467524983000014));
#347283=CARTESIAN_POINT('Ctrl Pts',(4.14891160699994,5.2,-0.467524983000014));
#347284=CARTESIAN_POINT('Ctrl Pts',(4.14891160699994,2.2,-0.467524983000014));
#347285=CARTESIAN_POINT('Ctrl Pts',(4.15032292699994,12.2,-0.467261899000011));
#347286=CARTESIAN_POINT('Ctrl Pts',(4.15032292699994,5.2,-0.467261899000011));
#347287=CARTESIAN_POINT('Ctrl Pts',(4.15032292699994,2.2,-0.467261899000011));
#347288=CARTESIAN_POINT('Ctrl Pts',(4.15173865799995,12.2,-0.466996269000015));
#347289=CARTESIAN_POINT('Ctrl Pts',(4.15173865799995,5.2,-0.466996269000015));
#347290=CARTESIAN_POINT('Ctrl Pts',(4.15173865799995,2.2,-0.466996269000015));
#347291=CARTESIAN_POINT('Ctrl Pts',(4.15315879199994,12.2,-0.466728082000016));
#347292=CARTESIAN_POINT('Ctrl Pts',(4.15315879199994,5.2,-0.466728082000016));
#347293=CARTESIAN_POINT('Ctrl Pts',(4.15315879199994,2.2,-0.466728082000016));
#347294=CARTESIAN_POINT('Ctrl Pts',(4.15458331499994,12.2,-0.466457333000014));
#347295=CARTESIAN_POINT('Ctrl Pts',(4.15458331499994,5.2,-0.466457333000014));
#347296=CARTESIAN_POINT('Ctrl Pts',(4.15458331499994,2.2,-0.466457333000014));
#347297=CARTESIAN_POINT('Ctrl Pts',(4.15601221799994,12.2,-0.466184012000017));
#347298=CARTESIAN_POINT('Ctrl Pts',(4.15601221799994,5.2,-0.466184012000017));
#347299=CARTESIAN_POINT('Ctrl Pts',(4.15601221799994,2.2,-0.466184012000017));
#347300=CARTESIAN_POINT('Ctrl Pts',(4.15744549099994,12.2,-0.465908110000015));
#347301=CARTESIAN_POINT('Ctrl Pts',(4.15744549099994,5.2,-0.465908110000015));
#347302=CARTESIAN_POINT('Ctrl Pts',(4.15744549099994,2.2,-0.465908110000015));
#347303=CARTESIAN_POINT('Ctrl Pts',(4.15888312199994,12.2,-0.465629618000012));
#347304=CARTESIAN_POINT('Ctrl Pts',(4.15888312199994,5.2,-0.465629618000012));
#347305=CARTESIAN_POINT('Ctrl Pts',(4.15888312199994,2.2,-0.465629618000012));
#347306=CARTESIAN_POINT('Ctrl Pts',(4.16032510199994,12.2,-0.465348529000016));
#347307=CARTESIAN_POINT('Ctrl Pts',(4.16032510199994,5.2,-0.465348529000016));
#347308=CARTESIAN_POINT('Ctrl Pts',(4.16032510199994,2.2,-0.465348529000016));
#347309=CARTESIAN_POINT('Ctrl Pts',(4.16177141899994,12.2,-0.465064834000017));
#347310=CARTESIAN_POINT('Ctrl Pts',(4.16177141899994,5.2,-0.465064834000017));
#347311=CARTESIAN_POINT('Ctrl Pts',(4.16177141899994,2.2,-0.465064834000017));
#347312=CARTESIAN_POINT('Ctrl Pts',(4.16322206499994,12.2,-0.464778525000016));
#347313=CARTESIAN_POINT('Ctrl Pts',(4.16322206499994,5.2,-0.464778525000016));
#347314=CARTESIAN_POINT('Ctrl Pts',(4.16322206499994,2.2,-0.464778525000016));
#347315=CARTESIAN_POINT('Ctrl Pts',(4.16467702499994,12.2,-0.464489593000015));
#347316=CARTESIAN_POINT('Ctrl Pts',(4.16467702499994,5.2,-0.464489593000015));
#347317=CARTESIAN_POINT('Ctrl Pts',(4.16467702499994,2.2,-0.464489593000015));
#347318=CARTESIAN_POINT('Ctrl Pts',(4.16613629199994,12.2,-0.464198030000014));
#347319=CARTESIAN_POINT('Ctrl Pts',(4.16613629199994,5.2,-0.464198030000014));
#347320=CARTESIAN_POINT('Ctrl Pts',(4.16613629199994,2.2,-0.464198030000014));
#347321=CARTESIAN_POINT('Ctrl Pts',(4.16759985399994,12.2,-0.463903826000016));
#347322=CARTESIAN_POINT('Ctrl Pts',(4.16759985399994,5.2,-0.463903826000016));
#347323=CARTESIAN_POINT('Ctrl Pts',(4.16759985399994,2.2,-0.463903826000016));
#347324=CARTESIAN_POINT('Ctrl Pts',(4.16906769999995,12.2,-0.463606975000013));
#347325=CARTESIAN_POINT('Ctrl Pts',(4.16906769999995,5.2,-0.463606975000013));
#347326=CARTESIAN_POINT('Ctrl Pts',(4.16906769999995,2.2,-0.463606975000013));
#347327=CARTESIAN_POINT('Ctrl Pts',(4.17053982099994,12.2,-0.463307468000016));
#347328=CARTESIAN_POINT('Ctrl Pts',(4.17053982099994,5.2,-0.463307468000016));
#347329=CARTESIAN_POINT('Ctrl Pts',(4.17053982099994,2.2,-0.463307468000016));
#347330=CARTESIAN_POINT('Ctrl Pts',(4.17201620699994,12.2,-0.463005298000017));
#347331=CARTESIAN_POINT('Ctrl Pts',(4.17201620699994,5.2,-0.463005298000017));
#347332=CARTESIAN_POINT('Ctrl Pts',(4.17201620699994,2.2,-0.463005298000017));
#347333=CARTESIAN_POINT('Ctrl Pts',(4.17349684399994,12.2,-0.462700453000018));
#347334=CARTESIAN_POINT('Ctrl Pts',(4.17349684399994,5.2,-0.462700453000018));
#347335=CARTESIAN_POINT('Ctrl Pts',(4.17349684399994,2.2,-0.462700453000018));
#347336=CARTESIAN_POINT('Ctrl Pts',(4.17498172499995,12.2,-0.462392929000015));
#347337=CARTESIAN_POINT('Ctrl Pts',(4.17498172499995,5.2,-0.462392929000015));
#347338=CARTESIAN_POINT('Ctrl Pts',(4.17498172499995,2.2,-0.462392929000015));
#347339=CARTESIAN_POINT('Ctrl Pts',(4.17647083799995,12.2,-0.462082716000012));
#347340=CARTESIAN_POINT('Ctrl Pts',(4.17647083799995,5.2,-0.462082716000012));
#347341=CARTESIAN_POINT('Ctrl Pts',(4.17647083799995,2.2,-0.462082716000012));
#347342=CARTESIAN_POINT('Ctrl Pts',(4.17796417399994,12.2,-0.461769807000016));
#347343=CARTESIAN_POINT('Ctrl Pts',(4.17796417399994,5.2,-0.461769807000016));
#347344=CARTESIAN_POINT('Ctrl Pts',(4.17796417399994,2.2,-0.461769807000016));
#347345=CARTESIAN_POINT('Ctrl Pts',(4.17946172099994,12.2,-0.461454192000015));
#347346=CARTESIAN_POINT('Ctrl Pts',(4.17946172099994,5.2,-0.461454192000015));
#347347=CARTESIAN_POINT('Ctrl Pts',(4.17946172099994,2.2,-0.461454192000015));
#347348=CARTESIAN_POINT('Ctrl Pts',(4.18096346899994,12.2,-0.461135864000015));
#347349=CARTESIAN_POINT('Ctrl Pts',(4.18096346899994,5.2,-0.461135864000015));
#347350=CARTESIAN_POINT('Ctrl Pts',(4.18096346899994,2.2,-0.461135864000015));
#347351=CARTESIAN_POINT('Ctrl Pts',(4.18246940699994,12.2,-0.460814815000017));
#347352=CARTESIAN_POINT('Ctrl Pts',(4.18246940699994,5.2,-0.460814815000017));
#347353=CARTESIAN_POINT('Ctrl Pts',(4.18246940699994,2.2,-0.460814815000017));
#347354=CARTESIAN_POINT('Ctrl Pts',(4.18397952499994,12.2,-0.460491039000015));
#347355=CARTESIAN_POINT('Ctrl Pts',(4.18397952499994,5.2,-0.460491039000015));
#347356=CARTESIAN_POINT('Ctrl Pts',(4.18397952499994,2.2,-0.460491039000015));
#347357=CARTESIAN_POINT('Ctrl Pts',(4.18549381299994,12.2,-0.460164523000017));
#347358=CARTESIAN_POINT('Ctrl Pts',(4.18549381299994,5.2,-0.460164523000017));
#347359=CARTESIAN_POINT('Ctrl Pts',(4.18549381299994,2.2,-0.460164523000017));
#347360=CARTESIAN_POINT('Ctrl Pts',(4.18701225999994,12.2,-0.459835264000015));
#347361=CARTESIAN_POINT('Ctrl Pts',(4.18701225999994,5.2,-0.459835264000015));
#347362=CARTESIAN_POINT('Ctrl Pts',(4.18701225999994,2.2,-0.459835264000015));
#347363=CARTESIAN_POINT('Ctrl Pts',(4.18853485599994,12.2,-0.459503253000015));
#347364=CARTESIAN_POINT('Ctrl Pts',(4.18853485599994,5.2,-0.459503253000015));
#347365=CARTESIAN_POINT('Ctrl Pts',(4.18853485599994,2.2,-0.459503253000015));
#347366=CARTESIAN_POINT('Ctrl Pts',(4.19006159099994,12.2,-0.459168479000014));
#347367=CARTESIAN_POINT('Ctrl Pts',(4.19006159099994,5.2,-0.459168479000014));
#347368=CARTESIAN_POINT('Ctrl Pts',(4.19006159099994,2.2,-0.459168479000014));
#347369=CARTESIAN_POINT('Ctrl Pts',(4.19159245399995,12.2,-0.458830938000014));
#347370=CARTESIAN_POINT('Ctrl Pts',(4.19159245399995,5.2,-0.458830938000014));
#347371=CARTESIAN_POINT('Ctrl Pts',(4.19159245399995,2.2,-0.458830938000014));
#347372=CARTESIAN_POINT('Ctrl Pts',(4.19312743399994,12.2,-0.458490621000016));
#347373=CARTESIAN_POINT('Ctrl Pts',(4.19312743399994,5.2,-0.458490621000016));
#347374=CARTESIAN_POINT('Ctrl Pts',(4.19312743399994,2.2,-0.458490621000016));
#347375=CARTESIAN_POINT('Ctrl Pts',(4.19466652199994,12.2,-0.458147520000014));
#347376=CARTESIAN_POINT('Ctrl Pts',(4.19466652199994,5.2,-0.458147520000014));
#347377=CARTESIAN_POINT('Ctrl Pts',(4.19466652199994,2.2,-0.458147520000014));
#347378=CARTESIAN_POINT('Ctrl Pts',(4.19620970699994,12.2,-0.457801626000016));
#347379=CARTESIAN_POINT('Ctrl Pts',(4.19620970699994,5.2,-0.457801626000016));
#347380=CARTESIAN_POINT('Ctrl Pts',(4.19620970699994,2.2,-0.457801626000016));
#347381=CARTESIAN_POINT('Ctrl Pts',(4.19775697799994,12.2,-0.457452935000013));
#347382=CARTESIAN_POINT('Ctrl Pts',(4.19775697799994,5.2,-0.457452935000013));
#347383=CARTESIAN_POINT('Ctrl Pts',(4.19775697799994,2.2,-0.457452935000013));
#347384=CARTESIAN_POINT('Ctrl Pts',(4.19930832699994,12.2,-0.457101434000013));
#347385=CARTESIAN_POINT('Ctrl Pts',(4.19930832699994,5.2,-0.457101434000013));
#347386=CARTESIAN_POINT('Ctrl Pts',(4.19930832699994,2.2,-0.457101434000013));
#347387=CARTESIAN_POINT('Ctrl Pts',(4.20086373999994,12.2,-0.456747121000016));
#347388=CARTESIAN_POINT('Ctrl Pts',(4.20086373999994,5.2,-0.456747121000016));
#347389=CARTESIAN_POINT('Ctrl Pts',(4.20086373999994,2.2,-0.456747121000016));
#347390=CARTESIAN_POINT('Ctrl Pts',(4.20242320999995,12.2,-0.456389984000012));
#347391=CARTESIAN_POINT('Ctrl Pts',(4.20242320999995,5.2,-0.456389984000012));
#347392=CARTESIAN_POINT('Ctrl Pts',(4.20242320999995,2.2,-0.456389984000012));
#347393=CARTESIAN_POINT('Ctrl Pts',(4.20398672499994,12.2,-0.456030016000017));
#347394=CARTESIAN_POINT('Ctrl Pts',(4.20398672499994,5.2,-0.456030016000017));
#347395=CARTESIAN_POINT('Ctrl Pts',(4.20398672499994,2.2,-0.456030016000017));
#347396=CARTESIAN_POINT('Ctrl Pts',(4.20555427599994,12.2,-0.455667212000015));
#347397=CARTESIAN_POINT('Ctrl Pts',(4.20555427599994,5.2,-0.455667212000015));
#347398=CARTESIAN_POINT('Ctrl Pts',(4.20555427599994,2.2,-0.455667212000015));
#347399=CARTESIAN_POINT('Ctrl Pts',(4.20712585099994,12.2,-0.455301563000017));
#347400=CARTESIAN_POINT('Ctrl Pts',(4.20712585099994,5.2,-0.455301563000017));
#347401=CARTESIAN_POINT('Ctrl Pts',(4.20712585099994,2.2,-0.455301563000017));
#347402=CARTESIAN_POINT('Ctrl Pts',(4.20870143999994,12.2,-0.454933060000013));
#347403=CARTESIAN_POINT('Ctrl Pts',(4.20870143999994,5.2,-0.454933060000013));
#347404=CARTESIAN_POINT('Ctrl Pts',(4.20870143999994,2.2,-0.454933060000013));
#347405=CARTESIAN_POINT('Ctrl Pts',(4.21028103499994,12.2,-0.454561698000013));
#347406=CARTESIAN_POINT('Ctrl Pts',(4.21028103499994,5.2,-0.454561698000013));
#347407=CARTESIAN_POINT('Ctrl Pts',(4.21028103499994,2.2,-0.454561698000013));
#347408=CARTESIAN_POINT('Ctrl Pts',(4.21186462299994,12.2,-0.454187467000011));
#347409=CARTESIAN_POINT('Ctrl Pts',(4.21186462299994,5.2,-0.454187467000011));
#347410=CARTESIAN_POINT('Ctrl Pts',(4.21186462299994,2.2,-0.454187467000011));
#347411=CARTESIAN_POINT('Ctrl Pts',(4.21345219499994,12.2,-0.453810363000016));
#347412=CARTESIAN_POINT('Ctrl Pts',(4.21345219499994,5.2,-0.453810363000016));
#347413=CARTESIAN_POINT('Ctrl Pts',(4.21345219499994,2.2,-0.453810363000016));
#347414=CARTESIAN_POINT('Ctrl Pts',(4.21504373999994,12.2,-0.453430375000017));
#347415=CARTESIAN_POINT('Ctrl Pts',(4.21504373999994,5.2,-0.453430375000017));
#347416=CARTESIAN_POINT('Ctrl Pts',(4.21504373999994,2.2,-0.453430375000017));
#347417=CARTESIAN_POINT('Ctrl Pts',(4.21663924899994,12.2,-0.453047497000014));
#347418=CARTESIAN_POINT('Ctrl Pts',(4.21663924899994,5.2,-0.453047497000014));
#347419=CARTESIAN_POINT('Ctrl Pts',(4.21663924899994,2.2,-0.453047497000014));
#347420=CARTESIAN_POINT('Ctrl Pts',(4.21823871099994,12.2,-0.452661723000016));
#347421=CARTESIAN_POINT('Ctrl Pts',(4.21823871099994,5.2,-0.452661723000016));
#347422=CARTESIAN_POINT('Ctrl Pts',(4.21823871099994,2.2,-0.452661723000016));
#347423=CARTESIAN_POINT('Ctrl Pts',(4.21984211599994,12.2,-0.452273044000013));
#347424=CARTESIAN_POINT('Ctrl Pts',(4.21984211599994,5.2,-0.452273044000013));
#347425=CARTESIAN_POINT('Ctrl Pts',(4.21984211599994,2.2,-0.452273044000013));
#347426=CARTESIAN_POINT('Ctrl Pts',(4.22144945399994,12.2,-0.451881453000014));
#347427=CARTESIAN_POINT('Ctrl Pts',(4.22144945399994,5.2,-0.451881453000014));
#347428=CARTESIAN_POINT('Ctrl Pts',(4.22144945399994,2.2,-0.451881453000014));
#347429=CARTESIAN_POINT('Ctrl Pts',(4.22306071499994,12.2,-0.451486943000017));
#347430=CARTESIAN_POINT('Ctrl Pts',(4.22306071499994,5.2,-0.451486943000017));
#347431=CARTESIAN_POINT('Ctrl Pts',(4.22306071499994,2.2,-0.451486943000017));
#347432=CARTESIAN_POINT('Ctrl Pts',(4.22467588799995,12.2,-0.451089507000013));
#347433=CARTESIAN_POINT('Ctrl Pts',(4.22467588799995,5.2,-0.451089507000013));
#347434=CARTESIAN_POINT('Ctrl Pts',(4.22467588799995,2.2,-0.451089507000013));
#347435=CARTESIAN_POINT('Ctrl Pts',(4.22629496199994,12.2,-0.450689138000016));
#347436=CARTESIAN_POINT('Ctrl Pts',(4.22629496199994,5.2,-0.450689138000016));
#347437=CARTESIAN_POINT('Ctrl Pts',(4.22629496199994,2.2,-0.450689138000016));
#347438=CARTESIAN_POINT('Ctrl Pts',(4.22791792999995,12.2,-0.450285826000014));
#347439=CARTESIAN_POINT('Ctrl Pts',(4.22791792999995,5.2,-0.450285826000014));
#347440=CARTESIAN_POINT('Ctrl Pts',(4.22791792999995,2.2,-0.450285826000014));
#347441=CARTESIAN_POINT('Ctrl Pts',(4.22954477799994,12.2,-0.449879568000018));
#347442=CARTESIAN_POINT('Ctrl Pts',(4.22954477799994,5.2,-0.449879568000018));
#347443=CARTESIAN_POINT('Ctrl Pts',(4.22954477799994,2.2,-0.449879568000018));
#347444=CARTESIAN_POINT('Ctrl Pts',(4.23117549899994,12.2,-0.449470355000017));
#347445=CARTESIAN_POINT('Ctrl Pts',(4.23117549899994,5.2,-0.449470355000017));
#347446=CARTESIAN_POINT('Ctrl Pts',(4.23117549899994,2.2,-0.449470355000017));
#347447=CARTESIAN_POINT('Ctrl Pts',(4.23281008199995,12.2,-0.449058180000015));
#347448=CARTESIAN_POINT('Ctrl Pts',(4.23281008199995,5.2,-0.449058180000015));
#347449=CARTESIAN_POINT('Ctrl Pts',(4.23281008199995,2.2,-0.449058180000015));
#347450=CARTESIAN_POINT('Ctrl Pts',(4.23444851499994,12.2,-0.448643035000016));
#347451=CARTESIAN_POINT('Ctrl Pts',(4.23444851499994,5.2,-0.448643035000016));
#347452=CARTESIAN_POINT('Ctrl Pts',(4.23444851499994,2.2,-0.448643035000016));
#347453=CARTESIAN_POINT('Ctrl Pts',(4.23609078999994,12.2,-0.448224914000015));
#347454=CARTESIAN_POINT('Ctrl Pts',(4.23609078999994,5.2,-0.448224914000015));
#347455=CARTESIAN_POINT('Ctrl Pts',(4.23609078999994,2.2,-0.448224914000015));
#347456=CARTESIAN_POINT('Ctrl Pts',(4.23773689699994,12.2,-0.447803810000016));
#347457=CARTESIAN_POINT('Ctrl Pts',(4.23773689699994,5.2,-0.447803810000016));
#347458=CARTESIAN_POINT('Ctrl Pts',(4.23773689699994,2.2,-0.447803810000016));
#347459=CARTESIAN_POINT('Ctrl Pts',(4.23938682399995,12.2,-0.447379715000018));
#347460=CARTESIAN_POINT('Ctrl Pts',(4.23938682399995,5.2,-0.447379715000018));
#347461=CARTESIAN_POINT('Ctrl Pts',(4.23938682399995,2.2,-0.447379715000018));
#347462=CARTESIAN_POINT('Ctrl Pts',(4.24104056399994,12.2,-0.446952624000012));
#347463=CARTESIAN_POINT('Ctrl Pts',(4.24104056399994,5.2,-0.446952624000012));
#347464=CARTESIAN_POINT('Ctrl Pts',(4.24104056399994,2.2,-0.446952624000012));
#347465=CARTESIAN_POINT('Ctrl Pts',(4.24269810399994,12.2,-0.446522529000015));
#347466=CARTESIAN_POINT('Ctrl Pts',(4.24269810399994,5.2,-0.446522529000015));
#347467=CARTESIAN_POINT('Ctrl Pts',(4.24269810399994,2.2,-0.446522529000015));
#347468=CARTESIAN_POINT('Ctrl Pts',(4.24435943499994,12.2,-0.446089421000018));
#347469=CARTESIAN_POINT('Ctrl Pts',(4.24435943499994,5.2,-0.446089421000018));
#347470=CARTESIAN_POINT('Ctrl Pts',(4.24435943499994,2.2,-0.446089421000018));
#347471=CARTESIAN_POINT('Ctrl Pts',(4.24602454599994,12.2,-0.445653297000015));
#347472=CARTESIAN_POINT('Ctrl Pts',(4.24602454599994,5.2,-0.445653297000015));
#347473=CARTESIAN_POINT('Ctrl Pts',(4.24602454599994,2.2,-0.445653297000015));
#347474=CARTESIAN_POINT('Ctrl Pts',(4.24769342899994,12.2,-0.445214148000015));
#347475=CARTESIAN_POINT('Ctrl Pts',(4.24769342899994,5.2,-0.445214148000015));
#347476=CARTESIAN_POINT('Ctrl Pts',(4.24769342899994,2.2,-0.445214148000015));
#347477=CARTESIAN_POINT('Ctrl Pts',(4.24936607299994,12.2,-0.444771966000013));
#347478=CARTESIAN_POINT('Ctrl Pts',(4.24936607299994,5.2,-0.444771966000013));
#347479=CARTESIAN_POINT('Ctrl Pts',(4.24936607299994,2.2,-0.444771966000013));
#347480=CARTESIAN_POINT('Ctrl Pts',(4.25104246699994,12.2,-0.444326746000012));
#347481=CARTESIAN_POINT('Ctrl Pts',(4.25104246699994,5.2,-0.444326746000012));
#347482=CARTESIAN_POINT('Ctrl Pts',(4.25104246699994,2.2,-0.444326746000012));
#347483=CARTESIAN_POINT('Ctrl Pts',(4.25272260199994,12.2,-0.443878482000013));
#347484=CARTESIAN_POINT('Ctrl Pts',(4.25272260199994,5.2,-0.443878482000013));
#347485=CARTESIAN_POINT('Ctrl Pts',(4.25272260199994,2.2,-0.443878482000013));
#347486=CARTESIAN_POINT('Ctrl Pts',(4.25440646699994,12.2,-0.443427164000014));
#347487=CARTESIAN_POINT('Ctrl Pts',(4.25440646699994,5.2,-0.443427164000014));
#347488=CARTESIAN_POINT('Ctrl Pts',(4.25440646699994,2.2,-0.443427164000014));
#347489=CARTESIAN_POINT('Ctrl Pts',(4.25609405399995,12.2,-0.442972788000016));
#347490=CARTESIAN_POINT('Ctrl Pts',(4.25609405399995,5.2,-0.442972788000016));
#347491=CARTESIAN_POINT('Ctrl Pts',(4.25609405399995,2.2,-0.442972788000016));
#347492=CARTESIAN_POINT('Ctrl Pts',(4.25778535099994,12.2,-0.442515347000012));
#347493=CARTESIAN_POINT('Ctrl Pts',(4.25778535099994,5.2,-0.442515347000012));
#347494=CARTESIAN_POINT('Ctrl Pts',(4.25778535099994,2.2,-0.442515347000012));
#347495=CARTESIAN_POINT('Ctrl Pts',(4.25948034899994,12.2,-0.442054834000012));
#347496=CARTESIAN_POINT('Ctrl Pts',(4.25948034899994,5.2,-0.442054834000012));
#347497=CARTESIAN_POINT('Ctrl Pts',(4.25948034899994,2.2,-0.442054834000012));
#347498=CARTESIAN_POINT('Ctrl Pts',(4.26117903799994,12.2,-0.441591242000015));
#347499=CARTESIAN_POINT('Ctrl Pts',(4.26117903799994,5.2,-0.441591242000015));
#347500=CARTESIAN_POINT('Ctrl Pts',(4.26117903799994,2.2,-0.441591242000015));
#347501=CARTESIAN_POINT('Ctrl Pts',(4.26288140799994,12.2,-0.441124564000015));
#347502=CARTESIAN_POINT('Ctrl Pts',(4.26288140799994,5.2,-0.441124564000015));
#347503=CARTESIAN_POINT('Ctrl Pts',(4.26288140799994,2.2,-0.441124564000015));
#347504=CARTESIAN_POINT('Ctrl Pts',(4.26458744799994,12.2,-0.440654794000017));
#347505=CARTESIAN_POINT('Ctrl Pts',(4.26458744799994,5.2,-0.440654794000017));
#347506=CARTESIAN_POINT('Ctrl Pts',(4.26458744799994,2.2,-0.440654794000017));
#347507=CARTESIAN_POINT('Ctrl Pts',(4.26629714899994,12.2,-0.440181925000012));
#347508=CARTESIAN_POINT('Ctrl Pts',(4.26629714899994,5.2,-0.440181925000012));
#347509=CARTESIAN_POINT('Ctrl Pts',(4.26629714899994,2.2,-0.440181925000012));
#347510=CARTESIAN_POINT('Ctrl Pts',(4.26801050199995,12.2,-0.439705951000011));
#347511=CARTESIAN_POINT('Ctrl Pts',(4.26801050199995,5.2,-0.439705951000011));
#347512=CARTESIAN_POINT('Ctrl Pts',(4.26801050199995,2.2,-0.439705951000011));
#347513=CARTESIAN_POINT('Ctrl Pts',(4.26972749499994,12.2,-0.439226866000015));
#347514=CARTESIAN_POINT('Ctrl Pts',(4.26972749499994,5.2,-0.439226866000015));
#347515=CARTESIAN_POINT('Ctrl Pts',(4.26972749499994,2.2,-0.439226866000015));
#347516=CARTESIAN_POINT('Ctrl Pts',(4.27144811999994,12.2,-0.438744662000015));
#347517=CARTESIAN_POINT('Ctrl Pts',(4.27144811999994,5.2,-0.438744662000015));
#347518=CARTESIAN_POINT('Ctrl Pts',(4.27144811999994,2.2,-0.438744662000015));
#347519=CARTESIAN_POINT('Ctrl Pts',(4.27317236499994,12.2,-0.438259334000013));
#347520=CARTESIAN_POINT('Ctrl Pts',(4.27317236499994,5.2,-0.438259334000013));
#347521=CARTESIAN_POINT('Ctrl Pts',(4.27317236499994,2.2,-0.438259334000013));
#347522=CARTESIAN_POINT('Ctrl Pts',(4.27490022199995,12.2,-0.437770874000014));
#347523=CARTESIAN_POINT('Ctrl Pts',(4.27490022199995,5.2,-0.437770874000014));
#347524=CARTESIAN_POINT('Ctrl Pts',(4.27490022199995,2.2,-0.437770874000014));
#347525=CARTESIAN_POINT('Ctrl Pts',(4.27663167999994,12.2,-0.437279276000013));
#347526=CARTESIAN_POINT('Ctrl Pts',(4.27663167999994,5.2,-0.437279276000013));
#347527=CARTESIAN_POINT('Ctrl Pts',(4.27663167999994,2.2,-0.437279276000013));
#347528=CARTESIAN_POINT('Ctrl Pts',(4.27836672999994,12.2,-0.436784535000014));
#347529=CARTESIAN_POINT('Ctrl Pts',(4.27836672999994,5.2,-0.436784535000014));
#347530=CARTESIAN_POINT('Ctrl Pts',(4.27836672999994,2.2,-0.436784535000014));
#347531=CARTESIAN_POINT('Ctrl Pts',(4.28010536099994,12.2,-0.436286643000017));
#347532=CARTESIAN_POINT('Ctrl Pts',(4.28010536099994,5.2,-0.436286643000017));
#347533=CARTESIAN_POINT('Ctrl Pts',(4.28010536099994,2.2,-0.436286643000017));
#347534=CARTESIAN_POINT('Ctrl Pts',(4.28184756399994,12.2,-0.435785595000016));
#347535=CARTESIAN_POINT('Ctrl Pts',(4.28184756399994,5.2,-0.435785595000016));
#347536=CARTESIAN_POINT('Ctrl Pts',(4.28184756399994,2.2,-0.435785595000016));
#347537=CARTESIAN_POINT('Ctrl Pts',(4.28359332899995,12.2,-0.435281384000015));
#347538=CARTESIAN_POINT('Ctrl Pts',(4.28359332899995,5.2,-0.435281384000015));
#347539=CARTESIAN_POINT('Ctrl Pts',(4.28359332899995,2.2,-0.435281384000015));
#347540=CARTESIAN_POINT('Ctrl Pts',(4.28534264599994,12.2,-0.434774002000013));
#347541=CARTESIAN_POINT('Ctrl Pts',(4.28534264599994,5.2,-0.434774002000013));
#347542=CARTESIAN_POINT('Ctrl Pts',(4.28534264599994,2.2,-0.434774002000013));
#347543=CARTESIAN_POINT('Ctrl Pts',(4.28709550499994,12.2,-0.434263445000016));
#347544=CARTESIAN_POINT('Ctrl Pts',(4.28709550499994,5.2,-0.434263445000016));
#347545=CARTESIAN_POINT('Ctrl Pts',(4.28709550499994,2.2,-0.434263445000016));
#347546=CARTESIAN_POINT('Ctrl Pts',(4.28885189599994,12.2,-0.433749706000013));
#347547=CARTESIAN_POINT('Ctrl Pts',(4.28885189599994,5.2,-0.433749706000013));
#347548=CARTESIAN_POINT('Ctrl Pts',(4.28885189599994,2.2,-0.433749706000013));
#347549=CARTESIAN_POINT('Ctrl Pts',(4.29061181099994,12.2,-0.433232780000012));
#347550=CARTESIAN_POINT('Ctrl Pts',(4.29061181099994,5.2,-0.433232780000012));
#347551=CARTESIAN_POINT('Ctrl Pts',(4.29061181099994,2.2,-0.433232780000012));
#347552=CARTESIAN_POINT('Ctrl Pts',(4.29237523699994,12.2,-0.432712658000014));
#347553=CARTESIAN_POINT('Ctrl Pts',(4.29237523699994,5.2,-0.432712658000014));
#347554=CARTESIAN_POINT('Ctrl Pts',(4.29237523699994,2.2,-0.432712658000014));
#347555=CARTESIAN_POINT('Ctrl Pts',(4.29414216599994,12.2,-0.432189335000013));
#347556=CARTESIAN_POINT('Ctrl Pts',(4.29414216599994,5.2,-0.432189335000013));
#347557=CARTESIAN_POINT('Ctrl Pts',(4.29414216599994,2.2,-0.432189335000013));
#347558=CARTESIAN_POINT('Ctrl Pts',(4.29591258899995,12.2,-0.431662807000013));
#347559=CARTESIAN_POINT('Ctrl Pts',(4.29591258899995,5.2,-0.431662807000013));
#347560=CARTESIAN_POINT('Ctrl Pts',(4.29591258899995,2.2,-0.431662807000013));
#347561=CARTESIAN_POINT('Ctrl Pts',(4.29768649499994,12.2,-0.431133065000013));
#347562=CARTESIAN_POINT('Ctrl Pts',(4.29768649499994,5.2,-0.431133065000013));
#347563=CARTESIAN_POINT('Ctrl Pts',(4.29768649499994,2.2,-0.431133065000013));
#347564=CARTESIAN_POINT('Ctrl Pts',(4.29946387299994,12.2,-0.430600104000014));
#347565=CARTESIAN_POINT('Ctrl Pts',(4.29946387299994,5.2,-0.430600104000014));
#347566=CARTESIAN_POINT('Ctrl Pts',(4.29946387299994,2.2,-0.430600104000014));
#347567=CARTESIAN_POINT('Ctrl Pts',(4.30124471599994,12.2,-0.430063918000014));
#347568=CARTESIAN_POINT('Ctrl Pts',(4.30124471599994,5.2,-0.430063918000014));
#347569=CARTESIAN_POINT('Ctrl Pts',(4.30124471599994,2.2,-0.430063918000014));
#347570=CARTESIAN_POINT('Ctrl Pts',(4.30302901299994,12.2,-0.429524501000014));
#347571=CARTESIAN_POINT('Ctrl Pts',(4.30302901299994,5.2,-0.429524501000014));
#347572=CARTESIAN_POINT('Ctrl Pts',(4.30302901299994,2.2,-0.429524501000014));
#347573=CARTESIAN_POINT('Ctrl Pts',(4.30481675399994,12.2,-0.428981846000016));
#347574=CARTESIAN_POINT('Ctrl Pts',(4.30481675399994,5.2,-0.428981846000016));
#347575=CARTESIAN_POINT('Ctrl Pts',(4.30481675399994,2.2,-0.428981846000016));
#347576=CARTESIAN_POINT('Ctrl Pts',(4.30660792899995,12.2,-0.428435948000012));
#347577=CARTESIAN_POINT('Ctrl Pts',(4.30660792899995,5.2,-0.428435948000012));
#347578=CARTESIAN_POINT('Ctrl Pts',(4.30660792899995,2.2,-0.428435948000012));
#347579=CARTESIAN_POINT('Ctrl Pts',(4.30840252899995,12.2,-0.427886801000015));
#347580=CARTESIAN_POINT('Ctrl Pts',(4.30840252899995,5.2,-0.427886801000015));
#347581=CARTESIAN_POINT('Ctrl Pts',(4.30840252899995,2.2,-0.427886801000015));
#347582=CARTESIAN_POINT('Ctrl Pts',(4.31020054399994,12.2,-0.427334398000014));
#347583=CARTESIAN_POINT('Ctrl Pts',(4.31020054399994,5.2,-0.427334398000014));
#347584=CARTESIAN_POINT('Ctrl Pts',(4.31020054399994,2.2,-0.427334398000014));
#347585=CARTESIAN_POINT('Ctrl Pts',(4.31200196399994,12.2,-0.426778735000015));
#347586=CARTESIAN_POINT('Ctrl Pts',(4.31200196399994,5.2,-0.426778735000015));
#347587=CARTESIAN_POINT('Ctrl Pts',(4.31200196399994,2.2,-0.426778735000015));
#347588=CARTESIAN_POINT('Ctrl Pts',(4.31380677899995,12.2,-0.426219804000016));
#347589=CARTESIAN_POINT('Ctrl Pts',(4.31380677899995,5.2,-0.426219804000016));
#347590=CARTESIAN_POINT('Ctrl Pts',(4.31380677899995,2.2,-0.426219804000016));
#347591=CARTESIAN_POINT('Ctrl Pts',(4.31561497899995,12.2,-0.425657600000013));
#347592=CARTESIAN_POINT('Ctrl Pts',(4.31561497899995,5.2,-0.425657600000013));
#347593=CARTESIAN_POINT('Ctrl Pts',(4.31561497899995,2.2,-0.425657600000013));
#347594=CARTESIAN_POINT('Ctrl Pts',(4.31742655599994,12.2,-0.425092117000014));
#347595=CARTESIAN_POINT('Ctrl Pts',(4.31742655599994,5.2,-0.425092117000014));
#347596=CARTESIAN_POINT('Ctrl Pts',(4.31742655599994,2.2,-0.425092117000014));
#347597=CARTESIAN_POINT('Ctrl Pts',(4.31924149999994,12.2,-0.424523350000015));
#347598=CARTESIAN_POINT('Ctrl Pts',(4.31924149999994,5.2,-0.424523350000015));
#347599=CARTESIAN_POINT('Ctrl Pts',(4.31924149999994,2.2,-0.424523350000015));
#347600=CARTESIAN_POINT('Ctrl Pts',(4.32105979999994,12.2,-0.423951292000013));
#347601=CARTESIAN_POINT('Ctrl Pts',(4.32105979999994,5.2,-0.423951292000013));
#347602=CARTESIAN_POINT('Ctrl Pts',(4.32105979999994,2.2,-0.423951292000013));
#347603=CARTESIAN_POINT('Ctrl Pts',(4.32288144699995,12.2,-0.423375938000015));
#347604=CARTESIAN_POINT('Ctrl Pts',(4.32288144699995,5.2,-0.423375938000015));
#347605=CARTESIAN_POINT('Ctrl Pts',(4.32288144699995,2.2,-0.423375938000015));
#347606=CARTESIAN_POINT('Ctrl Pts',(4.32470643099994,12.2,-0.422797280000013));
#347607=CARTESIAN_POINT('Ctrl Pts',(4.32470643099994,5.2,-0.422797280000013));
#347608=CARTESIAN_POINT('Ctrl Pts',(4.32470643099994,2.2,-0.422797280000013));
#347609=CARTESIAN_POINT('Ctrl Pts',(4.32653474299994,12.2,-0.422215316000014));
#347610=CARTESIAN_POINT('Ctrl Pts',(4.32653474299994,5.2,-0.422215316000014));
#347611=CARTESIAN_POINT('Ctrl Pts',(4.32653474299994,2.2,-0.422215316000014));
#347612=CARTESIAN_POINT('Ctrl Pts',(4.32836637299994,12.2,-0.421630037000016));
#347613=CARTESIAN_POINT('Ctrl Pts',(4.32836637299994,5.2,-0.421630037000016));
#347614=CARTESIAN_POINT('Ctrl Pts',(4.32836637299994,2.2,-0.421630037000016));
#347615=CARTESIAN_POINT('Ctrl Pts',(4.33020131099994,12.2,-0.421041438000014));
#347616=CARTESIAN_POINT('Ctrl Pts',(4.33020131099994,5.2,-0.421041438000014));
#347617=CARTESIAN_POINT('Ctrl Pts',(4.33020131099994,2.2,-0.421041438000014));
#347618=CARTESIAN_POINT('Ctrl Pts',(4.33203954699994,12.2,-0.420449516000012));
#347619=CARTESIAN_POINT('Ctrl Pts',(4.33203954699994,5.2,-0.420449516000012));
#347620=CARTESIAN_POINT('Ctrl Pts',(4.33203954699994,2.2,-0.420449516000012));
#347621=CARTESIAN_POINT('Ctrl Pts',(4.33388107299994,12.2,-0.419854261000014));
#347622=CARTESIAN_POINT('Ctrl Pts',(4.33388107299994,5.2,-0.419854261000014));
#347623=CARTESIAN_POINT('Ctrl Pts',(4.33388107299994,2.2,-0.419854261000014));
#347624=CARTESIAN_POINT('Ctrl Pts',(4.33572587799994,12.2,-0.419255671000016));
#347625=CARTESIAN_POINT('Ctrl Pts',(4.33572587799994,5.2,-0.419255671000016));
#347626=CARTESIAN_POINT('Ctrl Pts',(4.33572587799994,2.2,-0.419255671000016));
#347627=CARTESIAN_POINT('Ctrl Pts',(4.33757395399994,12.2,-0.418653738000017));
#347628=CARTESIAN_POINT('Ctrl Pts',(4.33757395399994,5.2,-0.418653738000017));
#347629=CARTESIAN_POINT('Ctrl Pts',(4.33757395399994,2.2,-0.418653738000017));
#347630=CARTESIAN_POINT('Ctrl Pts',(4.33942528899994,12.2,-0.418048457000015));
#347631=CARTESIAN_POINT('Ctrl Pts',(4.33942528899994,5.2,-0.418048457000015));
#347632=CARTESIAN_POINT('Ctrl Pts',(4.33942528899994,2.2,-0.418048457000015));
#347633=CARTESIAN_POINT('Ctrl Pts',(4.34127987499994,12.2,-0.417439823000016));
#347634=CARTESIAN_POINT('Ctrl Pts',(4.34127987499994,5.2,-0.417439823000016));
#347635=CARTESIAN_POINT('Ctrl Pts',(4.34127987499994,2.2,-0.417439823000016));
#347636=CARTESIAN_POINT('Ctrl Pts',(4.34313770199994,12.2,-0.416827830000015));
#347637=CARTESIAN_POINT('Ctrl Pts',(4.34313770199994,5.2,-0.416827830000015));
#347638=CARTESIAN_POINT('Ctrl Pts',(4.34313770199994,2.2,-0.416827830000015));
#347639=CARTESIAN_POINT('Ctrl Pts',(4.34499875999994,12.2,-0.416212473000015));
#347640=CARTESIAN_POINT('Ctrl Pts',(4.34499875999994,5.2,-0.416212473000015));
#347641=CARTESIAN_POINT('Ctrl Pts',(4.34499875999994,2.2,-0.416212473000015));
#347642=CARTESIAN_POINT('Ctrl Pts',(4.34686303899994,12.2,-0.415593746000016));
#347643=CARTESIAN_POINT('Ctrl Pts',(4.34686303899994,5.2,-0.415593746000016));
#347644=CARTESIAN_POINT('Ctrl Pts',(4.34686303899994,2.2,-0.415593746000016));
#347645=CARTESIAN_POINT('Ctrl Pts',(4.34873053199994,12.2,-0.414971643000013));
#347646=CARTESIAN_POINT('Ctrl Pts',(4.34873053199994,5.2,-0.414971643000013));
#347647=CARTESIAN_POINT('Ctrl Pts',(4.34873053199994,2.2,-0.414971643000013));
#347648=CARTESIAN_POINT('Ctrl Pts',(4.35060122699995,12.2,-0.414346159000014));
#347649=CARTESIAN_POINT('Ctrl Pts',(4.35060122699995,5.2,-0.414346159000014));
#347650=CARTESIAN_POINT('Ctrl Pts',(4.35060122699995,2.2,-0.414346159000014));
#347651=CARTESIAN_POINT('Ctrl Pts',(4.35247511499994,12.2,-0.413717289000015));
#347652=CARTESIAN_POINT('Ctrl Pts',(4.35247511499994,5.2,-0.413717289000015));
#347653=CARTESIAN_POINT('Ctrl Pts',(4.35247511499994,2.2,-0.413717289000015));
#347654=CARTESIAN_POINT('Ctrl Pts',(4.35435218699994,12.2,-0.413085027000015));
#347655=CARTESIAN_POINT('Ctrl Pts',(4.35435218699994,5.2,-0.413085027000015));
#347656=CARTESIAN_POINT('Ctrl Pts',(4.35435218699994,2.2,-0.413085027000015));
#347657=CARTESIAN_POINT('Ctrl Pts',(4.35623243299994,12.2,-0.412449368000014));
#347658=CARTESIAN_POINT('Ctrl Pts',(4.35623243299994,5.2,-0.412449368000014));
#347659=CARTESIAN_POINT('Ctrl Pts',(4.35623243299994,2.2,-0.412449368000014));
#347660=CARTESIAN_POINT('Ctrl Pts',(4.35811584299994,12.2,-0.411810305000015));
#347661=CARTESIAN_POINT('Ctrl Pts',(4.35811584299994,5.2,-0.411810305000015));
#347662=CARTESIAN_POINT('Ctrl Pts',(4.35811584299994,2.2,-0.411810305000015));
#347663=CARTESIAN_POINT('Ctrl Pts',(4.36000240899994,12.2,-0.411167836000015));
#347664=CARTESIAN_POINT('Ctrl Pts',(4.36000240899994,5.2,-0.411167836000015));
#347665=CARTESIAN_POINT('Ctrl Pts',(4.36000240899994,2.2,-0.411167836000015));
#347666=CARTESIAN_POINT('Ctrl Pts',(4.36189211999995,12.2,-0.410521953000016));
#347667=CARTESIAN_POINT('Ctrl Pts',(4.36189211999995,5.2,-0.410521953000016));
#347668=CARTESIAN_POINT('Ctrl Pts',(4.36189211999995,2.2,-0.410521953000016));
#347669=CARTESIAN_POINT('Ctrl Pts',(4.36378496799994,12.2,-0.409872651000014));
#347670=CARTESIAN_POINT('Ctrl Pts',(4.36378496799994,5.2,-0.409872651000014));
#347671=CARTESIAN_POINT('Ctrl Pts',(4.36378496799994,2.2,-0.409872651000014));
#347672=CARTESIAN_POINT('Ctrl Pts',(4.36568093999994,12.2,-0.409219925000013));
#347673=CARTESIAN_POINT('Ctrl Pts',(4.36568093999994,5.2,-0.409219925000013));
#347674=CARTESIAN_POINT('Ctrl Pts',(4.36568093999994,2.2,-0.409219925000013));
#347675=CARTESIAN_POINT('Ctrl Pts',(4.36758003099994,12.2,-0.408563769000012));
#347676=CARTESIAN_POINT('Ctrl Pts',(4.36758003099994,5.2,-0.408563769000012));
#347677=CARTESIAN_POINT('Ctrl Pts',(4.36758003099994,2.2,-0.408563769000012));
#347678=CARTESIAN_POINT('Ctrl Pts',(4.36948222999994,12.2,-0.407904179000016));
#347679=CARTESIAN_POINT('Ctrl Pts',(4.36948222999994,5.2,-0.407904179000016));
#347680=CARTESIAN_POINT('Ctrl Pts',(4.36948222999994,2.2,-0.407904179000016));
#347681=CARTESIAN_POINT('Ctrl Pts',(4.37138752599994,12.2,-0.407241150000015));
#347682=CARTESIAN_POINT('Ctrl Pts',(4.37138752599994,5.2,-0.407241150000015));
#347683=CARTESIAN_POINT('Ctrl Pts',(4.37138752599994,2.2,-0.407241150000015));
#347684=CARTESIAN_POINT('Ctrl Pts',(4.37329590999994,12.2,-0.406574675000013));
#347685=CARTESIAN_POINT('Ctrl Pts',(4.37329590999994,5.2,-0.406574675000013));
#347686=CARTESIAN_POINT('Ctrl Pts',(4.37329590999994,2.2,-0.406574675000013));
#347687=CARTESIAN_POINT('Ctrl Pts',(4.37520737499994,12.2,-0.405904750000015));
#347688=CARTESIAN_POINT('Ctrl Pts',(4.37520737499994,5.2,-0.405904750000015));
#347689=CARTESIAN_POINT('Ctrl Pts',(4.37520737499994,2.2,-0.405904750000015));
#347690=CARTESIAN_POINT('Ctrl Pts',(4.37712190899994,12.2,-0.405231370000014));
#347691=CARTESIAN_POINT('Ctrl Pts',(4.37712190899994,5.2,-0.405231370000014));
#347692=CARTESIAN_POINT('Ctrl Pts',(4.37712190899994,2.2,-0.405231370000014));
#347693=CARTESIAN_POINT('Ctrl Pts',(4.37903950299994,12.2,-0.404554529000016));
#347694=CARTESIAN_POINT('Ctrl Pts',(4.37903950299994,5.2,-0.404554529000016));
#347695=CARTESIAN_POINT('Ctrl Pts',(4.37903950299994,2.2,-0.404554529000016));
#347696=CARTESIAN_POINT('Ctrl Pts',(4.38096014699994,12.2,-0.403874222000016));
#347697=CARTESIAN_POINT('Ctrl Pts',(4.38096014699994,5.2,-0.403874222000016));
#347698=CARTESIAN_POINT('Ctrl Pts',(4.38096014699994,2.2,-0.403874222000016));
#347699=CARTESIAN_POINT('Ctrl Pts',(4.38288383399995,12.2,-0.403190444000017));
#347700=CARTESIAN_POINT('Ctrl Pts',(4.38288383399995,5.2,-0.403190444000017));
#347701=CARTESIAN_POINT('Ctrl Pts',(4.38288383399995,2.2,-0.403190444000017));
#347702=CARTESIAN_POINT('Ctrl Pts',(4.38481055199994,12.2,-0.402503192000014));
#347703=CARTESIAN_POINT('Ctrl Pts',(4.38481055199994,5.2,-0.402503192000014));
#347704=CARTESIAN_POINT('Ctrl Pts',(4.38481055199994,2.2,-0.402503192000014));
#347705=CARTESIAN_POINT('Ctrl Pts',(4.38674029299994,12.2,-0.401812457000013));
#347706=CARTESIAN_POINT('Ctrl Pts',(4.38674029299994,5.2,-0.401812457000013));
#347707=CARTESIAN_POINT('Ctrl Pts',(4.38674029299994,2.2,-0.401812457000013));
#347708=CARTESIAN_POINT('Ctrl Pts',(4.38867304799994,12.2,-0.401118237000015));
#347709=CARTESIAN_POINT('Ctrl Pts',(4.38867304799994,5.2,-0.401118237000015));
#347710=CARTESIAN_POINT('Ctrl Pts',(4.38867304799994,2.2,-0.401118237000015));
#347711=CARTESIAN_POINT('Ctrl Pts',(4.39060880499994,12.2,-0.400420526000014));
#347712=CARTESIAN_POINT('Ctrl Pts',(4.39060880499994,5.2,-0.400420526000014));
#347713=CARTESIAN_POINT('Ctrl Pts',(4.39060880499994,2.2,-0.400420526000014));
#347714=CARTESIAN_POINT('Ctrl Pts',(4.39254755799994,12.2,-0.399719319000016));
#347715=CARTESIAN_POINT('Ctrl Pts',(4.39254755799994,5.2,-0.399719319000016));
#347716=CARTESIAN_POINT('Ctrl Pts',(4.39254755799994,2.2,-0.399719319000016));
#347717=CARTESIAN_POINT('Ctrl Pts',(4.39448929499994,12.2,-0.399014611000013));
#347718=CARTESIAN_POINT('Ctrl Pts',(4.39448929499994,5.2,-0.399014611000013));
#347719=CARTESIAN_POINT('Ctrl Pts',(4.39448929499994,2.2,-0.399014611000013));
#347720=CARTESIAN_POINT('Ctrl Pts',(4.39643400699994,12.2,-0.398306396000017));
#347721=CARTESIAN_POINT('Ctrl Pts',(4.39643400699994,5.2,-0.398306396000017));
#347722=CARTESIAN_POINT('Ctrl Pts',(4.39643400699994,2.2,-0.398306396000017));
#347723=CARTESIAN_POINT('Ctrl Pts',(4.39838168799994,12.2,-0.397594671000014));
#347724=CARTESIAN_POINT('Ctrl Pts',(4.39838168799994,5.2,-0.397594671000014));
#347725=CARTESIAN_POINT('Ctrl Pts',(4.39838168799994,2.2,-0.397594671000014));
#347726=CARTESIAN_POINT('Ctrl Pts',(4.40033232399994,12.2,-0.396879430000014));
#347727=CARTESIAN_POINT('Ctrl Pts',(4.40033232399994,5.2,-0.396879430000014));
#347728=CARTESIAN_POINT('Ctrl Pts',(4.40033232399994,2.2,-0.396879430000014));
#347729=CARTESIAN_POINT('Ctrl Pts',(4.40228590799994,12.2,-0.396160667000016));
#347730=CARTESIAN_POINT('Ctrl Pts',(4.40228590799994,5.2,-0.396160667000016));
#347731=CARTESIAN_POINT('Ctrl Pts',(4.40228590799994,2.2,-0.396160667000016));
#347732=CARTESIAN_POINT('Ctrl Pts',(4.40424242999994,12.2,-0.395438380000015));
#347733=CARTESIAN_POINT('Ctrl Pts',(4.40424242999994,5.2,-0.395438380000015));
#347734=CARTESIAN_POINT('Ctrl Pts',(4.40424242999994,2.2,-0.395438380000015));
#347735=CARTESIAN_POINT('Ctrl Pts',(4.40620187999994,12.2,-0.394712561000015));
#347736=CARTESIAN_POINT('Ctrl Pts',(4.40620187999994,5.2,-0.394712561000015));
#347737=CARTESIAN_POINT('Ctrl Pts',(4.40620187999994,2.2,-0.394712561000015));
#347738=CARTESIAN_POINT('Ctrl Pts',(4.40816425099994,12.2,-0.393983207000015));
#347739=CARTESIAN_POINT('Ctrl Pts',(4.40816425099994,5.2,-0.393983207000015));
#347740=CARTESIAN_POINT('Ctrl Pts',(4.40816425099994,2.2,-0.393983207000015));
#347741=CARTESIAN_POINT('Ctrl Pts',(4.41012953199994,12.2,-0.393250314000015));
#347742=CARTESIAN_POINT('Ctrl Pts',(4.41012953199994,5.2,-0.393250314000015));
#347743=CARTESIAN_POINT('Ctrl Pts',(4.41012953199994,2.2,-0.393250314000015));
#347744=CARTESIAN_POINT('Ctrl Pts',(4.41209771399994,12.2,-0.392513875000016));
#347745=CARTESIAN_POINT('Ctrl Pts',(4.41209771399994,5.2,-0.392513875000016));
#347746=CARTESIAN_POINT('Ctrl Pts',(4.41209771399994,2.2,-0.392513875000016));
#347747=CARTESIAN_POINT('Ctrl Pts',(4.41406878699994,12.2,-0.391773886000015));
#347748=CARTESIAN_POINT('Ctrl Pts',(4.41406878699994,5.2,-0.391773886000015));
#347749=CARTESIAN_POINT('Ctrl Pts',(4.41406878699994,2.2,-0.391773886000015));
#347750=CARTESIAN_POINT('Ctrl Pts',(4.41604274299995,12.2,-0.391030343000014));
#347751=CARTESIAN_POINT('Ctrl Pts',(4.41604274299995,5.2,-0.391030343000014));
#347752=CARTESIAN_POINT('Ctrl Pts',(4.41604274299995,2.2,-0.391030343000014));
#347753=CARTESIAN_POINT('Ctrl Pts',(4.41801957099995,12.2,-0.390283240000016));
#347754=CARTESIAN_POINT('Ctrl Pts',(4.41801957099995,5.2,-0.390283240000016));
#347755=CARTESIAN_POINT('Ctrl Pts',(4.41801957099995,2.2,-0.390283240000016));
#347756=CARTESIAN_POINT('Ctrl Pts',(4.41999926399994,12.2,-0.389532573000011));
#347757=CARTESIAN_POINT('Ctrl Pts',(4.41999926399994,5.2,-0.389532573000011));
#347758=CARTESIAN_POINT('Ctrl Pts',(4.41999926399994,2.2,-0.389532573000011));
#347759=CARTESIAN_POINT('Ctrl Pts',(4.42198181199995,12.2,-0.388778337000013));
#347760=CARTESIAN_POINT('Ctrl Pts',(4.42198181199995,5.2,-0.388778337000013));
#347761=CARTESIAN_POINT('Ctrl Pts',(4.42198181199995,2.2,-0.388778337000013));
#347762=CARTESIAN_POINT('Ctrl Pts',(4.42396720399994,12.2,-0.388020528000013));
#347763=CARTESIAN_POINT('Ctrl Pts',(4.42396720399994,5.2,-0.388020528000013));
#347764=CARTESIAN_POINT('Ctrl Pts',(4.42396720399994,2.2,-0.388020528000013));
#347765=CARTESIAN_POINT('Ctrl Pts',(4.42595543299994,12.2,-0.387259141000014));
#347766=CARTESIAN_POINT('Ctrl Pts',(4.42595543299994,5.2,-0.387259141000014));
#347767=CARTESIAN_POINT('Ctrl Pts',(4.42595543299994,2.2,-0.387259141000014));
#347768=CARTESIAN_POINT('Ctrl Pts',(4.42794648799994,12.2,-0.386494172000016));
#347769=CARTESIAN_POINT('Ctrl Pts',(4.42794648799994,5.2,-0.386494172000016));
#347770=CARTESIAN_POINT('Ctrl Pts',(4.42794648799994,2.2,-0.386494172000016));
#347771=CARTESIAN_POINT('Ctrl Pts',(4.42994036099994,12.2,-0.385725614000014));
#347772=CARTESIAN_POINT('Ctrl Pts',(4.42994036099994,5.2,-0.385725614000014));
#347773=CARTESIAN_POINT('Ctrl Pts',(4.42994036099994,2.2,-0.385725614000014));
#347774=CARTESIAN_POINT('Ctrl Pts',(4.43193704199994,12.2,-0.384953465000013));
#347775=CARTESIAN_POINT('Ctrl Pts',(4.43193704199994,5.2,-0.384953465000013));
#347776=CARTESIAN_POINT('Ctrl Pts',(4.43193704199994,2.2,-0.384953465000013));
#347777=CARTESIAN_POINT('Ctrl Pts',(4.43393652199994,12.2,-0.384177719000016));
#347778=CARTESIAN_POINT('Ctrl Pts',(4.43393652199994,5.2,-0.384177719000016));
#347779=CARTESIAN_POINT('Ctrl Pts',(4.43393652199994,2.2,-0.384177719000016));
#347780=CARTESIAN_POINT('Ctrl Pts',(4.43593879199994,12.2,-0.383398371000014));
#347781=CARTESIAN_POINT('Ctrl Pts',(4.43593879199994,5.2,-0.383398371000014));
#347782=CARTESIAN_POINT('Ctrl Pts',(4.43593879199994,2.2,-0.383398371000014));
#347783=CARTESIAN_POINT('Ctrl Pts',(4.43794384199994,12.2,-0.382615419000012));
#347784=CARTESIAN_POINT('Ctrl Pts',(4.43794384199994,5.2,-0.382615419000012));
#347785=CARTESIAN_POINT('Ctrl Pts',(4.43794384199994,2.2,-0.382615419000012));
#347786=CARTESIAN_POINT('Ctrl Pts',(4.43995166399994,12.2,-0.381828856000013));
#347787=CARTESIAN_POINT('Ctrl Pts',(4.43995166399994,5.2,-0.381828856000013));
#347788=CARTESIAN_POINT('Ctrl Pts',(4.43995166399994,2.2,-0.381828856000013));
#347789=CARTESIAN_POINT('Ctrl Pts',(4.44196224799995,12.2,-0.381038678000016));
#347790=CARTESIAN_POINT('Ctrl Pts',(4.44196224799995,5.2,-0.381038678000016));
#347791=CARTESIAN_POINT('Ctrl Pts',(4.44196224799995,2.2,-0.381038678000016));
#347792=CARTESIAN_POINT('Ctrl Pts',(4.44397558499994,12.2,-0.380244880000014));
#347793=CARTESIAN_POINT('Ctrl Pts',(4.44397558499994,5.2,-0.380244880000014));
#347794=CARTESIAN_POINT('Ctrl Pts',(4.44397558499994,2.2,-0.380244880000014));
#347795=CARTESIAN_POINT('Ctrl Pts',(4.44599166599995,12.2,-0.379447460000013));
#347796=CARTESIAN_POINT('Ctrl Pts',(4.44599166599995,5.2,-0.379447460000013));
#347797=CARTESIAN_POINT('Ctrl Pts',(4.44599166599995,2.2,-0.379447460000013));
#347798=CARTESIAN_POINT('Ctrl Pts',(4.44801048099994,12.2,-0.378646411000014));
#347799=CARTESIAN_POINT('Ctrl Pts',(4.44801048099994,5.2,-0.378646411000014));
#347800=CARTESIAN_POINT('Ctrl Pts',(4.44801048099994,2.2,-0.378646411000014));
#347801=CARTESIAN_POINT('Ctrl Pts',(4.45003202299994,12.2,-0.377841729000017));
#347802=CARTESIAN_POINT('Ctrl Pts',(4.45003202299994,5.2,-0.377841729000017));
#347803=CARTESIAN_POINT('Ctrl Pts',(4.45003202299994,2.2,-0.377841729000017));
#347804=CARTESIAN_POINT('Ctrl Pts',(4.45205627999994,12.2,-0.377033410000016));
#347805=CARTESIAN_POINT('Ctrl Pts',(4.45205627999994,5.2,-0.377033410000016));
#347806=CARTESIAN_POINT('Ctrl Pts',(4.45205627999994,2.2,-0.377033410000016));
#347807=CARTESIAN_POINT('Ctrl Pts',(4.45408324399994,12.2,-0.376221450000016));
#347808=CARTESIAN_POINT('Ctrl Pts',(4.45408324399994,5.2,-0.376221450000016));
#347809=CARTESIAN_POINT('Ctrl Pts',(4.45408324399994,2.2,-0.376221450000016));
#347810=CARTESIAN_POINT('Ctrl Pts',(4.45611290699994,12.2,-0.375405844000016));
#347811=CARTESIAN_POINT('Ctrl Pts',(4.45611290699994,5.2,-0.375405844000016));
#347812=CARTESIAN_POINT('Ctrl Pts',(4.45611290699994,2.2,-0.375405844000016));
#347813=CARTESIAN_POINT('Ctrl Pts',(4.45814525899995,12.2,-0.374586587000016));
#347814=CARTESIAN_POINT('Ctrl Pts',(4.45814525899995,5.2,-0.374586587000016));
#347815=CARTESIAN_POINT('Ctrl Pts',(4.45814525899995,2.2,-0.374586587000016));
#347816=CARTESIAN_POINT('Ctrl Pts',(4.46018028999995,12.2,-0.373763677000016));
#347817=CARTESIAN_POINT('Ctrl Pts',(4.46018028999995,5.2,-0.373763677000016));
#347818=CARTESIAN_POINT('Ctrl Pts',(4.46018028999995,2.2,-0.373763677000016));
#347819=CARTESIAN_POINT('Ctrl Pts',(4.46221799099995,12.2,-0.372937107000015));
#347820=CARTESIAN_POINT('Ctrl Pts',(4.46221799099995,5.2,-0.372937107000015));
#347821=CARTESIAN_POINT('Ctrl Pts',(4.46221799099995,2.2,-0.372937107000015));
#347822=CARTESIAN_POINT('Ctrl Pts',(4.46425835499995,12.2,-0.372106875000018));
#347823=CARTESIAN_POINT('Ctrl Pts',(4.46425835499995,5.2,-0.372106875000018));
#347824=CARTESIAN_POINT('Ctrl Pts',(4.46425835499995,2.2,-0.372106875000018));
#347825=CARTESIAN_POINT('Ctrl Pts',(4.46630137099994,12.2,-0.371272974000014));
#347826=CARTESIAN_POINT('Ctrl Pts',(4.46630137099994,5.2,-0.371272974000014));
#347827=CARTESIAN_POINT('Ctrl Pts',(4.46630137099994,2.2,-0.371272974000014));
#347828=CARTESIAN_POINT('Ctrl Pts',(4.46834702999995,12.2,-0.370435403000013));
#347829=CARTESIAN_POINT('Ctrl Pts',(4.46834702999995,5.2,-0.370435403000013));
#347830=CARTESIAN_POINT('Ctrl Pts',(4.46834702999995,2.2,-0.370435403000013));
#347831=CARTESIAN_POINT('Ctrl Pts',(4.47039532399994,12.2,-0.369594155000015));
#347832=CARTESIAN_POINT('Ctrl Pts',(4.47039532399994,5.2,-0.369594155000015));
#347833=CARTESIAN_POINT('Ctrl Pts',(4.47039532399994,2.2,-0.369594155000015));
#347834=CARTESIAN_POINT('Ctrl Pts',(4.47244624199994,12.2,-0.368749227000014));
#347835=CARTESIAN_POINT('Ctrl Pts',(4.47244624199994,5.2,-0.368749227000014));
#347836=CARTESIAN_POINT('Ctrl Pts',(4.47244624199994,2.2,-0.368749227000014));
#347837=CARTESIAN_POINT('Ctrl Pts',(4.47449977699994,12.2,-0.367900614000014));
#347838=CARTESIAN_POINT('Ctrl Pts',(4.47449977699994,5.2,-0.367900614000014));
#347839=CARTESIAN_POINT('Ctrl Pts',(4.47449977699994,2.2,-0.367900614000014));
#347840=CARTESIAN_POINT('Ctrl Pts',(4.47655591799994,12.2,-0.367048314000016));
#347841=CARTESIAN_POINT('Ctrl Pts',(4.47655591799994,5.2,-0.367048314000016));
#347842=CARTESIAN_POINT('Ctrl Pts',(4.47655591799994,2.2,-0.367048314000016));
#347843=CARTESIAN_POINT('Ctrl Pts',(4.47861465699994,12.2,-0.366192320000014));
#347844=CARTESIAN_POINT('Ctrl Pts',(4.47861465699994,5.2,-0.366192320000014));
#347845=CARTESIAN_POINT('Ctrl Pts',(4.47861465699994,2.2,-0.366192320000014));
#347846=CARTESIAN_POINT('Ctrl Pts',(4.48067598499994,12.2,-0.365332629000013));
#347847=CARTESIAN_POINT('Ctrl Pts',(4.48067598499994,5.2,-0.365332629000013));
#347848=CARTESIAN_POINT('Ctrl Pts',(4.48067598499994,2.2,-0.365332629000013));
#347849=CARTESIAN_POINT('Ctrl Pts',(4.48273989399994,12.2,-0.364469238000016));
#347850=CARTESIAN_POINT('Ctrl Pts',(4.48273989399994,5.2,-0.364469238000016));
#347851=CARTESIAN_POINT('Ctrl Pts',(4.48273989399994,2.2,-0.364469238000016));
#347852=CARTESIAN_POINT('Ctrl Pts',(4.48480637199994,12.2,-0.363602142000015));
#347853=CARTESIAN_POINT('Ctrl Pts',(4.48480637199994,5.2,-0.363602142000015));
#347854=CARTESIAN_POINT('Ctrl Pts',(4.48480637199994,2.2,-0.363602142000015));
#347855=CARTESIAN_POINT('Ctrl Pts',(4.48687541199994,12.2,-0.362731335000017));
#347856=CARTESIAN_POINT('Ctrl Pts',(4.48687541199994,5.2,-0.362731335000017));
#347857=CARTESIAN_POINT('Ctrl Pts',(4.48687541199994,2.2,-0.362731335000017));
#347858=CARTESIAN_POINT('Ctrl Pts',(4.48894700499994,12.2,-0.361856816000015));
#347859=CARTESIAN_POINT('Ctrl Pts',(4.48894700499994,5.2,-0.361856816000015));
#347860=CARTESIAN_POINT('Ctrl Pts',(4.48894700499994,2.2,-0.361856816000015));
#347861=CARTESIAN_POINT('Ctrl Pts',(4.49102114199994,12.2,-0.360978579000015));
#347862=CARTESIAN_POINT('Ctrl Pts',(4.49102114199994,5.2,-0.360978579000015));
#347863=CARTESIAN_POINT('Ctrl Pts',(4.49102114199994,2.2,-0.360978579000015));
#347864=CARTESIAN_POINT('Ctrl Pts',(4.49309781399994,12.2,-0.360096621000014));
#347865=CARTESIAN_POINT('Ctrl Pts',(4.49309781399994,5.2,-0.360096621000014));
#347866=CARTESIAN_POINT('Ctrl Pts',(4.49309781399994,2.2,-0.360096621000014));
#347867=CARTESIAN_POINT('Ctrl Pts',(4.49517701099994,12.2,-0.359210937000016));
#347868=CARTESIAN_POINT('Ctrl Pts',(4.49517701099994,5.2,-0.359210937000016));
#347869=CARTESIAN_POINT('Ctrl Pts',(4.49517701099994,2.2,-0.359210937000016));
#347870=CARTESIAN_POINT('Ctrl Pts',(4.49725872399994,12.2,-0.358321524000011));
#347871=CARTESIAN_POINT('Ctrl Pts',(4.49725872399994,5.2,-0.358321524000011));
#347872=CARTESIAN_POINT('Ctrl Pts',(4.49725872399994,2.2,-0.358321524000011));
#347873=CARTESIAN_POINT('Ctrl Pts',(4.49934294599994,12.2,-0.357428377000013));
#347874=CARTESIAN_POINT('Ctrl Pts',(4.49934294599994,5.2,-0.357428377000013));
#347875=CARTESIAN_POINT('Ctrl Pts',(4.49934294599994,2.2,-0.357428377000013));
#347876=CARTESIAN_POINT('Ctrl Pts',(4.50142966599994,12.2,-0.356531493000016));
#347877=CARTESIAN_POINT('Ctrl Pts',(4.50142966599994,5.2,-0.356531493000016));
#347878=CARTESIAN_POINT('Ctrl Pts',(4.50142966599994,2.2,-0.356531493000016));
#347879=CARTESIAN_POINT('Ctrl Pts',(4.50351887499994,12.2,-0.355630868000016));
#347880=CARTESIAN_POINT('Ctrl Pts',(4.50351887499994,5.2,-0.355630868000016));
#347881=CARTESIAN_POINT('Ctrl Pts',(4.50351887499994,2.2,-0.355630868000016));
#347882=CARTESIAN_POINT('Ctrl Pts',(4.50561056499994,12.2,-0.354726498000013));
#347883=CARTESIAN_POINT('Ctrl Pts',(4.50561056499994,5.2,-0.354726498000013));
#347884=CARTESIAN_POINT('Ctrl Pts',(4.50561056499994,2.2,-0.354726498000013));
#347885=CARTESIAN_POINT('Ctrl Pts',(4.50770472699994,12.2,-0.353818377000015));
#347886=CARTESIAN_POINT('Ctrl Pts',(4.50770472699994,5.2,-0.353818377000015));
#347887=CARTESIAN_POINT('Ctrl Pts',(4.50770472699994,2.2,-0.353818377000015));
#347888=CARTESIAN_POINT('Ctrl Pts',(4.50980135199994,12.2,-0.352906504000017));
#347889=CARTESIAN_POINT('Ctrl Pts',(4.50980135199994,5.2,-0.352906504000017));
#347890=CARTESIAN_POINT('Ctrl Pts',(4.50980135199994,2.2,-0.352906504000017));
#347891=CARTESIAN_POINT('Ctrl Pts',(4.51190043099994,12.2,-0.351990873000014));
#347892=CARTESIAN_POINT('Ctrl Pts',(4.51190043099994,5.2,-0.351990873000014));
#347893=CARTESIAN_POINT('Ctrl Pts',(4.51190043099994,2.2,-0.351990873000014));
#347894=CARTESIAN_POINT('Ctrl Pts',(4.51400195399994,12.2,-0.351071482000016));
#347895=CARTESIAN_POINT('Ctrl Pts',(4.51400195399994,5.2,-0.351071482000016));
#347896=CARTESIAN_POINT('Ctrl Pts',(4.51400195399994,2.2,-0.351071482000016));
#347897=CARTESIAN_POINT('Ctrl Pts',(4.51610591499994,12.2,-0.350148326000017));
#347898=CARTESIAN_POINT('Ctrl Pts',(4.51610591499994,5.2,-0.350148326000017));
#347899=CARTESIAN_POINT('Ctrl Pts',(4.51610591499994,2.2,-0.350148326000017));
#347900=CARTESIAN_POINT('Ctrl Pts',(4.51821229999995,12.2,-0.349221402000013));
#347901=CARTESIAN_POINT('Ctrl Pts',(4.51821229999995,5.2,-0.349221402000013));
#347902=CARTESIAN_POINT('Ctrl Pts',(4.51821229999995,2.2,-0.349221402000013));
#347903=CARTESIAN_POINT('Ctrl Pts',(4.52032110499994,12.2,-0.348290705000016));
#347904=CARTESIAN_POINT('Ctrl Pts',(4.52032110499994,5.2,-0.348290705000016));
#347905=CARTESIAN_POINT('Ctrl Pts',(4.52032110499994,2.2,-0.348290705000016));
#347906=CARTESIAN_POINT('Ctrl Pts',(4.52243231899994,12.2,-0.347356232000013));
#347907=CARTESIAN_POINT('Ctrl Pts',(4.52243231899994,5.2,-0.347356232000013));
#347908=CARTESIAN_POINT('Ctrl Pts',(4.52243231899994,2.2,-0.347356232000013));
#347909=CARTESIAN_POINT('Ctrl Pts',(4.52454593299994,12.2,-0.346417978000013));
#347910=CARTESIAN_POINT('Ctrl Pts',(4.52454593299994,5.2,-0.346417978000013));
#347911=CARTESIAN_POINT('Ctrl Pts',(4.52454593299994,2.2,-0.346417978000013));
#347912=CARTESIAN_POINT('Ctrl Pts',(4.52666193799994,12.2,-0.345475941000015));
#347913=CARTESIAN_POINT('Ctrl Pts',(4.52666193799994,5.2,-0.345475941000015));
#347914=CARTESIAN_POINT('Ctrl Pts',(4.52666193799994,2.2,-0.345475941000015));
#347915=CARTESIAN_POINT('Ctrl Pts',(4.52878032599994,12.2,-0.344530117000015));
#347916=CARTESIAN_POINT('Ctrl Pts',(4.52878032599994,5.2,-0.344530117000015));
#347917=CARTESIAN_POINT('Ctrl Pts',(4.52878032599994,2.2,-0.344530117000015));
#347918=CARTESIAN_POINT('Ctrl Pts',(4.53090108699994,12.2,-0.343580501000016));
#347919=CARTESIAN_POINT('Ctrl Pts',(4.53090108699994,5.2,-0.343580501000016));
#347920=CARTESIAN_POINT('Ctrl Pts',(4.53090108699994,2.2,-0.343580501000016));
#347921=CARTESIAN_POINT('Ctrl Pts',(4.53302421399994,12.2,-0.342627090000014));
#347922=CARTESIAN_POINT('Ctrl Pts',(4.53302421399994,5.2,-0.342627090000014));
#347923=CARTESIAN_POINT('Ctrl Pts',(4.53302421399994,2.2,-0.342627090000014));
#347924=CARTESIAN_POINT('Ctrl Pts',(4.53514969499994,12.2,-0.341669881000013));
#347925=CARTESIAN_POINT('Ctrl Pts',(4.53514969499994,5.2,-0.341669881000013));
#347926=CARTESIAN_POINT('Ctrl Pts',(4.53514969499994,2.2,-0.341669881000013));
#347927=CARTESIAN_POINT('Ctrl Pts',(4.53727752399994,12.2,-0.340708870000017));
#347928=CARTESIAN_POINT('Ctrl Pts',(4.53727752399994,5.2,-0.340708870000017));
#347929=CARTESIAN_POINT('Ctrl Pts',(4.53727752399994,2.2,-0.340708870000017));
#347930=CARTESIAN_POINT('Ctrl Pts',(4.53940769099995,12.2,-0.339744052000013));
#347931=CARTESIAN_POINT('Ctrl Pts',(4.53940769099995,5.2,-0.339744052000013));
#347932=CARTESIAN_POINT('Ctrl Pts',(4.53940769099995,2.2,-0.339744052000013));
#347933=CARTESIAN_POINT('Ctrl Pts',(4.54154018699994,12.2,-0.338775425000013));
#347934=CARTESIAN_POINT('Ctrl Pts',(4.54154018699994,5.2,-0.338775425000013));
#347935=CARTESIAN_POINT('Ctrl Pts',(4.54154018699994,2.2,-0.338775425000013));
#347936=CARTESIAN_POINT('Ctrl Pts',(4.54367500399994,12.2,-0.337802984000017));
#347937=CARTESIAN_POINT('Ctrl Pts',(4.54367500399994,5.2,-0.337802984000017));
#347938=CARTESIAN_POINT('Ctrl Pts',(4.54367500399994,2.2,-0.337802984000017));
#347939=CARTESIAN_POINT('Ctrl Pts',(4.54581213099994,12.2,-0.336826727000012));
#347940=CARTESIAN_POINT('Ctrl Pts',(4.54581213099994,5.2,-0.336826727000012));
#347941=CARTESIAN_POINT('Ctrl Pts',(4.54581213099994,2.2,-0.336826727000012));
#347942=CARTESIAN_POINT('Ctrl Pts',(4.54795156299994,12.2,-0.335846649000011));
#347943=CARTESIAN_POINT('Ctrl Pts',(4.54795156299994,5.2,-0.335846649000011));
#347944=CARTESIAN_POINT('Ctrl Pts',(4.54795156299994,2.2,-0.335846649000011));
#347945=CARTESIAN_POINT('Ctrl Pts',(4.55009328699994,12.2,-0.334862747000013));
#347946=CARTESIAN_POINT('Ctrl Pts',(4.55009328699994,5.2,-0.334862747000013));
#347947=CARTESIAN_POINT('Ctrl Pts',(4.55009328699994,2.2,-0.334862747000013));
#347948=CARTESIAN_POINT('Ctrl Pts',(4.55223729599994,12.2,-0.333875018000014));
#347949=CARTESIAN_POINT('Ctrl Pts',(4.55223729599994,5.2,-0.333875018000014));
#347950=CARTESIAN_POINT('Ctrl Pts',(4.55223729599994,2.2,-0.333875018000014));
#347951=CARTESIAN_POINT('Ctrl Pts',(4.55438358299994,12.2,-0.332883458000013));
#347952=CARTESIAN_POINT('Ctrl Pts',(4.55438358299994,5.2,-0.332883458000013));
#347953=CARTESIAN_POINT('Ctrl Pts',(4.55438358299994,2.2,-0.332883458000013));
#347954=CARTESIAN_POINT('Ctrl Pts',(4.55653213599994,12.2,-0.331888063000014));
#347955=CARTESIAN_POINT('Ctrl Pts',(4.55653213599994,5.2,-0.331888063000014));
#347956=CARTESIAN_POINT('Ctrl Pts',(4.55653213599994,2.2,-0.331888063000014));
#347957=CARTESIAN_POINT('Ctrl Pts',(4.55868294799994,12.2,-0.330888829000013));
#347958=CARTESIAN_POINT('Ctrl Pts',(4.55868294799994,5.2,-0.330888829000013));
#347959=CARTESIAN_POINT('Ctrl Pts',(4.55868294799994,2.2,-0.330888829000013));
#347960=CARTESIAN_POINT('Ctrl Pts',(4.56083600999994,12.2,-0.329885755000014));
#347961=CARTESIAN_POINT('Ctrl Pts',(4.56083600999994,5.2,-0.329885755000014));
#347962=CARTESIAN_POINT('Ctrl Pts',(4.56083600999994,2.2,-0.329885755000014));
#347963=CARTESIAN_POINT('Ctrl Pts',(4.56299131399994,12.2,-0.328878835000013));
#347964=CARTESIAN_POINT('Ctrl Pts',(4.56299131399994,5.2,-0.328878835000013));
#347965=CARTESIAN_POINT('Ctrl Pts',(4.56299131399994,2.2,-0.328878835000013));
#347966=CARTESIAN_POINT('Ctrl Pts',(4.56514884899994,12.2,-0.327868067000012));
#347967=CARTESIAN_POINT('Ctrl Pts',(4.56514884899994,5.2,-0.327868067000012));
#347968=CARTESIAN_POINT('Ctrl Pts',(4.56514884899994,2.2,-0.327868067000012));
#347969=CARTESIAN_POINT('Ctrl Pts',(4.56730860799994,12.2,-0.326853447000013));
#347970=CARTESIAN_POINT('Ctrl Pts',(4.56730860799994,5.2,-0.326853447000013));
#347971=CARTESIAN_POINT('Ctrl Pts',(4.56730860799994,2.2,-0.326853447000013));
#347972=CARTESIAN_POINT('Ctrl Pts',(4.56947058099994,12.2,-0.325834970000014));
#347973=CARTESIAN_POINT('Ctrl Pts',(4.56947058099994,5.2,-0.325834970000014));
#347974=CARTESIAN_POINT('Ctrl Pts',(4.56947058099994,2.2,-0.325834970000014));
#347975=CARTESIAN_POINT('Ctrl Pts',(4.57163476099994,12.2,-0.324812636000011));
#347976=CARTESIAN_POINT('Ctrl Pts',(4.57163476099994,5.2,-0.324812636000011));
#347977=CARTESIAN_POINT('Ctrl Pts',(4.57163476099994,2.2,-0.324812636000011));
#347978=CARTESIAN_POINT('Ctrl Pts',(4.57380113799994,12.2,-0.323786439000013));
#347979=CARTESIAN_POINT('Ctrl Pts',(4.57380113799994,5.2,-0.323786439000013));
#347980=CARTESIAN_POINT('Ctrl Pts',(4.57380113799994,2.2,-0.323786439000013));
#347981=CARTESIAN_POINT('Ctrl Pts',(4.57596970299994,12.2,-0.322756377000015));
#347982=CARTESIAN_POINT('Ctrl Pts',(4.57596970299994,5.2,-0.322756377000015));
#347983=CARTESIAN_POINT('Ctrl Pts',(4.57596970299994,2.2,-0.322756377000015));
#347984=CARTESIAN_POINT('Ctrl Pts',(4.57814044899994,12.2,-0.321722446000017));
#347985=CARTESIAN_POINT('Ctrl Pts',(4.57814044899994,5.2,-0.321722446000017));
#347986=CARTESIAN_POINT('Ctrl Pts',(4.57814044899994,2.2,-0.321722446000017));
#347987=CARTESIAN_POINT('Ctrl Pts',(4.58031336499994,12.2,-0.320684641000017));
#347988=CARTESIAN_POINT('Ctrl Pts',(4.58031336499994,5.2,-0.320684641000017));
#347989=CARTESIAN_POINT('Ctrl Pts',(4.58031336499994,2.2,-0.320684641000017));
#347990=CARTESIAN_POINT('Ctrl Pts',(4.58248844399994,12.2,-0.319642962000017));
#347991=CARTESIAN_POINT('Ctrl Pts',(4.58248844399994,5.2,-0.319642962000017));
#347992=CARTESIAN_POINT('Ctrl Pts',(4.58248844399994,2.2,-0.319642962000017));
#347993=CARTESIAN_POINT('Ctrl Pts',(4.58466567599994,12.2,-0.318597404000016));
#347994=CARTESIAN_POINT('Ctrl Pts',(4.58466567599994,5.2,-0.318597404000016));
#347995=CARTESIAN_POINT('Ctrl Pts',(4.58466567599994,2.2,-0.318597404000016));
#347996=CARTESIAN_POINT('Ctrl Pts',(4.58684505399994,12.2,-0.317547963000013));
#347997=CARTESIAN_POINT('Ctrl Pts',(4.58684505399994,5.2,-0.317547963000013));
#347998=CARTESIAN_POINT('Ctrl Pts',(4.58684505399994,2.2,-0.317547963000013));
#347999=CARTESIAN_POINT('Ctrl Pts',(4.58902656699994,12.2,-0.316494638000013));
#348000=CARTESIAN_POINT('Ctrl Pts',(4.58902656699994,5.2,-0.316494638000013));
#348001=CARTESIAN_POINT('Ctrl Pts',(4.58902656699994,2.2,-0.316494638000013));
#348002=CARTESIAN_POINT('Ctrl Pts',(4.59121020699994,12.2,-0.315437423000016));
#348003=CARTESIAN_POINT('Ctrl Pts',(4.59121020699994,5.2,-0.315437423000016));
#348004=CARTESIAN_POINT('Ctrl Pts',(4.59121020699994,2.2,-0.315437423000016));
#348005=CARTESIAN_POINT('Ctrl Pts',(4.59339596799994,12.2,-0.314376316000011));
#348006=CARTESIAN_POINT('Ctrl Pts',(4.59339596799994,5.2,-0.314376316000011));
#348007=CARTESIAN_POINT('Ctrl Pts',(4.59339596799994,2.2,-0.314376316000011));
#348008=CARTESIAN_POINT('Ctrl Pts',(4.59558383799994,12.2,-0.313311314000018));
#348009=CARTESIAN_POINT('Ctrl Pts',(4.59558383799994,5.2,-0.313311314000018));
#348010=CARTESIAN_POINT('Ctrl Pts',(4.59558383799994,2.2,-0.313311314000018));
#348011=CARTESIAN_POINT('Ctrl Pts',(4.59777380999994,12.2,-0.312242414000017));
#348012=CARTESIAN_POINT('Ctrl Pts',(4.59777380999994,5.2,-0.312242414000017));
#348013=CARTESIAN_POINT('Ctrl Pts',(4.59777380999994,2.2,-0.312242414000017));
#348014=CARTESIAN_POINT('Ctrl Pts',(4.59996587399994,12.2,-0.311169612000013));
#348015=CARTESIAN_POINT('Ctrl Pts',(4.59996587399994,5.2,-0.311169612000013));
#348016=CARTESIAN_POINT('Ctrl Pts',(4.59996587399994,2.2,-0.311169612000013));
#348017=CARTESIAN_POINT('Ctrl Pts',(4.60216002199994,12.2,-0.310092905000015));
#348018=CARTESIAN_POINT('Ctrl Pts',(4.60216002199994,5.2,-0.310092905000015));
#348019=CARTESIAN_POINT('Ctrl Pts',(4.60216002199994,2.2,-0.310092905000015));
#348020=CARTESIAN_POINT('Ctrl Pts',(4.60435624599994,12.2,-0.309012290000013));
#348021=CARTESIAN_POINT('Ctrl Pts',(4.60435624599994,5.2,-0.309012290000013));
#348022=CARTESIAN_POINT('Ctrl Pts',(4.60435624599994,2.2,-0.309012290000013));
#348023=CARTESIAN_POINT('Ctrl Pts',(4.60655453599994,12.2,-0.307927764000016));
#348024=CARTESIAN_POINT('Ctrl Pts',(4.60655453599994,5.2,-0.307927764000016));
#348025=CARTESIAN_POINT('Ctrl Pts',(4.60655453599994,2.2,-0.307927764000016));
#348026=CARTESIAN_POINT('Ctrl Pts',(4.60875488599994,12.2,-0.306839323000014));
#348027=CARTESIAN_POINT('Ctrl Pts',(4.60875488599994,5.2,-0.306839323000014));
#348028=CARTESIAN_POINT('Ctrl Pts',(4.60875488599994,2.2,-0.306839323000014));
#348029=CARTESIAN_POINT('Ctrl Pts',(4.61095728299994,12.2,-0.305746966000013));
#348030=CARTESIAN_POINT('Ctrl Pts',(4.61095728299994,5.2,-0.305746966000013));
#348031=CARTESIAN_POINT('Ctrl Pts',(4.61095728299994,2.2,-0.305746966000013));
#348032=CARTESIAN_POINT('Ctrl Pts',(4.61316172299994,12.2,-0.304650688000017));
#348033=CARTESIAN_POINT('Ctrl Pts',(4.61316172299994,5.2,-0.304650688000017));
#348034=CARTESIAN_POINT('Ctrl Pts',(4.61316172299994,2.2,-0.304650688000017));
#348035=CARTESIAN_POINT('Ctrl Pts',(4.61536819599994,12.2,-0.303550486000015));
#348036=CARTESIAN_POINT('Ctrl Pts',(4.61536819599994,5.2,-0.303550486000015));
#348037=CARTESIAN_POINT('Ctrl Pts',(4.61536819599994,2.2,-0.303550486000015));
#348038=CARTESIAN_POINT('Ctrl Pts',(4.61757669099994,12.2,-0.302446358000013));
#348039=CARTESIAN_POINT('Ctrl Pts',(4.61757669099994,5.2,-0.302446358000013));
#348040=CARTESIAN_POINT('Ctrl Pts',(4.61757669099994,2.2,-0.302446358000013));
#348041=CARTESIAN_POINT('Ctrl Pts',(4.61978720099994,12.2,-0.301338300000014));
#348042=CARTESIAN_POINT('Ctrl Pts',(4.61978720099994,5.2,-0.301338300000014));
#348043=CARTESIAN_POINT('Ctrl Pts',(4.61978720099994,2.2,-0.301338300000014));
#348044=CARTESIAN_POINT('Ctrl Pts',(4.62199971899994,12.2,-0.300226309000013));
#348045=CARTESIAN_POINT('Ctrl Pts',(4.62199971899994,5.2,-0.300226309000013));
#348046=CARTESIAN_POINT('Ctrl Pts',(4.62199971899994,2.2,-0.300226309000013));
#348047=CARTESIAN_POINT('Ctrl Pts',(4.62421423299994,12.2,-0.299110383000016));
#348048=CARTESIAN_POINT('Ctrl Pts',(4.62421423299994,5.2,-0.299110383000016));
#348049=CARTESIAN_POINT('Ctrl Pts',(4.62421423299994,2.2,-0.299110383000016));
#348050=CARTESIAN_POINT('Ctrl Pts',(4.62643073799994,12.2,-0.297990517000013));
#348051=CARTESIAN_POINT('Ctrl Pts',(4.62643073799994,5.2,-0.297990517000013));
#348052=CARTESIAN_POINT('Ctrl Pts',(4.62643073799994,2.2,-0.297990517000013));
#348053=CARTESIAN_POINT('Ctrl Pts',(4.62864922299994,12.2,-0.296866710000017));
#348054=CARTESIAN_POINT('Ctrl Pts',(4.62864922299994,5.2,-0.296866710000017));
#348055=CARTESIAN_POINT('Ctrl Pts',(4.62864922299994,2.2,-0.296866710000017));
#348056=CARTESIAN_POINT('Ctrl Pts',(4.63086967999994,12.2,-0.295738958000014));
#348057=CARTESIAN_POINT('Ctrl Pts',(4.63086967999994,5.2,-0.295738958000014));
#348058=CARTESIAN_POINT('Ctrl Pts',(4.63086967999994,2.2,-0.295738958000014));
#348059=CARTESIAN_POINT('Ctrl Pts',(4.63309210099994,12.2,-0.294607259000017));
#348060=CARTESIAN_POINT('Ctrl Pts',(4.63309210099994,5.2,-0.294607259000017));
#348061=CARTESIAN_POINT('Ctrl Pts',(4.63309210099994,2.2,-0.294607259000017));
#348062=CARTESIAN_POINT('Ctrl Pts',(4.63531647699994,12.2,-0.293471608000013));
#348063=CARTESIAN_POINT('Ctrl Pts',(4.63531647699994,5.2,-0.293471608000013));
#348064=CARTESIAN_POINT('Ctrl Pts',(4.63531647699994,2.2,-0.293471608000013));
#348065=CARTESIAN_POINT('Ctrl Pts',(4.63754279899994,12.2,-0.292332005000016));
#348066=CARTESIAN_POINT('Ctrl Pts',(4.63754279899994,5.2,-0.292332005000016));
#348067=CARTESIAN_POINT('Ctrl Pts',(4.63754279899994,2.2,-0.292332005000016));
#348068=CARTESIAN_POINT('Ctrl Pts',(4.63977105899995,12.2,-0.291188445000015));
#348069=CARTESIAN_POINT('Ctrl Pts',(4.63977105899995,5.2,-0.291188445000015));
#348070=CARTESIAN_POINT('Ctrl Pts',(4.63977105899995,2.2,-0.291188445000015));
#348071=CARTESIAN_POINT('Ctrl Pts',(4.64200124899994,12.2,-0.290040925000015));
#348072=CARTESIAN_POINT('Ctrl Pts',(4.64200124899994,5.2,-0.290040925000015));
#348073=CARTESIAN_POINT('Ctrl Pts',(4.64200124899994,2.2,-0.290040925000015));
#348074=CARTESIAN_POINT('Ctrl Pts',(4.64423335999994,12.2,-0.288889443000016));
#348075=CARTESIAN_POINT('Ctrl Pts',(4.64423335999994,5.2,-0.288889443000016));
#348076=CARTESIAN_POINT('Ctrl Pts',(4.64423335999994,2.2,-0.288889443000016));
#348077=CARTESIAN_POINT('Ctrl Pts',(4.64646738299994,12.2,-0.287733996000017));
#348078=CARTESIAN_POINT('Ctrl Pts',(4.64646738299994,5.2,-0.287733996000017));
#348079=CARTESIAN_POINT('Ctrl Pts',(4.64646738299994,2.2,-0.287733996000017));
#348080=CARTESIAN_POINT('Ctrl Pts',(4.64870330999994,12.2,-0.286574581000014));
#348081=CARTESIAN_POINT('Ctrl Pts',(4.64870330999994,5.2,-0.286574581000014));
#348082=CARTESIAN_POINT('Ctrl Pts',(4.64870330999994,2.2,-0.286574581000014));
#348083=CARTESIAN_POINT('Ctrl Pts',(4.65094113199994,12.2,-0.285411196000016));
#348084=CARTESIAN_POINT('Ctrl Pts',(4.65094113199994,5.2,-0.285411196000016));
#348085=CARTESIAN_POINT('Ctrl Pts',(4.65094113199994,2.2,-0.285411196000016));
#348086=CARTESIAN_POINT('Ctrl Pts',(4.65318083999995,12.2,-0.284243837000013));
#348087=CARTESIAN_POINT('Ctrl Pts',(4.65318083999995,5.2,-0.284243837000013));
#348088=CARTESIAN_POINT('Ctrl Pts',(4.65318083999995,2.2,-0.284243837000013));
#348089=CARTESIAN_POINT('Ctrl Pts',(4.65542242799994,12.2,-0.283072500000014));
#348090=CARTESIAN_POINT('Ctrl Pts',(4.65542242799994,5.2,-0.283072500000014));
#348091=CARTESIAN_POINT('Ctrl Pts',(4.65542242799994,2.2,-0.283072500000014));
#348092=CARTESIAN_POINT('Ctrl Pts',(4.65766588499995,12.2,-0.281897186000015));
#348093=CARTESIAN_POINT('Ctrl Pts',(4.65766588499995,5.2,-0.281897186000015));
#348094=CARTESIAN_POINT('Ctrl Pts',(4.65766588499995,2.2,-0.281897186000015));
#348095=CARTESIAN_POINT('Ctrl Pts',(4.65991120199994,12.2,-0.280717888000015));
#348096=CARTESIAN_POINT('Ctrl Pts',(4.65991120199994,5.2,-0.280717888000015));
#348097=CARTESIAN_POINT('Ctrl Pts',(4.65991120199994,2.2,-0.280717888000015));
#348098=CARTESIAN_POINT('Ctrl Pts',(4.66215837399994,12.2,-0.279534606000014));
#348099=CARTESIAN_POINT('Ctrl Pts',(4.66215837399994,5.2,-0.279534606000014));
#348100=CARTESIAN_POINT('Ctrl Pts',(4.66215837399994,2.2,-0.279534606000014));
#348101=CARTESIAN_POINT('Ctrl Pts',(4.66440738899994,12.2,-0.278347336000015));
#348102=CARTESIAN_POINT('Ctrl Pts',(4.66440738899994,5.2,-0.278347336000015));
#348103=CARTESIAN_POINT('Ctrl Pts',(4.66440738899994,2.2,-0.278347336000015));
#348104=CARTESIAN_POINT('Ctrl Pts',(4.66665823999994,12.2,-0.277156077000011));
#348105=CARTESIAN_POINT('Ctrl Pts',(4.66665823999994,5.2,-0.277156077000011));
#348106=CARTESIAN_POINT('Ctrl Pts',(4.66665823999994,2.2,-0.277156077000011));
#348107=CARTESIAN_POINT('Ctrl Pts',(4.66891091999995,12.2,-0.275960824000014));
#348108=CARTESIAN_POINT('Ctrl Pts',(4.66891091999995,5.2,-0.275960824000014));
#348109=CARTESIAN_POINT('Ctrl Pts',(4.66891091999995,2.2,-0.275960824000014));
#348110=CARTESIAN_POINT('Ctrl Pts',(4.67116541799994,12.2,-0.274761575000015));
#348111=CARTESIAN_POINT('Ctrl Pts',(4.67116541799994,5.2,-0.274761575000015));
#348112=CARTESIAN_POINT('Ctrl Pts',(4.67116541799994,2.2,-0.274761575000015));
#348113=CARTESIAN_POINT('Ctrl Pts',(4.67342172599994,12.2,-0.273558329000014));
#348114=CARTESIAN_POINT('Ctrl Pts',(4.67342172599994,5.2,-0.273558329000014));
#348115=CARTESIAN_POINT('Ctrl Pts',(4.67342172599994,2.2,-0.273558329000014));
#348116=CARTESIAN_POINT('Ctrl Pts',(4.67567983699994,12.2,-0.272351081000015));
#348117=CARTESIAN_POINT('Ctrl Pts',(4.67567983699994,5.2,-0.272351081000015));
#348118=CARTESIAN_POINT('Ctrl Pts',(4.67567983699994,2.2,-0.272351081000015));
#348119=CARTESIAN_POINT('Ctrl Pts',(4.67793973999994,12.2,-0.271139829000013));
#348120=CARTESIAN_POINT('Ctrl Pts',(4.67793973999994,5.2,-0.271139829000013));
#348121=CARTESIAN_POINT('Ctrl Pts',(4.67793973999994,2.2,-0.271139829000013));
#348122=CARTESIAN_POINT('Ctrl Pts',(4.68020142899994,12.2,-0.269924571000013));
#348123=CARTESIAN_POINT('Ctrl Pts',(4.68020142899994,5.2,-0.269924571000013));
#348124=CARTESIAN_POINT('Ctrl Pts',(4.68020142899994,2.2,-0.269924571000013));
#348125=CARTESIAN_POINT('Ctrl Pts',(4.68246489399994,12.2,-0.268705303000014));
#348126=CARTESIAN_POINT('Ctrl Pts',(4.68246489399994,5.2,-0.268705303000014));
#348127=CARTESIAN_POINT('Ctrl Pts',(4.68246489399994,2.2,-0.268705303000014));
#348128=CARTESIAN_POINT('Ctrl Pts',(4.68473012899994,12.2,-0.267482024000016));
#348129=CARTESIAN_POINT('Ctrl Pts',(4.68473012899994,5.2,-0.267482024000016));
#348130=CARTESIAN_POINT('Ctrl Pts',(4.68473012899994,2.2,-0.267482024000016));
#348131=CARTESIAN_POINT('Ctrl Pts',(4.68699712299994,12.2,-0.266254731000015));
#348132=CARTESIAN_POINT('Ctrl Pts',(4.68699712299994,5.2,-0.266254731000015));
#348133=CARTESIAN_POINT('Ctrl Pts',(4.68699712299994,2.2,-0.266254731000015));
#348134=CARTESIAN_POINT('Ctrl Pts',(4.68926586999994,12.2,-0.265023422000015));
#348135=CARTESIAN_POINT('Ctrl Pts',(4.68926586999994,5.2,-0.265023422000015));
#348136=CARTESIAN_POINT('Ctrl Pts',(4.68926586999994,2.2,-0.265023422000015));
#348137=CARTESIAN_POINT('Ctrl Pts',(4.69153635799994,12.2,-0.263788092000015));
#348138=CARTESIAN_POINT('Ctrl Pts',(4.69153635799994,5.2,-0.263788092000015));
#348139=CARTESIAN_POINT('Ctrl Pts',(4.69153635799994,2.2,-0.263788092000015));
#348140=CARTESIAN_POINT('Ctrl Pts',(4.69380858299994,12.2,-0.262548742000015));
#348141=CARTESIAN_POINT('Ctrl Pts',(4.69380858299994,5.2,-0.262548742000015));
#348142=CARTESIAN_POINT('Ctrl Pts',(4.69380858299994,2.2,-0.262548742000015));
#348143=CARTESIAN_POINT('Ctrl Pts',(4.69608253499994,12.2,-0.261305367000015));
#348144=CARTESIAN_POINT('Ctrl Pts',(4.69608253499994,5.2,-0.261305367000015));
#348145=CARTESIAN_POINT('Ctrl Pts',(4.69608253499994,2.2,-0.261305367000015));
#348146=CARTESIAN_POINT('Ctrl Pts',(4.69835820499994,12.2,-0.260057964000016));
#348147=CARTESIAN_POINT('Ctrl Pts',(4.69835820499994,5.2,-0.260057964000016));
#348148=CARTESIAN_POINT('Ctrl Pts',(4.69835820499994,2.2,-0.260057964000016));
#348149=CARTESIAN_POINT('Ctrl Pts',(4.70063558299994,12.2,-0.258806532000015));
#348150=CARTESIAN_POINT('Ctrl Pts',(4.70063558299994,5.2,-0.258806532000015));
#348151=CARTESIAN_POINT('Ctrl Pts',(4.70063558299994,2.2,-0.258806532000015));
#348152=CARTESIAN_POINT('Ctrl Pts',(4.70291466199994,12.2,-0.257551068000015));
#348153=CARTESIAN_POINT('Ctrl Pts',(4.70291466199994,5.2,-0.257551068000015));
#348154=CARTESIAN_POINT('Ctrl Pts',(4.70291466199994,2.2,-0.257551068000015));
#348155=CARTESIAN_POINT('Ctrl Pts',(4.70519543299995,12.2,-0.256291568000013));
#348156=CARTESIAN_POINT('Ctrl Pts',(4.70519543299995,5.2,-0.256291568000013));
#348157=CARTESIAN_POINT('Ctrl Pts',(4.70519543299995,2.2,-0.256291568000013));
#348158=CARTESIAN_POINT('Ctrl Pts',(4.70747788699994,12.2,-0.255028032000015));
#348159=CARTESIAN_POINT('Ctrl Pts',(4.70747788699994,5.2,-0.255028032000015));
#348160=CARTESIAN_POINT('Ctrl Pts',(4.70747788699994,2.2,-0.255028032000015));
#348161=CARTESIAN_POINT('Ctrl Pts',(4.70976201899994,12.2,-0.253760456000016));
#348162=CARTESIAN_POINT('Ctrl Pts',(4.70976201899994,5.2,-0.253760456000016));
#348163=CARTESIAN_POINT('Ctrl Pts',(4.70976201899994,2.2,-0.253760456000016));
#348164=CARTESIAN_POINT('Ctrl Pts',(4.71204781699994,12.2,-0.252488839000016));
#348165=CARTESIAN_POINT('Ctrl Pts',(4.71204781699994,5.2,-0.252488839000016));
#348166=CARTESIAN_POINT('Ctrl Pts',(4.71204781699994,2.2,-0.252488839000016));
#348167=CARTESIAN_POINT('Ctrl Pts',(4.71433527799995,12.2,-0.251213177000014));
#348168=CARTESIAN_POINT('Ctrl Pts',(4.71433527799995,5.2,-0.251213177000014));
#348169=CARTESIAN_POINT('Ctrl Pts',(4.71433527799995,2.2,-0.251213177000014));
#348170=CARTESIAN_POINT('Ctrl Pts',(4.71662439299994,12.2,-0.249933470000014));
#348171=CARTESIAN_POINT('Ctrl Pts',(4.71662439299994,5.2,-0.249933470000014));
#348172=CARTESIAN_POINT('Ctrl Pts',(4.71662439299994,2.2,-0.249933470000014));
#348173=CARTESIAN_POINT('Ctrl Pts',(4.71891515199994,12.2,-0.248649714000013));
#348174=CARTESIAN_POINT('Ctrl Pts',(4.71891515199994,5.2,-0.248649714000013));
#348175=CARTESIAN_POINT('Ctrl Pts',(4.71891515199994,2.2,-0.248649714000013));
#348176=CARTESIAN_POINT('Ctrl Pts',(4.72120754799994,12.2,-0.247361908000014));
#348177=CARTESIAN_POINT('Ctrl Pts',(4.72120754799994,5.2,-0.247361908000014));
#348178=CARTESIAN_POINT('Ctrl Pts',(4.72120754799994,2.2,-0.247361908000014));
#348179=CARTESIAN_POINT('Ctrl Pts',(4.72350156999994,12.2,-0.246070046000018));
#348180=CARTESIAN_POINT('Ctrl Pts',(4.72350156999994,5.2,-0.246070046000018));
#348181=CARTESIAN_POINT('Ctrl Pts',(4.72350156999994,2.2,-0.246070046000018));
#348182=CARTESIAN_POINT('Ctrl Pts',(4.72579720499995,12.2,-0.244774128000014));
#348183=CARTESIAN_POINT('Ctrl Pts',(4.72579720499995,5.2,-0.244774128000014));
#348184=CARTESIAN_POINT('Ctrl Pts',(4.72579720499995,2.2,-0.244774128000014));
#348185=CARTESIAN_POINT('Ctrl Pts',(4.72809444799994,12.2,-0.243474151000012));
#348186=CARTESIAN_POINT('Ctrl Pts',(4.72809444799994,5.2,-0.243474151000012));
#348187=CARTESIAN_POINT('Ctrl Pts',(4.72809444799994,2.2,-0.243474151000012));
#348188=CARTESIAN_POINT('Ctrl Pts',(4.73039328499994,12.2,-0.242170110000015));
#348189=CARTESIAN_POINT('Ctrl Pts',(4.73039328499994,5.2,-0.242170110000015));
#348190=CARTESIAN_POINT('Ctrl Pts',(4.73039328499994,2.2,-0.242170110000015));
#348191=CARTESIAN_POINT('Ctrl Pts',(4.73269371199994,12.2,-0.240862004000015));
#348192=CARTESIAN_POINT('Ctrl Pts',(4.73269371199994,5.2,-0.240862004000015));
#348193=CARTESIAN_POINT('Ctrl Pts',(4.73269371199994,2.2,-0.240862004000015));
#348194=CARTESIAN_POINT('Ctrl Pts',(4.73499571799994,12.2,-0.239549833000012));
#348195=CARTESIAN_POINT('Ctrl Pts',(4.73499571799994,5.2,-0.239549833000012));
#348196=CARTESIAN_POINT('Ctrl Pts',(4.73499571799994,2.2,-0.239549833000012));
#348197=CARTESIAN_POINT('Ctrl Pts',(4.73729930399994,12.2,-0.238233593000015));
#348198=CARTESIAN_POINT('Ctrl Pts',(4.73729930399994,5.2,-0.238233593000015));
#348199=CARTESIAN_POINT('Ctrl Pts',(4.73729930399994,2.2,-0.238233593000015));
#348200=CARTESIAN_POINT('Ctrl Pts',(4.73960446599994,12.2,-0.236913286000018));
#348201=CARTESIAN_POINT('Ctrl Pts',(4.73960446599994,5.2,-0.236913286000018));
#348202=CARTESIAN_POINT('Ctrl Pts',(4.73960446599994,2.2,-0.236913286000018));
#348203=CARTESIAN_POINT('Ctrl Pts',(4.74144985399994,12.2,-0.235853787000018));
#348204=CARTESIAN_POINT('Ctrl Pts',(4.74144985399994,5.2,-0.235853787000018));
#348205=CARTESIAN_POINT('Ctrl Pts',(4.74144985399994,2.2,-0.235853787000018));
#348206=CARTESIAN_POINT('Ctrl Pts',(4.74283460399994,12.2,-0.235057331000017));
#348207=CARTESIAN_POINT('Ctrl Pts',(4.74283460399994,5.2,-0.235057331000017));
#348208=CARTESIAN_POINT('Ctrl Pts',(4.74283460399994,2.2,-0.235057331000017));
#348209=CARTESIAN_POINT('Ctrl Pts',(4.74375808599994,12.2,-0.234525546000013));
#348210=CARTESIAN_POINT('Ctrl Pts',(4.74375808599994,5.2,-0.234525546000013));
#348211=CARTESIAN_POINT('Ctrl Pts',(4.74375808599994,2.2,-0.234525546000013));
#348212=CARTESIAN_POINT('Ctrl Pts',(4.74421990499994,12.2,-0.234259451000014));
#348213=CARTESIAN_POINT('Ctrl Pts',(4.74421990499994,5.2,-0.234259451000014));
#348214=CARTESIAN_POINT('Ctrl Pts',(4.74421990499994,2.2,-0.234259451000014));
#348215=CARTESIAN_POINT('Origin',(3.84237632699994,15.2,-1.08891369700002));
#348216=CARTESIAN_POINT('',(3.48765214499994,2.2,-0.988386318000014));
#348217=CARTESIAN_POINT('',(3.84242569899994,12.2,-1.08892768900001));
#348218=CARTESIAN_POINT('Origin',(-5.66300478732629E-14,15.2,-1.77635683940025E-14));
#348219=CARTESIAN_POINT('',(3.52236167599994,12.2,-1.88224078000002));
#348220=CARTESIAN_POINT('',(3.19715352599995,12.2,-1.70845963700001));
#348221=CARTESIAN_POINT('Ctrl Pts',(4.46529931499995,12.2,-1.61975369200002));
#348222=CARTESIAN_POINT('Ctrl Pts',(4.46529931499995,5.2,-1.61975369200002));
#348223=CARTESIAN_POINT('Ctrl Pts',(4.46529931499995,2.2,-1.61975369200002));
#348224=CARTESIAN_POINT('Ctrl Pts',(4.46497643499994,12.2,-1.61932962500002));
#348225=CARTESIAN_POINT('Ctrl Pts',(4.46497643499994,5.2,-1.61932962500002));
#348226=CARTESIAN_POINT('Ctrl Pts',(4.46497643499994,2.2,-1.61932962500002));
#348227=CARTESIAN_POINT('Ctrl Pts',(4.46433066499995,12.2,-1.61848192700001));
#348228=CARTESIAN_POINT('Ctrl Pts',(4.46433066499995,5.2,-1.61848192700001));
#348229=CARTESIAN_POINT('Ctrl Pts',(4.46433066499995,2.2,-1.61848192700001));
#348230=CARTESIAN_POINT('Ctrl Pts',(4.46336197099995,12.2,-1.61721168800002));
#348231=CARTESIAN_POINT('Ctrl Pts',(4.46336197099995,5.2,-1.61721168800002));
#348232=CARTESIAN_POINT('Ctrl Pts',(4.46336197099995,2.2,-1.61721168800002));
#348233=CARTESIAN_POINT('Ctrl Pts',(4.46207030599994,12.2,-1.61552065300001));
#348234=CARTESIAN_POINT('Ctrl Pts',(4.46207030599994,5.2,-1.61552065300001));
#348235=CARTESIAN_POINT('Ctrl Pts',(4.46207030599994,2.2,-1.61552065300001));
#348236=CARTESIAN_POINT('Ctrl Pts',(4.46045560299994,12.2,-1.61341121800001));
#348237=CARTESIAN_POINT('Ctrl Pts',(4.46045560299994,5.2,-1.61341121800001));
#348238=CARTESIAN_POINT('Ctrl Pts',(4.46045560299994,2.2,-1.61341121800001));
#348239=CARTESIAN_POINT('Ctrl Pts',(4.45884077799994,12.2,-1.61130614500001));
#348240=CARTESIAN_POINT('Ctrl Pts',(4.45884077799994,5.2,-1.61130614500001));
#348241=CARTESIAN_POINT('Ctrl Pts',(4.45884077799994,2.2,-1.61130614500001));
#348242=CARTESIAN_POINT('Ctrl Pts',(4.45722583399994,12.2,-1.60920543300001));
#348243=CARTESIAN_POINT('Ctrl Pts',(4.45722583399994,5.2,-1.60920543300001));
#348244=CARTESIAN_POINT('Ctrl Pts',(4.45722583399994,2.2,-1.60920543300001));
#348245=CARTESIAN_POINT('Ctrl Pts',(4.45561077699994,12.2,-1.60710908300001));
#348246=CARTESIAN_POINT('Ctrl Pts',(4.45561077699994,5.2,-1.60710908300001));
#348247=CARTESIAN_POINT('Ctrl Pts',(4.45561077699994,2.2,-1.60710908300001));
#348248=CARTESIAN_POINT('Ctrl Pts',(4.45399560999994,12.2,-1.60501709500001));
#348249=CARTESIAN_POINT('Ctrl Pts',(4.45399560999994,5.2,-1.60501709500001));
#348250=CARTESIAN_POINT('Ctrl Pts',(4.45399560999994,2.2,-1.60501709500001));
#348251=CARTESIAN_POINT('Ctrl Pts',(4.45238034299994,12.2,-1.60292947100002));
#348252=CARTESIAN_POINT('Ctrl Pts',(4.45238034299994,5.2,-1.60292947100002));
#348253=CARTESIAN_POINT('Ctrl Pts',(4.45238034299994,2.2,-1.60292947100002));
#348254=CARTESIAN_POINT('Ctrl Pts',(4.45076498499995,12.2,-1.60084621100001));
#348255=CARTESIAN_POINT('Ctrl Pts',(4.45076498499995,5.2,-1.60084621100001));
#348256=CARTESIAN_POINT('Ctrl Pts',(4.45076498499995,2.2,-1.60084621100001));
#348257=CARTESIAN_POINT('Ctrl Pts',(4.44914954699995,12.2,-1.59876731800002));
#348258=CARTESIAN_POINT('Ctrl Pts',(4.44914954699995,5.2,-1.59876731800002));
#348259=CARTESIAN_POINT('Ctrl Pts',(4.44914954699995,2.2,-1.59876731800002));
#348260=CARTESIAN_POINT('Ctrl Pts',(4.44753403899994,12.2,-1.59669279200001));
#348261=CARTESIAN_POINT('Ctrl Pts',(4.44753403899994,5.2,-1.59669279200001));
#348262=CARTESIAN_POINT('Ctrl Pts',(4.44753403899994,2.2,-1.59669279200001));
#348263=CARTESIAN_POINT('Ctrl Pts',(4.44591847199994,12.2,-1.59462263400002));
#348264=CARTESIAN_POINT('Ctrl Pts',(4.44591847199994,5.2,-1.59462263400002));
#348265=CARTESIAN_POINT('Ctrl Pts',(4.44591847199994,2.2,-1.59462263400002));
#348266=CARTESIAN_POINT('Ctrl Pts',(4.44430285599995,12.2,-1.59255684700002));
#348267=CARTESIAN_POINT('Ctrl Pts',(4.44430285599995,5.2,-1.59255684700002));
#348268=CARTESIAN_POINT('Ctrl Pts',(4.44430285599995,2.2,-1.59255684700002));
#348269=CARTESIAN_POINT('Ctrl Pts',(4.44268719799994,12.2,-1.59049542900001));
#348270=CARTESIAN_POINT('Ctrl Pts',(4.44268719799994,5.2,-1.59049542900001));
#348271=CARTESIAN_POINT('Ctrl Pts',(4.44268719799994,2.2,-1.59049542900001));
#348272=CARTESIAN_POINT('Ctrl Pts',(4.44107150699994,12.2,-1.58843838400001));
#348273=CARTESIAN_POINT('Ctrl Pts',(4.44107150699994,5.2,-1.58843838400001));
#348274=CARTESIAN_POINT('Ctrl Pts',(4.44107150699994,2.2,-1.58843838400001));
#348275=CARTESIAN_POINT('Ctrl Pts',(4.43945579199994,12.2,-1.58638571200001));
#348276=CARTESIAN_POINT('Ctrl Pts',(4.43945579199994,5.2,-1.58638571200001));
#348277=CARTESIAN_POINT('Ctrl Pts',(4.43945579199994,2.2,-1.58638571200001));
#348278=CARTESIAN_POINT('Ctrl Pts',(4.43784005899994,12.2,-1.58433741300001));
#348279=CARTESIAN_POINT('Ctrl Pts',(4.43784005899994,5.2,-1.58433741300001));
#348280=CARTESIAN_POINT('Ctrl Pts',(4.43784005899994,2.2,-1.58433741300001));
#348281=CARTESIAN_POINT('Ctrl Pts',(4.43622431699994,12.2,-1.58229348700001));
#348282=CARTESIAN_POINT('Ctrl Pts',(4.43622431699994,5.2,-1.58229348700001));
#348283=CARTESIAN_POINT('Ctrl Pts',(4.43622431699994,2.2,-1.58229348700001));
#348284=CARTESIAN_POINT('Ctrl Pts',(4.43460857399994,12.2,-1.58025393700001));
#348285=CARTESIAN_POINT('Ctrl Pts',(4.43460857399994,5.2,-1.58025393700001));
#348286=CARTESIAN_POINT('Ctrl Pts',(4.43460857399994,2.2,-1.58025393700001));
#348287=CARTESIAN_POINT('Ctrl Pts',(4.43299283799994,12.2,-1.57821876300002));
#348288=CARTESIAN_POINT('Ctrl Pts',(4.43299283799994,5.2,-1.57821876300002));
#348289=CARTESIAN_POINT('Ctrl Pts',(4.43299283799994,2.2,-1.57821876300002));
#348290=CARTESIAN_POINT('Ctrl Pts',(4.43137711899994,12.2,-1.57618796700001));
#348291=CARTESIAN_POINT('Ctrl Pts',(4.43137711899994,5.2,-1.57618796700001));
#348292=CARTESIAN_POINT('Ctrl Pts',(4.43137711899994,2.2,-1.57618796700001));
#348293=CARTESIAN_POINT('Ctrl Pts',(4.42976142499994,12.2,-1.57416154700002));
#348294=CARTESIAN_POINT('Ctrl Pts',(4.42976142499994,5.2,-1.57416154700002));
#348295=CARTESIAN_POINT('Ctrl Pts',(4.42976142499994,2.2,-1.57416154700002));
#348296=CARTESIAN_POINT('Ctrl Pts',(4.42814576699995,12.2,-1.57213950800001));
#348297=CARTESIAN_POINT('Ctrl Pts',(4.42814576699995,5.2,-1.57213950800001));
#348298=CARTESIAN_POINT('Ctrl Pts',(4.42814576699995,2.2,-1.57213950800001));
#348299=CARTESIAN_POINT('Ctrl Pts',(4.42653015199994,12.2,-1.57012184800001));
#348300=CARTESIAN_POINT('Ctrl Pts',(4.42653015199994,5.2,-1.57012184800001));
#348301=CARTESIAN_POINT('Ctrl Pts',(4.42653015199994,2.2,-1.57012184800001));
#348302=CARTESIAN_POINT('Ctrl Pts',(4.42491458999995,12.2,-1.56810856900002));
#348303=CARTESIAN_POINT('Ctrl Pts',(4.42491458999995,5.2,-1.56810856900002));
#348304=CARTESIAN_POINT('Ctrl Pts',(4.42491458999995,2.2,-1.56810856900002));
#348305=CARTESIAN_POINT('Ctrl Pts',(4.42329908899994,12.2,-1.56609967300001));
#348306=CARTESIAN_POINT('Ctrl Pts',(4.42329908899994,5.2,-1.56609967300001));
#348307=CARTESIAN_POINT('Ctrl Pts',(4.42329908899994,2.2,-1.56609967300001));
#348308=CARTESIAN_POINT('Ctrl Pts',(4.42168365699994,12.2,-1.56409515800001));
#348309=CARTESIAN_POINT('Ctrl Pts',(4.42168365699994,5.2,-1.56409515800001));
#348310=CARTESIAN_POINT('Ctrl Pts',(4.42168365699994,2.2,-1.56409515800001));
#348311=CARTESIAN_POINT('Ctrl Pts',(4.42006830399994,12.2,-1.56209502700001));
#348312=CARTESIAN_POINT('Ctrl Pts',(4.42006830399994,5.2,-1.56209502700001));
#348313=CARTESIAN_POINT('Ctrl Pts',(4.42006830399994,2.2,-1.56209502700001));
#348314=CARTESIAN_POINT('Ctrl Pts',(4.41845303799994,12.2,-1.56009928000001));
#348315=CARTESIAN_POINT('Ctrl Pts',(4.41845303799994,5.2,-1.56009928000001));
#348316=CARTESIAN_POINT('Ctrl Pts',(4.41845303799994,2.2,-1.56009928000001));
#348317=CARTESIAN_POINT('Ctrl Pts',(4.41683786899994,12.2,-1.55810791900001));
#348318=CARTESIAN_POINT('Ctrl Pts',(4.41683786899994,5.2,-1.55810791900001));
#348319=CARTESIAN_POINT('Ctrl Pts',(4.41683786899994,2.2,-1.55810791900001));
#348320=CARTESIAN_POINT('Ctrl Pts',(4.41522280299994,12.2,-1.55612094300002));
#348321=CARTESIAN_POINT('Ctrl Pts',(4.41522280299994,5.2,-1.55612094300002));
#348322=CARTESIAN_POINT('Ctrl Pts',(4.41522280299994,2.2,-1.55612094300002));
#348323=CARTESIAN_POINT('Ctrl Pts',(4.41360785099994,12.2,-1.55413835300001));
#348324=CARTESIAN_POINT('Ctrl Pts',(4.41360785099994,5.2,-1.55413835300001));
#348325=CARTESIAN_POINT('Ctrl Pts',(4.41360785099994,2.2,-1.55413835300001));
#348326=CARTESIAN_POINT('Ctrl Pts',(4.41199301999994,12.2,-1.55216015100001));
#348327=CARTESIAN_POINT('Ctrl Pts',(4.41199301999994,5.2,-1.55216015100001));
#348328=CARTESIAN_POINT('Ctrl Pts',(4.41199301999994,2.2,-1.55216015100001));
#348329=CARTESIAN_POINT('Ctrl Pts',(4.41037832099994,12.2,-1.55018633800001));
#348330=CARTESIAN_POINT('Ctrl Pts',(4.41037832099994,5.2,-1.55018633800001));
#348331=CARTESIAN_POINT('Ctrl Pts',(4.41037832099994,2.2,-1.55018633800001));
#348332=CARTESIAN_POINT('Ctrl Pts',(4.40876376299994,12.2,-1.54821691400001));
#348333=CARTESIAN_POINT('Ctrl Pts',(4.40876376299994,5.2,-1.54821691400001));
#348334=CARTESIAN_POINT('Ctrl Pts',(4.40876376299994,2.2,-1.54821691400001));
#348335=CARTESIAN_POINT('Ctrl Pts',(4.40714935399994,12.2,-1.54625187900002));
#348336=CARTESIAN_POINT('Ctrl Pts',(4.40714935399994,5.2,-1.54625187900002));
#348337=CARTESIAN_POINT('Ctrl Pts',(4.40714935399994,2.2,-1.54625187900002));
#348338=CARTESIAN_POINT('Ctrl Pts',(4.40553510099994,12.2,-1.54429123500002));
#348339=CARTESIAN_POINT('Ctrl Pts',(4.40553510099994,5.2,-1.54429123500002));
#348340=CARTESIAN_POINT('Ctrl Pts',(4.40553510099994,2.2,-1.54429123500002));
#348341=CARTESIAN_POINT('Ctrl Pts',(4.40392101499994,12.2,-1.54233498200002));
#348342=CARTESIAN_POINT('Ctrl Pts',(4.40392101499994,5.2,-1.54233498200002));
#348343=CARTESIAN_POINT('Ctrl Pts',(4.40392101499994,2.2,-1.54233498200002));
#348344=CARTESIAN_POINT('Ctrl Pts',(4.40230710599994,12.2,-1.54038312200001));
#348345=CARTESIAN_POINT('Ctrl Pts',(4.40230710599994,5.2,-1.54038312200001));
#348346=CARTESIAN_POINT('Ctrl Pts',(4.40230710599994,2.2,-1.54038312200001));
#348347=CARTESIAN_POINT('Ctrl Pts',(4.40069337999994,12.2,-1.53843565400001));
#348348=CARTESIAN_POINT('Ctrl Pts',(4.40069337999994,5.2,-1.53843565400001));
#348349=CARTESIAN_POINT('Ctrl Pts',(4.40069337999994,2.2,-1.53843565400001));
#348350=CARTESIAN_POINT('Ctrl Pts',(4.39907984799994,12.2,-1.53649258000002));
#348351=CARTESIAN_POINT('Ctrl Pts',(4.39907984799994,5.2,-1.53649258000002));
#348352=CARTESIAN_POINT('Ctrl Pts',(4.39907984799994,2.2,-1.53649258000002));
#348353=CARTESIAN_POINT('Ctrl Pts',(4.39746651799994,12.2,-1.53455390100001));
#348354=CARTESIAN_POINT('Ctrl Pts',(4.39746651799994,5.2,-1.53455390100001));
#348355=CARTESIAN_POINT('Ctrl Pts',(4.39746651799994,2.2,-1.53455390100001));
#348356=CARTESIAN_POINT('Ctrl Pts',(4.39585339899994,12.2,-1.53261961500001));
#348357=CARTESIAN_POINT('Ctrl Pts',(4.39585339899994,5.2,-1.53261961500001));
#348358=CARTESIAN_POINT('Ctrl Pts',(4.39585339899994,2.2,-1.53261961500001));
#348359=CARTESIAN_POINT('Ctrl Pts',(4.39424049999994,12.2,-1.53068972600002));
#348360=CARTESIAN_POINT('Ctrl Pts',(4.39424049999994,5.2,-1.53068972600002));
#348361=CARTESIAN_POINT('Ctrl Pts',(4.39424049999994,2.2,-1.53068972600002));
#348362=CARTESIAN_POINT('Ctrl Pts',(4.39262782999994,12.2,-1.52876423300001));
#348363=CARTESIAN_POINT('Ctrl Pts',(4.39262782999994,5.2,-1.52876423300001));
#348364=CARTESIAN_POINT('Ctrl Pts',(4.39262782999994,2.2,-1.52876423300001));
#348365=CARTESIAN_POINT('Ctrl Pts',(4.39101539899994,12.2,-1.52684313600002));
#348366=CARTESIAN_POINT('Ctrl Pts',(4.39101539899994,5.2,-1.52684313600002));
#348367=CARTESIAN_POINT('Ctrl Pts',(4.39101539899994,2.2,-1.52684313600002));
#348368=CARTESIAN_POINT('Ctrl Pts',(4.38940321399994,12.2,-1.52492643700001));
#348369=CARTESIAN_POINT('Ctrl Pts',(4.38940321399994,5.2,-1.52492643700001));
#348370=CARTESIAN_POINT('Ctrl Pts',(4.38940321399994,2.2,-1.52492643700001));
#348371=CARTESIAN_POINT('Ctrl Pts',(4.38779128499994,12.2,-1.52301413600001));
#348372=CARTESIAN_POINT('Ctrl Pts',(4.38779128499994,5.2,-1.52301413600001));
#348373=CARTESIAN_POINT('Ctrl Pts',(4.38779128499994,2.2,-1.52301413600001));
#348374=CARTESIAN_POINT('Ctrl Pts',(4.38617962199995,12.2,-1.52110623500001));
#348375=CARTESIAN_POINT('Ctrl Pts',(4.38617962199995,5.2,-1.52110623500001));
#348376=CARTESIAN_POINT('Ctrl Pts',(4.38617962199995,2.2,-1.52110623500001));
#348377=CARTESIAN_POINT('Ctrl Pts',(4.38456823199994,12.2,-1.51920273300002));
#348378=CARTESIAN_POINT('Ctrl Pts',(4.38456823199994,5.2,-1.51920273300002));
#348379=CARTESIAN_POINT('Ctrl Pts',(4.38456823199994,2.2,-1.51920273300002));
#348380=CARTESIAN_POINT('Ctrl Pts',(4.38295712499994,12.2,-1.51730363000001));
#348381=CARTESIAN_POINT('Ctrl Pts',(4.38295712499994,5.2,-1.51730363000001));
#348382=CARTESIAN_POINT('Ctrl Pts',(4.38295712499994,2.2,-1.51730363000001));
#348383=CARTESIAN_POINT('Ctrl Pts',(4.38134631099994,12.2,-1.51540892800002));
#348384=CARTESIAN_POINT('Ctrl Pts',(4.38134631099994,5.2,-1.51540892800002));
#348385=CARTESIAN_POINT('Ctrl Pts',(4.38134631099994,2.2,-1.51540892800002));
#348386=CARTESIAN_POINT('Ctrl Pts',(4.37973579799994,12.2,-1.51351862700002));
#348387=CARTESIAN_POINT('Ctrl Pts',(4.37973579799994,5.2,-1.51351862700002));
#348388=CARTESIAN_POINT('Ctrl Pts',(4.37973579799994,2.2,-1.51351862700002));
#348389=CARTESIAN_POINT('Ctrl Pts',(4.37812559599995,12.2,-1.51163272800002));
#348390=CARTESIAN_POINT('Ctrl Pts',(4.37812559599995,5.2,-1.51163272800002));
#348391=CARTESIAN_POINT('Ctrl Pts',(4.37812559599995,2.2,-1.51163272800002));
#348392=CARTESIAN_POINT('Ctrl Pts',(4.37651571199994,12.2,-1.50975123100002));
#348393=CARTESIAN_POINT('Ctrl Pts',(4.37651571199994,5.2,-1.50975123100002));
#348394=CARTESIAN_POINT('Ctrl Pts',(4.37651571199994,2.2,-1.50975123100002));
#348395=CARTESIAN_POINT('Ctrl Pts',(4.37490615699994,12.2,-1.50787413700002));
#348396=CARTESIAN_POINT('Ctrl Pts',(4.37490615699994,5.2,-1.50787413700002));
#348397=CARTESIAN_POINT('Ctrl Pts',(4.37490615699994,2.2,-1.50787413700002));
#348398=CARTESIAN_POINT('Ctrl Pts',(4.37329693899995,12.2,-1.50600144600002));
#348399=CARTESIAN_POINT('Ctrl Pts',(4.37329693899995,5.2,-1.50600144600002));
#348400=CARTESIAN_POINT('Ctrl Pts',(4.37329693899995,2.2,-1.50600144600002));
#348401=CARTESIAN_POINT('Ctrl Pts',(4.37168806799995,12.2,-1.50413316000002));
#348402=CARTESIAN_POINT('Ctrl Pts',(4.37168806799995,5.2,-1.50413316000002));
#348403=CARTESIAN_POINT('Ctrl Pts',(4.37168806799995,2.2,-1.50413316000002));
#348404=CARTESIAN_POINT('Ctrl Pts',(4.37007955299994,12.2,-1.50226927600002));
#348405=CARTESIAN_POINT('Ctrl Pts',(4.37007955299994,5.2,-1.50226927600002));
#348406=CARTESIAN_POINT('Ctrl Pts',(4.37007955299994,2.2,-1.50226927600002));
#348407=CARTESIAN_POINT('Ctrl Pts',(4.36847140299994,12.2,-1.50040979900002));
#348408=CARTESIAN_POINT('Ctrl Pts',(4.36847140299994,5.2,-1.50040979900002));
#348409=CARTESIAN_POINT('Ctrl Pts',(4.36847140299994,2.2,-1.50040979900002));
#348410=CARTESIAN_POINT('Ctrl Pts',(4.36686362699994,12.2,-1.49855472700001));
#348411=CARTESIAN_POINT('Ctrl Pts',(4.36686362699994,5.2,-1.49855472700001));
#348412=CARTESIAN_POINT('Ctrl Pts',(4.36686362699994,2.2,-1.49855472700001));
#348413=CARTESIAN_POINT('Ctrl Pts',(4.36525623399994,12.2,-1.49670406000002));
#348414=CARTESIAN_POINT('Ctrl Pts',(4.36525623399994,5.2,-1.49670406000002));
#348415=CARTESIAN_POINT('Ctrl Pts',(4.36525623399994,2.2,-1.49670406000002));
#348416=CARTESIAN_POINT('Ctrl Pts',(4.36364923399994,12.2,-1.49485779900001));
#348417=CARTESIAN_POINT('Ctrl Pts',(4.36364923399994,5.2,-1.49485779900001));
#348418=CARTESIAN_POINT('Ctrl Pts',(4.36364923399994,2.2,-1.49485779900001));
#348419=CARTESIAN_POINT('Ctrl Pts',(4.36204263499994,12.2,-1.49301594600002));
#348420=CARTESIAN_POINT('Ctrl Pts',(4.36204263499994,5.2,-1.49301594600002));
#348421=CARTESIAN_POINT('Ctrl Pts',(4.36204263499994,2.2,-1.49301594600002));
#348422=CARTESIAN_POINT('Ctrl Pts',(4.36043644699994,12.2,-1.49117849900001));
#348423=CARTESIAN_POINT('Ctrl Pts',(4.36043644699994,5.2,-1.49117849900001));
#348424=CARTESIAN_POINT('Ctrl Pts',(4.36043644699994,2.2,-1.49117849900001));
#348425=CARTESIAN_POINT('Ctrl Pts',(4.35883067899994,12.2,-1.48934546000001));
#348426=CARTESIAN_POINT('Ctrl Pts',(4.35883067899994,5.2,-1.48934546000001));
#348427=CARTESIAN_POINT('Ctrl Pts',(4.35883067899994,2.2,-1.48934546000001));
#348428=CARTESIAN_POINT('Ctrl Pts',(4.35722534099994,12.2,-1.48751682800001));
#348429=CARTESIAN_POINT('Ctrl Pts',(4.35722534099994,5.2,-1.48751682800001));
#348430=CARTESIAN_POINT('Ctrl Pts',(4.35722534099994,2.2,-1.48751682800001));
#348431=CARTESIAN_POINT('Ctrl Pts',(4.35562043999994,12.2,-1.48569260600001));
#348432=CARTESIAN_POINT('Ctrl Pts',(4.35562043999994,5.2,-1.48569260600001));
#348433=CARTESIAN_POINT('Ctrl Pts',(4.35562043999994,2.2,-1.48569260600001));
#348434=CARTESIAN_POINT('Ctrl Pts',(4.35401598799994,12.2,-1.48387279100001));
#348435=CARTESIAN_POINT('Ctrl Pts',(4.35401598799994,5.2,-1.48387279100001));
#348436=CARTESIAN_POINT('Ctrl Pts',(4.35401598799994,2.2,-1.48387279100001));
#348437=CARTESIAN_POINT('Ctrl Pts',(4.35241199299994,12.2,-1.48205738700002));
#348438=CARTESIAN_POINT('Ctrl Pts',(4.35241199299994,5.2,-1.48205738700002));
#348439=CARTESIAN_POINT('Ctrl Pts',(4.35241199299994,2.2,-1.48205738700002));
#348440=CARTESIAN_POINT('Ctrl Pts',(4.35080846399994,12.2,-1.48024639000001));
#348441=CARTESIAN_POINT('Ctrl Pts',(4.35080846399994,5.2,-1.48024639000001));
#348442=CARTESIAN_POINT('Ctrl Pts',(4.35080846399994,2.2,-1.48024639000001));
#348443=CARTESIAN_POINT('Ctrl Pts',(4.34920541099994,12.2,-1.47843980500001));
#348444=CARTESIAN_POINT('Ctrl Pts',(4.34920541099994,5.2,-1.47843980500001));
#348445=CARTESIAN_POINT('Ctrl Pts',(4.34920541099994,2.2,-1.47843980500001));
#348446=CARTESIAN_POINT('Ctrl Pts',(4.34760284299994,12.2,-1.47663762900001));
#348447=CARTESIAN_POINT('Ctrl Pts',(4.34760284299994,5.2,-1.47663762900001));
#348448=CARTESIAN_POINT('Ctrl Pts',(4.34760284299994,2.2,-1.47663762900001));
#348449=CARTESIAN_POINT('Ctrl Pts',(4.34600076899994,12.2,-1.47483986400001));
#348450=CARTESIAN_POINT('Ctrl Pts',(4.34600076899994,5.2,-1.47483986400001));
#348451=CARTESIAN_POINT('Ctrl Pts',(4.34600076899994,2.2,-1.47483986400001));
#348452=CARTESIAN_POINT('Ctrl Pts',(4.34439919799994,12.2,-1.47304650900002));
#348453=CARTESIAN_POINT('Ctrl Pts',(4.34439919799994,5.2,-1.47304650900002));
#348454=CARTESIAN_POINT('Ctrl Pts',(4.34439919799994,2.2,-1.47304650900002));
#348455=CARTESIAN_POINT('Ctrl Pts',(4.34279813999995,12.2,-1.47125756500001));
#348456=CARTESIAN_POINT('Ctrl Pts',(4.34279813999995,5.2,-1.47125756500001));
#348457=CARTESIAN_POINT('Ctrl Pts',(4.34279813999995,2.2,-1.47125756500001));
#348458=CARTESIAN_POINT('Ctrl Pts',(4.34119760499994,12.2,-1.46947303300001));
#348459=CARTESIAN_POINT('Ctrl Pts',(4.34119760499994,5.2,-1.46947303300001));
#348460=CARTESIAN_POINT('Ctrl Pts',(4.34119760499994,2.2,-1.46947303300001));
#348461=CARTESIAN_POINT('Ctrl Pts',(4.33959760099994,12.2,-1.46769291200001));
#348462=CARTESIAN_POINT('Ctrl Pts',(4.33959760099994,5.2,-1.46769291200001));
#348463=CARTESIAN_POINT('Ctrl Pts',(4.33959760099994,2.2,-1.46769291200001));
#348464=CARTESIAN_POINT('Ctrl Pts',(4.33799813899994,12.2,-1.46591720300002));
#348465=CARTESIAN_POINT('Ctrl Pts',(4.33799813899994,5.2,-1.46591720300002));
#348466=CARTESIAN_POINT('Ctrl Pts',(4.33799813899994,2.2,-1.46591720300002));
#348467=CARTESIAN_POINT('Ctrl Pts',(4.33639922599994,12.2,-1.46414590600001));
#348468=CARTESIAN_POINT('Ctrl Pts',(4.33639922599994,5.2,-1.46414590600001));
#348469=CARTESIAN_POINT('Ctrl Pts',(4.33639922599994,2.2,-1.46414590600001));
#348470=CARTESIAN_POINT('Ctrl Pts',(4.33480087399994,12.2,-1.46237902200001));
#348471=CARTESIAN_POINT('Ctrl Pts',(4.33480087399994,5.2,-1.46237902200001));
#348472=CARTESIAN_POINT('Ctrl Pts',(4.33480087399994,2.2,-1.46237902200001));
#348473=CARTESIAN_POINT('Ctrl Pts',(4.33320308999994,12.2,-1.46061655000001));
#348474=CARTESIAN_POINT('Ctrl Pts',(4.33320308999994,5.2,-1.46061655000001));
#348475=CARTESIAN_POINT('Ctrl Pts',(4.33320308999994,2.2,-1.46061655000001));
#348476=CARTESIAN_POINT('Ctrl Pts',(4.33160588499994,12.2,-1.45885849100001));
#348477=CARTESIAN_POINT('Ctrl Pts',(4.33160588499994,5.2,-1.45885849100001));
#348478=CARTESIAN_POINT('Ctrl Pts',(4.33160588499994,2.2,-1.45885849100001));
#348479=CARTESIAN_POINT('Ctrl Pts',(4.33000926899994,12.2,-1.45710484400002));
#348480=CARTESIAN_POINT('Ctrl Pts',(4.33000926899994,5.2,-1.45710484400002));
#348481=CARTESIAN_POINT('Ctrl Pts',(4.33000926899994,2.2,-1.45710484400002));
#348482=CARTESIAN_POINT('Ctrl Pts',(4.32841324999994,12.2,-1.45535561100001));
#348483=CARTESIAN_POINT('Ctrl Pts',(4.32841324999994,5.2,-1.45535561100001));
#348484=CARTESIAN_POINT('Ctrl Pts',(4.32841324999994,2.2,-1.45535561100001));
#348485=CARTESIAN_POINT('Ctrl Pts',(4.32681783699994,12.2,-1.45361079200002));
#348486=CARTESIAN_POINT('Ctrl Pts',(4.32681783699994,5.2,-1.45361079200002));
#348487=CARTESIAN_POINT('Ctrl Pts',(4.32681783699994,2.2,-1.45361079200002));
#348488=CARTESIAN_POINT('Ctrl Pts',(4.32522304199995,12.2,-1.45187038500001));
#348489=CARTESIAN_POINT('Ctrl Pts',(4.32522304199995,5.2,-1.45187038500001));
#348490=CARTESIAN_POINT('Ctrl Pts',(4.32522304199995,2.2,-1.45187038500001));
#348491=CARTESIAN_POINT('Ctrl Pts',(4.32362887299994,12.2,-1.45013439300001));
#348492=CARTESIAN_POINT('Ctrl Pts',(4.32362887299994,5.2,-1.45013439300001));
#348493=CARTESIAN_POINT('Ctrl Pts',(4.32362887299994,2.2,-1.45013439300001));
#348494=CARTESIAN_POINT('Ctrl Pts',(4.32203533899994,12.2,-1.44840281300001));
#348495=CARTESIAN_POINT('Ctrl Pts',(4.32203533899994,5.2,-1.44840281300001));
#348496=CARTESIAN_POINT('Ctrl Pts',(4.32203533899994,2.2,-1.44840281300001));
#348497=CARTESIAN_POINT('Ctrl Pts',(4.32044244999994,12.2,-1.44667564900002));
#348498=CARTESIAN_POINT('Ctrl Pts',(4.32044244999994,5.2,-1.44667564900002));
#348499=CARTESIAN_POINT('Ctrl Pts',(4.32044244999994,2.2,-1.44667564900002));
#348500=CARTESIAN_POINT('Ctrl Pts',(4.31885021599994,12.2,-1.44495289700002));
#348501=CARTESIAN_POINT('Ctrl Pts',(4.31885021599994,5.2,-1.44495289700002));
#348502=CARTESIAN_POINT('Ctrl Pts',(4.31885021599994,2.2,-1.44495289700002));
#348503=CARTESIAN_POINT('Ctrl Pts',(4.31725864499994,12.2,-1.44323456000001));
#348504=CARTESIAN_POINT('Ctrl Pts',(4.31725864499994,5.2,-1.44323456000001));
#348505=CARTESIAN_POINT('Ctrl Pts',(4.31725864499994,2.2,-1.44323456000001));
#348506=CARTESIAN_POINT('Ctrl Pts',(4.31566774799994,12.2,-1.44152063700002));
#348507=CARTESIAN_POINT('Ctrl Pts',(4.31566774799994,5.2,-1.44152063700002));
#348508=CARTESIAN_POINT('Ctrl Pts',(4.31566774799994,2.2,-1.44152063700002));
#348509=CARTESIAN_POINT('Ctrl Pts',(4.31407753499994,12.2,-1.43981112800001));
#348510=CARTESIAN_POINT('Ctrl Pts',(4.31407753499994,5.2,-1.43981112800001));
#348511=CARTESIAN_POINT('Ctrl Pts',(4.31407753499994,2.2,-1.43981112800001));
#348512=CARTESIAN_POINT('Ctrl Pts',(4.31248801499994,12.2,-1.43810603400001));
#348513=CARTESIAN_POINT('Ctrl Pts',(4.31248801499994,5.2,-1.43810603400001));
#348514=CARTESIAN_POINT('Ctrl Pts',(4.31248801499994,2.2,-1.43810603400001));
#348515=CARTESIAN_POINT('Ctrl Pts',(4.31089919699994,12.2,-1.43640535400001));
#348516=CARTESIAN_POINT('Ctrl Pts',(4.31089919699994,5.2,-1.43640535400001));
#348517=CARTESIAN_POINT('Ctrl Pts',(4.31089919699994,2.2,-1.43640535400001));
#348518=CARTESIAN_POINT('Ctrl Pts',(4.30931109099994,12.2,-1.43470908800001));
#348519=CARTESIAN_POINT('Ctrl Pts',(4.30931109099994,5.2,-1.43470908800001));
#348520=CARTESIAN_POINT('Ctrl Pts',(4.30931109099994,2.2,-1.43470908800001));
#348521=CARTESIAN_POINT('Ctrl Pts',(4.30772370599994,12.2,-1.43301723600001));
#348522=CARTESIAN_POINT('Ctrl Pts',(4.30772370599994,5.2,-1.43301723600001));
#348523=CARTESIAN_POINT('Ctrl Pts',(4.30772370599994,2.2,-1.43301723600001));
#348524=CARTESIAN_POINT('Ctrl Pts',(4.30613705299994,12.2,-1.43132979900002));
#348525=CARTESIAN_POINT('Ctrl Pts',(4.30613705299994,5.2,-1.43132979900002));
#348526=CARTESIAN_POINT('Ctrl Pts',(4.30613705299994,2.2,-1.43132979900002));
#348527=CARTESIAN_POINT('Ctrl Pts',(4.30455114099995,12.2,-1.42964677700002));
#348528=CARTESIAN_POINT('Ctrl Pts',(4.30455114099995,5.2,-1.42964677700002));
#348529=CARTESIAN_POINT('Ctrl Pts',(4.30455114099995,2.2,-1.42964677700002));
#348530=CARTESIAN_POINT('Ctrl Pts',(4.30296597899994,12.2,-1.42796816700002));
#348531=CARTESIAN_POINT('Ctrl Pts',(4.30296597899994,5.2,-1.42796816700002));
#348532=CARTESIAN_POINT('Ctrl Pts',(4.30296597899994,2.2,-1.42796816700002));
#348533=CARTESIAN_POINT('Ctrl Pts',(4.30138157799994,12.2,-1.42629397300002));
#348534=CARTESIAN_POINT('Ctrl Pts',(4.30138157799994,5.2,-1.42629397300002));
#348535=CARTESIAN_POINT('Ctrl Pts',(4.30138157799994,2.2,-1.42629397300002));
#348536=CARTESIAN_POINT('Ctrl Pts',(4.29979794699994,12.2,-1.42462419400001));
#348537=CARTESIAN_POINT('Ctrl Pts',(4.29979794699994,5.2,-1.42462419400001));
#348538=CARTESIAN_POINT('Ctrl Pts',(4.29979794699994,2.2,-1.42462419400001));
#348539=CARTESIAN_POINT('Ctrl Pts',(4.29821509599994,12.2,-1.42295882700001));
#348540=CARTESIAN_POINT('Ctrl Pts',(4.29821509599994,5.2,-1.42295882700001));
#348541=CARTESIAN_POINT('Ctrl Pts',(4.29821509599994,2.2,-1.42295882700001));
#348542=CARTESIAN_POINT('Ctrl Pts',(4.29663303399995,12.2,-1.42129787500001));
#348543=CARTESIAN_POINT('Ctrl Pts',(4.29663303399995,5.2,-1.42129787500001));
#348544=CARTESIAN_POINT('Ctrl Pts',(4.29663303399995,2.2,-1.42129787500001));
#348545=CARTESIAN_POINT('Ctrl Pts',(4.29505177099994,12.2,-1.41964133800002));
#348546=CARTESIAN_POINT('Ctrl Pts',(4.29505177099994,5.2,-1.41964133800002));
#348547=CARTESIAN_POINT('Ctrl Pts',(4.29505177099994,2.2,-1.41964133800002));
#348548=CARTESIAN_POINT('Ctrl Pts',(4.29347131599994,12.2,-1.41798921400001));
#348549=CARTESIAN_POINT('Ctrl Pts',(4.29347131599994,5.2,-1.41798921400001));
#348550=CARTESIAN_POINT('Ctrl Pts',(4.29347131599994,2.2,-1.41798921400001));
#348551=CARTESIAN_POINT('Ctrl Pts',(4.29189168099995,12.2,-1.41634150400002));
#348552=CARTESIAN_POINT('Ctrl Pts',(4.29189168099995,5.2,-1.41634150400002));
#348553=CARTESIAN_POINT('Ctrl Pts',(4.29189168099995,2.2,-1.41634150400002));
#348554=CARTESIAN_POINT('Ctrl Pts',(4.29031287399994,12.2,-1.41469820800001));
#348555=CARTESIAN_POINT('Ctrl Pts',(4.29031287399994,5.2,-1.41469820800001));
#348556=CARTESIAN_POINT('Ctrl Pts',(4.29031287399994,2.2,-1.41469820800001));
#348557=CARTESIAN_POINT('Ctrl Pts',(4.28873490499995,12.2,-1.41305932400002));
#348558=CARTESIAN_POINT('Ctrl Pts',(4.28873490499995,5.2,-1.41305932400002));
#348559=CARTESIAN_POINT('Ctrl Pts',(4.28873490499995,2.2,-1.41305932400002));
#348560=CARTESIAN_POINT('Ctrl Pts',(4.28715778399994,12.2,-1.41142485500001));
#348561=CARTESIAN_POINT('Ctrl Pts',(4.28715778399994,5.2,-1.41142485500001));
#348562=CARTESIAN_POINT('Ctrl Pts',(4.28715778399994,2.2,-1.41142485500001));
#348563=CARTESIAN_POINT('Ctrl Pts',(4.28558152199995,12.2,-1.40979479800002));
#348564=CARTESIAN_POINT('Ctrl Pts',(4.28558152199995,5.2,-1.40979479800002));
#348565=CARTESIAN_POINT('Ctrl Pts',(4.28558152199995,2.2,-1.40979479800002));
#348566=CARTESIAN_POINT('Ctrl Pts',(4.28400612599994,12.2,-1.40816915500002));
#348567=CARTESIAN_POINT('Ctrl Pts',(4.28400612599994,5.2,-1.40816915500002));
#348568=CARTESIAN_POINT('Ctrl Pts',(4.28400612599994,2.2,-1.40816915500002));
#348569=CARTESIAN_POINT('Ctrl Pts',(4.28243160799994,12.2,-1.40654792400001));
#348570=CARTESIAN_POINT('Ctrl Pts',(4.28243160799994,5.2,-1.40654792400001));
#348571=CARTESIAN_POINT('Ctrl Pts',(4.28243160799994,2.2,-1.40654792400001));
#348572=CARTESIAN_POINT('Ctrl Pts',(4.28085797699994,12.2,-1.40493110600001));
#348573=CARTESIAN_POINT('Ctrl Pts',(4.28085797699994,5.2,-1.40493110600001));
#348574=CARTESIAN_POINT('Ctrl Pts',(4.28085797699994,2.2,-1.40493110600001));
#348575=CARTESIAN_POINT('Ctrl Pts',(4.27928524499994,12.2,-1.40331870000002));
#348576=CARTESIAN_POINT('Ctrl Pts',(4.27928524499994,5.2,-1.40331870000002));
#348577=CARTESIAN_POINT('Ctrl Pts',(4.27928524499994,2.2,-1.40331870000002));
#348578=CARTESIAN_POINT('Ctrl Pts',(4.27771341799995,12.2,-1.40171070500001));
#348579=CARTESIAN_POINT('Ctrl Pts',(4.27771341799995,5.2,-1.40171070500001));
#348580=CARTESIAN_POINT('Ctrl Pts',(4.27771341799995,2.2,-1.40171070500001));
#348581=CARTESIAN_POINT('Ctrl Pts',(4.27614250899994,12.2,-1.40010712400001));
#348582=CARTESIAN_POINT('Ctrl Pts',(4.27614250899994,5.2,-1.40010712400001));
#348583=CARTESIAN_POINT('Ctrl Pts',(4.27614250899994,2.2,-1.40010712400001));
#348584=CARTESIAN_POINT('Ctrl Pts',(4.27457252599994,12.2,-1.39850795300001));
#348585=CARTESIAN_POINT('Ctrl Pts',(4.27457252599994,5.2,-1.39850795300001));
#348586=CARTESIAN_POINT('Ctrl Pts',(4.27457252599994,2.2,-1.39850795300001));
#348587=CARTESIAN_POINT('Ctrl Pts',(4.27300347999994,12.2,-1.39691319500002));
#348588=CARTESIAN_POINT('Ctrl Pts',(4.27300347999994,5.2,-1.39691319500002));
#348589=CARTESIAN_POINT('Ctrl Pts',(4.27300347999994,2.2,-1.39691319500002));
#348590=CARTESIAN_POINT('Ctrl Pts',(4.27143538199994,12.2,-1.39532284600001));
#348591=CARTESIAN_POINT('Ctrl Pts',(4.27143538199994,5.2,-1.39532284600001));
#348592=CARTESIAN_POINT('Ctrl Pts',(4.27143538199994,2.2,-1.39532284600001));
#348593=CARTESIAN_POINT('Ctrl Pts',(4.26986823899994,12.2,-1.39373690900001));
#348594=CARTESIAN_POINT('Ctrl Pts',(4.26986823899994,5.2,-1.39373690900001));
#348595=CARTESIAN_POINT('Ctrl Pts',(4.26986823899994,2.2,-1.39373690900001));
#348596=CARTESIAN_POINT('Ctrl Pts',(4.26830206399995,12.2,-1.39215538100002));
#348597=CARTESIAN_POINT('Ctrl Pts',(4.26830206399995,5.2,-1.39215538100002));
#348598=CARTESIAN_POINT('Ctrl Pts',(4.26830206399995,2.2,-1.39215538100002));
#348599=CARTESIAN_POINT('Ctrl Pts',(4.26673686399995,12.2,-1.39057826400002));
#348600=CARTESIAN_POINT('Ctrl Pts',(4.26673686399995,5.2,-1.39057826400002));
#348601=CARTESIAN_POINT('Ctrl Pts',(4.26673686399995,2.2,-1.39057826400002));
#348602=CARTESIAN_POINT('Ctrl Pts',(4.26517265199994,12.2,-1.38900555700001));
#348603=CARTESIAN_POINT('Ctrl Pts',(4.26517265199994,5.2,-1.38900555700001));
#348604=CARTESIAN_POINT('Ctrl Pts',(4.26517265199994,2.2,-1.38900555700001));
#348605=CARTESIAN_POINT('Ctrl Pts',(4.26360943599995,12.2,-1.38743725800001));
#348606=CARTESIAN_POINT('Ctrl Pts',(4.26360943599995,5.2,-1.38743725800001));
#348607=CARTESIAN_POINT('Ctrl Pts',(4.26360943599995,2.2,-1.38743725800001));
#348608=CARTESIAN_POINT('Ctrl Pts',(4.26204722699994,12.2,-1.38587336900001));
#348609=CARTESIAN_POINT('Ctrl Pts',(4.26204722699994,5.2,-1.38587336900001));
#348610=CARTESIAN_POINT('Ctrl Pts',(4.26204722699994,2.2,-1.38587336900001));
#348611=CARTESIAN_POINT('Ctrl Pts',(4.26048603399994,12.2,-1.38431388800001));
#348612=CARTESIAN_POINT('Ctrl Pts',(4.26048603399994,5.2,-1.38431388800001));
#348613=CARTESIAN_POINT('Ctrl Pts',(4.26048603399994,2.2,-1.38431388800001));
#348614=CARTESIAN_POINT('Ctrl Pts',(4.25892586799994,12.2,-1.38275881500002));
#348615=CARTESIAN_POINT('Ctrl Pts',(4.25892586799994,5.2,-1.38275881500002));
#348616=CARTESIAN_POINT('Ctrl Pts',(4.25892586799994,2.2,-1.38275881500002));
#348617=CARTESIAN_POINT('Ctrl Pts',(4.25736673899994,12.2,-1.38120815000002));
#348618=CARTESIAN_POINT('Ctrl Pts',(4.25736673899994,5.2,-1.38120815000002));
#348619=CARTESIAN_POINT('Ctrl Pts',(4.25736673899994,2.2,-1.38120815000002));
#348620=CARTESIAN_POINT('Ctrl Pts',(4.25580865599995,12.2,-1.37966189200001));
#348621=CARTESIAN_POINT('Ctrl Pts',(4.25580865599995,5.2,-1.37966189200001));
#348622=CARTESIAN_POINT('Ctrl Pts',(4.25580865599995,2.2,-1.37966189200001));
#348623=CARTESIAN_POINT('Ctrl Pts',(4.25425163099994,12.2,-1.37812004100001));
#348624=CARTESIAN_POINT('Ctrl Pts',(4.25425163099994,5.2,-1.37812004100001));
#348625=CARTESIAN_POINT('Ctrl Pts',(4.25425163099994,2.2,-1.37812004100001));
#348626=CARTESIAN_POINT('Ctrl Pts',(4.25269567199994,12.2,-1.37658259600002));
#348627=CARTESIAN_POINT('Ctrl Pts',(4.25269567199994,5.2,-1.37658259600002));
#348628=CARTESIAN_POINT('Ctrl Pts',(4.25269567199994,2.2,-1.37658259600002));
#348629=CARTESIAN_POINT('Ctrl Pts',(4.25114079099994,12.2,-1.37504955700001));
#348630=CARTESIAN_POINT('Ctrl Pts',(4.25114079099994,5.2,-1.37504955700001));
#348631=CARTESIAN_POINT('Ctrl Pts',(4.25114079099994,2.2,-1.37504955700001));
#348632=CARTESIAN_POINT('Ctrl Pts',(4.24958699699994,12.2,-1.37352092300001));
#348633=CARTESIAN_POINT('Ctrl Pts',(4.24958699699994,5.2,-1.37352092300001));
#348634=CARTESIAN_POINT('Ctrl Pts',(4.24958699699994,2.2,-1.37352092300001));
#348635=CARTESIAN_POINT('Ctrl Pts',(4.24803429999994,12.2,-1.37199669400002));
#348636=CARTESIAN_POINT('Ctrl Pts',(4.24803429999994,5.2,-1.37199669400002));
#348637=CARTESIAN_POINT('Ctrl Pts',(4.24803429999994,2.2,-1.37199669400002));
#348638=CARTESIAN_POINT('Ctrl Pts',(4.24648271099994,12.2,-1.37047686900001));
#348639=CARTESIAN_POINT('Ctrl Pts',(4.24648271099994,5.2,-1.37047686900001));
#348640=CARTESIAN_POINT('Ctrl Pts',(4.24648271099994,2.2,-1.37047686900001));
#348641=CARTESIAN_POINT('Ctrl Pts',(4.24493223999994,12.2,-1.36896144900001));
#348642=CARTESIAN_POINT('Ctrl Pts',(4.24493223999994,5.2,-1.36896144900001));
#348643=CARTESIAN_POINT('Ctrl Pts',(4.24493223999994,2.2,-1.36896144900001));
#348644=CARTESIAN_POINT('Ctrl Pts',(4.24338289699994,12.2,-1.36745043100001));
#348645=CARTESIAN_POINT('Ctrl Pts',(4.24338289699994,5.2,-1.36745043100001));
#348646=CARTESIAN_POINT('Ctrl Pts',(4.24338289699994,2.2,-1.36745043100001));
#348647=CARTESIAN_POINT('Ctrl Pts',(4.24183469099995,12.2,-1.36594381500001));
#348648=CARTESIAN_POINT('Ctrl Pts',(4.24183469099995,5.2,-1.36594381500001));
#348649=CARTESIAN_POINT('Ctrl Pts',(4.24183469099995,2.2,-1.36594381500001));
#348650=CARTESIAN_POINT('Ctrl Pts',(4.24028763399994,12.2,-1.36444160200002));
#348651=CARTESIAN_POINT('Ctrl Pts',(4.24028763399994,5.2,-1.36444160200002));
#348652=CARTESIAN_POINT('Ctrl Pts',(4.24028763399994,2.2,-1.36444160200002));
#348653=CARTESIAN_POINT('Ctrl Pts',(4.23874173499994,12.2,-1.36294379100002));
#348654=CARTESIAN_POINT('Ctrl Pts',(4.23874173499994,5.2,-1.36294379100002));
#348655=CARTESIAN_POINT('Ctrl Pts',(4.23874173499994,2.2,-1.36294379100002));
#348656=CARTESIAN_POINT('Ctrl Pts',(4.23719700499994,12.2,-1.36145038000001));
#348657=CARTESIAN_POINT('Ctrl Pts',(4.23719700499994,5.2,-1.36145038000001));
#348658=CARTESIAN_POINT('Ctrl Pts',(4.23719700499994,2.2,-1.36145038000001));
#348659=CARTESIAN_POINT('Ctrl Pts',(4.23565345399994,12.2,-1.35996136900001));
#348660=CARTESIAN_POINT('Ctrl Pts',(4.23565345399994,5.2,-1.35996136900001));
#348661=CARTESIAN_POINT('Ctrl Pts',(4.23565345399994,2.2,-1.35996136900001));
#348662=CARTESIAN_POINT('Ctrl Pts',(4.23411109299995,12.2,-1.35847675800001));
#348663=CARTESIAN_POINT('Ctrl Pts',(4.23411109299995,5.2,-1.35847675800001));
#348664=CARTESIAN_POINT('Ctrl Pts',(4.23411109299995,2.2,-1.35847675800001));
#348665=CARTESIAN_POINT('Ctrl Pts',(4.23256993099994,12.2,-1.35699654500002));
#348666=CARTESIAN_POINT('Ctrl Pts',(4.23256993099994,5.2,-1.35699654500002));
#348667=CARTESIAN_POINT('Ctrl Pts',(4.23256993099994,2.2,-1.35699654500002));
#348668=CARTESIAN_POINT('Ctrl Pts',(4.23102997899994,12.2,-1.35552073100001));
#348669=CARTESIAN_POINT('Ctrl Pts',(4.23102997899994,5.2,-1.35552073100001));
#348670=CARTESIAN_POINT('Ctrl Pts',(4.23102997899994,2.2,-1.35552073100001));
#348671=CARTESIAN_POINT('Ctrl Pts',(4.22949124699994,12.2,-1.35404931500001));
#348672=CARTESIAN_POINT('Ctrl Pts',(4.22949124699994,5.2,-1.35404931500001));
#348673=CARTESIAN_POINT('Ctrl Pts',(4.22949124699994,2.2,-1.35404931500001));
#348674=CARTESIAN_POINT('Ctrl Pts',(4.22795374499994,12.2,-1.35258229500002));
#348675=CARTESIAN_POINT('Ctrl Pts',(4.22795374499994,5.2,-1.35258229500002));
#348676=CARTESIAN_POINT('Ctrl Pts',(4.22795374499994,2.2,-1.35258229500002));
#348677=CARTESIAN_POINT('Ctrl Pts',(4.22641748499994,12.2,-1.35111967100002));
#348678=CARTESIAN_POINT('Ctrl Pts',(4.22641748499994,5.2,-1.35111967100002));
#348679=CARTESIAN_POINT('Ctrl Pts',(4.22641748499994,2.2,-1.35111967100002));
#348680=CARTESIAN_POINT('Ctrl Pts',(4.22488247499994,12.2,-1.34966144200002));
#348681=CARTESIAN_POINT('Ctrl Pts',(4.22488247499994,5.2,-1.34966144200002));
#348682=CARTESIAN_POINT('Ctrl Pts',(4.22488247499994,2.2,-1.34966144200002));
#348683=CARTESIAN_POINT('Ctrl Pts',(4.22334872799994,12.2,-1.34820760900002));
#348684=CARTESIAN_POINT('Ctrl Pts',(4.22334872799994,5.2,-1.34820760900002));
#348685=CARTESIAN_POINT('Ctrl Pts',(4.22334872799994,2.2,-1.34820760900002));
#348686=CARTESIAN_POINT('Ctrl Pts',(4.22181625199994,12.2,-1.34675816800002));
#348687=CARTESIAN_POINT('Ctrl Pts',(4.22181625199994,5.2,-1.34675816800002));
#348688=CARTESIAN_POINT('Ctrl Pts',(4.22181625199994,2.2,-1.34675816800002));
#348689=CARTESIAN_POINT('Ctrl Pts',(4.22028505899994,12.2,-1.34531312100002));
#348690=CARTESIAN_POINT('Ctrl Pts',(4.22028505899994,5.2,-1.34531312100002));
#348691=CARTESIAN_POINT('Ctrl Pts',(4.22028505899994,2.2,-1.34531312100002));
#348692=CARTESIAN_POINT('Ctrl Pts',(4.21875515899994,12.2,-1.34387246600001));
#348693=CARTESIAN_POINT('Ctrl Pts',(4.21875515899994,5.2,-1.34387246600001));
#348694=CARTESIAN_POINT('Ctrl Pts',(4.21875515899994,2.2,-1.34387246600001));
#348695=CARTESIAN_POINT('Ctrl Pts',(4.21722656199994,12.2,-1.34243620300001));
#348696=CARTESIAN_POINT('Ctrl Pts',(4.21722656199994,5.2,-1.34243620300001));
#348697=CARTESIAN_POINT('Ctrl Pts',(4.21722656199994,2.2,-1.34243620300001));
#348698=CARTESIAN_POINT('Ctrl Pts',(4.21569927799994,12.2,-1.34100433000001));
#348699=CARTESIAN_POINT('Ctrl Pts',(4.21569927799994,5.2,-1.34100433000001));
#348700=CARTESIAN_POINT('Ctrl Pts',(4.21569927799994,2.2,-1.34100433000001));
#348701=CARTESIAN_POINT('Ctrl Pts',(4.21417331899994,12.2,-1.33957684700002));
#348702=CARTESIAN_POINT('Ctrl Pts',(4.21417331899994,5.2,-1.33957684700002));
#348703=CARTESIAN_POINT('Ctrl Pts',(4.21417331899994,2.2,-1.33957684700002));
#348704=CARTESIAN_POINT('Ctrl Pts',(4.21264869399994,12.2,-1.33815375200002));
#348705=CARTESIAN_POINT('Ctrl Pts',(4.21264869399994,5.2,-1.33815375200002));
#348706=CARTESIAN_POINT('Ctrl Pts',(4.21264869399994,2.2,-1.33815375200002));
#348707=CARTESIAN_POINT('Ctrl Pts',(4.21112541399994,12.2,-1.33673504600001));
#348708=CARTESIAN_POINT('Ctrl Pts',(4.21112541399994,5.2,-1.33673504600001));
#348709=CARTESIAN_POINT('Ctrl Pts',(4.21112541399994,2.2,-1.33673504600001));
#348710=CARTESIAN_POINT('Ctrl Pts',(4.20960348999994,12.2,-1.33532072700001));
#348711=CARTESIAN_POINT('Ctrl Pts',(4.20960348999994,5.2,-1.33532072700001));
#348712=CARTESIAN_POINT('Ctrl Pts',(4.20960348999994,2.2,-1.33532072700001));
#348713=CARTESIAN_POINT('Ctrl Pts',(4.20808293199994,12.2,-1.33391079400001));
#348714=CARTESIAN_POINT('Ctrl Pts',(4.20808293199994,5.2,-1.33391079400001));
#348715=CARTESIAN_POINT('Ctrl Pts',(4.20808293199994,2.2,-1.33391079400001));
#348716=CARTESIAN_POINT('Ctrl Pts',(4.20656375099994,12.2,-1.33250524600002));
#348717=CARTESIAN_POINT('Ctrl Pts',(4.20656375099994,5.2,-1.33250524600002));
#348718=CARTESIAN_POINT('Ctrl Pts',(4.20656375099994,2.2,-1.33250524600002));
#348719=CARTESIAN_POINT('Ctrl Pts',(4.20504595699995,12.2,-1.33110408200002));
#348720=CARTESIAN_POINT('Ctrl Pts',(4.20504595699995,5.2,-1.33110408200002));
#348721=CARTESIAN_POINT('Ctrl Pts',(4.20504595699995,2.2,-1.33110408200002));
#348722=CARTESIAN_POINT('Ctrl Pts',(4.20352956099994,12.2,-1.32970730200002));
#348723=CARTESIAN_POINT('Ctrl Pts',(4.20352956099994,5.2,-1.32970730200002));
#348724=CARTESIAN_POINT('Ctrl Pts',(4.20352956099994,2.2,-1.32970730200002));
#348725=CARTESIAN_POINT('Ctrl Pts',(4.20201457299994,12.2,-1.32831490500001));
#348726=CARTESIAN_POINT('Ctrl Pts',(4.20201457299994,5.2,-1.32831490500001));
#348727=CARTESIAN_POINT('Ctrl Pts',(4.20201457299994,2.2,-1.32831490500001));
#348728=CARTESIAN_POINT('Ctrl Pts',(4.20050100399994,12.2,-1.32692688800002));
#348729=CARTESIAN_POINT('Ctrl Pts',(4.20050100399994,5.2,-1.32692688800002));
#348730=CARTESIAN_POINT('Ctrl Pts',(4.20050100399994,2.2,-1.32692688800002));
#348731=CARTESIAN_POINT('Ctrl Pts',(4.19898886499994,12.2,-1.32554325300001));
#348732=CARTESIAN_POINT('Ctrl Pts',(4.19898886499994,5.2,-1.32554325300001));
#348733=CARTESIAN_POINT('Ctrl Pts',(4.19898886499994,2.2,-1.32554325300001));
#348734=CARTESIAN_POINT('Ctrl Pts',(4.19747816499994,12.2,-1.32416399600002));
#348735=CARTESIAN_POINT('Ctrl Pts',(4.19747816499994,5.2,-1.32416399600002));
#348736=CARTESIAN_POINT('Ctrl Pts',(4.19747816499994,2.2,-1.32416399600002));
#348737=CARTESIAN_POINT('Ctrl Pts',(4.19596891699995,12.2,-1.32278911800002));
#348738=CARTESIAN_POINT('Ctrl Pts',(4.19596891699995,5.2,-1.32278911800002));
#348739=CARTESIAN_POINT('Ctrl Pts',(4.19596891699995,2.2,-1.32278911800002));
#348740=CARTESIAN_POINT('Ctrl Pts',(4.19446112999994,12.2,-1.32141861700001));
#348741=CARTESIAN_POINT('Ctrl Pts',(4.19446112999994,5.2,-1.32141861700001));
#348742=CARTESIAN_POINT('Ctrl Pts',(4.19446112999994,2.2,-1.32141861700001));
#348743=CARTESIAN_POINT('Ctrl Pts',(4.19295481499994,12.2,-1.32005249200001));
#348744=CARTESIAN_POINT('Ctrl Pts',(4.19295481499994,5.2,-1.32005249200001));
#348745=CARTESIAN_POINT('Ctrl Pts',(4.19295481499994,2.2,-1.32005249200001));
#348746=CARTESIAN_POINT('Ctrl Pts',(4.19144998399995,12.2,-1.31869074300001));
#348747=CARTESIAN_POINT('Ctrl Pts',(4.19144998399995,5.2,-1.31869074300001));
#348748=CARTESIAN_POINT('Ctrl Pts',(4.19144998399995,2.2,-1.31869074300001));
#348749=CARTESIAN_POINT('Ctrl Pts',(4.18994664499994,12.2,-1.31733336700002));
#348750=CARTESIAN_POINT('Ctrl Pts',(4.18994664499994,5.2,-1.31733336700002));
#348751=CARTESIAN_POINT('Ctrl Pts',(4.18994664499994,2.2,-1.31733336700002));
#348752=CARTESIAN_POINT('Ctrl Pts',(4.18844481099994,12.2,-1.31598036500002));
#348753=CARTESIAN_POINT('Ctrl Pts',(4.18844481099994,5.2,-1.31598036500002));
#348754=CARTESIAN_POINT('Ctrl Pts',(4.18844481099994,2.2,-1.31598036500002));
#348755=CARTESIAN_POINT('Ctrl Pts',(4.18694449099995,12.2,-1.31463173400002));
#348756=CARTESIAN_POINT('Ctrl Pts',(4.18694449099995,5.2,-1.31463173400002));
#348757=CARTESIAN_POINT('Ctrl Pts',(4.18694449099995,2.2,-1.31463173400002));
#348758=CARTESIAN_POINT('Ctrl Pts',(4.18544569799994,12.2,-1.31328747400001));
#348759=CARTESIAN_POINT('Ctrl Pts',(4.18544569799994,5.2,-1.31328747400001));
#348760=CARTESIAN_POINT('Ctrl Pts',(4.18544569799994,2.2,-1.31328747400001));
#348761=CARTESIAN_POINT('Ctrl Pts',(4.18394844199994,12.2,-1.31194758300001));
#348762=CARTESIAN_POINT('Ctrl Pts',(4.18394844199994,5.2,-1.31194758300001));
#348763=CARTESIAN_POINT('Ctrl Pts',(4.18394844199994,2.2,-1.31194758300001));
#348764=CARTESIAN_POINT('Ctrl Pts',(4.18245273199994,12.2,-1.31061206100001));
#348765=CARTESIAN_POINT('Ctrl Pts',(4.18245273199994,5.2,-1.31061206100001));
#348766=CARTESIAN_POINT('Ctrl Pts',(4.18245273199994,2.2,-1.31061206100001));
#348767=CARTESIAN_POINT('Ctrl Pts',(4.18095858099994,12.2,-1.30928090600001));
#348768=CARTESIAN_POINT('Ctrl Pts',(4.18095858099994,5.2,-1.30928090600001));
#348769=CARTESIAN_POINT('Ctrl Pts',(4.18095858099994,2.2,-1.30928090600001));
#348770=CARTESIAN_POINT('Ctrl Pts',(4.17946599699994,12.2,-1.30795411700001));
#348771=CARTESIAN_POINT('Ctrl Pts',(4.17946599699994,5.2,-1.30795411700001));
#348772=CARTESIAN_POINT('Ctrl Pts',(4.17946599699994,2.2,-1.30795411700001));
#348773=CARTESIAN_POINT('Ctrl Pts',(4.17797499499994,12.2,-1.30663169200002));
#348774=CARTESIAN_POINT('Ctrl Pts',(4.17797499499994,5.2,-1.30663169200002));
#348775=CARTESIAN_POINT('Ctrl Pts',(4.17797499499994,2.2,-1.30663169200002));
#348776=CARTESIAN_POINT('Ctrl Pts',(4.17648558199994,12.2,-1.30531363000001));
#348777=CARTESIAN_POINT('Ctrl Pts',(4.17648558199994,5.2,-1.30531363000001));
#348778=CARTESIAN_POINT('Ctrl Pts',(4.17648558199994,2.2,-1.30531363000001));
#348779=CARTESIAN_POINT('Ctrl Pts',(4.17499777099995,12.2,-1.30399993100001));
#348780=CARTESIAN_POINT('Ctrl Pts',(4.17499777099995,5.2,-1.30399993100001));
#348781=CARTESIAN_POINT('Ctrl Pts',(4.17499777099995,2.2,-1.30399993100001));
#348782=CARTESIAN_POINT('Ctrl Pts',(4.17351157199994,12.2,-1.30269059300002));
#348783=CARTESIAN_POINT('Ctrl Pts',(4.17351157199994,5.2,-1.30269059300002));
#348784=CARTESIAN_POINT('Ctrl Pts',(4.17351157199994,2.2,-1.30269059300002));
#348785=CARTESIAN_POINT('Ctrl Pts',(4.17202699599994,12.2,-1.30138561400001));
#348786=CARTESIAN_POINT('Ctrl Pts',(4.17202699599994,5.2,-1.30138561400001));
#348787=CARTESIAN_POINT('Ctrl Pts',(4.17202699599994,2.2,-1.30138561400001));
#348788=CARTESIAN_POINT('Ctrl Pts',(4.17054405399994,12.2,-1.30008499300001));
#348789=CARTESIAN_POINT('Ctrl Pts',(4.17054405399994,5.2,-1.30008499300001));
#348790=CARTESIAN_POINT('Ctrl Pts',(4.17054405399994,2.2,-1.30008499300001));
#348791=CARTESIAN_POINT('Ctrl Pts',(4.16906275799994,12.2,-1.29878873000001));
#348792=CARTESIAN_POINT('Ctrl Pts',(4.16906275799994,5.2,-1.29878873000001));
#348793=CARTESIAN_POINT('Ctrl Pts',(4.16906275799994,2.2,-1.29878873000001));
#348794=CARTESIAN_POINT('Ctrl Pts',(4.16758311699994,12.2,-1.29749682100002));
#348795=CARTESIAN_POINT('Ctrl Pts',(4.16758311699994,5.2,-1.29749682100002));
#348796=CARTESIAN_POINT('Ctrl Pts',(4.16758311699994,2.2,-1.29749682100002));
#348797=CARTESIAN_POINT('Ctrl Pts',(4.16610514399994,12.2,-1.29620926700001));
#348798=CARTESIAN_POINT('Ctrl Pts',(4.16610514399994,5.2,-1.29620926700001));
#348799=CARTESIAN_POINT('Ctrl Pts',(4.16610514399994,2.2,-1.29620926700001));
#348800=CARTESIAN_POINT('Ctrl Pts',(4.16462884799994,12.2,-1.29492606500001));
#348801=CARTESIAN_POINT('Ctrl Pts',(4.16462884799994,5.2,-1.29492606500001));
#348802=CARTESIAN_POINT('Ctrl Pts',(4.16462884799994,2.2,-1.29492606500001));
#348803=CARTESIAN_POINT('Ctrl Pts',(4.16315424099994,12.2,-1.29364721600002));
#348804=CARTESIAN_POINT('Ctrl Pts',(4.16315424099994,5.2,-1.29364721600002));
#348805=CARTESIAN_POINT('Ctrl Pts',(4.16315424099994,2.2,-1.29364721600002));
#348806=CARTESIAN_POINT('Ctrl Pts',(4.16168133299994,12.2,-1.29237271600001));
#348807=CARTESIAN_POINT('Ctrl Pts',(4.16168133299994,5.2,-1.29237271600001));
#348808=CARTESIAN_POINT('Ctrl Pts',(4.16168133299994,2.2,-1.29237271600001));
#348809=CARTESIAN_POINT('Ctrl Pts',(4.16021013599994,12.2,-1.29110256400002));
#348810=CARTESIAN_POINT('Ctrl Pts',(4.16021013599994,5.2,-1.29110256400002));
#348811=CARTESIAN_POINT('Ctrl Pts',(4.16021013599994,2.2,-1.29110256400002));
#348812=CARTESIAN_POINT('Ctrl Pts',(4.15874066199994,12.2,-1.28983676000002));
#348813=CARTESIAN_POINT('Ctrl Pts',(4.15874066199994,5.2,-1.28983676000002));
#348814=CARTESIAN_POINT('Ctrl Pts',(4.15874066199994,2.2,-1.28983676000002));
#348815=CARTESIAN_POINT('Ctrl Pts',(4.15727291999994,12.2,-1.28857530100001));
#348816=CARTESIAN_POINT('Ctrl Pts',(4.15727291999994,5.2,-1.28857530100001));
#348817=CARTESIAN_POINT('Ctrl Pts',(4.15727291999994,2.2,-1.28857530100001));
#348818=CARTESIAN_POINT('Ctrl Pts',(4.15580692199994,12.2,-1.28731818500002));
#348819=CARTESIAN_POINT('Ctrl Pts',(4.15580692199994,5.2,-1.28731818500002));
#348820=CARTESIAN_POINT('Ctrl Pts',(4.15580692199994,2.2,-1.28731818500002));
#348821=CARTESIAN_POINT('Ctrl Pts',(4.15434267899994,12.2,-1.28606541400002));
#348822=CARTESIAN_POINT('Ctrl Pts',(4.15434267899994,5.2,-1.28606541400002));
#348823=CARTESIAN_POINT('Ctrl Pts',(4.15434267899994,2.2,-1.28606541400002));
#348824=CARTESIAN_POINT('Ctrl Pts',(4.15288020299994,12.2,-1.28481698200002));
#348825=CARTESIAN_POINT('Ctrl Pts',(4.15288020299994,5.2,-1.28481698200002));
#348826=CARTESIAN_POINT('Ctrl Pts',(4.15288020299994,2.2,-1.28481698200002));
#348827=CARTESIAN_POINT('Ctrl Pts',(4.15141950299994,12.2,-1.28357289000002));
#348828=CARTESIAN_POINT('Ctrl Pts',(4.15141950299994,5.2,-1.28357289000002));
#348829=CARTESIAN_POINT('Ctrl Pts',(4.15141950299994,2.2,-1.28357289000002));
#348830=CARTESIAN_POINT('Ctrl Pts',(4.14996059099995,12.2,-1.28233313700001));
#348831=CARTESIAN_POINT('Ctrl Pts',(4.14996059099995,5.2,-1.28233313700001));
#348832=CARTESIAN_POINT('Ctrl Pts',(4.14996059099995,2.2,-1.28233313700001));
#348833=CARTESIAN_POINT('Ctrl Pts',(4.14850347999994,12.2,-1.28109772000002));
#348834=CARTESIAN_POINT('Ctrl Pts',(4.14850347999994,5.2,-1.28109772000002));
#348835=CARTESIAN_POINT('Ctrl Pts',(4.14850347999994,2.2,-1.28109772000002));
#348836=CARTESIAN_POINT('Ctrl Pts',(4.14704817999994,12.2,-1.27986663600002));
#348837=CARTESIAN_POINT('Ctrl Pts',(4.14704817999994,5.2,-1.27986663600002));
#348838=CARTESIAN_POINT('Ctrl Pts',(4.14704817999994,2.2,-1.27986663600002));
#348839=CARTESIAN_POINT('Ctrl Pts',(4.14559469999995,12.2,-1.27863988700001));
#348840=CARTESIAN_POINT('Ctrl Pts',(4.14559469999995,5.2,-1.27863988700001));
#348841=CARTESIAN_POINT('Ctrl Pts',(4.14559469999995,2.2,-1.27863988700001));
#348842=CARTESIAN_POINT('Ctrl Pts',(4.14414305399994,12.2,-1.27741746900002));
#348843=CARTESIAN_POINT('Ctrl Pts',(4.14414305399994,5.2,-1.27741746900002));
#348844=CARTESIAN_POINT('Ctrl Pts',(4.14414305399994,2.2,-1.27741746900002));
#348845=CARTESIAN_POINT('Ctrl Pts',(4.14269325199994,12.2,-1.27619938100001));
#348846=CARTESIAN_POINT('Ctrl Pts',(4.14269325199994,5.2,-1.27619938100001));
#348847=CARTESIAN_POINT('Ctrl Pts',(4.14269325199994,2.2,-1.27619938100001));
#348848=CARTESIAN_POINT('Ctrl Pts',(4.14124530599994,12.2,-1.27498562100001));
#348849=CARTESIAN_POINT('Ctrl Pts',(4.14124530599994,5.2,-1.27498562100001));
#348850=CARTESIAN_POINT('Ctrl Pts',(4.14124530599994,2.2,-1.27498562100001));
#348851=CARTESIAN_POINT('Ctrl Pts',(4.13979922699994,12.2,-1.27377618700002));
#348852=CARTESIAN_POINT('Ctrl Pts',(4.13979922699994,5.2,-1.27377618700002));
#348853=CARTESIAN_POINT('Ctrl Pts',(4.13979922699994,2.2,-1.27377618700002));
#348854=CARTESIAN_POINT('Ctrl Pts',(4.13835502499994,12.2,-1.27257107800002));
#348855=CARTESIAN_POINT('Ctrl Pts',(4.13835502499994,5.2,-1.27257107800002));
#348856=CARTESIAN_POINT('Ctrl Pts',(4.13835502499994,2.2,-1.27257107800002));
#348857=CARTESIAN_POINT('Ctrl Pts',(4.13691271299994,12.2,-1.27137029300001));
#348858=CARTESIAN_POINT('Ctrl Pts',(4.13691271299994,5.2,-1.27137029300001));
#348859=CARTESIAN_POINT('Ctrl Pts',(4.13691271299994,2.2,-1.27137029300001));
#348860=CARTESIAN_POINT('Ctrl Pts',(4.13547230099994,12.2,-1.27017382800001));
#348861=CARTESIAN_POINT('Ctrl Pts',(4.13547230099994,5.2,-1.27017382800001));
#348862=CARTESIAN_POINT('Ctrl Pts',(4.13547230099994,2.2,-1.27017382800001));
#348863=CARTESIAN_POINT('Ctrl Pts',(4.13403380099994,12.2,-1.26898168400002));
#348864=CARTESIAN_POINT('Ctrl Pts',(4.13403380099994,5.2,-1.26898168400002));
#348865=CARTESIAN_POINT('Ctrl Pts',(4.13403380099994,2.2,-1.26898168400002));
#348866=CARTESIAN_POINT('Ctrl Pts',(4.13259722399994,12.2,-1.26779385600001));
#348867=CARTESIAN_POINT('Ctrl Pts',(4.13259722399994,5.2,-1.26779385600001));
#348868=CARTESIAN_POINT('Ctrl Pts',(4.13259722399994,2.2,-1.26779385600001));
#348869=CARTESIAN_POINT('Ctrl Pts',(4.13116258199994,12.2,-1.26661034500001));
#348870=CARTESIAN_POINT('Ctrl Pts',(4.13116258199994,5.2,-1.26661034500001));
#348871=CARTESIAN_POINT('Ctrl Pts',(4.13116258199994,2.2,-1.26661034500001));
#348872=CARTESIAN_POINT('Ctrl Pts',(4.12972988599994,12.2,-1.26543114900001));
#348873=CARTESIAN_POINT('Ctrl Pts',(4.12972988599994,5.2,-1.26543114900001));
#348874=CARTESIAN_POINT('Ctrl Pts',(4.12972988599994,2.2,-1.26543114900001));
#348875=CARTESIAN_POINT('Ctrl Pts',(4.12829914699994,12.2,-1.26425626500001));
#348876=CARTESIAN_POINT('Ctrl Pts',(4.12829914699994,5.2,-1.26425626500001));
#348877=CARTESIAN_POINT('Ctrl Pts',(4.12829914699994,2.2,-1.26425626500001));
#348878=CARTESIAN_POINT('Ctrl Pts',(4.12687037699994,12.2,-1.26308569100001));
#348879=CARTESIAN_POINT('Ctrl Pts',(4.12687037699994,5.2,-1.26308569100001));
#348880=CARTESIAN_POINT('Ctrl Pts',(4.12687037699994,2.2,-1.26308569100001));
#348881=CARTESIAN_POINT('Ctrl Pts',(4.12544358599995,12.2,-1.26191942500002));
#348882=CARTESIAN_POINT('Ctrl Pts',(4.12544358599995,5.2,-1.26191942500002));
#348883=CARTESIAN_POINT('Ctrl Pts',(4.12544358599995,2.2,-1.26191942500002));
#348884=CARTESIAN_POINT('Ctrl Pts',(4.12401878699994,12.2,-1.26075746600002));
#348885=CARTESIAN_POINT('Ctrl Pts',(4.12401878699994,5.2,-1.26075746600002));
#348886=CARTESIAN_POINT('Ctrl Pts',(4.12401878699994,2.2,-1.26075746600002));
#348887=CARTESIAN_POINT('Ctrl Pts',(4.12259599199994,12.2,-1.25959981300001));
#348888=CARTESIAN_POINT('Ctrl Pts',(4.12259599199994,5.2,-1.25959981300001));
#348889=CARTESIAN_POINT('Ctrl Pts',(4.12259599199994,2.2,-1.25959981300001));
#348890=CARTESIAN_POINT('Ctrl Pts',(4.12117520999994,12.2,-1.25844646100001));
#348891=CARTESIAN_POINT('Ctrl Pts',(4.12117520999994,5.2,-1.25844646100001));
#348892=CARTESIAN_POINT('Ctrl Pts',(4.12117520999994,2.2,-1.25844646100001));
#348893=CARTESIAN_POINT('Ctrl Pts',(4.11975645499994,12.2,-1.25729741200002));
#348894=CARTESIAN_POINT('Ctrl Pts',(4.11975645499994,5.2,-1.25729741200002));
#348895=CARTESIAN_POINT('Ctrl Pts',(4.11975645499994,2.2,-1.25729741200002));
#348896=CARTESIAN_POINT('Ctrl Pts',(4.11833973699994,12.2,-1.25615266000001));
#348897=CARTESIAN_POINT('Ctrl Pts',(4.11833973699994,5.2,-1.25615266000001));
#348898=CARTESIAN_POINT('Ctrl Pts',(4.11833973699994,2.2,-1.25615266000001));
#348899=CARTESIAN_POINT('Ctrl Pts',(4.11692506799994,12.2,-1.25501220700002));
#348900=CARTESIAN_POINT('Ctrl Pts',(4.11692506799994,5.2,-1.25501220700002));
#348901=CARTESIAN_POINT('Ctrl Pts',(4.11692506799994,2.2,-1.25501220700002));
#348902=CARTESIAN_POINT('Ctrl Pts',(4.11551245899994,12.2,-1.25387604800002));
#348903=CARTESIAN_POINT('Ctrl Pts',(4.11551245899994,5.2,-1.25387604800002));
#348904=CARTESIAN_POINT('Ctrl Pts',(4.11551245899994,2.2,-1.25387604800002));
#348905=CARTESIAN_POINT('Ctrl Pts',(4.11410192199994,12.2,-1.25274418100001));
#348906=CARTESIAN_POINT('Ctrl Pts',(4.11410192199994,5.2,-1.25274418100001));
#348907=CARTESIAN_POINT('Ctrl Pts',(4.11410192199994,2.2,-1.25274418100001));
#348908=CARTESIAN_POINT('Ctrl Pts',(4.11269346899994,12.2,-1.25161660600002));
#348909=CARTESIAN_POINT('Ctrl Pts',(4.11269346899994,5.2,-1.25161660600002));
#348910=CARTESIAN_POINT('Ctrl Pts',(4.11269346899994,2.2,-1.25161660600002));
#348911=CARTESIAN_POINT('Ctrl Pts',(4.11128710999995,12.2,-1.25049332000001));
#348912=CARTESIAN_POINT('Ctrl Pts',(4.11128710999995,5.2,-1.25049332000001));
#348913=CARTESIAN_POINT('Ctrl Pts',(4.11128710999995,2.2,-1.25049332000001));
#348914=CARTESIAN_POINT('Ctrl Pts',(4.10988285899994,12.2,-1.24937432000001));
#348915=CARTESIAN_POINT('Ctrl Pts',(4.10988285899994,5.2,-1.24937432000001));
#348916=CARTESIAN_POINT('Ctrl Pts',(4.10988285899994,2.2,-1.24937432000001));
#348917=CARTESIAN_POINT('Ctrl Pts',(4.10848072599994,12.2,-1.24825960500001));
#348918=CARTESIAN_POINT('Ctrl Pts',(4.10848072599994,5.2,-1.24825960500001));
#348919=CARTESIAN_POINT('Ctrl Pts',(4.10848072599994,2.2,-1.24825960500001));
#348920=CARTESIAN_POINT('Ctrl Pts',(4.10708072299994,12.2,-1.24714917200002));
#348921=CARTESIAN_POINT('Ctrl Pts',(4.10708072299994,5.2,-1.24714917200002));
#348922=CARTESIAN_POINT('Ctrl Pts',(4.10708072299994,2.2,-1.24714917200002));
#348923=CARTESIAN_POINT('Ctrl Pts',(4.10568286099994,12.2,-1.24604302000002));
#348924=CARTESIAN_POINT('Ctrl Pts',(4.10568286099994,5.2,-1.24604302000002));
#348925=CARTESIAN_POINT('Ctrl Pts',(4.10568286099994,2.2,-1.24604302000002));
#348926=CARTESIAN_POINT('Ctrl Pts',(4.10428715299994,12.2,-1.24494114600001));
#348927=CARTESIAN_POINT('Ctrl Pts',(4.10428715299994,5.2,-1.24494114600001));
#348928=CARTESIAN_POINT('Ctrl Pts',(4.10428715299994,2.2,-1.24494114600001));
#348929=CARTESIAN_POINT('Ctrl Pts',(4.10289360999994,12.2,-1.24384354800001));
#348930=CARTESIAN_POINT('Ctrl Pts',(4.10289360999994,5.2,-1.24384354800001));
#348931=CARTESIAN_POINT('Ctrl Pts',(4.10289360999994,2.2,-1.24384354800001));
#348932=CARTESIAN_POINT('Ctrl Pts',(4.10150224399994,12.2,-1.24275022400001));
#348933=CARTESIAN_POINT('Ctrl Pts',(4.10150224399994,5.2,-1.24275022400001));
#348934=CARTESIAN_POINT('Ctrl Pts',(4.10150224399994,2.2,-1.24275022400001));
#348935=CARTESIAN_POINT('Ctrl Pts',(4.10011306599994,12.2,-1.24166117200001));
#348936=CARTESIAN_POINT('Ctrl Pts',(4.10011306599994,5.2,-1.24166117200001));
#348937=CARTESIAN_POINT('Ctrl Pts',(4.10011306599994,2.2,-1.24166117200001));
#348938=CARTESIAN_POINT('Ctrl Pts',(4.09872608799995,12.2,-1.24057638900001));
#348939=CARTESIAN_POINT('Ctrl Pts',(4.09872608799995,5.2,-1.24057638900001));
#348940=CARTESIAN_POINT('Ctrl Pts',(4.09872608799995,2.2,-1.24057638900001));
#348941=CARTESIAN_POINT('Ctrl Pts',(4.09734132199994,12.2,-1.23949587400002));
#348942=CARTESIAN_POINT('Ctrl Pts',(4.09734132199994,5.2,-1.23949587400002));
#348943=CARTESIAN_POINT('Ctrl Pts',(4.09734132199994,2.2,-1.23949587400002));
#348944=CARTESIAN_POINT('Ctrl Pts',(4.09595877899994,12.2,-1.23841962300002));
#348945=CARTESIAN_POINT('Ctrl Pts',(4.09595877899994,5.2,-1.23841962300002));
#348946=CARTESIAN_POINT('Ctrl Pts',(4.09595877899994,2.2,-1.23841962300002));
#348947=CARTESIAN_POINT('Ctrl Pts',(4.09457847299994,12.2,-1.23734763400002));
#348948=CARTESIAN_POINT('Ctrl Pts',(4.09457847299994,5.2,-1.23734763400002));
#348949=CARTESIAN_POINT('Ctrl Pts',(4.09457847299994,2.2,-1.23734763400002));
#348950=CARTESIAN_POINT('Ctrl Pts',(4.09320041299994,12.2,-1.23627990700002));
#348951=CARTESIAN_POINT('Ctrl Pts',(4.09320041299994,5.2,-1.23627990700002));
#348952=CARTESIAN_POINT('Ctrl Pts',(4.09320041299994,2.2,-1.23627990700002));
#348953=CARTESIAN_POINT('Ctrl Pts',(4.09182461299994,12.2,-1.23521643600002));
#348954=CARTESIAN_POINT('Ctrl Pts',(4.09182461299994,5.2,-1.23521643600002));
#348955=CARTESIAN_POINT('Ctrl Pts',(4.09182461299994,2.2,-1.23521643600002));
#348956=CARTESIAN_POINT('Ctrl Pts',(4.09045108399994,12.2,-1.23415722100002));
#348957=CARTESIAN_POINT('Ctrl Pts',(4.09045108399994,5.2,-1.23415722100002));
#348958=CARTESIAN_POINT('Ctrl Pts',(4.09045108399994,2.2,-1.23415722100002));
#348959=CARTESIAN_POINT('Ctrl Pts',(4.08907983799994,12.2,-1.23310226000001));
#348960=CARTESIAN_POINT('Ctrl Pts',(4.08907983799994,5.2,-1.23310226000001));
#348961=CARTESIAN_POINT('Ctrl Pts',(4.08907983799994,2.2,-1.23310226000001));
#348962=CARTESIAN_POINT('Ctrl Pts',(4.08771088599994,12.2,-1.23205154900001));
#348963=CARTESIAN_POINT('Ctrl Pts',(4.08771088599994,5.2,-1.23205154900001));
#348964=CARTESIAN_POINT('Ctrl Pts',(4.08771088599994,2.2,-1.23205154900001));
#348965=CARTESIAN_POINT('Ctrl Pts',(4.08634424099994,12.2,-1.23100508600002));
#348966=CARTESIAN_POINT('Ctrl Pts',(4.08634424099994,5.2,-1.23100508600002));
#348967=CARTESIAN_POINT('Ctrl Pts',(4.08634424099994,2.2,-1.23100508600002));
#348968=CARTESIAN_POINT('Ctrl Pts',(4.08497991499994,12.2,-1.22996287000001));
#348969=CARTESIAN_POINT('Ctrl Pts',(4.08497991499994,5.2,-1.22996287000001));
#348970=CARTESIAN_POINT('Ctrl Pts',(4.08497991499994,2.2,-1.22996287000001));
#348971=CARTESIAN_POINT('Ctrl Pts',(4.08361791899994,12.2,-1.22892489700002));
#348972=CARTESIAN_POINT('Ctrl Pts',(4.08361791899994,5.2,-1.22892489700002));
#348973=CARTESIAN_POINT('Ctrl Pts',(4.08361791899994,2.2,-1.22892489700002));
#348974=CARTESIAN_POINT('Ctrl Pts',(4.08225826499994,12.2,-1.22789116500002));
#348975=CARTESIAN_POINT('Ctrl Pts',(4.08225826499994,5.2,-1.22789116500002));
#348976=CARTESIAN_POINT('Ctrl Pts',(4.08225826499994,2.2,-1.22789116500002));
#348977=CARTESIAN_POINT('Ctrl Pts',(4.08090096699994,12.2,-1.22686167100001));
#348978=CARTESIAN_POINT('Ctrl Pts',(4.08090096699994,5.2,-1.22686167100001));
#348979=CARTESIAN_POINT('Ctrl Pts',(4.08090096699994,2.2,-1.22686167100001));
#348980=CARTESIAN_POINT('Ctrl Pts',(4.07954603499994,12.2,-1.22583641400002));
#348981=CARTESIAN_POINT('Ctrl Pts',(4.07954603499994,5.2,-1.22583641400002));
#348982=CARTESIAN_POINT('Ctrl Pts',(4.07954603499994,2.2,-1.22583641400002));
#348983=CARTESIAN_POINT('Ctrl Pts',(4.07819348099994,12.2,-1.22481538900002));
#348984=CARTESIAN_POINT('Ctrl Pts',(4.07819348099994,5.2,-1.22481538900002));
#348985=CARTESIAN_POINT('Ctrl Pts',(4.07819348099994,2.2,-1.22481538900002));
#348986=CARTESIAN_POINT('Ctrl Pts',(4.07684331699994,12.2,-1.22379859500001));
#348987=CARTESIAN_POINT('Ctrl Pts',(4.07684331699994,5.2,-1.22379859500001));
#348988=CARTESIAN_POINT('Ctrl Pts',(4.07684331699994,2.2,-1.22379859500001));
#348989=CARTESIAN_POINT('Ctrl Pts',(4.07549555599994,12.2,-1.22278602900002));
#348990=CARTESIAN_POINT('Ctrl Pts',(4.07549555599994,5.2,-1.22278602900002));
#348991=CARTESIAN_POINT('Ctrl Pts',(4.07549555599994,2.2,-1.22278602900002));
#348992=CARTESIAN_POINT('Ctrl Pts',(4.07415020999994,12.2,-1.22177768900002));
#348993=CARTESIAN_POINT('Ctrl Pts',(4.07415020999994,5.2,-1.22177768900002));
#348994=CARTESIAN_POINT('Ctrl Pts',(4.07415020999994,2.2,-1.22177768900002));
#348995=CARTESIAN_POINT('Ctrl Pts',(4.07280729099995,12.2,-1.22077357300002));
#348996=CARTESIAN_POINT('Ctrl Pts',(4.07280729099995,5.2,-1.22077357300002));
#348997=CARTESIAN_POINT('Ctrl Pts',(4.07280729099995,2.2,-1.22077357300002));
#348998=CARTESIAN_POINT('Ctrl Pts',(4.07146680999994,12.2,-1.21977367600001));
#348999=CARTESIAN_POINT('Ctrl Pts',(4.07146680999994,5.2,-1.21977367600001));
#349000=CARTESIAN_POINT('Ctrl Pts',(4.07146680999994,2.2,-1.21977367600001));
#349001=CARTESIAN_POINT('Ctrl Pts',(4.07012877999995,12.2,-1.21877799800002));
#349002=CARTESIAN_POINT('Ctrl Pts',(4.07012877999995,5.2,-1.21877799800002));
#349003=CARTESIAN_POINT('Ctrl Pts',(4.07012877999995,2.2,-1.21877799800002));
#349004=CARTESIAN_POINT('Ctrl Pts',(4.06879321399995,12.2,-1.21778653400002));
#349005=CARTESIAN_POINT('Ctrl Pts',(4.06879321399995,5.2,-1.21778653400002));
#349006=CARTESIAN_POINT('Ctrl Pts',(4.06879321399995,2.2,-1.21778653400002));
#349007=CARTESIAN_POINT('Ctrl Pts',(4.06746012299994,12.2,-1.21679928200002));
#349008=CARTESIAN_POINT('Ctrl Pts',(4.06746012299994,5.2,-1.21679928200002));
#349009=CARTESIAN_POINT('Ctrl Pts',(4.06746012299994,2.2,-1.21679928200002));
#349010=CARTESIAN_POINT('Ctrl Pts',(4.06612951899994,12.2,-1.21581624000001));
#349011=CARTESIAN_POINT('Ctrl Pts',(4.06612951899994,5.2,-1.21581624000001));
#349012=CARTESIAN_POINT('Ctrl Pts',(4.06612951899994,2.2,-1.21581624000001));
#349013=CARTESIAN_POINT('Ctrl Pts',(4.06480141499994,12.2,-1.21483740400001));
#349014=CARTESIAN_POINT('Ctrl Pts',(4.06480141499994,5.2,-1.21483740400001));
#349015=CARTESIAN_POINT('Ctrl Pts',(4.06480141499994,2.2,-1.21483740400001));
#349016=CARTESIAN_POINT('Ctrl Pts',(4.06347582299994,12.2,-1.21386277300001));
#349017=CARTESIAN_POINT('Ctrl Pts',(4.06347582299994,5.2,-1.21386277300001));
#349018=CARTESIAN_POINT('Ctrl Pts',(4.06347582299994,2.2,-1.21386277300001));
#349019=CARTESIAN_POINT('Ctrl Pts',(4.06215275499994,12.2,-1.21289234200002));
#349020=CARTESIAN_POINT('Ctrl Pts',(4.06215275499994,5.2,-1.21289234200002));
#349021=CARTESIAN_POINT('Ctrl Pts',(4.06215275499994,2.2,-1.21289234200002));
#349022=CARTESIAN_POINT('Ctrl Pts',(4.06083222399995,12.2,-1.21192611000001));
#349023=CARTESIAN_POINT('Ctrl Pts',(4.06083222399995,5.2,-1.21192611000001));
#349024=CARTESIAN_POINT('Ctrl Pts',(4.06083222399995,2.2,-1.21192611000001));
#349025=CARTESIAN_POINT('Ctrl Pts',(4.05951424099994,12.2,-1.21096407400001));
#349026=CARTESIAN_POINT('Ctrl Pts',(4.05951424099994,5.2,-1.21096407400001));
#349027=CARTESIAN_POINT('Ctrl Pts',(4.05951424099994,2.2,-1.21096407400001));
#349028=CARTESIAN_POINT('Ctrl Pts',(4.05819881799994,12.2,-1.21000623000001));
#349029=CARTESIAN_POINT('Ctrl Pts',(4.05819881799994,5.2,-1.21000623000001));
#349030=CARTESIAN_POINT('Ctrl Pts',(4.05819881799994,2.2,-1.21000623000001));
#349031=CARTESIAN_POINT('Ctrl Pts',(4.05688596999994,12.2,-1.20905257600001));
#349032=CARTESIAN_POINT('Ctrl Pts',(4.05688596999994,5.2,-1.20905257600001));
#349033=CARTESIAN_POINT('Ctrl Pts',(4.05688596999994,2.2,-1.20905257600001));
#349034=CARTESIAN_POINT('Ctrl Pts',(4.05557570699994,12.2,-1.20810310800001));
#349035=CARTESIAN_POINT('Ctrl Pts',(4.05557570699994,5.2,-1.20810310800001));
#349036=CARTESIAN_POINT('Ctrl Pts',(4.05557570699994,2.2,-1.20810310800001));
#349037=CARTESIAN_POINT('Ctrl Pts',(4.05426804299994,12.2,-1.20715782500001));
#349038=CARTESIAN_POINT('Ctrl Pts',(4.05426804299994,5.2,-1.20715782500001));
#349039=CARTESIAN_POINT('Ctrl Pts',(4.05426804299994,2.2,-1.20715782500001));
#349040=CARTESIAN_POINT('Ctrl Pts',(4.05296298799994,12.2,-1.20621672300001));
#349041=CARTESIAN_POINT('Ctrl Pts',(4.05296298799994,5.2,-1.20621672300001));
#349042=CARTESIAN_POINT('Ctrl Pts',(4.05296298799994,2.2,-1.20621672300001));
#349043=CARTESIAN_POINT('Ctrl Pts',(4.05166055699994,12.2,-1.20527979800002));
#349044=CARTESIAN_POINT('Ctrl Pts',(4.05166055699994,5.2,-1.20527979800002));
#349045=CARTESIAN_POINT('Ctrl Pts',(4.05166055699994,2.2,-1.20527979800002));
#349046=CARTESIAN_POINT('Ctrl Pts',(4.05036075999995,12.2,-1.20434704800001));
#349047=CARTESIAN_POINT('Ctrl Pts',(4.05036075999995,5.2,-1.20434704800001));
#349048=CARTESIAN_POINT('Ctrl Pts',(4.05036075999995,2.2,-1.20434704800001));
#349049=CARTESIAN_POINT('Ctrl Pts',(4.04906361199994,12.2,-1.20341847100002));
#349050=CARTESIAN_POINT('Ctrl Pts',(4.04906361199994,5.2,-1.20341847100002));
#349051=CARTESIAN_POINT('Ctrl Pts',(4.04906361199994,2.2,-1.20341847100002));
#349052=CARTESIAN_POINT('Ctrl Pts',(4.04776912299995,12.2,-1.20249406100001));
#349053=CARTESIAN_POINT('Ctrl Pts',(4.04776912299995,5.2,-1.20249406100001));
#349054=CARTESIAN_POINT('Ctrl Pts',(4.04776912299995,2.2,-1.20249406100001));
#349055=CARTESIAN_POINT('Ctrl Pts',(4.04647730599994,12.2,-1.20157381900002));
#349056=CARTESIAN_POINT('Ctrl Pts',(4.04647730599994,5.2,-1.20157381900002));
#349057=CARTESIAN_POINT('Ctrl Pts',(4.04647730599994,2.2,-1.20157381900002));
#349058=CARTESIAN_POINT('Ctrl Pts',(4.04518817599994,12.2,-1.20065773800001));
#349059=CARTESIAN_POINT('Ctrl Pts',(4.04518817599994,5.2,-1.20065773800001));
#349060=CARTESIAN_POINT('Ctrl Pts',(4.04518817599994,2.2,-1.20065773800001));
#349061=CARTESIAN_POINT('Ctrl Pts',(4.04390174199994,12.2,-1.19974581800002));
#349062=CARTESIAN_POINT('Ctrl Pts',(4.04390174199994,5.2,-1.19974581800002));
#349063=CARTESIAN_POINT('Ctrl Pts',(4.04390174199994,2.2,-1.19974581800002));
#349064=CARTESIAN_POINT('Ctrl Pts',(4.04261801999994,12.2,-1.19883805300002));
#349065=CARTESIAN_POINT('Ctrl Pts',(4.04261801999994,5.2,-1.19883805300002));
#349066=CARTESIAN_POINT('Ctrl Pts',(4.04261801999994,2.2,-1.19883805300002));
#349067=CARTESIAN_POINT('Ctrl Pts',(4.04133701899995,12.2,-1.19793444300001));
#349068=CARTESIAN_POINT('Ctrl Pts',(4.04133701899995,5.2,-1.19793444300001));
#349069=CARTESIAN_POINT('Ctrl Pts',(4.04133701899995,2.2,-1.19793444300001));
#349070=CARTESIAN_POINT('Ctrl Pts',(4.04005875299995,12.2,-1.19703498200002));
#349071=CARTESIAN_POINT('Ctrl Pts',(4.04005875299995,5.2,-1.19703498200002));
#349072=CARTESIAN_POINT('Ctrl Pts',(4.04005875299995,2.2,-1.19703498200002));
#349073=CARTESIAN_POINT('Ctrl Pts',(4.03878323699994,12.2,-1.19613966800001));
#349074=CARTESIAN_POINT('Ctrl Pts',(4.03878323699994,5.2,-1.19613966800001));
#349075=CARTESIAN_POINT('Ctrl Pts',(4.03878323699994,2.2,-1.19613966800001));
#349076=CARTESIAN_POINT('Ctrl Pts',(4.03751047999994,12.2,-1.19524849800001));
#349077=CARTESIAN_POINT('Ctrl Pts',(4.03751047999994,5.2,-1.19524849800001));
#349078=CARTESIAN_POINT('Ctrl Pts',(4.03751047999994,2.2,-1.19524849800001));
#349079=CARTESIAN_POINT('Ctrl Pts',(4.03624049699994,12.2,-1.19436146800001));
#349080=CARTESIAN_POINT('Ctrl Pts',(4.03624049699994,5.2,-1.19436146800001));
#349081=CARTESIAN_POINT('Ctrl Pts',(4.03624049699994,2.2,-1.19436146800001));
#349082=CARTESIAN_POINT('Ctrl Pts',(4.03497329899994,12.2,-1.19347857500001));
#349083=CARTESIAN_POINT('Ctrl Pts',(4.03497329899994,5.2,-1.19347857500001));
#349084=CARTESIAN_POINT('Ctrl Pts',(4.03497329899994,2.2,-1.19347857500001));
#349085=CARTESIAN_POINT('Ctrl Pts',(4.03370889999994,12.2,-1.19259981700001));
#349086=CARTESIAN_POINT('Ctrl Pts',(4.03370889999994,5.2,-1.19259981700001));
#349087=CARTESIAN_POINT('Ctrl Pts',(4.03370889999994,2.2,-1.19259981700001));
#349088=CARTESIAN_POINT('Ctrl Pts',(4.03244731199994,12.2,-1.19172518900001));
#349089=CARTESIAN_POINT('Ctrl Pts',(4.03244731199994,5.2,-1.19172518900001));
#349090=CARTESIAN_POINT('Ctrl Pts',(4.03244731199994,2.2,-1.19172518900001));
#349091=CARTESIAN_POINT('Ctrl Pts',(4.03118854799995,12.2,-1.19085468800002));
#349092=CARTESIAN_POINT('Ctrl Pts',(4.03118854799995,5.2,-1.19085468800002));
#349093=CARTESIAN_POINT('Ctrl Pts',(4.03118854799995,2.2,-1.19085468800002));
#349094=CARTESIAN_POINT('Ctrl Pts',(4.02993262099994,12.2,-1.18998831000001));
#349095=CARTESIAN_POINT('Ctrl Pts',(4.02993262099994,5.2,-1.18998831000001));
#349096=CARTESIAN_POINT('Ctrl Pts',(4.02993262099994,2.2,-1.18998831000001));
#349097=CARTESIAN_POINT('Ctrl Pts',(4.02867954299994,12.2,-1.18912605400002));
#349098=CARTESIAN_POINT('Ctrl Pts',(4.02867954299994,5.2,-1.18912605400002));
#349099=CARTESIAN_POINT('Ctrl Pts',(4.02867954299994,2.2,-1.18912605400002));
#349100=CARTESIAN_POINT('Ctrl Pts',(4.02742932799994,12.2,-1.18826791300001));
#349101=CARTESIAN_POINT('Ctrl Pts',(4.02742932799994,5.2,-1.18826791300001));
#349102=CARTESIAN_POINT('Ctrl Pts',(4.02742932799994,2.2,-1.18826791300001));
#349103=CARTESIAN_POINT('Ctrl Pts',(4.02618198699995,12.2,-1.18741388700002));
#349104=CARTESIAN_POINT('Ctrl Pts',(4.02618198699995,5.2,-1.18741388700002));
#349105=CARTESIAN_POINT('Ctrl Pts',(4.02618198699995,2.2,-1.18741388700002));
#349106=CARTESIAN_POINT('Ctrl Pts',(4.02493753399995,12.2,-1.18656397000001));
#349107=CARTESIAN_POINT('Ctrl Pts',(4.02493753399995,5.2,-1.18656397000001));
#349108=CARTESIAN_POINT('Ctrl Pts',(4.02493753399995,2.2,-1.18656397000001));
#349109=CARTESIAN_POINT('Ctrl Pts',(4.02369598199994,12.2,-1.18571816200001));
#349110=CARTESIAN_POINT('Ctrl Pts',(4.02369598199994,5.2,-1.18571816200001));
#349111=CARTESIAN_POINT('Ctrl Pts',(4.02369598199994,2.2,-1.18571816200001));
#349112=CARTESIAN_POINT('Ctrl Pts',(4.02245734399994,12.2,-1.18487645500001));
#349113=CARTESIAN_POINT('Ctrl Pts',(4.02245734399994,5.2,-1.18487645500001));
#349114=CARTESIAN_POINT('Ctrl Pts',(4.02245734399994,2.2,-1.18487645500001));
#349115=CARTESIAN_POINT('Ctrl Pts',(4.02122163199994,12.2,-1.18403884800002));
#349116=CARTESIAN_POINT('Ctrl Pts',(4.02122163199994,5.2,-1.18403884800002));
#349117=CARTESIAN_POINT('Ctrl Pts',(4.02122163199994,2.2,-1.18403884800002));
#349118=CARTESIAN_POINT('Ctrl Pts',(4.01998885999994,12.2,-1.18320533800001));
#349119=CARTESIAN_POINT('Ctrl Pts',(4.01998885999994,5.2,-1.18320533800001));
#349120=CARTESIAN_POINT('Ctrl Pts',(4.01998885999994,2.2,-1.18320533800001));
#349121=CARTESIAN_POINT('Ctrl Pts',(4.01875903999994,12.2,-1.18237591900002));
#349122=CARTESIAN_POINT('Ctrl Pts',(4.01875903999994,5.2,-1.18237591900002));
#349123=CARTESIAN_POINT('Ctrl Pts',(4.01875903999994,2.2,-1.18237591900002));
#349124=CARTESIAN_POINT('Ctrl Pts',(4.01753218399994,12.2,-1.18155058800001));
#349125=CARTESIAN_POINT('Ctrl Pts',(4.01753218399994,5.2,-1.18155058800001));
#349126=CARTESIAN_POINT('Ctrl Pts',(4.01753218399994,2.2,-1.18155058800001));
#349127=CARTESIAN_POINT('Ctrl Pts',(4.01630830799994,12.2,-1.18072934400002));
#349128=CARTESIAN_POINT('Ctrl Pts',(4.01630830799994,5.2,-1.18072934400002));
#349129=CARTESIAN_POINT('Ctrl Pts',(4.01630830799994,2.2,-1.18072934400002));
#349130=CARTESIAN_POINT('Ctrl Pts',(4.01508742299994,12.2,-1.17991218100002));
#349131=CARTESIAN_POINT('Ctrl Pts',(4.01508742299994,5.2,-1.17991218100002));
#349132=CARTESIAN_POINT('Ctrl Pts',(4.01508742299994,2.2,-1.17991218100002));
#349133=CARTESIAN_POINT('Ctrl Pts',(4.01386954199995,12.2,-1.17909909600002));
#349134=CARTESIAN_POINT('Ctrl Pts',(4.01386954199995,5.2,-1.17909909600002));
#349135=CARTESIAN_POINT('Ctrl Pts',(4.01386954199995,2.2,-1.17909909600002));
#349136=CARTESIAN_POINT('Ctrl Pts',(4.01265467899994,12.2,-1.17829008400001));
#349137=CARTESIAN_POINT('Ctrl Pts',(4.01265467899994,5.2,-1.17829008400001));
#349138=CARTESIAN_POINT('Ctrl Pts',(4.01265467899994,2.2,-1.17829008400001));
#349139=CARTESIAN_POINT('Ctrl Pts',(4.01144284499994,12.2,-1.17748514300001));
#349140=CARTESIAN_POINT('Ctrl Pts',(4.01144284499994,5.2,-1.17748514300001));
#349141=CARTESIAN_POINT('Ctrl Pts',(4.01144284499994,2.2,-1.17748514300001));
#349142=CARTESIAN_POINT('Ctrl Pts',(4.01023405599994,12.2,-1.17668426800002));
#349143=CARTESIAN_POINT('Ctrl Pts',(4.01023405599994,5.2,-1.17668426800002));
#349144=CARTESIAN_POINT('Ctrl Pts',(4.01023405599994,2.2,-1.17668426800002));
#349145=CARTESIAN_POINT('Ctrl Pts',(4.00902832299994,12.2,-1.17588745700001));
#349146=CARTESIAN_POINT('Ctrl Pts',(4.00902832299994,5.2,-1.17588745700001));
#349147=CARTESIAN_POINT('Ctrl Pts',(4.00902832299994,2.2,-1.17588745700001));
#349148=CARTESIAN_POINT('Ctrl Pts',(4.00782565899994,12.2,-1.17509470400002));
#349149=CARTESIAN_POINT('Ctrl Pts',(4.00782565899994,5.2,-1.17509470400002));
#349150=CARTESIAN_POINT('Ctrl Pts',(4.00782565899994,2.2,-1.17509470400002));
#349151=CARTESIAN_POINT('Ctrl Pts',(4.00662607899995,12.2,-1.17430600600001));
#349152=CARTESIAN_POINT('Ctrl Pts',(4.00662607899995,5.2,-1.17430600600001));
#349153=CARTESIAN_POINT('Ctrl Pts',(4.00662607899995,2.2,-1.17430600600001));
#349154=CARTESIAN_POINT('Ctrl Pts',(4.00542959399994,12.2,-1.17352136000001));
#349155=CARTESIAN_POINT('Ctrl Pts',(4.00542959399994,5.2,-1.17352136000001));
#349156=CARTESIAN_POINT('Ctrl Pts',(4.00542959399994,2.2,-1.17352136000001));
#349157=CARTESIAN_POINT('Ctrl Pts',(4.00423621899994,12.2,-1.17274076200002));
#349158=CARTESIAN_POINT('Ctrl Pts',(4.00423621899994,5.2,-1.17274076200002));
#349159=CARTESIAN_POINT('Ctrl Pts',(4.00423621899994,2.2,-1.17274076200002));
#349160=CARTESIAN_POINT('Ctrl Pts',(4.00304596699994,12.2,-1.17196420600001));
#349161=CARTESIAN_POINT('Ctrl Pts',(4.00304596699994,5.2,-1.17196420600001));
#349162=CARTESIAN_POINT('Ctrl Pts',(4.00304596699994,2.2,-1.17196420600001));
#349163=CARTESIAN_POINT('Ctrl Pts',(4.00185884899994,12.2,-1.17119169100001));
#349164=CARTESIAN_POINT('Ctrl Pts',(4.00185884899994,5.2,-1.17119169100001));
#349165=CARTESIAN_POINT('Ctrl Pts',(4.00185884899994,2.2,-1.17119169100001));
#349166=CARTESIAN_POINT('Ctrl Pts',(4.00067488099995,12.2,-1.17042321100001));
#349167=CARTESIAN_POINT('Ctrl Pts',(4.00067488099995,5.2,-1.17042321100001));
#349168=CARTESIAN_POINT('Ctrl Pts',(4.00067488099995,2.2,-1.17042321100001));
#349169=CARTESIAN_POINT('Ctrl Pts',(3.99949407599994,12.2,-1.16965876200001));
#349170=CARTESIAN_POINT('Ctrl Pts',(3.99949407599994,5.2,-1.16965876200001));
#349171=CARTESIAN_POINT('Ctrl Pts',(3.99949407599994,2.2,-1.16965876200001));
#349172=CARTESIAN_POINT('Ctrl Pts',(3.99831644599994,12.2,-1.16889834000002));
#349173=CARTESIAN_POINT('Ctrl Pts',(3.99831644599994,5.2,-1.16889834000002));
#349174=CARTESIAN_POINT('Ctrl Pts',(3.99831644599994,2.2,-1.16889834000002));
#349175=CARTESIAN_POINT('Ctrl Pts',(3.99714200399994,12.2,-1.16814194300002));
#349176=CARTESIAN_POINT('Ctrl Pts',(3.99714200399994,5.2,-1.16814194300002));
#349177=CARTESIAN_POINT('Ctrl Pts',(3.99714200399994,2.2,-1.16814194300002));
#349178=CARTESIAN_POINT('Ctrl Pts',(3.99597076499994,12.2,-1.16738956500001));
#349179=CARTESIAN_POINT('Ctrl Pts',(3.99597076499994,5.2,-1.16738956500001));
#349180=CARTESIAN_POINT('Ctrl Pts',(3.99597076499994,2.2,-1.16738956500001));
#349181=CARTESIAN_POINT('Ctrl Pts',(3.99480274199994,12.2,-1.16664120200001));
#349182=CARTESIAN_POINT('Ctrl Pts',(3.99480274199994,5.2,-1.16664120200001));
#349183=CARTESIAN_POINT('Ctrl Pts',(3.99480274199994,2.2,-1.16664120200001));
#349184=CARTESIAN_POINT('Ctrl Pts',(3.99363794799994,12.2,-1.16589685100001));
#349185=CARTESIAN_POINT('Ctrl Pts',(3.99363794799994,5.2,-1.16589685100001));
#349186=CARTESIAN_POINT('Ctrl Pts',(3.99363794799994,2.2,-1.16589685100001));
#349187=CARTESIAN_POINT('Ctrl Pts',(3.99247639599994,12.2,-1.16515650600002));
#349188=CARTESIAN_POINT('Ctrl Pts',(3.99247639599994,5.2,-1.16515650600002));
#349189=CARTESIAN_POINT('Ctrl Pts',(3.99247639599994,2.2,-1.16515650600002));
#349190=CARTESIAN_POINT('Ctrl Pts',(3.99131809999994,12.2,-1.16442016400002));
#349191=CARTESIAN_POINT('Ctrl Pts',(3.99131809999994,5.2,-1.16442016400002));
#349192=CARTESIAN_POINT('Ctrl Pts',(3.99131809999994,2.2,-1.16442016400002));
#349193=CARTESIAN_POINT('Ctrl Pts',(3.99016307399994,12.2,-1.16368782100002));
#349194=CARTESIAN_POINT('Ctrl Pts',(3.99016307399994,5.2,-1.16368782100002));
#349195=CARTESIAN_POINT('Ctrl Pts',(3.99016307399994,2.2,-1.16368782100002));
#349196=CARTESIAN_POINT('Ctrl Pts',(3.98901132899994,12.2,-1.16295947300001));
#349197=CARTESIAN_POINT('Ctrl Pts',(3.98901132899994,5.2,-1.16295947300001));
#349198=CARTESIAN_POINT('Ctrl Pts',(3.98901132899994,2.2,-1.16295947300001));
#349199=CARTESIAN_POINT('Ctrl Pts',(3.98786288299994,12.2,-1.16223511500001));
#349200=CARTESIAN_POINT('Ctrl Pts',(3.98786288299994,5.2,-1.16223511500001));
#349201=CARTESIAN_POINT('Ctrl Pts',(3.98786288299994,2.2,-1.16223511500001));
#349202=CARTESIAN_POINT('Ctrl Pts',(3.98671774499994,12.2,-1.16151474200001));
#349203=CARTESIAN_POINT('Ctrl Pts',(3.98671774499994,5.2,-1.16151474200001));
#349204=CARTESIAN_POINT('Ctrl Pts',(3.98671774499994,2.2,-1.16151474200001));
#349205=CARTESIAN_POINT('Ctrl Pts',(3.98557593099994,12.2,-1.16079835100001));
#349206=CARTESIAN_POINT('Ctrl Pts',(3.98557593099994,5.2,-1.16079835100001));
#349207=CARTESIAN_POINT('Ctrl Pts',(3.98557593099994,2.2,-1.16079835100001));
#349208=CARTESIAN_POINT('Ctrl Pts',(3.98443745399994,12.2,-1.16008593800002));
#349209=CARTESIAN_POINT('Ctrl Pts',(3.98443745399994,5.2,-1.16008593800002));
#349210=CARTESIAN_POINT('Ctrl Pts',(3.98443745399994,2.2,-1.16008593800002));
#349211=CARTESIAN_POINT('Ctrl Pts',(3.98330232899994,12.2,-1.15937749700001));
#349212=CARTESIAN_POINT('Ctrl Pts',(3.98330232899994,5.2,-1.15937749700001));
#349213=CARTESIAN_POINT('Ctrl Pts',(3.98330232899994,2.2,-1.15937749700001));
#349214=CARTESIAN_POINT('Ctrl Pts',(3.98217056699994,12.2,-1.15867302500002));
#349215=CARTESIAN_POINT('Ctrl Pts',(3.98217056699994,5.2,-1.15867302500002));
#349216=CARTESIAN_POINT('Ctrl Pts',(3.98217056699994,2.2,-1.15867302500002));
#349217=CARTESIAN_POINT('Ctrl Pts',(3.98104218299994,12.2,-1.15797251600001));
#349218=CARTESIAN_POINT('Ctrl Pts',(3.98104218299994,5.2,-1.15797251600001));
#349219=CARTESIAN_POINT('Ctrl Pts',(3.98104218299994,2.2,-1.15797251600001));
#349220=CARTESIAN_POINT('Ctrl Pts',(3.97991719099994,12.2,-1.15727596800001));
#349221=CARTESIAN_POINT('Ctrl Pts',(3.97991719099994,5.2,-1.15727596800001));
#349222=CARTESIAN_POINT('Ctrl Pts',(3.97991719099994,2.2,-1.15727596800001));
#349223=CARTESIAN_POINT('Ctrl Pts',(3.97879560399994,12.2,-1.15658337500002));
#349224=CARTESIAN_POINT('Ctrl Pts',(3.97879560399994,5.2,-1.15658337500002));
#349225=CARTESIAN_POINT('Ctrl Pts',(3.97879560399994,2.2,-1.15658337500002));
#349226=CARTESIAN_POINT('Ctrl Pts',(3.97767743699994,12.2,-1.15589473300002));
#349227=CARTESIAN_POINT('Ctrl Pts',(3.97767743699994,5.2,-1.15589473300002));
#349228=CARTESIAN_POINT('Ctrl Pts',(3.97767743699994,2.2,-1.15589473300002));
#349229=CARTESIAN_POINT('Ctrl Pts',(3.97656270199994,12.2,-1.15521003600001));
#349230=CARTESIAN_POINT('Ctrl Pts',(3.97656270199994,5.2,-1.15521003600001));
#349231=CARTESIAN_POINT('Ctrl Pts',(3.97656270199994,2.2,-1.15521003600001));
#349232=CARTESIAN_POINT('Ctrl Pts',(3.97545141399994,12.2,-1.15452928100002));
#349233=CARTESIAN_POINT('Ctrl Pts',(3.97545141399994,5.2,-1.15452928100002));
#349234=CARTESIAN_POINT('Ctrl Pts',(3.97545141399994,2.2,-1.15452928100002));
#349235=CARTESIAN_POINT('Ctrl Pts',(3.97434358599994,12.2,-1.15385246300002));
#349236=CARTESIAN_POINT('Ctrl Pts',(3.97434358599994,5.2,-1.15385246300002));
#349237=CARTESIAN_POINT('Ctrl Pts',(3.97434358599994,2.2,-1.15385246300002));
#349238=CARTESIAN_POINT('Ctrl Pts',(3.97323923299994,12.2,-1.15317957800002));
#349239=CARTESIAN_POINT('Ctrl Pts',(3.97323923299994,5.2,-1.15317957800002));
#349240=CARTESIAN_POINT('Ctrl Pts',(3.97323923299994,2.2,-1.15317957800002));
#349241=CARTESIAN_POINT('Ctrl Pts',(3.97213836699994,12.2,-1.15251062000001));
#349242=CARTESIAN_POINT('Ctrl Pts',(3.97213836699994,5.2,-1.15251062000001));
#349243=CARTESIAN_POINT('Ctrl Pts',(3.97213836699994,2.2,-1.15251062000001));
#349244=CARTESIAN_POINT('Ctrl Pts',(3.97104100499994,12.2,-1.15184558400002));
#349245=CARTESIAN_POINT('Ctrl Pts',(3.97104100499994,5.2,-1.15184558400002));
#349246=CARTESIAN_POINT('Ctrl Pts',(3.97104100499994,2.2,-1.15184558400002));
#349247=CARTESIAN_POINT('Ctrl Pts',(3.96994715599994,12.2,-1.15118446800002));
#349248=CARTESIAN_POINT('Ctrl Pts',(3.96994715599994,5.2,-1.15118446800002));
#349249=CARTESIAN_POINT('Ctrl Pts',(3.96994715599994,2.2,-1.15118446800002));
#349250=CARTESIAN_POINT('Ctrl Pts',(3.96885683999994,12.2,-1.15052726600001));
#349251=CARTESIAN_POINT('Ctrl Pts',(3.96885683999994,5.2,-1.15052726600001));
#349252=CARTESIAN_POINT('Ctrl Pts',(3.96885683999994,2.2,-1.15052726600001));
#349253=CARTESIAN_POINT('Ctrl Pts',(3.96777006599994,12.2,-1.14987397200002));
#349254=CARTESIAN_POINT('Ctrl Pts',(3.96777006599994,5.2,-1.14987397200002));
#349255=CARTESIAN_POINT('Ctrl Pts',(3.96777006599994,2.2,-1.14987397200002));
#349256=CARTESIAN_POINT('Ctrl Pts',(3.96668684899994,12.2,-1.14922458200001));
#349257=CARTESIAN_POINT('Ctrl Pts',(3.96668684899994,5.2,-1.14922458200001));
#349258=CARTESIAN_POINT('Ctrl Pts',(3.96668684899994,2.2,-1.14922458200001));
#349259=CARTESIAN_POINT('Ctrl Pts',(3.96560720599994,12.2,-1.14857909000001));
#349260=CARTESIAN_POINT('Ctrl Pts',(3.96560720599994,5.2,-1.14857909000001));
#349261=CARTESIAN_POINT('Ctrl Pts',(3.96560720599994,2.2,-1.14857909000001));
#349262=CARTESIAN_POINT('Ctrl Pts',(3.96453114699994,12.2,-1.14793749400001));
#349263=CARTESIAN_POINT('Ctrl Pts',(3.96453114699994,5.2,-1.14793749400001));
#349264=CARTESIAN_POINT('Ctrl Pts',(3.96453114699994,2.2,-1.14793749400001));
#349265=CARTESIAN_POINT('Ctrl Pts',(3.96345868799994,12.2,-1.14729978700002));
#349266=CARTESIAN_POINT('Ctrl Pts',(3.96345868799994,5.2,-1.14729978700002));
#349267=CARTESIAN_POINT('Ctrl Pts',(3.96345868799994,2.2,-1.14729978700002));
#349268=CARTESIAN_POINT('Ctrl Pts',(3.96238984399994,12.2,-1.14666596600001));
#349269=CARTESIAN_POINT('Ctrl Pts',(3.96238984399994,5.2,-1.14666596600001));
#349270=CARTESIAN_POINT('Ctrl Pts',(3.96238984399994,2.2,-1.14666596600001));
#349271=CARTESIAN_POINT('Ctrl Pts',(3.96132462599994,12.2,-1.14603602300001));
#349272=CARTESIAN_POINT('Ctrl Pts',(3.96132462599994,5.2,-1.14603602300001));
#349273=CARTESIAN_POINT('Ctrl Pts',(3.96132462599994,2.2,-1.14603602300001));
#349274=CARTESIAN_POINT('Ctrl Pts',(3.96026305099995,12.2,-1.14540995500001));
#349275=CARTESIAN_POINT('Ctrl Pts',(3.96026305099995,5.2,-1.14540995500001));
#349276=CARTESIAN_POINT('Ctrl Pts',(3.96026305099995,2.2,-1.14540995500001));
#349277=CARTESIAN_POINT('Ctrl Pts',(3.95920513399994,12.2,-1.14478775700002));
#349278=CARTESIAN_POINT('Ctrl Pts',(3.95920513399994,5.2,-1.14478775700002));
#349279=CARTESIAN_POINT('Ctrl Pts',(3.95920513399994,2.2,-1.14478775700002));
#349280=CARTESIAN_POINT('Ctrl Pts',(3.95815088599994,12.2,-1.14416942400001));
#349281=CARTESIAN_POINT('Ctrl Pts',(3.95815088599994,5.2,-1.14416942400001));
#349282=CARTESIAN_POINT('Ctrl Pts',(3.95815088599994,2.2,-1.14416942400001));
#349283=CARTESIAN_POINT('Ctrl Pts',(3.95710032199994,12.2,-1.14355494900002));
#349284=CARTESIAN_POINT('Ctrl Pts',(3.95710032199994,5.2,-1.14355494900002));
#349285=CARTESIAN_POINT('Ctrl Pts',(3.95710032199994,2.2,-1.14355494900002));
#349286=CARTESIAN_POINT('Ctrl Pts',(3.95605345899994,12.2,-1.14294433000001));
#349287=CARTESIAN_POINT('Ctrl Pts',(3.95605345899994,5.2,-1.14294433000001));
#349288=CARTESIAN_POINT('Ctrl Pts',(3.95605345899994,2.2,-1.14294433000001));
#349289=CARTESIAN_POINT('Ctrl Pts',(3.95501030799994,12.2,-1.14233756100001));
#349290=CARTESIAN_POINT('Ctrl Pts',(3.95501030799994,5.2,-1.14233756100001));
#349291=CARTESIAN_POINT('Ctrl Pts',(3.95501030799994,2.2,-1.14233756100001));
#349292=CARTESIAN_POINT('Ctrl Pts',(3.95397088399994,12.2,-1.14173463500002));
#349293=CARTESIAN_POINT('Ctrl Pts',(3.95397088399994,5.2,-1.14173463500002));
#349294=CARTESIAN_POINT('Ctrl Pts',(3.95397088399994,2.2,-1.14173463500002));
#349295=CARTESIAN_POINT('Ctrl Pts',(3.95293520099994,12.2,-1.14113554900001));
#349296=CARTESIAN_POINT('Ctrl Pts',(3.95293520099994,5.2,-1.14113554900001));
#349297=CARTESIAN_POINT('Ctrl Pts',(3.95293520099994,2.2,-1.14113554900001));
#349298=CARTESIAN_POINT('Ctrl Pts',(3.95190327599994,12.2,-1.14054029600001));
#349299=CARTESIAN_POINT('Ctrl Pts',(3.95190327599994,5.2,-1.14054029600001));
#349300=CARTESIAN_POINT('Ctrl Pts',(3.95190327599994,2.2,-1.14054029600001));
#349301=CARTESIAN_POINT('Ctrl Pts',(3.95087511999995,12.2,-1.13994887300001));
#349302=CARTESIAN_POINT('Ctrl Pts',(3.95087511999995,5.2,-1.13994887300001));
#349303=CARTESIAN_POINT('Ctrl Pts',(3.95087511999995,2.2,-1.13994887300001));
#349304=CARTESIAN_POINT('Ctrl Pts',(3.94985074899994,12.2,-1.13936127100001));
#349305=CARTESIAN_POINT('Ctrl Pts',(3.94985074899994,5.2,-1.13936127100001));
#349306=CARTESIAN_POINT('Ctrl Pts',(3.94985074899994,2.2,-1.13936127100001));
#349307=CARTESIAN_POINT('Ctrl Pts',(3.94883017799994,12.2,-1.13877749000002));
#349308=CARTESIAN_POINT('Ctrl Pts',(3.94883017799994,5.2,-1.13877749000002));
#349309=CARTESIAN_POINT('Ctrl Pts',(3.94883017799994,2.2,-1.13877749000002));
#349310=CARTESIAN_POINT('Ctrl Pts',(3.94781342099995,12.2,-1.13819752000001));
#349311=CARTESIAN_POINT('Ctrl Pts',(3.94781342099995,5.2,-1.13819752000001));
#349312=CARTESIAN_POINT('Ctrl Pts',(3.94781342099995,2.2,-1.13819752000001));
#349313=CARTESIAN_POINT('Ctrl Pts',(3.94680049099994,12.2,-1.13762135800001));
#349314=CARTESIAN_POINT('Ctrl Pts',(3.94680049099994,5.2,-1.13762135800001));
#349315=CARTESIAN_POINT('Ctrl Pts',(3.94680049099994,2.2,-1.13762135800001));
#349316=CARTESIAN_POINT('Ctrl Pts',(3.94579140499994,12.2,-1.13704899800001));
#349317=CARTESIAN_POINT('Ctrl Pts',(3.94579140499994,5.2,-1.13704899800001));
#349318=CARTESIAN_POINT('Ctrl Pts',(3.94579140499994,2.2,-1.13704899800001));
#349319=CARTESIAN_POINT('Ctrl Pts',(3.94478617499994,12.2,-1.13648043400001));
#349320=CARTESIAN_POINT('Ctrl Pts',(3.94478617499994,5.2,-1.13648043400001));
#349321=CARTESIAN_POINT('Ctrl Pts',(3.94478617499994,2.2,-1.13648043400001));
#349322=CARTESIAN_POINT('Ctrl Pts',(3.94378481699994,12.2,-1.13591566200002));
#349323=CARTESIAN_POINT('Ctrl Pts',(3.94378481699994,5.2,-1.13591566200002));
#349324=CARTESIAN_POINT('Ctrl Pts',(3.94378481699994,2.2,-1.13591566200002));
#349325=CARTESIAN_POINT('Ctrl Pts',(3.94278734499994,12.2,-1.13535467600002));
#349326=CARTESIAN_POINT('Ctrl Pts',(3.94278734499994,5.2,-1.13535467600002));
#349327=CARTESIAN_POINT('Ctrl Pts',(3.94278734499994,2.2,-1.13535467600002));
#349328=CARTESIAN_POINT('Ctrl Pts',(3.94179377499994,12.2,-1.13479746900001));
#349329=CARTESIAN_POINT('Ctrl Pts',(3.94179377499994,5.2,-1.13479746900001));
#349330=CARTESIAN_POINT('Ctrl Pts',(3.94179377499994,2.2,-1.13479746900001));
#349331=CARTESIAN_POINT('Ctrl Pts',(3.94080411899994,12.2,-1.13424403700002));
#349332=CARTESIAN_POINT('Ctrl Pts',(3.94080411899994,5.2,-1.13424403700002));
#349333=CARTESIAN_POINT('Ctrl Pts',(3.94080411899994,2.2,-1.13424403700002));
#349334=CARTESIAN_POINT('Ctrl Pts',(3.93981839399994,12.2,-1.13369437400001));
#349335=CARTESIAN_POINT('Ctrl Pts',(3.93981839399994,5.2,-1.13369437400001));
#349336=CARTESIAN_POINT('Ctrl Pts',(3.93981839399994,2.2,-1.13369437400001));
#349337=CARTESIAN_POINT('Ctrl Pts',(3.93883661399994,12.2,-1.13314847400002));
#349338=CARTESIAN_POINT('Ctrl Pts',(3.93883661399994,5.2,-1.13314847400002));
#349339=CARTESIAN_POINT('Ctrl Pts',(3.93883661399994,2.2,-1.13314847400002));
#349340=CARTESIAN_POINT('Ctrl Pts',(3.93785879399994,12.2,-1.13260633200001));
#349341=CARTESIAN_POINT('Ctrl Pts',(3.93785879399994,5.2,-1.13260633200001));
#349342=CARTESIAN_POINT('Ctrl Pts',(3.93785879399994,2.2,-1.13260633200001));
#349343=CARTESIAN_POINT('Ctrl Pts',(3.93688494699994,12.2,-1.13206794200002));
#349344=CARTESIAN_POINT('Ctrl Pts',(3.93688494699994,5.2,-1.13206794200002));
#349345=CARTESIAN_POINT('Ctrl Pts',(3.93688494699994,2.2,-1.13206794200002));
#349346=CARTESIAN_POINT('Ctrl Pts',(3.93591508999994,12.2,-1.13153329900001));
#349347=CARTESIAN_POINT('Ctrl Pts',(3.93591508999994,5.2,-1.13153329900001));
#349348=CARTESIAN_POINT('Ctrl Pts',(3.93591508999994,2.2,-1.13153329900001));
#349349=CARTESIAN_POINT('Ctrl Pts',(3.93494923699994,12.2,-1.13100239600001));
#349350=CARTESIAN_POINT('Ctrl Pts',(3.93494923699994,5.2,-1.13100239600001));
#349351=CARTESIAN_POINT('Ctrl Pts',(3.93494923699994,2.2,-1.13100239600001));
#349352=CARTESIAN_POINT('Ctrl Pts',(3.93398740299994,12.2,-1.13047522900001));
#349353=CARTESIAN_POINT('Ctrl Pts',(3.93398740299994,5.2,-1.13047522900001));
#349354=CARTESIAN_POINT('Ctrl Pts',(3.93398740299994,2.2,-1.13047522900001));
#349355=CARTESIAN_POINT('Ctrl Pts',(3.93302960199994,12.2,-1.12995179000002));
#349356=CARTESIAN_POINT('Ctrl Pts',(3.93302960199994,5.2,-1.12995179000002));
#349357=CARTESIAN_POINT('Ctrl Pts',(3.93302960199994,2.2,-1.12995179000002));
#349358=CARTESIAN_POINT('Ctrl Pts',(3.93207584999994,12.2,-1.12943207300002));
#349359=CARTESIAN_POINT('Ctrl Pts',(3.93207584999994,5.2,-1.12943207300002));
#349360=CARTESIAN_POINT('Ctrl Pts',(3.93207584999994,2.2,-1.12943207300002));
#349361=CARTESIAN_POINT('Ctrl Pts',(3.93112616099994,12.2,-1.12891607400002));
#349362=CARTESIAN_POINT('Ctrl Pts',(3.93112616099994,5.2,-1.12891607400002));
#349363=CARTESIAN_POINT('Ctrl Pts',(3.93112616099994,2.2,-1.12891607400002));
#349364=CARTESIAN_POINT('Ctrl Pts',(3.93018054999994,12.2,-1.12840378800001));
#349365=CARTESIAN_POINT('Ctrl Pts',(3.93018054999994,5.2,-1.12840378800001));
#349366=CARTESIAN_POINT('Ctrl Pts',(3.93018054999994,2.2,-1.12840378800001));
#349367=CARTESIAN_POINT('Ctrl Pts',(3.92923903199994,12.2,-1.12789520600002));
#349368=CARTESIAN_POINT('Ctrl Pts',(3.92923903199994,5.2,-1.12789520600002));
#349369=CARTESIAN_POINT('Ctrl Pts',(3.92923903199994,2.2,-1.12789520600002));
#349370=CARTESIAN_POINT('Ctrl Pts',(3.92830162399994,12.2,-1.12739032400002));
#349371=CARTESIAN_POINT('Ctrl Pts',(3.92830162399994,5.2,-1.12739032400002));
#349372=CARTESIAN_POINT('Ctrl Pts',(3.92830162399994,2.2,-1.12739032400002));
#349373=CARTESIAN_POINT('Ctrl Pts',(3.92736833799994,12.2,-1.12688913500001));
#349374=CARTESIAN_POINT('Ctrl Pts',(3.92736833799994,5.2,-1.12688913500001));
#349375=CARTESIAN_POINT('Ctrl Pts',(3.92736833799994,2.2,-1.12688913500001));
#349376=CARTESIAN_POINT('Ctrl Pts',(3.92643918999994,12.2,-1.12639163300001));
#349377=CARTESIAN_POINT('Ctrl Pts',(3.92643918999994,5.2,-1.12639163300001));
#349378=CARTESIAN_POINT('Ctrl Pts',(3.92643918999994,2.2,-1.12639163300001));
#349379=CARTESIAN_POINT('Ctrl Pts',(3.92551419599994,12.2,-1.12589781300001));
#349380=CARTESIAN_POINT('Ctrl Pts',(3.92551419599994,5.2,-1.12589781300001));
#349381=CARTESIAN_POINT('Ctrl Pts',(3.92551419599994,2.2,-1.12589781300001));
#349382=CARTESIAN_POINT('Ctrl Pts',(3.92459337099994,12.2,-1.12540766800001));
#349383=CARTESIAN_POINT('Ctrl Pts',(3.92459337099994,5.2,-1.12540766800001));
#349384=CARTESIAN_POINT('Ctrl Pts',(3.92459337099994,2.2,-1.12540766800001));
#349385=CARTESIAN_POINT('Ctrl Pts',(3.92367672899994,12.2,-1.12492119200001));
#349386=CARTESIAN_POINT('Ctrl Pts',(3.92367672899994,5.2,-1.12492119200001));
#349387=CARTESIAN_POINT('Ctrl Pts',(3.92367672899994,2.2,-1.12492119200001));
#349388=CARTESIAN_POINT('Ctrl Pts',(3.92276428599994,12.2,-1.12443837900001));
#349389=CARTESIAN_POINT('Ctrl Pts',(3.92276428599994,5.2,-1.12443837900001));
#349390=CARTESIAN_POINT('Ctrl Pts',(3.92276428599994,2.2,-1.12443837900001));
#349391=CARTESIAN_POINT('Ctrl Pts',(3.92185605799994,12.2,-1.12395922300002));
#349392=CARTESIAN_POINT('Ctrl Pts',(3.92185605799994,5.2,-1.12395922300002));
#349393=CARTESIAN_POINT('Ctrl Pts',(3.92185605799994,2.2,-1.12395922300002));
#349394=CARTESIAN_POINT('Ctrl Pts',(3.92095205899994,12.2,-1.12348371700001));
#349395=CARTESIAN_POINT('Ctrl Pts',(3.92095205899994,5.2,-1.12348371700001));
#349396=CARTESIAN_POINT('Ctrl Pts',(3.92095205899994,2.2,-1.12348371700001));
#349397=CARTESIAN_POINT('Ctrl Pts',(3.92005230299994,12.2,-1.12301185500002));
#349398=CARTESIAN_POINT('Ctrl Pts',(3.92005230299994,5.2,-1.12301185500002));
#349399=CARTESIAN_POINT('Ctrl Pts',(3.92005230299994,2.2,-1.12301185500002));
#349400=CARTESIAN_POINT('Ctrl Pts',(3.91915680899994,12.2,-1.12254363000002));
#349401=CARTESIAN_POINT('Ctrl Pts',(3.91915680899994,5.2,-1.12254363000002));
#349402=CARTESIAN_POINT('Ctrl Pts',(3.91915680899994,2.2,-1.12254363000002));
#349403=CARTESIAN_POINT('Ctrl Pts',(3.91826558899994,12.2,-1.12207903800002));
#349404=CARTESIAN_POINT('Ctrl Pts',(3.91826558899994,5.2,-1.12207903800002));
#349405=CARTESIAN_POINT('Ctrl Pts',(3.91826558899994,2.2,-1.12207903800002));
#349406=CARTESIAN_POINT('Ctrl Pts',(3.91737865999994,12.2,-1.12161807000001));
#349407=CARTESIAN_POINT('Ctrl Pts',(3.91737865999994,5.2,-1.12161807000001));
#349408=CARTESIAN_POINT('Ctrl Pts',(3.91737865999994,2.2,-1.12161807000001));
#349409=CARTESIAN_POINT('Ctrl Pts',(3.91649603699994,12.2,-1.12116072100001));
#349410=CARTESIAN_POINT('Ctrl Pts',(3.91649603699994,5.2,-1.12116072100001));
#349411=CARTESIAN_POINT('Ctrl Pts',(3.91649603699994,2.2,-1.12116072100001));
#349412=CARTESIAN_POINT('Ctrl Pts',(3.91561773599994,12.2,-1.12070698400002));
#349413=CARTESIAN_POINT('Ctrl Pts',(3.91561773599994,5.2,-1.12070698400002));
#349414=CARTESIAN_POINT('Ctrl Pts',(3.91561773599994,2.2,-1.12070698400002));
#349415=CARTESIAN_POINT('Ctrl Pts',(3.91474376999994,12.2,-1.12025685300001));
#349416=CARTESIAN_POINT('Ctrl Pts',(3.91474376999994,5.2,-1.12025685300001));
#349417=CARTESIAN_POINT('Ctrl Pts',(3.91474376999994,2.2,-1.12025685300001));
#349418=CARTESIAN_POINT('Ctrl Pts',(3.91387415799994,12.2,-1.11981032100001));
#349419=CARTESIAN_POINT('Ctrl Pts',(3.91387415799994,5.2,-1.11981032100001));
#349420=CARTESIAN_POINT('Ctrl Pts',(3.91387415799994,2.2,-1.11981032100001));
#349421=CARTESIAN_POINT('Ctrl Pts',(3.91300891299994,12.2,-1.11936738000002));
#349422=CARTESIAN_POINT('Ctrl Pts',(3.91300891299994,5.2,-1.11936738000002));
#349423=CARTESIAN_POINT('Ctrl Pts',(3.91300891299994,2.2,-1.11936738000002));
#349424=CARTESIAN_POINT('Ctrl Pts',(3.91214805199994,12.2,-1.11892802700002));
#349425=CARTESIAN_POINT('Ctrl Pts',(3.91214805199994,5.2,-1.11892802700002));
#349426=CARTESIAN_POINT('Ctrl Pts',(3.91214805199994,2.2,-1.11892802700002));
#349427=CARTESIAN_POINT('Ctrl Pts',(3.91129158899994,12.2,-1.11849225200002));
#349428=CARTESIAN_POINT('Ctrl Pts',(3.91129158899994,5.2,-1.11849225200002));
#349429=CARTESIAN_POINT('Ctrl Pts',(3.91129158899994,2.2,-1.11849225200002));
#349430=CARTESIAN_POINT('Ctrl Pts',(3.91043954099994,12.2,-1.11806005100001));
#349431=CARTESIAN_POINT('Ctrl Pts',(3.91043954099994,5.2,-1.11806005100001));
#349432=CARTESIAN_POINT('Ctrl Pts',(3.91043954099994,2.2,-1.11806005100001));
#349433=CARTESIAN_POINT('Ctrl Pts',(3.90959192299994,12.2,-1.11763141400001));
#349434=CARTESIAN_POINT('Ctrl Pts',(3.90959192299994,5.2,-1.11763141400001));
#349435=CARTESIAN_POINT('Ctrl Pts',(3.90959192299994,2.2,-1.11763141400001));
#349436=CARTESIAN_POINT('Ctrl Pts',(3.90874875099994,12.2,-1.11720633700001));
#349437=CARTESIAN_POINT('Ctrl Pts',(3.90874875099994,5.2,-1.11720633700001));
#349438=CARTESIAN_POINT('Ctrl Pts',(3.90874875099994,2.2,-1.11720633700001));
#349439=CARTESIAN_POINT('Ctrl Pts',(3.90791004099994,12.2,-1.11678481200002));
#349440=CARTESIAN_POINT('Ctrl Pts',(3.90791004099994,5.2,-1.11678481200002));
#349441=CARTESIAN_POINT('Ctrl Pts',(3.90791004099994,2.2,-1.11678481200002));
#349442=CARTESIAN_POINT('Ctrl Pts',(3.90707580699994,12.2,-1.11636683300001));
#349443=CARTESIAN_POINT('Ctrl Pts',(3.90707580699994,5.2,-1.11636683300001));
#349444=CARTESIAN_POINT('Ctrl Pts',(3.90707580699994,2.2,-1.11636683300001));
#349445=CARTESIAN_POINT('Ctrl Pts',(3.90624606799994,12.2,-1.11595239200001));
#349446=CARTESIAN_POINT('Ctrl Pts',(3.90624606799994,5.2,-1.11595239200001));
#349447=CARTESIAN_POINT('Ctrl Pts',(3.90624606799994,2.2,-1.11595239200001));
#349448=CARTESIAN_POINT('Ctrl Pts',(3.90542083599994,12.2,-1.11554148300002));
#349449=CARTESIAN_POINT('Ctrl Pts',(3.90542083599994,5.2,-1.11554148300002));
#349450=CARTESIAN_POINT('Ctrl Pts',(3.90542083599994,2.2,-1.11554148300002));
#349451=CARTESIAN_POINT('Ctrl Pts',(3.90460012899994,12.2,-1.11513409800001));
#349452=CARTESIAN_POINT('Ctrl Pts',(3.90460012899994,5.2,-1.11513409800001));
#349453=CARTESIAN_POINT('Ctrl Pts',(3.90460012899994,2.2,-1.11513409800001));
#349454=CARTESIAN_POINT('Ctrl Pts',(3.90378396299994,12.2,-1.11473023200002));
#349455=CARTESIAN_POINT('Ctrl Pts',(3.90378396299994,5.2,-1.11473023200002));
#349456=CARTESIAN_POINT('Ctrl Pts',(3.90378396299994,2.2,-1.11473023200002));
#349457=CARTESIAN_POINT('Ctrl Pts',(3.90297235299994,12.2,-1.11432987500002));
#349458=CARTESIAN_POINT('Ctrl Pts',(3.90297235299994,5.2,-1.11432987500002));
#349459=CARTESIAN_POINT('Ctrl Pts',(3.90297235299994,2.2,-1.11432987500002));
#349460=CARTESIAN_POINT('Ctrl Pts',(3.90216531599994,12.2,-1.11393302300002));
#349461=CARTESIAN_POINT('Ctrl Pts',(3.90216531599994,5.2,-1.11393302300002));
#349462=CARTESIAN_POINT('Ctrl Pts',(3.90216531599994,2.2,-1.11393302300002));
#349463=CARTESIAN_POINT('Ctrl Pts',(3.90136286599994,12.2,-1.11353966700001));
#349464=CARTESIAN_POINT('Ctrl Pts',(3.90136286599994,5.2,-1.11353966700001));
#349465=CARTESIAN_POINT('Ctrl Pts',(3.90136286599994,2.2,-1.11353966700001));
#349466=CARTESIAN_POINT('Ctrl Pts',(3.90056502099994,12.2,-1.11314980100001));
#349467=CARTESIAN_POINT('Ctrl Pts',(3.90056502099994,5.2,-1.11314980100001));
#349468=CARTESIAN_POINT('Ctrl Pts',(3.90056502099994,2.2,-1.11314980100001));
#349469=CARTESIAN_POINT('Ctrl Pts',(3.89977179699994,12.2,-1.11276341700002));
#349470=CARTESIAN_POINT('Ctrl Pts',(3.89977179699994,5.2,-1.11276341700002));
#349471=CARTESIAN_POINT('Ctrl Pts',(3.89977179699994,2.2,-1.11276341700002));
#349472=CARTESIAN_POINT('Ctrl Pts',(3.89898320899994,12.2,-1.11238050800001));
#349473=CARTESIAN_POINT('Ctrl Pts',(3.89898320899994,5.2,-1.11238050800001));
#349474=CARTESIAN_POINT('Ctrl Pts',(3.89898320899994,2.2,-1.11238050800001));
#349475=CARTESIAN_POINT('Ctrl Pts',(3.89819927199994,12.2,-1.11200106700001));
#349476=CARTESIAN_POINT('Ctrl Pts',(3.89819927199994,5.2,-1.11200106700001));
#349477=CARTESIAN_POINT('Ctrl Pts',(3.89819927199994,2.2,-1.11200106700001));
#349478=CARTESIAN_POINT('Ctrl Pts',(3.89742000499994,12.2,-1.11162508500001));
#349479=CARTESIAN_POINT('Ctrl Pts',(3.89742000499994,5.2,-1.11162508500001));
#349480=CARTESIAN_POINT('Ctrl Pts',(3.89742000499994,2.2,-1.11162508500001));
#349481=CARTESIAN_POINT('Ctrl Pts',(3.89664542199994,12.2,-1.11125255800001));
#349482=CARTESIAN_POINT('Ctrl Pts',(3.89664542199994,5.2,-1.11125255800001));
#349483=CARTESIAN_POINT('Ctrl Pts',(3.89664542199994,2.2,-1.11125255800001));
#349484=CARTESIAN_POINT('Ctrl Pts',(3.89587553999994,12.2,-1.11088347600001));
#349485=CARTESIAN_POINT('Ctrl Pts',(3.89587553999994,5.2,-1.11088347600001));
#349486=CARTESIAN_POINT('Ctrl Pts',(3.89587553999994,2.2,-1.11088347600001));
#349487=CARTESIAN_POINT('Ctrl Pts',(3.89511037599994,12.2,-1.11051783300002));
#349488=CARTESIAN_POINT('Ctrl Pts',(3.89511037599994,5.2,-1.11051783300002));
#349489=CARTESIAN_POINT('Ctrl Pts',(3.89511037599994,2.2,-1.11051783300002));
#349490=CARTESIAN_POINT('Ctrl Pts',(3.89434994499994,12.2,-1.11015562000001));
#349491=CARTESIAN_POINT('Ctrl Pts',(3.89434994499994,5.2,-1.11015562000001));
#349492=CARTESIAN_POINT('Ctrl Pts',(3.89434994499994,2.2,-1.11015562000001));
#349493=CARTESIAN_POINT('Ctrl Pts',(3.89359426299994,12.2,-1.10979683100001));
#349494=CARTESIAN_POINT('Ctrl Pts',(3.89359426299994,5.2,-1.10979683100001));
#349495=CARTESIAN_POINT('Ctrl Pts',(3.89359426299994,2.2,-1.10979683100001));
#349496=CARTESIAN_POINT('Ctrl Pts',(3.89284334799994,12.2,-1.10944145700001));
#349497=CARTESIAN_POINT('Ctrl Pts',(3.89284334799994,5.2,-1.10944145700001));
#349498=CARTESIAN_POINT('Ctrl Pts',(3.89284334799994,2.2,-1.10944145700001));
#349499=CARTESIAN_POINT('Ctrl Pts',(3.89209721499994,12.2,-1.10908949200001));
#349500=CARTESIAN_POINT('Ctrl Pts',(3.89209721499994,5.2,-1.10908949200001));
#349501=CARTESIAN_POINT('Ctrl Pts',(3.89209721499994,2.2,-1.10908949200001));
#349502=CARTESIAN_POINT('Ctrl Pts',(3.89135587999994,12.2,-1.10874092700001));
#349503=CARTESIAN_POINT('Ctrl Pts',(3.89135587999994,5.2,-1.10874092700001));
#349504=CARTESIAN_POINT('Ctrl Pts',(3.89135587999994,2.2,-1.10874092700001));
#349505=CARTESIAN_POINT('Ctrl Pts',(3.89061936199994,12.2,-1.10839575600002));
#349506=CARTESIAN_POINT('Ctrl Pts',(3.89061936199994,5.2,-1.10839575600002));
#349507=CARTESIAN_POINT('Ctrl Pts',(3.89061936199994,2.2,-1.10839575600002));
#349508=CARTESIAN_POINT('Ctrl Pts',(3.88988767399994,12.2,-1.10805397000002));
#349509=CARTESIAN_POINT('Ctrl Pts',(3.88988767399994,5.2,-1.10805397000002));
#349510=CARTESIAN_POINT('Ctrl Pts',(3.88988767399994,2.2,-1.10805397000002));
#349511=CARTESIAN_POINT('Ctrl Pts',(3.88916083499994,12.2,-1.10771556200001));
#349512=CARTESIAN_POINT('Ctrl Pts',(3.88916083499994,5.2,-1.10771556200001));
#349513=CARTESIAN_POINT('Ctrl Pts',(3.88916083499994,2.2,-1.10771556200001));
#349514=CARTESIAN_POINT('Ctrl Pts',(3.88843886099994,12.2,-1.10738052300002));
#349515=CARTESIAN_POINT('Ctrl Pts',(3.88843886099994,5.2,-1.10738052300002));
#349516=CARTESIAN_POINT('Ctrl Pts',(3.88843886099994,2.2,-1.10738052300002));
#349517=CARTESIAN_POINT('Ctrl Pts',(3.88772176899994,12.2,-1.10704884600001));
#349518=CARTESIAN_POINT('Ctrl Pts',(3.88772176899994,5.2,-1.10704884600001));
#349519=CARTESIAN_POINT('Ctrl Pts',(3.88772176899994,2.2,-1.10704884600001));
#349520=CARTESIAN_POINT('Ctrl Pts',(3.88700957299994,12.2,-1.10672052300002));
#349521=CARTESIAN_POINT('Ctrl Pts',(3.88700957299994,5.2,-1.10672052300002));
#349522=CARTESIAN_POINT('Ctrl Pts',(3.88700957299994,2.2,-1.10672052300002));
#349523=CARTESIAN_POINT('Ctrl Pts',(3.88630229399994,12.2,-1.10639554700001));
#349524=CARTESIAN_POINT('Ctrl Pts',(3.88630229399994,5.2,-1.10639554700001));
#349525=CARTESIAN_POINT('Ctrl Pts',(3.88630229399994,2.2,-1.10639554700001));
#349526=CARTESIAN_POINT('Ctrl Pts',(3.88559994499994,12.2,-1.10607390800002));
#349527=CARTESIAN_POINT('Ctrl Pts',(3.88559994499994,5.2,-1.10607390800002));
#349528=CARTESIAN_POINT('Ctrl Pts',(3.88559994499994,2.2,-1.10607390800002));
#349529=CARTESIAN_POINT('Ctrl Pts',(3.88490254399994,12.2,-1.10575560000001));
#349530=CARTESIAN_POINT('Ctrl Pts',(3.88490254399994,5.2,-1.10575560000001));
#349531=CARTESIAN_POINT('Ctrl Pts',(3.88490254399994,2.2,-1.10575560000001));
#349532=CARTESIAN_POINT('Ctrl Pts',(3.88421010699994,12.2,-1.10544061400002));
#349533=CARTESIAN_POINT('Ctrl Pts',(3.88421010699994,5.2,-1.10544061400002));
#349534=CARTESIAN_POINT('Ctrl Pts',(3.88421010699994,2.2,-1.10544061400002));
#349535=CARTESIAN_POINT('Ctrl Pts',(3.88352265299994,12.2,-1.10512894300001));
#349536=CARTESIAN_POINT('Ctrl Pts',(3.88352265299994,5.2,-1.10512894300001));
#349537=CARTESIAN_POINT('Ctrl Pts',(3.88352265299994,2.2,-1.10512894300001));
#349538=CARTESIAN_POINT('Ctrl Pts',(3.88284019699995,12.2,-1.10482057600001));
#349539=CARTESIAN_POINT('Ctrl Pts',(3.88284019699995,5.2,-1.10482057600001));
#349540=CARTESIAN_POINT('Ctrl Pts',(3.88284019699995,2.2,-1.10482057600001));
#349541=CARTESIAN_POINT('Ctrl Pts',(3.88216275599994,12.2,-1.10451550900001));
#349542=CARTESIAN_POINT('Ctrl Pts',(3.88216275599994,5.2,-1.10451550900001));
#349543=CARTESIAN_POINT('Ctrl Pts',(3.88216275599994,2.2,-1.10451550900001));
#349544=CARTESIAN_POINT('Ctrl Pts',(3.88149034799994,12.2,-1.10421373100001));
#349545=CARTESIAN_POINT('Ctrl Pts',(3.88149034799994,5.2,-1.10421373100001));
#349546=CARTESIAN_POINT('Ctrl Pts',(3.88149034799994,2.2,-1.10421373100001));
#349547=CARTESIAN_POINT('Ctrl Pts',(3.88082298799994,12.2,-1.10391523400001));
#349548=CARTESIAN_POINT('Ctrl Pts',(3.88082298799994,5.2,-1.10391523400001));
#349549=CARTESIAN_POINT('Ctrl Pts',(3.88082298799994,2.2,-1.10391523400001));
#349550=CARTESIAN_POINT('Ctrl Pts',(3.88016069499994,12.2,-1.10362001000002));
#349551=CARTESIAN_POINT('Ctrl Pts',(3.88016069499994,5.2,-1.10362001000002));
#349552=CARTESIAN_POINT('Ctrl Pts',(3.88016069499994,2.2,-1.10362001000002));
#349553=CARTESIAN_POINT('Ctrl Pts',(3.87950348599994,12.2,-1.10332805000001));
#349554=CARTESIAN_POINT('Ctrl Pts',(3.87950348599994,5.2,-1.10332805000001));
#349555=CARTESIAN_POINT('Ctrl Pts',(3.87950348599994,2.2,-1.10332805000001));
#349556=CARTESIAN_POINT('Ctrl Pts',(3.87885137499994,12.2,-1.10303934700001));
#349557=CARTESIAN_POINT('Ctrl Pts',(3.87885137499994,5.2,-1.10303934700001));
#349558=CARTESIAN_POINT('Ctrl Pts',(3.87885137499994,2.2,-1.10303934700001));
#349559=CARTESIAN_POINT('Ctrl Pts',(3.87820438299994,12.2,-1.10275389300002));
#349560=CARTESIAN_POINT('Ctrl Pts',(3.87820438299994,5.2,-1.10275389300002));
#349561=CARTESIAN_POINT('Ctrl Pts',(3.87820438299994,2.2,-1.10275389300002));
#349562=CARTESIAN_POINT('Ctrl Pts',(3.87756252599994,12.2,-1.10247167700001));
#349563=CARTESIAN_POINT('Ctrl Pts',(3.87756252599994,5.2,-1.10247167700001));
#349564=CARTESIAN_POINT('Ctrl Pts',(3.87756252599994,2.2,-1.10247167700001));
#349565=CARTESIAN_POINT('Ctrl Pts',(3.87692581899994,12.2,-1.10219269300002));
#349566=CARTESIAN_POINT('Ctrl Pts',(3.87692581899994,5.2,-1.10219269300002));
#349567=CARTESIAN_POINT('Ctrl Pts',(3.87692581899994,2.2,-1.10219269300002));
#349568=CARTESIAN_POINT('Ctrl Pts',(3.87629428199994,12.2,-1.10191693100001));
#349569=CARTESIAN_POINT('Ctrl Pts',(3.87629428199994,5.2,-1.10191693100001));
#349570=CARTESIAN_POINT('Ctrl Pts',(3.87629428199994,2.2,-1.10191693100001));
#349571=CARTESIAN_POINT('Ctrl Pts',(3.87566793099994,12.2,-1.10164438200002));
#349572=CARTESIAN_POINT('Ctrl Pts',(3.87566793099994,5.2,-1.10164438200002));
#349573=CARTESIAN_POINT('Ctrl Pts',(3.87566793099994,2.2,-1.10164438200002));
#349574=CARTESIAN_POINT('Ctrl Pts',(3.87504678299994,12.2,-1.10137503800001));
#349575=CARTESIAN_POINT('Ctrl Pts',(3.87504678299994,5.2,-1.10137503800001));
#349576=CARTESIAN_POINT('Ctrl Pts',(3.87504678299994,2.2,-1.10137503800001));
#349577=CARTESIAN_POINT('Ctrl Pts',(3.87443085699994,12.2,-1.10110889100001));
#349578=CARTESIAN_POINT('Ctrl Pts',(3.87443085699994,5.2,-1.10110889100001));
#349579=CARTESIAN_POINT('Ctrl Pts',(3.87443085699994,2.2,-1.10110889100001));
#349580=CARTESIAN_POINT('Ctrl Pts',(3.87382016699994,12.2,-1.10084593200002));
#349581=CARTESIAN_POINT('Ctrl Pts',(3.87382016699994,5.2,-1.10084593200002));
#349582=CARTESIAN_POINT('Ctrl Pts',(3.87382016699994,2.2,-1.10084593200002));
#349583=CARTESIAN_POINT('Ctrl Pts',(3.87321473399994,12.2,-1.10058615200002));
#349584=CARTESIAN_POINT('Ctrl Pts',(3.87321473399994,5.2,-1.10058615200002));
#349585=CARTESIAN_POINT('Ctrl Pts',(3.87321473399994,2.2,-1.10058615200002));
#349586=CARTESIAN_POINT('Ctrl Pts',(3.87261457399994,12.2,-1.10032954000001));
#349587=CARTESIAN_POINT('Ctrl Pts',(3.87261457399994,5.2,-1.10032954000001));
#349588=CARTESIAN_POINT('Ctrl Pts',(3.87261457399994,2.2,-1.10032954000001));
#349589=CARTESIAN_POINT('Ctrl Pts',(3.87201970499994,12.2,-1.10007609000002));
#349590=CARTESIAN_POINT('Ctrl Pts',(3.87201970499994,5.2,-1.10007609000002));
#349591=CARTESIAN_POINT('Ctrl Pts',(3.87201970499994,2.2,-1.10007609000002));
#349592=CARTESIAN_POINT('Ctrl Pts',(3.87143014299994,12.2,-1.09982579300001));
#349593=CARTESIAN_POINT('Ctrl Pts',(3.87143014299994,5.2,-1.09982579300001));
#349594=CARTESIAN_POINT('Ctrl Pts',(3.87143014299994,2.2,-1.09982579300001));
#349595=CARTESIAN_POINT('Ctrl Pts',(3.87084590699994,12.2,-1.09957863800001));
#349596=CARTESIAN_POINT('Ctrl Pts',(3.87084590699994,5.2,-1.09957863800001));
#349597=CARTESIAN_POINT('Ctrl Pts',(3.87084590699994,2.2,-1.09957863800001));
#349598=CARTESIAN_POINT('Ctrl Pts',(3.87026701399994,12.2,-1.09933461800001));
#349599=CARTESIAN_POINT('Ctrl Pts',(3.87026701399994,5.2,-1.09933461800001));
#349600=CARTESIAN_POINT('Ctrl Pts',(3.87026701399994,2.2,-1.09933461800001));
#349601=CARTESIAN_POINT('Ctrl Pts',(3.86969348299994,12.2,-1.09909372300002));
#349602=CARTESIAN_POINT('Ctrl Pts',(3.86969348299994,5.2,-1.09909372300002));
#349603=CARTESIAN_POINT('Ctrl Pts',(3.86969348299994,2.2,-1.09909372300002));
#349604=CARTESIAN_POINT('Ctrl Pts',(3.86912532999994,12.2,-1.09885594400001));
#349605=CARTESIAN_POINT('Ctrl Pts',(3.86912532999994,5.2,-1.09885594400001));
#349606=CARTESIAN_POINT('Ctrl Pts',(3.86912532999994,2.2,-1.09885594400001));
#349607=CARTESIAN_POINT('Ctrl Pts',(3.86856257199994,12.2,-1.09862127100001));
#349608=CARTESIAN_POINT('Ctrl Pts',(3.86856257199994,5.2,-1.09862127100001));
#349609=CARTESIAN_POINT('Ctrl Pts',(3.86856257199994,2.2,-1.09862127100001));
#349610=CARTESIAN_POINT('Ctrl Pts',(3.86800522999994,12.2,-1.09838969500001));
#349611=CARTESIAN_POINT('Ctrl Pts',(3.86800522999994,5.2,-1.09838969500001));
#349612=CARTESIAN_POINT('Ctrl Pts',(3.86800522999994,2.2,-1.09838969500001));
#349613=CARTESIAN_POINT('Ctrl Pts',(3.86745331999994,12.2,-1.09816120800001));
#349614=CARTESIAN_POINT('Ctrl Pts',(3.86745331999994,5.2,-1.09816120800001));
#349615=CARTESIAN_POINT('Ctrl Pts',(3.86745331999994,2.2,-1.09816120800001));
#349616=CARTESIAN_POINT('Ctrl Pts',(3.86690685899994,12.2,-1.09793580000002));
#349617=CARTESIAN_POINT('Ctrl Pts',(3.86690685899994,5.2,-1.09793580000002));
#349618=CARTESIAN_POINT('Ctrl Pts',(3.86690685899994,2.2,-1.09793580000002));
#349619=CARTESIAN_POINT('Ctrl Pts',(3.86636586599994,12.2,-1.09771346200001));
#349620=CARTESIAN_POINT('Ctrl Pts',(3.86636586599994,5.2,-1.09771346200001));
#349621=CARTESIAN_POINT('Ctrl Pts',(3.86636586599994,2.2,-1.09771346200001));
#349622=CARTESIAN_POINT('Ctrl Pts',(3.86583035899994,12.2,-1.09749418300002));
#349623=CARTESIAN_POINT('Ctrl Pts',(3.86583035899994,5.2,-1.09749418300002));
#349624=CARTESIAN_POINT('Ctrl Pts',(3.86583035899994,2.2,-1.09749418300002));
#349625=CARTESIAN_POINT('Ctrl Pts',(3.86530035599994,12.2,-1.09727795600001));
#349626=CARTESIAN_POINT('Ctrl Pts',(3.86530035599994,5.2,-1.09727795600001));
#349627=CARTESIAN_POINT('Ctrl Pts',(3.86530035599994,2.2,-1.09727795600001));
#349628=CARTESIAN_POINT('Ctrl Pts',(3.86477587299995,12.2,-1.09706476800001));
#349629=CARTESIAN_POINT('Ctrl Pts',(3.86477587299995,5.2,-1.09706476800001));
#349630=CARTESIAN_POINT('Ctrl Pts',(3.86477587299995,2.2,-1.09706476800001));
#349631=CARTESIAN_POINT('Ctrl Pts',(3.86425693199994,12.2,-1.09685461300002));
#349632=CARTESIAN_POINT('Ctrl Pts',(3.86425693199994,5.2,-1.09685461300002));
#349633=CARTESIAN_POINT('Ctrl Pts',(3.86425693199994,2.2,-1.09685461300002));
#349634=CARTESIAN_POINT('Ctrl Pts',(3.86374354899994,12.2,-1.09664748000001));
#349635=CARTESIAN_POINT('Ctrl Pts',(3.86374354899994,5.2,-1.09664748000001));
#349636=CARTESIAN_POINT('Ctrl Pts',(3.86374354899994,2.2,-1.09664748000001));
#349637=CARTESIAN_POINT('Ctrl Pts',(3.86323573999994,12.2,-1.09644335800001));
#349638=CARTESIAN_POINT('Ctrl Pts',(3.86323573999994,5.2,-1.09644335800001));
#349639=CARTESIAN_POINT('Ctrl Pts',(3.86323573999994,2.2,-1.09644335800001));
#349640=CARTESIAN_POINT('Ctrl Pts',(3.86273352699994,12.2,-1.09624223900001));
#349641=CARTESIAN_POINT('Ctrl Pts',(3.86273352699994,5.2,-1.09624223900001));
#349642=CARTESIAN_POINT('Ctrl Pts',(3.86273352699994,2.2,-1.09624223900001));
#349643=CARTESIAN_POINT('Ctrl Pts',(3.86223692699994,12.2,-1.09604411300001));
#349644=CARTESIAN_POINT('Ctrl Pts',(3.86223692699994,5.2,-1.09604411300001));
#349645=CARTESIAN_POINT('Ctrl Pts',(3.86223692699994,2.2,-1.09604411300001));
#349646=CARTESIAN_POINT('Ctrl Pts',(3.86174595699994,12.2,-1.09584897000001));
#349647=CARTESIAN_POINT('Ctrl Pts',(3.86174595699994,5.2,-1.09584897000001));
#349648=CARTESIAN_POINT('Ctrl Pts',(3.86174595699994,2.2,-1.09584897000001));
#349649=CARTESIAN_POINT('Ctrl Pts',(3.86126063599994,12.2,-1.09565680000001));
#349650=CARTESIAN_POINT('Ctrl Pts',(3.86126063599994,5.2,-1.09565680000001));
#349651=CARTESIAN_POINT('Ctrl Pts',(3.86126063599994,2.2,-1.09565680000001));
#349652=CARTESIAN_POINT('Ctrl Pts',(3.86078098399994,12.2,-1.09546759400001));
#349653=CARTESIAN_POINT('Ctrl Pts',(3.86078098399994,5.2,-1.09546759400001));
#349654=CARTESIAN_POINT('Ctrl Pts',(3.86078098399994,2.2,-1.09546759400001));
#349655=CARTESIAN_POINT('Ctrl Pts',(3.86030701699994,12.2,-1.09528133900001));
#349656=CARTESIAN_POINT('Ctrl Pts',(3.86030701699994,5.2,-1.09528133900001));
#349657=CARTESIAN_POINT('Ctrl Pts',(3.86030701699994,2.2,-1.09528133900001));
#349658=CARTESIAN_POINT('Ctrl Pts',(3.85983875499994,12.2,-1.09509802800002));
#349659=CARTESIAN_POINT('Ctrl Pts',(3.85983875499994,5.2,-1.09509802800002));
#349660=CARTESIAN_POINT('Ctrl Pts',(3.85983875499994,2.2,-1.09509802800002));
#349661=CARTESIAN_POINT('Ctrl Pts',(3.85937621599994,12.2,-1.09491765000001));
#349662=CARTESIAN_POINT('Ctrl Pts',(3.85937621599994,5.2,-1.09491765000001));
#349663=CARTESIAN_POINT('Ctrl Pts',(3.85937621599994,2.2,-1.09491765000001));
#349664=CARTESIAN_POINT('Ctrl Pts',(3.85891941899994,12.2,-1.09474019500002));
#349665=CARTESIAN_POINT('Ctrl Pts',(3.85891941899994,5.2,-1.09474019500002));
#349666=CARTESIAN_POINT('Ctrl Pts',(3.85891941899994,2.2,-1.09474019500002));
#349667=CARTESIAN_POINT('Ctrl Pts',(3.85846838299994,12.2,-1.09456565200002));
#349668=CARTESIAN_POINT('Ctrl Pts',(3.85846838299994,5.2,-1.09456565200002));
#349669=CARTESIAN_POINT('Ctrl Pts',(3.85846838299994,2.2,-1.09456565200002));
#349670=CARTESIAN_POINT('Ctrl Pts',(3.85802312499994,12.2,-1.09439401100001));
#349671=CARTESIAN_POINT('Ctrl Pts',(3.85802312499994,5.2,-1.09439401100001));
#349672=CARTESIAN_POINT('Ctrl Pts',(3.85802312499994,2.2,-1.09439401100001));
#349673=CARTESIAN_POINT('Ctrl Pts',(3.85758366499994,12.2,-1.09422526300001));
#349674=CARTESIAN_POINT('Ctrl Pts',(3.85758366499994,5.2,-1.09422526300001));
#349675=CARTESIAN_POINT('Ctrl Pts',(3.85758366499994,2.2,-1.09422526300001));
#349676=CARTESIAN_POINT('Ctrl Pts',(3.85715002099994,12.2,-1.09405939600002));
#349677=CARTESIAN_POINT('Ctrl Pts',(3.85715002099994,5.2,-1.09405939600002));
#349678=CARTESIAN_POINT('Ctrl Pts',(3.85715002099994,2.2,-1.09405939600002));
#349679=CARTESIAN_POINT('Ctrl Pts',(3.85672221399994,12.2,-1.09389640100002));
#349680=CARTESIAN_POINT('Ctrl Pts',(3.85672221399994,5.2,-1.09389640100002));
#349681=CARTESIAN_POINT('Ctrl Pts',(3.85672221399994,2.2,-1.09389640100002));
#349682=CARTESIAN_POINT('Ctrl Pts',(3.85630025899994,12.2,-1.09373626600001));
#349683=CARTESIAN_POINT('Ctrl Pts',(3.85630025899994,5.2,-1.09373626600001));
#349684=CARTESIAN_POINT('Ctrl Pts',(3.85630025899994,2.2,-1.09373626600001));
#349685=CARTESIAN_POINT('Ctrl Pts',(3.85588417899994,12.2,-1.09357898100002));
#349686=CARTESIAN_POINT('Ctrl Pts',(3.85588417899994,5.2,-1.09357898100002));
#349687=CARTESIAN_POINT('Ctrl Pts',(3.85588417899994,2.2,-1.09357898100002));
#349688=CARTESIAN_POINT('Ctrl Pts',(3.85547399099994,12.2,-1.09342453700001));
#349689=CARTESIAN_POINT('Ctrl Pts',(3.85547399099994,5.2,-1.09342453700001));
#349690=CARTESIAN_POINT('Ctrl Pts',(3.85547399099994,2.2,-1.09342453700001));
#349691=CARTESIAN_POINT('Ctrl Pts',(3.85506971299994,12.2,-1.09327292100001));
#349692=CARTESIAN_POINT('Ctrl Pts',(3.85506971299994,5.2,-1.09327292100001));
#349693=CARTESIAN_POINT('Ctrl Pts',(3.85506971299994,2.2,-1.09327292100001));
#349694=CARTESIAN_POINT('Ctrl Pts',(3.85467136599994,12.2,-1.09312412300001));
#349695=CARTESIAN_POINT('Ctrl Pts',(3.85467136599994,5.2,-1.09312412300001));
#349696=CARTESIAN_POINT('Ctrl Pts',(3.85467136599994,2.2,-1.09312412300001));
#349697=CARTESIAN_POINT('Ctrl Pts',(3.85427896699994,12.2,-1.09297813400001));
#349698=CARTESIAN_POINT('Ctrl Pts',(3.85427896699994,5.2,-1.09297813400001));
#349699=CARTESIAN_POINT('Ctrl Pts',(3.85427896699994,2.2,-1.09297813400001));
#349700=CARTESIAN_POINT('Ctrl Pts',(3.85389253799994,12.2,-1.09283494100001));
#349701=CARTESIAN_POINT('Ctrl Pts',(3.85389253799994,5.2,-1.09283494100001));
#349702=CARTESIAN_POINT('Ctrl Pts',(3.85389253799994,2.2,-1.09283494100001));
#349703=CARTESIAN_POINT('Ctrl Pts',(3.85351209599994,12.2,-1.09269453300001));
#349704=CARTESIAN_POINT('Ctrl Pts',(3.85351209599994,5.2,-1.09269453300001));
#349705=CARTESIAN_POINT('Ctrl Pts',(3.85351209599994,2.2,-1.09269453300001));
#349706=CARTESIAN_POINT('Ctrl Pts',(3.85313766099994,12.2,-1.09255690100001));
#349707=CARTESIAN_POINT('Ctrl Pts',(3.85313766099994,5.2,-1.09255690100001));
#349708=CARTESIAN_POINT('Ctrl Pts',(3.85313766099994,2.2,-1.09255690100001));
#349709=CARTESIAN_POINT('Ctrl Pts',(3.85276925099994,12.2,-1.09242203300001));
#349710=CARTESIAN_POINT('Ctrl Pts',(3.85276925099994,5.2,-1.09242203300001));
#349711=CARTESIAN_POINT('Ctrl Pts',(3.85276925099994,2.2,-1.09242203300001));
#349712=CARTESIAN_POINT('Ctrl Pts',(3.85240688799994,12.2,-1.09228991700002));
#349713=CARTESIAN_POINT('Ctrl Pts',(3.85240688799994,5.2,-1.09228991700002));
#349714=CARTESIAN_POINT('Ctrl Pts',(3.85240688799994,2.2,-1.09228991700002));
#349715=CARTESIAN_POINT('Ctrl Pts',(3.85205058899994,12.2,-1.09216054400001));
#349716=CARTESIAN_POINT('Ctrl Pts',(3.85205058899994,5.2,-1.09216054400001));
#349717=CARTESIAN_POINT('Ctrl Pts',(3.85205058899994,2.2,-1.09216054400001));
#349718=CARTESIAN_POINT('Ctrl Pts',(3.85170037499994,12.2,-1.09203390100001));
#349719=CARTESIAN_POINT('Ctrl Pts',(3.85170037499994,5.2,-1.09203390100001));
#349720=CARTESIAN_POINT('Ctrl Pts',(3.85170037499994,2.2,-1.09203390100001));
#349721=CARTESIAN_POINT('Ctrl Pts',(3.85135626499994,12.2,-1.09190997700002));
#349722=CARTESIAN_POINT('Ctrl Pts',(3.85135626499994,5.2,-1.09190997700002));
#349723=CARTESIAN_POINT('Ctrl Pts',(3.85135626499994,2.2,-1.09190997700002));
#349724=CARTESIAN_POINT('Ctrl Pts',(3.85101827699994,12.2,-1.09178876200001));
#349725=CARTESIAN_POINT('Ctrl Pts',(3.85101827699994,5.2,-1.09178876200001));
#349726=CARTESIAN_POINT('Ctrl Pts',(3.85101827699994,2.2,-1.09178876200001));
#349727=CARTESIAN_POINT('Ctrl Pts',(3.85068643399994,12.2,-1.09167024400001));
#349728=CARTESIAN_POINT('Ctrl Pts',(3.85068643399994,5.2,-1.09167024400001));
#349729=CARTESIAN_POINT('Ctrl Pts',(3.85068643399994,2.2,-1.09167024400001));
#349730=CARTESIAN_POINT('Ctrl Pts',(3.85036075299994,12.2,-1.09155441100001));
#349731=CARTESIAN_POINT('Ctrl Pts',(3.85036075299994,5.2,-1.09155441100001));
#349732=CARTESIAN_POINT('Ctrl Pts',(3.85036075299994,2.2,-1.09155441100001));
#349733=CARTESIAN_POINT('Ctrl Pts',(3.85004125399994,12.2,-1.09144125200002));
#349734=CARTESIAN_POINT('Ctrl Pts',(3.85004125399994,5.2,-1.09144125200002));
#349735=CARTESIAN_POINT('Ctrl Pts',(3.85004125399994,2.2,-1.09144125200002));
#349736=CARTESIAN_POINT('Ctrl Pts',(3.84972795699994,12.2,-1.09133075600001));
#349737=CARTESIAN_POINT('Ctrl Pts',(3.84972795699994,5.2,-1.09133075600001));
#349738=CARTESIAN_POINT('Ctrl Pts',(3.84972795699994,2.2,-1.09133075600001));
#349739=CARTESIAN_POINT('Ctrl Pts',(3.84942088299994,12.2,-1.09122291000002));
#349740=CARTESIAN_POINT('Ctrl Pts',(3.84942088299994,5.2,-1.09122291000002));
#349741=CARTESIAN_POINT('Ctrl Pts',(3.84942088299994,2.2,-1.09122291000002));
#349742=CARTESIAN_POINT('Ctrl Pts',(3.84912005099994,12.2,-1.09111770400002));
#349743=CARTESIAN_POINT('Ctrl Pts',(3.84912005099994,5.2,-1.09111770400002));
#349744=CARTESIAN_POINT('Ctrl Pts',(3.84912005099994,2.2,-1.09111770400002));
#349745=CARTESIAN_POINT('Ctrl Pts',(3.84882547999994,12.2,-1.09101512600001));
#349746=CARTESIAN_POINT('Ctrl Pts',(3.84882547999994,5.2,-1.09101512600001));
#349747=CARTESIAN_POINT('Ctrl Pts',(3.84882547999994,2.2,-1.09101512600001));
#349748=CARTESIAN_POINT('Ctrl Pts',(3.84853719099994,12.2,-1.09091516300001));
#349749=CARTESIAN_POINT('Ctrl Pts',(3.84853719099994,5.2,-1.09091516300001));
#349750=CARTESIAN_POINT('Ctrl Pts',(3.84853719099994,2.2,-1.09091516300001));
#349751=CARTESIAN_POINT('Ctrl Pts',(3.84825520499994,12.2,-1.09081780400002));
#349752=CARTESIAN_POINT('Ctrl Pts',(3.84825520499994,5.2,-1.09081780400002));
#349753=CARTESIAN_POINT('Ctrl Pts',(3.84825520499994,2.2,-1.09081780400002));
#349754=CARTESIAN_POINT('Ctrl Pts',(3.84797953999994,12.2,-1.09072303800001));
#349755=CARTESIAN_POINT('Ctrl Pts',(3.84797953999994,5.2,-1.09072303800001));
#349756=CARTESIAN_POINT('Ctrl Pts',(3.84797953999994,2.2,-1.09072303800001));
#349757=CARTESIAN_POINT('Ctrl Pts',(3.84771021599994,12.2,-1.09063085100002));
#349758=CARTESIAN_POINT('Ctrl Pts',(3.84771021599994,5.2,-1.09063085100002));
#349759=CARTESIAN_POINT('Ctrl Pts',(3.84771021599994,2.2,-1.09063085100002));
#349760=CARTESIAN_POINT('Ctrl Pts',(3.84744725699994,12.2,-1.09054123300002));
#349761=CARTESIAN_POINT('Ctrl Pts',(3.84744725699994,5.2,-1.09054123300002));
#349762=CARTESIAN_POINT('Ctrl Pts',(3.84744725699994,2.2,-1.09054123300002));
#349763=CARTESIAN_POINT('Ctrl Pts',(3.84719067799994,12.2,-1.09045417100001));
#349764=CARTESIAN_POINT('Ctrl Pts',(3.84719067799994,5.2,-1.09045417100001));
#349765=CARTESIAN_POINT('Ctrl Pts',(3.84719067799994,2.2,-1.09045417100001));
#349766=CARTESIAN_POINT('Ctrl Pts',(3.84694050299994,12.2,-1.09036965200001));
#349767=CARTESIAN_POINT('Ctrl Pts',(3.84694050299994,5.2,-1.09036965200001));
#349768=CARTESIAN_POINT('Ctrl Pts',(3.84694050299994,2.2,-1.09036965200001));
#349769=CARTESIAN_POINT('Ctrl Pts',(3.84669675099994,12.2,-1.09028766600002));
#349770=CARTESIAN_POINT('Ctrl Pts',(3.84669675099994,5.2,-1.09028766600002));
#349771=CARTESIAN_POINT('Ctrl Pts',(3.84669675099994,2.2,-1.09028766600002));
#349772=CARTESIAN_POINT('Ctrl Pts',(3.84645944399994,12.2,-1.09020819900001));
#349773=CARTESIAN_POINT('Ctrl Pts',(3.84645944399994,5.2,-1.09020819900001));
#349774=CARTESIAN_POINT('Ctrl Pts',(3.84645944399994,2.2,-1.09020819900001));
#349775=CARTESIAN_POINT('Ctrl Pts',(3.84622859999994,12.2,-1.09013123800001));
#349776=CARTESIAN_POINT('Ctrl Pts',(3.84622859999994,5.2,-1.09013123800001));
#349777=CARTESIAN_POINT('Ctrl Pts',(3.84622859999994,2.2,-1.09013123800001));
#349778=CARTESIAN_POINT('Ctrl Pts',(3.84600424099994,12.2,-1.09005677300001));
#349779=CARTESIAN_POINT('Ctrl Pts',(3.84600424099994,5.2,-1.09005677300001));
#349780=CARTESIAN_POINT('Ctrl Pts',(3.84600424099994,2.2,-1.09005677300001));
#349781=CARTESIAN_POINT('Ctrl Pts',(3.84578638699994,12.2,-1.08998479000002));
#349782=CARTESIAN_POINT('Ctrl Pts',(3.84578638699994,5.2,-1.08998479000002));
#349783=CARTESIAN_POINT('Ctrl Pts',(3.84578638699994,2.2,-1.08998479000002));
#349784=CARTESIAN_POINT('Ctrl Pts',(3.84557505899994,12.2,-1.08991527600002));
#349785=CARTESIAN_POINT('Ctrl Pts',(3.84557505899994,5.2,-1.08991527600002));
#349786=CARTESIAN_POINT('Ctrl Pts',(3.84557505899994,2.2,-1.08991527600002));
#349787=CARTESIAN_POINT('Ctrl Pts',(3.84537027799994,12.2,-1.08984822000001));
#349788=CARTESIAN_POINT('Ctrl Pts',(3.84537027799994,5.2,-1.08984822000001));
#349789=CARTESIAN_POINT('Ctrl Pts',(3.84537027799994,2.2,-1.08984822000001));
#349790=CARTESIAN_POINT('Ctrl Pts',(3.84517206499994,12.2,-1.08978360800001));
#349791=CARTESIAN_POINT('Ctrl Pts',(3.84517206499994,5.2,-1.08978360800001));
#349792=CARTESIAN_POINT('Ctrl Pts',(3.84517206499994,2.2,-1.08978360800001));
#349793=CARTESIAN_POINT('Ctrl Pts',(3.84498043899994,12.2,-1.08972142800001));
#349794=CARTESIAN_POINT('Ctrl Pts',(3.84498043899994,5.2,-1.08972142800001));
#349795=CARTESIAN_POINT('Ctrl Pts',(3.84498043899994,2.2,-1.08972142800001));
#349796=CARTESIAN_POINT('Ctrl Pts',(3.84479542399994,12.2,-1.08966166700001));
#349797=CARTESIAN_POINT('Ctrl Pts',(3.84479542399994,5.2,-1.08966166700001));
#349798=CARTESIAN_POINT('Ctrl Pts',(3.84479542399994,2.2,-1.08966166700001));
#349799=CARTESIAN_POINT('Ctrl Pts',(3.84461703899994,12.2,-1.08960431100002));
#349800=CARTESIAN_POINT('Ctrl Pts',(3.84461703899994,5.2,-1.08960431100002));
#349801=CARTESIAN_POINT('Ctrl Pts',(3.84461703899994,2.2,-1.08960431100002));
#349802=CARTESIAN_POINT('Ctrl Pts',(3.84444530599994,12.2,-1.08954934800002));
#349803=CARTESIAN_POINT('Ctrl Pts',(3.84444530599994,5.2,-1.08954934800002));
#349804=CARTESIAN_POINT('Ctrl Pts',(3.84444530599994,2.2,-1.08954934800002));
#349805=CARTESIAN_POINT('Ctrl Pts',(3.84428024399994,12.2,-1.08949676500002));
#349806=CARTESIAN_POINT('Ctrl Pts',(3.84428024399994,5.2,-1.08949676500002));
#349807=CARTESIAN_POINT('Ctrl Pts',(3.84428024399994,2.2,-1.08949676500002));
#349808=CARTESIAN_POINT('Ctrl Pts',(3.84412187499994,12.2,-1.08944655000002));
#349809=CARTESIAN_POINT('Ctrl Pts',(3.84412187499994,5.2,-1.08944655000002));
#349810=CARTESIAN_POINT('Ctrl Pts',(3.84412187499994,2.2,-1.08944655000002));
#349811=CARTESIAN_POINT('Ctrl Pts',(3.84397021999995,12.2,-1.08939869000002));
#349812=CARTESIAN_POINT('Ctrl Pts',(3.84397021999995,5.2,-1.08939869000002));
#349813=CARTESIAN_POINT('Ctrl Pts',(3.84397021999995,2.2,-1.08939869000002));
#349814=CARTESIAN_POINT('Ctrl Pts',(3.84382529999994,12.2,-1.08935317000002));
#349815=CARTESIAN_POINT('Ctrl Pts',(3.84382529999994,5.2,-1.08935317000002));
#349816=CARTESIAN_POINT('Ctrl Pts',(3.84382529999994,2.2,-1.08935317000002));
#349817=CARTESIAN_POINT('Ctrl Pts',(3.84368713799994,12.2,-1.08930997700002));
#349818=CARTESIAN_POINT('Ctrl Pts',(3.84368713799994,5.2,-1.08930997700002));
#349819=CARTESIAN_POINT('Ctrl Pts',(3.84368713799994,2.2,-1.08930997700002));
#349820=CARTESIAN_POINT('Ctrl Pts',(3.84355575699994,12.2,-1.08926909700001));
#349821=CARTESIAN_POINT('Ctrl Pts',(3.84355575699994,5.2,-1.08926909700001));
#349822=CARTESIAN_POINT('Ctrl Pts',(3.84355575699994,2.2,-1.08926909700001));
#349823=CARTESIAN_POINT('Ctrl Pts',(3.84343117799994,12.2,-1.08923051600001));
#349824=CARTESIAN_POINT('Ctrl Pts',(3.84343117799994,5.2,-1.08923051600001));
#349825=CARTESIAN_POINT('Ctrl Pts',(3.84343117799994,2.2,-1.08923051600001));
#349826=CARTESIAN_POINT('Ctrl Pts',(3.84331342199994,12.2,-1.08919422100001));
#349827=CARTESIAN_POINT('Ctrl Pts',(3.84331342199994,5.2,-1.08919422100001));
#349828=CARTESIAN_POINT('Ctrl Pts',(3.84331342199994,2.2,-1.08919422100001));
#349829=CARTESIAN_POINT('Ctrl Pts',(3.84320250899994,12.2,-1.08916020000001));
#349830=CARTESIAN_POINT('Ctrl Pts',(3.84320250899994,5.2,-1.08916020000001));
#349831=CARTESIAN_POINT('Ctrl Pts',(3.84320250899994,2.2,-1.08916020000001));
#349832=CARTESIAN_POINT('Ctrl Pts',(3.84309845699994,12.2,-1.08912844000002));
#349833=CARTESIAN_POINT('Ctrl Pts',(3.84309845699994,5.2,-1.08912844000002));
#349834=CARTESIAN_POINT('Ctrl Pts',(3.84309845699994,2.2,-1.08912844000002));
#349835=CARTESIAN_POINT('Ctrl Pts',(3.84300128699994,12.2,-1.08909893100002));
#349836=CARTESIAN_POINT('Ctrl Pts',(3.84300128699994,5.2,-1.08909893100002));
#349837=CARTESIAN_POINT('Ctrl Pts',(3.84300128699994,2.2,-1.08909893100002));
#349838=CARTESIAN_POINT('Ctrl Pts',(3.84291102199994,12.2,-1.08907165500002));
#349839=CARTESIAN_POINT('Ctrl Pts',(3.84291102199994,5.2,-1.08907165500002));
#349840=CARTESIAN_POINT('Ctrl Pts',(3.84291102199994,2.2,-1.08907165500002));
#349841=CARTESIAN_POINT('Ctrl Pts',(3.84282768499994,12.2,-1.08904659800002));
#349842=CARTESIAN_POINT('Ctrl Pts',(3.84282768499994,5.2,-1.08904659800002));
#349843=CARTESIAN_POINT('Ctrl Pts',(3.84282768499994,2.2,-1.08904659800002));
#349844=CARTESIAN_POINT('Ctrl Pts',(3.84275130599994,12.2,-1.08902374300001));
#349845=CARTESIAN_POINT('Ctrl Pts',(3.84275130599994,5.2,-1.08902374300001));
#349846=CARTESIAN_POINT('Ctrl Pts',(3.84275130599994,2.2,-1.08902374300001));
#349847=CARTESIAN_POINT('Ctrl Pts',(3.84268191099994,12.2,-1.08900307200001));
#349848=CARTESIAN_POINT('Ctrl Pts',(3.84268191099994,5.2,-1.08900307200001));
#349849=CARTESIAN_POINT('Ctrl Pts',(3.84268191099994,2.2,-1.08900307200001));
#349850=CARTESIAN_POINT('Ctrl Pts',(3.84261952399994,12.2,-1.08898456900001));
#349851=CARTESIAN_POINT('Ctrl Pts',(3.84261952399994,5.2,-1.08898456900001));
#349852=CARTESIAN_POINT('Ctrl Pts',(3.84261952399994,2.2,-1.08898456900001));
#349853=CARTESIAN_POINT('Ctrl Pts',(3.84256416399994,12.2,-1.08896822300002));
#349854=CARTESIAN_POINT('Ctrl Pts',(3.84256416399994,5.2,-1.08896822300002));
#349855=CARTESIAN_POINT('Ctrl Pts',(3.84256416399994,2.2,-1.08896822300002));
#349856=CARTESIAN_POINT('Ctrl Pts',(3.84251066686886,12.2,-1.0889525084115));
#349857=CARTESIAN_POINT('Ctrl Pts',(3.84251066686886,5.2,-1.0889525084115));
#349858=CARTESIAN_POINT('Ctrl Pts',(3.84251066686886,2.2,-1.0889525084115));
#349859=CARTESIAN_POINT('Ctrl Pts',(3.84247407877687,12.2,-1.08894183751314));
#349860=CARTESIAN_POINT('Ctrl Pts',(3.84247407877687,5.2,-1.08894183751314));
#349861=CARTESIAN_POINT('Ctrl Pts',(3.84247407877687,2.2,-1.08894183751314));
#349862=CARTESIAN_POINT('Ctrl Pts',(3.84244995866238,12.2,-1.08893486249907));
#349863=CARTESIAN_POINT('Ctrl Pts',(3.84244995866238,5.2,-1.08893486249907));
#349864=CARTESIAN_POINT('Ctrl Pts',(3.84244995866238,2.2,-1.08893486249907));
#349865=CARTESIAN_POINT('Ctrl Pts',(3.84243492681053,12.2,-1.0889305491042));
#349866=CARTESIAN_POINT('Ctrl Pts',(3.84243492681053,5.2,-1.0889305491042));
#349867=CARTESIAN_POINT('Ctrl Pts',(3.84243492681053,2.2,-1.0889305491042));
#349868=CARTESIAN_POINT('Ctrl Pts',(3.84242564299994,12.2,-1.08892788300002));
#349869=CARTESIAN_POINT('Ctrl Pts',(3.84242564299994,5.2,-1.08892788300002));
#349870=CARTESIAN_POINT('Ctrl Pts',(3.84242564299994,2.2,-1.08892788300002));
#349871=CARTESIAN_POINT('',(4.46529931499995,12.2,-1.61975369200002));
#349872=CARTESIAN_POINT('Origin',(-5.66300478732629E-14,15.2,-1.77635683940025E-14));
#349873=CARTESIAN_POINT('',(4.33922903699994,12.2,-1.93225033600001));
#349874=CARTESIAN_POINT('Ctrl Pts',(3.52236173899994,12.2,-1.88224066100001));
#349875=CARTESIAN_POINT('Ctrl Pts',(3.52236173899994,5.2,-1.88224066100001));
#349876=CARTESIAN_POINT('Ctrl Pts',(3.52236173899994,2.2,-1.88224066100001));
#349877=CARTESIAN_POINT('Ctrl Pts',(3.52236778764287,12.2,-1.88224386181091));
#349878=CARTESIAN_POINT('Ctrl Pts',(3.52236778764287,5.2,-1.88224386181091));
#349879=CARTESIAN_POINT('Ctrl Pts',(3.52236778764287,2.2,-1.88224386181091));
#349880=CARTESIAN_POINT('Ctrl Pts',(3.52237948178093,12.2,-1.88225005510073));
#349881=CARTESIAN_POINT('Ctrl Pts',(3.52237948178093,5.2,-1.88225005510073));
#349882=CARTESIAN_POINT('Ctrl Pts',(3.52237948178093,2.2,-1.88225005510073));
#349883=CARTESIAN_POINT('Ctrl Pts',(3.52239682951887,12.2,-1.88225923963477));
#349884=CARTESIAN_POINT('Ctrl Pts',(3.52239682951887,5.2,-1.88225923963477));
#349885=CARTESIAN_POINT('Ctrl Pts',(3.52239682951887,2.2,-1.88225923963477));
#349886=CARTESIAN_POINT('Ctrl Pts',(3.52241983802047,12.2,-1.88227141541148));
#349887=CARTESIAN_POINT('Ctrl Pts',(3.52241983802047,5.2,-1.88227141541148));
#349888=CARTESIAN_POINT('Ctrl Pts',(3.52241983802047,2.2,-1.88227141541148));
#349889=CARTESIAN_POINT('Ctrl Pts',(3.52245994599994,12.2,-1.88229242900002));
#349890=CARTESIAN_POINT('Ctrl Pts',(3.52245994599994,5.2,-1.88229242900002));
#349891=CARTESIAN_POINT('Ctrl Pts',(3.52245994599994,2.2,-1.88229242900002));
#349892=CARTESIAN_POINT('Ctrl Pts',(3.52250459199994,12.2,-1.88231573900001));
#349893=CARTESIAN_POINT('Ctrl Pts',(3.52250459199994,5.2,-1.88231573900001));
#349894=CARTESIAN_POINT('Ctrl Pts',(3.52250459199994,2.2,-1.88231573900001));
#349895=CARTESIAN_POINT('Ctrl Pts',(3.52255579699994,12.2,-1.88234238500002));
#349896=CARTESIAN_POINT('Ctrl Pts',(3.52255579699994,5.2,-1.88234238500002));
#349897=CARTESIAN_POINT('Ctrl Pts',(3.52255579699994,2.2,-1.88234238500002));
#349898=CARTESIAN_POINT('Ctrl Pts',(3.52261355799994,12.2,-1.88237235300001));
#349899=CARTESIAN_POINT('Ctrl Pts',(3.52261355799994,5.2,-1.88237235300001));
#349900=CARTESIAN_POINT('Ctrl Pts',(3.52261355799994,2.2,-1.88237235300001));
#349901=CARTESIAN_POINT('Ctrl Pts',(3.52267787099994,12.2,-1.88240562300001));
#349902=CARTESIAN_POINT('Ctrl Pts',(3.52267787099994,5.2,-1.88240562300001));
#349903=CARTESIAN_POINT('Ctrl Pts',(3.52267787099994,2.2,-1.88240562300001));
#349904=CARTESIAN_POINT('Ctrl Pts',(3.52274872699994,12.2,-1.88244216800001));
#349905=CARTESIAN_POINT('Ctrl Pts',(3.52274872699994,5.2,-1.88244216800001));
#349906=CARTESIAN_POINT('Ctrl Pts',(3.52274872699994,2.2,-1.88244216800001));
#349907=CARTESIAN_POINT('Ctrl Pts',(3.52282612199994,12.2,-1.88248195500002));
#349908=CARTESIAN_POINT('Ctrl Pts',(3.52282612199994,5.2,-1.88248195500002));
#349909=CARTESIAN_POINT('Ctrl Pts',(3.52282612199994,2.2,-1.88248195500002));
#349910=CARTESIAN_POINT('Ctrl Pts',(3.52291004499994,12.2,-1.88252495200001));
#349911=CARTESIAN_POINT('Ctrl Pts',(3.52291004499994,5.2,-1.88252495200001));
#349912=CARTESIAN_POINT('Ctrl Pts',(3.52291004499994,2.2,-1.88252495200001));
#349913=CARTESIAN_POINT('Ctrl Pts',(3.52300048899994,12.2,-1.88257113000001));
#349914=CARTESIAN_POINT('Ctrl Pts',(3.52300048899994,5.2,-1.88257113000001));
#349915=CARTESIAN_POINT('Ctrl Pts',(3.52300048899994,2.2,-1.88257113000001));
#349916=CARTESIAN_POINT('Ctrl Pts',(3.52309744999994,12.2,-1.88262046600002));
#349917=CARTESIAN_POINT('Ctrl Pts',(3.52309744999994,5.2,-1.88262046600002));
#349918=CARTESIAN_POINT('Ctrl Pts',(3.52309744999994,2.2,-1.88262046600002));
#349919=CARTESIAN_POINT('Ctrl Pts',(3.52320092099994,12.2,-1.88267293300001));
#349920=CARTESIAN_POINT('Ctrl Pts',(3.52320092099994,5.2,-1.88267293300001));
#349921=CARTESIAN_POINT('Ctrl Pts',(3.52320092099994,2.2,-1.88267293300001));
#349922=CARTESIAN_POINT('Ctrl Pts',(3.52331089799994,12.2,-1.88272851300002));
#349923=CARTESIAN_POINT('Ctrl Pts',(3.52331089799994,5.2,-1.88272851300002));
#349924=CARTESIAN_POINT('Ctrl Pts',(3.52331089799994,2.2,-1.88272851300002));
#349925=CARTESIAN_POINT('Ctrl Pts',(3.52342737399994,12.2,-1.88278718000001));
#349926=CARTESIAN_POINT('Ctrl Pts',(3.52342737399994,5.2,-1.88278718000001));
#349927=CARTESIAN_POINT('Ctrl Pts',(3.52342737399994,2.2,-1.88278718000001));
#349928=CARTESIAN_POINT('Ctrl Pts',(3.52355034299995,12.2,-1.88284891300002));
#349929=CARTESIAN_POINT('Ctrl Pts',(3.52355034299995,5.2,-1.88284891300002));
#349930=CARTESIAN_POINT('Ctrl Pts',(3.52355034299995,2.2,-1.88284891300002));
#349931=CARTESIAN_POINT('Ctrl Pts',(3.52367979899994,12.2,-1.88291368400002));
#349932=CARTESIAN_POINT('Ctrl Pts',(3.52367979899994,5.2,-1.88291368400002));
#349933=CARTESIAN_POINT('Ctrl Pts',(3.52367979899994,2.2,-1.88291368400002));
#349934=CARTESIAN_POINT('Ctrl Pts',(3.52381573499994,12.2,-1.88298147000001));
#349935=CARTESIAN_POINT('Ctrl Pts',(3.52381573499994,5.2,-1.88298147000001));
#349936=CARTESIAN_POINT('Ctrl Pts',(3.52381573499994,2.2,-1.88298147000001));
#349937=CARTESIAN_POINT('Ctrl Pts',(3.52395814699995,12.2,-1.88305224500001));
#349938=CARTESIAN_POINT('Ctrl Pts',(3.52395814699995,5.2,-1.88305224500001));
#349939=CARTESIAN_POINT('Ctrl Pts',(3.52395814699995,2.2,-1.88305224500001));
#349940=CARTESIAN_POINT('Ctrl Pts',(3.52410702599994,12.2,-1.88312598300001));
#349941=CARTESIAN_POINT('Ctrl Pts',(3.52410702599994,5.2,-1.88312598300001));
#349942=CARTESIAN_POINT('Ctrl Pts',(3.52410702599994,2.2,-1.88312598300001));
#349943=CARTESIAN_POINT('Ctrl Pts',(3.52426236699994,12.2,-1.88320266000002));
#349944=CARTESIAN_POINT('Ctrl Pts',(3.52426236699994,5.2,-1.88320266000002));
#349945=CARTESIAN_POINT('Ctrl Pts',(3.52426236699994,2.2,-1.88320266000002));
#349946=CARTESIAN_POINT('Ctrl Pts',(3.52442416399994,12.2,-1.88328225300001));
#349947=CARTESIAN_POINT('Ctrl Pts',(3.52442416399994,5.2,-1.88328225300001));
#349948=CARTESIAN_POINT('Ctrl Pts',(3.52442416399994,2.2,-1.88328225300001));
#349949=CARTESIAN_POINT('Ctrl Pts',(3.52459241099994,12.2,-1.88336473900002));
#349950=CARTESIAN_POINT('Ctrl Pts',(3.52459241099994,5.2,-1.88336473900002));
#349951=CARTESIAN_POINT('Ctrl Pts',(3.52459241099994,2.2,-1.88336473900002));
#349952=CARTESIAN_POINT('Ctrl Pts',(3.52476710199995,12.2,-1.88345009300001));
#349953=CARTESIAN_POINT('Ctrl Pts',(3.52476710199995,5.2,-1.88345009300001));
#349954=CARTESIAN_POINT('Ctrl Pts',(3.52476710199995,2.2,-1.88345009300001));
#349955=CARTESIAN_POINT('Ctrl Pts',(3.52494822899994,12.2,-1.88353829200001));
#349956=CARTESIAN_POINT('Ctrl Pts',(3.52494822899994,5.2,-1.88353829200001));
#349957=CARTESIAN_POINT('Ctrl Pts',(3.52494822899994,2.2,-1.88353829200001));
#349958=CARTESIAN_POINT('Ctrl Pts',(3.52513578899994,12.2,-1.88362931300002));
#349959=CARTESIAN_POINT('Ctrl Pts',(3.52513578899994,5.2,-1.88362931300002));
#349960=CARTESIAN_POINT('Ctrl Pts',(3.52513578899994,2.2,-1.88362931300002));
#349961=CARTESIAN_POINT('Ctrl Pts',(3.52532977399994,12.2,-1.88372313000002));
#349962=CARTESIAN_POINT('Ctrl Pts',(3.52532977399994,5.2,-1.88372313000002));
#349963=CARTESIAN_POINT('Ctrl Pts',(3.52532977399994,2.2,-1.88372313000002));
#349964=CARTESIAN_POINT('Ctrl Pts',(3.52553017799994,12.2,-1.88381972200002));
#349965=CARTESIAN_POINT('Ctrl Pts',(3.52553017799994,5.2,-1.88381972200002));
#349966=CARTESIAN_POINT('Ctrl Pts',(3.52553017799994,2.2,-1.88381972200002));
#349967=CARTESIAN_POINT('Ctrl Pts',(3.52573699499994,12.2,-1.88391906300001));
#349968=CARTESIAN_POINT('Ctrl Pts',(3.52573699499994,5.2,-1.88391906300001));
#349969=CARTESIAN_POINT('Ctrl Pts',(3.52573699499994,2.2,-1.88391906300001));
#349970=CARTESIAN_POINT('Ctrl Pts',(3.52595021799994,12.2,-1.88402113000001));
#349971=CARTESIAN_POINT('Ctrl Pts',(3.52595021799994,5.2,-1.88402113000001));
#349972=CARTESIAN_POINT('Ctrl Pts',(3.52595021799994,2.2,-1.88402113000001));
#349973=CARTESIAN_POINT('Ctrl Pts',(3.52616984199994,12.2,-1.88412590200001));
#349974=CARTESIAN_POINT('Ctrl Pts',(3.52616984199994,5.2,-1.88412590200001));
#349975=CARTESIAN_POINT('Ctrl Pts',(3.52616984199994,2.2,-1.88412590200001));
#349976=CARTESIAN_POINT('Ctrl Pts',(3.52639585899994,12.2,-1.88423335500001));
#349977=CARTESIAN_POINT('Ctrl Pts',(3.52639585899994,5.2,-1.88423335500001));
#349978=CARTESIAN_POINT('Ctrl Pts',(3.52639585899994,2.2,-1.88423335500001));
#349979=CARTESIAN_POINT('Ctrl Pts',(3.52662826599994,12.2,-1.88434346400001));
#349980=CARTESIAN_POINT('Ctrl Pts',(3.52662826599994,5.2,-1.88434346400001));
#349981=CARTESIAN_POINT('Ctrl Pts',(3.52662826599994,2.2,-1.88434346400001));
#349982=CARTESIAN_POINT('Ctrl Pts',(3.52686705399994,12.2,-1.88445620700001));
#349983=CARTESIAN_POINT('Ctrl Pts',(3.52686705399994,5.2,-1.88445620700001));
#349984=CARTESIAN_POINT('Ctrl Pts',(3.52686705399994,2.2,-1.88445620700001));
#349985=CARTESIAN_POINT('Ctrl Pts',(3.52711221799995,12.2,-1.88457156200001));
#349986=CARTESIAN_POINT('Ctrl Pts',(3.52711221799995,5.2,-1.88457156200001));
#349987=CARTESIAN_POINT('Ctrl Pts',(3.52711221799995,2.2,-1.88457156200001));
#349988=CARTESIAN_POINT('Ctrl Pts',(3.52736375099994,12.2,-1.88468950600001));
#349989=CARTESIAN_POINT('Ctrl Pts',(3.52736375099994,5.2,-1.88468950600001));
#349990=CARTESIAN_POINT('Ctrl Pts',(3.52736375099994,2.2,-1.88468950600001));
#349991=CARTESIAN_POINT('Ctrl Pts',(3.52762164799994,12.2,-1.88481001500001));
#349992=CARTESIAN_POINT('Ctrl Pts',(3.52762164799994,5.2,-1.88481001500001));
#349993=CARTESIAN_POINT('Ctrl Pts',(3.52762164799994,2.2,-1.88481001500001));
#349994=CARTESIAN_POINT('Ctrl Pts',(3.52788590099994,12.2,-1.88493306700002));
#349995=CARTESIAN_POINT('Ctrl Pts',(3.52788590099994,5.2,-1.88493306700002));
#349996=CARTESIAN_POINT('Ctrl Pts',(3.52788590099994,2.2,-1.88493306700002));
#349997=CARTESIAN_POINT('Ctrl Pts',(3.52815650599994,12.2,-1.88505864000001));
#349998=CARTESIAN_POINT('Ctrl Pts',(3.52815650599994,5.2,-1.88505864000001));
#349999=CARTESIAN_POINT('Ctrl Pts',(3.52815650599994,2.2,-1.88505864000001));
#350000=CARTESIAN_POINT('Ctrl Pts',(3.52843345499994,12.2,-1.88518671200002));
#350001=CARTESIAN_POINT('Ctrl Pts',(3.52843345499994,5.2,-1.88518671200002));
#350002=CARTESIAN_POINT('Ctrl Pts',(3.52843345499994,2.2,-1.88518671200002));
#350003=CARTESIAN_POINT('Ctrl Pts',(3.52871674199994,12.2,-1.88531725700001));
#350004=CARTESIAN_POINT('Ctrl Pts',(3.52871674199994,5.2,-1.88531725700001));
#350005=CARTESIAN_POINT('Ctrl Pts',(3.52871674199994,2.2,-1.88531725700001));
#350006=CARTESIAN_POINT('Ctrl Pts',(3.52900636199994,12.2,-1.88545025700002));
#350007=CARTESIAN_POINT('Ctrl Pts',(3.52900636199994,5.2,-1.88545025700002));
#350008=CARTESIAN_POINT('Ctrl Pts',(3.52900636199994,2.2,-1.88545025700002));
#350009=CARTESIAN_POINT('Ctrl Pts',(3.52930230799994,12.2,-1.88558568800001));
#350010=CARTESIAN_POINT('Ctrl Pts',(3.52930230799994,5.2,-1.88558568800001));
#350011=CARTESIAN_POINT('Ctrl Pts',(3.52930230799994,2.2,-1.88558568800001));
#350012=CARTESIAN_POINT('Ctrl Pts',(3.52960457399994,12.2,-1.88572352700001));
#350013=CARTESIAN_POINT('Ctrl Pts',(3.52960457399994,5.2,-1.88572352700001));
#350014=CARTESIAN_POINT('Ctrl Pts',(3.52960457399994,2.2,-1.88572352700001));
#350015=CARTESIAN_POINT('Ctrl Pts',(3.52991315199994,12.2,-1.88586375300002));
#350016=CARTESIAN_POINT('Ctrl Pts',(3.52991315199994,5.2,-1.88586375300002));
#350017=CARTESIAN_POINT('Ctrl Pts',(3.52991315199994,2.2,-1.88586375300002));
#350018=CARTESIAN_POINT('Ctrl Pts',(3.53022803899994,12.2,-1.88600634300002));
#350019=CARTESIAN_POINT('Ctrl Pts',(3.53022803899994,5.2,-1.88600634300002));
#350020=CARTESIAN_POINT('Ctrl Pts',(3.53022803899994,2.2,-1.88600634300002));
#350021=CARTESIAN_POINT('Ctrl Pts',(3.53054922599994,12.2,-1.88615127700002));
#350022=CARTESIAN_POINT('Ctrl Pts',(3.53054922599994,5.2,-1.88615127700002));
#350023=CARTESIAN_POINT('Ctrl Pts',(3.53054922599994,2.2,-1.88615127700002));
#350024=CARTESIAN_POINT('Ctrl Pts',(3.53087670799995,12.2,-1.88629853200001));
#350025=CARTESIAN_POINT('Ctrl Pts',(3.53087670799995,5.2,-1.88629853200001));
#350026=CARTESIAN_POINT('Ctrl Pts',(3.53087670799995,2.2,-1.88629853200001));
#350027=CARTESIAN_POINT('Ctrl Pts',(3.53121047799994,12.2,-1.88644808500001));
#350028=CARTESIAN_POINT('Ctrl Pts',(3.53121047799994,5.2,-1.88644808500001));
#350029=CARTESIAN_POINT('Ctrl Pts',(3.53121047799994,2.2,-1.88644808500001));
#350030=CARTESIAN_POINT('Ctrl Pts',(3.53155053099994,12.2,-1.88659991600002));
#350031=CARTESIAN_POINT('Ctrl Pts',(3.53155053099994,5.2,-1.88659991600002));
#350032=CARTESIAN_POINT('Ctrl Pts',(3.53155053099994,2.2,-1.88659991600002));
#350033=CARTESIAN_POINT('Ctrl Pts',(3.53189685999994,12.2,-1.88675400300002));
#350034=CARTESIAN_POINT('Ctrl Pts',(3.53189685999994,5.2,-1.88675400300002));
#350035=CARTESIAN_POINT('Ctrl Pts',(3.53189685999994,2.2,-1.88675400300002));
#350036=CARTESIAN_POINT('Ctrl Pts',(3.53224945799994,12.2,-1.88691032400001));
#350037=CARTESIAN_POINT('Ctrl Pts',(3.53224945799994,5.2,-1.88691032400001));
#350038=CARTESIAN_POINT('Ctrl Pts',(3.53224945799994,2.2,-1.88691032400001));
#350039=CARTESIAN_POINT('Ctrl Pts',(3.53260831999994,12.2,-1.88706885800002));
#350040=CARTESIAN_POINT('Ctrl Pts',(3.53260831999994,5.2,-1.88706885800002));
#350041=CARTESIAN_POINT('Ctrl Pts',(3.53260831999994,2.2,-1.88706885800002));
#350042=CARTESIAN_POINT('Ctrl Pts',(3.53297343799994,12.2,-1.88722958300001));
#350043=CARTESIAN_POINT('Ctrl Pts',(3.53297343799994,5.2,-1.88722958300001));
#350044=CARTESIAN_POINT('Ctrl Pts',(3.53297343799994,2.2,-1.88722958300001));
#350045=CARTESIAN_POINT('Ctrl Pts',(3.53334480699994,12.2,-1.88739247900001));
#350046=CARTESIAN_POINT('Ctrl Pts',(3.53334480699994,5.2,-1.88739247900001));
#350047=CARTESIAN_POINT('Ctrl Pts',(3.53334480699994,2.2,-1.88739247900001));
#350048=CARTESIAN_POINT('Ctrl Pts',(3.53372242199994,12.2,-1.88755752400001));
#350049=CARTESIAN_POINT('Ctrl Pts',(3.53372242199994,5.2,-1.88755752400001));
#350050=CARTESIAN_POINT('Ctrl Pts',(3.53372242199994,2.2,-1.88755752400001));
#350051=CARTESIAN_POINT('Ctrl Pts',(3.53410627399994,12.2,-1.88772469600002));
#350052=CARTESIAN_POINT('Ctrl Pts',(3.53410627399994,5.2,-1.88772469600002));
#350053=CARTESIAN_POINT('Ctrl Pts',(3.53410627399994,2.2,-1.88772469600002));
#350054=CARTESIAN_POINT('Ctrl Pts',(3.53449635899994,12.2,-1.88789397500001));
#350055=CARTESIAN_POINT('Ctrl Pts',(3.53449635899994,5.2,-1.88789397500001));
#350056=CARTESIAN_POINT('Ctrl Pts',(3.53449635899994,2.2,-1.88789397500001));
#350057=CARTESIAN_POINT('Ctrl Pts',(3.53489266999994,12.2,-1.88806533900001));
#350058=CARTESIAN_POINT('Ctrl Pts',(3.53489266999994,5.2,-1.88806533900001));
#350059=CARTESIAN_POINT('Ctrl Pts',(3.53489266999994,2.2,-1.88806533900001));
#350060=CARTESIAN_POINT('Ctrl Pts',(3.53529519999995,12.2,-1.88823876900001));
#350061=CARTESIAN_POINT('Ctrl Pts',(3.53529519999995,5.2,-1.88823876900001));
#350062=CARTESIAN_POINT('Ctrl Pts',(3.53529519999995,2.2,-1.88823876900001));
#350063=CARTESIAN_POINT('Ctrl Pts',(3.53570394199994,12.2,-1.88841424200001));
#350064=CARTESIAN_POINT('Ctrl Pts',(3.53570394199994,5.2,-1.88841424200001));
#350065=CARTESIAN_POINT('Ctrl Pts',(3.53570394199994,2.2,-1.88841424200001));
#350066=CARTESIAN_POINT('Ctrl Pts',(3.53611889099994,12.2,-1.88859173900001));
#350067=CARTESIAN_POINT('Ctrl Pts',(3.53611889099994,5.2,-1.88859173900001));
#350068=CARTESIAN_POINT('Ctrl Pts',(3.53611889099994,2.2,-1.88859173900001));
#350069=CARTESIAN_POINT('Ctrl Pts',(3.53654004199994,12.2,-1.88877123800001));
#350070=CARTESIAN_POINT('Ctrl Pts',(3.53654004199994,5.2,-1.88877123800001));
#350071=CARTESIAN_POINT('Ctrl Pts',(3.53654004199994,2.2,-1.88877123800001));
#350072=CARTESIAN_POINT('Ctrl Pts',(3.53696738599994,12.2,-1.88895271800002));
#350073=CARTESIAN_POINT('Ctrl Pts',(3.53696738599994,5.2,-1.88895271800002));
#350074=CARTESIAN_POINT('Ctrl Pts',(3.53696738599994,2.2,-1.88895271800002));
#350075=CARTESIAN_POINT('Ctrl Pts',(3.53740091799994,12.2,-1.88913616000002));
#350076=CARTESIAN_POINT('Ctrl Pts',(3.53740091799994,5.2,-1.88913616000002));
#350077=CARTESIAN_POINT('Ctrl Pts',(3.53740091799994,2.2,-1.88913616000002));
#350078=CARTESIAN_POINT('Ctrl Pts',(3.53784063199994,12.2,-1.88932154300002));
#350079=CARTESIAN_POINT('Ctrl Pts',(3.53784063199994,5.2,-1.88932154300002));
#350080=CARTESIAN_POINT('Ctrl Pts',(3.53784063199994,2.2,-1.88932154300002));
#350081=CARTESIAN_POINT('Ctrl Pts',(3.53828651899994,12.2,-1.88950884700001));
#350082=CARTESIAN_POINT('Ctrl Pts',(3.53828651899994,5.2,-1.88950884700001));
#350083=CARTESIAN_POINT('Ctrl Pts',(3.53828651899994,2.2,-1.88950884700001));
#350084=CARTESIAN_POINT('Ctrl Pts',(3.53873857699994,12.2,-1.88969805000001));
#350085=CARTESIAN_POINT('Ctrl Pts',(3.53873857699994,5.2,-1.88969805000001));
#350086=CARTESIAN_POINT('Ctrl Pts',(3.53873857699994,2.2,-1.88969805000001));
#350087=CARTESIAN_POINT('Ctrl Pts',(3.53919679799994,12.2,-1.88988913300001));
#350088=CARTESIAN_POINT('Ctrl Pts',(3.53919679799994,5.2,-1.88988913300001));
#350089=CARTESIAN_POINT('Ctrl Pts',(3.53919679799994,2.2,-1.88988913300001));
#350090=CARTESIAN_POINT('Ctrl Pts',(3.53966117399994,12.2,-1.89008207500001));
#350091=CARTESIAN_POINT('Ctrl Pts',(3.53966117399994,5.2,-1.89008207500001));
#350092=CARTESIAN_POINT('Ctrl Pts',(3.53966117399994,2.2,-1.89008207500001));
#350093=CARTESIAN_POINT('Ctrl Pts',(3.54013169999994,12.2,-1.89027685700002));
#350094=CARTESIAN_POINT('Ctrl Pts',(3.54013169999994,5.2,-1.89027685700002));
#350095=CARTESIAN_POINT('Ctrl Pts',(3.54013169999994,2.2,-1.89027685700002));
#350096=CARTESIAN_POINT('Ctrl Pts',(3.54060836999994,12.2,-1.89047345800001));
#350097=CARTESIAN_POINT('Ctrl Pts',(3.54060836999994,5.2,-1.89047345800001));
#350098=CARTESIAN_POINT('Ctrl Pts',(3.54060836999994,2.2,-1.89047345800001));
#350099=CARTESIAN_POINT('Ctrl Pts',(3.54109117699994,12.2,-1.89067186000001));
#350100=CARTESIAN_POINT('Ctrl Pts',(3.54109117699994,5.2,-1.89067186000001));
#350101=CARTESIAN_POINT('Ctrl Pts',(3.54109117699994,2.2,-1.89067186000001));
#350102=CARTESIAN_POINT('Ctrl Pts',(3.54158011499994,12.2,-1.89087203900002));
#350103=CARTESIAN_POINT('Ctrl Pts',(3.54158011499994,5.2,-1.89087203900002));
#350104=CARTESIAN_POINT('Ctrl Pts',(3.54158011499994,2.2,-1.89087203900002));
#350105=CARTESIAN_POINT('Ctrl Pts',(3.54207517599994,12.2,-1.89107397900001));
#350106=CARTESIAN_POINT('Ctrl Pts',(3.54207517599994,5.2,-1.89107397900001));
#350107=CARTESIAN_POINT('Ctrl Pts',(3.54207517599994,2.2,-1.89107397900001));
#350108=CARTESIAN_POINT('Ctrl Pts',(3.54257635599994,12.2,-1.89127765800002));
#350109=CARTESIAN_POINT('Ctrl Pts',(3.54257635599994,5.2,-1.89127765800002));
#350110=CARTESIAN_POINT('Ctrl Pts',(3.54257635599994,2.2,-1.89127765800002));
#350111=CARTESIAN_POINT('Ctrl Pts',(3.54308364899994,12.2,-1.89148305800002));
#350112=CARTESIAN_POINT('Ctrl Pts',(3.54308364899994,5.2,-1.89148305800002));
#350113=CARTESIAN_POINT('Ctrl Pts',(3.54308364899994,2.2,-1.89148305800002));
#350114=CARTESIAN_POINT('Ctrl Pts',(3.54359704599994,12.2,-1.89169015800001));
#350115=CARTESIAN_POINT('Ctrl Pts',(3.54359704599994,5.2,-1.89169015800001));
#350116=CARTESIAN_POINT('Ctrl Pts',(3.54359704599994,2.2,-1.89169015800001));
#350117=CARTESIAN_POINT('Ctrl Pts',(3.54411654299994,12.2,-1.89189893900001));
#350118=CARTESIAN_POINT('Ctrl Pts',(3.54411654299994,5.2,-1.89189893900001));
#350119=CARTESIAN_POINT('Ctrl Pts',(3.54411654299994,2.2,-1.89189893900001));
#350120=CARTESIAN_POINT('Ctrl Pts',(3.54464213099994,12.2,-1.89210938200001));
#350121=CARTESIAN_POINT('Ctrl Pts',(3.54464213099994,5.2,-1.89210938200001));
#350122=CARTESIAN_POINT('Ctrl Pts',(3.54464213099994,2.2,-1.89210938200001));
#350123=CARTESIAN_POINT('Ctrl Pts',(3.54517380599995,12.2,-1.89232146600002));
#350124=CARTESIAN_POINT('Ctrl Pts',(3.54517380599995,5.2,-1.89232146600002));
#350125=CARTESIAN_POINT('Ctrl Pts',(3.54517380599995,2.2,-1.89232146600002));
#350126=CARTESIAN_POINT('Ctrl Pts',(3.54571156199994,12.2,-1.89253517200001));
#350127=CARTESIAN_POINT('Ctrl Pts',(3.54571156199994,5.2,-1.89253517200001));
#350128=CARTESIAN_POINT('Ctrl Pts',(3.54571156199994,2.2,-1.89253517200001));
#350129=CARTESIAN_POINT('Ctrl Pts',(3.54625538999994,12.2,-1.89275048300001));
#350130=CARTESIAN_POINT('Ctrl Pts',(3.54625538999994,5.2,-1.89275048300001));
#350131=CARTESIAN_POINT('Ctrl Pts',(3.54625538999994,2.2,-1.89275048300001));
#350132=CARTESIAN_POINT('Ctrl Pts',(3.54680528599994,12.2,-1.89296737700001));
#350133=CARTESIAN_POINT('Ctrl Pts',(3.54680528599994,5.2,-1.89296737700001));
#350134=CARTESIAN_POINT('Ctrl Pts',(3.54680528599994,2.2,-1.89296737700001));
#350135=CARTESIAN_POINT('Ctrl Pts',(3.54736124099994,12.2,-1.89318583500001));
#350136=CARTESIAN_POINT('Ctrl Pts',(3.54736124099994,5.2,-1.89318583500001));
#350137=CARTESIAN_POINT('Ctrl Pts',(3.54736124099994,2.2,-1.89318583500001));
#350138=CARTESIAN_POINT('Ctrl Pts',(3.54792325099994,12.2,-1.89340584000002));
#350139=CARTESIAN_POINT('Ctrl Pts',(3.54792325099994,5.2,-1.89340584000002));
#350140=CARTESIAN_POINT('Ctrl Pts',(3.54792325099994,2.2,-1.89340584000002));
#350141=CARTESIAN_POINT('Ctrl Pts',(3.54849131099995,12.2,-1.89362737100002));
#350142=CARTESIAN_POINT('Ctrl Pts',(3.54849131099995,5.2,-1.89362737100002));
#350143=CARTESIAN_POINT('Ctrl Pts',(3.54849131099995,2.2,-1.89362737100002));
#350144=CARTESIAN_POINT('Ctrl Pts',(3.54906540999994,12.2,-1.89385041000001));
#350145=CARTESIAN_POINT('Ctrl Pts',(3.54906540999994,5.2,-1.89385041000001));
#350146=CARTESIAN_POINT('Ctrl Pts',(3.54906540999994,2.2,-1.89385041000001));
#350147=CARTESIAN_POINT('Ctrl Pts',(3.54964554499994,12.2,-1.89407493700001));
#350148=CARTESIAN_POINT('Ctrl Pts',(3.54964554499994,5.2,-1.89407493700001));
#350149=CARTESIAN_POINT('Ctrl Pts',(3.54964554499994,2.2,-1.89407493700001));
#350150=CARTESIAN_POINT('Ctrl Pts',(3.55023170899994,12.2,-1.89430093400001));
#350151=CARTESIAN_POINT('Ctrl Pts',(3.55023170899994,5.2,-1.89430093400001));
#350152=CARTESIAN_POINT('Ctrl Pts',(3.55023170899994,2.2,-1.89430093400001));
#350153=CARTESIAN_POINT('Ctrl Pts',(3.55082389399994,12.2,-1.89452838300001));
#350154=CARTESIAN_POINT('Ctrl Pts',(3.55082389399994,5.2,-1.89452838300001));
#350155=CARTESIAN_POINT('Ctrl Pts',(3.55082389399994,2.2,-1.89452838300001));
#350156=CARTESIAN_POINT('Ctrl Pts',(3.55142209599994,12.2,-1.89475726400001));
#350157=CARTESIAN_POINT('Ctrl Pts',(3.55142209599994,5.2,-1.89475726400001));
#350158=CARTESIAN_POINT('Ctrl Pts',(3.55142209599994,2.2,-1.89475726400001));
#350159=CARTESIAN_POINT('Ctrl Pts',(3.55202630799994,12.2,-1.89498755800001));
#350160=CARTESIAN_POINT('Ctrl Pts',(3.55202630799994,5.2,-1.89498755800001));
#350161=CARTESIAN_POINT('Ctrl Pts',(3.55202630799994,2.2,-1.89498755800001));
#350162=CARTESIAN_POINT('Ctrl Pts',(3.55263652199994,12.2,-1.89521924800002));
#350163=CARTESIAN_POINT('Ctrl Pts',(3.55263652199994,5.2,-1.89521924800002));
#350164=CARTESIAN_POINT('Ctrl Pts',(3.55263652199994,2.2,-1.89521924800002));
#350165=CARTESIAN_POINT('Ctrl Pts',(3.55325273199994,12.2,-1.89545231400002));
#350166=CARTESIAN_POINT('Ctrl Pts',(3.55325273199994,5.2,-1.89545231400002));
#350167=CARTESIAN_POINT('Ctrl Pts',(3.55325273199994,2.2,-1.89545231400002));
#350168=CARTESIAN_POINT('Ctrl Pts',(3.55387493299994,12.2,-1.89568673900002));
#350169=CARTESIAN_POINT('Ctrl Pts',(3.55387493299994,5.2,-1.89568673900002));
#350170=CARTESIAN_POINT('Ctrl Pts',(3.55387493299994,2.2,-1.89568673900002));
#350171=CARTESIAN_POINT('Ctrl Pts',(3.55450311699994,12.2,-1.89592250200001));
#350172=CARTESIAN_POINT('Ctrl Pts',(3.55450311699994,5.2,-1.89592250200001));
#350173=CARTESIAN_POINT('Ctrl Pts',(3.55450311699994,2.2,-1.89592250200001));
#350174=CARTESIAN_POINT('Ctrl Pts',(3.55513727899994,12.2,-1.89615958700001));
#350175=CARTESIAN_POINT('Ctrl Pts',(3.55513727899994,5.2,-1.89615958700001));
#350176=CARTESIAN_POINT('Ctrl Pts',(3.55513727899994,2.2,-1.89615958700001));
#350177=CARTESIAN_POINT('Ctrl Pts',(3.55577741199994,12.2,-1.89639797500002));
#350178=CARTESIAN_POINT('Ctrl Pts',(3.55577741199994,5.2,-1.89639797500002));
#350179=CARTESIAN_POINT('Ctrl Pts',(3.55577741199994,2.2,-1.89639797500002));
#350180=CARTESIAN_POINT('Ctrl Pts',(3.55642350799994,12.2,-1.89663764800001));
#350181=CARTESIAN_POINT('Ctrl Pts',(3.55642350799994,5.2,-1.89663764800001));
#350182=CARTESIAN_POINT('Ctrl Pts',(3.55642350799994,2.2,-1.89663764800001));
#350183=CARTESIAN_POINT('Ctrl Pts',(3.55707556299994,12.2,-1.89687858700001));
#350184=CARTESIAN_POINT('Ctrl Pts',(3.55707556299994,5.2,-1.89687858700001));
#350185=CARTESIAN_POINT('Ctrl Pts',(3.55707556299994,2.2,-1.89687858700001));
#350186=CARTESIAN_POINT('Ctrl Pts',(3.55773356999994,12.2,-1.89712077500001));
#350187=CARTESIAN_POINT('Ctrl Pts',(3.55773356999994,5.2,-1.89712077500001));
#350188=CARTESIAN_POINT('Ctrl Pts',(3.55773356999994,2.2,-1.89712077500001));
#350189=CARTESIAN_POINT('Ctrl Pts',(3.55839752099994,12.2,-1.89736419200001));
#350190=CARTESIAN_POINT('Ctrl Pts',(3.55839752099994,5.2,-1.89736419200001));
#350191=CARTESIAN_POINT('Ctrl Pts',(3.55839752099994,2.2,-1.89736419200001));
#350192=CARTESIAN_POINT('Ctrl Pts',(3.55906741099994,12.2,-1.89760882400002));
#350193=CARTESIAN_POINT('Ctrl Pts',(3.55906741099994,5.2,-1.89760882400002));
#350194=CARTESIAN_POINT('Ctrl Pts',(3.55906741099994,2.2,-1.89760882400002));
#350195=CARTESIAN_POINT('Ctrl Pts',(3.55974323299994,12.2,-1.89785464800002));
#350196=CARTESIAN_POINT('Ctrl Pts',(3.55974323299994,5.2,-1.89785464800002));
#350197=CARTESIAN_POINT('Ctrl Pts',(3.55974323299994,2.2,-1.89785464800002));
#350198=CARTESIAN_POINT('Ctrl Pts',(3.56042498099994,12.2,-1.89810164900001));
#350199=CARTESIAN_POINT('Ctrl Pts',(3.56042498099994,5.2,-1.89810164900001));
#350200=CARTESIAN_POINT('Ctrl Pts',(3.56042498099994,2.2,-1.89810164900001));
#350201=CARTESIAN_POINT('Ctrl Pts',(3.56111264699994,12.2,-1.89834981000002));
#350202=CARTESIAN_POINT('Ctrl Pts',(3.56111264699994,5.2,-1.89834981000002));
#350203=CARTESIAN_POINT('Ctrl Pts',(3.56111264699994,2.2,-1.89834981000002));
#350204=CARTESIAN_POINT('Ctrl Pts',(3.56180622499994,12.2,-1.89859911000001));
#350205=CARTESIAN_POINT('Ctrl Pts',(3.56180622499994,5.2,-1.89859911000001));
#350206=CARTESIAN_POINT('Ctrl Pts',(3.56180622499994,2.2,-1.89859911000001));
#350207=CARTESIAN_POINT('Ctrl Pts',(3.56250571199995,12.2,-1.89884953500002));
#350208=CARTESIAN_POINT('Ctrl Pts',(3.56250571199995,5.2,-1.89884953500002));
#350209=CARTESIAN_POINT('Ctrl Pts',(3.56250571199995,2.2,-1.89884953500002));
#350210=CARTESIAN_POINT('Ctrl Pts',(3.56321109699994,12.2,-1.89910106400001));
#350211=CARTESIAN_POINT('Ctrl Pts',(3.56321109699994,5.2,-1.89910106400001));
#350212=CARTESIAN_POINT('Ctrl Pts',(3.56321109699994,2.2,-1.89910106400001));
#350213=CARTESIAN_POINT('Ctrl Pts',(3.56392237499994,12.2,-1.89935368300001));
#350214=CARTESIAN_POINT('Ctrl Pts',(3.56392237499994,5.2,-1.89935368300001));
#350215=CARTESIAN_POINT('Ctrl Pts',(3.56392237499994,2.2,-1.89935368300001));
#350216=CARTESIAN_POINT('Ctrl Pts',(3.56463954099994,12.2,-1.89960737100002));
#350217=CARTESIAN_POINT('Ctrl Pts',(3.56463954099994,5.2,-1.89960737100002));
#350218=CARTESIAN_POINT('Ctrl Pts',(3.56463954099994,2.2,-1.89960737100002));
#350219=CARTESIAN_POINT('Ctrl Pts',(3.56536258599994,12.2,-1.89986211300001));
#350220=CARTESIAN_POINT('Ctrl Pts',(3.56536258599994,5.2,-1.89986211300001));
#350221=CARTESIAN_POINT('Ctrl Pts',(3.56536258599994,2.2,-1.89986211300001));
#350222=CARTESIAN_POINT('Ctrl Pts',(3.56609150599994,12.2,-1.90011789000001));
#350223=CARTESIAN_POINT('Ctrl Pts',(3.56609150599994,5.2,-1.90011789000001));
#350224=CARTESIAN_POINT('Ctrl Pts',(3.56609150599994,2.2,-1.90011789000001));
#350225=CARTESIAN_POINT('Ctrl Pts',(3.56682629199994,12.2,-1.90037468600002));
#350226=CARTESIAN_POINT('Ctrl Pts',(3.56682629199994,5.2,-1.90037468600002));
#350227=CARTESIAN_POINT('Ctrl Pts',(3.56682629199994,2.2,-1.90037468600002));
#350228=CARTESIAN_POINT('Ctrl Pts',(3.56756693899994,12.2,-1.90063248200001));
#350229=CARTESIAN_POINT('Ctrl Pts',(3.56756693899994,5.2,-1.90063248200001));
#350230=CARTESIAN_POINT('Ctrl Pts',(3.56756693899994,2.2,-1.90063248200001));
#350231=CARTESIAN_POINT('Ctrl Pts',(3.56831343999994,12.2,-1.90089126100002));
#350232=CARTESIAN_POINT('Ctrl Pts',(3.56831343999994,5.2,-1.90089126100002));
#350233=CARTESIAN_POINT('Ctrl Pts',(3.56831343999994,2.2,-1.90089126100002));
#350234=CARTESIAN_POINT('Ctrl Pts',(3.56906578999994,12.2,-1.90115100800002));
#350235=CARTESIAN_POINT('Ctrl Pts',(3.56906578999994,5.2,-1.90115100800002));
#350236=CARTESIAN_POINT('Ctrl Pts',(3.56906578999994,2.2,-1.90115100800002));
#350237=CARTESIAN_POINT('Ctrl Pts',(3.56982398099994,12.2,-1.90141170400001));
#350238=CARTESIAN_POINT('Ctrl Pts',(3.56982398099994,5.2,-1.90141170400001));
#350239=CARTESIAN_POINT('Ctrl Pts',(3.56982398099994,2.2,-1.90141170400001));
#350240=CARTESIAN_POINT('Ctrl Pts',(3.57058800599994,12.2,-1.90167333200002));
#350241=CARTESIAN_POINT('Ctrl Pts',(3.57058800599994,5.2,-1.90167333200002));
#350242=CARTESIAN_POINT('Ctrl Pts',(3.57058800599994,2.2,-1.90167333200002));
#350243=CARTESIAN_POINT('Ctrl Pts',(3.57135785899994,12.2,-1.90193587500001));
#350244=CARTESIAN_POINT('Ctrl Pts',(3.57135785899994,5.2,-1.90193587500001));
#350245=CARTESIAN_POINT('Ctrl Pts',(3.57135785899994,2.2,-1.90193587500001));
#350246=CARTESIAN_POINT('Ctrl Pts',(3.57213353499994,12.2,-1.90219931700002));
#350247=CARTESIAN_POINT('Ctrl Pts',(3.57213353499994,5.2,-1.90219931700002));
#350248=CARTESIAN_POINT('Ctrl Pts',(3.57213353499994,2.2,-1.90219931700002));
#350249=CARTESIAN_POINT('Ctrl Pts',(3.57291502499994,12.2,-1.90246364000001));
#350250=CARTESIAN_POINT('Ctrl Pts',(3.57291502499994,5.2,-1.90246364000001));
#350251=CARTESIAN_POINT('Ctrl Pts',(3.57291502499994,2.2,-1.90246364000001));
#350252=CARTESIAN_POINT('Ctrl Pts',(3.57370232399994,12.2,-1.90272882600001));
#350253=CARTESIAN_POINT('Ctrl Pts',(3.57370232399994,5.2,-1.90272882600001));
#350254=CARTESIAN_POINT('Ctrl Pts',(3.57370232399994,2.2,-1.90272882600001));
#350255=CARTESIAN_POINT('Ctrl Pts',(3.57449542499995,12.2,-1.90299486200002));
#350256=CARTESIAN_POINT('Ctrl Pts',(3.57449542499995,5.2,-1.90299486200002));
#350257=CARTESIAN_POINT('Ctrl Pts',(3.57449542499995,2.2,-1.90299486200002));
#350258=CARTESIAN_POINT('Ctrl Pts',(3.57529432199994,12.2,-1.90326172800001));
#350259=CARTESIAN_POINT('Ctrl Pts',(3.57529432199994,5.2,-1.90326172800001));
#350260=CARTESIAN_POINT('Ctrl Pts',(3.57529432199994,2.2,-1.90326172800001));
#350261=CARTESIAN_POINT('Ctrl Pts',(3.57609900899994,12.2,-1.90352940700001));
#350262=CARTESIAN_POINT('Ctrl Pts',(3.57609900899994,5.2,-1.90352940700001));
#350263=CARTESIAN_POINT('Ctrl Pts',(3.57609900899994,2.2,-1.90352940700001));
#350264=CARTESIAN_POINT('Ctrl Pts',(3.57690947699994,12.2,-1.90379788500001));
#350265=CARTESIAN_POINT('Ctrl Pts',(3.57690947699994,5.2,-1.90379788500001));
#350266=CARTESIAN_POINT('Ctrl Pts',(3.57690947699994,2.2,-1.90379788500001));
#350267=CARTESIAN_POINT('Ctrl Pts',(3.57772572199994,12.2,-1.90406714400002));
#350268=CARTESIAN_POINT('Ctrl Pts',(3.57772572199994,5.2,-1.90406714400002));
#350269=CARTESIAN_POINT('Ctrl Pts',(3.57772572199994,2.2,-1.90406714400002));
#350270=CARTESIAN_POINT('Ctrl Pts',(3.57854773599994,12.2,-1.90433716600001));
#350271=CARTESIAN_POINT('Ctrl Pts',(3.57854773599994,5.2,-1.90433716600001));
#350272=CARTESIAN_POINT('Ctrl Pts',(3.57854773599994,2.2,-1.90433716600001));
#350273=CARTESIAN_POINT('Ctrl Pts',(3.57937551199994,12.2,-1.90460793700002));
#350274=CARTESIAN_POINT('Ctrl Pts',(3.57937551199994,5.2,-1.90460793700002));
#350275=CARTESIAN_POINT('Ctrl Pts',(3.57937551199994,2.2,-1.90460793700002));
#350276=CARTESIAN_POINT('Ctrl Pts',(3.58020904499994,12.2,-1.90487943900001));
#350277=CARTESIAN_POINT('Ctrl Pts',(3.58020904499994,5.2,-1.90487943900001));
#350278=CARTESIAN_POINT('Ctrl Pts',(3.58020904499994,2.2,-1.90487943900001));
#350279=CARTESIAN_POINT('Ctrl Pts',(3.58104832799994,12.2,-1.90515165700001));
#350280=CARTESIAN_POINT('Ctrl Pts',(3.58104832799994,5.2,-1.90515165700001));
#350281=CARTESIAN_POINT('Ctrl Pts',(3.58104832799994,2.2,-1.90515165700001));
#350282=CARTESIAN_POINT('Ctrl Pts',(3.58189335499994,12.2,-1.90542457200001));
#350283=CARTESIAN_POINT('Ctrl Pts',(3.58189335499994,5.2,-1.90542457200001));
#350284=CARTESIAN_POINT('Ctrl Pts',(3.58189335499994,2.2,-1.90542457200001));
#350285=CARTESIAN_POINT('Ctrl Pts',(3.58274411699994,12.2,-1.90569817000001));
#350286=CARTESIAN_POINT('Ctrl Pts',(3.58274411699994,5.2,-1.90569817000001));
#350287=CARTESIAN_POINT('Ctrl Pts',(3.58274411699994,2.2,-1.90569817000001));
#350288=CARTESIAN_POINT('Ctrl Pts',(3.58360060999994,12.2,-1.90597243600001));
#350289=CARTESIAN_POINT('Ctrl Pts',(3.58360060999994,5.2,-1.90597243600001));
#350290=CARTESIAN_POINT('Ctrl Pts',(3.58360060999994,2.2,-1.90597243600001));
#350291=CARTESIAN_POINT('Ctrl Pts',(3.58446282799994,12.2,-1.90624734900001));
#350292=CARTESIAN_POINT('Ctrl Pts',(3.58446282799994,5.2,-1.90624734900001));
#350293=CARTESIAN_POINT('Ctrl Pts',(3.58446282799994,2.2,-1.90624734900001));
#350294=CARTESIAN_POINT('Ctrl Pts',(3.58533076099994,12.2,-1.90652289800001));
#350295=CARTESIAN_POINT('Ctrl Pts',(3.58533076099994,5.2,-1.90652289800001));
#350296=CARTESIAN_POINT('Ctrl Pts',(3.58533076099994,2.2,-1.90652289800001));
#350297=CARTESIAN_POINT('Ctrl Pts',(3.58620440499994,12.2,-1.90679906400002));
#350298=CARTESIAN_POINT('Ctrl Pts',(3.58620440499994,5.2,-1.90679906400002));
#350299=CARTESIAN_POINT('Ctrl Pts',(3.58620440499994,2.2,-1.90679906400002));
#350300=CARTESIAN_POINT('Ctrl Pts',(3.58708375299994,12.2,-1.90707583300001));
#350301=CARTESIAN_POINT('Ctrl Pts',(3.58708375299994,5.2,-1.90707583300001));
#350302=CARTESIAN_POINT('Ctrl Pts',(3.58708375299994,2.2,-1.90707583300001));
#350303=CARTESIAN_POINT('Ctrl Pts',(3.58796879799994,12.2,-1.90735318600002));
#350304=CARTESIAN_POINT('Ctrl Pts',(3.58796879799994,5.2,-1.90735318600002));
#350305=CARTESIAN_POINT('Ctrl Pts',(3.58796879799994,2.2,-1.90735318600002));
#350306=CARTESIAN_POINT('Ctrl Pts',(3.58885953399994,12.2,-1.90763110900001));
#350307=CARTESIAN_POINT('Ctrl Pts',(3.58885953399994,5.2,-1.90763110900001));
#350308=CARTESIAN_POINT('Ctrl Pts',(3.58885953399994,2.2,-1.90763110900001));
#350309=CARTESIAN_POINT('Ctrl Pts',(3.58975595399994,12.2,-1.90790958700001));
#350310=CARTESIAN_POINT('Ctrl Pts',(3.58975595399994,5.2,-1.90790958700001));
#350311=CARTESIAN_POINT('Ctrl Pts',(3.58975595399994,2.2,-1.90790958700001));
#350312=CARTESIAN_POINT('Ctrl Pts',(3.59065805099994,12.2,-1.90818860300002));
#350313=CARTESIAN_POINT('Ctrl Pts',(3.59065805099994,5.2,-1.90818860300002));
#350314=CARTESIAN_POINT('Ctrl Pts',(3.59065805099994,2.2,-1.90818860300002));
#350315=CARTESIAN_POINT('Ctrl Pts',(3.59156581999994,12.2,-1.90846814100002));
#350316=CARTESIAN_POINT('Ctrl Pts',(3.59156581999994,5.2,-1.90846814100002));
#350317=CARTESIAN_POINT('Ctrl Pts',(3.59156581999994,2.2,-1.90846814100002));
#350318=CARTESIAN_POINT('Ctrl Pts',(3.59247925199994,12.2,-1.90874818500001));
#350319=CARTESIAN_POINT('Ctrl Pts',(3.59247925199994,5.2,-1.90874818500001));
#350320=CARTESIAN_POINT('Ctrl Pts',(3.59247925199994,2.2,-1.90874818500001));
#350321=CARTESIAN_POINT('Ctrl Pts',(3.59339834299994,12.2,-1.90902872000001));
#350322=CARTESIAN_POINT('Ctrl Pts',(3.59339834299994,5.2,-1.90902872000001));
#350323=CARTESIAN_POINT('Ctrl Pts',(3.59339834299994,2.2,-1.90902872000001));
#350324=CARTESIAN_POINT('Ctrl Pts',(3.59432308499994,12.2,-1.90930973100001));
#350325=CARTESIAN_POINT('Ctrl Pts',(3.59432308499994,5.2,-1.90930973100001));
#350326=CARTESIAN_POINT('Ctrl Pts',(3.59432308499994,2.2,-1.90930973100001));
#350327=CARTESIAN_POINT('Ctrl Pts',(3.59525347199994,12.2,-1.90959120200001));
#350328=CARTESIAN_POINT('Ctrl Pts',(3.59525347199994,5.2,-1.90959120200001));
#350329=CARTESIAN_POINT('Ctrl Pts',(3.59525347199994,2.2,-1.90959120200001));
#350330=CARTESIAN_POINT('Ctrl Pts',(3.59618949499994,12.2,-1.90987311600002));
#350331=CARTESIAN_POINT('Ctrl Pts',(3.59618949499994,5.2,-1.90987311600002));
#350332=CARTESIAN_POINT('Ctrl Pts',(3.59618949499994,2.2,-1.90987311600002));
#350333=CARTESIAN_POINT('Ctrl Pts',(3.59713115099995,12.2,-1.91015545800001));
#350334=CARTESIAN_POINT('Ctrl Pts',(3.59713115099995,5.2,-1.91015545800001));
#350335=CARTESIAN_POINT('Ctrl Pts',(3.59713115099995,2.2,-1.91015545800001));
#350336=CARTESIAN_POINT('Ctrl Pts',(3.59807843099994,12.2,-1.91043821500001));
#350337=CARTESIAN_POINT('Ctrl Pts',(3.59807843099994,5.2,-1.91043821500001));
#350338=CARTESIAN_POINT('Ctrl Pts',(3.59807843099994,2.2,-1.91043821500001));
#350339=CARTESIAN_POINT('Ctrl Pts',(3.59903132999994,12.2,-1.91072136800001));
#350340=CARTESIAN_POINT('Ctrl Pts',(3.59903132999994,5.2,-1.91072136800001));
#350341=CARTESIAN_POINT('Ctrl Pts',(3.59903132999994,2.2,-1.91072136800001));
#350342=CARTESIAN_POINT('Ctrl Pts',(3.59998983999994,12.2,-1.91100490500002));
#350343=CARTESIAN_POINT('Ctrl Pts',(3.59998983999994,5.2,-1.91100490500002));
#350344=CARTESIAN_POINT('Ctrl Pts',(3.59998983999994,2.2,-1.91100490500002));
#350345=CARTESIAN_POINT('Ctrl Pts',(3.60095395499994,12.2,-1.91128880900001));
#350346=CARTESIAN_POINT('Ctrl Pts',(3.60095395499994,5.2,-1.91128880900001));
#350347=CARTESIAN_POINT('Ctrl Pts',(3.60095395499994,2.2,-1.91128880900001));
#350348=CARTESIAN_POINT('Ctrl Pts',(3.60192366899994,12.2,-1.91157306400001));
#350349=CARTESIAN_POINT('Ctrl Pts',(3.60192366899994,5.2,-1.91157306400001));
#350350=CARTESIAN_POINT('Ctrl Pts',(3.60192366899994,2.2,-1.91157306400001));
#350351=CARTESIAN_POINT('Ctrl Pts',(3.60289897299995,12.2,-1.91185765600002));
#350352=CARTESIAN_POINT('Ctrl Pts',(3.60289897299995,5.2,-1.91185765600002));
#350353=CARTESIAN_POINT('Ctrl Pts',(3.60289897299995,2.2,-1.91185765600002));
#350354=CARTESIAN_POINT('Ctrl Pts',(3.60387986299994,12.2,-1.91214256900002));
#350355=CARTESIAN_POINT('Ctrl Pts',(3.60387986299994,5.2,-1.91214256900002));
#350356=CARTESIAN_POINT('Ctrl Pts',(3.60387986299994,2.2,-1.91214256900002));
#350357=CARTESIAN_POINT('Ctrl Pts',(3.60486633099994,12.2,-1.91242778900001));
#350358=CARTESIAN_POINT('Ctrl Pts',(3.60486633099994,5.2,-1.91242778900001));
#350359=CARTESIAN_POINT('Ctrl Pts',(3.60486633099994,2.2,-1.91242778900001));
#350360=CARTESIAN_POINT('Ctrl Pts',(3.60585837199995,12.2,-1.91271330000002));
#350361=CARTESIAN_POINT('Ctrl Pts',(3.60585837199995,5.2,-1.91271330000002));
#350362=CARTESIAN_POINT('Ctrl Pts',(3.60585837199995,2.2,-1.91271330000002));
#350363=CARTESIAN_POINT('Ctrl Pts',(3.60685597699994,12.2,-1.91299908700001));
#350364=CARTESIAN_POINT('Ctrl Pts',(3.60685597699994,5.2,-1.91299908700001));
#350365=CARTESIAN_POINT('Ctrl Pts',(3.60685597699994,2.2,-1.91299908700001));
#350366=CARTESIAN_POINT('Ctrl Pts',(3.60785914099994,12.2,-1.91328513500002));
#350367=CARTESIAN_POINT('Ctrl Pts',(3.60785914099994,5.2,-1.91328513500002));
#350368=CARTESIAN_POINT('Ctrl Pts',(3.60785914099994,2.2,-1.91328513500002));
#350369=CARTESIAN_POINT('Ctrl Pts',(3.60886785599994,12.2,-1.91357143000001));
#350370=CARTESIAN_POINT('Ctrl Pts',(3.60886785599994,5.2,-1.91357143000001));
#350371=CARTESIAN_POINT('Ctrl Pts',(3.60886785599994,2.2,-1.91357143000001));
#350372=CARTESIAN_POINT('Ctrl Pts',(3.60988211699994,12.2,-1.91385795700001));
#350373=CARTESIAN_POINT('Ctrl Pts',(3.60988211699994,5.2,-1.91385795700001));
#350374=CARTESIAN_POINT('Ctrl Pts',(3.60988211699994,2.2,-1.91385795700001));
#350375=CARTESIAN_POINT('Ctrl Pts',(3.61090191699994,12.2,-1.91414470000002));
#350376=CARTESIAN_POINT('Ctrl Pts',(3.61090191699994,5.2,-1.91414470000002));
#350377=CARTESIAN_POINT('Ctrl Pts',(3.61090191699994,2.2,-1.91414470000002));
#350378=CARTESIAN_POINT('Ctrl Pts',(3.61192724899994,12.2,-1.91443164400001));
#350379=CARTESIAN_POINT('Ctrl Pts',(3.61192724899994,5.2,-1.91443164400001));
#350380=CARTESIAN_POINT('Ctrl Pts',(3.61192724899994,2.2,-1.91443164400001));
#350381=CARTESIAN_POINT('Ctrl Pts',(3.61295810599994,12.2,-1.91471877600002));
#350382=CARTESIAN_POINT('Ctrl Pts',(3.61295810599994,5.2,-1.91471877600002));
#350383=CARTESIAN_POINT('Ctrl Pts',(3.61295810599994,2.2,-1.91471877600002));
#350384=CARTESIAN_POINT('Ctrl Pts',(3.61399448099994,12.2,-1.91500608000001));
#350385=CARTESIAN_POINT('Ctrl Pts',(3.61399448099994,5.2,-1.91500608000001));
#350386=CARTESIAN_POINT('Ctrl Pts',(3.61399448099994,2.2,-1.91500608000001));
#350387=CARTESIAN_POINT('Ctrl Pts',(3.61503636899994,12.2,-1.91529354200001));
#350388=CARTESIAN_POINT('Ctrl Pts',(3.61503636899994,5.2,-1.91529354200001));
#350389=CARTESIAN_POINT('Ctrl Pts',(3.61503636899994,2.2,-1.91529354200001));
#350390=CARTESIAN_POINT('Ctrl Pts',(3.61608376199994,12.2,-1.91558114600001));
#350391=CARTESIAN_POINT('Ctrl Pts',(3.61608376199994,5.2,-1.91558114600001));
#350392=CARTESIAN_POINT('Ctrl Pts',(3.61608376199994,2.2,-1.91558114600001));
#350393=CARTESIAN_POINT('Ctrl Pts',(3.61713665199995,12.2,-1.91586887900002));
#350394=CARTESIAN_POINT('Ctrl Pts',(3.61713665199995,5.2,-1.91586887900002));
#350395=CARTESIAN_POINT('Ctrl Pts',(3.61713665199995,2.2,-1.91586887900002));
#350396=CARTESIAN_POINT('Ctrl Pts',(3.61819503599994,12.2,-1.91615672600001));
#350397=CARTESIAN_POINT('Ctrl Pts',(3.61819503599994,5.2,-1.91615672600001));
#350398=CARTESIAN_POINT('Ctrl Pts',(3.61819503599994,2.2,-1.91615672600001));
#350399=CARTESIAN_POINT('Ctrl Pts',(3.61925890499994,12.2,-1.91644467300002));
#350400=CARTESIAN_POINT('Ctrl Pts',(3.61925890499994,5.2,-1.91644467300002));
#350401=CARTESIAN_POINT('Ctrl Pts',(3.61925890499994,2.2,-1.91644467300002));
#350402=CARTESIAN_POINT('Ctrl Pts',(3.62032825299994,12.2,-1.91673270400001));
#350403=CARTESIAN_POINT('Ctrl Pts',(3.62032825299994,5.2,-1.91673270400001));
#350404=CARTESIAN_POINT('Ctrl Pts',(3.62032825299994,2.2,-1.91673270400001));
#350405=CARTESIAN_POINT('Ctrl Pts',(3.62140307199994,12.2,-1.91702080600002));
#350406=CARTESIAN_POINT('Ctrl Pts',(3.62140307199994,5.2,-1.91702080600002));
#350407=CARTESIAN_POINT('Ctrl Pts',(3.62140307199994,2.2,-1.91702080600002));
#350408=CARTESIAN_POINT('Ctrl Pts',(3.62248335699995,12.2,-1.91730896300002));
#350409=CARTESIAN_POINT('Ctrl Pts',(3.62248335699995,5.2,-1.91730896300002));
#350410=CARTESIAN_POINT('Ctrl Pts',(3.62248335699995,2.2,-1.91730896300002));
#350411=CARTESIAN_POINT('Ctrl Pts',(3.62356910199995,12.2,-1.91759716300002));
#350412=CARTESIAN_POINT('Ctrl Pts',(3.62356910199995,5.2,-1.91759716300002));
#350413=CARTESIAN_POINT('Ctrl Pts',(3.62356910199995,2.2,-1.91759716300002));
#350414=CARTESIAN_POINT('Ctrl Pts',(3.62466029599994,12.2,-1.91788539100001));
#350415=CARTESIAN_POINT('Ctrl Pts',(3.62466029599994,5.2,-1.91788539100001));
#350416=CARTESIAN_POINT('Ctrl Pts',(3.62466029599994,2.2,-1.91788539100001));
#350417=CARTESIAN_POINT('Ctrl Pts',(3.62575693799994,12.2,-1.91817363200002));
#350418=CARTESIAN_POINT('Ctrl Pts',(3.62575693799994,5.2,-1.91817363200002));
#350419=CARTESIAN_POINT('Ctrl Pts',(3.62575693799994,2.2,-1.91817363200002));
#350420=CARTESIAN_POINT('Ctrl Pts',(3.62685901799995,12.2,-1.91846187200001));
#350421=CARTESIAN_POINT('Ctrl Pts',(3.62685901799995,5.2,-1.91846187200001));
#350422=CARTESIAN_POINT('Ctrl Pts',(3.62685901799995,2.2,-1.91846187200001));
#350423=CARTESIAN_POINT('Ctrl Pts',(3.62796652899994,12.2,-1.91875009700002));
#350424=CARTESIAN_POINT('Ctrl Pts',(3.62796652899994,5.2,-1.91875009700002));
#350425=CARTESIAN_POINT('Ctrl Pts',(3.62796652899994,2.2,-1.91875009700002));
#350426=CARTESIAN_POINT('Ctrl Pts',(3.62907946699994,12.2,-1.91903829300001));
#350427=CARTESIAN_POINT('Ctrl Pts',(3.62907946699994,5.2,-1.91903829300001));
#350428=CARTESIAN_POINT('Ctrl Pts',(3.62907946699994,2.2,-1.91903829300001));
#350429=CARTESIAN_POINT('Ctrl Pts',(3.63019782199994,12.2,-1.91932644600001));
#350430=CARTESIAN_POINT('Ctrl Pts',(3.63019782199994,5.2,-1.91932644600001));
#350431=CARTESIAN_POINT('Ctrl Pts',(3.63019782199994,2.2,-1.91932644600001));
#350432=CARTESIAN_POINT('Ctrl Pts',(3.63132158899994,12.2,-1.91961454100001));
#350433=CARTESIAN_POINT('Ctrl Pts',(3.63132158899994,5.2,-1.91961454100001));
#350434=CARTESIAN_POINT('Ctrl Pts',(3.63132158899994,2.2,-1.91961454100001));
#350435=CARTESIAN_POINT('Ctrl Pts',(3.63245076099994,12.2,-1.91990256600001));
#350436=CARTESIAN_POINT('Ctrl Pts',(3.63245076099994,5.2,-1.91990256600001));
#350437=CARTESIAN_POINT('Ctrl Pts',(3.63245076099994,2.2,-1.91990256600001));
#350438=CARTESIAN_POINT('Ctrl Pts',(3.63358533199994,12.2,-1.92019050500001));
#350439=CARTESIAN_POINT('Ctrl Pts',(3.63358533199994,5.2,-1.92019050500001));
#350440=CARTESIAN_POINT('Ctrl Pts',(3.63358533199994,2.2,-1.92019050500001));
#350441=CARTESIAN_POINT('Ctrl Pts',(3.63472529599994,12.2,-1.92047834600002));
#350442=CARTESIAN_POINT('Ctrl Pts',(3.63472529599994,5.2,-1.92047834600002));
#350443=CARTESIAN_POINT('Ctrl Pts',(3.63472529599994,2.2,-1.92047834600002));
#350444=CARTESIAN_POINT('Ctrl Pts',(3.63587064399994,12.2,-1.92076607300002));
#350445=CARTESIAN_POINT('Ctrl Pts',(3.63587064399994,5.2,-1.92076607300002));
#350446=CARTESIAN_POINT('Ctrl Pts',(3.63587064399994,2.2,-1.92076607300002));
#350447=CARTESIAN_POINT('Ctrl Pts',(3.63702136999994,12.2,-1.92105367400002));
#350448=CARTESIAN_POINT('Ctrl Pts',(3.63702136999994,5.2,-1.92105367400002));
#350449=CARTESIAN_POINT('Ctrl Pts',(3.63702136999994,2.2,-1.92105367400002));
#350450=CARTESIAN_POINT('Ctrl Pts',(3.63817746799994,12.2,-1.92134113500002));
#350451=CARTESIAN_POINT('Ctrl Pts',(3.63817746799994,5.2,-1.92134113500002));
#350452=CARTESIAN_POINT('Ctrl Pts',(3.63817746799994,2.2,-1.92134113500002));
#350453=CARTESIAN_POINT('Ctrl Pts',(3.63933893199994,12.2,-1.92162844100002));
#350454=CARTESIAN_POINT('Ctrl Pts',(3.63933893199994,5.2,-1.92162844100002));
#350455=CARTESIAN_POINT('Ctrl Pts',(3.63933893199994,2.2,-1.92162844100002));
#350456=CARTESIAN_POINT('Ctrl Pts',(3.64050575399994,12.2,-1.92191557900002));
#350457=CARTESIAN_POINT('Ctrl Pts',(3.64050575399994,5.2,-1.92191557900002));
#350458=CARTESIAN_POINT('Ctrl Pts',(3.64050575399994,2.2,-1.92191557900002));
#350459=CARTESIAN_POINT('Ctrl Pts',(3.64167792599994,12.2,-1.92220253500002));
#350460=CARTESIAN_POINT('Ctrl Pts',(3.64167792599994,5.2,-1.92220253500002));
#350461=CARTESIAN_POINT('Ctrl Pts',(3.64167792599994,2.2,-1.92220253500002));
#350462=CARTESIAN_POINT('Ctrl Pts',(3.64285544499994,12.2,-1.92248929700002));
#350463=CARTESIAN_POINT('Ctrl Pts',(3.64285544499994,5.2,-1.92248929700002));
#350464=CARTESIAN_POINT('Ctrl Pts',(3.64285544499994,2.2,-1.92248929700002));
#350465=CARTESIAN_POINT('Ctrl Pts',(3.64403829999994,12.2,-1.92277585000001));
#350466=CARTESIAN_POINT('Ctrl Pts',(3.64403829999994,5.2,-1.92277585000001));
#350467=CARTESIAN_POINT('Ctrl Pts',(3.64403829999994,2.2,-1.92277585000001));
#350468=CARTESIAN_POINT('Ctrl Pts',(3.64522648799994,12.2,-1.92306218100001));
#350469=CARTESIAN_POINT('Ctrl Pts',(3.64522648799994,5.2,-1.92306218100001));
#350470=CARTESIAN_POINT('Ctrl Pts',(3.64522648799994,2.2,-1.92306218100001));
#350471=CARTESIAN_POINT('Ctrl Pts',(3.64641999999994,12.2,-1.92334827500002));
#350472=CARTESIAN_POINT('Ctrl Pts',(3.64641999999994,5.2,-1.92334827500002));
#350473=CARTESIAN_POINT('Ctrl Pts',(3.64641999999994,2.2,-1.92334827500002));
#350474=CARTESIAN_POINT('Ctrl Pts',(3.64761883099994,12.2,-1.92363412100002));
#350475=CARTESIAN_POINT('Ctrl Pts',(3.64761883099994,5.2,-1.92363412100002));
#350476=CARTESIAN_POINT('Ctrl Pts',(3.64761883099994,2.2,-1.92363412100002));
#350477=CARTESIAN_POINT('Ctrl Pts',(3.64882297099994,12.2,-1.92391970400001));
#350478=CARTESIAN_POINT('Ctrl Pts',(3.64882297099994,5.2,-1.92391970400001));
#350479=CARTESIAN_POINT('Ctrl Pts',(3.64882297099994,2.2,-1.92391970400001));
#350480=CARTESIAN_POINT('Ctrl Pts',(3.65003241699994,12.2,-1.92420501000001));
#350481=CARTESIAN_POINT('Ctrl Pts',(3.65003241699994,5.2,-1.92420501000001));
#350482=CARTESIAN_POINT('Ctrl Pts',(3.65003241699994,2.2,-1.92420501000001));
#350483=CARTESIAN_POINT('Ctrl Pts',(3.65124716099994,12.2,-1.92449002800001));
#350484=CARTESIAN_POINT('Ctrl Pts',(3.65124716099994,5.2,-1.92449002800001));
#350485=CARTESIAN_POINT('Ctrl Pts',(3.65124716099994,2.2,-1.92449002800001));
#350486=CARTESIAN_POINT('Ctrl Pts',(3.65246719699994,12.2,-1.92477474300001));
#350487=CARTESIAN_POINT('Ctrl Pts',(3.65246719699994,5.2,-1.92477474300001));
#350488=CARTESIAN_POINT('Ctrl Pts',(3.65246719699994,2.2,-1.92477474300001));
#350489=CARTESIAN_POINT('Ctrl Pts',(3.65369251599994,12.2,-1.92505914200002));
#350490=CARTESIAN_POINT('Ctrl Pts',(3.65369251599994,5.2,-1.92505914200002));
#350491=CARTESIAN_POINT('Ctrl Pts',(3.65369251599994,2.2,-1.92505914200002));
#350492=CARTESIAN_POINT('Ctrl Pts',(3.65492311299994,12.2,-1.92534321200001));
#350493=CARTESIAN_POINT('Ctrl Pts',(3.65492311299994,5.2,-1.92534321200001));
#350494=CARTESIAN_POINT('Ctrl Pts',(3.65492311299994,2.2,-1.92534321200001));
#350495=CARTESIAN_POINT('Ctrl Pts',(3.65615898099994,12.2,-1.92562693900001));
#350496=CARTESIAN_POINT('Ctrl Pts',(3.65615898099994,5.2,-1.92562693900001));
#350497=CARTESIAN_POINT('Ctrl Pts',(3.65615898099994,2.2,-1.92562693900001));
#350498=CARTESIAN_POINT('Ctrl Pts',(3.65740011199994,12.2,-1.92591031100001));
#350499=CARTESIAN_POINT('Ctrl Pts',(3.65740011199994,5.2,-1.92591031100001));
#350500=CARTESIAN_POINT('Ctrl Pts',(3.65740011199994,2.2,-1.92591031100001));
#350501=CARTESIAN_POINT('Ctrl Pts',(3.65864650099994,12.2,-1.92619331400001));
#350502=CARTESIAN_POINT('Ctrl Pts',(3.65864650099994,5.2,-1.92619331400001));
#350503=CARTESIAN_POINT('Ctrl Pts',(3.65864650099994,2.2,-1.92619331400001));
#350504=CARTESIAN_POINT('Ctrl Pts',(3.65989814199994,12.2,-1.92647593600002));
#350505=CARTESIAN_POINT('Ctrl Pts',(3.65989814199994,5.2,-1.92647593600002));
#350506=CARTESIAN_POINT('Ctrl Pts',(3.65989814199994,2.2,-1.92647593600002));
#350507=CARTESIAN_POINT('Ctrl Pts',(3.66115502599994,12.2,-1.92675816300001));
#350508=CARTESIAN_POINT('Ctrl Pts',(3.66115502599994,5.2,-1.92675816300001));
#350509=CARTESIAN_POINT('Ctrl Pts',(3.66115502599994,2.2,-1.92675816300001));
#350510=CARTESIAN_POINT('Ctrl Pts',(3.66241714699994,12.2,-1.92703998200002));
#350511=CARTESIAN_POINT('Ctrl Pts',(3.66241714699994,5.2,-1.92703998200002));
#350512=CARTESIAN_POINT('Ctrl Pts',(3.66241714699994,2.2,-1.92703998200002));
#350513=CARTESIAN_POINT('Ctrl Pts',(3.66368449699995,12.2,-1.92732138100002));
#350514=CARTESIAN_POINT('Ctrl Pts',(3.66368449699995,5.2,-1.92732138100002));
#350515=CARTESIAN_POINT('Ctrl Pts',(3.66368449699995,2.2,-1.92732138100002));
#350516=CARTESIAN_POINT('Ctrl Pts',(3.66495707299994,12.2,-1.92760234600001));
#350517=CARTESIAN_POINT('Ctrl Pts',(3.66495707299994,5.2,-1.92760234600001));
#350518=CARTESIAN_POINT('Ctrl Pts',(3.66495707299994,2.2,-1.92760234600001));
#350519=CARTESIAN_POINT('Ctrl Pts',(3.66623486499994,12.2,-1.92788286500001));
#350520=CARTESIAN_POINT('Ctrl Pts',(3.66623486499994,5.2,-1.92788286500001));
#350521=CARTESIAN_POINT('Ctrl Pts',(3.66623486499994,2.2,-1.92788286500001));
#350522=CARTESIAN_POINT('Ctrl Pts',(3.66751786599994,12.2,-1.92816292400002));
#350523=CARTESIAN_POINT('Ctrl Pts',(3.66751786599994,5.2,-1.92816292400002));
#350524=CARTESIAN_POINT('Ctrl Pts',(3.66751786599994,2.2,-1.92816292400002));
#350525=CARTESIAN_POINT('Ctrl Pts',(3.66880607199994,12.2,-1.92844251200002));
#350526=CARTESIAN_POINT('Ctrl Pts',(3.66880607199994,5.2,-1.92844251200002));
#350527=CARTESIAN_POINT('Ctrl Pts',(3.66880607199994,2.2,-1.92844251200002));
#350528=CARTESIAN_POINT('Ctrl Pts',(3.67009947399994,12.2,-1.92872161400001));
#350529=CARTESIAN_POINT('Ctrl Pts',(3.67009947399994,5.2,-1.92872161400001));
#350530=CARTESIAN_POINT('Ctrl Pts',(3.67009947399994,2.2,-1.92872161400001));
#350531=CARTESIAN_POINT('Ctrl Pts',(3.67139806599994,12.2,-1.92900021900002));
#350532=CARTESIAN_POINT('Ctrl Pts',(3.67139806599994,5.2,-1.92900021900002));
#350533=CARTESIAN_POINT('Ctrl Pts',(3.67139806599994,2.2,-1.92900021900002));
#350534=CARTESIAN_POINT('Ctrl Pts',(3.67270184099994,12.2,-1.92927831300001));
#350535=CARTESIAN_POINT('Ctrl Pts',(3.67270184099994,5.2,-1.92927831300001));
#350536=CARTESIAN_POINT('Ctrl Pts',(3.67270184099994,2.2,-1.92927831300001));
#350537=CARTESIAN_POINT('Ctrl Pts',(3.67401079199994,12.2,-1.92955588400002));
#350538=CARTESIAN_POINT('Ctrl Pts',(3.67401079199994,5.2,-1.92955588400002));
#350539=CARTESIAN_POINT('Ctrl Pts',(3.67401079199994,2.2,-1.92955588400002));
#350540=CARTESIAN_POINT('Ctrl Pts',(3.67532491199994,12.2,-1.92983292100001));
#350541=CARTESIAN_POINT('Ctrl Pts',(3.67532491199994,5.2,-1.92983292100001));
#350542=CARTESIAN_POINT('Ctrl Pts',(3.67532491199994,2.2,-1.92983292100001));
#350543=CARTESIAN_POINT('Ctrl Pts',(3.67664419599994,12.2,-1.93010940900002));
#350544=CARTESIAN_POINT('Ctrl Pts',(3.67664419599994,5.2,-1.93010940900002));
#350545=CARTESIAN_POINT('Ctrl Pts',(3.67664419599994,2.2,-1.93010940900002));
#350546=CARTESIAN_POINT('Ctrl Pts',(3.67796863599994,12.2,-1.93038533600001));
#350547=CARTESIAN_POINT('Ctrl Pts',(3.67796863599994,5.2,-1.93038533600001));
#350548=CARTESIAN_POINT('Ctrl Pts',(3.67796863599994,2.2,-1.93038533600001));
#350549=CARTESIAN_POINT('Ctrl Pts',(3.67929822499994,12.2,-1.93066069000002));
#350550=CARTESIAN_POINT('Ctrl Pts',(3.67929822499994,5.2,-1.93066069000002));
#350551=CARTESIAN_POINT('Ctrl Pts',(3.67929822499994,2.2,-1.93066069000002));
#350552=CARTESIAN_POINT('Ctrl Pts',(3.68063295599994,12.2,-1.93093545700001));
#350553=CARTESIAN_POINT('Ctrl Pts',(3.68063295599994,5.2,-1.93093545700001));
#350554=CARTESIAN_POINT('Ctrl Pts',(3.68063295599994,2.2,-1.93093545700001));
#350555=CARTESIAN_POINT('Ctrl Pts',(3.68197282299994,12.2,-1.93120962700001));
#350556=CARTESIAN_POINT('Ctrl Pts',(3.68197282299994,5.2,-1.93120962700001));
#350557=CARTESIAN_POINT('Ctrl Pts',(3.68197282299994,2.2,-1.93120962700001));
#350558=CARTESIAN_POINT('Ctrl Pts',(3.68331781899994,12.2,-1.93148318700001));
#350559=CARTESIAN_POINT('Ctrl Pts',(3.68331781899994,5.2,-1.93148318700001));
#350560=CARTESIAN_POINT('Ctrl Pts',(3.68331781899994,2.2,-1.93148318700001));
#350561=CARTESIAN_POINT('Ctrl Pts',(3.68466793599994,12.2,-1.93175612300001));
#350562=CARTESIAN_POINT('Ctrl Pts',(3.68466793599994,5.2,-1.93175612300001));
#350563=CARTESIAN_POINT('Ctrl Pts',(3.68466793599994,2.2,-1.93175612300001));
#350564=CARTESIAN_POINT('Ctrl Pts',(3.68602316999994,12.2,-1.93202842500002));
#350565=CARTESIAN_POINT('Ctrl Pts',(3.68602316999994,5.2,-1.93202842500002));
#350566=CARTESIAN_POINT('Ctrl Pts',(3.68602316999994,2.2,-1.93202842500002));
#350567=CARTESIAN_POINT('Ctrl Pts',(3.68738351099994,12.2,-1.93230007800001));
#350568=CARTESIAN_POINT('Ctrl Pts',(3.68738351099994,5.2,-1.93230007800001));
#350569=CARTESIAN_POINT('Ctrl Pts',(3.68738351099994,2.2,-1.93230007800001));
#350570=CARTESIAN_POINT('Ctrl Pts',(3.68874895499994,12.2,-1.93257107200001));
#350571=CARTESIAN_POINT('Ctrl Pts',(3.68874895499994,5.2,-1.93257107200001));
#350572=CARTESIAN_POINT('Ctrl Pts',(3.68874895499994,2.2,-1.93257107200001));
#350573=CARTESIAN_POINT('Ctrl Pts',(3.69011949399995,12.2,-1.93284139300001));
#350574=CARTESIAN_POINT('Ctrl Pts',(3.69011949399995,5.2,-1.93284139300001));
#350575=CARTESIAN_POINT('Ctrl Pts',(3.69011949399995,2.2,-1.93284139300001));
#350576=CARTESIAN_POINT('Ctrl Pts',(3.69149512099994,12.2,-1.93311103000001));
#350577=CARTESIAN_POINT('Ctrl Pts',(3.69149512099994,5.2,-1.93311103000001));
#350578=CARTESIAN_POINT('Ctrl Pts',(3.69149512099994,2.2,-1.93311103000001));
#350579=CARTESIAN_POINT('Ctrl Pts',(3.69287582899994,12.2,-1.93337997100001));
#350580=CARTESIAN_POINT('Ctrl Pts',(3.69287582899994,5.2,-1.93337997100001));
#350581=CARTESIAN_POINT('Ctrl Pts',(3.69287582899994,2.2,-1.93337997100001));
#350582=CARTESIAN_POINT('Ctrl Pts',(3.69426161099994,12.2,-1.93364820300001));
#350583=CARTESIAN_POINT('Ctrl Pts',(3.69426161099994,5.2,-1.93364820300001));
#350584=CARTESIAN_POINT('Ctrl Pts',(3.69426161099994,2.2,-1.93364820300001));
#350585=CARTESIAN_POINT('Ctrl Pts',(3.69565246199994,12.2,-1.93391571500001));
#350586=CARTESIAN_POINT('Ctrl Pts',(3.69565246199994,5.2,-1.93391571500001));
#350587=CARTESIAN_POINT('Ctrl Pts',(3.69565246199994,2.2,-1.93391571500001));
#350588=CARTESIAN_POINT('Ctrl Pts',(3.69704837299994,12.2,-1.93418249400001));
#350589=CARTESIAN_POINT('Ctrl Pts',(3.69704837299994,5.2,-1.93418249400001));
#350590=CARTESIAN_POINT('Ctrl Pts',(3.69704837299994,2.2,-1.93418249400001));
#350591=CARTESIAN_POINT('Ctrl Pts',(3.69844933899994,12.2,-1.93444852900001));
#350592=CARTESIAN_POINT('Ctrl Pts',(3.69844933899994,5.2,-1.93444852900001));
#350593=CARTESIAN_POINT('Ctrl Pts',(3.69844933899994,2.2,-1.93444852900001));
#350594=CARTESIAN_POINT('Ctrl Pts',(3.69985535199994,12.2,-1.93471380500001));
#350595=CARTESIAN_POINT('Ctrl Pts',(3.69985535199994,5.2,-1.93471380500001));
#350596=CARTESIAN_POINT('Ctrl Pts',(3.69985535199994,2.2,-1.93471380500001));
#350597=CARTESIAN_POINT('Ctrl Pts',(3.70126640599994,12.2,-1.93497831400002));
#350598=CARTESIAN_POINT('Ctrl Pts',(3.70126640599994,5.2,-1.93497831400002));
#350599=CARTESIAN_POINT('Ctrl Pts',(3.70126640599994,2.2,-1.93497831400002));
#350600=CARTESIAN_POINT('Ctrl Pts',(3.70268249299994,12.2,-1.93524204200001));
#350601=CARTESIAN_POINT('Ctrl Pts',(3.70268249299994,5.2,-1.93524204200001));
#350602=CARTESIAN_POINT('Ctrl Pts',(3.70268249299994,2.2,-1.93524204200001));
#350603=CARTESIAN_POINT('Ctrl Pts',(3.70410360799994,12.2,-1.93550497700001));
#350604=CARTESIAN_POINT('Ctrl Pts',(3.70410360799994,5.2,-1.93550497700001));
#350605=CARTESIAN_POINT('Ctrl Pts',(3.70410360799994,2.2,-1.93550497700001));
#350606=CARTESIAN_POINT('Ctrl Pts',(3.70552974199994,12.2,-1.93576710800002));
#350607=CARTESIAN_POINT('Ctrl Pts',(3.70552974199994,5.2,-1.93576710800002));
#350608=CARTESIAN_POINT('Ctrl Pts',(3.70552974199994,2.2,-1.93576710800002));
#350609=CARTESIAN_POINT('Ctrl Pts',(3.70696088999994,12.2,-1.93602842300002));
#350610=CARTESIAN_POINT('Ctrl Pts',(3.70696088999994,5.2,-1.93602842300002));
#350611=CARTESIAN_POINT('Ctrl Pts',(3.70696088999994,2.2,-1.93602842300002));
#350612=CARTESIAN_POINT('Ctrl Pts',(3.70839704399994,12.2,-1.93628891000001));
#350613=CARTESIAN_POINT('Ctrl Pts',(3.70839704399994,5.2,-1.93628891000001));
#350614=CARTESIAN_POINT('Ctrl Pts',(3.70839704399994,2.2,-1.93628891000001));
#350615=CARTESIAN_POINT('Ctrl Pts',(3.70983819799994,12.2,-1.93654855800002));
#350616=CARTESIAN_POINT('Ctrl Pts',(3.70983819799994,5.2,-1.93654855800002));
#350617=CARTESIAN_POINT('Ctrl Pts',(3.70983819799994,2.2,-1.93654855800002));
#350618=CARTESIAN_POINT('Ctrl Pts',(3.71128434599994,12.2,-1.93680735200001));
#350619=CARTESIAN_POINT('Ctrl Pts',(3.71128434599994,5.2,-1.93680735200001));
#350620=CARTESIAN_POINT('Ctrl Pts',(3.71128434599994,2.2,-1.93680735200001));
#350621=CARTESIAN_POINT('Ctrl Pts',(3.71273547899994,12.2,-1.93706528500002));
#350622=CARTESIAN_POINT('Ctrl Pts',(3.71273547899994,5.2,-1.93706528500002));
#350623=CARTESIAN_POINT('Ctrl Pts',(3.71273547899994,2.2,-1.93706528500002));
#350624=CARTESIAN_POINT('Ctrl Pts',(3.71419159099994,12.2,-1.93732234200001));
#350625=CARTESIAN_POINT('Ctrl Pts',(3.71419159099994,5.2,-1.93732234200001));
#350626=CARTESIAN_POINT('Ctrl Pts',(3.71419159099994,2.2,-1.93732234200001));
#350627=CARTESIAN_POINT('Ctrl Pts',(3.71565267599994,12.2,-1.93757851400001));
#350628=CARTESIAN_POINT('Ctrl Pts',(3.71565267599994,5.2,-1.93757851400001));
#350629=CARTESIAN_POINT('Ctrl Pts',(3.71565267599994,2.2,-1.93757851400001));
#350630=CARTESIAN_POINT('Ctrl Pts',(3.71711872599994,12.2,-1.93783378700001));
#350631=CARTESIAN_POINT('Ctrl Pts',(3.71711872599994,5.2,-1.93783378700001));
#350632=CARTESIAN_POINT('Ctrl Pts',(3.71711872599994,2.2,-1.93783378700001));
#350633=CARTESIAN_POINT('Ctrl Pts',(3.71858973499994,12.2,-1.93808815000001));
#350634=CARTESIAN_POINT('Ctrl Pts',(3.71858973499994,5.2,-1.93808815000001));
#350635=CARTESIAN_POINT('Ctrl Pts',(3.71858973499994,2.2,-1.93808815000001));
#350636=CARTESIAN_POINT('Ctrl Pts',(3.72006569699994,12.2,-1.93834159200001));
#350637=CARTESIAN_POINT('Ctrl Pts',(3.72006569699994,5.2,-1.93834159200001));
#350638=CARTESIAN_POINT('Ctrl Pts',(3.72006569699994,2.2,-1.93834159200001));
#350639=CARTESIAN_POINT('Ctrl Pts',(3.72154660299994,12.2,-1.93859410200002));
#350640=CARTESIAN_POINT('Ctrl Pts',(3.72154660299994,5.2,-1.93859410200002));
#350641=CARTESIAN_POINT('Ctrl Pts',(3.72154660299994,2.2,-1.93859410200002));
#350642=CARTESIAN_POINT('Ctrl Pts',(3.72303244799994,12.2,-1.93884566800001));
#350643=CARTESIAN_POINT('Ctrl Pts',(3.72303244799994,5.2,-1.93884566800001));
#350644=CARTESIAN_POINT('Ctrl Pts',(3.72303244799994,2.2,-1.93884566800001));
#350645=CARTESIAN_POINT('Ctrl Pts',(3.72452322399994,12.2,-1.93909627800001));
#350646=CARTESIAN_POINT('Ctrl Pts',(3.72452322399994,5.2,-1.93909627800001));
#350647=CARTESIAN_POINT('Ctrl Pts',(3.72452322399994,2.2,-1.93909627800001));
#350648=CARTESIAN_POINT('Ctrl Pts',(3.72601892499994,12.2,-1.93934592100002));
#350649=CARTESIAN_POINT('Ctrl Pts',(3.72601892499994,5.2,-1.93934592100002));
#350650=CARTESIAN_POINT('Ctrl Pts',(3.72601892499994,2.2,-1.93934592100002));
#350651=CARTESIAN_POINT('Ctrl Pts',(3.72751954399994,12.2,-1.93959458600002));
#350652=CARTESIAN_POINT('Ctrl Pts',(3.72751954399994,5.2,-1.93959458600002));
#350653=CARTESIAN_POINT('Ctrl Pts',(3.72751954399994,2.2,-1.93959458600002));
#350654=CARTESIAN_POINT('Ctrl Pts',(3.72902507299994,12.2,-1.93984226100001));
#350655=CARTESIAN_POINT('Ctrl Pts',(3.72902507299994,5.2,-1.93984226100001));
#350656=CARTESIAN_POINT('Ctrl Pts',(3.72902507299994,2.2,-1.93984226100001));
#350657=CARTESIAN_POINT('Ctrl Pts',(3.73053550699994,12.2,-1.94008893500001));
#350658=CARTESIAN_POINT('Ctrl Pts',(3.73053550699994,5.2,-1.94008893500001));
#350659=CARTESIAN_POINT('Ctrl Pts',(3.73053550699994,2.2,-1.94008893500001));
#350660=CARTESIAN_POINT('Ctrl Pts',(3.73205083799994,12.2,-1.94033459700002));
#350661=CARTESIAN_POINT('Ctrl Pts',(3.73205083799994,5.2,-1.94033459700002));
#350662=CARTESIAN_POINT('Ctrl Pts',(3.73205083799994,2.2,-1.94033459700002));
#350663=CARTESIAN_POINT('Ctrl Pts',(3.73357105999994,12.2,-1.94057923600001));
#350664=CARTESIAN_POINT('Ctrl Pts',(3.73357105999994,5.2,-1.94057923600001));
#350665=CARTESIAN_POINT('Ctrl Pts',(3.73357105999994,2.2,-1.94057923600001));
#350666=CARTESIAN_POINT('Ctrl Pts',(3.73509616599994,12.2,-1.94082284000002));
#350667=CARTESIAN_POINT('Ctrl Pts',(3.73509616599994,5.2,-1.94082284000002));
#350668=CARTESIAN_POINT('Ctrl Pts',(3.73509616599994,2.2,-1.94082284000002));
#350669=CARTESIAN_POINT('Ctrl Pts',(3.73662614799994,12.2,-1.94106539800002));
#350670=CARTESIAN_POINT('Ctrl Pts',(3.73662614799994,5.2,-1.94106539800002));
#350671=CARTESIAN_POINT('Ctrl Pts',(3.73662614799994,2.2,-1.94106539800002));
#350672=CARTESIAN_POINT('Ctrl Pts',(3.73816099999994,12.2,-1.94130689900001));
#350673=CARTESIAN_POINT('Ctrl Pts',(3.73816099999994,5.2,-1.94130689900001));
#350674=CARTESIAN_POINT('Ctrl Pts',(3.73816099999994,2.2,-1.94130689900001));
#350675=CARTESIAN_POINT('Ctrl Pts',(3.73970071499994,12.2,-1.94154733200001));
#350676=CARTESIAN_POINT('Ctrl Pts',(3.73970071499994,5.2,-1.94154733200001));
#350677=CARTESIAN_POINT('Ctrl Pts',(3.73970071499994,2.2,-1.94154733200001));
#350678=CARTESIAN_POINT('Ctrl Pts',(3.74124528699994,12.2,-1.94178668600001));
#350679=CARTESIAN_POINT('Ctrl Pts',(3.74124528699994,5.2,-1.94178668600001));
#350680=CARTESIAN_POINT('Ctrl Pts',(3.74124528699994,2.2,-1.94178668600001));
#350681=CARTESIAN_POINT('Ctrl Pts',(3.74279470799994,12.2,-1.94202495000001));
#350682=CARTESIAN_POINT('Ctrl Pts',(3.74279470799994,5.2,-1.94202495000001));
#350683=CARTESIAN_POINT('Ctrl Pts',(3.74279470799994,2.2,-1.94202495000001));
#350684=CARTESIAN_POINT('Ctrl Pts',(3.74434896999994,12.2,-1.94226211300002));
#350685=CARTESIAN_POINT('Ctrl Pts',(3.74434896999994,5.2,-1.94226211300002));
#350686=CARTESIAN_POINT('Ctrl Pts',(3.74434896999994,2.2,-1.94226211300002));
#350687=CARTESIAN_POINT('Ctrl Pts',(3.74590806999994,12.2,-1.94249816300001));
#350688=CARTESIAN_POINT('Ctrl Pts',(3.74590806999994,5.2,-1.94249816300001));
#350689=CARTESIAN_POINT('Ctrl Pts',(3.74590806999994,2.2,-1.94249816300001));
#350690=CARTESIAN_POINT('Ctrl Pts',(3.74747199799994,12.2,-1.94273309000002));
#350691=CARTESIAN_POINT('Ctrl Pts',(3.74747199799994,5.2,-1.94273309000002));
#350692=CARTESIAN_POINT('Ctrl Pts',(3.74747199799994,2.2,-1.94273309000002));
#350693=CARTESIAN_POINT('Ctrl Pts',(3.74904074799994,12.2,-1.94296688300001));
#350694=CARTESIAN_POINT('Ctrl Pts',(3.74904074799994,5.2,-1.94296688300001));
#350695=CARTESIAN_POINT('Ctrl Pts',(3.74904074799994,2.2,-1.94296688300001));
#350696=CARTESIAN_POINT('Ctrl Pts',(3.75061431399994,12.2,-1.94319953000001));
#350697=CARTESIAN_POINT('Ctrl Pts',(3.75061431399994,5.2,-1.94319953000001));
#350698=CARTESIAN_POINT('Ctrl Pts',(3.75061431399994,2.2,-1.94319953000001));
#350699=CARTESIAN_POINT('Ctrl Pts',(3.75219268599994,12.2,-1.94343102300001));
#350700=CARTESIAN_POINT('Ctrl Pts',(3.75219268599994,5.2,-1.94343102300001));
#350701=CARTESIAN_POINT('Ctrl Pts',(3.75219268599994,2.2,-1.94343102300001));
#350702=CARTESIAN_POINT('Ctrl Pts',(3.75377586099995,12.2,-1.94366134800001));
#350703=CARTESIAN_POINT('Ctrl Pts',(3.75377586099995,5.2,-1.94366134800001));
#350704=CARTESIAN_POINT('Ctrl Pts',(3.75377586099995,2.2,-1.94366134800001));
#350705=CARTESIAN_POINT('Ctrl Pts',(3.75536383099994,12.2,-1.94389049600002));
#350706=CARTESIAN_POINT('Ctrl Pts',(3.75536383099994,5.2,-1.94389049600002));
#350707=CARTESIAN_POINT('Ctrl Pts',(3.75536383099994,2.2,-1.94389049600002));
#350708=CARTESIAN_POINT('Ctrl Pts',(3.75695658799994,12.2,-1.94411845500001));
#350709=CARTESIAN_POINT('Ctrl Pts',(3.75695658799994,5.2,-1.94411845500001));
#350710=CARTESIAN_POINT('Ctrl Pts',(3.75695658799994,2.2,-1.94411845500001));
#350711=CARTESIAN_POINT('Ctrl Pts',(3.75855412599994,12.2,-1.94434521600002));
#350712=CARTESIAN_POINT('Ctrl Pts',(3.75855412599994,5.2,-1.94434521600002));
#350713=CARTESIAN_POINT('Ctrl Pts',(3.75855412599994,2.2,-1.94434521600002));
#350714=CARTESIAN_POINT('Ctrl Pts',(3.76015643799994,12.2,-1.94457076600001));
#350715=CARTESIAN_POINT('Ctrl Pts',(3.76015643799994,5.2,-1.94457076600001));
#350716=CARTESIAN_POINT('Ctrl Pts',(3.76015643799994,2.2,-1.94457076600001));
#350717=CARTESIAN_POINT('Ctrl Pts',(3.76176351799994,12.2,-1.94479509600002));
#350718=CARTESIAN_POINT('Ctrl Pts',(3.76176351799994,5.2,-1.94479509600002));
#350719=CARTESIAN_POINT('Ctrl Pts',(3.76176351799994,2.2,-1.94479509600002));
#350720=CARTESIAN_POINT('Ctrl Pts',(3.76337535699994,12.2,-1.94501819400001));
#350721=CARTESIAN_POINT('Ctrl Pts',(3.76337535699994,5.2,-1.94501819400001));
#350722=CARTESIAN_POINT('Ctrl Pts',(3.76337535699994,2.2,-1.94501819400001));
#350723=CARTESIAN_POINT('Ctrl Pts',(3.76499194999994,12.2,-1.94524005200002));
#350724=CARTESIAN_POINT('Ctrl Pts',(3.76499194999994,5.2,-1.94524005200002));
#350725=CARTESIAN_POINT('Ctrl Pts',(3.76499194999994,2.2,-1.94524005200002));
#350726=CARTESIAN_POINT('Ctrl Pts',(3.76661328999994,12.2,-1.94546065700001));
#350727=CARTESIAN_POINT('Ctrl Pts',(3.76661328999994,5.2,-1.94546065700001));
#350728=CARTESIAN_POINT('Ctrl Pts',(3.76661328999994,2.2,-1.94546065700001));
#350729=CARTESIAN_POINT('Ctrl Pts',(3.76823936799994,12.2,-1.94567999800002));
#350730=CARTESIAN_POINT('Ctrl Pts',(3.76823936799994,5.2,-1.94567999800002));
#350731=CARTESIAN_POINT('Ctrl Pts',(3.76823936799994,2.2,-1.94567999800002));
#350732=CARTESIAN_POINT('Ctrl Pts',(3.76987017999994,12.2,-1.94589806700002));
#350733=CARTESIAN_POINT('Ctrl Pts',(3.76987017999994,5.2,-1.94589806700002));
#350734=CARTESIAN_POINT('Ctrl Pts',(3.76987017999994,2.2,-1.94589806700002));
#350735=CARTESIAN_POINT('Ctrl Pts',(3.77150571799994,12.2,-1.94611485100001));
#350736=CARTESIAN_POINT('Ctrl Pts',(3.77150571799994,5.2,-1.94611485100001));
#350737=CARTESIAN_POINT('Ctrl Pts',(3.77150571799994,2.2,-1.94611485100001));
#350738=CARTESIAN_POINT('Ctrl Pts',(3.77314597499994,12.2,-1.94633034000002));
#350739=CARTESIAN_POINT('Ctrl Pts',(3.77314597499994,5.2,-1.94633034000002));
#350740=CARTESIAN_POINT('Ctrl Pts',(3.77314597499994,2.2,-1.94633034000002));
#350741=CARTESIAN_POINT('Ctrl Pts',(3.77479094399995,12.2,-1.94654452600002));
#350742=CARTESIAN_POINT('Ctrl Pts',(3.77479094399995,5.2,-1.94654452600002));
#350743=CARTESIAN_POINT('Ctrl Pts',(3.77479094399995,2.2,-1.94654452600002));
#350744=CARTESIAN_POINT('Ctrl Pts',(3.77644061799994,12.2,-1.94675739500001));
#350745=CARTESIAN_POINT('Ctrl Pts',(3.77644061799994,5.2,-1.94675739500001));
#350746=CARTESIAN_POINT('Ctrl Pts',(3.77644061799994,2.2,-1.94675739500001));
#350747=CARTESIAN_POINT('Ctrl Pts',(3.77809499099994,12.2,-1.94696893800002));
#350748=CARTESIAN_POINT('Ctrl Pts',(3.77809499099994,5.2,-1.94696893800002));
#350749=CARTESIAN_POINT('Ctrl Pts',(3.77809499099994,2.2,-1.94696893800002));
#350750=CARTESIAN_POINT('Ctrl Pts',(3.77975405499994,12.2,-1.94717914600002));
#350751=CARTESIAN_POINT('Ctrl Pts',(3.77975405499994,5.2,-1.94717914600002));
#350752=CARTESIAN_POINT('Ctrl Pts',(3.77975405499994,2.2,-1.94717914600002));
#350753=CARTESIAN_POINT('Ctrl Pts',(3.78141780399994,12.2,-1.94738800700001));
#350754=CARTESIAN_POINT('Ctrl Pts',(3.78141780399994,5.2,-1.94738800700001));
#350755=CARTESIAN_POINT('Ctrl Pts',(3.78141780399994,2.2,-1.94738800700001));
#350756=CARTESIAN_POINT('Ctrl Pts',(3.78308623099994,12.2,-1.94759551100002));
#350757=CARTESIAN_POINT('Ctrl Pts',(3.78308623099994,5.2,-1.94759551100002));
#350758=CARTESIAN_POINT('Ctrl Pts',(3.78308623099994,2.2,-1.94759551100002));
#350759=CARTESIAN_POINT('Ctrl Pts',(3.78475932799994,12.2,-1.94780164800001));
#350760=CARTESIAN_POINT('Ctrl Pts',(3.78475932799994,5.2,-1.94780164800001));
#350761=CARTESIAN_POINT('Ctrl Pts',(3.78475932799994,2.2,-1.94780164800001));
#350762=CARTESIAN_POINT('Ctrl Pts',(3.78643708899994,12.2,-1.94800640900001));
#350763=CARTESIAN_POINT('Ctrl Pts',(3.78643708899994,5.2,-1.94800640900001));
#350764=CARTESIAN_POINT('Ctrl Pts',(3.78643708899994,2.2,-1.94800640900001));
#350765=CARTESIAN_POINT('Ctrl Pts',(3.78811950799994,12.2,-1.94820978100001));
#350766=CARTESIAN_POINT('Ctrl Pts',(3.78811950799994,5.2,-1.94820978100001));
#350767=CARTESIAN_POINT('Ctrl Pts',(3.78811950799994,2.2,-1.94820978100001));
#350768=CARTESIAN_POINT('Ctrl Pts',(3.78980657699994,12.2,-1.94841175400001));
#350769=CARTESIAN_POINT('Ctrl Pts',(3.78980657699994,5.2,-1.94841175400001));
#350770=CARTESIAN_POINT('Ctrl Pts',(3.78980657699994,2.2,-1.94841175400001));
#350771=CARTESIAN_POINT('Ctrl Pts',(3.79149828999994,12.2,-1.94861232100001));
#350772=CARTESIAN_POINT('Ctrl Pts',(3.79149828999994,5.2,-1.94861232100001));
#350773=CARTESIAN_POINT('Ctrl Pts',(3.79149828999994,2.2,-1.94861232100001));
#350774=CARTESIAN_POINT('Ctrl Pts',(3.79319463899995,12.2,-1.94881147000002));
#350775=CARTESIAN_POINT('Ctrl Pts',(3.79319463899995,5.2,-1.94881147000002));
#350776=CARTESIAN_POINT('Ctrl Pts',(3.79319463899995,2.2,-1.94881147000002));
#350777=CARTESIAN_POINT('Ctrl Pts',(3.79489561699994,12.2,-1.94900919000002));
#350778=CARTESIAN_POINT('Ctrl Pts',(3.79489561699994,5.2,-1.94900919000002));
#350779=CARTESIAN_POINT('Ctrl Pts',(3.79489561699994,2.2,-1.94900919000002));
#350780=CARTESIAN_POINT('Ctrl Pts',(3.79660121799994,12.2,-1.94920547100002));
#350781=CARTESIAN_POINT('Ctrl Pts',(3.79660121799994,5.2,-1.94920547100002));
#350782=CARTESIAN_POINT('Ctrl Pts',(3.79660121799994,2.2,-1.94920547100002));
#350783=CARTESIAN_POINT('Ctrl Pts',(3.79831143499994,12.2,-1.94940030600002));
#350784=CARTESIAN_POINT('Ctrl Pts',(3.79831143499994,5.2,-1.94940030600002));
#350785=CARTESIAN_POINT('Ctrl Pts',(3.79831143499994,2.2,-1.94940030600002));
#350786=CARTESIAN_POINT('Ctrl Pts',(3.80002626099994,12.2,-1.94959368100001));
#350787=CARTESIAN_POINT('Ctrl Pts',(3.80002626099994,5.2,-1.94959368100001));
#350788=CARTESIAN_POINT('Ctrl Pts',(3.80002626099994,2.2,-1.94959368100001));
#350789=CARTESIAN_POINT('Ctrl Pts',(3.80174568899994,12.2,-1.94978558700001));
#350790=CARTESIAN_POINT('Ctrl Pts',(3.80174568899994,5.2,-1.94978558700001));
#350791=CARTESIAN_POINT('Ctrl Pts',(3.80174568899994,2.2,-1.94978558700001));
#350792=CARTESIAN_POINT('Ctrl Pts',(3.80346971199994,12.2,-1.94997601600001));
#350793=CARTESIAN_POINT('Ctrl Pts',(3.80346971199994,5.2,-1.94997601600001));
#350794=CARTESIAN_POINT('Ctrl Pts',(3.80346971199994,2.2,-1.94997601600001));
#350795=CARTESIAN_POINT('Ctrl Pts',(3.80519832299994,12.2,-1.95016495500001));
#350796=CARTESIAN_POINT('Ctrl Pts',(3.80519832299994,5.2,-1.95016495500001));
#350797=CARTESIAN_POINT('Ctrl Pts',(3.80519832299994,2.2,-1.95016495500001));
#350798=CARTESIAN_POINT('Ctrl Pts',(3.80693151599994,12.2,-1.95035239700001));
#350799=CARTESIAN_POINT('Ctrl Pts',(3.80693151599994,5.2,-1.95035239700001));
#350800=CARTESIAN_POINT('Ctrl Pts',(3.80693151599994,2.2,-1.95035239700001));
#350801=CARTESIAN_POINT('Ctrl Pts',(3.80866928199994,12.2,-1.95053833200001));
#350802=CARTESIAN_POINT('Ctrl Pts',(3.80866928199994,5.2,-1.95053833200001));
#350803=CARTESIAN_POINT('Ctrl Pts',(3.80866928199994,2.2,-1.95053833200001));
#350804=CARTESIAN_POINT('Ctrl Pts',(3.81041161799994,12.2,-1.95072274600002));
#350805=CARTESIAN_POINT('Ctrl Pts',(3.81041161799994,5.2,-1.95072274600002));
#350806=CARTESIAN_POINT('Ctrl Pts',(3.81041161799994,2.2,-1.95072274600002));
#350807=CARTESIAN_POINT('Ctrl Pts',(3.81215851299994,12.2,-1.95090563500001));
#350808=CARTESIAN_POINT('Ctrl Pts',(3.81215851299994,5.2,-1.95090563500001));
#350809=CARTESIAN_POINT('Ctrl Pts',(3.81215851299994,2.2,-1.95090563500001));
#350810=CARTESIAN_POINT('Ctrl Pts',(3.81390996099995,12.2,-1.95108698500002));
#350811=CARTESIAN_POINT('Ctrl Pts',(3.81390996099995,5.2,-1.95108698500002));
#350812=CARTESIAN_POINT('Ctrl Pts',(3.81390996099995,2.2,-1.95108698500002));
#350813=CARTESIAN_POINT('Ctrl Pts',(3.81566595699994,12.2,-1.95126678800001));
#350814=CARTESIAN_POINT('Ctrl Pts',(3.81566595699994,5.2,-1.95126678800001));
#350815=CARTESIAN_POINT('Ctrl Pts',(3.81566595699994,2.2,-1.95126678800001));
#350816=CARTESIAN_POINT('Ctrl Pts',(3.81742649299994,12.2,-1.95144503300002));
#350817=CARTESIAN_POINT('Ctrl Pts',(3.81742649299994,5.2,-1.95144503300002));
#350818=CARTESIAN_POINT('Ctrl Pts',(3.81742649299994,2.2,-1.95144503300002));
#350819=CARTESIAN_POINT('Ctrl Pts',(3.81919156199995,12.2,-1.95162171200002));
#350820=CARTESIAN_POINT('Ctrl Pts',(3.81919156199995,5.2,-1.95162171200002));
#350821=CARTESIAN_POINT('Ctrl Pts',(3.81919156199995,2.2,-1.95162171200002));
#350822=CARTESIAN_POINT('Ctrl Pts',(3.82096115699994,12.2,-1.95179681300001));
#350823=CARTESIAN_POINT('Ctrl Pts',(3.82096115699994,5.2,-1.95179681300001));
#350824=CARTESIAN_POINT('Ctrl Pts',(3.82096115699994,2.2,-1.95179681300001));
#350825=CARTESIAN_POINT('Ctrl Pts',(3.82273527099994,12.2,-1.95197032900001));
#350826=CARTESIAN_POINT('Ctrl Pts',(3.82273527099994,5.2,-1.95197032900001));
#350827=CARTESIAN_POINT('Ctrl Pts',(3.82273527099994,2.2,-1.95197032900001));
#350828=CARTESIAN_POINT('Ctrl Pts',(3.82451389799995,12.2,-1.95214224900001));
#350829=CARTESIAN_POINT('Ctrl Pts',(3.82451389799995,5.2,-1.95214224900001));
#350830=CARTESIAN_POINT('Ctrl Pts',(3.82451389799995,2.2,-1.95214224900001));
#350831=CARTESIAN_POINT('Ctrl Pts',(3.82629703099994,12.2,-1.95231256300001));
#350832=CARTESIAN_POINT('Ctrl Pts',(3.82629703099994,5.2,-1.95231256300001));
#350833=CARTESIAN_POINT('Ctrl Pts',(3.82629703099994,2.2,-1.95231256300001));
#350834=CARTESIAN_POINT('Ctrl Pts',(3.82808465999994,12.2,-1.95248126200001));
#350835=CARTESIAN_POINT('Ctrl Pts',(3.82808465999994,5.2,-1.95248126200001));
#350836=CARTESIAN_POINT('Ctrl Pts',(3.82808465999994,2.2,-1.95248126200001));
#350837=CARTESIAN_POINT('Ctrl Pts',(3.82987678299994,12.2,-1.95264833600001));
#350838=CARTESIAN_POINT('Ctrl Pts',(3.82987678299994,5.2,-1.95264833600001));
#350839=CARTESIAN_POINT('Ctrl Pts',(3.82987678299994,2.2,-1.95264833600001));
#350840=CARTESIAN_POINT('Ctrl Pts',(3.83167338899994,12.2,-1.95281377600002));
#350841=CARTESIAN_POINT('Ctrl Pts',(3.83167338899994,5.2,-1.95281377600002));
#350842=CARTESIAN_POINT('Ctrl Pts',(3.83167338899994,2.2,-1.95281377600002));
#350843=CARTESIAN_POINT('Ctrl Pts',(3.83347447499994,12.2,-1.95297757100001));
#350844=CARTESIAN_POINT('Ctrl Pts',(3.83347447499994,5.2,-1.95297757100001));
#350845=CARTESIAN_POINT('Ctrl Pts',(3.83347447499994,2.2,-1.95297757100001));
#350846=CARTESIAN_POINT('Ctrl Pts',(3.83528002999994,12.2,-1.95313971300001));
#350847=CARTESIAN_POINT('Ctrl Pts',(3.83528002999994,5.2,-1.95313971300001));
#350848=CARTESIAN_POINT('Ctrl Pts',(3.83528002999994,2.2,-1.95313971300001));
#350849=CARTESIAN_POINT('Ctrl Pts',(3.83709004999994,12.2,-1.95330019300001));
#350850=CARTESIAN_POINT('Ctrl Pts',(3.83709004999994,5.2,-1.95330019300001));
#350851=CARTESIAN_POINT('Ctrl Pts',(3.83709004999994,2.2,-1.95330019300001));
#350852=CARTESIAN_POINT('Ctrl Pts',(3.83890452599994,12.2,-1.95345900100001));
#350853=CARTESIAN_POINT('Ctrl Pts',(3.83890452599994,5.2,-1.95345900100001));
#350854=CARTESIAN_POINT('Ctrl Pts',(3.83890452599994,2.2,-1.95345900100001));
#350855=CARTESIAN_POINT('Ctrl Pts',(3.84072345299994,12.2,-1.95361612600002));
#350856=CARTESIAN_POINT('Ctrl Pts',(3.84072345299994,5.2,-1.95361612600002));
#350857=CARTESIAN_POINT('Ctrl Pts',(3.84072345299994,2.2,-1.95361612600002));
#350858=CARTESIAN_POINT('Ctrl Pts',(3.84254682399995,12.2,-1.95377156100002));
#350859=CARTESIAN_POINT('Ctrl Pts',(3.84254682399995,5.2,-1.95377156100002));
#350860=CARTESIAN_POINT('Ctrl Pts',(3.84254682399995,2.2,-1.95377156100002));
#350861=CARTESIAN_POINT('Ctrl Pts',(3.84437462999994,12.2,-1.95392529400001));
#350862=CARTESIAN_POINT('Ctrl Pts',(3.84437462999994,5.2,-1.95392529400001));
#350863=CARTESIAN_POINT('Ctrl Pts',(3.84437462999994,2.2,-1.95392529400001));
#350864=CARTESIAN_POINT('Ctrl Pts',(3.84620686599995,12.2,-1.95407731900001));
#350865=CARTESIAN_POINT('Ctrl Pts',(3.84620686599995,5.2,-1.95407731900001));
#350866=CARTESIAN_POINT('Ctrl Pts',(3.84620686599995,2.2,-1.95407731900001));
#350867=CARTESIAN_POINT('Ctrl Pts',(3.84804352399994,12.2,-1.95422762400002));
#350868=CARTESIAN_POINT('Ctrl Pts',(3.84804352399994,5.2,-1.95422762400002));
#350869=CARTESIAN_POINT('Ctrl Pts',(3.84804352399994,2.2,-1.95422762400002));
#350870=CARTESIAN_POINT('Ctrl Pts',(3.84988459799994,12.2,-1.95437620100002));
#350871=CARTESIAN_POINT('Ctrl Pts',(3.84988459799994,5.2,-1.95437620100002));
#350872=CARTESIAN_POINT('Ctrl Pts',(3.84988459799994,2.2,-1.95437620100002));
#350873=CARTESIAN_POINT('Ctrl Pts',(3.85173007999994,12.2,-1.95452304000002));
#350874=CARTESIAN_POINT('Ctrl Pts',(3.85173007999994,5.2,-1.95452304000002));
#350875=CARTESIAN_POINT('Ctrl Pts',(3.85173007999994,2.2,-1.95452304000002));
#350876=CARTESIAN_POINT('Ctrl Pts',(3.85357996499994,12.2,-1.95466813200001));
#350877=CARTESIAN_POINT('Ctrl Pts',(3.85357996499994,5.2,-1.95466813200001));
#350878=CARTESIAN_POINT('Ctrl Pts',(3.85357996499994,2.2,-1.95466813200001));
#350879=CARTESIAN_POINT('Ctrl Pts',(3.85543424399994,12.2,-1.95481146900002));
#350880=CARTESIAN_POINT('Ctrl Pts',(3.85543424399994,5.2,-1.95481146900002));
#350881=CARTESIAN_POINT('Ctrl Pts',(3.85543424399994,2.2,-1.95481146900002));
#350882=CARTESIAN_POINT('Ctrl Pts',(3.85729291099994,12.2,-1.95495303900001));
#350883=CARTESIAN_POINT('Ctrl Pts',(3.85729291099994,5.2,-1.95495303900001));
#350884=CARTESIAN_POINT('Ctrl Pts',(3.85729291099994,2.2,-1.95495303900001));
#350885=CARTESIAN_POINT('Ctrl Pts',(3.85915595899994,12.2,-1.95509283500002));
#350886=CARTESIAN_POINT('Ctrl Pts',(3.85915595899994,5.2,-1.95509283500002));
#350887=CARTESIAN_POINT('Ctrl Pts',(3.85915595899994,2.2,-1.95509283500002));
#350888=CARTESIAN_POINT('Ctrl Pts',(3.86102338099994,12.2,-1.95523084800001));
#350889=CARTESIAN_POINT('Ctrl Pts',(3.86102338099994,5.2,-1.95523084800001));
#350890=CARTESIAN_POINT('Ctrl Pts',(3.86102338099994,2.2,-1.95523084800001));
#350891=CARTESIAN_POINT('Ctrl Pts',(3.86289516999994,12.2,-1.95536706700001));
#350892=CARTESIAN_POINT('Ctrl Pts',(3.86289516999994,5.2,-1.95536706700001));
#350893=CARTESIAN_POINT('Ctrl Pts',(3.86289516999994,2.2,-1.95536706700001));
#350894=CARTESIAN_POINT('Ctrl Pts',(3.86477131999994,12.2,-1.95550148500002));
#350895=CARTESIAN_POINT('Ctrl Pts',(3.86477131999994,5.2,-1.95550148500002));
#350896=CARTESIAN_POINT('Ctrl Pts',(3.86477131999994,2.2,-1.95550148500002));
#350897=CARTESIAN_POINT('Ctrl Pts',(3.86665182199994,12.2,-1.95563409200001));
#350898=CARTESIAN_POINT('Ctrl Pts',(3.86665182199994,5.2,-1.95563409200001));
#350899=CARTESIAN_POINT('Ctrl Pts',(3.86665182199994,2.2,-1.95563409200001));
#350900=CARTESIAN_POINT('Ctrl Pts',(3.86853667099994,12.2,-1.95576487900002));
#350901=CARTESIAN_POINT('Ctrl Pts',(3.86853667099994,5.2,-1.95576487900002));
#350902=CARTESIAN_POINT('Ctrl Pts',(3.86853667099994,2.2,-1.95576487900002));
#350903=CARTESIAN_POINT('Ctrl Pts',(3.87042586099994,12.2,-1.95589383700002));
#350904=CARTESIAN_POINT('Ctrl Pts',(3.87042586099994,5.2,-1.95589383700002));
#350905=CARTESIAN_POINT('Ctrl Pts',(3.87042586099994,2.2,-1.95589383700002));
#350906=CARTESIAN_POINT('Ctrl Pts',(3.87231938099994,12.2,-1.95602095700002));
#350907=CARTESIAN_POINT('Ctrl Pts',(3.87231938099994,5.2,-1.95602095700002));
#350908=CARTESIAN_POINT('Ctrl Pts',(3.87231938099994,2.2,-1.95602095700002));
#350909=CARTESIAN_POINT('Ctrl Pts',(3.87421722899994,12.2,-1.95614623000001));
#350910=CARTESIAN_POINT('Ctrl Pts',(3.87421722899994,5.2,-1.95614623000001));
#350911=CARTESIAN_POINT('Ctrl Pts',(3.87421722899994,2.2,-1.95614623000001));
#350912=CARTESIAN_POINT('Ctrl Pts',(3.87611939399994,12.2,-1.95626964900002));
#350913=CARTESIAN_POINT('Ctrl Pts',(3.87611939399994,5.2,-1.95626964900002));
#350914=CARTESIAN_POINT('Ctrl Pts',(3.87611939399994,2.2,-1.95626964900002));
#350915=CARTESIAN_POINT('Ctrl Pts',(3.87802587099995,12.2,-1.95639120100001));
#350916=CARTESIAN_POINT('Ctrl Pts',(3.87802587099995,5.2,-1.95639120100001));
#350917=CARTESIAN_POINT('Ctrl Pts',(3.87802587099995,2.2,-1.95639120100001));
#350918=CARTESIAN_POINT('Ctrl Pts',(3.87993665399994,12.2,-1.95651088000002));
#350919=CARTESIAN_POINT('Ctrl Pts',(3.87993665399994,5.2,-1.95651088000002));
#350920=CARTESIAN_POINT('Ctrl Pts',(3.87993665399994,2.2,-1.95651088000002));
#350921=CARTESIAN_POINT('Ctrl Pts',(3.88185173299994,12.2,-1.95662867600001));
#350922=CARTESIAN_POINT('Ctrl Pts',(3.88185173299994,5.2,-1.95662867600001));
#350923=CARTESIAN_POINT('Ctrl Pts',(3.88185173299994,2.2,-1.95662867600001));
#350924=CARTESIAN_POINT('Ctrl Pts',(3.88377110399994,12.2,-1.95674458100001));
#350925=CARTESIAN_POINT('Ctrl Pts',(3.88377110399994,5.2,-1.95674458100001));
#350926=CARTESIAN_POINT('Ctrl Pts',(3.88377110399994,2.2,-1.95674458100001));
#350927=CARTESIAN_POINT('Ctrl Pts',(3.88569475899994,12.2,-1.95685858600001));
#350928=CARTESIAN_POINT('Ctrl Pts',(3.88569475899994,5.2,-1.95685858600001));
#350929=CARTESIAN_POINT('Ctrl Pts',(3.88569475899994,2.2,-1.95685858600001));
#350930=CARTESIAN_POINT('Ctrl Pts',(3.88762269099994,12.2,-1.95697068200001));
#350931=CARTESIAN_POINT('Ctrl Pts',(3.88762269099994,5.2,-1.95697068200001));
#350932=CARTESIAN_POINT('Ctrl Pts',(3.88762269099994,2.2,-1.95697068200001));
#350933=CARTESIAN_POINT('Ctrl Pts',(3.88955489299994,12.2,-1.95708085900002));
#350934=CARTESIAN_POINT('Ctrl Pts',(3.88955489299994,5.2,-1.95708085900002));
#350935=CARTESIAN_POINT('Ctrl Pts',(3.88955489299994,2.2,-1.95708085900002));
#350936=CARTESIAN_POINT('Ctrl Pts',(3.89149135899994,12.2,-1.95718911000001));
#350937=CARTESIAN_POINT('Ctrl Pts',(3.89149135899994,5.2,-1.95718911000001));
#350938=CARTESIAN_POINT('Ctrl Pts',(3.89149135899994,2.2,-1.95718911000001));
#350939=CARTESIAN_POINT('Ctrl Pts',(3.89343207999994,12.2,-1.95729542700001));
#350940=CARTESIAN_POINT('Ctrl Pts',(3.89343207999994,5.2,-1.95729542700001));
#350941=CARTESIAN_POINT('Ctrl Pts',(3.89343207999994,2.2,-1.95729542700001));
#350942=CARTESIAN_POINT('Ctrl Pts',(3.89537705199994,12.2,-1.95739979900001));
#350943=CARTESIAN_POINT('Ctrl Pts',(3.89537705199994,5.2,-1.95739979900001));
#350944=CARTESIAN_POINT('Ctrl Pts',(3.89537705199994,2.2,-1.95739979900001));
#350945=CARTESIAN_POINT('Ctrl Pts',(3.89732626499994,12.2,-1.95750221800001));
#350946=CARTESIAN_POINT('Ctrl Pts',(3.89732626499994,5.2,-1.95750221800001));
#350947=CARTESIAN_POINT('Ctrl Pts',(3.89732626499994,2.2,-1.95750221800001));
#350948=CARTESIAN_POINT('Ctrl Pts',(3.89927971499994,12.2,-1.95760267600001));
#350949=CARTESIAN_POINT('Ctrl Pts',(3.89927971499994,5.2,-1.95760267600001));
#350950=CARTESIAN_POINT('Ctrl Pts',(3.89927971499994,2.2,-1.95760267600001));
#350951=CARTESIAN_POINT('Ctrl Pts',(3.90123739199994,12.2,-1.95770116400002));
#350952=CARTESIAN_POINT('Ctrl Pts',(3.90123739199994,5.2,-1.95770116400002));
#350953=CARTESIAN_POINT('Ctrl Pts',(3.90123739199994,2.2,-1.95770116400002));
#350954=CARTESIAN_POINT('Ctrl Pts',(3.90319929199994,12.2,-1.95779767400001));
#350955=CARTESIAN_POINT('Ctrl Pts',(3.90319929199994,5.2,-1.95779767400001));
#350956=CARTESIAN_POINT('Ctrl Pts',(3.90319929199994,2.2,-1.95779767400001));
#350957=CARTESIAN_POINT('Ctrl Pts',(3.90516540699994,12.2,-1.95789219700002));
#350958=CARTESIAN_POINT('Ctrl Pts',(3.90516540699994,5.2,-1.95789219700002));
#350959=CARTESIAN_POINT('Ctrl Pts',(3.90516540699994,2.2,-1.95789219700002));
#350960=CARTESIAN_POINT('Ctrl Pts',(3.90713572899994,12.2,-1.95798472300002));
#350961=CARTESIAN_POINT('Ctrl Pts',(3.90713572899994,5.2,-1.95798472300002));
#350962=CARTESIAN_POINT('Ctrl Pts',(3.90713572899994,2.2,-1.95798472300002));
#350963=CARTESIAN_POINT('Ctrl Pts',(3.90911025099994,12.2,-1.95807524500001));
#350964=CARTESIAN_POINT('Ctrl Pts',(3.90911025099994,5.2,-1.95807524500001));
#350965=CARTESIAN_POINT('Ctrl Pts',(3.90911025099994,2.2,-1.95807524500001));
#350966=CARTESIAN_POINT('Ctrl Pts',(3.91108896799994,12.2,-1.95816375500002));
#350967=CARTESIAN_POINT('Ctrl Pts',(3.91108896799994,5.2,-1.95816375500002));
#350968=CARTESIAN_POINT('Ctrl Pts',(3.91108896799994,2.2,-1.95816375500002));
#350969=CARTESIAN_POINT('Ctrl Pts',(3.91307187099994,12.2,-1.95825024400001));
#350970=CARTESIAN_POINT('Ctrl Pts',(3.91307187099994,5.2,-1.95825024400001));
#350971=CARTESIAN_POINT('Ctrl Pts',(3.91307187099994,2.2,-1.95825024400001));
#350972=CARTESIAN_POINT('Ctrl Pts',(3.91505895599995,12.2,-1.95833470300002));
#350973=CARTESIAN_POINT('Ctrl Pts',(3.91505895599995,5.2,-1.95833470300002));
#350974=CARTESIAN_POINT('Ctrl Pts',(3.91505895599995,2.2,-1.95833470300002));
#350975=CARTESIAN_POINT('Ctrl Pts',(3.91705021199994,12.2,-1.95841712400001));
#350976=CARTESIAN_POINT('Ctrl Pts',(3.91705021199994,5.2,-1.95841712400001));
#350977=CARTESIAN_POINT('Ctrl Pts',(3.91705021199994,2.2,-1.95841712400001));
#350978=CARTESIAN_POINT('Ctrl Pts',(3.91904563499994,12.2,-1.95849749800002));
#350979=CARTESIAN_POINT('Ctrl Pts',(3.91904563499994,5.2,-1.95849749800002));
#350980=CARTESIAN_POINT('Ctrl Pts',(3.91904563499994,2.2,-1.95849749800002));
#350981=CARTESIAN_POINT('Ctrl Pts',(3.92104521699994,12.2,-1.95857581700002));
#350982=CARTESIAN_POINT('Ctrl Pts',(3.92104521699994,5.2,-1.95857581700002));
#350983=CARTESIAN_POINT('Ctrl Pts',(3.92104521699994,2.2,-1.95857581700002));
#350984=CARTESIAN_POINT('Ctrl Pts',(3.92304895199994,12.2,-1.95865207300002));
#350985=CARTESIAN_POINT('Ctrl Pts',(3.92304895199994,5.2,-1.95865207300002));
#350986=CARTESIAN_POINT('Ctrl Pts',(3.92304895199994,2.2,-1.95865207300002));
#350987=CARTESIAN_POINT('Ctrl Pts',(3.92505683199994,12.2,-1.95872625700002));
#350988=CARTESIAN_POINT('Ctrl Pts',(3.92505683199994,5.2,-1.95872625700002));
#350989=CARTESIAN_POINT('Ctrl Pts',(3.92505683199994,2.2,-1.95872625700002));
#350990=CARTESIAN_POINT('Ctrl Pts',(3.92706884999994,12.2,-1.95879836000001));
#350991=CARTESIAN_POINT('Ctrl Pts',(3.92706884999994,5.2,-1.95879836000001));
#350992=CARTESIAN_POINT('Ctrl Pts',(3.92706884999994,2.2,-1.95879836000001));
#350993=CARTESIAN_POINT('Ctrl Pts',(3.92908500099994,12.2,-1.95886837500002));
#350994=CARTESIAN_POINT('Ctrl Pts',(3.92908500099994,5.2,-1.95886837500002));
#350995=CARTESIAN_POINT('Ctrl Pts',(3.92908500099994,2.2,-1.95886837500002));
#350996=CARTESIAN_POINT('Ctrl Pts',(3.93110527499994,12.2,-1.95893629500001));
#350997=CARTESIAN_POINT('Ctrl Pts',(3.93110527499994,5.2,-1.95893629500001));
#350998=CARTESIAN_POINT('Ctrl Pts',(3.93110527499994,2.2,-1.95893629500001));
#350999=CARTESIAN_POINT('Ctrl Pts',(3.93312966599995,12.2,-1.95900210900001));
#351000=CARTESIAN_POINT('Ctrl Pts',(3.93312966599995,5.2,-1.95900210900001));
#351001=CARTESIAN_POINT('Ctrl Pts',(3.93312966599995,2.2,-1.95900210900001));
#351002=CARTESIAN_POINT('Ctrl Pts',(3.93515816899995,12.2,-1.95906581000001));
#351003=CARTESIAN_POINT('Ctrl Pts',(3.93515816899995,5.2,-1.95906581000001));
#351004=CARTESIAN_POINT('Ctrl Pts',(3.93515816899995,2.2,-1.95906581000001));
#351005=CARTESIAN_POINT('Ctrl Pts',(3.93719077599994,12.2,-1.95912739000002));
#351006=CARTESIAN_POINT('Ctrl Pts',(3.93719077599994,5.2,-1.95912739000002));
#351007=CARTESIAN_POINT('Ctrl Pts',(3.93719077599994,2.2,-1.95912739000002));
#351008=CARTESIAN_POINT('Ctrl Pts',(3.93922747899994,12.2,-1.95918683900001));
#351009=CARTESIAN_POINT('Ctrl Pts',(3.93922747899994,5.2,-1.95918683900001));
#351010=CARTESIAN_POINT('Ctrl Pts',(3.93922747899994,2.2,-1.95918683900001));
#351011=CARTESIAN_POINT('Ctrl Pts',(3.94126827199994,12.2,-1.95924415200002));
#351012=CARTESIAN_POINT('Ctrl Pts',(3.94126827199994,5.2,-1.95924415200002));
#351013=CARTESIAN_POINT('Ctrl Pts',(3.94126827199994,2.2,-1.95924415200002));
#351014=CARTESIAN_POINT('Ctrl Pts',(3.94331314799994,12.2,-1.95929931800002));
#351015=CARTESIAN_POINT('Ctrl Pts',(3.94331314799994,5.2,-1.95929931800002));
#351016=CARTESIAN_POINT('Ctrl Pts',(3.94331314799994,2.2,-1.95929931800002));
#351017=CARTESIAN_POINT('Ctrl Pts',(3.94536209899994,12.2,-1.95935233100001));
#351018=CARTESIAN_POINT('Ctrl Pts',(3.94536209899994,5.2,-1.95935233100001));
#351019=CARTESIAN_POINT('Ctrl Pts',(3.94536209899994,2.2,-1.95935233100001));
#351020=CARTESIAN_POINT('Ctrl Pts',(3.94741511999994,12.2,-1.95940318100002));
#351021=CARTESIAN_POINT('Ctrl Pts',(3.94741511999994,5.2,-1.95940318100002));
#351022=CARTESIAN_POINT('Ctrl Pts',(3.94741511999994,2.2,-1.95940318100002));
#351023=CARTESIAN_POINT('Ctrl Pts',(3.94947220299994,12.2,-1.95945186100001));
#351024=CARTESIAN_POINT('Ctrl Pts',(3.94947220299994,5.2,-1.95945186100001));
#351025=CARTESIAN_POINT('Ctrl Pts',(3.94947220299994,2.2,-1.95945186100001));
#351026=CARTESIAN_POINT('Ctrl Pts',(3.95153334099994,12.2,-1.95949836300001));
#351027=CARTESIAN_POINT('Ctrl Pts',(3.95153334099994,5.2,-1.95949836300001));
#351028=CARTESIAN_POINT('Ctrl Pts',(3.95153334099994,2.2,-1.95949836300001));
#351029=CARTESIAN_POINT('Ctrl Pts',(3.95359852699994,12.2,-1.95954267800001));
#351030=CARTESIAN_POINT('Ctrl Pts',(3.95359852699994,5.2,-1.95954267800001));
#351031=CARTESIAN_POINT('Ctrl Pts',(3.95359852699994,2.2,-1.95954267800001));
#351032=CARTESIAN_POINT('Ctrl Pts',(3.95566775399994,12.2,-1.95958480000002));
#351033=CARTESIAN_POINT('Ctrl Pts',(3.95566775399994,5.2,-1.95958480000002));
#351034=CARTESIAN_POINT('Ctrl Pts',(3.95566775399994,2.2,-1.95958480000002));
#351035=CARTESIAN_POINT('Ctrl Pts',(3.95774101599994,12.2,-1.95962471800001));
#351036=CARTESIAN_POINT('Ctrl Pts',(3.95774101599994,5.2,-1.95962471800001));
#351037=CARTESIAN_POINT('Ctrl Pts',(3.95774101599994,2.2,-1.95962471800001));
#351038=CARTESIAN_POINT('Ctrl Pts',(3.95981830499994,12.2,-1.95966242600001));
#351039=CARTESIAN_POINT('Ctrl Pts',(3.95981830499994,5.2,-1.95966242600001));
#351040=CARTESIAN_POINT('Ctrl Pts',(3.95981830499994,2.2,-1.95966242600001));
#351041=CARTESIAN_POINT('Ctrl Pts',(3.96189961499994,12.2,-1.95969791700001));
#351042=CARTESIAN_POINT('Ctrl Pts',(3.96189961499994,5.2,-1.95969791700001));
#351043=CARTESIAN_POINT('Ctrl Pts',(3.96189961499994,2.2,-1.95969791700001));
#351044=CARTESIAN_POINT('Ctrl Pts',(3.96398493799994,12.2,-1.95973118100001));
#351045=CARTESIAN_POINT('Ctrl Pts',(3.96398493799994,5.2,-1.95973118100001));
#351046=CARTESIAN_POINT('Ctrl Pts',(3.96398493799994,2.2,-1.95973118100001));
#351047=CARTESIAN_POINT('Ctrl Pts',(3.96607426699994,12.2,-1.95976221100001));
#351048=CARTESIAN_POINT('Ctrl Pts',(3.96607426699994,5.2,-1.95976221100001));
#351049=CARTESIAN_POINT('Ctrl Pts',(3.96607426699994,2.2,-1.95976221100001));
#351050=CARTESIAN_POINT('Ctrl Pts',(3.96816759599994,12.2,-1.95979099800001));
#351051=CARTESIAN_POINT('Ctrl Pts',(3.96816759599994,5.2,-1.95979099800001));
#351052=CARTESIAN_POINT('Ctrl Pts',(3.96816759599994,2.2,-1.95979099800001));
#351053=CARTESIAN_POINT('Ctrl Pts',(3.97026491799994,12.2,-1.95981753700002));
#351054=CARTESIAN_POINT('Ctrl Pts',(3.97026491799994,5.2,-1.95981753700002));
#351055=CARTESIAN_POINT('Ctrl Pts',(3.97026491799994,2.2,-1.95981753700002));
#351056=CARTESIAN_POINT('Ctrl Pts',(3.97236622599995,12.2,-1.95984181700001));
#351057=CARTESIAN_POINT('Ctrl Pts',(3.97236622599995,5.2,-1.95984181700001));
#351058=CARTESIAN_POINT('Ctrl Pts',(3.97236622599995,2.2,-1.95984181700001));
#351059=CARTESIAN_POINT('Ctrl Pts',(3.97447151099994,12.2,-1.95986383200002));
#351060=CARTESIAN_POINT('Ctrl Pts',(3.97447151099994,5.2,-1.95986383200002));
#351061=CARTESIAN_POINT('Ctrl Pts',(3.97447151099994,2.2,-1.95986383200002));
#351062=CARTESIAN_POINT('Ctrl Pts',(3.97658076899994,12.2,-1.95988357400001));
#351063=CARTESIAN_POINT('Ctrl Pts',(3.97658076899994,5.2,-1.95988357400001));
#351064=CARTESIAN_POINT('Ctrl Pts',(3.97658076899994,2.2,-1.95988357400001));
#351065=CARTESIAN_POINT('Ctrl Pts',(3.97869399199994,12.2,-1.95990103400002));
#351066=CARTESIAN_POINT('Ctrl Pts',(3.97869399199994,5.2,-1.95990103400002));
#351067=CARTESIAN_POINT('Ctrl Pts',(3.97869399199994,2.2,-1.95990103400002));
#351068=CARTESIAN_POINT('Ctrl Pts',(3.98081117199994,12.2,-1.95991620600001));
#351069=CARTESIAN_POINT('Ctrl Pts',(3.98081117199994,5.2,-1.95991620600001));
#351070=CARTESIAN_POINT('Ctrl Pts',(3.98081117199994,2.2,-1.95991620600001));
#351071=CARTESIAN_POINT('Ctrl Pts',(3.98293230399994,12.2,-1.95992908000001));
#351072=CARTESIAN_POINT('Ctrl Pts',(3.98293230399994,5.2,-1.95992908000001));
#351073=CARTESIAN_POINT('Ctrl Pts',(3.98293230399994,2.2,-1.95992908000001));
#351074=CARTESIAN_POINT('Ctrl Pts',(3.98505737899994,12.2,-1.95993965100001));
#351075=CARTESIAN_POINT('Ctrl Pts',(3.98505737899994,5.2,-1.95993965100001));
#351076=CARTESIAN_POINT('Ctrl Pts',(3.98505737899994,2.2,-1.95993965100001));
#351077=CARTESIAN_POINT('Ctrl Pts',(3.98718639199994,12.2,-1.95994791000001));
#351078=CARTESIAN_POINT('Ctrl Pts',(3.98718639199994,5.2,-1.95994791000001));
#351079=CARTESIAN_POINT('Ctrl Pts',(3.98718639199994,2.2,-1.95994791000001));
#351080=CARTESIAN_POINT('Ctrl Pts',(3.98931933399994,12.2,-1.95995384900002));
#351081=CARTESIAN_POINT('Ctrl Pts',(3.98931933399994,5.2,-1.95995384900002));
#351082=CARTESIAN_POINT('Ctrl Pts',(3.98931933399994,2.2,-1.95995384900002));
#351083=CARTESIAN_POINT('Ctrl Pts',(3.99145619999994,12.2,-1.95995746100001));
#351084=CARTESIAN_POINT('Ctrl Pts',(3.99145619999994,5.2,-1.95995746100001));
#351085=CARTESIAN_POINT('Ctrl Pts',(3.99145619999994,2.2,-1.95995746100001));
#351086=CARTESIAN_POINT('Ctrl Pts',(3.99359698299994,12.2,-1.95995873700001));
#351087=CARTESIAN_POINT('Ctrl Pts',(3.99359698299994,5.2,-1.95995873700001));
#351088=CARTESIAN_POINT('Ctrl Pts',(3.99359698299994,2.2,-1.95995873700001));
#351089=CARTESIAN_POINT('Ctrl Pts',(3.99574167399994,12.2,-1.95995767100001));
#351090=CARTESIAN_POINT('Ctrl Pts',(3.99574167399994,5.2,-1.95995767100001));
#351091=CARTESIAN_POINT('Ctrl Pts',(3.99574167399994,2.2,-1.95995767100001));
#351092=CARTESIAN_POINT('Ctrl Pts',(3.99789026699994,12.2,-1.95995425500001));
#351093=CARTESIAN_POINT('Ctrl Pts',(3.99789026699994,5.2,-1.95995425500001));
#351094=CARTESIAN_POINT('Ctrl Pts',(3.99789026699994,2.2,-1.95995425500001));
#351095=CARTESIAN_POINT('Ctrl Pts',(4.00004275699995,12.2,-1.95994848100002));
#351096=CARTESIAN_POINT('Ctrl Pts',(4.00004275699995,5.2,-1.95994848100002));
#351097=CARTESIAN_POINT('Ctrl Pts',(4.00004275699995,2.2,-1.95994848100002));
#351098=CARTESIAN_POINT('Ctrl Pts',(4.00219913399994,12.2,-1.95994034100002));
#351099=CARTESIAN_POINT('Ctrl Pts',(4.00219913399994,5.2,-1.95994034100002));
#351100=CARTESIAN_POINT('Ctrl Pts',(4.00219913399994,2.2,-1.95994034100002));
#351101=CARTESIAN_POINT('Ctrl Pts',(4.00435939399994,12.2,-1.95992982900002));
#351102=CARTESIAN_POINT('Ctrl Pts',(4.00435939399994,5.2,-1.95992982900002));
#351103=CARTESIAN_POINT('Ctrl Pts',(4.00435939399994,2.2,-1.95992982900002));
#351104=CARTESIAN_POINT('Ctrl Pts',(4.00652352699994,12.2,-1.95991693600002));
#351105=CARTESIAN_POINT('Ctrl Pts',(4.00652352699994,5.2,-1.95991693600002));
#351106=CARTESIAN_POINT('Ctrl Pts',(4.00652352699994,2.2,-1.95991693600002));
#351107=CARTESIAN_POINT('Ctrl Pts',(4.00869152799994,12.2,-1.95990165600001));
#351108=CARTESIAN_POINT('Ctrl Pts',(4.00869152799994,5.2,-1.95990165600001));
#351109=CARTESIAN_POINT('Ctrl Pts',(4.00869152799994,2.2,-1.95990165600001));
#351110=CARTESIAN_POINT('Ctrl Pts',(4.01086338899994,12.2,-1.95988398100001));
#351111=CARTESIAN_POINT('Ctrl Pts',(4.01086338899994,5.2,-1.95988398100001));
#351112=CARTESIAN_POINT('Ctrl Pts',(4.01086338899994,2.2,-1.95988398100001));
#351113=CARTESIAN_POINT('Ctrl Pts',(4.01303910599994,12.2,-1.95986390200002));
#351114=CARTESIAN_POINT('Ctrl Pts',(4.01303910599994,5.2,-1.95986390200002));
#351115=CARTESIAN_POINT('Ctrl Pts',(4.01303910599994,2.2,-1.95986390200002));
#351116=CARTESIAN_POINT('Ctrl Pts',(4.01521866799994,12.2,-1.95984141300002));
#351117=CARTESIAN_POINT('Ctrl Pts',(4.01521866799994,5.2,-1.95984141300002));
#351118=CARTESIAN_POINT('Ctrl Pts',(4.01521866799994,2.2,-1.95984141300002));
#351119=CARTESIAN_POINT('Ctrl Pts',(4.01740206999994,12.2,-1.95981650700002));
#351120=CARTESIAN_POINT('Ctrl Pts',(4.01740206999994,5.2,-1.95981650700002));
#351121=CARTESIAN_POINT('Ctrl Pts',(4.01740206999994,2.2,-1.95981650700002));
#351122=CARTESIAN_POINT('Ctrl Pts',(4.01958930399995,12.2,-1.95978917600002));
#351123=CARTESIAN_POINT('Ctrl Pts',(4.01958930399995,5.2,-1.95978917600002));
#351124=CARTESIAN_POINT('Ctrl Pts',(4.01958930399995,2.2,-1.95978917600002));
#351125=CARTESIAN_POINT('Ctrl Pts',(4.02178036499994,12.2,-1.95975941200001));
#351126=CARTESIAN_POINT('Ctrl Pts',(4.02178036499994,5.2,-1.95975941200001));
#351127=CARTESIAN_POINT('Ctrl Pts',(4.02178036499994,2.2,-1.95975941200001));
#351128=CARTESIAN_POINT('Ctrl Pts',(4.02397524499994,12.2,-1.95972720900001));
#351129=CARTESIAN_POINT('Ctrl Pts',(4.02397524499994,5.2,-1.95972720900001));
#351130=CARTESIAN_POINT('Ctrl Pts',(4.02397524499994,2.2,-1.95972720900001));
#351131=CARTESIAN_POINT('Ctrl Pts',(4.02617393699995,12.2,-1.95969255800001));
#351132=CARTESIAN_POINT('Ctrl Pts',(4.02617393699995,5.2,-1.95969255800001));
#351133=CARTESIAN_POINT('Ctrl Pts',(4.02617393699995,2.2,-1.95969255800001));
#351134=CARTESIAN_POINT('Ctrl Pts',(4.02837643299994,12.2,-1.95965545400002));
#351135=CARTESIAN_POINT('Ctrl Pts',(4.02837643299994,5.2,-1.95965545400002));
#351136=CARTESIAN_POINT('Ctrl Pts',(4.02837643299994,2.2,-1.95965545400002));
#351137=CARTESIAN_POINT('Ctrl Pts',(4.03058272899994,12.2,-1.95961588700001));
#351138=CARTESIAN_POINT('Ctrl Pts',(4.03058272899994,5.2,-1.95961588700001));
#351139=CARTESIAN_POINT('Ctrl Pts',(4.03058272899994,2.2,-1.95961588700001));
#351140=CARTESIAN_POINT('Ctrl Pts',(4.03279281399994,12.2,-1.95957385300002));
#351141=CARTESIAN_POINT('Ctrl Pts',(4.03279281399994,5.2,-1.95957385300002));
#351142=CARTESIAN_POINT('Ctrl Pts',(4.03279281399994,2.2,-1.95957385300002));
#351143=CARTESIAN_POINT('Ctrl Pts',(4.03500668499994,12.2,-1.95952934100001));
#351144=CARTESIAN_POINT('Ctrl Pts',(4.03500668499994,5.2,-1.95952934100001));
#351145=CARTESIAN_POINT('Ctrl Pts',(4.03500668499994,2.2,-1.95952934100001));
#351146=CARTESIAN_POINT('Ctrl Pts',(4.03722433299994,12.2,-1.95948234700001));
#351147=CARTESIAN_POINT('Ctrl Pts',(4.03722433299994,5.2,-1.95948234700001));
#351148=CARTESIAN_POINT('Ctrl Pts',(4.03722433299994,2.2,-1.95948234700001));
#351149=CARTESIAN_POINT('Ctrl Pts',(4.03944575099994,12.2,-1.95943286200002));
#351150=CARTESIAN_POINT('Ctrl Pts',(4.03944575099994,5.2,-1.95943286200002));
#351151=CARTESIAN_POINT('Ctrl Pts',(4.03944575099994,2.2,-1.95943286200002));
#351152=CARTESIAN_POINT('Ctrl Pts',(4.04167093199994,12.2,-1.95938087800001));
#351153=CARTESIAN_POINT('Ctrl Pts',(4.04167093199994,5.2,-1.95938087800001));
#351154=CARTESIAN_POINT('Ctrl Pts',(4.04167093199994,2.2,-1.95938087800001));
#351155=CARTESIAN_POINT('Ctrl Pts',(4.04389986999994,12.2,-1.95932639000001));
#351156=CARTESIAN_POINT('Ctrl Pts',(4.04389986999994,5.2,-1.95932639000001));
#351157=CARTESIAN_POINT('Ctrl Pts',(4.04389986999994,2.2,-1.95932639000001));
#351158=CARTESIAN_POINT('Ctrl Pts',(4.04613255699994,12.2,-1.95926939100001));
#351159=CARTESIAN_POINT('Ctrl Pts',(4.04613255699994,5.2,-1.95926939100001));
#351160=CARTESIAN_POINT('Ctrl Pts',(4.04613255699994,2.2,-1.95926939100001));
#351161=CARTESIAN_POINT('Ctrl Pts',(4.04836898699994,12.2,-1.95920987100001));
#351162=CARTESIAN_POINT('Ctrl Pts',(4.04836898699994,5.2,-1.95920987100001));
#351163=CARTESIAN_POINT('Ctrl Pts',(4.04836898699994,2.2,-1.95920987100001));
#351164=CARTESIAN_POINT('Ctrl Pts',(4.05060915299994,12.2,-1.95914782500001));
#351165=CARTESIAN_POINT('Ctrl Pts',(4.05060915299994,5.2,-1.95914782500001));
#351166=CARTESIAN_POINT('Ctrl Pts',(4.05060915299994,2.2,-1.95914782500001));
#351167=CARTESIAN_POINT('Ctrl Pts',(4.05285304699994,12.2,-1.95908324700001));
#351168=CARTESIAN_POINT('Ctrl Pts',(4.05285304699994,5.2,-1.95908324700001));
#351169=CARTESIAN_POINT('Ctrl Pts',(4.05285304699994,2.2,-1.95908324700001));
#351170=CARTESIAN_POINT('Ctrl Pts',(4.05510066299995,12.2,-1.95901612800002));
#351171=CARTESIAN_POINT('Ctrl Pts',(4.05510066299995,5.2,-1.95901612800002));
#351172=CARTESIAN_POINT('Ctrl Pts',(4.05510066299995,2.2,-1.95901612800002));
#351173=CARTESIAN_POINT('Ctrl Pts',(4.05735199399994,12.2,-1.95894646100002));
#351174=CARTESIAN_POINT('Ctrl Pts',(4.05735199399994,5.2,-1.95894646100002));
#351175=CARTESIAN_POINT('Ctrl Pts',(4.05735199399994,2.2,-1.95894646100002));
#351176=CARTESIAN_POINT('Ctrl Pts',(4.05960703199994,12.2,-1.95887423900002));
#351177=CARTESIAN_POINT('Ctrl Pts',(4.05960703199994,5.2,-1.95887423900002));
#351178=CARTESIAN_POINT('Ctrl Pts',(4.05960703199994,2.2,-1.95887423900002));
#351179=CARTESIAN_POINT('Ctrl Pts',(4.06186577099994,12.2,-1.95879945700002));
#351180=CARTESIAN_POINT('Ctrl Pts',(4.06186577099994,5.2,-1.95879945700002));
#351181=CARTESIAN_POINT('Ctrl Pts',(4.06186577099994,2.2,-1.95879945700002));
#351182=CARTESIAN_POINT('Ctrl Pts',(4.06412820499995,12.2,-1.95872210500001));
#351183=CARTESIAN_POINT('Ctrl Pts',(4.06412820499995,5.2,-1.95872210500001));
#351184=CARTESIAN_POINT('Ctrl Pts',(4.06412820499995,2.2,-1.95872210500001));
#351185=CARTESIAN_POINT('Ctrl Pts',(4.06639432499994,12.2,-1.95864217800001));
#351186=CARTESIAN_POINT('Ctrl Pts',(4.06639432499994,5.2,-1.95864217800001));
#351187=CARTESIAN_POINT('Ctrl Pts',(4.06639432499994,2.2,-1.95864217800001));
#351188=CARTESIAN_POINT('Ctrl Pts',(4.06866412499994,12.2,-1.95855966900002));
#351189=CARTESIAN_POINT('Ctrl Pts',(4.06866412499994,5.2,-1.95855966900002));
#351190=CARTESIAN_POINT('Ctrl Pts',(4.06866412499994,2.2,-1.95855966900002));
#351191=CARTESIAN_POINT('Ctrl Pts',(4.07093759899994,12.2,-1.95847457000002));
#351192=CARTESIAN_POINT('Ctrl Pts',(4.07093759899994,5.2,-1.95847457000002));
#351193=CARTESIAN_POINT('Ctrl Pts',(4.07093759899994,2.2,-1.95847457000002));
#351194=CARTESIAN_POINT('Ctrl Pts',(4.07321473899994,12.2,-1.95838687600002));
#351195=CARTESIAN_POINT('Ctrl Pts',(4.07321473899994,5.2,-1.95838687600002));
#351196=CARTESIAN_POINT('Ctrl Pts',(4.07321473899994,2.2,-1.95838687600002));
#351197=CARTESIAN_POINT('Ctrl Pts',(4.07549553699995,12.2,-1.95829657700001));
#351198=CARTESIAN_POINT('Ctrl Pts',(4.07549553699995,5.2,-1.95829657700001));
#351199=CARTESIAN_POINT('Ctrl Pts',(4.07549553699995,2.2,-1.95829657700001));
#351200=CARTESIAN_POINT('Ctrl Pts',(4.07777998799994,12.2,-1.95820366900001));
#351201=CARTESIAN_POINT('Ctrl Pts',(4.07777998799994,5.2,-1.95820366900001));
#351202=CARTESIAN_POINT('Ctrl Pts',(4.07777998799994,2.2,-1.95820366900001));
#351203=CARTESIAN_POINT('Ctrl Pts',(4.08006808399994,12.2,-1.95810814400001));
#351204=CARTESIAN_POINT('Ctrl Pts',(4.08006808399994,5.2,-1.95810814400001));
#351205=CARTESIAN_POINT('Ctrl Pts',(4.08006808399994,2.2,-1.95810814400001));
#351206=CARTESIAN_POINT('Ctrl Pts',(4.08235981899994,12.2,-1.95800999500001));
#351207=CARTESIAN_POINT('Ctrl Pts',(4.08235981899994,5.2,-1.95800999500001));
#351208=CARTESIAN_POINT('Ctrl Pts',(4.08235981899994,2.2,-1.95800999500001));
#351209=CARTESIAN_POINT('Ctrl Pts',(4.08465518599994,12.2,-1.95790921500001));
#351210=CARTESIAN_POINT('Ctrl Pts',(4.08465518599994,5.2,-1.95790921500001));
#351211=CARTESIAN_POINT('Ctrl Pts',(4.08465518599994,2.2,-1.95790921500001));
#351212=CARTESIAN_POINT('Ctrl Pts',(4.08695417599994,12.2,-1.95780579800001));
#351213=CARTESIAN_POINT('Ctrl Pts',(4.08695417599994,5.2,-1.95780579800001));
#351214=CARTESIAN_POINT('Ctrl Pts',(4.08695417599994,2.2,-1.95780579800001));
#351215=CARTESIAN_POINT('Ctrl Pts',(4.08925678399994,12.2,-1.95769973800001));
#351216=CARTESIAN_POINT('Ctrl Pts',(4.08925678399994,5.2,-1.95769973800001));
#351217=CARTESIAN_POINT('Ctrl Pts',(4.08925678399994,2.2,-1.95769973800001));
#351218=CARTESIAN_POINT('Ctrl Pts',(4.09156300299994,12.2,-1.95759102500002));
#351219=CARTESIAN_POINT('Ctrl Pts',(4.09156300299994,5.2,-1.95759102500002));
#351220=CARTESIAN_POINT('Ctrl Pts',(4.09156300299994,2.2,-1.95759102500002));
#351221=CARTESIAN_POINT('Ctrl Pts',(4.09387282499994,12.2,-1.95747965600002));
#351222=CARTESIAN_POINT('Ctrl Pts',(4.09387282499994,5.2,-1.95747965600002));
#351223=CARTESIAN_POINT('Ctrl Pts',(4.09387282499994,2.2,-1.95747965600002));
#351224=CARTESIAN_POINT('Ctrl Pts',(4.09618624499995,12.2,-1.95736562200001));
#351225=CARTESIAN_POINT('Ctrl Pts',(4.09618624499995,5.2,-1.95736562200001));
#351226=CARTESIAN_POINT('Ctrl Pts',(4.09618624499995,2.2,-1.95736562200001));
#351227=CARTESIAN_POINT('Ctrl Pts',(4.09850325399994,12.2,-1.95724891700001));
#351228=CARTESIAN_POINT('Ctrl Pts',(4.09850325399994,5.2,-1.95724891700001));
#351229=CARTESIAN_POINT('Ctrl Pts',(4.09850325399994,2.2,-1.95724891700001));
#351230=CARTESIAN_POINT('Ctrl Pts',(4.10082384499994,12.2,-1.95712953400001));
#351231=CARTESIAN_POINT('Ctrl Pts',(4.10082384499994,5.2,-1.95712953400001));
#351232=CARTESIAN_POINT('Ctrl Pts',(4.10082384499994,2.2,-1.95712953400001));
#351233=CARTESIAN_POINT('Ctrl Pts',(4.10314801299995,12.2,-1.95700746600001));
#351234=CARTESIAN_POINT('Ctrl Pts',(4.10314801299995,5.2,-1.95700746600001));
#351235=CARTESIAN_POINT('Ctrl Pts',(4.10314801299995,2.2,-1.95700746600001));
#351236=CARTESIAN_POINT('Ctrl Pts',(4.10547574999994,12.2,-1.95688270800002));
#351237=CARTESIAN_POINT('Ctrl Pts',(4.10547574999994,5.2,-1.95688270800002));
#351238=CARTESIAN_POINT('Ctrl Pts',(4.10547574999994,2.2,-1.95688270800002));
#351239=CARTESIAN_POINT('Ctrl Pts',(4.10780704799994,12.2,-1.95675525200001));
#351240=CARTESIAN_POINT('Ctrl Pts',(4.10780704799994,5.2,-1.95675525200001));
#351241=CARTESIAN_POINT('Ctrl Pts',(4.10780704799994,2.2,-1.95675525200001));
#351242=CARTESIAN_POINT('Ctrl Pts',(4.11014190199994,12.2,-1.95662509100002));
#351243=CARTESIAN_POINT('Ctrl Pts',(4.11014190199994,5.2,-1.95662509100002));
#351244=CARTESIAN_POINT('Ctrl Pts',(4.11014190199994,2.2,-1.95662509100002));
#351245=CARTESIAN_POINT('Ctrl Pts',(4.11248030499994,12.2,-1.95649222000001));
#351246=CARTESIAN_POINT('Ctrl Pts',(4.11248030499994,5.2,-1.95649222000001));
#351247=CARTESIAN_POINT('Ctrl Pts',(4.11248030499994,2.2,-1.95649222000001));
#351248=CARTESIAN_POINT('Ctrl Pts',(4.11482224699994,12.2,-1.95635663100001));
#351249=CARTESIAN_POINT('Ctrl Pts',(4.11482224699994,5.2,-1.95635663100001));
#351250=CARTESIAN_POINT('Ctrl Pts',(4.11482224699994,2.2,-1.95635663100001));
#351251=CARTESIAN_POINT('Ctrl Pts',(4.11716772399994,12.2,-1.95621831700001));
#351252=CARTESIAN_POINT('Ctrl Pts',(4.11716772399994,5.2,-1.95621831700001));
#351253=CARTESIAN_POINT('Ctrl Pts',(4.11716772399994,2.2,-1.95621831700001));
#351254=CARTESIAN_POINT('Ctrl Pts',(4.11951672899994,12.2,-1.95607727400001));
#351255=CARTESIAN_POINT('Ctrl Pts',(4.11951672899994,5.2,-1.95607727400001));
#351256=CARTESIAN_POINT('Ctrl Pts',(4.11951672899994,2.2,-1.95607727400001));
#351257=CARTESIAN_POINT('Ctrl Pts',(4.12186925499994,12.2,-1.95593349300001));
#351258=CARTESIAN_POINT('Ctrl Pts',(4.12186925499994,5.2,-1.95593349300001));
#351259=CARTESIAN_POINT('Ctrl Pts',(4.12186925499994,2.2,-1.95593349300001));
#351260=CARTESIAN_POINT('Ctrl Pts',(4.12422529299994,12.2,-1.95578696800002));
#351261=CARTESIAN_POINT('Ctrl Pts',(4.12422529299994,5.2,-1.95578696800002));
#351262=CARTESIAN_POINT('Ctrl Pts',(4.12422529299994,2.2,-1.95578696800002));
#351263=CARTESIAN_POINT('Ctrl Pts',(4.12658483799994,12.2,-1.95563769400001));
#351264=CARTESIAN_POINT('Ctrl Pts',(4.12658483799994,5.2,-1.95563769400001));
#351265=CARTESIAN_POINT('Ctrl Pts',(4.12658483799994,2.2,-1.95563769400001));
#351266=CARTESIAN_POINT('Ctrl Pts',(4.12894788199995,12.2,-1.95548566200001));
#351267=CARTESIAN_POINT('Ctrl Pts',(4.12894788199995,5.2,-1.95548566200001));
#351268=CARTESIAN_POINT('Ctrl Pts',(4.12894788199995,2.2,-1.95548566200001));
#351269=CARTESIAN_POINT('Ctrl Pts',(4.13131441899994,12.2,-1.95533086900001));
#351270=CARTESIAN_POINT('Ctrl Pts',(4.13131441899994,5.2,-1.95533086900001));
#351271=CARTESIAN_POINT('Ctrl Pts',(4.13131441899994,2.2,-1.95533086900001));
#351272=CARTESIAN_POINT('Ctrl Pts',(4.13368444199994,12.2,-1.95517330500001));
#351273=CARTESIAN_POINT('Ctrl Pts',(4.13368444199994,5.2,-1.95517330500001));
#351274=CARTESIAN_POINT('Ctrl Pts',(4.13368444199994,2.2,-1.95517330500001));
#351275=CARTESIAN_POINT('Ctrl Pts',(4.13605794499994,12.2,-1.95501296600002));
#351276=CARTESIAN_POINT('Ctrl Pts',(4.13605794499994,5.2,-1.95501296600002));
#351277=CARTESIAN_POINT('Ctrl Pts',(4.13605794499994,2.2,-1.95501296600002));
#351278=CARTESIAN_POINT('Ctrl Pts',(4.13843491799994,12.2,-1.95484984400002));
#351279=CARTESIAN_POINT('Ctrl Pts',(4.13843491799994,5.2,-1.95484984400002));
#351280=CARTESIAN_POINT('Ctrl Pts',(4.13843491799994,2.2,-1.95484984400002));
#351281=CARTESIAN_POINT('Ctrl Pts',(4.14081535599994,12.2,-1.95468393300001));
#351282=CARTESIAN_POINT('Ctrl Pts',(4.14081535599994,5.2,-1.95468393300001));
#351283=CARTESIAN_POINT('Ctrl Pts',(4.14081535599994,2.2,-1.95468393300001));
#351284=CARTESIAN_POINT('Ctrl Pts',(4.14319925299994,12.2,-1.95451522700001));
#351285=CARTESIAN_POINT('Ctrl Pts',(4.14319925299994,5.2,-1.95451522700001));
#351286=CARTESIAN_POINT('Ctrl Pts',(4.14319925299994,2.2,-1.95451522700001));
#351287=CARTESIAN_POINT('Ctrl Pts',(4.14558659999994,12.2,-1.95434372100001));
#351288=CARTESIAN_POINT('Ctrl Pts',(4.14558659999994,5.2,-1.95434372100001));
#351289=CARTESIAN_POINT('Ctrl Pts',(4.14558659999994,2.2,-1.95434372100001));
#351290=CARTESIAN_POINT('Ctrl Pts',(4.14797739099994,12.2,-1.95416940600001));
#351291=CARTESIAN_POINT('Ctrl Pts',(4.14797739099994,5.2,-1.95416940600001));
#351292=CARTESIAN_POINT('Ctrl Pts',(4.14797739099994,2.2,-1.95416940600001));
#351293=CARTESIAN_POINT('Ctrl Pts',(4.15037161999994,12.2,-1.95399227800001));
#351294=CARTESIAN_POINT('Ctrl Pts',(4.15037161999994,5.2,-1.95399227800001));
#351295=CARTESIAN_POINT('Ctrl Pts',(4.15037161999994,2.2,-1.95399227800001));
#351296=CARTESIAN_POINT('Ctrl Pts',(4.15276927899995,12.2,-1.95381233000001));
#351297=CARTESIAN_POINT('Ctrl Pts',(4.15276927899995,5.2,-1.95381233000001));
#351298=CARTESIAN_POINT('Ctrl Pts',(4.15276927899995,2.2,-1.95381233000001));
#351299=CARTESIAN_POINT('Ctrl Pts',(4.15517036099994,12.2,-1.95362955500002));
#351300=CARTESIAN_POINT('Ctrl Pts',(4.15517036099994,5.2,-1.95362955500002));
#351301=CARTESIAN_POINT('Ctrl Pts',(4.15517036099994,2.2,-1.95362955500002));
#351302=CARTESIAN_POINT('Ctrl Pts',(4.15757485899994,12.2,-1.95344394600002));
#351303=CARTESIAN_POINT('Ctrl Pts',(4.15757485899994,5.2,-1.95344394600002));
#351304=CARTESIAN_POINT('Ctrl Pts',(4.15757485899994,2.2,-1.95344394600002));
#351305=CARTESIAN_POINT('Ctrl Pts',(4.15998276699994,12.2,-1.95325549900002));
#351306=CARTESIAN_POINT('Ctrl Pts',(4.15998276699994,5.2,-1.95325549900002));
#351307=CARTESIAN_POINT('Ctrl Pts',(4.15998276699994,2.2,-1.95325549900002));
#351308=CARTESIAN_POINT('Ctrl Pts',(4.16239407799995,12.2,-1.95306420700001));
#351309=CARTESIAN_POINT('Ctrl Pts',(4.16239407799995,5.2,-1.95306420700001));
#351310=CARTESIAN_POINT('Ctrl Pts',(4.16239407799995,2.2,-1.95306420700001));
#351311=CARTESIAN_POINT('Ctrl Pts',(4.16480878399994,12.2,-1.95287006400001));
#351312=CARTESIAN_POINT('Ctrl Pts',(4.16480878399994,5.2,-1.95287006400001));
#351313=CARTESIAN_POINT('Ctrl Pts',(4.16480878399994,2.2,-1.95287006400001));
#351314=CARTESIAN_POINT('Ctrl Pts',(4.16722687799994,12.2,-1.95267306200002));
#351315=CARTESIAN_POINT('Ctrl Pts',(4.16722687799994,5.2,-1.95267306200002));
#351316=CARTESIAN_POINT('Ctrl Pts',(4.16722687799994,2.2,-1.95267306200002));
#351317=CARTESIAN_POINT('Ctrl Pts',(4.16964835399994,12.2,-1.95247319700002));
#351318=CARTESIAN_POINT('Ctrl Pts',(4.16964835399994,5.2,-1.95247319700002));
#351319=CARTESIAN_POINT('Ctrl Pts',(4.16964835399994,2.2,-1.95247319700002));
#351320=CARTESIAN_POINT('Ctrl Pts',(4.17207320499995,12.2,-1.95227046200001));
#351321=CARTESIAN_POINT('Ctrl Pts',(4.17207320499995,5.2,-1.95227046200001));
#351322=CARTESIAN_POINT('Ctrl Pts',(4.17207320499995,2.2,-1.95227046200001));
#351323=CARTESIAN_POINT('Ctrl Pts',(4.17450142499994,12.2,-1.95206485100002));
#351324=CARTESIAN_POINT('Ctrl Pts',(4.17450142499994,5.2,-1.95206485100002));
#351325=CARTESIAN_POINT('Ctrl Pts',(4.17450142499994,2.2,-1.95206485100002));
#351326=CARTESIAN_POINT('Ctrl Pts',(4.17693300399994,12.2,-1.95185635800001));
#351327=CARTESIAN_POINT('Ctrl Pts',(4.17693300399994,5.2,-1.95185635800001));
#351328=CARTESIAN_POINT('Ctrl Pts',(4.17693300399994,2.2,-1.95185635800001));
#351329=CARTESIAN_POINT('Ctrl Pts',(4.17936793799994,12.2,-1.95164497700001));
#351330=CARTESIAN_POINT('Ctrl Pts',(4.17936793799994,5.2,-1.95164497700001));
#351331=CARTESIAN_POINT('Ctrl Pts',(4.17936793799994,2.2,-1.95164497700001));
#351332=CARTESIAN_POINT('Ctrl Pts',(4.18180621899995,12.2,-1.95143070000002));
#351333=CARTESIAN_POINT('Ctrl Pts',(4.18180621899995,5.2,-1.95143070000002));
#351334=CARTESIAN_POINT('Ctrl Pts',(4.18180621899995,2.2,-1.95143070000002));
#351335=CARTESIAN_POINT('Ctrl Pts',(4.18424783999995,12.2,-1.95121352400002));
#351336=CARTESIAN_POINT('Ctrl Pts',(4.18424783999995,5.2,-1.95121352400002));
#351337=CARTESIAN_POINT('Ctrl Pts',(4.18424783999995,2.2,-1.95121352400002));
#351338=CARTESIAN_POINT('Ctrl Pts',(4.18669279499994,12.2,-1.95099344200001));
#351339=CARTESIAN_POINT('Ctrl Pts',(4.18669279499994,5.2,-1.95099344200001));
#351340=CARTESIAN_POINT('Ctrl Pts',(4.18669279499994,2.2,-1.95099344200001));
#351341=CARTESIAN_POINT('Ctrl Pts',(4.18914107499995,12.2,-1.95077044700001));
#351342=CARTESIAN_POINT('Ctrl Pts',(4.18914107499995,5.2,-1.95077044700001));
#351343=CARTESIAN_POINT('Ctrl Pts',(4.18914107499995,2.2,-1.95077044700001));
#351344=CARTESIAN_POINT('Ctrl Pts',(4.19159267499994,12.2,-1.95054453300001));
#351345=CARTESIAN_POINT('Ctrl Pts',(4.19159267499994,5.2,-1.95054453300001));
#351346=CARTESIAN_POINT('Ctrl Pts',(4.19159267499994,2.2,-1.95054453300001));
#351347=CARTESIAN_POINT('Ctrl Pts',(4.19404758699994,12.2,-1.95031569600001));
#351348=CARTESIAN_POINT('Ctrl Pts',(4.19404758699994,5.2,-1.95031569600001));
#351349=CARTESIAN_POINT('Ctrl Pts',(4.19404758699994,2.2,-1.95031569600001));
#351350=CARTESIAN_POINT('Ctrl Pts',(4.19650580499995,12.2,-1.95008392700001));
#351351=CARTESIAN_POINT('Ctrl Pts',(4.19650580499995,5.2,-1.95008392700001));
#351352=CARTESIAN_POINT('Ctrl Pts',(4.19650580499995,2.2,-1.95008392700001));
#351353=CARTESIAN_POINT('Ctrl Pts',(4.19896732099994,12.2,-1.94984922200002));
#351354=CARTESIAN_POINT('Ctrl Pts',(4.19896732099994,5.2,-1.94984922200002));
#351355=CARTESIAN_POINT('Ctrl Pts',(4.19896732099994,2.2,-1.94984922200002));
#351356=CARTESIAN_POINT('Ctrl Pts',(4.20143212999994,12.2,-1.94961157500002));
#351357=CARTESIAN_POINT('Ctrl Pts',(4.20143212999994,5.2,-1.94961157500002));
#351358=CARTESIAN_POINT('Ctrl Pts',(4.20143212999994,2.2,-1.94961157500002));
#351359=CARTESIAN_POINT('Ctrl Pts',(4.20390022299994,12.2,-1.94937098000001));
#351360=CARTESIAN_POINT('Ctrl Pts',(4.20390022299994,5.2,-1.94937098000001));
#351361=CARTESIAN_POINT('Ctrl Pts',(4.20390022299994,2.2,-1.94937098000001));
#351362=CARTESIAN_POINT('Ctrl Pts',(4.20637159399995,12.2,-1.94912743000001));
#351363=CARTESIAN_POINT('Ctrl Pts',(4.20637159399995,5.2,-1.94912743000001));
#351364=CARTESIAN_POINT('Ctrl Pts',(4.20637159399995,2.2,-1.94912743000001));
#351365=CARTESIAN_POINT('Ctrl Pts',(4.20884623499994,12.2,-1.94888092100001));
#351366=CARTESIAN_POINT('Ctrl Pts',(4.20884623499994,5.2,-1.94888092100001));
#351367=CARTESIAN_POINT('Ctrl Pts',(4.20884623499994,2.2,-1.94888092100001));
#351368=CARTESIAN_POINT('Ctrl Pts',(4.21132414099994,12.2,-1.94863144500002));
#351369=CARTESIAN_POINT('Ctrl Pts',(4.21132414099994,5.2,-1.94863144500002));
#351370=CARTESIAN_POINT('Ctrl Pts',(4.21132414099994,2.2,-1.94863144500002));
#351371=CARTESIAN_POINT('Ctrl Pts',(4.21380530299994,12.2,-1.94837899800001));
#351372=CARTESIAN_POINT('Ctrl Pts',(4.21380530299994,5.2,-1.94837899800001));
#351373=CARTESIAN_POINT('Ctrl Pts',(4.21380530299994,2.2,-1.94837899800001));
#351374=CARTESIAN_POINT('Ctrl Pts',(4.21628971599994,12.2,-1.94812357300002));
#351375=CARTESIAN_POINT('Ctrl Pts',(4.21628971599994,5.2,-1.94812357300002));
#351376=CARTESIAN_POINT('Ctrl Pts',(4.21628971599994,2.2,-1.94812357300002));
#351377=CARTESIAN_POINT('Ctrl Pts',(4.21877737199994,12.2,-1.94786516400002));
#351378=CARTESIAN_POINT('Ctrl Pts',(4.21877737199994,5.2,-1.94786516400002));
#351379=CARTESIAN_POINT('Ctrl Pts',(4.21877737199994,2.2,-1.94786516400002));
#351380=CARTESIAN_POINT('Ctrl Pts',(4.22126826399994,12.2,-1.94760376700001));
#351381=CARTESIAN_POINT('Ctrl Pts',(4.22126826399994,5.2,-1.94760376700001));
#351382=CARTESIAN_POINT('Ctrl Pts',(4.22126826399994,2.2,-1.94760376700001));
#351383=CARTESIAN_POINT('Ctrl Pts',(4.22376238699994,12.2,-1.94733937400001));
#351384=CARTESIAN_POINT('Ctrl Pts',(4.22376238699994,5.2,-1.94733937400001));
#351385=CARTESIAN_POINT('Ctrl Pts',(4.22376238699994,2.2,-1.94733937400001));
#351386=CARTESIAN_POINT('Ctrl Pts',(4.22625973099994,12.2,-1.94707198100001));
#351387=CARTESIAN_POINT('Ctrl Pts',(4.22625973099994,5.2,-1.94707198100001));
#351388=CARTESIAN_POINT('Ctrl Pts',(4.22625973099994,2.2,-1.94707198100001));
#351389=CARTESIAN_POINT('Ctrl Pts',(4.22876029099994,12.2,-1.94680158100001));
#351390=CARTESIAN_POINT('Ctrl Pts',(4.22876029099994,5.2,-1.94680158100001));
#351391=CARTESIAN_POINT('Ctrl Pts',(4.22876029099994,2.2,-1.94680158100001));
#351392=CARTESIAN_POINT('Ctrl Pts',(4.23126405899994,12.2,-1.94652816800001));
#351393=CARTESIAN_POINT('Ctrl Pts',(4.23126405899994,5.2,-1.94652816800001));
#351394=CARTESIAN_POINT('Ctrl Pts',(4.23126405899994,2.2,-1.94652816800001));
#351395=CARTESIAN_POINT('Ctrl Pts',(4.23377102899994,12.2,-1.94625173800001));
#351396=CARTESIAN_POINT('Ctrl Pts',(4.23377102899994,5.2,-1.94625173800001));
#351397=CARTESIAN_POINT('Ctrl Pts',(4.23377102899994,2.2,-1.94625173800001));
#351398=CARTESIAN_POINT('Ctrl Pts',(4.23628119499995,12.2,-1.94597228400001));
#351399=CARTESIAN_POINT('Ctrl Pts',(4.23628119499995,5.2,-1.94597228400001));
#351400=CARTESIAN_POINT('Ctrl Pts',(4.23628119499995,2.2,-1.94597228400001));
#351401=CARTESIAN_POINT('Ctrl Pts',(4.23879454799994,12.2,-1.94568980000001));
#351402=CARTESIAN_POINT('Ctrl Pts',(4.23879454799994,5.2,-1.94568980000001));
#351403=CARTESIAN_POINT('Ctrl Pts',(4.23879454799994,2.2,-1.94568980000001));
#351404=CARTESIAN_POINT('Ctrl Pts',(4.24131108199994,12.2,-1.94540428100002));
#351405=CARTESIAN_POINT('Ctrl Pts',(4.24131108199994,5.2,-1.94540428100002));
#351406=CARTESIAN_POINT('Ctrl Pts',(4.24131108199994,2.2,-1.94540428100002));
#351407=CARTESIAN_POINT('Ctrl Pts',(4.24383078999994,12.2,-1.94511572200001));
#351408=CARTESIAN_POINT('Ctrl Pts',(4.24383078999994,5.2,-1.94511572200001));
#351409=CARTESIAN_POINT('Ctrl Pts',(4.24383078999994,2.2,-1.94511572200001));
#351410=CARTESIAN_POINT('Ctrl Pts',(4.24635366599994,12.2,-1.94482411700001));
#351411=CARTESIAN_POINT('Ctrl Pts',(4.24635366599994,5.2,-1.94482411700001));
#351412=CARTESIAN_POINT('Ctrl Pts',(4.24635366599994,2.2,-1.94482411700001));
#351413=CARTESIAN_POINT('Ctrl Pts',(4.24887970099994,12.2,-1.94452945900002));
#351414=CARTESIAN_POINT('Ctrl Pts',(4.24887970099994,5.2,-1.94452945900002));
#351415=CARTESIAN_POINT('Ctrl Pts',(4.24887970099994,2.2,-1.94452945900002));
#351416=CARTESIAN_POINT('Ctrl Pts',(4.25140889099994,12.2,-1.94423174300002));
#351417=CARTESIAN_POINT('Ctrl Pts',(4.25140889099994,5.2,-1.94423174300002));
#351418=CARTESIAN_POINT('Ctrl Pts',(4.25140889099994,2.2,-1.94423174300002));
#351419=CARTESIAN_POINT('Ctrl Pts',(4.25394122599995,12.2,-1.94393096500002));
#351420=CARTESIAN_POINT('Ctrl Pts',(4.25394122599995,5.2,-1.94393096500002));
#351421=CARTESIAN_POINT('Ctrl Pts',(4.25394122599995,2.2,-1.94393096500002));
#351422=CARTESIAN_POINT('Ctrl Pts',(4.25647670199994,12.2,-1.94362711800002));
#351423=CARTESIAN_POINT('Ctrl Pts',(4.25647670199994,5.2,-1.94362711800002));
#351424=CARTESIAN_POINT('Ctrl Pts',(4.25647670199994,2.2,-1.94362711800002));
#351425=CARTESIAN_POINT('Ctrl Pts',(4.25901530899994,12.2,-1.94332019600001));
#351426=CARTESIAN_POINT('Ctrl Pts',(4.25901530899994,5.2,-1.94332019600001));
#351427=CARTESIAN_POINT('Ctrl Pts',(4.25901530899994,2.2,-1.94332019600001));
#351428=CARTESIAN_POINT('Ctrl Pts',(4.26155704199994,12.2,-1.94301019400001));
#351429=CARTESIAN_POINT('Ctrl Pts',(4.26155704199994,5.2,-1.94301019400001));
#351430=CARTESIAN_POINT('Ctrl Pts',(4.26155704199994,2.2,-1.94301019400001));
#351431=CARTESIAN_POINT('Ctrl Pts',(4.26410189499994,12.2,-1.94269710600001));
#351432=CARTESIAN_POINT('Ctrl Pts',(4.26410189499994,5.2,-1.94269710600001));
#351433=CARTESIAN_POINT('Ctrl Pts',(4.26410189499994,2.2,-1.94269710600001));
#351434=CARTESIAN_POINT('Ctrl Pts',(4.26664985899994,12.2,-1.94238092900001));
#351435=CARTESIAN_POINT('Ctrl Pts',(4.26664985899994,5.2,-1.94238092900001));
#351436=CARTESIAN_POINT('Ctrl Pts',(4.26664985899994,2.2,-1.94238092900001));
#351437=CARTESIAN_POINT('Ctrl Pts',(4.26920092799994,12.2,-1.94206165400002));
#351438=CARTESIAN_POINT('Ctrl Pts',(4.26920092799994,5.2,-1.94206165400002));
#351439=CARTESIAN_POINT('Ctrl Pts',(4.26920092799994,2.2,-1.94206165400002));
#351440=CARTESIAN_POINT('Ctrl Pts',(4.27175509499994,12.2,-1.94173927700001));
#351441=CARTESIAN_POINT('Ctrl Pts',(4.27175509499994,5.2,-1.94173927700001));
#351442=CARTESIAN_POINT('Ctrl Pts',(4.27175509499994,2.2,-1.94173927700001));
#351443=CARTESIAN_POINT('Ctrl Pts',(4.27431235399994,12.2,-1.94141379400001));
#351444=CARTESIAN_POINT('Ctrl Pts',(4.27431235399994,5.2,-1.94141379400001));
#351445=CARTESIAN_POINT('Ctrl Pts',(4.27431235399994,2.2,-1.94141379400001));
#351446=CARTESIAN_POINT('Ctrl Pts',(4.27687269699994,12.2,-1.94108519700002));
#351447=CARTESIAN_POINT('Ctrl Pts',(4.27687269699994,5.2,-1.94108519700002));
#351448=CARTESIAN_POINT('Ctrl Pts',(4.27687269699994,2.2,-1.94108519700002));
#351449=CARTESIAN_POINT('Ctrl Pts',(4.27943611799994,12.2,-1.94075348200001));
#351450=CARTESIAN_POINT('Ctrl Pts',(4.27943611799994,5.2,-1.94075348200001));
#351451=CARTESIAN_POINT('Ctrl Pts',(4.27943611799994,2.2,-1.94075348200001));
#351452=CARTESIAN_POINT('Ctrl Pts',(4.28200260999995,12.2,-1.94041864400001));
#351453=CARTESIAN_POINT('Ctrl Pts',(4.28200260999995,5.2,-1.94041864400001));
#351454=CARTESIAN_POINT('Ctrl Pts',(4.28200260999995,2.2,-1.94041864400001));
#351455=CARTESIAN_POINT('Ctrl Pts',(4.28457216599995,12.2,-1.94008067700001));
#351456=CARTESIAN_POINT('Ctrl Pts',(4.28457216599995,5.2,-1.94008067700001));
#351457=CARTESIAN_POINT('Ctrl Pts',(4.28457216599995,2.2,-1.94008067700001));
#351458=CARTESIAN_POINT('Ctrl Pts',(4.28714477699994,12.2,-1.93973957500001));
#351459=CARTESIAN_POINT('Ctrl Pts',(4.28714477699994,5.2,-1.93973957500001));
#351460=CARTESIAN_POINT('Ctrl Pts',(4.28714477699994,2.2,-1.93973957500001));
#351461=CARTESIAN_POINT('Ctrl Pts',(4.28972043899994,12.2,-1.93939533400002));
#351462=CARTESIAN_POINT('Ctrl Pts',(4.28972043899994,5.2,-1.93939533400002));
#351463=CARTESIAN_POINT('Ctrl Pts',(4.28972043899994,2.2,-1.93939533400002));
#351464=CARTESIAN_POINT('Ctrl Pts',(4.29229914299994,12.2,-1.93904794600002));
#351465=CARTESIAN_POINT('Ctrl Pts',(4.29229914299994,5.2,-1.93904794600002));
#351466=CARTESIAN_POINT('Ctrl Pts',(4.29229914299994,2.2,-1.93904794600002));
#351467=CARTESIAN_POINT('Ctrl Pts',(4.29488088199994,12.2,-1.93869740900002));
#351468=CARTESIAN_POINT('Ctrl Pts',(4.29488088199994,5.2,-1.93869740900002));
#351469=CARTESIAN_POINT('Ctrl Pts',(4.29488088199994,2.2,-1.93869740900002));
#351470=CARTESIAN_POINT('Ctrl Pts',(4.29746564899994,12.2,-1.93834371400001));
#351471=CARTESIAN_POINT('Ctrl Pts',(4.29746564899994,5.2,-1.93834371400001));
#351472=CARTESIAN_POINT('Ctrl Pts',(4.29746564899994,2.2,-1.93834371400001));
#351473=CARTESIAN_POINT('Ctrl Pts',(4.30005343899994,12.2,-1.93798685700001));
#351474=CARTESIAN_POINT('Ctrl Pts',(4.30005343899994,5.2,-1.93798685700001));
#351475=CARTESIAN_POINT('Ctrl Pts',(4.30005343899994,2.2,-1.93798685700001));
#351476=CARTESIAN_POINT('Ctrl Pts',(4.30264424499994,12.2,-1.93762683600001));
#351477=CARTESIAN_POINT('Ctrl Pts',(4.30264424499994,5.2,-1.93762683600001));
#351478=CARTESIAN_POINT('Ctrl Pts',(4.30264424499994,2.2,-1.93762683600001));
#351479=CARTESIAN_POINT('Ctrl Pts',(4.30523806099994,12.2,-1.93726364300002));
#351480=CARTESIAN_POINT('Ctrl Pts',(4.30523806099994,5.2,-1.93726364300002));
#351481=CARTESIAN_POINT('Ctrl Pts',(4.30523806099994,2.2,-1.93726364300002));
#351482=CARTESIAN_POINT('Ctrl Pts',(4.30783487999994,12.2,-1.93689727500002));
#351483=CARTESIAN_POINT('Ctrl Pts',(4.30783487999994,5.2,-1.93689727500002));
#351484=CARTESIAN_POINT('Ctrl Pts',(4.30783487999994,2.2,-1.93689727500002));
#351485=CARTESIAN_POINT('Ctrl Pts',(4.31043469599994,12.2,-1.93652772600001));
#351486=CARTESIAN_POINT('Ctrl Pts',(4.31043469599994,5.2,-1.93652772600001));
#351487=CARTESIAN_POINT('Ctrl Pts',(4.31043469599994,2.2,-1.93652772600001));
#351488=CARTESIAN_POINT('Ctrl Pts',(4.31303749999994,12.2,-1.93615499100002));
#351489=CARTESIAN_POINT('Ctrl Pts',(4.31303749999994,5.2,-1.93615499100002));
#351490=CARTESIAN_POINT('Ctrl Pts',(4.31303749999994,2.2,-1.93615499100002));
#351491=CARTESIAN_POINT('Ctrl Pts',(4.31564328599995,12.2,-1.93577906200002));
#351492=CARTESIAN_POINT('Ctrl Pts',(4.31564328599995,5.2,-1.93577906200002));
#351493=CARTESIAN_POINT('Ctrl Pts',(4.31564328599995,2.2,-1.93577906200002));
#351494=CARTESIAN_POINT('Ctrl Pts',(4.31825204199995,12.2,-1.93539993400002));
#351495=CARTESIAN_POINT('Ctrl Pts',(4.31825204199995,5.2,-1.93539993400002));
#351496=CARTESIAN_POINT('Ctrl Pts',(4.31825204199995,2.2,-1.93539993400002));
#351497=CARTESIAN_POINT('Ctrl Pts',(4.32086376199995,12.2,-1.93501760000002));
#351498=CARTESIAN_POINT('Ctrl Pts',(4.32086376199995,5.2,-1.93501760000002));
#351499=CARTESIAN_POINT('Ctrl Pts',(4.32086376199995,2.2,-1.93501760000002));
#351500=CARTESIAN_POINT('Ctrl Pts',(4.32347843899994,12.2,-1.93463205400001));
#351501=CARTESIAN_POINT('Ctrl Pts',(4.32347843899994,5.2,-1.93463205400001));
#351502=CARTESIAN_POINT('Ctrl Pts',(4.32347843899994,2.2,-1.93463205400001));
#351503=CARTESIAN_POINT('Ctrl Pts',(4.32609606399994,12.2,-1.93424329200001));
#351504=CARTESIAN_POINT('Ctrl Pts',(4.32609606399994,5.2,-1.93424329200001));
#351505=CARTESIAN_POINT('Ctrl Pts',(4.32609606399994,2.2,-1.93424329200001));
#351506=CARTESIAN_POINT('Ctrl Pts',(4.32871663299994,12.2,-1.93385130900001));
#351507=CARTESIAN_POINT('Ctrl Pts',(4.32871663299994,5.2,-1.93385130900001));
#351508=CARTESIAN_POINT('Ctrl Pts',(4.32871663299994,2.2,-1.93385130900001));
#351509=CARTESIAN_POINT('Ctrl Pts',(4.33134014299995,12.2,-1.93345610400002));
#351510=CARTESIAN_POINT('Ctrl Pts',(4.33134014299995,5.2,-1.93345610400002));
#351511=CARTESIAN_POINT('Ctrl Pts',(4.33134014299995,2.2,-1.93345610400002));
#351512=CARTESIAN_POINT('Ctrl Pts',(4.33396659199994,12.2,-1.93305767500001));
#351513=CARTESIAN_POINT('Ctrl Pts',(4.33396659199994,5.2,-1.93305767500001));
#351514=CARTESIAN_POINT('Ctrl Pts',(4.33396659199994,2.2,-1.93305767500001));
#351515=CARTESIAN_POINT('Ctrl Pts',(4.33607010199994,12.2,-1.93273635200002));
#351516=CARTESIAN_POINT('Ctrl Pts',(4.33607010199994,5.2,-1.93273635200002));
#351517=CARTESIAN_POINT('Ctrl Pts',(4.33607010199994,2.2,-1.93273635200002));
#351518=CARTESIAN_POINT('Ctrl Pts',(4.33764905499994,12.2,-1.93249390800001));
#351519=CARTESIAN_POINT('Ctrl Pts',(4.33764905499994,5.2,-1.93249390800001));
#351520=CARTESIAN_POINT('Ctrl Pts',(4.33764905499994,2.2,-1.93249390800001));
#351521=CARTESIAN_POINT('Ctrl Pts',(4.33870227899994,12.2,-1.93233163400001));
#351522=CARTESIAN_POINT('Ctrl Pts',(4.33870227899994,5.2,-1.93233163400001));
#351523=CARTESIAN_POINT('Ctrl Pts',(4.33870227899994,2.2,-1.93233163400001));
#351524=CARTESIAN_POINT('Ctrl Pts',(4.33922903699994,12.2,-1.93225033600001));
#351525=CARTESIAN_POINT('Ctrl Pts',(4.33922903699994,5.2,-1.93225033600001));
#351526=CARTESIAN_POINT('Ctrl Pts',(4.33922903699994,2.2,-1.93225033600001));
#351527=CARTESIAN_POINT('Origin',(-5.66300478732629E-14,15.2,-1.77635683940025E-14));
#351528=CARTESIAN_POINT('',(2.89509244999994,2.2,-2.18152806500001));
#351529=CARTESIAN_POINT('Origin',(3.18954822099994,15.2,-2.40340820900002));
#351530=CARTESIAN_POINT('',(3.18958920499994,12.2,-2.40343909200002));
#351531=CARTESIAN_POINT('Ctrl Pts',(3.57864508499994,12.2,-3.12342750100001));
#351532=CARTESIAN_POINT('Ctrl Pts',(3.57864508499994,5.2,-3.12342750100001));
#351533=CARTESIAN_POINT('Ctrl Pts',(3.57864508499994,2.2,-3.12342750100001));
#351534=CARTESIAN_POINT('Ctrl Pts',(3.57849719899995,12.2,-3.12291543200002));
#351535=CARTESIAN_POINT('Ctrl Pts',(3.57849719899995,5.2,-3.12291543200002));
#351536=CARTESIAN_POINT('Ctrl Pts',(3.57849719899995,2.2,-3.12291543200002));
#351537=CARTESIAN_POINT('Ctrl Pts',(3.57820125899994,12.2,-3.12189169800002));
#351538=CARTESIAN_POINT('Ctrl Pts',(3.57820125899994,5.2,-3.12189169800002));
#351539=CARTESIAN_POINT('Ctrl Pts',(3.57820125899994,2.2,-3.12189169800002));
#351540=CARTESIAN_POINT('Ctrl Pts',(3.57775684299994,12.2,-3.12035730300002));
#351541=CARTESIAN_POINT('Ctrl Pts',(3.57775684299994,5.2,-3.12035730300002));
#351542=CARTESIAN_POINT('Ctrl Pts',(3.57775684299994,2.2,-3.12035730300002));
#351543=CARTESIAN_POINT('Ctrl Pts',(3.57716327299994,12.2,-3.11831385700001));
#351544=CARTESIAN_POINT('Ctrl Pts',(3.57716327299994,5.2,-3.11831385700001));
#351545=CARTESIAN_POINT('Ctrl Pts',(3.57716327299994,2.2,-3.11831385700001));
#351546=CARTESIAN_POINT('Ctrl Pts',(3.57641962299994,12.2,-3.11576357000002));
#351547=CARTESIAN_POINT('Ctrl Pts',(3.57641962299994,5.2,-3.11576357000002));
#351548=CARTESIAN_POINT('Ctrl Pts',(3.57641962299994,2.2,-3.11576357000002));
#351549=CARTESIAN_POINT('Ctrl Pts',(3.57567428399994,12.2,-3.11321730600001));
#351550=CARTESIAN_POINT('Ctrl Pts',(3.57567428399994,5.2,-3.11321730600001));
#351551=CARTESIAN_POINT('Ctrl Pts',(3.57567428399994,2.2,-3.11321730600001));
#351552=CARTESIAN_POINT('Ctrl Pts',(3.57492725899994,12.2,-3.11067506500001));
#351553=CARTESIAN_POINT('Ctrl Pts',(3.57492725899994,5.2,-3.11067506500001));
#351554=CARTESIAN_POINT('Ctrl Pts',(3.57492725899994,2.2,-3.11067506500001));
#351555=CARTESIAN_POINT('Ctrl Pts',(3.57417855099994,12.2,-3.10813685000001));
#351556=CARTESIAN_POINT('Ctrl Pts',(3.57417855099994,5.2,-3.10813685000001));
#351557=CARTESIAN_POINT('Ctrl Pts',(3.57417855099994,2.2,-3.10813685000001));
#351558=CARTESIAN_POINT('Ctrl Pts',(3.57342816699994,12.2,-3.10560266400001));
#351559=CARTESIAN_POINT('Ctrl Pts',(3.57342816699994,5.2,-3.10560266400001));
#351560=CARTESIAN_POINT('Ctrl Pts',(3.57342816699994,2.2,-3.10560266400001));
#351561=CARTESIAN_POINT('Ctrl Pts',(3.57267611199994,12.2,-3.10307251000001));
#351562=CARTESIAN_POINT('Ctrl Pts',(3.57267611199994,5.2,-3.10307251000001));
#351563=CARTESIAN_POINT('Ctrl Pts',(3.57267611199994,2.2,-3.10307251000001));
#351564=CARTESIAN_POINT('Ctrl Pts',(3.57192239599994,12.2,-3.10054639500001));
#351565=CARTESIAN_POINT('Ctrl Pts',(3.57192239599994,5.2,-3.10054639500001));
#351566=CARTESIAN_POINT('Ctrl Pts',(3.57192239599994,2.2,-3.10054639500001));
#351567=CARTESIAN_POINT('Ctrl Pts',(3.57116702699994,12.2,-3.09802432100001));
#351568=CARTESIAN_POINT('Ctrl Pts',(3.57116702699994,5.2,-3.09802432100001));
#351569=CARTESIAN_POINT('Ctrl Pts',(3.57116702699994,2.2,-3.09802432100001));
#351570=CARTESIAN_POINT('Ctrl Pts',(3.57041001599994,12.2,-3.09550629400002));
#351571=CARTESIAN_POINT('Ctrl Pts',(3.57041001599994,5.2,-3.09550629400002));
#351572=CARTESIAN_POINT('Ctrl Pts',(3.57041001599994,2.2,-3.09550629400002));
#351573=CARTESIAN_POINT('Ctrl Pts',(3.56965137099994,12.2,-3.09299232000001));
#351574=CARTESIAN_POINT('Ctrl Pts',(3.56965137099994,5.2,-3.09299232000001));
#351575=CARTESIAN_POINT('Ctrl Pts',(3.56965137099994,2.2,-3.09299232000001));
#351576=CARTESIAN_POINT('Ctrl Pts',(3.56889110299994,12.2,-3.09048240200001));
#351577=CARTESIAN_POINT('Ctrl Pts',(3.56889110299994,5.2,-3.09048240200001));
#351578=CARTESIAN_POINT('Ctrl Pts',(3.56889110299994,2.2,-3.09048240200001));
#351579=CARTESIAN_POINT('Ctrl Pts',(3.56812921699994,12.2,-3.08797654500002));
#351580=CARTESIAN_POINT('Ctrl Pts',(3.56812921699994,5.2,-3.08797654500002));
#351581=CARTESIAN_POINT('Ctrl Pts',(3.56812921699994,2.2,-3.08797654500002));
#351582=CARTESIAN_POINT('Ctrl Pts',(3.56736572099994,12.2,-3.08547475200001));
#351583=CARTESIAN_POINT('Ctrl Pts',(3.56736572099994,5.2,-3.08547475200001));
#351584=CARTESIAN_POINT('Ctrl Pts',(3.56736572099994,2.2,-3.08547475200001));
#351585=CARTESIAN_POINT('Ctrl Pts',(3.56660062199994,12.2,-3.08297702800001));
#351586=CARTESIAN_POINT('Ctrl Pts',(3.56660062199994,5.2,-3.08297702800001));
#351587=CARTESIAN_POINT('Ctrl Pts',(3.56660062199994,2.2,-3.08297702800001));
#351588=CARTESIAN_POINT('Ctrl Pts',(3.56583392699994,12.2,-3.08048337600002));
#351589=CARTESIAN_POINT('Ctrl Pts',(3.56583392699994,5.2,-3.08048337600002));
#351590=CARTESIAN_POINT('Ctrl Pts',(3.56583392699994,2.2,-3.08048337600002));
#351591=CARTESIAN_POINT('Ctrl Pts',(3.56506564299994,12.2,-3.07799380000001));
#351592=CARTESIAN_POINT('Ctrl Pts',(3.56506564299994,5.2,-3.07799380000001));
#351593=CARTESIAN_POINT('Ctrl Pts',(3.56506564299994,2.2,-3.07799380000001));
#351594=CARTESIAN_POINT('Ctrl Pts',(3.56429577799994,12.2,-3.07550830200002));
#351595=CARTESIAN_POINT('Ctrl Pts',(3.56429577799994,5.2,-3.07550830200002));
#351596=CARTESIAN_POINT('Ctrl Pts',(3.56429577799994,2.2,-3.07550830200002));
#351597=CARTESIAN_POINT('Ctrl Pts',(3.56352433899994,12.2,-3.07302688700001));
#351598=CARTESIAN_POINT('Ctrl Pts',(3.56352433899994,5.2,-3.07302688700001));
#351599=CARTESIAN_POINT('Ctrl Pts',(3.56352433899994,2.2,-3.07302688700001));
#351600=CARTESIAN_POINT('Ctrl Pts',(3.56275133299994,12.2,-3.07054956100002));
#351601=CARTESIAN_POINT('Ctrl Pts',(3.56275133299994,5.2,-3.07054956100002));
#351602=CARTESIAN_POINT('Ctrl Pts',(3.56275133299994,2.2,-3.07054956100002));
#351603=CARTESIAN_POINT('Ctrl Pts',(3.56197677199994,12.2,-3.06807632600002));
#351604=CARTESIAN_POINT('Ctrl Pts',(3.56197677199994,5.2,-3.06807632600002));
#351605=CARTESIAN_POINT('Ctrl Pts',(3.56197677199994,2.2,-3.06807632600002));
#351606=CARTESIAN_POINT('Ctrl Pts',(3.56120065999994,12.2,-3.06560718700001));
#351607=CARTESIAN_POINT('Ctrl Pts',(3.56120065999994,5.2,-3.06560718700001));
#351608=CARTESIAN_POINT('Ctrl Pts',(3.56120065999994,2.2,-3.06560718700001));
#351609=CARTESIAN_POINT('Ctrl Pts',(3.56042300699994,12.2,-3.06314214800001));
#351610=CARTESIAN_POINT('Ctrl Pts',(3.56042300699994,5.2,-3.06314214800001));
#351611=CARTESIAN_POINT('Ctrl Pts',(3.56042300699994,2.2,-3.06314214800001));
#351612=CARTESIAN_POINT('Ctrl Pts',(3.55964381999994,12.2,-3.06068121400001));
#351613=CARTESIAN_POINT('Ctrl Pts',(3.55964381999994,5.2,-3.06068121400001));
#351614=CARTESIAN_POINT('Ctrl Pts',(3.55964381999994,2.2,-3.06068121400001));
#351615=CARTESIAN_POINT('Ctrl Pts',(3.55886310799994,12.2,-3.05822438600002));
#351616=CARTESIAN_POINT('Ctrl Pts',(3.55886310799994,5.2,-3.05822438600002));
#351617=CARTESIAN_POINT('Ctrl Pts',(3.55886310799994,2.2,-3.05822438600002));
#351618=CARTESIAN_POINT('Ctrl Pts',(3.55808087699994,12.2,-3.05577167100001));
#351619=CARTESIAN_POINT('Ctrl Pts',(3.55808087699994,5.2,-3.05577167100001));
#351620=CARTESIAN_POINT('Ctrl Pts',(3.55808087699994,2.2,-3.05577167100001));
#351621=CARTESIAN_POINT('Ctrl Pts',(3.55729713599994,12.2,-3.05332307200001));
#351622=CARTESIAN_POINT('Ctrl Pts',(3.55729713599994,5.2,-3.05332307200001));
#351623=CARTESIAN_POINT('Ctrl Pts',(3.55729713599994,2.2,-3.05332307200001));
#351624=CARTESIAN_POINT('Ctrl Pts',(3.55651189199994,12.2,-3.05087859200002));
#351625=CARTESIAN_POINT('Ctrl Pts',(3.55651189199994,5.2,-3.05087859200002));
#351626=CARTESIAN_POINT('Ctrl Pts',(3.55651189199994,2.2,-3.05087859200002));
#351627=CARTESIAN_POINT('Ctrl Pts',(3.55572515299994,12.2,-3.04843823600002));
#351628=CARTESIAN_POINT('Ctrl Pts',(3.55572515299994,5.2,-3.04843823600002));
#351629=CARTESIAN_POINT('Ctrl Pts',(3.55572515299994,2.2,-3.04843823600002));
#351630=CARTESIAN_POINT('Ctrl Pts',(3.55493692799994,12.2,-3.04600200600001));
#351631=CARTESIAN_POINT('Ctrl Pts',(3.55493692799994,5.2,-3.04600200600001));
#351632=CARTESIAN_POINT('Ctrl Pts',(3.55493692799994,2.2,-3.04600200600001));
#351633=CARTESIAN_POINT('Ctrl Pts',(3.55414722399995,12.2,-3.04356990900001));
#351634=CARTESIAN_POINT('Ctrl Pts',(3.55414722399995,5.2,-3.04356990900001));
#351635=CARTESIAN_POINT('Ctrl Pts',(3.55414722399995,2.2,-3.04356990900001));
#351636=CARTESIAN_POINT('Ctrl Pts',(3.55335604899994,12.2,-3.04114194700002));
#351637=CARTESIAN_POINT('Ctrl Pts',(3.55335604899994,5.2,-3.04114194700002));
#351638=CARTESIAN_POINT('Ctrl Pts',(3.55335604899994,2.2,-3.04114194700002));
#351639=CARTESIAN_POINT('Ctrl Pts',(3.55256340999994,12.2,-3.03871812400001));
#351640=CARTESIAN_POINT('Ctrl Pts',(3.55256340999994,5.2,-3.03871812400001));
#351641=CARTESIAN_POINT('Ctrl Pts',(3.55256340999994,2.2,-3.03871812400001));
#351642=CARTESIAN_POINT('Ctrl Pts',(3.55176931699994,12.2,-3.03629844500001));
#351643=CARTESIAN_POINT('Ctrl Pts',(3.55176931699994,5.2,-3.03629844500001));
#351644=CARTESIAN_POINT('Ctrl Pts',(3.55176931699994,2.2,-3.03629844500001));
#351645=CARTESIAN_POINT('Ctrl Pts',(3.55097377799994,12.2,-3.03388291200001));
#351646=CARTESIAN_POINT('Ctrl Pts',(3.55097377799994,5.2,-3.03388291200001));
#351647=CARTESIAN_POINT('Ctrl Pts',(3.55097377799994,2.2,-3.03388291200001));
#351648=CARTESIAN_POINT('Ctrl Pts',(3.55017679899994,12.2,-3.03147153100001));
#351649=CARTESIAN_POINT('Ctrl Pts',(3.55017679899994,5.2,-3.03147153100001));
#351650=CARTESIAN_POINT('Ctrl Pts',(3.55017679899994,2.2,-3.03147153100001));
#351651=CARTESIAN_POINT('Ctrl Pts',(3.54937838799994,12.2,-3.02906430500002));
#351652=CARTESIAN_POINT('Ctrl Pts',(3.54937838799994,5.2,-3.02906430500002));
#351653=CARTESIAN_POINT('Ctrl Pts',(3.54937838799994,2.2,-3.02906430500002));
#351654=CARTESIAN_POINT('Ctrl Pts',(3.54857855599994,12.2,-3.02666123800002));
#351655=CARTESIAN_POINT('Ctrl Pts',(3.54857855599994,5.2,-3.02666123800002));
#351656=CARTESIAN_POINT('Ctrl Pts',(3.54857855599994,2.2,-3.02666123800002));
#351657=CARTESIAN_POINT('Ctrl Pts',(3.54777730799994,12.2,-3.02426233300002));
#351658=CARTESIAN_POINT('Ctrl Pts',(3.54777730799994,5.2,-3.02426233300002));
#351659=CARTESIAN_POINT('Ctrl Pts',(3.54777730799994,2.2,-3.02426233300002));
#351660=CARTESIAN_POINT('Ctrl Pts',(3.54697465399994,12.2,-3.02186759600001));
#351661=CARTESIAN_POINT('Ctrl Pts',(3.54697465399994,5.2,-3.02186759600001));
#351662=CARTESIAN_POINT('Ctrl Pts',(3.54697465399994,2.2,-3.02186759600001));
#351663=CARTESIAN_POINT('Ctrl Pts',(3.54617059999994,12.2,-3.01947702900002));
#351664=CARTESIAN_POINT('Ctrl Pts',(3.54617059999994,5.2,-3.01947702900002));
#351665=CARTESIAN_POINT('Ctrl Pts',(3.54617059999994,2.2,-3.01947702900002));
#351666=CARTESIAN_POINT('Ctrl Pts',(3.54536515599994,12.2,-3.01709063600001));
#351667=CARTESIAN_POINT('Ctrl Pts',(3.54536515599994,5.2,-3.01709063600001));
#351668=CARTESIAN_POINT('Ctrl Pts',(3.54536515599994,2.2,-3.01709063600001));
#351669=CARTESIAN_POINT('Ctrl Pts',(3.54455832799994,12.2,-3.01470842100001));
#351670=CARTESIAN_POINT('Ctrl Pts',(3.54455832799994,5.2,-3.01470842100001));
#351671=CARTESIAN_POINT('Ctrl Pts',(3.54455832799994,2.2,-3.01470842100001));
#351672=CARTESIAN_POINT('Ctrl Pts',(3.54375012699994,12.2,-3.01233038900001));
#351673=CARTESIAN_POINT('Ctrl Pts',(3.54375012699994,5.2,-3.01233038900001));
#351674=CARTESIAN_POINT('Ctrl Pts',(3.54375012699994,2.2,-3.01233038900001));
#351675=CARTESIAN_POINT('Ctrl Pts',(3.54294055999994,12.2,-3.00995654200001));
#351676=CARTESIAN_POINT('Ctrl Pts',(3.54294055999994,5.2,-3.00995654200001));
#351677=CARTESIAN_POINT('Ctrl Pts',(3.54294055999994,2.2,-3.00995654200001));
#351678=CARTESIAN_POINT('Ctrl Pts',(3.54212963399994,12.2,-3.00758688500002));
#351679=CARTESIAN_POINT('Ctrl Pts',(3.54212963399994,5.2,-3.00758688500002));
#351680=CARTESIAN_POINT('Ctrl Pts',(3.54212963399994,2.2,-3.00758688500002));
#351681=CARTESIAN_POINT('Ctrl Pts',(3.54131735699994,12.2,-3.00522142200002));
#351682=CARTESIAN_POINT('Ctrl Pts',(3.54131735699994,5.2,-3.00522142200002));
#351683=CARTESIAN_POINT('Ctrl Pts',(3.54131735699994,2.2,-3.00522142200002));
#351684=CARTESIAN_POINT('Ctrl Pts',(3.54050373999994,12.2,-3.00286015700001));
#351685=CARTESIAN_POINT('Ctrl Pts',(3.54050373999994,5.2,-3.00286015700001));
#351686=CARTESIAN_POINT('Ctrl Pts',(3.54050373999994,2.2,-3.00286015700001));
#351687=CARTESIAN_POINT('Ctrl Pts',(3.53968878799995,12.2,-3.00050309300001));
#351688=CARTESIAN_POINT('Ctrl Pts',(3.53968878799995,5.2,-3.00050309300001));
#351689=CARTESIAN_POINT('Ctrl Pts',(3.53968878799995,2.2,-3.00050309300001));
#351690=CARTESIAN_POINT('Ctrl Pts',(3.53887251099994,12.2,-2.99815023300001));
#351691=CARTESIAN_POINT('Ctrl Pts',(3.53887251099994,5.2,-2.99815023300001));
#351692=CARTESIAN_POINT('Ctrl Pts',(3.53887251099994,2.2,-2.99815023300001));
#351693=CARTESIAN_POINT('Ctrl Pts',(3.53805491599994,12.2,-2.99580158300001));
#351694=CARTESIAN_POINT('Ctrl Pts',(3.53805491599994,5.2,-2.99580158300001));
#351695=CARTESIAN_POINT('Ctrl Pts',(3.53805491599994,2.2,-2.99580158300001));
#351696=CARTESIAN_POINT('Ctrl Pts',(3.53723601399994,12.2,-2.99345714500001));
#351697=CARTESIAN_POINT('Ctrl Pts',(3.53723601399994,5.2,-2.99345714500001));
#351698=CARTESIAN_POINT('Ctrl Pts',(3.53723601399994,2.2,-2.99345714500001));
#351699=CARTESIAN_POINT('Ctrl Pts',(3.53641580999994,12.2,-2.99111692500002));
#351700=CARTESIAN_POINT('Ctrl Pts',(3.53641580999994,5.2,-2.99111692500002));
#351701=CARTESIAN_POINT('Ctrl Pts',(3.53641580999994,2.2,-2.99111692500002));
#351702=CARTESIAN_POINT('Ctrl Pts',(3.53559431299994,12.2,-2.98878092400002));
#351703=CARTESIAN_POINT('Ctrl Pts',(3.53559431299994,5.2,-2.98878092400002));
#351704=CARTESIAN_POINT('Ctrl Pts',(3.53559431299994,2.2,-2.98878092400002));
#351705=CARTESIAN_POINT('Ctrl Pts',(3.53477153199994,12.2,-2.98644914800001));
#351706=CARTESIAN_POINT('Ctrl Pts',(3.53477153199994,5.2,-2.98644914800001));
#351707=CARTESIAN_POINT('Ctrl Pts',(3.53477153199994,2.2,-2.98644914800001));
#351708=CARTESIAN_POINT('Ctrl Pts',(3.53394747499994,12.2,-2.98412160000002));
#351709=CARTESIAN_POINT('Ctrl Pts',(3.53394747499994,5.2,-2.98412160000002));
#351710=CARTESIAN_POINT('Ctrl Pts',(3.53394747499994,2.2,-2.98412160000002));
#351711=CARTESIAN_POINT('Ctrl Pts',(3.53312214999994,12.2,-2.98179828200002));
#351712=CARTESIAN_POINT('Ctrl Pts',(3.53312214999994,5.2,-2.98179828200002));
#351713=CARTESIAN_POINT('Ctrl Pts',(3.53312214999994,2.2,-2.98179828200002));
#351714=CARTESIAN_POINT('Ctrl Pts',(3.53229556699994,12.2,-2.97947920200002));
#351715=CARTESIAN_POINT('Ctrl Pts',(3.53229556699994,5.2,-2.97947920200002));
#351716=CARTESIAN_POINT('Ctrl Pts',(3.53229556699994,2.2,-2.97947920200002));
#351717=CARTESIAN_POINT('Ctrl Pts',(3.53146773199994,12.2,-2.97716435900002));
#351718=CARTESIAN_POINT('Ctrl Pts',(3.53146773199994,5.2,-2.97716435900002));
#351719=CARTESIAN_POINT('Ctrl Pts',(3.53146773199994,2.2,-2.97716435900002));
#351720=CARTESIAN_POINT('Ctrl Pts',(3.53063865499994,12.2,-2.97485375900001));
#351721=CARTESIAN_POINT('Ctrl Pts',(3.53063865499994,5.2,-2.97485375900001));
#351722=CARTESIAN_POINT('Ctrl Pts',(3.53063865499994,2.2,-2.97485375900001));
#351723=CARTESIAN_POINT('Ctrl Pts',(3.52980834499994,12.2,-2.97254740700001));
#351724=CARTESIAN_POINT('Ctrl Pts',(3.52980834499994,5.2,-2.97254740700001));
#351725=CARTESIAN_POINT('Ctrl Pts',(3.52980834499994,2.2,-2.97254740700001));
#351726=CARTESIAN_POINT('Ctrl Pts',(3.52897680699995,12.2,-2.97024530500002));
#351727=CARTESIAN_POINT('Ctrl Pts',(3.52897680699995,5.2,-2.97024530500002));
#351728=CARTESIAN_POINT('Ctrl Pts',(3.52897680699995,2.2,-2.97024530500002));
#351729=CARTESIAN_POINT('Ctrl Pts',(3.52814405299994,12.2,-2.96794745700002));
#351730=CARTESIAN_POINT('Ctrl Pts',(3.52814405299994,5.2,-2.96794745700002));
#351731=CARTESIAN_POINT('Ctrl Pts',(3.52814405299994,2.2,-2.96794745700002));
#351732=CARTESIAN_POINT('Ctrl Pts',(3.52731008999994,12.2,-2.96565386600002));
#351733=CARTESIAN_POINT('Ctrl Pts',(3.52731008999994,5.2,-2.96565386600002));
#351734=CARTESIAN_POINT('Ctrl Pts',(3.52731008999994,2.2,-2.96565386600002));
#351735=CARTESIAN_POINT('Ctrl Pts',(3.52647492599994,12.2,-2.96336453900001));
#351736=CARTESIAN_POINT('Ctrl Pts',(3.52647492599994,5.2,-2.96336453900001));
#351737=CARTESIAN_POINT('Ctrl Pts',(3.52647492599994,2.2,-2.96336453900001));
#351738=CARTESIAN_POINT('Ctrl Pts',(3.52563856999994,12.2,-2.96107947500001));
#351739=CARTESIAN_POINT('Ctrl Pts',(3.52563856999994,5.2,-2.96107947500001));
#351740=CARTESIAN_POINT('Ctrl Pts',(3.52563856999994,2.2,-2.96107947500001));
#351741=CARTESIAN_POINT('Ctrl Pts',(3.52480103099994,12.2,-2.95879868200001));
#351742=CARTESIAN_POINT('Ctrl Pts',(3.52480103099994,5.2,-2.95879868200001));
#351743=CARTESIAN_POINT('Ctrl Pts',(3.52480103099994,2.2,-2.95879868200001));
#351744=CARTESIAN_POINT('Ctrl Pts',(3.52396231599994,12.2,-2.95652216000001));
#351745=CARTESIAN_POINT('Ctrl Pts',(3.52396231599994,5.2,-2.95652216000001));
#351746=CARTESIAN_POINT('Ctrl Pts',(3.52396231599994,2.2,-2.95652216000001));
#351747=CARTESIAN_POINT('Ctrl Pts',(3.52312243499994,12.2,-2.95424991500001));
#351748=CARTESIAN_POINT('Ctrl Pts',(3.52312243499994,5.2,-2.95424991500001));
#351749=CARTESIAN_POINT('Ctrl Pts',(3.52312243499994,2.2,-2.95424991500001));
#351750=CARTESIAN_POINT('Ctrl Pts',(3.52228139599994,12.2,-2.95198195100001));
#351751=CARTESIAN_POINT('Ctrl Pts',(3.52228139599994,5.2,-2.95198195100001));
#351752=CARTESIAN_POINT('Ctrl Pts',(3.52228139599994,2.2,-2.95198195100001));
#351753=CARTESIAN_POINT('Ctrl Pts',(3.52143920699994,12.2,-2.94971827000001));
#351754=CARTESIAN_POINT('Ctrl Pts',(3.52143920699994,5.2,-2.94971827000001));
#351755=CARTESIAN_POINT('Ctrl Pts',(3.52143920699994,2.2,-2.94971827000001));
#351756=CARTESIAN_POINT('Ctrl Pts',(3.52059587799994,12.2,-2.94745887700001));
#351757=CARTESIAN_POINT('Ctrl Pts',(3.52059587799994,5.2,-2.94745887700001));
#351758=CARTESIAN_POINT('Ctrl Pts',(3.52059587799994,2.2,-2.94745887700001));
#351759=CARTESIAN_POINT('Ctrl Pts',(3.51975141499994,12.2,-2.94520377500001));
#351760=CARTESIAN_POINT('Ctrl Pts',(3.51975141499994,5.2,-2.94520377500001));
#351761=CARTESIAN_POINT('Ctrl Pts',(3.51975141499994,2.2,-2.94520377500001));
#351762=CARTESIAN_POINT('Ctrl Pts',(3.51890582999994,12.2,-2.94295296700001));
#351763=CARTESIAN_POINT('Ctrl Pts',(3.51890582999994,5.2,-2.94295296700001));
#351764=CARTESIAN_POINT('Ctrl Pts',(3.51890582999994,2.2,-2.94295296700001));
#351765=CARTESIAN_POINT('Ctrl Pts',(3.51805912899994,12.2,-2.94070645800002));
#351766=CARTESIAN_POINT('Ctrl Pts',(3.51805912899994,5.2,-2.94070645800002));
#351767=CARTESIAN_POINT('Ctrl Pts',(3.51805912899994,2.2,-2.94070645800002));
#351768=CARTESIAN_POINT('Ctrl Pts',(3.51721132199994,12.2,-2.93846425100002));
#351769=CARTESIAN_POINT('Ctrl Pts',(3.51721132199994,5.2,-2.93846425100002));
#351770=CARTESIAN_POINT('Ctrl Pts',(3.51721132199994,2.2,-2.93846425100002));
#351771=CARTESIAN_POINT('Ctrl Pts',(3.51636241699994,12.2,-2.93622635000002));
#351772=CARTESIAN_POINT('Ctrl Pts',(3.51636241699994,5.2,-2.93622635000002));
#351773=CARTESIAN_POINT('Ctrl Pts',(3.51636241699994,2.2,-2.93622635000002));
#351774=CARTESIAN_POINT('Ctrl Pts',(3.51551242199994,12.2,-2.93399275800001));
#351775=CARTESIAN_POINT('Ctrl Pts',(3.51551242199994,5.2,-2.93399275800001));
#351776=CARTESIAN_POINT('Ctrl Pts',(3.51551242199994,2.2,-2.93399275800001));
#351777=CARTESIAN_POINT('Ctrl Pts',(3.51466134699994,12.2,-2.93176347900001));
#351778=CARTESIAN_POINT('Ctrl Pts',(3.51466134699994,5.2,-2.93176347900001));
#351779=CARTESIAN_POINT('Ctrl Pts',(3.51466134699994,2.2,-2.93176347900001));
#351780=CARTESIAN_POINT('Ctrl Pts',(3.51380919999994,12.2,-2.92953851700001));
#351781=CARTESIAN_POINT('Ctrl Pts',(3.51380919999994,5.2,-2.92953851700001));
#351782=CARTESIAN_POINT('Ctrl Pts',(3.51380919999994,2.2,-2.92953851700001));
#351783=CARTESIAN_POINT('Ctrl Pts',(3.51295598899994,12.2,-2.92731787500002));
#351784=CARTESIAN_POINT('Ctrl Pts',(3.51295598899994,5.2,-2.92731787500002));
#351785=CARTESIAN_POINT('Ctrl Pts',(3.51295598899994,2.2,-2.92731787500002));
#351786=CARTESIAN_POINT('Ctrl Pts',(3.51210172499994,12.2,-2.92510155600001));
#351787=CARTESIAN_POINT('Ctrl Pts',(3.51210172499994,5.2,-2.92510155600001));
#351788=CARTESIAN_POINT('Ctrl Pts',(3.51210172499994,2.2,-2.92510155600001));
#351789=CARTESIAN_POINT('Ctrl Pts',(3.51124641399994,12.2,-2.92288956500002));
#351790=CARTESIAN_POINT('Ctrl Pts',(3.51124641399994,5.2,-2.92288956500002));
#351791=CARTESIAN_POINT('Ctrl Pts',(3.51124641399994,2.2,-2.92288956500002));
#351792=CARTESIAN_POINT('Ctrl Pts',(3.51039006699994,12.2,-2.92068190600002));
#351793=CARTESIAN_POINT('Ctrl Pts',(3.51039006699994,5.2,-2.92068190600002));
#351794=CARTESIAN_POINT('Ctrl Pts',(3.51039006699994,2.2,-2.92068190600002));
#351795=CARTESIAN_POINT('Ctrl Pts',(3.50953269099994,12.2,-2.91847858000001));
#351796=CARTESIAN_POINT('Ctrl Pts',(3.50953269099994,5.2,-2.91847858000001));
#351797=CARTESIAN_POINT('Ctrl Pts',(3.50953269099994,2.2,-2.91847858000001));
#351798=CARTESIAN_POINT('Ctrl Pts',(3.50867429599994,12.2,-2.91627959300001));
#351799=CARTESIAN_POINT('Ctrl Pts',(3.50867429599994,5.2,-2.91627959300001));
#351800=CARTESIAN_POINT('Ctrl Pts',(3.50867429599994,2.2,-2.91627959300001));
#351801=CARTESIAN_POINT('Ctrl Pts',(3.50781488999994,12.2,-2.91408494800002));
#351802=CARTESIAN_POINT('Ctrl Pts',(3.50781488999994,5.2,-2.91408494800002));
#351803=CARTESIAN_POINT('Ctrl Pts',(3.50781488999994,2.2,-2.91408494800002));
#351804=CARTESIAN_POINT('Ctrl Pts',(3.50695448299994,12.2,-2.91189464800001));
#351805=CARTESIAN_POINT('Ctrl Pts',(3.50695448299994,5.2,-2.91189464800001));
#351806=CARTESIAN_POINT('Ctrl Pts',(3.50695448299994,2.2,-2.91189464800001));
#351807=CARTESIAN_POINT('Ctrl Pts',(3.50609308099994,12.2,-2.90970869600002));
#351808=CARTESIAN_POINT('Ctrl Pts',(3.50609308099994,5.2,-2.90970869600002));
#351809=CARTESIAN_POINT('Ctrl Pts',(3.50609308099994,2.2,-2.90970869600002));
#351810=CARTESIAN_POINT('Ctrl Pts',(3.50523069599994,12.2,-2.90752709800001));
#351811=CARTESIAN_POINT('Ctrl Pts',(3.50523069599994,5.2,-2.90752709800001));
#351812=CARTESIAN_POINT('Ctrl Pts',(3.50523069599994,2.2,-2.90752709800001));
#351813=CARTESIAN_POINT('Ctrl Pts',(3.50436733599994,12.2,-2.90534985400001));
#351814=CARTESIAN_POINT('Ctrl Pts',(3.50436733599994,5.2,-2.90534985400001));
#351815=CARTESIAN_POINT('Ctrl Pts',(3.50436733599994,2.2,-2.90534985400001));
#351816=CARTESIAN_POINT('Ctrl Pts',(3.50350300999994,12.2,-2.90317697000001));
#351817=CARTESIAN_POINT('Ctrl Pts',(3.50350300999994,5.2,-2.90317697000001));
#351818=CARTESIAN_POINT('Ctrl Pts',(3.50350300999994,2.2,-2.90317697000001));
#351819=CARTESIAN_POINT('Ctrl Pts',(3.50263772599994,12.2,-2.90100844900001));
#351820=CARTESIAN_POINT('Ctrl Pts',(3.50263772599994,5.2,-2.90100844900001));
#351821=CARTESIAN_POINT('Ctrl Pts',(3.50263772599994,2.2,-2.90100844900001));
#351822=CARTESIAN_POINT('Ctrl Pts',(3.50177149399994,12.2,-2.89884429600002));
#351823=CARTESIAN_POINT('Ctrl Pts',(3.50177149399994,5.2,-2.89884429600002));
#351824=CARTESIAN_POINT('Ctrl Pts',(3.50177149399994,2.2,-2.89884429600002));
#351825=CARTESIAN_POINT('Ctrl Pts',(3.50090432099994,12.2,-2.89668451100002));
#351826=CARTESIAN_POINT('Ctrl Pts',(3.50090432099994,5.2,-2.89668451100002));
#351827=CARTESIAN_POINT('Ctrl Pts',(3.50090432099994,2.2,-2.89668451100002));
#351828=CARTESIAN_POINT('Ctrl Pts',(3.50003621799994,12.2,-2.89452910100001));
#351829=CARTESIAN_POINT('Ctrl Pts',(3.50003621799994,5.2,-2.89452910100001));
#351830=CARTESIAN_POINT('Ctrl Pts',(3.50003621799994,2.2,-2.89452910100001));
#351831=CARTESIAN_POINT('Ctrl Pts',(3.49916719399994,12.2,-2.89237806600001));
#351832=CARTESIAN_POINT('Ctrl Pts',(3.49916719399994,5.2,-2.89237806600001));
#351833=CARTESIAN_POINT('Ctrl Pts',(3.49916719399994,2.2,-2.89237806600001));
#351834=CARTESIAN_POINT('Ctrl Pts',(3.49829725599994,12.2,-2.89023141200001));
#351835=CARTESIAN_POINT('Ctrl Pts',(3.49829725599994,5.2,-2.89023141200001));
#351836=CARTESIAN_POINT('Ctrl Pts',(3.49829725599994,2.2,-2.89023141200001));
#351837=CARTESIAN_POINT('Ctrl Pts',(3.49742641599994,12.2,-2.88808914300001));
#351838=CARTESIAN_POINT('Ctrl Pts',(3.49742641599994,5.2,-2.88808914300001));
#351839=CARTESIAN_POINT('Ctrl Pts',(3.49742641599994,2.2,-2.88808914300001));
#351840=CARTESIAN_POINT('Ctrl Pts',(3.49655467999994,12.2,-2.88595126100001));
#351841=CARTESIAN_POINT('Ctrl Pts',(3.49655467999994,5.2,-2.88595126100001));
#351842=CARTESIAN_POINT('Ctrl Pts',(3.49655467999994,2.2,-2.88595126100001));
#351843=CARTESIAN_POINT('Ctrl Pts',(3.49568205799994,12.2,-2.88381777000001));
#351844=CARTESIAN_POINT('Ctrl Pts',(3.49568205799994,5.2,-2.88381777000001));
#351845=CARTESIAN_POINT('Ctrl Pts',(3.49568205799994,2.2,-2.88381777000001));
#351846=CARTESIAN_POINT('Ctrl Pts',(3.49480855999994,12.2,-2.88168867300001));
#351847=CARTESIAN_POINT('Ctrl Pts',(3.49480855999994,5.2,-2.88168867300001));
#351848=CARTESIAN_POINT('Ctrl Pts',(3.49480855999994,2.2,-2.88168867300001));
#351849=CARTESIAN_POINT('Ctrl Pts',(3.49393419499994,12.2,-2.87956397300002));
#351850=CARTESIAN_POINT('Ctrl Pts',(3.49393419499994,5.2,-2.87956397300002));
#351851=CARTESIAN_POINT('Ctrl Pts',(3.49393419499994,2.2,-2.87956397300002));
#351852=CARTESIAN_POINT('Ctrl Pts',(3.49305897099994,12.2,-2.87744367500002));
#351853=CARTESIAN_POINT('Ctrl Pts',(3.49305897099994,5.2,-2.87744367500002));
#351854=CARTESIAN_POINT('Ctrl Pts',(3.49305897099994,2.2,-2.87744367500002));
#351855=CARTESIAN_POINT('Ctrl Pts',(3.49218289699994,12.2,-2.87532778100001));
#351856=CARTESIAN_POINT('Ctrl Pts',(3.49218289699994,5.2,-2.87532778100001));
#351857=CARTESIAN_POINT('Ctrl Pts',(3.49218289699994,2.2,-2.87532778100001));
#351858=CARTESIAN_POINT('Ctrl Pts',(3.49130598399995,12.2,-2.87321629600001));
#351859=CARTESIAN_POINT('Ctrl Pts',(3.49130598399995,5.2,-2.87321629600001));
#351860=CARTESIAN_POINT('Ctrl Pts',(3.49130598399995,2.2,-2.87321629600001));
#351861=CARTESIAN_POINT('Ctrl Pts',(3.49042823899994,12.2,-2.87110922200001));
#351862=CARTESIAN_POINT('Ctrl Pts',(3.49042823899994,5.2,-2.87110922200001));
#351863=CARTESIAN_POINT('Ctrl Pts',(3.49042823899994,2.2,-2.87110922200001));
#351864=CARTESIAN_POINT('Ctrl Pts',(3.48954967299994,12.2,-2.86900656300002));
#351865=CARTESIAN_POINT('Ctrl Pts',(3.48954967299994,5.2,-2.86900656300002));
#351866=CARTESIAN_POINT('Ctrl Pts',(3.48954967299994,2.2,-2.86900656300002));
#351867=CARTESIAN_POINT('Ctrl Pts',(3.48867029399994,12.2,-2.86690832200001));
#351868=CARTESIAN_POINT('Ctrl Pts',(3.48867029399994,5.2,-2.86690832200001));
#351869=CARTESIAN_POINT('Ctrl Pts',(3.48867029399994,2.2,-2.86690832200001));
#351870=CARTESIAN_POINT('Ctrl Pts',(3.48779011099994,12.2,-2.86481450300001));
#351871=CARTESIAN_POINT('Ctrl Pts',(3.48779011099994,5.2,-2.86481450300001));
#351872=CARTESIAN_POINT('Ctrl Pts',(3.48779011099994,2.2,-2.86481450300001));
#351873=CARTESIAN_POINT('Ctrl Pts',(3.48690913399994,12.2,-2.86272510700002));
#351874=CARTESIAN_POINT('Ctrl Pts',(3.48690913399994,5.2,-2.86272510700002));
#351875=CARTESIAN_POINT('Ctrl Pts',(3.48690913399994,2.2,-2.86272510700002));
#351876=CARTESIAN_POINT('Ctrl Pts',(3.48602737199994,12.2,-2.86064014200001));
#351877=CARTESIAN_POINT('Ctrl Pts',(3.48602737199994,5.2,-2.86064014200001));
#351878=CARTESIAN_POINT('Ctrl Pts',(3.48602737199994,2.2,-2.86064014200001));
#351879=CARTESIAN_POINT('Ctrl Pts',(3.48514483399994,12.2,-2.85855960700002));
#351880=CARTESIAN_POINT('Ctrl Pts',(3.48514483399994,5.2,-2.85855960700002));
#351881=CARTESIAN_POINT('Ctrl Pts',(3.48514483399994,2.2,-2.85855960700002));
#351882=CARTESIAN_POINT('Ctrl Pts',(3.48426152799994,12.2,-2.85648350800002));
#351883=CARTESIAN_POINT('Ctrl Pts',(3.48426152799994,5.2,-2.85648350800002));
#351884=CARTESIAN_POINT('Ctrl Pts',(3.48426152799994,2.2,-2.85648350800002));
#351885=CARTESIAN_POINT('Ctrl Pts',(3.48337746699994,12.2,-2.85441184800002));
#351886=CARTESIAN_POINT('Ctrl Pts',(3.48337746699994,5.2,-2.85441184800002));
#351887=CARTESIAN_POINT('Ctrl Pts',(3.48337746699994,2.2,-2.85441184800002));
#351888=CARTESIAN_POINT('Ctrl Pts',(3.48249265699994,12.2,-2.85234462900001));
#351889=CARTESIAN_POINT('Ctrl Pts',(3.48249265699994,5.2,-2.85234462900001));
#351890=CARTESIAN_POINT('Ctrl Pts',(3.48249265699994,2.2,-2.85234462900001));
#351891=CARTESIAN_POINT('Ctrl Pts',(3.48160710799994,12.2,-2.85028185600002));
#351892=CARTESIAN_POINT('Ctrl Pts',(3.48160710799994,5.2,-2.85028185600002));
#351893=CARTESIAN_POINT('Ctrl Pts',(3.48160710799994,2.2,-2.85028185600002));
#351894=CARTESIAN_POINT('Ctrl Pts',(3.48072082999995,12.2,-2.84822353100001));
#351895=CARTESIAN_POINT('Ctrl Pts',(3.48072082999995,5.2,-2.84822353100001));
#351896=CARTESIAN_POINT('Ctrl Pts',(3.48072082999995,2.2,-2.84822353100001));
#351897=CARTESIAN_POINT('Ctrl Pts',(3.47983383199994,12.2,-2.84616965800002));
#351898=CARTESIAN_POINT('Ctrl Pts',(3.47983383199994,5.2,-2.84616965800002));
#351899=CARTESIAN_POINT('Ctrl Pts',(3.47983383199994,2.2,-2.84616965800002));
#351900=CARTESIAN_POINT('Ctrl Pts',(3.47894612299994,12.2,-2.84412023900002));
#351901=CARTESIAN_POINT('Ctrl Pts',(3.47894612299994,5.2,-2.84412023900002));
#351902=CARTESIAN_POINT('Ctrl Pts',(3.47894612299994,2.2,-2.84412023900002));
#351903=CARTESIAN_POINT('Ctrl Pts',(3.47805771399994,12.2,-2.84207527900001));
#351904=CARTESIAN_POINT('Ctrl Pts',(3.47805771399994,5.2,-2.84207527900001));
#351905=CARTESIAN_POINT('Ctrl Pts',(3.47805771399994,2.2,-2.84207527900001));
#351906=CARTESIAN_POINT('Ctrl Pts',(3.47716861199994,12.2,-2.84003478100002));
#351907=CARTESIAN_POINT('Ctrl Pts',(3.47716861199994,5.2,-2.84003478100002));
#351908=CARTESIAN_POINT('Ctrl Pts',(3.47716861199994,2.2,-2.84003478100002));
#351909=CARTESIAN_POINT('Ctrl Pts',(3.47627882699994,12.2,-2.83799874900001));
#351910=CARTESIAN_POINT('Ctrl Pts',(3.47627882699994,5.2,-2.83799874900001));
#351911=CARTESIAN_POINT('Ctrl Pts',(3.47627882699994,2.2,-2.83799874900001));
#351912=CARTESIAN_POINT('Ctrl Pts',(3.47538836999994,12.2,-2.83596718400001));
#351913=CARTESIAN_POINT('Ctrl Pts',(3.47538836999994,5.2,-2.83596718400001));
#351914=CARTESIAN_POINT('Ctrl Pts',(3.47538836999994,2.2,-2.83596718400001));
#351915=CARTESIAN_POINT('Ctrl Pts',(3.47449724999994,12.2,-2.83394009000002));
#351916=CARTESIAN_POINT('Ctrl Pts',(3.47449724999994,5.2,-2.83394009000002));
#351917=CARTESIAN_POINT('Ctrl Pts',(3.47449724999994,2.2,-2.83394009000002));
#351918=CARTESIAN_POINT('Ctrl Pts',(3.47360547499994,12.2,-2.83191747100001));
#351919=CARTESIAN_POINT('Ctrl Pts',(3.47360547499994,5.2,-2.83191747100001));
#351920=CARTESIAN_POINT('Ctrl Pts',(3.47360547499994,2.2,-2.83191747100001));
#351921=CARTESIAN_POINT('Ctrl Pts',(3.47271305499994,12.2,-2.82989933100001));
#351922=CARTESIAN_POINT('Ctrl Pts',(3.47271305499994,5.2,-2.82989933100001));
#351923=CARTESIAN_POINT('Ctrl Pts',(3.47271305499994,2.2,-2.82989933100001));
#351924=CARTESIAN_POINT('Ctrl Pts',(3.47182000099994,12.2,-2.82788567200001));
#351925=CARTESIAN_POINT('Ctrl Pts',(3.47182000099994,5.2,-2.82788567200001));
#351926=CARTESIAN_POINT('Ctrl Pts',(3.47182000099994,2.2,-2.82788567200001));
#351927=CARTESIAN_POINT('Ctrl Pts',(3.47092632099995,12.2,-2.82587649700002));
#351928=CARTESIAN_POINT('Ctrl Pts',(3.47092632099995,5.2,-2.82587649700002));
#351929=CARTESIAN_POINT('Ctrl Pts',(3.47092632099995,2.2,-2.82587649700002));
#351930=CARTESIAN_POINT('Ctrl Pts',(3.47003202499995,12.2,-2.82387181000002));
#351931=CARTESIAN_POINT('Ctrl Pts',(3.47003202499995,5.2,-2.82387181000002));
#351932=CARTESIAN_POINT('Ctrl Pts',(3.47003202499995,2.2,-2.82387181000002));
#351933=CARTESIAN_POINT('Ctrl Pts',(3.46913712299994,12.2,-2.82187161500001));
#351934=CARTESIAN_POINT('Ctrl Pts',(3.46913712299994,5.2,-2.82187161500001));
#351935=CARTESIAN_POINT('Ctrl Pts',(3.46913712299994,2.2,-2.82187161500001));
#351936=CARTESIAN_POINT('Ctrl Pts',(3.46824162499995,12.2,-2.81987591300001));
#351937=CARTESIAN_POINT('Ctrl Pts',(3.46824162499995,5.2,-2.81987591300001));
#351938=CARTESIAN_POINT('Ctrl Pts',(3.46824162499995,2.2,-2.81987591300001));
#351939=CARTESIAN_POINT('Ctrl Pts',(3.46734553799994,12.2,-2.81788470800001));
#351940=CARTESIAN_POINT('Ctrl Pts',(3.46734553799994,5.2,-2.81788470800001));
#351941=CARTESIAN_POINT('Ctrl Pts',(3.46734553799994,2.2,-2.81788470800001));
#351942=CARTESIAN_POINT('Ctrl Pts',(3.46644887499994,12.2,-2.81589800400001));
#351943=CARTESIAN_POINT('Ctrl Pts',(3.46644887499994,5.2,-2.81589800400001));
#351944=CARTESIAN_POINT('Ctrl Pts',(3.46644887499994,2.2,-2.81589800400001));
#351945=CARTESIAN_POINT('Ctrl Pts',(3.46555164299994,12.2,-2.81391580500001));
#351946=CARTESIAN_POINT('Ctrl Pts',(3.46555164299994,5.2,-2.81391580500001));
#351947=CARTESIAN_POINT('Ctrl Pts',(3.46555164299994,2.2,-2.81391580500001));
#351948=CARTESIAN_POINT('Ctrl Pts',(3.46465385299994,12.2,-2.81193811200001));
#351949=CARTESIAN_POINT('Ctrl Pts',(3.46465385299994,5.2,-2.81193811200001));
#351950=CARTESIAN_POINT('Ctrl Pts',(3.46465385299994,2.2,-2.81193811200001));
#351951=CARTESIAN_POINT('Ctrl Pts',(3.46375551499994,12.2,-2.80996492900002));
#351952=CARTESIAN_POINT('Ctrl Pts',(3.46375551499994,5.2,-2.80996492900002));
#351953=CARTESIAN_POINT('Ctrl Pts',(3.46375551499994,2.2,-2.80996492900002));
#351954=CARTESIAN_POINT('Ctrl Pts',(3.46285663699994,12.2,-2.80799625900002));
#351955=CARTESIAN_POINT('Ctrl Pts',(3.46285663699994,5.2,-2.80799625900002));
#351956=CARTESIAN_POINT('Ctrl Pts',(3.46285663699994,2.2,-2.80799625900002));
#351957=CARTESIAN_POINT('Ctrl Pts',(3.46195723099994,12.2,-2.80603210700002));
#351958=CARTESIAN_POINT('Ctrl Pts',(3.46195723099994,5.2,-2.80603210700002));
#351959=CARTESIAN_POINT('Ctrl Pts',(3.46195723099994,2.2,-2.80603210700002));
#351960=CARTESIAN_POINT('Ctrl Pts',(3.46105730499994,12.2,-2.80407247300001));
#351961=CARTESIAN_POINT('Ctrl Pts',(3.46105730499994,5.2,-2.80407247300001));
#351962=CARTESIAN_POINT('Ctrl Pts',(3.46105730499994,2.2,-2.80407247300001));
#351963=CARTESIAN_POINT('Ctrl Pts',(3.46015686899994,12.2,-2.80211736300001));
#351964=CARTESIAN_POINT('Ctrl Pts',(3.46015686899994,5.2,-2.80211736300001));
#351965=CARTESIAN_POINT('Ctrl Pts',(3.46015686899994,2.2,-2.80211736300001));
#351966=CARTESIAN_POINT('Ctrl Pts',(3.45925593399994,12.2,-2.80016677700001));
#351967=CARTESIAN_POINT('Ctrl Pts',(3.45925593399994,5.2,-2.80016677700001));
#351968=CARTESIAN_POINT('Ctrl Pts',(3.45925593399994,2.2,-2.80016677700001));
#351969=CARTESIAN_POINT('Ctrl Pts',(3.45835450899994,12.2,-2.79822072100002));
#351970=CARTESIAN_POINT('Ctrl Pts',(3.45835450899994,5.2,-2.79822072100002));
#351971=CARTESIAN_POINT('Ctrl Pts',(3.45835450899994,2.2,-2.79822072100002));
#351972=CARTESIAN_POINT('Ctrl Pts',(3.45745260299994,12.2,-2.79627919700001));
#351973=CARTESIAN_POINT('Ctrl Pts',(3.45745260299994,5.2,-2.79627919700001));
#351974=CARTESIAN_POINT('Ctrl Pts',(3.45745260299994,2.2,-2.79627919700001));
#351975=CARTESIAN_POINT('Ctrl Pts',(3.45655022599994,12.2,-2.79434220800002));
#351976=CARTESIAN_POINT('Ctrl Pts',(3.45655022599994,5.2,-2.79434220800002));
#351977=CARTESIAN_POINT('Ctrl Pts',(3.45655022599994,2.2,-2.79434220800002));
#351978=CARTESIAN_POINT('Ctrl Pts',(3.45564738899995,12.2,-2.79240975700001));
#351979=CARTESIAN_POINT('Ctrl Pts',(3.45564738899995,5.2,-2.79240975700001));
#351980=CARTESIAN_POINT('Ctrl Pts',(3.45564738899995,2.2,-2.79240975700001));
#351981=CARTESIAN_POINT('Ctrl Pts',(3.45474410099994,12.2,-2.79048184900001));
#351982=CARTESIAN_POINT('Ctrl Pts',(3.45474410099994,5.2,-2.79048184900001));
#351983=CARTESIAN_POINT('Ctrl Pts',(3.45474410099994,2.2,-2.79048184900001));
#351984=CARTESIAN_POINT('Ctrl Pts',(3.45384037299994,12.2,-2.78855848300001));
#351985=CARTESIAN_POINT('Ctrl Pts',(3.45384037299994,5.2,-2.78855848300001));
#351986=CARTESIAN_POINT('Ctrl Pts',(3.45384037299994,2.2,-2.78855848300001));
#351987=CARTESIAN_POINT('Ctrl Pts',(3.45293621399994,12.2,-2.78663966600002));
#351988=CARTESIAN_POINT('Ctrl Pts',(3.45293621399994,5.2,-2.78663966600002));
#351989=CARTESIAN_POINT('Ctrl Pts',(3.45293621399994,2.2,-2.78663966600002));
#351990=CARTESIAN_POINT('Ctrl Pts',(3.45203163299994,12.2,-2.78472539900001));
#351991=CARTESIAN_POINT('Ctrl Pts',(3.45203163299994,5.2,-2.78472539900001));
#351992=CARTESIAN_POINT('Ctrl Pts',(3.45203163299994,2.2,-2.78472539900001));
#351993=CARTESIAN_POINT('Ctrl Pts',(3.45112664199994,12.2,-2.78281568600002));
#351994=CARTESIAN_POINT('Ctrl Pts',(3.45112664199994,5.2,-2.78281568600002));
#351995=CARTESIAN_POINT('Ctrl Pts',(3.45112664199994,2.2,-2.78281568600002));
#351996=CARTESIAN_POINT('Ctrl Pts',(3.45022124899995,12.2,-2.78091052900002));
#351997=CARTESIAN_POINT('Ctrl Pts',(3.45022124899995,5.2,-2.78091052900002));
#351998=CARTESIAN_POINT('Ctrl Pts',(3.45022124899995,2.2,-2.78091052900002));
#351999=CARTESIAN_POINT('Ctrl Pts',(3.44931546499994,12.2,-2.77900993200001));
#352000=CARTESIAN_POINT('Ctrl Pts',(3.44931546499994,5.2,-2.77900993200001));
#352001=CARTESIAN_POINT('Ctrl Pts',(3.44931546499994,2.2,-2.77900993200001));
#352002=CARTESIAN_POINT('Ctrl Pts',(3.44840929999994,12.2,-2.77711389800002));
#352003=CARTESIAN_POINT('Ctrl Pts',(3.44840929999994,5.2,-2.77711389800002));
#352004=CARTESIAN_POINT('Ctrl Pts',(3.44840929999994,2.2,-2.77711389800002));
#352005=CARTESIAN_POINT('Ctrl Pts',(3.44750276299994,12.2,-2.77522242900002));
#352006=CARTESIAN_POINT('Ctrl Pts',(3.44750276299994,5.2,-2.77522242900002));
#352007=CARTESIAN_POINT('Ctrl Pts',(3.44750276299994,2.2,-2.77522242900002));
#352008=CARTESIAN_POINT('Ctrl Pts',(3.44659586599994,12.2,-2.77333552900001));
#352009=CARTESIAN_POINT('Ctrl Pts',(3.44659586599994,5.2,-2.77333552900001));
#352010=CARTESIAN_POINT('Ctrl Pts',(3.44659586599994,2.2,-2.77333552900001));
#352011=CARTESIAN_POINT('Ctrl Pts',(3.44568861799994,12.2,-2.77145320000002));
#352012=CARTESIAN_POINT('Ctrl Pts',(3.44568861799994,5.2,-2.77145320000002));
#352013=CARTESIAN_POINT('Ctrl Pts',(3.44568861799994,2.2,-2.77145320000002));
#352014=CARTESIAN_POINT('Ctrl Pts',(3.44478102899994,12.2,-2.76957544600001));
#352015=CARTESIAN_POINT('Ctrl Pts',(3.44478102899994,5.2,-2.76957544600001));
#352016=CARTESIAN_POINT('Ctrl Pts',(3.44478102899994,2.2,-2.76957544600001));
#352017=CARTESIAN_POINT('Ctrl Pts',(3.44387310799994,12.2,-2.76770227000001));
#352018=CARTESIAN_POINT('Ctrl Pts',(3.44387310799994,5.2,-2.76770227000001));
#352019=CARTESIAN_POINT('Ctrl Pts',(3.44387310799994,2.2,-2.76770227000001));
#352020=CARTESIAN_POINT('Ctrl Pts',(3.44296486699994,12.2,-2.76583367300002));
#352021=CARTESIAN_POINT('Ctrl Pts',(3.44296486699994,5.2,-2.76583367300002));
#352022=CARTESIAN_POINT('Ctrl Pts',(3.44296486699994,2.2,-2.76583367300002));
#352023=CARTESIAN_POINT('Ctrl Pts',(3.44205631599994,12.2,-2.76396966100001));
#352024=CARTESIAN_POINT('Ctrl Pts',(3.44205631599994,5.2,-2.76396966100001));
#352025=CARTESIAN_POINT('Ctrl Pts',(3.44205631599994,2.2,-2.76396966100001));
#352026=CARTESIAN_POINT('Ctrl Pts',(3.44114746399995,12.2,-2.76211023600001));
#352027=CARTESIAN_POINT('Ctrl Pts',(3.44114746399995,5.2,-2.76211023600001));
#352028=CARTESIAN_POINT('Ctrl Pts',(3.44114746399995,2.2,-2.76211023600001));
#352029=CARTESIAN_POINT('Ctrl Pts',(3.44023832099994,12.2,-2.76025539900001));
#352030=CARTESIAN_POINT('Ctrl Pts',(3.44023832099994,5.2,-2.76025539900001));
#352031=CARTESIAN_POINT('Ctrl Pts',(3.44023832099994,2.2,-2.76025539900001));
#352032=CARTESIAN_POINT('Ctrl Pts',(3.43932889999994,12.2,-2.75840515500001));
#352033=CARTESIAN_POINT('Ctrl Pts',(3.43932889999994,5.2,-2.75840515500001));
#352034=CARTESIAN_POINT('Ctrl Pts',(3.43932889999994,2.2,-2.75840515500001));
#352035=CARTESIAN_POINT('Ctrl Pts',(3.43841920699994,12.2,-2.75655950600001));
#352036=CARTESIAN_POINT('Ctrl Pts',(3.43841920699994,5.2,-2.75655950600001));
#352037=CARTESIAN_POINT('Ctrl Pts',(3.43841920699994,2.2,-2.75655950600001));
#352038=CARTESIAN_POINT('Ctrl Pts',(3.43750925599994,12.2,-2.75471845600002));
#352039=CARTESIAN_POINT('Ctrl Pts',(3.43750925599994,5.2,-2.75471845600002));
#352040=CARTESIAN_POINT('Ctrl Pts',(3.43750925599994,2.2,-2.75471845600002));
#352041=CARTESIAN_POINT('Ctrl Pts',(3.43659905399994,12.2,-2.75288200500002));
#352042=CARTESIAN_POINT('Ctrl Pts',(3.43659905399994,5.2,-2.75288200500002));
#352043=CARTESIAN_POINT('Ctrl Pts',(3.43659905399994,2.2,-2.75288200500002));
#352044=CARTESIAN_POINT('Ctrl Pts',(3.43568861399994,12.2,-2.75105016000001));
#352045=CARTESIAN_POINT('Ctrl Pts',(3.43568861399994,5.2,-2.75105016000001));
#352046=CARTESIAN_POINT('Ctrl Pts',(3.43568861399994,2.2,-2.75105016000001));
#352047=CARTESIAN_POINT('Ctrl Pts',(3.43477794499994,12.2,-2.74922292100001));
#352048=CARTESIAN_POINT('Ctrl Pts',(3.43477794499994,5.2,-2.74922292100001));
#352049=CARTESIAN_POINT('Ctrl Pts',(3.43477794499994,2.2,-2.74922292100001));
#352050=CARTESIAN_POINT('Ctrl Pts',(3.43386705799994,12.2,-2.74740029100002));
#352051=CARTESIAN_POINT('Ctrl Pts',(3.43386705799994,5.2,-2.74740029100002));
#352052=CARTESIAN_POINT('Ctrl Pts',(3.43386705799994,2.2,-2.74740029100002));
#352053=CARTESIAN_POINT('Ctrl Pts',(3.43295596299994,12.2,-2.74558227400002));
#352054=CARTESIAN_POINT('Ctrl Pts',(3.43295596299994,5.2,-2.74558227400002));
#352055=CARTESIAN_POINT('Ctrl Pts',(3.43295596299994,2.2,-2.74558227400002));
#352056=CARTESIAN_POINT('Ctrl Pts',(3.43204466899994,12.2,-2.74376887300001));
#352057=CARTESIAN_POINT('Ctrl Pts',(3.43204466899994,5.2,-2.74376887300001));
#352058=CARTESIAN_POINT('Ctrl Pts',(3.43204466899994,2.2,-2.74376887300001));
#352059=CARTESIAN_POINT('Ctrl Pts',(3.43113318899994,12.2,-2.74196008900002));
#352060=CARTESIAN_POINT('Ctrl Pts',(3.43113318899994,5.2,-2.74196008900002));
#352061=CARTESIAN_POINT('Ctrl Pts',(3.43113318899994,2.2,-2.74196008900002));
#352062=CARTESIAN_POINT('Ctrl Pts',(3.43022152999994,12.2,-2.74015592700001));
#352063=CARTESIAN_POINT('Ctrl Pts',(3.43022152999994,5.2,-2.74015592700001));
#352064=CARTESIAN_POINT('Ctrl Pts',(3.43022152999994,2.2,-2.74015592700001));
#352065=CARTESIAN_POINT('Ctrl Pts',(3.42930970599994,12.2,-2.73835638800001));
#352066=CARTESIAN_POINT('Ctrl Pts',(3.42930970599994,5.2,-2.73835638800001));
#352067=CARTESIAN_POINT('Ctrl Pts',(3.42930970599994,2.2,-2.73835638800001));
#352068=CARTESIAN_POINT('Ctrl Pts',(3.42839772599994,12.2,-2.73656147700001));
#352069=CARTESIAN_POINT('Ctrl Pts',(3.42839772599994,5.2,-2.73656147700001));
#352070=CARTESIAN_POINT('Ctrl Pts',(3.42839772599994,2.2,-2.73656147700001));
#352071=CARTESIAN_POINT('Ctrl Pts',(3.42748559899994,12.2,-2.73477119400001));
#352072=CARTESIAN_POINT('Ctrl Pts',(3.42748559899994,5.2,-2.73477119400001));
#352073=CARTESIAN_POINT('Ctrl Pts',(3.42748559899994,2.2,-2.73477119400001));
#352074=CARTESIAN_POINT('Ctrl Pts',(3.42657333799994,12.2,-2.73298554400002));
#352075=CARTESIAN_POINT('Ctrl Pts',(3.42657333799994,5.2,-2.73298554400002));
#352076=CARTESIAN_POINT('Ctrl Pts',(3.42657333799994,2.2,-2.73298554400002));
#352077=CARTESIAN_POINT('Ctrl Pts',(3.42566095199994,12.2,-2.73120452900002));
#352078=CARTESIAN_POINT('Ctrl Pts',(3.42566095199994,5.2,-2.73120452900002));
#352079=CARTESIAN_POINT('Ctrl Pts',(3.42566095199994,2.2,-2.73120452900002));
#352080=CARTESIAN_POINT('Ctrl Pts',(3.42474845199995,12.2,-2.72942815200001));
#352081=CARTESIAN_POINT('Ctrl Pts',(3.42474845199995,5.2,-2.72942815200001));
#352082=CARTESIAN_POINT('Ctrl Pts',(3.42474845199995,2.2,-2.72942815200001));
#352083=CARTESIAN_POINT('Ctrl Pts',(3.42383584799994,12.2,-2.72765641500001));
#352084=CARTESIAN_POINT('Ctrl Pts',(3.42383584799994,5.2,-2.72765641500001));
#352085=CARTESIAN_POINT('Ctrl Pts',(3.42383584799994,2.2,-2.72765641500001));
#352086=CARTESIAN_POINT('Ctrl Pts',(3.42292315099994,12.2,-2.72588932200001));
#352087=CARTESIAN_POINT('Ctrl Pts',(3.42292315099994,5.2,-2.72588932200001));
#352088=CARTESIAN_POINT('Ctrl Pts',(3.42292315099994,2.2,-2.72588932200001));
#352089=CARTESIAN_POINT('Ctrl Pts',(3.42201037099994,12.2,-2.72412687400001));
#352090=CARTESIAN_POINT('Ctrl Pts',(3.42201037099994,5.2,-2.72412687400001));
#352091=CARTESIAN_POINT('Ctrl Pts',(3.42201037099994,2.2,-2.72412687400001));
#352092=CARTESIAN_POINT('Ctrl Pts',(3.42109751999994,12.2,-2.72236907600002));
#352093=CARTESIAN_POINT('Ctrl Pts',(3.42109751999994,5.2,-2.72236907600002));
#352094=CARTESIAN_POINT('Ctrl Pts',(3.42109751999994,2.2,-2.72236907600002));
#352095=CARTESIAN_POINT('Ctrl Pts',(3.42018460699994,12.2,-2.72061592900001));
#352096=CARTESIAN_POINT('Ctrl Pts',(3.42018460699994,5.2,-2.72061592900001));
#352097=CARTESIAN_POINT('Ctrl Pts',(3.42018460699994,2.2,-2.72061592900001));
#352098=CARTESIAN_POINT('Ctrl Pts',(3.41927164399995,12.2,-2.71886743500001));
#352099=CARTESIAN_POINT('Ctrl Pts',(3.41927164399995,5.2,-2.71886743500001));
#352100=CARTESIAN_POINT('Ctrl Pts',(3.41927164399995,2.2,-2.71886743500001));
#352101=CARTESIAN_POINT('Ctrl Pts',(3.41835863999994,12.2,-2.71712360000001));
#352102=CARTESIAN_POINT('Ctrl Pts',(3.41835863999994,5.2,-2.71712360000001));
#352103=CARTESIAN_POINT('Ctrl Pts',(3.41835863999994,2.2,-2.71712360000001));
#352104=CARTESIAN_POINT('Ctrl Pts',(3.41744560799994,12.2,-2.71538442300002));
#352105=CARTESIAN_POINT('Ctrl Pts',(3.41744560799994,5.2,-2.71538442300002));
#352106=CARTESIAN_POINT('Ctrl Pts',(3.41744560799994,2.2,-2.71538442300002));
#352107=CARTESIAN_POINT('Ctrl Pts',(3.41653255599994,12.2,-2.71364990900001));
#352108=CARTESIAN_POINT('Ctrl Pts',(3.41653255599994,5.2,-2.71364990900001));
#352109=CARTESIAN_POINT('Ctrl Pts',(3.41653255599994,2.2,-2.71364990900001));
#352110=CARTESIAN_POINT('Ctrl Pts',(3.41561949699994,12.2,-2.71192005900001));
#352111=CARTESIAN_POINT('Ctrl Pts',(3.41561949699994,5.2,-2.71192005900001));
#352112=CARTESIAN_POINT('Ctrl Pts',(3.41561949699994,2.2,-2.71192005900001));
#352113=CARTESIAN_POINT('Ctrl Pts',(3.41470643999994,12.2,-2.71019487800002));
#352114=CARTESIAN_POINT('Ctrl Pts',(3.41470643999994,5.2,-2.71019487800002));
#352115=CARTESIAN_POINT('Ctrl Pts',(3.41470643999994,2.2,-2.71019487800002));
#352116=CARTESIAN_POINT('Ctrl Pts',(3.41379339799994,12.2,-2.70847436600001));
#352117=CARTESIAN_POINT('Ctrl Pts',(3.41379339799994,5.2,-2.70847436600001));
#352118=CARTESIAN_POINT('Ctrl Pts',(3.41379339799994,2.2,-2.70847436600001));
#352119=CARTESIAN_POINT('Ctrl Pts',(3.41288037899994,12.2,-2.70675852800002));
#352120=CARTESIAN_POINT('Ctrl Pts',(3.41288037899994,5.2,-2.70675852800002));
#352121=CARTESIAN_POINT('Ctrl Pts',(3.41288037899994,2.2,-2.70675852800002));
#352122=CARTESIAN_POINT('Ctrl Pts',(3.41196739599994,12.2,-2.70504736500001));
#352123=CARTESIAN_POINT('Ctrl Pts',(3.41196739599994,5.2,-2.70504736500001));
#352124=CARTESIAN_POINT('Ctrl Pts',(3.41196739599994,2.2,-2.70504736500001));
#352125=CARTESIAN_POINT('Ctrl Pts',(3.41105445899994,12.2,-2.70334088000002));
#352126=CARTESIAN_POINT('Ctrl Pts',(3.41105445899994,5.2,-2.70334088000002));
#352127=CARTESIAN_POINT('Ctrl Pts',(3.41105445899994,2.2,-2.70334088000002));
#352128=CARTESIAN_POINT('Ctrl Pts',(3.41014157899994,12.2,-2.70163907500002));
#352129=CARTESIAN_POINT('Ctrl Pts',(3.41014157899994,5.2,-2.70163907500002));
#352130=CARTESIAN_POINT('Ctrl Pts',(3.41014157899994,2.2,-2.70163907500002));
#352131=CARTESIAN_POINT('Ctrl Pts',(3.40922876599994,12.2,-2.69994195500002));
#352132=CARTESIAN_POINT('Ctrl Pts',(3.40922876599994,5.2,-2.69994195500002));
#352133=CARTESIAN_POINT('Ctrl Pts',(3.40922876599994,2.2,-2.69994195500002));
#352134=CARTESIAN_POINT('Ctrl Pts',(3.40831603299995,12.2,-2.69824951900001));
#352135=CARTESIAN_POINT('Ctrl Pts',(3.40831603299995,5.2,-2.69824951900001));
#352136=CARTESIAN_POINT('Ctrl Pts',(3.40831603299995,2.2,-2.69824951900001));
#352137=CARTESIAN_POINT('Ctrl Pts',(3.40740338899994,12.2,-2.69656177300002));
#352138=CARTESIAN_POINT('Ctrl Pts',(3.40740338899994,5.2,-2.69656177300002));
#352139=CARTESIAN_POINT('Ctrl Pts',(3.40740338899994,2.2,-2.69656177300002));
#352140=CARTESIAN_POINT('Ctrl Pts',(3.40649084599994,12.2,-2.69487871800001));
#352141=CARTESIAN_POINT('Ctrl Pts',(3.40649084599994,5.2,-2.69487871800001));
#352142=CARTESIAN_POINT('Ctrl Pts',(3.40649084599994,2.2,-2.69487871800001));
#352143=CARTESIAN_POINT('Ctrl Pts',(3.40557841399994,12.2,-2.69320035500002));
#352144=CARTESIAN_POINT('Ctrl Pts',(3.40557841399994,5.2,-2.69320035500002));
#352145=CARTESIAN_POINT('Ctrl Pts',(3.40557841399994,2.2,-2.69320035500002));
#352146=CARTESIAN_POINT('Ctrl Pts',(3.40466610499994,12.2,-2.69152669000002));
#352147=CARTESIAN_POINT('Ctrl Pts',(3.40466610499994,5.2,-2.69152669000002));
#352148=CARTESIAN_POINT('Ctrl Pts',(3.40466610499994,2.2,-2.69152669000002));
#352149=CARTESIAN_POINT('Ctrl Pts',(3.40375392899994,12.2,-2.68985772300002));
#352150=CARTESIAN_POINT('Ctrl Pts',(3.40375392899994,5.2,-2.68985772300002));
#352151=CARTESIAN_POINT('Ctrl Pts',(3.40375392899994,2.2,-2.68985772300002));
#352152=CARTESIAN_POINT('Ctrl Pts',(3.40284189799994,12.2,-2.68819345700001));
#352153=CARTESIAN_POINT('Ctrl Pts',(3.40284189799994,5.2,-2.68819345700001));
#352154=CARTESIAN_POINT('Ctrl Pts',(3.40284189799994,2.2,-2.68819345700001));
#352155=CARTESIAN_POINT('Ctrl Pts',(3.40193002199995,12.2,-2.68653389500002));
#352156=CARTESIAN_POINT('Ctrl Pts',(3.40193002199995,5.2,-2.68653389500002));
#352157=CARTESIAN_POINT('Ctrl Pts',(3.40193002199995,2.2,-2.68653389500002));
#352158=CARTESIAN_POINT('Ctrl Pts',(3.40101831299994,12.2,-2.68487903900001));
#352159=CARTESIAN_POINT('Ctrl Pts',(3.40101831299994,5.2,-2.68487903900001));
#352160=CARTESIAN_POINT('Ctrl Pts',(3.40101831299994,2.2,-2.68487903900001));
#352161=CARTESIAN_POINT('Ctrl Pts',(3.40010678199994,12.2,-2.68322889200002));
#352162=CARTESIAN_POINT('Ctrl Pts',(3.40010678199994,5.2,-2.68322889200002));
#352163=CARTESIAN_POINT('Ctrl Pts',(3.40010678199994,2.2,-2.68322889200002));
#352164=CARTESIAN_POINT('Ctrl Pts',(3.39919543899994,12.2,-2.68158345600002));
#352165=CARTESIAN_POINT('Ctrl Pts',(3.39919543899994,5.2,-2.68158345600002));
#352166=CARTESIAN_POINT('Ctrl Pts',(3.39919543899994,2.2,-2.68158345600002));
#352167=CARTESIAN_POINT('Ctrl Pts',(3.39828429699994,12.2,-2.67994273300001));
#352168=CARTESIAN_POINT('Ctrl Pts',(3.39828429699994,5.2,-2.67994273300001));
#352169=CARTESIAN_POINT('Ctrl Pts',(3.39828429699994,2.2,-2.67994273300001));
#352170=CARTESIAN_POINT('Ctrl Pts',(3.39737336599994,12.2,-2.67830672600001));
#352171=CARTESIAN_POINT('Ctrl Pts',(3.39737336599994,5.2,-2.67830672600001));
#352172=CARTESIAN_POINT('Ctrl Pts',(3.39737336599994,2.2,-2.67830672600001));
#352173=CARTESIAN_POINT('Ctrl Pts',(3.39646265699994,12.2,-2.67667543800002));
#352174=CARTESIAN_POINT('Ctrl Pts',(3.39646265699994,5.2,-2.67667543800002));
#352175=CARTESIAN_POINT('Ctrl Pts',(3.39646265699994,2.2,-2.67667543800002));
#352176=CARTESIAN_POINT('Ctrl Pts',(3.39555218099994,12.2,-2.67504887100001));
#352177=CARTESIAN_POINT('Ctrl Pts',(3.39555218099994,5.2,-2.67504887100001));
#352178=CARTESIAN_POINT('Ctrl Pts',(3.39555218099994,2.2,-2.67504887100001));
#352179=CARTESIAN_POINT('Ctrl Pts',(3.39464195099994,12.2,-2.67342702700001));
#352180=CARTESIAN_POINT('Ctrl Pts',(3.39464195099994,5.2,-2.67342702700001));
#352181=CARTESIAN_POINT('Ctrl Pts',(3.39464195099994,2.2,-2.67342702700001));
#352182=CARTESIAN_POINT('Ctrl Pts',(3.39373197699994,12.2,-2.67180991000001));
#352183=CARTESIAN_POINT('Ctrl Pts',(3.39373197699994,5.2,-2.67180991000001));
#352184=CARTESIAN_POINT('Ctrl Pts',(3.39373197699994,2.2,-2.67180991000001));
#352185=CARTESIAN_POINT('Ctrl Pts',(3.39282226999994,12.2,-2.67019752000001));
#352186=CARTESIAN_POINT('Ctrl Pts',(3.39282226999994,5.2,-2.67019752000001));
#352187=CARTESIAN_POINT('Ctrl Pts',(3.39282226999994,2.2,-2.67019752000001));
#352188=CARTESIAN_POINT('Ctrl Pts',(3.39191284199994,12.2,-2.66858986100001));
#352189=CARTESIAN_POINT('Ctrl Pts',(3.39191284199994,5.2,-2.66858986100001));
#352190=CARTESIAN_POINT('Ctrl Pts',(3.39191284199994,2.2,-2.66858986100001));
#352191=CARTESIAN_POINT('Ctrl Pts',(3.39100370299994,12.2,-2.66698693500001));
#352192=CARTESIAN_POINT('Ctrl Pts',(3.39100370299994,5.2,-2.66698693500001));
#352193=CARTESIAN_POINT('Ctrl Pts',(3.39100370299994,2.2,-2.66698693500001));
#352194=CARTESIAN_POINT('Ctrl Pts',(3.39009486499994,12.2,-2.66538874400001));
#352195=CARTESIAN_POINT('Ctrl Pts',(3.39009486499994,5.2,-2.66538874400001));
#352196=CARTESIAN_POINT('Ctrl Pts',(3.39009486499994,2.2,-2.66538874400001));
#352197=CARTESIAN_POINT('Ctrl Pts',(3.38918633999994,12.2,-2.66379529100002));
#352198=CARTESIAN_POINT('Ctrl Pts',(3.38918633999994,5.2,-2.66379529100002));
#352199=CARTESIAN_POINT('Ctrl Pts',(3.38918633999994,2.2,-2.66379529100002));
#352200=CARTESIAN_POINT('Ctrl Pts',(3.38827813999994,12.2,-2.66220657700002));
#352201=CARTESIAN_POINT('Ctrl Pts',(3.38827813999994,5.2,-2.66220657700002));
#352202=CARTESIAN_POINT('Ctrl Pts',(3.38827813999994,2.2,-2.66220657700002));
#352203=CARTESIAN_POINT('Ctrl Pts',(3.38737027399994,12.2,-2.66062260600001));
#352204=CARTESIAN_POINT('Ctrl Pts',(3.38737027399994,5.2,-2.66062260600001));
#352205=CARTESIAN_POINT('Ctrl Pts',(3.38737027399994,2.2,-2.66062260600001));
#352206=CARTESIAN_POINT('Ctrl Pts',(3.38646275499995,12.2,-2.65904338000002));
#352207=CARTESIAN_POINT('Ctrl Pts',(3.38646275499995,5.2,-2.65904338000002));
#352208=CARTESIAN_POINT('Ctrl Pts',(3.38646275499995,2.2,-2.65904338000002));
#352209=CARTESIAN_POINT('Ctrl Pts',(3.38555559599994,12.2,-2.65746890100001));
#352210=CARTESIAN_POINT('Ctrl Pts',(3.38555559599994,5.2,-2.65746890100001));
#352211=CARTESIAN_POINT('Ctrl Pts',(3.38555559599994,2.2,-2.65746890100001));
#352212=CARTESIAN_POINT('Ctrl Pts',(3.38464880499994,12.2,-2.65589917200002));
#352213=CARTESIAN_POINT('Ctrl Pts',(3.38464880499994,5.2,-2.65589917200002));
#352214=CARTESIAN_POINT('Ctrl Pts',(3.38464880499994,2.2,-2.65589917200002));
#352215=CARTESIAN_POINT('Ctrl Pts',(3.38374239599994,12.2,-2.65433419300001));
#352216=CARTESIAN_POINT('Ctrl Pts',(3.38374239599994,5.2,-2.65433419300001));
#352217=CARTESIAN_POINT('Ctrl Pts',(3.38374239599994,2.2,-2.65433419300001));
#352218=CARTESIAN_POINT('Ctrl Pts',(3.38283637899994,12.2,-2.65277396800002));
#352219=CARTESIAN_POINT('Ctrl Pts',(3.38283637899994,5.2,-2.65277396800002));
#352220=CARTESIAN_POINT('Ctrl Pts',(3.38283637899994,2.2,-2.65277396800002));
#352221=CARTESIAN_POINT('Ctrl Pts',(3.38193076699994,12.2,-2.65121849900002));
#352222=CARTESIAN_POINT('Ctrl Pts',(3.38193076699994,5.2,-2.65121849900002));
#352223=CARTESIAN_POINT('Ctrl Pts',(3.38193076699994,2.2,-2.65121849900002));
#352224=CARTESIAN_POINT('Ctrl Pts',(3.38102557099994,12.2,-2.64966778900002));
#352225=CARTESIAN_POINT('Ctrl Pts',(3.38102557099994,5.2,-2.64966778900002));
#352226=CARTESIAN_POINT('Ctrl Pts',(3.38102557099994,2.2,-2.64966778900002));
#352227=CARTESIAN_POINT('Ctrl Pts',(3.38012080199994,12.2,-2.64812183900001));
#352228=CARTESIAN_POINT('Ctrl Pts',(3.38012080199994,5.2,-2.64812183900001));
#352229=CARTESIAN_POINT('Ctrl Pts',(3.38012080199994,2.2,-2.64812183900001));
#352230=CARTESIAN_POINT('Ctrl Pts',(3.37921647399994,12.2,-2.64658065300001));
#352231=CARTESIAN_POINT('Ctrl Pts',(3.37921647399994,5.2,-2.64658065300001));
#352232=CARTESIAN_POINT('Ctrl Pts',(3.37921647399994,2.2,-2.64658065300001));
#352233=CARTESIAN_POINT('Ctrl Pts',(3.37831259399994,12.2,-2.64504423000002));
#352234=CARTESIAN_POINT('Ctrl Pts',(3.37831259399994,5.2,-2.64504423000002));
#352235=CARTESIAN_POINT('Ctrl Pts',(3.37831259399994,2.2,-2.64504423000002));
#352236=CARTESIAN_POINT('Ctrl Pts',(3.37740917799994,12.2,-2.64351257600001));
#352237=CARTESIAN_POINT('Ctrl Pts',(3.37740917799994,5.2,-2.64351257600001));
#352238=CARTESIAN_POINT('Ctrl Pts',(3.37740917799994,2.2,-2.64351257600001));
#352239=CARTESIAN_POINT('Ctrl Pts',(3.37650623599994,12.2,-2.64198569100001));
#352240=CARTESIAN_POINT('Ctrl Pts',(3.37650623599994,5.2,-2.64198569100001));
#352241=CARTESIAN_POINT('Ctrl Pts',(3.37650623599994,2.2,-2.64198569100001));
#352242=CARTESIAN_POINT('Ctrl Pts',(3.37560377899994,12.2,-2.64046357700002));
#352243=CARTESIAN_POINT('Ctrl Pts',(3.37560377899994,5.2,-2.64046357700002));
#352244=CARTESIAN_POINT('Ctrl Pts',(3.37560377899994,2.2,-2.64046357700002));
#352245=CARTESIAN_POINT('Ctrl Pts',(3.37470181999994,12.2,-2.63894623700001));
#352246=CARTESIAN_POINT('Ctrl Pts',(3.37470181999994,5.2,-2.63894623700001));
#352247=CARTESIAN_POINT('Ctrl Pts',(3.37470181999994,2.2,-2.63894623700001));
#352248=CARTESIAN_POINT('Ctrl Pts',(3.37380037099994,12.2,-2.63743367300001));
#352249=CARTESIAN_POINT('Ctrl Pts',(3.37380037099994,5.2,-2.63743367300001));
#352250=CARTESIAN_POINT('Ctrl Pts',(3.37380037099994,2.2,-2.63743367300001));
#352251=CARTESIAN_POINT('Ctrl Pts',(3.37289944199994,12.2,-2.63592588700002));
#352252=CARTESIAN_POINT('Ctrl Pts',(3.37289944199994,5.2,-2.63592588700002));
#352253=CARTESIAN_POINT('Ctrl Pts',(3.37289944199994,2.2,-2.63592588700002));
#352254=CARTESIAN_POINT('Ctrl Pts',(3.37199904699995,12.2,-2.63442288100002));
#352255=CARTESIAN_POINT('Ctrl Pts',(3.37199904699995,5.2,-2.63442288100002));
#352256=CARTESIAN_POINT('Ctrl Pts',(3.37199904699995,2.2,-2.63442288100002));
#352257=CARTESIAN_POINT('Ctrl Pts',(3.37109919599994,12.2,-2.63292465700002));
#352258=CARTESIAN_POINT('Ctrl Pts',(3.37109919599994,5.2,-2.63292465700002));
#352259=CARTESIAN_POINT('Ctrl Pts',(3.37109919599994,2.2,-2.63292465700002));
#352260=CARTESIAN_POINT('Ctrl Pts',(3.37019990199994,12.2,-2.63143121700002));
#352261=CARTESIAN_POINT('Ctrl Pts',(3.37019990199994,5.2,-2.63143121700002));
#352262=CARTESIAN_POINT('Ctrl Pts',(3.37019990199994,2.2,-2.63143121700002));
#352263=CARTESIAN_POINT('Ctrl Pts',(3.36930117599994,12.2,-2.62994256500001));
#352264=CARTESIAN_POINT('Ctrl Pts',(3.36930117599994,5.2,-2.62994256500001));
#352265=CARTESIAN_POINT('Ctrl Pts',(3.36930117599994,2.2,-2.62994256500001));
#352266=CARTESIAN_POINT('Ctrl Pts',(3.36840302999994,12.2,-2.62845870100001));
#352267=CARTESIAN_POINT('Ctrl Pts',(3.36840302999994,5.2,-2.62845870100001));
#352268=CARTESIAN_POINT('Ctrl Pts',(3.36840302999994,2.2,-2.62845870100001));
#352269=CARTESIAN_POINT('Ctrl Pts',(3.36750547699994,12.2,-2.62697962700001));
#352270=CARTESIAN_POINT('Ctrl Pts',(3.36750547699994,5.2,-2.62697962700001));
#352271=CARTESIAN_POINT('Ctrl Pts',(3.36750547699994,2.2,-2.62697962700001));
#352272=CARTESIAN_POINT('Ctrl Pts',(3.36660852899994,12.2,-2.62550534600001));
#352273=CARTESIAN_POINT('Ctrl Pts',(3.36660852899994,5.2,-2.62550534600001));
#352274=CARTESIAN_POINT('Ctrl Pts',(3.36660852899994,2.2,-2.62550534600001));
#352275=CARTESIAN_POINT('Ctrl Pts',(3.36571219499994,12.2,-2.62403586000001));
#352276=CARTESIAN_POINT('Ctrl Pts',(3.36571219499994,5.2,-2.62403586000001));
#352277=CARTESIAN_POINT('Ctrl Pts',(3.36571219499994,2.2,-2.62403586000001));
#352278=CARTESIAN_POINT('Ctrl Pts',(3.36481649099994,12.2,-2.62257117000001));
#352279=CARTESIAN_POINT('Ctrl Pts',(3.36481649099994,5.2,-2.62257117000001));
#352280=CARTESIAN_POINT('Ctrl Pts',(3.36481649099994,2.2,-2.62257117000001));
#352281=CARTESIAN_POINT('Ctrl Pts',(3.36392142799995,12.2,-2.62111128000001));
#352282=CARTESIAN_POINT('Ctrl Pts',(3.36392142799995,5.2,-2.62111128000001));
#352283=CARTESIAN_POINT('Ctrl Pts',(3.36392142799995,2.2,-2.62111128000001));
#352284=CARTESIAN_POINT('Ctrl Pts',(3.36302701599994,12.2,-2.61965619000001));
#352285=CARTESIAN_POINT('Ctrl Pts',(3.36302701599994,5.2,-2.61965619000001));
#352286=CARTESIAN_POINT('Ctrl Pts',(3.36302701599994,2.2,-2.61965619000001));
#352287=CARTESIAN_POINT('Ctrl Pts',(3.36213326799994,12.2,-2.61820590300001));
#352288=CARTESIAN_POINT('Ctrl Pts',(3.36213326799994,5.2,-2.61820590300001));
#352289=CARTESIAN_POINT('Ctrl Pts',(3.36213326799994,2.2,-2.61820590300001));
#352290=CARTESIAN_POINT('Ctrl Pts',(3.36124019699994,12.2,-2.61676042000001));
#352291=CARTESIAN_POINT('Ctrl Pts',(3.36124019699994,5.2,-2.61676042000001));
#352292=CARTESIAN_POINT('Ctrl Pts',(3.36124019699994,2.2,-2.61676042000001));
#352293=CARTESIAN_POINT('Ctrl Pts',(3.36034781499994,12.2,-2.61531974400001));
#352294=CARTESIAN_POINT('Ctrl Pts',(3.36034781499994,5.2,-2.61531974400001));
#352295=CARTESIAN_POINT('Ctrl Pts',(3.36034781499994,2.2,-2.61531974400001));
#352296=CARTESIAN_POINT('Ctrl Pts',(3.35945613299995,12.2,-2.61388387700002));
#352297=CARTESIAN_POINT('Ctrl Pts',(3.35945613299995,5.2,-2.61388387700002));
#352298=CARTESIAN_POINT('Ctrl Pts',(3.35945613299995,2.2,-2.61388387700002));
#352299=CARTESIAN_POINT('Ctrl Pts',(3.35856516399994,12.2,-2.61245282100001));
#352300=CARTESIAN_POINT('Ctrl Pts',(3.35856516399994,5.2,-2.61245282100001));
#352301=CARTESIAN_POINT('Ctrl Pts',(3.35856516399994,2.2,-2.61245282100001));
#352302=CARTESIAN_POINT('Ctrl Pts',(3.35767492099994,12.2,-2.61102657700001));
#352303=CARTESIAN_POINT('Ctrl Pts',(3.35767492099994,5.2,-2.61102657700001));
#352304=CARTESIAN_POINT('Ctrl Pts',(3.35767492099994,2.2,-2.61102657700001));
#352305=CARTESIAN_POINT('Ctrl Pts',(3.35678541399994,12.2,-2.60960514700002));
#352306=CARTESIAN_POINT('Ctrl Pts',(3.35678541399994,5.2,-2.60960514700002));
#352307=CARTESIAN_POINT('Ctrl Pts',(3.35678541399994,2.2,-2.60960514700002));
#352308=CARTESIAN_POINT('Ctrl Pts',(3.35589665799994,12.2,-2.60818853300002));
#352309=CARTESIAN_POINT('Ctrl Pts',(3.35589665799994,5.2,-2.60818853300002));
#352310=CARTESIAN_POINT('Ctrl Pts',(3.35589665799994,2.2,-2.60818853300002));
#352311=CARTESIAN_POINT('Ctrl Pts',(3.35500866399994,12.2,-2.60677673900001));
#352312=CARTESIAN_POINT('Ctrl Pts',(3.35500866399994,5.2,-2.60677673900001));
#352313=CARTESIAN_POINT('Ctrl Pts',(3.35500866399994,2.2,-2.60677673900001));
#352314=CARTESIAN_POINT('Ctrl Pts',(3.35412144299994,12.2,-2.60536976400001));
#352315=CARTESIAN_POINT('Ctrl Pts',(3.35412144299994,5.2,-2.60536976400001));
#352316=CARTESIAN_POINT('Ctrl Pts',(3.35412144299994,2.2,-2.60536976400001));
#352317=CARTESIAN_POINT('Ctrl Pts',(3.35323500899994,12.2,-2.60396761000001));
#352318=CARTESIAN_POINT('Ctrl Pts',(3.35323500899994,5.2,-2.60396761000001));
#352319=CARTESIAN_POINT('Ctrl Pts',(3.35323500899994,2.2,-2.60396761000001));
#352320=CARTESIAN_POINT('Ctrl Pts',(3.35234937399994,12.2,-2.60257028200002));
#352321=CARTESIAN_POINT('Ctrl Pts',(3.35234937399994,5.2,-2.60257028200002));
#352322=CARTESIAN_POINT('Ctrl Pts',(3.35234937399994,2.2,-2.60257028200002));
#352323=CARTESIAN_POINT('Ctrl Pts',(3.35146454899995,12.2,-2.60117777900001));
#352324=CARTESIAN_POINT('Ctrl Pts',(3.35146454899995,5.2,-2.60117777900001));
#352325=CARTESIAN_POINT('Ctrl Pts',(3.35146454899995,2.2,-2.60117777900001));
#352326=CARTESIAN_POINT('Ctrl Pts',(3.35058054899994,12.2,-2.59979010200002));
#352327=CARTESIAN_POINT('Ctrl Pts',(3.35058054899994,5.2,-2.59979010200002));
#352328=CARTESIAN_POINT('Ctrl Pts',(3.35058054899994,2.2,-2.59979010200002));
#352329=CARTESIAN_POINT('Ctrl Pts',(3.34969738399994,12.2,-2.59840725600001));
#352330=CARTESIAN_POINT('Ctrl Pts',(3.34969738399994,5.2,-2.59840725600001));
#352331=CARTESIAN_POINT('Ctrl Pts',(3.34969738399994,2.2,-2.59840725600001));
#352332=CARTESIAN_POINT('Ctrl Pts',(3.34881506899994,12.2,-2.59702924100001));
#352333=CARTESIAN_POINT('Ctrl Pts',(3.34881506899994,5.2,-2.59702924100001));
#352334=CARTESIAN_POINT('Ctrl Pts',(3.34881506899994,2.2,-2.59702924100001));
#352335=CARTESIAN_POINT('Ctrl Pts',(3.34793361399994,12.2,-2.59565605800002));
#352336=CARTESIAN_POINT('Ctrl Pts',(3.34793361399994,5.2,-2.59565605800002));
#352337=CARTESIAN_POINT('Ctrl Pts',(3.34793361399994,2.2,-2.59565605800002));
#352338=CARTESIAN_POINT('Ctrl Pts',(3.34705303299994,12.2,-2.59428771000001));
#352339=CARTESIAN_POINT('Ctrl Pts',(3.34705303299994,5.2,-2.59428771000001));
#352340=CARTESIAN_POINT('Ctrl Pts',(3.34705303299994,2.2,-2.59428771000001));
#352341=CARTESIAN_POINT('Ctrl Pts',(3.34617333799994,12.2,-2.59292419800001));
#352342=CARTESIAN_POINT('Ctrl Pts',(3.34617333799994,5.2,-2.59292419800001));
#352343=CARTESIAN_POINT('Ctrl Pts',(3.34617333799994,2.2,-2.59292419800001));
#352344=CARTESIAN_POINT('Ctrl Pts',(3.34529454199994,12.2,-2.59156552500002));
#352345=CARTESIAN_POINT('Ctrl Pts',(3.34529454199994,5.2,-2.59156552500002));
#352346=CARTESIAN_POINT('Ctrl Pts',(3.34529454199994,2.2,-2.59156552500002));
#352347=CARTESIAN_POINT('Ctrl Pts',(3.34441665599994,12.2,-2.59021169100001));
#352348=CARTESIAN_POINT('Ctrl Pts',(3.34441665599994,5.2,-2.59021169100001));
#352349=CARTESIAN_POINT('Ctrl Pts',(3.34441665599994,2.2,-2.59021169100001));
#352350=CARTESIAN_POINT('Ctrl Pts',(3.34353969499994,12.2,-2.58886269900001));
#352351=CARTESIAN_POINT('Ctrl Pts',(3.34353969499994,5.2,-2.58886269900001));
#352352=CARTESIAN_POINT('Ctrl Pts',(3.34353969499994,2.2,-2.58886269900001));
#352353=CARTESIAN_POINT('Ctrl Pts',(3.34266366899994,12.2,-2.58751855100002));
#352354=CARTESIAN_POINT('Ctrl Pts',(3.34266366899994,5.2,-2.58751855100002));
#352355=CARTESIAN_POINT('Ctrl Pts',(3.34266366899994,2.2,-2.58751855100002));
#352356=CARTESIAN_POINT('Ctrl Pts',(3.34178859299994,12.2,-2.58617924600001));
#352357=CARTESIAN_POINT('Ctrl Pts',(3.34178859299994,5.2,-2.58617924600001));
#352358=CARTESIAN_POINT('Ctrl Pts',(3.34178859299994,2.2,-2.58617924600001));
#352359=CARTESIAN_POINT('Ctrl Pts',(3.34091447899994,12.2,-2.58484479000002));
#352360=CARTESIAN_POINT('Ctrl Pts',(3.34091447899994,5.2,-2.58484479000002));
#352361=CARTESIAN_POINT('Ctrl Pts',(3.34091447899994,2.2,-2.58484479000002));
#352362=CARTESIAN_POINT('Ctrl Pts',(3.34004133899994,12.2,-2.58351518100001));
#352363=CARTESIAN_POINT('Ctrl Pts',(3.34004133899994,5.2,-2.58351518100001));
#352364=CARTESIAN_POINT('Ctrl Pts',(3.34004133899994,2.2,-2.58351518100001));
#352365=CARTESIAN_POINT('Ctrl Pts',(3.33916918599994,12.2,-2.58219042200002));
#352366=CARTESIAN_POINT('Ctrl Pts',(3.33916918599994,5.2,-2.58219042200002));
#352367=CARTESIAN_POINT('Ctrl Pts',(3.33916918599994,2.2,-2.58219042200002));
#352368=CARTESIAN_POINT('Ctrl Pts',(3.33829803499994,12.2,-2.58087051500001));
#352369=CARTESIAN_POINT('Ctrl Pts',(3.33829803499994,5.2,-2.58087051500001));
#352370=CARTESIAN_POINT('Ctrl Pts',(3.33829803499994,2.2,-2.58087051500001));
#352371=CARTESIAN_POINT('Ctrl Pts',(3.33742789499994,12.2,-2.57955546100002));
#352372=CARTESIAN_POINT('Ctrl Pts',(3.33742789499994,5.2,-2.57955546100002));
#352373=CARTESIAN_POINT('Ctrl Pts',(3.33742789499994,2.2,-2.57955546100002));
#352374=CARTESIAN_POINT('Ctrl Pts',(3.33655878199994,12.2,-2.57824526200002));
#352375=CARTESIAN_POINT('Ctrl Pts',(3.33655878199994,5.2,-2.57824526200002));
#352376=CARTESIAN_POINT('Ctrl Pts',(3.33655878199994,2.2,-2.57824526200002));
#352377=CARTESIAN_POINT('Ctrl Pts',(3.33569070599995,12.2,-2.57693991900001));
#352378=CARTESIAN_POINT('Ctrl Pts',(3.33569070599995,5.2,-2.57693991900001));
#352379=CARTESIAN_POINT('Ctrl Pts',(3.33569070599995,2.2,-2.57693991900001));
#352380=CARTESIAN_POINT('Ctrl Pts',(3.33482368199994,12.2,-2.57563943400001));
#352381=CARTESIAN_POINT('Ctrl Pts',(3.33482368199994,5.2,-2.57563943400001));
#352382=CARTESIAN_POINT('Ctrl Pts',(3.33482368199994,2.2,-2.57563943400001));
#352383=CARTESIAN_POINT('Ctrl Pts',(3.33395772199995,12.2,-2.57434380900001));
#352384=CARTESIAN_POINT('Ctrl Pts',(3.33395772199995,5.2,-2.57434380900001));
#352385=CARTESIAN_POINT('Ctrl Pts',(3.33395772199995,2.2,-2.57434380900001));
#352386=CARTESIAN_POINT('Ctrl Pts',(3.33309283999994,12.2,-2.57305304400001));
#352387=CARTESIAN_POINT('Ctrl Pts',(3.33309283999994,5.2,-2.57305304400001));
#352388=CARTESIAN_POINT('Ctrl Pts',(3.33309283999994,2.2,-2.57305304400001));
#352389=CARTESIAN_POINT('Ctrl Pts',(3.33222904799995,12.2,-2.57176714300002));
#352390=CARTESIAN_POINT('Ctrl Pts',(3.33222904799995,5.2,-2.57176714300002));
#352391=CARTESIAN_POINT('Ctrl Pts',(3.33222904799995,2.2,-2.57176714300002));
#352392=CARTESIAN_POINT('Ctrl Pts',(3.33136635799994,12.2,-2.57048610500001));
#352393=CARTESIAN_POINT('Ctrl Pts',(3.33136635799994,5.2,-2.57048610500001));
#352394=CARTESIAN_POINT('Ctrl Pts',(3.33136635799994,2.2,-2.57048610500001));
#352395=CARTESIAN_POINT('Ctrl Pts',(3.33050478599994,12.2,-2.56920993400001));
#352396=CARTESIAN_POINT('Ctrl Pts',(3.33050478599994,5.2,-2.56920993400001));
#352397=CARTESIAN_POINT('Ctrl Pts',(3.33050478599994,2.2,-2.56920993400001));
#352398=CARTESIAN_POINT('Ctrl Pts',(3.32964434199994,12.2,-2.56793862900001));
#352399=CARTESIAN_POINT('Ctrl Pts',(3.32964434199994,5.2,-2.56793862900001));
#352400=CARTESIAN_POINT('Ctrl Pts',(3.32964434199994,2.2,-2.56793862900001));
#352401=CARTESIAN_POINT('Ctrl Pts',(3.32878504099994,12.2,-2.56667219300001));
#352402=CARTESIAN_POINT('Ctrl Pts',(3.32878504099994,5.2,-2.56667219300001));
#352403=CARTESIAN_POINT('Ctrl Pts',(3.32878504099994,2.2,-2.56667219300001));
#352404=CARTESIAN_POINT('Ctrl Pts',(3.32792689599994,12.2,-2.56541062700002));
#352405=CARTESIAN_POINT('Ctrl Pts',(3.32792689599994,5.2,-2.56541062700002));
#352406=CARTESIAN_POINT('Ctrl Pts',(3.32792689599994,2.2,-2.56541062700002));
#352407=CARTESIAN_POINT('Ctrl Pts',(3.32706991799995,12.2,-2.56415393300002));
#352408=CARTESIAN_POINT('Ctrl Pts',(3.32706991799995,5.2,-2.56415393300002));
#352409=CARTESIAN_POINT('Ctrl Pts',(3.32706991799995,2.2,-2.56415393300002));
#352410=CARTESIAN_POINT('Ctrl Pts',(3.32621412299994,12.2,-2.56290211100001));
#352411=CARTESIAN_POINT('Ctrl Pts',(3.32621412299994,5.2,-2.56290211100001));
#352412=CARTESIAN_POINT('Ctrl Pts',(3.32621412299994,2.2,-2.56290211100001));
#352413=CARTESIAN_POINT('Ctrl Pts',(3.32535952199994,12.2,-2.56165516400001));
#352414=CARTESIAN_POINT('Ctrl Pts',(3.32535952199994,5.2,-2.56165516400001));
#352415=CARTESIAN_POINT('Ctrl Pts',(3.32535952199994,2.2,-2.56165516400001));
#352416=CARTESIAN_POINT('Ctrl Pts',(3.32450612999994,12.2,-2.56041309300001));
#352417=CARTESIAN_POINT('Ctrl Pts',(3.32450612999994,5.2,-2.56041309300001));
#352418=CARTESIAN_POINT('Ctrl Pts',(3.32450612999994,2.2,-2.56041309300001));
#352419=CARTESIAN_POINT('Ctrl Pts',(3.32365395799994,12.2,-2.55917589900001));
#352420=CARTESIAN_POINT('Ctrl Pts',(3.32365395799994,5.2,-2.55917589900001));
#352421=CARTESIAN_POINT('Ctrl Pts',(3.32365395799994,2.2,-2.55917589900001));
#352422=CARTESIAN_POINT('Ctrl Pts',(3.32280302199994,12.2,-2.55794358200002));
#352423=CARTESIAN_POINT('Ctrl Pts',(3.32280302199994,5.2,-2.55794358200002));
#352424=CARTESIAN_POINT('Ctrl Pts',(3.32280302199994,2.2,-2.55794358200002));
#352425=CARTESIAN_POINT('Ctrl Pts',(3.32195333399994,12.2,-2.55671614800002));
#352426=CARTESIAN_POINT('Ctrl Pts',(3.32195333399994,5.2,-2.55671614800002));
#352427=CARTESIAN_POINT('Ctrl Pts',(3.32195333399994,2.2,-2.55671614800002));
#352428=CARTESIAN_POINT('Ctrl Pts',(3.32110490699994,12.2,-2.55549359300002));
#352429=CARTESIAN_POINT('Ctrl Pts',(3.32110490699994,5.2,-2.55549359300002));
#352430=CARTESIAN_POINT('Ctrl Pts',(3.32110490699994,2.2,-2.55549359300002));
#352431=CARTESIAN_POINT('Ctrl Pts',(3.32025775399994,12.2,-2.55427592000002));
#352432=CARTESIAN_POINT('Ctrl Pts',(3.32025775399994,5.2,-2.55427592000002));
#352433=CARTESIAN_POINT('Ctrl Pts',(3.32025775399994,2.2,-2.55427592000002));
#352434=CARTESIAN_POINT('Ctrl Pts',(3.31941188999994,12.2,-2.55306313200002));
#352435=CARTESIAN_POINT('Ctrl Pts',(3.31941188999994,5.2,-2.55306313200002));
#352436=CARTESIAN_POINT('Ctrl Pts',(3.31941188999994,2.2,-2.55306313200002));
#352437=CARTESIAN_POINT('Ctrl Pts',(3.31856732599995,12.2,-2.55185522900002));
#352438=CARTESIAN_POINT('Ctrl Pts',(3.31856732599995,5.2,-2.55185522900002));
#352439=CARTESIAN_POINT('Ctrl Pts',(3.31856732599995,2.2,-2.55185522900002));
#352440=CARTESIAN_POINT('Ctrl Pts',(3.31772407899994,12.2,-2.55065221300002));
#352441=CARTESIAN_POINT('Ctrl Pts',(3.31772407899994,5.2,-2.55065221300002));
#352442=CARTESIAN_POINT('Ctrl Pts',(3.31772407899994,2.2,-2.55065221300002));
#352443=CARTESIAN_POINT('Ctrl Pts',(3.31688215899994,12.2,-2.54945408300001));
#352444=CARTESIAN_POINT('Ctrl Pts',(3.31688215899994,5.2,-2.54945408300001));
#352445=CARTESIAN_POINT('Ctrl Pts',(3.31688215899994,2.2,-2.54945408300001));
#352446=CARTESIAN_POINT('Ctrl Pts',(3.31604158099994,12.2,-2.54826084400001));
#352447=CARTESIAN_POINT('Ctrl Pts',(3.31604158099994,5.2,-2.54826084400001));
#352448=CARTESIAN_POINT('Ctrl Pts',(3.31604158099994,2.2,-2.54826084400001));
#352449=CARTESIAN_POINT('Ctrl Pts',(3.31520235799994,12.2,-2.54707249400001));
#352450=CARTESIAN_POINT('Ctrl Pts',(3.31520235799994,5.2,-2.54707249400001));
#352451=CARTESIAN_POINT('Ctrl Pts',(3.31520235799994,2.2,-2.54707249400001));
#352452=CARTESIAN_POINT('Ctrl Pts',(3.31436450499994,12.2,-2.54588903500002));
#352453=CARTESIAN_POINT('Ctrl Pts',(3.31436450499994,5.2,-2.54588903500002));
#352454=CARTESIAN_POINT('Ctrl Pts',(3.31436450499994,2.2,-2.54588903500002));
#352455=CARTESIAN_POINT('Ctrl Pts',(3.31352803299994,12.2,-2.54471047000001));
#352456=CARTESIAN_POINT('Ctrl Pts',(3.31352803299994,5.2,-2.54471047000001));
#352457=CARTESIAN_POINT('Ctrl Pts',(3.31352803299994,2.2,-2.54471047000001));
#352458=CARTESIAN_POINT('Ctrl Pts',(3.31269295899994,12.2,-2.54353679800001));
#352459=CARTESIAN_POINT('Ctrl Pts',(3.31269295899994,5.2,-2.54353679800001));
#352460=CARTESIAN_POINT('Ctrl Pts',(3.31269295899994,2.2,-2.54353679800001));
#352461=CARTESIAN_POINT('Ctrl Pts',(3.31185929299994,12.2,-2.54236802100001));
#352462=CARTESIAN_POINT('Ctrl Pts',(3.31185929299994,5.2,-2.54236802100001));
#352463=CARTESIAN_POINT('Ctrl Pts',(3.31185929299994,2.2,-2.54236802100001));
#352464=CARTESIAN_POINT('Ctrl Pts',(3.31102705199994,12.2,-2.54120414000001));
#352465=CARTESIAN_POINT('Ctrl Pts',(3.31102705199994,5.2,-2.54120414000001));
#352466=CARTESIAN_POINT('Ctrl Pts',(3.31102705199994,2.2,-2.54120414000001));
#352467=CARTESIAN_POINT('Ctrl Pts',(3.31019624799994,12.2,-2.54004515600001));
#352468=CARTESIAN_POINT('Ctrl Pts',(3.31019624799994,5.2,-2.54004515600001));
#352469=CARTESIAN_POINT('Ctrl Pts',(3.31019624799994,2.2,-2.54004515600001));
#352470=CARTESIAN_POINT('Ctrl Pts',(3.30936689399994,12.2,-2.53889107200001));
#352471=CARTESIAN_POINT('Ctrl Pts',(3.30936689399994,5.2,-2.53889107200001));
#352472=CARTESIAN_POINT('Ctrl Pts',(3.30936689399994,2.2,-2.53889107200001));
#352473=CARTESIAN_POINT('Ctrl Pts',(3.30853900499994,12.2,-2.53774188600001));
#352474=CARTESIAN_POINT('Ctrl Pts',(3.30853900499994,5.2,-2.53774188600001));
#352475=CARTESIAN_POINT('Ctrl Pts',(3.30853900499994,2.2,-2.53774188600001));
#352476=CARTESIAN_POINT('Ctrl Pts',(3.30771259499994,12.2,-2.53659760000001));
#352477=CARTESIAN_POINT('Ctrl Pts',(3.30771259499994,5.2,-2.53659760000001));
#352478=CARTESIAN_POINT('Ctrl Pts',(3.30771259499994,2.2,-2.53659760000001));
#352479=CARTESIAN_POINT('Ctrl Pts',(3.30688767699994,12.2,-2.53545821700001));
#352480=CARTESIAN_POINT('Ctrl Pts',(3.30688767699994,5.2,-2.53545821700001));
#352481=CARTESIAN_POINT('Ctrl Pts',(3.30688767699994,2.2,-2.53545821700001));
#352482=CARTESIAN_POINT('Ctrl Pts',(3.30606426599994,12.2,-2.53432373600001));
#352483=CARTESIAN_POINT('Ctrl Pts',(3.30606426599994,5.2,-2.53432373600001));
#352484=CARTESIAN_POINT('Ctrl Pts',(3.30606426599994,2.2,-2.53432373600001));
#352485=CARTESIAN_POINT('Ctrl Pts',(3.30524237399994,12.2,-2.53319416000001));
#352486=CARTESIAN_POINT('Ctrl Pts',(3.30524237399994,5.2,-2.53319416000001));
#352487=CARTESIAN_POINT('Ctrl Pts',(3.30524237399994,2.2,-2.53319416000001));
#352488=CARTESIAN_POINT('Ctrl Pts',(3.30442201699995,12.2,-2.53206948800001));
#352489=CARTESIAN_POINT('Ctrl Pts',(3.30442201699995,5.2,-2.53206948800001));
#352490=CARTESIAN_POINT('Ctrl Pts',(3.30442201699995,2.2,-2.53206948800001));
#352491=CARTESIAN_POINT('Ctrl Pts',(3.30360320699994,12.2,-2.53094972100001));
#352492=CARTESIAN_POINT('Ctrl Pts',(3.30360320699994,5.2,-2.53094972100001));
#352493=CARTESIAN_POINT('Ctrl Pts',(3.30360320699994,2.2,-2.53094972100001));
#352494=CARTESIAN_POINT('Ctrl Pts',(3.30278595899994,12.2,-2.52983486200002));
#352495=CARTESIAN_POINT('Ctrl Pts',(3.30278595899994,5.2,-2.52983486200002));
#352496=CARTESIAN_POINT('Ctrl Pts',(3.30278595899994,2.2,-2.52983486200002));
#352497=CARTESIAN_POINT('Ctrl Pts',(3.30197028899994,12.2,-2.52872491000002));
#352498=CARTESIAN_POINT('Ctrl Pts',(3.30197028899994,5.2,-2.52872491000002));
#352499=CARTESIAN_POINT('Ctrl Pts',(3.30197028899994,2.2,-2.52872491000002));
#352500=CARTESIAN_POINT('Ctrl Pts',(3.30115620599994,12.2,-2.52761986800001));
#352501=CARTESIAN_POINT('Ctrl Pts',(3.30115620599994,5.2,-2.52761986800001));
#352502=CARTESIAN_POINT('Ctrl Pts',(3.30115620599994,2.2,-2.52761986800001));
#352503=CARTESIAN_POINT('Ctrl Pts',(3.30034372899994,12.2,-2.52651973400001));
#352504=CARTESIAN_POINT('Ctrl Pts',(3.30034372899994,5.2,-2.52651973400001));
#352505=CARTESIAN_POINT('Ctrl Pts',(3.30034372899994,2.2,-2.52651973400001));
#352506=CARTESIAN_POINT('Ctrl Pts',(3.29953286999995,12.2,-2.52542451100001));
#352507=CARTESIAN_POINT('Ctrl Pts',(3.29953286999995,5.2,-2.52542451100001));
#352508=CARTESIAN_POINT('Ctrl Pts',(3.29953286999995,2.2,-2.52542451100001));
#352509=CARTESIAN_POINT('Ctrl Pts',(3.29872364399994,12.2,-2.52433420000001));
#352510=CARTESIAN_POINT('Ctrl Pts',(3.29872364399994,5.2,-2.52433420000001));
#352511=CARTESIAN_POINT('Ctrl Pts',(3.29872364399994,2.2,-2.52433420000001));
#352512=CARTESIAN_POINT('Ctrl Pts',(3.29791606299994,12.2,-2.52324880100002));
#352513=CARTESIAN_POINT('Ctrl Pts',(3.29791606299994,5.2,-2.52324880100002));
#352514=CARTESIAN_POINT('Ctrl Pts',(3.29791606299994,2.2,-2.52324880100002));
#352515=CARTESIAN_POINT('Ctrl Pts',(3.29711014399994,12.2,-2.52216831700002));
#352516=CARTESIAN_POINT('Ctrl Pts',(3.29711014399994,5.2,-2.52216831700002));
#352517=CARTESIAN_POINT('Ctrl Pts',(3.29711014399994,2.2,-2.52216831700002));
#352518=CARTESIAN_POINT('Ctrl Pts',(3.29630589899994,12.2,-2.52109274600001));
#352519=CARTESIAN_POINT('Ctrl Pts',(3.29630589899994,5.2,-2.52109274600001));
#352520=CARTESIAN_POINT('Ctrl Pts',(3.29630589899994,2.2,-2.52109274600001));
#352521=CARTESIAN_POINT('Ctrl Pts',(3.29550334399995,12.2,-2.52002208900001));
#352522=CARTESIAN_POINT('Ctrl Pts',(3.29550334399995,5.2,-2.52002208900001));
#352523=CARTESIAN_POINT('Ctrl Pts',(3.29550334399995,2.2,-2.52002208900001));
#352524=CARTESIAN_POINT('Ctrl Pts',(3.29470249199994,12.2,-2.51895634900002));
#352525=CARTESIAN_POINT('Ctrl Pts',(3.29470249199994,5.2,-2.51895634900002));
#352526=CARTESIAN_POINT('Ctrl Pts',(3.29470249199994,2.2,-2.51895634900002));
#352527=CARTESIAN_POINT('Ctrl Pts',(3.29390335899994,12.2,-2.51789552600002));
#352528=CARTESIAN_POINT('Ctrl Pts',(3.29390335899994,5.2,-2.51789552600002));
#352529=CARTESIAN_POINT('Ctrl Pts',(3.29390335899994,2.2,-2.51789552600002));
#352530=CARTESIAN_POINT('Ctrl Pts',(3.29310595699994,12.2,-2.51683961900001));
#352531=CARTESIAN_POINT('Ctrl Pts',(3.29310595699994,5.2,-2.51683961900001));
#352532=CARTESIAN_POINT('Ctrl Pts',(3.29310595699994,2.2,-2.51683961900001));
#352533=CARTESIAN_POINT('Ctrl Pts',(3.29231030199994,12.2,-2.51578863100002));
#352534=CARTESIAN_POINT('Ctrl Pts',(3.29231030199994,5.2,-2.51578863100002));
#352535=CARTESIAN_POINT('Ctrl Pts',(3.29231030199994,2.2,-2.51578863100002));
#352536=CARTESIAN_POINT('Ctrl Pts',(3.29151640799994,12.2,-2.51474256300002));
#352537=CARTESIAN_POINT('Ctrl Pts',(3.29151640799994,5.2,-2.51474256300002));
#352538=CARTESIAN_POINT('Ctrl Pts',(3.29151640799994,2.2,-2.51474256300002));
#352539=CARTESIAN_POINT('Ctrl Pts',(3.29072428899994,12.2,-2.51370141400002));
#352540=CARTESIAN_POINT('Ctrl Pts',(3.29072428899994,5.2,-2.51370141400002));
#352541=CARTESIAN_POINT('Ctrl Pts',(3.29072428899994,2.2,-2.51370141400002));
#352542=CARTESIAN_POINT('Ctrl Pts',(3.28993396199994,12.2,-2.51266518600001));
#352543=CARTESIAN_POINT('Ctrl Pts',(3.28993396199994,5.2,-2.51266518600001));
#352544=CARTESIAN_POINT('Ctrl Pts',(3.28993396199994,2.2,-2.51266518600001));
#352545=CARTESIAN_POINT('Ctrl Pts',(3.28914543799995,12.2,-2.51163387800001));
#352546=CARTESIAN_POINT('Ctrl Pts',(3.28914543799995,5.2,-2.51163387800001));
#352547=CARTESIAN_POINT('Ctrl Pts',(3.28914543799995,2.2,-2.51163387800001));
#352548=CARTESIAN_POINT('Ctrl Pts',(3.28835873299994,12.2,-2.51060749200001));
#352549=CARTESIAN_POINT('Ctrl Pts',(3.28835873299994,5.2,-2.51060749200001));
#352550=CARTESIAN_POINT('Ctrl Pts',(3.28835873299994,2.2,-2.51060749200001));
#352551=CARTESIAN_POINT('Ctrl Pts',(3.28757386299994,12.2,-2.50958602900001));
#352552=CARTESIAN_POINT('Ctrl Pts',(3.28757386299994,5.2,-2.50958602900001));
#352553=CARTESIAN_POINT('Ctrl Pts',(3.28757386299994,2.2,-2.50958602900001));
#352554=CARTESIAN_POINT('Ctrl Pts',(3.28679083999994,12.2,-2.50856948900001));
#352555=CARTESIAN_POINT('Ctrl Pts',(3.28679083999994,5.2,-2.50856948900001));
#352556=CARTESIAN_POINT('Ctrl Pts',(3.28679083999994,2.2,-2.50856948900001));
#352557=CARTESIAN_POINT('Ctrl Pts',(3.28600967999995,12.2,-2.50755787300001));
#352558=CARTESIAN_POINT('Ctrl Pts',(3.28600967999995,5.2,-2.50755787300001));
#352559=CARTESIAN_POINT('Ctrl Pts',(3.28600967999995,2.2,-2.50755787300001));
#352560=CARTESIAN_POINT('Ctrl Pts',(3.28523039899994,12.2,-2.50655118100001));
#352561=CARTESIAN_POINT('Ctrl Pts',(3.28523039899994,5.2,-2.50655118100001));
#352562=CARTESIAN_POINT('Ctrl Pts',(3.28523039899994,2.2,-2.50655118100001));
#352563=CARTESIAN_POINT('Ctrl Pts',(3.28445300899994,12.2,-2.50554941500001));
#352564=CARTESIAN_POINT('Ctrl Pts',(3.28445300899994,5.2,-2.50554941500001));
#352565=CARTESIAN_POINT('Ctrl Pts',(3.28445300899994,2.2,-2.50554941500001));
#352566=CARTESIAN_POINT('Ctrl Pts',(3.28367752699994,12.2,-2.50455257400001));
#352567=CARTESIAN_POINT('Ctrl Pts',(3.28367752699994,5.2,-2.50455257400001));
#352568=CARTESIAN_POINT('Ctrl Pts',(3.28367752699994,2.2,-2.50455257400001));
#352569=CARTESIAN_POINT('Ctrl Pts',(3.28290396699995,12.2,-2.50356065900001));
#352570=CARTESIAN_POINT('Ctrl Pts',(3.28290396699995,5.2,-2.50356065900001));
#352571=CARTESIAN_POINT('Ctrl Pts',(3.28290396699995,2.2,-2.50356065900001));
#352572=CARTESIAN_POINT('Ctrl Pts',(3.28213234399994,12.2,-2.50257367100001));
#352573=CARTESIAN_POINT('Ctrl Pts',(3.28213234399994,5.2,-2.50257367100001));
#352574=CARTESIAN_POINT('Ctrl Pts',(3.28213234399994,2.2,-2.50257367100001));
#352575=CARTESIAN_POINT('Ctrl Pts',(3.28136267199994,12.2,-2.50159161100001));
#352576=CARTESIAN_POINT('Ctrl Pts',(3.28136267199994,5.2,-2.50159161100001));
#352577=CARTESIAN_POINT('Ctrl Pts',(3.28136267199994,2.2,-2.50159161100001));
#352578=CARTESIAN_POINT('Ctrl Pts',(3.28059496699994,12.2,-2.50061447800002));
#352579=CARTESIAN_POINT('Ctrl Pts',(3.28059496699994,5.2,-2.50061447800002));
#352580=CARTESIAN_POINT('Ctrl Pts',(3.28059496699994,2.2,-2.50061447800002));
#352581=CARTESIAN_POINT('Ctrl Pts',(3.27982924299994,12.2,-2.49964227300001));
#352582=CARTESIAN_POINT('Ctrl Pts',(3.27982924299994,5.2,-2.49964227300001));
#352583=CARTESIAN_POINT('Ctrl Pts',(3.27982924299994,2.2,-2.49964227300001));
#352584=CARTESIAN_POINT('Ctrl Pts',(3.27906551599995,12.2,-2.49867499700001));
#352585=CARTESIAN_POINT('Ctrl Pts',(3.27906551599995,5.2,-2.49867499700001));
#352586=CARTESIAN_POINT('Ctrl Pts',(3.27906551599995,2.2,-2.49867499700001));
#352587=CARTESIAN_POINT('Ctrl Pts',(3.27830380099994,12.2,-2.49771265100001));
#352588=CARTESIAN_POINT('Ctrl Pts',(3.27830380099994,5.2,-2.49771265100001));
#352589=CARTESIAN_POINT('Ctrl Pts',(3.27830380099994,2.2,-2.49771265100001));
#352590=CARTESIAN_POINT('Ctrl Pts',(3.27754411199995,12.2,-2.49675523400001));
#352591=CARTESIAN_POINT('Ctrl Pts',(3.27754411199995,5.2,-2.49675523400001));
#352592=CARTESIAN_POINT('Ctrl Pts',(3.27754411199995,2.2,-2.49675523400001));
#352593=CARTESIAN_POINT('Ctrl Pts',(3.27678646399994,12.2,-2.49580274700001));
#352594=CARTESIAN_POINT('Ctrl Pts',(3.27678646399994,5.2,-2.49580274700001));
#352595=CARTESIAN_POINT('Ctrl Pts',(3.27678646399994,2.2,-2.49580274700001));
#352596=CARTESIAN_POINT('Ctrl Pts',(3.27603087399994,12.2,-2.49485519100002));
#352597=CARTESIAN_POINT('Ctrl Pts',(3.27603087399994,5.2,-2.49485519100002));
#352598=CARTESIAN_POINT('Ctrl Pts',(3.27603087399994,2.2,-2.49485519100002));
#352599=CARTESIAN_POINT('Ctrl Pts',(3.27527735399994,12.2,-2.49391256500001));
#352600=CARTESIAN_POINT('Ctrl Pts',(3.27527735399994,5.2,-2.49391256500001));
#352601=CARTESIAN_POINT('Ctrl Pts',(3.27527735399994,2.2,-2.49391256500001));
#352602=CARTESIAN_POINT('Ctrl Pts',(3.27452592299994,12.2,-2.49297487000002));
#352603=CARTESIAN_POINT('Ctrl Pts',(3.27452592299994,5.2,-2.49297487000002));
#352604=CARTESIAN_POINT('Ctrl Pts',(3.27452592299994,2.2,-2.49297487000002));
#352605=CARTESIAN_POINT('Ctrl Pts',(3.27377659299994,12.2,-2.49204210700002));
#352606=CARTESIAN_POINT('Ctrl Pts',(3.27377659299994,5.2,-2.49204210700002));
#352607=CARTESIAN_POINT('Ctrl Pts',(3.27377659299994,2.2,-2.49204210700002));
#352608=CARTESIAN_POINT('Ctrl Pts',(3.27302938099994,12.2,-2.49111427700001));
#352609=CARTESIAN_POINT('Ctrl Pts',(3.27302938099994,5.2,-2.49111427700001));
#352610=CARTESIAN_POINT('Ctrl Pts',(3.27302938099994,2.2,-2.49111427700001));
#352611=CARTESIAN_POINT('Ctrl Pts',(3.27228430099994,12.2,-2.49019137800001));
#352612=CARTESIAN_POINT('Ctrl Pts',(3.27228430099994,5.2,-2.49019137800001));
#352613=CARTESIAN_POINT('Ctrl Pts',(3.27228430099994,2.2,-2.49019137800001));
#352614=CARTESIAN_POINT('Ctrl Pts',(3.27154136999994,12.2,-2.48927341100002));
#352615=CARTESIAN_POINT('Ctrl Pts',(3.27154136999994,5.2,-2.48927341100002));
#352616=CARTESIAN_POINT('Ctrl Pts',(3.27154136999994,2.2,-2.48927341100002));
#352617=CARTESIAN_POINT('Ctrl Pts',(3.27080060199994,12.2,-2.48836037800002));
#352618=CARTESIAN_POINT('Ctrl Pts',(3.27080060199994,5.2,-2.48836037800002));
#352619=CARTESIAN_POINT('Ctrl Pts',(3.27080060199994,2.2,-2.48836037800002));
#352620=CARTESIAN_POINT('Ctrl Pts',(3.27006201299994,12.2,-2.48745227700002));
#352621=CARTESIAN_POINT('Ctrl Pts',(3.27006201299994,5.2,-2.48745227700002));
#352622=CARTESIAN_POINT('Ctrl Pts',(3.27006201299994,2.2,-2.48745227700002));
#352623=CARTESIAN_POINT('Ctrl Pts',(3.26932561799994,12.2,-2.48654910900001));
#352624=CARTESIAN_POINT('Ctrl Pts',(3.26932561799994,5.2,-2.48654910900001));
#352625=CARTESIAN_POINT('Ctrl Pts',(3.26932561799994,2.2,-2.48654910900001));
#352626=CARTESIAN_POINT('Ctrl Pts',(3.26859143299994,12.2,-2.48565087500001));
#352627=CARTESIAN_POINT('Ctrl Pts',(3.26859143299994,5.2,-2.48565087500001));
#352628=CARTESIAN_POINT('Ctrl Pts',(3.26859143299994,2.2,-2.48565087500001));
#352629=CARTESIAN_POINT('Ctrl Pts',(3.26785947299994,12.2,-2.48475757400001));
#352630=CARTESIAN_POINT('Ctrl Pts',(3.26785947299994,5.2,-2.48475757400001));
#352631=CARTESIAN_POINT('Ctrl Pts',(3.26785947299994,2.2,-2.48475757400001));
#352632=CARTESIAN_POINT('Ctrl Pts',(3.26712975399994,12.2,-2.48386920800002));
#352633=CARTESIAN_POINT('Ctrl Pts',(3.26712975399994,5.2,-2.48386920800002));
#352634=CARTESIAN_POINT('Ctrl Pts',(3.26712975399994,2.2,-2.48386920800002));
#352635=CARTESIAN_POINT('Ctrl Pts',(3.26640229099994,12.2,-2.48298577500002));
#352636=CARTESIAN_POINT('Ctrl Pts',(3.26640229099994,5.2,-2.48298577500002));
#352637=CARTESIAN_POINT('Ctrl Pts',(3.26640229099994,2.2,-2.48298577500002));
#352638=CARTESIAN_POINT('Ctrl Pts',(3.26567710099994,12.2,-2.48210727600001));
#352639=CARTESIAN_POINT('Ctrl Pts',(3.26567710099994,5.2,-2.48210727600001));
#352640=CARTESIAN_POINT('Ctrl Pts',(3.26567710099994,2.2,-2.48210727600001));
#352641=CARTESIAN_POINT('Ctrl Pts',(3.26495419599994,12.2,-2.48123371200001));
#352642=CARTESIAN_POINT('Ctrl Pts',(3.26495419599994,5.2,-2.48123371200001));
#352643=CARTESIAN_POINT('Ctrl Pts',(3.26495419599994,2.2,-2.48123371200001));
#352644=CARTESIAN_POINT('Ctrl Pts',(3.26423359699994,12.2,-2.48036508100002));
#352645=CARTESIAN_POINT('Ctrl Pts',(3.26423359699994,5.2,-2.48036508100002));
#352646=CARTESIAN_POINT('Ctrl Pts',(3.26423359699994,2.2,-2.48036508100002));
#352647=CARTESIAN_POINT('Ctrl Pts',(3.26351531599995,12.2,-2.47950138600002));
#352648=CARTESIAN_POINT('Ctrl Pts',(3.26351531599995,5.2,-2.47950138600002));
#352649=CARTESIAN_POINT('Ctrl Pts',(3.26351531599995,2.2,-2.47950138600002));
#352650=CARTESIAN_POINT('Ctrl Pts',(3.26279936899994,12.2,-2.47864262300002));
#352651=CARTESIAN_POINT('Ctrl Pts',(3.26279936899994,5.2,-2.47864262300002));
#352652=CARTESIAN_POINT('Ctrl Pts',(3.26279936899994,2.2,-2.47864262300002));
#352653=CARTESIAN_POINT('Ctrl Pts',(3.26208577399994,12.2,-2.47778879600002));
#352654=CARTESIAN_POINT('Ctrl Pts',(3.26208577399994,5.2,-2.47778879600002));
#352655=CARTESIAN_POINT('Ctrl Pts',(3.26208577399994,2.2,-2.47778879600002));
#352656=CARTESIAN_POINT('Ctrl Pts',(3.26137454399994,12.2,-2.47693990400002));
#352657=CARTESIAN_POINT('Ctrl Pts',(3.26137454399994,5.2,-2.47693990400002));
#352658=CARTESIAN_POINT('Ctrl Pts',(3.26137454399994,2.2,-2.47693990400002));
#352659=CARTESIAN_POINT('Ctrl Pts',(3.26066569699994,12.2,-2.47609594400001));
#352660=CARTESIAN_POINT('Ctrl Pts',(3.26066569699994,5.2,-2.47609594400001));
#352661=CARTESIAN_POINT('Ctrl Pts',(3.26066569699994,2.2,-2.47609594400001));
#352662=CARTESIAN_POINT('Ctrl Pts',(3.25995924799994,12.2,-2.47525692100002));
#352663=CARTESIAN_POINT('Ctrl Pts',(3.25995924799994,5.2,-2.47525692100002));
#352664=CARTESIAN_POINT('Ctrl Pts',(3.25995924799994,2.2,-2.47525692100002));
#352665=CARTESIAN_POINT('Ctrl Pts',(3.25925521399994,12.2,-2.47442283100002));
#352666=CARTESIAN_POINT('Ctrl Pts',(3.25925521399994,5.2,-2.47442283100002));
#352667=CARTESIAN_POINT('Ctrl Pts',(3.25925521399994,2.2,-2.47442283100002));
#352668=CARTESIAN_POINT('Ctrl Pts',(3.25855360899994,12.2,-2.47359367500001));
#352669=CARTESIAN_POINT('Ctrl Pts',(3.25855360899994,5.2,-2.47359367500001));
#352670=CARTESIAN_POINT('Ctrl Pts',(3.25855360899994,2.2,-2.47359367500001));
#352671=CARTESIAN_POINT('Ctrl Pts',(3.25785445099994,12.2,-2.47276945400001));
#352672=CARTESIAN_POINT('Ctrl Pts',(3.25785445099994,5.2,-2.47276945400001));
#352673=CARTESIAN_POINT('Ctrl Pts',(3.25785445099994,2.2,-2.47276945400001));
#352674=CARTESIAN_POINT('Ctrl Pts',(3.25715775499994,12.2,-2.47195016500001));
#352675=CARTESIAN_POINT('Ctrl Pts',(3.25715775499994,5.2,-2.47195016500001));
#352676=CARTESIAN_POINT('Ctrl Pts',(3.25715775499994,2.2,-2.47195016500001));
#352677=CARTESIAN_POINT('Ctrl Pts',(3.25646353699995,12.2,-2.47113581200002));
#352678=CARTESIAN_POINT('Ctrl Pts',(3.25646353699995,5.2,-2.47113581200002));
#352679=CARTESIAN_POINT('Ctrl Pts',(3.25646353699995,2.2,-2.47113581200002));
#352680=CARTESIAN_POINT('Ctrl Pts',(3.25577181299994,12.2,-2.47032639200001));
#352681=CARTESIAN_POINT('Ctrl Pts',(3.25577181299994,5.2,-2.47032639200001));
#352682=CARTESIAN_POINT('Ctrl Pts',(3.25577181299994,2.2,-2.47032639200001));
#352683=CARTESIAN_POINT('Ctrl Pts',(3.25508260099994,12.2,-2.46952190600001));
#352684=CARTESIAN_POINT('Ctrl Pts',(3.25508260099994,5.2,-2.46952190600001));
#352685=CARTESIAN_POINT('Ctrl Pts',(3.25508260099994,2.2,-2.46952190600001));
#352686=CARTESIAN_POINT('Ctrl Pts',(3.25439591399994,12.2,-2.46872235300001));
#352687=CARTESIAN_POINT('Ctrl Pts',(3.25439591399994,5.2,-2.46872235300001));
#352688=CARTESIAN_POINT('Ctrl Pts',(3.25439591399994,2.2,-2.46872235300001));
#352689=CARTESIAN_POINT('Ctrl Pts',(3.25371177099994,12.2,-2.46792773300001));
#352690=CARTESIAN_POINT('Ctrl Pts',(3.25371177099994,5.2,-2.46792773300001));
#352691=CARTESIAN_POINT('Ctrl Pts',(3.25371177099994,2.2,-2.46792773300001));
#352692=CARTESIAN_POINT('Ctrl Pts',(3.25303018899994,12.2,-2.46713804600001));
#352693=CARTESIAN_POINT('Ctrl Pts',(3.25303018899994,5.2,-2.46713804600001));
#352694=CARTESIAN_POINT('Ctrl Pts',(3.25303018899994,2.2,-2.46713804600001));
#352695=CARTESIAN_POINT('Ctrl Pts',(3.25235118099994,12.2,-2.46635329200001));
#352696=CARTESIAN_POINT('Ctrl Pts',(3.25235118099994,5.2,-2.46635329200001));
#352697=CARTESIAN_POINT('Ctrl Pts',(3.25235118099994,2.2,-2.46635329200001));
#352698=CARTESIAN_POINT('Ctrl Pts',(3.25167476499994,12.2,-2.46557346900001));
#352699=CARTESIAN_POINT('Ctrl Pts',(3.25167476499994,5.2,-2.46557346900001));
#352700=CARTESIAN_POINT('Ctrl Pts',(3.25167476499994,2.2,-2.46557346900001));
#352701=CARTESIAN_POINT('Ctrl Pts',(3.25100095899994,12.2,-2.46479857900002));
#352702=CARTESIAN_POINT('Ctrl Pts',(3.25100095899994,5.2,-2.46479857900002));
#352703=CARTESIAN_POINT('Ctrl Pts',(3.25100095899994,2.2,-2.46479857900002));
#352704=CARTESIAN_POINT('Ctrl Pts',(3.25032977699995,12.2,-2.46402862100001));
#352705=CARTESIAN_POINT('Ctrl Pts',(3.25032977699995,5.2,-2.46402862100001));
#352706=CARTESIAN_POINT('Ctrl Pts',(3.25032977699995,2.2,-2.46402862100001));
#352707=CARTESIAN_POINT('Ctrl Pts',(3.24966123699994,12.2,-2.46326359400001));
#352708=CARTESIAN_POINT('Ctrl Pts',(3.24966123699994,5.2,-2.46326359400001));
#352709=CARTESIAN_POINT('Ctrl Pts',(3.24966123699994,2.2,-2.46326359400001));
#352710=CARTESIAN_POINT('Ctrl Pts',(3.24899535499994,12.2,-2.46250349800002));
#352711=CARTESIAN_POINT('Ctrl Pts',(3.24899535499994,5.2,-2.46250349800002));
#352712=CARTESIAN_POINT('Ctrl Pts',(3.24899535499994,2.2,-2.46250349800002));
#352713=CARTESIAN_POINT('Ctrl Pts',(3.24833214799995,12.2,-2.46174833200001));
#352714=CARTESIAN_POINT('Ctrl Pts',(3.24833214799995,5.2,-2.46174833200001));
#352715=CARTESIAN_POINT('Ctrl Pts',(3.24833214799995,2.2,-2.46174833200001));
#352716=CARTESIAN_POINT('Ctrl Pts',(3.24767163199994,12.2,-2.46099809700001));
#352717=CARTESIAN_POINT('Ctrl Pts',(3.24767163199994,5.2,-2.46099809700001));
#352718=CARTESIAN_POINT('Ctrl Pts',(3.24767163199994,2.2,-2.46099809700001));
#352719=CARTESIAN_POINT('Ctrl Pts',(3.24701382399994,12.2,-2.46025279100001));
#352720=CARTESIAN_POINT('Ctrl Pts',(3.24701382399994,5.2,-2.46025279100001));
#352721=CARTESIAN_POINT('Ctrl Pts',(3.24701382399994,2.2,-2.46025279100001));
#352722=CARTESIAN_POINT('Ctrl Pts',(3.24635874099994,12.2,-2.45951241500002));
#352723=CARTESIAN_POINT('Ctrl Pts',(3.24635874099994,5.2,-2.45951241500002));
#352724=CARTESIAN_POINT('Ctrl Pts',(3.24635874099994,2.2,-2.45951241500002));
#352725=CARTESIAN_POINT('Ctrl Pts',(3.24570639899994,12.2,-2.45877696800001));
#352726=CARTESIAN_POINT('Ctrl Pts',(3.24570639899994,5.2,-2.45877696800001));
#352727=CARTESIAN_POINT('Ctrl Pts',(3.24570639899994,2.2,-2.45877696800001));
#352728=CARTESIAN_POINT('Ctrl Pts',(3.24505681599994,12.2,-2.45804644900002));
#352729=CARTESIAN_POINT('Ctrl Pts',(3.24505681599994,5.2,-2.45804644900002));
#352730=CARTESIAN_POINT('Ctrl Pts',(3.24505681599994,2.2,-2.45804644900002));
#352731=CARTESIAN_POINT('Ctrl Pts',(3.24441000699994,12.2,-2.45732085700002));
#352732=CARTESIAN_POINT('Ctrl Pts',(3.24441000699994,5.2,-2.45732085700002));
#352733=CARTESIAN_POINT('Ctrl Pts',(3.24441000699994,2.2,-2.45732085700002));
#352734=CARTESIAN_POINT('Ctrl Pts',(3.24376599099995,12.2,-2.45660019300002));
#352735=CARTESIAN_POINT('Ctrl Pts',(3.24376599099995,5.2,-2.45660019300002));
#352736=CARTESIAN_POINT('Ctrl Pts',(3.24376599099995,2.2,-2.45660019300002));
#352737=CARTESIAN_POINT('Ctrl Pts',(3.24312478299994,12.2,-2.45588445400001));
#352738=CARTESIAN_POINT('Ctrl Pts',(3.24312478299994,5.2,-2.45588445400001));
#352739=CARTESIAN_POINT('Ctrl Pts',(3.24312478299994,2.2,-2.45588445400001));
#352740=CARTESIAN_POINT('Ctrl Pts',(3.24248640099994,12.2,-2.45517364300001));
#352741=CARTESIAN_POINT('Ctrl Pts',(3.24248640099994,5.2,-2.45517364300001));
#352742=CARTESIAN_POINT('Ctrl Pts',(3.24248640099994,2.2,-2.45517364300001));
#352743=CARTESIAN_POINT('Ctrl Pts',(3.24185086299994,12.2,-2.45446775600001));
#352744=CARTESIAN_POINT('Ctrl Pts',(3.24185086299994,5.2,-2.45446775600001));
#352745=CARTESIAN_POINT('Ctrl Pts',(3.24185086299994,2.2,-2.45446775600001));
#352746=CARTESIAN_POINT('Ctrl Pts',(3.24121818399994,12.2,-2.45376679500001));
#352747=CARTESIAN_POINT('Ctrl Pts',(3.24121818399994,5.2,-2.45376679500001));
#352748=CARTESIAN_POINT('Ctrl Pts',(3.24121818399994,2.2,-2.45376679500001));
#352749=CARTESIAN_POINT('Ctrl Pts',(3.24058838199994,12.2,-2.45307075800001));
#352750=CARTESIAN_POINT('Ctrl Pts',(3.24058838199994,5.2,-2.45307075800001));
#352751=CARTESIAN_POINT('Ctrl Pts',(3.24058838199994,2.2,-2.45307075800001));
#352752=CARTESIAN_POINT('Ctrl Pts',(3.23996147399995,12.2,-2.45237964400001));
#352753=CARTESIAN_POINT('Ctrl Pts',(3.23996147399995,5.2,-2.45237964400001));
#352754=CARTESIAN_POINT('Ctrl Pts',(3.23996147399995,2.2,-2.45237964400001));
#352755=CARTESIAN_POINT('Ctrl Pts',(3.23933747799994,12.2,-2.45169345300001));
#352756=CARTESIAN_POINT('Ctrl Pts',(3.23933747799994,5.2,-2.45169345300001));
#352757=CARTESIAN_POINT('Ctrl Pts',(3.23933747799994,2.2,-2.45169345300001));
#352758=CARTESIAN_POINT('Ctrl Pts',(3.23871640999994,12.2,-2.45101218300002));
#352759=CARTESIAN_POINT('Ctrl Pts',(3.23871640999994,5.2,-2.45101218300002));
#352760=CARTESIAN_POINT('Ctrl Pts',(3.23871640999994,2.2,-2.45101218300002));
#352761=CARTESIAN_POINT('Ctrl Pts',(3.23809828799994,12.2,-2.45033583500001));
#352762=CARTESIAN_POINT('Ctrl Pts',(3.23809828799994,5.2,-2.45033583500001));
#352763=CARTESIAN_POINT('Ctrl Pts',(3.23809828799994,2.2,-2.45033583500001));
#352764=CARTESIAN_POINT('Ctrl Pts',(3.23748312899995,12.2,-2.44966440700002));
#352765=CARTESIAN_POINT('Ctrl Pts',(3.23748312899995,5.2,-2.44966440700002));
#352766=CARTESIAN_POINT('Ctrl Pts',(3.23748312899995,2.2,-2.44966440700002));
#352767=CARTESIAN_POINT('Ctrl Pts',(3.23687094999995,12.2,-2.44899789900002));
#352768=CARTESIAN_POINT('Ctrl Pts',(3.23687094999995,5.2,-2.44899789900002));
#352769=CARTESIAN_POINT('Ctrl Pts',(3.23687094999995,2.2,-2.44899789900002));
#352770=CARTESIAN_POINT('Ctrl Pts',(3.23626176999994,12.2,-2.44833630900001));
#352771=CARTESIAN_POINT('Ctrl Pts',(3.23626176999994,5.2,-2.44833630900001));
#352772=CARTESIAN_POINT('Ctrl Pts',(3.23626176999994,2.2,-2.44833630900001));
#352773=CARTESIAN_POINT('Ctrl Pts',(3.23565560499994,12.2,-2.44767963800001));
#352774=CARTESIAN_POINT('Ctrl Pts',(3.23565560499994,5.2,-2.44767963800001));
#352775=CARTESIAN_POINT('Ctrl Pts',(3.23565560499994,2.2,-2.44767963800001));
#352776=CARTESIAN_POINT('Ctrl Pts',(3.23505247299994,12.2,-2.44702788400001));
#352777=CARTESIAN_POINT('Ctrl Pts',(3.23505247299994,5.2,-2.44702788400001));
#352778=CARTESIAN_POINT('Ctrl Pts',(3.23505247299994,2.2,-2.44702788400001));
#352779=CARTESIAN_POINT('Ctrl Pts',(3.23445239099994,12.2,-2.44638104600002));
#352780=CARTESIAN_POINT('Ctrl Pts',(3.23445239099994,5.2,-2.44638104600002));
#352781=CARTESIAN_POINT('Ctrl Pts',(3.23445239099994,2.2,-2.44638104600002));
#352782=CARTESIAN_POINT('Ctrl Pts',(3.23385537699994,12.2,-2.44573912300002));
#352783=CARTESIAN_POINT('Ctrl Pts',(3.23385537699994,5.2,-2.44573912300002));
#352784=CARTESIAN_POINT('Ctrl Pts',(3.23385537699994,2.2,-2.44573912300002));
#352785=CARTESIAN_POINT('Ctrl Pts',(3.23326144799994,12.2,-2.44510211400002));
#352786=CARTESIAN_POINT('Ctrl Pts',(3.23326144799994,5.2,-2.44510211400002));
#352787=CARTESIAN_POINT('Ctrl Pts',(3.23326144799994,2.2,-2.44510211400002));
#352788=CARTESIAN_POINT('Ctrl Pts',(3.23267062299994,12.2,-2.44447001800001));
#352789=CARTESIAN_POINT('Ctrl Pts',(3.23267062299994,5.2,-2.44447001800001));
#352790=CARTESIAN_POINT('Ctrl Pts',(3.23267062299994,2.2,-2.44447001800001));
#352791=CARTESIAN_POINT('Ctrl Pts',(3.23208291799994,12.2,-2.44384283500001));
#352792=CARTESIAN_POINT('Ctrl Pts',(3.23208291799994,5.2,-2.44384283500001));
#352793=CARTESIAN_POINT('Ctrl Pts',(3.23208291799994,2.2,-2.44384283500001));
#352794=CARTESIAN_POINT('Ctrl Pts',(3.23149835299994,12.2,-2.44322056300001));
#352795=CARTESIAN_POINT('Ctrl Pts',(3.23149835299994,5.2,-2.44322056300001));
#352796=CARTESIAN_POINT('Ctrl Pts',(3.23149835299994,2.2,-2.44322056300001));
#352797=CARTESIAN_POINT('Ctrl Pts',(3.23091694299994,12.2,-2.44260320100001));
#352798=CARTESIAN_POINT('Ctrl Pts',(3.23091694299994,5.2,-2.44260320100001));
#352799=CARTESIAN_POINT('Ctrl Pts',(3.23091694299994,2.2,-2.44260320100001));
#352800=CARTESIAN_POINT('Ctrl Pts',(3.23033870899994,12.2,-2.44199074800001));
#352801=CARTESIAN_POINT('Ctrl Pts',(3.23033870899994,5.2,-2.44199074800001));
#352802=CARTESIAN_POINT('Ctrl Pts',(3.23033870899994,2.2,-2.44199074800001));
#352803=CARTESIAN_POINT('Ctrl Pts',(3.22976366699995,12.2,-2.44138320400001));
#352804=CARTESIAN_POINT('Ctrl Pts',(3.22976366699995,5.2,-2.44138320400001));
#352805=CARTESIAN_POINT('Ctrl Pts',(3.22976366699995,2.2,-2.44138320400001));
#352806=CARTESIAN_POINT('Ctrl Pts',(3.22919183499994,12.2,-2.44078056700001));
#352807=CARTESIAN_POINT('Ctrl Pts',(3.22919183499994,5.2,-2.44078056700001));
#352808=CARTESIAN_POINT('Ctrl Pts',(3.22919183499994,2.2,-2.44078056700001));
#352809=CARTESIAN_POINT('Ctrl Pts',(3.22862323099995,12.2,-2.44018283400001));
#352810=CARTESIAN_POINT('Ctrl Pts',(3.22862323099995,5.2,-2.44018283400001));
#352811=CARTESIAN_POINT('Ctrl Pts',(3.22862323099995,2.2,-2.44018283400001));
#352812=CARTESIAN_POINT('Ctrl Pts',(3.22805787299994,12.2,-2.43959000700002));
#352813=CARTESIAN_POINT('Ctrl Pts',(3.22805787299994,5.2,-2.43959000700002));
#352814=CARTESIAN_POINT('Ctrl Pts',(3.22805787299994,2.2,-2.43959000700002));
#352815=CARTESIAN_POINT('Ctrl Pts',(3.22749577999994,12.2,-2.43900208300001));
#352816=CARTESIAN_POINT('Ctrl Pts',(3.22749577999994,5.2,-2.43900208300001));
#352817=CARTESIAN_POINT('Ctrl Pts',(3.22749577999994,2.2,-2.43900208300001));
#352818=CARTESIAN_POINT('Ctrl Pts',(3.22693696999994,12.2,-2.43841906100001));
#352819=CARTESIAN_POINT('Ctrl Pts',(3.22693696999994,5.2,-2.43841906100001));
#352820=CARTESIAN_POINT('Ctrl Pts',(3.22693696999994,2.2,-2.43841906100001));
#352821=CARTESIAN_POINT('Ctrl Pts',(3.22638145999994,12.2,-2.43784093900001));
#352822=CARTESIAN_POINT('Ctrl Pts',(3.22638145999994,5.2,-2.43784093900001));
#352823=CARTESIAN_POINT('Ctrl Pts',(3.22638145999994,2.2,-2.43784093900001));
#352824=CARTESIAN_POINT('Ctrl Pts',(3.22582926899994,12.2,-2.43726771800001));
#352825=CARTESIAN_POINT('Ctrl Pts',(3.22582926899994,5.2,-2.43726771800001));
#352826=CARTESIAN_POINT('Ctrl Pts',(3.22582926899994,2.2,-2.43726771800001));
#352827=CARTESIAN_POINT('Ctrl Pts',(3.22528041499994,12.2,-2.43669939500001));
#352828=CARTESIAN_POINT('Ctrl Pts',(3.22528041499994,5.2,-2.43669939500001));
#352829=CARTESIAN_POINT('Ctrl Pts',(3.22528041499994,2.2,-2.43669939500001));
#352830=CARTESIAN_POINT('Ctrl Pts',(3.22473491699995,12.2,-2.43613596900001));
#352831=CARTESIAN_POINT('Ctrl Pts',(3.22473491699995,5.2,-2.43613596900001));
#352832=CARTESIAN_POINT('Ctrl Pts',(3.22473491699995,2.2,-2.43613596900001));
#352833=CARTESIAN_POINT('Ctrl Pts',(3.22419279299994,12.2,-2.43557743800002));
#352834=CARTESIAN_POINT('Ctrl Pts',(3.22419279299994,5.2,-2.43557743800002));
#352835=CARTESIAN_POINT('Ctrl Pts',(3.22419279299994,2.2,-2.43557743800002));
#352836=CARTESIAN_POINT('Ctrl Pts',(3.22365406099994,12.2,-2.43502380100002));
#352837=CARTESIAN_POINT('Ctrl Pts',(3.22365406099994,5.2,-2.43502380100002));
#352838=CARTESIAN_POINT('Ctrl Pts',(3.22365406099994,2.2,-2.43502380100002));
#352839=CARTESIAN_POINT('Ctrl Pts',(3.22311873999995,12.2,-2.43447505800002));
#352840=CARTESIAN_POINT('Ctrl Pts',(3.22311873999995,5.2,-2.43447505800002));
#352841=CARTESIAN_POINT('Ctrl Pts',(3.22311873999995,2.2,-2.43447505800002));
#352842=CARTESIAN_POINT('Ctrl Pts',(3.22258684899994,12.2,-2.43393120500001));
#352843=CARTESIAN_POINT('Ctrl Pts',(3.22258684899994,5.2,-2.43393120500001));
#352844=CARTESIAN_POINT('Ctrl Pts',(3.22258684899994,2.2,-2.43393120500001));
#352845=CARTESIAN_POINT('Ctrl Pts',(3.22205840599994,12.2,-2.43339224300001));
#352846=CARTESIAN_POINT('Ctrl Pts',(3.22205840599994,5.2,-2.43339224300001));
#352847=CARTESIAN_POINT('Ctrl Pts',(3.22205840599994,2.2,-2.43339224300001));
#352848=CARTESIAN_POINT('Ctrl Pts',(3.22153342899994,12.2,-2.43285816900002));
#352849=CARTESIAN_POINT('Ctrl Pts',(3.22153342899994,5.2,-2.43285816900002));
#352850=CARTESIAN_POINT('Ctrl Pts',(3.22153342899994,2.2,-2.43285816900002));
#352851=CARTESIAN_POINT('Ctrl Pts',(3.22101193699994,12.2,-2.43232898100001));
#352852=CARTESIAN_POINT('Ctrl Pts',(3.22101193699994,5.2,-2.43232898100001));
#352853=CARTESIAN_POINT('Ctrl Pts',(3.22101193699994,2.2,-2.43232898100001));
#352854=CARTESIAN_POINT('Ctrl Pts',(3.22049394999994,12.2,-2.43180467900002));
#352855=CARTESIAN_POINT('Ctrl Pts',(3.22049394999994,5.2,-2.43180467900002));
#352856=CARTESIAN_POINT('Ctrl Pts',(3.22049394999994,2.2,-2.43180467900002));
#352857=CARTESIAN_POINT('Ctrl Pts',(3.21997948499994,12.2,-2.43128526200001));
#352858=CARTESIAN_POINT('Ctrl Pts',(3.21997948499994,5.2,-2.43128526200001));
#352859=CARTESIAN_POINT('Ctrl Pts',(3.21997948499994,2.2,-2.43128526200001));
#352860=CARTESIAN_POINT('Ctrl Pts',(3.21946856199995,12.2,-2.43077072500002));
#352861=CARTESIAN_POINT('Ctrl Pts',(3.21946856199995,5.2,-2.43077072500002));
#352862=CARTESIAN_POINT('Ctrl Pts',(3.21946856199995,2.2,-2.43077072500002));
#352863=CARTESIAN_POINT('Ctrl Pts',(3.21896119999994,12.2,-2.43026107000002));
#352864=CARTESIAN_POINT('Ctrl Pts',(3.21896119999994,5.2,-2.43026107000002));
#352865=CARTESIAN_POINT('Ctrl Pts',(3.21896119999994,2.2,-2.43026107000002));
#352866=CARTESIAN_POINT('Ctrl Pts',(3.21845741799994,12.2,-2.42975629300001));
#352867=CARTESIAN_POINT('Ctrl Pts',(3.21845741799994,5.2,-2.42975629300001));
#352868=CARTESIAN_POINT('Ctrl Pts',(3.21845741799994,2.2,-2.42975629300001));
#352869=CARTESIAN_POINT('Ctrl Pts',(3.21795723299994,12.2,-2.42925639400001));
#352870=CARTESIAN_POINT('Ctrl Pts',(3.21795723299994,5.2,-2.42925639400001));
#352871=CARTESIAN_POINT('Ctrl Pts',(3.21795723299994,2.2,-2.42925639400001));
#352872=CARTESIAN_POINT('Ctrl Pts',(3.21746066699995,12.2,-2.42876137000001));
#352873=CARTESIAN_POINT('Ctrl Pts',(3.21746066699995,5.2,-2.42876137000001));
#352874=CARTESIAN_POINT('Ctrl Pts',(3.21746066699995,2.2,-2.42876137000001));
#352875=CARTESIAN_POINT('Ctrl Pts',(3.21696773699994,12.2,-2.42827122000001));
#352876=CARTESIAN_POINT('Ctrl Pts',(3.21696773699994,5.2,-2.42827122000001));
#352877=CARTESIAN_POINT('Ctrl Pts',(3.21696773699994,2.2,-2.42827122000001));
#352878=CARTESIAN_POINT('Ctrl Pts',(3.21647846299994,12.2,-2.42778594200002));
#352879=CARTESIAN_POINT('Ctrl Pts',(3.21647846299994,5.2,-2.42778594200002));
#352880=CARTESIAN_POINT('Ctrl Pts',(3.21647846299994,2.2,-2.42778594200002));
#352881=CARTESIAN_POINT('Ctrl Pts',(3.21599286399994,12.2,-2.42730553400001));
#352882=CARTESIAN_POINT('Ctrl Pts',(3.21599286399994,5.2,-2.42730553400001));
#352883=CARTESIAN_POINT('Ctrl Pts',(3.21599286399994,2.2,-2.42730553400001));
#352884=CARTESIAN_POINT('Ctrl Pts',(3.21551095899994,12.2,-2.42682999400001));
#352885=CARTESIAN_POINT('Ctrl Pts',(3.21551095899994,5.2,-2.42682999400001));
#352886=CARTESIAN_POINT('Ctrl Pts',(3.21551095899994,2.2,-2.42682999400001));
#352887=CARTESIAN_POINT('Ctrl Pts',(3.21503276799994,12.2,-2.42635932000002));
#352888=CARTESIAN_POINT('Ctrl Pts',(3.21503276799994,5.2,-2.42635932000002));
#352889=CARTESIAN_POINT('Ctrl Pts',(3.21503276799994,2.2,-2.42635932000002));
#352890=CARTESIAN_POINT('Ctrl Pts',(3.21455830899994,12.2,-2.42589351200001));
#352891=CARTESIAN_POINT('Ctrl Pts',(3.21455830899994,5.2,-2.42589351200001));
#352892=CARTESIAN_POINT('Ctrl Pts',(3.21455830899994,2.2,-2.42589351200001));
#352893=CARTESIAN_POINT('Ctrl Pts',(3.21408760299994,12.2,-2.42543256700001));
#352894=CARTESIAN_POINT('Ctrl Pts',(3.21408760299994,5.2,-2.42543256700001));
#352895=CARTESIAN_POINT('Ctrl Pts',(3.21408760299994,2.2,-2.42543256700001));
#352896=CARTESIAN_POINT('Ctrl Pts',(3.21362066899994,12.2,-2.42497648100001));
#352897=CARTESIAN_POINT('Ctrl Pts',(3.21362066899994,5.2,-2.42497648100001));
#352898=CARTESIAN_POINT('Ctrl Pts',(3.21362066899994,2.2,-2.42497648100001));
#352899=CARTESIAN_POINT('Ctrl Pts',(3.21315752599994,12.2,-2.42452525400001));
#352900=CARTESIAN_POINT('Ctrl Pts',(3.21315752599994,5.2,-2.42452525400001));
#352901=CARTESIAN_POINT('Ctrl Pts',(3.21315752599994,2.2,-2.42452525400001));
#352902=CARTESIAN_POINT('Ctrl Pts',(3.21269819499994,12.2,-2.42407888400002));
#352903=CARTESIAN_POINT('Ctrl Pts',(3.21269819499994,5.2,-2.42407888400002));
#352904=CARTESIAN_POINT('Ctrl Pts',(3.21269819499994,2.2,-2.42407888400002));
#352905=CARTESIAN_POINT('Ctrl Pts',(3.21224269299994,12.2,-2.42363736900002));
#352906=CARTESIAN_POINT('Ctrl Pts',(3.21224269299994,5.2,-2.42363736900002));
#352907=CARTESIAN_POINT('Ctrl Pts',(3.21224269299994,2.2,-2.42363736900002));
#352908=CARTESIAN_POINT('Ctrl Pts',(3.21179104199994,12.2,-2.42320070700002));
#352909=CARTESIAN_POINT('Ctrl Pts',(3.21179104199994,5.2,-2.42320070700002));
#352910=CARTESIAN_POINT('Ctrl Pts',(3.21179104199994,2.2,-2.42320070700002));
#352911=CARTESIAN_POINT('Ctrl Pts',(3.21134326099994,12.2,-2.42276889600001));
#352912=CARTESIAN_POINT('Ctrl Pts',(3.21134326099994,5.2,-2.42276889600001));
#352913=CARTESIAN_POINT('Ctrl Pts',(3.21134326099994,2.2,-2.42276889600001));
#352914=CARTESIAN_POINT('Ctrl Pts',(3.21089936999994,12.2,-2.42234193200002));
#352915=CARTESIAN_POINT('Ctrl Pts',(3.21089936999994,5.2,-2.42234193200002));
#352916=CARTESIAN_POINT('Ctrl Pts',(3.21089936999994,2.2,-2.42234193200002));
#352917=CARTESIAN_POINT('Ctrl Pts',(3.21045938799994,12.2,-2.42191981500001));
#352918=CARTESIAN_POINT('Ctrl Pts',(3.21045938799994,5.2,-2.42191981500001));
#352919=CARTESIAN_POINT('Ctrl Pts',(3.21045938799994,2.2,-2.42191981500001));
#352920=CARTESIAN_POINT('Ctrl Pts',(3.21002333599994,12.2,-2.42150254300002));
#352921=CARTESIAN_POINT('Ctrl Pts',(3.21002333599994,5.2,-2.42150254300002));
#352922=CARTESIAN_POINT('Ctrl Pts',(3.21002333599994,2.2,-2.42150254300002));
#352923=CARTESIAN_POINT('Ctrl Pts',(3.20959123499994,12.2,-2.42109011200002));
#352924=CARTESIAN_POINT('Ctrl Pts',(3.20959123499994,5.2,-2.42109011200002));
#352925=CARTESIAN_POINT('Ctrl Pts',(3.20959123499994,2.2,-2.42109011200002));
#352926=CARTESIAN_POINT('Ctrl Pts',(3.20916310199994,12.2,-2.42068252000001));
#352927=CARTESIAN_POINT('Ctrl Pts',(3.20916310199994,5.2,-2.42068252000001));
#352928=CARTESIAN_POINT('Ctrl Pts',(3.20916310199994,2.2,-2.42068252000001));
#352929=CARTESIAN_POINT('Ctrl Pts',(3.20873895899994,12.2,-2.42027976700002));
#352930=CARTESIAN_POINT('Ctrl Pts',(3.20873895899994,5.2,-2.42027976700002));
#352931=CARTESIAN_POINT('Ctrl Pts',(3.20873895899994,2.2,-2.42027976700002));
#352932=CARTESIAN_POINT('Ctrl Pts',(3.20831882599995,12.2,-2.41988184800002));
#352933=CARTESIAN_POINT('Ctrl Pts',(3.20831882599995,5.2,-2.41988184800002));
#352934=CARTESIAN_POINT('Ctrl Pts',(3.20831882599995,2.2,-2.41988184800002));
#352935=CARTESIAN_POINT('Ctrl Pts',(3.20790272299994,12.2,-2.41948876200002));
#352936=CARTESIAN_POINT('Ctrl Pts',(3.20790272299994,5.2,-2.41948876200002));
#352937=CARTESIAN_POINT('Ctrl Pts',(3.20790272299994,2.2,-2.41948876200002));
#352938=CARTESIAN_POINT('Ctrl Pts',(3.20749066999995,12.2,-2.41910050600001));
#352939=CARTESIAN_POINT('Ctrl Pts',(3.20749066999995,5.2,-2.41910050600001));
#352940=CARTESIAN_POINT('Ctrl Pts',(3.20749066999995,2.2,-2.41910050600001));
#352941=CARTESIAN_POINT('Ctrl Pts',(3.20708268799994,12.2,-2.41871707900001));
#352942=CARTESIAN_POINT('Ctrl Pts',(3.20708268799994,5.2,-2.41871707900001));
#352943=CARTESIAN_POINT('Ctrl Pts',(3.20708268799994,2.2,-2.41871707900001));
#352944=CARTESIAN_POINT('Ctrl Pts',(3.20667879699994,12.2,-2.41833847700001));
#352945=CARTESIAN_POINT('Ctrl Pts',(3.20667879699994,5.2,-2.41833847700001));
#352946=CARTESIAN_POINT('Ctrl Pts',(3.20667879699994,2.2,-2.41833847700001));
#352947=CARTESIAN_POINT('Ctrl Pts',(3.20627901799994,12.2,-2.41796469800001));
#352948=CARTESIAN_POINT('Ctrl Pts',(3.20627901799994,5.2,-2.41796469800001));
#352949=CARTESIAN_POINT('Ctrl Pts',(3.20627901799994,2.2,-2.41796469800001));
#352950=CARTESIAN_POINT('Ctrl Pts',(3.20588337099994,12.2,-2.41759574100001));
#352951=CARTESIAN_POINT('Ctrl Pts',(3.20588337099994,5.2,-2.41759574100001));
#352952=CARTESIAN_POINT('Ctrl Pts',(3.20588337099994,2.2,-2.41759574100001));
#352953=CARTESIAN_POINT('Ctrl Pts',(3.20549187599994,12.2,-2.41723160100001));
#352954=CARTESIAN_POINT('Ctrl Pts',(3.20549187599994,5.2,-2.41723160100001));
#352955=CARTESIAN_POINT('Ctrl Pts',(3.20549187599994,2.2,-2.41723160100001));
#352956=CARTESIAN_POINT('Ctrl Pts',(3.20510455399994,12.2,-2.41687227600002));
#352957=CARTESIAN_POINT('Ctrl Pts',(3.20510455399994,5.2,-2.41687227600002));
#352958=CARTESIAN_POINT('Ctrl Pts',(3.20510455399994,2.2,-2.41687227600002));
#352959=CARTESIAN_POINT('Ctrl Pts',(3.20472142599994,12.2,-2.41651776500001));
#352960=CARTESIAN_POINT('Ctrl Pts',(3.20472142599994,5.2,-2.41651776500001));
#352961=CARTESIAN_POINT('Ctrl Pts',(3.20472142599994,2.2,-2.41651776500001));
#352962=CARTESIAN_POINT('Ctrl Pts',(3.20434251199994,12.2,-2.41616806400001));
#352963=CARTESIAN_POINT('Ctrl Pts',(3.20434251199994,5.2,-2.41616806400001));
#352964=CARTESIAN_POINT('Ctrl Pts',(3.20434251199994,2.2,-2.41616806400001));
#352965=CARTESIAN_POINT('Ctrl Pts',(3.20396783399994,12.2,-2.41582317100002));
#352966=CARTESIAN_POINT('Ctrl Pts',(3.20396783399994,5.2,-2.41582317100002));
#352967=CARTESIAN_POINT('Ctrl Pts',(3.20396783399994,2.2,-2.41582317100002));
#352968=CARTESIAN_POINT('Ctrl Pts',(3.20359741299994,12.2,-2.41548308200001));
#352969=CARTESIAN_POINT('Ctrl Pts',(3.20359741299994,5.2,-2.41548308200001));
#352970=CARTESIAN_POINT('Ctrl Pts',(3.20359741299994,2.2,-2.41548308200001));
#352971=CARTESIAN_POINT('Ctrl Pts',(3.20323126799994,12.2,-2.41514779700001));
#352972=CARTESIAN_POINT('Ctrl Pts',(3.20323126799994,5.2,-2.41514779700001));
#352973=CARTESIAN_POINT('Ctrl Pts',(3.20323126799994,2.2,-2.41514779700001));
#352974=CARTESIAN_POINT('Ctrl Pts',(3.20286942299994,12.2,-2.41481731100002));
#352975=CARTESIAN_POINT('Ctrl Pts',(3.20286942299994,5.2,-2.41481731100002));
#352976=CARTESIAN_POINT('Ctrl Pts',(3.20286942299994,2.2,-2.41481731100002));
#352977=CARTESIAN_POINT('Ctrl Pts',(3.20251189499994,12.2,-2.41449162100002));
#352978=CARTESIAN_POINT('Ctrl Pts',(3.20251189499994,5.2,-2.41449162100002));
#352979=CARTESIAN_POINT('Ctrl Pts',(3.20251189499994,2.2,-2.41449162100002));
#352980=CARTESIAN_POINT('Ctrl Pts',(3.20215870799994,12.2,-2.41417072600001));
#352981=CARTESIAN_POINT('Ctrl Pts',(3.20215870799994,5.2,-2.41417072600001));
#352982=CARTESIAN_POINT('Ctrl Pts',(3.20215870799994,2.2,-2.41417072600001));
#352983=CARTESIAN_POINT('Ctrl Pts',(3.20180988299994,12.2,-2.41385462100002));
#352984=CARTESIAN_POINT('Ctrl Pts',(3.20180988299994,5.2,-2.41385462100002));
#352985=CARTESIAN_POINT('Ctrl Pts',(3.20180988299994,2.2,-2.41385462100002));
#352986=CARTESIAN_POINT('Ctrl Pts',(3.20146543999994,12.2,-2.41354330500001));
#352987=CARTESIAN_POINT('Ctrl Pts',(3.20146543999994,5.2,-2.41354330500001));
#352988=CARTESIAN_POINT('Ctrl Pts',(3.20146543999994,2.2,-2.41354330500001));
#352989=CARTESIAN_POINT('Ctrl Pts',(3.20112540199994,12.2,-2.41323677400001));
#352990=CARTESIAN_POINT('Ctrl Pts',(3.20112540199994,5.2,-2.41323677400001));
#352991=CARTESIAN_POINT('Ctrl Pts',(3.20112540199994,2.2,-2.41323677400001));
#352992=CARTESIAN_POINT('Ctrl Pts',(3.20078978999994,12.2,-2.41293502500001));
#352993=CARTESIAN_POINT('Ctrl Pts',(3.20078978999994,5.2,-2.41293502500001));
#352994=CARTESIAN_POINT('Ctrl Pts',(3.20078978999994,2.2,-2.41293502500001));
#352995=CARTESIAN_POINT('Ctrl Pts',(3.20045862399994,12.2,-2.41263805700001));
#352996=CARTESIAN_POINT('Ctrl Pts',(3.20045862399994,5.2,-2.41263805700001));
#352997=CARTESIAN_POINT('Ctrl Pts',(3.20045862399994,2.2,-2.41263805700001));
#352998=CARTESIAN_POINT('Ctrl Pts',(3.20013192599995,12.2,-2.41234586400001));
#352999=CARTESIAN_POINT('Ctrl Pts',(3.20013192599995,5.2,-2.41234586400001));
#353000=CARTESIAN_POINT('Ctrl Pts',(3.20013192599995,2.2,-2.41234586400001));
#353001=CARTESIAN_POINT('Ctrl Pts',(3.19980971799994,12.2,-2.41205844500001));
#353002=CARTESIAN_POINT('Ctrl Pts',(3.19980971799994,5.2,-2.41205844500001));
#353003=CARTESIAN_POINT('Ctrl Pts',(3.19980971799994,2.2,-2.41205844500001));
#353004=CARTESIAN_POINT('Ctrl Pts',(3.19949202199994,12.2,-2.41177579500001));
#353005=CARTESIAN_POINT('Ctrl Pts',(3.19949202199994,5.2,-2.41177579500001));
#353006=CARTESIAN_POINT('Ctrl Pts',(3.19949202199994,2.2,-2.41177579500001));
#353007=CARTESIAN_POINT('Ctrl Pts',(3.19917885999994,12.2,-2.41149791400002));
#353008=CARTESIAN_POINT('Ctrl Pts',(3.19917885999994,5.2,-2.41149791400002));
#353009=CARTESIAN_POINT('Ctrl Pts',(3.19917885999994,2.2,-2.41149791400002));
#353010=CARTESIAN_POINT('Ctrl Pts',(3.19887025199994,12.2,-2.41122479400001));
#353011=CARTESIAN_POINT('Ctrl Pts',(3.19887025199994,5.2,-2.41122479400001));
#353012=CARTESIAN_POINT('Ctrl Pts',(3.19887025199994,2.2,-2.41122479400001));
#353013=CARTESIAN_POINT('Ctrl Pts',(3.19856622099994,12.2,-2.41095643700001));
#353014=CARTESIAN_POINT('Ctrl Pts',(3.19856622099994,5.2,-2.41095643700001));
#353015=CARTESIAN_POINT('Ctrl Pts',(3.19856622099994,2.2,-2.41095643700001));
#353016=CARTESIAN_POINT('Ctrl Pts',(3.19826678899994,12.2,-2.41069283800002));
#353017=CARTESIAN_POINT('Ctrl Pts',(3.19826678899994,5.2,-2.41069283800002));
#353018=CARTESIAN_POINT('Ctrl Pts',(3.19826678899994,2.2,-2.41069283800002));
#353019=CARTESIAN_POINT('Ctrl Pts',(3.19797197799994,12.2,-2.41043399200001));
#353020=CARTESIAN_POINT('Ctrl Pts',(3.19797197799994,5.2,-2.41043399200001));
#353021=CARTESIAN_POINT('Ctrl Pts',(3.19797197799994,2.2,-2.41043399200001));
#353022=CARTESIAN_POINT('Ctrl Pts',(3.19768180899994,12.2,-2.41017989700001));
#353023=CARTESIAN_POINT('Ctrl Pts',(3.19768180899994,5.2,-2.41017989700001));
#353024=CARTESIAN_POINT('Ctrl Pts',(3.19768180899994,2.2,-2.41017989700001));
#353025=CARTESIAN_POINT('Ctrl Pts',(3.19739630699994,12.2,-2.40993055000001));
#353026=CARTESIAN_POINT('Ctrl Pts',(3.19739630699994,5.2,-2.40993055000001));
#353027=CARTESIAN_POINT('Ctrl Pts',(3.19739630699994,2.2,-2.40993055000001));
#353028=CARTESIAN_POINT('Ctrl Pts',(3.19711548999994,12.2,-2.40968594700002));
#353029=CARTESIAN_POINT('Ctrl Pts',(3.19711548999994,5.2,-2.40968594700002));
#353030=CARTESIAN_POINT('Ctrl Pts',(3.19711548999994,2.2,-2.40968594700002));
#353031=CARTESIAN_POINT('Ctrl Pts',(3.19683938199995,12.2,-2.40944608600001));
#353032=CARTESIAN_POINT('Ctrl Pts',(3.19683938199995,5.2,-2.40944608600001));
#353033=CARTESIAN_POINT('Ctrl Pts',(3.19683938199995,2.2,-2.40944608600001));
#353034=CARTESIAN_POINT('Ctrl Pts',(3.19656800699994,12.2,-2.40921096100001));
#353035=CARTESIAN_POINT('Ctrl Pts',(3.19656800699994,5.2,-2.40921096100001));
#353036=CARTESIAN_POINT('Ctrl Pts',(3.19656800699994,2.2,-2.40921096100001));
#353037=CARTESIAN_POINT('Ctrl Pts',(3.19630138499994,12.2,-2.40898056900001));
#353038=CARTESIAN_POINT('Ctrl Pts',(3.19630138499994,5.2,-2.40898056900001));
#353039=CARTESIAN_POINT('Ctrl Pts',(3.19630138499994,2.2,-2.40898056900001));
#353040=CARTESIAN_POINT('Ctrl Pts',(3.19603954099994,12.2,-2.40875490900001));
#353041=CARTESIAN_POINT('Ctrl Pts',(3.19603954099994,5.2,-2.40875490900001));
#353042=CARTESIAN_POINT('Ctrl Pts',(3.19603954099994,2.2,-2.40875490900001));
#353043=CARTESIAN_POINT('Ctrl Pts',(3.19578249499994,12.2,-2.40853397500001));
#353044=CARTESIAN_POINT('Ctrl Pts',(3.19578249499994,5.2,-2.40853397500001));
#353045=CARTESIAN_POINT('Ctrl Pts',(3.19578249499994,2.2,-2.40853397500001));
#353046=CARTESIAN_POINT('Ctrl Pts',(3.19553027099994,12.2,-2.40831776500002));
#353047=CARTESIAN_POINT('Ctrl Pts',(3.19553027099994,5.2,-2.40831776500002));
#353048=CARTESIAN_POINT('Ctrl Pts',(3.19553027099994,2.2,-2.40831776500002));
#353049=CARTESIAN_POINT('Ctrl Pts',(3.19528289099994,12.2,-2.40810627400001));
#353050=CARTESIAN_POINT('Ctrl Pts',(3.19528289099994,5.2,-2.40810627400001));
#353051=CARTESIAN_POINT('Ctrl Pts',(3.19528289099994,2.2,-2.40810627400001));
#353052=CARTESIAN_POINT('Ctrl Pts',(3.19504037699994,12.2,-2.40789949900002));
#353053=CARTESIAN_POINT('Ctrl Pts',(3.19504037699994,5.2,-2.40789949900002));
#353054=CARTESIAN_POINT('Ctrl Pts',(3.19504037699994,2.2,-2.40789949900002));
#353055=CARTESIAN_POINT('Ctrl Pts',(3.19480275399994,12.2,-2.40769743600001));
#353056=CARTESIAN_POINT('Ctrl Pts',(3.19480275399994,5.2,-2.40769743600001));
#353057=CARTESIAN_POINT('Ctrl Pts',(3.19480275399994,2.2,-2.40769743600001));
#353058=CARTESIAN_POINT('Ctrl Pts',(3.19457004399994,12.2,-2.40750008200001));
#353059=CARTESIAN_POINT('Ctrl Pts',(3.19457004399994,5.2,-2.40750008200001));
#353060=CARTESIAN_POINT('Ctrl Pts',(3.19457004399994,2.2,-2.40750008200001));
#353061=CARTESIAN_POINT('Ctrl Pts',(3.19434226799994,12.2,-2.40730743200002));
#353062=CARTESIAN_POINT('Ctrl Pts',(3.19434226799994,5.2,-2.40730743200002));
#353063=CARTESIAN_POINT('Ctrl Pts',(3.19434226799994,2.2,-2.40730743200002));
#353064=CARTESIAN_POINT('Ctrl Pts',(3.19411945299994,12.2,-2.40711948300001));
#353065=CARTESIAN_POINT('Ctrl Pts',(3.19411945299994,5.2,-2.40711948300001));
#353066=CARTESIAN_POINT('Ctrl Pts',(3.19411945299994,2.2,-2.40711948300001));
#353067=CARTESIAN_POINT('Ctrl Pts',(3.19390161799994,12.2,-2.40693623100002));
#353068=CARTESIAN_POINT('Ctrl Pts',(3.19390161799994,5.2,-2.40693623100002));
#353069=CARTESIAN_POINT('Ctrl Pts',(3.19390161799994,2.2,-2.40693623100002));
#353070=CARTESIAN_POINT('Ctrl Pts',(3.19368878899994,12.2,-2.40675767200001));
#353071=CARTESIAN_POINT('Ctrl Pts',(3.19368878899994,5.2,-2.40675767200001));
#353072=CARTESIAN_POINT('Ctrl Pts',(3.19368878899994,2.2,-2.40675767200001));
#353073=CARTESIAN_POINT('Ctrl Pts',(3.19348098699994,12.2,-2.40658380300002));
#353074=CARTESIAN_POINT('Ctrl Pts',(3.19348098699994,5.2,-2.40658380300002));
#353075=CARTESIAN_POINT('Ctrl Pts',(3.19348098699994,2.2,-2.40658380300002));
#353076=CARTESIAN_POINT('Ctrl Pts',(3.19327823699994,12.2,-2.40641461800001));
#353077=CARTESIAN_POINT('Ctrl Pts',(3.19327823699994,5.2,-2.40641461800001));
#353078=CARTESIAN_POINT('Ctrl Pts',(3.19327823699994,2.2,-2.40641461800001));
#353079=CARTESIAN_POINT('Ctrl Pts',(3.19308056199994,12.2,-2.40625011400001));
#353080=CARTESIAN_POINT('Ctrl Pts',(3.19308056199994,5.2,-2.40625011400001));
#353081=CARTESIAN_POINT('Ctrl Pts',(3.19308056199994,2.2,-2.40625011400001));
#353082=CARTESIAN_POINT('Ctrl Pts',(3.19288798699994,12.2,-2.40609028800002));
#353083=CARTESIAN_POINT('Ctrl Pts',(3.19288798699994,5.2,-2.40609028800002));
#353084=CARTESIAN_POINT('Ctrl Pts',(3.19288798699994,2.2,-2.40609028800002));
#353085=CARTESIAN_POINT('Ctrl Pts',(3.19270053199994,12.2,-2.40593513400002));
#353086=CARTESIAN_POINT('Ctrl Pts',(3.19270053199994,5.2,-2.40593513400002));
#353087=CARTESIAN_POINT('Ctrl Pts',(3.19270053199994,2.2,-2.40593513400002));
#353088=CARTESIAN_POINT('Ctrl Pts',(3.19251822399994,12.2,-2.40578464900001));
#353089=CARTESIAN_POINT('Ctrl Pts',(3.19251822399994,5.2,-2.40578464900001));
#353090=CARTESIAN_POINT('Ctrl Pts',(3.19251822399994,2.2,-2.40578464900001));
#353091=CARTESIAN_POINT('Ctrl Pts',(3.19234108499994,12.2,-2.40563882900001));
#353092=CARTESIAN_POINT('Ctrl Pts',(3.19234108499994,5.2,-2.40563882900001));
#353093=CARTESIAN_POINT('Ctrl Pts',(3.19234108499994,2.2,-2.40563882900001));
#353094=CARTESIAN_POINT('Ctrl Pts',(3.19216913799994,12.2,-2.40549766900001));
#353095=CARTESIAN_POINT('Ctrl Pts',(3.19216913799994,5.2,-2.40549766900001));
#353096=CARTESIAN_POINT('Ctrl Pts',(3.19216913799994,2.2,-2.40549766900001));
#353097=CARTESIAN_POINT('Ctrl Pts',(3.19200240899994,12.2,-2.40536116600001));
#353098=CARTESIAN_POINT('Ctrl Pts',(3.19200240899994,5.2,-2.40536116600001));
#353099=CARTESIAN_POINT('Ctrl Pts',(3.19200240899994,2.2,-2.40536116600001));
#353100=CARTESIAN_POINT('Ctrl Pts',(3.19184092099994,12.2,-2.40522931500001));
#353101=CARTESIAN_POINT('Ctrl Pts',(3.19184092099994,5.2,-2.40522931500001));
#353102=CARTESIAN_POINT('Ctrl Pts',(3.19184092099994,2.2,-2.40522931500001));
#353103=CARTESIAN_POINT('Ctrl Pts',(3.19168469799994,12.2,-2.40510211000001));
#353104=CARTESIAN_POINT('Ctrl Pts',(3.19168469799994,5.2,-2.40510211000001));
#353105=CARTESIAN_POINT('Ctrl Pts',(3.19168469799994,2.2,-2.40510211000001));
#353106=CARTESIAN_POINT('Ctrl Pts',(3.19153376499994,12.2,-2.40497954800002));
#353107=CARTESIAN_POINT('Ctrl Pts',(3.19153376499994,5.2,-2.40497954800002));
#353108=CARTESIAN_POINT('Ctrl Pts',(3.19153376499994,2.2,-2.40497954800002));
#353109=CARTESIAN_POINT('Ctrl Pts',(3.19138814499994,12.2,-2.40486162600002));
#353110=CARTESIAN_POINT('Ctrl Pts',(3.19138814499994,5.2,-2.40486162600002));
#353111=CARTESIAN_POINT('Ctrl Pts',(3.19138814499994,2.2,-2.40486162600002));
#353112=CARTESIAN_POINT('Ctrl Pts',(3.19124786299994,12.2,-2.40474833800001));
#353113=CARTESIAN_POINT('Ctrl Pts',(3.19124786299994,5.2,-2.40474833800001));
#353114=CARTESIAN_POINT('Ctrl Pts',(3.19124786299994,2.2,-2.40474833800001));
#353115=CARTESIAN_POINT('Ctrl Pts',(3.19111294299995,12.2,-2.40463967800002));
#353116=CARTESIAN_POINT('Ctrl Pts',(3.19111294299995,5.2,-2.40463967800002));
#353117=CARTESIAN_POINT('Ctrl Pts',(3.19111294299995,2.2,-2.40463967800002));
#353118=CARTESIAN_POINT('Ctrl Pts',(3.19098340799994,12.2,-2.40453564500001));
#353119=CARTESIAN_POINT('Ctrl Pts',(3.19098340799994,5.2,-2.40453564500001));
#353120=CARTESIAN_POINT('Ctrl Pts',(3.19098340799994,2.2,-2.40453564500001));
#353121=CARTESIAN_POINT('Ctrl Pts',(3.19085928299994,12.2,-2.40443623200001));
#353122=CARTESIAN_POINT('Ctrl Pts',(3.19085928299994,5.2,-2.40443623200001));
#353123=CARTESIAN_POINT('Ctrl Pts',(3.19085928299994,2.2,-2.40443623200001));
#353124=CARTESIAN_POINT('Ctrl Pts',(3.19074059299994,12.2,-2.40434143500002));
#353125=CARTESIAN_POINT('Ctrl Pts',(3.19074059299994,5.2,-2.40434143500002));
#353126=CARTESIAN_POINT('Ctrl Pts',(3.19074059299994,2.2,-2.40434143500002));
#353127=CARTESIAN_POINT('Ctrl Pts',(3.19062736399994,12.2,-2.40425124900002));
#353128=CARTESIAN_POINT('Ctrl Pts',(3.19062736399994,5.2,-2.40425124900002));
#353129=CARTESIAN_POINT('Ctrl Pts',(3.19062736399994,2.2,-2.40425124900002));
#353130=CARTESIAN_POINT('Ctrl Pts',(3.19051962099994,12.2,-2.40416566900001));
#353131=CARTESIAN_POINT('Ctrl Pts',(3.19051962099994,5.2,-2.40416566900001));
#353132=CARTESIAN_POINT('Ctrl Pts',(3.19051962099994,2.2,-2.40416566900001));
#353133=CARTESIAN_POINT('Ctrl Pts',(3.19041739199994,12.2,-2.40408469100001));
#353134=CARTESIAN_POINT('Ctrl Pts',(3.19041739199994,5.2,-2.40408469100001));
#353135=CARTESIAN_POINT('Ctrl Pts',(3.19041739199994,2.2,-2.40408469100001));
#353136=CARTESIAN_POINT('Ctrl Pts',(3.19032069899994,12.2,-2.40400830800001));
#353137=CARTESIAN_POINT('Ctrl Pts',(3.19032069899994,5.2,-2.40400830800001));
#353138=CARTESIAN_POINT('Ctrl Pts',(3.19032069899994,2.2,-2.40400830800001));
#353139=CARTESIAN_POINT('Ctrl Pts',(3.19022956499994,12.2,-2.40393651800002));
#353140=CARTESIAN_POINT('Ctrl Pts',(3.19022956499994,5.2,-2.40393651800002));
#353141=CARTESIAN_POINT('Ctrl Pts',(3.19022956499994,2.2,-2.40393651800002));
#353142=CARTESIAN_POINT('Ctrl Pts',(3.19014401299994,12.2,-2.40386931500002));
#353143=CARTESIAN_POINT('Ctrl Pts',(3.19014401299994,5.2,-2.40386931500002));
#353144=CARTESIAN_POINT('Ctrl Pts',(3.19014401299994,2.2,-2.40386931500002));
#353145=CARTESIAN_POINT('Ctrl Pts',(3.19006406599994,12.2,-2.40380669500002));
#353146=CARTESIAN_POINT('Ctrl Pts',(3.19006406599994,5.2,-2.40380669500002));
#353147=CARTESIAN_POINT('Ctrl Pts',(3.19006406599994,2.2,-2.40380669500002));
#353148=CARTESIAN_POINT('Ctrl Pts',(3.18998974899994,12.2,-2.40374865400002));
#353149=CARTESIAN_POINT('Ctrl Pts',(3.18998974899994,5.2,-2.40374865400002));
#353150=CARTESIAN_POINT('Ctrl Pts',(3.18998974899994,2.2,-2.40374865400002));
#353151=CARTESIAN_POINT('Ctrl Pts',(3.18992109099994,12.2,-2.40369518600001));
#353152=CARTESIAN_POINT('Ctrl Pts',(3.18992109099994,5.2,-2.40369518600001));
#353153=CARTESIAN_POINT('Ctrl Pts',(3.18992109099994,2.2,-2.40369518600001));
#353154=CARTESIAN_POINT('Ctrl Pts',(3.18985812499994,12.2,-2.40364628200001));
#353155=CARTESIAN_POINT('Ctrl Pts',(3.18985812499994,5.2,-2.40364628200001));
#353156=CARTESIAN_POINT('Ctrl Pts',(3.18985812499994,2.2,-2.40364628200001));
#353157=CARTESIAN_POINT('Ctrl Pts',(3.18980088399994,12.2,-2.40360193900001));
#353158=CARTESIAN_POINT('Ctrl Pts',(3.18980088399994,5.2,-2.40360193900001));
#353159=CARTESIAN_POINT('Ctrl Pts',(3.18980088399994,2.2,-2.40360193900001));
#353160=CARTESIAN_POINT('Ctrl Pts',(3.18974939399994,12.2,-2.40356214900002));
#353161=CARTESIAN_POINT('Ctrl Pts',(3.18974939399994,5.2,-2.40356214900002));
#353162=CARTESIAN_POINT('Ctrl Pts',(3.18974939399994,2.2,-2.40356214900002));
#353163=CARTESIAN_POINT('Ctrl Pts',(3.18970367699994,12.2,-2.40352690800002));
#353164=CARTESIAN_POINT('Ctrl Pts',(3.18970367699994,5.2,-2.40352690800002));
#353165=CARTESIAN_POINT('Ctrl Pts',(3.18970367699994,2.2,-2.40352690800002));
#353166=CARTESIAN_POINT('Ctrl Pts',(3.18965947128237,12.2,-2.40349292812735));
#353167=CARTESIAN_POINT('Ctrl Pts',(3.18965947128237,5.2,-2.40349292812735));
#353168=CARTESIAN_POINT('Ctrl Pts',(3.18965947128237,2.2,-2.40349292812735));
#353169=CARTESIAN_POINT('Ctrl Pts',(3.18962920612091,12.2,-2.40346976281444));
#353170=CARTESIAN_POINT('Ctrl Pts',(3.18962920612091,5.2,-2.40346976281444));
#353171=CARTESIAN_POINT('Ctrl Pts',(3.18962920612091,2.2,-2.40346976281444));
#353172=CARTESIAN_POINT('Ctrl Pts',(3.18960923616151,12.2,-2.40345454411699));
#353173=CARTESIAN_POINT('Ctrl Pts',(3.18960923616151,5.2,-2.40345454411699));
#353174=CARTESIAN_POINT('Ctrl Pts',(3.18960923616151,2.2,-2.40345454411699));
#353175=CARTESIAN_POINT('Ctrl Pts',(3.18959677471721,12.2,-2.40344508870311));
#353176=CARTESIAN_POINT('Ctrl Pts',(3.18959677471721,5.2,-2.40344508870311));
#353177=CARTESIAN_POINT('Ctrl Pts',(3.18959677471721,2.2,-2.40344508870311));
#353178=CARTESIAN_POINT('Ctrl Pts',(3.18958908299994,12.2,-2.40343925200001));
#353179=CARTESIAN_POINT('Ctrl Pts',(3.18958908299994,5.2,-2.40343925200001));
#353180=CARTESIAN_POINT('Ctrl Pts',(3.18958908299994,2.2,-2.40343925200001));
#353181=CARTESIAN_POINT('',(3.57864508499994,12.2,-3.12342750100001));
#353182=CARTESIAN_POINT('Origin',(-5.66300478732629E-14,15.2,-1.77635683940025E-14));
#353183=CARTESIAN_POINT('',(3.34820124399994,12.2,-3.36928010500001));
#353184=CARTESIAN_POINT('Ctrl Pts',(2.60456075099994,12.2,-3.02756096900001));
#353185=CARTESIAN_POINT('Ctrl Pts',(2.60456075099994,5.2,-3.02756096900001));
#353186=CARTESIAN_POINT('Ctrl Pts',(2.60456075099994,2.2,-3.02756096900001));
#353187=CARTESIAN_POINT('Ctrl Pts',(2.60456523372611,12.2,-3.02756613868415));
#353188=CARTESIAN_POINT('Ctrl Pts',(2.60456523372611,5.2,-3.02756613868415));
#353189=CARTESIAN_POINT('Ctrl Pts',(2.60456523372611,2.2,-3.02756613868415));
#353190=CARTESIAN_POINT('Ctrl Pts',(2.60457390279746,12.2,-3.02757613848311));
#353191=CARTESIAN_POINT('Ctrl Pts',(2.60457390279746,5.2,-3.02757613848311));
#353192=CARTESIAN_POINT('Ctrl Pts',(2.60457390279746,2.2,-3.02757613848311));
#353193=CARTESIAN_POINT('Ctrl Pts',(2.60458675887381,12.2,-3.02759096800462));
#353194=CARTESIAN_POINT('Ctrl Pts',(2.60458675887381,5.2,-3.02759096800462));
#353195=CARTESIAN_POINT('Ctrl Pts',(2.60458675887381,2.2,-3.02759096800462));
#353196=CARTESIAN_POINT('Ctrl Pts',(2.60460382305029,12.2,-3.0276106272463));
#353197=CARTESIAN_POINT('Ctrl Pts',(2.60460382305029,5.19999999999999,-3.0276106272463));
#353198=CARTESIAN_POINT('Ctrl Pts',(2.60460382305029,2.2,-3.0276106272463));
#353199=CARTESIAN_POINT('Ctrl Pts',(2.60463362599994,12.2,-3.02764471800002));
#353200=CARTESIAN_POINT('Ctrl Pts',(2.60463362599994,5.2,-3.02764471800002));
#353201=CARTESIAN_POINT('Ctrl Pts',(2.60463362599994,2.2,-3.02764471800002));
#353202=CARTESIAN_POINT('Ctrl Pts',(2.60466683599994,12.2,-3.02768258200001));
#353203=CARTESIAN_POINT('Ctrl Pts',(2.60466683599994,5.2,-3.02768258200001));
#353204=CARTESIAN_POINT('Ctrl Pts',(2.60466683599994,2.2,-3.02768258200001));
#353205=CARTESIAN_POINT('Ctrl Pts',(2.60470495699994,12.2,-3.02772592500002));
#353206=CARTESIAN_POINT('Ctrl Pts',(2.60470495699994,5.2,-3.02772592500002));
#353207=CARTESIAN_POINT('Ctrl Pts',(2.60470495699994,2.2,-3.02772592500002));
#353208=CARTESIAN_POINT('Ctrl Pts',(2.60474799299995,12.2,-3.02777473600001));
#353209=CARTESIAN_POINT('Ctrl Pts',(2.60474799299995,5.2,-3.02777473600001));
#353210=CARTESIAN_POINT('Ctrl Pts',(2.60474799299995,2.2,-3.02777473600001));
#353211=CARTESIAN_POINT('Ctrl Pts',(2.60479594299994,12.2,-3.02782899200002));
#353212=CARTESIAN_POINT('Ctrl Pts',(2.60479594299994,5.2,-3.02782899200002));
#353213=CARTESIAN_POINT('Ctrl Pts',(2.60479594299994,2.2,-3.02782899200002));
#353214=CARTESIAN_POINT('Ctrl Pts',(2.60484881399994,12.2,-3.02788866500002));
#353215=CARTESIAN_POINT('Ctrl Pts',(2.60484881399994,5.2,-3.02788866500002));
#353216=CARTESIAN_POINT('Ctrl Pts',(2.60484881399994,2.2,-3.02788866500002));
#353217=CARTESIAN_POINT('Ctrl Pts',(2.60490660899994,12.2,-3.02795372300002));
#353218=CARTESIAN_POINT('Ctrl Pts',(2.60490660899994,5.2,-3.02795372300002));
#353219=CARTESIAN_POINT('Ctrl Pts',(2.60490660899994,2.2,-3.02795372300002));
#353220=CARTESIAN_POINT('Ctrl Pts',(2.60496933299994,12.2,-3.02802413400002));
#353221=CARTESIAN_POINT('Ctrl Pts',(2.60496933299994,5.2,-3.02802413400002));
#353222=CARTESIAN_POINT('Ctrl Pts',(2.60496933299994,2.2,-3.02802413400002));
#353223=CARTESIAN_POINT('Ctrl Pts',(2.60503698899994,12.2,-3.02809986600002));
#353224=CARTESIAN_POINT('Ctrl Pts',(2.60503698899994,5.2,-3.02809986600002));
#353225=CARTESIAN_POINT('Ctrl Pts',(2.60503698899994,2.2,-3.02809986600002));
#353226=CARTESIAN_POINT('Ctrl Pts',(2.60510957999994,12.2,-3.02818089600001));
#353227=CARTESIAN_POINT('Ctrl Pts',(2.60510957999994,5.2,-3.02818089600001));
#353228=CARTESIAN_POINT('Ctrl Pts',(2.60510957999994,2.2,-3.02818089600001));
#353229=CARTESIAN_POINT('Ctrl Pts',(2.60518711099994,12.2,-3.02826719900001));
#353230=CARTESIAN_POINT('Ctrl Pts',(2.60518711099994,5.2,-3.02826719900001));
#353231=CARTESIAN_POINT('Ctrl Pts',(2.60518711099994,2.2,-3.02826719900001));
#353232=CARTESIAN_POINT('Ctrl Pts',(2.60526958299995,12.2,-3.02835875300001));
#353233=CARTESIAN_POINT('Ctrl Pts',(2.60526958299995,5.2,-3.02835875300001));
#353234=CARTESIAN_POINT('Ctrl Pts',(2.60526958299995,2.2,-3.02835875300001));
#353235=CARTESIAN_POINT('Ctrl Pts',(2.60535699999994,12.2,-3.02845553400001));
#353236=CARTESIAN_POINT('Ctrl Pts',(2.60535699999994,5.2,-3.02845553400001));
#353237=CARTESIAN_POINT('Ctrl Pts',(2.60535699999994,2.2,-3.02845553400001));
#353238=CARTESIAN_POINT('Ctrl Pts',(2.60544936499994,12.2,-3.02855752000001));
#353239=CARTESIAN_POINT('Ctrl Pts',(2.60544936499994,5.2,-3.02855752000001));
#353240=CARTESIAN_POINT('Ctrl Pts',(2.60544936499994,2.2,-3.02855752000001));
#353241=CARTESIAN_POINT('Ctrl Pts',(2.60554668099994,12.2,-3.02866468300001));
#353242=CARTESIAN_POINT('Ctrl Pts',(2.60554668099994,5.2,-3.02866468300001));
#353243=CARTESIAN_POINT('Ctrl Pts',(2.60554668099994,2.2,-3.02866468300001));
#353244=CARTESIAN_POINT('Ctrl Pts',(2.60564895099994,12.2,-3.02877699800002));
#353245=CARTESIAN_POINT('Ctrl Pts',(2.60564895099994,5.2,-3.02877699800002));
#353246=CARTESIAN_POINT('Ctrl Pts',(2.60564895099994,2.2,-3.02877699800002));
#353247=CARTESIAN_POINT('Ctrl Pts',(2.60575617899995,12.2,-3.02889443700002));
#353248=CARTESIAN_POINT('Ctrl Pts',(2.60575617899995,5.2,-3.02889443700002));
#353249=CARTESIAN_POINT('Ctrl Pts',(2.60575617899995,2.2,-3.02889443700002));
#353250=CARTESIAN_POINT('Ctrl Pts',(2.60586836799995,12.2,-3.02901697700001));
#353251=CARTESIAN_POINT('Ctrl Pts',(2.60586836799995,5.2,-3.02901697700001));
#353252=CARTESIAN_POINT('Ctrl Pts',(2.60586836799995,2.2,-3.02901697700001));
#353253=CARTESIAN_POINT('Ctrl Pts',(2.60598551899994,12.2,-3.02914459200001));
#353254=CARTESIAN_POINT('Ctrl Pts',(2.60598551899994,5.2,-3.02914459200001));
#353255=CARTESIAN_POINT('Ctrl Pts',(2.60598551899994,2.2,-3.02914459200001));
#353256=CARTESIAN_POINT('Ctrl Pts',(2.60610763899995,12.2,-3.02927725900001));
#353257=CARTESIAN_POINT('Ctrl Pts',(2.60610763899995,5.2,-3.02927725900001));
#353258=CARTESIAN_POINT('Ctrl Pts',(2.60610763899995,2.2,-3.02927725900001));
#353259=CARTESIAN_POINT('Ctrl Pts',(2.60623472699994,12.2,-3.02941495200002));
#353260=CARTESIAN_POINT('Ctrl Pts',(2.60623472699994,5.2,-3.02941495200002));
#353261=CARTESIAN_POINT('Ctrl Pts',(2.60623472699994,2.2,-3.02941495200002));
#353262=CARTESIAN_POINT('Ctrl Pts',(2.60636678699994,12.2,-3.02955764800001));
#353263=CARTESIAN_POINT('Ctrl Pts',(2.60636678699994,5.2,-3.02955764800001));
#353264=CARTESIAN_POINT('Ctrl Pts',(2.60636678699994,2.2,-3.02955764800001));
#353265=CARTESIAN_POINT('Ctrl Pts',(2.60650382299994,12.2,-3.02970532200002));
#353266=CARTESIAN_POINT('Ctrl Pts',(2.60650382299994,5.2,-3.02970532200002));
#353267=CARTESIAN_POINT('Ctrl Pts',(2.60650382299994,2.2,-3.02970532200002));
#353268=CARTESIAN_POINT('Ctrl Pts',(2.60664583599994,12.2,-3.02985795000001));
#353269=CARTESIAN_POINT('Ctrl Pts',(2.60664583599994,5.2,-3.02985795000001));
#353270=CARTESIAN_POINT('Ctrl Pts',(2.60664583599994,2.2,-3.02985795000001));
#353271=CARTESIAN_POINT('Ctrl Pts',(2.60679283099994,12.2,-3.03001550900001));
#353272=CARTESIAN_POINT('Ctrl Pts',(2.60679283099994,5.2,-3.03001550900001));
#353273=CARTESIAN_POINT('Ctrl Pts',(2.60679283099994,2.2,-3.03001550900001));
#353274=CARTESIAN_POINT('Ctrl Pts',(2.60694480999994,12.2,-3.03017797100001));
#353275=CARTESIAN_POINT('Ctrl Pts',(2.60694480999994,5.2,-3.03017797100001));
#353276=CARTESIAN_POINT('Ctrl Pts',(2.60694480999994,2.2,-3.03017797100001));
#353277=CARTESIAN_POINT('Ctrl Pts',(2.60710177399994,12.2,-3.03034531500002));
#353278=CARTESIAN_POINT('Ctrl Pts',(2.60710177399994,5.2,-3.03034531500002));
#353279=CARTESIAN_POINT('Ctrl Pts',(2.60710177399994,2.2,-3.03034531500002));
#353280=CARTESIAN_POINT('Ctrl Pts',(2.60726372699994,12.2,-3.03051751600002));
#353281=CARTESIAN_POINT('Ctrl Pts',(2.60726372699994,5.2,-3.03051751600002));
#353282=CARTESIAN_POINT('Ctrl Pts',(2.60726372699994,2.2,-3.03051751600002));
#353283=CARTESIAN_POINT('Ctrl Pts',(2.60743067299994,12.2,-3.03069454900001));
#353284=CARTESIAN_POINT('Ctrl Pts',(2.60743067299994,5.2,-3.03069454900001));
#353285=CARTESIAN_POINT('Ctrl Pts',(2.60743067299994,2.2,-3.03069454900001));
#353286=CARTESIAN_POINT('Ctrl Pts',(2.60760261299994,12.2,-3.03087639200001));
#353287=CARTESIAN_POINT('Ctrl Pts',(2.60760261299994,5.2,-3.03087639200001));
#353288=CARTESIAN_POINT('Ctrl Pts',(2.60760261299994,2.2,-3.03087639200001));
#353289=CARTESIAN_POINT('Ctrl Pts',(2.60777954899994,12.2,-3.03106302100002));
#353290=CARTESIAN_POINT('Ctrl Pts',(2.60777954899994,5.2,-3.03106302100002));
#353291=CARTESIAN_POINT('Ctrl Pts',(2.60777954899994,2.2,-3.03106302100002));
#353292=CARTESIAN_POINT('Ctrl Pts',(2.60796148499994,12.2,-3.03125441200002));
#353293=CARTESIAN_POINT('Ctrl Pts',(2.60796148499994,5.2,-3.03125441200002));
#353294=CARTESIAN_POINT('Ctrl Pts',(2.60796148499994,2.2,-3.03125441200002));
#353295=CARTESIAN_POINT('Ctrl Pts',(2.60814842099995,12.2,-3.03145054100002));
#353296=CARTESIAN_POINT('Ctrl Pts',(2.60814842099995,5.2,-3.03145054100002));
#353297=CARTESIAN_POINT('Ctrl Pts',(2.60814842099995,2.2,-3.03145054100002));
#353298=CARTESIAN_POINT('Ctrl Pts',(2.60834036299994,12.2,-3.03165138400002));
#353299=CARTESIAN_POINT('Ctrl Pts',(2.60834036299994,5.2,-3.03165138400002));
#353300=CARTESIAN_POINT('Ctrl Pts',(2.60834036299994,2.2,-3.03165138400002));
#353301=CARTESIAN_POINT('Ctrl Pts',(2.60853731199994,12.2,-3.03185691800001));
#353302=CARTESIAN_POINT('Ctrl Pts',(2.60853731199994,5.2,-3.03185691800001));
#353303=CARTESIAN_POINT('Ctrl Pts',(2.60853731199994,2.2,-3.03185691800001));
#353304=CARTESIAN_POINT('Ctrl Pts',(2.60873926899994,12.2,-3.03206712000001));
#353305=CARTESIAN_POINT('Ctrl Pts',(2.60873926899994,5.2,-3.03206712000001));
#353306=CARTESIAN_POINT('Ctrl Pts',(2.60873926899994,2.2,-3.03206712000001));
#353307=CARTESIAN_POINT('Ctrl Pts',(2.60894623799994,12.2,-3.03228196800001));
#353308=CARTESIAN_POINT('Ctrl Pts',(2.60894623799994,5.2,-3.03228196800001));
#353309=CARTESIAN_POINT('Ctrl Pts',(2.60894623799994,2.2,-3.03228196800001));
#353310=CARTESIAN_POINT('Ctrl Pts',(2.60915822099994,12.2,-3.03250143600001));
#353311=CARTESIAN_POINT('Ctrl Pts',(2.60915822099994,5.2,-3.03250143600001));
#353312=CARTESIAN_POINT('Ctrl Pts',(2.60915822099994,2.2,-3.03250143600001));
#353313=CARTESIAN_POINT('Ctrl Pts',(2.60937522099994,12.2,-3.03272550100001));
#353314=CARTESIAN_POINT('Ctrl Pts',(2.60937522099994,5.2,-3.03272550100001));
#353315=CARTESIAN_POINT('Ctrl Pts',(2.60937522099994,2.2,-3.03272550100001));
#353316=CARTESIAN_POINT('Ctrl Pts',(2.60959723799994,12.2,-3.03295414300001));
#353317=CARTESIAN_POINT('Ctrl Pts',(2.60959723799994,5.2,-3.03295414300001));
#353318=CARTESIAN_POINT('Ctrl Pts',(2.60959723799994,2.2,-3.03295414300001));
#353319=CARTESIAN_POINT('Ctrl Pts',(2.60982427499994,12.2,-3.03318733600001));
#353320=CARTESIAN_POINT('Ctrl Pts',(2.60982427499994,5.2,-3.03318733600001));
#353321=CARTESIAN_POINT('Ctrl Pts',(2.60982427499994,2.2,-3.03318733600001));
#353322=CARTESIAN_POINT('Ctrl Pts',(2.61005633599994,12.2,-3.03342505900002));
#353323=CARTESIAN_POINT('Ctrl Pts',(2.61005633599994,5.2,-3.03342505900002));
#353324=CARTESIAN_POINT('Ctrl Pts',(2.61005633599994,2.2,-3.03342505900002));
#353325=CARTESIAN_POINT('Ctrl Pts',(2.61029342199994,12.2,-3.03366728700002));
#353326=CARTESIAN_POINT('Ctrl Pts',(2.61029342199994,5.2,-3.03366728700002));
#353327=CARTESIAN_POINT('Ctrl Pts',(2.61029342199994,2.2,-3.03366728700002));
#353328=CARTESIAN_POINT('Ctrl Pts',(2.61053553499994,12.2,-3.03391399900002));
#353329=CARTESIAN_POINT('Ctrl Pts',(2.61053553499994,5.2,-3.03391399900002));
#353330=CARTESIAN_POINT('Ctrl Pts',(2.61053553499994,2.2,-3.03391399900002));
#353331=CARTESIAN_POINT('Ctrl Pts',(2.61078267799994,12.2,-3.03416517100001));
#353332=CARTESIAN_POINT('Ctrl Pts',(2.61078267799994,5.2,-3.03416517100001));
#353333=CARTESIAN_POINT('Ctrl Pts',(2.61078267799994,2.2,-3.03416517100001));
#353334=CARTESIAN_POINT('Ctrl Pts',(2.61103485099994,12.2,-3.03442078200002));
#353335=CARTESIAN_POINT('Ctrl Pts',(2.61103485099994,5.2,-3.03442078200002));
#353336=CARTESIAN_POINT('Ctrl Pts',(2.61103485099994,2.2,-3.03442078200002));
#353337=CARTESIAN_POINT('Ctrl Pts',(2.61129205699994,12.2,-3.03468080800001));
#353338=CARTESIAN_POINT('Ctrl Pts',(2.61129205699994,5.2,-3.03468080800001));
#353339=CARTESIAN_POINT('Ctrl Pts',(2.61129205699994,2.2,-3.03468080800001));
#353340=CARTESIAN_POINT('Ctrl Pts',(2.61155429899994,12.2,-3.03494522800001));
#353341=CARTESIAN_POINT('Ctrl Pts',(2.61155429899994,5.2,-3.03494522800001));
#353342=CARTESIAN_POINT('Ctrl Pts',(2.61155429899994,2.2,-3.03494522800001));
#353343=CARTESIAN_POINT('Ctrl Pts',(2.61182157899994,12.2,-3.03521401800001));
#353344=CARTESIAN_POINT('Ctrl Pts',(2.61182157899994,5.2,-3.03521401800001));
#353345=CARTESIAN_POINT('Ctrl Pts',(2.61182157899994,2.2,-3.03521401800001));
#353346=CARTESIAN_POINT('Ctrl Pts',(2.61209389699995,12.2,-3.03548715600002));
#353347=CARTESIAN_POINT('Ctrl Pts',(2.61209389699995,5.2,-3.03548715600002));
#353348=CARTESIAN_POINT('Ctrl Pts',(2.61209389699995,2.2,-3.03548715600002));
#353349=CARTESIAN_POINT('Ctrl Pts',(2.61237125599994,12.2,-3.03576462000001));
#353350=CARTESIAN_POINT('Ctrl Pts',(2.61237125599994,5.2,-3.03576462000001));
#353351=CARTESIAN_POINT('Ctrl Pts',(2.61237125599994,2.2,-3.03576462000001));
#353352=CARTESIAN_POINT('Ctrl Pts',(2.61265365899995,12.2,-3.03604638900001));
#353353=CARTESIAN_POINT('Ctrl Pts',(2.61265365899995,5.2,-3.03604638900001));
#353354=CARTESIAN_POINT('Ctrl Pts',(2.61265365899995,2.2,-3.03604638900001));
#353355=CARTESIAN_POINT('Ctrl Pts',(2.61294110599994,12.2,-3.03633243900002));
#353356=CARTESIAN_POINT('Ctrl Pts',(2.61294110599994,5.2,-3.03633243900002));
#353357=CARTESIAN_POINT('Ctrl Pts',(2.61294110599994,2.2,-3.03633243900002));
#353358=CARTESIAN_POINT('Ctrl Pts',(2.61323359999994,12.2,-3.03662274800002));
#353359=CARTESIAN_POINT('Ctrl Pts',(2.61323359999994,5.2,-3.03662274800002));
#353360=CARTESIAN_POINT('Ctrl Pts',(2.61323359999994,2.2,-3.03662274800002));
#353361=CARTESIAN_POINT('Ctrl Pts',(2.61353114199995,12.2,-3.03691729500001));
#353362=CARTESIAN_POINT('Ctrl Pts',(2.61353114199995,5.2,-3.03691729500001));
#353363=CARTESIAN_POINT('Ctrl Pts',(2.61353114199995,2.2,-3.03691729500001));
#353364=CARTESIAN_POINT('Ctrl Pts',(2.61383373399994,12.2,-3.03721605800002));
#353365=CARTESIAN_POINT('Ctrl Pts',(2.61383373399994,5.2,-3.03721605800002));
#353366=CARTESIAN_POINT('Ctrl Pts',(2.61383373399994,2.2,-3.03721605800002));
#353367=CARTESIAN_POINT('Ctrl Pts',(2.61414137899994,12.2,-3.03751901400001));
#353368=CARTESIAN_POINT('Ctrl Pts',(2.61414137899994,5.2,-3.03751901400001));
#353369=CARTESIAN_POINT('Ctrl Pts',(2.61414137899994,2.2,-3.03751901400001));
#353370=CARTESIAN_POINT('Ctrl Pts',(2.61445407699994,12.2,-3.03782614300002));
#353371=CARTESIAN_POINT('Ctrl Pts',(2.61445407699994,5.2,-3.03782614300002));
#353372=CARTESIAN_POINT('Ctrl Pts',(2.61445407699994,2.2,-3.03782614300002));
#353373=CARTESIAN_POINT('Ctrl Pts',(2.61477182999994,12.2,-3.03813742200001));
#353374=CARTESIAN_POINT('Ctrl Pts',(2.61477182999994,5.2,-3.03813742200001));
#353375=CARTESIAN_POINT('Ctrl Pts',(2.61477182999994,2.2,-3.03813742200001));
#353376=CARTESIAN_POINT('Ctrl Pts',(2.61509463899994,12.2,-3.03845282900001));
#353377=CARTESIAN_POINT('Ctrl Pts',(2.61509463899994,5.2,-3.03845282900001));
#353378=CARTESIAN_POINT('Ctrl Pts',(2.61509463899994,2.2,-3.03845282900001));
#353379=CARTESIAN_POINT('Ctrl Pts',(2.61542250699994,12.2,-3.03877234400002));
#353380=CARTESIAN_POINT('Ctrl Pts',(2.61542250699994,5.2,-3.03877234400002));
#353381=CARTESIAN_POINT('Ctrl Pts',(2.61542250699994,2.2,-3.03877234400002));
#353382=CARTESIAN_POINT('Ctrl Pts',(2.61575543499994,12.2,-3.03909594400002));
#353383=CARTESIAN_POINT('Ctrl Pts',(2.61575543499994,5.2,-3.03909594400002));
#353384=CARTESIAN_POINT('Ctrl Pts',(2.61575543499994,2.2,-3.03909594400002));
#353385=CARTESIAN_POINT('Ctrl Pts',(2.61609342599994,12.2,-3.03942360900002));
#353386=CARTESIAN_POINT('Ctrl Pts',(2.61609342599994,5.2,-3.03942360900002));
#353387=CARTESIAN_POINT('Ctrl Pts',(2.61609342599994,2.2,-3.03942360900002));
#353388=CARTESIAN_POINT('Ctrl Pts',(2.61643647899994,12.2,-3.03975531600001));
#353389=CARTESIAN_POINT('Ctrl Pts',(2.61643647899994,5.2,-3.03975531600001));
#353390=CARTESIAN_POINT('Ctrl Pts',(2.61643647899994,2.2,-3.03975531600001));
#353391=CARTESIAN_POINT('Ctrl Pts',(2.61678459599994,12.2,-3.04009104500001));
#353392=CARTESIAN_POINT('Ctrl Pts',(2.61678459599994,5.2,-3.04009104500001));
#353393=CARTESIAN_POINT('Ctrl Pts',(2.61678459599994,2.2,-3.04009104500001));
#353394=CARTESIAN_POINT('Ctrl Pts',(2.61713777799994,12.2,-3.04043077300001));
#353395=CARTESIAN_POINT('Ctrl Pts',(2.61713777799994,5.2,-3.04043077300001));
#353396=CARTESIAN_POINT('Ctrl Pts',(2.61713777799994,2.2,-3.04043077300001));
#353397=CARTESIAN_POINT('Ctrl Pts',(2.61749602899994,12.2,-3.04077448100001));
#353398=CARTESIAN_POINT('Ctrl Pts',(2.61749602899994,5.2,-3.04077448100001));
#353399=CARTESIAN_POINT('Ctrl Pts',(2.61749602899994,2.2,-3.04077448100001));
#353400=CARTESIAN_POINT('Ctrl Pts',(2.61785934799994,12.2,-3.04112214700002));
#353401=CARTESIAN_POINT('Ctrl Pts',(2.61785934799994,5.2,-3.04112214700002));
#353402=CARTESIAN_POINT('Ctrl Pts',(2.61785934799994,2.2,-3.04112214700002));
#353403=CARTESIAN_POINT('Ctrl Pts',(2.61822773799994,12.2,-3.04147374900001));
#353404=CARTESIAN_POINT('Ctrl Pts',(2.61822773799994,5.2,-3.04147374900001));
#353405=CARTESIAN_POINT('Ctrl Pts',(2.61822773799994,2.2,-3.04147374900001));
#353406=CARTESIAN_POINT('Ctrl Pts',(2.61860119799994,12.2,-3.04182926700001));
#353407=CARTESIAN_POINT('Ctrl Pts',(2.61860119799994,5.2,-3.04182926700001));
#353408=CARTESIAN_POINT('Ctrl Pts',(2.61860119799994,2.2,-3.04182926700001));
#353409=CARTESIAN_POINT('Ctrl Pts',(2.61897973099994,12.2,-3.04218868100001));
#353410=CARTESIAN_POINT('Ctrl Pts',(2.61897973099994,5.2,-3.04218868100001));
#353411=CARTESIAN_POINT('Ctrl Pts',(2.61897973099994,2.2,-3.04218868100001));
#353412=CARTESIAN_POINT('Ctrl Pts',(2.61936333899994,12.2,-3.04255196700002));
#353413=CARTESIAN_POINT('Ctrl Pts',(2.61936333899994,5.2,-3.04255196700002));
#353414=CARTESIAN_POINT('Ctrl Pts',(2.61936333899994,2.2,-3.04255196700002));
#353415=CARTESIAN_POINT('Ctrl Pts',(2.61975202199995,12.2,-3.04291910800002));
#353416=CARTESIAN_POINT('Ctrl Pts',(2.61975202199995,5.2,-3.04291910800002));
#353417=CARTESIAN_POINT('Ctrl Pts',(2.61975202199995,2.2,-3.04291910800002));
#353418=CARTESIAN_POINT('Ctrl Pts',(2.62014577999994,12.2,-3.04329008000002));
#353419=CARTESIAN_POINT('Ctrl Pts',(2.62014577999994,5.2,-3.04329008000002));
#353420=CARTESIAN_POINT('Ctrl Pts',(2.62014577999994,2.2,-3.04329008000002));
#353421=CARTESIAN_POINT('Ctrl Pts',(2.62054461699994,12.2,-3.04366486500002));
#353422=CARTESIAN_POINT('Ctrl Pts',(2.62054461699994,5.2,-3.04366486500002));
#353423=CARTESIAN_POINT('Ctrl Pts',(2.62054461699994,2.2,-3.04366486500002));
#353424=CARTESIAN_POINT('Ctrl Pts',(2.62094853299994,12.2,-3.04404344100002));
#353425=CARTESIAN_POINT('Ctrl Pts',(2.62094853299994,5.2,-3.04404344100002));
#353426=CARTESIAN_POINT('Ctrl Pts',(2.62094853299994,2.2,-3.04404344100002));
#353427=CARTESIAN_POINT('Ctrl Pts',(2.62135752799994,12.2,-3.04442578600002));
#353428=CARTESIAN_POINT('Ctrl Pts',(2.62135752799994,5.2,-3.04442578600002));
#353429=CARTESIAN_POINT('Ctrl Pts',(2.62135752799994,2.2,-3.04442578600002));
#353430=CARTESIAN_POINT('Ctrl Pts',(2.62177160499995,12.2,-3.04481188200001));
#353431=CARTESIAN_POINT('Ctrl Pts',(2.62177160499995,5.2,-3.04481188200001));
#353432=CARTESIAN_POINT('Ctrl Pts',(2.62177160499995,2.2,-3.04481188200001));
#353433=CARTESIAN_POINT('Ctrl Pts',(2.62219076399994,12.2,-3.04520170900001));
#353434=CARTESIAN_POINT('Ctrl Pts',(2.62219076399994,5.2,-3.04520170900001));
#353435=CARTESIAN_POINT('Ctrl Pts',(2.62219076399994,2.2,-3.04520170900001));
#353436=CARTESIAN_POINT('Ctrl Pts',(2.62261500499994,12.2,-3.04559524400001));
#353437=CARTESIAN_POINT('Ctrl Pts',(2.62261500499994,5.2,-3.04559524400001));
#353438=CARTESIAN_POINT('Ctrl Pts',(2.62261500499994,2.2,-3.04559524400001));
#353439=CARTESIAN_POINT('Ctrl Pts',(2.62304433199994,12.2,-3.04599246800001));
#353440=CARTESIAN_POINT('Ctrl Pts',(2.62304433199994,5.2,-3.04599246800001));
#353441=CARTESIAN_POINT('Ctrl Pts',(2.62304433199994,2.2,-3.04599246800001));
#353442=CARTESIAN_POINT('Ctrl Pts',(2.62347874199994,12.2,-3.04639336100001));
#353443=CARTESIAN_POINT('Ctrl Pts',(2.62347874199994,5.2,-3.04639336100001));
#353444=CARTESIAN_POINT('Ctrl Pts',(2.62347874199994,2.2,-3.04639336100001));
#353445=CARTESIAN_POINT('Ctrl Pts',(2.62391823999995,12.2,-3.04679790300002));
#353446=CARTESIAN_POINT('Ctrl Pts',(2.62391823999995,5.2,-3.04679790300002));
#353447=CARTESIAN_POINT('Ctrl Pts',(2.62391823999995,2.2,-3.04679790300002));
#353448=CARTESIAN_POINT('Ctrl Pts',(2.62436282399995,12.2,-3.04720607100001));
#353449=CARTESIAN_POINT('Ctrl Pts',(2.62436282399995,5.2,-3.04720607100001));
#353450=CARTESIAN_POINT('Ctrl Pts',(2.62436282399995,2.2,-3.04720607100001));
#353451=CARTESIAN_POINT('Ctrl Pts',(2.62481249599994,12.2,-3.04761785000002));
#353452=CARTESIAN_POINT('Ctrl Pts',(2.62481249599994,5.2,-3.04761785000002));
#353453=CARTESIAN_POINT('Ctrl Pts',(2.62481249599994,2.2,-3.04761785000002));
#353454=CARTESIAN_POINT('Ctrl Pts',(2.62526725699994,12.2,-3.04803321600001));
#353455=CARTESIAN_POINT('Ctrl Pts',(2.62526725699994,5.2,-3.04803321600001));
#353456=CARTESIAN_POINT('Ctrl Pts',(2.62526725699994,2.2,-3.04803321600001));
#353457=CARTESIAN_POINT('Ctrl Pts',(2.62572710899994,12.2,-3.04845215000002));
#353458=CARTESIAN_POINT('Ctrl Pts',(2.62572710899994,5.2,-3.04845215000002));
#353459=CARTESIAN_POINT('Ctrl Pts',(2.62572710899994,2.2,-3.04845215000002));
#353460=CARTESIAN_POINT('Ctrl Pts',(2.62619204999994,12.2,-3.04887463400001));
#353461=CARTESIAN_POINT('Ctrl Pts',(2.62619204999994,5.2,-3.04887463400001));
#353462=CARTESIAN_POINT('Ctrl Pts',(2.62619204999994,2.2,-3.04887463400001));
#353463=CARTESIAN_POINT('Ctrl Pts',(2.62666208299994,12.2,-3.04930064600001));
#353464=CARTESIAN_POINT('Ctrl Pts',(2.62666208299994,5.2,-3.04930064600001));
#353465=CARTESIAN_POINT('Ctrl Pts',(2.62666208299994,2.2,-3.04930064600001));
#353466=CARTESIAN_POINT('Ctrl Pts',(2.62713720799994,12.2,-3.04973016600002));
#353467=CARTESIAN_POINT('Ctrl Pts',(2.62713720799994,5.2,-3.04973016600002));
#353468=CARTESIAN_POINT('Ctrl Pts',(2.62713720799994,2.2,-3.04973016600002));
#353469=CARTESIAN_POINT('Ctrl Pts',(2.62761742699994,12.2,-3.05016317500002));
#353470=CARTESIAN_POINT('Ctrl Pts',(2.62761742699994,5.2,-3.05016317500002));
#353471=CARTESIAN_POINT('Ctrl Pts',(2.62761742699994,2.2,-3.05016317500002));
#353472=CARTESIAN_POINT('Ctrl Pts',(2.62810273799994,12.2,-3.05059965400002));
#353473=CARTESIAN_POINT('Ctrl Pts',(2.62810273799994,5.2,-3.05059965400002));
#353474=CARTESIAN_POINT('Ctrl Pts',(2.62810273799994,2.2,-3.05059965400002));
#353475=CARTESIAN_POINT('Ctrl Pts',(2.62859314499994,12.2,-3.05103958300001));
#353476=CARTESIAN_POINT('Ctrl Pts',(2.62859314499994,5.2,-3.05103958300001));
#353477=CARTESIAN_POINT('Ctrl Pts',(2.62859314499994,2.2,-3.05103958300001));
#353478=CARTESIAN_POINT('Ctrl Pts',(2.62908864599994,12.2,-3.05148294100002));
#353479=CARTESIAN_POINT('Ctrl Pts',(2.62908864599994,5.2,-3.05148294100002));
#353480=CARTESIAN_POINT('Ctrl Pts',(2.62908864599994,2.2,-3.05148294100002));
#353481=CARTESIAN_POINT('Ctrl Pts',(2.62958924299994,12.2,-3.05192971100002));
#353482=CARTESIAN_POINT('Ctrl Pts',(2.62958924299994,5.2,-3.05192971100002));
#353483=CARTESIAN_POINT('Ctrl Pts',(2.62958924299994,2.2,-3.05192971100002));
#353484=CARTESIAN_POINT('Ctrl Pts',(2.63009493599994,12.2,-3.05237987200002));
#353485=CARTESIAN_POINT('Ctrl Pts',(2.63009493599994,5.2,-3.05237987200002));
#353486=CARTESIAN_POINT('Ctrl Pts',(2.63009493599994,2.2,-3.05237987200002));
#353487=CARTESIAN_POINT('Ctrl Pts',(2.63060572599994,12.2,-3.05283340500001));
#353488=CARTESIAN_POINT('Ctrl Pts',(2.63060572599994,5.2,-3.05283340500001));
#353489=CARTESIAN_POINT('Ctrl Pts',(2.63060572599994,2.2,-3.05283340500001));
#353490=CARTESIAN_POINT('Ctrl Pts',(2.63112161299994,12.2,-3.05329029000001));
#353491=CARTESIAN_POINT('Ctrl Pts',(2.63112161299994,5.2,-3.05329029000001));
#353492=CARTESIAN_POINT('Ctrl Pts',(2.63112161299994,2.2,-3.05329029000001));
#353493=CARTESIAN_POINT('Ctrl Pts',(2.63164259999995,12.2,-3.05375050800002));
#353494=CARTESIAN_POINT('Ctrl Pts',(2.63164259999995,5.2,-3.05375050800002));
#353495=CARTESIAN_POINT('Ctrl Pts',(2.63164259999995,2.2,-3.05375050800002));
#353496=CARTESIAN_POINT('Ctrl Pts',(2.63216868399994,12.2,-3.05421404000001));
#353497=CARTESIAN_POINT('Ctrl Pts',(2.63216868399994,5.2,-3.05421404000001));
#353498=CARTESIAN_POINT('Ctrl Pts',(2.63216868399994,2.2,-3.05421404000001));
#353499=CARTESIAN_POINT('Ctrl Pts',(2.63269986699994,12.2,-3.05468086800001));
#353500=CARTESIAN_POINT('Ctrl Pts',(2.63269986699994,5.2,-3.05468086800001));
#353501=CARTESIAN_POINT('Ctrl Pts',(2.63269986699994,2.2,-3.05468086800001));
#353502=CARTESIAN_POINT('Ctrl Pts',(2.63323614999994,12.2,-3.05515097100002));
#353503=CARTESIAN_POINT('Ctrl Pts',(2.63323614999994,5.2,-3.05515097100002));
#353504=CARTESIAN_POINT('Ctrl Pts',(2.63323614999994,2.2,-3.05515097100002));
#353505=CARTESIAN_POINT('Ctrl Pts',(2.63377753299994,12.2,-3.05562433100001));
#353506=CARTESIAN_POINT('Ctrl Pts',(2.63377753299994,5.2,-3.05562433100001));
#353507=CARTESIAN_POINT('Ctrl Pts',(2.63377753299994,2.2,-3.05562433100001));
#353508=CARTESIAN_POINT('Ctrl Pts',(2.63432401599994,12.2,-3.05610092900002));
#353509=CARTESIAN_POINT('Ctrl Pts',(2.63432401599994,5.2,-3.05610092900002));
#353510=CARTESIAN_POINT('Ctrl Pts',(2.63432401599994,2.2,-3.05610092900002));
#353511=CARTESIAN_POINT('Ctrl Pts',(2.63487559999994,12.2,-3.05658074500001));
#353512=CARTESIAN_POINT('Ctrl Pts',(2.63487559999994,5.2,-3.05658074500001));
#353513=CARTESIAN_POINT('Ctrl Pts',(2.63487559999994,2.2,-3.05658074500001));
#353514=CARTESIAN_POINT('Ctrl Pts',(2.63543228599994,12.2,-3.05706376100002));
#353515=CARTESIAN_POINT('Ctrl Pts',(2.63543228599994,5.2,-3.05706376100002));
#353516=CARTESIAN_POINT('Ctrl Pts',(2.63543228599994,2.2,-3.05706376100002));
#353517=CARTESIAN_POINT('Ctrl Pts',(2.63599407299994,12.2,-3.05754995900001));
#353518=CARTESIAN_POINT('Ctrl Pts',(2.63599407299994,5.2,-3.05754995900001));
#353519=CARTESIAN_POINT('Ctrl Pts',(2.63599407299994,2.2,-3.05754995900001));
#353520=CARTESIAN_POINT('Ctrl Pts',(2.63656096199994,12.2,-3.05803931700002));
#353521=CARTESIAN_POINT('Ctrl Pts',(2.63656096199994,5.2,-3.05803931700002));
#353522=CARTESIAN_POINT('Ctrl Pts',(2.63656096199994,2.2,-3.05803931700002));
#353523=CARTESIAN_POINT('Ctrl Pts',(2.63713295299994,12.2,-3.05853182000002));
#353524=CARTESIAN_POINT('Ctrl Pts',(2.63713295299994,5.2,-3.05853182000002));
#353525=CARTESIAN_POINT('Ctrl Pts',(2.63713295299994,2.2,-3.05853182000002));
#353526=CARTESIAN_POINT('Ctrl Pts',(2.63771004699994,12.2,-3.05902744800001));
#353527=CARTESIAN_POINT('Ctrl Pts',(2.63771004699994,5.2,-3.05902744800001));
#353528=CARTESIAN_POINT('Ctrl Pts',(2.63771004699994,2.2,-3.05902744800001));
#353529=CARTESIAN_POINT('Ctrl Pts',(2.63829224399994,12.2,-3.05952618200001));
#353530=CARTESIAN_POINT('Ctrl Pts',(2.63829224399994,5.2,-3.05952618200001));
#353531=CARTESIAN_POINT('Ctrl Pts',(2.63829224399994,2.2,-3.05952618200001));
#353532=CARTESIAN_POINT('Ctrl Pts',(2.63887954299994,12.2,-3.06002800200002));
#353533=CARTESIAN_POINT('Ctrl Pts',(2.63887954299994,5.2,-3.06002800200002));
#353534=CARTESIAN_POINT('Ctrl Pts',(2.63887954299994,2.2,-3.06002800200002));
#353535=CARTESIAN_POINT('Ctrl Pts',(2.63947194599994,12.2,-3.06053289200001));
#353536=CARTESIAN_POINT('Ctrl Pts',(2.63947194599994,5.2,-3.06053289200001));
#353537=CARTESIAN_POINT('Ctrl Pts',(2.63947194599994,2.2,-3.06053289200001));
#353538=CARTESIAN_POINT('Ctrl Pts',(2.64006945299994,12.2,-3.06104083300001));
#353539=CARTESIAN_POINT('Ctrl Pts',(2.64006945299994,5.2,-3.06104083300001));
#353540=CARTESIAN_POINT('Ctrl Pts',(2.64006945299994,2.2,-3.06104083300001));
#353541=CARTESIAN_POINT('Ctrl Pts',(2.64067206299994,12.2,-3.06155180600001));
#353542=CARTESIAN_POINT('Ctrl Pts',(2.64067206299994,5.2,-3.06155180600001));
#353543=CARTESIAN_POINT('Ctrl Pts',(2.64067206299994,2.2,-3.06155180600001));
#353544=CARTESIAN_POINT('Ctrl Pts',(2.64127977599995,12.2,-3.06206579200001));
#353545=CARTESIAN_POINT('Ctrl Pts',(2.64127977599995,5.2,-3.06206579200001));
#353546=CARTESIAN_POINT('Ctrl Pts',(2.64127977599995,2.2,-3.06206579200001));
#353547=CARTESIAN_POINT('Ctrl Pts',(2.64189259399994,12.2,-3.06258277400001));
#353548=CARTESIAN_POINT('Ctrl Pts',(2.64189259399994,5.2,-3.06258277400001));
#353549=CARTESIAN_POINT('Ctrl Pts',(2.64189259399994,2.2,-3.06258277400001));
#353550=CARTESIAN_POINT('Ctrl Pts',(2.64251051499994,12.2,-3.06310273200001));
#353551=CARTESIAN_POINT('Ctrl Pts',(2.64251051499994,5.2,-3.06310273200001));
#353552=CARTESIAN_POINT('Ctrl Pts',(2.64251051499994,2.2,-3.06310273200001));
#353553=CARTESIAN_POINT('Ctrl Pts',(2.64313353999994,12.2,-3.06362564900001));
#353554=CARTESIAN_POINT('Ctrl Pts',(2.64313353999994,5.2,-3.06362564900001));
#353555=CARTESIAN_POINT('Ctrl Pts',(2.64313353999994,2.2,-3.06362564900001));
#353556=CARTESIAN_POINT('Ctrl Pts',(2.64376166999994,12.2,-3.06415150700001));
#353557=CARTESIAN_POINT('Ctrl Pts',(2.64376166999994,5.2,-3.06415150700001));
#353558=CARTESIAN_POINT('Ctrl Pts',(2.64376166999994,2.2,-3.06415150700001));
#353559=CARTESIAN_POINT('Ctrl Pts',(2.64439490399994,12.2,-3.06468028800001));
#353560=CARTESIAN_POINT('Ctrl Pts',(2.64439490399994,5.2,-3.06468028800001));
#353561=CARTESIAN_POINT('Ctrl Pts',(2.64439490399994,2.2,-3.06468028800001));
#353562=CARTESIAN_POINT('Ctrl Pts',(2.64503324199994,12.2,-3.06521197300002));
#353563=CARTESIAN_POINT('Ctrl Pts',(2.64503324199994,5.2,-3.06521197300002));
#353564=CARTESIAN_POINT('Ctrl Pts',(2.64503324199994,2.2,-3.06521197300002));
#353565=CARTESIAN_POINT('Ctrl Pts',(2.64567668399994,12.2,-3.06574654400002));
#353566=CARTESIAN_POINT('Ctrl Pts',(2.64567668399994,5.2,-3.06574654400002));
#353567=CARTESIAN_POINT('Ctrl Pts',(2.64567668399994,2.2,-3.06574654400002));
#353568=CARTESIAN_POINT('Ctrl Pts',(2.64632522999994,12.2,-3.06628398400001));
#353569=CARTESIAN_POINT('Ctrl Pts',(2.64632522999994,5.2,-3.06628398400001));
#353570=CARTESIAN_POINT('Ctrl Pts',(2.64632522999994,2.2,-3.06628398400001));
#353571=CARTESIAN_POINT('Ctrl Pts',(2.64697887999994,12.2,-3.06682427500002));
#353572=CARTESIAN_POINT('Ctrl Pts',(2.64697887999994,5.2,-3.06682427500002));
#353573=CARTESIAN_POINT('Ctrl Pts',(2.64697887999994,2.2,-3.06682427500002));
#353574=CARTESIAN_POINT('Ctrl Pts',(2.64763763499994,12.2,-3.06736739700002));
#353575=CARTESIAN_POINT('Ctrl Pts',(2.64763763499994,5.2,-3.06736739700002));
#353576=CARTESIAN_POINT('Ctrl Pts',(2.64763763499994,2.2,-3.06736739700002));
#353577=CARTESIAN_POINT('Ctrl Pts',(2.64830149199994,12.2,-3.06791333600001));
#353578=CARTESIAN_POINT('Ctrl Pts',(2.64830149199994,5.2,-3.06791333600001));
#353579=CARTESIAN_POINT('Ctrl Pts',(2.64830149199994,2.2,-3.06791333600001));
#353580=CARTESIAN_POINT('Ctrl Pts',(2.64897045499994,12.2,-3.06846207000001));
#353581=CARTESIAN_POINT('Ctrl Pts',(2.64897045499994,5.2,-3.06846207000001));
#353582=CARTESIAN_POINT('Ctrl Pts',(2.64897045499994,2.2,-3.06846207000001));
#353583=CARTESIAN_POINT('Ctrl Pts',(2.64964451899994,12.2,-3.06901358300002));
#353584=CARTESIAN_POINT('Ctrl Pts',(2.64964451899994,5.2,-3.06901358300002));
#353585=CARTESIAN_POINT('Ctrl Pts',(2.64964451899994,2.2,-3.06901358300002));
#353586=CARTESIAN_POINT('Ctrl Pts',(2.65032368799994,12.2,-3.06956785900002));
#353587=CARTESIAN_POINT('Ctrl Pts',(2.65032368799994,5.2,-3.06956785900002));
#353588=CARTESIAN_POINT('Ctrl Pts',(2.65032368799994,2.2,-3.06956785900002));
#353589=CARTESIAN_POINT('Ctrl Pts',(2.65100795999994,12.2,-3.07012487700002));
#353590=CARTESIAN_POINT('Ctrl Pts',(2.65100795999994,5.2,-3.07012487700002));
#353591=CARTESIAN_POINT('Ctrl Pts',(2.65100795999994,2.2,-3.07012487700002));
#353592=CARTESIAN_POINT('Ctrl Pts',(2.65169733399994,12.2,-3.07068462200002));
#353593=CARTESIAN_POINT('Ctrl Pts',(2.65169733399994,5.2,-3.07068462200002));
#353594=CARTESIAN_POINT('Ctrl Pts',(2.65169733399994,2.2,-3.07068462200002));
#353595=CARTESIAN_POINT('Ctrl Pts',(2.65239181199994,12.2,-3.07124707700002));
#353596=CARTESIAN_POINT('Ctrl Pts',(2.65239181199994,5.2,-3.07124707700002));
#353597=CARTESIAN_POINT('Ctrl Pts',(2.65239181199994,2.2,-3.07124707700002));
#353598=CARTESIAN_POINT('Ctrl Pts',(2.65309139299994,12.2,-3.07181222200001));
#353599=CARTESIAN_POINT('Ctrl Pts',(2.65309139299994,5.2,-3.07181222200001));
#353600=CARTESIAN_POINT('Ctrl Pts',(2.65309139299994,2.2,-3.07181222200001));
#353601=CARTESIAN_POINT('Ctrl Pts',(2.65379607499994,12.2,-3.07238004000002));
#353602=CARTESIAN_POINT('Ctrl Pts',(2.65379607499994,5.2,-3.07238004000002));
#353603=CARTESIAN_POINT('Ctrl Pts',(2.65379607499994,2.2,-3.07238004000002));
#353604=CARTESIAN_POINT('Ctrl Pts',(2.65450585899994,12.2,-3.07295051500001));
#353605=CARTESIAN_POINT('Ctrl Pts',(2.65450585899994,5.2,-3.07295051500001));
#353606=CARTESIAN_POINT('Ctrl Pts',(2.65450585899994,2.2,-3.07295051500001));
#353607=CARTESIAN_POINT('Ctrl Pts',(2.65522074599994,12.2,-3.07352363000001));
#353608=CARTESIAN_POINT('Ctrl Pts',(2.65522074599994,5.2,-3.07352363000001));
#353609=CARTESIAN_POINT('Ctrl Pts',(2.65522074599994,2.2,-3.07352363000001));
#353610=CARTESIAN_POINT('Ctrl Pts',(2.65594073299994,12.2,-3.07409936400001));
#353611=CARTESIAN_POINT('Ctrl Pts',(2.65594073299994,5.2,-3.07409936400001));
#353612=CARTESIAN_POINT('Ctrl Pts',(2.65594073299994,2.2,-3.07409936400001));
#353613=CARTESIAN_POINT('Ctrl Pts',(2.65666582099994,12.2,-3.07467770500002));
#353614=CARTESIAN_POINT('Ctrl Pts',(2.65666582099994,5.2,-3.07467770500002));
#353615=CARTESIAN_POINT('Ctrl Pts',(2.65666582099994,2.2,-3.07467770500002));
#353616=CARTESIAN_POINT('Ctrl Pts',(2.65739600999995,12.2,-3.07525863200001));
#353617=CARTESIAN_POINT('Ctrl Pts',(2.65739600999995,5.2,-3.07525863200001));
#353618=CARTESIAN_POINT('Ctrl Pts',(2.65739600999995,2.2,-3.07525863200001));
#353619=CARTESIAN_POINT('Ctrl Pts',(2.65813129899994,12.2,-3.07584212800001));
#353620=CARTESIAN_POINT('Ctrl Pts',(2.65813129899994,5.2,-3.07584212800001));
#353621=CARTESIAN_POINT('Ctrl Pts',(2.65813129899994,2.2,-3.07584212800001));
#353622=CARTESIAN_POINT('Ctrl Pts',(2.65887168799994,12.2,-3.07642817700001));
#353623=CARTESIAN_POINT('Ctrl Pts',(2.65887168799994,5.2,-3.07642817700001));
#353624=CARTESIAN_POINT('Ctrl Pts',(2.65887168799994,2.2,-3.07642817700001));
#353625=CARTESIAN_POINT('Ctrl Pts',(2.65961717599994,12.2,-3.07701676300002));
#353626=CARTESIAN_POINT('Ctrl Pts',(2.65961717599994,5.2,-3.07701676300002));
#353627=CARTESIAN_POINT('Ctrl Pts',(2.65961717599994,2.2,-3.07701676300002));
#353628=CARTESIAN_POINT('Ctrl Pts',(2.66036776299994,12.2,-3.07760786700001));
#353629=CARTESIAN_POINT('Ctrl Pts',(2.66036776299994,5.2,-3.07760786700001));
#353630=CARTESIAN_POINT('Ctrl Pts',(2.66036776299994,2.2,-3.07760786700001));
#353631=CARTESIAN_POINT('Ctrl Pts',(2.66112344799994,12.2,-3.07820147200002));
#353632=CARTESIAN_POINT('Ctrl Pts',(2.66112344799994,5.2,-3.07820147200002));
#353633=CARTESIAN_POINT('Ctrl Pts',(2.66112344799994,2.2,-3.07820147200002));
#353634=CARTESIAN_POINT('Ctrl Pts',(2.66188423199994,12.2,-3.07879756100002));
#353635=CARTESIAN_POINT('Ctrl Pts',(2.66188423199994,5.2,-3.07879756100002));
#353636=CARTESIAN_POINT('Ctrl Pts',(2.66188423199994,2.2,-3.07879756100002));
#353637=CARTESIAN_POINT('Ctrl Pts',(2.66265011199994,12.2,-3.07939611900002));
#353638=CARTESIAN_POINT('Ctrl Pts',(2.66265011199994,5.2,-3.07939611900002));
#353639=CARTESIAN_POINT('Ctrl Pts',(2.66265011199994,2.2,-3.07939611900002));
#353640=CARTESIAN_POINT('Ctrl Pts',(2.66342108999994,12.2,-3.07999712700001));
#353641=CARTESIAN_POINT('Ctrl Pts',(2.66342108999994,5.2,-3.07999712700001));
#353642=CARTESIAN_POINT('Ctrl Pts',(2.66342108999994,2.2,-3.07999712700001));
#353643=CARTESIAN_POINT('Ctrl Pts',(2.66419716399994,12.2,-3.08060056900001));
#353644=CARTESIAN_POINT('Ctrl Pts',(2.66419716399994,5.2,-3.08060056900001));
#353645=CARTESIAN_POINT('Ctrl Pts',(2.66419716399994,2.2,-3.08060056900001));
#353646=CARTESIAN_POINT('Ctrl Pts',(2.66497833299994,12.2,-3.08120642900001));
#353647=CARTESIAN_POINT('Ctrl Pts',(2.66497833299994,5.2,-3.08120642900001));
#353648=CARTESIAN_POINT('Ctrl Pts',(2.66497833299994,2.2,-3.08120642900001));
#353649=CARTESIAN_POINT('Ctrl Pts',(2.66576459699994,12.2,-3.08181468900001));
#353650=CARTESIAN_POINT('Ctrl Pts',(2.66576459699994,5.2,-3.08181468900001));
#353651=CARTESIAN_POINT('Ctrl Pts',(2.66576459699994,2.2,-3.08181468900001));
#353652=CARTESIAN_POINT('Ctrl Pts',(2.66655595599994,12.2,-3.08242533300001));
#353653=CARTESIAN_POINT('Ctrl Pts',(2.66655595599994,5.2,-3.08242533300001));
#353654=CARTESIAN_POINT('Ctrl Pts',(2.66655595599994,2.2,-3.08242533300001));
#353655=CARTESIAN_POINT('Ctrl Pts',(2.66735240899994,12.2,-3.08303834300002));
#353656=CARTESIAN_POINT('Ctrl Pts',(2.66735240899994,5.2,-3.08303834300002));
#353657=CARTESIAN_POINT('Ctrl Pts',(2.66735240899994,2.2,-3.08303834300002));
#353658=CARTESIAN_POINT('Ctrl Pts',(2.66815395399994,12.2,-3.08365370400002));
#353659=CARTESIAN_POINT('Ctrl Pts',(2.66815395399994,5.2,-3.08365370400002));
#353660=CARTESIAN_POINT('Ctrl Pts',(2.66815395399994,2.2,-3.08365370400002));
#353661=CARTESIAN_POINT('Ctrl Pts',(2.66896059199994,12.2,-3.08427139900001));
#353662=CARTESIAN_POINT('Ctrl Pts',(2.66896059199994,5.2,-3.08427139900001));
#353663=CARTESIAN_POINT('Ctrl Pts',(2.66896059199994,2.2,-3.08427139900001));
#353664=CARTESIAN_POINT('Ctrl Pts',(2.66977232299995,12.2,-3.08489141100001));
#353665=CARTESIAN_POINT('Ctrl Pts',(2.66977232299995,5.2,-3.08489141100001));
#353666=CARTESIAN_POINT('Ctrl Pts',(2.66977232299995,2.2,-3.08489141100001));
#353667=CARTESIAN_POINT('Ctrl Pts',(2.67058914399994,12.2,-3.08551372400002));
#353668=CARTESIAN_POINT('Ctrl Pts',(2.67058914399994,5.2,-3.08551372400002));
#353669=CARTESIAN_POINT('Ctrl Pts',(2.67058914399994,2.2,-3.08551372400002));
#353670=CARTESIAN_POINT('Ctrl Pts',(2.67141105599995,12.2,-3.08613832200002));
#353671=CARTESIAN_POINT('Ctrl Pts',(2.67141105599995,5.2,-3.08613832200002));
#353672=CARTESIAN_POINT('Ctrl Pts',(2.67141105599995,2.2,-3.08613832200002));
#353673=CARTESIAN_POINT('Ctrl Pts',(2.67223805599994,12.2,-3.08676518600001));
#353674=CARTESIAN_POINT('Ctrl Pts',(2.67223805599994,5.2,-3.08676518600001));
#353675=CARTESIAN_POINT('Ctrl Pts',(2.67223805599994,2.2,-3.08676518600001));
#353676=CARTESIAN_POINT('Ctrl Pts',(2.67307014599994,12.2,-3.08739430300002));
#353677=CARTESIAN_POINT('Ctrl Pts',(2.67307014599994,5.2,-3.08739430300002));
#353678=CARTESIAN_POINT('Ctrl Pts',(2.67307014599994,2.2,-3.08739430300002));
#353679=CARTESIAN_POINT('Ctrl Pts',(2.67390732399994,12.2,-3.08802565600002));
#353680=CARTESIAN_POINT('Ctrl Pts',(2.67390732399994,5.2,-3.08802565600002));
#353681=CARTESIAN_POINT('Ctrl Pts',(2.67390732399994,2.2,-3.08802565600002));
#353682=CARTESIAN_POINT('Ctrl Pts',(2.67474958899995,12.2,-3.08865922700001));
#353683=CARTESIAN_POINT('Ctrl Pts',(2.67474958899995,5.2,-3.08865922700001));
#353684=CARTESIAN_POINT('Ctrl Pts',(2.67474958899995,2.2,-3.08865922700001));
#353685=CARTESIAN_POINT('Ctrl Pts',(2.67559693999994,12.2,-3.08929500100001));
#353686=CARTESIAN_POINT('Ctrl Pts',(2.67559693999994,5.2,-3.08929500100001));
#353687=CARTESIAN_POINT('Ctrl Pts',(2.67559693999994,2.2,-3.08929500100001));
#353688=CARTESIAN_POINT('Ctrl Pts',(2.67644937699994,12.2,-3.08993296100001));
#353689=CARTESIAN_POINT('Ctrl Pts',(2.67644937699994,5.2,-3.08993296100001));
#353690=CARTESIAN_POINT('Ctrl Pts',(2.67644937699994,2.2,-3.08993296100001));
#353691=CARTESIAN_POINT('Ctrl Pts',(2.67730689799994,12.2,-3.09057309200002));
#353692=CARTESIAN_POINT('Ctrl Pts',(2.67730689799994,5.2,-3.09057309200002));
#353693=CARTESIAN_POINT('Ctrl Pts',(2.67730689799994,2.2,-3.09057309200002));
#353694=CARTESIAN_POINT('Ctrl Pts',(2.67816950399994,12.2,-3.09121537600001));
#353695=CARTESIAN_POINT('Ctrl Pts',(2.67816950399994,5.2,-3.09121537600001));
#353696=CARTESIAN_POINT('Ctrl Pts',(2.67816950399994,2.2,-3.09121537600001));
#353697=CARTESIAN_POINT('Ctrl Pts',(2.67903719199994,12.2,-3.09185980000001));
#353698=CARTESIAN_POINT('Ctrl Pts',(2.67903719199994,5.2,-3.09185980000001));
#353699=CARTESIAN_POINT('Ctrl Pts',(2.67903719199994,2.2,-3.09185980000001));
#353700=CARTESIAN_POINT('Ctrl Pts',(2.67990996199994,12.2,-3.09250634500001));
#353701=CARTESIAN_POINT('Ctrl Pts',(2.67990996199994,5.2,-3.09250634500001));
#353702=CARTESIAN_POINT('Ctrl Pts',(2.67990996199994,2.2,-3.09250634500001));
#353703=CARTESIAN_POINT('Ctrl Pts',(2.68078781199995,12.2,-3.09315499600002));
#353704=CARTESIAN_POINT('Ctrl Pts',(2.68078781199995,5.2,-3.09315499600002));
#353705=CARTESIAN_POINT('Ctrl Pts',(2.68078781199995,2.2,-3.09315499600002));
#353706=CARTESIAN_POINT('Ctrl Pts',(2.68167074299994,12.2,-3.09380573700002));
#353707=CARTESIAN_POINT('Ctrl Pts',(2.68167074299994,5.2,-3.09380573700002));
#353708=CARTESIAN_POINT('Ctrl Pts',(2.68167074299994,2.2,-3.09380573700002));
#353709=CARTESIAN_POINT('Ctrl Pts',(2.68255875399994,12.2,-3.09445855300002));
#353710=CARTESIAN_POINT('Ctrl Pts',(2.68255875399994,5.2,-3.09445855300002));
#353711=CARTESIAN_POINT('Ctrl Pts',(2.68255875399994,2.2,-3.09445855300002));
#353712=CARTESIAN_POINT('Ctrl Pts',(2.68345184199994,12.2,-3.09511342700001));
#353713=CARTESIAN_POINT('Ctrl Pts',(2.68345184199994,5.2,-3.09511342700001));
#353714=CARTESIAN_POINT('Ctrl Pts',(2.68345184199994,2.2,-3.09511342700001));
#353715=CARTESIAN_POINT('Ctrl Pts',(2.68435000699994,12.2,-3.09577034500002));
#353716=CARTESIAN_POINT('Ctrl Pts',(2.68435000699994,5.2,-3.09577034500002));
#353717=CARTESIAN_POINT('Ctrl Pts',(2.68435000699994,2.2,-3.09577034500002));
#353718=CARTESIAN_POINT('Ctrl Pts',(2.68525324699994,12.2,-3.09642928700002));
#353719=CARTESIAN_POINT('Ctrl Pts',(2.68525324699994,5.2,-3.09642928700002));
#353720=CARTESIAN_POINT('Ctrl Pts',(2.68525324699994,2.2,-3.09642928700002));
#353721=CARTESIAN_POINT('Ctrl Pts',(2.68616156399994,12.2,-3.09709024200002));
#353722=CARTESIAN_POINT('Ctrl Pts',(2.68616156399994,5.2,-3.09709024200002));
#353723=CARTESIAN_POINT('Ctrl Pts',(2.68616156399994,2.2,-3.09709024200002));
#353724=CARTESIAN_POINT('Ctrl Pts',(2.68707495399994,12.2,-3.09775319100002));
#353725=CARTESIAN_POINT('Ctrl Pts',(2.68707495399994,5.2,-3.09775319100002));
#353726=CARTESIAN_POINT('Ctrl Pts',(2.68707495399994,2.2,-3.09775319100002));
#353727=CARTESIAN_POINT('Ctrl Pts',(2.68799341599995,12.2,-3.09841812100002));
#353728=CARTESIAN_POINT('Ctrl Pts',(2.68799341599995,5.2,-3.09841812100002));
#353729=CARTESIAN_POINT('Ctrl Pts',(2.68799341599995,2.2,-3.09841812100002));
#353730=CARTESIAN_POINT('Ctrl Pts',(2.68891695099994,12.2,-3.09908501400002));
#353731=CARTESIAN_POINT('Ctrl Pts',(2.68891695099994,5.2,-3.09908501400002));
#353732=CARTESIAN_POINT('Ctrl Pts',(2.68891695099994,2.2,-3.09908501400002));
#353733=CARTESIAN_POINT('Ctrl Pts',(2.68984555499994,12.2,-3.09975385400001));
#353734=CARTESIAN_POINT('Ctrl Pts',(2.68984555499994,5.2,-3.09975385400001));
#353735=CARTESIAN_POINT('Ctrl Pts',(2.68984555499994,2.2,-3.09975385400001));
#353736=CARTESIAN_POINT('Ctrl Pts',(2.69077922999994,12.2,-3.10042462800002));
#353737=CARTESIAN_POINT('Ctrl Pts',(2.69077922999994,5.2,-3.10042462800002));
#353738=CARTESIAN_POINT('Ctrl Pts',(2.69077922999994,2.2,-3.10042462800002));
#353739=CARTESIAN_POINT('Ctrl Pts',(2.69171797199995,12.2,-3.10109732000001));
#353740=CARTESIAN_POINT('Ctrl Pts',(2.69171797199995,5.2,-3.10109732000001));
#353741=CARTESIAN_POINT('Ctrl Pts',(2.69171797199995,2.2,-3.10109732000001));
#353742=CARTESIAN_POINT('Ctrl Pts',(2.69266178199994,12.2,-3.10177191300001));
#353743=CARTESIAN_POINT('Ctrl Pts',(2.69266178199994,5.2,-3.10177191300001));
#353744=CARTESIAN_POINT('Ctrl Pts',(2.69266178199994,2.2,-3.10177191300001));
#353745=CARTESIAN_POINT('Ctrl Pts',(2.69361065799994,12.2,-3.10244839200001));
#353746=CARTESIAN_POINT('Ctrl Pts',(2.69361065799994,5.2,-3.10244839200001));
#353747=CARTESIAN_POINT('Ctrl Pts',(2.69361065799994,2.2,-3.10244839200001));
#353748=CARTESIAN_POINT('Ctrl Pts',(2.69456459899994,12.2,-3.10312674100001));
#353749=CARTESIAN_POINT('Ctrl Pts',(2.69456459899994,5.2,-3.10312674100001));
#353750=CARTESIAN_POINT('Ctrl Pts',(2.69456459899994,2.2,-3.10312674100001));
#353751=CARTESIAN_POINT('Ctrl Pts',(2.69552360299994,12.2,-3.10380694600001));
#353752=CARTESIAN_POINT('Ctrl Pts',(2.69552360299994,5.2,-3.10380694600001));
#353753=CARTESIAN_POINT('Ctrl Pts',(2.69552360299994,2.2,-3.10380694600001));
#353754=CARTESIAN_POINT('Ctrl Pts',(2.69648766799994,12.2,-3.10448899200002));
#353755=CARTESIAN_POINT('Ctrl Pts',(2.69648766799994,5.2,-3.10448899200002));
#353756=CARTESIAN_POINT('Ctrl Pts',(2.69648766799994,2.2,-3.10448899200002));
#353757=CARTESIAN_POINT('Ctrl Pts',(2.69745679499994,12.2,-3.10517286200001));
#353758=CARTESIAN_POINT('Ctrl Pts',(2.69745679499994,5.2,-3.10517286200001));
#353759=CARTESIAN_POINT('Ctrl Pts',(2.69745679499994,2.2,-3.10517286200001));
#353760=CARTESIAN_POINT('Ctrl Pts',(2.69843098199994,12.2,-3.10585854200002));
#353761=CARTESIAN_POINT('Ctrl Pts',(2.69843098199994,5.2,-3.10585854200002));
#353762=CARTESIAN_POINT('Ctrl Pts',(2.69843098199994,2.2,-3.10585854200002));
#353763=CARTESIAN_POINT('Ctrl Pts',(2.69941022799994,12.2,-3.10654601500001));
#353764=CARTESIAN_POINT('Ctrl Pts',(2.69941022799994,5.2,-3.10654601500001));
#353765=CARTESIAN_POINT('Ctrl Pts',(2.69941022799994,2.2,-3.10654601500001));
#353766=CARTESIAN_POINT('Ctrl Pts',(2.70039452999994,12.2,-3.10723526900002));
#353767=CARTESIAN_POINT('Ctrl Pts',(2.70039452999994,5.2,-3.10723526900002));
#353768=CARTESIAN_POINT('Ctrl Pts',(2.70039452999994,2.2,-3.10723526900002));
#353769=CARTESIAN_POINT('Ctrl Pts',(2.70138388799994,12.2,-3.10792628600002));
#353770=CARTESIAN_POINT('Ctrl Pts',(2.70138388799994,5.2,-3.10792628600002));
#353771=CARTESIAN_POINT('Ctrl Pts',(2.70138388799994,2.2,-3.10792628600002));
#353772=CARTESIAN_POINT('Ctrl Pts',(2.70237829999994,12.2,-3.10861905100001));
#353773=CARTESIAN_POINT('Ctrl Pts',(2.70237829999994,5.2,-3.10861905100001));
#353774=CARTESIAN_POINT('Ctrl Pts',(2.70237829999994,2.2,-3.10861905100001));
#353775=CARTESIAN_POINT('Ctrl Pts',(2.70337776599994,12.2,-3.10931355100001));
#353776=CARTESIAN_POINT('Ctrl Pts',(2.70337776599994,5.2,-3.10931355100001));
#353777=CARTESIAN_POINT('Ctrl Pts',(2.70337776599994,2.2,-3.10931355100001));
#353778=CARTESIAN_POINT('Ctrl Pts',(2.70438228399994,12.2,-3.11000976900001));
#353779=CARTESIAN_POINT('Ctrl Pts',(2.70438228399994,5.2,-3.11000976900001));
#353780=CARTESIAN_POINT('Ctrl Pts',(2.70438228399994,2.2,-3.11000976900001));
#353781=CARTESIAN_POINT('Ctrl Pts',(2.70539185199994,12.2,-3.11070769100001));
#353782=CARTESIAN_POINT('Ctrl Pts',(2.70539185199994,5.2,-3.11070769100001));
#353783=CARTESIAN_POINT('Ctrl Pts',(2.70539185199994,2.2,-3.11070769100001));
#353784=CARTESIAN_POINT('Ctrl Pts',(2.70640646799994,12.2,-3.11140730100002));
#353785=CARTESIAN_POINT('Ctrl Pts',(2.70640646799994,5.2,-3.11140730100002));
#353786=CARTESIAN_POINT('Ctrl Pts',(2.70640646799994,2.2,-3.11140730100002));
#353787=CARTESIAN_POINT('Ctrl Pts',(2.70742613199995,12.2,-3.11210858600001));
#353788=CARTESIAN_POINT('Ctrl Pts',(2.70742613199995,5.2,-3.11210858600001));
#353789=CARTESIAN_POINT('Ctrl Pts',(2.70742613199995,2.2,-3.11210858600001));
#353790=CARTESIAN_POINT('Ctrl Pts',(2.70845084199994,12.2,-3.11281152900001));
#353791=CARTESIAN_POINT('Ctrl Pts',(2.70845084199994,5.2,-3.11281152900001));
#353792=CARTESIAN_POINT('Ctrl Pts',(2.70845084199994,2.2,-3.11281152900001));
#353793=CARTESIAN_POINT('Ctrl Pts',(2.70948059699994,12.2,-3.11351611600001));
#353794=CARTESIAN_POINT('Ctrl Pts',(2.70948059699994,5.2,-3.11351611600001));
#353795=CARTESIAN_POINT('Ctrl Pts',(2.70948059699994,2.2,-3.11351611600001));
#353796=CARTESIAN_POINT('Ctrl Pts',(2.71051539499994,12.2,-3.11422233200001));
#353797=CARTESIAN_POINT('Ctrl Pts',(2.71051539499994,5.2,-3.11422233200001));
#353798=CARTESIAN_POINT('Ctrl Pts',(2.71051539499994,2.2,-3.11422233200001));
#353799=CARTESIAN_POINT('Ctrl Pts',(2.71155523399994,12.2,-3.11493016200002));
#353800=CARTESIAN_POINT('Ctrl Pts',(2.71155523399994,5.2,-3.11493016200002));
#353801=CARTESIAN_POINT('Ctrl Pts',(2.71155523399994,2.2,-3.11493016200002));
#353802=CARTESIAN_POINT('Ctrl Pts',(2.71260011399994,12.2,-3.11563959200001));
#353803=CARTESIAN_POINT('Ctrl Pts',(2.71260011399994,5.2,-3.11563959200001));
#353804=CARTESIAN_POINT('Ctrl Pts',(2.71260011399994,2.2,-3.11563959200001));
#353805=CARTESIAN_POINT('Ctrl Pts',(2.71365003199994,12.2,-3.11635060700001));
#353806=CARTESIAN_POINT('Ctrl Pts',(2.71365003199994,5.2,-3.11635060700001));
#353807=CARTESIAN_POINT('Ctrl Pts',(2.71365003199994,2.2,-3.11635060700001));
#353808=CARTESIAN_POINT('Ctrl Pts',(2.71470498699995,12.2,-3.11706319200002));
#353809=CARTESIAN_POINT('Ctrl Pts',(2.71470498699995,5.2,-3.11706319200002));
#353810=CARTESIAN_POINT('Ctrl Pts',(2.71470498699995,2.2,-3.11706319200002));
#353811=CARTESIAN_POINT('Ctrl Pts',(2.71576497699995,12.2,-3.11777733300001));
#353812=CARTESIAN_POINT('Ctrl Pts',(2.71576497699995,5.2,-3.11777733300001));
#353813=CARTESIAN_POINT('Ctrl Pts',(2.71576497699995,2.2,-3.11777733300001));
#353814=CARTESIAN_POINT('Ctrl Pts',(2.71683000299995,12.2,-3.11849301300001));
#353815=CARTESIAN_POINT('Ctrl Pts',(2.71683000299995,5.2,-3.11849301300001));
#353816=CARTESIAN_POINT('Ctrl Pts',(2.71683000299995,2.2,-3.11849301300001));
#353817=CARTESIAN_POINT('Ctrl Pts',(2.71790005899994,12.2,-3.11921022100002));
#353818=CARTESIAN_POINT('Ctrl Pts',(2.71790005899994,5.2,-3.11921022100002));
#353819=CARTESIAN_POINT('Ctrl Pts',(2.71790005899994,2.2,-3.11921022100002));
#353820=CARTESIAN_POINT('Ctrl Pts',(2.71897514799994,12.2,-3.11992894100001));
#353821=CARTESIAN_POINT('Ctrl Pts',(2.71897514799994,5.2,-3.11992894100001));
#353822=CARTESIAN_POINT('Ctrl Pts',(2.71897514799994,2.2,-3.11992894100001));
#353823=CARTESIAN_POINT('Ctrl Pts',(2.72005526399994,12.2,-3.12064915700001));
#353824=CARTESIAN_POINT('Ctrl Pts',(2.72005526399994,5.2,-3.12064915700001));
#353825=CARTESIAN_POINT('Ctrl Pts',(2.72005526399994,2.2,-3.12064915700001));
#353826=CARTESIAN_POINT('Ctrl Pts',(2.72114040899994,12.2,-3.12137085700002));
#353827=CARTESIAN_POINT('Ctrl Pts',(2.72114040899994,5.2,-3.12137085700002));
#353828=CARTESIAN_POINT('Ctrl Pts',(2.72114040899994,2.2,-3.12137085700002));
#353829=CARTESIAN_POINT('Ctrl Pts',(2.72223057899994,12.2,-3.12209402400002));
#353830=CARTESIAN_POINT('Ctrl Pts',(2.72223057899994,5.2,-3.12209402400002));
#353831=CARTESIAN_POINT('Ctrl Pts',(2.72223057899994,2.2,-3.12209402400002));
#353832=CARTESIAN_POINT('Ctrl Pts',(2.72332577399995,12.2,-3.12281864500001));
#353833=CARTESIAN_POINT('Ctrl Pts',(2.72332577399995,5.2,-3.12281864500001));
#353834=CARTESIAN_POINT('Ctrl Pts',(2.72332577399995,2.2,-3.12281864500001));
#353835=CARTESIAN_POINT('Ctrl Pts',(2.72442599199994,12.2,-3.12354470700001));
#353836=CARTESIAN_POINT('Ctrl Pts',(2.72442599199994,5.2,-3.12354470700001));
#353837=CARTESIAN_POINT('Ctrl Pts',(2.72442599199994,2.2,-3.12354470700001));
#353838=CARTESIAN_POINT('Ctrl Pts',(2.72553122899994,12.2,-3.12427219300002));
#353839=CARTESIAN_POINT('Ctrl Pts',(2.72553122899994,5.2,-3.12427219300002));
#353840=CARTESIAN_POINT('Ctrl Pts',(2.72553122899994,2.2,-3.12427219300002));
#353841=CARTESIAN_POINT('Ctrl Pts',(2.72664148599994,12.2,-3.12500108900001));
#353842=CARTESIAN_POINT('Ctrl Pts',(2.72664148599994,5.2,-3.12500108900001));
#353843=CARTESIAN_POINT('Ctrl Pts',(2.72664148599994,2.2,-3.12500108900001));
#353844=CARTESIAN_POINT('Ctrl Pts',(2.72775676099994,12.2,-3.12573138200001));
#353845=CARTESIAN_POINT('Ctrl Pts',(2.72775676099994,5.2,-3.12573138200001));
#353846=CARTESIAN_POINT('Ctrl Pts',(2.72775676099994,2.2,-3.12573138200001));
#353847=CARTESIAN_POINT('Ctrl Pts',(2.72887705099994,12.2,-3.12646305800001));
#353848=CARTESIAN_POINT('Ctrl Pts',(2.72887705099994,5.2,-3.12646305800001));
#353849=CARTESIAN_POINT('Ctrl Pts',(2.72887705099994,2.2,-3.12646305800001));
#353850=CARTESIAN_POINT('Ctrl Pts',(2.73000235499994,12.2,-3.12719610100002));
#353851=CARTESIAN_POINT('Ctrl Pts',(2.73000235499994,5.2,-3.12719610100002));
#353852=CARTESIAN_POINT('Ctrl Pts',(2.73000235499994,2.2,-3.12719610100002));
#353853=CARTESIAN_POINT('Ctrl Pts',(2.73113267199995,12.2,-3.12793049800002));
#353854=CARTESIAN_POINT('Ctrl Pts',(2.73113267199995,5.2,-3.12793049800002));
#353855=CARTESIAN_POINT('Ctrl Pts',(2.73113267199995,2.2,-3.12793049800002));
#353856=CARTESIAN_POINT('Ctrl Pts',(2.73226799899994,12.2,-3.12866623600002));
#353857=CARTESIAN_POINT('Ctrl Pts',(2.73226799899994,5.2,-3.12866623600002));
#353858=CARTESIAN_POINT('Ctrl Pts',(2.73226799899994,2.2,-3.12866623600002));
#353859=CARTESIAN_POINT('Ctrl Pts',(2.73340833399994,12.2,-3.12940329900002));
#353860=CARTESIAN_POINT('Ctrl Pts',(2.73340833399994,5.2,-3.12940329900002));
#353861=CARTESIAN_POINT('Ctrl Pts',(2.73340833399994,2.2,-3.12940329900002));
#353862=CARTESIAN_POINT('Ctrl Pts',(2.73455367599994,12.2,-3.13014167200001));
#353863=CARTESIAN_POINT('Ctrl Pts',(2.73455367599994,5.2,-3.13014167200001));
#353864=CARTESIAN_POINT('Ctrl Pts',(2.73455367599994,2.2,-3.13014167200001));
#353865=CARTESIAN_POINT('Ctrl Pts',(2.73570402299995,12.2,-3.13088134400001));
#353866=CARTESIAN_POINT('Ctrl Pts',(2.73570402299995,5.2,-3.13088134400001));
#353867=CARTESIAN_POINT('Ctrl Pts',(2.73570402299995,2.2,-3.13088134400001));
#353868=CARTESIAN_POINT('Ctrl Pts',(2.73685937399994,12.2,-3.13162229900001));
#353869=CARTESIAN_POINT('Ctrl Pts',(2.73685937399994,5.2,-3.13162229900001));
#353870=CARTESIAN_POINT('Ctrl Pts',(2.73685937399994,2.2,-3.13162229900001));
#353871=CARTESIAN_POINT('Ctrl Pts',(2.73801972499994,12.2,-3.13236452400002));
#353872=CARTESIAN_POINT('Ctrl Pts',(2.73801972499994,5.2,-3.13236452400002));
#353873=CARTESIAN_POINT('Ctrl Pts',(2.73801972499994,2.2,-3.13236452400002));
#353874=CARTESIAN_POINT('Ctrl Pts',(2.73918507599994,12.2,-3.13310800400001));
#353875=CARTESIAN_POINT('Ctrl Pts',(2.73918507599994,5.2,-3.13310800400001));
#353876=CARTESIAN_POINT('Ctrl Pts',(2.73918507599994,2.2,-3.13310800400001));
#353877=CARTESIAN_POINT('Ctrl Pts',(2.74035542399994,12.2,-3.13385272500001));
#353878=CARTESIAN_POINT('Ctrl Pts',(2.74035542399994,5.2,-3.13385272500001));
#353879=CARTESIAN_POINT('Ctrl Pts',(2.74035542399994,2.2,-3.13385272500001));
#353880=CARTESIAN_POINT('Ctrl Pts',(2.74153076699994,12.2,-3.13459867400002));
#353881=CARTESIAN_POINT('Ctrl Pts',(2.74153076699994,5.2,-3.13459867400002));
#353882=CARTESIAN_POINT('Ctrl Pts',(2.74153076699994,2.2,-3.13459867400002));
#353883=CARTESIAN_POINT('Ctrl Pts',(2.74271110499994,12.2,-3.13534583800001));
#353884=CARTESIAN_POINT('Ctrl Pts',(2.74271110499994,5.2,-3.13534583800001));
#353885=CARTESIAN_POINT('Ctrl Pts',(2.74271110499994,2.2,-3.13534583800001));
#353886=CARTESIAN_POINT('Ctrl Pts',(2.74389643499994,12.2,-3.13609420100001));
#353887=CARTESIAN_POINT('Ctrl Pts',(2.74389643499994,5.2,-3.13609420100001));
#353888=CARTESIAN_POINT('Ctrl Pts',(2.74389643499994,2.2,-3.13609420100001));
#353889=CARTESIAN_POINT('Ctrl Pts',(2.74508675499994,12.2,-3.13684375000001));
#353890=CARTESIAN_POINT('Ctrl Pts',(2.74508675499994,5.2,-3.13684375000001));
#353891=CARTESIAN_POINT('Ctrl Pts',(2.74508675499994,2.2,-3.13684375000001));
#353892=CARTESIAN_POINT('Ctrl Pts',(2.74628206099994,12.2,-3.13759447100002));
#353893=CARTESIAN_POINT('Ctrl Pts',(2.74628206099994,5.2,-3.13759447100002));
#353894=CARTESIAN_POINT('Ctrl Pts',(2.74628206099994,2.2,-3.13759447100002));
#353895=CARTESIAN_POINT('Ctrl Pts',(2.74748235499994,12.2,-3.13834635100001));
#353896=CARTESIAN_POINT('Ctrl Pts',(2.74748235499994,5.2,-3.13834635100001));
#353897=CARTESIAN_POINT('Ctrl Pts',(2.74748235499994,2.2,-3.13834635100001));
#353898=CARTESIAN_POINT('Ctrl Pts',(2.74868763199994,12.2,-3.13909937600001));
#353899=CARTESIAN_POINT('Ctrl Pts',(2.74868763199994,5.2,-3.13909937600001));
#353900=CARTESIAN_POINT('Ctrl Pts',(2.74868763199994,2.2,-3.13909937600001));
#353901=CARTESIAN_POINT('Ctrl Pts',(2.74989788999994,12.2,-3.13985353400001));
#353902=CARTESIAN_POINT('Ctrl Pts',(2.74989788999994,5.2,-3.13985353400001));
#353903=CARTESIAN_POINT('Ctrl Pts',(2.74989788999994,2.2,-3.13985353400001));
#353904=CARTESIAN_POINT('Ctrl Pts',(2.75111312999994,12.2,-3.14060880700001));
#353905=CARTESIAN_POINT('Ctrl Pts',(2.75111312999994,5.2,-3.14060880700001));
#353906=CARTESIAN_POINT('Ctrl Pts',(2.75111312999994,2.2,-3.14060880700001));
#353907=CARTESIAN_POINT('Ctrl Pts',(2.75233334699994,12.2,-3.14136518500002));
#353908=CARTESIAN_POINT('Ctrl Pts',(2.75233334699994,5.2,-3.14136518500002));
#353909=CARTESIAN_POINT('Ctrl Pts',(2.75233334699994,2.2,-3.14136518500002));
#353910=CARTESIAN_POINT('Ctrl Pts',(2.75355853999995,12.2,-3.14212265500001));
#353911=CARTESIAN_POINT('Ctrl Pts',(2.75355853999995,5.2,-3.14212265500001));
#353912=CARTESIAN_POINT('Ctrl Pts',(2.75355853999995,2.2,-3.14212265500001));
#353913=CARTESIAN_POINT('Ctrl Pts',(2.75478870599994,12.2,-3.14288120000001));
#353914=CARTESIAN_POINT('Ctrl Pts',(2.75478870599994,5.2,-3.14288120000001));
#353915=CARTESIAN_POINT('Ctrl Pts',(2.75478870599994,2.2,-3.14288120000001));
#353916=CARTESIAN_POINT('Ctrl Pts',(2.75602384399994,12.2,-3.14364080900001));
#353917=CARTESIAN_POINT('Ctrl Pts',(2.75602384399994,5.2,-3.14364080900001));
#353918=CARTESIAN_POINT('Ctrl Pts',(2.75602384399994,2.2,-3.14364080900001));
#353919=CARTESIAN_POINT('Ctrl Pts',(2.75726395199994,12.2,-3.14440146800001));
#353920=CARTESIAN_POINT('Ctrl Pts',(2.75726395199994,5.2,-3.14440146800001));
#353921=CARTESIAN_POINT('Ctrl Pts',(2.75726395199994,2.2,-3.14440146800001));
#353922=CARTESIAN_POINT('Ctrl Pts',(2.75850902699994,12.2,-3.14516316300002));
#353923=CARTESIAN_POINT('Ctrl Pts',(2.75850902699994,5.2,-3.14516316300002));
#353924=CARTESIAN_POINT('Ctrl Pts',(2.75850902699994,2.2,-3.14516316300002));
#353925=CARTESIAN_POINT('Ctrl Pts',(2.75975906799995,12.2,-3.14592588300001));
#353926=CARTESIAN_POINT('Ctrl Pts',(2.75975906799995,5.2,-3.14592588300001));
#353927=CARTESIAN_POINT('Ctrl Pts',(2.75975906799995,2.2,-3.14592588300001));
#353928=CARTESIAN_POINT('Ctrl Pts',(2.76101407199994,12.2,-3.14668961000002));
#353929=CARTESIAN_POINT('Ctrl Pts',(2.76101407199994,5.2,-3.14668961000002));
#353930=CARTESIAN_POINT('Ctrl Pts',(2.76101407199994,2.2,-3.14668961000002));
#353931=CARTESIAN_POINT('Ctrl Pts',(2.76227403799994,12.2,-3.14745433500002));
#353932=CARTESIAN_POINT('Ctrl Pts',(2.76227403799994,5.2,-3.14745433500002));
#353933=CARTESIAN_POINT('Ctrl Pts',(2.76227403799994,2.2,-3.14745433500002));
#353934=CARTESIAN_POINT('Ctrl Pts',(2.76353896199995,12.2,-3.14822004300002));
#353935=CARTESIAN_POINT('Ctrl Pts',(2.76353896199995,5.2,-3.14822004300002));
#353936=CARTESIAN_POINT('Ctrl Pts',(2.76353896199995,2.2,-3.14822004300002));
#353937=CARTESIAN_POINT('Ctrl Pts',(2.76480884399994,12.2,-3.14898672000002));
#353938=CARTESIAN_POINT('Ctrl Pts',(2.76480884399994,5.2,-3.14898672000002));
#353939=CARTESIAN_POINT('Ctrl Pts',(2.76480884399994,2.2,-3.14898672000002));
#353940=CARTESIAN_POINT('Ctrl Pts',(2.76608367999994,12.2,-3.14975435300001));
#353941=CARTESIAN_POINT('Ctrl Pts',(2.76608367999994,5.2,-3.14975435300001));
#353942=CARTESIAN_POINT('Ctrl Pts',(2.76608367999994,2.2,-3.14975435300001));
#353943=CARTESIAN_POINT('Ctrl Pts',(2.76736346799995,12.2,-3.15052293000001));
#353944=CARTESIAN_POINT('Ctrl Pts',(2.76736346799995,5.2,-3.15052293000001));
#353945=CARTESIAN_POINT('Ctrl Pts',(2.76736346799995,2.2,-3.15052293000001));
#353946=CARTESIAN_POINT('Ctrl Pts',(2.76864820699994,12.2,-3.15129243700001));
#353947=CARTESIAN_POINT('Ctrl Pts',(2.76864820699994,5.2,-3.15129243700001));
#353948=CARTESIAN_POINT('Ctrl Pts',(2.76864820699994,2.2,-3.15129243700001));
#353949=CARTESIAN_POINT('Ctrl Pts',(2.76993789399994,12.2,-3.15206286000001));
#353950=CARTESIAN_POINT('Ctrl Pts',(2.76993789399994,5.2,-3.15206286000001));
#353951=CARTESIAN_POINT('Ctrl Pts',(2.76993789399994,2.2,-3.15206286000001));
#353952=CARTESIAN_POINT('Ctrl Pts',(2.77123252699994,12.2,-3.15283418700002));
#353953=CARTESIAN_POINT('Ctrl Pts',(2.77123252699994,5.2,-3.15283418700002));
#353954=CARTESIAN_POINT('Ctrl Pts',(2.77123252699994,2.2,-3.15283418700002));
#353955=CARTESIAN_POINT('Ctrl Pts',(2.77253210399994,12.2,-3.15360640400002));
#353956=CARTESIAN_POINT('Ctrl Pts',(2.77253210399994,5.2,-3.15360640400002));
#353957=CARTESIAN_POINT('Ctrl Pts',(2.77253210399994,2.2,-3.15360640400002));
#353958=CARTESIAN_POINT('Ctrl Pts',(2.77383662199994,12.2,-3.15437949900002));
#353959=CARTESIAN_POINT('Ctrl Pts',(2.77383662199994,5.2,-3.15437949900002));
#353960=CARTESIAN_POINT('Ctrl Pts',(2.77383662199994,2.2,-3.15437949900002));
#353961=CARTESIAN_POINT('Ctrl Pts',(2.77514607899994,12.2,-3.15515345800002));
#353962=CARTESIAN_POINT('Ctrl Pts',(2.77514607899994,5.2,-3.15515345800002));
#353963=CARTESIAN_POINT('Ctrl Pts',(2.77514607899994,2.2,-3.15515345800002));
#353964=CARTESIAN_POINT('Ctrl Pts',(2.77646047299994,12.2,-3.15592826800001));
#353965=CARTESIAN_POINT('Ctrl Pts',(2.77646047299994,5.2,-3.15592826800001));
#353966=CARTESIAN_POINT('Ctrl Pts',(2.77646047299994,2.2,-3.15592826800001));
#353967=CARTESIAN_POINT('Ctrl Pts',(2.77777980199994,12.2,-3.15670391700001));
#353968=CARTESIAN_POINT('Ctrl Pts',(2.77777980199994,5.2,-3.15670391700001));
#353969=CARTESIAN_POINT('Ctrl Pts',(2.77777980199994,2.2,-3.15670391700001));
#353970=CARTESIAN_POINT('Ctrl Pts',(2.77910406199994,12.2,-3.15748039100002));
#353971=CARTESIAN_POINT('Ctrl Pts',(2.77910406199994,5.2,-3.15748039100002));
#353972=CARTESIAN_POINT('Ctrl Pts',(2.77910406199994,2.2,-3.15748039100002));
#353973=CARTESIAN_POINT('Ctrl Pts',(2.78043325399994,12.2,-3.15825767700002));
#353974=CARTESIAN_POINT('Ctrl Pts',(2.78043325399994,5.2,-3.15825767700002));
#353975=CARTESIAN_POINT('Ctrl Pts',(2.78043325399994,2.2,-3.15825767700002));
#353976=CARTESIAN_POINT('Ctrl Pts',(2.78176737199994,12.2,-3.15903576300002));
#353977=CARTESIAN_POINT('Ctrl Pts',(2.78176737199994,5.2,-3.15903576300002));
#353978=CARTESIAN_POINT('Ctrl Pts',(2.78176737199994,2.2,-3.15903576300002));
#353979=CARTESIAN_POINT('Ctrl Pts',(2.78310641599994,12.2,-3.15981463500002));
#353980=CARTESIAN_POINT('Ctrl Pts',(2.78310641599994,5.2,-3.15981463500002));
#353981=CARTESIAN_POINT('Ctrl Pts',(2.78310641599994,2.2,-3.15981463500002));
#353982=CARTESIAN_POINT('Ctrl Pts',(2.78445038299994,12.2,-3.16059428000001));
#353983=CARTESIAN_POINT('Ctrl Pts',(2.78445038299994,5.2,-3.16059428000001));
#353984=CARTESIAN_POINT('Ctrl Pts',(2.78445038299994,2.2,-3.16059428000001));
#353985=CARTESIAN_POINT('Ctrl Pts',(2.78579926999994,12.2,-3.16137468700001));
#353986=CARTESIAN_POINT('Ctrl Pts',(2.78579926999994,5.2,-3.16137468700001));
#353987=CARTESIAN_POINT('Ctrl Pts',(2.78579926999994,2.2,-3.16137468700001));
#353988=CARTESIAN_POINT('Ctrl Pts',(2.78715307499994,12.2,-3.16215584200001));
#353989=CARTESIAN_POINT('Ctrl Pts',(2.78715307499994,5.2,-3.16215584200001));
#353990=CARTESIAN_POINT('Ctrl Pts',(2.78715307499994,2.2,-3.16215584200001));
#353991=CARTESIAN_POINT('Ctrl Pts',(2.78851179699994,12.2,-3.16293773100002));
#353992=CARTESIAN_POINT('Ctrl Pts',(2.78851179699994,5.2,-3.16293773100002));
#353993=CARTESIAN_POINT('Ctrl Pts',(2.78851179699994,2.2,-3.16293773100002));
#353994=CARTESIAN_POINT('Ctrl Pts',(2.78987543099994,12.2,-3.16372034300001));
#353995=CARTESIAN_POINT('Ctrl Pts',(2.78987543099994,5.2,-3.16372034300001));
#353996=CARTESIAN_POINT('Ctrl Pts',(2.78987543099994,2.2,-3.16372034300001));
#353997=CARTESIAN_POINT('Ctrl Pts',(2.79124397599994,12.2,-3.16450366500002));
#353998=CARTESIAN_POINT('Ctrl Pts',(2.79124397599994,5.2,-3.16450366500002));
#353999=CARTESIAN_POINT('Ctrl Pts',(2.79124397599994,2.2,-3.16450366500002));
#354000=CARTESIAN_POINT('Ctrl Pts',(2.79261742999994,12.2,-3.16528768500001));
#354001=CARTESIAN_POINT('Ctrl Pts',(2.79261742999994,5.2,-3.16528768500001));
#354002=CARTESIAN_POINT('Ctrl Pts',(2.79261742999994,2.2,-3.16528768500001));
#354003=CARTESIAN_POINT('Ctrl Pts',(2.79399578999994,12.2,-3.16607238700001));
#354004=CARTESIAN_POINT('Ctrl Pts',(2.79399578999994,5.2,-3.16607238700001));
#354005=CARTESIAN_POINT('Ctrl Pts',(2.79399578999994,2.2,-3.16607238700001));
#354006=CARTESIAN_POINT('Ctrl Pts',(2.79537905499994,12.2,-3.16685776300002));
#354007=CARTESIAN_POINT('Ctrl Pts',(2.79537905499994,5.2,-3.16685776300002));
#354008=CARTESIAN_POINT('Ctrl Pts',(2.79537905499994,2.2,-3.16685776300002));
#354009=CARTESIAN_POINT('Ctrl Pts',(2.79676721799994,12.2,-3.16764379600002));
#354010=CARTESIAN_POINT('Ctrl Pts',(2.79676721799994,5.2,-3.16764379600002));
#354011=CARTESIAN_POINT('Ctrl Pts',(2.79676721799994,2.2,-3.16764379600002));
#354012=CARTESIAN_POINT('Ctrl Pts',(2.79816028199994,12.2,-3.16843047700001));
#354013=CARTESIAN_POINT('Ctrl Pts',(2.79816028199994,5.2,-3.16843047700001));
#354014=CARTESIAN_POINT('Ctrl Pts',(2.79816028199994,2.2,-3.16843047700001));
#354015=CARTESIAN_POINT('Ctrl Pts',(2.79955824199994,12.2,-3.16921779200001));
#354016=CARTESIAN_POINT('Ctrl Pts',(2.79955824199994,5.2,-3.16921779200001));
#354017=CARTESIAN_POINT('Ctrl Pts',(2.79955824199994,2.2,-3.16921779200001));
#354018=CARTESIAN_POINT('Ctrl Pts',(2.80096109499994,12.2,-3.17000572800001));
#354019=CARTESIAN_POINT('Ctrl Pts',(2.80096109499994,5.2,-3.17000572800001));
#354020=CARTESIAN_POINT('Ctrl Pts',(2.80096109499994,2.2,-3.17000572800001));
#354021=CARTESIAN_POINT('Ctrl Pts',(2.80236883999994,12.2,-3.17079427300001));
#354022=CARTESIAN_POINT('Ctrl Pts',(2.80236883999994,5.2,-3.17079427300001));
#354023=CARTESIAN_POINT('Ctrl Pts',(2.80236883999994,2.2,-3.17079427300001));
#354024=CARTESIAN_POINT('Ctrl Pts',(2.80378147399994,12.2,-3.17158341500001));
#354025=CARTESIAN_POINT('Ctrl Pts',(2.80378147399994,5.2,-3.17158341500001));
#354026=CARTESIAN_POINT('Ctrl Pts',(2.80378147399994,2.2,-3.17158341500001));
#354027=CARTESIAN_POINT('Ctrl Pts',(2.80519899199994,12.2,-3.17237314000002));
#354028=CARTESIAN_POINT('Ctrl Pts',(2.80519899199994,5.2,-3.17237314000002));
#354029=CARTESIAN_POINT('Ctrl Pts',(2.80519899199994,2.2,-3.17237314000002));
#354030=CARTESIAN_POINT('Ctrl Pts',(2.80662139499994,12.2,-3.17316343700002));
#354031=CARTESIAN_POINT('Ctrl Pts',(2.80662139499994,5.2,-3.17316343700002));
#354032=CARTESIAN_POINT('Ctrl Pts',(2.80662139499994,2.2,-3.17316343700002));
#354033=CARTESIAN_POINT('Ctrl Pts',(2.80804867999994,12.2,-3.17395429300001));
#354034=CARTESIAN_POINT('Ctrl Pts',(2.80804867999994,5.2,-3.17395429300001));
#354035=CARTESIAN_POINT('Ctrl Pts',(2.80804867999994,2.2,-3.17395429300001));
#354036=CARTESIAN_POINT('Ctrl Pts',(2.80948084099994,12.2,-3.17474569600002));
#354037=CARTESIAN_POINT('Ctrl Pts',(2.80948084099994,5.2,-3.17474569600002));
#354038=CARTESIAN_POINT('Ctrl Pts',(2.80948084099994,2.2,-3.17474569600002));
#354039=CARTESIAN_POINT('Ctrl Pts',(2.81091787999994,12.2,-3.17553763400001));
#354040=CARTESIAN_POINT('Ctrl Pts',(2.81091787999994,5.2,-3.17553763400001));
#354041=CARTESIAN_POINT('Ctrl Pts',(2.81091787999994,2.2,-3.17553763400001));
#354042=CARTESIAN_POINT('Ctrl Pts',(2.81235979099994,12.2,-3.17633009400001));
#354043=CARTESIAN_POINT('Ctrl Pts',(2.81235979099994,5.2,-3.17633009400001));
#354044=CARTESIAN_POINT('Ctrl Pts',(2.81235979099994,2.2,-3.17633009400001));
#354045=CARTESIAN_POINT('Ctrl Pts',(2.81380657399994,12.2,-3.17712306300002));
#354046=CARTESIAN_POINT('Ctrl Pts',(2.81380657399994,5.2,-3.17712306300002));
#354047=CARTESIAN_POINT('Ctrl Pts',(2.81380657399994,2.2,-3.17712306300002));
#354048=CARTESIAN_POINT('Ctrl Pts',(2.81525822399994,12.2,-3.17791653100001));
#354049=CARTESIAN_POINT('Ctrl Pts',(2.81525822399994,5.2,-3.17791653100001));
#354050=CARTESIAN_POINT('Ctrl Pts',(2.81525822399994,2.2,-3.17791653100001));
#354051=CARTESIAN_POINT('Ctrl Pts',(2.81671473899994,12.2,-3.17871048300002));
#354052=CARTESIAN_POINT('Ctrl Pts',(2.81671473899994,5.2,-3.17871048300002));
#354053=CARTESIAN_POINT('Ctrl Pts',(2.81671473899994,2.2,-3.17871048300002));
#354054=CARTESIAN_POINT('Ctrl Pts',(2.81817611699994,12.2,-3.17950490900001));
#354055=CARTESIAN_POINT('Ctrl Pts',(2.81817611699994,5.2,-3.17950490900001));
#354056=CARTESIAN_POINT('Ctrl Pts',(2.81817611699994,2.2,-3.17950490900001));
#354057=CARTESIAN_POINT('Ctrl Pts',(2.81964235599995,12.2,-3.18029979600002));
#354058=CARTESIAN_POINT('Ctrl Pts',(2.81964235599995,5.2,-3.18029979600002));
#354059=CARTESIAN_POINT('Ctrl Pts',(2.81964235599995,2.2,-3.18029979600002));
#354060=CARTESIAN_POINT('Ctrl Pts',(2.82111345099994,12.2,-3.18109513200001));
#354061=CARTESIAN_POINT('Ctrl Pts',(2.82111345099994,5.2,-3.18109513200001));
#354062=CARTESIAN_POINT('Ctrl Pts',(2.82111345099994,2.2,-3.18109513200001));
#354063=CARTESIAN_POINT('Ctrl Pts',(2.82258940099994,12.2,-3.18189090400002));
#354064=CARTESIAN_POINT('Ctrl Pts',(2.82258940099994,5.2,-3.18189090400002));
#354065=CARTESIAN_POINT('Ctrl Pts',(2.82258940099994,2.2,-3.18189090400002));
#354066=CARTESIAN_POINT('Ctrl Pts',(2.82407020299994,12.2,-3.18268710200002));
#354067=CARTESIAN_POINT('Ctrl Pts',(2.82407020299994,5.2,-3.18268710200002));
#354068=CARTESIAN_POINT('Ctrl Pts',(2.82407020299994,2.2,-3.18268710200002));
#354069=CARTESIAN_POINT('Ctrl Pts',(2.82555585599995,12.2,-3.18348371100001));
#354070=CARTESIAN_POINT('Ctrl Pts',(2.82555585599995,5.2,-3.18348371100001));
#354071=CARTESIAN_POINT('Ctrl Pts',(2.82555585599995,2.2,-3.18348371100001));
#354072=CARTESIAN_POINT('Ctrl Pts',(2.82704635399994,12.2,-3.18428072100001));
#354073=CARTESIAN_POINT('Ctrl Pts',(2.82704635399994,5.2,-3.18428072100001));
#354074=CARTESIAN_POINT('Ctrl Pts',(2.82704635399994,2.2,-3.18428072100001));
#354075=CARTESIAN_POINT('Ctrl Pts',(2.82854169599994,12.2,-3.18507812000002));
#354076=CARTESIAN_POINT('Ctrl Pts',(2.82854169599994,5.2,-3.18507812000002));
#354077=CARTESIAN_POINT('Ctrl Pts',(2.82854169599994,2.2,-3.18507812000002));
#354078=CARTESIAN_POINT('Ctrl Pts',(2.83004187899994,12.2,-3.18587589500002));
#354079=CARTESIAN_POINT('Ctrl Pts',(2.83004187899994,5.2,-3.18587589500002));
#354080=CARTESIAN_POINT('Ctrl Pts',(2.83004187899994,2.2,-3.18587589500002));
#354081=CARTESIAN_POINT('Ctrl Pts',(2.83154690099995,12.2,-3.18667403500001));
#354082=CARTESIAN_POINT('Ctrl Pts',(2.83154690099995,5.2,-3.18667403500001));
#354083=CARTESIAN_POINT('Ctrl Pts',(2.83154690099995,2.2,-3.18667403500001));
#354084=CARTESIAN_POINT('Ctrl Pts',(2.83305675899994,12.2,-3.18747252700001));
#354085=CARTESIAN_POINT('Ctrl Pts',(2.83305675899994,5.2,-3.18747252700001));
#354086=CARTESIAN_POINT('Ctrl Pts',(2.83305675899994,2.2,-3.18747252700001));
#354087=CARTESIAN_POINT('Ctrl Pts',(2.83457144899995,12.2,-3.18827136000001));
#354088=CARTESIAN_POINT('Ctrl Pts',(2.83457144899995,5.2,-3.18827136000001));
#354089=CARTESIAN_POINT('Ctrl Pts',(2.83457144899995,2.2,-3.18827136000001));
#354090=CARTESIAN_POINT('Ctrl Pts',(2.83609096999994,12.2,-3.18907052200001));
#354091=CARTESIAN_POINT('Ctrl Pts',(2.83609096999994,5.2,-3.18907052200001));
#354092=CARTESIAN_POINT('Ctrl Pts',(2.83609096999994,2.2,-3.18907052200001));
#354093=CARTESIAN_POINT('Ctrl Pts',(2.83761531699994,12.2,-3.18987000000002));
#354094=CARTESIAN_POINT('Ctrl Pts',(2.83761531699994,5.2,-3.18987000000002));
#354095=CARTESIAN_POINT('Ctrl Pts',(2.83761531699994,2.2,-3.18987000000002));
#354096=CARTESIAN_POINT('Ctrl Pts',(2.83914448999994,12.2,-3.19066978400001));
#354097=CARTESIAN_POINT('Ctrl Pts',(2.83914448999994,5.2,-3.19066978400001));
#354098=CARTESIAN_POINT('Ctrl Pts',(2.83914448999994,2.2,-3.19066978400001));
#354099=CARTESIAN_POINT('Ctrl Pts',(2.84067848399994,12.2,-3.19146986100002));
#354100=CARTESIAN_POINT('Ctrl Pts',(2.84067848399994,5.2,-3.19146986100002));
#354101=CARTESIAN_POINT('Ctrl Pts',(2.84067848399994,2.2,-3.19146986100002));
#354102=CARTESIAN_POINT('Ctrl Pts',(2.84221729699994,12.2,-3.19227021900002));
#354103=CARTESIAN_POINT('Ctrl Pts',(2.84221729699994,5.2,-3.19227021900002));
#354104=CARTESIAN_POINT('Ctrl Pts',(2.84221729699994,2.2,-3.19227021900002));
#354105=CARTESIAN_POINT('Ctrl Pts',(2.84376092599994,12.2,-3.19307084600001));
#354106=CARTESIAN_POINT('Ctrl Pts',(2.84376092599994,5.2,-3.19307084600001));
#354107=CARTESIAN_POINT('Ctrl Pts',(2.84376092599994,2.2,-3.19307084600001));
#354108=CARTESIAN_POINT('Ctrl Pts',(2.84530936799994,12.2,-3.19387173300001));
#354109=CARTESIAN_POINT('Ctrl Pts',(2.84530936799994,5.2,-3.19387173300001));
#354110=CARTESIAN_POINT('Ctrl Pts',(2.84530936799994,2.2,-3.19387173300001));
#354111=CARTESIAN_POINT('Ctrl Pts',(2.84686261999994,12.2,-3.19467286400001));
#354112=CARTESIAN_POINT('Ctrl Pts',(2.84686261999994,5.2,-3.19467286400001));
#354113=CARTESIAN_POINT('Ctrl Pts',(2.84686261999994,2.2,-3.19467286400001));
#354114=CARTESIAN_POINT('Ctrl Pts',(2.84842067999994,12.2,-3.19547423000001));
#354115=CARTESIAN_POINT('Ctrl Pts',(2.84842067999994,5.2,-3.19547423000001));
#354116=CARTESIAN_POINT('Ctrl Pts',(2.84842067999994,2.2,-3.19547423000001));
#354117=CARTESIAN_POINT('Ctrl Pts',(2.84998354499994,12.2,-3.19627582000001));
#354118=CARTESIAN_POINT('Ctrl Pts',(2.84998354499994,5.2,-3.19627582000001));
#354119=CARTESIAN_POINT('Ctrl Pts',(2.84998354499994,2.2,-3.19627582000001));
#354120=CARTESIAN_POINT('Ctrl Pts',(2.85155121099995,12.2,-3.19707762000002));
#354121=CARTESIAN_POINT('Ctrl Pts',(2.85155121099995,5.2,-3.19707762000002));
#354122=CARTESIAN_POINT('Ctrl Pts',(2.85155121099995,2.2,-3.19707762000002));
#354123=CARTESIAN_POINT('Ctrl Pts',(2.85312367599994,12.2,-3.19787962000001));
#354124=CARTESIAN_POINT('Ctrl Pts',(2.85312367599994,5.2,-3.19787962000001));
#354125=CARTESIAN_POINT('Ctrl Pts',(2.85312367599994,2.2,-3.19787962000001));
#354126=CARTESIAN_POINT('Ctrl Pts',(2.85470093699994,12.2,-3.19868180800002));
#354127=CARTESIAN_POINT('Ctrl Pts',(2.85470093699994,5.2,-3.19868180800002));
#354128=CARTESIAN_POINT('Ctrl Pts',(2.85470093699994,2.2,-3.19868180800002));
#354129=CARTESIAN_POINT('Ctrl Pts',(2.85628299099994,12.2,-3.19948417200001));
#354130=CARTESIAN_POINT('Ctrl Pts',(2.85628299099994,5.2,-3.19948417200001));
#354131=CARTESIAN_POINT('Ctrl Pts',(2.85628299099994,2.2,-3.19948417200001));
#354132=CARTESIAN_POINT('Ctrl Pts',(2.85786983499994,12.2,-3.20028670200001));
#354133=CARTESIAN_POINT('Ctrl Pts',(2.85786983499994,5.2,-3.20028670200001));
#354134=CARTESIAN_POINT('Ctrl Pts',(2.85786983499994,2.2,-3.20028670200001));
#354135=CARTESIAN_POINT('Ctrl Pts',(2.85946146699994,12.2,-3.20108938400002));
#354136=CARTESIAN_POINT('Ctrl Pts',(2.85946146699994,5.2,-3.20108938400002));
#354137=CARTESIAN_POINT('Ctrl Pts',(2.85946146699994,2.2,-3.20108938400002));
#354138=CARTESIAN_POINT('Ctrl Pts',(2.86105788299994,12.2,-3.20189220800001));
#354139=CARTESIAN_POINT('Ctrl Pts',(2.86105788299994,5.2,-3.20189220800001));
#354140=CARTESIAN_POINT('Ctrl Pts',(2.86105788299994,2.2,-3.20189220800001));
#354141=CARTESIAN_POINT('Ctrl Pts',(2.86265907899995,12.2,-3.20269516300002));
#354142=CARTESIAN_POINT('Ctrl Pts',(2.86265907899995,5.2,-3.20269516300002));
#354143=CARTESIAN_POINT('Ctrl Pts',(2.86265907899995,2.2,-3.20269516300002));
#354144=CARTESIAN_POINT('Ctrl Pts',(2.86426505399994,12.2,-3.20349823600001));
#354145=CARTESIAN_POINT('Ctrl Pts',(2.86426505399994,5.2,-3.20349823600001));
#354146=CARTESIAN_POINT('Ctrl Pts',(2.86426505399994,2.2,-3.20349823600001));
#354147=CARTESIAN_POINT('Ctrl Pts',(2.86587580399994,12.2,-3.20430141700002));
#354148=CARTESIAN_POINT('Ctrl Pts',(2.86587580399994,5.2,-3.20430141700002));
#354149=CARTESIAN_POINT('Ctrl Pts',(2.86587580399994,2.2,-3.20430141700002));
#354150=CARTESIAN_POINT('Ctrl Pts',(2.86749132599994,12.2,-3.20510469500002));
#354151=CARTESIAN_POINT('Ctrl Pts',(2.86749132599994,5.2,-3.20510469500002));
#354152=CARTESIAN_POINT('Ctrl Pts',(2.86749132599994,2.2,-3.20510469500002));
#354153=CARTESIAN_POINT('Ctrl Pts',(2.86911161699994,12.2,-3.20590805700002));
#354154=CARTESIAN_POINT('Ctrl Pts',(2.86911161699994,5.2,-3.20590805700002));
#354155=CARTESIAN_POINT('Ctrl Pts',(2.86911161699994,2.2,-3.20590805700002));
#354156=CARTESIAN_POINT('Ctrl Pts',(2.87073667499994,12.2,-3.20671149100002));
#354157=CARTESIAN_POINT('Ctrl Pts',(2.87073667499994,5.2,-3.20671149100002));
#354158=CARTESIAN_POINT('Ctrl Pts',(2.87073667499994,2.2,-3.20671149100002));
#354159=CARTESIAN_POINT('Ctrl Pts',(2.87236649699994,12.2,-3.20751498800002));
#354160=CARTESIAN_POINT('Ctrl Pts',(2.87236649699994,5.2,-3.20751498800002));
#354161=CARTESIAN_POINT('Ctrl Pts',(2.87236649699994,2.2,-3.20751498800002));
#354162=CARTESIAN_POINT('Ctrl Pts',(2.87400107799994,12.2,-3.20831853700001));
#354163=CARTESIAN_POINT('Ctrl Pts',(2.87400107799994,5.2,-3.20831853700001));
#354164=CARTESIAN_POINT('Ctrl Pts',(2.87400107799994,2.2,-3.20831853700001));
#354165=CARTESIAN_POINT('Ctrl Pts',(2.87564041599994,12.2,-3.20912212400001));
#354166=CARTESIAN_POINT('Ctrl Pts',(2.87564041599994,5.2,-3.20912212400001));
#354167=CARTESIAN_POINT('Ctrl Pts',(2.87564041599994,2.2,-3.20912212400001));
#354168=CARTESIAN_POINT('Ctrl Pts',(2.87728450899994,12.2,-3.20992574000002));
#354169=CARTESIAN_POINT('Ctrl Pts',(2.87728450899994,5.2,-3.20992574000002));
#354170=CARTESIAN_POINT('Ctrl Pts',(2.87728450899994,2.2,-3.20992574000002));
#354171=CARTESIAN_POINT('Ctrl Pts',(2.87893335299994,12.2,-3.21072937300002));
#354172=CARTESIAN_POINT('Ctrl Pts',(2.87893335299994,5.2,-3.21072937300002));
#354173=CARTESIAN_POINT('Ctrl Pts',(2.87893335299994,2.2,-3.21072937300002));
#354174=CARTESIAN_POINT('Ctrl Pts',(2.88058694399994,12.2,-3.21153301100002));
#354175=CARTESIAN_POINT('Ctrl Pts',(2.88058694399994,5.2,-3.21153301100002));
#354176=CARTESIAN_POINT('Ctrl Pts',(2.88058694399994,2.2,-3.21153301100002));
#354177=CARTESIAN_POINT('Ctrl Pts',(2.88224527999994,12.2,-3.21233664400001));
#354178=CARTESIAN_POINT('Ctrl Pts',(2.88224527999994,5.2,-3.21233664400001));
#354179=CARTESIAN_POINT('Ctrl Pts',(2.88224527999994,2.2,-3.21233664400001));
#354180=CARTESIAN_POINT('Ctrl Pts',(2.88390835799994,12.2,-3.21314026000001));
#354181=CARTESIAN_POINT('Ctrl Pts',(2.88390835799994,5.2,-3.21314026000001));
#354182=CARTESIAN_POINT('Ctrl Pts',(2.88390835799994,2.2,-3.21314026000001));
#354183=CARTESIAN_POINT('Ctrl Pts',(2.88557617499994,12.2,-3.21394384900001));
#354184=CARTESIAN_POINT('Ctrl Pts',(2.88557617499994,5.2,-3.21394384900001));
#354185=CARTESIAN_POINT('Ctrl Pts',(2.88557617499994,2.2,-3.21394384900001));
#354186=CARTESIAN_POINT('Ctrl Pts',(2.88724872799994,12.2,-3.21474739800002));
#354187=CARTESIAN_POINT('Ctrl Pts',(2.88724872799994,5.2,-3.21474739800002));
#354188=CARTESIAN_POINT('Ctrl Pts',(2.88724872799994,2.2,-3.21474739800002));
#354189=CARTESIAN_POINT('Ctrl Pts',(2.88892601299994,12.2,-3.21555089800002));
#354190=CARTESIAN_POINT('Ctrl Pts',(2.88892601299994,5.2,-3.21555089800002));
#354191=CARTESIAN_POINT('Ctrl Pts',(2.88892601299994,2.2,-3.21555089800002));
#354192=CARTESIAN_POINT('Ctrl Pts',(2.89060802699994,12.2,-3.21635433700001));
#354193=CARTESIAN_POINT('Ctrl Pts',(2.89060802699994,5.2,-3.21635433700001));
#354194=CARTESIAN_POINT('Ctrl Pts',(2.89060802699994,2.2,-3.21635433700001));
#354195=CARTESIAN_POINT('Ctrl Pts',(2.89229476699994,12.2,-3.21715770300001));
#354196=CARTESIAN_POINT('Ctrl Pts',(2.89229476699994,5.2,-3.21715770300001));
#354197=CARTESIAN_POINT('Ctrl Pts',(2.89229476699994,2.2,-3.21715770300001));
#354198=CARTESIAN_POINT('Ctrl Pts',(2.89398623099994,12.2,-3.21796098700001));
#354199=CARTESIAN_POINT('Ctrl Pts',(2.89398623099994,5.2,-3.21796098700001));
#354200=CARTESIAN_POINT('Ctrl Pts',(2.89398623099994,2.2,-3.21796098700001));
#354201=CARTESIAN_POINT('Ctrl Pts',(2.89568241399994,12.2,-3.21876417600001));
#354202=CARTESIAN_POINT('Ctrl Pts',(2.89568241399994,5.2,-3.21876417600001));
#354203=CARTESIAN_POINT('Ctrl Pts',(2.89568241399994,2.2,-3.21876417600001));
#354204=CARTESIAN_POINT('Ctrl Pts',(2.89738331399994,12.2,-3.21956726100002));
#354205=CARTESIAN_POINT('Ctrl Pts',(2.89738331399994,5.2,-3.21956726100002));
#354206=CARTESIAN_POINT('Ctrl Pts',(2.89738331399994,2.2,-3.21956726100002));
#354207=CARTESIAN_POINT('Ctrl Pts',(2.89908892699994,12.2,-3.22037022900002));
#354208=CARTESIAN_POINT('Ctrl Pts',(2.89908892699994,5.2,-3.22037022900002));
#354209=CARTESIAN_POINT('Ctrl Pts',(2.89908892699994,2.2,-3.22037022900002));
#354210=CARTESIAN_POINT('Ctrl Pts',(2.90079925099994,12.2,-3.22117307100001));
#354211=CARTESIAN_POINT('Ctrl Pts',(2.90079925099994,5.2,-3.22117307100001));
#354212=CARTESIAN_POINT('Ctrl Pts',(2.90079925099994,2.2,-3.22117307100001));
#354213=CARTESIAN_POINT('Ctrl Pts',(2.90251428199995,12.2,-3.22197577400001));
#354214=CARTESIAN_POINT('Ctrl Pts',(2.90251428199995,5.2,-3.22197577400001));
#354215=CARTESIAN_POINT('Ctrl Pts',(2.90251428199995,2.2,-3.22197577400001));
#354216=CARTESIAN_POINT('Ctrl Pts',(2.90423401699994,12.2,-3.22277832900001));
#354217=CARTESIAN_POINT('Ctrl Pts',(2.90423401699994,5.2,-3.22277832900001));
#354218=CARTESIAN_POINT('Ctrl Pts',(2.90423401699994,2.2,-3.22277832900001));
#354219=CARTESIAN_POINT('Ctrl Pts',(2.90595845199995,12.2,-3.22358072300001));
#354220=CARTESIAN_POINT('Ctrl Pts',(2.90595845199995,5.2,-3.22358072300001));
#354221=CARTESIAN_POINT('Ctrl Pts',(2.90595845199995,2.2,-3.22358072300001));
#354222=CARTESIAN_POINT('Ctrl Pts',(2.90768758499994,12.2,-3.22438294800001));
#354223=CARTESIAN_POINT('Ctrl Pts',(2.90768758499994,5.2,-3.22438294800001));
#354224=CARTESIAN_POINT('Ctrl Pts',(2.90768758499994,2.2,-3.22438294800001));
#354225=CARTESIAN_POINT('Ctrl Pts',(2.90942141199994,12.2,-3.22518499100001));
#354226=CARTESIAN_POINT('Ctrl Pts',(2.90942141199994,5.2,-3.22518499100001));
#354227=CARTESIAN_POINT('Ctrl Pts',(2.90942141199994,2.2,-3.22518499100001));
#354228=CARTESIAN_POINT('Ctrl Pts',(2.91115992999994,12.2,-3.22598684300001));
#354229=CARTESIAN_POINT('Ctrl Pts',(2.91115992999994,5.2,-3.22598684300001));
#354230=CARTESIAN_POINT('Ctrl Pts',(2.91115992999994,2.2,-3.22598684300001));
#354231=CARTESIAN_POINT('Ctrl Pts',(2.91290313599994,12.2,-3.22678849200001));
#354232=CARTESIAN_POINT('Ctrl Pts',(2.91290313599994,5.2,-3.22678849200001));
#354233=CARTESIAN_POINT('Ctrl Pts',(2.91290313599994,2.2,-3.22678849200001));
#354234=CARTESIAN_POINT('Ctrl Pts',(2.91465102699994,12.2,-3.22758992600002));
#354235=CARTESIAN_POINT('Ctrl Pts',(2.91465102699994,5.2,-3.22758992600002));
#354236=CARTESIAN_POINT('Ctrl Pts',(2.91465102699994,2.2,-3.22758992600002));
#354237=CARTESIAN_POINT('Ctrl Pts',(2.91640359899994,12.2,-3.22839113700002));
#354238=CARTESIAN_POINT('Ctrl Pts',(2.91640359899994,5.2,-3.22839113700002));
#354239=CARTESIAN_POINT('Ctrl Pts',(2.91640359899994,2.2,-3.22839113700002));
#354240=CARTESIAN_POINT('Ctrl Pts',(2.91816084799994,12.2,-3.22919211200002));
#354241=CARTESIAN_POINT('Ctrl Pts',(2.91816084799994,5.2,-3.22919211200002));
#354242=CARTESIAN_POINT('Ctrl Pts',(2.91816084799994,2.2,-3.22919211200002));
#354243=CARTESIAN_POINT('Ctrl Pts',(2.91992277299994,12.2,-3.22999284300002));
#354244=CARTESIAN_POINT('Ctrl Pts',(2.91992277299994,5.2,-3.22999284300002));
#354245=CARTESIAN_POINT('Ctrl Pts',(2.91992277299994,2.2,-3.22999284300002));
#354246=CARTESIAN_POINT('Ctrl Pts',(2.92168936799994,12.2,-3.23079331600002));
#354247=CARTESIAN_POINT('Ctrl Pts',(2.92168936799994,5.2,-3.23079331600002));
#354248=CARTESIAN_POINT('Ctrl Pts',(2.92168936799994,2.2,-3.23079331600002));
#354249=CARTESIAN_POINT('Ctrl Pts',(2.92346063199994,12.2,-3.23159352200001));
#354250=CARTESIAN_POINT('Ctrl Pts',(2.92346063199994,5.2,-3.23159352200001));
#354251=CARTESIAN_POINT('Ctrl Pts',(2.92346063199994,2.2,-3.23159352200001));
#354252=CARTESIAN_POINT('Ctrl Pts',(2.92523655999994,12.2,-3.23239345100002));
#354253=CARTESIAN_POINT('Ctrl Pts',(2.92523655999994,5.2,-3.23239345100002));
#354254=CARTESIAN_POINT('Ctrl Pts',(2.92523655999994,2.2,-3.23239345100002));
#354255=CARTESIAN_POINT('Ctrl Pts',(2.92701714899994,12.2,-3.23319309200001));
#354256=CARTESIAN_POINT('Ctrl Pts',(2.92701714899994,5.2,-3.23319309200001));
#354257=CARTESIAN_POINT('Ctrl Pts',(2.92701714899994,2.2,-3.23319309200001));
#354258=CARTESIAN_POINT('Ctrl Pts',(2.92880239599994,12.2,-3.23399243300001));
#354259=CARTESIAN_POINT('Ctrl Pts',(2.92880239599994,5.2,-3.23399243300001));
#354260=CARTESIAN_POINT('Ctrl Pts',(2.92880239599994,2.2,-3.23399243300001));
#354261=CARTESIAN_POINT('Ctrl Pts',(2.93059229899994,12.2,-3.23479146500001));
#354262=CARTESIAN_POINT('Ctrl Pts',(2.93059229899994,5.2,-3.23479146500001));
#354263=CARTESIAN_POINT('Ctrl Pts',(2.93059229899994,2.2,-3.23479146500001));
#354264=CARTESIAN_POINT('Ctrl Pts',(2.93238685199994,12.2,-3.23559017800001));
#354265=CARTESIAN_POINT('Ctrl Pts',(2.93238685199994,5.2,-3.23559017800001));
#354266=CARTESIAN_POINT('Ctrl Pts',(2.93238685199994,2.2,-3.23559017800001));
#354267=CARTESIAN_POINT('Ctrl Pts',(2.93418605299994,12.2,-3.23638855900001));
#354268=CARTESIAN_POINT('Ctrl Pts',(2.93418605299994,5.2,-3.23638855900001));
#354269=CARTESIAN_POINT('Ctrl Pts',(2.93418605299994,2.2,-3.23638855900001));
#354270=CARTESIAN_POINT('Ctrl Pts',(2.93598989899994,12.2,-3.23718660000001));
#354271=CARTESIAN_POINT('Ctrl Pts',(2.93598989899994,5.2,-3.23718660000001));
#354272=CARTESIAN_POINT('Ctrl Pts',(2.93598989899994,2.2,-3.23718660000001));
#354273=CARTESIAN_POINT('Ctrl Pts',(2.93779838599994,12.2,-3.23798429000002));
#354274=CARTESIAN_POINT('Ctrl Pts',(2.93779838599994,5.2,-3.23798429000002));
#354275=CARTESIAN_POINT('Ctrl Pts',(2.93779838599994,2.2,-3.23798429000002));
#354276=CARTESIAN_POINT('Ctrl Pts',(2.93961151099994,12.2,-3.23878161800002));
#354277=CARTESIAN_POINT('Ctrl Pts',(2.93961151099994,5.2,-3.23878161800002));
#354278=CARTESIAN_POINT('Ctrl Pts',(2.93961151099994,2.2,-3.23878161800002));
#354279=CARTESIAN_POINT('Ctrl Pts',(2.94142926999994,12.2,-3.23957857300002));
#354280=CARTESIAN_POINT('Ctrl Pts',(2.94142926999994,5.2,-3.23957857300002));
#354281=CARTESIAN_POINT('Ctrl Pts',(2.94142926999994,2.2,-3.23957857300002));
#354282=CARTESIAN_POINT('Ctrl Pts',(2.94325166099994,12.2,-3.24037514600001));
#354283=CARTESIAN_POINT('Ctrl Pts',(2.94325166099994,5.2,-3.24037514600001));
#354284=CARTESIAN_POINT('Ctrl Pts',(2.94325166099994,2.2,-3.24037514600001));
#354285=CARTESIAN_POINT('Ctrl Pts',(2.94507867899994,12.2,-3.24117132700001));
#354286=CARTESIAN_POINT('Ctrl Pts',(2.94507867899994,5.2,-3.24117132700001));
#354287=CARTESIAN_POINT('Ctrl Pts',(2.94507867899994,2.2,-3.24117132700001));
#354288=CARTESIAN_POINT('Ctrl Pts',(2.94691032199994,12.2,-3.24196710300001));
#354289=CARTESIAN_POINT('Ctrl Pts',(2.94691032199994,5.2,-3.24196710300001));
#354290=CARTESIAN_POINT('Ctrl Pts',(2.94691032199994,2.2,-3.24196710300001));
#354291=CARTESIAN_POINT('Ctrl Pts',(2.94874658399995,12.2,-3.24276246600002));
#354292=CARTESIAN_POINT('Ctrl Pts',(2.94874658399995,5.2,-3.24276246600002));
#354293=CARTESIAN_POINT('Ctrl Pts',(2.94874658399995,2.2,-3.24276246600002));
#354294=CARTESIAN_POINT('Ctrl Pts',(2.95058746399994,12.2,-3.24355740400001));
#354295=CARTESIAN_POINT('Ctrl Pts',(2.95058746399994,5.2,-3.24355740400001));
#354296=CARTESIAN_POINT('Ctrl Pts',(2.95058746399994,2.2,-3.24355740400001));
#354297=CARTESIAN_POINT('Ctrl Pts',(2.95243295799994,12.2,-3.24435190900001));
#354298=CARTESIAN_POINT('Ctrl Pts',(2.95243295799994,5.2,-3.24435190900001));
#354299=CARTESIAN_POINT('Ctrl Pts',(2.95243295799994,2.2,-3.24435190900001));
#354300=CARTESIAN_POINT('Ctrl Pts',(2.95428306199994,12.2,-3.24514596900002));
#354301=CARTESIAN_POINT('Ctrl Pts',(2.95428306199994,5.2,-3.24514596900002));
#354302=CARTESIAN_POINT('Ctrl Pts',(2.95428306199994,2.2,-3.24514596900002));
#354303=CARTESIAN_POINT('Ctrl Pts',(2.95613777399995,12.2,-3.24593957400001));
#354304=CARTESIAN_POINT('Ctrl Pts',(2.95613777399995,5.2,-3.24593957400001));
#354305=CARTESIAN_POINT('Ctrl Pts',(2.95613777399995,2.2,-3.24593957400001));
#354306=CARTESIAN_POINT('Ctrl Pts',(2.95799708799994,12.2,-3.24673271300002));
#354307=CARTESIAN_POINT('Ctrl Pts',(2.95799708799994,5.2,-3.24673271300002));
#354308=CARTESIAN_POINT('Ctrl Pts',(2.95799708799994,2.2,-3.24673271300002));
#354309=CARTESIAN_POINT('Ctrl Pts',(2.95986100299995,12.2,-3.24752537800002));
#354310=CARTESIAN_POINT('Ctrl Pts',(2.95986100299995,5.2,-3.24752537800002));
#354311=CARTESIAN_POINT('Ctrl Pts',(2.95986100299995,2.2,-3.24752537800002));
#354312=CARTESIAN_POINT('Ctrl Pts',(2.96172951299994,12.2,-3.24831755800002));
#354313=CARTESIAN_POINT('Ctrl Pts',(2.96172951299994,5.2,-3.24831755800002));
#354314=CARTESIAN_POINT('Ctrl Pts',(2.96172951299994,2.2,-3.24831755800002));
#354315=CARTESIAN_POINT('Ctrl Pts',(2.96360261799994,12.2,-3.24910924000001));
#354316=CARTESIAN_POINT('Ctrl Pts',(2.96360261799994,5.2,-3.24910924000001));
#354317=CARTESIAN_POINT('Ctrl Pts',(2.96360261799994,2.2,-3.24910924000001));
#354318=CARTESIAN_POINT('Ctrl Pts',(2.96548031099995,12.2,-3.24990041900001));
#354319=CARTESIAN_POINT('Ctrl Pts',(2.96548031099995,5.2,-3.24990041900001));
#354320=CARTESIAN_POINT('Ctrl Pts',(2.96548031099995,2.2,-3.24990041900001));
#354321=CARTESIAN_POINT('Ctrl Pts',(2.96736258999994,12.2,-3.25069108000001));
#354322=CARTESIAN_POINT('Ctrl Pts',(2.96736258999994,5.2,-3.25069108000001));
#354323=CARTESIAN_POINT('Ctrl Pts',(2.96736258999994,2.2,-3.25069108000001));
#354324=CARTESIAN_POINT('Ctrl Pts',(2.96924945199994,12.2,-3.25148121500002));
#354325=CARTESIAN_POINT('Ctrl Pts',(2.96924945199994,5.2,-3.25148121500002));
#354326=CARTESIAN_POINT('Ctrl Pts',(2.96924945199994,2.2,-3.25148121500002));
#354327=CARTESIAN_POINT('Ctrl Pts',(2.97114089099995,12.2,-3.25227081400001));
#354328=CARTESIAN_POINT('Ctrl Pts',(2.97114089099995,5.2,-3.25227081400001));
#354329=CARTESIAN_POINT('Ctrl Pts',(2.97114089099995,2.2,-3.25227081400001));
#354330=CARTESIAN_POINT('Ctrl Pts',(2.97303690699994,12.2,-3.25305986700001));
#354331=CARTESIAN_POINT('Ctrl Pts',(2.97303690699994,5.2,-3.25305986700001));
#354332=CARTESIAN_POINT('Ctrl Pts',(2.97303690699994,2.2,-3.25305986700001));
#354333=CARTESIAN_POINT('Ctrl Pts',(2.97493749499994,12.2,-3.25384836400001));
#354334=CARTESIAN_POINT('Ctrl Pts',(2.97493749499994,5.2,-3.25384836400001));
#354335=CARTESIAN_POINT('Ctrl Pts',(2.97493749499994,2.2,-3.25384836400001));
#354336=CARTESIAN_POINT('Ctrl Pts',(2.97684265099994,12.2,-3.25463629500002));
#354337=CARTESIAN_POINT('Ctrl Pts',(2.97684265099994,5.2,-3.25463629500002));
#354338=CARTESIAN_POINT('Ctrl Pts',(2.97684265099994,2.2,-3.25463629500002));
#354339=CARTESIAN_POINT('Ctrl Pts',(2.97875237099994,12.2,-3.25542364900001));
#354340=CARTESIAN_POINT('Ctrl Pts',(2.97875237099994,5.2,-3.25542364900001));
#354341=CARTESIAN_POINT('Ctrl Pts',(2.97875237099994,2.2,-3.25542364900001));
#354342=CARTESIAN_POINT('Ctrl Pts',(2.98066665199994,12.2,-3.25621041800002));
#354343=CARTESIAN_POINT('Ctrl Pts',(2.98066665199994,5.2,-3.25621041800002));
#354344=CARTESIAN_POINT('Ctrl Pts',(2.98066665199994,2.2,-3.25621041800002));
#354345=CARTESIAN_POINT('Ctrl Pts',(2.98258548999994,12.2,-3.25699658900001));
#354346=CARTESIAN_POINT('Ctrl Pts',(2.98258548999994,5.2,-3.25699658900001));
#354347=CARTESIAN_POINT('Ctrl Pts',(2.98258548999994,2.2,-3.25699658900001));
#354348=CARTESIAN_POINT('Ctrl Pts',(2.98450888299994,12.2,-3.25778215400002));
#354349=CARTESIAN_POINT('Ctrl Pts',(2.98450888299994,5.2,-3.25778215400002));
#354350=CARTESIAN_POINT('Ctrl Pts',(2.98450888299994,2.2,-3.25778215400002));
#354351=CARTESIAN_POINT('Ctrl Pts',(2.98643682599995,12.2,-3.25856710300001));
#354352=CARTESIAN_POINT('Ctrl Pts',(2.98643682599995,5.2,-3.25856710300001));
#354353=CARTESIAN_POINT('Ctrl Pts',(2.98643682599995,2.2,-3.25856710300001));
#354354=CARTESIAN_POINT('Ctrl Pts',(2.98836931499994,12.2,-3.25935142800001));
#354355=CARTESIAN_POINT('Ctrl Pts',(2.98836931499994,5.2,-3.25935142800001));
#354356=CARTESIAN_POINT('Ctrl Pts',(2.98836931499994,2.2,-3.25935142800001));
#354357=CARTESIAN_POINT('Ctrl Pts',(2.99030634799994,12.2,-3.26013511400001));
#354358=CARTESIAN_POINT('Ctrl Pts',(2.99030634799994,5.2,-3.26013511400001));
#354359=CARTESIAN_POINT('Ctrl Pts',(2.99030634799994,2.2,-3.26013511400001));
#354360=CARTESIAN_POINT('Ctrl Pts',(2.99224791899994,12.2,-3.26091815600002));
#354361=CARTESIAN_POINT('Ctrl Pts',(2.99224791899994,5.2,-3.26091815600002));
#354362=CARTESIAN_POINT('Ctrl Pts',(2.99224791899994,2.2,-3.26091815600002));
#354363=CARTESIAN_POINT('Ctrl Pts',(2.99419402599994,12.2,-3.26170054200002));
#354364=CARTESIAN_POINT('Ctrl Pts',(2.99419402599994,5.2,-3.26170054200002));
#354365=CARTESIAN_POINT('Ctrl Pts',(2.99419402599994,2.2,-3.26170054200002));
#354366=CARTESIAN_POINT('Ctrl Pts',(2.99614466599994,12.2,-3.26248226200001));
#354367=CARTESIAN_POINT('Ctrl Pts',(2.99614466599994,5.2,-3.26248226200001));
#354368=CARTESIAN_POINT('Ctrl Pts',(2.99614466599994,2.2,-3.26248226200001));
#354369=CARTESIAN_POINT('Ctrl Pts',(2.99809983499994,12.2,-3.26326330800002));
#354370=CARTESIAN_POINT('Ctrl Pts',(2.99809983499994,5.2,-3.26326330800002));
#354371=CARTESIAN_POINT('Ctrl Pts',(2.99809983499994,2.2,-3.26326330800002));
#354372=CARTESIAN_POINT('Ctrl Pts',(3.00005952799994,12.2,-3.26404366800002));
#354373=CARTESIAN_POINT('Ctrl Pts',(3.00005952799994,5.2,-3.26404366800002));
#354374=CARTESIAN_POINT('Ctrl Pts',(3.00005952799994,2.2,-3.26404366800002));
#354375=CARTESIAN_POINT('Ctrl Pts',(3.00202374199994,12.2,-3.26482333400001));
#354376=CARTESIAN_POINT('Ctrl Pts',(3.00202374199994,5.2,-3.26482333400001));
#354377=CARTESIAN_POINT('Ctrl Pts',(3.00202374199994,2.2,-3.26482333400001));
#354378=CARTESIAN_POINT('Ctrl Pts',(3.00399247299994,12.2,-3.26560229400001));
#354379=CARTESIAN_POINT('Ctrl Pts',(3.00399247299994,5.2,-3.26560229400001));
#354380=CARTESIAN_POINT('Ctrl Pts',(3.00399247299994,2.2,-3.26560229400001));
#354381=CARTESIAN_POINT('Ctrl Pts',(3.00596571799994,12.2,-3.26638054100002));
#354382=CARTESIAN_POINT('Ctrl Pts',(3.00596571799994,5.2,-3.26638054100002));
#354383=CARTESIAN_POINT('Ctrl Pts',(3.00596571799994,2.2,-3.26638054100002));
#354384=CARTESIAN_POINT('Ctrl Pts',(3.00794347399994,12.2,-3.26715806400002));
#354385=CARTESIAN_POINT('Ctrl Pts',(3.00794347399994,5.2,-3.26715806400002));
#354386=CARTESIAN_POINT('Ctrl Pts',(3.00794347399994,2.2,-3.26715806400002));
#354387=CARTESIAN_POINT('Ctrl Pts',(3.00992573499994,12.2,-3.26793485300001));
#354388=CARTESIAN_POINT('Ctrl Pts',(3.00992573499994,5.2,-3.26793485300001));
#354389=CARTESIAN_POINT('Ctrl Pts',(3.00992573499994,2.2,-3.26793485300001));
#354390=CARTESIAN_POINT('Ctrl Pts',(3.01191249899994,12.2,-3.26871089900001));
#354391=CARTESIAN_POINT('Ctrl Pts',(3.01191249899994,5.2,-3.26871089900001));
#354392=CARTESIAN_POINT('Ctrl Pts',(3.01191249899994,2.2,-3.26871089900001));
#354393=CARTESIAN_POINT('Ctrl Pts',(3.01390376299994,12.2,-3.26948619100001));
#354394=CARTESIAN_POINT('Ctrl Pts',(3.01390376299994,5.2,-3.26948619100001));
#354395=CARTESIAN_POINT('Ctrl Pts',(3.01390376299994,2.2,-3.26948619100001));
#354396=CARTESIAN_POINT('Ctrl Pts',(3.01589952199994,12.2,-3.27026072100002));
#354397=CARTESIAN_POINT('Ctrl Pts',(3.01589952199994,5.2,-3.27026072100002));
#354398=CARTESIAN_POINT('Ctrl Pts',(3.01589952199994,2.2,-3.27026072100002));
#354399=CARTESIAN_POINT('Ctrl Pts',(3.01789977199994,12.2,-3.27103447900001));
#354400=CARTESIAN_POINT('Ctrl Pts',(3.01789977199994,5.2,-3.27103447900001));
#354401=CARTESIAN_POINT('Ctrl Pts',(3.01789977199994,2.2,-3.27103447900001));
#354402=CARTESIAN_POINT('Ctrl Pts',(3.01990450999994,12.2,-3.27180745500002));
#354403=CARTESIAN_POINT('Ctrl Pts',(3.01990450999994,5.2,-3.27180745500002));
#354404=CARTESIAN_POINT('Ctrl Pts',(3.01990450999994,2.2,-3.27180745500002));
#354405=CARTESIAN_POINT('Ctrl Pts',(3.02191373299994,12.2,-3.27257964000002));
#354406=CARTESIAN_POINT('Ctrl Pts',(3.02191373299994,5.2,-3.27257964000002));
#354407=CARTESIAN_POINT('Ctrl Pts',(3.02191373299994,2.2,-3.27257964000002));
#354408=CARTESIAN_POINT('Ctrl Pts',(3.02392743499994,12.2,-3.27335102300002));
#354409=CARTESIAN_POINT('Ctrl Pts',(3.02392743499994,5.2,-3.27335102300002));
#354410=CARTESIAN_POINT('Ctrl Pts',(3.02392743499994,2.2,-3.27335102300002));
#354411=CARTESIAN_POINT('Ctrl Pts',(3.02594561299995,12.2,-3.27412159700001));
#354412=CARTESIAN_POINT('Ctrl Pts',(3.02594561299995,5.2,-3.27412159700001));
#354413=CARTESIAN_POINT('Ctrl Pts',(3.02594561299995,2.2,-3.27412159700001));
#354414=CARTESIAN_POINT('Ctrl Pts',(3.02796826499995,12.2,-3.27489135000001));
#354415=CARTESIAN_POINT('Ctrl Pts',(3.02796826499995,5.2,-3.27489135000001));
#354416=CARTESIAN_POINT('Ctrl Pts',(3.02796826499995,2.2,-3.27489135000001));
#354417=CARTESIAN_POINT('Ctrl Pts',(3.02999538599994,12.2,-3.27566027400001));
#354418=CARTESIAN_POINT('Ctrl Pts',(3.02999538599994,5.2,-3.27566027400001));
#354419=CARTESIAN_POINT('Ctrl Pts',(3.02999538599994,2.2,-3.27566027400001));
#354420=CARTESIAN_POINT('Ctrl Pts',(3.03202697199994,12.2,-3.27642835800001));
#354421=CARTESIAN_POINT('Ctrl Pts',(3.03202697199994,5.2,-3.27642835800001));
#354422=CARTESIAN_POINT('Ctrl Pts',(3.03202697199994,2.2,-3.27642835800001));
#354423=CARTESIAN_POINT('Ctrl Pts',(3.03406301999994,12.2,-3.27719559500002));
#354424=CARTESIAN_POINT('Ctrl Pts',(3.03406301999994,5.2,-3.27719559500002));
#354425=CARTESIAN_POINT('Ctrl Pts',(3.03406301999994,2.2,-3.27719559500002));
#354426=CARTESIAN_POINT('Ctrl Pts',(3.03610352499994,12.2,-3.27796197400001));
#354427=CARTESIAN_POINT('Ctrl Pts',(3.03610352499994,5.2,-3.27796197400001));
#354428=CARTESIAN_POINT('Ctrl Pts',(3.03610352499994,2.2,-3.27796197400001));
#354429=CARTESIAN_POINT('Ctrl Pts',(3.03814848399994,12.2,-3.27872748400001));
#354430=CARTESIAN_POINT('Ctrl Pts',(3.03814848399994,5.2,-3.27872748400001));
#354431=CARTESIAN_POINT('Ctrl Pts',(3.03814848399994,2.2,-3.27872748400001));
#354432=CARTESIAN_POINT('Ctrl Pts',(3.04019789299995,12.2,-3.27949211900001));
#354433=CARTESIAN_POINT('Ctrl Pts',(3.04019789299995,5.2,-3.27949211900001));
#354434=CARTESIAN_POINT('Ctrl Pts',(3.04019789299995,2.2,-3.27949211900001));
#354435=CARTESIAN_POINT('Ctrl Pts',(3.04225174799994,12.2,-3.28025586800001));
#354436=CARTESIAN_POINT('Ctrl Pts',(3.04225174799994,5.2,-3.28025586800001));
#354437=CARTESIAN_POINT('Ctrl Pts',(3.04225174799994,2.2,-3.28025586800001));
#354438=CARTESIAN_POINT('Ctrl Pts',(3.04431004599994,12.2,-3.28101872200001));
#354439=CARTESIAN_POINT('Ctrl Pts',(3.04431004599994,5.2,-3.28101872200001));
#354440=CARTESIAN_POINT('Ctrl Pts',(3.04431004599994,2.2,-3.28101872200001));
#354441=CARTESIAN_POINT('Ctrl Pts',(3.04637278199994,12.2,-3.28178067000001));
#354442=CARTESIAN_POINT('Ctrl Pts',(3.04637278199994,5.2,-3.28178067000001));
#354443=CARTESIAN_POINT('Ctrl Pts',(3.04637278199994,2.2,-3.28178067000001));
#354444=CARTESIAN_POINT('Ctrl Pts',(3.04843995199994,12.2,-3.28254170400001));
#354445=CARTESIAN_POINT('Ctrl Pts',(3.04843995199994,5.2,-3.28254170400001));
#354446=CARTESIAN_POINT('Ctrl Pts',(3.04843995199994,2.2,-3.28254170400001));
#354447=CARTESIAN_POINT('Ctrl Pts',(3.05051155499994,12.2,-3.28330181600001));
#354448=CARTESIAN_POINT('Ctrl Pts',(3.05051155499994,5.2,-3.28330181600001));
#354449=CARTESIAN_POINT('Ctrl Pts',(3.05051155499994,2.2,-3.28330181600001));
#354450=CARTESIAN_POINT('Ctrl Pts',(3.05258758299995,12.2,-3.28406099500001));
#354451=CARTESIAN_POINT('Ctrl Pts',(3.05258758299995,5.2,-3.28406099500001));
#354452=CARTESIAN_POINT('Ctrl Pts',(3.05258758299995,2.2,-3.28406099500001));
#354453=CARTESIAN_POINT('Ctrl Pts',(3.05466803499994,12.2,-3.28481923100002));
#354454=CARTESIAN_POINT('Ctrl Pts',(3.05466803499994,5.2,-3.28481923100002));
#354455=CARTESIAN_POINT('Ctrl Pts',(3.05466803499994,2.2,-3.28481923100002));
#354456=CARTESIAN_POINT('Ctrl Pts',(3.05675290699994,12.2,-3.28557651600001));
#354457=CARTESIAN_POINT('Ctrl Pts',(3.05675290699994,5.2,-3.28557651600001));
#354458=CARTESIAN_POINT('Ctrl Pts',(3.05675290699994,2.2,-3.28557651600001));
#354459=CARTESIAN_POINT('Ctrl Pts',(3.05884219399994,12.2,-3.28633284200002));
#354460=CARTESIAN_POINT('Ctrl Pts',(3.05884219399994,5.2,-3.28633284200002));
#354461=CARTESIAN_POINT('Ctrl Pts',(3.05884219399994,2.2,-3.28633284200002));
#354462=CARTESIAN_POINT('Ctrl Pts',(3.06093589199994,12.2,-3.28708819800001));
#354463=CARTESIAN_POINT('Ctrl Pts',(3.06093589199994,5.2,-3.28708819800001));
#354464=CARTESIAN_POINT('Ctrl Pts',(3.06093589199994,2.2,-3.28708819800001));
#354465=CARTESIAN_POINT('Ctrl Pts',(3.06303399699994,12.2,-3.28784257500002));
#354466=CARTESIAN_POINT('Ctrl Pts',(3.06303399699994,5.2,-3.28784257500002));
#354467=CARTESIAN_POINT('Ctrl Pts',(3.06303399699994,2.2,-3.28784257500002));
#354468=CARTESIAN_POINT('Ctrl Pts',(3.06513650699994,12.2,-3.28859596300001));
#354469=CARTESIAN_POINT('Ctrl Pts',(3.06513650699994,5.2,-3.28859596300001));
#354470=CARTESIAN_POINT('Ctrl Pts',(3.06513650699994,2.2,-3.28859596300001));
#354471=CARTESIAN_POINT('Ctrl Pts',(3.06724341699995,12.2,-3.28934835500001));
#354472=CARTESIAN_POINT('Ctrl Pts',(3.06724341699995,5.2,-3.28934835500001));
#354473=CARTESIAN_POINT('Ctrl Pts',(3.06724341699995,2.2,-3.28934835500001));
#354474=CARTESIAN_POINT('Ctrl Pts',(3.06935472199994,12.2,-3.29009974000002));
#354475=CARTESIAN_POINT('Ctrl Pts',(3.06935472199994,5.2,-3.29009974000002));
#354476=CARTESIAN_POINT('Ctrl Pts',(3.06935472199994,2.2,-3.29009974000002));
#354477=CARTESIAN_POINT('Ctrl Pts',(3.07147041999994,12.2,-3.29085011100001));
#354478=CARTESIAN_POINT('Ctrl Pts',(3.07147041999994,5.2,-3.29085011100001));
#354479=CARTESIAN_POINT('Ctrl Pts',(3.07147041999994,2.2,-3.29085011100001));
#354480=CARTESIAN_POINT('Ctrl Pts',(3.07359050599994,12.2,-3.29159945600002));
#354481=CARTESIAN_POINT('Ctrl Pts',(3.07359050599994,5.2,-3.29159945600002));
#354482=CARTESIAN_POINT('Ctrl Pts',(3.07359050599994,2.2,-3.29159945600002));
#354483=CARTESIAN_POINT('Ctrl Pts',(3.07571497499994,12.2,-3.29234776800002));
#354484=CARTESIAN_POINT('Ctrl Pts',(3.07571497499994,5.2,-3.29234776800002));
#354485=CARTESIAN_POINT('Ctrl Pts',(3.07571497499994,2.2,-3.29234776800002));
#354486=CARTESIAN_POINT('Ctrl Pts',(3.07784382499994,12.2,-3.29309503700001));
#354487=CARTESIAN_POINT('Ctrl Pts',(3.07784382499994,5.2,-3.29309503700001));
#354488=CARTESIAN_POINT('Ctrl Pts',(3.07784382499994,2.2,-3.29309503700001));
#354489=CARTESIAN_POINT('Ctrl Pts',(3.07997705199994,12.2,-3.29384125500002));
#354490=CARTESIAN_POINT('Ctrl Pts',(3.07997705199994,5.2,-3.29384125500002));
#354491=CARTESIAN_POINT('Ctrl Pts',(3.07997705199994,2.2,-3.29384125500002));
#354492=CARTESIAN_POINT('Ctrl Pts',(3.08211465099994,12.2,-3.29458641300001));
#354493=CARTESIAN_POINT('Ctrl Pts',(3.08211465099994,5.2,-3.29458641300001));
#354494=CARTESIAN_POINT('Ctrl Pts',(3.08211465099994,2.2,-3.29458641300001));
#354495=CARTESIAN_POINT('Ctrl Pts',(3.08425661699995,12.2,-3.29533050000002));
#354496=CARTESIAN_POINT('Ctrl Pts',(3.08425661699995,5.2,-3.29533050000002));
#354497=CARTESIAN_POINT('Ctrl Pts',(3.08425661699995,2.2,-3.29533050000002));
#354498=CARTESIAN_POINT('Ctrl Pts',(3.08640294899994,12.2,-3.29607351000002));
#354499=CARTESIAN_POINT('Ctrl Pts',(3.08640294899994,5.2,-3.29607351000002));
#354500=CARTESIAN_POINT('Ctrl Pts',(3.08640294899994,2.2,-3.29607351000002));
#354501=CARTESIAN_POINT('Ctrl Pts',(3.08855364099994,12.2,-3.29681543000001));
#354502=CARTESIAN_POINT('Ctrl Pts',(3.08855364099994,5.2,-3.29681543000001));
#354503=CARTESIAN_POINT('Ctrl Pts',(3.08855364099994,2.2,-3.29681543000001));
#354504=CARTESIAN_POINT('Ctrl Pts',(3.09070868999994,12.2,-3.29755625500002));
#354505=CARTESIAN_POINT('Ctrl Pts',(3.09070868999994,5.2,-3.29755625500002));
#354506=CARTESIAN_POINT('Ctrl Pts',(3.09070868999994,2.2,-3.29755625500002));
#354507=CARTESIAN_POINT('Ctrl Pts',(3.09286808999994,12.2,-3.29829597400002));
#354508=CARTESIAN_POINT('Ctrl Pts',(3.09286808999994,5.2,-3.29829597400002));
#354509=CARTESIAN_POINT('Ctrl Pts',(3.09286808999994,2.2,-3.29829597400002));
#354510=CARTESIAN_POINT('Ctrl Pts',(3.09503183999994,12.2,-3.29903457800001));
#354511=CARTESIAN_POINT('Ctrl Pts',(3.09503183999994,5.2,-3.29903457800001));
#354512=CARTESIAN_POINT('Ctrl Pts',(3.09503183999994,2.2,-3.29903457800001));
#354513=CARTESIAN_POINT('Ctrl Pts',(3.09719993399994,12.2,-3.29977205900001));
#354514=CARTESIAN_POINT('Ctrl Pts',(3.09719993399994,5.2,-3.29977205900001));
#354515=CARTESIAN_POINT('Ctrl Pts',(3.09719993399994,2.2,-3.29977205900001));
#354516=CARTESIAN_POINT('Ctrl Pts',(3.09937236799994,12.2,-3.30050840800002));
#354517=CARTESIAN_POINT('Ctrl Pts',(3.09937236799994,5.2,-3.30050840800002));
#354518=CARTESIAN_POINT('Ctrl Pts',(3.09937236799994,2.2,-3.30050840800002));
#354519=CARTESIAN_POINT('Ctrl Pts',(3.10154913999994,12.2,-3.30124361600001));
#354520=CARTESIAN_POINT('Ctrl Pts',(3.10154913999994,5.2,-3.30124361600001));
#354521=CARTESIAN_POINT('Ctrl Pts',(3.10154913999994,2.2,-3.30124361600001));
#354522=CARTESIAN_POINT('Ctrl Pts',(3.10373024299994,12.2,-3.30197767400001));
#354523=CARTESIAN_POINT('Ctrl Pts',(3.10373024299994,5.2,-3.30197767400001));
#354524=CARTESIAN_POINT('Ctrl Pts',(3.10373024299994,2.2,-3.30197767400001));
#354525=CARTESIAN_POINT('Ctrl Pts',(3.10591567499995,12.2,-3.30271057300001));
#354526=CARTESIAN_POINT('Ctrl Pts',(3.10591567499995,5.2,-3.30271057300001));
#354527=CARTESIAN_POINT('Ctrl Pts',(3.10591567499995,2.2,-3.30271057300001));
#354528=CARTESIAN_POINT('Ctrl Pts',(3.10810543099994,12.2,-3.30344230400001));
#354529=CARTESIAN_POINT('Ctrl Pts',(3.10810543099994,5.2,-3.30344230400001));
#354530=CARTESIAN_POINT('Ctrl Pts',(3.10810543099994,2.2,-3.30344230400001));
#354531=CARTESIAN_POINT('Ctrl Pts',(3.11029950799994,12.2,-3.30417286000001));
#354532=CARTESIAN_POINT('Ctrl Pts',(3.11029950799994,5.2,-3.30417286000001));
#354533=CARTESIAN_POINT('Ctrl Pts',(3.11029950799994,2.2,-3.30417286000001));
#354534=CARTESIAN_POINT('Ctrl Pts',(3.11249790099994,12.2,-3.30490222900002));
#354535=CARTESIAN_POINT('Ctrl Pts',(3.11249790099994,5.2,-3.30490222900002));
#354536=CARTESIAN_POINT('Ctrl Pts',(3.11249790099994,2.2,-3.30490222900002));
#354537=CARTESIAN_POINT('Ctrl Pts',(3.11470060599994,12.2,-3.30563040500001));
#354538=CARTESIAN_POINT('Ctrl Pts',(3.11470060599994,5.2,-3.30563040500001));
#354539=CARTESIAN_POINT('Ctrl Pts',(3.11470060599994,2.2,-3.30563040500001));
#354540=CARTESIAN_POINT('Ctrl Pts',(3.11690761999994,12.2,-3.30635737800002));
#354541=CARTESIAN_POINT('Ctrl Pts',(3.11690761999994,5.2,-3.30635737800002));
#354542=CARTESIAN_POINT('Ctrl Pts',(3.11690761999994,2.2,-3.30635737800002));
#354543=CARTESIAN_POINT('Ctrl Pts',(3.11911893699994,12.2,-3.30708314000002));
#354544=CARTESIAN_POINT('Ctrl Pts',(3.11911893699994,5.2,-3.30708314000002));
#354545=CARTESIAN_POINT('Ctrl Pts',(3.11911893699994,2.2,-3.30708314000002));
#354546=CARTESIAN_POINT('Ctrl Pts',(3.12133455499994,12.2,-3.30780768200002));
#354547=CARTESIAN_POINT('Ctrl Pts',(3.12133455499994,5.2,-3.30780768200002));
#354548=CARTESIAN_POINT('Ctrl Pts',(3.12133455499994,2.2,-3.30780768200002));
#354549=CARTESIAN_POINT('Ctrl Pts',(3.12355446899995,12.2,-3.30853099500001));
#354550=CARTESIAN_POINT('Ctrl Pts',(3.12355446899995,5.2,-3.30853099500001));
#354551=CARTESIAN_POINT('Ctrl Pts',(3.12355446899995,2.2,-3.30853099500001));
#354552=CARTESIAN_POINT('Ctrl Pts',(3.12577867499995,12.2,-3.30925307000001));
#354553=CARTESIAN_POINT('Ctrl Pts',(3.12577867499995,5.2,-3.30925307000001));
#354554=CARTESIAN_POINT('Ctrl Pts',(3.12577867499995,2.2,-3.30925307000001));
#354555=CARTESIAN_POINT('Ctrl Pts',(3.12800716799994,12.2,-3.30997389900002));
#354556=CARTESIAN_POINT('Ctrl Pts',(3.12800716799994,5.2,-3.30997389900002));
#354557=CARTESIAN_POINT('Ctrl Pts',(3.12800716799994,2.2,-3.30997389900002));
#354558=CARTESIAN_POINT('Ctrl Pts',(3.13023994599994,12.2,-3.31069347300001));
#354559=CARTESIAN_POINT('Ctrl Pts',(3.13023994599994,5.2,-3.31069347300001));
#354560=CARTESIAN_POINT('Ctrl Pts',(3.13023994599994,2.2,-3.31069347300001));
#354561=CARTESIAN_POINT('Ctrl Pts',(3.13247700299994,12.2,-3.31141178400001));
#354562=CARTESIAN_POINT('Ctrl Pts',(3.13247700299994,5.2,-3.31141178400001));
#354563=CARTESIAN_POINT('Ctrl Pts',(3.13247700299994,2.2,-3.31141178400001));
#354564=CARTESIAN_POINT('Ctrl Pts',(3.13471833499994,12.2,-3.31212882300001));
#354565=CARTESIAN_POINT('Ctrl Pts',(3.13471833499994,5.2,-3.31212882300001));
#354566=CARTESIAN_POINT('Ctrl Pts',(3.13471833499994,2.2,-3.31212882300001));
#354567=CARTESIAN_POINT('Ctrl Pts',(3.13696393899995,12.2,-3.31284458200001));
#354568=CARTESIAN_POINT('Ctrl Pts',(3.13696393899995,5.2,-3.31284458200001));
#354569=CARTESIAN_POINT('Ctrl Pts',(3.13696393899995,2.2,-3.31284458200001));
#354570=CARTESIAN_POINT('Ctrl Pts',(3.13921380999994,12.2,-3.31355905100001));
#354571=CARTESIAN_POINT('Ctrl Pts',(3.13921380999994,5.2,-3.31355905100001));
#354572=CARTESIAN_POINT('Ctrl Pts',(3.13921380999994,2.2,-3.31355905100001));
#354573=CARTESIAN_POINT('Ctrl Pts',(3.14146794399994,12.2,-3.31427222300002));
#354574=CARTESIAN_POINT('Ctrl Pts',(3.14146794399994,5.2,-3.31427222300002));
#354575=CARTESIAN_POINT('Ctrl Pts',(3.14146794399994,2.2,-3.31427222300002));
#354576=CARTESIAN_POINT('Ctrl Pts',(3.14372633799994,12.2,-3.31498408800002));
#354577=CARTESIAN_POINT('Ctrl Pts',(3.14372633799994,5.2,-3.31498408800002));
#354578=CARTESIAN_POINT('Ctrl Pts',(3.14372633799994,2.2,-3.31498408800002));
#354579=CARTESIAN_POINT('Ctrl Pts',(3.14598898599994,12.2,-3.31569463800002));
#354580=CARTESIAN_POINT('Ctrl Pts',(3.14598898599994,5.2,-3.31569463800002));
#354581=CARTESIAN_POINT('Ctrl Pts',(3.14598898599994,2.2,-3.31569463800002));
#354582=CARTESIAN_POINT('Ctrl Pts',(3.14825588499994,12.2,-3.31640386600002));
#354583=CARTESIAN_POINT('Ctrl Pts',(3.14825588499994,5.2,-3.31640386600002));
#354584=CARTESIAN_POINT('Ctrl Pts',(3.14825588499994,2.2,-3.31640386600002));
#354585=CARTESIAN_POINT('Ctrl Pts',(3.15052703099994,12.2,-3.31711176200002));
#354586=CARTESIAN_POINT('Ctrl Pts',(3.15052703099994,5.2,-3.31711176200002));
#354587=CARTESIAN_POINT('Ctrl Pts',(3.15052703099994,2.2,-3.31711176200002));
#354588=CARTESIAN_POINT('Ctrl Pts',(3.15280241899994,12.2,-3.31781831700001));
#354589=CARTESIAN_POINT('Ctrl Pts',(3.15280241899994,5.2,-3.31781831700001));
#354590=CARTESIAN_POINT('Ctrl Pts',(3.15280241899994,2.2,-3.31781831700001));
#354591=CARTESIAN_POINT('Ctrl Pts',(3.15508204599994,12.2,-3.31852352400002));
#354592=CARTESIAN_POINT('Ctrl Pts',(3.15508204599994,5.2,-3.31852352400002));
#354593=CARTESIAN_POINT('Ctrl Pts',(3.15508204599994,2.2,-3.31852352400002));
#354594=CARTESIAN_POINT('Ctrl Pts',(3.15736590599994,12.2,-3.31922737400001));
#354595=CARTESIAN_POINT('Ctrl Pts',(3.15736590599994,5.2,-3.31922737400001));
#354596=CARTESIAN_POINT('Ctrl Pts',(3.15736590599994,2.2,-3.31922737400001));
#354597=CARTESIAN_POINT('Ctrl Pts',(3.15965399599994,12.2,-3.31992985800001));
#354598=CARTESIAN_POINT('Ctrl Pts',(3.15965399599994,5.2,-3.31992985800001));
#354599=CARTESIAN_POINT('Ctrl Pts',(3.15965399599994,2.2,-3.31992985800001));
#354600=CARTESIAN_POINT('Ctrl Pts',(3.16194631299994,12.2,-3.32063096700002));
#354601=CARTESIAN_POINT('Ctrl Pts',(3.16194631299994,5.2,-3.32063096700002));
#354602=CARTESIAN_POINT('Ctrl Pts',(3.16194631299994,2.2,-3.32063096700002));
#354603=CARTESIAN_POINT('Ctrl Pts',(3.16424285099994,12.2,-3.32133069500001));
#354604=CARTESIAN_POINT('Ctrl Pts',(3.16424285099994,5.2,-3.32133069500001));
#354605=CARTESIAN_POINT('Ctrl Pts',(3.16424285099994,2.2,-3.32133069500001));
#354606=CARTESIAN_POINT('Ctrl Pts',(3.16654360599995,12.2,-3.32202903200002));
#354607=CARTESIAN_POINT('Ctrl Pts',(3.16654360599995,5.2,-3.32202903200002));
#354608=CARTESIAN_POINT('Ctrl Pts',(3.16654360599995,2.2,-3.32202903200002));
#354609=CARTESIAN_POINT('Ctrl Pts',(3.16884857399995,12.2,-3.32272597000001));
#354610=CARTESIAN_POINT('Ctrl Pts',(3.16884857399995,5.2,-3.32272597000001));
#354611=CARTESIAN_POINT('Ctrl Pts',(3.16884857399995,2.2,-3.32272597000001));
#354612=CARTESIAN_POINT('Ctrl Pts',(3.17115775199994,12.2,-3.32342150100001));
#354613=CARTESIAN_POINT('Ctrl Pts',(3.17115775199994,5.2,-3.32342150100001));
#354614=CARTESIAN_POINT('Ctrl Pts',(3.17115775199994,2.2,-3.32342150100001));
#354615=CARTESIAN_POINT('Ctrl Pts',(3.17347113499994,12.2,-3.32411561600002));
#354616=CARTESIAN_POINT('Ctrl Pts',(3.17347113499994,5.2,-3.32411561600002));
#354617=CARTESIAN_POINT('Ctrl Pts',(3.17347113499994,2.2,-3.32411561600002));
#354618=CARTESIAN_POINT('Ctrl Pts',(3.17578871699994,12.2,-3.32480830800002));
#354619=CARTESIAN_POINT('Ctrl Pts',(3.17578871699994,5.2,-3.32480830800002));
#354620=CARTESIAN_POINT('Ctrl Pts',(3.17578871699994,2.2,-3.32480830800002));
#354621=CARTESIAN_POINT('Ctrl Pts',(3.17811049599994,12.2,-3.32549956700001));
#354622=CARTESIAN_POINT('Ctrl Pts',(3.17811049599994,5.2,-3.32549956700001));
#354623=CARTESIAN_POINT('Ctrl Pts',(3.17811049599994,2.2,-3.32549956700001));
#354624=CARTESIAN_POINT('Ctrl Pts',(3.18043646699994,12.2,-3.32618938500001));
#354625=CARTESIAN_POINT('Ctrl Pts',(3.18043646699994,5.2,-3.32618938500001));
#354626=CARTESIAN_POINT('Ctrl Pts',(3.18043646699994,2.2,-3.32618938500001));
#354627=CARTESIAN_POINT('Ctrl Pts',(3.18276662599994,12.2,-3.32687775400001));
#354628=CARTESIAN_POINT('Ctrl Pts',(3.18276662599994,5.2,-3.32687775400001));
#354629=CARTESIAN_POINT('Ctrl Pts',(3.18276662599994,2.2,-3.32687775400001));
#354630=CARTESIAN_POINT('Ctrl Pts',(3.18510096799994,12.2,-3.32756466700001));
#354631=CARTESIAN_POINT('Ctrl Pts',(3.18510096799994,5.2,-3.32756466700001));
#354632=CARTESIAN_POINT('Ctrl Pts',(3.18510096799994,2.2,-3.32756466700001));
#354633=CARTESIAN_POINT('Ctrl Pts',(3.18743949099995,12.2,-3.32825011400002));
#354634=CARTESIAN_POINT('Ctrl Pts',(3.18743949099995,5.2,-3.32825011400002));
#354635=CARTESIAN_POINT('Ctrl Pts',(3.18743949099995,2.2,-3.32825011400002));
#354636=CARTESIAN_POINT('Ctrl Pts',(3.18978218799994,12.2,-3.32893408800001));
#354637=CARTESIAN_POINT('Ctrl Pts',(3.18978218799994,5.2,-3.32893408800001));
#354638=CARTESIAN_POINT('Ctrl Pts',(3.18978218799994,2.2,-3.32893408800001));
#354639=CARTESIAN_POINT('Ctrl Pts',(3.19212905499994,12.2,-3.32961658000002));
#354640=CARTESIAN_POINT('Ctrl Pts',(3.19212905499994,5.2,-3.32961658000002));
#354641=CARTESIAN_POINT('Ctrl Pts',(3.19212905499994,2.2,-3.32961658000002));
#354642=CARTESIAN_POINT('Ctrl Pts',(3.19448009099994,12.2,-3.33029758200002));
#354643=CARTESIAN_POINT('Ctrl Pts',(3.19448009099994,5.2,-3.33029758200002));
#354644=CARTESIAN_POINT('Ctrl Pts',(3.19448009099994,2.2,-3.33029758200002));
#354645=CARTESIAN_POINT('Ctrl Pts',(3.19683528699994,12.2,-3.33097708700001));
#354646=CARTESIAN_POINT('Ctrl Pts',(3.19683528699994,5.2,-3.33097708700001));
#354647=CARTESIAN_POINT('Ctrl Pts',(3.19683528699994,2.2,-3.33097708700001));
#354648=CARTESIAN_POINT('Ctrl Pts',(3.19919464199995,12.2,-3.33165508500001));
#354649=CARTESIAN_POINT('Ctrl Pts',(3.19919464199995,5.2,-3.33165508500001));
#354650=CARTESIAN_POINT('Ctrl Pts',(3.19919464199995,2.2,-3.33165508500001));
#354651=CARTESIAN_POINT('Ctrl Pts',(3.20155814999994,12.2,-3.33233157000001));
#354652=CARTESIAN_POINT('Ctrl Pts',(3.20155814999994,5.2,-3.33233157000001));
#354653=CARTESIAN_POINT('Ctrl Pts',(3.20155814999994,2.2,-3.33233157000001));
#354654=CARTESIAN_POINT('Ctrl Pts',(3.20392580899994,12.2,-3.33300653200002));
#354655=CARTESIAN_POINT('Ctrl Pts',(3.20392580899994,5.2,-3.33300653200002));
#354656=CARTESIAN_POINT('Ctrl Pts',(3.20392580899994,2.2,-3.33300653200002));
#354657=CARTESIAN_POINT('Ctrl Pts',(3.20629761299994,12.2,-3.33367996300002));
#354658=CARTESIAN_POINT('Ctrl Pts',(3.20629761299994,5.2,-3.33367996300002));
#354659=CARTESIAN_POINT('Ctrl Pts',(3.20629761299994,2.2,-3.33367996300002));
#354660=CARTESIAN_POINT('Ctrl Pts',(3.20867355699994,12.2,-3.33435185700001));
#354661=CARTESIAN_POINT('Ctrl Pts',(3.20867355699994,5.2,-3.33435185700001));
#354662=CARTESIAN_POINT('Ctrl Pts',(3.20867355699994,2.2,-3.33435185700001));
#354663=CARTESIAN_POINT('Ctrl Pts',(3.21105363699994,12.2,-3.33502220300002));
#354664=CARTESIAN_POINT('Ctrl Pts',(3.21105363699994,5.2,-3.33502220300002));
#354665=CARTESIAN_POINT('Ctrl Pts',(3.21105363699994,2.2,-3.33502220300002));
#354666=CARTESIAN_POINT('Ctrl Pts',(3.21343785099995,12.2,-3.33569099500002));
#354667=CARTESIAN_POINT('Ctrl Pts',(3.21343785099995,5.2,-3.33569099500002));
#354668=CARTESIAN_POINT('Ctrl Pts',(3.21343785099995,2.2,-3.33569099500002));
#354669=CARTESIAN_POINT('Ctrl Pts',(3.21582619199994,12.2,-3.33635822400002));
#354670=CARTESIAN_POINT('Ctrl Pts',(3.21582619199994,5.2,-3.33635822400002));
#354671=CARTESIAN_POINT('Ctrl Pts',(3.21582619199994,2.2,-3.33635822400002));
#354672=CARTESIAN_POINT('Ctrl Pts',(3.21821865699994,12.2,-3.33702388300001));
#354673=CARTESIAN_POINT('Ctrl Pts',(3.21821865699994,5.2,-3.33702388300001));
#354674=CARTESIAN_POINT('Ctrl Pts',(3.21821865699994,2.2,-3.33702388300001));
#354675=CARTESIAN_POINT('Ctrl Pts',(3.22061524099994,12.2,-3.33768796400001));
#354676=CARTESIAN_POINT('Ctrl Pts',(3.22061524099994,5.2,-3.33768796400001));
#354677=CARTESIAN_POINT('Ctrl Pts',(3.22061524099994,2.2,-3.33768796400001));
#354678=CARTESIAN_POINT('Ctrl Pts',(3.22301593999994,12.2,-3.33835045800001));
#354679=CARTESIAN_POINT('Ctrl Pts',(3.22301593999994,5.2,-3.33835045800001));
#354680=CARTESIAN_POINT('Ctrl Pts',(3.22301593999994,2.2,-3.33835045800001));
#354681=CARTESIAN_POINT('Ctrl Pts',(3.22542074999994,12.2,-3.33901135600001));
#354682=CARTESIAN_POINT('Ctrl Pts',(3.22542074999994,5.2,-3.33901135600001));
#354683=CARTESIAN_POINT('Ctrl Pts',(3.22542074999994,2.2,-3.33901135600001));
#354684=CARTESIAN_POINT('Ctrl Pts',(3.22782966599994,12.2,-3.33967065300001));
#354685=CARTESIAN_POINT('Ctrl Pts',(3.22782966599994,5.2,-3.33967065300001));
#354686=CARTESIAN_POINT('Ctrl Pts',(3.22782966599994,2.2,-3.33967065300001));
#354687=CARTESIAN_POINT('Ctrl Pts',(3.23024268399994,12.2,-3.34032834000002));
#354688=CARTESIAN_POINT('Ctrl Pts',(3.23024268399994,5.2,-3.34032834000002));
#354689=CARTESIAN_POINT('Ctrl Pts',(3.23024268399994,2.2,-3.34032834000002));
#354690=CARTESIAN_POINT('Ctrl Pts',(3.23265979899995,12.2,-3.34098440800001));
#354691=CARTESIAN_POINT('Ctrl Pts',(3.23265979899995,5.2,-3.34098440800001));
#354692=CARTESIAN_POINT('Ctrl Pts',(3.23265979899995,2.2,-3.34098440800001));
#354693=CARTESIAN_POINT('Ctrl Pts',(3.23508100799994,12.2,-3.34163885000001));
#354694=CARTESIAN_POINT('Ctrl Pts',(3.23508100799994,5.2,-3.34163885000001));
#354695=CARTESIAN_POINT('Ctrl Pts',(3.23508100799994,2.2,-3.34163885000001));
#354696=CARTESIAN_POINT('Ctrl Pts',(3.23750630699994,12.2,-3.34229165800001));
#354697=CARTESIAN_POINT('Ctrl Pts',(3.23750630699994,5.2,-3.34229165800001));
#354698=CARTESIAN_POINT('Ctrl Pts',(3.23750630699994,2.2,-3.34229165800001));
#354699=CARTESIAN_POINT('Ctrl Pts',(3.23993568899994,12.2,-3.34294282300001));
#354700=CARTESIAN_POINT('Ctrl Pts',(3.23993568899994,5.2,-3.34294282300001));
#354701=CARTESIAN_POINT('Ctrl Pts',(3.23993568899994,2.2,-3.34294282300001));
#354702=CARTESIAN_POINT('Ctrl Pts',(3.24236915199994,12.2,-3.34359234000001));
#354703=CARTESIAN_POINT('Ctrl Pts',(3.24236915199994,5.2,-3.34359234000001));
#354704=CARTESIAN_POINT('Ctrl Pts',(3.24236915199994,2.2,-3.34359234000001));
#354705=CARTESIAN_POINT('Ctrl Pts',(3.24480668999994,12.2,-3.34424019800001));
#354706=CARTESIAN_POINT('Ctrl Pts',(3.24480668999994,5.2,-3.34424019800001));
#354707=CARTESIAN_POINT('Ctrl Pts',(3.24480668999994,2.2,-3.34424019800001));
#354708=CARTESIAN_POINT('Ctrl Pts',(3.24724830099994,12.2,-3.34488639100002));
#354709=CARTESIAN_POINT('Ctrl Pts',(3.24724830099994,5.2,-3.34488639100002));
#354710=CARTESIAN_POINT('Ctrl Pts',(3.24724830099994,2.2,-3.34488639100002));
#354711=CARTESIAN_POINT('Ctrl Pts',(3.24969397699994,12.2,-3.34553091100001));
#354712=CARTESIAN_POINT('Ctrl Pts',(3.24969397699994,5.2,-3.34553091100001));
#354713=CARTESIAN_POINT('Ctrl Pts',(3.24969397699994,2.2,-3.34553091100001));
#354714=CARTESIAN_POINT('Ctrl Pts',(3.25214371599994,12.2,-3.34617375000001));
#354715=CARTESIAN_POINT('Ctrl Pts',(3.25214371599994,5.2,-3.34617375000001));
#354716=CARTESIAN_POINT('Ctrl Pts',(3.25214371599994,2.2,-3.34617375000001));
#354717=CARTESIAN_POINT('Ctrl Pts',(3.25459751399995,12.2,-3.34681490000001));
#354718=CARTESIAN_POINT('Ctrl Pts',(3.25459751399995,5.2,-3.34681490000001));
#354719=CARTESIAN_POINT('Ctrl Pts',(3.25459751399995,2.2,-3.34681490000001));
#354720=CARTESIAN_POINT('Ctrl Pts',(3.25705536499994,12.2,-3.34745435300002));
#354721=CARTESIAN_POINT('Ctrl Pts',(3.25705536499994,5.2,-3.34745435300002));
#354722=CARTESIAN_POINT('Ctrl Pts',(3.25705536499994,2.2,-3.34745435300002));
#354723=CARTESIAN_POINT('Ctrl Pts',(3.25951726499994,12.2,-3.34809210200001));
#354724=CARTESIAN_POINT('Ctrl Pts',(3.25951726499994,5.2,-3.34809210200001));
#354725=CARTESIAN_POINT('Ctrl Pts',(3.25951726499994,2.2,-3.34809210200001));
#354726=CARTESIAN_POINT('Ctrl Pts',(3.26198321199994,12.2,-3.34872814000001));
#354727=CARTESIAN_POINT('Ctrl Pts',(3.26198321199994,5.2,-3.34872814000001));
#354728=CARTESIAN_POINT('Ctrl Pts',(3.26198321199994,2.2,-3.34872814000001));
#354729=CARTESIAN_POINT('Ctrl Pts',(3.26445319799994,12.2,-3.34936245700002));
#354730=CARTESIAN_POINT('Ctrl Pts',(3.26445319799994,5.2,-3.34936245700002));
#354731=CARTESIAN_POINT('Ctrl Pts',(3.26445319799994,2.2,-3.34936245700002));
#354732=CARTESIAN_POINT('Ctrl Pts',(3.26692722099994,12.2,-3.34999504700002));
#354733=CARTESIAN_POINT('Ctrl Pts',(3.26692722099994,5.2,-3.34999504700002));
#354734=CARTESIAN_POINT('Ctrl Pts',(3.26692722099994,2.2,-3.34999504700002));
#354735=CARTESIAN_POINT('Ctrl Pts',(3.26940527499994,12.2,-3.35062590200002));
#354736=CARTESIAN_POINT('Ctrl Pts',(3.26940527499994,5.2,-3.35062590200002));
#354737=CARTESIAN_POINT('Ctrl Pts',(3.26940527499994,2.2,-3.35062590200002));
#354738=CARTESIAN_POINT('Ctrl Pts',(3.27188735699994,12.2,-3.35125501400002));
#354739=CARTESIAN_POINT('Ctrl Pts',(3.27188735699994,5.2,-3.35125501400002));
#354740=CARTESIAN_POINT('Ctrl Pts',(3.27188735699994,2.2,-3.35125501400002));
#354741=CARTESIAN_POINT('Ctrl Pts',(3.27437345999994,12.2,-3.35188237600001));
#354742=CARTESIAN_POINT('Ctrl Pts',(3.27437345999994,5.2,-3.35188237600001));
#354743=CARTESIAN_POINT('Ctrl Pts',(3.27437345999994,2.2,-3.35188237600001));
#354744=CARTESIAN_POINT('Ctrl Pts',(3.27686358299994,12.2,-3.35250797900001));
#354745=CARTESIAN_POINT('Ctrl Pts',(3.27686358299994,5.2,-3.35250797900001));
#354746=CARTESIAN_POINT('Ctrl Pts',(3.27686358299994,2.2,-3.35250797900001));
#354747=CARTESIAN_POINT('Ctrl Pts',(3.27935771899994,12.2,-3.35313181700001));
#354748=CARTESIAN_POINT('Ctrl Pts',(3.27935771899994,5.2,-3.35313181700001));
#354749=CARTESIAN_POINT('Ctrl Pts',(3.27935771899994,2.2,-3.35313181700001));
#354750=CARTESIAN_POINT('Ctrl Pts',(3.28185586499994,12.2,-3.35375388100001));
#354751=CARTESIAN_POINT('Ctrl Pts',(3.28185586499994,5.2,-3.35375388100001));
#354752=CARTESIAN_POINT('Ctrl Pts',(3.28185586499994,2.2,-3.35375388100001));
#354753=CARTESIAN_POINT('Ctrl Pts',(3.28435801599994,12.2,-3.35437416500001));
#354754=CARTESIAN_POINT('Ctrl Pts',(3.28435801599994,5.2,-3.35437416500001));
#354755=CARTESIAN_POINT('Ctrl Pts',(3.28435801599994,2.2,-3.35437416500001));
#354756=CARTESIAN_POINT('Ctrl Pts',(3.28686416799994,12.2,-3.35499266000001));
#354757=CARTESIAN_POINT('Ctrl Pts',(3.28686416799994,5.2,-3.35499266000001));
#354758=CARTESIAN_POINT('Ctrl Pts',(3.28686416799994,2.2,-3.35499266000001));
#354759=CARTESIAN_POINT('Ctrl Pts',(3.28937431499994,12.2,-3.35560936000002));
#354760=CARTESIAN_POINT('Ctrl Pts',(3.28937431499994,5.2,-3.35560936000002));
#354761=CARTESIAN_POINT('Ctrl Pts',(3.28937431499994,2.2,-3.35560936000002));
#354762=CARTESIAN_POINT('Ctrl Pts',(3.29188845499994,12.2,-3.35622425600001));
#354763=CARTESIAN_POINT('Ctrl Pts',(3.29188845499994,5.2,-3.35622425600001));
#354764=CARTESIAN_POINT('Ctrl Pts',(3.29188845499994,2.2,-3.35622425600001));
#354765=CARTESIAN_POINT('Ctrl Pts',(3.29440658299994,12.2,-3.35683734200002));
#354766=CARTESIAN_POINT('Ctrl Pts',(3.29440658299994,5.2,-3.35683734200002));
#354767=CARTESIAN_POINT('Ctrl Pts',(3.29440658299994,2.2,-3.35683734200002));
#354768=CARTESIAN_POINT('Ctrl Pts',(3.29692869199994,12.2,-3.35744860900002));
#354769=CARTESIAN_POINT('Ctrl Pts',(3.29692869199994,5.2,-3.35744860900002));
#354770=CARTESIAN_POINT('Ctrl Pts',(3.29692869199994,2.2,-3.35744860900002));
#354771=CARTESIAN_POINT('Ctrl Pts',(3.29945477899994,12.2,-3.35805805000001));
#354772=CARTESIAN_POINT('Ctrl Pts',(3.29945477899994,5.2,-3.35805805000001));
#354773=CARTESIAN_POINT('Ctrl Pts',(3.29945477899994,2.2,-3.35805805000001));
#354774=CARTESIAN_POINT('Ctrl Pts',(3.30198483999995,12.2,-3.35866565600002));
#354775=CARTESIAN_POINT('Ctrl Pts',(3.30198483999995,5.2,-3.35866565600002));
#354776=CARTESIAN_POINT('Ctrl Pts',(3.30198483999995,2.2,-3.35866565600002));
#354777=CARTESIAN_POINT('Ctrl Pts',(3.30451886899994,12.2,-3.35927142000001));
#354778=CARTESIAN_POINT('Ctrl Pts',(3.30451886899994,5.2,-3.35927142000001));
#354779=CARTESIAN_POINT('Ctrl Pts',(3.30451886899994,2.2,-3.35927142000001));
#354780=CARTESIAN_POINT('Ctrl Pts',(3.30705686199994,12.2,-3.35987533600001));
#354781=CARTESIAN_POINT('Ctrl Pts',(3.30705686199994,5.2,-3.35987533600001));
#354782=CARTESIAN_POINT('Ctrl Pts',(3.30705686199994,2.2,-3.35987533600001));
#354783=CARTESIAN_POINT('Ctrl Pts',(3.30959881599994,12.2,-3.36047739500001));
#354784=CARTESIAN_POINT('Ctrl Pts',(3.30959881599994,5.2,-3.36047739500001));
#354785=CARTESIAN_POINT('Ctrl Pts',(3.30959881599994,2.2,-3.36047739500001));
#354786=CARTESIAN_POINT('Ctrl Pts',(3.31214472499994,12.2,-3.36107759100001));
#354787=CARTESIAN_POINT('Ctrl Pts',(3.31214472499994,5.2,-3.36107759100001));
#354788=CARTESIAN_POINT('Ctrl Pts',(3.31214472499994,2.2,-3.36107759100001));
#354789=CARTESIAN_POINT('Ctrl Pts',(3.31469458699994,12.2,-3.36167591800002));
#354790=CARTESIAN_POINT('Ctrl Pts',(3.31469458699994,5.2,-3.36167591800002));
#354791=CARTESIAN_POINT('Ctrl Pts',(3.31469458699994,2.2,-3.36167591800002));
#354792=CARTESIAN_POINT('Ctrl Pts',(3.31724839599994,12.2,-3.36227237000001));
#354793=CARTESIAN_POINT('Ctrl Pts',(3.31724839599994,5.2,-3.36227237000001));
#354794=CARTESIAN_POINT('Ctrl Pts',(3.31724839599994,2.2,-3.36227237000001));
#354795=CARTESIAN_POINT('Ctrl Pts',(3.31980614799994,12.2,-3.36286693800002));
#354796=CARTESIAN_POINT('Ctrl Pts',(3.31980614799994,5.2,-3.36286693800002));
#354797=CARTESIAN_POINT('Ctrl Pts',(3.31980614799994,2.2,-3.36286693800002));
#354798=CARTESIAN_POINT('Ctrl Pts',(3.32236783799994,12.2,-3.36345961400002));
#354799=CARTESIAN_POINT('Ctrl Pts',(3.32236783799994,5.2,-3.36345961400002));
#354800=CARTESIAN_POINT('Ctrl Pts',(3.32236783799994,2.2,-3.36345961400002));
#354801=CARTESIAN_POINT('Ctrl Pts',(3.32493346199994,12.2,-3.36405038900002));
#354802=CARTESIAN_POINT('Ctrl Pts',(3.32493346199994,5.2,-3.36405038900002));
#354803=CARTESIAN_POINT('Ctrl Pts',(3.32493346199994,2.2,-3.36405038900002));
#354804=CARTESIAN_POINT('Ctrl Pts',(3.32750301199995,12.2,-3.36463925400002));
#354805=CARTESIAN_POINT('Ctrl Pts',(3.32750301199995,5.2,-3.36463925400002));
#354806=CARTESIAN_POINT('Ctrl Pts',(3.32750301199995,2.2,-3.36463925400002));
#354807=CARTESIAN_POINT('Ctrl Pts',(3.33007648399994,12.2,-3.36522620100002));
#354808=CARTESIAN_POINT('Ctrl Pts',(3.33007648399994,5.2,-3.36522620100002));
#354809=CARTESIAN_POINT('Ctrl Pts',(3.33007648399994,2.2,-3.36522620100002));
#354810=CARTESIAN_POINT('Ctrl Pts',(3.33265387199994,12.2,-3.36581122000001));
#354811=CARTESIAN_POINT('Ctrl Pts',(3.33265387199994,5.2,-3.36581122000001));
#354812=CARTESIAN_POINT('Ctrl Pts',(3.33265387199994,2.2,-3.36581122000001));
#354813=CARTESIAN_POINT('Ctrl Pts',(3.33523517199994,12.2,-3.36639430500002));
#354814=CARTESIAN_POINT('Ctrl Pts',(3.33523517199994,5.2,-3.36639430500002));
#354815=CARTESIAN_POINT('Ctrl Pts',(3.33523517199994,2.2,-3.36639430500002));
#354816=CARTESIAN_POINT('Ctrl Pts',(3.33782038099995,12.2,-3.36697545100002));
#354817=CARTESIAN_POINT('Ctrl Pts',(3.33782038099995,5.2,-3.36697545100002));
#354818=CARTESIAN_POINT('Ctrl Pts',(3.33782038099995,2.2,-3.36697545100002));
#354819=CARTESIAN_POINT('Ctrl Pts',(3.34040949499995,12.2,-3.36755465400001));
#354820=CARTESIAN_POINT('Ctrl Pts',(3.34040949499995,5.2,-3.36755465400001));
#354821=CARTESIAN_POINT('Ctrl Pts',(3.34040949499995,2.2,-3.36755465400001));
#354822=CARTESIAN_POINT('Ctrl Pts',(3.34300251499994,12.2,-3.36813191300001));
#354823=CARTESIAN_POINT('Ctrl Pts',(3.34300251499994,5.2,-3.36813191300001));
#354824=CARTESIAN_POINT('Ctrl Pts',(3.34300251499994,2.2,-3.36813191300001));
#354825=CARTESIAN_POINT('Ctrl Pts',(3.34508005499994,12.2,-3.36859216300001));
#354826=CARTESIAN_POINT('Ctrl Pts',(3.34508005499994,5.2,-3.36859216300001));
#354827=CARTESIAN_POINT('Ctrl Pts',(3.34508005499994,2.2,-3.36859216300001));
#354828=CARTESIAN_POINT('Ctrl Pts',(3.34663996599994,12.2,-3.36893647500002));
#354829=CARTESIAN_POINT('Ctrl Pts',(3.34663996599994,5.2,-3.36893647500002));
#354830=CARTESIAN_POINT('Ctrl Pts',(3.34663996599994,2.2,-3.36893647500002));
#354831=CARTESIAN_POINT('Ctrl Pts',(3.34768068699994,12.2,-3.36916562700001));
#354832=CARTESIAN_POINT('Ctrl Pts',(3.34768068699994,5.2,-3.36916562700001));
#354833=CARTESIAN_POINT('Ctrl Pts',(3.34768068699994,2.2,-3.36916562700001));
#354834=CARTESIAN_POINT('Ctrl Pts',(3.34820124399994,12.2,-3.36928010500001));
#354835=CARTESIAN_POINT('Ctrl Pts',(3.34820124399994,5.2,-3.36928010500001));
#354836=CARTESIAN_POINT('Ctrl Pts',(3.34820124399994,2.2,-3.36928010500001));
#354837=CARTESIAN_POINT('',(2.60456064899994,12.2,-3.02756105800002));
#354838=CARTESIAN_POINT('Origin',(-5.66300478732629E-14,15.2,-1.77635683940025E-14));
#354839=CARTESIAN_POINT('',(2.36409006999994,12.2,-2.74803623300001));
#354840=CARTESIAN_POINT('Origin',(-5.66300478732629E-14,15.2,-1.77635683940025E-14));
#354841=CARTESIAN_POINT('Origin',(-5.66300478732629E-14,15.2,-1.77635683940025E-14));
#354842=CARTESIAN_POINT('',(1.91153447899994,2.2,-3.08004235900002));
#354843=CARTESIAN_POINT('Origin',(-5.66300478732629E-14,15.2,-1.77635683940025E-14));
#354844=CARTESIAN_POINT('',(1.33499927399995,12.2,-3.76399243800002));
#354845=CARTESIAN_POINT('',(1.21174314999994,12.2,-3.41647530900001));
#354846=CARTESIAN_POINT('Origin',(2.10595395499994,15.2,-3.39330912400001));
#354847=CARTESIAN_POINT('',(2.10598101599994,12.2,-3.39335272700001));
#354848=CARTESIAN_POINT('Ctrl Pts',(2.20867500599994,12.2,-4.20526511900002));
#354849=CARTESIAN_POINT('Ctrl Pts',(2.20867500599994,5.2,-4.20526511900002));
#354850=CARTESIAN_POINT('Ctrl Pts',(2.20867500599994,2.2,-4.20526511900002));
#354851=CARTESIAN_POINT('Ctrl Pts',(2.20872208699994,12.2,-4.20473420700001));
#354852=CARTESIAN_POINT('Ctrl Pts',(2.20872208699994,5.2,-4.20473420700001));
#354853=CARTESIAN_POINT('Ctrl Pts',(2.20872208699994,2.2,-4.20473420700001));
#354854=CARTESIAN_POINT('Ctrl Pts',(2.20881594599994,12.2,-4.20367269700002));
#354855=CARTESIAN_POINT('Ctrl Pts',(2.20881594599994,5.2,-4.20367269700002));
#354856=CARTESIAN_POINT('Ctrl Pts',(2.20881594599994,2.2,-4.20367269700002));
#354857=CARTESIAN_POINT('Ctrl Pts',(2.20895582799994,12.2,-4.20208137500001));
#354858=CARTESIAN_POINT('Ctrl Pts',(2.20895582799994,5.2,-4.20208137500001));
#354859=CARTESIAN_POINT('Ctrl Pts',(2.20895582799994,2.2,-4.20208137500001));
#354860=CARTESIAN_POINT('Ctrl Pts',(2.20914051899994,12.2,-4.19996149500002));
#354861=CARTESIAN_POINT('Ctrl Pts',(2.20914051899994,5.2,-4.19996149500002));
#354862=CARTESIAN_POINT('Ctrl Pts',(2.20914051899994,2.2,-4.19996149500002));
#354863=CARTESIAN_POINT('Ctrl Pts',(2.20936835599994,12.2,-4.19731478600001));
#354864=CARTESIAN_POINT('Ctrl Pts',(2.20936835599994,5.2,-4.19731478600001));
#354865=CARTESIAN_POINT('Ctrl Pts',(2.20936835599994,2.2,-4.19731478600001));
#354866=CARTESIAN_POINT('Ctrl Pts',(2.20959316499994,12.2,-4.19467121700002));
#354867=CARTESIAN_POINT('Ctrl Pts',(2.20959316499994,5.2,-4.19467121700002));
#354868=CARTESIAN_POINT('Ctrl Pts',(2.20959316499994,2.2,-4.19467121700002));
#354869=CARTESIAN_POINT('Ctrl Pts',(2.20981494699994,12.2,-4.19203079200001));
#354870=CARTESIAN_POINT('Ctrl Pts',(2.20981494699994,5.2,-4.19203079200001));
#354871=CARTESIAN_POINT('Ctrl Pts',(2.20981494699994,2.2,-4.19203079200001));
#354872=CARTESIAN_POINT('Ctrl Pts',(2.21003370799994,12.2,-4.18939351300001));
#354873=CARTESIAN_POINT('Ctrl Pts',(2.21003370799994,5.2,-4.18939351300001));
#354874=CARTESIAN_POINT('Ctrl Pts',(2.21003370799994,2.2,-4.18939351300001));
#354875=CARTESIAN_POINT('Ctrl Pts',(2.21024944899994,12.2,-4.18675938500002));
#354876=CARTESIAN_POINT('Ctrl Pts',(2.21024944899994,5.2,-4.18675938500002));
#354877=CARTESIAN_POINT('Ctrl Pts',(2.21024944899994,2.2,-4.18675938500002));
#354878=CARTESIAN_POINT('Ctrl Pts',(2.21046217399994,12.2,-4.18412841400002));
#354879=CARTESIAN_POINT('Ctrl Pts',(2.21046217399994,5.2,-4.18412841400002));
#354880=CARTESIAN_POINT('Ctrl Pts',(2.21046217399994,2.2,-4.18412841400002));
#354881=CARTESIAN_POINT('Ctrl Pts',(2.21067189399994,12.2,-4.18150060600002));
#354882=CARTESIAN_POINT('Ctrl Pts',(2.21067189399994,5.2,-4.18150060600002));
#354883=CARTESIAN_POINT('Ctrl Pts',(2.21067189399994,2.2,-4.18150060600002));
#354884=CARTESIAN_POINT('Ctrl Pts',(2.21087861199994,12.2,-4.17887597200002));
#354885=CARTESIAN_POINT('Ctrl Pts',(2.21087861199994,5.2,-4.17887597200002));
#354886=CARTESIAN_POINT('Ctrl Pts',(2.21087861199994,2.2,-4.17887597200002));
#354887=CARTESIAN_POINT('Ctrl Pts',(2.21108233599994,12.2,-4.17625451800001));
#354888=CARTESIAN_POINT('Ctrl Pts',(2.21108233599994,5.2,-4.17625451800001));
#354889=CARTESIAN_POINT('Ctrl Pts',(2.21108233599994,2.2,-4.17625451800001));
#354890=CARTESIAN_POINT('Ctrl Pts',(2.21128307299994,12.2,-4.17363625300001));
#354891=CARTESIAN_POINT('Ctrl Pts',(2.21128307299994,5.2,-4.17363625300001));
#354892=CARTESIAN_POINT('Ctrl Pts',(2.21128307299994,2.2,-4.17363625300001));
#354893=CARTESIAN_POINT('Ctrl Pts',(2.21148083099994,12.2,-4.17102118400001));
#354894=CARTESIAN_POINT('Ctrl Pts',(2.21148083099994,5.2,-4.17102118400001));
#354895=CARTESIAN_POINT('Ctrl Pts',(2.21148083099994,2.2,-4.17102118400001));
#354896=CARTESIAN_POINT('Ctrl Pts',(2.21167561299994,12.2,-4.16840931700001));
#354897=CARTESIAN_POINT('Ctrl Pts',(2.21167561299994,5.2,-4.16840931700001));
#354898=CARTESIAN_POINT('Ctrl Pts',(2.21167561299994,2.2,-4.16840931700001));
#354899=CARTESIAN_POINT('Ctrl Pts',(2.21186742599994,12.2,-4.16580065900002));
#354900=CARTESIAN_POINT('Ctrl Pts',(2.21186742599994,5.2,-4.16580065900002));
#354901=CARTESIAN_POINT('Ctrl Pts',(2.21186742599994,2.2,-4.16580065900002));
#354902=CARTESIAN_POINT('Ctrl Pts',(2.21205627499994,12.2,-4.16319521500002));
#354903=CARTESIAN_POINT('Ctrl Pts',(2.21205627499994,5.2,-4.16319521500002));
#354904=CARTESIAN_POINT('Ctrl Pts',(2.21205627499994,2.2,-4.16319521500002));
#354905=CARTESIAN_POINT('Ctrl Pts',(2.21224216399994,12.2,-4.16059299100001));
#354906=CARTESIAN_POINT('Ctrl Pts',(2.21224216399994,5.2,-4.16059299100001));
#354907=CARTESIAN_POINT('Ctrl Pts',(2.21224216399994,2.2,-4.16059299100001));
#354908=CARTESIAN_POINT('Ctrl Pts',(2.21242509999994,12.2,-4.15799399300001));
#354909=CARTESIAN_POINT('Ctrl Pts',(2.21242509999994,5.2,-4.15799399300001));
#354910=CARTESIAN_POINT('Ctrl Pts',(2.21242509999994,2.2,-4.15799399300001));
#354911=CARTESIAN_POINT('Ctrl Pts',(2.21260508699994,12.2,-4.15539822800001));
#354912=CARTESIAN_POINT('Ctrl Pts',(2.21260508699994,5.2,-4.15539822800001));
#354913=CARTESIAN_POINT('Ctrl Pts',(2.21260508699994,2.2,-4.15539822800001));
#354914=CARTESIAN_POINT('Ctrl Pts',(2.21278213099994,12.2,-4.15280570200002));
#354915=CARTESIAN_POINT('Ctrl Pts',(2.21278213099994,5.2,-4.15280570200002));
#354916=CARTESIAN_POINT('Ctrl Pts',(2.21278213099994,2.2,-4.15280570200002));
#354917=CARTESIAN_POINT('Ctrl Pts',(2.21295623999994,12.2,-4.15021642300001));
#354918=CARTESIAN_POINT('Ctrl Pts',(2.21295623999994,5.2,-4.15021642300001));
#354919=CARTESIAN_POINT('Ctrl Pts',(2.21295623999994,2.2,-4.15021642300001));
#354920=CARTESIAN_POINT('Ctrl Pts',(2.21312741799994,12.2,-4.14763039500002));
#354921=CARTESIAN_POINT('Ctrl Pts',(2.21312741799994,5.2,-4.14763039500002));
#354922=CARTESIAN_POINT('Ctrl Pts',(2.21312741799994,2.2,-4.14763039500002));
#354923=CARTESIAN_POINT('Ctrl Pts',(2.21329566999994,12.2,-4.14504762800001));
#354924=CARTESIAN_POINT('Ctrl Pts',(2.21329566999994,5.2,-4.14504762800001));
#354925=CARTESIAN_POINT('Ctrl Pts',(2.21329566999994,2.2,-4.14504762800001));
#354926=CARTESIAN_POINT('Ctrl Pts',(2.21346100499995,12.2,-4.14246812800001));
#354927=CARTESIAN_POINT('Ctrl Pts',(2.21346100499995,5.2,-4.14246812800001));
#354928=CARTESIAN_POINT('Ctrl Pts',(2.21346100499995,2.2,-4.14246812800001));
#354929=CARTESIAN_POINT('Ctrl Pts',(2.21362342699994,12.2,-4.13989189900001));
#354930=CARTESIAN_POINT('Ctrl Pts',(2.21362342699994,5.2,-4.13989189900001));
#354931=CARTESIAN_POINT('Ctrl Pts',(2.21362342699994,2.2,-4.13989189900001));
#354932=CARTESIAN_POINT('Ctrl Pts',(2.21378294299994,12.2,-4.13731895000002));
#354933=CARTESIAN_POINT('Ctrl Pts',(2.21378294299994,5.2,-4.13731895000002));
#354934=CARTESIAN_POINT('Ctrl Pts',(2.21378294299994,2.2,-4.13731895000002));
#354935=CARTESIAN_POINT('Ctrl Pts',(2.21393955699994,12.2,-4.13474928700001));
#354936=CARTESIAN_POINT('Ctrl Pts',(2.21393955699994,5.2,-4.13474928700001));
#354937=CARTESIAN_POINT('Ctrl Pts',(2.21393955699994,2.2,-4.13474928700001));
#354938=CARTESIAN_POINT('Ctrl Pts',(2.21409327699994,12.2,-4.13218291600002));
#354939=CARTESIAN_POINT('Ctrl Pts',(2.21409327699994,5.2,-4.13218291600002));
#354940=CARTESIAN_POINT('Ctrl Pts',(2.21409327699994,2.2,-4.13218291600002));
#354941=CARTESIAN_POINT('Ctrl Pts',(2.21424410699994,12.2,-4.12961984400001));
#354942=CARTESIAN_POINT('Ctrl Pts',(2.21424410699994,5.2,-4.12961984400001));
#354943=CARTESIAN_POINT('Ctrl Pts',(2.21424410699994,2.2,-4.12961984400001));
#354944=CARTESIAN_POINT('Ctrl Pts',(2.21439205399994,12.2,-4.12706007600002));
#354945=CARTESIAN_POINT('Ctrl Pts',(2.21439205399994,5.2,-4.12706007600002));
#354946=CARTESIAN_POINT('Ctrl Pts',(2.21439205399994,2.2,-4.12706007600002));
#354947=CARTESIAN_POINT('Ctrl Pts',(2.21453712299994,12.2,-4.12450362100001));
#354948=CARTESIAN_POINT('Ctrl Pts',(2.21453712299994,5.2,-4.12450362100001));
#354949=CARTESIAN_POINT('Ctrl Pts',(2.21453712299994,2.2,-4.12450362100001));
#354950=CARTESIAN_POINT('Ctrl Pts',(2.21467932099995,12.2,-4.12195048400001));
#354951=CARTESIAN_POINT('Ctrl Pts',(2.21467932099995,5.2,-4.12195048400001));
#354952=CARTESIAN_POINT('Ctrl Pts',(2.21467932099995,2.2,-4.12195048400001));
#354953=CARTESIAN_POINT('Ctrl Pts',(2.21481865199994,12.2,-4.11940067100002));
#354954=CARTESIAN_POINT('Ctrl Pts',(2.21481865199994,5.2,-4.11940067100002));
#354955=CARTESIAN_POINT('Ctrl Pts',(2.21481865199994,2.2,-4.11940067100002));
#354956=CARTESIAN_POINT('Ctrl Pts',(2.21495512599994,12.2,-4.11685419000001));
#354957=CARTESIAN_POINT('Ctrl Pts',(2.21495512599994,5.2,-4.11685419000001));
#354958=CARTESIAN_POINT('Ctrl Pts',(2.21495512599994,2.2,-4.11685419000001));
#354959=CARTESIAN_POINT('Ctrl Pts',(2.21508874499994,12.2,-4.11431104600001));
#354960=CARTESIAN_POINT('Ctrl Pts',(2.21508874499994,5.2,-4.11431104600001));
#354961=CARTESIAN_POINT('Ctrl Pts',(2.21508874499994,2.2,-4.11431104600001));
#354962=CARTESIAN_POINT('Ctrl Pts',(2.21521951699994,12.2,-4.11177124700002));
#354963=CARTESIAN_POINT('Ctrl Pts',(2.21521951699994,5.2,-4.11177124700002));
#354964=CARTESIAN_POINT('Ctrl Pts',(2.21521951699994,2.2,-4.11177124700002));
#354965=CARTESIAN_POINT('Ctrl Pts',(2.21534744799994,12.2,-4.10923479900001));
#354966=CARTESIAN_POINT('Ctrl Pts',(2.21534744799994,5.2,-4.10923479900001));
#354967=CARTESIAN_POINT('Ctrl Pts',(2.21534744799994,2.2,-4.10923479900001));
#354968=CARTESIAN_POINT('Ctrl Pts',(2.21547254299994,12.2,-4.10670170900001));
#354969=CARTESIAN_POINT('Ctrl Pts',(2.21547254299994,5.2,-4.10670170900001));
#354970=CARTESIAN_POINT('Ctrl Pts',(2.21547254299994,2.2,-4.10670170900001));
#354971=CARTESIAN_POINT('Ctrl Pts',(2.21559480899994,12.2,-4.10417198300001));
#354972=CARTESIAN_POINT('Ctrl Pts',(2.21559480899994,5.2,-4.10417198300001));
#354973=CARTESIAN_POINT('Ctrl Pts',(2.21559480899994,2.2,-4.10417198300001));
#354974=CARTESIAN_POINT('Ctrl Pts',(2.21571425199994,12.2,-4.10164562700002));
#354975=CARTESIAN_POINT('Ctrl Pts',(2.21571425199994,5.2,-4.10164562700002));
#354976=CARTESIAN_POINT('Ctrl Pts',(2.21571425199994,2.2,-4.10164562700002));
#354977=CARTESIAN_POINT('Ctrl Pts',(2.21583087799994,12.2,-4.09912264800001));
#354978=CARTESIAN_POINT('Ctrl Pts',(2.21583087799994,5.2,-4.09912264800001));
#354979=CARTESIAN_POINT('Ctrl Pts',(2.21583087799994,2.2,-4.09912264800001));
#354980=CARTESIAN_POINT('Ctrl Pts',(2.21594469199994,12.2,-4.09660305300001));
#354981=CARTESIAN_POINT('Ctrl Pts',(2.21594469199994,5.2,-4.09660305300001));
#354982=CARTESIAN_POINT('Ctrl Pts',(2.21594469199994,2.2,-4.09660305300001));
#354983=CARTESIAN_POINT('Ctrl Pts',(2.21605570199995,12.2,-4.09408684800002));
#354984=CARTESIAN_POINT('Ctrl Pts',(2.21605570199995,5.2,-4.09408684800002));
#354985=CARTESIAN_POINT('Ctrl Pts',(2.21605570199995,2.2,-4.09408684800002));
#354986=CARTESIAN_POINT('Ctrl Pts',(2.21616391399994,12.2,-4.09157403900001));
#354987=CARTESIAN_POINT('Ctrl Pts',(2.21616391399994,5.2,-4.09157403900001));
#354988=CARTESIAN_POINT('Ctrl Pts',(2.21616391399994,2.2,-4.09157403900001));
#354989=CARTESIAN_POINT('Ctrl Pts',(2.21626933299994,12.2,-4.08906463400001));
#354990=CARTESIAN_POINT('Ctrl Pts',(2.21626933299994,5.2,-4.08906463400001));
#354991=CARTESIAN_POINT('Ctrl Pts',(2.21626933299994,2.2,-4.08906463400001));
#354992=CARTESIAN_POINT('Ctrl Pts',(2.21637196599994,12.2,-4.08655863900002));
#354993=CARTESIAN_POINT('Ctrl Pts',(2.21637196599994,5.2,-4.08655863900002));
#354994=CARTESIAN_POINT('Ctrl Pts',(2.21637196599994,2.2,-4.08655863900002));
#354995=CARTESIAN_POINT('Ctrl Pts',(2.21647181899994,12.2,-4.08405605900001));
#354996=CARTESIAN_POINT('Ctrl Pts',(2.21647181899994,5.2,-4.08405605900001));
#354997=CARTESIAN_POINT('Ctrl Pts',(2.21647181899994,2.2,-4.08405605900001));
#354998=CARTESIAN_POINT('Ctrl Pts',(2.21656889799994,12.2,-4.08155690200001));
#354999=CARTESIAN_POINT('Ctrl Pts',(2.21656889799994,5.2,-4.08155690200001));
#355000=CARTESIAN_POINT('Ctrl Pts',(2.21656889799994,2.2,-4.08155690200001));
#355001=CARTESIAN_POINT('Ctrl Pts',(2.21666320899994,12.2,-4.07906117500001));
#355002=CARTESIAN_POINT('Ctrl Pts',(2.21666320899994,5.2,-4.07906117500001));
#355003=CARTESIAN_POINT('Ctrl Pts',(2.21666320899994,2.2,-4.07906117500001));
#355004=CARTESIAN_POINT('Ctrl Pts',(2.21675475899994,12.2,-4.07656888400002));
#355005=CARTESIAN_POINT('Ctrl Pts',(2.21675475899994,5.2,-4.07656888400002));
#355006=CARTESIAN_POINT('Ctrl Pts',(2.21675475899994,2.2,-4.07656888400002));
#355007=CARTESIAN_POINT('Ctrl Pts',(2.21684355399994,12.2,-4.07408003500001));
#355008=CARTESIAN_POINT('Ctrl Pts',(2.21684355399994,5.2,-4.07408003500001));
#355009=CARTESIAN_POINT('Ctrl Pts',(2.21684355399994,2.2,-4.07408003500001));
#355010=CARTESIAN_POINT('Ctrl Pts',(2.21692959999995,12.2,-4.07159463400002));
#355011=CARTESIAN_POINT('Ctrl Pts',(2.21692959999995,5.2,-4.07159463400002));
#355012=CARTESIAN_POINT('Ctrl Pts',(2.21692959999995,2.2,-4.07159463400002));
#355013=CARTESIAN_POINT('Ctrl Pts',(2.21701290399994,12.2,-4.06911268900001));
#355014=CARTESIAN_POINT('Ctrl Pts',(2.21701290399994,5.2,-4.06911268900001));
#355015=CARTESIAN_POINT('Ctrl Pts',(2.21701290399994,2.2,-4.06911268900001));
#355016=CARTESIAN_POINT('Ctrl Pts',(2.21709347199994,12.2,-4.06663420700001));
#355017=CARTESIAN_POINT('Ctrl Pts',(2.21709347199994,5.2,-4.06663420700001));
#355018=CARTESIAN_POINT('Ctrl Pts',(2.21709347199994,2.2,-4.06663420700001));
#355019=CARTESIAN_POINT('Ctrl Pts',(2.21717130999994,12.2,-4.06415919200001));
#355020=CARTESIAN_POINT('Ctrl Pts',(2.21717130999994,5.2,-4.06415919200001));
#355021=CARTESIAN_POINT('Ctrl Pts',(2.21717130999994,2.2,-4.06415919200001));
#355022=CARTESIAN_POINT('Ctrl Pts',(2.21724642399994,12.2,-4.06168765200002));
#355023=CARTESIAN_POINT('Ctrl Pts',(2.21724642399994,5.2,-4.06168765200002));
#355024=CARTESIAN_POINT('Ctrl Pts',(2.21724642399994,2.2,-4.06168765200002));
#355025=CARTESIAN_POINT('Ctrl Pts',(2.21731882199994,12.2,-4.05921959500001));
#355026=CARTESIAN_POINT('Ctrl Pts',(2.21731882199994,5.2,-4.05921959500001));
#355027=CARTESIAN_POINT('Ctrl Pts',(2.21731882199994,2.2,-4.05921959500001));
#355028=CARTESIAN_POINT('Ctrl Pts',(2.21738850899994,12.2,-4.05675502500001));
#355029=CARTESIAN_POINT('Ctrl Pts',(2.21738850899994,5.2,-4.05675502500001));
#355030=CARTESIAN_POINT('Ctrl Pts',(2.21738850899994,2.2,-4.05675502500001));
#355031=CARTESIAN_POINT('Ctrl Pts',(2.21745549199994,12.2,-4.05429394900001));
#355032=CARTESIAN_POINT('Ctrl Pts',(2.21745549199994,5.2,-4.05429394900001));
#355033=CARTESIAN_POINT('Ctrl Pts',(2.21745549199994,2.2,-4.05429394900001));
#355034=CARTESIAN_POINT('Ctrl Pts',(2.21751977599994,12.2,-4.05183637500001));
#355035=CARTESIAN_POINT('Ctrl Pts',(2.21751977599994,5.2,-4.05183637500001));
#355036=CARTESIAN_POINT('Ctrl Pts',(2.21751977599994,2.2,-4.05183637500001));
#355037=CARTESIAN_POINT('Ctrl Pts',(2.21758136999994,12.2,-4.04938230800001));
#355038=CARTESIAN_POINT('Ctrl Pts',(2.21758136999994,5.2,-4.04938230800001));
#355039=CARTESIAN_POINT('Ctrl Pts',(2.21758136999994,2.2,-4.04938230800001));
#355040=CARTESIAN_POINT('Ctrl Pts',(2.21764027799995,12.2,-4.04693175500002));
#355041=CARTESIAN_POINT('Ctrl Pts',(2.21764027799995,5.2,-4.04693175500002));
#355042=CARTESIAN_POINT('Ctrl Pts',(2.21764027799995,2.2,-4.04693175500002));
#355043=CARTESIAN_POINT('Ctrl Pts',(2.21769650799994,12.2,-4.04448472300002));
#355044=CARTESIAN_POINT('Ctrl Pts',(2.21769650799994,5.2,-4.04448472300002));
#355045=CARTESIAN_POINT('Ctrl Pts',(2.21769650799994,2.2,-4.04448472300002));
#355046=CARTESIAN_POINT('Ctrl Pts',(2.21775006599994,12.2,-4.04204121900001));
#355047=CARTESIAN_POINT('Ctrl Pts',(2.21775006599994,5.2,-4.04204121900001));
#355048=CARTESIAN_POINT('Ctrl Pts',(2.21775006599994,2.2,-4.04204121900001));
#355049=CARTESIAN_POINT('Ctrl Pts',(2.21780095899994,12.2,-4.03960124700002));
#355050=CARTESIAN_POINT('Ctrl Pts',(2.21780095899994,5.2,-4.03960124700002));
#355051=CARTESIAN_POINT('Ctrl Pts',(2.21780095899994,2.2,-4.03960124700002));
#355052=CARTESIAN_POINT('Ctrl Pts',(2.21784919199994,12.2,-4.03716481500001));
#355053=CARTESIAN_POINT('Ctrl Pts',(2.21784919199994,5.2,-4.03716481500001));
#355054=CARTESIAN_POINT('Ctrl Pts',(2.21784919199994,2.2,-4.03716481500001));
#355055=CARTESIAN_POINT('Ctrl Pts',(2.21789477399994,12.2,-4.03473193200002));
#355056=CARTESIAN_POINT('Ctrl Pts',(2.21789477399994,5.2,-4.03473193200002));
#355057=CARTESIAN_POINT('Ctrl Pts',(2.21789477399994,2.2,-4.03473193200002));
#355058=CARTESIAN_POINT('Ctrl Pts',(2.21793770999994,12.2,-4.03230260000001));
#355059=CARTESIAN_POINT('Ctrl Pts',(2.21793770999994,5.2,-4.03230260000001));
#355060=CARTESIAN_POINT('Ctrl Pts',(2.21793770999994,2.2,-4.03230260000001));
#355061=CARTESIAN_POINT('Ctrl Pts',(2.21797800499994,12.2,-4.02987682900001));
#355062=CARTESIAN_POINT('Ctrl Pts',(2.21797800499994,5.2,-4.02987682900001));
#355063=CARTESIAN_POINT('Ctrl Pts',(2.21797800499994,2.2,-4.02987682900001));
#355064=CARTESIAN_POINT('Ctrl Pts',(2.21801566999994,12.2,-4.02745462400001));
#355065=CARTESIAN_POINT('Ctrl Pts',(2.21801566999994,5.2,-4.02745462400001));
#355066=CARTESIAN_POINT('Ctrl Pts',(2.21801566999994,2.2,-4.02745462400001));
#355067=CARTESIAN_POINT('Ctrl Pts',(2.21805070699994,12.2,-4.02503599200001));
#355068=CARTESIAN_POINT('Ctrl Pts',(2.21805070699994,5.2,-4.02503599200001));
#355069=CARTESIAN_POINT('Ctrl Pts',(2.21805070699994,2.2,-4.02503599200001));
#355070=CARTESIAN_POINT('Ctrl Pts',(2.21808312599994,12.2,-4.02262093800001));
#355071=CARTESIAN_POINT('Ctrl Pts',(2.21808312599994,5.2,-4.02262093800001));
#355072=CARTESIAN_POINT('Ctrl Pts',(2.21808312599994,2.2,-4.02262093800001));
#355073=CARTESIAN_POINT('Ctrl Pts',(2.21811293099994,12.2,-4.02020947100001));
#355074=CARTESIAN_POINT('Ctrl Pts',(2.21811293099994,5.2,-4.02020947100001));
#355075=CARTESIAN_POINT('Ctrl Pts',(2.21811293099994,2.2,-4.02020947100001));
#355076=CARTESIAN_POINT('Ctrl Pts',(2.21814013099995,12.2,-4.01780159600001));
#355077=CARTESIAN_POINT('Ctrl Pts',(2.21814013099995,5.2,-4.01780159600001));
#355078=CARTESIAN_POINT('Ctrl Pts',(2.21814013099995,2.2,-4.01780159600001));
#355079=CARTESIAN_POINT('Ctrl Pts',(2.21816473099994,12.2,-4.01539731900002));
#355080=CARTESIAN_POINT('Ctrl Pts',(2.21816473099994,5.2,-4.01539731900002));
#355081=CARTESIAN_POINT('Ctrl Pts',(2.21816473099994,2.2,-4.01539731900002));
#355082=CARTESIAN_POINT('Ctrl Pts',(2.21818673899994,12.2,-4.01299664900002));
#355083=CARTESIAN_POINT('Ctrl Pts',(2.21818673899994,5.2,-4.01299664900002));
#355084=CARTESIAN_POINT('Ctrl Pts',(2.21818673899994,2.2,-4.01299664900002));
#355085=CARTESIAN_POINT('Ctrl Pts',(2.21820616099994,12.2,-4.01059959000001));
#355086=CARTESIAN_POINT('Ctrl Pts',(2.21820616099994,5.2,-4.01059959000001));
#355087=CARTESIAN_POINT('Ctrl Pts',(2.21820616099994,2.2,-4.01059959000001));
#355088=CARTESIAN_POINT('Ctrl Pts',(2.21822300299995,12.2,-4.00820614800002));
#355089=CARTESIAN_POINT('Ctrl Pts',(2.21822300299995,5.2,-4.00820614800002));
#355090=CARTESIAN_POINT('Ctrl Pts',(2.21822300299995,2.2,-4.00820614800002));
#355091=CARTESIAN_POINT('Ctrl Pts',(2.21823727299994,12.2,-4.00581633300002));
#355092=CARTESIAN_POINT('Ctrl Pts',(2.21823727299994,5.2,-4.00581633300002));
#355093=CARTESIAN_POINT('Ctrl Pts',(2.21823727299994,2.2,-4.00581633300002));
#355094=CARTESIAN_POINT('Ctrl Pts',(2.21824897699994,12.2,-4.00343014800002));
#355095=CARTESIAN_POINT('Ctrl Pts',(2.21824897699994,5.2,-4.00343014800002));
#355096=CARTESIAN_POINT('Ctrl Pts',(2.21824897699994,2.2,-4.00343014800002));
#355097=CARTESIAN_POINT('Ctrl Pts',(2.21825812299994,12.2,-4.00104760200001));
#355098=CARTESIAN_POINT('Ctrl Pts',(2.21825812299994,5.2,-4.00104760200001));
#355099=CARTESIAN_POINT('Ctrl Pts',(2.21825812299994,2.2,-4.00104760200001));
#355100=CARTESIAN_POINT('Ctrl Pts',(2.21826471699994,12.2,-3.99866870000002));
#355101=CARTESIAN_POINT('Ctrl Pts',(2.21826471699994,5.2,-3.99866870000002));
#355102=CARTESIAN_POINT('Ctrl Pts',(2.21826471699994,2.2,-3.99866870000002));
#355103=CARTESIAN_POINT('Ctrl Pts',(2.21826876399994,12.2,-3.99629344800001));
#355104=CARTESIAN_POINT('Ctrl Pts',(2.21826876399994,5.2,-3.99629344800001));
#355105=CARTESIAN_POINT('Ctrl Pts',(2.21826876399994,2.2,-3.99629344800001));
#355106=CARTESIAN_POINT('Ctrl Pts',(2.21827027499994,12.2,-3.99392185500002));
#355107=CARTESIAN_POINT('Ctrl Pts',(2.21827027499994,5.2,-3.99392185500002));
#355108=CARTESIAN_POINT('Ctrl Pts',(2.21827027499994,2.2,-3.99392185500002));
#355109=CARTESIAN_POINT('Ctrl Pts',(2.21826925299994,12.2,-3.99155392500001));
#355110=CARTESIAN_POINT('Ctrl Pts',(2.21826925299994,5.2,-3.99155392500001));
#355111=CARTESIAN_POINT('Ctrl Pts',(2.21826925299994,2.2,-3.99155392500001));
#355112=CARTESIAN_POINT('Ctrl Pts',(2.21826570699994,12.2,-3.98918966500001));
#355113=CARTESIAN_POINT('Ctrl Pts',(2.21826570699994,5.2,-3.98918966500001));
#355114=CARTESIAN_POINT('Ctrl Pts',(2.21826570699994,2.2,-3.98918966500001));
#355115=CARTESIAN_POINT('Ctrl Pts',(2.21825964399994,12.2,-3.98682908300001));
#355116=CARTESIAN_POINT('Ctrl Pts',(2.21825964399994,5.2,-3.98682908300001));
#355117=CARTESIAN_POINT('Ctrl Pts',(2.21825964399994,2.2,-3.98682908300001));
#355118=CARTESIAN_POINT('Ctrl Pts',(2.21825106799994,12.2,-3.98447218300001));
#355119=CARTESIAN_POINT('Ctrl Pts',(2.21825106799994,5.2,-3.98447218300001));
#355120=CARTESIAN_POINT('Ctrl Pts',(2.21825106799994,2.2,-3.98447218300001));
#355121=CARTESIAN_POINT('Ctrl Pts',(2.21823998999994,12.2,-3.98211897400001));
#355122=CARTESIAN_POINT('Ctrl Pts',(2.21823998999994,5.2,-3.98211897400001));
#355123=CARTESIAN_POINT('Ctrl Pts',(2.21823998999994,2.2,-3.98211897400001));
#355124=CARTESIAN_POINT('Ctrl Pts',(2.21822641399994,12.2,-3.97976946200002));
#355125=CARTESIAN_POINT('Ctrl Pts',(2.21822641399994,5.2,-3.97976946200002));
#355126=CARTESIAN_POINT('Ctrl Pts',(2.21822641399994,2.2,-3.97976946200002));
#355127=CARTESIAN_POINT('Ctrl Pts',(2.21821034899994,12.2,-3.97742365200001));
#355128=CARTESIAN_POINT('Ctrl Pts',(2.21821034899994,5.2,-3.97742365200001));
#355129=CARTESIAN_POINT('Ctrl Pts',(2.21821034899994,2.2,-3.97742365200001));
#355130=CARTESIAN_POINT('Ctrl Pts',(2.21819180099994,12.2,-3.97508155100001));
#355131=CARTESIAN_POINT('Ctrl Pts',(2.21819180099994,5.2,-3.97508155100001));
#355132=CARTESIAN_POINT('Ctrl Pts',(2.21819180099994,2.2,-3.97508155100001));
#355133=CARTESIAN_POINT('Ctrl Pts',(2.21817077599994,12.2,-3.97274316600001));
#355134=CARTESIAN_POINT('Ctrl Pts',(2.21817077599994,5.2,-3.97274316600001));
#355135=CARTESIAN_POINT('Ctrl Pts',(2.21817077599994,2.2,-3.97274316600001));
#355136=CARTESIAN_POINT('Ctrl Pts',(2.21814728299994,12.2,-3.97040850500002));
#355137=CARTESIAN_POINT('Ctrl Pts',(2.21814728299994,5.2,-3.97040850500002));
#355138=CARTESIAN_POINT('Ctrl Pts',(2.21814728299994,2.2,-3.97040850500002));
#355139=CARTESIAN_POINT('Ctrl Pts',(2.21812132799994,12.2,-3.96807757200001));
#355140=CARTESIAN_POINT('Ctrl Pts',(2.21812132799994,5.2,-3.96807757200001));
#355141=CARTESIAN_POINT('Ctrl Pts',(2.21812132799994,2.2,-3.96807757200001));
#355142=CARTESIAN_POINT('Ctrl Pts',(2.21809291799994,12.2,-3.96575037400002));
#355143=CARTESIAN_POINT('Ctrl Pts',(2.21809291799994,5.2,-3.96575037400002));
#355144=CARTESIAN_POINT('Ctrl Pts',(2.21809291799994,2.2,-3.96575037400002));
#355145=CARTESIAN_POINT('Ctrl Pts',(2.21806205999994,12.2,-3.96342691800001));
#355146=CARTESIAN_POINT('Ctrl Pts',(2.21806205999994,5.2,-3.96342691800001));
#355147=CARTESIAN_POINT('Ctrl Pts',(2.21806205999994,2.2,-3.96342691800001));
#355148=CARTESIAN_POINT('Ctrl Pts',(2.21802876299994,12.2,-3.96110721100001));
#355149=CARTESIAN_POINT('Ctrl Pts',(2.21802876299994,5.2,-3.96110721100001));
#355150=CARTESIAN_POINT('Ctrl Pts',(2.21802876299994,2.2,-3.96110721100001));
#355151=CARTESIAN_POINT('Ctrl Pts',(2.21799303099994,12.2,-3.95879125900001));
#355152=CARTESIAN_POINT('Ctrl Pts',(2.21799303099994,5.2,-3.95879125900001));
#355153=CARTESIAN_POINT('Ctrl Pts',(2.21799303099994,2.2,-3.95879125900001));
#355154=CARTESIAN_POINT('Ctrl Pts',(2.21795487199994,12.2,-3.95647906800002));
#355155=CARTESIAN_POINT('Ctrl Pts',(2.21795487199994,5.2,-3.95647906800002));
#355156=CARTESIAN_POINT('Ctrl Pts',(2.21795487199994,2.2,-3.95647906800002));
#355157=CARTESIAN_POINT('Ctrl Pts',(2.21791429499994,12.2,-3.95417064500001));
#355158=CARTESIAN_POINT('Ctrl Pts',(2.21791429499994,5.2,-3.95417064500001));
#355159=CARTESIAN_POINT('Ctrl Pts',(2.21791429499994,2.2,-3.95417064500001));
#355160=CARTESIAN_POINT('Ctrl Pts',(2.21787130599994,12.2,-3.95186599600001));
#355161=CARTESIAN_POINT('Ctrl Pts',(2.21787130599994,5.2,-3.95186599600001));
#355162=CARTESIAN_POINT('Ctrl Pts',(2.21787130599994,2.2,-3.95186599600001));
#355163=CARTESIAN_POINT('Ctrl Pts',(2.21782591199994,12.2,-3.94956512800002));
#355164=CARTESIAN_POINT('Ctrl Pts',(2.21782591199994,5.2,-3.94956512800002));
#355165=CARTESIAN_POINT('Ctrl Pts',(2.21782591199994,2.2,-3.94956512800002));
#355166=CARTESIAN_POINT('Ctrl Pts',(2.21777812099994,12.2,-3.94726804800001));
#355167=CARTESIAN_POINT('Ctrl Pts',(2.21777812099994,5.2,-3.94726804800001));
#355168=CARTESIAN_POINT('Ctrl Pts',(2.21777812099994,2.2,-3.94726804800001));
#355169=CARTESIAN_POINT('Ctrl Pts',(2.21772793799994,12.2,-3.94497476100002));
#355170=CARTESIAN_POINT('Ctrl Pts',(2.21772793799994,5.2,-3.94497476100002));
#355171=CARTESIAN_POINT('Ctrl Pts',(2.21772793799994,2.2,-3.94497476100002));
#355172=CARTESIAN_POINT('Ctrl Pts',(2.21767537399994,12.2,-3.94268527500001));
#355173=CARTESIAN_POINT('Ctrl Pts',(2.21767537399994,5.2,-3.94268527500001));
#355174=CARTESIAN_POINT('Ctrl Pts',(2.21767537399994,2.2,-3.94268527500001));
#355175=CARTESIAN_POINT('Ctrl Pts',(2.21762043199994,12.2,-3.94039959600001));
#355176=CARTESIAN_POINT('Ctrl Pts',(2.21762043199994,5.2,-3.94039959600001));
#355177=CARTESIAN_POINT('Ctrl Pts',(2.21762043199994,2.2,-3.94039959600001));
#355178=CARTESIAN_POINT('Ctrl Pts',(2.21756312299994,12.2,-3.93811773000001));
#355179=CARTESIAN_POINT('Ctrl Pts',(2.21756312299994,5.2,-3.93811773000001));
#355180=CARTESIAN_POINT('Ctrl Pts',(2.21756312299994,2.2,-3.93811773000001));
#355181=CARTESIAN_POINT('Ctrl Pts',(2.21750345199994,12.2,-3.93583968300002));
#355182=CARTESIAN_POINT('Ctrl Pts',(2.21750345199994,5.2,-3.93583968300002));
#355183=CARTESIAN_POINT('Ctrl Pts',(2.21750345199994,2.2,-3.93583968300002));
#355184=CARTESIAN_POINT('Ctrl Pts',(2.21744142799994,12.2,-3.93356546400002));
#355185=CARTESIAN_POINT('Ctrl Pts',(2.21744142799994,5.2,-3.93356546400002));
#355186=CARTESIAN_POINT('Ctrl Pts',(2.21744142799994,2.2,-3.93356546400002));
#355187=CARTESIAN_POINT('Ctrl Pts',(2.21737705699994,12.2,-3.93129507700001));
#355188=CARTESIAN_POINT('Ctrl Pts',(2.21737705699994,5.2,-3.93129507700001));
#355189=CARTESIAN_POINT('Ctrl Pts',(2.21737705699994,2.2,-3.93129507700001));
#355190=CARTESIAN_POINT('Ctrl Pts',(2.21731034499994,12.2,-3.92902852900002));
#355191=CARTESIAN_POINT('Ctrl Pts',(2.21731034499994,5.2,-3.92902852900002));
#355192=CARTESIAN_POINT('Ctrl Pts',(2.21731034499994,2.2,-3.92902852900002));
#355193=CARTESIAN_POINT('Ctrl Pts',(2.21724130399994,12.2,-3.92676582700001));
#355194=CARTESIAN_POINT('Ctrl Pts',(2.21724130399994,5.2,-3.92676582700001));
#355195=CARTESIAN_POINT('Ctrl Pts',(2.21724130399994,2.2,-3.92676582700001));
#355196=CARTESIAN_POINT('Ctrl Pts',(2.21716993699994,12.2,-3.92450697700002));
#355197=CARTESIAN_POINT('Ctrl Pts',(2.21716993699994,5.2,-3.92450697700002));
#355198=CARTESIAN_POINT('Ctrl Pts',(2.21716993699994,2.2,-3.92450697700002));
#355199=CARTESIAN_POINT('Ctrl Pts',(2.21709625399995,12.2,-3.92225198600002));
#355200=CARTESIAN_POINT('Ctrl Pts',(2.21709625399995,5.2,-3.92225198600002));
#355201=CARTESIAN_POINT('Ctrl Pts',(2.21709625399995,2.2,-3.92225198600002));
#355202=CARTESIAN_POINT('Ctrl Pts',(2.21702025999994,12.2,-3.92000086000001));
#355203=CARTESIAN_POINT('Ctrl Pts',(2.21702025999994,5.2,-3.92000086000001));
#355204=CARTESIAN_POINT('Ctrl Pts',(2.21702025999994,2.2,-3.92000086000001));
#355205=CARTESIAN_POINT('Ctrl Pts',(2.21694196499994,12.2,-3.91775360500001));
#355206=CARTESIAN_POINT('Ctrl Pts',(2.21694196499994,5.2,-3.91775360500001));
#355207=CARTESIAN_POINT('Ctrl Pts',(2.21694196499994,2.2,-3.91775360500001));
#355208=CARTESIAN_POINT('Ctrl Pts',(2.21686137499994,12.2,-3.91551022900002));
#355209=CARTESIAN_POINT('Ctrl Pts',(2.21686137499994,5.2,-3.91551022900002));
#355210=CARTESIAN_POINT('Ctrl Pts',(2.21686137499994,2.2,-3.91551022900002));
#355211=CARTESIAN_POINT('Ctrl Pts',(2.21677849799994,12.2,-3.91327073800001));
#355212=CARTESIAN_POINT('Ctrl Pts',(2.21677849799994,5.2,-3.91327073800001));
#355213=CARTESIAN_POINT('Ctrl Pts',(2.21677849799994,2.2,-3.91327073800001));
#355214=CARTESIAN_POINT('Ctrl Pts',(2.21669334199994,12.2,-3.91103513700001));
#355215=CARTESIAN_POINT('Ctrl Pts',(2.21669334199994,5.2,-3.91103513700001));
#355216=CARTESIAN_POINT('Ctrl Pts',(2.21669334199994,2.2,-3.91103513700001));
#355217=CARTESIAN_POINT('Ctrl Pts',(2.21660591299994,12.2,-3.90880343400001));
#355218=CARTESIAN_POINT('Ctrl Pts',(2.21660591299994,5.2,-3.90880343400001));
#355219=CARTESIAN_POINT('Ctrl Pts',(2.21660591299994,2.2,-3.90880343400001));
#355220=CARTESIAN_POINT('Ctrl Pts',(2.21651622099994,12.2,-3.90657563500001));
#355221=CARTESIAN_POINT('Ctrl Pts',(2.21651622099994,5.2,-3.90657563500001));
#355222=CARTESIAN_POINT('Ctrl Pts',(2.21651622099994,2.2,-3.90657563500001));
#355223=CARTESIAN_POINT('Ctrl Pts',(2.21642427099995,12.2,-3.90435174700002));
#355224=CARTESIAN_POINT('Ctrl Pts',(2.21642427099995,5.2,-3.90435174700002));
#355225=CARTESIAN_POINT('Ctrl Pts',(2.21642427099995,2.2,-3.90435174700002));
#355226=CARTESIAN_POINT('Ctrl Pts',(2.21633007199994,12.2,-3.90213177500002));
#355227=CARTESIAN_POINT('Ctrl Pts',(2.21633007199994,5.2,-3.90213177500002));
#355228=CARTESIAN_POINT('Ctrl Pts',(2.21633007199994,2.2,-3.90213177500002));
#355229=CARTESIAN_POINT('Ctrl Pts',(2.21623363099994,12.2,-3.89991572700001));
#355230=CARTESIAN_POINT('Ctrl Pts',(2.21623363099994,5.2,-3.89991572700001));
#355231=CARTESIAN_POINT('Ctrl Pts',(2.21623363099994,2.2,-3.89991572700001));
#355232=CARTESIAN_POINT('Ctrl Pts',(2.21613495599994,12.2,-3.89770360900001));
#355233=CARTESIAN_POINT('Ctrl Pts',(2.21613495599994,5.2,-3.89770360900001));
#355234=CARTESIAN_POINT('Ctrl Pts',(2.21613495599994,2.2,-3.89770360900001));
#355235=CARTESIAN_POINT('Ctrl Pts',(2.21603405499994,12.2,-3.89549542700002));
#355236=CARTESIAN_POINT('Ctrl Pts',(2.21603405499994,5.2,-3.89549542700002));
#355237=CARTESIAN_POINT('Ctrl Pts',(2.21603405499994,2.2,-3.89549542700002));
#355238=CARTESIAN_POINT('Ctrl Pts',(2.21593093499994,12.2,-3.89329118800001));
#355239=CARTESIAN_POINT('Ctrl Pts',(2.21593093499994,5.2,-3.89329118800001));
#355240=CARTESIAN_POINT('Ctrl Pts',(2.21593093499994,2.2,-3.89329118800001));
#355241=CARTESIAN_POINT('Ctrl Pts',(2.21582560499994,12.2,-3.89109089900002));
#355242=CARTESIAN_POINT('Ctrl Pts',(2.21582560499994,5.2,-3.89109089900002));
#355243=CARTESIAN_POINT('Ctrl Pts',(2.21582560499994,2.2,-3.89109089900002));
#355244=CARTESIAN_POINT('Ctrl Pts',(2.21571806999994,12.2,-3.88889456500001));
#355245=CARTESIAN_POINT('Ctrl Pts',(2.21571806999994,5.2,-3.88889456500001));
#355246=CARTESIAN_POINT('Ctrl Pts',(2.21571806999994,2.2,-3.88889456500001));
#355247=CARTESIAN_POINT('Ctrl Pts',(2.21560834099995,12.2,-3.88670219300002));
#355248=CARTESIAN_POINT('Ctrl Pts',(2.21560834099995,5.2,-3.88670219300002));
#355249=CARTESIAN_POINT('Ctrl Pts',(2.21560834099995,2.2,-3.88670219300002));
#355250=CARTESIAN_POINT('Ctrl Pts',(2.21549642299994,12.2,-3.88451379100001));
#355251=CARTESIAN_POINT('Ctrl Pts',(2.21549642299994,5.2,-3.88451379100001));
#355252=CARTESIAN_POINT('Ctrl Pts',(2.21549642299994,2.2,-3.88451379100001));
#355253=CARTESIAN_POINT('Ctrl Pts',(2.21538232599995,12.2,-3.88232936200001));
#355254=CARTESIAN_POINT('Ctrl Pts',(2.21538232599995,5.2,-3.88232936200001));
#355255=CARTESIAN_POINT('Ctrl Pts',(2.21538232599995,2.2,-3.88232936200001));
#355256=CARTESIAN_POINT('Ctrl Pts',(2.21526605699994,12.2,-3.88014891600001));
#355257=CARTESIAN_POINT('Ctrl Pts',(2.21526605699994,5.2,-3.88014891600001));
#355258=CARTESIAN_POINT('Ctrl Pts',(2.21526605699994,2.2,-3.88014891600001));
#355259=CARTESIAN_POINT('Ctrl Pts',(2.21514762299994,12.2,-3.87797245700002));
#355260=CARTESIAN_POINT('Ctrl Pts',(2.21514762299994,5.2,-3.87797245700002));
#355261=CARTESIAN_POINT('Ctrl Pts',(2.21514762299994,2.2,-3.87797245700002));
#355262=CARTESIAN_POINT('Ctrl Pts',(2.21502703299994,12.2,-3.87579999400002));
#355263=CARTESIAN_POINT('Ctrl Pts',(2.21502703299994,5.2,-3.87579999400002));
#355264=CARTESIAN_POINT('Ctrl Pts',(2.21502703299994,2.2,-3.87579999400002));
#355265=CARTESIAN_POINT('Ctrl Pts',(2.21490429399994,12.2,-3.87363153100001));
#355266=CARTESIAN_POINT('Ctrl Pts',(2.21490429399994,5.2,-3.87363153100001));
#355267=CARTESIAN_POINT('Ctrl Pts',(2.21490429399994,2.2,-3.87363153100001));
#355268=CARTESIAN_POINT('Ctrl Pts',(2.21477941399994,12.2,-3.87146707600001));
#355269=CARTESIAN_POINT('Ctrl Pts',(2.21477941399994,5.2,-3.87146707600001));
#355270=CARTESIAN_POINT('Ctrl Pts',(2.21477941399994,2.2,-3.87146707600001));
#355271=CARTESIAN_POINT('Ctrl Pts',(2.21465240199994,12.2,-3.86930663400001));
#355272=CARTESIAN_POINT('Ctrl Pts',(2.21465240199994,5.2,-3.86930663400001));
#355273=CARTESIAN_POINT('Ctrl Pts',(2.21465240199994,2.2,-3.86930663400001));
#355274=CARTESIAN_POINT('Ctrl Pts',(2.21452326299994,12.2,-3.86715021300001));
#355275=CARTESIAN_POINT('Ctrl Pts',(2.21452326299994,5.2,-3.86715021300001));
#355276=CARTESIAN_POINT('Ctrl Pts',(2.21452326299994,2.2,-3.86715021300001));
#355277=CARTESIAN_POINT('Ctrl Pts',(2.21439200899994,12.2,-3.86499781800001));
#355278=CARTESIAN_POINT('Ctrl Pts',(2.21439200899994,5.2,-3.86499781800001));
#355279=CARTESIAN_POINT('Ctrl Pts',(2.21439200899994,2.2,-3.86499781800001));
#355280=CARTESIAN_POINT('Ctrl Pts',(2.21425864499994,12.2,-3.86284945600002));
#355281=CARTESIAN_POINT('Ctrl Pts',(2.21425864499994,5.2,-3.86284945600002));
#355282=CARTESIAN_POINT('Ctrl Pts',(2.21425864499994,2.2,-3.86284945600002));
#355283=CARTESIAN_POINT('Ctrl Pts',(2.21412318099994,12.2,-3.86070513500002));
#355284=CARTESIAN_POINT('Ctrl Pts',(2.21412318099994,5.2,-3.86070513500002));
#355285=CARTESIAN_POINT('Ctrl Pts',(2.21412318099994,2.2,-3.86070513500002));
#355286=CARTESIAN_POINT('Ctrl Pts',(2.21398562199994,12.2,-3.85856485900002));
#355287=CARTESIAN_POINT('Ctrl Pts',(2.21398562199994,5.2,-3.85856485900002));
#355288=CARTESIAN_POINT('Ctrl Pts',(2.21398562199994,2.2,-3.85856485900002));
#355289=CARTESIAN_POINT('Ctrl Pts',(2.21384597999994,12.2,-3.85642863600001));
#355290=CARTESIAN_POINT('Ctrl Pts',(2.21384597999994,5.2,-3.85642863600001));
#355291=CARTESIAN_POINT('Ctrl Pts',(2.21384597999994,2.2,-3.85642863600001));
#355292=CARTESIAN_POINT('Ctrl Pts',(2.21370425999994,12.2,-3.85429647200001));
#355293=CARTESIAN_POINT('Ctrl Pts',(2.21370425999994,5.2,-3.85429647200001));
#355294=CARTESIAN_POINT('Ctrl Pts',(2.21370425999994,2.2,-3.85429647200001));
#355295=CARTESIAN_POINT('Ctrl Pts',(2.21356047199994,12.2,-3.85216837300002));
#355296=CARTESIAN_POINT('Ctrl Pts',(2.21356047199994,5.2,-3.85216837300002));
#355297=CARTESIAN_POINT('Ctrl Pts',(2.21356047199994,2.2,-3.85216837300002));
#355298=CARTESIAN_POINT('Ctrl Pts',(2.21341462199994,12.2,-3.85004434600001));
#355299=CARTESIAN_POINT('Ctrl Pts',(2.21341462199994,5.2,-3.85004434600001));
#355300=CARTESIAN_POINT('Ctrl Pts',(2.21341462199994,2.2,-3.85004434600001));
#355301=CARTESIAN_POINT('Ctrl Pts',(2.21326671999994,12.2,-3.84792439700002));
#355302=CARTESIAN_POINT('Ctrl Pts',(2.21326671999994,5.2,-3.84792439700002));
#355303=CARTESIAN_POINT('Ctrl Pts',(2.21326671999994,2.2,-3.84792439700002));
#355304=CARTESIAN_POINT('Ctrl Pts',(2.21311677299994,12.2,-3.84580853300001));
#355305=CARTESIAN_POINT('Ctrl Pts',(2.21311677299994,5.2,-3.84580853300001));
#355306=CARTESIAN_POINT('Ctrl Pts',(2.21311677299994,2.2,-3.84580853300001));
#355307=CARTESIAN_POINT('Ctrl Pts',(2.21296478899994,12.2,-3.84369676000002));
#355308=CARTESIAN_POINT('Ctrl Pts',(2.21296478899994,5.2,-3.84369676000002));
#355309=CARTESIAN_POINT('Ctrl Pts',(2.21296478899994,2.2,-3.84369676000002));
#355310=CARTESIAN_POINT('Ctrl Pts',(2.21281077799994,12.2,-3.84158908500002));
#355311=CARTESIAN_POINT('Ctrl Pts',(2.21281077799994,5.2,-3.84158908500002));
#355312=CARTESIAN_POINT('Ctrl Pts',(2.21281077799994,2.2,-3.84158908500002));
#355313=CARTESIAN_POINT('Ctrl Pts',(2.21265474699994,12.2,-3.83948551400001));
#355314=CARTESIAN_POINT('Ctrl Pts',(2.21265474699994,5.2,-3.83948551400001));
#355315=CARTESIAN_POINT('Ctrl Pts',(2.21265474699994,2.2,-3.83948551400001));
#355316=CARTESIAN_POINT('Ctrl Pts',(2.21249670299994,12.2,-3.83738605300001));
#355317=CARTESIAN_POINT('Ctrl Pts',(2.21249670299994,5.2,-3.83738605300001));
#355318=CARTESIAN_POINT('Ctrl Pts',(2.21249670299994,2.2,-3.83738605300001));
#355319=CARTESIAN_POINT('Ctrl Pts',(2.21233665499994,12.2,-3.83529070900002));
#355320=CARTESIAN_POINT('Ctrl Pts',(2.21233665499994,5.2,-3.83529070900002));
#355321=CARTESIAN_POINT('Ctrl Pts',(2.21233665499994,2.2,-3.83529070900002));
#355322=CARTESIAN_POINT('Ctrl Pts',(2.21217461299994,12.2,-3.83319948700001));
#355323=CARTESIAN_POINT('Ctrl Pts',(2.21217461299994,5.2,-3.83319948700001));
#355324=CARTESIAN_POINT('Ctrl Pts',(2.21217461299994,2.2,-3.83319948700001));
#355325=CARTESIAN_POINT('Ctrl Pts',(2.21201058399994,12.2,-3.83111239700002));
#355326=CARTESIAN_POINT('Ctrl Pts',(2.21201058399994,5.2,-3.83111239700002));
#355327=CARTESIAN_POINT('Ctrl Pts',(2.21201058399994,2.2,-3.83111239700002));
#355328=CARTESIAN_POINT('Ctrl Pts',(2.21184457499994,12.2,-3.82902944200001));
#355329=CARTESIAN_POINT('Ctrl Pts',(2.21184457499994,5.2,-3.82902944200001));
#355330=CARTESIAN_POINT('Ctrl Pts',(2.21184457499994,2.2,-3.82902944200001));
#355331=CARTESIAN_POINT('Ctrl Pts',(2.21167659699994,12.2,-3.82695062900002));
#355332=CARTESIAN_POINT('Ctrl Pts',(2.21167659699994,5.2,-3.82695062900002));
#355333=CARTESIAN_POINT('Ctrl Pts',(2.21167659699994,2.2,-3.82695062900002));
#355334=CARTESIAN_POINT('Ctrl Pts',(2.21150665499994,12.2,-3.82487596600001));
#355335=CARTESIAN_POINT('Ctrl Pts',(2.21150665499994,5.2,-3.82487596600001));
#355336=CARTESIAN_POINT('Ctrl Pts',(2.21150665499994,2.2,-3.82487596600001));
#355337=CARTESIAN_POINT('Ctrl Pts',(2.21133475999994,12.2,-3.82280545700001));
#355338=CARTESIAN_POINT('Ctrl Pts',(2.21133475999994,5.2,-3.82280545700001));
#355339=CARTESIAN_POINT('Ctrl Pts',(2.21133475999994,2.2,-3.82280545700001));
#355340=CARTESIAN_POINT('Ctrl Pts',(2.21116091999995,12.2,-3.82073911100001));
#355341=CARTESIAN_POINT('Ctrl Pts',(2.21116091999995,5.2,-3.82073911100001));
#355342=CARTESIAN_POINT('Ctrl Pts',(2.21116091999995,2.2,-3.82073911100001));
#355343=CARTESIAN_POINT('Ctrl Pts',(2.21098514299995,12.2,-3.81867693300002));
#355344=CARTESIAN_POINT('Ctrl Pts',(2.21098514299995,5.2,-3.81867693300002));
#355345=CARTESIAN_POINT('Ctrl Pts',(2.21098514299995,2.2,-3.81867693300002));
#355346=CARTESIAN_POINT('Ctrl Pts',(2.21080743799994,12.2,-3.81661893000001));
#355347=CARTESIAN_POINT('Ctrl Pts',(2.21080743799994,5.2,-3.81661893000001));
#355348=CARTESIAN_POINT('Ctrl Pts',(2.21080743799994,2.2,-3.81661893000001));
#355349=CARTESIAN_POINT('Ctrl Pts',(2.21062781199994,12.2,-3.81456510700001));
#355350=CARTESIAN_POINT('Ctrl Pts',(2.21062781199994,5.2,-3.81456510700001));
#355351=CARTESIAN_POINT('Ctrl Pts',(2.21062781199994,2.2,-3.81456510700001));
#355352=CARTESIAN_POINT('Ctrl Pts',(2.21044627499994,12.2,-3.81251547200002));
#355353=CARTESIAN_POINT('Ctrl Pts',(2.21044627499994,5.2,-3.81251547200002));
#355354=CARTESIAN_POINT('Ctrl Pts',(2.21044627499994,2.2,-3.81251547200002));
#355355=CARTESIAN_POINT('Ctrl Pts',(2.21026283499994,12.2,-3.81047003000001));
#355356=CARTESIAN_POINT('Ctrl Pts',(2.21026283499994,5.2,-3.81047003000001));
#355357=CARTESIAN_POINT('Ctrl Pts',(2.21026283499994,2.2,-3.81047003000001));
#355358=CARTESIAN_POINT('Ctrl Pts',(2.21007749899994,12.2,-3.80842879000001));
#355359=CARTESIAN_POINT('Ctrl Pts',(2.21007749899994,5.2,-3.80842879000001));
#355360=CARTESIAN_POINT('Ctrl Pts',(2.21007749899994,2.2,-3.80842879000001));
#355361=CARTESIAN_POINT('Ctrl Pts',(2.20989027799994,12.2,-3.80639175500002));
#355362=CARTESIAN_POINT('Ctrl Pts',(2.20989027799994,5.2,-3.80639175500002));
#355363=CARTESIAN_POINT('Ctrl Pts',(2.20989027799994,2.2,-3.80639175500002));
#355364=CARTESIAN_POINT('Ctrl Pts',(2.20970117999994,12.2,-3.80435893400001));
#355365=CARTESIAN_POINT('Ctrl Pts',(2.20970117999994,5.2,-3.80435893400001));
#355366=CARTESIAN_POINT('Ctrl Pts',(2.20970117999994,2.2,-3.80435893400001));
#355367=CARTESIAN_POINT('Ctrl Pts',(2.20951021199994,12.2,-3.80233033200001));
#355368=CARTESIAN_POINT('Ctrl Pts',(2.20951021199994,5.2,-3.80233033200001));
#355369=CARTESIAN_POINT('Ctrl Pts',(2.20951021199994,2.2,-3.80233033200001));
#355370=CARTESIAN_POINT('Ctrl Pts',(2.20931738399994,12.2,-3.80030595700001));
#355371=CARTESIAN_POINT('Ctrl Pts',(2.20931738399994,5.2,-3.80030595700001));
#355372=CARTESIAN_POINT('Ctrl Pts',(2.20931738399994,2.2,-3.80030595700001));
#355373=CARTESIAN_POINT('Ctrl Pts',(2.20912270499994,12.2,-3.79828581200002));
#355374=CARTESIAN_POINT('Ctrl Pts',(2.20912270499994,5.2,-3.79828581200002));
#355375=CARTESIAN_POINT('Ctrl Pts',(2.20912270499994,2.2,-3.79828581200002));
#355376=CARTESIAN_POINT('Ctrl Pts',(2.20892618299994,12.2,-3.79626990800002));
#355377=CARTESIAN_POINT('Ctrl Pts',(2.20892618299994,5.2,-3.79626990800002));
#355378=CARTESIAN_POINT('Ctrl Pts',(2.20892618299994,2.2,-3.79626990800002));
#355379=CARTESIAN_POINT('Ctrl Pts',(2.20872782499994,12.2,-3.79425824700002));
#355380=CARTESIAN_POINT('Ctrl Pts',(2.20872782499994,5.2,-3.79425824700002));
#355381=CARTESIAN_POINT('Ctrl Pts',(2.20872782499994,2.2,-3.79425824700002));
#355382=CARTESIAN_POINT('Ctrl Pts',(2.20852764299994,12.2,-3.79225083900002));
#355383=CARTESIAN_POINT('Ctrl Pts',(2.20852764299994,5.2,-3.79225083900002));
#355384=CARTESIAN_POINT('Ctrl Pts',(2.20852764299994,2.2,-3.79225083900002));
#355385=CARTESIAN_POINT('Ctrl Pts',(2.20832564299994,12.2,-3.79024768800001));
#355386=CARTESIAN_POINT('Ctrl Pts',(2.20832564299994,5.2,-3.79024768800001));
#355387=CARTESIAN_POINT('Ctrl Pts',(2.20832564299994,2.2,-3.79024768800001));
#355388=CARTESIAN_POINT('Ctrl Pts',(2.20812183599994,12.2,-3.78824880200002));
#355389=CARTESIAN_POINT('Ctrl Pts',(2.20812183599994,5.2,-3.78824880200002));
#355390=CARTESIAN_POINT('Ctrl Pts',(2.20812183599994,2.2,-3.78824880200002));
#355391=CARTESIAN_POINT('Ctrl Pts',(2.20791622799994,12.2,-3.78625418600001));
#355392=CARTESIAN_POINT('Ctrl Pts',(2.20791622799994,5.2,-3.78625418600001));
#355393=CARTESIAN_POINT('Ctrl Pts',(2.20791622799994,2.2,-3.78625418600001));
#355394=CARTESIAN_POINT('Ctrl Pts',(2.20770883099994,12.2,-3.78426384700001));
#355395=CARTESIAN_POINT('Ctrl Pts',(2.20770883099994,5.2,-3.78426384700001));
#355396=CARTESIAN_POINT('Ctrl Pts',(2.20770883099994,2.2,-3.78426384700001));
#355397=CARTESIAN_POINT('Ctrl Pts',(2.20749965099994,12.2,-3.78227779100001));
#355398=CARTESIAN_POINT('Ctrl Pts',(2.20749965099994,5.2,-3.78227779100001));
#355399=CARTESIAN_POINT('Ctrl Pts',(2.20749965099994,2.2,-3.78227779100001));
#355400=CARTESIAN_POINT('Ctrl Pts',(2.20728869799994,12.2,-3.78029602500002));
#355401=CARTESIAN_POINT('Ctrl Pts',(2.20728869799994,5.2,-3.78029602500002));
#355402=CARTESIAN_POINT('Ctrl Pts',(2.20728869799994,2.2,-3.78029602500002));
#355403=CARTESIAN_POINT('Ctrl Pts',(2.20707598099994,12.2,-3.77831855500002));
#355404=CARTESIAN_POINT('Ctrl Pts',(2.20707598099994,5.2,-3.77831855500002));
#355405=CARTESIAN_POINT('Ctrl Pts',(2.20707598099994,2.2,-3.77831855500002));
#355406=CARTESIAN_POINT('Ctrl Pts',(2.20686150899994,12.2,-3.77634538800002));
#355407=CARTESIAN_POINT('Ctrl Pts',(2.20686150899994,5.2,-3.77634538800002));
#355408=CARTESIAN_POINT('Ctrl Pts',(2.20686150899994,2.2,-3.77634538800002));
#355409=CARTESIAN_POINT('Ctrl Pts',(2.20664529099994,12.2,-3.77437653000001));
#355410=CARTESIAN_POINT('Ctrl Pts',(2.20664529099994,5.2,-3.77437653000001));
#355411=CARTESIAN_POINT('Ctrl Pts',(2.20664529099994,2.2,-3.77437653000001));
#355412=CARTESIAN_POINT('Ctrl Pts',(2.20642733399994,12.2,-3.77241198700002));
#355413=CARTESIAN_POINT('Ctrl Pts',(2.20642733399994,5.2,-3.77241198700002));
#355414=CARTESIAN_POINT('Ctrl Pts',(2.20642733399994,2.2,-3.77241198700002));
#355415=CARTESIAN_POINT('Ctrl Pts',(2.20620764899994,12.2,-3.77045176500001));
#355416=CARTESIAN_POINT('Ctrl Pts',(2.20620764899994,5.2,-3.77045176500001));
#355417=CARTESIAN_POINT('Ctrl Pts',(2.20620764899994,2.2,-3.77045176500001));
#355418=CARTESIAN_POINT('Ctrl Pts',(2.20598624599994,12.2,-3.76849587100001));
#355419=CARTESIAN_POINT('Ctrl Pts',(2.20598624599994,5.2,-3.76849587100001));
#355420=CARTESIAN_POINT('Ctrl Pts',(2.20598624599994,2.2,-3.76849587100001));
#355421=CARTESIAN_POINT('Ctrl Pts',(2.20576313099994,12.2,-3.76654431200001));
#355422=CARTESIAN_POINT('Ctrl Pts',(2.20576313099994,5.2,-3.76654431200001));
#355423=CARTESIAN_POINT('Ctrl Pts',(2.20576313099994,2.2,-3.76654431200001));
#355424=CARTESIAN_POINT('Ctrl Pts',(2.20553831499994,12.2,-3.76459709300001));
#355425=CARTESIAN_POINT('Ctrl Pts',(2.20553831499994,5.2,-3.76459709300001));
#355426=CARTESIAN_POINT('Ctrl Pts',(2.20553831499994,2.2,-3.76459709300001));
#355427=CARTESIAN_POINT('Ctrl Pts',(2.20531180499994,12.2,-3.76265422200001));
#355428=CARTESIAN_POINT('Ctrl Pts',(2.20531180499994,5.2,-3.76265422200001));
#355429=CARTESIAN_POINT('Ctrl Pts',(2.20531180499994,2.2,-3.76265422200001));
#355430=CARTESIAN_POINT('Ctrl Pts',(2.20508361399994,12.2,-3.76071570400001));
#355431=CARTESIAN_POINT('Ctrl Pts',(2.20508361399994,5.2,-3.76071570400001));
#355432=CARTESIAN_POINT('Ctrl Pts',(2.20508361399994,2.2,-3.76071570400001));
#355433=CARTESIAN_POINT('Ctrl Pts',(2.20485374699994,12.2,-3.75878154600001));
#355434=CARTESIAN_POINT('Ctrl Pts',(2.20485374699994,5.2,-3.75878154600001));
#355435=CARTESIAN_POINT('Ctrl Pts',(2.20485374699994,2.2,-3.75878154600001));
#355436=CARTESIAN_POINT('Ctrl Pts',(2.20462221499994,12.2,-3.75685175400001));
#355437=CARTESIAN_POINT('Ctrl Pts',(2.20462221499994,5.2,-3.75685175400001));
#355438=CARTESIAN_POINT('Ctrl Pts',(2.20462221499994,2.2,-3.75685175400001));
#355439=CARTESIAN_POINT('Ctrl Pts',(2.20438902699994,12.2,-3.75492633400001));
#355440=CARTESIAN_POINT('Ctrl Pts',(2.20438902699994,5.2,-3.75492633400001));
#355441=CARTESIAN_POINT('Ctrl Pts',(2.20438902699994,2.2,-3.75492633400001));
#355442=CARTESIAN_POINT('Ctrl Pts',(2.20415419199994,12.2,-3.75300529300001));
#355443=CARTESIAN_POINT('Ctrl Pts',(2.20415419199994,5.2,-3.75300529300001));
#355444=CARTESIAN_POINT('Ctrl Pts',(2.20415419199994,2.2,-3.75300529300001));
#355445=CARTESIAN_POINT('Ctrl Pts',(2.20391771899994,12.2,-3.75108863800001));
#355446=CARTESIAN_POINT('Ctrl Pts',(2.20391771899994,5.2,-3.75108863800001));
#355447=CARTESIAN_POINT('Ctrl Pts',(2.20391771899994,2.2,-3.75108863800001));
#355448=CARTESIAN_POINT('Ctrl Pts',(2.20367961799994,12.2,-3.74917637400001));
#355449=CARTESIAN_POINT('Ctrl Pts',(2.20367961799994,5.2,-3.74917637400001));
#355450=CARTESIAN_POINT('Ctrl Pts',(2.20367961799994,2.2,-3.74917637400001));
#355451=CARTESIAN_POINT('Ctrl Pts',(2.20343989799994,12.2,-3.74726850800001));
#355452=CARTESIAN_POINT('Ctrl Pts',(2.20343989799994,5.2,-3.74726850800001));
#355453=CARTESIAN_POINT('Ctrl Pts',(2.20343989799994,2.2,-3.74726850800001));
#355454=CARTESIAN_POINT('Ctrl Pts',(2.20319856699994,12.2,-3.74536504600002));
#355455=CARTESIAN_POINT('Ctrl Pts',(2.20319856699994,5.2,-3.74536504600002));
#355456=CARTESIAN_POINT('Ctrl Pts',(2.20319856699994,2.2,-3.74536504600002));
#355457=CARTESIAN_POINT('Ctrl Pts',(2.20295563499994,12.2,-3.74346599500001));
#355458=CARTESIAN_POINT('Ctrl Pts',(2.20295563499994,5.2,-3.74346599500001));
#355459=CARTESIAN_POINT('Ctrl Pts',(2.20295563499994,2.2,-3.74346599500001));
#355460=CARTESIAN_POINT('Ctrl Pts',(2.20271111199994,12.2,-3.74157136100001));
#355461=CARTESIAN_POINT('Ctrl Pts',(2.20271111199994,5.2,-3.74157136100001));
#355462=CARTESIAN_POINT('Ctrl Pts',(2.20271111199994,2.2,-3.74157136100001));
#355463=CARTESIAN_POINT('Ctrl Pts',(2.20246500699994,12.2,-3.73968114900002));
#355464=CARTESIAN_POINT('Ctrl Pts',(2.20246500699994,5.2,-3.73968114900002));
#355465=CARTESIAN_POINT('Ctrl Pts',(2.20246500699994,2.2,-3.73968114900002));
#355466=CARTESIAN_POINT('Ctrl Pts',(2.20221732899994,12.2,-3.73779536900001));
#355467=CARTESIAN_POINT('Ctrl Pts',(2.20221732899994,5.2,-3.73779536900001));
#355468=CARTESIAN_POINT('Ctrl Pts',(2.20221732899994,2.2,-3.73779536900001));
#355469=CARTESIAN_POINT('Ctrl Pts',(2.20196808699994,12.2,-3.73591402400002));
#355470=CARTESIAN_POINT('Ctrl Pts',(2.20196808699994,5.2,-3.73591402400002));
#355471=CARTESIAN_POINT('Ctrl Pts',(2.20196808699994,2.2,-3.73591402400002));
#355472=CARTESIAN_POINT('Ctrl Pts',(2.20171729099994,12.2,-3.73403712000002));
#355473=CARTESIAN_POINT('Ctrl Pts',(2.20171729099994,5.2,-3.73403712000002));
#355474=CARTESIAN_POINT('Ctrl Pts',(2.20171729099994,2.2,-3.73403712000002));
#355475=CARTESIAN_POINT('Ctrl Pts',(2.20146495099994,12.2,-3.73216466500002));
#355476=CARTESIAN_POINT('Ctrl Pts',(2.20146495099994,5.2,-3.73216466500002));
#355477=CARTESIAN_POINT('Ctrl Pts',(2.20146495099994,2.2,-3.73216466500002));
#355478=CARTESIAN_POINT('Ctrl Pts',(2.20121107499994,12.2,-3.73029666600001));
#355479=CARTESIAN_POINT('Ctrl Pts',(2.20121107499994,5.2,-3.73029666600001));
#355480=CARTESIAN_POINT('Ctrl Pts',(2.20121107499994,2.2,-3.73029666600001));
#355481=CARTESIAN_POINT('Ctrl Pts',(2.20095567399994,12.2,-3.72843312700001));
#355482=CARTESIAN_POINT('Ctrl Pts',(2.20095567399994,5.2,-3.72843312700001));
#355483=CARTESIAN_POINT('Ctrl Pts',(2.20095567399994,2.2,-3.72843312700001));
#355484=CARTESIAN_POINT('Ctrl Pts',(2.20069875599994,12.2,-3.72657405600001));
#355485=CARTESIAN_POINT('Ctrl Pts',(2.20069875599994,5.2,-3.72657405600001));
#355486=CARTESIAN_POINT('Ctrl Pts',(2.20069875599994,2.2,-3.72657405600001));
#355487=CARTESIAN_POINT('Ctrl Pts',(2.20044033199994,12.2,-3.72471946000001));
#355488=CARTESIAN_POINT('Ctrl Pts',(2.20044033199994,5.2,-3.72471946000001));
#355489=CARTESIAN_POINT('Ctrl Pts',(2.20044033199994,2.2,-3.72471946000001));
#355490=CARTESIAN_POINT('Ctrl Pts',(2.20018040999994,12.2,-3.72286934200002));
#355491=CARTESIAN_POINT('Ctrl Pts',(2.20018040999994,5.2,-3.72286934200002));
#355492=CARTESIAN_POINT('Ctrl Pts',(2.20018040999994,2.2,-3.72286934200002));
#355493=CARTESIAN_POINT('Ctrl Pts',(2.19991900199994,12.2,-3.72102371200001));
#355494=CARTESIAN_POINT('Ctrl Pts',(2.19991900199994,5.2,-3.72102371200001));
#355495=CARTESIAN_POINT('Ctrl Pts',(2.19991900199994,2.2,-3.72102371200001));
#355496=CARTESIAN_POINT('Ctrl Pts',(2.19965611499994,12.2,-3.71918257500001));
#355497=CARTESIAN_POINT('Ctrl Pts',(2.19965611499994,5.2,-3.71918257500001));
#355498=CARTESIAN_POINT('Ctrl Pts',(2.19965611499994,2.2,-3.71918257500001));
#355499=CARTESIAN_POINT('Ctrl Pts',(2.19939175899994,12.2,-3.71734593700001));
#355500=CARTESIAN_POINT('Ctrl Pts',(2.19939175899994,5.2,-3.71734593700001));
#355501=CARTESIAN_POINT('Ctrl Pts',(2.19939175899994,2.2,-3.71734593700001));
#355502=CARTESIAN_POINT('Ctrl Pts',(2.19912594399994,12.2,-3.71551380500001));
#355503=CARTESIAN_POINT('Ctrl Pts',(2.19912594399994,5.2,-3.71551380500001));
#355504=CARTESIAN_POINT('Ctrl Pts',(2.19912594399994,2.2,-3.71551380500001));
#355505=CARTESIAN_POINT('Ctrl Pts',(2.19885868099994,12.2,-3.71368618300002));
#355506=CARTESIAN_POINT('Ctrl Pts',(2.19885868099994,5.2,-3.71368618300002));
#355507=CARTESIAN_POINT('Ctrl Pts',(2.19885868099994,2.2,-3.71368618300002));
#355508=CARTESIAN_POINT('Ctrl Pts',(2.19858997799994,12.2,-3.71186308000001));
#355509=CARTESIAN_POINT('Ctrl Pts',(2.19858997799994,5.2,-3.71186308000001));
#355510=CARTESIAN_POINT('Ctrl Pts',(2.19858997799994,2.2,-3.71186308000001));
#355511=CARTESIAN_POINT('Ctrl Pts',(2.19831984599994,12.2,-3.71004450200001));
#355512=CARTESIAN_POINT('Ctrl Pts',(2.19831984599994,5.2,-3.71004450200001));
#355513=CARTESIAN_POINT('Ctrl Pts',(2.19831984599994,2.2,-3.71004450200001));
#355514=CARTESIAN_POINT('Ctrl Pts',(2.19804829299994,12.2,-3.70823045400002));
#355515=CARTESIAN_POINT('Ctrl Pts',(2.19804829299994,5.2,-3.70823045400002));
#355516=CARTESIAN_POINT('Ctrl Pts',(2.19804829299994,2.2,-3.70823045400002));
#355517=CARTESIAN_POINT('Ctrl Pts',(2.19777532999994,12.2,-3.70642094300001));
#355518=CARTESIAN_POINT('Ctrl Pts',(2.19777532999994,5.2,-3.70642094300001));
#355519=CARTESIAN_POINT('Ctrl Pts',(2.19777532999994,2.2,-3.70642094300001));
#355520=CARTESIAN_POINT('Ctrl Pts',(2.19750096799994,12.2,-3.70461597600002));
#355521=CARTESIAN_POINT('Ctrl Pts',(2.19750096799994,5.2,-3.70461597600002));
#355522=CARTESIAN_POINT('Ctrl Pts',(2.19750096799994,2.2,-3.70461597600002));
#355523=CARTESIAN_POINT('Ctrl Pts',(2.19722521399994,12.2,-3.70281555800001));
#355524=CARTESIAN_POINT('Ctrl Pts',(2.19722521399994,5.2,-3.70281555800001));
#355525=CARTESIAN_POINT('Ctrl Pts',(2.19722521399994,2.2,-3.70281555800001));
#355526=CARTESIAN_POINT('Ctrl Pts',(2.19694808099994,12.2,-3.70101969500002));
#355527=CARTESIAN_POINT('Ctrl Pts',(2.19694808099994,5.2,-3.70101969500002));
#355528=CARTESIAN_POINT('Ctrl Pts',(2.19694808099994,2.2,-3.70101969500002));
#355529=CARTESIAN_POINT('Ctrl Pts',(2.19666957499994,12.2,-3.69922839500001));
#355530=CARTESIAN_POINT('Ctrl Pts',(2.19666957499994,5.2,-3.69922839500001));
#355531=CARTESIAN_POINT('Ctrl Pts',(2.19666957499994,2.2,-3.69922839500001));
#355532=CARTESIAN_POINT('Ctrl Pts',(2.19638970899994,12.2,-3.69744166300002));
#355533=CARTESIAN_POINT('Ctrl Pts',(2.19638970899994,5.2,-3.69744166300002));
#355534=CARTESIAN_POINT('Ctrl Pts',(2.19638970899994,2.2,-3.69744166300002));
#355535=CARTESIAN_POINT('Ctrl Pts',(2.19610849199994,12.2,-3.69565950700002));
#355536=CARTESIAN_POINT('Ctrl Pts',(2.19610849199994,5.2,-3.69565950700002));
#355537=CARTESIAN_POINT('Ctrl Pts',(2.19610849199994,2.2,-3.69565950700002));
#355538=CARTESIAN_POINT('Ctrl Pts',(2.19582593399994,12.2,-3.69388193000002));
#355539=CARTESIAN_POINT('Ctrl Pts',(2.19582593399994,5.2,-3.69388193000002));
#355540=CARTESIAN_POINT('Ctrl Pts',(2.19582593399994,2.2,-3.69388193000002));
#355541=CARTESIAN_POINT('Ctrl Pts',(2.19554204499994,12.2,-3.69210894200001));
#355542=CARTESIAN_POINT('Ctrl Pts',(2.19554204499994,5.2,-3.69210894200001));
#355543=CARTESIAN_POINT('Ctrl Pts',(2.19554204499994,2.2,-3.69210894200001));
#355544=CARTESIAN_POINT('Ctrl Pts',(2.19525683499994,12.2,-3.69034054600001));
#355545=CARTESIAN_POINT('Ctrl Pts',(2.19525683499994,5.2,-3.69034054600001));
#355546=CARTESIAN_POINT('Ctrl Pts',(2.19525683499994,2.2,-3.69034054600001));
#355547=CARTESIAN_POINT('Ctrl Pts',(2.19497031399994,12.2,-3.68857675100001));
#355548=CARTESIAN_POINT('Ctrl Pts',(2.19497031399994,5.2,-3.68857675100001));
#355549=CARTESIAN_POINT('Ctrl Pts',(2.19497031399994,2.2,-3.68857675100001));
#355550=CARTESIAN_POINT('Ctrl Pts',(2.19468249099994,12.2,-3.68681756100001));
#355551=CARTESIAN_POINT('Ctrl Pts',(2.19468249099994,5.2,-3.68681756100001));
#355552=CARTESIAN_POINT('Ctrl Pts',(2.19468249099994,2.2,-3.68681756100001));
#355553=CARTESIAN_POINT('Ctrl Pts',(2.19439337899995,12.2,-3.68506298400002));
#355554=CARTESIAN_POINT('Ctrl Pts',(2.19439337899995,5.2,-3.68506298400002));
#355555=CARTESIAN_POINT('Ctrl Pts',(2.19439337899995,2.2,-3.68506298400002));
#355556=CARTESIAN_POINT('Ctrl Pts',(2.19410298499994,12.2,-3.68331302600001));
#355557=CARTESIAN_POINT('Ctrl Pts',(2.19410298499994,5.2,-3.68331302600001));
#355558=CARTESIAN_POINT('Ctrl Pts',(2.19410298499994,2.2,-3.68331302600001));
#355559=CARTESIAN_POINT('Ctrl Pts',(2.19381131999994,12.2,-3.68156769100001));
#355560=CARTESIAN_POINT('Ctrl Pts',(2.19381131999994,5.2,-3.68156769100001));
#355561=CARTESIAN_POINT('Ctrl Pts',(2.19381131999994,2.2,-3.68156769100001));
#355562=CARTESIAN_POINT('Ctrl Pts',(2.19351839399994,12.2,-3.67982699000001));
#355563=CARTESIAN_POINT('Ctrl Pts',(2.19351839399994,5.2,-3.67982699000001));
#355564=CARTESIAN_POINT('Ctrl Pts',(2.19351839399994,2.2,-3.67982699000001));
#355565=CARTESIAN_POINT('Ctrl Pts',(2.19322421899994,12.2,-3.67809092400002));
#355566=CARTESIAN_POINT('Ctrl Pts',(2.19322421899994,5.2,-3.67809092400002));
#355567=CARTESIAN_POINT('Ctrl Pts',(2.19322421899994,2.2,-3.67809092400002));
#355568=CARTESIAN_POINT('Ctrl Pts',(2.19292880299994,12.2,-3.67635950300001));
#355569=CARTESIAN_POINT('Ctrl Pts',(2.19292880299994,5.2,-3.67635950300001));
#355570=CARTESIAN_POINT('Ctrl Pts',(2.19292880299994,2.2,-3.67635950300001));
#355571=CARTESIAN_POINT('Ctrl Pts',(2.19263215699994,12.2,-3.67463273100002));
#355572=CARTESIAN_POINT('Ctrl Pts',(2.19263215699994,5.2,-3.67463273100002));
#355573=CARTESIAN_POINT('Ctrl Pts',(2.19263215699994,2.2,-3.67463273100002));
#355574=CARTESIAN_POINT('Ctrl Pts',(2.19233429299994,12.2,-3.67291061600001));
#355575=CARTESIAN_POINT('Ctrl Pts',(2.19233429299994,5.2,-3.67291061600001));
#355576=CARTESIAN_POINT('Ctrl Pts',(2.19233429299994,2.2,-3.67291061600001));
#355577=CARTESIAN_POINT('Ctrl Pts',(2.19203521899995,12.2,-3.67119316200001));
#355578=CARTESIAN_POINT('Ctrl Pts',(2.19203521899995,5.2,-3.67119316200001));
#355579=CARTESIAN_POINT('Ctrl Pts',(2.19203521899995,2.2,-3.67119316200001));
#355580=CARTESIAN_POINT('Ctrl Pts',(2.19173494499994,12.2,-3.66948037700002));
#355581=CARTESIAN_POINT('Ctrl Pts',(2.19173494499994,5.2,-3.66948037700002));
#355582=CARTESIAN_POINT('Ctrl Pts',(2.19173494499994,2.2,-3.66948037700002));
#355583=CARTESIAN_POINT('Ctrl Pts',(2.19143348299994,12.2,-3.66777226800002));
#355584=CARTESIAN_POINT('Ctrl Pts',(2.19143348299994,5.2,-3.66777226800002));
#355585=CARTESIAN_POINT('Ctrl Pts',(2.19143348299994,2.2,-3.66777226800002));
#355586=CARTESIAN_POINT('Ctrl Pts',(2.19113084199994,12.2,-3.66606883900001));
#355587=CARTESIAN_POINT('Ctrl Pts',(2.19113084199994,5.2,-3.66606883900001));
#355588=CARTESIAN_POINT('Ctrl Pts',(2.19113084199994,2.2,-3.66606883900001));
#355589=CARTESIAN_POINT('Ctrl Pts',(2.19082703499994,12.2,-3.66437009700002));
#355590=CARTESIAN_POINT('Ctrl Pts',(2.19082703499994,5.2,-3.66437009700002));
#355591=CARTESIAN_POINT('Ctrl Pts',(2.19082703499994,2.2,-3.66437009700002));
#355592=CARTESIAN_POINT('Ctrl Pts',(2.19052206899994,12.2,-3.66267605000001));
#355593=CARTESIAN_POINT('Ctrl Pts',(2.19052206899994,5.2,-3.66267605000001));
#355594=CARTESIAN_POINT('Ctrl Pts',(2.19052206899994,2.2,-3.66267605000001));
#355595=CARTESIAN_POINT('Ctrl Pts',(2.19021595699994,12.2,-3.66098670100001));
#355596=CARTESIAN_POINT('Ctrl Pts',(2.19021595699994,5.2,-3.66098670100001));
#355597=CARTESIAN_POINT('Ctrl Pts',(2.19021595699994,2.2,-3.66098670100001));
#355598=CARTESIAN_POINT('Ctrl Pts',(2.18990870699994,12.2,-3.65930206000002));
#355599=CARTESIAN_POINT('Ctrl Pts',(2.18990870699994,5.2,-3.65930206000002));
#355600=CARTESIAN_POINT('Ctrl Pts',(2.18990870699994,2.2,-3.65930206000002));
#355601=CARTESIAN_POINT('Ctrl Pts',(2.18960033199994,12.2,-3.65762213000002));
#355602=CARTESIAN_POINT('Ctrl Pts',(2.18960033199994,5.2,-3.65762213000002));
#355603=CARTESIAN_POINT('Ctrl Pts',(2.18960033199994,2.2,-3.65762213000002));
#355604=CARTESIAN_POINT('Ctrl Pts',(2.18929084099994,12.2,-3.65594691900001));
#355605=CARTESIAN_POINT('Ctrl Pts',(2.18929084099994,5.2,-3.65594691900001));
#355606=CARTESIAN_POINT('Ctrl Pts',(2.18929084099994,2.2,-3.65594691900001));
#355607=CARTESIAN_POINT('Ctrl Pts',(2.18898024599994,12.2,-3.65427643200002));
#355608=CARTESIAN_POINT('Ctrl Pts',(2.18898024599994,5.2,-3.65427643200002));
#355609=CARTESIAN_POINT('Ctrl Pts',(2.18898024599994,2.2,-3.65427643200002));
#355610=CARTESIAN_POINT('Ctrl Pts',(2.18866855699994,12.2,-3.65261067600001));
#355611=CARTESIAN_POINT('Ctrl Pts',(2.18866855699994,5.2,-3.65261067600001));
#355612=CARTESIAN_POINT('Ctrl Pts',(2.18866855699994,2.2,-3.65261067600001));
#355613=CARTESIAN_POINT('Ctrl Pts',(2.18835578299994,12.2,-3.65094965700001));
#355614=CARTESIAN_POINT('Ctrl Pts',(2.18835578299994,5.2,-3.65094965700001));
#355615=CARTESIAN_POINT('Ctrl Pts',(2.18835578299994,2.2,-3.65094965700001));
#355616=CARTESIAN_POINT('Ctrl Pts',(2.18804193699994,12.2,-3.64929338100001));
#355617=CARTESIAN_POINT('Ctrl Pts',(2.18804193699994,5.2,-3.64929338100001));
#355618=CARTESIAN_POINT('Ctrl Pts',(2.18804193699994,2.2,-3.64929338100001));
#355619=CARTESIAN_POINT('Ctrl Pts',(2.18772702799995,12.2,-3.64764185600002));
#355620=CARTESIAN_POINT('Ctrl Pts',(2.18772702799995,5.2,-3.64764185600002));
#355621=CARTESIAN_POINT('Ctrl Pts',(2.18772702799995,2.2,-3.64764185600002));
#355622=CARTESIAN_POINT('Ctrl Pts',(2.18741106799994,12.2,-3.64599508600001));
#355623=CARTESIAN_POINT('Ctrl Pts',(2.18741106799994,5.2,-3.64599508600001));
#355624=CARTESIAN_POINT('Ctrl Pts',(2.18741106799994,2.2,-3.64599508600001));
#355625=CARTESIAN_POINT('Ctrl Pts',(2.18709406699995,12.2,-3.64435307700001));
#355626=CARTESIAN_POINT('Ctrl Pts',(2.18709406699995,5.2,-3.64435307700001));
#355627=CARTESIAN_POINT('Ctrl Pts',(2.18709406699995,2.2,-3.64435307700001));
#355628=CARTESIAN_POINT('Ctrl Pts',(2.18677603499994,12.2,-3.64271583700001));
#355629=CARTESIAN_POINT('Ctrl Pts',(2.18677603499994,5.2,-3.64271583700001));
#355630=CARTESIAN_POINT('Ctrl Pts',(2.18677603499994,2.2,-3.64271583700001));
#355631=CARTESIAN_POINT('Ctrl Pts',(2.18645698499994,12.2,-3.64108337100001));
#355632=CARTESIAN_POINT('Ctrl Pts',(2.18645698499994,5.2,-3.64108337100001));
#355633=CARTESIAN_POINT('Ctrl Pts',(2.18645698499994,2.2,-3.64108337100001));
#355634=CARTESIAN_POINT('Ctrl Pts',(2.18613692599994,12.2,-3.63945568500001));
#355635=CARTESIAN_POINT('Ctrl Pts',(2.18613692599994,5.2,-3.63945568500001));
#355636=CARTESIAN_POINT('Ctrl Pts',(2.18613692599994,2.2,-3.63945568500001));
#355637=CARTESIAN_POINT('Ctrl Pts',(2.18581586899994,12.2,-3.63783278600001));
#355638=CARTESIAN_POINT('Ctrl Pts',(2.18581586899994,5.2,-3.63783278600001));
#355639=CARTESIAN_POINT('Ctrl Pts',(2.18581586899994,2.2,-3.63783278600001));
#355640=CARTESIAN_POINT('Ctrl Pts',(2.18549382499994,12.2,-3.63621468100002));
#355641=CARTESIAN_POINT('Ctrl Pts',(2.18549382499994,5.2,-3.63621468100002));
#355642=CARTESIAN_POINT('Ctrl Pts',(2.18549382499994,2.2,-3.63621468100002));
#355643=CARTESIAN_POINT('Ctrl Pts',(2.18517080599994,12.2,-3.63460137400001));
#355644=CARTESIAN_POINT('Ctrl Pts',(2.18517080599994,5.2,-3.63460137400001));
#355645=CARTESIAN_POINT('Ctrl Pts',(2.18517080599994,2.2,-3.63460137400001));
#355646=CARTESIAN_POINT('Ctrl Pts',(2.18484682099994,12.2,-3.63299287100002));
#355647=CARTESIAN_POINT('Ctrl Pts',(2.18484682099994,5.2,-3.63299287100002));
#355648=CARTESIAN_POINT('Ctrl Pts',(2.18484682099994,2.2,-3.63299287100002));
#355649=CARTESIAN_POINT('Ctrl Pts',(2.18452188399994,12.2,-3.63138918100002));
#355650=CARTESIAN_POINT('Ctrl Pts',(2.18452188399994,5.2,-3.63138918100002));
#355651=CARTESIAN_POINT('Ctrl Pts',(2.18452188399994,2.2,-3.63138918100002));
#355652=CARTESIAN_POINT('Ctrl Pts',(2.18419600199994,12.2,-3.62979030800001));
#355653=CARTESIAN_POINT('Ctrl Pts',(2.18419600199994,5.2,-3.62979030800001));
#355654=CARTESIAN_POINT('Ctrl Pts',(2.18419600199994,2.2,-3.62979030800001));
#355655=CARTESIAN_POINT('Ctrl Pts',(2.18386918899994,12.2,-3.62819625900002));
#355656=CARTESIAN_POINT('Ctrl Pts',(2.18386918899994,5.2,-3.62819625900002));
#355657=CARTESIAN_POINT('Ctrl Pts',(2.18386918899994,2.2,-3.62819625900002));
#355658=CARTESIAN_POINT('Ctrl Pts',(2.18354145499994,12.2,-3.62660704000001));
#355659=CARTESIAN_POINT('Ctrl Pts',(2.18354145499994,5.2,-3.62660704000001));
#355660=CARTESIAN_POINT('Ctrl Pts',(2.18354145499994,2.2,-3.62660704000001));
#355661=CARTESIAN_POINT('Ctrl Pts',(2.18321280999994,12.2,-3.62502265600002));
#355662=CARTESIAN_POINT('Ctrl Pts',(2.18321280999994,5.2,-3.62502265600002));
#355663=CARTESIAN_POINT('Ctrl Pts',(2.18321280999994,2.2,-3.62502265600002));
#355664=CARTESIAN_POINT('Ctrl Pts',(2.18288326799994,12.2,-3.62344311600001));
#355665=CARTESIAN_POINT('Ctrl Pts',(2.18288326799994,5.2,-3.62344311600001));
#355666=CARTESIAN_POINT('Ctrl Pts',(2.18288326799994,2.2,-3.62344311600001));
#355667=CARTESIAN_POINT('Ctrl Pts',(2.18255283799994,12.2,-3.62186842300002));
#355668=CARTESIAN_POINT('Ctrl Pts',(2.18255283799994,5.2,-3.62186842300002));
#355669=CARTESIAN_POINT('Ctrl Pts',(2.18255283799994,2.2,-3.62186842300002));
#355670=CARTESIAN_POINT('Ctrl Pts',(2.18222153099994,12.2,-3.62029858500001));
#355671=CARTESIAN_POINT('Ctrl Pts',(2.18222153099994,5.2,-3.62029858500001));
#355672=CARTESIAN_POINT('Ctrl Pts',(2.18222153099994,2.2,-3.62029858500001));
#355673=CARTESIAN_POINT('Ctrl Pts',(2.18188935999994,12.2,-3.61873360700002));
#355674=CARTESIAN_POINT('Ctrl Pts',(2.18188935999994,5.2,-3.61873360700002));
#355675=CARTESIAN_POINT('Ctrl Pts',(2.18188935999994,2.2,-3.61873360700002));
#355676=CARTESIAN_POINT('Ctrl Pts',(2.18155633399994,12.2,-3.61717349600001));
#355677=CARTESIAN_POINT('Ctrl Pts',(2.18155633399994,5.2,-3.61717349600001));
#355678=CARTESIAN_POINT('Ctrl Pts',(2.18155633399994,2.2,-3.61717349600001));
#355679=CARTESIAN_POINT('Ctrl Pts',(2.18122246499994,12.2,-3.61561825900001));
#355680=CARTESIAN_POINT('Ctrl Pts',(2.18122246499994,5.2,-3.61561825900001));
#355681=CARTESIAN_POINT('Ctrl Pts',(2.18122246499994,2.2,-3.61561825900001));
#355682=CARTESIAN_POINT('Ctrl Pts',(2.18088776599994,12.2,-3.61406790100002));
#355683=CARTESIAN_POINT('Ctrl Pts',(2.18088776599994,5.2,-3.61406790100002));
#355684=CARTESIAN_POINT('Ctrl Pts',(2.18088776599994,2.2,-3.61406790100002));
#355685=CARTESIAN_POINT('Ctrl Pts',(2.18055224499994,12.2,-3.61252242700001));
#355686=CARTESIAN_POINT('Ctrl Pts',(2.18055224499994,5.2,-3.61252242700001));
#355687=CARTESIAN_POINT('Ctrl Pts',(2.18055224499994,2.2,-3.61252242700001));
#355688=CARTESIAN_POINT('Ctrl Pts',(2.18021591699994,12.2,-3.61098184500001));
#355689=CARTESIAN_POINT('Ctrl Pts',(2.18021591699994,5.2,-3.61098184500001));
#355690=CARTESIAN_POINT('Ctrl Pts',(2.18021591699994,2.2,-3.61098184500001));
#355691=CARTESIAN_POINT('Ctrl Pts',(2.17987879099994,12.2,-3.60944616000001));
#355692=CARTESIAN_POINT('Ctrl Pts',(2.17987879099994,5.2,-3.60944616000001));
#355693=CARTESIAN_POINT('Ctrl Pts',(2.17987879099994,2.2,-3.60944616000001));
#355694=CARTESIAN_POINT('Ctrl Pts',(2.17954087899995,12.2,-3.60791538000001));
#355695=CARTESIAN_POINT('Ctrl Pts',(2.17954087899995,5.2,-3.60791538000001));
#355696=CARTESIAN_POINT('Ctrl Pts',(2.17954087899995,2.2,-3.60791538000001));
#355697=CARTESIAN_POINT('Ctrl Pts',(2.17920219199994,12.2,-3.60638950800002));
#355698=CARTESIAN_POINT('Ctrl Pts',(2.17920219199994,5.2,-3.60638950800002));
#355699=CARTESIAN_POINT('Ctrl Pts',(2.17920219199994,2.2,-3.60638950800002));
#355700=CARTESIAN_POINT('Ctrl Pts',(2.17886274299994,12.2,-3.60486855300001));
#355701=CARTESIAN_POINT('Ctrl Pts',(2.17886274299994,5.2,-3.60486855300001));
#355702=CARTESIAN_POINT('Ctrl Pts',(2.17886274299994,2.2,-3.60486855300001));
#355703=CARTESIAN_POINT('Ctrl Pts',(2.17852254199994,12.2,-3.60335252000001));
#355704=CARTESIAN_POINT('Ctrl Pts',(2.17852254199994,5.2,-3.60335252000001));
#355705=CARTESIAN_POINT('Ctrl Pts',(2.17852254199994,2.2,-3.60335252000001));
#355706=CARTESIAN_POINT('Ctrl Pts',(2.17818160099994,12.2,-3.60184141400001));
#355707=CARTESIAN_POINT('Ctrl Pts',(2.17818160099994,5.2,-3.60184141400001));
#355708=CARTESIAN_POINT('Ctrl Pts',(2.17818160099994,2.2,-3.60184141400001));
#355709=CARTESIAN_POINT('Ctrl Pts',(2.17783993199994,12.2,-3.60033524400002));
#355710=CARTESIAN_POINT('Ctrl Pts',(2.17783993199994,5.2,-3.60033524400002));
#355711=CARTESIAN_POINT('Ctrl Pts',(2.17783993199994,2.2,-3.60033524400002));
#355712=CARTESIAN_POINT('Ctrl Pts',(2.17749754499994,12.2,-3.59883401300001));
#355713=CARTESIAN_POINT('Ctrl Pts',(2.17749754499994,5.2,-3.59883401300001));
#355714=CARTESIAN_POINT('Ctrl Pts',(2.17749754499994,2.2,-3.59883401300001));
#355715=CARTESIAN_POINT('Ctrl Pts',(2.17715445399994,12.2,-3.59733772900002));
#355716=CARTESIAN_POINT('Ctrl Pts',(2.17715445399994,5.2,-3.59733772900002));
#355717=CARTESIAN_POINT('Ctrl Pts',(2.17715445399994,2.2,-3.59733772900002));
#355718=CARTESIAN_POINT('Ctrl Pts',(2.17681066799994,12.2,-3.59584639700001));
#355719=CARTESIAN_POINT('Ctrl Pts',(2.17681066799994,5.2,-3.59584639700001));
#355720=CARTESIAN_POINT('Ctrl Pts',(2.17681066799994,2.2,-3.59584639700001));
#355721=CARTESIAN_POINT('Ctrl Pts',(2.17646620199994,12.2,-3.59436002300002));
#355722=CARTESIAN_POINT('Ctrl Pts',(2.17646620199994,5.2,-3.59436002300002));
#355723=CARTESIAN_POINT('Ctrl Pts',(2.17646620199994,2.2,-3.59436002300002));
#355724=CARTESIAN_POINT('Ctrl Pts',(2.17612106499994,12.2,-3.59287861500002));
#355725=CARTESIAN_POINT('Ctrl Pts',(2.17612106499994,5.2,-3.59287861500002));
#355726=CARTESIAN_POINT('Ctrl Pts',(2.17612106499994,2.2,-3.59287861500002));
#355727=CARTESIAN_POINT('Ctrl Pts',(2.17577526999994,12.2,-3.59140217700002));
#355728=CARTESIAN_POINT('Ctrl Pts',(2.17577526999994,5.2,-3.59140217700002));
#355729=CARTESIAN_POINT('Ctrl Pts',(2.17577526999994,2.2,-3.59140217700002));
#355730=CARTESIAN_POINT('Ctrl Pts',(2.17542882699994,12.2,-3.58993071600001));
#355731=CARTESIAN_POINT('Ctrl Pts',(2.17542882699994,5.2,-3.58993071600001));
#355732=CARTESIAN_POINT('Ctrl Pts',(2.17542882699994,2.2,-3.58993071600001));
#355733=CARTESIAN_POINT('Ctrl Pts',(2.17508175099994,12.2,-3.58846423800002));
#355734=CARTESIAN_POINT('Ctrl Pts',(2.17508175099994,5.2,-3.58846423800002));
#355735=CARTESIAN_POINT('Ctrl Pts',(2.17508175099994,2.2,-3.58846423800002));
#355736=CARTESIAN_POINT('Ctrl Pts',(2.17473405099994,12.2,-3.58700275000002));
#355737=CARTESIAN_POINT('Ctrl Pts',(2.17473405099994,5.2,-3.58700275000002));
#355738=CARTESIAN_POINT('Ctrl Pts',(2.17473405099994,2.2,-3.58700275000002));
#355739=CARTESIAN_POINT('Ctrl Pts',(2.17438574099994,12.2,-3.58554625600001));
#355740=CARTESIAN_POINT('Ctrl Pts',(2.17438574099994,5.2,-3.58554625600001));
#355741=CARTESIAN_POINT('Ctrl Pts',(2.17438574099994,2.2,-3.58554625600001));
#355742=CARTESIAN_POINT('Ctrl Pts',(2.17403682999994,12.2,-3.58409476300002));
#355743=CARTESIAN_POINT('Ctrl Pts',(2.17403682999994,5.2,-3.58409476300002));
#355744=CARTESIAN_POINT('Ctrl Pts',(2.17403682999994,2.2,-3.58409476300002));
#355745=CARTESIAN_POINT('Ctrl Pts',(2.17368733399994,12.2,-3.58264827700001));
#355746=CARTESIAN_POINT('Ctrl Pts',(2.17368733399994,5.2,-3.58264827700001));
#355747=CARTESIAN_POINT('Ctrl Pts',(2.17368733399994,2.2,-3.58264827700001));
#355748=CARTESIAN_POINT('Ctrl Pts',(2.17333726099994,12.2,-3.58120680500001));
#355749=CARTESIAN_POINT('Ctrl Pts',(2.17333726099994,5.2,-3.58120680500001));
#355750=CARTESIAN_POINT('Ctrl Pts',(2.17333726099994,2.2,-3.58120680500001));
#355751=CARTESIAN_POINT('Ctrl Pts',(2.17298662499994,12.2,-3.57977035300001));
#355752=CARTESIAN_POINT('Ctrl Pts',(2.17298662499994,5.2,-3.57977035300001));
#355753=CARTESIAN_POINT('Ctrl Pts',(2.17298662499994,2.2,-3.57977035300001));
#355754=CARTESIAN_POINT('Ctrl Pts',(2.17263543799994,12.2,-3.57833892500001));
#355755=CARTESIAN_POINT('Ctrl Pts',(2.17263543799994,5.2,-3.57833892500001));
#355756=CARTESIAN_POINT('Ctrl Pts',(2.17263543799994,2.2,-3.57833892500001));
#355757=CARTESIAN_POINT('Ctrl Pts',(2.17228371199994,12.2,-3.57691252900001));
#355758=CARTESIAN_POINT('Ctrl Pts',(2.17228371199994,5.2,-3.57691252900001));
#355759=CARTESIAN_POINT('Ctrl Pts',(2.17228371199994,2.2,-3.57691252900001));
#355760=CARTESIAN_POINT('Ctrl Pts',(2.17193145999994,12.2,-3.57549117100001));
#355761=CARTESIAN_POINT('Ctrl Pts',(2.17193145999994,5.2,-3.57549117100001));
#355762=CARTESIAN_POINT('Ctrl Pts',(2.17193145999994,2.2,-3.57549117100001));
#355763=CARTESIAN_POINT('Ctrl Pts',(2.17157869199994,12.2,-3.57407485600001));
#355764=CARTESIAN_POINT('Ctrl Pts',(2.17157869199994,5.2,-3.57407485600001));
#355765=CARTESIAN_POINT('Ctrl Pts',(2.17157869199994,2.2,-3.57407485600001));
#355766=CARTESIAN_POINT('Ctrl Pts',(2.17122542199994,12.2,-3.57266359000001));
#355767=CARTESIAN_POINT('Ctrl Pts',(2.17122542199994,5.2,-3.57266359000001));
#355768=CARTESIAN_POINT('Ctrl Pts',(2.17122542199994,2.2,-3.57266359000001));
#355769=CARTESIAN_POINT('Ctrl Pts',(2.17087166199994,12.2,-3.57125738100001));
#355770=CARTESIAN_POINT('Ctrl Pts',(2.17087166199994,5.2,-3.57125738100001));
#355771=CARTESIAN_POINT('Ctrl Pts',(2.17087166199994,2.2,-3.57125738100001));
#355772=CARTESIAN_POINT('Ctrl Pts',(2.17051742299994,12.2,-3.56985623300002));
#355773=CARTESIAN_POINT('Ctrl Pts',(2.17051742299994,5.2,-3.56985623300002));
#355774=CARTESIAN_POINT('Ctrl Pts',(2.17051742299994,2.2,-3.56985623300002));
#355775=CARTESIAN_POINT('Ctrl Pts',(2.17016271799995,12.2,-3.56846015200002));
#355776=CARTESIAN_POINT('Ctrl Pts',(2.17016271799995,5.2,-3.56846015200002));
#355777=CARTESIAN_POINT('Ctrl Pts',(2.17016271799995,2.2,-3.56846015200002));
#355778=CARTESIAN_POINT('Ctrl Pts',(2.16980755899994,12.2,-3.56706914600001));
#355779=CARTESIAN_POINT('Ctrl Pts',(2.16980755899994,5.2,-3.56706914600001));
#355780=CARTESIAN_POINT('Ctrl Pts',(2.16980755899994,2.2,-3.56706914600001));
#355781=CARTESIAN_POINT('Ctrl Pts',(2.16945195799994,12.2,-3.56568321900002));
#355782=CARTESIAN_POINT('Ctrl Pts',(2.16945195799994,5.2,-3.56568321900002));
#355783=CARTESIAN_POINT('Ctrl Pts',(2.16945195799994,2.2,-3.56568321900002));
#355784=CARTESIAN_POINT('Ctrl Pts',(2.16909592999994,12.2,-3.56430237800001));
#355785=CARTESIAN_POINT('Ctrl Pts',(2.16909592999994,5.2,-3.56430237800001));
#355786=CARTESIAN_POINT('Ctrl Pts',(2.16909592999994,2.2,-3.56430237800001));
#355787=CARTESIAN_POINT('Ctrl Pts',(2.16873948499994,12.2,-3.56292662800001));
#355788=CARTESIAN_POINT('Ctrl Pts',(2.16873948499994,5.2,-3.56292662800001));
#355789=CARTESIAN_POINT('Ctrl Pts',(2.16873948499994,2.2,-3.56292662800001));
#355790=CARTESIAN_POINT('Ctrl Pts',(2.16838263499994,12.2,-3.56155597700001));
#355791=CARTESIAN_POINT('Ctrl Pts',(2.16838263499994,5.2,-3.56155597700001));
#355792=CARTESIAN_POINT('Ctrl Pts',(2.16838263499994,2.2,-3.56155597700001));
#355793=CARTESIAN_POINT('Ctrl Pts',(2.16802539399994,12.2,-3.56019042900002));
#355794=CARTESIAN_POINT('Ctrl Pts',(2.16802539399994,5.2,-3.56019042900002));
#355795=CARTESIAN_POINT('Ctrl Pts',(2.16802539399994,2.2,-3.56019042900002));
#355796=CARTESIAN_POINT('Ctrl Pts',(2.16766777399994,12.2,-3.55882999100002));
#355797=CARTESIAN_POINT('Ctrl Pts',(2.16766777399994,5.2,-3.55882999100002));
#355798=CARTESIAN_POINT('Ctrl Pts',(2.16766777399994,2.2,-3.55882999100002));
#355799=CARTESIAN_POINT('Ctrl Pts',(2.16730978699994,12.2,-3.55747466800001));
#355800=CARTESIAN_POINT('Ctrl Pts',(2.16730978699994,5.2,-3.55747466800001));
#355801=CARTESIAN_POINT('Ctrl Pts',(2.16730978699994,2.2,-3.55747466800001));
#355802=CARTESIAN_POINT('Ctrl Pts',(2.16695144699994,12.2,-3.55612446800002));
#355803=CARTESIAN_POINT('Ctrl Pts',(2.16695144699994,5.2,-3.55612446800002));
#355804=CARTESIAN_POINT('Ctrl Pts',(2.16695144699994,2.2,-3.55612446800002));
#355805=CARTESIAN_POINT('Ctrl Pts',(2.16659276399994,12.2,-3.55477939500001));
#355806=CARTESIAN_POINT('Ctrl Pts',(2.16659276399994,5.2,-3.55477939500001));
#355807=CARTESIAN_POINT('Ctrl Pts',(2.16659276399994,2.2,-3.55477939500001));
#355808=CARTESIAN_POINT('Ctrl Pts',(2.16623375399994,12.2,-3.55343945600001));
#355809=CARTESIAN_POINT('Ctrl Pts',(2.16623375399994,5.2,-3.55343945600001));
#355810=CARTESIAN_POINT('Ctrl Pts',(2.16623375399994,2.2,-3.55343945600001));
#355811=CARTESIAN_POINT('Ctrl Pts',(2.16587442599994,12.2,-3.55210465600001));
#355812=CARTESIAN_POINT('Ctrl Pts',(2.16587442599994,5.2,-3.55210465600001));
#355813=CARTESIAN_POINT('Ctrl Pts',(2.16587442599994,2.2,-3.55210465600001));
#355814=CARTESIAN_POINT('Ctrl Pts',(2.16551479599994,12.2,-3.55077500300002));
#355815=CARTESIAN_POINT('Ctrl Pts',(2.16551479599994,5.2,-3.55077500300002));
#355816=CARTESIAN_POINT('Ctrl Pts',(2.16551479599994,2.2,-3.55077500300002));
#355817=CARTESIAN_POINT('Ctrl Pts',(2.16515487499994,12.2,-3.54945050100001));
#355818=CARTESIAN_POINT('Ctrl Pts',(2.16515487499994,5.2,-3.54945050100001));
#355819=CARTESIAN_POINT('Ctrl Pts',(2.16515487499994,2.2,-3.54945050100001));
#355820=CARTESIAN_POINT('Ctrl Pts',(2.16479467599994,12.2,-3.54813115700002));
#355821=CARTESIAN_POINT('Ctrl Pts',(2.16479467599994,5.2,-3.54813115700002));
#355822=CARTESIAN_POINT('Ctrl Pts',(2.16479467599994,2.2,-3.54813115700002));
#355823=CARTESIAN_POINT('Ctrl Pts',(2.16443421299994,12.2,-3.54681697600002));
#355824=CARTESIAN_POINT('Ctrl Pts',(2.16443421299994,5.2,-3.54681697600002));
#355825=CARTESIAN_POINT('Ctrl Pts',(2.16443421299994,2.2,-3.54681697600002));
#355826=CARTESIAN_POINT('Ctrl Pts',(2.16407349699994,12.2,-3.54550796500002));
#355827=CARTESIAN_POINT('Ctrl Pts',(2.16407349699994,5.2,-3.54550796500002));
#355828=CARTESIAN_POINT('Ctrl Pts',(2.16407349699994,2.2,-3.54550796500002));
#355829=CARTESIAN_POINT('Ctrl Pts',(2.16371254199994,12.2,-3.54420412900001));
#355830=CARTESIAN_POINT('Ctrl Pts',(2.16371254199994,5.2,-3.54420412900001));
#355831=CARTESIAN_POINT('Ctrl Pts',(2.16371254199994,2.2,-3.54420412900001));
#355832=CARTESIAN_POINT('Ctrl Pts',(2.16335136099994,12.2,-3.54290547500002));
#355833=CARTESIAN_POINT('Ctrl Pts',(2.16335136099994,5.2,-3.54290547500002));
#355834=CARTESIAN_POINT('Ctrl Pts',(2.16335136099994,2.2,-3.54290547500002));
#355835=CARTESIAN_POINT('Ctrl Pts',(2.16298996699994,12.2,-3.54161200800001));
#355836=CARTESIAN_POINT('Ctrl Pts',(2.16298996699994,5.2,-3.54161200800001));
#355837=CARTESIAN_POINT('Ctrl Pts',(2.16298996699994,2.2,-3.54161200800001));
#355838=CARTESIAN_POINT('Ctrl Pts',(2.16262837099995,12.2,-3.54032373500001));
#355839=CARTESIAN_POINT('Ctrl Pts',(2.16262837099995,5.2,-3.54032373500001));
#355840=CARTESIAN_POINT('Ctrl Pts',(2.16262837099995,2.2,-3.54032373500001));
#355841=CARTESIAN_POINT('Ctrl Pts',(2.16226658899994,12.2,-3.53904066100001));
#355842=CARTESIAN_POINT('Ctrl Pts',(2.16226658899994,5.2,-3.53904066100001));
#355843=CARTESIAN_POINT('Ctrl Pts',(2.16226658899994,2.2,-3.53904066100001));
#355844=CARTESIAN_POINT('Ctrl Pts',(2.16190463199994,12.2,-3.53776279200002));
#355845=CARTESIAN_POINT('Ctrl Pts',(2.16190463199994,5.2,-3.53776279200002));
#355846=CARTESIAN_POINT('Ctrl Pts',(2.16190463199994,2.2,-3.53776279200002));
#355847=CARTESIAN_POINT('Ctrl Pts',(2.16154251599994,12.2,-3.53649013400001));
#355848=CARTESIAN_POINT('Ctrl Pts',(2.16154251599994,5.2,-3.53649013400001));
#355849=CARTESIAN_POINT('Ctrl Pts',(2.16154251599994,2.2,-3.53649013400001));
#355850=CARTESIAN_POINT('Ctrl Pts',(2.16118024999994,12.2,-3.53522269300001));
#355851=CARTESIAN_POINT('Ctrl Pts',(2.16118024999994,5.2,-3.53522269300001));
#355852=CARTESIAN_POINT('Ctrl Pts',(2.16118024999994,2.2,-3.53522269300001));
#355853=CARTESIAN_POINT('Ctrl Pts',(2.16081784999994,12.2,-3.53396047500001));
#355854=CARTESIAN_POINT('Ctrl Pts',(2.16081784999994,5.2,-3.53396047500001));
#355855=CARTESIAN_POINT('Ctrl Pts',(2.16081784999994,2.2,-3.53396047500001));
#355856=CARTESIAN_POINT('Ctrl Pts',(2.16045532699995,12.2,-3.53270348700002));
#355857=CARTESIAN_POINT('Ctrl Pts',(2.16045532699995,5.2,-3.53270348700002));
#355858=CARTESIAN_POINT('Ctrl Pts',(2.16045532699995,2.2,-3.53270348700002));
#355859=CARTESIAN_POINT('Ctrl Pts',(2.16009269699994,12.2,-3.53145173300002));
#355860=CARTESIAN_POINT('Ctrl Pts',(2.16009269699994,5.2,-3.53145173300002));
#355861=CARTESIAN_POINT('Ctrl Pts',(2.16009269699994,2.2,-3.53145173300002));
#355862=CARTESIAN_POINT('Ctrl Pts',(2.15972997299994,12.2,-3.53020522000001));
#355863=CARTESIAN_POINT('Ctrl Pts',(2.15972997299994,5.2,-3.53020522000001));
#355864=CARTESIAN_POINT('Ctrl Pts',(2.15972997299994,2.2,-3.53020522000001));
#355865=CARTESIAN_POINT('Ctrl Pts',(2.15936716599994,12.2,-3.52896395300001));
#355866=CARTESIAN_POINT('Ctrl Pts',(2.15936716599994,5.2,-3.52896395300001));
#355867=CARTESIAN_POINT('Ctrl Pts',(2.15936716599994,2.2,-3.52896395300001));
#355868=CARTESIAN_POINT('Ctrl Pts',(2.15900428999994,12.2,-3.52772793900002));
#355869=CARTESIAN_POINT('Ctrl Pts',(2.15900428999994,5.2,-3.52772793900002));
#355870=CARTESIAN_POINT('Ctrl Pts',(2.15900428999994,2.2,-3.52772793900002));
#355871=CARTESIAN_POINT('Ctrl Pts',(2.15864135999994,12.2,-3.52649718400002));
#355872=CARTESIAN_POINT('Ctrl Pts',(2.15864135999994,5.2,-3.52649718400002));
#355873=CARTESIAN_POINT('Ctrl Pts',(2.15864135999994,2.2,-3.52649718400002));
#355874=CARTESIAN_POINT('Ctrl Pts',(2.15827838899994,12.2,-3.52527169200001));
#355875=CARTESIAN_POINT('Ctrl Pts',(2.15827838899994,5.2,-3.52527169200001));
#355876=CARTESIAN_POINT('Ctrl Pts',(2.15827838899994,2.2,-3.52527169200001));
#355877=CARTESIAN_POINT('Ctrl Pts',(2.15791538899994,12.2,-3.52405147100002));
#355878=CARTESIAN_POINT('Ctrl Pts',(2.15791538899994,5.2,-3.52405147100002));
#355879=CARTESIAN_POINT('Ctrl Pts',(2.15791538899994,2.2,-3.52405147100002));
#355880=CARTESIAN_POINT('Ctrl Pts',(2.15755237499994,12.2,-3.52283652600001));
#355881=CARTESIAN_POINT('Ctrl Pts',(2.15755237499994,5.2,-3.52283652600001));
#355882=CARTESIAN_POINT('Ctrl Pts',(2.15755237499994,2.2,-3.52283652600001));
#355883=CARTESIAN_POINT('Ctrl Pts',(2.15718935999994,12.2,-3.52162686400002));
#355884=CARTESIAN_POINT('Ctrl Pts',(2.15718935999994,5.2,-3.52162686400002));
#355885=CARTESIAN_POINT('Ctrl Pts',(2.15718935999994,2.2,-3.52162686400002));
#355886=CARTESIAN_POINT('Ctrl Pts',(2.15682635699994,12.2,-3.52042248900001));
#355887=CARTESIAN_POINT('Ctrl Pts',(2.15682635699994,5.2,-3.52042248900001));
#355888=CARTESIAN_POINT('Ctrl Pts',(2.15682635699994,2.2,-3.52042248900001));
#355889=CARTESIAN_POINT('Ctrl Pts',(2.15646338099994,12.2,-3.51922340700002));
#355890=CARTESIAN_POINT('Ctrl Pts',(2.15646338099994,5.2,-3.51922340700002));
#355891=CARTESIAN_POINT('Ctrl Pts',(2.15646338099994,2.2,-3.51922340700002));
#355892=CARTESIAN_POINT('Ctrl Pts',(2.15610044499994,12.2,-3.51802962600001));
#355893=CARTESIAN_POINT('Ctrl Pts',(2.15610044499994,5.2,-3.51802962600001));
#355894=CARTESIAN_POINT('Ctrl Pts',(2.15610044499994,2.2,-3.51802962600001));
#355895=CARTESIAN_POINT('Ctrl Pts',(2.15573756299994,12.2,-3.51684114900001));
#355896=CARTESIAN_POINT('Ctrl Pts',(2.15573756299994,5.2,-3.51684114900001));
#355897=CARTESIAN_POINT('Ctrl Pts',(2.15573756299994,2.2,-3.51684114900001));
#355898=CARTESIAN_POINT('Ctrl Pts',(2.15537474699994,12.2,-3.51565798400001));
#355899=CARTESIAN_POINT('Ctrl Pts',(2.15537474699994,5.2,-3.51565798400001));
#355900=CARTESIAN_POINT('Ctrl Pts',(2.15537474699994,2.2,-3.51565798400001));
#355901=CARTESIAN_POINT('Ctrl Pts',(2.15501201299995,12.2,-3.51448013600002));
#355902=CARTESIAN_POINT('Ctrl Pts',(2.15501201299995,5.2,-3.51448013600002));
#355903=CARTESIAN_POINT('Ctrl Pts',(2.15501201299995,2.2,-3.51448013600002));
#355904=CARTESIAN_POINT('Ctrl Pts',(2.15464937399994,12.2,-3.51330761100002));
#355905=CARTESIAN_POINT('Ctrl Pts',(2.15464937399994,5.2,-3.51330761100002));
#355906=CARTESIAN_POINT('Ctrl Pts',(2.15464937399994,2.2,-3.51330761100002));
#355907=CARTESIAN_POINT('Ctrl Pts',(2.15428684399994,12.2,-3.51214041500001));
#355908=CARTESIAN_POINT('Ctrl Pts',(2.15428684399994,5.2,-3.51214041500001));
#355909=CARTESIAN_POINT('Ctrl Pts',(2.15428684399994,2.2,-3.51214041500001));
#355910=CARTESIAN_POINT('Ctrl Pts',(2.15392443699994,12.2,-3.51097855400001));
#355911=CARTESIAN_POINT('Ctrl Pts',(2.15392443699994,5.2,-3.51097855400001));
#355912=CARTESIAN_POINT('Ctrl Pts',(2.15392443699994,2.2,-3.51097855400001));
#355913=CARTESIAN_POINT('Ctrl Pts',(2.15356216599994,12.2,-3.50982203300001));
#355914=CARTESIAN_POINT('Ctrl Pts',(2.15356216599994,5.2,-3.50982203300001));
#355915=CARTESIAN_POINT('Ctrl Pts',(2.15356216599994,2.2,-3.50982203300001));
#355916=CARTESIAN_POINT('Ctrl Pts',(2.15320004599994,12.2,-3.50867085800001));
#355917=CARTESIAN_POINT('Ctrl Pts',(2.15320004599994,5.2,-3.50867085800001));
#355918=CARTESIAN_POINT('Ctrl Pts',(2.15320004599994,2.2,-3.50867085800001));
#355919=CARTESIAN_POINT('Ctrl Pts',(2.15283809099994,12.2,-3.50752503500001));
#355920=CARTESIAN_POINT('Ctrl Pts',(2.15283809099994,5.2,-3.50752503500001));
#355921=CARTESIAN_POINT('Ctrl Pts',(2.15283809099994,2.2,-3.50752503500001));
#355922=CARTESIAN_POINT('Ctrl Pts',(2.15247631499994,12.2,-3.50638457100001));
#355923=CARTESIAN_POINT('Ctrl Pts',(2.15247631499994,5.2,-3.50638457100001));
#355924=CARTESIAN_POINT('Ctrl Pts',(2.15247631499994,2.2,-3.50638457100001));
#355925=CARTESIAN_POINT('Ctrl Pts',(2.15211473199994,12.2,-3.50524947100002));
#355926=CARTESIAN_POINT('Ctrl Pts',(2.15211473199994,5.2,-3.50524947100002));
#355927=CARTESIAN_POINT('Ctrl Pts',(2.15211473199994,2.2,-3.50524947100002));
#355928=CARTESIAN_POINT('Ctrl Pts',(2.15175335499994,12.2,-3.50411974000002));
#355929=CARTESIAN_POINT('Ctrl Pts',(2.15175335499994,5.2,-3.50411974000002));
#355930=CARTESIAN_POINT('Ctrl Pts',(2.15175335499994,2.2,-3.50411974000002));
#355931=CARTESIAN_POINT('Ctrl Pts',(2.15139219999994,12.2,-3.50299538300002));
#355932=CARTESIAN_POINT('Ctrl Pts',(2.15139219999994,5.2,-3.50299538300002));
#355933=CARTESIAN_POINT('Ctrl Pts',(2.15139219999994,2.2,-3.50299538300002));
#355934=CARTESIAN_POINT('Ctrl Pts',(2.15103127999994,12.2,-3.50187640800002));
#355935=CARTESIAN_POINT('Ctrl Pts',(2.15103127999994,5.2,-3.50187640800002));
#355936=CARTESIAN_POINT('Ctrl Pts',(2.15103127999994,2.2,-3.50187640800002));
#355937=CARTESIAN_POINT('Ctrl Pts',(2.15067060999994,12.2,-3.50076282000002));
#355938=CARTESIAN_POINT('Ctrl Pts',(2.15067060999994,5.2,-3.50076282000002));
#355939=CARTESIAN_POINT('Ctrl Pts',(2.15067060999994,2.2,-3.50076282000002));
#355940=CARTESIAN_POINT('Ctrl Pts',(2.15031020399994,12.2,-3.49965462500001));
#355941=CARTESIAN_POINT('Ctrl Pts',(2.15031020399994,5.2,-3.49965462500001));
#355942=CARTESIAN_POINT('Ctrl Pts',(2.15031020399994,2.2,-3.49965462500001));
#355943=CARTESIAN_POINT('Ctrl Pts',(2.14995007699994,12.2,-3.49855182900002));
#355944=CARTESIAN_POINT('Ctrl Pts',(2.14995007699994,5.2,-3.49855182900002));
#355945=CARTESIAN_POINT('Ctrl Pts',(2.14995007699994,2.2,-3.49855182900002));
#355946=CARTESIAN_POINT('Ctrl Pts',(2.14959024099994,12.2,-3.49745443600002));
#355947=CARTESIAN_POINT('Ctrl Pts',(2.14959024099994,5.2,-3.49745443600002));
#355948=CARTESIAN_POINT('Ctrl Pts',(2.14959024099994,2.2,-3.49745443600002));
#355949=CARTESIAN_POINT('Ctrl Pts',(2.14923071399994,12.2,-3.49636245400001));
#355950=CARTESIAN_POINT('Ctrl Pts',(2.14923071399994,5.2,-3.49636245400001));
#355951=CARTESIAN_POINT('Ctrl Pts',(2.14923071399994,2.2,-3.49636245400001));
#355952=CARTESIAN_POINT('Ctrl Pts',(2.14887150799994,12.2,-3.49527588800001));
#355953=CARTESIAN_POINT('Ctrl Pts',(2.14887150799994,5.2,-3.49527588800001));
#355954=CARTESIAN_POINT('Ctrl Pts',(2.14887150799994,2.2,-3.49527588800001));
#355955=CARTESIAN_POINT('Ctrl Pts',(2.14851263799994,12.2,-3.49419474300001));
#355956=CARTESIAN_POINT('Ctrl Pts',(2.14851263799994,5.2,-3.49419474300001));
#355957=CARTESIAN_POINT('Ctrl Pts',(2.14851263799994,2.2,-3.49419474300001));
#355958=CARTESIAN_POINT('Ctrl Pts',(2.14815411799994,12.2,-3.49311902500002));
#355959=CARTESIAN_POINT('Ctrl Pts',(2.14815411799994,5.2,-3.49311902500002));
#355960=CARTESIAN_POINT('Ctrl Pts',(2.14815411799994,2.2,-3.49311902500002));
#355961=CARTESIAN_POINT('Ctrl Pts',(2.14779596399994,12.2,-3.49204874100002));
#355962=CARTESIAN_POINT('Ctrl Pts',(2.14779596399994,5.2,-3.49204874100002));
#355963=CARTESIAN_POINT('Ctrl Pts',(2.14779596399994,2.2,-3.49204874100002));
#355964=CARTESIAN_POINT('Ctrl Pts',(2.14743819099994,12.2,-3.49098389500002));
#355965=CARTESIAN_POINT('Ctrl Pts',(2.14743819099994,5.2,-3.49098389500002));
#355966=CARTESIAN_POINT('Ctrl Pts',(2.14743819099994,2.2,-3.49098389500002));
#355967=CARTESIAN_POINT('Ctrl Pts',(2.14708081099994,12.2,-3.48992449400002));
#355968=CARTESIAN_POINT('Ctrl Pts',(2.14708081099994,5.2,-3.48992449400002));
#355969=CARTESIAN_POINT('Ctrl Pts',(2.14708081099994,2.2,-3.48992449400002));
#355970=CARTESIAN_POINT('Ctrl Pts',(2.14672384099994,12.2,-3.48887054300001));
#355971=CARTESIAN_POINT('Ctrl Pts',(2.14672384099994,5.2,-3.48887054300001));
#355972=CARTESIAN_POINT('Ctrl Pts',(2.14672384099994,2.2,-3.48887054300001));
#355973=CARTESIAN_POINT('Ctrl Pts',(2.14636729499994,12.2,-3.48782204800001));
#355974=CARTESIAN_POINT('Ctrl Pts',(2.14636729499994,5.2,-3.48782204800001));
#355975=CARTESIAN_POINT('Ctrl Pts',(2.14636729499994,2.2,-3.48782204800001));
#355976=CARTESIAN_POINT('Ctrl Pts',(2.14601118799994,12.2,-3.48677901500002));
#355977=CARTESIAN_POINT('Ctrl Pts',(2.14601118799994,5.2,-3.48677901500002));
#355978=CARTESIAN_POINT('Ctrl Pts',(2.14601118799994,2.2,-3.48677901500002));
#355979=CARTESIAN_POINT('Ctrl Pts',(2.14565553399995,12.2,-3.48574145000002));
#355980=CARTESIAN_POINT('Ctrl Pts',(2.14565553399995,5.2,-3.48574145000002));
#355981=CARTESIAN_POINT('Ctrl Pts',(2.14565553399995,2.2,-3.48574145000002));
#355982=CARTESIAN_POINT('Ctrl Pts',(2.14530034899994,12.2,-3.48470935700002));
#355983=CARTESIAN_POINT('Ctrl Pts',(2.14530034899994,5.2,-3.48470935700002));
#355984=CARTESIAN_POINT('Ctrl Pts',(2.14530034899994,2.2,-3.48470935700002));
#355985=CARTESIAN_POINT('Ctrl Pts',(2.14494564799994,12.2,-3.48368274400002));
#355986=CARTESIAN_POINT('Ctrl Pts',(2.14494564799994,5.2,-3.48368274400002));
#355987=CARTESIAN_POINT('Ctrl Pts',(2.14494564799994,2.2,-3.48368274400002));
#355988=CARTESIAN_POINT('Ctrl Pts',(2.14459144499994,12.2,-3.48266161500002));
#355989=CARTESIAN_POINT('Ctrl Pts',(2.14459144499994,5.2,-3.48266161500002));
#355990=CARTESIAN_POINT('Ctrl Pts',(2.14459144499994,2.2,-3.48266161500002));
#355991=CARTESIAN_POINT('Ctrl Pts',(2.14423775599994,12.2,-3.48164597700002));
#355992=CARTESIAN_POINT('Ctrl Pts',(2.14423775599994,5.2,-3.48164597700002));
#355993=CARTESIAN_POINT('Ctrl Pts',(2.14423775599994,2.2,-3.48164597700002));
#355994=CARTESIAN_POINT('Ctrl Pts',(2.14388459599994,12.2,-3.48063583400001));
#355995=CARTESIAN_POINT('Ctrl Pts',(2.14388459599994,5.2,-3.48063583400001));
#355996=CARTESIAN_POINT('Ctrl Pts',(2.14388459599994,2.2,-3.48063583400001));
#355997=CARTESIAN_POINT('Ctrl Pts',(2.14353197899994,12.2,-3.47963119300001));
#355998=CARTESIAN_POINT('Ctrl Pts',(2.14353197899994,5.2,-3.47963119300001));
#355999=CARTESIAN_POINT('Ctrl Pts',(2.14353197899994,2.2,-3.47963119300001));
#356000=CARTESIAN_POINT('Ctrl Pts',(2.14317992199994,12.2,-3.47863205900001));
#356001=CARTESIAN_POINT('Ctrl Pts',(2.14317992199994,5.2,-3.47863205900001));
#356002=CARTESIAN_POINT('Ctrl Pts',(2.14317992199994,2.2,-3.47863205900001));
#356003=CARTESIAN_POINT('Ctrl Pts',(2.14282843799994,12.2,-3.47763843900001));
#356004=CARTESIAN_POINT('Ctrl Pts',(2.14282843799994,5.2,-3.47763843900001));
#356005=CARTESIAN_POINT('Ctrl Pts',(2.14282843799994,2.2,-3.47763843900001));
#356006=CARTESIAN_POINT('Ctrl Pts',(2.14247754299994,12.2,-3.47665033700002));
#356007=CARTESIAN_POINT('Ctrl Pts',(2.14247754299994,5.2,-3.47665033700002));
#356008=CARTESIAN_POINT('Ctrl Pts',(2.14247754299994,2.2,-3.47665033700002));
#356009=CARTESIAN_POINT('Ctrl Pts',(2.14212725399994,12.2,-3.47566776000001));
#356010=CARTESIAN_POINT('Ctrl Pts',(2.14212725399994,5.2,-3.47566776000001));
#356011=CARTESIAN_POINT('Ctrl Pts',(2.14212725399994,2.2,-3.47566776000001));
#356012=CARTESIAN_POINT('Ctrl Pts',(2.14177758399994,12.2,-3.47469071200001));
#356013=CARTESIAN_POINT('Ctrl Pts',(2.14177758399994,5.2,-3.47469071200001));
#356014=CARTESIAN_POINT('Ctrl Pts',(2.14177758399994,2.2,-3.47469071200001));
#356015=CARTESIAN_POINT('Ctrl Pts',(2.14142854999994,12.2,-3.47371920000001));
#356016=CARTESIAN_POINT('Ctrl Pts',(2.14142854999994,5.2,-3.47371920000001));
#356017=CARTESIAN_POINT('Ctrl Pts',(2.14142854999994,2.2,-3.47371920000001));
#356018=CARTESIAN_POINT('Ctrl Pts',(2.14108016699994,12.2,-3.47275323000002));
#356019=CARTESIAN_POINT('Ctrl Pts',(2.14108016699994,5.2,-3.47275323000002));
#356020=CARTESIAN_POINT('Ctrl Pts',(2.14108016699994,2.2,-3.47275323000002));
#356021=CARTESIAN_POINT('Ctrl Pts',(2.14073244999994,12.2,-3.47179280600002));
#356022=CARTESIAN_POINT('Ctrl Pts',(2.14073244999994,5.2,-3.47179280600002));
#356023=CARTESIAN_POINT('Ctrl Pts',(2.14073244999994,2.2,-3.47179280600002));
#356024=CARTESIAN_POINT('Ctrl Pts',(2.14038541399994,12.2,-3.47083793500001));
#356025=CARTESIAN_POINT('Ctrl Pts',(2.14038541399994,5.2,-3.47083793500001));
#356026=CARTESIAN_POINT('Ctrl Pts',(2.14038541399994,2.2,-3.47083793500001));
#356027=CARTESIAN_POINT('Ctrl Pts',(2.14003907599994,12.2,-3.46988862200002));
#356028=CARTESIAN_POINT('Ctrl Pts',(2.14003907599994,5.2,-3.46988862200002));
#356029=CARTESIAN_POINT('Ctrl Pts',(2.14003907599994,2.2,-3.46988862200002));
#356030=CARTESIAN_POINT('Ctrl Pts',(2.13969345099994,12.2,-3.46894487300001));
#356031=CARTESIAN_POINT('Ctrl Pts',(2.13969345099994,5.2,-3.46894487300001));
#356032=CARTESIAN_POINT('Ctrl Pts',(2.13969345099994,2.2,-3.46894487300001));
#356033=CARTESIAN_POINT('Ctrl Pts',(2.13934855399994,12.2,-3.46800669400002));
#356034=CARTESIAN_POINT('Ctrl Pts',(2.13934855399994,5.2,-3.46800669400002));
#356035=CARTESIAN_POINT('Ctrl Pts',(2.13934855399994,2.2,-3.46800669400002));
#356036=CARTESIAN_POINT('Ctrl Pts',(2.13900440199994,12.2,-3.46707408900001));
#356037=CARTESIAN_POINT('Ctrl Pts',(2.13900440199994,5.2,-3.46707408900001));
#356038=CARTESIAN_POINT('Ctrl Pts',(2.13900440199994,2.2,-3.46707408900001));
#356039=CARTESIAN_POINT('Ctrl Pts',(2.13866100999994,12.2,-3.46614706600001));
#356040=CARTESIAN_POINT('Ctrl Pts',(2.13866100999994,5.2,-3.46614706600001));
#356041=CARTESIAN_POINT('Ctrl Pts',(2.13866100999994,2.2,-3.46614706600001));
#356042=CARTESIAN_POINT('Ctrl Pts',(2.13831839299994,12.2,-3.46522562800001));
#356043=CARTESIAN_POINT('Ctrl Pts',(2.13831839299994,5.2,-3.46522562800001));
#356044=CARTESIAN_POINT('Ctrl Pts',(2.13831839299994,2.2,-3.46522562800001));
#356045=CARTESIAN_POINT('Ctrl Pts',(2.13797656899994,12.2,-3.46430978300001));
#356046=CARTESIAN_POINT('Ctrl Pts',(2.13797656899994,5.2,-3.46430978300001));
#356047=CARTESIAN_POINT('Ctrl Pts',(2.13797656899994,2.2,-3.46430978300001));
#356048=CARTESIAN_POINT('Ctrl Pts',(2.13763555199994,12.2,-3.46339953500001));
#356049=CARTESIAN_POINT('Ctrl Pts',(2.13763555199994,5.2,-3.46339953500001));
#356050=CARTESIAN_POINT('Ctrl Pts',(2.13763555199994,2.2,-3.46339953500001));
#356051=CARTESIAN_POINT('Ctrl Pts',(2.13729535799994,12.2,-3.46249489000002));
#356052=CARTESIAN_POINT('Ctrl Pts',(2.13729535799994,5.2,-3.46249489000002));
#356053=CARTESIAN_POINT('Ctrl Pts',(2.13729535799994,2.2,-3.46249489000002));
#356054=CARTESIAN_POINT('Ctrl Pts',(2.13695600499994,12.2,-3.46159585300001));
#356055=CARTESIAN_POINT('Ctrl Pts',(2.13695600499994,5.2,-3.46159585300001));
#356056=CARTESIAN_POINT('Ctrl Pts',(2.13695600499994,2.2,-3.46159585300001));
#356057=CARTESIAN_POINT('Ctrl Pts',(2.13661750599994,12.2,-3.46070243100002));
#356058=CARTESIAN_POINT('Ctrl Pts',(2.13661750599994,5.2,-3.46070243100002));
#356059=CARTESIAN_POINT('Ctrl Pts',(2.13661750599994,2.2,-3.46070243100002));
#356060=CARTESIAN_POINT('Ctrl Pts',(2.13627987899994,12.2,-3.45981462900002));
#356061=CARTESIAN_POINT('Ctrl Pts',(2.13627987899994,5.2,-3.45981462900002));
#356062=CARTESIAN_POINT('Ctrl Pts',(2.13627987899994,2.2,-3.45981462900002));
#356063=CARTESIAN_POINT('Ctrl Pts',(2.13594314099994,12.2,-3.45893245100001));
#356064=CARTESIAN_POINT('Ctrl Pts',(2.13594314099994,5.2,-3.45893245100001));
#356065=CARTESIAN_POINT('Ctrl Pts',(2.13594314099994,2.2,-3.45893245100001));
#356066=CARTESIAN_POINT('Ctrl Pts',(2.13560730499994,12.2,-3.45805590500001));
#356067=CARTESIAN_POINT('Ctrl Pts',(2.13560730499994,5.2,-3.45805590500001));
#356068=CARTESIAN_POINT('Ctrl Pts',(2.13560730499994,2.2,-3.45805590500001));
#356069=CARTESIAN_POINT('Ctrl Pts',(2.13527238999994,12.2,-3.45718499500002));
#356070=CARTESIAN_POINT('Ctrl Pts',(2.13527238999994,5.2,-3.45718499500002));
#356071=CARTESIAN_POINT('Ctrl Pts',(2.13527238999994,2.2,-3.45718499500002));
#356072=CARTESIAN_POINT('Ctrl Pts',(2.13493841199994,12.2,-3.45631972700001));
#356073=CARTESIAN_POINT('Ctrl Pts',(2.13493841199994,5.2,-3.45631972700001));
#356074=CARTESIAN_POINT('Ctrl Pts',(2.13493841199994,2.2,-3.45631972700001));
#356075=CARTESIAN_POINT('Ctrl Pts',(2.13460538699994,12.2,-3.45546010700001));
#356076=CARTESIAN_POINT('Ctrl Pts',(2.13460538699994,5.2,-3.45546010700001));
#356077=CARTESIAN_POINT('Ctrl Pts',(2.13460538699994,2.2,-3.45546010700001));
#356078=CARTESIAN_POINT('Ctrl Pts',(2.13427332999994,12.2,-3.45460614000002));
#356079=CARTESIAN_POINT('Ctrl Pts',(2.13427332999994,5.2,-3.45460614000002));
#356080=CARTESIAN_POINT('Ctrl Pts',(2.13427332999994,2.2,-3.45460614000002));
#356081=CARTESIAN_POINT('Ctrl Pts',(2.13394225899994,12.2,-3.45375783200002));
#356082=CARTESIAN_POINT('Ctrl Pts',(2.13394225899994,5.2,-3.45375783200002));
#356083=CARTESIAN_POINT('Ctrl Pts',(2.13394225899994,2.2,-3.45375783200002));
#356084=CARTESIAN_POINT('Ctrl Pts',(2.13361218999994,12.2,-3.45291518600002));
#356085=CARTESIAN_POINT('Ctrl Pts',(2.13361218999994,5.2,-3.45291518600002));
#356086=CARTESIAN_POINT('Ctrl Pts',(2.13361218999994,2.2,-3.45291518600002));
#356087=CARTESIAN_POINT('Ctrl Pts',(2.13328313999994,12.2,-3.45207821100002));
#356088=CARTESIAN_POINT('Ctrl Pts',(2.13328313999994,5.2,-3.45207821100002));
#356089=CARTESIAN_POINT('Ctrl Pts',(2.13328313999994,2.2,-3.45207821100002));
#356090=CARTESIAN_POINT('Ctrl Pts',(2.13295512499994,12.2,-3.45124691100001));
#356091=CARTESIAN_POINT('Ctrl Pts',(2.13295512499994,5.2,-3.45124691100001));
#356092=CARTESIAN_POINT('Ctrl Pts',(2.13295512499994,2.2,-3.45124691100001));
#356093=CARTESIAN_POINT('Ctrl Pts',(2.13262816099994,12.2,-3.45042129200001));
#356094=CARTESIAN_POINT('Ctrl Pts',(2.13262816099994,5.2,-3.45042129200001));
#356095=CARTESIAN_POINT('Ctrl Pts',(2.13262816099994,2.2,-3.45042129200001));
#356096=CARTESIAN_POINT('Ctrl Pts',(2.13230226599994,12.2,-3.44960135800001));
#356097=CARTESIAN_POINT('Ctrl Pts',(2.13230226599994,5.2,-3.44960135800001));
#356098=CARTESIAN_POINT('Ctrl Pts',(2.13230226599994,2.2,-3.44960135800001));
#356099=CARTESIAN_POINT('Ctrl Pts',(2.13197745699994,12.2,-3.44878711700002));
#356100=CARTESIAN_POINT('Ctrl Pts',(2.13197745699994,5.2,-3.44878711700002));
#356101=CARTESIAN_POINT('Ctrl Pts',(2.13197745699994,2.2,-3.44878711700002));
#356102=CARTESIAN_POINT('Ctrl Pts',(2.13165374899994,12.2,-3.44797857200001));
#356103=CARTESIAN_POINT('Ctrl Pts',(2.13165374899994,5.2,-3.44797857200001));
#356104=CARTESIAN_POINT('Ctrl Pts',(2.13165374899994,2.2,-3.44797857200001));
#356105=CARTESIAN_POINT('Ctrl Pts',(2.13133115999994,12.2,-3.44717573000001));
#356106=CARTESIAN_POINT('Ctrl Pts',(2.13133115999994,5.2,-3.44717573000001));
#356107=CARTESIAN_POINT('Ctrl Pts',(2.13133115999994,2.2,-3.44717573000001));
#356108=CARTESIAN_POINT('Ctrl Pts',(2.13100970599994,12.2,-3.44637859500001));
#356109=CARTESIAN_POINT('Ctrl Pts',(2.13100970599994,5.2,-3.44637859500001));
#356110=CARTESIAN_POINT('Ctrl Pts',(2.13100970599994,2.2,-3.44637859500001));
#356111=CARTESIAN_POINT('Ctrl Pts',(2.13068940599995,12.2,-3.44558717500002));
#356112=CARTESIAN_POINT('Ctrl Pts',(2.13068940599995,5.2,-3.44558717500002));
#356113=CARTESIAN_POINT('Ctrl Pts',(2.13068940599995,2.2,-3.44558717500002));
#356114=CARTESIAN_POINT('Ctrl Pts',(2.13037027499994,12.2,-3.44480147200001));
#356115=CARTESIAN_POINT('Ctrl Pts',(2.13037027499994,5.2,-3.44480147200001));
#356116=CARTESIAN_POINT('Ctrl Pts',(2.13037027499994,2.2,-3.44480147200001));
#356117=CARTESIAN_POINT('Ctrl Pts',(2.13005233099994,12.2,-3.44402149500001));
#356118=CARTESIAN_POINT('Ctrl Pts',(2.13005233099994,5.2,-3.44402149500001));
#356119=CARTESIAN_POINT('Ctrl Pts',(2.13005233099994,2.2,-3.44402149500001));
#356120=CARTESIAN_POINT('Ctrl Pts',(2.12973558999995,12.2,-3.44324724700002));
#356121=CARTESIAN_POINT('Ctrl Pts',(2.12973558999995,5.2,-3.44324724700002));
#356122=CARTESIAN_POINT('Ctrl Pts',(2.12973558999995,2.2,-3.44324724700002));
#356123=CARTESIAN_POINT('Ctrl Pts',(2.12942007099994,12.2,-3.44247873500001));
#356124=CARTESIAN_POINT('Ctrl Pts',(2.12942007099994,5.2,-3.44247873500001));
#356125=CARTESIAN_POINT('Ctrl Pts',(2.12942007099994,2.2,-3.44247873500001));
#356126=CARTESIAN_POINT('Ctrl Pts',(2.12910578899994,12.2,-3.44171596300002));
#356127=CARTESIAN_POINT('Ctrl Pts',(2.12910578899994,5.2,-3.44171596300002));
#356128=CARTESIAN_POINT('Ctrl Pts',(2.12910578899994,2.2,-3.44171596300002));
#356129=CARTESIAN_POINT('Ctrl Pts',(2.12879276299994,12.2,-3.44095893700001));
#356130=CARTESIAN_POINT('Ctrl Pts',(2.12879276299994,5.2,-3.44095893700001));
#356131=CARTESIAN_POINT('Ctrl Pts',(2.12879276299994,2.2,-3.44095893700001));
#356132=CARTESIAN_POINT('Ctrl Pts',(2.12848100899994,12.2,-3.44020766300002));
#356133=CARTESIAN_POINT('Ctrl Pts',(2.12848100899994,5.2,-3.44020766300002));
#356134=CARTESIAN_POINT('Ctrl Pts',(2.12848100899994,2.2,-3.44020766300002));
#356135=CARTESIAN_POINT('Ctrl Pts',(2.12817054599994,12.2,-3.43946214500002));
#356136=CARTESIAN_POINT('Ctrl Pts',(2.12817054599994,5.2,-3.43946214500002));
#356137=CARTESIAN_POINT('Ctrl Pts',(2.12817054599994,2.2,-3.43946214500002));
#356138=CARTESIAN_POINT('Ctrl Pts',(2.12786138899994,12.2,-3.43872239000001));
#356139=CARTESIAN_POINT('Ctrl Pts',(2.12786138899994,5.2,-3.43872239000001));
#356140=CARTESIAN_POINT('Ctrl Pts',(2.12786138899994,2.2,-3.43872239000001));
#356141=CARTESIAN_POINT('Ctrl Pts',(2.12755355799994,12.2,-3.43798840300002));
#356142=CARTESIAN_POINT('Ctrl Pts',(2.12755355799994,5.2,-3.43798840300002));
#356143=CARTESIAN_POINT('Ctrl Pts',(2.12755355799994,2.2,-3.43798840300002));
#356144=CARTESIAN_POINT('Ctrl Pts',(2.12724706999994,12.2,-3.43726018800002));
#356145=CARTESIAN_POINT('Ctrl Pts',(2.12724706999994,5.2,-3.43726018800002));
#356146=CARTESIAN_POINT('Ctrl Pts',(2.12724706999994,2.2,-3.43726018800002));
#356147=CARTESIAN_POINT('Ctrl Pts',(2.12694194099994,12.2,-3.43653775300002));
#356148=CARTESIAN_POINT('Ctrl Pts',(2.12694194099994,5.2,-3.43653775300002));
#356149=CARTESIAN_POINT('Ctrl Pts',(2.12694194099994,2.2,-3.43653775300002));
#356150=CARTESIAN_POINT('Ctrl Pts',(2.12663818999994,12.2,-3.43582110000002));
#356151=CARTESIAN_POINT('Ctrl Pts',(2.12663818999994,5.2,-3.43582110000002));
#356152=CARTESIAN_POINT('Ctrl Pts',(2.12663818999994,2.2,-3.43582110000002));
#356153=CARTESIAN_POINT('Ctrl Pts',(2.12633583399994,12.2,-3.43511023700001));
#356154=CARTESIAN_POINT('Ctrl Pts',(2.12633583399994,5.2,-3.43511023700001));
#356155=CARTESIAN_POINT('Ctrl Pts',(2.12633583399994,2.2,-3.43511023700001));
#356156=CARTESIAN_POINT('Ctrl Pts',(2.12603489099994,12.2,-3.43440516800001));
#356157=CARTESIAN_POINT('Ctrl Pts',(2.12603489099994,5.2,-3.43440516800001));
#356158=CARTESIAN_POINT('Ctrl Pts',(2.12603489099994,2.2,-3.43440516800001));
#356159=CARTESIAN_POINT('Ctrl Pts',(2.12573537999994,12.2,-3.43370590000001));
#356160=CARTESIAN_POINT('Ctrl Pts',(2.12573537999994,5.2,-3.43370590000001));
#356161=CARTESIAN_POINT('Ctrl Pts',(2.12573537999994,2.2,-3.43370590000001));
#356162=CARTESIAN_POINT('Ctrl Pts',(2.12543731699994,12.2,-3.43301243700001));
#356163=CARTESIAN_POINT('Ctrl Pts',(2.12543731699994,5.2,-3.43301243700001));
#356164=CARTESIAN_POINT('Ctrl Pts',(2.12543731699994,2.2,-3.43301243700001));
#356165=CARTESIAN_POINT('Ctrl Pts',(2.12514071999994,12.2,-3.43232478400001));
#356166=CARTESIAN_POINT('Ctrl Pts',(2.12514071999994,5.2,-3.43232478400001));
#356167=CARTESIAN_POINT('Ctrl Pts',(2.12514071999994,2.2,-3.43232478400001));
#356168=CARTESIAN_POINT('Ctrl Pts',(2.12484560899994,12.2,-3.43164294800001));
#356169=CARTESIAN_POINT('Ctrl Pts',(2.12484560899994,5.2,-3.43164294800001));
#356170=CARTESIAN_POINT('Ctrl Pts',(2.12484560899994,2.2,-3.43164294800001));
#356171=CARTESIAN_POINT('Ctrl Pts',(2.12455199899994,12.2,-3.43096693100001));
#356172=CARTESIAN_POINT('Ctrl Pts',(2.12455199899994,5.2,-3.43096693100001));
#356173=CARTESIAN_POINT('Ctrl Pts',(2.12455199899994,2.2,-3.43096693100001));
#356174=CARTESIAN_POINT('Ctrl Pts',(2.12425991099995,12.2,-3.43029674300002));
#356175=CARTESIAN_POINT('Ctrl Pts',(2.12425991099995,5.2,-3.43029674300002));
#356176=CARTESIAN_POINT('Ctrl Pts',(2.12425991099995,2.2,-3.43029674300002));
#356177=CARTESIAN_POINT('Ctrl Pts',(2.12396936099994,12.2,-3.42963238600001));
#356178=CARTESIAN_POINT('Ctrl Pts',(2.12396936099994,5.2,-3.42963238600001));
#356179=CARTESIAN_POINT('Ctrl Pts',(2.12396936099994,2.2,-3.42963238600001));
#356180=CARTESIAN_POINT('Ctrl Pts',(2.12368036799994,12.2,-3.42897386600002));
#356181=CARTESIAN_POINT('Ctrl Pts',(2.12368036799994,5.2,-3.42897386600002));
#356182=CARTESIAN_POINT('Ctrl Pts',(2.12368036799994,2.2,-3.42897386600002));
#356183=CARTESIAN_POINT('Ctrl Pts',(2.12339295199994,12.2,-3.42832118800001));
#356184=CARTESIAN_POINT('Ctrl Pts',(2.12339295199994,5.2,-3.42832118800001));
#356185=CARTESIAN_POINT('Ctrl Pts',(2.12339295199994,2.2,-3.42832118800001));
#356186=CARTESIAN_POINT('Ctrl Pts',(2.12310712799994,12.2,-3.42767435900001));
#356187=CARTESIAN_POINT('Ctrl Pts',(2.12310712799994,5.2,-3.42767435900001));
#356188=CARTESIAN_POINT('Ctrl Pts',(2.12310712799994,2.2,-3.42767435900001));
#356189=CARTESIAN_POINT('Ctrl Pts',(2.12282291699994,12.2,-3.42703338200002));
#356190=CARTESIAN_POINT('Ctrl Pts',(2.12282291699994,5.2,-3.42703338200002));
#356191=CARTESIAN_POINT('Ctrl Pts',(2.12282291699994,2.2,-3.42703338200002));
#356192=CARTESIAN_POINT('Ctrl Pts',(2.12254033599994,12.2,-3.42639826400001));
#356193=CARTESIAN_POINT('Ctrl Pts',(2.12254033599994,5.2,-3.42639826400001));
#356194=CARTESIAN_POINT('Ctrl Pts',(2.12254033599994,2.2,-3.42639826400001));
#356195=CARTESIAN_POINT('Ctrl Pts',(2.12225940399994,12.2,-3.42576900900001));
#356196=CARTESIAN_POINT('Ctrl Pts',(2.12225940399994,5.2,-3.42576900900001));
#356197=CARTESIAN_POINT('Ctrl Pts',(2.12225940399994,2.2,-3.42576900900001));
#356198=CARTESIAN_POINT('Ctrl Pts',(2.12198013999994,12.2,-3.42514562300002));
#356199=CARTESIAN_POINT('Ctrl Pts',(2.12198013999994,5.2,-3.42514562300002));
#356200=CARTESIAN_POINT('Ctrl Pts',(2.12198013999994,2.2,-3.42514562300002));
#356201=CARTESIAN_POINT('Ctrl Pts',(2.12170256199994,12.2,-3.42452811200001));
#356202=CARTESIAN_POINT('Ctrl Pts',(2.12170256199994,5.2,-3.42452811200001));
#356203=CARTESIAN_POINT('Ctrl Pts',(2.12170256199994,2.2,-3.42452811200001));
#356204=CARTESIAN_POINT('Ctrl Pts',(2.12142668899994,12.2,-3.42391647900001));
#356205=CARTESIAN_POINT('Ctrl Pts',(2.12142668899994,5.2,-3.42391647900001));
#356206=CARTESIAN_POINT('Ctrl Pts',(2.12142668899994,2.2,-3.42391647900001));
#356207=CARTESIAN_POINT('Ctrl Pts',(2.12115253899994,12.2,-3.42331073200001));
#356208=CARTESIAN_POINT('Ctrl Pts',(2.12115253899994,5.2,-3.42331073200001));
#356209=CARTESIAN_POINT('Ctrl Pts',(2.12115253899994,2.2,-3.42331073200001));
#356210=CARTESIAN_POINT('Ctrl Pts',(2.12088013199994,12.2,-3.42271087300002));
#356211=CARTESIAN_POINT('Ctrl Pts',(2.12088013199994,5.2,-3.42271087300002));
#356212=CARTESIAN_POINT('Ctrl Pts',(2.12088013199994,2.2,-3.42271087300002));
#356213=CARTESIAN_POINT('Ctrl Pts',(2.12060948599994,12.2,-3.42211691100001));
#356214=CARTESIAN_POINT('Ctrl Pts',(2.12060948599994,5.2,-3.42211691100001));
#356215=CARTESIAN_POINT('Ctrl Pts',(2.12060948599994,2.2,-3.42211691100001));
#356216=CARTESIAN_POINT('Ctrl Pts',(2.12034061999994,12.2,-3.42152884800001));
#356217=CARTESIAN_POINT('Ctrl Pts',(2.12034061999994,5.2,-3.42152884800001));
#356218=CARTESIAN_POINT('Ctrl Pts',(2.12034061999994,2.2,-3.42152884800001));
#356219=CARTESIAN_POINT('Ctrl Pts',(2.12007355199994,12.2,-3.42094669100002));
#356220=CARTESIAN_POINT('Ctrl Pts',(2.12007355199994,5.2,-3.42094669100002));
#356221=CARTESIAN_POINT('Ctrl Pts',(2.12007355199994,2.2,-3.42094669100002));
#356222=CARTESIAN_POINT('Ctrl Pts',(2.11980830399995,12.2,-3.42037044400001));
#356223=CARTESIAN_POINT('Ctrl Pts',(2.11980830399995,5.2,-3.42037044400001));
#356224=CARTESIAN_POINT('Ctrl Pts',(2.11980830399995,2.2,-3.42037044400001));
#356225=CARTESIAN_POINT('Ctrl Pts',(2.11954489199994,12.2,-3.41980011300001));
#356226=CARTESIAN_POINT('Ctrl Pts',(2.11954489199994,5.2,-3.41980011300001));
#356227=CARTESIAN_POINT('Ctrl Pts',(2.11954489199994,2.2,-3.41980011300001));
#356228=CARTESIAN_POINT('Ctrl Pts',(2.11928333699994,12.2,-3.41923570400001));
#356229=CARTESIAN_POINT('Ctrl Pts',(2.11928333699994,5.2,-3.41923570400001));
#356230=CARTESIAN_POINT('Ctrl Pts',(2.11928333699994,2.2,-3.41923570400001));
#356231=CARTESIAN_POINT('Ctrl Pts',(2.11902365799994,12.2,-3.41867722100002));
#356232=CARTESIAN_POINT('Ctrl Pts',(2.11902365799994,5.2,-3.41867722100002));
#356233=CARTESIAN_POINT('Ctrl Pts',(2.11902365799994,2.2,-3.41867722100002));
#356234=CARTESIAN_POINT('Ctrl Pts',(2.11876587399995,12.2,-3.41812466800001));
#356235=CARTESIAN_POINT('Ctrl Pts',(2.11876587399995,5.2,-3.41812466800001));
#356236=CARTESIAN_POINT('Ctrl Pts',(2.11876587399995,2.2,-3.41812466800001));
#356237=CARTESIAN_POINT('Ctrl Pts',(2.11851000399994,12.2,-3.41757805300002));
#356238=CARTESIAN_POINT('Ctrl Pts',(2.11851000399994,5.2,-3.41757805300002));
#356239=CARTESIAN_POINT('Ctrl Pts',(2.11851000399994,2.2,-3.41757805300002));
#356240=CARTESIAN_POINT('Ctrl Pts',(2.11825606799994,12.2,-3.41703738000001));
#356241=CARTESIAN_POINT('Ctrl Pts',(2.11825606799994,5.2,-3.41703738000001));
#356242=CARTESIAN_POINT('Ctrl Pts',(2.11825606799994,2.2,-3.41703738000001));
#356243=CARTESIAN_POINT('Ctrl Pts',(2.11800408499994,12.2,-3.41650265300002));
#356244=CARTESIAN_POINT('Ctrl Pts',(2.11800408499994,5.2,-3.41650265300002));
#356245=CARTESIAN_POINT('Ctrl Pts',(2.11800408499994,2.2,-3.41650265300002));
#356246=CARTESIAN_POINT('Ctrl Pts',(2.11775407499994,12.2,-3.41597387700002));
#356247=CARTESIAN_POINT('Ctrl Pts',(2.11775407499994,5.2,-3.41597387700002));
#356248=CARTESIAN_POINT('Ctrl Pts',(2.11775407499994,2.2,-3.41597387700002));
#356249=CARTESIAN_POINT('Ctrl Pts',(2.11750605799994,12.2,-3.41545106000002));
#356250=CARTESIAN_POINT('Ctrl Pts',(2.11750605799994,5.2,-3.41545106000002));
#356251=CARTESIAN_POINT('Ctrl Pts',(2.11750605799994,2.2,-3.41545106000002));
#356252=CARTESIAN_POINT('Ctrl Pts',(2.11726005199994,12.2,-3.41493420500001));
#356253=CARTESIAN_POINT('Ctrl Pts',(2.11726005199994,5.2,-3.41493420500001));
#356254=CARTESIAN_POINT('Ctrl Pts',(2.11726005199994,2.2,-3.41493420500001));
#356255=CARTESIAN_POINT('Ctrl Pts',(2.11701607899994,12.2,-3.41442331700001));
#356256=CARTESIAN_POINT('Ctrl Pts',(2.11701607899994,5.2,-3.41442331700001));
#356257=CARTESIAN_POINT('Ctrl Pts',(2.11701607899994,2.2,-3.41442331700001));
#356258=CARTESIAN_POINT('Ctrl Pts',(2.11677415599994,12.2,-3.41391840100002));
#356259=CARTESIAN_POINT('Ctrl Pts',(2.11677415599994,5.2,-3.41391840100002));
#356260=CARTESIAN_POINT('Ctrl Pts',(2.11677415599994,2.2,-3.41391840100002));
#356261=CARTESIAN_POINT('Ctrl Pts',(2.11653430599994,12.2,-3.41341946400001));
#356262=CARTESIAN_POINT('Ctrl Pts',(2.11653430599994,5.2,-3.41341946400001));
#356263=CARTESIAN_POINT('Ctrl Pts',(2.11653430599994,2.2,-3.41341946400001));
#356264=CARTESIAN_POINT('Ctrl Pts',(2.11629654699994,12.2,-3.41292650800002));
#356265=CARTESIAN_POINT('Ctrl Pts',(2.11629654699994,5.2,-3.41292650800002));
#356266=CARTESIAN_POINT('Ctrl Pts',(2.11629654699994,2.2,-3.41292650800002));
#356267=CARTESIAN_POINT('Ctrl Pts',(2.11606089999994,12.2,-3.41243954100001));
#356268=CARTESIAN_POINT('Ctrl Pts',(2.11606089999994,5.2,-3.41243954100001));
#356269=CARTESIAN_POINT('Ctrl Pts',(2.11606089999994,2.2,-3.41243954100001));
#356270=CARTESIAN_POINT('Ctrl Pts',(2.11582738399994,12.2,-3.41195856600002));
#356271=CARTESIAN_POINT('Ctrl Pts',(2.11582738399994,5.2,-3.41195856600002));
#356272=CARTESIAN_POINT('Ctrl Pts',(2.11582738399994,2.2,-3.41195856600002));
#356273=CARTESIAN_POINT('Ctrl Pts',(2.11559601999994,12.2,-3.41148358900002));
#356274=CARTESIAN_POINT('Ctrl Pts',(2.11559601999994,5.2,-3.41148358900002));
#356275=CARTESIAN_POINT('Ctrl Pts',(2.11559601999994,2.2,-3.41148358900002));
#356276=CARTESIAN_POINT('Ctrl Pts',(2.11536682799994,12.2,-3.41101461600001));
#356277=CARTESIAN_POINT('Ctrl Pts',(2.11536682799994,5.2,-3.41101461600001));
#356278=CARTESIAN_POINT('Ctrl Pts',(2.11536682799994,2.2,-3.41101461600001));
#356279=CARTESIAN_POINT('Ctrl Pts',(2.11513982899994,12.2,-3.41055165000002));
#356280=CARTESIAN_POINT('Ctrl Pts',(2.11513982899994,5.2,-3.41055165000002));
#356281=CARTESIAN_POINT('Ctrl Pts',(2.11513982899994,2.2,-3.41055165000002));
#356282=CARTESIAN_POINT('Ctrl Pts',(2.11491504099994,12.2,-3.41009469700001));
#356283=CARTESIAN_POINT('Ctrl Pts',(2.11491504099994,5.2,-3.41009469700001));
#356284=CARTESIAN_POINT('Ctrl Pts',(2.11491504099994,2.2,-3.41009469700001));
#356285=CARTESIAN_POINT('Ctrl Pts',(2.11469248799994,12.2,-3.40964376300001));
#356286=CARTESIAN_POINT('Ctrl Pts',(2.11469248799994,5.2,-3.40964376300001));
#356287=CARTESIAN_POINT('Ctrl Pts',(2.11469248799994,2.2,-3.40964376300001));
#356288=CARTESIAN_POINT('Ctrl Pts',(2.11447218799994,12.2,-3.40919885100002));
#356289=CARTESIAN_POINT('Ctrl Pts',(2.11447218799994,5.2,-3.40919885100002));
#356290=CARTESIAN_POINT('Ctrl Pts',(2.11447218799994,2.2,-3.40919885100002));
#356291=CARTESIAN_POINT('Ctrl Pts',(2.11425416099994,12.2,-3.40875996800001));
#356292=CARTESIAN_POINT('Ctrl Pts',(2.11425416099994,5.2,-3.40875996800001));
#356293=CARTESIAN_POINT('Ctrl Pts',(2.11425416099994,2.2,-3.40875996800001));
#356294=CARTESIAN_POINT('Ctrl Pts',(2.11403842999994,12.2,-3.40832711800001));
#356295=CARTESIAN_POINT('Ctrl Pts',(2.11403842999994,5.2,-3.40832711800001));
#356296=CARTESIAN_POINT('Ctrl Pts',(2.11403842999994,2.2,-3.40832711800001));
#356297=CARTESIAN_POINT('Ctrl Pts',(2.11382501399994,12.2,-3.40790030600001));
#356298=CARTESIAN_POINT('Ctrl Pts',(2.11382501399994,5.2,-3.40790030600001));
#356299=CARTESIAN_POINT('Ctrl Pts',(2.11382501399994,2.2,-3.40790030600001));
#356300=CARTESIAN_POINT('Ctrl Pts',(2.11361393499994,12.2,-3.40747953700001));
#356301=CARTESIAN_POINT('Ctrl Pts',(2.11361393499994,5.2,-3.40747953700001));
#356302=CARTESIAN_POINT('Ctrl Pts',(2.11361393499994,2.2,-3.40747953700001));
#356303=CARTESIAN_POINT('Ctrl Pts',(2.11340521199994,12.2,-3.40706481700002));
#356304=CARTESIAN_POINT('Ctrl Pts',(2.11340521199994,5.2,-3.40706481700002));
#356305=CARTESIAN_POINT('Ctrl Pts',(2.11340521199994,2.2,-3.40706481700002));
#356306=CARTESIAN_POINT('Ctrl Pts',(2.11319886699994,12.2,-3.40665614900002));
#356307=CARTESIAN_POINT('Ctrl Pts',(2.11319886699994,5.2,-3.40665614900002));
#356308=CARTESIAN_POINT('Ctrl Pts',(2.11319886699994,2.2,-3.40665614900002));
#356309=CARTESIAN_POINT('Ctrl Pts',(2.11299492199994,12.2,-3.40625353900001));
#356310=CARTESIAN_POINT('Ctrl Pts',(2.11299492199994,5.2,-3.40625353900001));
#356311=CARTESIAN_POINT('Ctrl Pts',(2.11299492199994,2.2,-3.40625353900001));
#356312=CARTESIAN_POINT('Ctrl Pts',(2.11279339699994,12.2,-3.40585699300001));
#356313=CARTESIAN_POINT('Ctrl Pts',(2.11279339699994,5.2,-3.40585699300001));
#356314=CARTESIAN_POINT('Ctrl Pts',(2.11279339699994,2.2,-3.40585699300001));
#356315=CARTESIAN_POINT('Ctrl Pts',(2.11259431199994,12.2,-3.40546651500001));
#356316=CARTESIAN_POINT('Ctrl Pts',(2.11259431199994,5.2,-3.40546651500001));
#356317=CARTESIAN_POINT('Ctrl Pts',(2.11259431199994,2.2,-3.40546651500001));
#356318=CARTESIAN_POINT('Ctrl Pts',(2.11239769099994,12.2,-3.40508211000001));
#356319=CARTESIAN_POINT('Ctrl Pts',(2.11239769099994,5.2,-3.40508211000001));
#356320=CARTESIAN_POINT('Ctrl Pts',(2.11239769099994,2.2,-3.40508211000001));
#356321=CARTESIAN_POINT('Ctrl Pts',(2.11220355199994,12.2,-3.40470378200001));
#356322=CARTESIAN_POINT('Ctrl Pts',(2.11220355199994,5.2,-3.40470378200001));
#356323=CARTESIAN_POINT('Ctrl Pts',(2.11220355199994,2.2,-3.40470378200001));
#356324=CARTESIAN_POINT('Ctrl Pts',(2.11201191899994,12.2,-3.40433153700001));
#356325=CARTESIAN_POINT('Ctrl Pts',(2.11201191899994,5.2,-3.40433153700001));
#356326=CARTESIAN_POINT('Ctrl Pts',(2.11201191899994,2.2,-3.40433153700001));
#356327=CARTESIAN_POINT('Ctrl Pts',(2.11182281299994,12.2,-3.40396538000002));
#356328=CARTESIAN_POINT('Ctrl Pts',(2.11182281299994,5.2,-3.40396538000002));
#356329=CARTESIAN_POINT('Ctrl Pts',(2.11182281299994,2.2,-3.40396538000002));
#356330=CARTESIAN_POINT('Ctrl Pts',(2.11163625399994,12.2,-3.40360531600002));
#356331=CARTESIAN_POINT('Ctrl Pts',(2.11163625399994,5.2,-3.40360531600002));
#356332=CARTESIAN_POINT('Ctrl Pts',(2.11163625399994,2.2,-3.40360531600002));
#356333=CARTESIAN_POINT('Ctrl Pts',(2.11145226499994,12.2,-3.40325134900001));
#356334=CARTESIAN_POINT('Ctrl Pts',(2.11145226499994,5.2,-3.40325134900001));
#356335=CARTESIAN_POINT('Ctrl Pts',(2.11145226499994,2.2,-3.40325134900001));
#356336=CARTESIAN_POINT('Ctrl Pts',(2.11127086799995,12.2,-3.40290348400002));
#356337=CARTESIAN_POINT('Ctrl Pts',(2.11127086799995,5.2,-3.40290348400002));
#356338=CARTESIAN_POINT('Ctrl Pts',(2.11127086799995,2.2,-3.40290348400002));
#356339=CARTESIAN_POINT('Ctrl Pts',(2.11109208399994,12.2,-3.40256172700002));
#356340=CARTESIAN_POINT('Ctrl Pts',(2.11109208399994,5.2,-3.40256172700002));
#356341=CARTESIAN_POINT('Ctrl Pts',(2.11109208399994,2.2,-3.40256172700002));
#356342=CARTESIAN_POINT('Ctrl Pts',(2.11091593499994,12.2,-3.40222608100001));
#356343=CARTESIAN_POINT('Ctrl Pts',(2.11091593499994,5.2,-3.40222608100001));
#356344=CARTESIAN_POINT('Ctrl Pts',(2.11091593499994,2.2,-3.40222608100001));
#356345=CARTESIAN_POINT('Ctrl Pts',(2.11074244199994,12.2,-3.40189655400001));
#356346=CARTESIAN_POINT('Ctrl Pts',(2.11074244199994,5.2,-3.40189655400001));
#356347=CARTESIAN_POINT('Ctrl Pts',(2.11074244199994,2.2,-3.40189655400001));
#356348=CARTESIAN_POINT('Ctrl Pts',(2.11057162799994,12.2,-3.40157314800001));
#356349=CARTESIAN_POINT('Ctrl Pts',(2.11057162799994,5.2,-3.40157314800001));
#356350=CARTESIAN_POINT('Ctrl Pts',(2.11057162799994,2.2,-3.40157314800001));
#356351=CARTESIAN_POINT('Ctrl Pts',(2.11040351499994,12.2,-3.40125586800001));
#356352=CARTESIAN_POINT('Ctrl Pts',(2.11040351499994,5.2,-3.40125586800001));
#356353=CARTESIAN_POINT('Ctrl Pts',(2.11040351499994,2.2,-3.40125586800001));
#356354=CARTESIAN_POINT('Ctrl Pts',(2.11023812499994,12.2,-3.40094472100001));
#356355=CARTESIAN_POINT('Ctrl Pts',(2.11023812499994,5.2,-3.40094472100001));
#356356=CARTESIAN_POINT('Ctrl Pts',(2.11023812499994,2.2,-3.40094472100001));
#356357=CARTESIAN_POINT('Ctrl Pts',(2.11007547899994,12.2,-3.40063970900002));
#356358=CARTESIAN_POINT('Ctrl Pts',(2.11007547899994,5.2,-3.40063970900002));
#356359=CARTESIAN_POINT('Ctrl Pts',(2.11007547899994,2.2,-3.40063970900002));
#356360=CARTESIAN_POINT('Ctrl Pts',(2.10991560099994,12.2,-3.40034083900001));
#356361=CARTESIAN_POINT('Ctrl Pts',(2.10991560099994,5.2,-3.40034083900001));
#356362=CARTESIAN_POINT('Ctrl Pts',(2.10991560099994,2.2,-3.40034083900001));
#356363=CARTESIAN_POINT('Ctrl Pts',(2.10975851299994,12.2,-3.40004811500001));
#356364=CARTESIAN_POINT('Ctrl Pts',(2.10975851299994,5.2,-3.40004811500001));
#356365=CARTESIAN_POINT('Ctrl Pts',(2.10975851299994,2.2,-3.40004811500001));
#356366=CARTESIAN_POINT('Ctrl Pts',(2.10960423699994,12.2,-3.39976154100002));
#356367=CARTESIAN_POINT('Ctrl Pts',(2.10960423699994,5.2,-3.39976154100002));
#356368=CARTESIAN_POINT('Ctrl Pts',(2.10960423699994,2.2,-3.39976154100002));
#356369=CARTESIAN_POINT('Ctrl Pts',(2.10945279699994,12.2,-3.39948112300001));
#356370=CARTESIAN_POINT('Ctrl Pts',(2.10945279699994,5.2,-3.39948112300001));
#356371=CARTESIAN_POINT('Ctrl Pts',(2.10945279699994,2.2,-3.39948112300001));
#356372=CARTESIAN_POINT('Ctrl Pts',(2.10930421299994,12.2,-3.39920686600002));
#356373=CARTESIAN_POINT('Ctrl Pts',(2.10930421299994,5.2,-3.39920686600002));
#356374=CARTESIAN_POINT('Ctrl Pts',(2.10930421299994,2.2,-3.39920686600002));
#356375=CARTESIAN_POINT('Ctrl Pts',(2.10915850899994,12.2,-3.39893877300002));
#356376=CARTESIAN_POINT('Ctrl Pts',(2.10915850899994,5.2,-3.39893877300002));
#356377=CARTESIAN_POINT('Ctrl Pts',(2.10915850899994,2.2,-3.39893877300002));
#356378=CARTESIAN_POINT('Ctrl Pts',(2.10901570899994,12.2,-3.39867685100002));
#356379=CARTESIAN_POINT('Ctrl Pts',(2.10901570899994,5.2,-3.39867685100002));
#356380=CARTESIAN_POINT('Ctrl Pts',(2.10901570899994,2.2,-3.39867685100002));
#356381=CARTESIAN_POINT('Ctrl Pts',(2.10887583399994,12.2,-3.39842110400001));
#356382=CARTESIAN_POINT('Ctrl Pts',(2.10887583399994,5.2,-3.39842110400001));
#356383=CARTESIAN_POINT('Ctrl Pts',(2.10887583399994,2.2,-3.39842110400001));
#356384=CARTESIAN_POINT('Ctrl Pts',(2.10873890799994,12.2,-3.39817153600002));
#356385=CARTESIAN_POINT('Ctrl Pts',(2.10873890799994,5.2,-3.39817153600002));
#356386=CARTESIAN_POINT('Ctrl Pts',(2.10873890799994,2.2,-3.39817153600002));
#356387=CARTESIAN_POINT('Ctrl Pts',(2.10860495299994,12.2,-3.39792815200001));
#356388=CARTESIAN_POINT('Ctrl Pts',(2.10860495299994,5.2,-3.39792815200001));
#356389=CARTESIAN_POINT('Ctrl Pts',(2.10860495299994,2.2,-3.39792815200001));
#356390=CARTESIAN_POINT('Ctrl Pts',(2.10847399199994,12.2,-3.39769095600001));
#356391=CARTESIAN_POINT('Ctrl Pts',(2.10847399199994,5.2,-3.39769095600001));
#356392=CARTESIAN_POINT('Ctrl Pts',(2.10847399199994,2.2,-3.39769095600001));
#356393=CARTESIAN_POINT('Ctrl Pts',(2.10834605099994,12.2,-3.39745995500001));
#356394=CARTESIAN_POINT('Ctrl Pts',(2.10834605099994,5.2,-3.39745995500001));
#356395=CARTESIAN_POINT('Ctrl Pts',(2.10834605099994,2.2,-3.39745995500001));
#356396=CARTESIAN_POINT('Ctrl Pts',(2.10822115099994,12.2,-3.39723515100002));
#356397=CARTESIAN_POINT('Ctrl Pts',(2.10822115099994,5.2,-3.39723515100002));
#356398=CARTESIAN_POINT('Ctrl Pts',(2.10822115099994,2.2,-3.39723515100002));
#356399=CARTESIAN_POINT('Ctrl Pts',(2.10809931399994,12.2,-3.39701655100002));
#356400=CARTESIAN_POINT('Ctrl Pts',(2.10809931399994,5.2,-3.39701655100002));
#356401=CARTESIAN_POINT('Ctrl Pts',(2.10809931399994,2.2,-3.39701655100002));
#356402=CARTESIAN_POINT('Ctrl Pts',(2.10798056699994,12.2,-3.39680415900002));
#356403=CARTESIAN_POINT('Ctrl Pts',(2.10798056699994,5.2,-3.39680415900002));
#356404=CARTESIAN_POINT('Ctrl Pts',(2.10798056699994,2.2,-3.39680415900002));
#356405=CARTESIAN_POINT('Ctrl Pts',(2.10786493099994,12.2,-3.39659797800001));
#356406=CARTESIAN_POINT('Ctrl Pts',(2.10786493099994,5.2,-3.39659797800001));
#356407=CARTESIAN_POINT('Ctrl Pts',(2.10786493099994,2.2,-3.39659797800001));
#356408=CARTESIAN_POINT('Ctrl Pts',(2.10775242999994,12.2,-3.39639801400001));
#356409=CARTESIAN_POINT('Ctrl Pts',(2.10775242999994,5.2,-3.39639801400001));
#356410=CARTESIAN_POINT('Ctrl Pts',(2.10775242999994,2.2,-3.39639801400001));
#356411=CARTESIAN_POINT('Ctrl Pts',(2.10764308699994,12.2,-3.39620427400002));
#356412=CARTESIAN_POINT('Ctrl Pts',(2.10764308699994,5.2,-3.39620427400002));
#356413=CARTESIAN_POINT('Ctrl Pts',(2.10764308699994,2.2,-3.39620427400002));
#356414=CARTESIAN_POINT('Ctrl Pts',(2.10753692699994,12.2,-3.39601675800001));
#356415=CARTESIAN_POINT('Ctrl Pts',(2.10753692699994,5.2,-3.39601675800001));
#356416=CARTESIAN_POINT('Ctrl Pts',(2.10753692699994,2.2,-3.39601675800001));
#356417=CARTESIAN_POINT('Ctrl Pts',(2.10743397399995,12.2,-3.39583547300002));
#356418=CARTESIAN_POINT('Ctrl Pts',(2.10743397399995,5.2,-3.39583547300002));
#356419=CARTESIAN_POINT('Ctrl Pts',(2.10743397399995,2.2,-3.39583547300002));
#356420=CARTESIAN_POINT('Ctrl Pts',(2.10733425199995,12.2,-3.39566042500001));
#356421=CARTESIAN_POINT('Ctrl Pts',(2.10733425199995,5.2,-3.39566042500001));
#356422=CARTESIAN_POINT('Ctrl Pts',(2.10733425199995,2.2,-3.39566042500001));
#356423=CARTESIAN_POINT('Ctrl Pts',(2.10723778599994,12.2,-3.39549161700001));
#356424=CARTESIAN_POINT('Ctrl Pts',(2.10723778599994,5.2,-3.39549161700001));
#356425=CARTESIAN_POINT('Ctrl Pts',(2.10723778599994,2.2,-3.39549161700001));
#356426=CARTESIAN_POINT('Ctrl Pts',(2.10714459799994,12.2,-3.39532905300001));
#356427=CARTESIAN_POINT('Ctrl Pts',(2.10714459799994,5.2,-3.39532905300001));
#356428=CARTESIAN_POINT('Ctrl Pts',(2.10714459799994,2.2,-3.39532905300001));
#356429=CARTESIAN_POINT('Ctrl Pts',(2.10705471299994,12.2,-3.39517273800002));
#356430=CARTESIAN_POINT('Ctrl Pts',(2.10705471299994,5.2,-3.39517273800002));
#356431=CARTESIAN_POINT('Ctrl Pts',(2.10705471299994,2.2,-3.39517273800002));
#356432=CARTESIAN_POINT('Ctrl Pts',(2.10696815599994,12.2,-3.39502267900002));
#356433=CARTESIAN_POINT('Ctrl Pts',(2.10696815599994,5.2,-3.39502267900002));
#356434=CARTESIAN_POINT('Ctrl Pts',(2.10696815599994,2.2,-3.39502267900002));
#356435=CARTESIAN_POINT('Ctrl Pts',(2.10688494999994,12.2,-3.39487887700002));
#356436=CARTESIAN_POINT('Ctrl Pts',(2.10688494999994,5.2,-3.39487887700002));
#356437=CARTESIAN_POINT('Ctrl Pts',(2.10688494999994,2.2,-3.39487887700002));
#356438=CARTESIAN_POINT('Ctrl Pts',(2.10680511899994,12.2,-3.39474133800001));
#356439=CARTESIAN_POINT('Ctrl Pts',(2.10680511899994,5.2,-3.39474133800001));
#356440=CARTESIAN_POINT('Ctrl Pts',(2.10680511899994,2.2,-3.39474133800001));
#356441=CARTESIAN_POINT('Ctrl Pts',(2.10672868799994,12.2,-3.39461006600001));
#356442=CARTESIAN_POINT('Ctrl Pts',(2.10672868799994,5.2,-3.39461006600001));
#356443=CARTESIAN_POINT('Ctrl Pts',(2.10672868799994,2.2,-3.39461006600001));
#356444=CARTESIAN_POINT('Ctrl Pts',(2.10665568499994,12.2,-3.39448506800001));
#356445=CARTESIAN_POINT('Ctrl Pts',(2.10665568499994,5.2,-3.39448506800001));
#356446=CARTESIAN_POINT('Ctrl Pts',(2.10665568499994,2.2,-3.39448506800001));
#356447=CARTESIAN_POINT('Ctrl Pts',(2.10658613299994,12.2,-3.39436634600002));
#356448=CARTESIAN_POINT('Ctrl Pts',(2.10658613299994,5.2,-3.39436634600002));
#356449=CARTESIAN_POINT('Ctrl Pts',(2.10658613299994,2.2,-3.39436634600002));
#356450=CARTESIAN_POINT('Ctrl Pts',(2.10652005899994,12.2,-3.39425390500002));
#356451=CARTESIAN_POINT('Ctrl Pts',(2.10652005899994,5.2,-3.39425390500002));
#356452=CARTESIAN_POINT('Ctrl Pts',(2.10652005899994,2.2,-3.39425390500002));
#356453=CARTESIAN_POINT('Ctrl Pts',(2.10645748799994,12.2,-3.39414775200002));
#356454=CARTESIAN_POINT('Ctrl Pts',(2.10645748799994,5.2,-3.39414775200002));
#356455=CARTESIAN_POINT('Ctrl Pts',(2.10645748799994,2.2,-3.39414775200002));
#356456=CARTESIAN_POINT('Ctrl Pts',(2.10639844199994,12.2,-3.39404788800001));
#356457=CARTESIAN_POINT('Ctrl Pts',(2.10639844199994,5.2,-3.39404788800001));
#356458=CARTESIAN_POINT('Ctrl Pts',(2.10639844199994,2.2,-3.39404788800001));
#356459=CARTESIAN_POINT('Ctrl Pts',(2.10634294299994,12.2,-3.39395431800002));
#356460=CARTESIAN_POINT('Ctrl Pts',(2.10634294299994,5.2,-3.39395431800002));
#356461=CARTESIAN_POINT('Ctrl Pts',(2.10634294299994,2.2,-3.39395431800002));
#356462=CARTESIAN_POINT('Ctrl Pts',(2.10629101599995,12.2,-3.39386704700001));
#356463=CARTESIAN_POINT('Ctrl Pts',(2.10629101599995,5.2,-3.39386704700001));
#356464=CARTESIAN_POINT('Ctrl Pts',(2.10629101599995,2.2,-3.39386704700001));
#356465=CARTESIAN_POINT('Ctrl Pts',(2.10624268299994,12.2,-3.39378607900001));
#356466=CARTESIAN_POINT('Ctrl Pts',(2.10624268299994,5.2,-3.39378607900001));
#356467=CARTESIAN_POINT('Ctrl Pts',(2.10624268299994,2.2,-3.39378607900001));
#356468=CARTESIAN_POINT('Ctrl Pts',(2.10619797799994,12.2,-3.39371141900001));
#356469=CARTESIAN_POINT('Ctrl Pts',(2.10619797799994,5.2,-3.39371141900001));
#356470=CARTESIAN_POINT('Ctrl Pts',(2.10619797799994,2.2,-3.39371141900001));
#356471=CARTESIAN_POINT('Ctrl Pts',(2.10615692999994,12.2,-3.39364307200002));
#356472=CARTESIAN_POINT('Ctrl Pts',(2.10615692999994,5.2,-3.39364307200002));
#356473=CARTESIAN_POINT('Ctrl Pts',(2.10615692999994,2.2,-3.39364307200002));
#356474=CARTESIAN_POINT('Ctrl Pts',(2.10611957199994,12.2,-3.39358104500001));
#356475=CARTESIAN_POINT('Ctrl Pts',(2.10611957199994,5.2,-3.39358104500001));
#356476=CARTESIAN_POINT('Ctrl Pts',(2.10611957199994,2.2,-3.39358104500001));
#356477=CARTESIAN_POINT('Ctrl Pts',(2.10608593399995,12.2,-3.39352534100001));
#356478=CARTESIAN_POINT('Ctrl Pts',(2.10608593399995,5.2,-3.39352534100001));
#356479=CARTESIAN_POINT('Ctrl Pts',(2.10608593399995,2.2,-3.39352534100001));
#356480=CARTESIAN_POINT('Ctrl Pts',(2.10605603399994,12.2,-3.39347596500001));
#356481=CARTESIAN_POINT('Ctrl Pts',(2.10605603399994,5.2,-3.39347596500001));
#356482=CARTESIAN_POINT('Ctrl Pts',(2.10605603399994,2.2,-3.39347596500001));
#356483=CARTESIAN_POINT('Ctrl Pts',(2.10602708695768,12.2,-3.3934283110922));
#356484=CARTESIAN_POINT('Ctrl Pts',(2.10602708695768,5.2,-3.3934283110922));
#356485=CARTESIAN_POINT('Ctrl Pts',(2.10602708695768,2.2,-3.3934283110922));
#356486=CARTESIAN_POINT('Ctrl Pts',(2.106007235588,12.2,-3.39339577600012));
#356487=CARTESIAN_POINT('Ctrl Pts',(2.106007235588,5.2,-3.39339577600012));
#356488=CARTESIAN_POINT('Ctrl Pts',(2.106007235588,2.2,-3.39339577600012));
#356489=CARTESIAN_POINT('Ctrl Pts',(2.10599411145374,12.2,-3.3933743724075));
#356490=CARTESIAN_POINT('Ctrl Pts',(2.10599411145374,5.2,-3.3933743724075));
#356491=CARTESIAN_POINT('Ctrl Pts',(2.10599411145374,2.2,-3.3933743724075));
#356492=CARTESIAN_POINT('Ctrl Pts',(2.10598590620568,12.2,-3.39336105859039));
#356493=CARTESIAN_POINT('Ctrl Pts',(2.10598590620568,5.2,-3.39336105859039));
#356494=CARTESIAN_POINT('Ctrl Pts',(2.10598590620568,2.2,-3.39336105859039));
#356495=CARTESIAN_POINT('Ctrl Pts',(2.10598084399995,12.2,-3.39335283300001));
#356496=CARTESIAN_POINT('Ctrl Pts',(2.10598084399995,5.2,-3.39335283300001));
#356497=CARTESIAN_POINT('Ctrl Pts',(2.10598084399995,2.2,-3.39335283300001));
#356498=CARTESIAN_POINT('',(2.20867500599994,12.2,-4.20526511800002));
#356499=CARTESIAN_POINT('Origin',(-5.66300478732629E-14,15.2,-1.77635683940025E-14));
#356500=CARTESIAN_POINT('',(1.90498031899994,12.2,-4.35126992700001));
#356501=CARTESIAN_POINT('Ctrl Pts',(1.33499940099994,12.2,-3.76399239200001));
#356502=CARTESIAN_POINT('Ctrl Pts',(1.33499940099994,5.2,-3.76399239200001));
#356503=CARTESIAN_POINT('Ctrl Pts',(1.33499940099994,2.2,-3.76399239200001));
#356504=CARTESIAN_POINT('Ctrl Pts',(1.3350017138634,12.2,-3.76399883261967));
#356505=CARTESIAN_POINT('Ctrl Pts',(1.3350017138634,5.2,-3.76399883261967));
#356506=CARTESIAN_POINT('Ctrl Pts',(1.3350017138634,2.2,-3.76399883261967));
#356507=CARTESIAN_POINT('Ctrl Pts',(1.33500618571269,12.2,-3.76401128880897));
#356508=CARTESIAN_POINT('Ctrl Pts',(1.33500618571269,5.2,-3.76401128880897));
#356509=CARTESIAN_POINT('Ctrl Pts',(1.33500618571269,2.2,-3.76401128880897));
#356510=CARTESIAN_POINT('Ctrl Pts',(1.33501281737833,12.2,-3.76402975554743));
#356511=CARTESIAN_POINT('Ctrl Pts',(1.33501281737833,5.2,-3.76402975554743));
#356512=CARTESIAN_POINT('Ctrl Pts',(1.33501281737833,2.2,-3.76402975554743));
#356513=CARTESIAN_POINT('Ctrl Pts',(1.33502160885941,12.2,-3.76405426785898));
#356514=CARTESIAN_POINT('Ctrl Pts',(1.33502160885941,5.2,-3.76405426785898));
#356515=CARTESIAN_POINT('Ctrl Pts',(1.33502160885941,2.2,-3.76405426785898));
#356516=CARTESIAN_POINT('Ctrl Pts',(1.33503710099994,12.2,-3.76409681100002));
#356517=CARTESIAN_POINT('Ctrl Pts',(1.33503710099994,5.2,-3.76409681100002));
#356518=CARTESIAN_POINT('Ctrl Pts',(1.33503710099994,2.2,-3.76409681100002));
#356519=CARTESIAN_POINT('Ctrl Pts',(1.33505439099994,12.2,-3.76414411500001));
#356520=CARTESIAN_POINT('Ctrl Pts',(1.33505439099994,5.2,-3.76414411500001));
#356521=CARTESIAN_POINT('Ctrl Pts',(1.33505439099994,2.2,-3.76414411500001));
#356522=CARTESIAN_POINT('Ctrl Pts',(1.33507428099994,12.2,-3.76419830300001));
#356523=CARTESIAN_POINT('Ctrl Pts',(1.33507428099994,5.2,-3.76419830300001));
#356524=CARTESIAN_POINT('Ctrl Pts',(1.33507428099994,2.2,-3.76419830300001));
#356525=CARTESIAN_POINT('Ctrl Pts',(1.33509677799994,12.2,-3.76425936300001));
#356526=CARTESIAN_POINT('Ctrl Pts',(1.33509677799994,5.2,-3.76425936300001));
#356527=CARTESIAN_POINT('Ctrl Pts',(1.33509677799994,2.2,-3.76425936300001));
#356528=CARTESIAN_POINT('Ctrl Pts',(1.33512189099994,12.2,-3.76432727700001));
#356529=CARTESIAN_POINT('Ctrl Pts',(1.33512189099994,5.2,-3.76432727700001));
#356530=CARTESIAN_POINT('Ctrl Pts',(1.33512189099994,2.2,-3.76432727700001));
#356531=CARTESIAN_POINT('Ctrl Pts',(1.33514963499994,12.2,-3.76440201900001));
#356532=CARTESIAN_POINT('Ctrl Pts',(1.33514963499994,5.2,-3.76440201900001));
#356533=CARTESIAN_POINT('Ctrl Pts',(1.33514963499994,2.2,-3.76440201900001));
#356534=CARTESIAN_POINT('Ctrl Pts',(1.33518002599994,12.2,-3.76448356300001));
#356535=CARTESIAN_POINT('Ctrl Pts',(1.33518002599994,5.2,-3.76448356300001));
#356536=CARTESIAN_POINT('Ctrl Pts',(1.33518002599994,2.2,-3.76448356300001));
#356537=CARTESIAN_POINT('Ctrl Pts',(1.33521307799994,12.2,-3.76457187700002));
#356538=CARTESIAN_POINT('Ctrl Pts',(1.33521307799994,5.2,-3.76457187700002));
#356539=CARTESIAN_POINT('Ctrl Pts',(1.33521307799994,2.2,-3.76457187700002));
#356540=CARTESIAN_POINT('Ctrl Pts',(1.33524880699994,12.2,-3.76466693600001));
#356541=CARTESIAN_POINT('Ctrl Pts',(1.33524880699994,5.2,-3.76466693600001));
#356542=CARTESIAN_POINT('Ctrl Pts',(1.33524880699994,2.2,-3.76466693600001));
#356543=CARTESIAN_POINT('Ctrl Pts',(1.33528722599994,12.2,-3.76476871700001));
#356544=CARTESIAN_POINT('Ctrl Pts',(1.33528722599994,5.2,-3.76476871700001));
#356545=CARTESIAN_POINT('Ctrl Pts',(1.33528722599994,2.2,-3.76476871700001));
#356546=CARTESIAN_POINT('Ctrl Pts',(1.33532834499994,12.2,-3.76487719900001));
#356547=CARTESIAN_POINT('Ctrl Pts',(1.33532834499994,5.2,-3.76487719900001));
#356548=CARTESIAN_POINT('Ctrl Pts',(1.33532834499994,2.2,-3.76487719900001));
#356549=CARTESIAN_POINT('Ctrl Pts',(1.33537217499994,12.2,-3.76499236300001));
#356550=CARTESIAN_POINT('Ctrl Pts',(1.33537217499994,5.2,-3.76499236300001));
#356551=CARTESIAN_POINT('Ctrl Pts',(1.33537217499994,2.2,-3.76499236300001));
#356552=CARTESIAN_POINT('Ctrl Pts',(1.33541872699994,12.2,-3.76511418800002));
#356553=CARTESIAN_POINT('Ctrl Pts',(1.33541872699994,5.2,-3.76511418800002));
#356554=CARTESIAN_POINT('Ctrl Pts',(1.33541872699994,2.2,-3.76511418800002));
#356555=CARTESIAN_POINT('Ctrl Pts',(1.33546801399994,12.2,-3.76524265300001));
#356556=CARTESIAN_POINT('Ctrl Pts',(1.33546801399994,5.2,-3.76524265300001));
#356557=CARTESIAN_POINT('Ctrl Pts',(1.33546801399994,2.2,-3.76524265300001));
#356558=CARTESIAN_POINT('Ctrl Pts',(1.33552004599994,12.2,-3.76537773400001));
#356559=CARTESIAN_POINT('Ctrl Pts',(1.33552004599994,5.2,-3.76537773400001));
#356560=CARTESIAN_POINT('Ctrl Pts',(1.33552004599994,2.2,-3.76537773400001));
#356561=CARTESIAN_POINT('Ctrl Pts',(1.33557483799994,12.2,-3.76551940800002));
#356562=CARTESIAN_POINT('Ctrl Pts',(1.33557483799994,5.2,-3.76551940800002));
#356563=CARTESIAN_POINT('Ctrl Pts',(1.33557483799994,2.2,-3.76551940800002));
#356564=CARTESIAN_POINT('Ctrl Pts',(1.33563239999994,12.2,-3.76566765300002));
#356565=CARTESIAN_POINT('Ctrl Pts',(1.33563239999994,5.2,-3.76566765300002));
#356566=CARTESIAN_POINT('Ctrl Pts',(1.33563239999994,2.2,-3.76566765300002));
#356567=CARTESIAN_POINT('Ctrl Pts',(1.33569274599994,12.2,-3.76582244500002));
#356568=CARTESIAN_POINT('Ctrl Pts',(1.33569274599994,5.2,-3.76582244500002));
#356569=CARTESIAN_POINT('Ctrl Pts',(1.33569274599994,2.2,-3.76582244500002));
#356570=CARTESIAN_POINT('Ctrl Pts',(1.33575588799994,12.2,-3.76598376200001));
#356571=CARTESIAN_POINT('Ctrl Pts',(1.33575588799994,5.2,-3.76598376200001));
#356572=CARTESIAN_POINT('Ctrl Pts',(1.33575588799994,2.2,-3.76598376200001));
#356573=CARTESIAN_POINT('Ctrl Pts',(1.33582183599994,12.2,-3.76615158500002));
#356574=CARTESIAN_POINT('Ctrl Pts',(1.33582183599994,5.2,-3.76615158500002));
#356575=CARTESIAN_POINT('Ctrl Pts',(1.33582183599994,2.2,-3.76615158500002));
#356576=CARTESIAN_POINT('Ctrl Pts',(1.33589060099994,12.2,-3.76632588900002));
#356577=CARTESIAN_POINT('Ctrl Pts',(1.33589060099994,5.2,-3.76632588900002));
#356578=CARTESIAN_POINT('Ctrl Pts',(1.33589060099994,2.2,-3.76632588900002));
#356579=CARTESIAN_POINT('Ctrl Pts',(1.33596219699994,12.2,-3.76650665500001));
#356580=CARTESIAN_POINT('Ctrl Pts',(1.33596219699994,5.2,-3.76650665500001));
#356581=CARTESIAN_POINT('Ctrl Pts',(1.33596219699994,2.2,-3.76650665500001));
#356582=CARTESIAN_POINT('Ctrl Pts',(1.33603663199994,12.2,-3.76669386000001));
#356583=CARTESIAN_POINT('Ctrl Pts',(1.33603663199994,5.2,-3.76669386000001));
#356584=CARTESIAN_POINT('Ctrl Pts',(1.33603663199994,2.2,-3.76669386000001));
#356585=CARTESIAN_POINT('Ctrl Pts',(1.33611392099994,12.2,-3.76688748400001));
#356586=CARTESIAN_POINT('Ctrl Pts',(1.33611392099994,5.2,-3.76688748400001));
#356587=CARTESIAN_POINT('Ctrl Pts',(1.33611392099994,2.2,-3.76688748400001));
#356588=CARTESIAN_POINT('Ctrl Pts',(1.33619407199994,12.2,-3.76708750200001));
#356589=CARTESIAN_POINT('Ctrl Pts',(1.33619407199994,5.2,-3.76708750200001));
#356590=CARTESIAN_POINT('Ctrl Pts',(1.33619407199994,2.2,-3.76708750200001));
#356591=CARTESIAN_POINT('Ctrl Pts',(1.33627709999994,12.2,-3.76729389500001));
#356592=CARTESIAN_POINT('Ctrl Pts',(1.33627709999994,5.2,-3.76729389500001));
#356593=CARTESIAN_POINT('Ctrl Pts',(1.33627709999994,2.2,-3.76729389500001));
#356594=CARTESIAN_POINT('Ctrl Pts',(1.33636301299994,12.2,-3.76750664100001));
#356595=CARTESIAN_POINT('Ctrl Pts',(1.33636301299994,5.2,-3.76750664100001));
#356596=CARTESIAN_POINT('Ctrl Pts',(1.33636301299994,2.2,-3.76750664100001));
#356597=CARTESIAN_POINT('Ctrl Pts',(1.33645182399994,12.2,-3.76772571800001));
#356598=CARTESIAN_POINT('Ctrl Pts',(1.33645182399994,5.2,-3.76772571800001));
#356599=CARTESIAN_POINT('Ctrl Pts',(1.33645182399994,2.2,-3.76772571800001));
#356600=CARTESIAN_POINT('Ctrl Pts',(1.33654354399994,12.2,-3.76795110400002));
#356601=CARTESIAN_POINT('Ctrl Pts',(1.33654354399994,5.2,-3.76795110400002));
#356602=CARTESIAN_POINT('Ctrl Pts',(1.33654354399994,2.2,-3.76795110400002));
#356603=CARTESIAN_POINT('Ctrl Pts',(1.33663818299994,12.2,-3.76818277900002));
#356604=CARTESIAN_POINT('Ctrl Pts',(1.33663818299994,5.2,-3.76818277900002));
#356605=CARTESIAN_POINT('Ctrl Pts',(1.33663818299994,2.2,-3.76818277900002));
#356606=CARTESIAN_POINT('Ctrl Pts',(1.33673575299994,12.2,-3.76842072200001));
#356607=CARTESIAN_POINT('Ctrl Pts',(1.33673575299994,5.2,-3.76842072200001));
#356608=CARTESIAN_POINT('Ctrl Pts',(1.33673575299994,2.2,-3.76842072200001));
#356609=CARTESIAN_POINT('Ctrl Pts',(1.33683626499994,12.2,-3.76866491200001));
#356610=CARTESIAN_POINT('Ctrl Pts',(1.33683626499994,5.2,-3.76866491200001));
#356611=CARTESIAN_POINT('Ctrl Pts',(1.33683626499994,2.2,-3.76866491200001));
#356612=CARTESIAN_POINT('Ctrl Pts',(1.33693972899994,12.2,-3.76891532600002));
#356613=CARTESIAN_POINT('Ctrl Pts',(1.33693972899994,5.2,-3.76891532600002));
#356614=CARTESIAN_POINT('Ctrl Pts',(1.33693972899994,2.2,-3.76891532600002));
#356615=CARTESIAN_POINT('Ctrl Pts',(1.33704615599994,12.2,-3.76917194300002));
#356616=CARTESIAN_POINT('Ctrl Pts',(1.33704615599994,5.2,-3.76917194300002));
#356617=CARTESIAN_POINT('Ctrl Pts',(1.33704615599994,2.2,-3.76917194300002));
#356618=CARTESIAN_POINT('Ctrl Pts',(1.33715555799994,12.2,-3.76943474500001));
#356619=CARTESIAN_POINT('Ctrl Pts',(1.33715555799994,5.2,-3.76943474500001));
#356620=CARTESIAN_POINT('Ctrl Pts',(1.33715555799994,2.2,-3.76943474500001));
#356621=CARTESIAN_POINT('Ctrl Pts',(1.33726794299994,12.2,-3.76970370800001));
#356622=CARTESIAN_POINT('Ctrl Pts',(1.33726794299994,5.2,-3.76970370800001));
#356623=CARTESIAN_POINT('Ctrl Pts',(1.33726794299994,2.2,-3.76970370800001));
#356624=CARTESIAN_POINT('Ctrl Pts',(1.33738332499994,12.2,-3.76997881300001));
#356625=CARTESIAN_POINT('Ctrl Pts',(1.33738332499994,5.2,-3.76997881300001));
#356626=CARTESIAN_POINT('Ctrl Pts',(1.33738332499994,2.2,-3.76997881300001));
#356627=CARTESIAN_POINT('Ctrl Pts',(1.33750171199994,12.2,-3.77026003800002));
#356628=CARTESIAN_POINT('Ctrl Pts',(1.33750171199994,5.2,-3.77026003800002));
#356629=CARTESIAN_POINT('Ctrl Pts',(1.33750171199994,2.2,-3.77026003800002));
#356630=CARTESIAN_POINT('Ctrl Pts',(1.33762311599994,12.2,-3.77054736200002));
#356631=CARTESIAN_POINT('Ctrl Pts',(1.33762311599994,5.2,-3.77054736200002));
#356632=CARTESIAN_POINT('Ctrl Pts',(1.33762311599994,2.2,-3.77054736200002));
#356633=CARTESIAN_POINT('Ctrl Pts',(1.33774754599994,12.2,-3.77084076600001));
#356634=CARTESIAN_POINT('Ctrl Pts',(1.33774754599994,5.2,-3.77084076600001));
#356635=CARTESIAN_POINT('Ctrl Pts',(1.33774754599994,2.2,-3.77084076600001));
#356636=CARTESIAN_POINT('Ctrl Pts',(1.33787501399994,12.2,-3.77114022700002));
#356637=CARTESIAN_POINT('Ctrl Pts',(1.33787501399994,5.2,-3.77114022700002));
#356638=CARTESIAN_POINT('Ctrl Pts',(1.33787501399994,2.2,-3.77114022700002));
#356639=CARTESIAN_POINT('Ctrl Pts',(1.33800552899994,12.2,-3.77144572600002));
#356640=CARTESIAN_POINT('Ctrl Pts',(1.33800552899994,5.2,-3.77144572600002));
#356641=CARTESIAN_POINT('Ctrl Pts',(1.33800552899994,2.2,-3.77144572600002));
#356642=CARTESIAN_POINT('Ctrl Pts',(1.33813910099994,12.2,-3.77175724400002));
#356643=CARTESIAN_POINT('Ctrl Pts',(1.33813910099994,5.2,-3.77175724400002));
#356644=CARTESIAN_POINT('Ctrl Pts',(1.33813910099994,2.2,-3.77175724400002));
#356645=CARTESIAN_POINT('Ctrl Pts',(1.33827574299994,12.2,-3.77207475700001));
#356646=CARTESIAN_POINT('Ctrl Pts',(1.33827574299994,5.2,-3.77207475700001));
#356647=CARTESIAN_POINT('Ctrl Pts',(1.33827574299994,2.2,-3.77207475700001));
#356648=CARTESIAN_POINT('Ctrl Pts',(1.33841546199994,12.2,-3.77239824600001));
#356649=CARTESIAN_POINT('Ctrl Pts',(1.33841546199994,5.2,-3.77239824600001));
#356650=CARTESIAN_POINT('Ctrl Pts',(1.33841546199994,2.2,-3.77239824600001));
#356651=CARTESIAN_POINT('Ctrl Pts',(1.33855826899994,12.2,-3.77272769200002));
#356652=CARTESIAN_POINT('Ctrl Pts',(1.33855826899994,5.2,-3.77272769200002));
#356653=CARTESIAN_POINT('Ctrl Pts',(1.33855826899994,2.2,-3.77272769200002));
#356654=CARTESIAN_POINT('Ctrl Pts',(1.33870417499994,12.2,-3.77306307200001));
#356655=CARTESIAN_POINT('Ctrl Pts',(1.33870417499994,5.2,-3.77306307200001));
#356656=CARTESIAN_POINT('Ctrl Pts',(1.33870417499994,2.2,-3.77306307200001));
#356657=CARTESIAN_POINT('Ctrl Pts',(1.33885318899994,12.2,-3.77340436900001));
#356658=CARTESIAN_POINT('Ctrl Pts',(1.33885318899994,5.2,-3.77340436900001));
#356659=CARTESIAN_POINT('Ctrl Pts',(1.33885318899994,2.2,-3.77340436900001));
#356660=CARTESIAN_POINT('Ctrl Pts',(1.33900532099994,12.2,-3.77375156100001));
#356661=CARTESIAN_POINT('Ctrl Pts',(1.33900532099994,5.2,-3.77375156100001));
#356662=CARTESIAN_POINT('Ctrl Pts',(1.33900532099994,2.2,-3.77375156100001));
#356663=CARTESIAN_POINT('Ctrl Pts',(1.33916058199994,12.2,-3.77410462700002));
#356664=CARTESIAN_POINT('Ctrl Pts',(1.33916058199994,5.2,-3.77410462700002));
#356665=CARTESIAN_POINT('Ctrl Pts',(1.33916058199994,2.2,-3.77410462700002));
#356666=CARTESIAN_POINT('Ctrl Pts',(1.33931897899994,12.2,-3.77446354900002));
#356667=CARTESIAN_POINT('Ctrl Pts',(1.33931897899994,5.2,-3.77446354900002));
#356668=CARTESIAN_POINT('Ctrl Pts',(1.33931897899994,2.2,-3.77446354900002));
#356669=CARTESIAN_POINT('Ctrl Pts',(1.33948052599994,12.2,-3.77482830500002));
#356670=CARTESIAN_POINT('Ctrl Pts',(1.33948052599994,5.2,-3.77482830500002));
#356671=CARTESIAN_POINT('Ctrl Pts',(1.33948052599994,2.2,-3.77482830500002));
#356672=CARTESIAN_POINT('Ctrl Pts',(1.33964522999994,12.2,-3.77519887600001));
#356673=CARTESIAN_POINT('Ctrl Pts',(1.33964522999994,5.2,-3.77519887600001));
#356674=CARTESIAN_POINT('Ctrl Pts',(1.33964522999994,2.2,-3.77519887600001));
#356675=CARTESIAN_POINT('Ctrl Pts',(1.33981309999994,12.2,-3.77557524300002));
#356676=CARTESIAN_POINT('Ctrl Pts',(1.33981309999994,5.2,-3.77557524300002));
#356677=CARTESIAN_POINT('Ctrl Pts',(1.33981309999994,2.2,-3.77557524300002));
#356678=CARTESIAN_POINT('Ctrl Pts',(1.33998414699994,12.2,-3.77595738500001));
#356679=CARTESIAN_POINT('Ctrl Pts',(1.33998414699994,5.2,-3.77595738500001));
#356680=CARTESIAN_POINT('Ctrl Pts',(1.33998414699994,2.2,-3.77595738500001));
#356681=CARTESIAN_POINT('Ctrl Pts',(1.34015838099994,12.2,-3.77634528200002));
#356682=CARTESIAN_POINT('Ctrl Pts',(1.34015838099994,5.2,-3.77634528200002));
#356683=CARTESIAN_POINT('Ctrl Pts',(1.34015838099994,2.2,-3.77634528200002));
#356684=CARTESIAN_POINT('Ctrl Pts',(1.34033580999994,12.2,-3.77673891500002));
#356685=CARTESIAN_POINT('Ctrl Pts',(1.34033580999994,5.2,-3.77673891500002));
#356686=CARTESIAN_POINT('Ctrl Pts',(1.34033580999994,2.2,-3.77673891500002));
#356687=CARTESIAN_POINT('Ctrl Pts',(1.34051644399994,12.2,-3.77713826300001));
#356688=CARTESIAN_POINT('Ctrl Pts',(1.34051644399994,5.2,-3.77713826300001));
#356689=CARTESIAN_POINT('Ctrl Pts',(1.34051644399994,2.2,-3.77713826300001));
#356690=CARTESIAN_POINT('Ctrl Pts',(1.34070029299994,12.2,-3.77754330800002));
#356691=CARTESIAN_POINT('Ctrl Pts',(1.34070029299994,5.2,-3.77754330800002));
#356692=CARTESIAN_POINT('Ctrl Pts',(1.34070029299994,2.2,-3.77754330800002));
#356693=CARTESIAN_POINT('Ctrl Pts',(1.34088736599994,12.2,-3.77795402900002));
#356694=CARTESIAN_POINT('Ctrl Pts',(1.34088736599994,5.2,-3.77795402900002));
#356695=CARTESIAN_POINT('Ctrl Pts',(1.34088736599994,2.2,-3.77795402900002));
#356696=CARTESIAN_POINT('Ctrl Pts',(1.34107767199994,12.2,-3.77837040700001));
#356697=CARTESIAN_POINT('Ctrl Pts',(1.34107767199994,5.2,-3.77837040700001));
#356698=CARTESIAN_POINT('Ctrl Pts',(1.34107767199994,2.2,-3.77837040700001));
#356699=CARTESIAN_POINT('Ctrl Pts',(1.34127121999994,12.2,-3.77879242300001));
#356700=CARTESIAN_POINT('Ctrl Pts',(1.34127121999994,5.2,-3.77879242300001));
#356701=CARTESIAN_POINT('Ctrl Pts',(1.34127121999994,2.2,-3.77879242300001));
#356702=CARTESIAN_POINT('Ctrl Pts',(1.34146801999994,12.2,-3.77922005700002));
#356703=CARTESIAN_POINT('Ctrl Pts',(1.34146801999994,5.2,-3.77922005700002));
#356704=CARTESIAN_POINT('Ctrl Pts',(1.34146801999994,2.2,-3.77922005700002));
#356705=CARTESIAN_POINT('Ctrl Pts',(1.34166807999994,12.2,-3.77965329000002));
#356706=CARTESIAN_POINT('Ctrl Pts',(1.34166807999994,5.2,-3.77965329000002));
#356707=CARTESIAN_POINT('Ctrl Pts',(1.34166807999994,2.2,-3.77965329000002));
#356708=CARTESIAN_POINT('Ctrl Pts',(1.34187141099994,12.2,-3.78009210100001));
#356709=CARTESIAN_POINT('Ctrl Pts',(1.34187141099994,5.2,-3.78009210100001));
#356710=CARTESIAN_POINT('Ctrl Pts',(1.34187141099994,2.2,-3.78009210100001));
#356711=CARTESIAN_POINT('Ctrl Pts',(1.34207802099994,12.2,-3.78053647300002));
#356712=CARTESIAN_POINT('Ctrl Pts',(1.34207802099994,5.2,-3.78053647300002));
#356713=CARTESIAN_POINT('Ctrl Pts',(1.34207802099994,2.2,-3.78053647300002));
#356714=CARTESIAN_POINT('Ctrl Pts',(1.34228791699994,12.2,-3.78098638700001));
#356715=CARTESIAN_POINT('Ctrl Pts',(1.34228791699994,5.2,-3.78098638700001));
#356716=CARTESIAN_POINT('Ctrl Pts',(1.34228791699994,2.2,-3.78098638700001));
#356717=CARTESIAN_POINT('Ctrl Pts',(1.34250111099994,12.2,-3.78144182100002));
#356718=CARTESIAN_POINT('Ctrl Pts',(1.34250111099994,5.2,-3.78144182100002));
#356719=CARTESIAN_POINT('Ctrl Pts',(1.34250111099994,2.2,-3.78144182100002));
#356720=CARTESIAN_POINT('Ctrl Pts',(1.34271760999994,12.2,-3.78190275800002));
#356721=CARTESIAN_POINT('Ctrl Pts',(1.34271760999994,5.2,-3.78190275800002));
#356722=CARTESIAN_POINT('Ctrl Pts',(1.34271760999994,2.2,-3.78190275800002));
#356723=CARTESIAN_POINT('Ctrl Pts',(1.34293742399994,12.2,-3.78236917900002));
#356724=CARTESIAN_POINT('Ctrl Pts',(1.34293742399994,5.2,-3.78236917900002));
#356725=CARTESIAN_POINT('Ctrl Pts',(1.34293742399994,2.2,-3.78236917900002));
#356726=CARTESIAN_POINT('Ctrl Pts',(1.34316056099994,12.2,-3.78284106400002));
#356727=CARTESIAN_POINT('Ctrl Pts',(1.34316056099994,5.2,-3.78284106400002));
#356728=CARTESIAN_POINT('Ctrl Pts',(1.34316056099994,2.2,-3.78284106400002));
#356729=CARTESIAN_POINT('Ctrl Pts',(1.34338702999994,12.2,-3.78331839300001));
#356730=CARTESIAN_POINT('Ctrl Pts',(1.34338702999994,5.2,-3.78331839300001));
#356731=CARTESIAN_POINT('Ctrl Pts',(1.34338702999994,2.2,-3.78331839300001));
#356732=CARTESIAN_POINT('Ctrl Pts',(1.34361683999994,12.2,-3.78380114900001));
#356733=CARTESIAN_POINT('Ctrl Pts',(1.34361683999994,5.2,-3.78380114900001));
#356734=CARTESIAN_POINT('Ctrl Pts',(1.34361683999994,2.2,-3.78380114900001));
#356735=CARTESIAN_POINT('Ctrl Pts',(1.34384999799994,12.2,-3.78428931300002));
#356736=CARTESIAN_POINT('Ctrl Pts',(1.34384999799994,5.2,-3.78428931300002));
#356737=CARTESIAN_POINT('Ctrl Pts',(1.34384999799994,2.2,-3.78428931300002));
#356738=CARTESIAN_POINT('Ctrl Pts',(1.34408651399994,12.2,-3.78478286600001));
#356739=CARTESIAN_POINT('Ctrl Pts',(1.34408651399994,5.2,-3.78478286600001));
#356740=CARTESIAN_POINT('Ctrl Pts',(1.34408651399994,2.2,-3.78478286600001));
#356741=CARTESIAN_POINT('Ctrl Pts',(1.34432639799994,12.2,-3.78528178900002));
#356742=CARTESIAN_POINT('Ctrl Pts',(1.34432639799994,5.2,-3.78528178900002));
#356743=CARTESIAN_POINT('Ctrl Pts',(1.34432639799994,2.2,-3.78528178900002));
#356744=CARTESIAN_POINT('Ctrl Pts',(1.34456965499994,12.2,-3.78578606200001));
#356745=CARTESIAN_POINT('Ctrl Pts',(1.34456965499994,5.2,-3.78578606200001));
#356746=CARTESIAN_POINT('Ctrl Pts',(1.34456965499994,2.2,-3.78578606200001));
#356747=CARTESIAN_POINT('Ctrl Pts',(1.34481629599994,12.2,-3.78629566700001));
#356748=CARTESIAN_POINT('Ctrl Pts',(1.34481629599994,5.2,-3.78629566700001));
#356749=CARTESIAN_POINT('Ctrl Pts',(1.34481629599994,2.2,-3.78629566700001));
#356750=CARTESIAN_POINT('Ctrl Pts',(1.34506632799994,12.2,-3.78681058700002));
#356751=CARTESIAN_POINT('Ctrl Pts',(1.34506632799994,5.2,-3.78681058700002));
#356752=CARTESIAN_POINT('Ctrl Pts',(1.34506632799994,2.2,-3.78681058700002));
#356753=CARTESIAN_POINT('Ctrl Pts',(1.34531975999994,12.2,-3.78733080100002));
#356754=CARTESIAN_POINT('Ctrl Pts',(1.34531975999994,5.2,-3.78733080100002));
#356755=CARTESIAN_POINT('Ctrl Pts',(1.34531975999994,2.2,-3.78733080100002));
#356756=CARTESIAN_POINT('Ctrl Pts',(1.34557660099994,12.2,-3.78785629200001));
#356757=CARTESIAN_POINT('Ctrl Pts',(1.34557660099994,5.2,-3.78785629200001));
#356758=CARTESIAN_POINT('Ctrl Pts',(1.34557660099994,2.2,-3.78785629200001));
#356759=CARTESIAN_POINT('Ctrl Pts',(1.34583685899994,12.2,-3.78838704100001));
#356760=CARTESIAN_POINT('Ctrl Pts',(1.34583685899994,5.2,-3.78838704100001));
#356761=CARTESIAN_POINT('Ctrl Pts',(1.34583685899994,2.2,-3.78838704100001));
#356762=CARTESIAN_POINT('Ctrl Pts',(1.34610053999994,12.2,-3.78892302900002));
#356763=CARTESIAN_POINT('Ctrl Pts',(1.34610053999994,5.2,-3.78892302900002));
#356764=CARTESIAN_POINT('Ctrl Pts',(1.34610053999994,2.2,-3.78892302900002));
#356765=CARTESIAN_POINT('Ctrl Pts',(1.34636765499994,12.2,-3.78946423800001));
#356766=CARTESIAN_POINT('Ctrl Pts',(1.34636765499994,5.2,-3.78946423800001));
#356767=CARTESIAN_POINT('Ctrl Pts',(1.34636765499994,2.2,-3.78946423800001));
#356768=CARTESIAN_POINT('Ctrl Pts',(1.34663820999994,12.2,-3.79001065000002));
#356769=CARTESIAN_POINT('Ctrl Pts',(1.34663820999994,5.2,-3.79001065000002));
#356770=CARTESIAN_POINT('Ctrl Pts',(1.34663820999994,2.2,-3.79001065000002));
#356771=CARTESIAN_POINT('Ctrl Pts',(1.34691221499994,12.2,-3.79056224700001));
#356772=CARTESIAN_POINT('Ctrl Pts',(1.34691221499994,5.2,-3.79056224700001));
#356773=CARTESIAN_POINT('Ctrl Pts',(1.34691221499994,2.2,-3.79056224700001));
#356774=CARTESIAN_POINT('Ctrl Pts',(1.34718967599994,12.2,-3.79111900900002));
#356775=CARTESIAN_POINT('Ctrl Pts',(1.34718967599994,5.2,-3.79111900900002));
#356776=CARTESIAN_POINT('Ctrl Pts',(1.34718967599994,2.2,-3.79111900900002));
#356777=CARTESIAN_POINT('Ctrl Pts',(1.34747060299994,12.2,-3.79168091900001));
#356778=CARTESIAN_POINT('Ctrl Pts',(1.34747060299994,5.2,-3.79168091900001));
#356779=CARTESIAN_POINT('Ctrl Pts',(1.34747060299994,2.2,-3.79168091900001));
#356780=CARTESIAN_POINT('Ctrl Pts',(1.34775500299994,12.2,-3.79224795900001));
#356781=CARTESIAN_POINT('Ctrl Pts',(1.34775500299994,5.2,-3.79224795900001));
#356782=CARTESIAN_POINT('Ctrl Pts',(1.34775500299994,2.2,-3.79224795900001));
#356783=CARTESIAN_POINT('Ctrl Pts',(1.34804288399994,12.2,-3.79282010900001));
#356784=CARTESIAN_POINT('Ctrl Pts',(1.34804288399994,5.2,-3.79282010900001));
#356785=CARTESIAN_POINT('Ctrl Pts',(1.34804288399994,2.2,-3.79282010900001));
#356786=CARTESIAN_POINT('Ctrl Pts',(1.34833425199994,12.2,-3.79339735300002));
#356787=CARTESIAN_POINT('Ctrl Pts',(1.34833425199994,5.2,-3.79339735300002));
#356788=CARTESIAN_POINT('Ctrl Pts',(1.34833425199994,2.2,-3.79339735300002));
#356789=CARTESIAN_POINT('Ctrl Pts',(1.34862911799994,12.2,-3.79397967200001));
#356790=CARTESIAN_POINT('Ctrl Pts',(1.34862911799994,5.2,-3.79397967200001));
#356791=CARTESIAN_POINT('Ctrl Pts',(1.34862911799994,2.2,-3.79397967200001));
#356792=CARTESIAN_POINT('Ctrl Pts',(1.34892748699994,12.2,-3.79456704900001));
#356793=CARTESIAN_POINT('Ctrl Pts',(1.34892748699994,5.2,-3.79456704900001));
#356794=CARTESIAN_POINT('Ctrl Pts',(1.34892748699994,2.2,-3.79456704900001));
#356795=CARTESIAN_POINT('Ctrl Pts',(1.34922936899994,12.2,-3.79515946400002));
#356796=CARTESIAN_POINT('Ctrl Pts',(1.34922936899994,5.2,-3.79515946400002));
#356797=CARTESIAN_POINT('Ctrl Pts',(1.34922936899994,2.2,-3.79515946400002));
#356798=CARTESIAN_POINT('Ctrl Pts',(1.34953476899994,12.2,-3.79575690100001));
#356799=CARTESIAN_POINT('Ctrl Pts',(1.34953476899994,5.2,-3.79575690100001));
#356800=CARTESIAN_POINT('Ctrl Pts',(1.34953476899994,2.2,-3.79575690100001));
#356801=CARTESIAN_POINT('Ctrl Pts',(1.34984369799994,12.2,-3.79635934100001));
#356802=CARTESIAN_POINT('Ctrl Pts',(1.34984369799994,5.2,-3.79635934100001));
#356803=CARTESIAN_POINT('Ctrl Pts',(1.34984369799994,2.2,-3.79635934100001));
#356804=CARTESIAN_POINT('Ctrl Pts',(1.35015615999994,12.2,-3.79696676700001));
#356805=CARTESIAN_POINT('Ctrl Pts',(1.35015615999994,5.2,-3.79696676700001));
#356806=CARTESIAN_POINT('Ctrl Pts',(1.35015615999994,2.2,-3.79696676700001));
#356807=CARTESIAN_POINT('Ctrl Pts',(1.35047216499994,12.2,-3.79757915900001));
#356808=CARTESIAN_POINT('Ctrl Pts',(1.35047216499994,5.2,-3.79757915900001));
#356809=CARTESIAN_POINT('Ctrl Pts',(1.35047216499994,2.2,-3.79757915900001));
#356810=CARTESIAN_POINT('Ctrl Pts',(1.35079171899994,12.2,-3.79819650200002));
#356811=CARTESIAN_POINT('Ctrl Pts',(1.35079171899994,5.2,-3.79819650200002));
#356812=CARTESIAN_POINT('Ctrl Pts',(1.35079171899994,2.2,-3.79819650200002));
#356813=CARTESIAN_POINT('Ctrl Pts',(1.35111483199994,12.2,-3.79881877700001));
#356814=CARTESIAN_POINT('Ctrl Pts',(1.35111483199994,5.2,-3.79881877700001));
#356815=CARTESIAN_POINT('Ctrl Pts',(1.35111483199994,2.2,-3.79881877700001));
#356816=CARTESIAN_POINT('Ctrl Pts',(1.35144150699994,12.2,-3.79944596600001));
#356817=CARTESIAN_POINT('Ctrl Pts',(1.35144150699994,5.2,-3.79944596600001));
#356818=CARTESIAN_POINT('Ctrl Pts',(1.35144150699994,2.2,-3.79944596600001));
#356819=CARTESIAN_POINT('Ctrl Pts',(1.35177175599994,12.2,-3.80007805200002));
#356820=CARTESIAN_POINT('Ctrl Pts',(1.35177175599994,5.2,-3.80007805200002));
#356821=CARTESIAN_POINT('Ctrl Pts',(1.35177175599994,2.2,-3.80007805200002));
#356822=CARTESIAN_POINT('Ctrl Pts',(1.35210558299994,12.2,-3.80071501700002));
#356823=CARTESIAN_POINT('Ctrl Pts',(1.35210558299994,5.2,-3.80071501700002));
#356824=CARTESIAN_POINT('Ctrl Pts',(1.35210558299994,2.2,-3.80071501700002));
#356825=CARTESIAN_POINT('Ctrl Pts',(1.35244299699994,12.2,-3.80135684400001));
#356826=CARTESIAN_POINT('Ctrl Pts',(1.35244299699994,5.2,-3.80135684400001));
#356827=CARTESIAN_POINT('Ctrl Pts',(1.35244299699994,2.2,-3.80135684400001));
#356828=CARTESIAN_POINT('Ctrl Pts',(1.35278400499994,12.2,-3.80200351400001));
#356829=CARTESIAN_POINT('Ctrl Pts',(1.35278400499994,5.2,-3.80200351400001));
#356830=CARTESIAN_POINT('Ctrl Pts',(1.35278400499994,2.2,-3.80200351400001));
#356831=CARTESIAN_POINT('Ctrl Pts',(1.35312861199994,12.2,-3.80265501100002));
#356832=CARTESIAN_POINT('Ctrl Pts',(1.35312861199994,5.2,-3.80265501100002));
#356833=CARTESIAN_POINT('Ctrl Pts',(1.35312861199994,2.2,-3.80265501100002));
#356834=CARTESIAN_POINT('Ctrl Pts',(1.35347682899994,12.2,-3.80331131700002));
#356835=CARTESIAN_POINT('Ctrl Pts',(1.35347682899994,5.2,-3.80331131700002));
#356836=CARTESIAN_POINT('Ctrl Pts',(1.35347682899994,2.2,-3.80331131700002));
#356837=CARTESIAN_POINT('Ctrl Pts',(1.35382865999994,12.2,-3.80397241500001));
#356838=CARTESIAN_POINT('Ctrl Pts',(1.35382865999994,5.2,-3.80397241500001));
#356839=CARTESIAN_POINT('Ctrl Pts',(1.35382865999994,2.2,-3.80397241500001));
#356840=CARTESIAN_POINT('Ctrl Pts',(1.35418411299994,12.2,-3.80463828700002));
#356841=CARTESIAN_POINT('Ctrl Pts',(1.35418411299994,5.2,-3.80463828700002));
#356842=CARTESIAN_POINT('Ctrl Pts',(1.35418411299994,2.2,-3.80463828700002));
#356843=CARTESIAN_POINT('Ctrl Pts',(1.35454319599994,12.2,-3.80530891600001));
#356844=CARTESIAN_POINT('Ctrl Pts',(1.35454319599994,5.2,-3.80530891600001));
#356845=CARTESIAN_POINT('Ctrl Pts',(1.35454319599994,2.2,-3.80530891600001));
#356846=CARTESIAN_POINT('Ctrl Pts',(1.35490591599994,12.2,-3.80598428600001));
#356847=CARTESIAN_POINT('Ctrl Pts',(1.35490591599994,5.2,-3.80598428600001));
#356848=CARTESIAN_POINT('Ctrl Pts',(1.35490591599994,2.2,-3.80598428600001));
#356849=CARTESIAN_POINT('Ctrl Pts',(1.35527227699994,12.2,-3.80666437600001));
#356850=CARTESIAN_POINT('Ctrl Pts',(1.35527227699994,5.2,-3.80666437600001));
#356851=CARTESIAN_POINT('Ctrl Pts',(1.35527227699994,2.2,-3.80666437600001));
#356852=CARTESIAN_POINT('Ctrl Pts',(1.35564228799994,12.2,-3.80734917300002));
#356853=CARTESIAN_POINT('Ctrl Pts',(1.35564228799994,5.2,-3.80734917300002));
#356854=CARTESIAN_POINT('Ctrl Pts',(1.35564228799994,2.2,-3.80734917300002));
#356855=CARTESIAN_POINT('Ctrl Pts',(1.35601595799994,12.2,-3.80803865800001));
#356856=CARTESIAN_POINT('Ctrl Pts',(1.35601595799994,5.2,-3.80803865800001));
#356857=CARTESIAN_POINT('Ctrl Pts',(1.35601595799994,2.2,-3.80803865800001));
#356858=CARTESIAN_POINT('Ctrl Pts',(1.35639328999994,12.2,-3.80873281300001));
#356859=CARTESIAN_POINT('Ctrl Pts',(1.35639328999994,5.2,-3.80873281300001));
#356860=CARTESIAN_POINT('Ctrl Pts',(1.35639328999994,2.2,-3.80873281300001));
#356861=CARTESIAN_POINT('Ctrl Pts',(1.35677429299994,12.2,-3.80943162300001));
#356862=CARTESIAN_POINT('Ctrl Pts',(1.35677429299994,5.2,-3.80943162300001));
#356863=CARTESIAN_POINT('Ctrl Pts',(1.35677429299994,2.2,-3.80943162300001));
#356864=CARTESIAN_POINT('Ctrl Pts',(1.35715897299994,12.2,-3.81013506900001));
#356865=CARTESIAN_POINT('Ctrl Pts',(1.35715897299994,5.2,-3.81013506900001));
#356866=CARTESIAN_POINT('Ctrl Pts',(1.35715897299994,2.2,-3.81013506900001));
#356867=CARTESIAN_POINT('Ctrl Pts',(1.35754733699994,12.2,-3.81084313500001));
#356868=CARTESIAN_POINT('Ctrl Pts',(1.35754733699994,5.2,-3.81084313500001));
#356869=CARTESIAN_POINT('Ctrl Pts',(1.35754733699994,2.2,-3.81084313500001));
#356870=CARTESIAN_POINT('Ctrl Pts',(1.35793939099994,12.2,-3.81155580400002));
#356871=CARTESIAN_POINT('Ctrl Pts',(1.35793939099994,5.2,-3.81155580400002));
#356872=CARTESIAN_POINT('Ctrl Pts',(1.35793939099994,2.2,-3.81155580400002));
#356873=CARTESIAN_POINT('Ctrl Pts',(1.35833514199994,12.2,-3.81227305800001));
#356874=CARTESIAN_POINT('Ctrl Pts',(1.35833514199994,5.2,-3.81227305800001));
#356875=CARTESIAN_POINT('Ctrl Pts',(1.35833514199994,2.2,-3.81227305800001));
#356876=CARTESIAN_POINT('Ctrl Pts',(1.35873459799994,12.2,-3.81299488200002));
#356877=CARTESIAN_POINT('Ctrl Pts',(1.35873459799994,5.2,-3.81299488200002));
#356878=CARTESIAN_POINT('Ctrl Pts',(1.35873459799994,2.2,-3.81299488200002));
#356879=CARTESIAN_POINT('Ctrl Pts',(1.35913776399994,12.2,-3.81372125800001));
#356880=CARTESIAN_POINT('Ctrl Pts',(1.35913776399994,5.2,-3.81372125800001));
#356881=CARTESIAN_POINT('Ctrl Pts',(1.35913776399994,2.2,-3.81372125800001));
#356882=CARTESIAN_POINT('Ctrl Pts',(1.35954464599994,12.2,-3.81445216800001));
#356883=CARTESIAN_POINT('Ctrl Pts',(1.35954464599994,5.2,-3.81445216800001));
#356884=CARTESIAN_POINT('Ctrl Pts',(1.35954464599994,2.2,-3.81445216800001));
#356885=CARTESIAN_POINT('Ctrl Pts',(1.35995525099994,12.2,-3.81518759900001));
#356886=CARTESIAN_POINT('Ctrl Pts',(1.35995525099994,5.2,-3.81518759900001));
#356887=CARTESIAN_POINT('Ctrl Pts',(1.35995525099994,2.2,-3.81518759900001));
#356888=CARTESIAN_POINT('Ctrl Pts',(1.36036958699994,12.2,-3.81592753000001));
#356889=CARTESIAN_POINT('Ctrl Pts',(1.36036958699994,5.2,-3.81592753000001));
#356890=CARTESIAN_POINT('Ctrl Pts',(1.36036958699994,2.2,-3.81592753000001));
#356891=CARTESIAN_POINT('Ctrl Pts',(1.36078765799994,12.2,-3.81667194600002));
#356892=CARTESIAN_POINT('Ctrl Pts',(1.36078765799994,5.2,-3.81667194600002));
#356893=CARTESIAN_POINT('Ctrl Pts',(1.36078765799994,2.2,-3.81667194600002));
#356894=CARTESIAN_POINT('Ctrl Pts',(1.36120947099994,12.2,-3.81742083100002));
#356895=CARTESIAN_POINT('Ctrl Pts',(1.36120947099994,5.2,-3.81742083100002));
#356896=CARTESIAN_POINT('Ctrl Pts',(1.36120947099994,2.2,-3.81742083100002));
#356897=CARTESIAN_POINT('Ctrl Pts',(1.36163503399994,12.2,-3.81817416700001));
#356898=CARTESIAN_POINT('Ctrl Pts',(1.36163503399994,5.2,-3.81817416700001));
#356899=CARTESIAN_POINT('Ctrl Pts',(1.36163503399994,2.2,-3.81817416700001));
#356900=CARTESIAN_POINT('Ctrl Pts',(1.36206435199994,12.2,-3.81893193900002));
#356901=CARTESIAN_POINT('Ctrl Pts',(1.36206435199994,5.2,-3.81893193900002));
#356902=CARTESIAN_POINT('Ctrl Pts',(1.36206435199994,2.2,-3.81893193900002));
#356903=CARTESIAN_POINT('Ctrl Pts',(1.36249743099994,12.2,-3.81969412900002));
#356904=CARTESIAN_POINT('Ctrl Pts',(1.36249743099994,5.2,-3.81969412900002));
#356905=CARTESIAN_POINT('Ctrl Pts',(1.36249743099994,2.2,-3.81969412900002));
#356906=CARTESIAN_POINT('Ctrl Pts',(1.36293427699994,12.2,-3.82046072100001));
#356907=CARTESIAN_POINT('Ctrl Pts',(1.36293427699994,5.2,-3.82046072100001));
#356908=CARTESIAN_POINT('Ctrl Pts',(1.36293427699994,2.2,-3.82046072100001));
#356909=CARTESIAN_POINT('Ctrl Pts',(1.36337489599994,12.2,-3.82123169900002));
#356910=CARTESIAN_POINT('Ctrl Pts',(1.36337489599994,5.2,-3.82123169900002));
#356911=CARTESIAN_POINT('Ctrl Pts',(1.36337489599994,2.2,-3.82123169900002));
#356912=CARTESIAN_POINT('Ctrl Pts',(1.36381929499994,12.2,-3.82200704600002));
#356913=CARTESIAN_POINT('Ctrl Pts',(1.36381929499994,5.2,-3.82200704600002));
#356914=CARTESIAN_POINT('Ctrl Pts',(1.36381929499994,2.2,-3.82200704600002));
#356915=CARTESIAN_POINT('Ctrl Pts',(1.36426748099994,12.2,-3.82278674500002));
#356916=CARTESIAN_POINT('Ctrl Pts',(1.36426748099994,5.2,-3.82278674500002));
#356917=CARTESIAN_POINT('Ctrl Pts',(1.36426748099994,2.2,-3.82278674500002));
#356918=CARTESIAN_POINT('Ctrl Pts',(1.36471945699994,12.2,-3.82357078100001));
#356919=CARTESIAN_POINT('Ctrl Pts',(1.36471945699994,5.2,-3.82357078100001));
#356920=CARTESIAN_POINT('Ctrl Pts',(1.36471945699994,2.2,-3.82357078100001));
#356921=CARTESIAN_POINT('Ctrl Pts',(1.36517523299994,12.2,-3.82435913800002));
#356922=CARTESIAN_POINT('Ctrl Pts',(1.36517523299994,5.2,-3.82435913800002));
#356923=CARTESIAN_POINT('Ctrl Pts',(1.36517523299994,2.2,-3.82435913800002));
#356924=CARTESIAN_POINT('Ctrl Pts',(1.36563481099994,12.2,-3.82515179700002));
#356925=CARTESIAN_POINT('Ctrl Pts',(1.36563481099994,5.2,-3.82515179700002));
#356926=CARTESIAN_POINT('Ctrl Pts',(1.36563481099994,2.2,-3.82515179700002));
#356927=CARTESIAN_POINT('Ctrl Pts',(1.36609819999994,12.2,-3.82594874400001));
#356928=CARTESIAN_POINT('Ctrl Pts',(1.36609819999994,5.2,-3.82594874400001));
#356929=CARTESIAN_POINT('Ctrl Pts',(1.36609819999994,2.2,-3.82594874400001));
#356930=CARTESIAN_POINT('Ctrl Pts',(1.36656540399994,12.2,-3.82674996100001));
#356931=CARTESIAN_POINT('Ctrl Pts',(1.36656540399994,5.2,-3.82674996100001));
#356932=CARTESIAN_POINT('Ctrl Pts',(1.36656540399994,2.2,-3.82674996100001));
#356933=CARTESIAN_POINT('Ctrl Pts',(1.36703642999994,12.2,-3.82755543500001));
#356934=CARTESIAN_POINT('Ctrl Pts',(1.36703642999994,5.2,-3.82755543500001));
#356935=CARTESIAN_POINT('Ctrl Pts',(1.36703642999994,2.2,-3.82755543500001));
#356936=CARTESIAN_POINT('Ctrl Pts',(1.36751128299994,12.2,-3.82836514600001));
#356937=CARTESIAN_POINT('Ctrl Pts',(1.36751128299994,5.2,-3.82836514600001));
#356938=CARTESIAN_POINT('Ctrl Pts',(1.36751128299994,2.2,-3.82836514600001));
#356939=CARTESIAN_POINT('Ctrl Pts',(1.36798996999994,12.2,-3.82917908000001));
#356940=CARTESIAN_POINT('Ctrl Pts',(1.36798996999994,5.2,-3.82917908000001));
#356941=CARTESIAN_POINT('Ctrl Pts',(1.36798996999994,2.2,-3.82917908000001));
#356942=CARTESIAN_POINT('Ctrl Pts',(1.36847249499994,12.2,-3.82999722100001));
#356943=CARTESIAN_POINT('Ctrl Pts',(1.36847249499994,5.2,-3.82999722100001));
#356944=CARTESIAN_POINT('Ctrl Pts',(1.36847249499994,2.2,-3.82999722100001));
#356945=CARTESIAN_POINT('Ctrl Pts',(1.36895886499994,12.2,-3.83081955200002));
#356946=CARTESIAN_POINT('Ctrl Pts',(1.36895886499994,5.2,-3.83081955200002));
#356947=CARTESIAN_POINT('Ctrl Pts',(1.36895886499994,2.2,-3.83081955200002));
#356948=CARTESIAN_POINT('Ctrl Pts',(1.36944908599994,12.2,-3.83164605800001));
#356949=CARTESIAN_POINT('Ctrl Pts',(1.36944908599994,5.2,-3.83164605800001));
#356950=CARTESIAN_POINT('Ctrl Pts',(1.36944908599994,2.2,-3.83164605800001));
#356951=CARTESIAN_POINT('Ctrl Pts',(1.36994316299994,12.2,-3.83247672100001));
#356952=CARTESIAN_POINT('Ctrl Pts',(1.36994316299994,5.2,-3.83247672100001));
#356953=CARTESIAN_POINT('Ctrl Pts',(1.36994316299994,2.2,-3.83247672100001));
#356954=CARTESIAN_POINT('Ctrl Pts',(1.37044110099994,12.2,-3.83331152800002));
#356955=CARTESIAN_POINT('Ctrl Pts',(1.37044110099994,5.2,-3.83331152800002));
#356956=CARTESIAN_POINT('Ctrl Pts',(1.37044110099994,2.2,-3.83331152800002));
#356957=CARTESIAN_POINT('Ctrl Pts',(1.37094290799994,12.2,-3.83415046100001));
#356958=CARTESIAN_POINT('Ctrl Pts',(1.37094290799994,5.2,-3.83415046100001));
#356959=CARTESIAN_POINT('Ctrl Pts',(1.37094290799994,2.2,-3.83415046100001));
#356960=CARTESIAN_POINT('Ctrl Pts',(1.37144858499994,12.2,-3.83499350300001));
#356961=CARTESIAN_POINT('Ctrl Pts',(1.37144858499994,5.2,-3.83499350300001));
#356962=CARTESIAN_POINT('Ctrl Pts',(1.37144858499994,2.2,-3.83499350300001));
#356963=CARTESIAN_POINT('Ctrl Pts',(1.37195814299994,12.2,-3.83584064200001));
#356964=CARTESIAN_POINT('Ctrl Pts',(1.37195814299994,5.2,-3.83584064200001));
#356965=CARTESIAN_POINT('Ctrl Pts',(1.37195814299994,2.2,-3.83584064200001));
#356966=CARTESIAN_POINT('Ctrl Pts',(1.37247158399994,12.2,-3.83669185900001));
#356967=CARTESIAN_POINT('Ctrl Pts',(1.37247158399994,5.2,-3.83669185900001));
#356968=CARTESIAN_POINT('Ctrl Pts',(1.37247158399994,2.2,-3.83669185900001));
#356969=CARTESIAN_POINT('Ctrl Pts',(1.37298891399994,12.2,-3.83754713800001));
#356970=CARTESIAN_POINT('Ctrl Pts',(1.37298891399994,5.2,-3.83754713800001));
#356971=CARTESIAN_POINT('Ctrl Pts',(1.37298891399994,2.2,-3.83754713800001));
#356972=CARTESIAN_POINT('Ctrl Pts',(1.37351013899994,12.2,-3.83840646500001));
#356973=CARTESIAN_POINT('Ctrl Pts',(1.37351013899994,5.2,-3.83840646500001));
#356974=CARTESIAN_POINT('Ctrl Pts',(1.37351013899994,2.2,-3.83840646500001));
#356975=CARTESIAN_POINT('Ctrl Pts',(1.37403526399994,12.2,-3.83926982500002));
#356976=CARTESIAN_POINT('Ctrl Pts',(1.37403526399994,5.2,-3.83926982500002));
#356977=CARTESIAN_POINT('Ctrl Pts',(1.37403526399994,2.2,-3.83926982500002));
#356978=CARTESIAN_POINT('Ctrl Pts',(1.37456429499994,12.2,-3.84013719900001));
#356979=CARTESIAN_POINT('Ctrl Pts',(1.37456429499994,5.2,-3.84013719900001));
#356980=CARTESIAN_POINT('Ctrl Pts',(1.37456429499994,2.2,-3.84013719900001));
#356981=CARTESIAN_POINT('Ctrl Pts',(1.37509723699994,12.2,-3.84100857400002));
#356982=CARTESIAN_POINT('Ctrl Pts',(1.37509723699994,5.2,-3.84100857400002));
#356983=CARTESIAN_POINT('Ctrl Pts',(1.37509723699994,2.2,-3.84100857400002));
#356984=CARTESIAN_POINT('Ctrl Pts',(1.37563409399994,12.2,-3.84188393300001));
#356985=CARTESIAN_POINT('Ctrl Pts',(1.37563409399994,5.2,-3.84188393300001));
#356986=CARTESIAN_POINT('Ctrl Pts',(1.37563409399994,2.2,-3.84188393300001));
#356987=CARTESIAN_POINT('Ctrl Pts',(1.37617487299994,12.2,-3.84276326100002));
#356988=CARTESIAN_POINT('Ctrl Pts',(1.37617487299994,5.2,-3.84276326100002));
#356989=CARTESIAN_POINT('Ctrl Pts',(1.37617487299994,2.2,-3.84276326100002));
#356990=CARTESIAN_POINT('Ctrl Pts',(1.37671957899994,12.2,-3.84364654300001));
#356991=CARTESIAN_POINT('Ctrl Pts',(1.37671957899994,5.2,-3.84364654300001));
#356992=CARTESIAN_POINT('Ctrl Pts',(1.37671957899994,2.2,-3.84364654300001));
#356993=CARTESIAN_POINT('Ctrl Pts',(1.37726821599994,12.2,-3.84453376200002));
#356994=CARTESIAN_POINT('Ctrl Pts',(1.37726821599994,5.2,-3.84453376200002));
#356995=CARTESIAN_POINT('Ctrl Pts',(1.37726821599994,2.2,-3.84453376200002));
#356996=CARTESIAN_POINT('Ctrl Pts',(1.37782079099994,12.2,-3.84542490400001));
#356997=CARTESIAN_POINT('Ctrl Pts',(1.37782079099994,5.2,-3.84542490400001));
#356998=CARTESIAN_POINT('Ctrl Pts',(1.37782079099994,2.2,-3.84542490400001));
#356999=CARTESIAN_POINT('Ctrl Pts',(1.37837730699994,12.2,-3.84631995400001));
#357000=CARTESIAN_POINT('Ctrl Pts',(1.37837730699994,5.2,-3.84631995400001));
#357001=CARTESIAN_POINT('Ctrl Pts',(1.37837730699994,2.2,-3.84631995400001));
#357002=CARTESIAN_POINT('Ctrl Pts',(1.37893776999994,12.2,-3.84721889300002));
#357003=CARTESIAN_POINT('Ctrl Pts',(1.37893776999994,5.2,-3.84721889300002));
#357004=CARTESIAN_POINT('Ctrl Pts',(1.37893776999994,2.2,-3.84721889300002));
#357005=CARTESIAN_POINT('Ctrl Pts',(1.37950218599994,12.2,-3.84812170900001));
#357006=CARTESIAN_POINT('Ctrl Pts',(1.37950218599994,5.2,-3.84812170900001));
#357007=CARTESIAN_POINT('Ctrl Pts',(1.37950218599994,2.2,-3.84812170900001));
#357008=CARTESIAN_POINT('Ctrl Pts',(1.38007055999994,12.2,-3.84902838500001));
#357009=CARTESIAN_POINT('Ctrl Pts',(1.38007055999994,5.2,-3.84902838500001));
#357010=CARTESIAN_POINT('Ctrl Pts',(1.38007055999994,2.2,-3.84902838500001));
#357011=CARTESIAN_POINT('Ctrl Pts',(1.38064289399994,12.2,-3.84993890800001));
#357012=CARTESIAN_POINT('Ctrl Pts',(1.38064289399994,5.2,-3.84993890800001));
#357013=CARTESIAN_POINT('Ctrl Pts',(1.38064289399994,2.2,-3.84993890800001));
#357014=CARTESIAN_POINT('Ctrl Pts',(1.38121919799994,12.2,-3.85085325900001));
#357015=CARTESIAN_POINT('Ctrl Pts',(1.38121919799994,5.2,-3.85085325900001));
#357016=CARTESIAN_POINT('Ctrl Pts',(1.38121919799994,2.2,-3.85085325900001));
#357017=CARTESIAN_POINT('Ctrl Pts',(1.38179947199994,12.2,-3.85177142500002));
#357018=CARTESIAN_POINT('Ctrl Pts',(1.38179947199994,5.2,-3.85177142500002));
#357019=CARTESIAN_POINT('Ctrl Pts',(1.38179947199994,2.2,-3.85177142500002));
#357020=CARTESIAN_POINT('Ctrl Pts',(1.38238372299994,12.2,-3.85269339200002));
#357021=CARTESIAN_POINT('Ctrl Pts',(1.38238372299994,5.2,-3.85269339200002));
#357022=CARTESIAN_POINT('Ctrl Pts',(1.38238372299994,2.2,-3.85269339200002));
#357023=CARTESIAN_POINT('Ctrl Pts',(1.38297195699994,12.2,-3.85361914100002));
#357024=CARTESIAN_POINT('Ctrl Pts',(1.38297195699994,5.2,-3.85361914100002));
#357025=CARTESIAN_POINT('Ctrl Pts',(1.38297195699994,2.2,-3.85361914100002));
#357026=CARTESIAN_POINT('Ctrl Pts',(1.38356417799994,12.2,-3.85454866000002));
#357027=CARTESIAN_POINT('Ctrl Pts',(1.38356417799994,5.2,-3.85454866000002));
#357028=CARTESIAN_POINT('Ctrl Pts',(1.38356417799994,2.2,-3.85454866000002));
#357029=CARTESIAN_POINT('Ctrl Pts',(1.38416038999994,12.2,-3.85548193300002));
#357030=CARTESIAN_POINT('Ctrl Pts',(1.38416038999994,5.2,-3.85548193300002));
#357031=CARTESIAN_POINT('Ctrl Pts',(1.38416038999994,2.2,-3.85548193300002));
#357032=CARTESIAN_POINT('Ctrl Pts',(1.38476059799994,12.2,-3.85641894400001));
#357033=CARTESIAN_POINT('Ctrl Pts',(1.38476059799994,5.2,-3.85641894400001));
#357034=CARTESIAN_POINT('Ctrl Pts',(1.38476059799994,2.2,-3.85641894400001));
#357035=CARTESIAN_POINT('Ctrl Pts',(1.38536480699994,12.2,-3.85735967900001));
#357036=CARTESIAN_POINT('Ctrl Pts',(1.38536480699994,5.2,-3.85735967900001));
#357037=CARTESIAN_POINT('Ctrl Pts',(1.38536480699994,2.2,-3.85735967900001));
#357038=CARTESIAN_POINT('Ctrl Pts',(1.38597302199994,12.2,-3.85830412200002));
#357039=CARTESIAN_POINT('Ctrl Pts',(1.38597302199994,5.2,-3.85830412200002));
#357040=CARTESIAN_POINT('Ctrl Pts',(1.38597302199994,2.2,-3.85830412200002));
#357041=CARTESIAN_POINT('Ctrl Pts',(1.38658524799994,12.2,-3.85925225800001));
#357042=CARTESIAN_POINT('Ctrl Pts',(1.38658524799994,5.2,-3.85925225800001));
#357043=CARTESIAN_POINT('Ctrl Pts',(1.38658524799994,2.2,-3.85925225800001));
#357044=CARTESIAN_POINT('Ctrl Pts',(1.38720148999994,12.2,-3.86020407300002));
#357045=CARTESIAN_POINT('Ctrl Pts',(1.38720148999994,5.2,-3.86020407300002));
#357046=CARTESIAN_POINT('Ctrl Pts',(1.38720148999994,2.2,-3.86020407300002));
#357047=CARTESIAN_POINT('Ctrl Pts',(1.38782174999994,12.2,-3.86115955100002));
#357048=CARTESIAN_POINT('Ctrl Pts',(1.38782174999994,5.2,-3.86115955100002));
#357049=CARTESIAN_POINT('Ctrl Pts',(1.38782174999994,2.2,-3.86115955100002));
#357050=CARTESIAN_POINT('Ctrl Pts',(1.38844603399994,12.2,-3.86211867800001));
#357051=CARTESIAN_POINT('Ctrl Pts',(1.38844603399994,5.2,-3.86211867800001));
#357052=CARTESIAN_POINT('Ctrl Pts',(1.38844603399994,2.2,-3.86211867800001));
#357053=CARTESIAN_POINT('Ctrl Pts',(1.38907434899994,12.2,-3.86308143800001));
#357054=CARTESIAN_POINT('Ctrl Pts',(1.38907434899994,5.2,-3.86308143800001));
#357055=CARTESIAN_POINT('Ctrl Pts',(1.38907434899994,2.2,-3.86308143800001));
#357056=CARTESIAN_POINT('Ctrl Pts',(1.38970669599994,12.2,-3.86404781700001));
#357057=CARTESIAN_POINT('Ctrl Pts',(1.38970669599994,5.2,-3.86404781700001));
#357058=CARTESIAN_POINT('Ctrl Pts',(1.38970669599994,2.2,-3.86404781700001));
#357059=CARTESIAN_POINT('Ctrl Pts',(1.39034308099994,12.2,-3.86501779900001));
#357060=CARTESIAN_POINT('Ctrl Pts',(1.39034308099994,5.2,-3.86501779900001));
#357061=CARTESIAN_POINT('Ctrl Pts',(1.39034308099994,2.2,-3.86501779900001));
#357062=CARTESIAN_POINT('Ctrl Pts',(1.39098350899994,12.2,-3.86599137000001));
#357063=CARTESIAN_POINT('Ctrl Pts',(1.39098350899994,5.2,-3.86599137000001));
#357064=CARTESIAN_POINT('Ctrl Pts',(1.39098350899994,2.2,-3.86599137000001));
#357065=CARTESIAN_POINT('Ctrl Pts',(1.39162798299994,12.2,-3.86696851600002));
#357066=CARTESIAN_POINT('Ctrl Pts',(1.39162798299994,5.2,-3.86696851600002));
#357067=CARTESIAN_POINT('Ctrl Pts',(1.39162798299994,2.2,-3.86696851600002));
#357068=CARTESIAN_POINT('Ctrl Pts',(1.39227650999994,12.2,-3.86794922000002));
#357069=CARTESIAN_POINT('Ctrl Pts',(1.39227650999994,5.2,-3.86794922000002));
#357070=CARTESIAN_POINT('Ctrl Pts',(1.39227650999994,2.2,-3.86794922000002));
#357071=CARTESIAN_POINT('Ctrl Pts',(1.39292909199994,12.2,-3.86893347000001));
#357072=CARTESIAN_POINT('Ctrl Pts',(1.39292909199994,5.2,-3.86893347000001));
#357073=CARTESIAN_POINT('Ctrl Pts',(1.39292909199994,2.2,-3.86893347000001));
#357074=CARTESIAN_POINT('Ctrl Pts',(1.39358573299994,12.2,-3.86992124900001));
#357075=CARTESIAN_POINT('Ctrl Pts',(1.39358573299994,5.2,-3.86992124900001));
#357076=CARTESIAN_POINT('Ctrl Pts',(1.39358573299994,2.2,-3.86992124900001));
#357077=CARTESIAN_POINT('Ctrl Pts',(1.39424643899994,12.2,-3.87091254300001));
#357078=CARTESIAN_POINT('Ctrl Pts',(1.39424643899994,5.2,-3.87091254300001));
#357079=CARTESIAN_POINT('Ctrl Pts',(1.39424643899994,2.2,-3.87091254300001));
#357080=CARTESIAN_POINT('Ctrl Pts',(1.39491121399994,12.2,-3.87190733700002));
#357081=CARTESIAN_POINT('Ctrl Pts',(1.39491121399994,5.2,-3.87190733700002));
#357082=CARTESIAN_POINT('Ctrl Pts',(1.39491121399994,2.2,-3.87190733700002));
#357083=CARTESIAN_POINT('Ctrl Pts',(1.39558006099994,12.2,-3.87290561800001));
#357084=CARTESIAN_POINT('Ctrl Pts',(1.39558006099994,5.2,-3.87290561800001));
#357085=CARTESIAN_POINT('Ctrl Pts',(1.39558006099994,2.2,-3.87290561800001));
#357086=CARTESIAN_POINT('Ctrl Pts',(1.39625298699994,12.2,-3.87390736900001));
#357087=CARTESIAN_POINT('Ctrl Pts',(1.39625298699994,5.2,-3.87390736900001));
#357088=CARTESIAN_POINT('Ctrl Pts',(1.39625298699994,2.2,-3.87390736900001));
#357089=CARTESIAN_POINT('Ctrl Pts',(1.39692999299994,12.2,-3.87491257700002));
#357090=CARTESIAN_POINT('Ctrl Pts',(1.39692999299994,5.2,-3.87491257700002));
#357091=CARTESIAN_POINT('Ctrl Pts',(1.39692999299994,2.2,-3.87491257700002));
#357092=CARTESIAN_POINT('Ctrl Pts',(1.39761108399994,12.2,-3.87592122700001));
#357093=CARTESIAN_POINT('Ctrl Pts',(1.39761108399994,5.2,-3.87592122700001));
#357094=CARTESIAN_POINT('Ctrl Pts',(1.39761108399994,2.2,-3.87592122700001));
#357095=CARTESIAN_POINT('Ctrl Pts',(1.39829626699994,12.2,-3.87693330500001));
#357096=CARTESIAN_POINT('Ctrl Pts',(1.39829626699994,5.2,-3.87693330500001));
#357097=CARTESIAN_POINT('Ctrl Pts',(1.39829626699994,2.2,-3.87693330500001));
#357098=CARTESIAN_POINT('Ctrl Pts',(1.39898554099994,12.2,-3.87794879600001));
#357099=CARTESIAN_POINT('Ctrl Pts',(1.39898554099994,5.2,-3.87794879600001));
#357100=CARTESIAN_POINT('Ctrl Pts',(1.39898554099994,2.2,-3.87794879600001));
#357101=CARTESIAN_POINT('Ctrl Pts',(1.39967891499994,12.2,-3.87896768400001));
#357102=CARTESIAN_POINT('Ctrl Pts',(1.39967891499994,5.2,-3.87896768400001));
#357103=CARTESIAN_POINT('Ctrl Pts',(1.39967891499994,2.2,-3.87896768400001));
#357104=CARTESIAN_POINT('Ctrl Pts',(1.40037638999994,12.2,-3.87998995800002));
#357105=CARTESIAN_POINT('Ctrl Pts',(1.40037638999994,5.2,-3.87998995800002));
#357106=CARTESIAN_POINT('Ctrl Pts',(1.40037638999994,2.2,-3.87998995800002));
#357107=CARTESIAN_POINT('Ctrl Pts',(1.40107797099994,12.2,-3.88101560100001));
#357108=CARTESIAN_POINT('Ctrl Pts',(1.40107797099994,5.2,-3.88101560100001));
#357109=CARTESIAN_POINT('Ctrl Pts',(1.40107797099994,2.2,-3.88101560100001));
#357110=CARTESIAN_POINT('Ctrl Pts',(1.40178366299994,12.2,-3.88204459900001));
#357111=CARTESIAN_POINT('Ctrl Pts',(1.40178366299994,5.2,-3.88204459900001));
#357112=CARTESIAN_POINT('Ctrl Pts',(1.40178366299994,2.2,-3.88204459900001));
#357113=CARTESIAN_POINT('Ctrl Pts',(1.40249346899994,12.2,-3.88307693800002));
#357114=CARTESIAN_POINT('Ctrl Pts',(1.40249346899994,5.2,-3.88307693800002));
#357115=CARTESIAN_POINT('Ctrl Pts',(1.40249346899994,2.2,-3.88307693800002));
#357116=CARTESIAN_POINT('Ctrl Pts',(1.40320739299994,12.2,-3.88411260400002));
#357117=CARTESIAN_POINT('Ctrl Pts',(1.40320739299994,5.2,-3.88411260400002));
#357118=CARTESIAN_POINT('Ctrl Pts',(1.40320739299994,2.2,-3.88411260400002));
#357119=CARTESIAN_POINT('Ctrl Pts',(1.40392543799994,12.2,-3.88515158100001));
#357120=CARTESIAN_POINT('Ctrl Pts',(1.40392543799994,5.2,-3.88515158100001));
#357121=CARTESIAN_POINT('Ctrl Pts',(1.40392543799994,2.2,-3.88515158100001));
#357122=CARTESIAN_POINT('Ctrl Pts',(1.40464760899994,12.2,-3.88619385700002));
#357123=CARTESIAN_POINT('Ctrl Pts',(1.40464760899994,5.2,-3.88619385700002));
#357124=CARTESIAN_POINT('Ctrl Pts',(1.40464760899994,2.2,-3.88619385700002));
#357125=CARTESIAN_POINT('Ctrl Pts',(1.40537391099994,12.2,-3.88723941700002));
#357126=CARTESIAN_POINT('Ctrl Pts',(1.40537391099994,5.2,-3.88723941700002));
#357127=CARTESIAN_POINT('Ctrl Pts',(1.40537391099994,2.2,-3.88723941700002));
#357128=CARTESIAN_POINT('Ctrl Pts',(1.40610434499994,12.2,-3.88828824600001));
#357129=CARTESIAN_POINT('Ctrl Pts',(1.40610434499994,5.2,-3.88828824600001));
#357130=CARTESIAN_POINT('Ctrl Pts',(1.40610434499994,2.2,-3.88828824600001));
#357131=CARTESIAN_POINT('Ctrl Pts',(1.40683891699994,12.2,-3.88934033000002));
#357132=CARTESIAN_POINT('Ctrl Pts',(1.40683891699994,5.2,-3.88934033000002));
#357133=CARTESIAN_POINT('Ctrl Pts',(1.40683891699994,2.2,-3.88934033000002));
#357134=CARTESIAN_POINT('Ctrl Pts',(1.40757762999994,12.2,-3.89039565500001));
#357135=CARTESIAN_POINT('Ctrl Pts',(1.40757762999994,5.2,-3.89039565500001));
#357136=CARTESIAN_POINT('Ctrl Pts',(1.40757762999994,2.2,-3.89039565500001));
#357137=CARTESIAN_POINT('Ctrl Pts',(1.40832048899994,12.2,-3.89145420800002));
#357138=CARTESIAN_POINT('Ctrl Pts',(1.40832048899994,5.2,-3.89145420800002));
#357139=CARTESIAN_POINT('Ctrl Pts',(1.40832048899994,2.2,-3.89145420800002));
#357140=CARTESIAN_POINT('Ctrl Pts',(1.40906749599994,12.2,-3.89251597300001));
#357141=CARTESIAN_POINT('Ctrl Pts',(1.40906749599994,5.2,-3.89251597300001));
#357142=CARTESIAN_POINT('Ctrl Pts',(1.40906749599994,2.2,-3.89251597300001));
#357143=CARTESIAN_POINT('Ctrl Pts',(1.40981865399994,12.2,-3.89358093600002));
#357144=CARTESIAN_POINT('Ctrl Pts',(1.40981865399994,5.2,-3.89358093600002));
#357145=CARTESIAN_POINT('Ctrl Pts',(1.40981865399994,2.2,-3.89358093600002));
#357146=CARTESIAN_POINT('Ctrl Pts',(1.41057396999994,12.2,-3.89464908600001));
#357147=CARTESIAN_POINT('Ctrl Pts',(1.41057396999994,5.2,-3.89464908600001));
#357148=CARTESIAN_POINT('Ctrl Pts',(1.41057396999994,2.2,-3.89464908600001));
#357149=CARTESIAN_POINT('Ctrl Pts',(1.41133344599994,12.2,-3.89572040500001));
#357150=CARTESIAN_POINT('Ctrl Pts',(1.41133344599994,5.2,-3.89572040500001));
#357151=CARTESIAN_POINT('Ctrl Pts',(1.41133344599994,2.2,-3.89572040500001));
#357152=CARTESIAN_POINT('Ctrl Pts',(1.41209708399994,12.2,-3.89679488000001));
#357153=CARTESIAN_POINT('Ctrl Pts',(1.41209708399994,5.2,-3.89679488000001));
#357154=CARTESIAN_POINT('Ctrl Pts',(1.41209708399994,2.2,-3.89679488000001));
#357155=CARTESIAN_POINT('Ctrl Pts',(1.41286488899994,12.2,-3.89787249900001));
#357156=CARTESIAN_POINT('Ctrl Pts',(1.41286488899994,5.2,-3.89787249900001));
#357157=CARTESIAN_POINT('Ctrl Pts',(1.41286488899994,2.2,-3.89787249900001));
#357158=CARTESIAN_POINT('Ctrl Pts',(1.41363686599994,12.2,-3.89895324600001));
#357159=CARTESIAN_POINT('Ctrl Pts',(1.41363686599994,5.2,-3.89895324600001));
#357160=CARTESIAN_POINT('Ctrl Pts',(1.41363686599994,2.2,-3.89895324600001));
#357161=CARTESIAN_POINT('Ctrl Pts',(1.41441301599994,12.2,-3.90003710800002));
#357162=CARTESIAN_POINT('Ctrl Pts',(1.41441301599994,5.2,-3.90003710800002));
#357163=CARTESIAN_POINT('Ctrl Pts',(1.41441301599994,2.2,-3.90003710800002));
#357164=CARTESIAN_POINT('Ctrl Pts',(1.41519334299994,12.2,-3.90112407000001));
#357165=CARTESIAN_POINT('Ctrl Pts',(1.41519334299994,5.2,-3.90112407000001));
#357166=CARTESIAN_POINT('Ctrl Pts',(1.41519334299994,2.2,-3.90112407000001));
#357167=CARTESIAN_POINT('Ctrl Pts',(1.41597785299994,12.2,-3.90221412000002));
#357168=CARTESIAN_POINT('Ctrl Pts',(1.41597785299994,5.2,-3.90221412000002));
#357169=CARTESIAN_POINT('Ctrl Pts',(1.41597785299994,2.2,-3.90221412000002));
#357170=CARTESIAN_POINT('Ctrl Pts',(1.41676654599994,12.2,-3.90330724300001));
#357171=CARTESIAN_POINT('Ctrl Pts',(1.41676654599994,5.2,-3.90330724300001));
#357172=CARTESIAN_POINT('Ctrl Pts',(1.41676654599994,2.2,-3.90330724300001));
#357173=CARTESIAN_POINT('Ctrl Pts',(1.41755942799994,12.2,-3.90440342500002));
#357174=CARTESIAN_POINT('Ctrl Pts',(1.41755942799994,5.2,-3.90440342500002));
#357175=CARTESIAN_POINT('Ctrl Pts',(1.41755942799994,2.2,-3.90440342500002));
#357176=CARTESIAN_POINT('Ctrl Pts',(1.41835650099994,12.2,-3.90550265100002));
#357177=CARTESIAN_POINT('Ctrl Pts',(1.41835650099994,5.2,-3.90550265100002));
#357178=CARTESIAN_POINT('Ctrl Pts',(1.41835650099994,2.2,-3.90550265100002));
#357179=CARTESIAN_POINT('Ctrl Pts',(1.41915776899994,12.2,-3.90660491100002));
#357180=CARTESIAN_POINT('Ctrl Pts',(1.41915776899994,5.2,-3.90660491100002));
#357181=CARTESIAN_POINT('Ctrl Pts',(1.41915776899994,2.2,-3.90660491100002));
#357182=CARTESIAN_POINT('Ctrl Pts',(1.41996323499994,12.2,-3.90771018600002));
#357183=CARTESIAN_POINT('Ctrl Pts',(1.41996323499994,5.2,-3.90771018600002));
#357184=CARTESIAN_POINT('Ctrl Pts',(1.41996323499994,2.2,-3.90771018600002));
#357185=CARTESIAN_POINT('Ctrl Pts',(1.42077290399994,12.2,-3.90881846700001));
#357186=CARTESIAN_POINT('Ctrl Pts',(1.42077290399994,5.2,-3.90881846700001));
#357187=CARTESIAN_POINT('Ctrl Pts',(1.42077290399994,2.2,-3.90881846700001));
#357188=CARTESIAN_POINT('Ctrl Pts',(1.42158677699994,12.2,-3.90992973900001));
#357189=CARTESIAN_POINT('Ctrl Pts',(1.42158677699994,5.2,-3.90992973900001));
#357190=CARTESIAN_POINT('Ctrl Pts',(1.42158677699994,2.2,-3.90992973900001));
#357191=CARTESIAN_POINT('Ctrl Pts',(1.42240485899994,12.2,-3.91104398600001));
#357192=CARTESIAN_POINT('Ctrl Pts',(1.42240485899994,5.2,-3.91104398600001));
#357193=CARTESIAN_POINT('Ctrl Pts',(1.42240485899994,2.2,-3.91104398600001));
#357194=CARTESIAN_POINT('Ctrl Pts',(1.42322715199994,12.2,-3.91216119700001));
#357195=CARTESIAN_POINT('Ctrl Pts',(1.42322715199994,5.2,-3.91216119700001));
#357196=CARTESIAN_POINT('Ctrl Pts',(1.42322715199994,2.2,-3.91216119700001));
#357197=CARTESIAN_POINT('Ctrl Pts',(1.42405365899994,12.2,-3.91328135700002));
#357198=CARTESIAN_POINT('Ctrl Pts',(1.42405365899994,5.2,-3.91328135700002));
#357199=CARTESIAN_POINT('Ctrl Pts',(1.42405365899994,2.2,-3.91328135700002));
#357200=CARTESIAN_POINT('Ctrl Pts',(1.42488438499994,12.2,-3.91440445300002));
#357201=CARTESIAN_POINT('Ctrl Pts',(1.42488438499994,5.2,-3.91440445300002));
#357202=CARTESIAN_POINT('Ctrl Pts',(1.42488438499994,2.2,-3.91440445300002));
#357203=CARTESIAN_POINT('Ctrl Pts',(1.42571933199994,12.2,-3.91553047100002));
#357204=CARTESIAN_POINT('Ctrl Pts',(1.42571933199994,5.2,-3.91553047100002));
#357205=CARTESIAN_POINT('Ctrl Pts',(1.42571933199994,2.2,-3.91553047100002));
#357206=CARTESIAN_POINT('Ctrl Pts',(1.42655850299994,12.2,-3.91665939700002));
#357207=CARTESIAN_POINT('Ctrl Pts',(1.42655850299994,5.2,-3.91665939700002));
#357208=CARTESIAN_POINT('Ctrl Pts',(1.42655850299994,2.2,-3.91665939700002));
#357209=CARTESIAN_POINT('Ctrl Pts',(1.42740190199994,12.2,-3.91779121900001));
#357210=CARTESIAN_POINT('Ctrl Pts',(1.42740190199994,5.2,-3.91779121900001));
#357211=CARTESIAN_POINT('Ctrl Pts',(1.42740190199994,2.2,-3.91779121900001));
#357212=CARTESIAN_POINT('Ctrl Pts',(1.42824953199994,12.2,-3.91892592300001));
#357213=CARTESIAN_POINT('Ctrl Pts',(1.42824953199994,5.2,-3.91892592300001));
#357214=CARTESIAN_POINT('Ctrl Pts',(1.42824953199994,2.2,-3.91892592300001));
#357215=CARTESIAN_POINT('Ctrl Pts',(1.42910139499994,12.2,-3.92006349400001));
#357216=CARTESIAN_POINT('Ctrl Pts',(1.42910139499994,5.2,-3.92006349400001));
#357217=CARTESIAN_POINT('Ctrl Pts',(1.42910139499994,2.2,-3.92006349400001));
#357218=CARTESIAN_POINT('Ctrl Pts',(1.42995749499994,12.2,-3.92120392000002));
#357219=CARTESIAN_POINT('Ctrl Pts',(1.42995749499994,5.2,-3.92120392000002));
#357220=CARTESIAN_POINT('Ctrl Pts',(1.42995749499994,2.2,-3.92120392000002));
#357221=CARTESIAN_POINT('Ctrl Pts',(1.43081783499994,12.2,-3.92234718700001));
#357222=CARTESIAN_POINT('Ctrl Pts',(1.43081783499994,5.2,-3.92234718700001));
#357223=CARTESIAN_POINT('Ctrl Pts',(1.43081783499994,2.2,-3.92234718700001));
#357224=CARTESIAN_POINT('Ctrl Pts',(1.43168241799994,12.2,-3.92349328200002));
#357225=CARTESIAN_POINT('Ctrl Pts',(1.43168241799994,5.2,-3.92349328200002));
#357226=CARTESIAN_POINT('Ctrl Pts',(1.43168241799994,2.2,-3.92349328200002));
#357227=CARTESIAN_POINT('Ctrl Pts',(1.43255124699994,12.2,-3.92464219200001));
#357228=CARTESIAN_POINT('Ctrl Pts',(1.43255124699994,5.2,-3.92464219200001));
#357229=CARTESIAN_POINT('Ctrl Pts',(1.43255124699994,2.2,-3.92464219200001));
#357230=CARTESIAN_POINT('Ctrl Pts',(1.43342432399994,12.2,-3.92579390100002));
#357231=CARTESIAN_POINT('Ctrl Pts',(1.43342432399994,5.2,-3.92579390100002));
#357232=CARTESIAN_POINT('Ctrl Pts',(1.43342432399994,2.2,-3.92579390100002));
#357233=CARTESIAN_POINT('Ctrl Pts',(1.43430165399994,12.2,-3.92694840000001));
#357234=CARTESIAN_POINT('Ctrl Pts',(1.43430165399994,5.2,-3.92694840000001));
#357235=CARTESIAN_POINT('Ctrl Pts',(1.43430165399994,2.2,-3.92694840000001));
#357236=CARTESIAN_POINT('Ctrl Pts',(1.43518323799994,12.2,-3.92810567100002));
#357237=CARTESIAN_POINT('Ctrl Pts',(1.43518323799994,5.2,-3.92810567100002));
#357238=CARTESIAN_POINT('Ctrl Pts',(1.43518323799994,2.2,-3.92810567100002));
#357239=CARTESIAN_POINT('Ctrl Pts',(1.43606908099994,12.2,-3.92926570500002));
#357240=CARTESIAN_POINT('Ctrl Pts',(1.43606908099994,5.2,-3.92926570500002));
#357241=CARTESIAN_POINT('Ctrl Pts',(1.43606908099994,2.2,-3.92926570500002));
#357242=CARTESIAN_POINT('Ctrl Pts',(1.43695918299994,12.2,-3.93042848500002));
#357243=CARTESIAN_POINT('Ctrl Pts',(1.43695918299994,5.2,-3.93042848500002));
#357244=CARTESIAN_POINT('Ctrl Pts',(1.43695918299994,2.2,-3.93042848500002));
#357245=CARTESIAN_POINT('Ctrl Pts',(1.43785354899994,12.2,-3.93159400000001));
#357246=CARTESIAN_POINT('Ctrl Pts',(1.43785354899994,5.2,-3.93159400000001));
#357247=CARTESIAN_POINT('Ctrl Pts',(1.43785354899994,2.2,-3.93159400000001));
#357248=CARTESIAN_POINT('Ctrl Pts',(1.43875218099994,12.2,-3.93276223700001));
#357249=CARTESIAN_POINT('Ctrl Pts',(1.43875218099994,5.2,-3.93276223700001));
#357250=CARTESIAN_POINT('Ctrl Pts',(1.43875218099994,2.2,-3.93276223700001));
#357251=CARTESIAN_POINT('Ctrl Pts',(1.43965508299994,12.2,-3.93393318100001));
#357252=CARTESIAN_POINT('Ctrl Pts',(1.43965508299994,5.2,-3.93393318100001));
#357253=CARTESIAN_POINT('Ctrl Pts',(1.43965508299994,2.2,-3.93393318100001));
#357254=CARTESIAN_POINT('Ctrl Pts',(1.44056225699994,12.2,-3.93510682000001));
#357255=CARTESIAN_POINT('Ctrl Pts',(1.44056225699994,5.2,-3.93510682000001));
#357256=CARTESIAN_POINT('Ctrl Pts',(1.44056225699994,2.2,-3.93510682000001));
#357257=CARTESIAN_POINT('Ctrl Pts',(1.44147370499994,12.2,-3.93628314200001));
#357258=CARTESIAN_POINT('Ctrl Pts',(1.44147370499994,5.2,-3.93628314200001));
#357259=CARTESIAN_POINT('Ctrl Pts',(1.44147370499994,2.2,-3.93628314200001));
#357260=CARTESIAN_POINT('Ctrl Pts',(1.44238943099994,12.2,-3.93746213100002));
#357261=CARTESIAN_POINT('Ctrl Pts',(1.44238943099994,5.2,-3.93746213100002));
#357262=CARTESIAN_POINT('Ctrl Pts',(1.44238943099994,2.2,-3.93746213100002));
#357263=CARTESIAN_POINT('Ctrl Pts',(1.44330943599994,12.2,-3.93864377500002));
#357264=CARTESIAN_POINT('Ctrl Pts',(1.44330943599994,5.2,-3.93864377500002));
#357265=CARTESIAN_POINT('Ctrl Pts',(1.44330943599994,2.2,-3.93864377500002));
#357266=CARTESIAN_POINT('Ctrl Pts',(1.44423372399994,12.2,-3.93982806200002));
#357267=CARTESIAN_POINT('Ctrl Pts',(1.44423372399994,5.2,-3.93982806200002));
#357268=CARTESIAN_POINT('Ctrl Pts',(1.44423372399994,2.2,-3.93982806200002));
#357269=CARTESIAN_POINT('Ctrl Pts',(1.44516229799994,12.2,-3.94101497900001));
#357270=CARTESIAN_POINT('Ctrl Pts',(1.44516229799994,5.2,-3.94101497900001));
#357271=CARTESIAN_POINT('Ctrl Pts',(1.44516229799994,2.2,-3.94101497900001));
#357272=CARTESIAN_POINT('Ctrl Pts',(1.44609515999994,12.2,-3.94220451100002));
#357273=CARTESIAN_POINT('Ctrl Pts',(1.44609515999994,5.2,-3.94220451100002));
#357274=CARTESIAN_POINT('Ctrl Pts',(1.44609515999994,2.2,-3.94220451100002));
#357275=CARTESIAN_POINT('Ctrl Pts',(1.44703231299994,12.2,-3.94339664700002));
#357276=CARTESIAN_POINT('Ctrl Pts',(1.44703231299994,5.2,-3.94339664700002));
#357277=CARTESIAN_POINT('Ctrl Pts',(1.44703231299994,2.2,-3.94339664700002));
#357278=CARTESIAN_POINT('Ctrl Pts',(1.44797375899994,12.2,-3.94459137300001));
#357279=CARTESIAN_POINT('Ctrl Pts',(1.44797375899994,5.2,-3.94459137300001));
#357280=CARTESIAN_POINT('Ctrl Pts',(1.44797375899994,2.2,-3.94459137300001));
#357281=CARTESIAN_POINT('Ctrl Pts',(1.44891950099994,12.2,-3.94578867600002));
#357282=CARTESIAN_POINT('Ctrl Pts',(1.44891950099994,5.2,-3.94578867600002));
#357283=CARTESIAN_POINT('Ctrl Pts',(1.44891950099994,2.2,-3.94578867600002));
#357284=CARTESIAN_POINT('Ctrl Pts',(1.44986954099994,12.2,-3.94698854300001));
#357285=CARTESIAN_POINT('Ctrl Pts',(1.44986954099994,5.2,-3.94698854300001));
#357286=CARTESIAN_POINT('Ctrl Pts',(1.44986954099994,2.2,-3.94698854300001));
#357287=CARTESIAN_POINT('Ctrl Pts',(1.45082388399994,12.2,-3.94819096100001));
#357288=CARTESIAN_POINT('Ctrl Pts',(1.45082388399994,5.2,-3.94819096100001));
#357289=CARTESIAN_POINT('Ctrl Pts',(1.45082388399994,2.2,-3.94819096100001));
#357290=CARTESIAN_POINT('Ctrl Pts',(1.45178252799994,12.2,-3.94939591800001));
#357291=CARTESIAN_POINT('Ctrl Pts',(1.45178252799994,5.2,-3.94939591800001));
#357292=CARTESIAN_POINT('Ctrl Pts',(1.45178252799994,2.2,-3.94939591800001));
#357293=CARTESIAN_POINT('Ctrl Pts',(1.45274548099994,12.2,-3.95060340000001));
#357294=CARTESIAN_POINT('Ctrl Pts',(1.45274548099994,5.2,-3.95060340000001));
#357295=CARTESIAN_POINT('Ctrl Pts',(1.45274548099994,2.2,-3.95060340000001));
#357296=CARTESIAN_POINT('Ctrl Pts',(1.45371273999994,12.2,-3.95181339600001));
#357297=CARTESIAN_POINT('Ctrl Pts',(1.45371273999994,5.2,-3.95181339600001));
#357298=CARTESIAN_POINT('Ctrl Pts',(1.45371273999994,2.2,-3.95181339600001));
#357299=CARTESIAN_POINT('Ctrl Pts',(1.45468431199994,12.2,-3.95302589000002));
#357300=CARTESIAN_POINT('Ctrl Pts',(1.45468431199994,5.2,-3.95302589000002));
#357301=CARTESIAN_POINT('Ctrl Pts',(1.45468431199994,2.2,-3.95302589000002));
#357302=CARTESIAN_POINT('Ctrl Pts',(1.45566019599994,12.2,-3.95424087200002));
#357303=CARTESIAN_POINT('Ctrl Pts',(1.45566019599994,5.2,-3.95424087200002));
#357304=CARTESIAN_POINT('Ctrl Pts',(1.45566019599994,2.2,-3.95424087200002));
#357305=CARTESIAN_POINT('Ctrl Pts',(1.45664039699994,12.2,-3.95545832800002));
#357306=CARTESIAN_POINT('Ctrl Pts',(1.45664039699994,5.2,-3.95545832800002));
#357307=CARTESIAN_POINT('Ctrl Pts',(1.45664039699994,2.2,-3.95545832800002));
#357308=CARTESIAN_POINT('Ctrl Pts',(1.45762491499994,12.2,-3.95667824600002));
#357309=CARTESIAN_POINT('Ctrl Pts',(1.45762491499994,5.2,-3.95667824600002));
#357310=CARTESIAN_POINT('Ctrl Pts',(1.45762491499994,2.2,-3.95667824600002));
#357311=CARTESIAN_POINT('Ctrl Pts',(1.45861375399994,12.2,-3.95790061100001));
#357312=CARTESIAN_POINT('Ctrl Pts',(1.45861375399994,5.2,-3.95790061100001));
#357313=CARTESIAN_POINT('Ctrl Pts',(1.45861375399994,2.2,-3.95790061100001));
#357314=CARTESIAN_POINT('Ctrl Pts',(1.45960691699994,12.2,-3.95912541200001));
#357315=CARTESIAN_POINT('Ctrl Pts',(1.45960691699994,5.2,-3.95912541200001));
#357316=CARTESIAN_POINT('Ctrl Pts',(1.45960691699994,2.2,-3.95912541200001));
#357317=CARTESIAN_POINT('Ctrl Pts',(1.46060440399994,12.2,-3.96035263700002));
#357318=CARTESIAN_POINT('Ctrl Pts',(1.46060440399994,5.2,-3.96035263700002));
#357319=CARTESIAN_POINT('Ctrl Pts',(1.46060440399994,2.2,-3.96035263700002));
#357320=CARTESIAN_POINT('Ctrl Pts',(1.46160621899994,12.2,-3.96158227200001));
#357321=CARTESIAN_POINT('Ctrl Pts',(1.46160621899994,5.2,-3.96158227200001));
#357322=CARTESIAN_POINT('Ctrl Pts',(1.46160621899994,2.2,-3.96158227200001));
#357323=CARTESIAN_POINT('Ctrl Pts',(1.46261236399994,12.2,-3.96281430500002));
#357324=CARTESIAN_POINT('Ctrl Pts',(1.46261236399994,5.2,-3.96281430500002));
#357325=CARTESIAN_POINT('Ctrl Pts',(1.46261236399994,2.2,-3.96281430500002));
#357326=CARTESIAN_POINT('Ctrl Pts',(1.46362284099994,12.2,-3.96404872300002));
#357327=CARTESIAN_POINT('Ctrl Pts',(1.46362284099994,5.2,-3.96404872300002));
#357328=CARTESIAN_POINT('Ctrl Pts',(1.46362284099994,2.2,-3.96404872300002));
#357329=CARTESIAN_POINT('Ctrl Pts',(1.46463765199994,12.2,-3.96528551300001));
#357330=CARTESIAN_POINT('Ctrl Pts',(1.46463765199994,5.2,-3.96528551300001));
#357331=CARTESIAN_POINT('Ctrl Pts',(1.46463765199994,2.2,-3.96528551300001));
#357332=CARTESIAN_POINT('Ctrl Pts',(1.46565679899994,12.2,-3.96652466400001));
#357333=CARTESIAN_POINT('Ctrl Pts',(1.46565679899994,5.2,-3.96652466400001));
#357334=CARTESIAN_POINT('Ctrl Pts',(1.46565679899994,2.2,-3.96652466400001));
#357335=CARTESIAN_POINT('Ctrl Pts',(1.46668028599994,12.2,-3.96776616100002));
#357336=CARTESIAN_POINT('Ctrl Pts',(1.46668028599994,5.2,-3.96776616100002));
#357337=CARTESIAN_POINT('Ctrl Pts',(1.46668028599994,2.2,-3.96776616100002));
#357338=CARTESIAN_POINT('Ctrl Pts',(1.46770811399994,12.2,-3.96900999400001));
#357339=CARTESIAN_POINT('Ctrl Pts',(1.46770811399994,5.2,-3.96900999400001));
#357340=CARTESIAN_POINT('Ctrl Pts',(1.46770811399994,2.2,-3.96900999400001));
#357341=CARTESIAN_POINT('Ctrl Pts',(1.46874028399994,12.2,-3.97025614800001));
#357342=CARTESIAN_POINT('Ctrl Pts',(1.46874028399994,5.2,-3.97025614800001));
#357343=CARTESIAN_POINT('Ctrl Pts',(1.46874028399994,2.2,-3.97025614800001));
#357344=CARTESIAN_POINT('Ctrl Pts',(1.46977679999994,12.2,-3.97150461300001));
#357345=CARTESIAN_POINT('Ctrl Pts',(1.46977679999994,5.2,-3.97150461300001));
#357346=CARTESIAN_POINT('Ctrl Pts',(1.46977679999994,2.2,-3.97150461300001));
#357347=CARTESIAN_POINT('Ctrl Pts',(1.47081766299994,12.2,-3.97275537400001));
#357348=CARTESIAN_POINT('Ctrl Pts',(1.47081766299994,5.2,-3.97275537400001));
#357349=CARTESIAN_POINT('Ctrl Pts',(1.47081766299994,2.2,-3.97275537400001));
#357350=CARTESIAN_POINT('Ctrl Pts',(1.47186287499994,12.2,-3.97400842000001));
#357351=CARTESIAN_POINT('Ctrl Pts',(1.47186287499994,5.2,-3.97400842000001));
#357352=CARTESIAN_POINT('Ctrl Pts',(1.47186287499994,2.2,-3.97400842000001));
#357353=CARTESIAN_POINT('Ctrl Pts',(1.47291243899994,12.2,-3.97526373800002));
#357354=CARTESIAN_POINT('Ctrl Pts',(1.47291243899994,5.2,-3.97526373800002));
#357355=CARTESIAN_POINT('Ctrl Pts',(1.47291243899994,2.2,-3.97526373800002));
#357356=CARTESIAN_POINT('Ctrl Pts',(1.47396635599994,12.2,-3.97652131600001));
#357357=CARTESIAN_POINT('Ctrl Pts',(1.47396635599994,5.2,-3.97652131600001));
#357358=CARTESIAN_POINT('Ctrl Pts',(1.47396635599994,2.2,-3.97652131600001));
#357359=CARTESIAN_POINT('Ctrl Pts',(1.47502462999994,12.2,-3.97778114100001));
#357360=CARTESIAN_POINT('Ctrl Pts',(1.47502462999994,5.2,-3.97778114100001));
#357361=CARTESIAN_POINT('Ctrl Pts',(1.47502462999994,2.2,-3.97778114100001));
#357362=CARTESIAN_POINT('Ctrl Pts',(1.47608725999994,12.2,-3.97904320100002));
#357363=CARTESIAN_POINT('Ctrl Pts',(1.47608725999994,5.2,-3.97904320100002));
#357364=CARTESIAN_POINT('Ctrl Pts',(1.47608725999994,2.2,-3.97904320100002));
#357365=CARTESIAN_POINT('Ctrl Pts',(1.47715424999994,12.2,-3.98030748400001));
#357366=CARTESIAN_POINT('Ctrl Pts',(1.47715424999994,5.2,-3.98030748400001));
#357367=CARTESIAN_POINT('Ctrl Pts',(1.47715424999994,2.2,-3.98030748400001));
#357368=CARTESIAN_POINT('Ctrl Pts',(1.47822560099994,12.2,-3.98157397600002));
#357369=CARTESIAN_POINT('Ctrl Pts',(1.47822560099994,5.2,-3.98157397600002));
#357370=CARTESIAN_POINT('Ctrl Pts',(1.47822560099994,2.2,-3.98157397600002));
#357371=CARTESIAN_POINT('Ctrl Pts',(1.47930131499994,12.2,-3.98284266800002));
#357372=CARTESIAN_POINT('Ctrl Pts',(1.47930131499994,5.2,-3.98284266800002));
#357373=CARTESIAN_POINT('Ctrl Pts',(1.47930131499994,2.2,-3.98284266800002));
#357374=CARTESIAN_POINT('Ctrl Pts',(1.48038139499994,12.2,-3.98411354400002));
#357375=CARTESIAN_POINT('Ctrl Pts',(1.48038139499994,5.2,-3.98411354400002));
#357376=CARTESIAN_POINT('Ctrl Pts',(1.48038139499994,2.2,-3.98411354400002));
#357377=CARTESIAN_POINT('Ctrl Pts',(1.48146584299994,12.2,-3.98538659300002));
#357378=CARTESIAN_POINT('Ctrl Pts',(1.48146584299994,5.2,-3.98538659300002));
#357379=CARTESIAN_POINT('Ctrl Pts',(1.48146584299994,2.2,-3.98538659300002));
#357380=CARTESIAN_POINT('Ctrl Pts',(1.48255465899994,12.2,-3.98666180400001));
#357381=CARTESIAN_POINT('Ctrl Pts',(1.48255465899994,5.2,-3.98666180400001));
#357382=CARTESIAN_POINT('Ctrl Pts',(1.48255465899994,2.2,-3.98666180400001));
#357383=CARTESIAN_POINT('Ctrl Pts',(1.48364784799994,12.2,-3.98793916300002));
#357384=CARTESIAN_POINT('Ctrl Pts',(1.48364784799994,5.2,-3.98793916300002));
#357385=CARTESIAN_POINT('Ctrl Pts',(1.48364784799994,2.2,-3.98793916300002));
#357386=CARTESIAN_POINT('Ctrl Pts',(1.48474540799994,12.2,-3.98921865900002));
#357387=CARTESIAN_POINT('Ctrl Pts',(1.48474540799994,5.2,-3.98921865900002));
#357388=CARTESIAN_POINT('Ctrl Pts',(1.48474540799994,2.2,-3.98921865900002));
#357389=CARTESIAN_POINT('Ctrl Pts',(1.48584734199994,12.2,-3.99050027900001));
#357390=CARTESIAN_POINT('Ctrl Pts',(1.48584734199994,5.2,-3.99050027900001));
#357391=CARTESIAN_POINT('Ctrl Pts',(1.48584734199994,2.2,-3.99050027900001));
#357392=CARTESIAN_POINT('Ctrl Pts',(1.48695365399994,12.2,-3.99178401100002));
#357393=CARTESIAN_POINT('Ctrl Pts',(1.48695365399994,5.2,-3.99178401100002));
#357394=CARTESIAN_POINT('Ctrl Pts',(1.48695365399994,2.2,-3.99178401100002));
#357395=CARTESIAN_POINT('Ctrl Pts',(1.48806434399994,12.2,-3.99306984300001));
#357396=CARTESIAN_POINT('Ctrl Pts',(1.48806434399994,5.2,-3.99306984300001));
#357397=CARTESIAN_POINT('Ctrl Pts',(1.48806434399994,2.2,-3.99306984300001));
#357398=CARTESIAN_POINT('Ctrl Pts',(1.48917941399994,12.2,-3.99435776200002));
#357399=CARTESIAN_POINT('Ctrl Pts',(1.48917941399994,5.2,-3.99435776200002));
#357400=CARTESIAN_POINT('Ctrl Pts',(1.48917941399994,2.2,-3.99435776200002));
#357401=CARTESIAN_POINT('Ctrl Pts',(1.49029886499994,12.2,-3.99564775700001));
#357402=CARTESIAN_POINT('Ctrl Pts',(1.49029886499994,5.2,-3.99564775700001));
#357403=CARTESIAN_POINT('Ctrl Pts',(1.49029886499994,2.2,-3.99564775700001));
#357404=CARTESIAN_POINT('Ctrl Pts',(1.49142269999994,12.2,-3.99693981600001));
#357405=CARTESIAN_POINT('Ctrl Pts',(1.49142269999994,5.2,-3.99693981600001));
#357406=CARTESIAN_POINT('Ctrl Pts',(1.49142269999994,2.2,-3.99693981600001));
#357407=CARTESIAN_POINT('Ctrl Pts',(1.49255091999994,12.2,-3.99823392700001));
#357408=CARTESIAN_POINT('Ctrl Pts',(1.49255091999994,5.2,-3.99823392700001));
#357409=CARTESIAN_POINT('Ctrl Pts',(1.49255091999994,2.2,-3.99823392700001));
#357410=CARTESIAN_POINT('Ctrl Pts',(1.49368352799994,12.2,-3.99953007600002));
#357411=CARTESIAN_POINT('Ctrl Pts',(1.49368352799994,5.2,-3.99953007600002));
#357412=CARTESIAN_POINT('Ctrl Pts',(1.49368352799994,2.2,-3.99953007600002));
#357413=CARTESIAN_POINT('Ctrl Pts',(1.49482052299994,12.2,-4.00082825200001));
#357414=CARTESIAN_POINT('Ctrl Pts',(1.49482052299994,5.2,-4.00082825200001));
#357415=CARTESIAN_POINT('Ctrl Pts',(1.49482052299994,2.2,-4.00082825200001));
#357416=CARTESIAN_POINT('Ctrl Pts',(1.49596190899994,12.2,-4.00212844500001));
#357417=CARTESIAN_POINT('Ctrl Pts',(1.49596190899994,5.2,-4.00212844500001));
#357418=CARTESIAN_POINT('Ctrl Pts',(1.49596190899994,2.2,-4.00212844500001));
#357419=CARTESIAN_POINT('Ctrl Pts',(1.49710768599994,12.2,-4.00343064000001));
#357420=CARTESIAN_POINT('Ctrl Pts',(1.49710768599994,5.2,-4.00343064000001));
#357421=CARTESIAN_POINT('Ctrl Pts',(1.49710768599994,2.2,-4.00343064000001));
#357422=CARTESIAN_POINT('Ctrl Pts',(1.49825785799994,12.2,-4.00473482600002));
#357423=CARTESIAN_POINT('Ctrl Pts',(1.49825785799994,5.2,-4.00473482600002));
#357424=CARTESIAN_POINT('Ctrl Pts',(1.49825785799994,2.2,-4.00473482600002));
#357425=CARTESIAN_POINT('Ctrl Pts',(1.49941242399994,12.2,-4.00604099200002));
#357426=CARTESIAN_POINT('Ctrl Pts',(1.49941242399994,5.2,-4.00604099200002));
#357427=CARTESIAN_POINT('Ctrl Pts',(1.49941242399994,2.2,-4.00604099200002));
#357428=CARTESIAN_POINT('Ctrl Pts',(1.50057138599994,12.2,-4.00734912400001));
#357429=CARTESIAN_POINT('Ctrl Pts',(1.50057138599994,5.2,-4.00734912400001));
#357430=CARTESIAN_POINT('Ctrl Pts',(1.50057138599994,2.2,-4.00734912400001));
#357431=CARTESIAN_POINT('Ctrl Pts',(1.50173474699994,12.2,-4.00865921200001));
#357432=CARTESIAN_POINT('Ctrl Pts',(1.50173474699994,5.2,-4.00865921200001));
#357433=CARTESIAN_POINT('Ctrl Pts',(1.50173474699994,2.2,-4.00865921200001));
#357434=CARTESIAN_POINT('Ctrl Pts',(1.50290250699994,12.2,-4.00997124400002));
#357435=CARTESIAN_POINT('Ctrl Pts',(1.50290250699994,5.2,-4.00997124400002));
#357436=CARTESIAN_POINT('Ctrl Pts',(1.50290250699994,2.2,-4.00997124400002));
#357437=CARTESIAN_POINT('Ctrl Pts',(1.50407466899994,12.2,-4.01128520700002));
#357438=CARTESIAN_POINT('Ctrl Pts',(1.50407466899994,5.2,-4.01128520700002));
#357439=CARTESIAN_POINT('Ctrl Pts',(1.50407466899994,2.2,-4.01128520700002));
#357440=CARTESIAN_POINT('Ctrl Pts',(1.50525123399994,12.2,-4.01260108900001));
#357441=CARTESIAN_POINT('Ctrl Pts',(1.50525123399994,5.2,-4.01260108900001));
#357442=CARTESIAN_POINT('Ctrl Pts',(1.50525123399994,2.2,-4.01260108900001));
#357443=CARTESIAN_POINT('Ctrl Pts',(1.50643220199994,12.2,-4.01391888000001));
#357444=CARTESIAN_POINT('Ctrl Pts',(1.50643220199994,5.2,-4.01391888000001));
#357445=CARTESIAN_POINT('Ctrl Pts',(1.50643220199994,2.2,-4.01391888000001));
#357446=CARTESIAN_POINT('Ctrl Pts',(1.50761757599994,12.2,-4.01523856600001));
#357447=CARTESIAN_POINT('Ctrl Pts',(1.50761757599994,5.2,-4.01523856600001));
#357448=CARTESIAN_POINT('Ctrl Pts',(1.50761757599994,2.2,-4.01523856600001));
#357449=CARTESIAN_POINT('Ctrl Pts',(1.50880735699994,12.2,-4.01656013600002));
#357450=CARTESIAN_POINT('Ctrl Pts',(1.50880735699994,5.2,-4.01656013600002));
#357451=CARTESIAN_POINT('Ctrl Pts',(1.50880735699994,2.2,-4.01656013600002));
#357452=CARTESIAN_POINT('Ctrl Pts',(1.51000154599994,12.2,-4.01788357900001));
#357453=CARTESIAN_POINT('Ctrl Pts',(1.51000154599994,5.2,-4.01788357900001));
#357454=CARTESIAN_POINT('Ctrl Pts',(1.51000154599994,2.2,-4.01788357900001));
#357455=CARTESIAN_POINT('Ctrl Pts',(1.51120014499994,12.2,-4.01920888300001));
#357456=CARTESIAN_POINT('Ctrl Pts',(1.51120014499994,5.2,-4.01920888300001));
#357457=CARTESIAN_POINT('Ctrl Pts',(1.51120014499994,2.2,-4.01920888300001));
#357458=CARTESIAN_POINT('Ctrl Pts',(1.51240315599994,12.2,-4.02053603400002));
#357459=CARTESIAN_POINT('Ctrl Pts',(1.51240315599994,5.2,-4.02053603400002));
#357460=CARTESIAN_POINT('Ctrl Pts',(1.51240315599994,2.2,-4.02053603400002));
#357461=CARTESIAN_POINT('Ctrl Pts',(1.51361057999994,12.2,-4.02186502300002));
#357462=CARTESIAN_POINT('Ctrl Pts',(1.51361057999994,5.2,-4.02186502300002));
#357463=CARTESIAN_POINT('Ctrl Pts',(1.51361057999994,2.2,-4.02186502300002));
#357464=CARTESIAN_POINT('Ctrl Pts',(1.51482241599994,12.2,-4.02319583700002));
#357465=CARTESIAN_POINT('Ctrl Pts',(1.51482241599994,5.2,-4.02319583700002));
#357466=CARTESIAN_POINT('Ctrl Pts',(1.51482241599994,2.2,-4.02319583700002));
#357467=CARTESIAN_POINT('Ctrl Pts',(1.51603866899994,12.2,-4.02452846500001));
#357468=CARTESIAN_POINT('Ctrl Pts',(1.51603866899994,5.2,-4.02452846500001));
#357469=CARTESIAN_POINT('Ctrl Pts',(1.51603866899994,2.2,-4.02452846500001));
#357470=CARTESIAN_POINT('Ctrl Pts',(1.51725933799994,12.2,-4.02586289400002));
#357471=CARTESIAN_POINT('Ctrl Pts',(1.51725933799994,5.2,-4.02586289400002));
#357472=CARTESIAN_POINT('Ctrl Pts',(1.51725933799994,2.2,-4.02586289400002));
#357473=CARTESIAN_POINT('Ctrl Pts',(1.51848442499994,12.2,-4.02719911400002));
#357474=CARTESIAN_POINT('Ctrl Pts',(1.51848442499994,5.2,-4.02719911400002));
#357475=CARTESIAN_POINT('Ctrl Pts',(1.51848442499994,2.2,-4.02719911400002));
#357476=CARTESIAN_POINT('Ctrl Pts',(1.51971393199994,12.2,-4.02853711200001));
#357477=CARTESIAN_POINT('Ctrl Pts',(1.51971393199994,5.2,-4.02853711200001));
#357478=CARTESIAN_POINT('Ctrl Pts',(1.51971393199994,2.2,-4.02853711200001));
#357479=CARTESIAN_POINT('Ctrl Pts',(1.52094785799994,12.2,-4.02987687700001));
#357480=CARTESIAN_POINT('Ctrl Pts',(1.52094785799994,5.2,-4.02987687700001));
#357481=CARTESIAN_POINT('Ctrl Pts',(1.52094785799994,2.2,-4.02987687700001));
#357482=CARTESIAN_POINT('Ctrl Pts',(1.52218620699994,12.2,-4.03121839800002));
#357483=CARTESIAN_POINT('Ctrl Pts',(1.52218620699994,5.2,-4.03121839800002));
#357484=CARTESIAN_POINT('Ctrl Pts',(1.52218620699994,2.2,-4.03121839800002));
#357485=CARTESIAN_POINT('Ctrl Pts',(1.52342897699994,12.2,-4.03256166200002));
#357486=CARTESIAN_POINT('Ctrl Pts',(1.52342897699994,5.2,-4.03256166200002));
#357487=CARTESIAN_POINT('Ctrl Pts',(1.52342897699994,2.2,-4.03256166200002));
#357488=CARTESIAN_POINT('Ctrl Pts',(1.52467617299994,12.2,-4.03390665700002));
#357489=CARTESIAN_POINT('Ctrl Pts',(1.52467617299994,5.2,-4.03390665700002));
#357490=CARTESIAN_POINT('Ctrl Pts',(1.52467617299994,2.2,-4.03390665700002));
#357491=CARTESIAN_POINT('Ctrl Pts',(1.52592779299994,12.2,-4.03525337300001));
#357492=CARTESIAN_POINT('Ctrl Pts',(1.52592779299994,5.2,-4.03525337300001));
#357493=CARTESIAN_POINT('Ctrl Pts',(1.52592779299994,2.2,-4.03525337300001));
#357494=CARTESIAN_POINT('Ctrl Pts',(1.52718384099994,12.2,-4.03660179900001));
#357495=CARTESIAN_POINT('Ctrl Pts',(1.52718384099994,5.2,-4.03660179900001));
#357496=CARTESIAN_POINT('Ctrl Pts',(1.52718384099994,2.2,-4.03660179900001));
#357497=CARTESIAN_POINT('Ctrl Pts',(1.52844431499994,12.2,-4.03795192300001));
#357498=CARTESIAN_POINT('Ctrl Pts',(1.52844431499994,5.2,-4.03795192300001));
#357499=CARTESIAN_POINT('Ctrl Pts',(1.52844431499994,2.2,-4.03795192300001));
#357500=CARTESIAN_POINT('Ctrl Pts',(1.52970921799994,12.2,-4.03930373100001));
#357501=CARTESIAN_POINT('Ctrl Pts',(1.52970921799994,5.2,-4.03930373100001));
#357502=CARTESIAN_POINT('Ctrl Pts',(1.52970921799994,2.2,-4.03930373100001));
#357503=CARTESIAN_POINT('Ctrl Pts',(1.53097855199994,12.2,-4.04065721500002));
#357504=CARTESIAN_POINT('Ctrl Pts',(1.53097855199994,5.2,-4.04065721500002));
#357505=CARTESIAN_POINT('Ctrl Pts',(1.53097855199994,2.2,-4.04065721500002));
#357506=CARTESIAN_POINT('Ctrl Pts',(1.53225231499994,12.2,-4.04201236100001));
#357507=CARTESIAN_POINT('Ctrl Pts',(1.53225231499994,5.2,-4.04201236100001));
#357508=CARTESIAN_POINT('Ctrl Pts',(1.53225231499994,2.2,-4.04201236100001));
#357509=CARTESIAN_POINT('Ctrl Pts',(1.53353051099994,12.2,-4.04336915800001));
#357510=CARTESIAN_POINT('Ctrl Pts',(1.53353051099994,5.2,-4.04336915800001));
#357511=CARTESIAN_POINT('Ctrl Pts',(1.53353051099994,2.2,-4.04336915800001));
#357512=CARTESIAN_POINT('Ctrl Pts',(1.53481314099994,12.2,-4.04472759700001));
#357513=CARTESIAN_POINT('Ctrl Pts',(1.53481314099994,5.2,-4.04472759700001));
#357514=CARTESIAN_POINT('Ctrl Pts',(1.53481314099994,2.2,-4.04472759700001));
#357515=CARTESIAN_POINT('Ctrl Pts',(1.53610020399994,12.2,-4.04608766400001));
#357516=CARTESIAN_POINT('Ctrl Pts',(1.53610020399994,5.2,-4.04608766400001));
#357517=CARTESIAN_POINT('Ctrl Pts',(1.53610020399994,2.2,-4.04608766400001));
#357518=CARTESIAN_POINT('Ctrl Pts',(1.53739170199994,12.2,-4.04744934700001));
#357519=CARTESIAN_POINT('Ctrl Pts',(1.53739170199994,5.2,-4.04744934700001));
#357520=CARTESIAN_POINT('Ctrl Pts',(1.53739170199994,2.2,-4.04744934700001));
#357521=CARTESIAN_POINT('Ctrl Pts',(1.53868763599994,12.2,-4.04881263700001));
#357522=CARTESIAN_POINT('Ctrl Pts',(1.53868763599994,5.2,-4.04881263700001));
#357523=CARTESIAN_POINT('Ctrl Pts',(1.53868763599994,2.2,-4.04881263700001));
#357524=CARTESIAN_POINT('Ctrl Pts',(1.53998800799994,12.2,-4.05017752100001));
#357525=CARTESIAN_POINT('Ctrl Pts',(1.53998800799994,5.2,-4.05017752100001));
#357526=CARTESIAN_POINT('Ctrl Pts',(1.53998800799994,2.2,-4.05017752100001));
#357527=CARTESIAN_POINT('Ctrl Pts',(1.54129281699994,12.2,-4.05154398900001));
#357528=CARTESIAN_POINT('Ctrl Pts',(1.54129281699994,5.2,-4.05154398900001));
#357529=CARTESIAN_POINT('Ctrl Pts',(1.54129281699994,2.2,-4.05154398900001));
#357530=CARTESIAN_POINT('Ctrl Pts',(1.54260206699994,12.2,-4.05291202800001));
#357531=CARTESIAN_POINT('Ctrl Pts',(1.54260206699994,5.2,-4.05291202800001));
#357532=CARTESIAN_POINT('Ctrl Pts',(1.54260206699994,2.2,-4.05291202800001));
#357533=CARTESIAN_POINT('Ctrl Pts',(1.54391575499994,12.2,-4.05428162800002));
#357534=CARTESIAN_POINT('Ctrl Pts',(1.54391575499994,5.2,-4.05428162800002));
#357535=CARTESIAN_POINT('Ctrl Pts',(1.54391575499994,2.2,-4.05428162800002));
#357536=CARTESIAN_POINT('Ctrl Pts',(1.54523388499994,12.2,-4.05565277800001));
#357537=CARTESIAN_POINT('Ctrl Pts',(1.54523388499994,5.2,-4.05565277800001));
#357538=CARTESIAN_POINT('Ctrl Pts',(1.54523388499994,2.2,-4.05565277800001));
#357539=CARTESIAN_POINT('Ctrl Pts',(1.54655645699994,12.2,-4.05702546500001));
#357540=CARTESIAN_POINT('Ctrl Pts',(1.54655645699994,5.2,-4.05702546500001));
#357541=CARTESIAN_POINT('Ctrl Pts',(1.54655645699994,2.2,-4.05702546500001));
#357542=CARTESIAN_POINT('Ctrl Pts',(1.54788346999994,12.2,-4.05839967900001));
#357543=CARTESIAN_POINT('Ctrl Pts',(1.54788346999994,5.2,-4.05839967900001));
#357544=CARTESIAN_POINT('Ctrl Pts',(1.54788346999994,2.2,-4.05839967900001));
#357545=CARTESIAN_POINT('Ctrl Pts',(1.54921492799994,12.2,-4.05977540800002));
#357546=CARTESIAN_POINT('Ctrl Pts',(1.54921492799994,5.2,-4.05977540800002));
#357547=CARTESIAN_POINT('Ctrl Pts',(1.54921492799994,2.2,-4.05977540800002));
#357548=CARTESIAN_POINT('Ctrl Pts',(1.55055082999994,12.2,-4.06115264200002));
#357549=CARTESIAN_POINT('Ctrl Pts',(1.55055082999994,5.2,-4.06115264200002));
#357550=CARTESIAN_POINT('Ctrl Pts',(1.55055082999994,2.2,-4.06115264200002));
#357551=CARTESIAN_POINT('Ctrl Pts',(1.55189117799994,12.2,-4.06253136800002));
#357552=CARTESIAN_POINT('Ctrl Pts',(1.55189117799994,5.2,-4.06253136800002));
#357553=CARTESIAN_POINT('Ctrl Pts',(1.55189117799994,2.2,-4.06253136800002));
#357554=CARTESIAN_POINT('Ctrl Pts',(1.55323597199994,12.2,-4.06391157600002));
#357555=CARTESIAN_POINT('Ctrl Pts',(1.55323597199994,5.2,-4.06391157600002));
#357556=CARTESIAN_POINT('Ctrl Pts',(1.55323597199994,2.2,-4.06391157600002));
#357557=CARTESIAN_POINT('Ctrl Pts',(1.55458521299994,12.2,-4.06529325500002));
#357558=CARTESIAN_POINT('Ctrl Pts',(1.55458521299994,5.2,-4.06529325500002));
#357559=CARTESIAN_POINT('Ctrl Pts',(1.55458521299994,2.2,-4.06529325500002));
#357560=CARTESIAN_POINT('Ctrl Pts',(1.55593890099994,12.2,-4.06667639400002));
#357561=CARTESIAN_POINT('Ctrl Pts',(1.55593890099994,5.2,-4.06667639400002));
#357562=CARTESIAN_POINT('Ctrl Pts',(1.55593890099994,2.2,-4.06667639400002));
#357563=CARTESIAN_POINT('Ctrl Pts',(1.55729703799994,12.2,-4.06806098100001));
#357564=CARTESIAN_POINT('Ctrl Pts',(1.55729703799994,5.2,-4.06806098100001));
#357565=CARTESIAN_POINT('Ctrl Pts',(1.55729703799994,2.2,-4.06806098100001));
#357566=CARTESIAN_POINT('Ctrl Pts',(1.55865962399994,12.2,-4.06944700500001));
#357567=CARTESIAN_POINT('Ctrl Pts',(1.55865962399994,5.2,-4.06944700500001));
#357568=CARTESIAN_POINT('Ctrl Pts',(1.55865962399994,2.2,-4.06944700500001));
#357569=CARTESIAN_POINT('Ctrl Pts',(1.56002665999994,12.2,-4.07083445600001));
#357570=CARTESIAN_POINT('Ctrl Pts',(1.56002665999994,5.2,-4.07083445600001));
#357571=CARTESIAN_POINT('Ctrl Pts',(1.56002665999994,2.2,-4.07083445600001));
#357572=CARTESIAN_POINT('Ctrl Pts',(1.56139814699994,12.2,-4.07222332200002));
#357573=CARTESIAN_POINT('Ctrl Pts',(1.56139814699994,5.2,-4.07222332200002));
#357574=CARTESIAN_POINT('Ctrl Pts',(1.56139814699994,2.2,-4.07222332200002));
#357575=CARTESIAN_POINT('Ctrl Pts',(1.56277408499994,12.2,-4.07361359200001));
#357576=CARTESIAN_POINT('Ctrl Pts',(1.56277408499994,5.2,-4.07361359200001));
#357577=CARTESIAN_POINT('Ctrl Pts',(1.56277408499994,2.2,-4.07361359200001));
#357578=CARTESIAN_POINT('Ctrl Pts',(1.56415447499994,12.2,-4.07500525400001));
#357579=CARTESIAN_POINT('Ctrl Pts',(1.56415447499994,5.2,-4.07500525400001));
#357580=CARTESIAN_POINT('Ctrl Pts',(1.56415447499994,2.2,-4.07500525400001));
#357581=CARTESIAN_POINT('Ctrl Pts',(1.56553931899994,12.2,-4.07639829800001));
#357582=CARTESIAN_POINT('Ctrl Pts',(1.56553931899994,5.2,-4.07639829800001));
#357583=CARTESIAN_POINT('Ctrl Pts',(1.56553931899994,2.2,-4.07639829800001));
#357584=CARTESIAN_POINT('Ctrl Pts',(1.56692861499994,12.2,-4.07779271500001));
#357585=CARTESIAN_POINT('Ctrl Pts',(1.56692861499994,5.2,-4.07779271500001));
#357586=CARTESIAN_POINT('Ctrl Pts',(1.56692861499994,2.2,-4.07779271500001));
#357587=CARTESIAN_POINT('Ctrl Pts',(1.56832236499994,12.2,-4.07918848900001));
#357588=CARTESIAN_POINT('Ctrl Pts',(1.56832236499994,5.2,-4.07918848900001));
#357589=CARTESIAN_POINT('Ctrl Pts',(1.56832236499994,2.2,-4.07918848900001));
#357590=CARTESIAN_POINT('Ctrl Pts',(1.56972057099994,12.2,-4.08058561400002));
#357591=CARTESIAN_POINT('Ctrl Pts',(1.56972057099994,5.2,-4.08058561400002));
#357592=CARTESIAN_POINT('Ctrl Pts',(1.56972057099994,2.2,-4.08058561400002));
#357593=CARTESIAN_POINT('Ctrl Pts',(1.57112323099994,12.2,-4.08198407600001));
#357594=CARTESIAN_POINT('Ctrl Pts',(1.57112323099994,5.2,-4.08198407600001));
#357595=CARTESIAN_POINT('Ctrl Pts',(1.57112323099994,2.2,-4.08198407600001));
#357596=CARTESIAN_POINT('Ctrl Pts',(1.57253034799994,12.2,-4.08338386600001));
#357597=CARTESIAN_POINT('Ctrl Pts',(1.57253034799994,5.2,-4.08338386600001));
#357598=CARTESIAN_POINT('Ctrl Pts',(1.57253034799994,2.2,-4.08338386600001));
#357599=CARTESIAN_POINT('Ctrl Pts',(1.57394192199994,12.2,-4.08478497100001));
#357600=CARTESIAN_POINT('Ctrl Pts',(1.57394192199994,5.2,-4.08478497100001));
#357601=CARTESIAN_POINT('Ctrl Pts',(1.57394192199994,2.2,-4.08478497100001));
#357602=CARTESIAN_POINT('Ctrl Pts',(1.57535795099994,12.2,-4.08618738200001));
#357603=CARTESIAN_POINT('Ctrl Pts',(1.57535795099994,5.2,-4.08618738200001));
#357604=CARTESIAN_POINT('Ctrl Pts',(1.57535795099994,2.2,-4.08618738200001));
#357605=CARTESIAN_POINT('Ctrl Pts',(1.57677843899994,12.2,-4.08759108600002));
#357606=CARTESIAN_POINT('Ctrl Pts',(1.57677843899994,5.2,-4.08759108600002));
#357607=CARTESIAN_POINT('Ctrl Pts',(1.57677843899994,2.2,-4.08759108600002));
#357608=CARTESIAN_POINT('Ctrl Pts',(1.57820338499994,12.2,-4.08899607600001));
#357609=CARTESIAN_POINT('Ctrl Pts',(1.57820338499994,5.2,-4.08899607600001));
#357610=CARTESIAN_POINT('Ctrl Pts',(1.57820338499994,2.2,-4.08899607600001));
#357611=CARTESIAN_POINT('Ctrl Pts',(1.57963278999994,12.2,-4.09040233600001));
#357612=CARTESIAN_POINT('Ctrl Pts',(1.57963278999994,5.2,-4.09040233600001));
#357613=CARTESIAN_POINT('Ctrl Pts',(1.57963278999994,2.2,-4.09040233600001));
#357614=CARTESIAN_POINT('Ctrl Pts',(1.58106665399994,12.2,-4.09180985900001));
#357615=CARTESIAN_POINT('Ctrl Pts',(1.58106665399994,5.2,-4.09180985900001));
#357616=CARTESIAN_POINT('Ctrl Pts',(1.58106665399994,2.2,-4.09180985900001));
#357617=CARTESIAN_POINT('Ctrl Pts',(1.58250497699994,12.2,-4.09321863300002));
#357618=CARTESIAN_POINT('Ctrl Pts',(1.58250497699994,5.2,-4.09321863300002));
#357619=CARTESIAN_POINT('Ctrl Pts',(1.58250497699994,2.2,-4.09321863300002));
#357620=CARTESIAN_POINT('Ctrl Pts',(1.58394776099994,12.2,-4.09462864600001));
#357621=CARTESIAN_POINT('Ctrl Pts',(1.58394776099994,5.2,-4.09462864600001));
#357622=CARTESIAN_POINT('Ctrl Pts',(1.58394776099994,2.2,-4.09462864600001));
#357623=CARTESIAN_POINT('Ctrl Pts',(1.58539500399994,12.2,-4.09603988900002));
#357624=CARTESIAN_POINT('Ctrl Pts',(1.58539500399994,5.2,-4.09603988900002));
#357625=CARTESIAN_POINT('Ctrl Pts',(1.58539500399994,2.2,-4.09603988900002));
#357626=CARTESIAN_POINT('Ctrl Pts',(1.58684670899994,12.2,-4.09745235000001));
#357627=CARTESIAN_POINT('Ctrl Pts',(1.58684670899994,5.2,-4.09745235000001));
#357628=CARTESIAN_POINT('Ctrl Pts',(1.58684670899994,2.2,-4.09745235000001));
#357629=CARTESIAN_POINT('Ctrl Pts',(1.58830287599994,12.2,-4.09886601900002));
#357630=CARTESIAN_POINT('Ctrl Pts',(1.58830287599994,5.2,-4.09886601900002));
#357631=CARTESIAN_POINT('Ctrl Pts',(1.58830287599994,2.2,-4.09886601900002));
#357632=CARTESIAN_POINT('Ctrl Pts',(1.58976350399994,12.2,-4.10028088500002));
#357633=CARTESIAN_POINT('Ctrl Pts',(1.58976350399994,5.2,-4.10028088500002));
#357634=CARTESIAN_POINT('Ctrl Pts',(1.58976350399994,2.2,-4.10028088500002));
#357635=CARTESIAN_POINT('Ctrl Pts',(1.59122859499994,12.2,-4.10169693700002));
#357636=CARTESIAN_POINT('Ctrl Pts',(1.59122859499994,5.2,-4.10169693700002));
#357637=CARTESIAN_POINT('Ctrl Pts',(1.59122859499994,2.2,-4.10169693700002));
#357638=CARTESIAN_POINT('Ctrl Pts',(1.59269814799994,12.2,-4.10311416500001));
#357639=CARTESIAN_POINT('Ctrl Pts',(1.59269814799994,5.2,-4.10311416500001));
#357640=CARTESIAN_POINT('Ctrl Pts',(1.59269814799994,2.2,-4.10311416500001));
#357641=CARTESIAN_POINT('Ctrl Pts',(1.59417216399994,12.2,-4.10453255700002));
#357642=CARTESIAN_POINT('Ctrl Pts',(1.59417216399994,5.2,-4.10453255700002));
#357643=CARTESIAN_POINT('Ctrl Pts',(1.59417216399994,2.2,-4.10453255700002));
#357644=CARTESIAN_POINT('Ctrl Pts',(1.59565064299994,12.2,-4.10595210300002));
#357645=CARTESIAN_POINT('Ctrl Pts',(1.59565064299994,5.2,-4.10595210300002));
#357646=CARTESIAN_POINT('Ctrl Pts',(1.59565064299994,2.2,-4.10595210300002));
#357647=CARTESIAN_POINT('Ctrl Pts',(1.59713358599994,12.2,-4.10737279300001));
#357648=CARTESIAN_POINT('Ctrl Pts',(1.59713358599994,5.2,-4.10737279300001));
#357649=CARTESIAN_POINT('Ctrl Pts',(1.59713358599994,2.2,-4.10737279300001));
#357650=CARTESIAN_POINT('Ctrl Pts',(1.59862099399994,12.2,-4.10879461600001));
#357651=CARTESIAN_POINT('Ctrl Pts',(1.59862099399994,5.2,-4.10879461600001));
#357652=CARTESIAN_POINT('Ctrl Pts',(1.59862099399994,2.2,-4.10879461600001));
#357653=CARTESIAN_POINT('Ctrl Pts',(1.60011286499994,12.2,-4.11021756100002));
#357654=CARTESIAN_POINT('Ctrl Pts',(1.60011286499994,5.2,-4.11021756100002));
#357655=CARTESIAN_POINT('Ctrl Pts',(1.60011286499994,2.2,-4.11021756100002));
#357656=CARTESIAN_POINT('Ctrl Pts',(1.60160920099994,12.2,-4.11164161700002));
#357657=CARTESIAN_POINT('Ctrl Pts',(1.60160920099994,5.2,-4.11164161700002));
#357658=CARTESIAN_POINT('Ctrl Pts',(1.60160920099994,2.2,-4.11164161700002));
#357659=CARTESIAN_POINT('Ctrl Pts',(1.60311000199994,12.2,-4.11306677500002));
#357660=CARTESIAN_POINT('Ctrl Pts',(1.60311000199994,5.2,-4.11306677500002));
#357661=CARTESIAN_POINT('Ctrl Pts',(1.60311000199994,2.2,-4.11306677500002));
#357662=CARTESIAN_POINT('Ctrl Pts',(1.60461526699994,12.2,-4.11449302300001));
#357663=CARTESIAN_POINT('Ctrl Pts',(1.60461526699994,5.2,-4.11449302300001));
#357664=CARTESIAN_POINT('Ctrl Pts',(1.60461526699994,2.2,-4.11449302300001));
#357665=CARTESIAN_POINT('Ctrl Pts',(1.60612499799994,12.2,-4.11592035000002));
#357666=CARTESIAN_POINT('Ctrl Pts',(1.60612499799994,5.2,-4.11592035000002));
#357667=CARTESIAN_POINT('Ctrl Pts',(1.60612499799994,2.2,-4.11592035000002));
#357668=CARTESIAN_POINT('Ctrl Pts',(1.60763919499994,12.2,-4.11734874700001));
#357669=CARTESIAN_POINT('Ctrl Pts',(1.60763919499994,5.2,-4.11734874700001));
#357670=CARTESIAN_POINT('Ctrl Pts',(1.60763919499994,2.2,-4.11734874700001));
#357671=CARTESIAN_POINT('Ctrl Pts',(1.60915785699994,12.2,-4.11877820300001));
#357672=CARTESIAN_POINT('Ctrl Pts',(1.60915785699994,5.2,-4.11877820300001));
#357673=CARTESIAN_POINT('Ctrl Pts',(1.60915785699994,2.2,-4.11877820300001));
#357674=CARTESIAN_POINT('Ctrl Pts',(1.61068098599994,12.2,-4.12020870600001));
#357675=CARTESIAN_POINT('Ctrl Pts',(1.61068098599994,5.2,-4.12020870600001));
#357676=CARTESIAN_POINT('Ctrl Pts',(1.61068098599994,2.2,-4.12020870600001));
#357677=CARTESIAN_POINT('Ctrl Pts',(1.61220857999994,12.2,-4.12164024700001));
#357678=CARTESIAN_POINT('Ctrl Pts',(1.61220857999994,5.2,-4.12164024700001));
#357679=CARTESIAN_POINT('Ctrl Pts',(1.61220857999994,2.2,-4.12164024700001));
#357680=CARTESIAN_POINT('Ctrl Pts',(1.61374064099994,12.2,-4.12307281500001));
#357681=CARTESIAN_POINT('Ctrl Pts',(1.61374064099994,5.2,-4.12307281500001));
#357682=CARTESIAN_POINT('Ctrl Pts',(1.61374064099994,2.2,-4.12307281500001));
#357683=CARTESIAN_POINT('Ctrl Pts',(1.61527716799994,12.2,-4.12450640100001));
#357684=CARTESIAN_POINT('Ctrl Pts',(1.61527716799994,5.2,-4.12450640100001));
#357685=CARTESIAN_POINT('Ctrl Pts',(1.61527716799994,2.2,-4.12450640100001));
#357686=CARTESIAN_POINT('Ctrl Pts',(1.61681816199994,12.2,-4.12594099200001));
#357687=CARTESIAN_POINT('Ctrl Pts',(1.61681816199994,5.2,-4.12594099200001));
#357688=CARTESIAN_POINT('Ctrl Pts',(1.61681816199994,2.2,-4.12594099200001));
#357689=CARTESIAN_POINT('Ctrl Pts',(1.61836362299994,12.2,-4.12737657900001));
#357690=CARTESIAN_POINT('Ctrl Pts',(1.61836362299994,5.2,-4.12737657900001));
#357691=CARTESIAN_POINT('Ctrl Pts',(1.61836362299994,2.2,-4.12737657900001));
#357692=CARTESIAN_POINT('Ctrl Pts',(1.61991354999994,12.2,-4.12881315000002));
#357693=CARTESIAN_POINT('Ctrl Pts',(1.61991354999994,5.2,-4.12881315000002));
#357694=CARTESIAN_POINT('Ctrl Pts',(1.61991354999994,2.2,-4.12881315000002));
#357695=CARTESIAN_POINT('Ctrl Pts',(1.62146794399994,12.2,-4.13025069800002));
#357696=CARTESIAN_POINT('Ctrl Pts',(1.62146794399994,5.2,-4.13025069800002));
#357697=CARTESIAN_POINT('Ctrl Pts',(1.62146794399994,2.2,-4.13025069800002));
#357698=CARTESIAN_POINT('Ctrl Pts',(1.62302680599994,12.2,-4.13168921000001));
#357699=CARTESIAN_POINT('Ctrl Pts',(1.62302680599994,5.2,-4.13168921000001));
#357700=CARTESIAN_POINT('Ctrl Pts',(1.62302680599994,2.2,-4.13168921000001));
#357701=CARTESIAN_POINT('Ctrl Pts',(1.62459013399994,12.2,-4.13312867500002));
#357702=CARTESIAN_POINT('Ctrl Pts',(1.62459013399994,5.2,-4.13312867500002));
#357703=CARTESIAN_POINT('Ctrl Pts',(1.62459013399994,2.2,-4.13312867500002));
#357704=CARTESIAN_POINT('Ctrl Pts',(1.62615792899994,12.2,-4.13456908500001));
#357705=CARTESIAN_POINT('Ctrl Pts',(1.62615792899994,5.2,-4.13456908500001));
#357706=CARTESIAN_POINT('Ctrl Pts',(1.62615792899994,2.2,-4.13456908500001));
#357707=CARTESIAN_POINT('Ctrl Pts',(1.62773019199994,12.2,-4.13601042800002));
#357708=CARTESIAN_POINT('Ctrl Pts',(1.62773019199994,5.2,-4.13601042800002));
#357709=CARTESIAN_POINT('Ctrl Pts',(1.62773019199994,2.2,-4.13601042800002));
#357710=CARTESIAN_POINT('Ctrl Pts',(1.62930692199994,12.2,-4.13745269500001));
#357711=CARTESIAN_POINT('Ctrl Pts',(1.62930692199994,5.2,-4.13745269500001));
#357712=CARTESIAN_POINT('Ctrl Pts',(1.62930692199994,2.2,-4.13745269500001));
#357713=CARTESIAN_POINT('Ctrl Pts',(1.63088811899994,12.2,-4.13889587300002));
#357714=CARTESIAN_POINT('Ctrl Pts',(1.63088811899994,5.2,-4.13889587300002));
#357715=CARTESIAN_POINT('Ctrl Pts',(1.63088811899994,2.2,-4.13889587300002));
#357716=CARTESIAN_POINT('Ctrl Pts',(1.63247378299994,12.2,-4.14033995500001));
#357717=CARTESIAN_POINT('Ctrl Pts',(1.63247378299994,5.2,-4.14033995500001));
#357718=CARTESIAN_POINT('Ctrl Pts',(1.63247378299994,2.2,-4.14033995500001));
#357719=CARTESIAN_POINT('Ctrl Pts',(1.63406391499994,12.2,-4.14178492800001));
#357720=CARTESIAN_POINT('Ctrl Pts',(1.63406391499994,5.2,-4.14178492800001));
#357721=CARTESIAN_POINT('Ctrl Pts',(1.63406391499994,2.2,-4.14178492800001));
#357722=CARTESIAN_POINT('Ctrl Pts',(1.63565851299994,12.2,-4.14323078500002));
#357723=CARTESIAN_POINT('Ctrl Pts',(1.63565851299994,5.2,-4.14323078500002));
#357724=CARTESIAN_POINT('Ctrl Pts',(1.63565851299994,2.2,-4.14323078500002));
#357725=CARTESIAN_POINT('Ctrl Pts',(1.63725757899994,12.2,-4.14467751100001));
#357726=CARTESIAN_POINT('Ctrl Pts',(1.63725757899994,5.2,-4.14467751100001));
#357727=CARTESIAN_POINT('Ctrl Pts',(1.63725757899994,2.2,-4.14467751100001));
#357728=CARTESIAN_POINT('Ctrl Pts',(1.63886111099994,12.2,-4.14612510000001));
#357729=CARTESIAN_POINT('Ctrl Pts',(1.63886111099994,5.2,-4.14612510000001));
#357730=CARTESIAN_POINT('Ctrl Pts',(1.63886111099994,2.2,-4.14612510000001));
#357731=CARTESIAN_POINT('Ctrl Pts',(1.64046911099994,12.2,-4.14757353900002));
#357732=CARTESIAN_POINT('Ctrl Pts',(1.64046911099994,5.2,-4.14757353900002));
#357733=CARTESIAN_POINT('Ctrl Pts',(1.64046911099994,2.2,-4.14757353900002));
#357734=CARTESIAN_POINT('Ctrl Pts',(1.64208157799994,12.2,-4.14902282000002));
#357735=CARTESIAN_POINT('Ctrl Pts',(1.64208157799994,5.2,-4.14902282000002));
#357736=CARTESIAN_POINT('Ctrl Pts',(1.64208157799994,2.2,-4.14902282000002));
#357737=CARTESIAN_POINT('Ctrl Pts',(1.64369851099994,12.2,-4.15047293100002));
#357738=CARTESIAN_POINT('Ctrl Pts',(1.64369851099994,5.2,-4.15047293100002));
#357739=CARTESIAN_POINT('Ctrl Pts',(1.64369851099994,2.2,-4.15047293100002));
#357740=CARTESIAN_POINT('Ctrl Pts',(1.64531990999994,12.2,-4.15192386300001));
#357741=CARTESIAN_POINT('Ctrl Pts',(1.64531990999994,5.2,-4.15192386300001));
#357742=CARTESIAN_POINT('Ctrl Pts',(1.64531990999994,2.2,-4.15192386300001));
#357743=CARTESIAN_POINT('Ctrl Pts',(1.64694577699994,12.2,-4.15337560500001));
#357744=CARTESIAN_POINT('Ctrl Pts',(1.64694577699994,5.2,-4.15337560500001));
#357745=CARTESIAN_POINT('Ctrl Pts',(1.64694577699994,2.2,-4.15337560500001));
#357746=CARTESIAN_POINT('Ctrl Pts',(1.64857610999994,12.2,-4.15482814800002));
#357747=CARTESIAN_POINT('Ctrl Pts',(1.64857610999994,5.2,-4.15482814800002));
#357748=CARTESIAN_POINT('Ctrl Pts',(1.64857610999994,2.2,-4.15482814800002));
#357749=CARTESIAN_POINT('Ctrl Pts',(1.65021090999994,12.2,-4.15628148000001));
#357750=CARTESIAN_POINT('Ctrl Pts',(1.65021090999994,5.2,-4.15628148000001));
#357751=CARTESIAN_POINT('Ctrl Pts',(1.65021090999994,2.2,-4.15628148000001));
#357752=CARTESIAN_POINT('Ctrl Pts',(1.65185017399994,12.2,-4.15773559300002));
#357753=CARTESIAN_POINT('Ctrl Pts',(1.65185017399994,5.2,-4.15773559300002));
#357754=CARTESIAN_POINT('Ctrl Pts',(1.65185017399994,2.2,-4.15773559300002));
#357755=CARTESIAN_POINT('Ctrl Pts',(1.65349390499994,12.2,-4.15919047500001));
#357756=CARTESIAN_POINT('Ctrl Pts',(1.65349390499994,5.2,-4.15919047500001));
#357757=CARTESIAN_POINT('Ctrl Pts',(1.65349390499994,2.2,-4.15919047500001));
#357758=CARTESIAN_POINT('Ctrl Pts',(1.65514210199994,12.2,-4.16064611800001));
#357759=CARTESIAN_POINT('Ctrl Pts',(1.65514210199994,5.2,-4.16064611800001));
#357760=CARTESIAN_POINT('Ctrl Pts',(1.65514210199994,2.2,-4.16064611800001));
#357761=CARTESIAN_POINT('Ctrl Pts',(1.65679476399994,12.2,-4.16210250900001));
#357762=CARTESIAN_POINT('Ctrl Pts',(1.65679476399994,5.2,-4.16210250900001));
#357763=CARTESIAN_POINT('Ctrl Pts',(1.65679476399994,2.2,-4.16210250900001));
#357764=CARTESIAN_POINT('Ctrl Pts',(1.65845189099994,12.2,-4.16355964100001));
#357765=CARTESIAN_POINT('Ctrl Pts',(1.65845189099994,5.2,-4.16355964100001));
#357766=CARTESIAN_POINT('Ctrl Pts',(1.65845189099994,2.2,-4.16355964100001));
#357767=CARTESIAN_POINT('Ctrl Pts',(1.66011348299994,12.2,-4.16501750200001));
#357768=CARTESIAN_POINT('Ctrl Pts',(1.66011348299994,5.2,-4.16501750200001));
#357769=CARTESIAN_POINT('Ctrl Pts',(1.66011348299994,2.2,-4.16501750200001));
#357770=CARTESIAN_POINT('Ctrl Pts',(1.66177954099994,12.2,-4.16647608300002));
#357771=CARTESIAN_POINT('Ctrl Pts',(1.66177954099994,5.2,-4.16647608300002));
#357772=CARTESIAN_POINT('Ctrl Pts',(1.66177954099994,2.2,-4.16647608300002));
#357773=CARTESIAN_POINT('Ctrl Pts',(1.66345006199994,12.2,-4.16793537300002));
#357774=CARTESIAN_POINT('Ctrl Pts',(1.66345006199994,5.2,-4.16793537300002));
#357775=CARTESIAN_POINT('Ctrl Pts',(1.66345006199994,2.2,-4.16793537300002));
#357776=CARTESIAN_POINT('Ctrl Pts',(1.66512504799994,12.2,-4.16939536200001));
#357777=CARTESIAN_POINT('Ctrl Pts',(1.66512504799994,5.2,-4.16939536200001));
#357778=CARTESIAN_POINT('Ctrl Pts',(1.66512504799994,2.2,-4.16939536200001));
#357779=CARTESIAN_POINT('Ctrl Pts',(1.66680449799994,12.2,-4.17085604100001));
#357780=CARTESIAN_POINT('Ctrl Pts',(1.66680449799994,5.2,-4.17085604100001));
#357781=CARTESIAN_POINT('Ctrl Pts',(1.66680449799994,2.2,-4.17085604100001));
#357782=CARTESIAN_POINT('Ctrl Pts',(1.66848840999994,12.2,-4.17231740000001));
#357783=CARTESIAN_POINT('Ctrl Pts',(1.66848840999994,5.2,-4.17231740000001));
#357784=CARTESIAN_POINT('Ctrl Pts',(1.66848840999994,2.2,-4.17231740000001));
#357785=CARTESIAN_POINT('Ctrl Pts',(1.67017678699994,12.2,-4.17377942800002));
#357786=CARTESIAN_POINT('Ctrl Pts',(1.67017678699994,5.2,-4.17377942800002));
#357787=CARTESIAN_POINT('Ctrl Pts',(1.67017678699994,2.2,-4.17377942800002));
#357788=CARTESIAN_POINT('Ctrl Pts',(1.67186962599994,12.2,-4.17524211600002));
#357789=CARTESIAN_POINT('Ctrl Pts',(1.67186962599994,5.2,-4.17524211600002));
#357790=CARTESIAN_POINT('Ctrl Pts',(1.67186962599994,2.2,-4.17524211600002));
#357791=CARTESIAN_POINT('Ctrl Pts',(1.67356692799994,12.2,-4.17670545400001));
#357792=CARTESIAN_POINT('Ctrl Pts',(1.67356692799994,5.2,-4.17670545400001));
#357793=CARTESIAN_POINT('Ctrl Pts',(1.67356692799994,2.2,-4.17670545400001));
#357794=CARTESIAN_POINT('Ctrl Pts',(1.67526869299994,12.2,-4.17816943100001));
#357795=CARTESIAN_POINT('Ctrl Pts',(1.67526869299994,5.2,-4.17816943100001));
#357796=CARTESIAN_POINT('Ctrl Pts',(1.67526869299994,2.2,-4.17816943100001));
#357797=CARTESIAN_POINT('Ctrl Pts',(1.67697491899994,12.2,-4.17963403800002));
#357798=CARTESIAN_POINT('Ctrl Pts',(1.67697491899994,5.2,-4.17963403800002));
#357799=CARTESIAN_POINT('Ctrl Pts',(1.67697491899994,2.2,-4.17963403800002));
#357800=CARTESIAN_POINT('Ctrl Pts',(1.67868560699994,12.2,-4.18109926600001));
#357801=CARTESIAN_POINT('Ctrl Pts',(1.67868560699994,5.2,-4.18109926600001));
#357802=CARTESIAN_POINT('Ctrl Pts',(1.67868560699994,2.2,-4.18109926600001));
#357803=CARTESIAN_POINT('Ctrl Pts',(1.68040075599994,12.2,-4.18256510300001));
#357804=CARTESIAN_POINT('Ctrl Pts',(1.68040075599994,5.2,-4.18256510300001));
#357805=CARTESIAN_POINT('Ctrl Pts',(1.68040075599994,2.2,-4.18256510300001));
#357806=CARTESIAN_POINT('Ctrl Pts',(1.68212036499994,12.2,-4.18403154100002));
#357807=CARTESIAN_POINT('Ctrl Pts',(1.68212036499994,5.2,-4.18403154100002));
#357808=CARTESIAN_POINT('Ctrl Pts',(1.68212036499994,2.2,-4.18403154100002));
#357809=CARTESIAN_POINT('Ctrl Pts',(1.68384443399994,12.2,-4.18549856900002));
#357810=CARTESIAN_POINT('Ctrl Pts',(1.68384443399994,5.2,-4.18549856900002));
#357811=CARTESIAN_POINT('Ctrl Pts',(1.68384443399994,2.2,-4.18549856900002));
#357812=CARTESIAN_POINT('Ctrl Pts',(1.68557296399995,12.2,-4.18696617800002));
#357813=CARTESIAN_POINT('Ctrl Pts',(1.68557296399995,5.2,-4.18696617800002));
#357814=CARTESIAN_POINT('Ctrl Pts',(1.68557296399995,2.2,-4.18696617800002));
#357815=CARTESIAN_POINT('Ctrl Pts',(1.68730595299994,12.2,-4.18843435700001));
#357816=CARTESIAN_POINT('Ctrl Pts',(1.68730595299994,5.2,-4.18843435700001));
#357817=CARTESIAN_POINT('Ctrl Pts',(1.68730595299994,2.2,-4.18843435700001));
#357818=CARTESIAN_POINT('Ctrl Pts',(1.68904340099994,12.2,-4.18990309800002));
#357819=CARTESIAN_POINT('Ctrl Pts',(1.68904340099994,5.2,-4.18990309800002));
#357820=CARTESIAN_POINT('Ctrl Pts',(1.68904340099994,2.2,-4.18990309800002));
#357821=CARTESIAN_POINT('Ctrl Pts',(1.69078530699994,12.2,-4.19137238900001));
#357822=CARTESIAN_POINT('Ctrl Pts',(1.69078530699994,5.2,-4.19137238900001));
#357823=CARTESIAN_POINT('Ctrl Pts',(1.69078530699994,2.2,-4.19137238900001));
#357824=CARTESIAN_POINT('Ctrl Pts',(1.69253167099994,12.2,-4.19284222200002));
#357825=CARTESIAN_POINT('Ctrl Pts',(1.69253167099994,5.2,-4.19284222200002));
#357826=CARTESIAN_POINT('Ctrl Pts',(1.69253167099994,2.2,-4.19284222200002));
#357827=CARTESIAN_POINT('Ctrl Pts',(1.69428249199994,12.2,-4.19431258800001));
#357828=CARTESIAN_POINT('Ctrl Pts',(1.69428249199994,5.2,-4.19431258800001));
#357829=CARTESIAN_POINT('Ctrl Pts',(1.69428249199994,2.2,-4.19431258800001));
#357830=CARTESIAN_POINT('Ctrl Pts',(1.69603777099994,12.2,-4.19578347300002));
#357831=CARTESIAN_POINT('Ctrl Pts',(1.69603777099994,5.2,-4.19578347300002));
#357832=CARTESIAN_POINT('Ctrl Pts',(1.69603777099994,2.2,-4.19578347300002));
#357833=CARTESIAN_POINT('Ctrl Pts',(1.69779750599994,12.2,-4.19725487200001));
#357834=CARTESIAN_POINT('Ctrl Pts',(1.69779750599994,5.2,-4.19725487200001));
#357835=CARTESIAN_POINT('Ctrl Pts',(1.69779750599994,2.2,-4.19725487200001));
#357836=CARTESIAN_POINT('Ctrl Pts',(1.69956169599994,12.2,-4.19872677300001));
#357837=CARTESIAN_POINT('Ctrl Pts',(1.69956169599994,5.2,-4.19872677300001));
#357838=CARTESIAN_POINT('Ctrl Pts',(1.69956169599994,2.2,-4.19872677300001));
#357839=CARTESIAN_POINT('Ctrl Pts',(1.70133034199994,12.2,-4.20019916800001));
#357840=CARTESIAN_POINT('Ctrl Pts',(1.70133034199994,5.2,-4.20019916800001));
#357841=CARTESIAN_POINT('Ctrl Pts',(1.70133034199994,2.2,-4.20019916800001));
#357842=CARTESIAN_POINT('Ctrl Pts',(1.70310344299994,12.2,-4.20167204400002));
#357843=CARTESIAN_POINT('Ctrl Pts',(1.70310344299994,5.2,-4.20167204400002));
#357844=CARTESIAN_POINT('Ctrl Pts',(1.70310344299994,2.2,-4.20167204400002));
#357845=CARTESIAN_POINT('Ctrl Pts',(1.70488099799994,12.2,-4.20314539500001));
#357846=CARTESIAN_POINT('Ctrl Pts',(1.70488099799994,5.2,-4.20314539500001));
#357847=CARTESIAN_POINT('Ctrl Pts',(1.70488099799994,2.2,-4.20314539500001));
#357848=CARTESIAN_POINT('Ctrl Pts',(1.70666300699994,12.2,-4.20461920900001));
#357849=CARTESIAN_POINT('Ctrl Pts',(1.70666300699994,5.2,-4.20461920900001));
#357850=CARTESIAN_POINT('Ctrl Pts',(1.70666300699994,2.2,-4.20461920900001));
#357851=CARTESIAN_POINT('Ctrl Pts',(1.70844946899994,12.2,-4.20609347800001));
#357852=CARTESIAN_POINT('Ctrl Pts',(1.70844946899994,5.2,-4.20609347800001));
#357853=CARTESIAN_POINT('Ctrl Pts',(1.70844946899994,2.2,-4.20609347800001));
#357854=CARTESIAN_POINT('Ctrl Pts',(1.71024038299994,12.2,-4.20756819000002));
#357855=CARTESIAN_POINT('Ctrl Pts',(1.71024038299994,5.2,-4.20756819000002));
#357856=CARTESIAN_POINT('Ctrl Pts',(1.71024038299994,2.2,-4.20756819000002));
#357857=CARTESIAN_POINT('Ctrl Pts',(1.71203574899994,12.2,-4.20904333800001));
#357858=CARTESIAN_POINT('Ctrl Pts',(1.71203574899994,5.2,-4.20904333800001));
#357859=CARTESIAN_POINT('Ctrl Pts',(1.71203574899994,2.2,-4.20904333800001));
#357860=CARTESIAN_POINT('Ctrl Pts',(1.71383556599994,12.2,-4.21051891000001));
#357861=CARTESIAN_POINT('Ctrl Pts',(1.71383556599994,5.2,-4.21051891000001));
#357862=CARTESIAN_POINT('Ctrl Pts',(1.71383556599994,2.2,-4.21051891000001));
#357863=CARTESIAN_POINT('Ctrl Pts',(1.71563983299994,12.2,-4.21199489900001));
#357864=CARTESIAN_POINT('Ctrl Pts',(1.71563983299994,5.2,-4.21199489900001));
#357865=CARTESIAN_POINT('Ctrl Pts',(1.71563983299994,2.2,-4.21199489900001));
#357866=CARTESIAN_POINT('Ctrl Pts',(1.71744855099994,12.2,-4.21347129300001));
#357867=CARTESIAN_POINT('Ctrl Pts',(1.71744855099994,5.2,-4.21347129300001));
#357868=CARTESIAN_POINT('Ctrl Pts',(1.71744855099994,2.2,-4.21347129300001));
#357869=CARTESIAN_POINT('Ctrl Pts',(1.71926171599994,12.2,-4.21494808400002));
#357870=CARTESIAN_POINT('Ctrl Pts',(1.71926171599994,5.2,-4.21494808400002));
#357871=CARTESIAN_POINT('Ctrl Pts',(1.71926171599994,2.2,-4.21494808400002));
#357872=CARTESIAN_POINT('Ctrl Pts',(1.72107933099995,12.2,-4.21642526200001));
#357873=CARTESIAN_POINT('Ctrl Pts',(1.72107933099995,5.2,-4.21642526200001));
#357874=CARTESIAN_POINT('Ctrl Pts',(1.72107933099995,2.2,-4.21642526200001));
#357875=CARTESIAN_POINT('Ctrl Pts',(1.72290139399994,12.2,-4.21790281800002));
#357876=CARTESIAN_POINT('Ctrl Pts',(1.72290139399994,5.2,-4.21790281800002));
#357877=CARTESIAN_POINT('Ctrl Pts',(1.72290139399994,2.2,-4.21790281800002));
#357878=CARTESIAN_POINT('Ctrl Pts',(1.72472790399994,12.2,-4.21938074100002));
#357879=CARTESIAN_POINT('Ctrl Pts',(1.72472790399994,5.2,-4.21938074100002));
#357880=CARTESIAN_POINT('Ctrl Pts',(1.72472790399994,2.2,-4.21938074100002));
#357881=CARTESIAN_POINT('Ctrl Pts',(1.72655885999994,12.2,-4.22085902300001));
#357882=CARTESIAN_POINT('Ctrl Pts',(1.72655885999994,5.2,-4.22085902300001));
#357883=CARTESIAN_POINT('Ctrl Pts',(1.72655885999994,2.2,-4.22085902300001));
#357884=CARTESIAN_POINT('Ctrl Pts',(1.72839426199994,12.2,-4.22233765400001));
#357885=CARTESIAN_POINT('Ctrl Pts',(1.72839426199994,5.2,-4.22233765400001));
#357886=CARTESIAN_POINT('Ctrl Pts',(1.72839426199994,2.2,-4.22233765400001));
#357887=CARTESIAN_POINT('Ctrl Pts',(1.73023410699994,12.2,-4.22381662300001));
#357888=CARTESIAN_POINT('Ctrl Pts',(1.73023410699994,5.2,-4.22381662300001));
#357889=CARTESIAN_POINT('Ctrl Pts',(1.73023410699994,2.2,-4.22381662300001));
#357890=CARTESIAN_POINT('Ctrl Pts',(1.73207839799994,12.2,-4.22529592300001));
#357891=CARTESIAN_POINT('Ctrl Pts',(1.73207839799994,5.2,-4.22529592300001));
#357892=CARTESIAN_POINT('Ctrl Pts',(1.73207839799994,2.2,-4.22529592300001));
#357893=CARTESIAN_POINT('Ctrl Pts',(1.73392713099994,12.2,-4.22677554400002));
#357894=CARTESIAN_POINT('Ctrl Pts',(1.73392713099994,5.2,-4.22677554400002));
#357895=CARTESIAN_POINT('Ctrl Pts',(1.73392713099994,2.2,-4.22677554400002));
#357896=CARTESIAN_POINT('Ctrl Pts',(1.73578030799994,12.2,-4.22825547500001));
#357897=CARTESIAN_POINT('Ctrl Pts',(1.73578030799994,5.2,-4.22825547500001));
#357898=CARTESIAN_POINT('Ctrl Pts',(1.73578030799994,2.2,-4.22825547500001));
#357899=CARTESIAN_POINT('Ctrl Pts',(1.73763792599994,12.2,-4.22973570900002));
#357900=CARTESIAN_POINT('Ctrl Pts',(1.73763792599994,5.2,-4.22973570900002));
#357901=CARTESIAN_POINT('Ctrl Pts',(1.73763792599994,2.2,-4.22973570900002));
#357902=CARTESIAN_POINT('Ctrl Pts',(1.73949998499994,12.2,-4.23121623300001));
#357903=CARTESIAN_POINT('Ctrl Pts',(1.73949998499994,5.2,-4.23121623300001));
#357904=CARTESIAN_POINT('Ctrl Pts',(1.73949998499994,2.2,-4.23121623300001));
#357905=CARTESIAN_POINT('Ctrl Pts',(1.74136648399994,12.2,-4.23269704200001));
#357906=CARTESIAN_POINT('Ctrl Pts',(1.74136648399994,5.2,-4.23269704200001));
#357907=CARTESIAN_POINT('Ctrl Pts',(1.74136648399994,2.2,-4.23269704200001));
#357908=CARTESIAN_POINT('Ctrl Pts',(1.74323742199994,12.2,-4.23417812300002));
#357909=CARTESIAN_POINT('Ctrl Pts',(1.74323742199994,5.2,-4.23417812300002));
#357910=CARTESIAN_POINT('Ctrl Pts',(1.74323742199994,2.2,-4.23417812300002));
#357911=CARTESIAN_POINT('Ctrl Pts',(1.74511279899994,12.2,-4.23565947000001));
#357912=CARTESIAN_POINT('Ctrl Pts',(1.74511279899994,5.2,-4.23565947000001));
#357913=CARTESIAN_POINT('Ctrl Pts',(1.74511279899994,2.2,-4.23565947000001));
#357914=CARTESIAN_POINT('Ctrl Pts',(1.74699261299994,12.2,-4.23714107000002));
#357915=CARTESIAN_POINT('Ctrl Pts',(1.74699261299994,5.2,-4.23714107000002));
#357916=CARTESIAN_POINT('Ctrl Pts',(1.74699261299994,2.2,-4.23714107000002));
#357917=CARTESIAN_POINT('Ctrl Pts',(1.74887686499994,12.2,-4.23862291600001));
#357918=CARTESIAN_POINT('Ctrl Pts',(1.74887686499994,5.2,-4.23862291600001));
#357919=CARTESIAN_POINT('Ctrl Pts',(1.74887686499994,2.2,-4.23862291600001));
#357920=CARTESIAN_POINT('Ctrl Pts',(1.75076555099994,12.2,-4.24010499800001));
#357921=CARTESIAN_POINT('Ctrl Pts',(1.75076555099994,5.2,-4.24010499800001));
#357922=CARTESIAN_POINT('Ctrl Pts',(1.75076555099994,2.2,-4.24010499800001));
#357923=CARTESIAN_POINT('Ctrl Pts',(1.75265867299994,12.2,-4.24158730600002));
#357924=CARTESIAN_POINT('Ctrl Pts',(1.75265867299994,5.2,-4.24158730600002));
#357925=CARTESIAN_POINT('Ctrl Pts',(1.75265867299994,2.2,-4.24158730600002));
#357926=CARTESIAN_POINT('Ctrl Pts',(1.75455622899995,12.2,-4.24306983200001));
#357927=CARTESIAN_POINT('Ctrl Pts',(1.75455622899995,5.2,-4.24306983200001));
#357928=CARTESIAN_POINT('Ctrl Pts',(1.75455622899995,2.2,-4.24306983200001));
#357929=CARTESIAN_POINT('Ctrl Pts',(1.75645821799994,12.2,-4.24455256600002));
#357930=CARTESIAN_POINT('Ctrl Pts',(1.75645821799994,5.2,-4.24455256600002));
#357931=CARTESIAN_POINT('Ctrl Pts',(1.75645821799994,2.2,-4.24455256600002));
#357932=CARTESIAN_POINT('Ctrl Pts',(1.75836463899994,12.2,-4.24603550000001));
#357933=CARTESIAN_POINT('Ctrl Pts',(1.75836463899994,5.2,-4.24603550000001));
#357934=CARTESIAN_POINT('Ctrl Pts',(1.75836463899994,2.2,-4.24603550000001));
#357935=CARTESIAN_POINT('Ctrl Pts',(1.76027549299994,12.2,-4.24751862300001));
#357936=CARTESIAN_POINT('Ctrl Pts',(1.76027549299994,5.2,-4.24751862300001));
#357937=CARTESIAN_POINT('Ctrl Pts',(1.76027549299994,2.2,-4.24751862300001));
#357938=CARTESIAN_POINT('Ctrl Pts',(1.76219077499994,12.2,-4.24900192600001));
#357939=CARTESIAN_POINT('Ctrl Pts',(1.76219077499994,5.2,-4.24900192600001));
#357940=CARTESIAN_POINT('Ctrl Pts',(1.76219077499994,2.2,-4.24900192600001));
#357941=CARTESIAN_POINT('Ctrl Pts',(1.76411048799994,12.2,-4.25048540000001));
#357942=CARTESIAN_POINT('Ctrl Pts',(1.76411048799994,5.2,-4.25048540000001));
#357943=CARTESIAN_POINT('Ctrl Pts',(1.76411048799994,2.2,-4.25048540000001));
#357944=CARTESIAN_POINT('Ctrl Pts',(1.76603462799994,12.2,-4.25196903500002));
#357945=CARTESIAN_POINT('Ctrl Pts',(1.76603462799994,5.2,-4.25196903500002));
#357946=CARTESIAN_POINT('Ctrl Pts',(1.76603462799994,2.2,-4.25196903500002));
#357947=CARTESIAN_POINT('Ctrl Pts',(1.76796319599994,12.2,-4.25345282400002));
#357948=CARTESIAN_POINT('Ctrl Pts',(1.76796319599994,5.2,-4.25345282400002));
#357949=CARTESIAN_POINT('Ctrl Pts',(1.76796319599994,2.2,-4.25345282400002));
#357950=CARTESIAN_POINT('Ctrl Pts',(1.76989619099994,12.2,-4.25493675600002));
#357951=CARTESIAN_POINT('Ctrl Pts',(1.76989619099994,5.2,-4.25493675600002));
#357952=CARTESIAN_POINT('Ctrl Pts',(1.76989619099994,2.2,-4.25493675600002));
#357953=CARTESIAN_POINT('Ctrl Pts',(1.77183361099994,12.2,-4.25642082300001));
#357954=CARTESIAN_POINT('Ctrl Pts',(1.77183361099994,5.2,-4.25642082300001));
#357955=CARTESIAN_POINT('Ctrl Pts',(1.77183361099994,2.2,-4.25642082300001));
#357956=CARTESIAN_POINT('Ctrl Pts',(1.77377545599994,12.2,-4.25790501400002));
#357957=CARTESIAN_POINT('Ctrl Pts',(1.77377545599994,5.2,-4.25790501400002));
#357958=CARTESIAN_POINT('Ctrl Pts',(1.77377545599994,2.2,-4.25790501400002));
#357959=CARTESIAN_POINT('Ctrl Pts',(1.77572172399994,12.2,-4.25938932200001));
#357960=CARTESIAN_POINT('Ctrl Pts',(1.77572172399994,5.2,-4.25938932200001));
#357961=CARTESIAN_POINT('Ctrl Pts',(1.77572172399994,2.2,-4.25938932200001));
#357962=CARTESIAN_POINT('Ctrl Pts',(1.77767241399994,12.2,-4.26087373600001));
#357963=CARTESIAN_POINT('Ctrl Pts',(1.77767241399994,5.2,-4.26087373600001));
#357964=CARTESIAN_POINT('Ctrl Pts',(1.77767241399994,2.2,-4.26087373600001));
#357965=CARTESIAN_POINT('Ctrl Pts',(1.77962752599994,12.2,-4.26235824800001));
#357966=CARTESIAN_POINT('Ctrl Pts',(1.77962752599994,5.2,-4.26235824800001));
#357967=CARTESIAN_POINT('Ctrl Pts',(1.77962752599994,2.2,-4.26235824800001));
#357968=CARTESIAN_POINT('Ctrl Pts',(1.78158705699994,12.2,-4.26384284800001));
#357969=CARTESIAN_POINT('Ctrl Pts',(1.78158705699994,5.2,-4.26384284800001));
#357970=CARTESIAN_POINT('Ctrl Pts',(1.78158705699994,2.2,-4.26384284800001));
#357971=CARTESIAN_POINT('Ctrl Pts',(1.78355100899994,12.2,-4.26532752900001));
#357972=CARTESIAN_POINT('Ctrl Pts',(1.78355100899994,5.2,-4.26532752900001));
#357973=CARTESIAN_POINT('Ctrl Pts',(1.78355100899994,2.2,-4.26532752900001));
#357974=CARTESIAN_POINT('Ctrl Pts',(1.78551937799994,12.2,-4.26681227900001));
#357975=CARTESIAN_POINT('Ctrl Pts',(1.78551937799994,5.2,-4.26681227900001));
#357976=CARTESIAN_POINT('Ctrl Pts',(1.78551937799994,2.2,-4.26681227900001));
#357977=CARTESIAN_POINT('Ctrl Pts',(1.78749216399994,12.2,-4.26829709100002));
#357978=CARTESIAN_POINT('Ctrl Pts',(1.78749216399994,5.2,-4.26829709100002));
#357979=CARTESIAN_POINT('Ctrl Pts',(1.78749216399994,2.2,-4.26829709100002));
#357980=CARTESIAN_POINT('Ctrl Pts',(1.78946936699994,12.2,-4.26978195500002));
#357981=CARTESIAN_POINT('Ctrl Pts',(1.78946936699994,5.2,-4.26978195500002));
#357982=CARTESIAN_POINT('Ctrl Pts',(1.78946936699994,2.2,-4.26978195500002));
#357983=CARTESIAN_POINT('Ctrl Pts',(1.79145098399994,12.2,-4.27126686200001));
#357984=CARTESIAN_POINT('Ctrl Pts',(1.79145098399994,5.2,-4.27126686200001));
#357985=CARTESIAN_POINT('Ctrl Pts',(1.79145098399994,2.2,-4.27126686200001));
#357986=CARTESIAN_POINT('Ctrl Pts',(1.79343701399994,12.2,-4.27275180300001));
#357987=CARTESIAN_POINT('Ctrl Pts',(1.79343701399994,5.2,-4.27275180300001));
#357988=CARTESIAN_POINT('Ctrl Pts',(1.79343701399994,2.2,-4.27275180300001));
#357989=CARTESIAN_POINT('Ctrl Pts',(1.79542745799994,12.2,-4.27423677000002));
#357990=CARTESIAN_POINT('Ctrl Pts',(1.79542745799994,5.2,-4.27423677000002));
#357991=CARTESIAN_POINT('Ctrl Pts',(1.79542745799994,2.2,-4.27423677000002));
#357992=CARTESIAN_POINT('Ctrl Pts',(1.79742231299994,12.2,-4.27572175300002));
#357993=CARTESIAN_POINT('Ctrl Pts',(1.79742231299994,5.2,-4.27572175300002));
#357994=CARTESIAN_POINT('Ctrl Pts',(1.79742231299994,2.2,-4.27572175300002));
#357995=CARTESIAN_POINT('Ctrl Pts',(1.79942157699994,12.2,-4.27720674200001));
#357996=CARTESIAN_POINT('Ctrl Pts',(1.79942157699994,5.2,-4.27720674200001));
#357997=CARTESIAN_POINT('Ctrl Pts',(1.79942157699994,2.2,-4.27720674200001));
#357998=CARTESIAN_POINT('Ctrl Pts',(1.80142525099994,12.2,-4.27869173000001));
#357999=CARTESIAN_POINT('Ctrl Pts',(1.80142525099994,5.2,-4.27869173000001));
#358000=CARTESIAN_POINT('Ctrl Pts',(1.80142525099994,2.2,-4.27869173000001));
#358001=CARTESIAN_POINT('Ctrl Pts',(1.80343333299994,12.2,-4.28017670600001));
#358002=CARTESIAN_POINT('Ctrl Pts',(1.80343333299994,5.2,-4.28017670600001));
#358003=CARTESIAN_POINT('Ctrl Pts',(1.80343333299994,2.2,-4.28017670600001));
#358004=CARTESIAN_POINT('Ctrl Pts',(1.80544582299994,12.2,-4.28166166300001));
#358005=CARTESIAN_POINT('Ctrl Pts',(1.80544582299994,5.2,-4.28166166300001));
#358006=CARTESIAN_POINT('Ctrl Pts',(1.80544582299994,2.2,-4.28166166300001));
#358007=CARTESIAN_POINT('Ctrl Pts',(1.80746271699994,12.2,-4.28314659200002));
#358008=CARTESIAN_POINT('Ctrl Pts',(1.80746271699994,5.2,-4.28314659200002));
#358009=CARTESIAN_POINT('Ctrl Pts',(1.80746271699994,2.2,-4.28314659200002));
#358010=CARTESIAN_POINT('Ctrl Pts',(1.80948401499994,12.2,-4.28463148200001));
#358011=CARTESIAN_POINT('Ctrl Pts',(1.80948401499994,5.2,-4.28463148200001));
#358012=CARTESIAN_POINT('Ctrl Pts',(1.80948401499994,2.2,-4.28463148200001));
#358013=CARTESIAN_POINT('Ctrl Pts',(1.81150971699994,12.2,-4.28611632600001));
#358014=CARTESIAN_POINT('Ctrl Pts',(1.81150971699994,5.2,-4.28611632600001));
#358015=CARTESIAN_POINT('Ctrl Pts',(1.81150971699994,2.2,-4.28611632600001));
#358016=CARTESIAN_POINT('Ctrl Pts',(1.81353981999994,12.2,-4.28760111400001));
#358017=CARTESIAN_POINT('Ctrl Pts',(1.81353981999994,5.2,-4.28760111400001));
#358018=CARTESIAN_POINT('Ctrl Pts',(1.81353981999994,2.2,-4.28760111400001));
#358019=CARTESIAN_POINT('Ctrl Pts',(1.81557432299994,12.2,-4.28908583800002));
#358020=CARTESIAN_POINT('Ctrl Pts',(1.81557432299994,5.2,-4.28908583800002));
#358021=CARTESIAN_POINT('Ctrl Pts',(1.81557432299994,2.2,-4.28908583800002));
#358022=CARTESIAN_POINT('Ctrl Pts',(1.81761322799994,12.2,-4.29057048800002));
#358023=CARTESIAN_POINT('Ctrl Pts',(1.81761322799994,5.2,-4.29057048800002));
#358024=CARTESIAN_POINT('Ctrl Pts',(1.81761322799994,2.2,-4.29057048800002));
#358025=CARTESIAN_POINT('Ctrl Pts',(1.81965652899994,12.2,-4.29205505700001));
#358026=CARTESIAN_POINT('Ctrl Pts',(1.81965652899994,5.2,-4.29205505700001));
#358027=CARTESIAN_POINT('Ctrl Pts',(1.81965652899994,2.2,-4.29205505700001));
#358028=CARTESIAN_POINT('Ctrl Pts',(1.82170422599994,12.2,-4.29353953400001));
#358029=CARTESIAN_POINT('Ctrl Pts',(1.82170422599994,5.2,-4.29353953400001));
#358030=CARTESIAN_POINT('Ctrl Pts',(1.82170422599994,2.2,-4.29353953400001));
#358031=CARTESIAN_POINT('Ctrl Pts',(1.82375632099994,12.2,-4.29502391100002));
#358032=CARTESIAN_POINT('Ctrl Pts',(1.82375632099994,5.2,-4.29502391100002));
#358033=CARTESIAN_POINT('Ctrl Pts',(1.82375632099994,2.2,-4.29502391100002));
#358034=CARTESIAN_POINT('Ctrl Pts',(1.82581280899994,12.2,-4.29650817900002));
#358035=CARTESIAN_POINT('Ctrl Pts',(1.82581280899994,5.2,-4.29650817900002));
#358036=CARTESIAN_POINT('Ctrl Pts',(1.82581280899994,2.2,-4.29650817900002));
#358037=CARTESIAN_POINT('Ctrl Pts',(1.82787368999994,12.2,-4.29799233100002));
#358038=CARTESIAN_POINT('Ctrl Pts',(1.82787368999994,5.2,-4.29799233100002));
#358039=CARTESIAN_POINT('Ctrl Pts',(1.82787368999994,2.2,-4.29799233100002));
#358040=CARTESIAN_POINT('Ctrl Pts',(1.82993896199994,12.2,-4.29947635400001));
#358041=CARTESIAN_POINT('Ctrl Pts',(1.82993896199994,5.2,-4.29947635400001));
#358042=CARTESIAN_POINT('Ctrl Pts',(1.82993896199994,2.2,-4.29947635400001));
#358043=CARTESIAN_POINT('Ctrl Pts',(1.83200862499994,12.2,-4.30096024400001));
#358044=CARTESIAN_POINT('Ctrl Pts',(1.83200862499994,5.2,-4.30096024400001));
#358045=CARTESIAN_POINT('Ctrl Pts',(1.83200862499994,2.2,-4.30096024400001));
#358046=CARTESIAN_POINT('Ctrl Pts',(1.83408267599994,12.2,-4.30244399000001));
#358047=CARTESIAN_POINT('Ctrl Pts',(1.83408267599994,5.2,-4.30244399000001));
#358048=CARTESIAN_POINT('Ctrl Pts',(1.83408267599994,2.2,-4.30244399000001));
#358049=CARTESIAN_POINT('Ctrl Pts',(1.83616111599994,12.2,-4.30392758200002));
#358050=CARTESIAN_POINT('Ctrl Pts',(1.83616111599994,5.2,-4.30392758200002));
#358051=CARTESIAN_POINT('Ctrl Pts',(1.83616111599994,2.2,-4.30392758200002));
#358052=CARTESIAN_POINT('Ctrl Pts',(1.83824394199994,12.2,-4.30541101400001));
#358053=CARTESIAN_POINT('Ctrl Pts',(1.83824394199994,5.2,-4.30541101400001));
#358054=CARTESIAN_POINT('Ctrl Pts',(1.83824394199994,2.2,-4.30541101400001));
#358055=CARTESIAN_POINT('Ctrl Pts',(1.84033115299994,12.2,-4.30689427400001));
#358056=CARTESIAN_POINT('Ctrl Pts',(1.84033115299994,5.2,-4.30689427400001));
#358057=CARTESIAN_POINT('Ctrl Pts',(1.84033115299994,2.2,-4.30689427400001));
#358058=CARTESIAN_POINT('Ctrl Pts',(1.84242274599994,12.2,-4.30837735600001));
#358059=CARTESIAN_POINT('Ctrl Pts',(1.84242274599994,5.2,-4.30837735600001));
#358060=CARTESIAN_POINT('Ctrl Pts',(1.84242274599994,2.2,-4.30837735600001));
#358061=CARTESIAN_POINT('Ctrl Pts',(1.84451872199994,12.2,-4.30986025000001));
#358062=CARTESIAN_POINT('Ctrl Pts',(1.84451872199994,5.2,-4.30986025000001));
#358063=CARTESIAN_POINT('Ctrl Pts',(1.84451872199994,2.2,-4.30986025000001));
#358064=CARTESIAN_POINT('Ctrl Pts',(1.84661907999994,12.2,-4.31134294700001));
#358065=CARTESIAN_POINT('Ctrl Pts',(1.84661907999994,5.2,-4.31134294700001));
#358066=CARTESIAN_POINT('Ctrl Pts',(1.84661907999994,2.2,-4.31134294700001));
#358067=CARTESIAN_POINT('Ctrl Pts',(1.84872381499994,12.2,-4.31282544000001));
#358068=CARTESIAN_POINT('Ctrl Pts',(1.84872381499994,5.2,-4.31282544000001));
#358069=CARTESIAN_POINT('Ctrl Pts',(1.84872381499994,2.2,-4.31282544000001));
#358070=CARTESIAN_POINT('Ctrl Pts',(1.85083292899994,12.2,-4.31430771700001));
#358071=CARTESIAN_POINT('Ctrl Pts',(1.85083292899994,5.2,-4.31430771700001));
#358072=CARTESIAN_POINT('Ctrl Pts',(1.85083292899994,2.2,-4.31430771700001));
#358073=CARTESIAN_POINT('Ctrl Pts',(1.85294641899994,12.2,-4.31578977400001));
#358074=CARTESIAN_POINT('Ctrl Pts',(1.85294641899994,5.2,-4.31578977400001));
#358075=CARTESIAN_POINT('Ctrl Pts',(1.85294641899994,2.2,-4.31578977400001));
#358076=CARTESIAN_POINT('Ctrl Pts',(1.85506428499994,12.2,-4.31727159900001));
#358077=CARTESIAN_POINT('Ctrl Pts',(1.85506428499994,5.2,-4.31727159900001));
#358078=CARTESIAN_POINT('Ctrl Pts',(1.85506428499994,2.2,-4.31727159900001));
#358079=CARTESIAN_POINT('Ctrl Pts',(1.85718652399994,12.2,-4.31875318500001));
#358080=CARTESIAN_POINT('Ctrl Pts',(1.85718652399994,5.2,-4.31875318500001));
#358081=CARTESIAN_POINT('Ctrl Pts',(1.85718652399994,2.2,-4.31875318500001));
#358082=CARTESIAN_POINT('Ctrl Pts',(1.85931313599994,12.2,-4.32023452300001));
#358083=CARTESIAN_POINT('Ctrl Pts',(1.85931313599994,5.2,-4.32023452300001));
#358084=CARTESIAN_POINT('Ctrl Pts',(1.85931313599994,2.2,-4.32023452300001));
#358085=CARTESIAN_POINT('Ctrl Pts',(1.86144411799994,12.2,-4.32171560400001));
#358086=CARTESIAN_POINT('Ctrl Pts',(1.86144411799994,5.2,-4.32171560400001));
#358087=CARTESIAN_POINT('Ctrl Pts',(1.86144411799994,2.2,-4.32171560400001));
#358088=CARTESIAN_POINT('Ctrl Pts',(1.86357946799994,12.2,-4.32319641900001));
#358089=CARTESIAN_POINT('Ctrl Pts',(1.86357946799994,5.2,-4.32319641900001));
#358090=CARTESIAN_POINT('Ctrl Pts',(1.86357946799994,2.2,-4.32319641900001));
#358091=CARTESIAN_POINT('Ctrl Pts',(1.86571918699994,12.2,-4.32467695700002));
#358092=CARTESIAN_POINT('Ctrl Pts',(1.86571918699994,5.2,-4.32467695700002));
#358093=CARTESIAN_POINT('Ctrl Pts',(1.86571918699994,2.2,-4.32467695700002));
#358094=CARTESIAN_POINT('Ctrl Pts',(1.86786327099994,12.2,-4.32615721200001));
#358095=CARTESIAN_POINT('Ctrl Pts',(1.86786327099994,5.2,-4.32615721200001));
#358096=CARTESIAN_POINT('Ctrl Pts',(1.86786327099994,2.2,-4.32615721200001));
#358097=CARTESIAN_POINT('Ctrl Pts',(1.87001172099994,12.2,-4.32763717500002));
#358098=CARTESIAN_POINT('Ctrl Pts',(1.87001172099994,5.2,-4.32763717500002));
#358099=CARTESIAN_POINT('Ctrl Pts',(1.87001172099994,2.2,-4.32763717500002));
#358100=CARTESIAN_POINT('Ctrl Pts',(1.87216453299994,12.2,-4.32911683800001));
#358101=CARTESIAN_POINT('Ctrl Pts',(1.87216453299994,5.2,-4.32911683800001));
#358102=CARTESIAN_POINT('Ctrl Pts',(1.87216453299994,2.2,-4.32911683800001));
#358103=CARTESIAN_POINT('Ctrl Pts',(1.87432170699994,12.2,-4.33059619400002));
#358104=CARTESIAN_POINT('Ctrl Pts',(1.87432170699994,5.2,-4.33059619400002));
#358105=CARTESIAN_POINT('Ctrl Pts',(1.87432170699994,2.2,-4.33059619400002));
#358106=CARTESIAN_POINT('Ctrl Pts',(1.87648324099994,12.2,-4.33207523400001));
#358107=CARTESIAN_POINT('Ctrl Pts',(1.87648324099994,5.2,-4.33207523400001));
#358108=CARTESIAN_POINT('Ctrl Pts',(1.87648324099994,2.2,-4.33207523400001));
#358109=CARTESIAN_POINT('Ctrl Pts',(1.87864913399994,12.2,-4.33355395000001));
#358110=CARTESIAN_POINT('Ctrl Pts',(1.87864913399994,5.2,-4.33355395000001));
#358111=CARTESIAN_POINT('Ctrl Pts',(1.87864913399994,2.2,-4.33355395000001));
#358112=CARTESIAN_POINT('Ctrl Pts',(1.88081938399994,12.2,-4.33503233500002));
#358113=CARTESIAN_POINT('Ctrl Pts',(1.88081938399994,5.2,-4.33503233500002));
#358114=CARTESIAN_POINT('Ctrl Pts',(1.88081938399994,2.2,-4.33503233500002));
#358115=CARTESIAN_POINT('Ctrl Pts',(1.88299399099994,12.2,-4.33651037800002));
#358116=CARTESIAN_POINT('Ctrl Pts',(1.88299399099994,5.2,-4.33651037800002));
#358117=CARTESIAN_POINT('Ctrl Pts',(1.88299399099994,2.2,-4.33651037800002));
#358118=CARTESIAN_POINT('Ctrl Pts',(1.88517294999994,12.2,-4.33798806900001));
#358119=CARTESIAN_POINT('Ctrl Pts',(1.88517294999994,5.2,-4.33798806900001));
#358120=CARTESIAN_POINT('Ctrl Pts',(1.88517294999994,2.2,-4.33798806900001));
#358121=CARTESIAN_POINT('Ctrl Pts',(1.88735626099994,12.2,-4.33946539900001));
#358122=CARTESIAN_POINT('Ctrl Pts',(1.88735626099994,5.2,-4.33946539900001));
#358123=CARTESIAN_POINT('Ctrl Pts',(1.88735626099994,2.2,-4.33946539900001));
#358124=CARTESIAN_POINT('Ctrl Pts',(1.88954392399994,12.2,-4.34094235600002));
#358125=CARTESIAN_POINT('Ctrl Pts',(1.88954392399994,5.2,-4.34094235600002));
#358126=CARTESIAN_POINT('Ctrl Pts',(1.88954392399994,2.2,-4.34094235600002));
#358127=CARTESIAN_POINT('Ctrl Pts',(1.89173593299994,12.2,-4.34241893000001));
#358128=CARTESIAN_POINT('Ctrl Pts',(1.89173593299994,5.2,-4.34241893000001));
#358129=CARTESIAN_POINT('Ctrl Pts',(1.89173593299994,2.2,-4.34241893000001));
#358130=CARTESIAN_POINT('Ctrl Pts',(1.89393228799994,12.2,-4.34389511400001));
#358131=CARTESIAN_POINT('Ctrl Pts',(1.89393228799994,5.2,-4.34389511400001));
#358132=CARTESIAN_POINT('Ctrl Pts',(1.89393228799994,2.2,-4.34389511400001));
#358133=CARTESIAN_POINT('Ctrl Pts',(1.89613298899994,12.2,-4.34537090000001));
#358134=CARTESIAN_POINT('Ctrl Pts',(1.89613298899994,5.2,-4.34537090000001));
#358135=CARTESIAN_POINT('Ctrl Pts',(1.89613298899994,2.2,-4.34537090000001));
#358136=CARTESIAN_POINT('Ctrl Pts',(1.89833803499994,12.2,-4.34684628800001));
#358137=CARTESIAN_POINT('Ctrl Pts',(1.89833803499994,5.2,-4.34684628800001));
#358138=CARTESIAN_POINT('Ctrl Pts',(1.89833803499994,2.2,-4.34684628800001));
#358139=CARTESIAN_POINT('Ctrl Pts',(1.90054742399994,12.2,-4.34832127200002));
#358140=CARTESIAN_POINT('Ctrl Pts',(1.90054742399994,5.2,-4.34832127200002));
#358141=CARTESIAN_POINT('Ctrl Pts',(1.90054742399994,2.2,-4.34832127200002));
#358142=CARTESIAN_POINT('Ctrl Pts',(1.90231840999994,12.2,-4.34950093700001));
#358143=CARTESIAN_POINT('Ctrl Pts',(1.90231840999994,5.2,-4.34950093700001));
#358144=CARTESIAN_POINT('Ctrl Pts',(1.90231840999994,2.2,-4.34950093700001));
#358145=CARTESIAN_POINT('Ctrl Pts',(1.90364860499994,12.2,-4.35038550300002));
#358146=CARTESIAN_POINT('Ctrl Pts',(1.90364860499994,5.2,-4.35038550300002));
#358147=CARTESIAN_POINT('Ctrl Pts',(1.90364860499994,2.2,-4.35038550300002));
#358148=CARTESIAN_POINT('Ctrl Pts',(1.90453626899994,12.2,-4.35097513300001));
#358149=CARTESIAN_POINT('Ctrl Pts',(1.90453626899994,5.2,-4.35097513300001));
#358150=CARTESIAN_POINT('Ctrl Pts',(1.90453626899994,2.2,-4.35097513300001));
#358151=CARTESIAN_POINT('Ctrl Pts',(1.90498031899994,12.2,-4.35126992800001));
#358152=CARTESIAN_POINT('Ctrl Pts',(1.90498031899994,5.2,-4.35126992800001));
#358153=CARTESIAN_POINT('Ctrl Pts',(1.90498031899994,2.2,-4.35126992800001));
#358154=CARTESIAN_POINT('Origin',(-5.66300478732629E-14,15.2,-1.77635683940025E-14));
#358155=CARTESIAN_POINT('Origin',(-5.66300478732629E-14,15.4,-1.77635683940025E-14));
#358156=CARTESIAN_POINT('',(-3.28892417320473,15.4,-1.19707050039253));
#358157=CARTESIAN_POINT('',(-3.28892417320473,15.4,-1.19707050039253));
#358158=CARTESIAN_POINT('Origin',(-5.66300478732629E-14,15.4,-1.77635683940025E-14));
#358159=CARTESIAN_POINT('Origin',(-5.66300478732629E-14,15.4,-1.77635683940025E-14));
#459200=UNCERTAINTY_MEASURE_WITH_UNIT(LENGTH_MEASURE(0.01),#459243,
'DISTANCE_ACCURACY_VALUE',
'Maximum model space distance between geometric entities at asserted c
onnectivities');
#459216=UNCERTAINTY_MEASURE_WITH_UNIT(LENGTH_MEASURE(0.01),#459243,
'DISTANCE_ACCURACY_VALUE',
'Maximum model space distance between geometric entities at asserted c
onnectivities');
#459226=(
GEOMETRIC_REPRESENTATION_CONTEXT(3)
GLOBAL_UNCERTAINTY_ASSIGNED_CONTEXT((#459200))
GLOBAL_UNIT_ASSIGNED_CONTEXT((#459243,#459245,#459246))
REPRESENTATION_CONTEXT('','3D')
);
#459242=(
GEOMETRIC_REPRESENTATION_CONTEXT(3)
GLOBAL_UNCERTAINTY_ASSIGNED_CONTEXT((#459216))
GLOBAL_UNIT_ASSIGNED_CONTEXT((#459243,#459245,#459246))
REPRESENTATION_CONTEXT('','3D')
);
#459243=(
LENGTH_UNIT()
NAMED_UNIT(*)
SI_UNIT(.MILLI.,.METRE.)
);
#459245=(
NAMED_UNIT(*)
PLANE_ANGLE_UNIT()
SI_UNIT($,.RADIAN.)
);
#459246=(
NAMED_UNIT(*)
SI_UNIT($,.STERADIAN.)
SOLID_ANGLE_UNIT()
);
#459256=SHAPE_DEFINITION_REPRESENTATION(#459281,#459337);
#459281=PRODUCT_DEFINITION_SHAPE('',$,#459363);
#459337=SHAPE_REPRESENTATION('',(#98432),#459226);
#459353=PRODUCT_DEFINITION_CONTEXT('part definition',#459430,'design');
#459363=PRODUCT_DEFINITION('Main Reduction Gear','Main Reduction Gear',
#459388,#459353);
#459388=PRODUCT_DEFINITION_FORMATION('',$,#459441);
#459430=APPLICATION_CONTEXT(
'Core Data for Automotive Mechanical Design Process');
#459431=PRODUCT_CONTEXT('part definition',#459430,'mechanical');
#459441=PRODUCT('Main Reduction Gear','Main Reduction Gear',$,(#459431));
#459513=COLOUR_RGB('Sky Blue',0.24,0.69,0.87);
#459514=FILL_AREA_STYLE_COLOUR('',#459513);
#459515=FILL_AREA_STYLE('',(#459514));
#459516=SURFACE_STYLE_FILL_AREA(#459515);
#459517=SURFACE_SIDE_STYLE('',(#459516));
#459518=SURFACE_STYLE_USAGE(.BOTH.,#459517);
#459519=PRESENTATION_STYLE_ASSIGNMENT((#459518));
ENDSEC;
END-ISO-10303-21;
